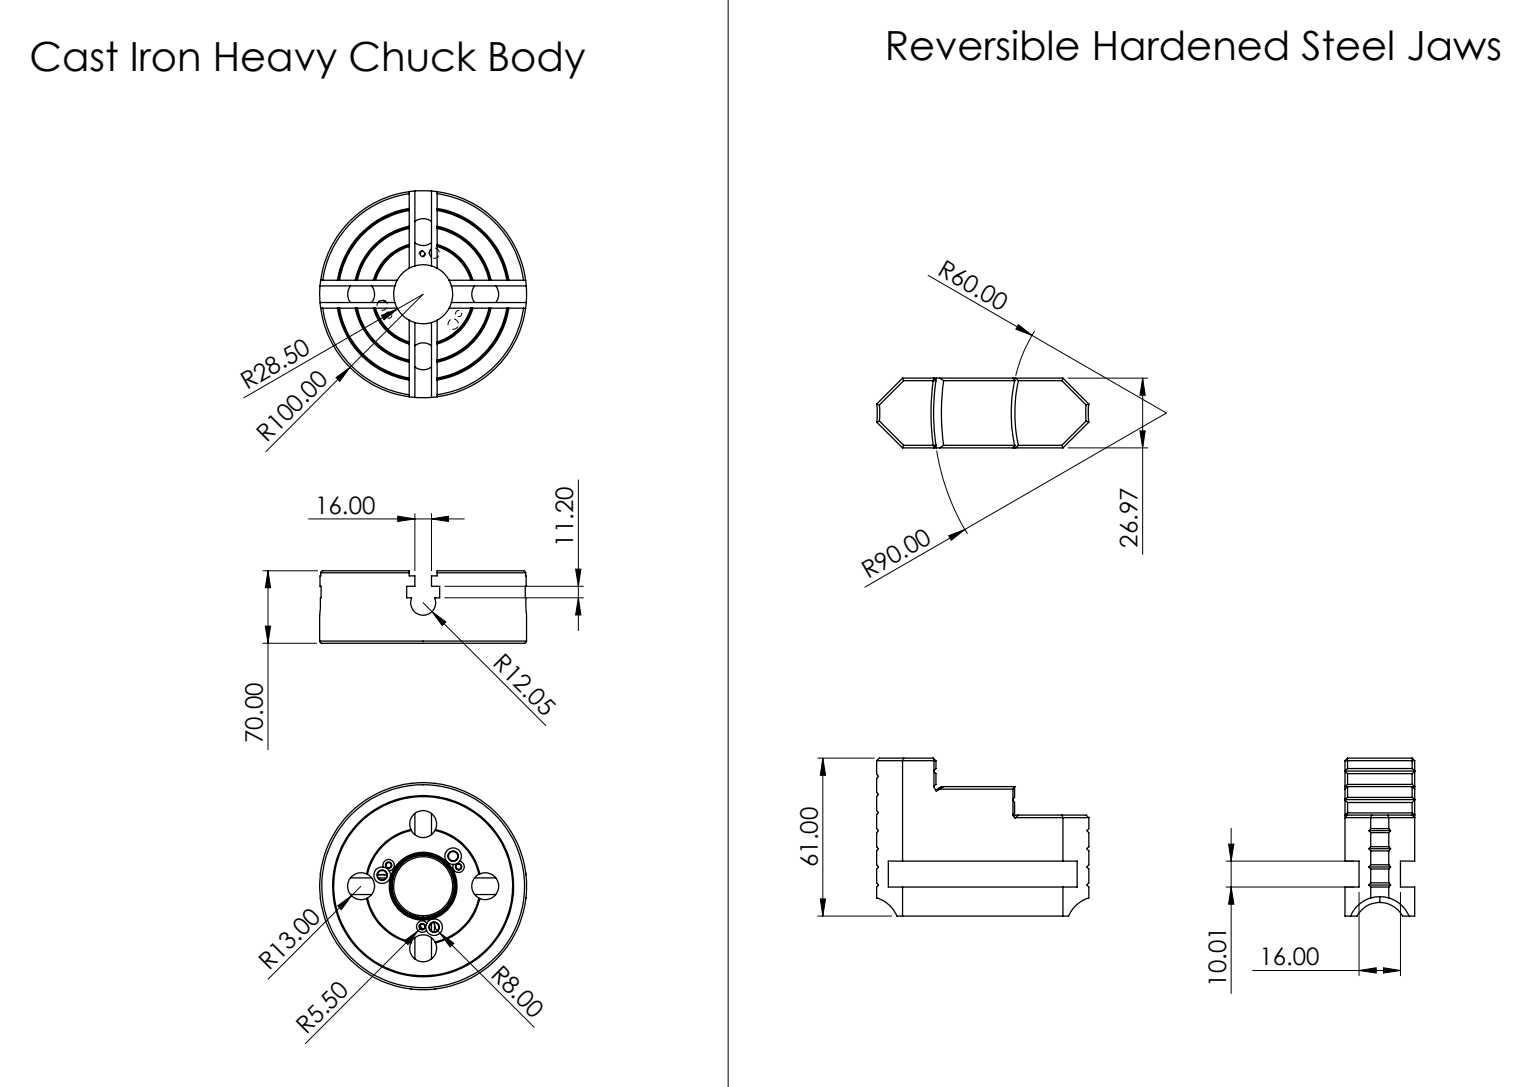
ISO-10303-21;
HEADER;
FILE_DESCRIPTION (('STEP AP214'),
    '1' );
FILE_NAME ('Reversible Hardened Steel Jaws.step',
    '2026-10-09T08:48:44',
    ( '' ),
    ( '' ),
    'SwSTEP 2.0',
    'SolidWorks 2026',
    '' );
FILE_SCHEMA (( 'AUTOMOTIVE_DESIGN' ));
ENDSEC;

DATA;
#3=CARTESIAN_POINT ( 'NONE',  ( -1.404199475065615932, -0.3690944881889765550, -0.3153832671262227771 ) ) ;
#4=CARTESIAN_POINT ( 'NONE',  ( 1.318897637795276356, 0.1660481256975883668, -0.3530559997133364547 ) ) ;
#5=CARTESIAN_POINT ( 'NONE',  ( 1.194225721784777594, 0.05413385826771666132, 0.4176697321401328100 ) ) ;
#6=CARTESIAN_POINT ( 'NONE',  ( 0.3018372703412079971, -0.004921259842519870586, -0.3153832671262229437 ) ) ;
#7=CARTESIAN_POINT ( 'NONE',  ( 1.003937007874016185, 0.1660481256975883668, -0.3530559997133364547 ) ) ;
#9=CARTESIAN_POINT ( 'NONE',  ( 0.1377952755905518800, 0.07958543189024071263, -0.2665933059059888421 ) ) ;
#10=CARTESIAN_POINT ( 'NONE',  ( 0.3149606299212603933, -0.1870078740157479769, 0.4822834645669291653 ) ) ;
#12=CARTESIAN_POINT ( 'NONE',  ( -1.043307086614172707, 0.1660481256975883668, -0.3530559997133364547 ) ) ;
#13=CARTESIAN_POINT ( 'NONE',  ( 0.4330708661417329575, -0.5511811023622047445, 6.969142054262312111E-17 ) ) ;
#14=PLANE ( 'NONE',  #11131 ) ;
#15=CARTESIAN_POINT ( 'NONE',  ( -0.1902887139107604098, -0.6692913385826771977, 0.1292274648535927661 ) ) ;
#16=CARTESIAN_POINT ( 'NONE',  ( -0.1574803149606292529, -0.1870078740157480601, -0.3641732283464567677 ) ) ;
#18=CARTESIAN_POINT ( 'NONE',  ( -0.2493438320209966919, 0.05413385826771626580, -0.4176697321401330321 ) ) ;
#19=CARTESIAN_POINT ( 'NONE',  ( 0.4002624671916016896, -0.2845877964562161244, -0.3641732283464567121 ) ) ;
#21=CARTESIAN_POINT ( 'NONE',  ( -0.03280839895013062252, 0.2952755905511810774, -0.1292274648535930714 ) ) ;
#24=CARTESIAN_POINT ( 'NONE',  ( 1.135170603674541256, -0.5511811023622048555, -0.09757992244046775898 ) ) ;
#26=CARTESIAN_POINT ( 'NONE',  ( -0.8530183727034112984, -0.3690944881889765550, -0.3153832671262227771 ) ) ;
#27=CARTESIAN_POINT ( 'NONE',  ( -0.8792650918635160906, -0.004921259842519870586, -0.3153832671262229437 ) ) ;
#28=CARTESIAN_POINT ( 'NONE',  ( -0.8530183727034112984, 0.05413385826771666132, 0.4176697321401328100 ) ) ;
#29=CARTESIAN_POINT ( 'NONE',  ( -0.3018372703412066094, 0.05413385826771666132, 0.4176697321401328100 ) ) ;
#30=CARTESIAN_POINT ( 'NONE',  ( 0.5905511811023629321, 0.1771653543307087630, 0.000000000000000000 ) ) ;
#32=CARTESIAN_POINT ( 'NONE',  ( 1.351706036745407458, -0.3690944881889765550, -0.3153832671262227771 ) ) ;
#33=CARTESIAN_POINT ( 'NONE',  ( 0.6758530183727039509, -0.6692913385826771977, 0.1292274648535927661 ) ) ;
#35=CARTESIAN_POINT ( 'NONE',  ( -0.09186351706036689768, 0.05413385826771626580, -0.4176697321401330321 ) ) ;
#37=CARTESIAN_POINT ( 'NONE',  ( 1.476377952755906220, 0.07958543189024071263, -0.2665933059059888421 ) ) ;
#38=CARTESIAN_POINT ( 'NONE',  ( 0.7874015748031503170, -0.1870078740157480879, -0.4822834645669291653 ) ) ;
#39=CARTESIAN_POINT ( 'NONE',  ( 8.195543980992789655E-16, -0.1870078740157480879, -0.4822834645669291653 ) ) ;
#41=CARTESIAN_POINT ( 'NONE',  ( 0.1706036745406830368, -0.3690944881889765550, -0.3153832671262227771 ) ) ;
#42=CARTESIAN_POINT ( 'NONE',  ( 1.141732283464567788, -0.6692913385826771977, 8.415575281601705876E-17 ) ) ;
#43=CARTESIAN_POINT ( 'NONE',  ( -0.2952755905511804668, 0.07958543189024085140, 0.2665933059059887866 ) ) ;
#44=CARTESIAN_POINT ( 'NONE',  ( -0.7152230971128602510, -0.3162353388693405765, 0.4822834645669290543 ) ) ;
#46=CARTESIAN_POINT ( 'NONE',  ( 0.3346456692913390985, 0.1660481256975885056, 0.3530559997133364547 ) ) ;
#47=CARTESIAN_POINT ( 'NONE',  ( -0.6758530183727028406, 0.2952755905511811885, 0.1292274648535926551 ) ) ;
#48=CARTESIAN_POINT ( 'NONE',  ( -0.7086614173228339419, -0.1870078740157480601, -0.3641732283464567677 ) ) ;
#49=CARTESIAN_POINT ( 'NONE',  ( 0.1837270341207354329, 0.2306618581243848609, 0.2411417322834645549 ) ) ;
#50=CARTESIAN_POINT ( 'NONE',  ( -1.135170603674539924, -0.6692913385826771977, 0.1292274648535927661 ) ) ;
#51=CARTESIAN_POINT ( 'NONE',  ( -0.3412073490813641308, 0.2306618581243847221, -0.2411417322834647770 ) ) ;
#53=CYLINDRICAL_SURFACE ( 'NONE', #64776, 0.3937007874015748254 ) ;
#54=CARTESIAN_POINT ( 'NONE',  ( 1.161417322834646271, 0.1660481256975883668, -0.3530559997133364547 ) ) ;
#55=CARTESIAN_POINT ( 'NONE',  ( 1.135170603674541256, -0.6692913385826773087, -0.1292274648535924053 ) ) ;
#57=CARTESIAN_POINT ( 'NONE',  ( -1.489501312335957062, -0.05778040916215522460, 0.4822834645669289988 ) ) ;
#58=CARTESIAN_POINT ( 'NONE',  ( -0.7217847769028863381, 0.05413385826771626580, -0.4176697321401330321 ) ) ;
#62=CARTESIAN_POINT ( 'NONE',  ( -0.08530183727034056085, -0.2845877964562159024, 0.3641732283464567677 ) ) ;
#65=CARTESIAN_POINT ( 'NONE',  ( 0.1837270341207354329, 0.2306618581243848609, 0.2411417322834645549 ) ) ;
#67=CYLINDRICAL_SURFACE ( 'NONE', #60105, 0.3937007874015748254 ) ;
#68=CARTESIAN_POINT ( 'NONE',  ( -0.4265091863517051496, -0.5511811023622046335, 0.09757992244046803654 ) ) ;
#69=CARTESIAN_POINT ( 'NONE',  ( 0.3346456692913390985, 0.1660481256975885056, 0.3530559997133364547 ) ) ;
#70=CARTESIAN_POINT ( 'NONE',  ( 1.220472440944882608, 0.2952755905511811885, 0.000000000000000000 ) ) ;
#71=CARTESIAN_POINT ( 'NONE',  ( 0.7283464566929140904, -0.4536011799217368745, -0.2665933059059886201 ) ) ;
#72=AXIS2_PLACEMENT_3D ( 'NONE', #38595, #24309, #82401 ) ;
#73=CARTESIAN_POINT ( 'NONE',  ( -0.04593175853018302557, 0.2952755905511811885, 0.1292274648535926551 ) ) ;
#75=CARTESIAN_POINT ( 'NONE',  ( -0.7414698162729651543, -0.6692913385826771977, 0.1292274648535927661 ) ) ;
#76=CARTESIAN_POINT ( 'NONE',  ( -1.351706036745406347, -0.004921259842519870586, -0.3153832671262229437 ) ) ;
#77=CARTESIAN_POINT ( 'NONE',  ( -0.5839895013123351797, 0.2952755905511810774, -0.1292274648535930714 ) ) ;
#79=CARTESIAN_POINT ( 'NONE',  ( 1.515748031496063408, 0.07958543189024085140, 0.2665933059059887866 ) ) ;
#82=CARTESIAN_POINT ( 'NONE',  ( 0.2362204724409456558, -0.1870078740157479769, 0.4822834645669291653 ) ) ;
#84=CARTESIAN_POINT ( 'NONE',  ( -0.6561679790026240244, -0.6046776061558807314, 0.2411417322834647770 ) ) ;
#85=CARTESIAN_POINT ( 'NONE',  ( 1.332020997375328974, -0.05778040916215560624, -0.4822834645669293319 ) ) ;
#86=CARTESIAN_POINT ( 'NONE',  ( 1.213910761154856299, -0.6692913385826773087, -0.1292274648535924053 ) ) ;
#87=CARTESIAN_POINT ( 'NONE',  ( 0.4724409448818904789, -0.1870078740157479769, 0.4822834645669291653 ) ) ;
#88=CARTESIAN_POINT ( 'NONE',  ( 0.1574803149606306130, -0.1870078740157480879, -0.4822834645669291653 ) ) ;
#90=CARTESIAN_POINT ( 'NONE',  ( -0.9120734908136475250, 0.2952755905511811885, 0.1292274648535926551 ) ) ;
#91=CARTESIAN_POINT ( 'NONE',  ( -0.1968503937007867743, 0.2952755905511811885, 0.000000000000000000 ) ) ;
#92=CARTESIAN_POINT ( 'NONE',  ( -0.006561679790025524116, -0.08942795157528024563, -0.3641732283464568787 ) ) ;
#94=CARTESIAN_POINT ( 'NONE',  ( 0.07217847769028949700, -0.05778040916215560624, -0.4822834645669293319 ) ) ;
#96=CARTESIAN_POINT ( 'NONE',  ( 1.253280839895013710, -0.3162353388693405765, 0.4822834645669290543 ) ) ;
#99=ORIENTED_EDGE ( 'NONE', *, *, #69485, .F. ) ;
#100=CARTESIAN_POINT ( 'NONE',  ( 0.3215223097112867578, -0.3162353388693409650, -0.4822834645669289433 ) ) ;
#101=CARTESIAN_POINT ( 'NONE',  ( -0.3543307086614165824, -0.5511811023622047445, 6.969142054262312111E-17 ) ) ;
#102=CARTESIAN_POINT ( 'NONE',  ( 1.377952755905512472, 0.1771653543307087630, 0.000000000000000000 ) ) ;
#103=CARTESIAN_POINT ( 'NONE',  ( -0.06764250034433647030, -3.915482057279200494E-15, 0.3954985857520088577 ) ) ;
#106=CARTESIAN_POINT ( 'NONE',  ( 1.410761154855643795, -0.08942795157528024563, -0.3641732283464568787 ) ) ;
#107=CARTESIAN_POINT ( 'NONE',  ( -1.423884514435694859, -0.05778040916215560624, -0.4822834645669293319 ) ) ;
#109=CARTESIAN_POINT ( 'NONE',  ( -0.1377952755905504645, 0.1660481256975885056, 0.3530559997133364547 ) ) ;
#110=CARTESIAN_POINT ( 'NONE',  ( -1.056430446194224881, -0.6692913385826771977, 0.1292274648535927661 ) ) ;
#111=CARTESIAN_POINT ( 'NONE',  ( -0.9645669291338575535, -0.5400638737290844871, 0.3530559997133364547 ) ) ;
#112=CARTESIAN_POINT ( 'NONE',  ( 0.1902887139107617975, 0.2952755905511811885, 0.1292274648535926551 ) ) ;
#114=CARTESIAN_POINT ( 'NONE',  ( -1.653543307086613234, -0.1870078740157479769, 0.3641732283464567677 ) ) ;
#115=CARTESIAN_POINT ( 'NONE',  ( 1.108923884514436242, -0.05778040916215522460, 0.4822834645669289988 ) ) ;
#116=CARTESIAN_POINT ( 'NONE',  ( 0.7545931758530189937, 0.1771653543307087075, -0.09757992244046823083 ) ) ;
#118=CARTESIAN_POINT ( 'NONE',  ( 0.9055118110236227702, 0.1771653543307087630, 0.000000000000000000 ) ) ;
#119=CARTESIAN_POINT ( 'NONE',  ( -1.200787401574802349, -0.5400638737290844871, 0.3530559997133364547 ) ) ;
#121=CARTESIAN_POINT ( 'NONE',  ( 1.358267716535433323, 0.1660481256975885056, 0.3530559997133364547 ) ) ;
#123=CARTESIAN_POINT ( 'NONE',  ( 0.6036745406824154392, 0.2306618581243847221, -0.2411417322834647770 ) ) ;
#125=CARTESIAN_POINT ( 'NONE',  ( -1.653543307086613234, -0.1870078740157480601, -0.3641732283464567677 ) ) ;
#126=CARTESIAN_POINT ( 'NONE',  ( 0.01968503937007957949, -0.5400638737290845981, -0.3530559997133363437 ) ) ;
#127=CARTESIAN_POINT ( 'NONE',  ( 0.6102362204724416372, -0.4536011799217367080, 0.2665933059059888421 ) ) ;
#128=CARTESIAN_POINT ( 'NONE',  ( 0.9776902887139113929, -0.6692913385826773087, -0.1292274648535924053 ) ) ;
#129=CARTESIAN_POINT ( 'NONE',  ( 1.640419947506562393, -0.3690944881889763329, 0.3153832671262228327 ) ) ;
#130=CARTESIAN_POINT ( 'NONE',  ( -0.6824146981627291497, -0.5023911411419708095, -0.1820866141732282451 ) ) ;
#131=CARTESIAN_POINT ( 'NONE',  ( -0.6430446194225716283, -0.4281496062992124485, 0.4176697321401328655 ) ) ;
#132=CARTESIAN_POINT ( 'NONE',  ( 1.574803149606299746, -0.1870078740157480879, -0.4822834645669291653 ) ) ;
#133=CARTESIAN_POINT ( 'NONE',  ( -1.246719160104986512, 0.05413385826771666132, 0.4176697321401328100 ) ) ;
#134=CONICAL_SURFACE ( 'NONE', #57903, 2.401574803149606918, 0.7125723459225955514 ) ;
#135=CARTESIAN_POINT ( 'NONE',  ( 0.8923884514435703741, 0.2306618581243848609, 0.2411417322834645549 ) ) ;
#136=CARTESIAN_POINT ( 'NONE',  ( -1.345144356955379816, -0.2845877964562159024, 0.3641732283464567677 ) ) ;
#138=CARTESIAN_POINT ( 'NONE',  ( 0.8070866141732288002, 0.1660481256975885056, 0.3530559997133364547 ) ) ;
#140=CARTESIAN_POINT ( 'NONE',  ( -1.561679790026246017, 0.05413385826771666132, 0.4176697321401328100 ) ) ;
#141=CARTESIAN_POINT ( 'NONE',  ( -1.555118110236219930, -0.4536011799217368745, -0.2665933059059886201 ) ) ;
#142=CARTESIAN_POINT ( 'NONE',  ( -0.8792650918635160906, -0.004921259842519870586, -0.3153832671262229437 ) ) ;
#143=B_SPLINE_CURVE_WITH_KNOTS ( 'NONE', 3,
 ( #64397, #13065, #45854, #433 ),
 .UNSPECIFIED., .F., .F.,
 ( 4, 4 ),
 ( 3.878959614448864246E-18, 0.001357026659661165861 ),
 .UNSPECIFIED. ) ;
#144=CARTESIAN_POINT ( 'NONE',  ( 1.496062992125985147, -0.1870078740157479769, 0.3641732283464567677 ) ) ;
#145=CARTESIAN_POINT ( 'NONE',  ( -0.3280839895013117347, 0.05413385826771626580, -0.4176697321401330321 ) ) ;
#146=CARTESIAN_POINT ( 'NONE',  ( -0.2230971128608915943, -0.004921259842519576551, 0.3153832671262227771 ) ) ;
#147=CARTESIAN_POINT ( 'NONE',  ( -1.660104986876639543, -0.08942795157528024563, -0.3641732283464568787 ) ) ;
#148=CARTESIAN_POINT ( 'NONE',  ( 0.9711286089238851948, 0.1283753931104748280, 0.1820866141732283561 ) ) ;
#149=CARTESIAN_POINT ( 'NONE',  ( 0.6299212598425204535, -0.1870078740157480879, -0.4822834645669291653 ) ) ;
#150=CARTESIAN_POINT ( 'NONE',  ( 1.489501312335958172, -0.05778040916215560624, -0.4822834645669293319 ) ) ;
#151=CARTESIAN_POINT ( 'NONE',  ( 0.4986876640419954376, -0.6046776061558809534, -0.2411417322834644161 ) ) ;
#154=CARTESIAN_POINT ( 'NONE',  ( 0.6889763779527563470, 0.07958543189024071263, -0.2665933059059888421 ) ) ;
#155=CARTESIAN_POINT ( 'NONE',  ( -1.443569553805773564, 0.2306618581243847221, -0.2411417322834647770 ) ) ;
#157=CARTESIAN_POINT ( 'NONE',  ( -1.351706036745406347, -0.4281496062992124485, 0.4176697321401328655 ) ) ;
#158=CARTESIAN_POINT ( 'NONE',  ( -0.4724409448818890911, -0.1870078740157479769, 0.4822834645669291653 ) ) ;
#161=CARTESIAN_POINT ( 'NONE',  ( -0.04593175853018302557, -0.6692913385826773087, -0.1292274648535924053 ) ) ;
#162=CARTESIAN_POINT ( 'NONE',  ( 1.187664041994751285, -0.2845877964562161244, -0.3641732283464567121 ) ) ;
#163=CARTESIAN_POINT ( 'NONE',  ( -0.3608923884514428360, 0.2952755905511811885, 0.1292274648535926551 ) ) ;
#164=CARTESIAN_POINT ( 'NONE',  ( 0.2952755905511816326, -0.5400638737290844871, 0.3530559997133364547 ) ) ;
#170=CARTESIAN_POINT ( 'NONE',  ( -0.8464566929133852113, -0.4536011799217368745, -0.2665933059059886201 ) ) ;
#171=CARTESIAN_POINT ( 'NONE',  ( -1.272965879265091305, -0.4281496062992124485, 0.4176697321401328655 ) ) ;
#173=CARTESIAN_POINT ( 'NONE',  ( 0.3280839895013130669, -0.4281496062992127816, -0.4176697321401328100 ) ) ;
#175=CARTESIAN_POINT ( 'NONE',  ( 1.233595800524935227, -0.6046776061558807314, 0.2411417322834647770 ) ) ;
#176=CARTESIAN_POINT ( 'NONE',  ( 0.8202099737532813073, 0.2952755905511811885, 0.1292274648535926551 ) ) ;
#180=CARTESIAN_POINT ( 'NONE',  ( 1.541994750656168645, 0.2952755905511810774, -0.1292274648535930714 ) ) ;
#181=CARTESIAN_POINT ( 'NONE',  ( 0.4330708661417329575, -0.6692913385826771977, 8.415575281601705876E-17 ) ) ;
#182=CARTESIAN_POINT ( 'NONE',  ( 0.07217847769028949700, -0.05778040916215560624, -0.4822834645669293319 ) ) ;
#183=CARTESIAN_POINT ( 'NONE',  ( 0.7480314960629927956, -0.5511811023622047445, 6.969142054262312111E-17 ) ) ;
#184=CARTESIAN_POINT ( 'NONE',  ( 1.371391076115485941, 0.2952755905511811885, 0.1292274648535926551 ) ) ;
#186=CARTESIAN_POINT ( 'NONE',  ( 0.5643044619422579178, -0.4281496062992127816, -0.4176697321401328100 ) ) ;
#187=CARTESIAN_POINT ( 'NONE',  ( 0.9514435695538062676, -0.3162353388693409650, -0.4822834645669289433 ) ) ;
#188=CARTESIAN_POINT ( 'NONE',  ( 0.2690288713910767848, 0.2952755905511811885, 0.1292274648535926551 ) ) ;
#189=CARTESIAN_POINT ( 'NONE',  ( 1.233595800524935227, 0.1283753931104746893, -0.1820866141732285504 ) ) ;
#190=CARTESIAN_POINT ( 'NONE',  ( -0.9448818897637790704, -0.1870078740157479769, 0.4822834645669291653 ) ) ;
#191=CARTESIAN_POINT ( 'NONE',  ( -1.102362204724408601, -0.1870078740157479769, 0.4822834645669291653 ) ) ;
#193=CARTESIAN_POINT ( 'NONE',  ( 1.089238845144357537, -0.4281496062992124485, 0.4176697321401328655 ) ) ;
#197=ORIENTED_EDGE ( 'NONE', *, *, #73267, .T. ) ;
#199=VERTEX_POINT ( 'NONE', #53305 ) ;
#200=CARTESIAN_POINT ( 'NONE',  ( 1.509186351706037543, 0.05413385826771666132, 0.4176697321401328100 ) ) ;
#201=CARTESIAN_POINT ( 'NONE',  ( 0.9317585301837276734, -0.3690944881889763329, 0.3153832671262228327 ) ) ;
#203=CARTESIAN_POINT ( 'NONE',  ( 1.213910761154856299, 0.1771653543307087630, 0.09757992244046791164 ) ) ;
#205=DIRECTION ( 'NONE',  ( 1.000000000000000000, 0.000000000000000000, -1.692413147294446216E-16 ) ) ;
#206=CARTESIAN_POINT ( 'NONE',  ( -0.6175017169405814244, 0.000000000000000000, 0.3464511005275205946 ) ) ;
#208=CARTESIAN_POINT ( 'NONE',  ( -0.9776902887139098386, 0.1771653543307087075, -0.09757992244046823083 ) ) ;
#209=CARTESIAN_POINT ( 'NONE',  ( -1.640419947506561060, -0.3690944881889765550, -0.3153832671262227771 ) ) ;
#210=CARTESIAN_POINT ( 'NONE',  ( -1.423884514435694859, -0.05778040916215560624, -0.4822834645669293319 ) ) ;
#211=CARTESIAN_POINT ( 'NONE',  ( 5.463695987328526437E-16, -0.1870078740157479769, 0.4822834645669291653 ) ) ;
#212=CARTESIAN_POINT ( 'NONE',  ( 1.312335958005249825, 0.2306618581243847221, -0.2411417322834647770 ) ) ;
#214=CARTESIAN_POINT ( 'NONE',  ( -1.122047244094487306, 0.1012011053420775880, -0.2882089793578256898 ) ) ;
#215=( CONVERSION_BASED_UNIT ( 'INCH', #44794 ) LENGTH_UNIT ( ) NAMED_UNIT ( #76065 ) );
#217=DIRECTION ( 'NONE',  ( 1.000000000000000000, -0.000000000000000000, -0.000000000000000000 ) ) ;
#218=LINE ( 'NONE', #70923, #26406 ) ;
#219=CARTESIAN_POINT ( 'NONE',  ( -0.8727034120734901146, -0.2845877964562159024, 0.3641732283464567677 ) ) ;
#220=CARTESIAN_POINT ( 'NONE',  ( -1.161417322834644716, 0.1660481256975885056, 0.3530559997133364547 ) ) ;
#221=CARTESIAN_POINT ( 'NONE',  ( 0.7283464566929143125, 0.1660481256975885056, 0.3530559997133364547 ) ) ;
#222=ORIENTED_EDGE ( 'NONE', *, *, #16494, .T. ) ;
#226=CARTESIAN_POINT ( 'NONE',  ( 1.161417322834646493, -0.5400638737290844871, 0.3530559997133364547 ) ) ;
#227=CARTESIAN_POINT ( 'NONE',  ( -1.240157480314959759, 0.1660481256975885056, 0.3530559997133364547 ) ) ;
#229=CARTESIAN_POINT ( 'NONE',  ( -0.5380577427821514602, -0.3690944881889765550, -0.3153832671262227771 ) ) ;
#230=CARTESIAN_POINT ( 'NONE',  ( -1.253280839895012377, -0.2845877964562161244, -0.3641732283464567121 ) ) ;
#232=CARTESIAN_POINT ( 'NONE',  ( -0.4855643044619415427, -0.004921259842519870586, -0.3153832671262229437 ) ) ;
#233=CARTESIAN_POINT ( 'NONE',  ( -0.07217847769028813698, -0.2845877964562161244, -0.3641732283464567121 ) ) ;
#234=CARTESIAN_POINT ( 'NONE',  ( 0.3215223097112867578, -0.05778040916215522460, 0.4822834645669289988 ) ) ;
#235=CARTESIAN_POINT ( 'NONE',  ( -1.076115485564303809, -0.5023911411419708095, -0.1820866141732282451 ) ) ;
#237=CARTESIAN_POINT ( 'NONE',  ( 1.167979002624672580, 0.05413385826771626580, -0.4176697321401330321 ) ) ;
#239=CARTESIAN_POINT ( 'NONE',  ( -1.345144356955379816, -0.3162353388693405765, 0.4822834645669290543 ) ) ;
#241=CARTESIAN_POINT ( 'NONE',  ( -0.2952755905511804668, 0.1660481256975885056, 0.3530559997133364547 ) ) ;
#242=CARTESIAN_POINT ( 'NONE',  ( -0.8923884514435688198, -0.6046776061558807314, 0.2411417322834647770 ) ) ;
#243=CARTESIAN_POINT ( 'NONE',  ( 0.9251968503937015864, 0.07958543189024071263, -0.2665933059059888421 ) ) ;
#244=CARTESIAN_POINT ( 'NONE',  ( -0.4986876640419942164, -0.5023911411419708095, 0.1820866141732285504 ) ) ;
#245=CARTESIAN_POINT ( 'NONE',  ( -0.5052493438320203589, -0.6692913385826771977, 0.1292274648535927661 ) ) ;
#246=CARTESIAN_POINT ( 'NONE',  ( -1.364829396325458521, -0.6046776061558807314, 0.2411417322834647770 ) ) ;
#248=CARTESIAN_POINT ( 'NONE',  ( 1.089238845144357759, -0.004921259842519870586, -0.3153832671262229437 ) ) ;
#249=CARTESIAN_POINT ( 'NONE',  ( -0.4330708661417315697, -0.6692913385826771977, 8.415575281601705876E-17 ) ) ;
#250=CARTESIAN_POINT ( 'NONE',  ( -1.561679790026246017, 0.05413385826771666132, 0.4176697321401328100 ) ) ;
#252=ORIENTED_EDGE ( 'NONE', *, *, #19019, .F. ) ;
#254=CARTESIAN_POINT ( 'NONE',  ( -0.9776902887139098386, 0.1771653543307087075, -0.09757992244046823083 ) ) ;
#255=CARTESIAN_POINT ( 'NONE',  ( 0.7349081364829402885, -0.6046776061558809534, -0.2411417322834644161 ) ) ;
#256=CARTESIAN_POINT ( 'NONE',  ( -1.135170603674539924, -0.5511811023622046335, 0.09757992244046803654 ) ) ;
#258=CARTESIAN_POINT ( 'NONE',  ( -1.017060367454067249, -0.3162353388693409650, -0.4822834645669289433 ) ) ;
#259=CARTESIAN_POINT ( 'NONE',  ( 0.7020997375328090762, -0.3162353388693405765, 0.4822834645669290543 ) ) ;
#260=CARTESIAN_POINT ( 'NONE',  ( 0.6955380577427828781, -0.4281496062992124485, 0.4176697321401328655 ) ) ;
#261=CARTESIAN_POINT ( 'NONE',  ( 1.463254593175853824, 0.2952755905511810774, -0.1292274648535930714 ) ) ;
#262=CARTESIAN_POINT ( 'NONE',  ( -1.377952755905511140, 0.1771653543307087630, 0.000000000000000000 ) ) ;
#266=LINE ( 'NONE', #58323, #72192 ) ;
#267=CARTESIAN_POINT ( 'NONE',  ( 1.043307086614173818, 0.07958543189024085140, 0.2665933059059887866 ) ) ;
#268=CARTESIAN_POINT ( 'NONE',  ( 0.3871391076115492380, -0.08942795157528024563, -0.3641732283464568787 ) ) ;
#269=CARTESIAN_POINT ( 'NONE',  ( 0.1377952755905518800, -0.5400638737290844871, 0.3530559997133364547 ) ) ;
#270=CARTESIAN_POINT ( 'NONE',  ( 1.161417322834646271, 0.1660481256975883668, -0.3530559997133364547 ) ) ;
#272=CARTESIAN_POINT ( 'NONE',  ( 0.2887139107611556010, 0.1283753931104746893, -0.1820866141732285504 ) ) ;
#273=CARTESIAN_POINT ( 'NONE',  ( -0.6036745406824141069, -0.6046776061558809534, -0.2411417322834644161 ) ) ;
#274=CARTESIAN_POINT ( 'NONE',  ( -1.246719160104985846, -0.4281496062992127816, -0.4176697321401328100 ) ) ;
#275=CARTESIAN_POINT ( 'NONE',  ( 0.6627296587926517768, -0.6692913385826773087, -0.1292274648535924053 ) ) ;
#279=ORIENTED_EDGE ( 'NONE', *, *, #37675, .F. ) ;
#280=CARTESIAN_POINT ( 'NONE',  ( -1.391076115485563758, 0.2306618581243848609, 0.2411417322834645549 ) ) ;
#281=CARTESIAN_POINT ( 'NONE',  ( -0.7742782152230962556, -0.4281496062992127816, -0.4176697321401328100 ) ) ;
#282=CARTESIAN_POINT ( 'NONE',  ( -0.7020997375328074108, -0.08942795157527998196, 0.3641732283464567121 ) ) ;
#283=CARTESIAN_POINT ( 'NONE',  ( -0.5971128608923877978, -0.6692913385826773087, -0.1292274648535924053 ) ) ;
#286=CARTESIAN_POINT ( 'NONE',  ( -1.607611548556429737, 0.1771653543307087075, -0.09757992244046823083 ) ) ;
#287=CARTESIAN_POINT ( 'NONE',  ( -1.069553805774277722, 0.2952755905511811885, 0.1292274648535926551 ) ) ;
#288=CARTESIAN_POINT ( 'NONE',  ( 0.2952755905511816326, -0.5400638737290844871, 0.3530559997133364547 ) ) ;
#289=CARTESIAN_POINT ( 'NONE',  ( -0.7349081364829387342, -0.6046776061558807314, 0.2411417322834647770 ) ) ;
#291=CARTESIAN_POINT ( 'NONE',  ( -0.8595800524934373854, -0.08942795157527998196, 0.3641732283464567121 ) ) ;
#295=CARTESIAN_POINT ( 'NONE',  ( -1.535433070866141225, 0.1771653543307087630, 0.000000000000000000 ) ) ;
#296=CARTESIAN_POINT ( 'NONE',  ( -1.240157480314959759, 0.1660481256975885056, 0.3530559997133364547 ) ) ;
#297=CARTESIAN_POINT ( 'NONE',  ( -0.7414698162729651543, -0.6692913385826771977, 0.1292274648535927661 ) ) ;
#299=CARTESIAN_POINT ( 'NONE',  ( -0.9645669291338575535, -0.5400638737290844871, 0.3530559997133364547 ) ) ;
#300=CARTESIAN_POINT ( 'NONE',  ( -1.410761154855642463, -0.05778040916215522460, 0.4822834645669289988 ) ) ;
#304=CARTESIAN_POINT ( 'NONE',  ( 0.5971128608923891301, 0.1771653543307087075, -0.09757992244046823083 ) ) ;
#305=DIRECTION ( 'NONE',  ( -3.096699300667737957E-16, 1.000000000000000000, -0.000000000000000000 ) ) ;
#307=CARTESIAN_POINT ( 'NONE',  ( -0.2034120734908131112, -0.5511811023622048555, -0.09757992244046775898 ) ) ;
#308=CARTESIAN_POINT ( 'NONE',  ( -0.6036745406824141069, -0.6046776061558809534, -0.2411417322834644161 ) ) ;
#309=ADVANCED_FACE ( 'NONE', ( #49336 ), #12419, .F. ) ;
#310=CARTESIAN_POINT ( 'NONE',  ( 1.555118110236221041, -0.5400638737290844871, 0.3530559997133364547 ) ) ;
#311=CARTESIAN_POINT ( 'NONE',  ( -0.6233595800524928121, -0.3162353388693409650, -0.4822834645669289433 ) ) ;
#315=CARTESIAN_POINT ( 'NONE',  ( -1.095800524934382292, -0.3162353388693409650, -0.4822834645669289433 ) ) ;
#317=CARTESIAN_POINT ( 'NONE',  ( 1.404199475065617264, -0.4281496062992124485, 0.4176697321401328655 ) ) ;
#318=CARTESIAN_POINT ( 'NONE',  ( -1.043307086614172707, 0.07958543189024071263, -0.2665933059059888421 ) ) ;
#319=CARTESIAN_POINT ( 'NONE',  ( -1.443569553805773564, -0.6046776061558807314, 0.2411417322834647770 ) ) ;
#324=CARTESIAN_POINT ( 'NONE',  ( 0.01312335958005323398, -0.4281496062992127816, -0.4176697321401328100 ) ) ;
#325=CARTESIAN_POINT ( 'NONE',  ( -1.135170603674539924, 0.1771653543307087075, -0.09757992244046823083 ) ) ;
#326=CARTESIAN_POINT ( 'NONE',  ( -0.6299212598425188991, -0.1870078740157479769, 0.4822834645669291653 ) ) ;
#328=CARTESIAN_POINT ( 'NONE',  ( -1.384514435695537005, 0.2952755905511811885, 0.1292274648535926551 ) ) ;
#329=CARTESIAN_POINT ( 'NONE',  ( -1.095800524934382292, -0.05778040916215522460, 0.4822834645669289988 ) ) ;
#330=CARTESIAN_POINT ( 'NONE',  ( 0.2362204724409456558, -0.1870078740157480879, -0.4822834645669291653 ) ) ;
#332=CARTESIAN_POINT ( 'NONE',  ( 0.7349081364829402885, -0.5023911411419708095, -0.1820866141732282451 ) ) ;
#333=CARTESIAN_POINT ( 'NONE',  ( -0.7742782152230965886, -0.004921259842519576551, 0.3153832671262227771 ) ) ;
#335=CARTESIAN_POINT ( 'NONE',  ( 0.8267716535433078384, -0.5511811023622047445, 6.969142054262312111E-17 ) ) ;
#336=CARTESIAN_POINT ( 'NONE',  ( 1.496062992125984703, -0.1870078740157480601, -0.3641732283464567677 ) ) ;
#337=CARTESIAN_POINT ( 'NONE',  ( 1.299212598425197429, 0.2952755905511811885, 0.000000000000000000 ) ) ;
#338=CARTESIAN_POINT ( 'NONE',  ( -0.05905511811023545637, 0.07958543189024085140, 0.2665933059059887866 ) ) ;
#340=CARTESIAN_POINT ( 'NONE',  ( -1.023622047244093558, -0.1870078740157479769, 0.4822834645669291653 ) ) ;
#341=CARTESIAN_POINT ( 'NONE',  ( 1.049868766404200127, -0.6046776061558809534, -0.2411417322834644161 ) ) ;
#343=CARTESIAN_POINT ( 'NONE',  ( -0.3215223097112853146, -0.08942795157528024563, -0.3641732283464568787 ) ) ;
#345=CARTESIAN_POINT ( 'NONE',  ( 0.3937007874015754361, -0.1870078740157479769, 0.4822834645669291653 ) ) ;
#347=CARTESIAN_POINT ( 'NONE',  ( 0.8398950131233602345, 0.1283753931104746893, -0.1820866141732285504 ) ) ;
#348=CARTESIAN_POINT ( 'NONE',  ( 0.02624671916010564918, 0.1283753931104748280, 0.1820866141732283561 ) ) ;
#349=CARTESIAN_POINT ( 'NONE',  ( 0.1181102362204730916, 0.2952755905511811885, 0.000000000000000000 ) ) ;
#350=CARTESIAN_POINT ( 'NONE',  ( -1.207349081364828880, 0.2306618581243847221, -0.2411417322834647770 ) ) ;
#351=CARTESIAN_POINT ( 'NONE',  ( -0.4986876640419939388, 0.1283753931104746893, -0.1820866141732285504 ) ) ;
#352=DIRECTION ( 'NONE',  ( 0.000000000000000000, 1.000000000000000000, 0.000000000000000000 ) ) ;
#353=CARTESIAN_POINT ( 'NONE',  ( -0.9580052493438311334, 0.05413385826771626580, -0.4176697321401330321 ) ) ;
#356=CARTESIAN_POINT ( 'NONE',  ( 0.3608923884514443348, 0.1771653543307087075, -0.09757992244046823083 ) ) ;
#357=CARTESIAN_POINT ( 'NONE',  ( -0.6692913385826764205, 0.2952755905511811885, 0.000000000000000000 ) ) ;
#358=CARTESIAN_POINT ( 'NONE',  ( -1.227034120734907141, -0.6692913385826773087, -0.1292274648535924053 ) ) ;
#359=CARTESIAN_POINT ( 'NONE',  ( -1.023622047244093558, -0.1870078740157479769, 0.3641732283464567677 ) ) ;
#360=CARTESIAN_POINT ( 'NONE',  ( 1.548556430446194954, 0.2306618581243847221, -0.2411417322834647770 ) ) ;
#361=( BOUNDED_SURFACE ( )  B_SPLINE_SURFACE ( 1, 2, ( 
 ( #63527, #18507, #32782, #810, #5858, #57610, #388, #44971, #24798, #82892, #31534, #44150, #60014, #57190, #26473, #37849, #12602, #7111, #44556, #25212, #19741, #21303, #64772, #58024, #6692, #14998, #13435, #70667, #78982, #53273, #58450, #50878, #46956, #26045, #64355, #32362, #76578, #6273, #18906, #63937, #31949, #50466, #72648, #38677, #83301, #25623, #40655, #51704, #51286, #76989, #77406, #19319, #66339, #69842, #8678, #34348, #76170, #12192, #71092, #13023, #39091, #16663, #53684, #36007, #28856, #73906, #54518, #67177, #42303, #79392, #49035, #68001, #22549, #15842, #17080, #21711, #47375, #73065, #16247, #54100, #10346, #68413, #9098, #9506, #10753, #22132, #35179, #29273, #60840, #74732, #22955, #34771, #41076, #47790, #15415, #3607, #66765, #41490, #60430, #2781, #28441, #61677, #4018, #29682, #42717, #73494, #54937, #55344, #79815, #3192, #81051, #23365, #80643, #48211, #2369, #48622, #41894, #80233, #67588, #9918, #36413, #61253, #28025, #35590, #74317, #24189, #49858, #11989, #70043, #37643, #82687, #38054, #12397, #63730, #6070, #51083, #75558, #5658, #31744, #4837, #62918, #57406, #83097, #63320, #82283, #62086, #31325, #18307, #55757, #30093, #68820, #76780, #56989, #44761, #81463, #75146, #17898, #43534, #25006, #25418, #50678, #76377, #19112, #43122, #11582, #18711, #24601, #4427, #36824, #17491, #23781, #12815, #11165, #70457, #62499, #69233, #44352, #81877, #30512, #49452, #56174, #37241, #5251, #43949, #30915, #56582, #50270, #75967, #69645, #65422, #70888, #7756, #1029, #7325, #32994, #45185, #603, #51494, #13238, #38887, #40148, #33422, #64990, #26259, #64566, #27095, #26682, #51920, #45609, #52337, #71302, #20790, #32159, #78465, #72139, #52757, #46446, #46025, #6903, #77625, #14074, #6489, #59083, #19958, #39303, #13650, #58664, #39727, #64156, #14495, #1438, #78044, #32574, #38472, #25835, #182, #77197, #20373, #58236, #57815, #19528, #71719, #55293, #42669, #10291, #35538, #10706, #61200, #28804, #11113, #54047, #81002, #16610, #15785, #47737, #48159, #3141, #23316, #54468, #48985, #55704, #73435, #3557, #29222, #81412, #75094, #80181, #22496, #62037, #54889, #35958, #74684, #23729, #17442, #35122, #17030, #49400, #68368, #68769, #36362, #36770, #62446, #43072, #4782, #60788, #48569, #61627, #41437, #67120, #9451, #4374, #73854, #30042, #79761, #80594, #74267, #16195, #3969, #22078, #41841, #67531, #9869, #22902, #42253, #67948, #29632, #69994, #11939, #70409, #37594, #5202, #70840, #30458, #57351, #76329, #75509, #24138, #24553, #62865, #31692, #30866, #12765, #56531, #82234, #83047, #64517, #37186, #38422, #49808, #12349, #19483, #25370, #63683, #77151, #6021, #13189, #38838, #63267, #5608, #24951, #44303, #51033, #56122, #64104, #131, #38005, #76732, #81828, #17848, #43482, #50219, #31276, #45136, #11529, #75915, #18254, #43896, #69593, #56941, #82638, #44712, #19064, #6439, #32111, #50624, #18659, #57769, #25786, #51447, #69178, #13601, #32948, #52291, #53123, #46397, #52707, #58614, #66197, #71672, #59039, #7708, #33786, #14024, #1802, #45559, #981, #59865, #8534, #27884, #39255, #7277, #14856, #33375, #72090, #27465, #34202, #53544, #71255, #78834, #2218, #21160, #21567, #46816, #47229, #15270, #79252, #72919, #64937, #1393, #14449, #26209, #51871, #77577, #40517, #26637, #59450, #72507, #65373, #27047, #77996, #40100, #40931, #6854, #19909, #20324, #556, #45977, #8121, #32524, #65788, #39681, #58186, #78418, #20747, #23629, #66611, #10195, #29126, #28294, #60287, #60696, #15690, #67857, #67029, #23218, #9361, #41348, #35864, #17347, #73342, #74589, #2637, #22813, #55604, #61529, #16518, #29940, #42162, #49300, #75001, #73764, #41744, #61109, #80497, #3875, #8947, #48888, #36267, #48470, #29534, #34623, #53955, #79668, #35032, #67438, #81316, #47647, #3046, #28711, #54375, #80085, #22405, #48062, #80904, #74171, #55197, #16933, #16099, #9772, #42573, #54794, #68275, #10610, #35443, #3461, #61936, #4279, #21985, #5511, #69080, #18964, #24450, #11845, #43790, #69897, #50118, #37907, #81731, #11431, #12661, #44207 ),
 ( #17751, #37086, #62772, #75405, #49710, #43380, #57247, #24856, #12251, #31592, #5106, #30773, #25269, #31174, #5918, #63584, #56434, #82136, #75815, #82951, #82538, #56840, #18158, #44612, #69496, #37498, #63173, #50935, #50524, #76633, #24040, #76230, #38322, #70308, #63996, #36669, #18564, #6337, #32010, #57670, #32, #25685, #51345, #77049, #42975, #68671, #11010, #62344, #4683, #30354, #56023, #8022, #34099, #65693, #59762, #27783, #21058, #72410, #451, #13922, #58938, #38739, #64416, #6751, #53020, #45456, #71993, #46298, #77893, #39578, #26106, #1296, #78735, #53446, #32423, #58085, #13086, #51768, #20645, #33685, #26946, #877, #59347, #26536, #77470, #2117, #19381, #14346, #65268, #19807, #71154, #13495, #39151, #40006, #64836, #1704, #7174, #32845, #27361, #45033, #58514, #46718, #52189, #52607, #8431, #14759, #78314, #66095, #40414, #70732, #20224, #45873, #71571, #7604, #33278, #16416, #4180, #35757, #34937, #15169, #34520, #72819, #3773, #55096, #29437, #68169, #41246, #22713, #80804, #21882, #79986, #48789, #23121, #80400, #16005, #79154, #48371, #35347, #40825, #47129, #2538, #10512, #54689, #61839, #66510, #8844, #66933, #9266, #29023, #74486, #74070, #42063, #16833, #60186, #28614, #67758, #41652, #21471, #53854, #28196, #79567, #29843, #47546, #42469, #73236, #60599, #61423, #15587, #2949, #10092, #36165, #54271, #22299, #61009, #47960, #73664, #67343, #9676, #3358, #64624, #55921, #37810, #31078, #11751, #37407, #30257, #36990, #36571, #81634, #23945, #7383, #6961, #69399, #62669, #75307, #51977, #56746, #5009, #24353, #5417, #50022, #45663, #74901, #20012, #13706, #77682, #71359, #18471, #49612, #30679, #69806, #23530, #32632, #82039, #43694, #75721, #56340, #12154, #49200, #39361, #58295, #18061, #68982, #65046, #17249, #42878, #68571, #63079, #17651, #660, #10913, #62249, #26316, #55507, #43283, #82444, #24761, #50429, #81215, #76129, #4586, #11330, #44114, #1085, #34308, #26737, #7811, #14553, #14131, #59139, #33477, #67132, #66720, #46917, #40205, #52813, #28399, #8637, #65888, #1908, #66298, #27569, #22088, #52391, #79772, #73447, #54057, #47748, #79353, #1497, #8223, #47333, #78100, #9056, #59553, #21262, #53228, #33887, #73023, #20431, #15797, #15373, #78944, #46500, #41447, #46084, #71777, #39784, #72610, #27149, #41034, #65479, #78523, #34729, #33051, #20847, #14958, #59969, #40615, #58722, #53645, #72200, #2329, #27985, #21672, #60389, #2739, #48580, #28815, #48169, #3151, #17453, #68780, #43083, #81839, #16621, #61211, #75520, #43494, #24150, #4385, #42680, #56134, #68378, #49820, #17859, #42263, #67960, #3979, #23326, #30054, #9461, #49413, #62458, #48996, #10717, #35135, #60797, #54479, #67544, #10302, #80191, #73864, #9879, #35548, #3566, #41852, #16205, #29233, #23740, #74695, #36374, #81425, #54897, #80603, #75106, #55304, #55715, #62048, #22912, #74277, #35968, #11124, #17040, #81013, #61638, #36781, #29643, #4793, #30470, #22508, #50635, #64116, #12360, #57363, #38018, #76340, #25798, #37197, #32534, #142, #6033, #82649, #566, #62878, #5213, #30877, #83059, #37606, #77161, #56544, #75926, #19493, #51882, #5621, #18670, #12776, #44315, #58198, #6451, #18266, #24564, #31287, #82245, #70421, #50230, #24964, #43907, #69605, #11951, #45147, #70850, #13201, #26219, #77587, #38848, #64528, #31705, #70005, #6865, #19921, #38433, #25381, #69190, #32121, #51044, #63280, #56952, #63694, #11541, #44723, #76745, #19075, #57779, #51458, #7717, #78843, #53553, #21169, #66206, #21576, #26646, #78428, #46825, #65797, #45570, #20334, #991, #64947, #79676, #78006, #47238, #58624, #33385, #27893, #65382, #52300, #40527, #40940, #2228, #72517, #27474, #34631, #34211, #8131, #15279, #72928, #79261, #45986, #66619, #14865, #1812, #53132, #71682, #27058, #14034, #39690, #59048, #71264, #8957, #59461, #52717, #1402, #60295, #8545, #20756, #14458, #59874, #40110, #2645, #7287, #28302, #53964, #13611, #39265, #32957, #46406, #72100, #33796, #73350, #55612, #23225, #15698, #61116, #41355, #60704, #67036, #29948, #81323, #23637, #11020 ) ),
 .UNSPECIFIED., .F., .F., .F. ) 
 B_SPLINE_SURFACE_WITH_KNOTS ( ( 2, 2 ),
 ( 3, 2, 2, 2, 2, 2, 2, 2, 2, 2, 2, 2, 2, 2, 2, 2, 2, 2, 2, 2, 2, 2, 2, 2, 2, 2, 2, 2, 2, 2, 2, 2, 2, 2, 2, 2, 2, 2, 2, 2, 2, 2, 2, 2, 2, 2, 2, 2, 2, 2, 2, 2, 2, 2, 2, 2, 2, 2, 2, 2, 2, 2, 2, 2, 2, 2, 2, 2, 2, 2, 2, 2, 2, 2, 2, 2, 2, 2, 2, 2, 2, 2, 2, 2, 2, 2, 2, 2, 2, 2, 2, 2, 2, 2, 2, 2, 2, 2, 2, 2, 2, 2, 2, 2, 2, 2, 2, 2, 2, 2, 2, 2, 2, 2, 2, 2, 2, 2, 2, 2, 2, 2, 2, 2, 2, 2, 2, 2, 2, 2, 2, 2, 2, 2, 2, 2, 2, 2, 2, 2, 2, 2, 2, 2, 2, 2, 2, 2, 2, 2, 2, 2, 2, 2, 2, 2, 2, 2, 2, 2, 2, 2, 2, 2, 2, 2, 2, 2, 2, 2, 2, 2, 2, 2, 2, 2, 2, 2, 2, 2, 2, 2, 2, 2, 2, 2, 2, 2, 2, 2, 2, 2, 2, 2, 2, 2, 2, 2, 2, 2, 2, 2, 2, 2, 2, 2, 2, 2, 2, 2, 2, 2, 2, 2, 2, 2, 2, 2, 2, 2, 2, 2, 2, 2, 2, 2, 2, 2, 2, 2, 2, 2, 2, 2, 2, 2, 2, 2, 2, 2, 2, 2, 2, 2, 2, 2, 2, 2, 2, 2, 2, 2, 2, 2, 2, 3 ),
 ( 0.000000000000000000, 1.000000000000000000 ),
 ( 0.000000000000000000, 0.003787878787878787984, 0.007575757575757575968, 0.01136363636363636395, 0.01515151515151515194, 0.01893939393939393992, 0.02272727272727272790, 0.02651515151515151589, 0.03030303030303030387, 0.03409090909090908839, 0.03787878787878787984, 0.04166666666666666435, 0.04545454545454545581, 0.04924242424242424032, 0.05303030303030303177, 0.05681818181818181629, 0.06060606060606060774, 0.06439393939393939226, 0.06818181818181817677, 0.07196969696969697516, 0.07575757575757575968, 0.07954545454545454419, 0.08333333333333332871, 0.08712121212121212710, 0.09090909090909091161, 0.09469696969696969613, 0.09848484848484848064, 0.1022727272727272790, 0.1060606060606060635, 0.1098484848484848481, 0.1136363636363636326, 0.1174242424242424310, 0.1212121212121212155, 0.1250000000000000000, 0.1287878787878787845, 0.1325757575757575690, 0.1363636363636363535, 0.1401515151515151381, 0.1439393939393939503, 0.1477272727272727348, 0.1515151515151515194, 0.1553030303030303039, 0.1590909090909090884, 0.1628787878787878729, 0.1666666666666666574, 0.1704545454545454419, 0.1742424242424242542, 0.1780303030303030387, 0.1818181818181818232, 0.1856060606060606077, 0.1893939393939393923, 0.1931818181818181768, 0.1969696969696969613, 0.2007575757575757458, 0.2045454545454545581, 0.2083333333333333426, 0.2121212121212121271, 0.2159090909090909116, 0.2196969696969696961, 0.2234848484848484806, 0.2272727272727272652, 0.2310606060606060497, 0.2348484848484848619, 0.2386363636363636465, 0.2424242424242424310, 0.2462121212121212155, 0.2500000000000000000, 0.2537878787878787845, 0.2575757575757575690, 0.2613636363636363535, 0.2651515151515151381, 0.2689393939393939226, 0.2727272727272727071, 0.2765151515151514916, 0.2803030303030302761, 0.2840909090909091161, 0.2878787878787879007, 0.2916666666666666852, 0.2954545454545454697, 0.2992424242424242542, 0.3030303030303030387, 0.3068181818181818232, 0.3106060606060606077, 0.3143939393939393923, 0.3181818181818181768, 0.3219696969696969613, 0.3257575757575757458, 0.3295454545454545303, 0.3333333333333333148, 0.3371212121212120993, 0.3409090909090908839, 0.3446969696969697239, 0.3484848484848485084, 0.3522727272727272929, 0.3560606060606060774, 0.3598484848484848619, 0.3636363636363636465, 0.3674242424242424310, 0.3712121212121212155, 0.3750000000000000000, 0.3787878787878787845, 0.3825757575757575690, 0.3863636363636363535, 0.3901515151515151381, 0.3939393939393939226, 0.3977272727272727071, 0.4015151515151514916, 0.4053030303030302761, 0.4090909090909091161, 0.4128787878787879007, 0.4166666666666666852, 0.4204545454545454697, 0.4242424242424242542, 0.4280303030303030387, 0.4318181818181818232, 0.4356060606060606077, 0.4393939393939393923, 0.4431818181818181768, 0.4469696969696969613, 0.4507575757575757458, 0.4545454545454545303, 0.4583333333333333148, 0.4621212121212120993, 0.4659090909090908839, 0.4696969696969697239, 0.4734848484848485084, 0.4772727272727272929, 0.4810606060606060774, 0.4848484848484848619, 0.4886363636363636465, 0.4924242424242424310, 0.4962121212121212155, 0.5000000000000000000, 0.5037878787878787845, 0.5075757575757575690, 0.5113636363636363535, 0.5151515151515151381, 0.5189393939393939226, 0.5227272727272727071, 0.5265151515151514916, 0.5303030303030302761, 0.5340909090909090606, 0.5378787878787878451, 0.5416666666666666297, 0.5454545454545454142, 0.5492424242424241987, 0.5530303030303029832, 0.5568181818181817677, 0.5606060606060605522, 0.5643939393939394478, 0.5681818181818182323, 0.5719696969696970168, 0.5757575757575758013, 0.5795454545454545858, 0.5833333333333333703, 0.5871212121212121549, 0.5909090909090909394, 0.5946969696969697239, 0.5984848484848485084, 0.6022727272727272929, 0.6060606060606060774, 0.6098484848484848619, 0.6136363636363636465, 0.6174242424242424310, 0.6212121212121212155, 0.6250000000000000000, 0.6287878787878787845, 0.6325757575757575690, 0.6363636363636363535, 0.6401515151515151381, 0.6439393939393939226, 0.6477272727272727071, 0.6515151515151514916, 0.6553030303030302761, 0.6590909090909090606, 0.6628787878787878451, 0.6666666666666666297, 0.6704545454545454142, 0.6742424242424241987, 0.6780303030303029832, 0.6818181818181817677, 0.6856060606060605522, 0.6893939393939394478, 0.6931818181818182323, 0.6969696969696970168, 0.7007575757575758013, 0.7045454545454545858, 0.7083333333333333703, 0.7121212121212121549, 0.7159090909090909394, 0.7196969696969697239, 0.7234848484848485084, 0.7272727272727272929, 0.7310606060606060774, 0.7348484848484848619, 0.7386363636363636465, 0.7424242424242424310, 0.7462121212121212155, 0.7500000000000000000, 0.7537878787878787845, 0.7575757575757575690, 0.7613636363636363535, 0.7651515151515151381, 0.7689393939393939226, 0.7727272727272727071, 0.7765151515151514916, 0.7803030303030302761, 0.7840909090909090606, 0.7878787878787878451, 0.7916666666666666297, 0.7954545454545454142, 0.7992424242424241987, 0.8030303030303029832, 0.8068181818181817677, 0.8106060606060605522, 0.8143939393939394478, 0.8181818181818182323, 0.8219696969696970168, 0.8257575757575758013, 0.8295454545454545858, 0.8333333333333333703, 0.8371212121212121549, 0.8409090909090909394, 0.8446969696969697239, 0.8484848484848485084, 0.8522727272727272929, 0.8560606060606060774, 0.8598484848484848619, 0.8636363636363636465, 0.8674242424242424310, 0.8712121212121212155, 0.8750000000000000000, 0.8787878787878787845, 0.8825757575757575690, 0.8863636363636363535, 0.8901515151515151381, 0.8939393939393939226, 0.8977272727272727071, 0.9015151515151514916, 0.9053030303030302761, 0.9090909090909090606, 0.9128787878787878451, 0.9166666666666666297, 0.9204545454545454142, 0.9242424242424241987, 0.9280303030303029832, 0.9318181818181817677, 0.9356060606060605522, 0.9393939393939394478, 0.9431818181818182323, 0.9469696969696970168, 0.9507575757575758013, 0.9545454545454545858, 0.9583333333333333703, 0.9621212121212121549, 0.9659090909090909394 ),
 .UNSPECIFIED. ) 
 GEOMETRIC_REPRESENTATION_ITEM ( )  RATIONAL_B_SPLINE_SURFACE ( (
 ( 1.000000000000000000, 0.9659258262890683122, 1.000000000000000000, 0.9659258262890683122, 1.000000000000000000, 0.9659258262890683122, 1.000000000000000000, 0.9659258262890683122, 1.000000000000000000, 0.9659258262890683122, 1.000000000000000000, 0.9659258262890683122, 1.000000000000000000, 0.9659258262890683122, 1.000000000000000000, 0.9659258262890683122, 1.000000000000000000, 0.9659258262890683122, 1.000000000000000000, 0.9659258262890683122, 1.000000000000000000, 0.9659258262890683122, 1.000000000000000000, 0.9659258262890683122, 1.000000000000000000, 0.9659258262890683122, 1.000000000000000000, 0.9659258262890683122, 1.000000000000000000, 0.9659258262890683122, 1.000000000000000000, 0.9659258262890683122, 1.000000000000000000, 0.9659258262890683122, 1.000000000000000000, 0.9659258262890683122, 1.000000000000000000, 0.9659258262890683122, 1.000000000000000000, 0.9659258262890683122, 1.000000000000000000, 0.9659258262890683122, 1.000000000000000000, 0.9659258262890683122, 1.000000000000000000, 0.9659258262890683122, 1.000000000000000000, 0.9659258262890683122, 1.000000000000000000, 0.9659258262890683122, 1.000000000000000000, 0.9659258262890683122, 1.000000000000000000, 0.9659258262890683122, 1.000000000000000000, 0.9659258262890683122, 1.000000000000000000, 0.9659258262890683122, 1.000000000000000000, 0.9659258262890683122, 1.000000000000000000, 0.9659258262890683122, 1.000000000000000000, 0.9659258262890683122, 1.000000000000000000, 0.9659258262890683122, 1.000000000000000000, 0.9659258262890683122, 1.000000000000000000, 0.9659258262890683122, 1.000000000000000000, 0.9659258262890683122, 1.000000000000000000, 0.9659258262890683122, 1.000000000000000000, 0.9659258262890683122, 1.000000000000000000, 0.9659258262890683122, 1.000000000000000000, 0.9659258262890683122, 1.000000000000000000, 0.9659258262890683122, 1.000000000000000000, 0.9659258262890683122, 1.000000000000000000, 0.9659258262890683122, 1.000000000000000000, 0.9659258262890683122, 1.000000000000000000, 0.9659258262890683122, 1.000000000000000000, 0.9659258262890683122, 1.000000000000000000, 0.9659258262890683122, 1.000000000000000000, 0.9659258262890683122, 1.000000000000000000, 0.9659258262890683122, 1.000000000000000000, 0.9659258262890683122, 1.000000000000000000, 0.9659258262890683122, 1.000000000000000000, 0.9659258262890683122, 1.000000000000000000, 0.9659258262890683122, 1.000000000000000000, 0.9659258262890683122, 1.000000000000000000, 0.9659258262890683122, 1.000000000000000000, 0.9659258262890683122, 1.000000000000000000, 0.9659258262890683122, 1.000000000000000000, 0.9659258262890683122, 1.000000000000000000, 0.9659258262890683122, 1.000000000000000000, 0.9659258262890683122, 1.000000000000000000, 0.9659258262890683122, 1.000000000000000000, 0.9659258262890683122, 1.000000000000000000, 0.9659258262890683122, 1.000000000000000000, 0.9659258262890683122, 1.000000000000000000, 0.9659258262890683122, 1.000000000000000000, 0.9659258262890683122, 1.000000000000000000, 0.9659258262890683122, 1.000000000000000000, 0.9659258262890683122, 1.000000000000000000, 0.9659258262890683122, 1.000000000000000000, 0.9659258262890683122, 1.000000000000000000, 0.9659258262890683122, 1.000000000000000000, 0.9659258262890683122, 1.000000000000000000, 0.9659258262890683122, 1.000000000000000000, 0.9659258262890683122, 1.000000000000000000, 0.9659258262890683122, 1.000000000000000000, 0.9659258262890683122, 1.000000000000000000, 0.9659258262890683122, 1.000000000000000000, 0.9659258262890683122, 1.000000000000000000, 0.9659258262890683122, 1.000000000000000000, 0.9659258262890683122, 1.000000000000000000, 0.9659258262890683122, 1.000000000000000000, 0.9659258262890683122, 1.000000000000000000, 0.9659258262890683122, 1.000000000000000000, 0.9659258262890683122, 1.000000000000000000, 0.9659258262890683122, 1.000000000000000000, 0.9659258262890683122, 1.000000000000000000, 0.9659258262890683122, 1.000000000000000000, 0.9659258262890683122, 1.000000000000000000, 0.9659258262890683122, 1.000000000000000000, 0.9659258262890683122, 1.000000000000000000, 0.9659258262890683122, 1.000000000000000000, 0.9659258262890683122, 1.000000000000000000, 0.9659258262890683122, 1.000000000000000000, 0.9659258262890683122, 1.000000000000000000, 0.9659258262890683122, 1.000000000000000000, 0.9659258262890683122, 1.000000000000000000, 0.9659258262890683122, 1.000000000000000000, 0.9659258262890683122, 1.000000000000000000, 0.9659258262890683122, 1.000000000000000000, 0.9659258262890683122, 1.000000000000000000, 0.9659258262890683122, 1.000000000000000000, 0.9659258262890683122, 1.000000000000000000, 0.9659258262890683122, 1.000000000000000000, 0.9659258262890683122, 1.000000000000000000, 0.9659258262890683122, 1.000000000000000000, 0.9659258262890683122, 1.000000000000000000, 0.9659258262890683122, 1.000000000000000000, 0.9659258262890683122, 1.000000000000000000, 0.9659258262890683122, 1.000000000000000000, 0.9659258262890683122, 1.000000000000000000, 0.9659258262890683122, 1.000000000000000000, 0.9659258262890683122, 1.000000000000000000, 0.9659258262890683122, 1.000000000000000000, 0.9659258262890683122, 1.000000000000000000, 0.9659258262890683122, 1.000000000000000000, 0.9659258262890683122, 1.000000000000000000, 0.9659258262890683122, 1.000000000000000000, 0.9659258262890683122, 1.000000000000000000, 0.9659258262890683122, 1.000000000000000000, 0.9659258262890683122, 1.000000000000000000, 0.9659258262890683122, 1.000000000000000000, 0.9659258262890683122, 1.000000000000000000, 0.9659258262890683122, 1.000000000000000000, 0.9659258262890683122, 1.000000000000000000, 0.9659258262890683122, 1.000000000000000000, 0.9659258262890683122, 1.000000000000000000, 0.9659258262890683122, 1.000000000000000000, 0.9659258262890683122, 1.000000000000000000, 0.9659258262890683122, 1.000000000000000000, 0.9659258262890683122, 1.000000000000000000, 0.9659258262890683122, 1.000000000000000000, 0.9659258262890683122, 1.000000000000000000, 0.9659258262890683122, 1.000000000000000000, 0.9659258262890683122, 1.000000000000000000, 0.9659258262890683122, 1.000000000000000000, 0.9659258262890683122, 1.000000000000000000, 0.9659258262890683122, 1.000000000000000000, 0.9659258262890683122, 1.000000000000000000, 0.9659258262890683122, 1.000000000000000000, 0.9659258262890683122, 1.000000000000000000, 0.9659258262890683122, 1.000000000000000000, 0.9659258262890683122, 1.000000000000000000, 0.9659258262890683122, 1.000000000000000000, 0.9659258262890683122, 1.000000000000000000, 0.9659258262890683122, 1.000000000000000000, 0.9659258262890683122, 1.000000000000000000, 0.9659258262890683122, 1.000000000000000000, 0.9659258262890683122, 1.000000000000000000, 0.9659258262890683122, 1.000000000000000000, 0.9659258262890683122, 1.000000000000000000, 0.9659258262890683122, 1.000000000000000000, 0.9659258262890683122, 1.000000000000000000, 0.9659258262890683122, 1.000000000000000000, 0.9659258262890683122, 1.000000000000000000, 0.9659258262890683122, 1.000000000000000000, 0.9659258262890683122, 1.000000000000000000, 0.9659258262890683122, 1.000000000000000000, 0.9659258262890683122, 1.000000000000000000, 0.9659258262890683122, 1.000000000000000000, 0.9659258262890683122, 1.000000000000000000, 0.9659258262890683122, 1.000000000000000000, 0.9659258262890683122, 1.000000000000000000, 0.9659258262890683122, 1.000000000000000000, 0.9659258262890683122, 1.000000000000000000, 0.9659258262890683122, 1.000000000000000000, 0.9659258262890683122, 1.000000000000000000, 0.9659258262890683122, 1.000000000000000000, 0.9659258262890683122, 1.000000000000000000, 0.9659258262890683122, 1.000000000000000000, 0.9659258262890683122, 1.000000000000000000, 0.9659258262890683122, 1.000000000000000000, 0.9659258262890683122, 1.000000000000000000, 0.9659258262890683122, 1.000000000000000000, 0.9659258262890683122, 1.000000000000000000, 0.9659258262890683122, 1.000000000000000000, 0.9659258262890683122, 1.000000000000000000, 0.9659258262890683122, 1.000000000000000000, 0.9659258262890683122, 1.000000000000000000, 0.9659258262890683122, 1.000000000000000000, 0.9659258262890683122, 1.000000000000000000, 0.9659258262890683122, 1.000000000000000000, 0.9659258262890683122, 1.000000000000000000, 0.9659258262890683122, 1.000000000000000000, 0.9659258262890683122, 1.000000000000000000, 0.9659258262890683122, 1.000000000000000000, 0.9659258262890683122, 1.000000000000000000, 0.9659258262890683122, 1.000000000000000000, 0.9659258262890683122, 1.000000000000000000, 0.9659258262890683122, 1.000000000000000000, 0.9659258262890683122, 1.000000000000000000, 0.9659258262890683122, 1.000000000000000000, 0.9659258262890683122, 1.000000000000000000, 0.9659258262890683122, 1.000000000000000000, 0.9659258262890683122, 1.000000000000000000, 0.9659258262890683122, 1.000000000000000000, 0.9659258262890683122, 1.000000000000000000, 0.9659258262890683122, 1.000000000000000000, 0.9659258262890683122, 1.000000000000000000, 0.9659258262890683122, 1.000000000000000000, 0.9659258262890683122, 1.000000000000000000, 0.9659258262890683122, 1.000000000000000000, 0.9659258262890683122, 1.000000000000000000, 0.9659258262890683122, 1.000000000000000000, 0.9659258262890683122, 1.000000000000000000, 0.9659258262890683122, 1.000000000000000000, 0.9659258262890683122, 1.000000000000000000, 0.9659258262890683122, 1.000000000000000000, 0.9659258262890683122, 1.000000000000000000, 0.9659258262890683122, 1.000000000000000000, 0.9659258262890683122, 1.000000000000000000, 0.9659258262890683122, 1.000000000000000000, 0.9659258262890683122, 1.000000000000000000, 0.9659258262890683122, 1.000000000000000000, 0.9659258262890683122, 1.000000000000000000, 0.9659258262890683122, 1.000000000000000000, 0.9659258262890683122, 1.000000000000000000, 0.9659258262890683122, 1.000000000000000000, 0.9659258262890683122, 1.000000000000000000, 0.9659258262890683122, 1.000000000000000000, 0.9659258262890683122, 1.000000000000000000, 0.9659258262890683122, 1.000000000000000000, 0.9659258262890683122, 1.000000000000000000, 0.9659258262890683122, 1.000000000000000000, 0.9659258262890683122, 1.000000000000000000, 0.9659258262890683122, 1.000000000000000000, 0.9659258262890683122, 1.000000000000000000, 0.9659258262890683122, 1.000000000000000000, 0.9659258262890683122, 1.000000000000000000, 0.9659258262890683122, 1.000000000000000000, 0.9659258262890683122, 1.000000000000000000, 0.9659258262890683122, 1.000000000000000000, 0.9659258262890683122, 1.000000000000000000, 0.9659258262890683122, 1.000000000000000000, 0.9659258262890683122, 1.000000000000000000, 0.9659258262890683122, 1.000000000000000000, 0.9659258262890683122, 1.000000000000000000, 0.9659258262890683122, 1.000000000000000000, 0.9659258262890683122, 1.000000000000000000, 0.9659258262890683122, 1.000000000000000000, 0.9659258262890683122, 1.000000000000000000, 0.9659258262890683122, 1.000000000000000000, 0.9659258262890683122, 1.000000000000000000, 0.9659258262890683122, 1.000000000000000000, 0.9659258262890683122, 1.000000000000000000, 0.9659258262890683122, 1.000000000000000000, 0.9659258262890683122, 1.000000000000000000, 0.9659258262890683122, 1.000000000000000000, 0.9659258262890683122, 1.000000000000000000, 0.9659258262890683122, 1.000000000000000000, 0.9659258262890683122, 1.000000000000000000, 0.9659258262890683122, 1.000000000000000000, 0.9659258262890683122, 1.000000000000000000, 0.9659258262890683122, 1.000000000000000000, 0.9659258262890683122, 1.000000000000000000, 0.9659258262890683122, 1.000000000000000000),
 ( 1.000000000000000000, 0.9659258262890683122, 1.000000000000000000, 0.9659258262890683122, 1.000000000000000000, 0.9659258262890683122, 1.000000000000000000, 0.9659258262890683122, 1.000000000000000000, 0.9659258262890683122, 1.000000000000000000, 0.9659258262890683122, 1.000000000000000000, 0.9659258262890683122, 1.000000000000000000, 0.9659258262890683122, 1.000000000000000000, 0.9659258262890683122, 1.000000000000000000, 0.9659258262890683122, 1.000000000000000000, 0.9659258262890683122, 1.000000000000000000, 0.9659258262890683122, 1.000000000000000000, 0.9659258262890683122, 1.000000000000000000, 0.9659258262890683122, 1.000000000000000000, 0.9659258262890683122, 1.000000000000000000, 0.9659258262890683122, 1.000000000000000000, 0.9659258262890683122, 1.000000000000000000, 0.9659258262890683122, 1.000000000000000000, 0.9659258262890683122, 1.000000000000000000, 0.9659258262890683122, 1.000000000000000000, 0.9659258262890683122, 1.000000000000000000, 0.9659258262890683122, 1.000000000000000000, 0.9659258262890683122, 1.000000000000000000, 0.9659258262890683122, 1.000000000000000000, 0.9659258262890683122, 1.000000000000000000, 0.9659258262890683122, 1.000000000000000000, 0.9659258262890683122, 1.000000000000000000, 0.9659258262890683122, 1.000000000000000000, 0.9659258262890683122, 1.000000000000000000, 0.9659258262890683122, 1.000000000000000000, 0.9659258262890683122, 1.000000000000000000, 0.9659258262890683122, 1.000000000000000000, 0.9659258262890683122, 1.000000000000000000, 0.9659258262890683122, 1.000000000000000000, 0.9659258262890683122, 1.000000000000000000, 0.9659258262890683122, 1.000000000000000000, 0.9659258262890683122, 1.000000000000000000, 0.9659258262890683122, 1.000000000000000000, 0.9659258262890683122, 1.000000000000000000, 0.9659258262890683122, 1.000000000000000000, 0.9659258262890683122, 1.000000000000000000, 0.9659258262890683122, 1.000000000000000000, 0.9659258262890683122, 1.000000000000000000, 0.9659258262890683122, 1.000000000000000000, 0.9659258262890683122, 1.000000000000000000, 0.9659258262890683122, 1.000000000000000000, 0.9659258262890683122, 1.000000000000000000, 0.9659258262890683122, 1.000000000000000000, 0.9659258262890683122, 1.000000000000000000, 0.9659258262890683122, 1.000000000000000000, 0.9659258262890683122, 1.000000000000000000, 0.9659258262890683122, 1.000000000000000000, 0.9659258262890683122, 1.000000000000000000, 0.9659258262890683122, 1.000000000000000000, 0.9659258262890683122, 1.000000000000000000, 0.9659258262890683122, 1.000000000000000000, 0.9659258262890683122, 1.000000000000000000, 0.9659258262890683122, 1.000000000000000000, 0.9659258262890683122, 1.000000000000000000, 0.9659258262890683122, 1.000000000000000000, 0.9659258262890683122, 1.000000000000000000, 0.9659258262890683122, 1.000000000000000000, 0.9659258262890683122, 1.000000000000000000, 0.9659258262890683122, 1.000000000000000000, 0.9659258262890683122, 1.000000000000000000, 0.9659258262890683122, 1.000000000000000000, 0.9659258262890683122, 1.000000000000000000, 0.9659258262890683122, 1.000000000000000000, 0.9659258262890683122, 1.000000000000000000, 0.9659258262890683122, 1.000000000000000000, 0.9659258262890683122, 1.000000000000000000, 0.9659258262890683122, 1.000000000000000000, 0.9659258262890683122, 1.000000000000000000, 0.9659258262890683122, 1.000000000000000000, 0.9659258262890683122, 1.000000000000000000, 0.9659258262890683122, 1.000000000000000000, 0.9659258262890683122, 1.000000000000000000, 0.9659258262890683122, 1.000000000000000000, 0.9659258262890683122, 1.000000000000000000, 0.9659258262890683122, 1.000000000000000000, 0.9659258262890683122, 1.000000000000000000, 0.9659258262890683122, 1.000000000000000000, 0.9659258262890683122, 1.000000000000000000, 0.9659258262890683122, 1.000000000000000000, 0.9659258262890683122, 1.000000000000000000, 0.9659258262890683122, 1.000000000000000000, 0.9659258262890683122, 1.000000000000000000, 0.9659258262890683122, 1.000000000000000000, 0.9659258262890683122, 1.000000000000000000, 0.9659258262890683122, 1.000000000000000000, 0.9659258262890683122, 1.000000000000000000, 0.9659258262890683122, 1.000000000000000000, 0.9659258262890683122, 1.000000000000000000, 0.9659258262890683122, 1.000000000000000000, 0.9659258262890683122, 1.000000000000000000, 0.9659258262890683122, 1.000000000000000000, 0.9659258262890683122, 1.000000000000000000, 0.9659258262890683122, 1.000000000000000000, 0.9659258262890683122, 1.000000000000000000, 0.9659258262890683122, 1.000000000000000000, 0.9659258262890683122, 1.000000000000000000, 0.9659258262890683122, 1.000000000000000000, 0.9659258262890683122, 1.000000000000000000, 0.9659258262890683122, 1.000000000000000000, 0.9659258262890683122, 1.000000000000000000, 0.9659258262890683122, 1.000000000000000000, 0.9659258262890683122, 1.000000000000000000, 0.9659258262890683122, 1.000000000000000000, 0.9659258262890683122, 1.000000000000000000, 0.9659258262890683122, 1.000000000000000000, 0.9659258262890683122, 1.000000000000000000, 0.9659258262890683122, 1.000000000000000000, 0.9659258262890683122, 1.000000000000000000, 0.9659258262890683122, 1.000000000000000000, 0.9659258262890683122, 1.000000000000000000, 0.9659258262890683122, 1.000000000000000000, 0.9659258262890683122, 1.000000000000000000, 0.9659258262890683122, 1.000000000000000000, 0.9659258262890683122, 1.000000000000000000, 0.9659258262890683122, 1.000000000000000000, 0.9659258262890683122, 1.000000000000000000, 0.9659258262890683122, 1.000000000000000000, 0.9659258262890683122, 1.000000000000000000, 0.9659258262890683122, 1.000000000000000000, 0.9659258262890683122, 1.000000000000000000, 0.9659258262890683122, 1.000000000000000000, 0.9659258262890683122, 1.000000000000000000, 0.9659258262890683122, 1.000000000000000000, 0.9659258262890683122, 1.000000000000000000, 0.9659258262890683122, 1.000000000000000000, 0.9659258262890683122, 1.000000000000000000, 0.9659258262890683122, 1.000000000000000000, 0.9659258262890683122, 1.000000000000000000, 0.9659258262890683122, 1.000000000000000000, 0.9659258262890683122, 1.000000000000000000, 0.9659258262890683122, 1.000000000000000000, 0.9659258262890683122, 1.000000000000000000, 0.9659258262890683122, 1.000000000000000000, 0.9659258262890683122, 1.000000000000000000, 0.9659258262890683122, 1.000000000000000000, 0.9659258262890683122, 1.000000000000000000, 0.9659258262890683122, 1.000000000000000000, 0.9659258262890683122, 1.000000000000000000, 0.9659258262890683122, 1.000000000000000000, 0.9659258262890683122, 1.000000000000000000, 0.9659258262890683122, 1.000000000000000000, 0.9659258262890683122, 1.000000000000000000, 0.9659258262890683122, 1.000000000000000000, 0.9659258262890683122, 1.000000000000000000, 0.9659258262890683122, 1.000000000000000000, 0.9659258262890683122, 1.000000000000000000, 0.9659258262890683122, 1.000000000000000000, 0.9659258262890683122, 1.000000000000000000, 0.9659258262890683122, 1.000000000000000000, 0.9659258262890683122, 1.000000000000000000, 0.9659258262890683122, 1.000000000000000000, 0.9659258262890683122, 1.000000000000000000, 0.9659258262890683122, 1.000000000000000000, 0.9659258262890683122, 1.000000000000000000, 0.9659258262890683122, 1.000000000000000000, 0.9659258262890683122, 1.000000000000000000, 0.9659258262890683122, 1.000000000000000000, 0.9659258262890683122, 1.000000000000000000, 0.9659258262890683122, 1.000000000000000000, 0.9659258262890683122, 1.000000000000000000, 0.9659258262890683122, 1.000000000000000000, 0.9659258262890683122, 1.000000000000000000, 0.9659258262890683122, 1.000000000000000000, 0.9659258262890683122, 1.000000000000000000, 0.9659258262890683122, 1.000000000000000000, 0.9659258262890683122, 1.000000000000000000, 0.9659258262890683122, 1.000000000000000000, 0.9659258262890683122, 1.000000000000000000, 0.9659258262890683122, 1.000000000000000000, 0.9659258262890683122, 1.000000000000000000, 0.9659258262890683122, 1.000000000000000000, 0.9659258262890683122, 1.000000000000000000, 0.9659258262890683122, 1.000000000000000000, 0.9659258262890683122, 1.000000000000000000, 0.9659258262890683122, 1.000000000000000000, 0.9659258262890683122, 1.000000000000000000, 0.9659258262890683122, 1.000000000000000000, 0.9659258262890683122, 1.000000000000000000, 0.9659258262890683122, 1.000000000000000000, 0.9659258262890683122, 1.000000000000000000, 0.9659258262890683122, 1.000000000000000000, 0.9659258262890683122, 1.000000000000000000, 0.9659258262890683122, 1.000000000000000000, 0.9659258262890683122, 1.000000000000000000, 0.9659258262890683122, 1.000000000000000000, 0.9659258262890683122, 1.000000000000000000, 0.9659258262890683122, 1.000000000000000000, 0.9659258262890683122, 1.000000000000000000, 0.9659258262890683122, 1.000000000000000000, 0.9659258262890683122, 1.000000000000000000, 0.9659258262890683122, 1.000000000000000000, 0.9659258262890683122, 1.000000000000000000, 0.9659258262890683122, 1.000000000000000000, 0.9659258262890683122, 1.000000000000000000, 0.9659258262890683122, 1.000000000000000000, 0.9659258262890683122, 1.000000000000000000, 0.9659258262890683122, 1.000000000000000000, 0.9659258262890683122, 1.000000000000000000, 0.9659258262890683122, 1.000000000000000000, 0.9659258262890683122, 1.000000000000000000, 0.9659258262890683122, 1.000000000000000000, 0.9659258262890683122, 1.000000000000000000, 0.9659258262890683122, 1.000000000000000000, 0.9659258262890683122, 1.000000000000000000, 0.9659258262890683122, 1.000000000000000000, 0.9659258262890683122, 1.000000000000000000, 0.9659258262890683122, 1.000000000000000000, 0.9659258262890683122, 1.000000000000000000, 0.9659258262890683122, 1.000000000000000000, 0.9659258262890683122, 1.000000000000000000, 0.9659258262890683122, 1.000000000000000000, 0.9659258262890683122, 1.000000000000000000, 0.9659258262890683122, 1.000000000000000000, 0.9659258262890683122, 1.000000000000000000, 0.9659258262890683122, 1.000000000000000000, 0.9659258262890683122, 1.000000000000000000, 0.9659258262890683122, 1.000000000000000000, 0.9659258262890683122, 1.000000000000000000, 0.9659258262890683122, 1.000000000000000000, 0.9659258262890683122, 1.000000000000000000, 0.9659258262890683122, 1.000000000000000000, 0.9659258262890683122, 1.000000000000000000, 0.9659258262890683122, 1.000000000000000000, 0.9659258262890683122, 1.000000000000000000, 0.9659258262890683122, 1.000000000000000000, 0.9659258262890683122, 1.000000000000000000, 0.9659258262890683122, 1.000000000000000000, 0.9659258262890683122, 1.000000000000000000, 0.9659258262890683122, 1.000000000000000000, 0.9659258262890683122, 1.000000000000000000, 0.9659258262890683122, 1.000000000000000000, 0.9659258262890683122, 1.000000000000000000, 0.9659258262890683122, 1.000000000000000000, 0.9659258262890683122, 1.000000000000000000, 0.9659258262890683122, 1.000000000000000000, 0.9659258262890683122, 1.000000000000000000, 0.9659258262890683122, 1.000000000000000000, 0.9659258262890683122, 1.000000000000000000, 0.9659258262890683122, 1.000000000000000000, 0.9659258262890683122, 1.000000000000000000, 0.9659258262890683122, 1.000000000000000000, 0.9659258262890683122, 1.000000000000000000, 0.9659258262890683122, 1.000000000000000000, 0.9659258262890683122, 1.000000000000000000, 0.9659258262890683122, 1.000000000000000000, 0.9659258262890683122, 1.000000000000000000, 0.9659258262890683122, 1.000000000000000000, 0.9659258262890683122, 1.000000000000000000, 0.9659258262890683122, 1.000000000000000000, 0.9659258262890683122, 1.000000000000000000) ) ) 
 REPRESENTATION_ITEM ( '' )  SURFACE ( )  );
#362=CARTESIAN_POINT ( 'NONE',  ( -0.9580052493438311334, -0.004921259842519870586, -0.3153832671262229437 ) ) ;
#363=CARTESIAN_POINT ( 'NONE',  ( -1.377952755905511140, 0.1771653543307087630, 0.000000000000000000 ) ) ;
#364=CARTESIAN_POINT ( 'NONE',  ( 1.450131233595801428, 0.2952755905511811885, 0.1292274648535926551 ) ) ;
#370=CARTESIAN_POINT ( 'NONE',  ( 1.410761154855643795, -0.2845877964562159024, 0.3641732283464567677 ) ) ;
#371=CARTESIAN_POINT ( 'NONE',  ( -1.351706036745406347, 0.05413385826771626580, -0.4176697321401330321 ) ) ;
#372=CARTESIAN_POINT ( 'NONE',  ( -1.594488188976377119, 0.1660481256975883668, -0.3530559997133364547 ) ) ;
#375=CARTESIAN_POINT ( 'NONE',  ( 0.5971128608923891301, 0.2952755905511810774, -0.1292274648535930714 ) ) ;
#376=CARTESIAN_POINT ( 'NONE',  ( 0.1181102362204730916, 0.2952755905511811885, 0.000000000000000000 ) ) ;
#378=CARTESIAN_POINT ( 'NONE',  ( -0.6430446194225712953, 0.05413385826771626580, -0.4176697321401330321 ) ) ;
#379=CARTESIAN_POINT ( 'NONE',  ( 0.6758530183727039509, 0.1771653543307087075, -0.09757992244046823083 ) ) ;
#384=CARTESIAN_POINT ( 'NONE',  ( -0.07874015748031421014, -0.1870078740157480879, -0.4822834645669291653 ) ) ;
#385=CARTESIAN_POINT ( 'NONE',  ( -1.332020997375327642, -0.05778040916215522460, 0.4822834645669289988 ) ) ;
#386=CARTESIAN_POINT ( 'NONE',  ( 0.5708661417322842269, 0.1660481256975885056, 0.3530559997133364547 ) ) ;
#387=CARTESIAN_POINT ( 'NONE',  ( 1.030183727034121421, -0.05778040916215522460, 0.4822834645669289988 ) ) ;
#388=CARTESIAN_POINT ( 'NONE',  ( 1.574803149606299746, -0.1870078740157479769, 0.4822834645669291653 ) ) ;
#389=CARTESIAN_POINT ( 'NONE',  ( -0.3543307086614165824, 0.2952755905511811885, 0.000000000000000000 ) ) ;
#390=CARTESIAN_POINT ( 'NONE',  ( -0.1640419947506555343, -0.3162353388693405765, 0.4822834645669290543 ) ) ;
#391=CARTESIAN_POINT ( 'NONE',  ( 1.482939632545932307, 0.05413385826771626580, -0.4176697321401330321 ) ) ;
#392=CARTESIAN_POINT ( 'NONE',  ( 1.443569553805774897, 0.2306618581243848609, 0.2411417322834645549 ) ) ;
#393=CARTESIAN_POINT ( 'NONE',  ( 1.345144356955381593, -0.05778040916215522460, 0.4822834645669289988 ) ) ;
#394=CARTESIAN_POINT ( 'NONE',  ( -0.3083989501312330295, -0.05778040916215522460, 0.4822834645669289988 ) ) ;
#396=CARTESIAN_POINT ( 'NONE',  ( 0.2755905511811031494, 0.1771653543307087630, 0.000000000000000000 ) ) ;
#399=B_SPLINE_CURVE_WITH_KNOTS ( 'NONE', 3,
 ( #14331, #45441, #8006, #13068 ),
 .UNSPECIFIED., .F., .F.,
 ( 4, 4 ),
 ( 0.05904796282231847965, 0.06105363127456257810 ),
 .UNSPECIFIED. ) ;
#401=CARTESIAN_POINT ( 'NONE',  ( -0.4593175853018366950, -0.004921259842519576551, 0.3153832671262227771 ) ) ;
#402=CARTESIAN_POINT ( 'NONE',  ( 1.614173228346456712, 2.401574803149606474, 0.5309055118110233007 ) ) ;
#403=CARTESIAN_POINT ( 'NONE',  ( 0.1706036745406830368, 0.05413385826771666132, 0.4176697321401328100 ) ) ;
#404=CARTESIAN_POINT ( 'NONE',  ( -0.1771653543307080136, -0.5400638737290844871, 0.3530559997133364547 ) ) ;
#405=EDGE_CURVE ( 'NONE', #79849, #33739, #16525, .T. ) ;
#406=CARTESIAN_POINT ( 'NONE',  ( -0.9120734908136475250, 0.2952755905511811885, 0.1292274648535926551 ) ) ;
#408=CARTESIAN_POINT ( 'NONE',  ( -1.338582677165353729, -0.1870078740157479769, 0.4822834645669291653 ) ) ;
#410=CARTESIAN_POINT ( 'NONE',  ( 1.056430446194226436, -0.5511811023622048555, -0.09757992244046775898 ) ) ;
#412=CARTESIAN_POINT ( 'NONE',  ( 0.4068241469816281097, 0.05413385826771666132, 0.4176697321401328100 ) ) ;
#413=CARTESIAN_POINT ( 'NONE',  ( 0.8858267716535438430, 0.1660481256975885056, 0.3530559997133364547 ) ) ;
#415=CARTESIAN_POINT ( 'NONE',  ( -1.568241469816272105, -0.05778040916215522460, 0.4822834645669289988 ) ) ;
#418=CARTESIAN_POINT ( 'NONE',  ( -0.01312335958005186876, -0.4281496062992124485, 0.4176697321401328655 ) ) ;
#421=CARTESIAN_POINT ( 'NONE',  ( -1.371391076115484609, -0.5511811023622046335, 0.09757992244046803654 ) ) ;
#422=CARTESIAN_POINT ( 'NONE',  ( 1.246719160104987623, -0.4281496062992124485, 0.4176697321401328655 ) ) ;
#423=CARTESIAN_POINT ( 'NONE',  ( 1.174540682414699111, -0.3162353388693405765, 0.4822834645669290543 ) ) ;
#424=CARTESIAN_POINT ( 'NONE',  ( 0.1049868766404206816, 0.1283753931104748280, 0.1820866141732283561 ) ) ;
#425=CARTESIAN_POINT ( 'NONE',  ( 0.5708661417322841158, -0.5400638737290845981, -0.3530559997133363437 ) ) ;
#427=CARTESIAN_POINT ( 'NONE',  ( 0.5314960629921267055, -0.4536011799217367080, 0.2665933059059888421 ) ) ;
#428=CARTESIAN_POINT ( 'NONE',  ( -0.1246719160104980823, 0.2952755905511811885, 0.1292274648535926551 ) ) ;
#431=CARTESIAN_POINT ( 'NONE',  ( -1.122047244094487306, -0.5400638737290844871, 0.3530559997133364547 ) ) ;
#432=CARTESIAN_POINT ( 'NONE',  ( 0.5971128608923890191, -0.5511811023622046335, 0.09757992244046803654 ) ) ;
#433=CARTESIAN_POINT ( 'NONE',  ( 0.4606732211678742361, 1.778019097314512686, 0.5309055118110234117 ) ) ;
#434=CARTESIAN_POINT ( 'NONE',  ( -0.6299212598425188991, -0.1870078740157479769, 0.4822834645669291653 ) ) ;
#435=CARTESIAN_POINT ( 'NONE',  ( -0.1640419947506553400, -0.08942795157528024563, -0.3641732283464568787 ) ) ;
#437=CARTESIAN_POINT ( 'NONE',  ( -0.2952755905511804668, 0.1660481256975885056, 0.3530559997133364547 ) ) ;
#438=CARTESIAN_POINT ( 'NONE',  ( -0.4002624671916004129, -0.3162353388693405765, 0.4822834645669290543 ) ) ;
#439=CARTESIAN_POINT ( 'NONE',  ( 0.4593175853018379162, -0.3690944881889763329, 0.3153832671262228327 ) ) ;
#441=CARTESIAN_POINT ( 'NONE',  ( -0.1312335958005241554, -0.6046776061558809534, -0.2411417322834644161 ) ) ;
#443=CARTESIAN_POINT ( 'NONE',  ( 0.8661417322834653598, -0.1870078740157479769, 0.3641732283464567677 ) ) ;
#444=CARTESIAN_POINT ( 'NONE',  ( 1.266404199475066328, -0.05778040916215522460, 0.4822834645669289988 ) ) ;
#445=CARTESIAN_POINT ( 'NONE',  ( -0.9842519685039365918, -0.5511811023622047445, 6.969142054262312111E-17 ) ) ;
#446=CARTESIAN_POINT ( 'NONE',  ( -0.7283464566929126471, 0.07958543189024071263, -0.2665933059059888421 ) ) ;
#447=CARTESIAN_POINT ( 'NONE',  ( -0.8727034120734901146, -0.3162353388693405765, 0.4822834645669290543 ) ) ;
#448=CARTESIAN_POINT ( 'NONE',  ( -0.2362204724409442680, -0.1870078740157480879, -0.4822834645669291653 ) ) ;
#449=CARTESIAN_POINT ( 'NONE',  ( 0.3871391076115493490, -0.2845877964562159024, 0.3641732283464567677 ) ) ;
#451=CARTESIAN_POINT ( 'NONE',  ( 1.233595800524935227, -0.5023911411419708095, 0.1820866141732285504 ) ) ;
#452=CARTESIAN_POINT ( 'NONE',  ( 0.5971128608923891301, 0.2952755905511810774, -0.1292274648535930714 ) ) ;
#454=CARTESIAN_POINT ( 'NONE',  ( -0.2362204724409442680, -0.1870078740157480879, -0.4822834645669291653 ) ) ;
#456=CARTESIAN_POINT ( 'NONE',  ( 1.364829396325459854, -0.5023911411419708095, -0.1820866141732282451 ) ) ;
#457=CARTESIAN_POINT ( 'NONE',  ( 0.4986876640419954376, -0.6046776061558809534, -0.2411417322834644161 ) ) ;
#458=CARTESIAN_POINT ( 'NONE',  ( 0.1181102362204730916, 0.2952755905511811885, 0.000000000000000000 ) ) ;
#460=CARTESIAN_POINT ( 'NONE',  ( 0.4986876640419954376, -0.5023911411419708095, -0.1820866141732282451 ) ) ;
#461=CARTESIAN_POINT ( 'NONE',  ( 0.8858267716535438430, 0.1660481256975885056, 0.3530559997133364547 ) ) ;
#462=CARTESIAN_POINT ( 'NONE',  ( -0.2427821522309703550, -0.08942795157528024563, -0.3641732283464568787 ) ) ;
#463=CARTESIAN_POINT ( 'NONE',  ( -0.7217847769028863381, -0.4281496062992124485, 0.4176697321401328655 ) ) ;
#465=CARTESIAN_POINT ( 'NONE',  ( -0.2887139107611542133, 0.2306618581243848609, 0.2411417322834645549 ) ) ;
#466=CARTESIAN_POINT ( 'NONE',  ( -1.200787401574802349, -0.5400638737290844871, 0.3530559997133364547 ) ) ;
#468=CARTESIAN_POINT ( 'NONE',  ( -0.5052493438320203589, -0.5511811023622046335, 0.09757992244046803654 ) ) ;
#469=CARTESIAN_POINT ( 'NONE',  ( 0.5643044619422579178, -0.4281496062992127816, -0.4176697321401328100 ) ) ;
#470=CARTESIAN_POINT ( 'NONE',  ( -1.364829396325458521, 0.2306618581243847221, -0.2411417322834647770 ) ) ;
#471=CARTESIAN_POINT ( 'NONE',  ( -0.5183727034120726440, 0.2952755905511811885, 0.1292274648535926551 ) ) ;
#473=FACE_OUTER_BOUND ( 'NONE', #49663, .T. ) ;
#474=CARTESIAN_POINT ( 'NONE',  ( 1.561679790026247350, -0.4281496062992124485, 0.4176697321401328655 ) ) ;
#475=CARTESIAN_POINT ( 'NONE',  ( 1.259842519685040019, -0.1870078740157480879, -0.4822834645669291653 ) ) ;
#477=CARTESIAN_POINT ( 'NONE',  ( -1.587926509186350810, 0.05413385826771626580, -0.4176697321401330321 ) ) ;
#478=CARTESIAN_POINT ( 'NONE',  ( -1.351706036745406347, 0.05413385826771626580, -0.4176697321401330321 ) ) ;
#481=ORIENTED_EDGE ( 'NONE', *, *, #70225, .T. ) ;
#482=CARTESIAN_POINT ( 'NONE',  ( 0.1181102362204730916, 0.1771653543307087630, 0.000000000000000000 ) ) ;
#486=CARTESIAN_POINT ( 'NONE',  ( 0.3674540682414705883, 0.2306618581243847221, -0.2411417322834647770 ) ) ;
#487=CARTESIAN_POINT ( 'NONE',  ( 0.5577427821522314977, -0.3162353388693409650, -0.4822834645669289433 ) ) ;
#489=CARTESIAN_POINT ( 'NONE',  ( -1.595398199321657717, 0.4829664696085547715, 0.1559797534342468595 ) ) ;
#490=CARTESIAN_POINT ( 'NONE',  ( -0.3215223097112853146, -0.08942795157528024563, -0.3641732283464568787 ) ) ;
#492=CARTESIAN_POINT ( 'NONE',  ( 0.8333333333333340365, -0.6692913385826771977, 0.1292274648535927661 ) ) ;
#493=CARTESIAN_POINT ( 'NONE',  ( 0.8858267716535438430, -0.4536011799217368745, -0.2665933059059886201 ) ) ;
#494=CARTESIAN_POINT ( 'NONE',  ( -0.4002624671916004129, -0.3162353388693405765, 0.4822834645669290543 ) ) ;
#496=CARTESIAN_POINT ( 'NONE',  ( -0.9186351706036736120, -0.6046776061558809534, -0.2411417322834644161 ) ) ;
#497=CARTESIAN_POINT ( 'NONE',  ( -1.135170603674539924, -0.5511811023622046335, 0.09757992244046803654 ) ) ;
#498=ADVANCED_FACE ( 'NONE', ( #29570 ), #56283, .F. ) ;
#499=CARTESIAN_POINT ( 'NONE',  ( -0.9055118110236215490, 0.2952755905511811885, 0.000000000000000000 ) ) ;
#501=CARTESIAN_POINT ( 'NONE',  ( 1.476377952755906442, -0.5400638737290844871, 0.3530559997133364547 ) ) ;
#505=CARTESIAN_POINT ( 'NONE',  ( 0.03937007874015833325, -0.6692913385826771977, 8.415575281601705876E-17 ) ) ;
#506=ORIENTED_EDGE ( 'NONE', *, *, #19297, .F. ) ;
#507=CARTESIAN_POINT ( 'NONE',  ( -0.8136482939632537770, -0.6046776061558807314, 0.2411417322834647770 ) ) ;
#508=CARTESIAN_POINT ( 'NONE',  ( 1.404199475065617264, -0.4281496062992124485, 0.4176697321401328655 ) ) ;
#509=CARTESIAN_POINT ( 'NONE',  ( 1.069553805774278610, -0.6692913385826771977, 0.1292274648535927661 ) ) ;
#510=CARTESIAN_POINT ( 'NONE',  ( 0.05905511811023681640, 0.1660481256975883668, -0.3530559997133364547 ) ) ;
#512=CARTESIAN_POINT ( 'NONE',  ( 0.05249343832021075018, -0.6046776061558807314, 0.2411417322834647770 ) ) ;
#514=CARTESIAN_POINT ( 'NONE',  ( -1.259842519685038686, -0.1870078740157479769, 0.4822834645669291653 ) ) ;
#515=CARTESIAN_POINT ( 'NONE',  ( -0.1115485564304453947, -0.6692913385826771977, 0.1292274648535927661 ) ) ;
#516=CARTESIAN_POINT ( 'NONE',  ( -0.2559055118110227234, -0.4536011799217367080, 0.2665933059059888421 ) ) ;
#517=CARTESIAN_POINT ( 'NONE',  ( 1.660104986876641320, -0.05778040916215522460, 0.4822834645669289988 ) ) ;
#518=CARTESIAN_POINT ( 'NONE',  ( 1.450131233595801428, -0.6692913385826773087, -0.1292274648535924053 ) ) ;
#519=CARTESIAN_POINT ( 'NONE',  ( -0.6036745406824141069, 0.2306618581243848609, 0.2411417322834645549 ) ) ;
#520=CARTESIAN_POINT ( 'NONE',  ( 0.2755905511811031494, 0.2066929133858268208, 0.000000000000000000 ) ) ;
#521=CARTESIAN_POINT ( 'NONE',  ( 1.259842519685040019, -0.1870078740157479769, 0.4822834645669291653 ) ) ;
#522=CARTESIAN_POINT ( 'NONE',  ( 0.5387615594602674918, 2.409604939980833412E-17, -0.3464511005275205946 ) ) ;
#525=CARTESIAN_POINT ( 'NONE',  ( 0.1115485564304470323, 0.2952755905511811885, 0.1292274648535926551 ) ) ;
#526=CARTESIAN_POINT ( 'NONE',  ( -0.3937007874015740483, -0.1870078740157480601, -0.3641732283464567677 ) ) ;
#527=CARTESIAN_POINT ( 'NONE',  ( 1.417322834645670104, -0.1870078740157480601, -0.3641732283464567677 ) ) ;
#530=CARTESIAN_POINT ( 'NONE',  ( 1.614173228346457378, -0.5511811023622047445, 6.969142054262312111E-17 ) ) ;
#531=CARTESIAN_POINT ( 'NONE',  ( -1.443569553805773564, 0.2306618581243847221, -0.2411417322834647770 ) ) ;
#533=CARTESIAN_POINT ( 'NONE',  ( -0.1181102362204717315, 0.2952755905511811885, 0.000000000000000000 ) ) ;
#534=CARTESIAN_POINT ( 'NONE',  ( -1.555118110236219930, -0.5400638737290845981, -0.3530559997133363437 ) ) ;
#536=CARTESIAN_POINT ( 'NONE',  ( -1.371391076115484831, 0.2952755905511810774, -0.1292274648535930714 ) ) ;
#537=CARTESIAN_POINT ( 'NONE',  ( 0.1837270341207354329, 0.2306618581243848609, 0.2411417322834645549 ) ) ;
#539=CARTESIAN_POINT ( 'NONE',  ( -1.646981627296586703, -0.08942795157527998196, 0.3641732283464567121 ) ) ;
#540=CARTESIAN_POINT ( 'NONE',  ( 0.3543307086614179147, 0.2952755905511811885, 0.000000000000000000 ) ) ;
#541=CARTESIAN_POINT ( 'NONE',  ( 0.8923884514435703741, 0.1283753931104748280, 0.1820866141732283561 ) ) ;
#542=CARTESIAN_POINT ( 'NONE',  ( -0.06561679790026180015, 0.05413385826771666132, 0.4176697321401328100 ) ) ;
#543=CARTESIAN_POINT ( 'NONE',  ( 0.6889763779527566800, -0.4536011799217367080, 0.2665933059059888421 ) ) ;
#544=CARTESIAN_POINT ( 'NONE',  ( -1.463254593175852492, 0.2952755905511811885, 0.1292274648535926551 ) ) ;
#546=CARTESIAN_POINT ( 'NONE',  ( 1.194225721784777594, 0.05413385826771666132, 0.4176697321401328100 ) ) ;
#548=CARTESIAN_POINT ( 'NONE',  ( 0.9055118110236227702, 0.2952755905511811885, 0.000000000000000000 ) ) ;
#549=CARTESIAN_POINT ( 'NONE',  ( 1.614173228346457378, 0.7794589730112001513, -0.1372047244094476148 ) ) ;
#551=CARTESIAN_POINT ( 'NONE',  ( 0.4002624671916016896, -0.2845877964562161244, -0.3641732283464567121 ) ) ;
#552=AXIS2_PLACEMENT_3D ( 'NONE', #45585, #8559, #7302 ) ;
#553=CARTESIAN_POINT ( 'NONE',  ( 0.5643044619422579178, 0.05413385826771666132, 0.4176697321401328100 ) ) ;
#554=CARTESIAN_POINT ( 'NONE',  ( 0.7349081364829403995, 0.1539470093639523085, 0.1968503937007873850 ) ) ;
#555=CARTESIAN_POINT ( 'NONE',  ( -0.9842519685039365918, -0.5511811023622047445, 6.969142054262312111E-17 ) ) ;
#556=CARTESIAN_POINT ( 'NONE',  ( -1.174540682414697335, -0.3162353388693409650, -0.4822834645669289433 ) ) ;
#557=CARTESIAN_POINT ( 'NONE',  ( 1.548556430446194954, 0.2306618581243847221, -0.2411417322834647770 ) ) ;
#558=CARTESIAN_POINT ( 'NONE',  ( -1.220472440944881054, 0.2952755905511811885, 0.000000000000000000 ) ) ;
#559=CARTESIAN_POINT ( 'NONE',  ( 0.7545931758530189937, 0.2952755905511810774, -0.1292274648535930714 ) ) ;
#560=CARTESIAN_POINT ( 'NONE',  ( -1.305774278215222184, 0.1771653543307087630, 0.09757992244046791164 ) ) ;
#561=LINE ( 'NONE', #45565, #71983 ) ;
#562=CARTESIAN_POINT ( 'NONE',  ( 0.9317585301837276734, -0.4281496062992124485, 0.4176697321401328655 ) ) ;
#564=CARTESIAN_POINT ( 'NONE',  ( -0.08874907683609993547, 8.471767977567108961E-16, -0.4445507791589058955 ) ) ;
#565=CARTESIAN_POINT ( 'NONE',  ( 1.207349081364829990, 0.2306618581243848609, 0.2411417322834645549 ) ) ;
#566=CARTESIAN_POINT ( 'NONE',  ( -0.8989501312335946848, 0.1771653543307087075, -0.09757992244046823083 ) ) ;
#567=CARTESIAN_POINT ( 'NONE',  ( 1.509186351706037543, -0.004921259842519576551, 0.3153832671262227771 ) ) ;
#568=CARTESIAN_POINT ( 'NONE',  ( -1.430446194225720724, -0.004921259842519870586, -0.3153832671262229437 ) ) ;
#569=CARTESIAN_POINT ( 'NONE',  ( -0.5118110236220466680, 0.1771653543307087630, 0.000000000000000000 ) ) ;
#570=CARTESIAN_POINT ( 'NONE',  ( -1.601049868766403650, -0.5023911411419708095, 0.1820866141732285504 ) ) ;
#571=CARTESIAN_POINT ( 'NONE',  ( 0.7611548556430451917, -0.5023911411419708095, 0.1820866141732285504 ) ) ;
#572=CARTESIAN_POINT ( 'NONE',  ( 0.6955380577427828781, -0.4281496062992124485, 0.4176697321401328655 ) ) ;
#573=CARTESIAN_POINT ( 'NONE',  ( 1.456692913385827515, 0.2952755905511811885, 0.000000000000000000 ) ) ;
#574=CARTESIAN_POINT ( 'NONE',  ( 0.03280839895013198948, -0.6692913385826773087, -0.1292274648535924053 ) ) ;
#575=CARTESIAN_POINT ( 'NONE',  ( 0.5971128608923890191, -0.5511811023622046335, 0.09757992244046803654 ) ) ;
#576=CARTESIAN_POINT ( 'NONE',  ( 1.601049868766404982, 0.2306618581243848609, 0.2411417322834645549 ) ) ;
#577=CARTESIAN_POINT ( 'NONE',  ( -1.364829396325458521, -0.6046776061558807314, 0.2411417322834647770 ) ) ;
#578=CARTESIAN_POINT ( 'NONE',  ( -0.5971128608923877978, 0.2952755905511811885, 0.1292274648535926551 ) ) ;
#581=CARTESIAN_POINT ( 'NONE',  ( 0.1115485564304467270, -0.6692913385826773087, -0.1292274648535924053 ) ) ;
#582=CARTESIAN_POINT ( 'NONE',  ( -0.2755905511811015396, -0.6692913385826771977, 8.415575281601705876E-17 ) ) ;
#583=CARTESIAN_POINT ( 'NONE',  ( 0.1771653543307093182, 0.1660481256975885056, 0.3530559997133364547 ) ) ;
#588=VECTOR ( 'NONE', #6530, 39.37007874015748143 ) ;
#590=CARTESIAN_POINT ( 'NONE',  ( -0.8267716535433065062, -0.5511811023622047445, 6.969142054262312111E-17 ) ) ;
#592=CARTESIAN_POINT ( 'NONE',  ( -1.305774278215222184, -0.6692913385826773087, -0.1292274648535924053 ) ) ;
#594=CARTESIAN_POINT ( 'NONE',  ( 0.5708661417322842269, 0.1660481256975885056, 0.3530559997133364547 ) ) ;
#595=CARTESIAN_POINT ( 'NONE',  ( 0.03937007874015806264, 0.1771653543307087630, 0.000000000000000000 ) ) ;
#596=CARTESIAN_POINT ( 'NONE',  ( 1.174540682414699111, -0.05778040916215560624, -0.4822834645669293319 ) ) ;
#597=CARTESIAN_POINT ( 'NONE',  ( 0.5511811023622054106, -0.1870078740157480879, -0.4822834645669291653 ) ) ;
#601=CARTESIAN_POINT ( 'NONE',  ( 1.141732283464567788, -0.6692913385826771977, 8.415575281601705876E-17 ) ) ;
#602=CARTESIAN_POINT ( 'NONE',  ( 0.5183727034120741983, 0.2952755905511810774, -0.1292274648535930714 ) ) ;
#603=CARTESIAN_POINT ( 'NONE',  ( 0.3280839895013130669, 0.05413385826771666132, 0.4176697321401328100 ) ) ;
#604=CARTESIAN_POINT ( 'NONE',  ( 0.9711286089238851948, 0.1283753931104748280, 0.1820866141732283561 ) ) ;
#605=CARTESIAN_POINT ( 'NONE',  ( 1.115485564304462551, -0.4281496062992127816, -0.4176697321401328100 ) ) ;
#607=CARTESIAN_POINT ( 'NONE',  ( 0.2296587926509192634, -0.05778040916215560624, -0.4822834645669293319 ) ) ;
#608=CARTESIAN_POINT ( 'NONE',  ( 1.062992125984252745, 0.2952755905511811885, 0.000000000000000000 ) ) ;
#609=CARTESIAN_POINT ( 'NONE',  ( 0.5446194225721792126, -0.3162353388693405765, 0.4822834645669290543 ) ) ;
#610=CARTESIAN_POINT ( 'NONE',  ( 1.030183727034121421, -0.08942795157527998196, 0.3641732283464567121 ) ) ;
#611=CARTESIAN_POINT ( 'NONE',  ( -1.017060367454067249, -0.3162353388693409650, -0.4822834645669289433 ) ) ;
#612=CARTESIAN_POINT ( 'NONE',  ( -1.476377952755905110, -0.5400638737290845981, -0.3530559997133363437 ) ) ;
#613=CARTESIAN_POINT ( 'NONE',  ( 1.082677165354331228, -0.5400638737290844871, 0.3530559997133364547 ) ) ;
#620=CARTESIAN_POINT ( 'NONE',  ( 1.404199475065617708, 0.05413385826771626580, -0.4176697321401330321 ) ) ;
#621=CARTESIAN_POINT ( 'NONE',  ( 0.8333333333333340365, 0.1771653543307087075, -0.09757992244046823083 ) ) ;
#624=DIRECTION ( 'NONE',  ( -1.000000000000000000, -3.050063254464715781E-16, 0.000000000000000000 ) ) ;
#626=CARTESIAN_POINT ( 'NONE',  ( -1.056430446194224881, -0.5511811023622046335, 0.09757992244046803654 ) ) ;
#627=CARTESIAN_POINT ( 'NONE',  ( -1.686351706036744558, 0.1771653543307087075, -0.09757992244046823083 ) ) ;
#628=CARTESIAN_POINT ( 'NONE',  ( -1.607611548556429737, 0.2952755905511810774, -0.1292274648535930714 ) ) ;
#629=CARTESIAN_POINT ( 'NONE',  ( -0.1377952755905504645, 0.1660481256975885056, 0.3530559997133364547 ) ) ;
#630=CARTESIAN_POINT ( 'NONE',  ( 1.496062992125984703, -0.1870078740157480879, -0.4822834645669291653 ) ) ;
#631=ORIENTED_EDGE ( 'NONE', *, *, #1460, .F. ) ;
#637=CARTESIAN_POINT ( 'NONE',  ( -1.049868766404198794, -0.5023911411419708095, 0.1820866141732285504 ) ) ;
#638=CARTESIAN_POINT ( 'NONE',  ( -1.443569553805773564, 0.2306618581243847221, -0.2411417322834647770 ) ) ;
#639=CARTESIAN_POINT ( 'NONE',  ( 0.4724409448818904789, -0.1870078740157480879, -0.4822834645669291653 ) ) ;
#642=FACE_OUTER_BOUND ( 'NONE', #22838, .T. ) ;
#643=CARTESIAN_POINT ( 'NONE',  ( 1.305774278215223960, -0.6692913385826771977, 0.1292274648535927661 ) ) ;
#644=CARTESIAN_POINT ( 'NONE',  ( -1.620734908136482577, -0.6692913385826773087, -0.1292274648535924053 ) ) ;
#646=CARTESIAN_POINT ( 'NONE',  ( -0.4330708661417315697, 0.1771653543307087630, 0.000000000000000000 ) ) ;
#647=CARTESIAN_POINT ( 'NONE',  ( -1.463254593175852492, 0.1771653543307087630, 0.09757992244046791164 ) ) ;
#650=CARTESIAN_POINT ( 'NONE',  ( -0.3674540682414689785, 0.1283753931104748280, 0.1820866141732283561 ) ) ;
#651=CARTESIAN_POINT ( 'NONE',  ( 0.1574803149606306130, -0.1870078740157479769, 0.3641732283464567677 ) ) ;
#652=CARTESIAN_POINT ( 'NONE',  ( 0.2493438320209980519, -0.4281496062992127816, -0.4176697321401328100 ) ) ;
#653=CARTESIAN_POINT ( 'NONE',  ( -1.194225721784776262, -0.3690944881889763329, 0.3153832671262228327 ) ) ;
#655=CARTESIAN_POINT ( 'NONE',  ( 0.6824146981627303710, 0.2306618581243847221, -0.2411417322834647770 ) ) ;
#657=CARTESIAN_POINT ( 'NONE',  ( -1.286089238845143479, 0.2306618581243847221, -0.2411417322834647770 ) ) ;
#659=CARTESIAN_POINT ( 'NONE',  ( -0.3280839895013117347, -0.4281496062992124485, 0.4176697321401328655 ) ) ;
#660=CARTESIAN_POINT ( 'NONE',  ( 0.1115485564304467270, -0.5511811023622048555, -0.09757992244046775898 ) ) ;
#661=CARTESIAN_POINT ( 'NONE',  ( -0.9711286089238838626, 0.2306618581243847221, -0.2411417322834647770 ) ) ;
#662=CARTESIAN_POINT ( 'NONE',  ( 0.8136482939632553313, -0.5023911411419708095, -0.1820866141732282451 ) ) ;
#664=CARTESIAN_POINT ( 'NONE',  ( -0.3412073490813641308, -0.5023911411419708095, 0.1820866141732285504 ) ) ;
#665=CARTESIAN_POINT ( 'NONE',  ( -0.4790026246719154557, -0.3162353388693405765, 0.4822834645669290543 ) ) ;
#666=CARTESIAN_POINT ( 'NONE',  ( -1.384514435695537005, -0.6692913385826773087, -0.1292274648535924053 ) ) ;
#667=CARTESIAN_POINT ( 'NONE',  ( -0.4043999638110875594, 5.961526036605507449E-15, -0.4118484887281962381 ) ) ;
#668=CARTESIAN_POINT ( 'NONE',  ( 1.305774278215223960, -0.5511811023622046335, 0.09757992244046803654 ) ) ;
#669=CARTESIAN_POINT ( 'NONE',  ( -1.594488188976377119, 0.1660481256975883668, -0.3530559997133364547 ) ) ;
#670=CARTESIAN_POINT ( 'NONE',  ( -1.417322834645668772, -0.1870078740157479769, 0.4822834645669291653 ) ) ;
#674=CARTESIAN_POINT ( 'NONE',  ( -0.7874015748031489847, -0.1870078740157480601, -0.3641732283464567677 ) ) ;
#675=CARTESIAN_POINT ( 'NONE',  ( 0.6036745406824153282, -0.6046776061558807314, 0.2411417322834647770 ) ) ;
#676=CARTESIAN_POINT ( 'NONE',  ( -0.9317585301837263412, -0.004921259842519576551, 0.3153832671262227771 ) ) ;
#678=CARTESIAN_POINT ( 'NONE',  ( -0.8530183727034112984, -0.4281496062992127816, -0.4176697321401328100 ) ) ;
#679=CARTESIAN_POINT ( 'NONE',  ( 0.9842519685039378130, -0.6692913385826771977, 8.415575281601705876E-17 ) ) ;
#680=CARTESIAN_POINT ( 'NONE',  ( 0.3937007874015754361, -0.1870078740157479769, 0.4822834645669291653 ) ) ;
#681=CARTESIAN_POINT ( 'NONE',  ( -1.351706036745406347, -0.004921259842519870586, -0.3153832671262229437 ) ) ;
#686=CARTESIAN_POINT ( 'NONE',  ( 0.8398950131233602345, -0.5023911411419708095, 0.1820866141732285504 ) ) ;
#687=CARTESIAN_POINT ( 'NONE',  ( 0.4133858267716541968, -0.4536011799217368745, -0.2665933059059886201 ) ) ;
#688=CARTESIAN_POINT ( 'NONE',  ( -0.04593175853018302557, -0.6692913385826773087, -0.1292274648535924053 ) ) ;
#689=CARTESIAN_POINT ( 'NONE',  ( 1.482939632545932307, 0.05413385826771626580, -0.4176697321401330321 ) ) ;
#691=CARTESIAN_POINT ( 'NONE',  ( 0.5446194225721792126, -0.2845877964562159024, 0.3641732283464567677 ) ) ;
#692=CARTESIAN_POINT ( 'NONE',  ( -0.9055118110236215490, -0.6692913385826771977, 8.415575281601705876E-17 ) ) ;
#693=CARTESIAN_POINT ( 'NONE',  ( -1.043307086614172041, -0.5400638737290844871, 0.3530559997133364547 ) ) ;
#694=CARTESIAN_POINT ( 'NONE',  ( 0.9908136482939640111, -0.6692913385826771977, 0.1292274648535927661 ) ) ;
#696=CARTESIAN_POINT ( 'NONE',  ( -0.7742782152230965886, 0.05413385826771666132, 0.4176697321401328100 ) ) ;
#699=CARTESIAN_POINT ( 'NONE',  ( -1.095800524934382292, -0.05778040916215522460, 0.4822834645669289988 ) ) ;
#700=CARTESIAN_POINT ( 'NONE',  ( -0.6692913385826764205, 0.2952755905511811885, 0.000000000000000000 ) ) ;
#701=CARTESIAN_POINT ( 'NONE',  ( -0.8792650918635160906, -0.3690944881889763329, 0.3153832671262228327 ) ) ;
#702=CARTESIAN_POINT ( 'NONE',  ( -0.9448818897637790704, -0.1870078740157480879, -0.4822834645669291653 ) ) ;
#705=CARTESIAN_POINT ( 'NONE',  ( 1.568241469816273659, -0.05778040916215560624, -0.4822834645669293319 ) ) ;
#706=CARTESIAN_POINT ( 'NONE',  ( -1.128608923884513837, -0.6046776061558807314, 0.2411417322834647770 ) ) ;
#707=CARTESIAN_POINT ( 'NONE',  ( 0.3412073490813655186, 0.2306618581243848609, 0.2411417322834645549 ) ) ;
#708=CARTESIAN_POINT ( 'NONE',  ( -0.8398950131233585692, 0.2306618581243848609, 0.2411417322834645549 ) ) ;
#709=CARTESIAN_POINT ( 'NONE',  ( 0.7939632545931766261, -0.05778040916215522460, 0.4822834645669289988 ) ) ;
#711=CARTESIAN_POINT ( 'NONE',  ( -0.8530183727034112984, -0.004921259842519576551, 0.3153832671262227771 ) ) ;
#715=CARTESIAN_POINT ( 'NONE',  ( -1.640419947506561060, -0.3690944881889765550, -0.3153832671262227771 ) ) ;
#717=CARTESIAN_POINT ( 'NONE',  ( -1.036745406824146176, 0.05413385826771626580, -0.4176697321401330321 ) ) ;
#718=CARTESIAN_POINT ( 'NONE',  ( -1.122047244094487306, 0.1660481256975883668, -0.3530559997133364547 ) ) ;
#720=CARTESIAN_POINT ( 'NONE',  ( -1.286089238845143479, -0.6046776061558807314, 0.2411417322834647770 ) ) ;
#721=CARTESIAN_POINT ( 'NONE',  ( -1.279527559055116948, -0.5400638737290844871, 0.3530559997133364547 ) ) ;
#722=CARTESIAN_POINT ( 'NONE',  ( -1.594488188976377119, 0.1660481256975883668, -0.3530559997133364547 ) ) ;
#724=CARTESIAN_POINT ( 'NONE',  ( -0.7426113562972000981, 2.362204724409448620, -0.5309055118110235227 ) ) ;
#726=CARTESIAN_POINT ( 'NONE',  ( 0.2952755905511819101, 0.07958543189024071263, -0.2665933059059888421 ) ) ;
#729=CARTESIAN_POINT ( 'NONE',  ( -0.1574803149606292529, -0.1870078740157479769, 0.3641732283464567677 ) ) ;
#730=CARTESIAN_POINT ( 'NONE',  ( -0.9776902887139098386, 0.2952755905511810774, -0.1292274648535930714 ) ) ;
#731=CARTESIAN_POINT ( 'NONE',  ( 1.220472440944882386, -0.6692913385826771977, 8.415575281601705876E-17 ) ) ;
#732=CARTESIAN_POINT ( 'NONE',  ( -0.3215223097112853146, -0.05778040916215560624, -0.4822834645669293319 ) ) ;
#734=EDGE_LOOP ( 'NONE', ( #77385, #67273, #78260, #71101 ) ) ;
#737=CARTESIAN_POINT ( 'NONE',  ( -0.7874015748031489847, -0.1870078740157480879, -0.4822834645669291653 ) ) ;
#738=CARTESIAN_POINT ( 'NONE',  ( 1.246719160104987623, -0.4281496062992124485, 0.4176697321401328655 ) ) ;
#744=CARTESIAN_POINT ( 'NONE',  ( -0.4461942257217840213, -0.6046776061558809534, -0.2411417322834644161 ) ) ;
#745=CARTESIAN_POINT ( 'NONE',  ( -1.338582677165353729, -0.1870078740157479769, 0.3641732283464567677 ) ) ;
#746=CARTESIAN_POINT ( 'NONE',  ( -0.7677165354330699465, 0.1660481256975885056, 0.3530559997133364547 ) ) ;
#748=CARTESIAN_POINT ( 'NONE',  ( -1.148293963254592542, -0.6692913385826773087, -0.1292274648535924053 ) ) ;
#750=CARTESIAN_POINT ( 'NONE',  ( -1.049868766404198794, 0.2306618581243847221, -0.2411417322834647770 ) ) ;
#751=CARTESIAN_POINT ( 'NONE',  ( -0.1968503937007867743, -0.6692913385826771977, 8.415575281601705876E-17 ) ) ;
#753=CARTESIAN_POINT ( 'NONE',  ( 0.9317585301837276734, -0.3690944881889763329, 0.3153832671262228327 ) ) ;
#755=CARTESIAN_POINT ( 'NONE',  ( 0.6430446194225729606, -0.3690944881889765550, -0.3153832671262227771 ) ) ;
#756=CARTESIAN_POINT ( 'NONE',  ( 1.397637795275591177, -0.4536011799217367080, 0.2665933059059888421 ) ) ;
#757=CARTESIAN_POINT ( 'NONE',  ( 1.469816272965879911, 0.2306618581243847221, -0.2411417322834647770 ) ) ;
#758=CARTESIAN_POINT ( 'NONE',  ( 0.2296587926509192634, -0.2845877964562159024, 0.3641732283464567677 ) ) ;
#760=CARTESIAN_POINT ( 'NONE',  ( -0.9908136482939626788, 0.2952755905511811885, 0.1292274648535926551 ) ) ;
#761=CARTESIAN_POINT ( 'NONE',  ( 1.391076115485564868, -0.6046776061558807314, 0.2411417322834647770 ) ) ;
#763=CARTESIAN_POINT ( 'NONE',  ( -0.5577427821522301654, -0.2845877964562159024, 0.3641732283464567677 ) ) ;
#764=CARTESIAN_POINT ( 'NONE',  ( 1.614173228346456712, 2.401574803149606474, -0.1372047244094476703 ) ) ;
#765=CARTESIAN_POINT ( 'NONE',  ( 0.4461942257217856311, 0.2306618581243847221, -0.2411417322834647770 ) ) ;
#767=CARTESIAN_POINT ( 'NONE',  ( 1.082677165354331228, -0.4536011799217367080, 0.2665933059059888421 ) ) ;
#768=CARTESIAN_POINT ( 'NONE',  ( -0.02624671916010428221, -0.5023911411419708095, 0.1820866141732285504 ) ) ;
#769=CARTESIAN_POINT ( 'NONE',  ( -0.4461942257217840213, -0.6046776061558809534, -0.2411417322834644161 ) ) ;
#770=CARTESIAN_POINT ( 'NONE',  ( -1.272965879265091305, -0.4281496062992124485, 0.4176697321401328655 ) ) ;
#771=CARTESIAN_POINT ( 'NONE',  ( -0.7939632545931750718, -0.08942795157528024563, -0.3641732283464568787 ) ) ;
#773=CARTESIAN_POINT ( 'NONE',  ( 0.7414698162729663755, 0.2952755905511811885, 0.1292274648535926551 ) ) ;
#774=CARTESIAN_POINT ( 'NONE',  ( -0.7939632545931750718, -0.05778040916215560624, -0.4822834645669293319 ) ) ;
#777=CARTESIAN_POINT ( 'NONE',  ( 0.3346456692913390985, 0.07958543189024085140, 0.2665933059059887866 ) ) ;
#778=CARTESIAN_POINT ( 'NONE',  ( -0.8661417322834640276, -0.1870078740157479769, 0.4822834645669291653 ) ) ;
#780=CARTESIAN_POINT ( 'NONE',  ( -1.272965879265091305, 0.05413385826771626580, -0.4176697321401330321 ) ) ;
#781=CARTESIAN_POINT ( 'NONE',  ( -1.108923884514435132, -0.08942795157528024563, -0.3641732283464568787 ) ) ;
#782=CARTESIAN_POINT ( 'NONE',  ( 1.646981627296588035, -0.3162353388693405765, 0.4822834645669290543 ) ) ;
#784=CARTESIAN_POINT ( 'NONE',  ( -1.089238845144356427, -0.3690944881889765550, -0.3153832671262227771 ) ) ;
#785=CARTESIAN_POINT ( 'NONE',  ( -1.541994750656167090, 0.1771653543307087630, 0.09757992244046791164 ) ) ;
#786=CARTESIAN_POINT ( 'NONE',  ( 1.095800524934383846, -0.3162353388693405765, 0.4822834645669290543 ) ) ;
#787=CARTESIAN_POINT ( 'NONE',  ( 0.01193304242178773455, 1.795490347638496118E-16, 0.3627985898453511826 ) ) ;
#789=ORIENTED_EDGE ( 'NONE', *, *, #46286, .F. ) ;
#792=CARTESIAN_POINT ( 'NONE',  ( -1.620734908136482577, -0.6692913385826773087, -0.1292274648535924053 ) ) ;
#793=CARTESIAN_POINT ( 'NONE',  ( -1.181102362204723644, -0.1870078740157480879, -0.4822834645669291653 ) ) ;
#794=CARTESIAN_POINT ( 'NONE',  ( 1.181102362204724976, -0.1870078740157480879, -0.4822834645669291653 ) ) ;
#796=CARTESIAN_POINT ( 'NONE',  ( 1.692913385826772421, 0.1771653543307087630, 0.000000000000000000 ) ) ;
#797=CARTESIAN_POINT ( 'NONE',  ( 0.4461942257217856311, 0.2306618581243847221, -0.2411417322834647770 ) ) ;
#798=CARTESIAN_POINT ( 'NONE',  ( -0.04593175853018302557, 0.2952755905511811885, 0.1292274648535926551 ) ) ;
#801=CARTESIAN_POINT ( 'NONE',  ( 0.7874015748031503170, -0.1870078740157479769, 0.3641732283464567677 ) ) ;
#806=CARTESIAN_POINT ( 'NONE',  ( 0.07217847769028949700, -0.05778040916215560624, -0.4822834645669293319 ) ) ;
#807=CARTESIAN_POINT ( 'NONE',  ( 1.148293963254593653, 0.2952755905511810774, -0.1292274648535930714 ) ) ;
#808=CARTESIAN_POINT ( 'NONE',  ( 0.6889763779527566800, -0.5400638737290844871, 0.3530559997133364547 ) ) ;
#809=CARTESIAN_POINT ( 'NONE',  ( 1.082677165354331228, 0.1660481256975883668, -0.3530559997133364547 ) ) ;
#810=CARTESIAN_POINT ( 'NONE',  ( 1.594488188976378673, 0.1660481256975885056, 0.3530559997133364547 ) ) ;
#811=CARTESIAN_POINT ( 'NONE',  ( -0.6758530183727028406, 0.2952755905511811885, 0.1292274648535926551 ) ) ;
#812=CARTESIAN_POINT ( 'NONE',  ( 0.08530183727034192087, -0.3162353388693409650, -0.4822834645669289433 ) ) ;
#813=CARTESIAN_POINT ( 'NONE',  ( 1.574803149606299746, -0.1870078740157479769, 0.4822834645669291653 ) ) ;
#814=CARTESIAN_POINT ( 'NONE',  ( 1.227034120734908917, -0.6692913385826771977, 0.1292274648535927661 ) ) ;
#815=EDGE_CURVE ( 'NONE', #64851, #29791, #21395, .T. ) ;
#816=CARTESIAN_POINT ( 'NONE',  ( 1.122047244094488860, -0.5400638737290845981, -0.3530559997133363437 ) ) ;
#817=CARTESIAN_POINT ( 'NONE',  ( -0.1968503937007867743, -0.6692913385826771977, 8.415575281601705876E-17 ) ) ;
#819=CARTESIAN_POINT ( 'NONE',  ( 0.6364829396325465405, -0.2845877964562161244, -0.3641732283464567121 ) ) ;
#820=VERTEX_POINT ( 'NONE', #82802 ) ;
#823=ORIENTED_EDGE ( 'NONE', *, *, #81853, .F. ) ;
#824=CARTESIAN_POINT ( 'NONE',  ( -0.4396325459317579898, 0.1771653543307087630, 0.09757992244046791164 ) ) ;
#826=VECTOR ( 'NONE', #11111, 39.37007874015748143 ) ;
#827=CARTESIAN_POINT ( 'NONE',  ( 0.02624671916010564918, -0.6046776061558809534, -0.2411417322834644161 ) ) ;
#829=CARTESIAN_POINT ( 'NONE',  ( -0.01968503937007793844, -0.5400638737290844871, 0.3530559997133364547 ) ) ;
#830=CARTESIAN_POINT ( 'NONE',  ( -0.1181102362204717315, 0.2952755905511811885, 0.000000000000000000 ) ) ;
#831=CARTESIAN_POINT ( 'NONE',  ( -0.8989501312335946848, 0.2952755905511810774, -0.1292274648535930714 ) ) ;
#832=ADVANCED_FACE ( 'NONE', ( #63850 ), #17200, .F. ) ;
#833=CARTESIAN_POINT ( 'NONE',  ( 1.194225721784777594, -0.004921259842519576551, 0.3153832671262227771 ) ) ;
#834=CARTESIAN_POINT ( 'NONE',  ( -1.463254593175852492, 0.2952755905511811885, 0.1292274648535926551 ) ) ;
#836=CARTESIAN_POINT ( 'NONE',  ( 0.8858267716535438430, -0.4536011799217368745, -0.2665933059059886201 ) ) ;
#837=CARTESIAN_POINT ( 'NONE',  ( 0.4921259842519691285, -0.5400638737290845981, -0.3530559997133363437 ) ) ;
#838=CARTESIAN_POINT ( 'NONE',  ( 0.9317585301837276734, 0.05413385826771626580, -0.4176697321401330321 ) ) ;
#840=CARTESIAN_POINT ( 'NONE',  ( -1.587926509186350810, -0.4281496062992124485, 0.4176697321401328655 ) ) ;
#843=CARTESIAN_POINT ( 'NONE',  ( 0.03280839895013198948, 0.2952755905511811885, 0.1292274648535926551 ) ) ;
#847=CARTESIAN_POINT ( 'NONE',  ( -1.122047244094487306, 0.07958543189024071263, -0.2665933059059888421 ) ) ;
#848=CARTESIAN_POINT ( 'NONE',  ( 1.128608923884514947, 0.2306618581243848609, 0.2411417322834645549 ) ) ;
#849=CARTESIAN_POINT ( 'NONE',  ( 1.240157480314961314, 0.1660481256975883668, -0.3530559997133364547 ) ) ;
#850=CARTESIAN_POINT ( 'NONE',  ( -0.4265091863517051496, -0.5511811023622046335, 0.09757992244046803654 ) ) ;
#851=CARTESIAN_POINT ( 'NONE',  ( 0.5905511811023629321, -0.6692913385826771977, 8.415575281601705876E-17 ) ) ;
#853=CARTESIAN_POINT ( 'NONE',  ( 0.2559055118110243332, 0.07958543189024085140, 0.2665933059059887866 ) ) ;
#854=CARTESIAN_POINT ( 'NONE',  ( -0.1509186351706028884, -0.05778040916215522460, 0.4822834645669289988 ) ) ;
#856=CARTESIAN_POINT ( 'NONE',  ( -1.017060367454067249, -0.3162353388693409650, -0.4822834645669289433 ) ) ;
#857=CARTESIAN_POINT ( 'NONE',  ( 0.5183727034120741983, 0.1771653543307087075, -0.09757992244046823083 ) ) ;
#859=CARTESIAN_POINT ( 'NONE',  ( -0.8136482939632537770, -0.6046776061558807314, 0.2411417322834647770 ) ) ;
#860=CARTESIAN_POINT ( 'NONE',  ( -0.3608923884514428360, 0.1771653543307087630, 0.09757992244046791164 ) ) ;
#861=CARTESIAN_POINT ( 'NONE',  ( -1.363814626685861287, 0.1354692512615926214, 0.3875633260700430682 ) ) ;
#862=CARTESIAN_POINT ( 'NONE',  ( -0.5774278215223089816, 0.2306618581243847221, -0.2411417322834647770 ) ) ;
#863=CARTESIAN_POINT ( 'NONE',  ( -0.3149606299212590610, -0.1870078740157480879, -0.4822834645669291653 ) ) ;
#864=CARTESIAN_POINT ( 'NONE',  ( 0.3674540682414705883, 0.1283753931104746893, -0.1820866141732285504 ) ) ;
#866=CARTESIAN_POINT ( 'NONE',  ( 0.08530183727034192087, -0.05778040916215522460, 0.4822834645669289988 ) ) ;
#868=CARTESIAN_POINT ( 'NONE',  ( -1.594488188976377563, -0.4536011799217367080, 0.2665933059059888421 ) ) ;
#869=CARTESIAN_POINT ( 'NONE',  ( 0.6299212598425204535, -0.1870078740157480601, -0.3641732283464567677 ) ) ;
#870=CARTESIAN_POINT ( 'NONE',  ( 1.568241469816273437, -0.3162353388693405765, 0.4822834645669290543 ) ) ;
#871=CARTESIAN_POINT ( 'NONE',  ( -0.6233595800524928121, -0.08942795157527998196, 0.3641732283464567121 ) ) ;
#872=CARTESIAN_POINT ( 'NONE',  ( -1.108923884514435132, -0.2845877964562159024, 0.3641732283464567677 ) ) ;
#873=CARTESIAN_POINT ( 'NONE',  ( -0.5511811023622038563, -0.1870078740157479769, 0.4822834645669291653 ) ) ;
#874=CARTESIAN_POINT ( 'NONE',  ( -0.2624671916010490880, 0.2306618581243847221, -0.2411417322834647770 ) ) ;
#875=CARTESIAN_POINT ( 'NONE',  ( 0.5314960629921267055, -0.4536011799217367080, 0.2665933059059888421 ) ) ;
#877=CARTESIAN_POINT ( 'NONE',  ( 1.082677165354331228, -0.4536011799217367080, 0.2665933059059888421 ) ) ;
#878=CARTESIAN_POINT ( 'NONE',  ( 0.1246719160104994284, 0.2952755905511810774, -0.1292274648535930714 ) ) ;
#880=CARTESIAN_POINT ( 'NONE',  ( -0.3805774278215216522, -0.4281496062992127816, -0.4176697321401328100 ) ) ;
#883=CARTESIAN_POINT ( 'NONE',  ( 1.358267716535433323, -0.4536011799217368745, -0.2665933059059886201 ) ) ;
#885=CARTESIAN_POINT ( 'NONE',  ( 0.6299212598425204535, -0.1870078740157480879, -0.4822834645669291653 ) ) ;
#887=CARTESIAN_POINT ( 'NONE',  ( 0.1640419947506569498, -0.3162353388693409650, -0.4822834645669289433 ) ) ;
#888=CARTESIAN_POINT ( 'NONE',  ( 0.1377952755905518800, 0.07958543189024071263, -0.2665933059059888421 ) ) ;
#889=CARTESIAN_POINT ( 'NONE',  ( 0.7086614173228353852, -0.1870078740157479769, 0.4822834645669291653 ) ) ;
#891=CARTESIAN_POINT ( 'NONE',  ( -0.4790026246719154557, -0.2845877964562159024, 0.3641732283464567677 ) ) ;
#892=CARTESIAN_POINT ( 'NONE',  ( -0.6955380577427815458, 0.05413385826771666132, 0.4176697321401328100 ) ) ;
#894=CARTESIAN_POINT ( 'NONE',  ( -0.2099737532808391705, -0.6046776061558809534, -0.2411417322834644161 ) ) ;
#896=CARTESIAN_POINT ( 'NONE',  ( -1.003937007874014853, 0.1660481256975885056, 0.3530559997133364547 ) ) ;
#897=CARTESIAN_POINT ( 'NONE',  ( -0.5118110236220466680, -0.5511811023622047445, 6.969142054262312111E-17 ) ) ;
#898=CARTESIAN_POINT ( 'NONE',  ( 0.09186351706036799403, -0.4281496062992127816, -0.4176697321401328100 ) ) ;
#899=CARTESIAN_POINT ( 'NONE',  ( -1.102362204724408601, -0.1870078740157479769, 0.4822834645669291653 ) ) ;
#900=CARTESIAN_POINT ( 'NONE',  ( -0.8267716535433065062, 0.2952755905511811885, 0.000000000000000000 ) ) ;
#902=CARTESIAN_POINT ( 'NONE',  ( 1.089238845144357759, 0.05413385826771626580, -0.4176697321401330321 ) ) ;
#903=CARTESIAN_POINT ( 'NONE',  ( 1.056430446194226436, -0.6692913385826773087, -0.1292274648535924053 ) ) ;
#904=CARTESIAN_POINT ( 'NONE',  ( 1.325459317585302665, -0.4281496062992124485, 0.4176697321401328655 ) ) ;
#906=CARTESIAN_POINT ( 'NONE',  ( -1.555118110236219930, -0.5400638737290845981, -0.3530559997133363437 ) ) ;
#907=VECTOR ( 'NONE', #66466, 39.37007874015748143 ) ;
#908=CARTESIAN_POINT ( 'NONE',  ( -1.240157480314959759, 0.1660481256975885056, 0.3530559997133364547 ) ) ;
#912=CARTESIAN_POINT ( 'NONE',  ( 0.08530183727034192087, -0.08942795157527998196, 0.3641732283464567121 ) ) ;
#915=CARTESIAN_POINT ( 'NONE',  ( 0.2427821522309716595, -0.3162353388693409650, -0.4822834645669289433 ) ) ;
#916=CARTESIAN_POINT ( 'NONE',  ( 0.2755905511811031494, -0.6692913385826771977, 8.415575281601705876E-17 ) ) ;
#918=CARTESIAN_POINT ( 'NONE',  ( -0.5400834452262261998, -4.992347309556208597E-15, 0.3954985857520076920 ) ) ;
#919=CARTESIAN_POINT ( 'NONE',  ( -0.9645669291338575535, 0.07958543189024071263, -0.2665933059059888421 ) ) ;
#921=CARTESIAN_POINT ( 'NONE',  ( 0.6561679790026253567, -0.6046776061558809534, -0.2411417322834644161 ) ) ;
#922=CARTESIAN_POINT ( 'NONE',  ( 0.9645669291338588858, 0.07958543189024085140, 0.2665933059059887866 ) ) ;
#923=CARTESIAN_POINT ( 'NONE',  ( -0.4068241469816264999, -0.4281496062992124485, 0.4176697321401328655 ) ) ;
#925=CARTESIAN_POINT ( 'NONE',  ( -0.9120734908136475250, -0.6692913385826773087, -0.1292274648535924053 ) ) ;
#927=CARTESIAN_POINT ( 'NONE',  ( 1.299212598425197429, -0.6692913385826771977, 8.415575281601705876E-17 ) ) ;
#928=CARTESIAN_POINT ( 'NONE',  ( 1.594488188976378673, -0.4536011799217368745, -0.2665933059059886201 ) ) ;
#931=CARTESIAN_POINT ( 'NONE',  ( 0.03280839895013198948, -0.6692913385826773087, -0.1292274648535924053 ) ) ;
#933=CARTESIAN_POINT ( 'NONE',  ( -0.6955380577427815458, -0.4281496062992127816, -0.4176697321401328100 ) ) ;
#934=CARTESIAN_POINT ( 'NONE',  ( 1.496062992125984703, -0.1870078740157480879, -0.4822834645669291653 ) ) ;
#935=CARTESIAN_POINT ( 'NONE',  ( 1.423884514435696191, -0.05778040916215522460, 0.4822834645669289988 ) ) ;
#936=CARTESIAN_POINT ( 'NONE',  ( 0.2755905511811031494, -0.6692913385826771977, 8.415575281601705876E-17 ) ) ;
#937=CARTESIAN_POINT ( 'NONE',  ( -0.5774278215223089816, -0.6046776061558807314, 0.2411417322834647770 ) ) ;
#939=CARTESIAN_POINT ( 'NONE',  ( -1.062992125984250968, 0.2952755905511811885, 0.000000000000000000 ) ) ;
#940=CARTESIAN_POINT ( 'NONE',  ( -0.1377952755905504645, -0.5400638737290845981, -0.3530559997133363437 ) ) ;
#941=CARTESIAN_POINT ( 'NONE',  ( -0.2821522309711278487, -0.5511811023622048555, -0.09757992244046775898 ) ) ;
#942=CARTESIAN_POINT ( 'NONE',  ( 1.568241469816273659, -0.05778040916215560624, -0.4822834645669293319 ) ) ;
#943=CARTESIAN_POINT ( 'NONE',  ( 1.292650918635171564, -0.6692913385826773087, -0.1292274648535924053 ) ) ;
#944=CARTESIAN_POINT ( 'NONE',  ( -0.4986876640419942164, -0.6046776061558807314, 0.2411417322834647770 ) ) ;
#947=CARTESIAN_POINT ( 'NONE',  ( 1.056430446194226436, -0.6692913385826773087, -0.1292274648535924053 ) ) ;
#949=VERTEX_POINT ( 'NONE', #43649 ) ;
#951=CARTESIAN_POINT ( 'NONE',  ( 0.4855643044619430415, -0.4281496062992127816, -0.4176697321401328100 ) ) ;
#952=CARTESIAN_POINT ( 'NONE',  ( -0.3346456692913377662, -0.4536011799217367080, 0.2665933059059888421 ) ) ;
#954=CARTESIAN_POINT ( 'NONE',  ( 1.338582677165355062, -0.1870078740157479769, 0.3641732283464567677 ) ) ;
#955=CARTESIAN_POINT ( 'NONE',  ( -1.614173228346457378, 0.7794589730111965986, 0.1372047244094476981 ) ) ;
#957=CARTESIAN_POINT ( 'NONE',  ( 1.522309711286089939, 0.1283753931104748280, 0.1820866141732283561 ) ) ;
#958=CARTESIAN_POINT ( 'NONE',  ( 1.108923884514436242, -0.05778040916215522460, 0.4822834645669289988 ) ) ;
#961=CARTESIAN_POINT ( 'NONE',  ( 0.1443569553805781891, -0.4281496062992124485, 0.4176697321401328655 ) ) ;
#963=CARTESIAN_POINT ( 'NONE',  ( -1.502624671916009680, -0.05778040916215560624, -0.4822834645669293319 ) ) ;
#964=CARTESIAN_POINT ( 'NONE',  ( -0.1640419947506555343, -0.3162353388693405765, 0.4822834645669290543 ) ) ;
#966=CARTESIAN_POINT ( 'NONE',  ( -1.450131233595799651, 0.1771653543307087075, -0.09757992244046823083 ) ) ;
#967=CARTESIAN_POINT ( 'NONE',  ( 0.6955380577427828781, 0.05413385826771626580, -0.4176697321401330321 ) ) ;
#968=CARTESIAN_POINT ( 'NONE',  ( 0.8989501312335964611, 0.1771653543307087630, 0.09757992244046791164 ) ) ;
#970=CARTESIAN_POINT ( 'NONE',  ( 0.8727034120734913358, -0.08942795157527998196, 0.3641732283464567121 ) ) ;
#971=CARTESIAN_POINT ( 'NONE',  ( -1.391076115485563314, -0.6046776061558809534, -0.2411417322834644161 ) ) ;
#973=CARTESIAN_POINT ( 'NONE',  ( 1.187664041994751285, -0.05778040916215522460, 0.4822834645669289988 ) ) ;
#975=CARTESIAN_POINT ( 'NONE',  ( 0.7349081364829403995, 0.2306618581243848609, 0.2411417322834645549 ) ) ;
#976=CARTESIAN_POINT ( 'NONE',  ( 0.8858267716535438430, 0.1660481256975885056, 0.3530559997133364547 ) ) ;
#977=CARTESIAN_POINT ( 'NONE',  ( -0.3809280630633181675, 0.004960608223778821026, 0.3437734562760189072 ) ) ;
#978=CARTESIAN_POINT ( 'NONE',  ( 0.4330708661417329575, -0.5511811023622047445, 6.969142054262312111E-17 ) ) ;
#979=CARTESIAN_POINT ( 'NONE',  ( 0.4330708661417329575, 0.2952755905511811885, 0.000000000000000000 ) ) ;
#980=CARTESIAN_POINT ( 'NONE',  ( -0.7939632545931754048, -0.2845877964562159024, 0.3641732283464567677 ) ) ;
#981=CARTESIAN_POINT ( 'NONE',  ( -0.9120734908136475250, 0.2952755905511811885, 0.1292274648535926551 ) ) ;
#982=CARTESIAN_POINT ( 'NONE',  ( -1.706036745406823485, 0.2306618581243848609, 0.2411417322834645549 ) ) ;
#983=CARTESIAN_POINT ( 'NONE',  ( 0.8661417322834653598, -0.1870078740157479769, 0.4822834645669291653 ) ) ;
#985=CARTESIAN_POINT ( 'NONE',  ( -1.653543307086613234, -0.1870078740157479769, 0.3641732283464567677 ) ) ;
#987=CARTESIAN_POINT ( 'NONE',  ( 1.108923884514436242, -0.05778040916215522460, 0.4822834645669289988 ) ) ;
#990=CARTESIAN_POINT ( 'NONE',  ( 1.502624671916010790, -0.05778040916215522460, 0.4822834645669289988 ) ) ;
#991=CARTESIAN_POINT ( 'NONE',  ( -1.318897637795274802, -0.4536011799217368745, -0.2665933059059886201 ) ) ;
#992=CARTESIAN_POINT ( 'NONE',  ( 1.122047244094488860, -0.4536011799217368745, -0.2665933059059886201 ) ) ;
#993=CARTESIAN_POINT ( 'NONE',  ( -1.476377952755905110, 0.07958543189024085140, 0.2665933059059887866 ) ) ;
#994=CARTESIAN_POINT ( 'NONE',  ( -0.5905511811023613777, -0.5511811023622047445, 6.969142054262312111E-17 ) ) ;
#996=CARTESIAN_POINT ( 'NONE',  ( -1.686351706036744558, 0.1771653543307087075, -0.09757992244046823083 ) ) ;
#997=CARTESIAN_POINT ( 'NONE',  ( 0.8595800524934390507, -0.08942795157528024563, -0.3641732283464568787 ) ) ;
#998=CARTESIAN_POINT ( 'NONE',  ( 0.5118110236220480003, -0.6692913385826771977, 8.415575281601705876E-17 ) ) ;
#999=CARTESIAN_POINT ( 'NONE',  ( 0.9973753280839902091, 0.2306618581243847221, -0.2411417322834647770 ) ) ;
#1000=CARTESIAN_POINT ( 'NONE',  ( -0.07217847769028787330, -0.05778040916215522460, 0.4822834645669289988 ) ) ;
#1001=CARTESIAN_POINT ( 'NONE',  ( 0.5052493438320215802, 0.1771653543307087630, 0.09757992244046791164 ) ) ;
#1002=CARTESIAN_POINT ( 'NONE',  ( 1.076115485564305141, -0.6046776061558807314, 0.2411417322834647770 ) ) ;
#1004=CARTESIAN_POINT ( 'NONE',  ( -0.7152230971128602510, -0.05778040916215560624, -0.4822834645669293319 ) ) ;
#1008=CARTESIAN_POINT ( 'NONE',  ( 0.2427821522309716595, -0.3162353388693409650, -0.4822834645669289433 ) ) ;
#1009=CARTESIAN_POINT ( 'NONE',  ( -0.5380577427821514602, 0.05413385826771666132, 0.4176697321401328100 ) ) ;
#1010=CARTESIAN_POINT ( 'NONE',  ( 0.09842519685039434474, -0.5400638737290845981, -0.3530559997133363437 ) ) ;
#1016=CARTESIAN_POINT ( 'NONE',  ( -0.7939632545931754048, -0.2845877964562159024, 0.3641732283464567677 ) ) ;
#1018=CARTESIAN_POINT ( 'NONE',  ( -1.351706036745406347, 0.05413385826771626580, -0.4176697321401330321 ) ) ;
#1020=CARTESIAN_POINT ( 'NONE',  ( 0.3018372703412079971, 0.05413385826771626580, -0.4176697321401330321 ) ) ;
#1021=CARTESIAN_POINT ( 'NONE',  ( -0.4724409448818890911, -0.1870078740157479769, 0.3641732283464567677 ) ) ;
#1022=CARTESIAN_POINT ( 'NONE',  ( 1.181102362204724976, -0.1870078740157480879, -0.4822834645669291653 ) ) ;
#1023=CARTESIAN_POINT ( 'NONE',  ( 0.2165354330708668673, 0.1660481256975883668, -0.3530559997133364547 ) ) ;
#1027=CARTESIAN_POINT ( 'NONE',  ( 1.056430446194226658, 0.2952755905511811885, 0.1292274648535926551 ) ) ;
#1028=CARTESIAN_POINT ( 'NONE',  ( 0.2952755905511816326, -0.5400638737290844871, 0.3530559997133364547 ) ) ;
#1029=CARTESIAN_POINT ( 'NONE',  ( 0.3543307086614179147, 0.2952755905511811885, 0.000000000000000000 ) ) ;
#1030=CARTESIAN_POINT ( 'NONE',  ( 1.351706036745407680, 0.05413385826771666132, 0.4176697321401328100 ) ) ;
#1032=CARTESIAN_POINT ( 'NONE',  ( -0.03937007874015669567, -0.6692913385826771977, 8.415575281601705876E-17 ) ) ;
#1033=CARTESIAN_POINT ( 'NONE',  ( 1.102362204724410155, -0.1870078740157480879, -0.4822834645669291653 ) ) ;
#1034=CARTESIAN_POINT ( 'NONE',  ( 0.2099737532808405305, -0.6046776061558807314, 0.2411417322834647770 ) ) ;
#1035=CARTESIAN_POINT ( 'NONE',  ( 0.9776902887139113929, -0.5511811023622048555, -0.09757992244046775898 ) ) ;
#1036=CARTESIAN_POINT ( 'NONE',  ( -1.102362204724408601, -0.1870078740157479769, 0.4822834645669291653 ) ) ;
#1037=CARTESIAN_POINT ( 'NONE',  ( -1.443569553805773564, -0.6046776061558807314, 0.2411417322834647770 ) ) ;
#1038=CARTESIAN_POINT ( 'NONE',  ( 0.7020997375328090762, -0.05778040916215560624, -0.4822834645669293319 ) ) ;
#1039=CARTESIAN_POINT ( 'NONE',  ( -0.7402641841139964152, 2.388450810264987734, -0.4916013665244729491 ) ) ;
#1044=CARTESIAN_POINT ( 'NONE',  ( 1.384514435695538559, 0.2952755905511810774, -0.1292274648535930714 ) ) ;
#1045=CARTESIAN_POINT ( 'NONE',  ( 1.128608923884514947, 0.1283753931104748280, 0.1820866141732283561 ) ) ;
#1050=CARTESIAN_POINT ( 'NONE',  ( -1.312335958005248715, 0.1283753931104748280, 0.1820866141732283561 ) ) ;
#1051=CARTESIAN_POINT ( 'NONE',  ( 1.561679790026247350, -0.4281496062992124485, 0.4176697321401328655 ) ) ;
#1053=CARTESIAN_POINT ( 'NONE',  ( -0.3674540682414692561, -0.6046776061558809534, -0.2411417322834644161 ) ) ;
#1054=CARTESIAN_POINT ( 'NONE',  ( 1.056430446194226436, -0.6692913385826773087, -0.1292274648535924053 ) ) ;
#1056=CARTESIAN_POINT ( 'NONE',  ( -1.522309711286088607, 0.2306618581243847221, -0.2411417322834647770 ) ) ;
#1057=CARTESIAN_POINT ( 'NONE',  ( -0.7190005367825885729, -1.283732188437465593E-15, -0.4281993546915544013 ) ) ;
#1061=CARTESIAN_POINT ( 'NONE',  ( -0.8202099737532799750, 0.1771653543307087075, -0.09757992244046823083 ) ) ;
#1062=CARTESIAN_POINT ( 'NONE',  ( -1.581364829396324945, -0.05778040916215560624, -0.4822834645669293319 ) ) ;
#1063=CARTESIAN_POINT ( 'NONE',  ( 0.4133858267716541968, 0.1660481256975885056, 0.3530559997133364547 ) ) ;
#1065=VERTEX_POINT ( 'NONE', #20078 ) ;
#1066=CARTESIAN_POINT ( 'NONE',  ( -0.7461015469960392554, 2.206450217141186609, 0.5309055118110236338 ) ) ;
#1067=CARTESIAN_POINT ( 'NONE',  ( -2.787279214012418738, 2.401574803149606474, 0.000000000000000000 ) ) ;
#1068=CARTESIAN_POINT ( 'NONE',  ( 1.312335958005250269, -0.6046776061558807314, 0.2411417322834647770 ) ) ;
#1069=CARTESIAN_POINT ( 'NONE',  ( -1.699475065616797398, 0.2952755905511811885, 0.1292274648535926551 ) ) ;
#1071=CARTESIAN_POINT ( 'NONE',  ( -0.9645669291338575535, -0.4536011799217367080, 0.2665933059059888421 ) ) ;
#1072=CARTESIAN_POINT ( 'NONE',  ( -1.489501312335957062, -0.08942795157527998196, 0.3641732283464567121 ) ) ;
#1074=CARTESIAN_POINT ( 'NONE',  ( 0.6036745406824153282, -0.6046776061558807314, 0.2411417322834647770 ) ) ;
#1075=CARTESIAN_POINT ( 'NONE',  ( -0.8727034120734901146, -0.2845877964562159024, 0.3641732283464567677 ) ) ;
#1076=CARTESIAN_POINT ( 'NONE',  ( 0.1115485564304467270, -0.5511811023622048555, -0.09757992244046775898 ) ) ;
#1077=CARTESIAN_POINT ( 'NONE',  ( 0.2624671916010504757, -0.6046776061558809534, -0.2411417322834644161 ) ) ;
#1078=CARTESIAN_POINT ( 'NONE',  ( -1.272965879265091305, -0.004921259842519870586, -0.3153832671262229437 ) ) ;
#1080=CARTESIAN_POINT ( 'NONE',  ( 0.7217847769028878924, -0.4281496062992127816, -0.4176697321401328100 ) ) ;
#1082=CARTESIAN_POINT ( 'NONE',  ( -1.456692913385826182, 0.2952755905511811885, 0.000000000000000000 ) ) ;
#1084=CARTESIAN_POINT ( 'NONE',  ( -0.6167979002624665030, 0.05413385826771666132, 0.4176697321401328100 ) ) ;
#1085=CARTESIAN_POINT ( 'NONE',  ( 0.01968503937007930540, 0.07958543189024085140, 0.2665933059059887866 ) ) ;
#1086=CARTESIAN_POINT ( 'NONE',  ( -1.108923884514435132, -0.05778040916215560624, -0.4822834645669293319 ) ) ;
#1087=CARTESIAN_POINT ( 'NONE',  ( 0.9055118110236227702, 0.1771653543307087630, 0.000000000000000000 ) ) ;
#1088=CARTESIAN_POINT ( 'NONE',  ( -0.1771653543307080136, -0.4536011799217367080, 0.2665933059059888421 ) ) ;
#1089=CARTESIAN_POINT ( 'NONE',  ( -0.6889763779527552368, -0.5400638737290845981, -0.3530559997133363437 ) ) ;
#1090=CARTESIAN_POINT ( 'NONE',  ( -1.017060367454067249, -0.3162353388693409650, -0.4822834645669289433 ) ) ;
#1091=CARTESIAN_POINT ( 'NONE',  ( 1.666666666666667185, 0.05413385826771666132, 0.4176697321401328100 ) ) ;
#1093=CARTESIAN_POINT ( 'NONE',  ( 1.325459317585302665, -0.3690944881889763329, 0.3153832671262228327 ) ) ;
#1094=CARTESIAN_POINT ( 'NONE',  ( 0.2427821522309719648, -0.05778040916215522460, 0.4822834645669289988 ) ) ;
#1096=CARTESIAN_POINT ( 'NONE',  ( -1.673228346456691717, 0.1660481256975883668, -0.3530559997133364547 ) ) ;
#1097=ORIENTED_EDGE ( 'NONE', *, *, #67975, .T. ) ;
#1099=CARTESIAN_POINT ( 'NONE',  ( -0.9908136482939626788, 0.1771653543307087630, 0.09757992244046791164 ) ) ;
#1100=CARTESIAN_POINT ( 'NONE',  ( 0.9055118110236227702, -0.6692913385826771977, 8.415575281601705876E-17 ) ) ;
#1101=CARTESIAN_POINT ( 'NONE',  ( -1.154855643044618851, -0.5023911411419708095, -0.1820866141732282451 ) ) ;
#1103=CARTESIAN_POINT ( 'NONE',  ( -0.9973753280839886548, -0.6046776061558809534, -0.2411417322834644161 ) ) ;
#1104=CARTESIAN_POINT ( 'NONE',  ( 1.036745406824147731, 0.05413385826771666132, 0.4176697321401328100 ) ) ;
#1105=CARTESIAN_POINT ( 'NONE',  ( 0.6167979002624679463, 0.05413385826771626580, -0.4176697321401330321 ) ) ;
#1106=CARTESIAN_POINT ( 'NONE',  ( 1.240157480314961314, -0.5400638737290844871, 0.3530559997133364547 ) ) ;
#1107=CARTESIAN_POINT ( 'NONE',  ( -1.496062992125983815, -0.1870078740157480601, -0.3641732283464567677 ) ) ;
#1112=CARTESIAN_POINT ( 'NONE',  ( 0.7939632545931766261, -0.2845877964562161244, -0.3641732283464567121 ) ) ;
#1113=CARTESIAN_POINT ( 'NONE',  ( 0.3805774278215230400, -0.004921259842519870586, -0.3153832671262229437 ) ) ;
#1114=CARTESIAN_POINT ( 'NONE',  ( 0.05905511811023681640, 0.1660481256975883668, -0.3530559997133364547 ) ) ;
#1115=CARTESIAN_POINT ( 'NONE',  ( 1.108923884514436242, -0.05778040916215522460, 0.4822834645669289988 ) ) ;
#1117=CARTESIAN_POINT ( 'NONE',  ( 0.2165354330708668673, -0.4536011799217367080, 0.2665933059059888421 ) ) ;
#1118=CARTESIAN_POINT ( 'NONE',  ( -0.7742782152230962556, -0.4281496062992127816, -0.4176697321401328100 ) ) ;
#1119=CARTESIAN_POINT ( 'NONE',  ( 1.443569553805774897, 0.2306618581243848609, 0.2411417322834645549 ) ) ;
#1120=CARTESIAN_POINT ( 'NONE',  ( 1.010498687664042716, -0.4281496062992124485, 0.4176697321401328655 ) ) ;
#1123=CARTESIAN_POINT ( 'NONE',  ( 1.167979002624672580, 0.05413385826771626580, -0.4176697321401330321 ) ) ;
#1126=CARTESIAN_POINT ( 'NONE',  ( -1.456692913385826182, -0.6692913385826771977, 8.415575281601705876E-17 ) ) ;
#1127=CARTESIAN_POINT ( 'NONE',  ( -0.8267716535433065062, 0.1771653543307087630, 0.000000000000000000 ) ) ;
#1128=CARTESIAN_POINT ( 'NONE',  ( -0.6561679790026240244, 0.2306618581243847221, -0.2411417322834647770 ) ) ;
#1131=CARTESIAN_POINT ( 'NONE',  ( 1.509186351706037543, 0.05413385826771666132, 0.4176697321401328100 ) ) ;
#1132=CARTESIAN_POINT ( 'NONE',  ( -1.167979002624671470, -0.4281496062992127816, -0.4176697321401328100 ) ) ;
#1133=CARTESIAN_POINT ( 'NONE',  ( 0.3280839895013130669, 0.05413385826771666132, 0.4176697321401328100 ) ) ;
#1134=CARTESIAN_POINT ( 'NONE',  ( -1.227034120734907141, -0.6692913385826773087, -0.1292274648535924053 ) ) ;
#1136=CARTESIAN_POINT ( 'NONE',  ( 0.7742782152230978099, -0.4281496062992124485, 0.4176697321401328655 ) ) ;
#1138=CARTESIAN_POINT ( 'NONE',  ( -0.8464566929133852113, 0.07958543189024085140, 0.2665933059059887866 ) ) ;
#1142=CARTESIAN_POINT ( 'NONE',  ( -0.7426113562971995430, 2.793565526369265584, 0.5309055118110235227 ) ) ;
#1143=CARTESIAN_POINT ( 'NONE',  ( -1.207349081364828880, 0.2306618581243847221, -0.2411417322834647770 ) ) ;
#1144=CARTESIAN_POINT ( 'NONE',  ( -1.456692913385826182, 0.2952755905511811885, 0.000000000000000000 ) ) ;
#1146=CARTESIAN_POINT ( 'NONE',  ( -1.706036745406823485, 0.2306618581243848609, 0.2411417322834645549 ) ) ;
#1147=CARTESIAN_POINT ( 'NONE',  ( -1.141732283464566011, -0.6692913385826771977, 8.415575281601705876E-17 ) ) ;
#1148=CARTESIAN_POINT ( 'NONE',  ( -1.312335958005248715, 0.2306618581243848609, 0.2411417322834645549 ) ) ;
#1149=CARTESIAN_POINT ( 'NONE',  ( -0.3836918680457887532, -2.191421614605370878E-15, 0.4445507791589071167 ) ) ;
#1150=CARTESIAN_POINT ( 'NONE',  ( -0.8136482939632537770, 0.2306618581243847221, -0.2411417322834647770 ) ) ;
#1151=CARTESIAN_POINT ( 'NONE',  ( 0.1312335958005257930, 0.1283753931104746893, -0.1820866141732285504 ) ) ;
#1154=CARTESIAN_POINT ( 'NONE',  ( -0.4855643044619415427, -0.3690944881889763329, 0.3153832671262228327 ) ) ;
#1155=CARTESIAN_POINT ( 'NONE',  ( -0.6364829396325453192, -0.05778040916215560624, -0.4822834645669293319 ) ) ;
#1156=CARTESIAN_POINT ( 'NONE',  ( 0.8727034120734912248, -0.3162353388693409650, -0.4822834645669289433 ) ) ;
#1157=CARTESIAN_POINT ( 'NONE',  ( -0.3871391076115476282, -0.05778040916215522460, 0.4822834645669289988 ) ) ;
#1158=ORIENTED_EDGE ( 'NONE', *, *, #12089, .T. ) ;
#1161=CARTESIAN_POINT ( 'NONE',  ( -1.030183727034119867, -0.3162353388693405765, 0.4822834645669290543 ) ) ;
#1162=CARTESIAN_POINT ( 'NONE',  ( 1.082677165354331228, -0.5400638737290844871, 0.3530559997133364547 ) ) ;
#1163=CARTESIAN_POINT ( 'NONE',  ( -1.732283464566928277, -0.1870078740157479769, 0.3641732283464567677 ) ) ;
#1169=CARTESIAN_POINT ( 'NONE',  ( -0.2624671916010490880, -0.6046776061558807314, 0.2411417322834647770 ) ) ;
#1170=CARTESIAN_POINT ( 'NONE',  ( -1.469816272965878357, 0.1283753931104748280, 0.1820866141732283561 ) ) ;
#1171=CARTESIAN_POINT ( 'NONE',  ( -0.8136482939632537770, -0.6046776061558807314, 0.2411417322834647770 ) ) ;
#1173=CARTESIAN_POINT ( 'NONE',  ( -1.259842519685038686, -0.1870078740157479769, 0.4822834645669291653 ) ) ;
#1175=CARTESIAN_POINT ( 'NONE',  ( -0.8464566929133852113, -0.5400638737290845981, -0.3530559997133363437 ) ) ;
#1176=CARTESIAN_POINT ( 'NONE',  ( -0.3543307086614165824, -0.6692913385826771977, 8.415575281601705876E-17 ) ) ;
#1178=CARTESIAN_POINT ( 'NONE',  ( 0.7939632545931766261, -0.08942795157527998196, 0.3641732283464567121 ) ) ;
#1180=CARTESIAN_POINT ( 'NONE',  ( 0.1246719160104994284, 0.1771653543307087075, -0.09757992244046823083 ) ) ;
#1181=CARTESIAN_POINT ( 'NONE',  ( 1.535433070866142335, -0.5511811023622047445, 6.969142054262312111E-17 ) ) ;
#1182=CARTESIAN_POINT ( 'NONE',  ( 1.548556430446194954, -0.6046776061558807314, 0.2411417322834647770 ) ) ;
#1183=CARTESIAN_POINT ( 'NONE',  ( 0.1574803149606306130, -0.1870078740157480601, -0.3641732283464567677 ) ) ;
#1185=CARTESIAN_POINT ( 'NONE',  ( -1.345144356955379816, -0.3162353388693405765, 0.4822834645669290543 ) ) ;
#1186=CARTESIAN_POINT ( 'NONE',  ( 1.213910761154856299, -0.6692913385826773087, -0.1292274648535924053 ) ) ;
#1189=CARTESIAN_POINT ( 'NONE',  ( -0.7020997375328074108, -0.08942795157527998196, 0.3641732283464567121 ) ) ;
#1190=CARTESIAN_POINT ( 'NONE',  ( -0.4593175853018366950, 0.05413385826771666132, 0.4176697321401328100 ) ) ;
#1191=CARTESIAN_POINT ( 'NONE',  ( 0.2887139107611556010, 0.2306618581243847221, -0.2411417322834647770 ) ) ;
#1193=CARTESIAN_POINT ( 'NONE',  ( 1.122047244094488860, 0.07958543189024085140, 0.2665933059059887866 ) ) ;
#1194=CARTESIAN_POINT ( 'NONE',  ( 0.3477690288713918276, 0.1771653543307087630, 0.09757992244046791164 ) ) ;
#1195=CARTESIAN_POINT ( 'NONE',  ( -0.1837270341207340729, 0.2306618581243847221, -0.2411417322834647770 ) ) ;
#1197=CARTESIAN_POINT ( 'NONE',  ( -0.8661417322834640276, -0.1870078740157479769, 0.3641732283464567677 ) ) ;
#1198=CARTESIAN_POINT ( 'NONE',  ( 0.4606732211678799538, 2.793565526369266028, -0.5309055118110236338 ) ) ;
#1199=CARTESIAN_POINT ( 'NONE',  ( 0.6496062992125991586, -0.5400638737290845981, -0.3530559997133363437 ) ) ;
#1200=CARTESIAN_POINT ( 'NONE',  ( -1.062992125984250968, -0.6692913385826771977, 8.415575281601705876E-17 ) ) ;
#1203=CARTESIAN_POINT ( 'NONE',  ( 0.1115485564304467270, -0.5511811023622048555, -0.09757992244046775898 ) ) ;
#1204=CARTESIAN_POINT ( 'NONE',  ( -0.8267716535433065062, 0.2952755905511811885, 0.000000000000000000 ) ) ;
#1205=CARTESIAN_POINT ( 'NONE',  ( -1.207349081364828436, -0.6046776061558807314, 0.2411417322834647770 ) ) ;
#1206=CARTESIAN_POINT ( 'NONE',  ( -1.148293963254592542, 0.1771653543307087630, 0.09757992244046791164 ) ) ;
#1208=CARTESIAN_POINT ( 'NONE',  ( -0.8398950131233585692, 0.1283753931104748280, 0.1820866141732283561 ) ) ;
#1209=CARTESIAN_POINT ( 'NONE',  ( -1.595398199321655497, 1.860919225514068076, 0.1559797534342490799 ) ) ;
#1210=CARTESIAN_POINT ( 'NONE',  ( 1.128608923884514947, 0.2306618581243848609, 0.2411417322834645549 ) ) ;
#1215=EDGE_CURVE ( 'NONE', #15840, #72947, #65515, .T. ) ;
#1216=CARTESIAN_POINT ( 'NONE',  ( -1.699475065616797398, 0.2952755905511811885, 0.1292274648535926551 ) ) ;
#1217=CARTESIAN_POINT ( 'NONE',  ( -1.417322834645668772, -0.1870078740157479769, 0.4822834645669291653 ) ) ;
#1218=CARTESIAN_POINT ( 'NONE',  ( 1.397637795275591177, -0.5400638737290844871, 0.3530559997133364547 ) ) ;
#1222=CARTESIAN_POINT ( 'NONE',  ( 0.3543307086614181922, -0.6692913385826771977, 8.415575281601705876E-17 ) ) ;
#1223=CARTESIAN_POINT ( 'NONE',  ( -0.4199475065616791736, -0.6046776061558807314, 0.2411417322834647770 ) ) ;
#1226=CARTESIAN_POINT ( 'NONE',  ( 0.7217847769028878924, -0.3690944881889765550, -0.3153832671262227771 ) ) ;
#1230=VERTEX_POINT ( 'NONE', #26801 ) ;
#1231=CARTESIAN_POINT ( 'NONE',  ( -0.1049868766404193215, 0.2306618581243847221, -0.2411417322834647770 ) ) ;
#1232=CARTESIAN_POINT ( 'NONE',  ( 1.456692913385827515, 0.2952755905511811885, 0.000000000000000000 ) ) ;
#1233=CARTESIAN_POINT ( 'NONE',  ( 0.4199475065616805614, 0.2306618581243848609, 0.2411417322834645549 ) ) ;
#1234=CARTESIAN_POINT ( 'NONE',  ( 1.404199475065617708, 0.05413385826771626580, -0.4176697321401330321 ) ) ;
#1235=CARTESIAN_POINT ( 'NONE',  ( -0.6364829396325453192, -0.05778040916215560624, -0.4822834645669293319 ) ) ;
#1236=CARTESIAN_POINT ( 'NONE',  ( 5.463695987328526437E-16, -0.1870078740157479769, 0.4822834645669291653 ) ) ;
#1237=CARTESIAN_POINT ( 'NONE',  ( 1.456692913385827515, 0.2952755905511811885, 0.000000000000000000 ) ) ;
#1238=CARTESIAN_POINT ( 'NONE',  ( 1.233595800524935227, -0.6046776061558807314, 0.2411417322834647770 ) ) ;
#1239=CARTESIAN_POINT ( 'NONE',  ( 1.351706036745407680, 0.05413385826771666132, 0.4176697321401328100 ) ) ;
#1242=CARTESIAN_POINT ( 'NONE',  ( 0.2296587926509192634, -0.2845877964562159024, 0.3641732283464567677 ) ) ;
#1246=CARTESIAN_POINT ( 'NONE',  ( -0.5314960629921254842, -0.4536011799217368745, -0.2665933059059886201 ) ) ;
#1247=CARTESIAN_POINT ( 'NONE',  ( 0.09186351706036827158, 0.05413385826771666132, 0.4176697321401328100 ) ) ;
#1249=CARTESIAN_POINT ( 'NONE',  ( 0.2559055118110243332, -0.5400638737290845981, -0.3530559997133363437 ) ) ;
#1250=CARTESIAN_POINT ( 'NONE',  ( 0.1771653543307093182, 0.1660481256975885056, 0.3530559997133364547 ) ) ;
#1251=EDGE_CURVE ( 'NONE', #57928, #4124, #72516, .T. ) ;
#1252=CARTESIAN_POINT ( 'NONE',  ( -0.7020997375328074108, -0.05778040916215522460, 0.4822834645669289988 ) ) ;
#1253=CARTESIAN_POINT ( 'NONE',  ( -0.8005249343832013809, -0.4281496062992124485, 0.4176697321401328655 ) ) ;
#1254=CARTESIAN_POINT ( 'NONE',  ( 1.200787401574803681, 0.07958543189024085140, 0.2665933059059887866 ) ) ;
#1255=CARTESIAN_POINT ( 'NONE',  ( 1.604771003085129433, 0.4514378173630680946, 0.1466069496707752551 ) ) ;
#1257=CARTESIAN_POINT ( 'NONE',  ( 1.030183727034121421, -0.2845877964562161244, -0.3641732283464567121 ) ) ;
#1258=CARTESIAN_POINT ( 'NONE',  ( 0.5905511811023629321, 0.2952755905511811885, 0.000000000000000000 ) ) ;
#1259=CARTESIAN_POINT ( 'NONE',  ( 0.9251968503937015864, 0.1660481256975883668, -0.3530559997133364547 ) ) ;
#1261=CARTESIAN_POINT ( 'NONE',  ( -1.594488188976377563, -0.5400638737290844871, 0.3530559997133364547 ) ) ;
#1264=CARTESIAN_POINT ( 'NONE',  ( -0.4790026246719154557, -0.3162353388693405765, 0.4822834645669290543 ) ) ;
#1267=CARTESIAN_POINT ( 'NONE',  ( -1.246719160104985846, -0.3690944881889765550, -0.3153832671262227771 ) ) ;
#1268=CARTESIAN_POINT ( 'NONE',  ( 1.213910761154856299, -0.6692913385826773087, -0.1292274648535924053 ) ) ;
#1269=CARTESIAN_POINT ( 'NONE',  ( 1.115485564304462551, -0.4281496062992127816, -0.4176697321401328100 ) ) ;
#1270=CARTESIAN_POINT ( 'NONE',  ( -0.3018372703412066094, -0.3690944881889765550, -0.3153832671262227771 ) ) ;
#1271=CARTESIAN_POINT ( 'NONE',  ( 0.2821522309711292364, -0.6692913385826771977, 0.1292274648535927661 ) ) ;
#1273=CARTESIAN_POINT ( 'NONE',  ( 0.3674540682414705883, -0.5023911411419708095, 0.1820866141732285504 ) ) ;
#1274=CARTESIAN_POINT ( 'NONE',  ( -0.09842519685039295696, 0.1660481256975883668, -0.3530559997133364547 ) ) ;
#1276=CARTESIAN_POINT ( 'NONE',  ( -1.259842519685038686, -0.1870078740157479769, 0.4822834645669291653 ) ) ;
#1277=CARTESIAN_POINT ( 'NONE',  ( 0.6430446194225728496, -0.004921259842519576551, 0.3153832671262227771 ) ) ;
#1278=CARTESIAN_POINT ( 'NONE',  ( 0.3805774278215230400, 0.009842519685039144428, -0.3409548833797004797 ) ) ;
#1279=CARTESIAN_POINT ( 'NONE',  ( -0.8923884514435688198, 0.2306618581243847221, -0.2411417322834647770 ) ) ;
#1280=CARTESIAN_POINT ( 'NONE',  ( -0.1443569553805765515, -0.3690944881889765550, -0.3153832671262227771 ) ) ;
#1281=FACE_OUTER_BOUND ( 'NONE', #60724, .T. ) ;
#1282=CARTESIAN_POINT ( 'NONE',  ( -0.8267716535433065062, -0.6692913385826771977, 8.415575281601705876E-17 ) ) ;
#1283=CARTESIAN_POINT ( 'NONE',  ( -0.7020997375328074108, -0.05778040916215522460, 0.4822834645669289988 ) ) ;
#1284=CARTESIAN_POINT ( 'NONE',  ( 0.1049868766404206816, 0.2306618581243848609, 0.2411417322834645549 ) ) ;
#1288=CARTESIAN_POINT ( 'NONE',  ( 0.8923884514435703741, 0.1283753931104748280, 0.1820866141732283561 ) ) ;
#1289=CARTESIAN_POINT ( 'NONE',  ( 1.450131233595801428, 0.2952755905511811885, 0.1292274648535926551 ) ) ;
#1290=CARTESIAN_POINT ( 'NONE',  ( -0.9055118110236215490, 0.1771653543307087630, 0.000000000000000000 ) ) ;
#1291=CARTESIAN_POINT ( 'NONE',  ( -1.003937007874015297, -0.4536011799217368745, -0.2665933059059886201 ) ) ;
#1292=CARTESIAN_POINT ( 'NONE',  ( -0.7086614173228339419, -0.1870078740157479769, 0.4822834645669291653 ) ) ;
#1293=CARTESIAN_POINT ( 'NONE',  ( -0.2493438320209966919, 0.05413385826771626580, -0.4176697321401330321 ) ) ;
#1294=CARTESIAN_POINT ( 'NONE',  ( 0.7086614173228353852, -0.1870078740157479769, 0.3641732283464567677 ) ) ;
#1296=CARTESIAN_POINT ( 'NONE',  ( 1.148293963254593653, 0.1771653543307087075, -0.09757992244046823083 ) ) ;
#1298=CARTESIAN_POINT ( 'NONE',  ( 0.3083989501312343062, -0.05778040916215560624, -0.4822834645669293319 ) ) ;
#1300=CARTESIAN_POINT ( 'NONE',  ( -0.5511811023622041894, -0.1870078740157480879, -0.4822834645669291653 ) ) ;
#1302=CARTESIAN_POINT ( 'NONE',  ( 1.266404199475066328, -0.08942795157527998196, 0.3641732283464567121 ) ) ;
#1303=CARTESIAN_POINT ( 'NONE',  ( 0.3083989501312343062, -0.05778040916215560624, -0.4822834645669293319 ) ) ;
#1304=CARTESIAN_POINT ( 'NONE',  ( 0.01312335958005323398, -0.4281496062992127816, -0.4176697321401328100 ) ) ;
#1305=CARTESIAN_POINT ( 'NONE',  ( 0.1706036745406830368, -0.3690944881889765550, -0.3153832671262227771 ) ) ;
#1307=CARTESIAN_POINT ( 'NONE',  ( -0.03280839895013062252, 0.1771653543307087075, -0.09757992244046823083 ) ) ;
#1308=CARTESIAN_POINT ( 'NONE',  ( 0.8595800524934390507, -0.3162353388693405765, 0.4822834645669290543 ) ) ;
#1309=CARTESIAN_POINT ( 'NONE',  ( -0.7611548556430438595, 0.1283753931104748280, 0.1820866141732283561 ) ) ;
#1310=CARTESIAN_POINT ( 'NONE',  ( -0.6692913385826764205, 0.2952755905511811885, 0.000000000000000000 ) ) ;
#1311=CARTESIAN_POINT ( 'NONE',  ( -0.8537221893815262197, -2.294479370626195693E-15, 0.3464511005275217603 ) ) ;
#1312=EDGE_LOOP ( 'NONE', ( #54492, #20805, #16795, #50693 ) ) ;
#1313=CARTESIAN_POINT ( 'NONE',  ( -1.279527559055116948, 0.1660481256975883668, -0.3530559997133364547 ) ) ;
#1314=CARTESIAN_POINT ( 'NONE',  ( -1.299212598425196097, -0.5511811023622047445, 6.969142054262312111E-17 ) ) ;
#1315=CARTESIAN_POINT ( 'NONE',  ( -0.03937007874015669567, -0.6692913385826771977, 8.415575281601705876E-17 ) ) ;
#1316=CARTESIAN_POINT ( 'NONE',  ( -1.489501312335957062, -0.3162353388693409650, -0.4822834645669289433 ) ) ;
#1317=CARTESIAN_POINT ( 'NONE',  ( -0.9317585301837263412, -0.4281496062992127816, -0.4176697321401328100 ) ) ;
#1319=CARTESIAN_POINT ( 'NONE',  ( 1.069553805774278832, 0.2952755905511810219, -0.1292274648535930437 ) ) ;
#1320=CARTESIAN_POINT ( 'NONE',  ( 1.069553805774278610, -0.6692913385826771977, 0.1292274648535927661 ) ) ;
#1321=CARTESIAN_POINT ( 'NONE',  ( 1.410761154855643795, -0.05778040916215560624, -0.4822834645669293319 ) ) ;
#1324=CARTESIAN_POINT ( 'NONE',  ( -1.187664041994750175, -0.05778040916215560624, -0.4822834645669293319 ) ) ;
#1328=CARTESIAN_POINT ( 'NONE',  ( -0.2624671916010490880, -0.5023911411419708095, 0.1820866141732285504 ) ) ;
#1331=CARTESIAN_POINT ( 'NONE',  ( 0.1246719160104994284, -0.6692913385826771977, 0.1292274648535927661 ) ) ;
#1332=CARTESIAN_POINT ( 'NONE',  ( 0.1181102362204730916, -0.6692913385826771977, 8.415575281601705876E-17 ) ) ;
#1333=CARTESIAN_POINT ( 'NONE',  ( -0.6561679790026240244, 0.2306618581243847221, -0.2411417322834647770 ) ) ;
#1335=CARTESIAN_POINT ( 'NONE',  ( -0.9514435695538050464, -0.08942795157528024563, -0.3641732283464568787 ) ) ;
#1336=CARTESIAN_POINT ( 'NONE',  ( 0.8070866141732289112, -0.5400638737290845981, -0.3530559997133363437 ) ) ;
#1337=CARTESIAN_POINT ( 'NONE',  ( 0.7152230971128614723, -0.2845877964562161244, -0.3641732283464567121 ) ) ;
#1338=CARTESIAN_POINT ( 'NONE',  ( -0.3346456692913377662, 0.1660481256975883668, -0.3530559997133364547 ) ) ;
#1340=CARTESIAN_POINT ( 'NONE',  ( -0.6561679790026240244, 0.2306618581243847221, -0.2411417322834647770 ) ) ;
#1341=CARTESIAN_POINT ( 'NONE',  ( -1.627296587926508442, -0.5023911411419708095, -0.1820866141732282451 ) ) ;
#1342=EDGE_CURVE ( 'NONE', #17299, #25966, #65115, .T. ) ;
#1343=CARTESIAN_POINT ( 'NONE',  ( 1.141732283464567788, -0.6692913385826771977, 8.415575281601705876E-17 ) ) ;
#1344=CARTESIAN_POINT ( 'NONE',  ( 1.509186351706037543, -0.004921259842519576551, 0.3153832671262227771 ) ) ;
#1347=CARTESIAN_POINT ( 'NONE',  ( -0.1771653543307080136, 0.1660481256975883668, -0.3530559997133364547 ) ) ;
#1349=CARTESIAN_POINT ( 'NONE',  ( -0.8923884514435688198, 0.2306618581243847221, -0.2411417322834647770 ) ) ;
#1350=CARTESIAN_POINT ( 'NONE',  ( 1.299212598425197429, 0.2952755905511811885, 0.000000000000000000 ) ) ;
#1351=CARTESIAN_POINT ( 'NONE',  ( 1.469816272965879911, 0.2306618581243847221, -0.2411417322834647770 ) ) ;
#1352=CARTESIAN_POINT ( 'NONE',  ( 0.08530183727034192087, -0.3162353388693409650, -0.4822834645669289433 ) ) ;
#1353=CARTESIAN_POINT ( 'NONE',  ( -0.2034120734908128059, 0.2952755905511811885, 0.1292274648535926551 ) ) ;
#1355=CARTESIAN_POINT ( 'NONE',  ( -1.049868766404198794, 0.2306618581243847221, -0.2411417322834647770 ) ) ;
#1356=CARTESIAN_POINT ( 'NONE',  ( -0.4199475065616791736, -0.6046776061558807314, 0.2411417322834647770 ) ) ;
#1357=CARTESIAN_POINT ( 'NONE',  ( -0.1246719160104980823, -0.5511811023622048555, -0.09757992244046775898 ) ) ;
#1358=CARTESIAN_POINT ( 'NONE',  ( 1.535433070866142558, 0.2952755905511811885, 0.000000000000000000 ) ) ;
#1359=CARTESIAN_POINT ( 'NONE',  ( -0.6627296587926503335, -0.6692913385826771977, 0.1292274648535927661 ) ) ;
#1360=CARTESIAN_POINT ( 'NONE',  ( -1.213910761154854967, 0.2952755905511810219, -0.1292274648535930437 ) ) ;
#1361=CARTESIAN_POINT ( 'NONE',  ( 0.8005249343832027131, 0.05413385826771666132, 0.4176697321401328100 ) ) ;
#1363=ORIENTED_EDGE ( 'NONE', *, *, #54694, .F. ) ;
#1364=CARTESIAN_POINT ( 'NONE',  ( -0.03937007874015669567, 0.2952755905511811885, 0.000000000000000000 ) ) ;
#1365=CARTESIAN_POINT ( 'NONE',  ( -0.2296587926509179312, -0.2845877964562161244, -0.3641732283464567121 ) ) ;
#1366=CARTESIAN_POINT ( 'NONE',  ( 1.220472440944882608, 0.1771653543307087630, 0.000000000000000000 ) ) ;
#1369=CARTESIAN_POINT ( 'NONE',  ( 1.646981627296588035, -0.2845877964562159024, 0.3641732283464567677 ) ) ;
#1371=CARTESIAN_POINT ( 'NONE',  ( 1.167979002624672580, 0.05413385826771626580, -0.4176697321401330321 ) ) ;
#1373=CARTESIAN_POINT ( 'NONE',  ( 0.2230971128608929543, 0.05413385826771626580, -0.4176697321401330321 ) ) ;
#1374=CARTESIAN_POINT ( 'NONE',  ( -1.489501312335957062, -0.3162353388693409650, -0.4822834645669289433 ) ) ;
#1375=CARTESIAN_POINT ( 'NONE',  ( -0.2690288713910754526, 0.2952755905511810774, -0.1292274648535930714 ) ) ;
#1378=CARTESIAN_POINT ( 'NONE',  ( -1.633858267716534529, 0.07958543189024085140, 0.2665933059059887866 ) ) ;
#1379=CARTESIAN_POINT ( 'NONE',  ( 0.5249343832021003964, 0.2306618581243847221, -0.2411417322834647770 ) ) ;
#1380=CARTESIAN_POINT ( 'NONE',  ( 0.8858267716535438430, 0.07958543189024085140, 0.2665933059059887866 ) ) ;
#1381=CARTESIAN_POINT ( 'NONE',  ( 0.2099737532808405305, -0.5023911411419708095, 0.1820866141732285504 ) ) ;
#1382=CARTESIAN_POINT ( 'NONE',  ( -1.318897637795274802, 0.1660481256975885056, 0.3530559997133364547 ) ) ;
#1384=CARTESIAN_POINT ( 'NONE',  ( 1.286089238845145033, -0.6046776061558809534, -0.2411417322834644161 ) ) ;
#1386=CARTESIAN_POINT ( 'NONE',  ( 0.8070866141732289112, -0.5400638737290845981, -0.3530559997133363437 ) ) ;
#1387=CARTESIAN_POINT ( 'NONE',  ( 0.8792650918635177559, 0.05413385826771666132, 0.4176697321401328100 ) ) ;
#1389=CARTESIAN_POINT ( 'NONE',  ( 0.4265091863517067039, -0.5511811023622048555, -0.09757992244046775898 ) ) ;
#1390=CARTESIAN_POINT ( 'NONE',  ( 0.5577427821522316087, -0.05778040916215522460, 0.4822834645669289988 ) ) ;
#1391=CARTESIAN_POINT ( 'NONE',  ( 1.627296587926509996, -0.5023911411419708095, 0.1820866141732285504 ) ) ;
#1392=CARTESIAN_POINT ( 'NONE',  ( -0.8595800524934373854, -0.2845877964562161244, -0.3641732283464567121 ) ) ;
#1393=CARTESIAN_POINT ( 'NONE',  ( -1.062992125984250968, 0.2952755905511811885, 0.000000000000000000 ) ) ;
#1394=CARTESIAN_POINT ( 'NONE',  ( -1.528871391076114250, 0.2952755905511810774, -0.1292274648535930714 ) ) ;
#1395=CARTESIAN_POINT ( 'NONE',  ( 0.8464566929133866546, -0.5400638737290844871, 0.3530559997133364547 ) ) ;
#1396=CARTESIAN_POINT ( 'NONE',  ( -1.561679790026246017, -0.3690944881889765550, -0.3153832671262227771 ) ) ;
#1398=CARTESIAN_POINT ( 'NONE',  ( 0.6561679790026253567, 0.2306618581243848609, 0.2411417322834645549 ) ) ;
#1400=DIRECTION ( 'NONE',  ( 1.000000000000000000, -0.000000000000000000, -0.000000000000000000 ) ) ;
#1401=CARTESIAN_POINT ( 'NONE',  ( 1.476377952755906442, -0.5400638737290844871, 0.3530559997133364547 ) ) ;
#1402=CARTESIAN_POINT ( 'NONE',  ( -1.548556430446193399, 0.1283753931104748280, 0.1820866141732283561 ) ) ;
#1403=CARTESIAN_POINT ( 'NONE',  ( 1.351706036745407680, -0.004921259842519576551, 0.3153832671262227771 ) ) ;
#1404=CARTESIAN_POINT ( 'NONE',  ( -1.154855643044618851, 0.1283753931104748280, 0.1820866141732283561 ) ) ;
#1405=CARTESIAN_POINT ( 'NONE',  ( -0.5380577427821514602, -0.004921259842519576551, 0.3153832671262227771 ) ) ;
#1407=CARTESIAN_POINT ( 'NONE',  ( 0.9580052493438326877, -0.004921259842519576551, 0.3153832671262227771 ) ) ;
#1408=CARTESIAN_POINT ( 'NONE',  ( 0.4396325459317593221, 0.2952755905511810774, -0.1292274648535930714 ) ) ;
#1409=CARTESIAN_POINT ( 'NONE',  ( 1.181102362204724976, -0.1870078740157480879, -0.4822834645669291653 ) ) ;
#1411=CARTESIAN_POINT ( 'NONE',  ( 0.2034120734908144990, -0.6692913385826771977, 0.1292274648535927661 ) ) ;
#1412=CARTESIAN_POINT ( 'NONE',  ( 0.4133858267716541968, -0.4536011799217368745, -0.2665933059059886201 ) ) ;
#1413=CARTESIAN_POINT ( 'NONE',  ( 1.115485564304462551, 0.05413385826771666132, 0.4176697321401328100 ) ) ;
#1415=CARTESIAN_POINT ( 'NONE',  ( -0.5183727034120726440, -0.6692913385826773087, -0.1292274648535924053 ) ) ;
#1418=CARTESIAN_POINT ( 'NONE',  ( -0.01312335958005186876, -0.4281496062992124485, 0.4176697321401328655 ) ) ;
#1419=CARTESIAN_POINT ( 'NONE',  ( -0.6299212598425188991, -0.1870078740157480879, -0.4822834645669291653 ) ) ;
#1420=CARTESIAN_POINT ( 'NONE',  ( -0.2296587926509179312, -0.3162353388693409650, -0.4822834645669289433 ) ) ;
#1425=CARTESIAN_POINT ( 'NONE',  ( -0.9580052493438311334, -0.3690944881889763329, 0.3153832671262228327 ) ) ;
#1427=CARTESIAN_POINT ( 'NONE',  ( -1.049868766404198794, 0.2306618581243847221, -0.2411417322834647770 ) ) ;
#1429=CARTESIAN_POINT ( 'NONE',  ( 0.4133858267716541968, 0.1660481256975885056, 0.3530559997133364547 ) ) ;
#1430=CARTESIAN_POINT ( 'NONE',  ( -0.4199475065616791736, 0.1283753931104746893, -0.1820866141732285504 ) ) ;
#1431=CARTESIAN_POINT ( 'NONE',  ( 1.437007874015748810, 0.1660481256975885056, 0.3530559997133364547 ) ) ;
#1432=CARTESIAN_POINT ( 'NONE',  ( 0.1968503937007881344, 0.2952755905511811885, 0.000000000000000000 ) ) ;
#1436=CARTESIAN_POINT ( 'NONE',  ( 1.213910761154856299, 0.2952755905511811885, 0.1292274648535926551 ) ) ;
#1437=CARTESIAN_POINT ( 'NONE',  ( 0.6430446194225728496, 0.05413385826771666132, 0.4176697321401328100 ) ) ;
#1438=CARTESIAN_POINT ( 'NONE',  ( 0.1049868766404206816, -0.6046776061558809534, -0.2411417322834644161 ) ) ;
#1439=CARTESIAN_POINT ( 'NONE',  ( 1.607611548556431069, 0.2952755905511811885, 0.1292274648535926551 ) ) ;
#1440=CARTESIAN_POINT ( 'NONE',  ( 0.9251968503937015864, 0.1660481256975883668, -0.3530559997133364547 ) ) ;
#1442=CARTESIAN_POINT ( 'NONE',  ( 0.09186351706036799403, -0.4281496062992127816, -0.4176697321401328100 ) ) ;
#1443=CARTESIAN_POINT ( 'NONE',  ( 1.108923884514436686, -0.3162353388693409650, -0.4822834645669289433 ) ) ;
#1444=CARTESIAN_POINT ( 'NONE',  ( 0.3280839895013130669, -0.4281496062992127816, -0.4176697321401328100 ) ) ;
#1445=CARTESIAN_POINT ( 'NONE',  ( 1.240157480314961314, 0.07958543189024071263, -0.2665933059059888421 ) ) ;
#1446=CARTESIAN_POINT ( 'NONE',  ( -1.489501312335957062, -0.3162353388693409650, -0.4822834645669289433 ) ) ;
#1447=CARTESIAN_POINT ( 'NONE',  ( -1.246719160104986512, 0.05413385826771666132, 0.4176697321401328100 ) ) ;
#1448=CARTESIAN_POINT ( 'NONE',  ( 0.5774278215223103139, -0.6046776061558809534, -0.2411417322834644161 ) ) ;
#1454=CARTESIAN_POINT ( 'NONE',  ( 1.627296587926509996, -0.6046776061558807314, 0.2411417322834647770 ) ) ;
#1455=CARTESIAN_POINT ( 'NONE',  ( 1.003937007874016185, 0.07958543189024071263, -0.2665933059059888421 ) ) ;
#1458=DIRECTION ( 'NONE',  ( -3.096699300667737957E-16, 1.000000000000000000, -0.000000000000000000 ) ) ;
#1460=EDGE_CURVE ( 'NONE', #74234, #57436, #76219, .T. ) ;
#1461=CARTESIAN_POINT ( 'NONE',  ( 1.364829396325459854, -0.6046776061558809534, -0.2411417322834644161 ) ) ;
#1463=CARTESIAN_POINT ( 'NONE',  ( -0.4855643044619415427, -0.4281496062992124485, 0.4176697321401328655 ) ) ;
#1464=CARTESIAN_POINT ( 'NONE',  ( 1.076115485564305141, -0.6046776061558807314, 0.2411417322834647770 ) ) ;
#1466=VECTOR ( 'NONE', #20081, 39.37007874015748143 ) ;
#1467=CARTESIAN_POINT ( 'NONE',  ( -1.502624671916009680, -0.05778040916215560624, -0.4822834645669293319 ) ) ;
#1470=B_SPLINE_CURVE_WITH_KNOTS ( 'NONE', 3,
 ( #22018, #9392, #8152, #74203 ),
 .UNSPECIFIED., .F., .F.,
 ( 4, 4 ),
 ( 0.03364299943132197795, 0.03394594375427735511 ),
 .UNSPECIFIED. ) ;
#1471=CARTESIAN_POINT ( 'NONE',  ( 1.679790026246720025, 0.1283753931104748280, 0.1820866141732283561 ) ) ;
#1472=DIRECTION ( 'NONE',  ( -3.096699300667737957E-16, 1.000000000000000000, -0.000000000000000000 ) ) ;
#1473=CARTESIAN_POINT ( 'NONE',  ( -0.8530183727034112984, -0.004921259842519576551, 0.3153832671262227771 ) ) ;
#1474=CARTESIAN_POINT ( 'NONE',  ( 0.8858267716535437319, 0.1012011053420777407, 0.2882089793578256898 ) ) ;
#1475=CARTESIAN_POINT ( 'NONE',  ( 0.7874015748031503170, -0.1870078740157480879, -0.4822834645669291653 ) ) ;
#1476=ORIENTED_EDGE ( 'NONE', *, *, #70755, .T. ) ;
#1478=DIRECTION ( 'NONE',  ( -0.000000000000000000, 1.000000000000000000, -0.000000000000000000 ) ) ;
#1479=CARTESIAN_POINT ( 'NONE',  ( 0.8727034120734913358, -0.05778040916215522460, 0.4822834645669289988 ) ) ;
#1480=CARTESIAN_POINT ( 'NONE',  ( 1.502624671916010790, -0.2845877964562161244, -0.3641732283464567121 ) ) ;
#1482=CARTESIAN_POINT ( 'NONE',  ( -0.5971128608923877978, 0.1771653543307087630, 0.09757992244046791164 ) ) ;
#1483=CARTESIAN_POINT ( 'NONE',  ( 1.646981627296588035, -0.3162353388693405765, 0.4822834645669290543 ) ) ;
#1485=CARTESIAN_POINT ( 'NONE',  ( 0.5118110236220478892, 0.2952755905511811885, 0.000000000000000000 ) ) ;
#1486=CARTESIAN_POINT ( 'NONE',  ( -1.095800524934382292, -0.2845877964562161244, -0.3641732283464567121 ) ) ;
#1487=CARTESIAN_POINT ( 'NONE',  ( 0.1312335958005255154, -0.5023911411419708095, 0.1820866141732285504 ) ) ;
#1488=AXIS2_PLACEMENT_3D ( 'NONE', #72842, #78337, #8046 ) ;
#1489=CARTESIAN_POINT ( 'NONE',  ( -0.4002624671916004129, -0.05778040916215560624, -0.4822834645669293319 ) ) ;
#1490=CARTESIAN_POINT ( 'NONE',  ( -1.207349081364828436, -0.5023911411419708095, 0.1820866141732285504 ) ) ;
#1492=CARTESIAN_POINT ( 'NONE',  ( 0.9120734908136489683, -0.6692913385826771977, 0.1292274648535927661 ) ) ;
#1493=( BOUNDED_CURVE ( )  B_SPLINE_CURVE ( 2, ( #10605, #74166, #55192, #80899, #29935, #73759, #2632, #61524, #42568, #35027, #41739, #68269, #28288 ),
 .UNSPECIFIED., .F., .F. ) 
 B_SPLINE_CURVE_WITH_KNOTS ( ( 3, 2, 2, 2, 2, 2, 3 ),
 ( 0.4460583673620736045, 0.4469696969696969613, 0.4507575757575757458, 0.4545454545454545303, 0.4583333333333333148, 0.4621212121212120993, 0.4630325417288355672 ),
 .UNSPECIFIED. ) 
 CURVE ( )  GEOMETRIC_REPRESENTATION_ITEM ( )  RATIONAL_B_SPLINE_CURVE ( ( 0.9875488213027530104, 0.9918020599134685922, 1.000000000000000000, 0.9659258262890683122, 1.000000000000000000, 0.9659258262890683122, 1.000000000000000000, 0.9659258262890683122, 1.000000000000000000, 0.9659258262890683122, 1.000000000000000000, 0.9918020599134675930, 0.9875488213027519002 ) ) 
 REPRESENTATION_ITEM ( '' )  );
#1496=CARTESIAN_POINT ( 'NONE',  ( -0.7808398950131225646, -0.05778040916215522460, 0.4822834645669289988 ) ) ;
#1497=CARTESIAN_POINT ( 'NONE',  ( -0.1509186351706028884, -0.08942795157527998196, 0.3641732283464567121 ) ) ;
#1498=CARTESIAN_POINT ( 'NONE',  ( -1.246719160104985846, -0.4281496062992127816, -0.4176697321401328100 ) ) ;
#1499=CARTESIAN_POINT ( 'NONE',  ( 0.8595800524934390507, -0.2845877964562159024, 0.3641732283464567677 ) ) ;
#1500=CARTESIAN_POINT ( 'NONE',  ( -0.7480314960629914633, 0.1771653543307087630, 0.000000000000000000 ) ) ;
#1501=CARTESIAN_POINT ( 'NONE',  ( -1.056430446194224881, 0.2952755905511810774, -0.1292274648535930714 ) ) ;
#1502=CARTESIAN_POINT ( 'NONE',  ( -0.9776902887139098386, -0.6692913385826771977, 0.1292274648535927661 ) ) ;
#1503=CARTESIAN_POINT ( 'NONE',  ( -1.620734908136482577, 0.2952755905511811885, 0.1292274648535926551 ) ) ;
#1505=CARTESIAN_POINT ( 'NONE',  ( 0.8989501312335964611, 0.1771653543307087630, 0.09757992244046791164 ) ) ;
#1506=CARTESIAN_POINT ( 'NONE',  ( 0.3477690288713918276, -0.6692913385826773087, -0.1292274648535924053 ) ) ;
#1507=CARTESIAN_POINT ( 'NONE',  ( -1.482939632545930975, 0.05413385826771666132, 0.4176697321401328100 ) ) ;
#1508=CARTESIAN_POINT ( 'NONE',  ( -1.666666666666665853, 0.05413385826771626580, -0.4176697321401330321 ) ) ;
#1511=CARTESIAN_POINT ( 'NONE',  ( -1.437007874015747477, 0.07958543189024071263, -0.2665933059059888421 ) ) ;
#1512=CARTESIAN_POINT ( 'NONE',  ( -0.4330708661417315697, -0.6692913385826771977, 8.415575281601705876E-17 ) ) ;
#1513=CARTESIAN_POINT ( 'NONE',  ( 0.7742782152230978099, -0.4281496062992124485, 0.4176697321401328655 ) ) ;
#1514=CARTESIAN_POINT ( 'NONE',  ( -1.443569553805773564, -0.5023911411419708095, 0.1820866141732285504 ) ) ;
#1516=CARTESIAN_POINT ( 'NONE',  ( -1.299212598425196097, -0.6692913385826771977, 8.415575281601705876E-17 ) ) ;
#1517=CARTESIAN_POINT ( 'NONE',  ( 1.010498687664042716, -0.4281496062992124485, 0.4176697321401328655 ) ) ;
#1518=CARTESIAN_POINT ( 'NONE',  ( 0.6299212598425204535, -0.1870078740157480879, -0.4822834645669291653 ) ) ;
#1519=CARTESIAN_POINT ( 'NONE',  ( 1.076115485564305141, -0.6046776061558807314, 0.2411417322834647770 ) ) ;
#1524=CARTESIAN_POINT ( 'NONE',  ( 0.4265091863517067039, -0.5511811023622048555, -0.09757992244046775898 ) ) ;
#1525=CARTESIAN_POINT ( 'NONE',  ( 0.1968503937007881344, 0.2952755905511811885, 0.000000000000000000 ) ) ;
#1526=CARTESIAN_POINT ( 'NONE',  ( 1.299212598425197429, 0.2952755905511811885, 0.000000000000000000 ) ) ;
#1528=CARTESIAN_POINT ( 'NONE',  ( 0.1771653543307093182, -0.4536011799217368745, -0.2665933059059886201 ) ) ;
#1529=CARTESIAN_POINT ( 'NONE',  ( -0.7874015748031489847, -0.1870078740157480879, -0.4822834645669291653 ) ) ;
#1530=CARTESIAN_POINT ( 'NONE',  ( 1.568241469816273437, -0.3162353388693405765, 0.4822834645669290543 ) ) ;
#1531=CARTESIAN_POINT ( 'NONE',  ( 0.3477690288713918276, -0.6692913385826773087, -0.1292274648535924053 ) ) ;
#1533=CARTESIAN_POINT ( 'NONE',  ( -0.7137454485294953965, 2.244094488188976388, -0.4917280318828581298 ) ) ;
#1536=CARTESIAN_POINT ( 'NONE',  ( 1.555118110236221041, -0.4536011799217367080, 0.2665933059059888421 ) ) ;
#1537=CARTESIAN_POINT ( 'NONE',  ( -1.154855643044618851, 0.1283753931104748280, 0.1820866141732283561 ) ) ;
#1538=CARTESIAN_POINT ( 'NONE',  ( -1.167979002624671470, 0.05413385826771666132, 0.4176697321401328100 ) ) ;
#1541=CARTESIAN_POINT ( 'NONE',  ( -1.541994750656167090, -0.5511811023622048555, -0.09757992244046775898 ) ) ;
#1543=CARTESIAN_POINT ( 'NONE',  ( -1.233595800524933894, 0.2306618581243848609, 0.2411417322834645549 ) ) ;
#1544=CARTESIAN_POINT ( 'NONE',  ( 0.2624671916010504757, -0.6046776061558809534, -0.2411417322834644161 ) ) ;
#1545=CARTESIAN_POINT ( 'NONE',  ( -1.469816272965878357, 0.2306618581243848609, 0.2411417322834645549 ) ) ;
#1548=CARTESIAN_POINT ( 'NONE',  ( 0.8070866141732288002, 0.1660481256975885056, 0.3530559997133364547 ) ) ;
#1550=CARTESIAN_POINT ( 'NONE',  ( -1.371391076115484609, -0.5511811023622046335, 0.09757992244046803654 ) ) ;
#1554=CARTESIAN_POINT ( 'NONE',  ( -1.587926509186350810, -0.3690944881889763329, 0.3153832671262228327 ) ) ;
#1555=CARTESIAN_POINT ( 'NONE',  ( -1.089238845144356427, 0.05413385826771666132, 0.4176697321401328100 ) ) ;
#1556=CARTESIAN_POINT ( 'NONE',  ( -1.384514435695537005, -0.6692913385826773087, -0.1292274648535924053 ) ) ;
#1558=CARTESIAN_POINT ( 'NONE',  ( -1.476377952755905110, -0.5400638737290845981, -0.3530559997133363437 ) ) ;
#1560=CARTESIAN_POINT ( 'NONE',  ( -1.423884514435694859, -0.05778040916215560624, -0.4822834645669293319 ) ) ;
#1561=CARTESIAN_POINT ( 'NONE',  ( -0.5411721830064186722, -2.191421614605370878E-15, 0.4445507791589071167 ) ) ;
#1563=EDGE_CURVE ( 'NONE', #58566, #38771, #73019, .T. ) ;
#1564=CARTESIAN_POINT ( 'NONE',  ( 0.2427821522309719648, -0.08942795157527998196, 0.3641732283464567121 ) ) ;
#1567=CARTESIAN_POINT ( 'NONE',  ( -0.5314960629921254842, -0.4536011799217368745, -0.2665933059059886201 ) ) ;
#1568=CARTESIAN_POINT ( 'NONE',  ( -0.6496062992125976043, 0.1660481256975883668, -0.3530559997133364547 ) ) ;
#1569=CARTESIAN_POINT ( 'NONE',  ( 1.082677165354331228, -0.5400638737290844871, 0.3530559997133364547 ) ) ;
#1570=CARTESIAN_POINT ( 'NONE',  ( -0.8989501312335946848, -0.6692913385826771977, 0.1292274648535927661 ) ) ;
#1573=CARTESIAN_POINT ( 'NONE',  ( -1.023622047244093558, -0.1870078740157479769, 0.4822834645669291653 ) ) ;
#1574=CARTESIAN_POINT ( 'NONE',  ( 0.6889763779527563470, 0.1660481256975883668, -0.3530559997133364547 ) ) ;
#1575=CARTESIAN_POINT ( 'NONE',  ( -1.581364829396324945, -0.2845877964562159024, 0.3641732283464567677 ) ) ;
#1576=CARTESIAN_POINT ( 'NONE',  ( -1.607611548556429737, -0.6692913385826771977, 0.1292274648535927661 ) ) ;
#1581=CARTESIAN_POINT ( 'NONE',  ( -0.3871391076115476282, -0.05778040916215522460, 0.4822834645669289988 ) ) ;
#1582=CARTESIAN_POINT ( 'NONE',  ( -1.384514435695537005, -0.5511811023622048555, -0.09757992244046775898 ) ) ;
#1584=CARTESIAN_POINT ( 'NONE',  ( -1.489501312335957062, -0.3162353388693409650, -0.4822834645669289433 ) ) ;
#1586=CARTESIAN_POINT ( 'NONE',  ( -1.594488188976377563, -0.5400638737290844871, 0.3530559997133364547 ) ) ;
#1587=CARTESIAN_POINT ( 'NONE',  ( -0.5118110236220466680, -0.6692913385826771977, 8.415575281601705876E-17 ) ) ;
#1589=CARTESIAN_POINT ( 'NONE',  ( 0.5380577427821529035, -0.004921259842519870586, -0.3153832671262229437 ) ) ;
#1591=CARTESIAN_POINT ( 'NONE',  ( 0.1640419947506569498, -0.2845877964562161244, -0.3641732283464567121 ) ) ;
#1592=CARTESIAN_POINT ( 'NONE',  ( 1.161417322834646271, 0.07958543189024071263, -0.2665933059059888421 ) ) ;
#1593=CARTESIAN_POINT ( 'NONE',  ( 0.8661417322834652488, -0.1870078740157480879, -0.4822834645669291653 ) ) ;
#1594=CARTESIAN_POINT ( 'NONE',  ( 0.1443569553805781891, -0.004921259842519870586, -0.3153832671262229437 ) ) ;
#1596=CARTESIAN_POINT ( 'NONE',  ( -1.279527559055116948, 0.1660481256975883668, -0.3530559997133364547 ) ) ;
#1597=CARTESIAN_POINT ( 'NONE',  ( -0.2230971128608915943, -0.3690944881889765550, -0.3153832671262227771 ) ) ;
#1599=CARTESIAN_POINT ( 'NONE',  ( -0.3477690288713902178, 0.1771653543307087075, -0.09757992244046823083 ) ) ;
#1600=CARTESIAN_POINT ( 'NONE',  ( 0.01968503937007957949, -0.5400638737290845981, -0.3530559997133363437 ) ) ;
#1602=CARTESIAN_POINT ( 'NONE',  ( 1.049868766404200127, -0.5023911411419708095, -0.1820866141732282451 ) ) ;
#1603=CARTESIAN_POINT ( 'NONE',  ( -0.3083989501312330295, -0.08942795157527998196, 0.3641732283464567121 ) ) ;
#1604=CARTESIAN_POINT ( 'NONE',  ( -0.1115485564304453947, -0.6692913385826771977, 0.1292274648535927661 ) ) ;
#1606=CARTESIAN_POINT ( 'NONE',  ( -1.305774278215222184, 0.1771653543307087630, 0.09757992244046791164 ) ) ;
#1608=CARTESIAN_POINT ( 'NONE',  ( 0.6955380577427828781, -0.4281496062992124485, 0.4176697321401328655 ) ) ;
#1609=CARTESIAN_POINT ( 'NONE',  ( -0.7808398950131222316, -0.3162353388693409650, -0.4822834645669289433 ) ) ;
#1612=CARTESIAN_POINT ( 'NONE',  ( 0.3215223097112867578, -0.08942795157527998196, 0.3641732283464567121 ) ) ;
#1613=CARTESIAN_POINT ( 'NONE',  ( -0.9908136482939626788, 0.2952755905511811885, 0.1292274648535926551 ) ) ;
#1614=CARTESIAN_POINT ( 'NONE',  ( -1.161417322834644716, 0.1660481256975885056, 0.3530559997133364547 ) ) ;
#1615=CARTESIAN_POINT ( 'NONE',  ( -1.135170603674539924, 0.1771653543307087075, -0.09757992244046823083 ) ) ;
#1616=CARTESIAN_POINT ( 'NONE',  ( 1.594488188976378673, -0.5400638737290845981, -0.3530559997133363437 ) ) ;
#1617=CARTESIAN_POINT ( 'NONE',  ( -0.8005249343832011588, -0.004921259842519870586, -0.3153832671262229437 ) ) ;
#1619=CARTESIAN_POINT ( 'NONE',  ( 0.6758530183727039509, 0.2952755905511810774, -0.1292274648535930714 ) ) ;
#1623=CARTESIAN_POINT ( 'NONE',  ( -1.594488188976377563, -0.5400638737290844871, 0.3530559997133364547 ) ) ;
#1624=CARTESIAN_POINT ( 'NONE',  ( -1.286089238845143479, -0.6046776061558807314, 0.2411417322834647770 ) ) ;
#1625=CARTESIAN_POINT ( 'NONE',  ( 1.043307086614173818, -0.5400638737290845981, -0.3530559997133363437 ) ) ;
#1628=CARTESIAN_POINT ( 'NONE',  ( 0.4068241469816281097, 0.05413385826771666132, 0.4176697321401328100 ) ) ;
#1629=CARTESIAN_POINT ( 'NONE',  ( -0.5446194225721777693, -0.05778040916215522460, 0.4822834645669289988 ) ) ;
#1632=CARTESIAN_POINT ( 'NONE',  ( 0.6036745406824153282, -0.5023911411419708095, 0.1820866141732285504 ) ) ;
#1637=CARTESIAN_POINT ( 'NONE',  ( -0.05249343832020938322, -0.6046776061558809534, -0.2411417322834644161 ) ) ;
#1639=CARTESIAN_POINT ( 'NONE',  ( 1.286089238845145033, 0.2306618581243848609, 0.2411417322834645549 ) ) ;
#1640=CARTESIAN_POINT ( 'NONE',  ( 0.3608923884514443348, -0.6692913385826771977, 0.1292274648535927661 ) ) ;
#1641=CARTESIAN_POINT ( 'NONE',  ( -0.2427821522309703550, -0.2845877964562159024, 0.3641732283464567677 ) ) ;
#1642=CARTESIAN_POINT ( 'NONE',  ( 1.128608923884515169, -0.6046776061558809534, -0.2411417322834644161 ) ) ;
#1643=CARTESIAN_POINT ( 'NONE',  ( -0.4986876640419939388, 0.2306618581243847221, -0.2411417322834647770 ) ) ;
#1644=CARTESIAN_POINT ( 'NONE',  ( -0.1443569553805768291, 0.05413385826771666132, 0.4176697321401328100 ) ) ;
#1645=CARTESIAN_POINT ( 'NONE',  ( -1.646981627296586703, -0.05778040916215522460, 0.4822834645669289988 ) ) ;
#1646=CONICAL_SURFACE ( 'NONE', #8374, 1.220472440944881942, 0.7853981633974621568 ) ;
#1647=CARTESIAN_POINT ( 'NONE',  ( 0.7152230971128614723, -0.3162353388693409650, -0.4822834645669289433 ) ) ;
#1648=CARTESIAN_POINT ( 'NONE',  ( 1.286089238845145033, -0.6046776061558809534, -0.2411417322834644161 ) ) ;
#1650=CARTESIAN_POINT ( 'NONE',  ( 0.4986876640419954376, -0.5023911411419708095, -0.1820866141732282451 ) ) ;
#1651=VERTEX_POINT ( 'NONE', #1773 ) ;
#1654=CARTESIAN_POINT ( 'NONE',  ( -0.6233595800524928121, -0.08942795157527998196, 0.3641732283464567121 ) ) ;
#1655=CARTESIAN_POINT ( 'NONE',  ( -0.2493438320209966919, -0.4281496062992124485, 0.4176697321401328655 ) ) ;
#1657=CARTESIAN_POINT ( 'NONE',  ( -0.2887139107611542133, 0.2306618581243848609, 0.2411417322834645549 ) ) ;
#1658=CARTESIAN_POINT ( 'NONE',  ( -0.07874015748031421014, -0.1870078740157480879, -0.4822834645669291653 ) ) ;
#1659=CARTESIAN_POINT ( 'NONE',  ( -0.9711286089238838626, 0.2306618581243847221, -0.2411417322834647770 ) ) ;
#1660=CARTESIAN_POINT ( 'NONE',  ( -1.108923884514435132, -0.3162353388693405765, 0.4822834645669290543 ) ) ;
#1661=CARTESIAN_POINT ( 'NONE',  ( 1.286089238845145033, -0.5023911411419708095, -0.1820866141732282451 ) ) ;
#1663=CARTESIAN_POINT ( 'NONE',  ( -0.1450607720586916394, 0.000000000000000000, 0.3464511005275205946 ) ) ;
#1664=CARTESIAN_POINT ( 'NONE',  ( 0.8464566929133865436, 0.07958543189024071263, -0.2665933059059888421 ) ) ;
#1665=CARTESIAN_POINT ( 'NONE',  ( 0.2952755905511819101, 0.1660481256975883668, -0.3530559997133364547 ) ) ;
#1666=CARTESIAN_POINT ( 'NONE',  ( 0.2559055118110243332, 0.1660481256975885056, 0.3530559997133364547 ) ) ;
#1668=CARTESIAN_POINT ( 'NONE',  ( 0.6492324815748310440, 2.230753248847788139, 0.2292861212309488528 ) ) ;
#1671=CARTESIAN_POINT ( 'NONE',  ( -0.7283464566929126471, 0.1660481256975883668, -0.3530559997133364547 ) ) ;
#1674=CARTESIAN_POINT ( 'NONE',  ( -1.266404199475064773, -0.08942795157528024563, -0.3641732283464568787 ) ) ;
#1675=CARTESIAN_POINT ( 'NONE',  ( 0.9580052493438326877, 0.05413385826771666132, 0.4176697321401328100 ) ) ;
#1676=CARTESIAN_POINT ( 'NONE',  ( 0.9383202099737538715, -0.05778040916215560624, -0.4822834645669293319 ) ) ;
#1677=CARTESIAN_POINT ( 'NONE',  ( -0.1443569553805765515, -0.3690944881889765550, -0.3153832671262227771 ) ) ;
#1678=CARTESIAN_POINT ( 'NONE',  ( 0.3871391076115492380, -0.05778040916215560624, -0.4822834645669293319 ) ) ;
#1680=CARTESIAN_POINT ( 'NONE',  ( -0.03280839895013062252, 0.1771653543307087075, -0.09757992244046823083 ) ) ;
#1681=CARTESIAN_POINT ( 'NONE',  ( 0.1115485564304467270, -0.6692913385826773087, -0.1292274648535924053 ) ) ;
#1683=CARTESIAN_POINT ( 'NONE',  ( -1.646981627296586703, -0.3162353388693409650, -0.4822834645669289433 ) ) ;
#1684=CARTESIAN_POINT ( 'NONE',  ( 0.4002624671916016896, -0.2845877964562161244, -0.3641732283464567121 ) ) ;
#1685=CARTESIAN_POINT ( 'NONE',  ( 1.535433070866142558, 0.1771653543307087630, 0.000000000000000000 ) ) ;
#1686=CARTESIAN_POINT ( 'NONE',  ( -0.9055118110236215490, 0.2952755905511811885, 0.000000000000000000 ) ) ;
#1687=EDGE_CURVE ( 'NONE', #58735, #20676, #8090, .T. ) ;
#1688=CARTESIAN_POINT ( 'NONE',  ( -0.1706036745406816491, -0.004921259842519870586, -0.3153832671262229437 ) ) ;
#1690=CARTESIAN_POINT ( 'NONE',  ( -0.6692913385826764205, -0.6692913385826771977, 8.415575281601705876E-17 ) ) ;
#1691=CARTESIAN_POINT ( 'NONE',  ( -0.5314960629921250401, 0.1660481256975885056, 0.3530559997133364547 ) ) ;
#1692=CARTESIAN_POINT ( 'NONE',  ( -0.04593175853018302557, 0.2952755905511811885, 0.1292274648535926551 ) ) ;
#1695=CARTESIAN_POINT ( 'NONE',  ( -1.541994750656167090, 0.1771653543307087630, 0.09757992244046791164 ) ) ;
#1696=CARTESIAN_POINT ( 'NONE',  ( 0.9120734908136490793, 0.1771653543307087075, -0.09757992244046823083 ) ) ;
#1697=CARTESIAN_POINT ( 'NONE',  ( 1.338582677165355062, -0.1870078740157480879, -0.4822834645669291653 ) ) ;
#1698=CARTESIAN_POINT ( 'NONE',  ( -0.6167979002624665030, -0.004921259842519576551, 0.3153832671262227771 ) ) ;
#1699=CARTESIAN_POINT ( 'NONE',  ( -1.240157480314959759, 0.07958543189024085140, 0.2665933059059887866 ) ) ;
#1701=CARTESIAN_POINT ( 'NONE',  ( -0.6824146981627291497, -0.6046776061558809534, -0.2411417322834644161 ) ) ;
#1702=CARTESIAN_POINT ( 'NONE',  ( 0.4396325459317593221, 0.1771653543307087075, -0.09757992244046823083 ) ) ;
#1704=CARTESIAN_POINT ( 'NONE',  ( 0.9908136482939640111, 0.1771653543307087075, -0.09757992244046823083 ) ) ;
#1706=CARTESIAN_POINT ( 'NONE',  ( 0.5314960629921267055, -0.5400638737290844871, 0.3530559997133364547 ) ) ;
#1709=CARTESIAN_POINT ( 'NONE',  ( -0.4790026246719154557, -0.3162353388693405765, 0.4822834645669290543 ) ) ;
#1711=CARTESIAN_POINT ( 'NONE',  ( 1.345144356955381593, -0.2845877964562161244, -0.3641732283464567121 ) ) ;
#1712=CARTESIAN_POINT ( 'NONE',  ( 0.6496062992125991586, -0.5400638737290845981, -0.3530559997133363437 ) ) ;
#1713=CARTESIAN_POINT ( 'NONE',  ( 0.1837270341207357105, -0.6046776061558809534, -0.2411417322834644161 ) ) ;
#1714=CARTESIAN_POINT ( 'NONE',  ( -0.05249343832020911260, 0.1283753931104748280, 0.1820866141732283561 ) ) ;
#1715=CARTESIAN_POINT ( 'NONE',  ( 1.113858370737683456, -1.206088964116209378E-16, 0.3791475997938230647 ) ) ;
#1716=CARTESIAN_POINT ( 'NONE',  ( -0.1968503937007867743, 0.1771653543307087630, 0.000000000000000000 ) ) ;
#1717=CARTESIAN_POINT ( 'NONE',  ( 0.8136482939632553313, -0.6046776061558809534, -0.2411417322834644161 ) ) ;
#1718=CARTESIAN_POINT ( 'NONE',  ( -0.7939632545931754048, -0.2845877964562159024, 0.3641732283464567677 ) ) ;
#1719=CARTESIAN_POINT ( 'NONE',  ( -1.095800524934382292, -0.3162353388693409650, -0.4822834645669289433 ) ) ;
#1720=FACE_OUTER_BOUND ( 'NONE', #59119, .T. ) ;
#1721=ORIENTED_EDGE ( 'NONE', *, *, #46438, .T. ) ;
#1722=CARTESIAN_POINT ( 'NONE',  ( -1.345144356955379816, -0.3162353388693405765, 0.4822834645669290543 ) ) ;
#1723=CARTESIAN_POINT ( 'NONE',  ( -1.076115485564303809, 0.1283753931104748280, 0.1820866141732283561 ) ) ;
#1724=CARTESIAN_POINT ( 'NONE',  ( -0.1377952755905504645, 0.1660481256975885056, 0.3530559997133364547 ) ) ;
#1725=CARTESIAN_POINT ( 'NONE',  ( -1.732283464566928277, -0.1870078740157479769, 0.4822834645669291653 ) ) ;
#1726=CARTESIAN_POINT ( 'NONE',  ( -0.7545931758530176614, -0.6692913385826773087, -0.1292274648535924053 ) ) ;
#1728=FACE_OUTER_BOUND ( 'NONE', #20258, .T. ) ;
#1729=CARTESIAN_POINT ( 'NONE',  ( 1.679790026246720025, 0.2306618581243848609, 0.2411417322834645549 ) ) ;
#1730=CARTESIAN_POINT ( 'NONE',  ( 0.9317585301837276734, -0.4281496062992124485, 0.4176697321401328655 ) ) ;
#1731=CARTESIAN_POINT ( 'NONE',  ( 0.9842519685039378130, -0.6692913385826771977, 8.415575281601705876E-17 ) ) ;
#1734=CARTESIAN_POINT ( 'NONE',  ( -1.364829396325458521, 0.2306618581243847221, -0.2411417322834647770 ) ) ;
#1737=CARTESIAN_POINT ( 'NONE',  ( -0.5380577427821514602, -0.004921259842519576551, 0.3153832671262227771 ) ) ;
#1739=ORIENTED_EDGE ( 'NONE', *, *, #20141, .T. ) ;
#1740=CARTESIAN_POINT ( 'NONE',  ( 0.4133858267716541968, -0.5400638737290845981, -0.3530559997133363437 ) ) ;
#1741=CARTESIAN_POINT ( 'NONE',  ( -0.03937007874015669567, -0.6692913385826771977, 8.415575281601705876E-17 ) ) ;
#1742=CARTESIAN_POINT ( 'NONE',  ( -0.7414698162729651543, -0.6692913385826771977, 0.1292274648535927661 ) ) ;
#1743=CARTESIAN_POINT ( 'NONE',  ( 1.437007874015748810, -0.5400638737290845981, -0.3530559997133363437 ) ) ;
#1744=CARTESIAN_POINT ( 'NONE',  ( -1.023622047244093558, -0.1870078740157479769, 0.3641732283464567677 ) ) ;
#1746=CARTESIAN_POINT ( 'NONE',  ( 0.8136482939632553313, -0.6046776061558809534, -0.2411417322834644161 ) ) ;
#1747=CARTESIAN_POINT ( 'NONE',  ( 0.5314960629921264834, 0.07958543189024071263, -0.2665933059059888421 ) ) ;
#1748=CARTESIAN_POINT ( 'NONE',  ( -0.3280839895013117347, 0.05413385826771626580, -0.4176697321401330321 ) ) ;
#1750=CARTESIAN_POINT ( 'NONE',  ( -0.6364829396325453192, -0.05778040916215560624, -0.4822834645669293319 ) ) ;
#1751=CARTESIAN_POINT ( 'NONE',  ( -1.640419947506561060, -0.3690944881889765550, -0.3153832671262227771 ) ) ;
#1752=CARTESIAN_POINT ( 'NONE',  ( 1.555118110236221041, 0.1660481256975883668, -0.3530559997133364547 ) ) ;
#1754=VERTEX_POINT ( 'NONE', #46787 ) ;
#1756=CARTESIAN_POINT ( 'NONE',  ( 0.02624671916010564918, -0.6046776061558809534, -0.2411417322834644161 ) ) ;
#1757=VERTEX_POINT ( 'NONE', #65338 ) ;
#1758=CARTESIAN_POINT ( 'NONE',  ( -1.377952755905511140, 0.2952755905511811885, 0.000000000000000000 ) ) ;
#1759=CARTESIAN_POINT ( 'NONE',  ( 1.030183727034121421, -0.3162353388693409650, -0.4822834645669289433 ) ) ;
#1760=CARTESIAN_POINT ( 'NONE',  ( 1.463254593175853824, 0.2952755905511810774, -0.1292274648535930714 ) ) ;
#1761=CARTESIAN_POINT ( 'NONE',  ( 0.3937007874015754361, -0.1870078740157480879, -0.4822834645669291653 ) ) ;
#1762=CARTESIAN_POINT ( 'NONE',  ( -0.4724409448818890911, -0.1870078740157480879, -0.4822834645669291653 ) ) ;
#1764=CARTESIAN_POINT ( 'NONE',  ( -1.233595800524933894, 0.2306618581243848609, 0.2411417322834645549 ) ) ;
#1765=CARTESIAN_POINT ( 'NONE',  ( -0.4855643044619415427, 0.05413385826771626580, -0.4176697321401330321 ) ) ;
#1766=CARTESIAN_POINT ( 'NONE',  ( -0.5183727034120726440, 0.1771653543307087630, 0.09757992244046791164 ) ) ;
#1768=CARTESIAN_POINT ( 'NONE',  ( -0.6889763779527552368, -0.5400638737290845981, -0.3530559997133363437 ) ) ;
#1771=CARTESIAN_POINT ( 'NONE',  ( 0.5774278215223103139, -0.6046776061558809534, -0.2411417322834644161 ) ) ;
#1773=CARTESIAN_POINT ( 'NONE',  ( -0.8761506516392493227, -2.567464376874931580E-15, -0.4445507791589072832 ) ) ;
#1774=CARTESIAN_POINT ( 'NONE',  ( 0.05905511811023709395, -0.5400638737290844871, 0.3530559997133364547 ) ) ;
#1775=CARTESIAN_POINT ( 'NONE',  ( 0.8398950131233602345, -0.5023911411419708095, 0.1820866141732285504 ) ) ;
#1778=CARTESIAN_POINT ( 'NONE',  ( 1.194225721784777594, -0.004921259842519576551, 0.3153832671262227771 ) ) ;
#1779=CARTESIAN_POINT ( 'NONE',  ( 1.384514435695538337, -0.6692913385826771977, 0.1292274648535927661 ) ) ;
#1781=CARTESIAN_POINT ( 'NONE',  ( 0.1246719160104994284, -0.6692913385826771977, 0.1292274648535927661 ) ) ;
#1783=CARTESIAN_POINT ( 'NONE',  ( -1.377952755905511140, 0.2952755905511811885, 0.000000000000000000 ) ) ;
#1784=CARTESIAN_POINT ( 'NONE',  ( -0.03280839895013062252, -0.6692913385826771977, 0.1292274648535927661 ) ) ;
#1786=CARTESIAN_POINT ( 'NONE',  ( 1.213910761154856299, 0.2952755905511811885, 0.1292274648535926551 ) ) ;
#1787=CARTESIAN_POINT ( 'NONE',  ( 0.4068241469816279987, -0.4281496062992127816, -0.4176697321401328100 ) ) ;
#1788=CARTESIAN_POINT ( 'NONE',  ( 0.9514435695538062676, -0.2845877964562161244, -0.3641732283464567121 ) ) ;
#1789=FACE_OUTER_BOUND ( 'NONE', #58870, .T. ) ;
#1790=CARTESIAN_POINT ( 'NONE',  ( 0.3215223097112867578, -0.2845877964562161244, -0.3641732283464567121 ) ) ;
#1791=CARTESIAN_POINT ( 'NONE',  ( -1.437007874015747477, 0.1660481256975883668, -0.3530559997133364547 ) ) ;
#1793=CARTESIAN_POINT ( 'NONE',  ( 1.154855643044620184, -0.6046776061558807314, 0.2411417322834647770 ) ) ;
#1795=CARTESIAN_POINT ( 'NONE',  ( 0.4986876640419954376, -0.6046776061558809534, -0.2411417322834644161 ) ) ;
#1796=CARTESIAN_POINT ( 'NONE',  ( 0.9186351706036752773, 0.2306618581243847221, -0.2411417322834647770 ) ) ;
#1798=CARTESIAN_POINT ( 'NONE',  ( 0.3280839895013130669, -0.004921259842519576551, 0.3153832671262227771 ) ) ;
#1799=CARTESIAN_POINT ( 'NONE',  ( 0.3871391076115493490, -0.3162353388693405765, 0.4822834645669290543 ) ) ;
#1800=CARTESIAN_POINT ( 'NONE',  ( 0.7749820319012125092, 2.784432375088962958E-17, -0.3464511005275205946 ) ) ;
#1801=CARTESIAN_POINT ( 'NONE',  ( -1.003937007874015297, -0.4536011799217368745, -0.2665933059059886201 ) ) ;
#1802=CARTESIAN_POINT ( 'NONE',  ( -0.8989501312335946848, 0.2952755905511810774, -0.1292274648535930714 ) ) ;
#1804=CARTESIAN_POINT ( 'NONE',  ( -1.391076115485563758, 0.2306618581243848609, 0.2411417322834645549 ) ) ;
#1805=CARTESIAN_POINT ( 'NONE',  ( 0.4527559055118117182, 0.1660481256975883668, -0.3530559997133364547 ) ) ;
#1806=CARTESIAN_POINT ( 'NONE',  ( 1.587926509186352586, -0.4281496062992127816, -0.4176697321401328100 ) ) ;
#1808=CARTESIAN_POINT ( 'NONE',  ( 0.6036745406824153282, -0.6046776061558807314, 0.2411417322834647770 ) ) ;
#1810=FACE_OUTER_BOUND ( 'NONE', #51817, .T. ) ;
#1811=CARTESIAN_POINT ( 'NONE',  ( 1.555118110236221041, 0.1660481256975883668, -0.3530559997133364547 ) ) ;
#1812=CARTESIAN_POINT ( 'NONE',  ( -1.476377952755905110, -0.4536011799217368745, -0.2665933059059886201 ) ) ;
#1813=CARTESIAN_POINT ( 'NONE',  ( 1.010498687664042716, -0.3690944881889763329, 0.3153832671262228327 ) ) ;
#1814=CARTESIAN_POINT ( 'NONE',  ( -1.305774278215222184, 0.1771653543307087630, 0.09757992244046791164 ) ) ;
#1815=CARTESIAN_POINT ( 'NONE',  ( -0.6955380577427815458, -0.004921259842519576551, 0.3153832671262227771 ) ) ;
#1817=CARTESIAN_POINT ( 'NONE',  ( 0.5249343832021003964, 0.1283753931104746893, -0.1820866141732285504 ) ) ;
#1819=CARTESIAN_POINT ( 'NONE',  ( 0.4068241469816281097, 0.05413385826771666132, 0.4176697321401328100 ) ) ;
#1820=CARTESIAN_POINT ( 'NONE',  ( 1.220472440944882386, -0.6692913385826771977, 8.415575281601705876E-17 ) ) ;
#1821=ADVANCED_FACE ( 'NONE', ( #64482 ), #46366, .F. ) ;
#1822=CARTESIAN_POINT ( 'NONE',  ( 0.1377952755905518800, 0.1660481256975883668, -0.3530559997133364547 ) ) ;
#1823=CARTESIAN_POINT ( 'NONE',  ( 0.03937007874015806264, 0.1771653543307087630, 0.000000000000000000 ) ) ;
#1824=CARTESIAN_POINT ( 'NONE',  ( 1.272965879265092637, 0.05413385826771666132, 0.4176697321401328100 ) ) ;
#1825=CARTESIAN_POINT ( 'NONE',  ( -0.1702530392988850783, 0.004960608223778509643, -0.3437734562760191848 ) ) ;
#1826=CARTESIAN_POINT ( 'NONE',  ( -0.9251968503937002541, 0.1660481256975885056, 0.3530559997133364547 ) ) ;
#1828=CARTESIAN_POINT ( 'NONE',  ( 2.795275590551181466, 1.968503937007874960, 0.000000000000000000 ) ) ;
#1829=CARTESIAN_POINT ( 'NONE',  ( -0.006561679790025524116, -0.3162353388693405765, 0.4822834645669290543 ) ) ;
#1830=CARTESIAN_POINT ( 'NONE',  ( -0.9908136482939626788, 0.2952755905511811885, 0.1292274648535926551 ) ) ;
#1831=CARTESIAN_POINT ( 'NONE',  ( 0.03937007874015806264, 0.2952755905511811885, 0.000000000000000000 ) ) ;
#1838=CARTESIAN_POINT ( 'NONE',  ( -1.377952755905511140, 0.1771653543307087630, 0.000000000000000000 ) ) ;
#1840=CARTESIAN_POINT ( 'NONE',  ( -1.646981627296586703, -0.3162353388693409650, -0.4822834645669289433 ) ) ;
#1842=CARTESIAN_POINT ( 'NONE',  ( 0.4396325459317593221, 0.2952755905511810774, -0.1292274648535930714 ) ) ;
#1843=CARTESIAN_POINT ( 'NONE',  ( -0.5643044619422565855, -0.004921259842519870586, -0.3153832671262229437 ) ) ;
#1844=CARTESIAN_POINT ( 'NONE',  ( 0.8464566929133865436, 0.1660481256975883668, -0.3530559997133364547 ) ) ;
#1845=CARTESIAN_POINT ( 'NONE',  ( 0.2230971128608929543, 0.05413385826771626580, -0.4176697321401330321 ) ) ;
#1849=CARTESIAN_POINT ( 'NONE',  ( 1.371391076115485941, 0.2952755905511811885, 0.1292274648535926551 ) ) ;
#1850=CARTESIAN_POINT ( 'NONE',  ( -0.1246719160104980823, 0.2952755905511811885, 0.1292274648535926551 ) ) ;
#1851=CARTESIAN_POINT ( 'NONE',  ( -1.555118110236219930, -0.5400638737290845981, -0.3530559997133363437 ) ) ;
#1852=CARTESIAN_POINT ( 'NONE',  ( 0.8595800524934390507, -0.3162353388693405765, 0.4822834645669290543 ) ) ;
#1854=CARTESIAN_POINT ( 'NONE',  ( 0.2690288713910767848, -0.6692913385826773087, -0.1292274648535924053 ) ) ;
#1855=CARTESIAN_POINT ( 'NONE',  ( 0.8464566929133866546, -0.5400638737290844871, 0.3530559997133364547 ) ) ;
#1856=CARTESIAN_POINT ( 'NONE',  ( -0.2230971128608915943, 0.05413385826771666132, 0.4176697321401328100 ) ) ;
#1857=CARTESIAN_POINT ( 'NONE',  ( 0.6627296587926517768, -0.5511811023622048555, -0.09757992244046775898 ) ) ;
#1858=CARTESIAN_POINT ( 'NONE',  ( -1.167979002624671470, -0.4281496062992127816, -0.4176697321401328100 ) ) ;
#1859=CARTESIAN_POINT ( 'NONE',  ( -1.279527559055116948, -0.5400638737290844871, 0.3530559997133364547 ) ) ;
#1860=CARTESIAN_POINT ( 'NONE',  ( 0.7545931758530188826, -0.6692913385826771977, 0.1292274648535927661 ) ) ;
#1867=CARTESIAN_POINT ( 'NONE',  ( 1.246719160104987623, 0.05413385826771626580, -0.4176697321401330321 ) ) ;
#1868=CARTESIAN_POINT ( 'NONE',  ( 1.023622047244095112, -0.1870078740157480601, -0.3641732283464567677 ) ) ;
#1873=EDGE_CURVE ( 'NONE', #60349, #22261, #70553, .T. ) ;
#1875=CARTESIAN_POINT ( 'NONE',  ( 1.502624671916010790, -0.3162353388693409650, -0.4822834645669289433 ) ) ;
#1877=CARTESIAN_POINT ( 'NONE',  ( -0.5183727034120726440, -0.6692913385826773087, -0.1292274648535924053 ) ) ;
#1878=CARTESIAN_POINT ( 'NONE',  ( 0.9645669291338588858, 0.1660481256975885056, 0.3530559997133364547 ) ) ;
#1880=CARTESIAN_POINT ( 'NONE',  ( -1.535433070866141225, 0.2952755905511811885, 0.000000000000000000 ) ) ;
#1881=CARTESIAN_POINT ( 'NONE',  ( 0.5027385518326215053, 1.496062992125283708, 0.5309055118110234117 ) ) ;
#1883=CARTESIAN_POINT ( 'NONE',  ( 1.502624671916010790, -0.08942795157527998196, 0.3641732283464567121 ) ) ;
#1884=CARTESIAN_POINT ( 'NONE',  ( -1.603475055217291612, 1.881749232079046097, -0.04573490813648262154 ) ) ;
#1885=CARTESIAN_POINT ( 'NONE',  ( -0.7677165354330699465, -0.4536011799217368745, -0.2665933059059886201 ) ) ;
#1886=CARTESIAN_POINT ( 'NONE',  ( -1.594488188976377119, 0.1660481256975883668, -0.3530559997133364547 ) ) ;
#1887=CARTESIAN_POINT ( 'NONE',  ( 0.4396325459317593221, 0.2952755905511810774, -0.1292274648535930714 ) ) ;
#1889=CARTESIAN_POINT ( 'NONE',  ( 1.502624671916010790, -0.05778040916215522460, 0.4822834645669289988 ) ) ;
#1891=CARTESIAN_POINT ( 'NONE',  ( -0.7677165354330699465, 0.07958543189024085140, 0.2665933059059887866 ) ) ;
#1892=CARTESIAN_POINT ( 'NONE',  ( 0.9186351706036752773, 0.2306618581243847221, -0.2411417322834647770 ) ) ;
#1893=CARTESIAN_POINT ( 'NONE',  ( -1.660104986876639543, -0.05778040916215560624, -0.4822834645669293319 ) ) ;
#1895=CARTESIAN_POINT ( 'NONE',  ( -0.7677165354330699465, 0.07958543189024085140, 0.2665933059059887866 ) ) ;
#1896=CARTESIAN_POINT ( 'NONE',  ( 1.640419947506562393, -0.4281496062992124485, 0.4176697321401328655 ) ) ;
#1898=CARTESIAN_POINT ( 'NONE',  ( 0.5380577427821529035, 0.05413385826771626580, -0.4176697321401330321 ) ) ;
#1899=CARTESIAN_POINT ( 'NONE',  ( -0.9186351706036736120, -0.5023911411419708095, -0.1820866141732282451 ) ) ;
#1900=CARTESIAN_POINT ( 'NONE',  ( -0.4921259842519677963, -0.4536011799217367080, 0.2665933059059888421 ) ) ;
#1901=CARTESIAN_POINT ( 'NONE',  ( -0.2427821522309703550, -0.05778040916215560624, -0.4822834645669293319 ) ) ;
#1902=CARTESIAN_POINT ( 'NONE',  ( -1.220472440944881054, -0.5511811023622047445, 6.969142054262312111E-17 ) ) ;
#1904=CARTESIAN_POINT ( 'NONE',  ( 0.6299212598425204535, -0.1870078740157479769, 0.4822834645669291653 ) ) ;
#1905=CARTESIAN_POINT ( 'NONE',  ( 0.8772393894194432384, 4.512065407040659715E-16, 0.3954985857520057491 ) ) ;
#1907=CARTESIAN_POINT ( 'NONE',  ( -0.8595800524934373854, -0.3162353388693409650, -0.4822834645669289433 ) ) ;
#1908=CARTESIAN_POINT ( 'NONE',  ( -0.08530183727034056085, -0.08942795157528024563, -0.3641732283464568787 ) ) ;
#1909=CARTESIAN_POINT ( 'NONE',  ( -1.364829396325458521, -0.6046776061558807314, 0.2411417322834647770 ) ) ;
#1910=CARTESIAN_POINT ( 'NONE',  ( 1.030183727034121421, -0.08942795157527998196, 0.3641732283464567121 ) ) ;
#1911=CARTESIAN_POINT ( 'NONE',  ( -0.6036745406824141069, 0.1283753931104748280, 0.1820866141732283561 ) ) ;
#1912=CARTESIAN_POINT ( 'NONE',  ( -1.115485564304461219, -0.4281496062992124485, 0.4176697321401328655 ) ) ;
#1913=CARTESIAN_POINT ( 'NONE',  ( -1.502624671916009680, -0.05778040916215560624, -0.4822834645669293319 ) ) ;
#1914=CARTESIAN_POINT ( 'NONE',  ( -1.587926509186350810, 0.05413385826771626580, -0.4176697321401330321 ) ) ;
#1916=CARTESIAN_POINT ( 'NONE',  ( 0.8923884514435703741, 0.1283753931104748280, 0.1820866141732283561 ) ) ;
#1917=VECTOR ( 'NONE', #49053, 39.37007874015748854 ) ;
#1918=CARTESIAN_POINT ( 'NONE',  ( 0.5643044619422579178, 0.05413385826771666132, 0.4176697321401328100 ) ) ;
#1919=CARTESIAN_POINT ( 'NONE',  ( -1.568241469816272105, -0.3162353388693409650, -0.4822834645669289433 ) ) ;
#1920=CARTESIAN_POINT ( 'NONE',  ( 1.299212598425197429, 0.1771653543307087630, 0.000000000000000000 ) ) ;
#1923=CARTESIAN_POINT ( 'NONE',  ( -1.318897637795274802, 0.07958543189024085140, 0.2665933059059887866 ) ) ;
#1924=CARTESIAN_POINT ( 'NONE',  ( -0.5905511811023613777, -0.6692913385826771977, 8.415575281601705876E-17 ) ) ;
#1925=CARTESIAN_POINT ( 'NONE',  ( 0.3805774278215230400, 0.05413385826771626580, -0.4176697321401330321 ) ) ;
#1926=CARTESIAN_POINT ( 'NONE',  ( -1.555118110236219930, 0.07958543189024085140, 0.2665933059059887866 ) ) ;
#1928=CARTESIAN_POINT ( 'NONE',  ( -1.364829396325458521, 0.2306618581243847221, -0.2411417322834647770 ) ) ;
#1929=CARTESIAN_POINT ( 'NONE',  ( 0.4986876640419954376, -0.6046776061558809534, -0.2411417322834644161 ) ) ;
#1930=CARTESIAN_POINT ( 'NONE',  ( -0.05905511811023545637, 0.1660481256975885056, 0.3530559997133364547 ) ) ;
#1931=CARTESIAN_POINT ( 'NONE',  ( 1.292650918635171564, 0.2952755905511811885, 0.1292274648535926551 ) ) ;
#1938=CARTESIAN_POINT ( 'NONE',  ( 0.4068241469816279987, -0.3690944881889765550, -0.3153832671262227771 ) ) ;
#1939=CARTESIAN_POINT ( 'NONE',  ( -0.3215223097112853146, -0.3162353388693405765, 0.4822834645669290543 ) ) ;
#1940=CARTESIAN_POINT ( 'NONE',  ( 1.305774278215223960, 0.2952755905511810774, -0.1292274648535930714 ) ) ;
#1942=CARTESIAN_POINT ( 'NONE',  ( 0.07217847769028949700, -0.2845877964562159024, 0.3641732283464567677 ) ) ;
#1943=CARTESIAN_POINT ( 'NONE',  ( -0.9711286089238838626, 0.2306618581243847221, -0.2411417322834647770 ) ) ;
#1944=CARTESIAN_POINT ( 'NONE',  ( 1.509186351706037543, -0.4281496062992127816, -0.4176697321401328100 ) ) ;
#1947=ORIENTED_EDGE ( 'NONE', *, *, #65602, .T. ) ;
#1948=ORIENTED_EDGE ( 'NONE', *, *, #50451, .F. ) ;
#1949=CARTESIAN_POINT ( 'NONE',  ( -1.601049868766403650, -0.6046776061558807314, 0.2411417322834647770 ) ) ;
#1950=CARTESIAN_POINT ( 'NONE',  ( -1.128608923884513837, 0.1283753931104746893, -0.1820866141732285504 ) ) ;
#1951=CARTESIAN_POINT ( 'NONE',  ( -1.332020997375327642, -0.05778040916215522460, 0.4822834645669289988 ) ) ;
#1953=CARTESIAN_POINT ( 'NONE',  ( -1.614173228346457378, 1.267785121476993293, 0.1372047244094476981 ) ) ;
#1954=CARTESIAN_POINT ( 'NONE',  ( 1.102362204724410155, -0.1870078740157480879, -0.4822834645669291653 ) ) ;
#1955=CARTESIAN_POINT ( 'NONE',  ( -1.082677165354329896, 0.1660481256975885056, 0.3530559997133364547 ) ) ;
#1956=CARTESIAN_POINT ( 'NONE',  ( -0.1246719160104980823, 0.2952755905511811885, 0.1292274648535926551 ) ) ;
#1957=CARTESIAN_POINT ( 'NONE',  ( -1.213910761154854745, -0.6692913385826771977, 0.1292274648535927661 ) ) ;
#1959=CARTESIAN_POINT ( 'NONE',  ( 0.4527559055118117182, -0.5400638737290844871, 0.3530559997133364547 ) ) ;
#1961=CARTESIAN_POINT ( 'NONE',  ( -1.207349081364828436, -0.5023911411419708095, 0.1820866141732285504 ) ) ;
#1964=ORIENTED_EDGE ( 'NONE', *, *, #33686, .F. ) ;
#1965=CARTESIAN_POINT ( 'NONE',  ( 1.614173228346456712, 1.267785121476991517, 0.1372047244094478646 ) ) ;
#1966=CARTESIAN_POINT ( 'NONE',  ( -1.076115485564303809, 0.2306618581243848609, 0.2411417322834645549 ) ) ;
#1967=CARTESIAN_POINT ( 'NONE',  ( -1.305774278215222184, 0.2952755905511811885, 0.1292274648535926551 ) ) ;
#1969=CARTESIAN_POINT ( 'NONE',  ( -1.377952755905511140, 0.2952755905511811885, 0.000000000000000000 ) ) ;
#1970=CARTESIAN_POINT ( 'NONE',  ( -1.601049868766403650, -0.6046776061558807314, 0.2411417322834647770 ) ) ;
#1971=CARTESIAN_POINT ( 'NONE',  ( -1.397637795275589623, -0.5400638737290845981, -0.3530559997133363437 ) ) ;
#1973=CARTESIAN_POINT ( 'NONE',  ( 0.2099737532808405305, -0.5023911411419708095, 0.1820866141732285504 ) ) ;
#1975=CARTESIAN_POINT ( 'NONE',  ( -0.8267716535433065062, -0.5511811023622047445, 6.969142054262312111E-17 ) ) ;
#1976=VECTOR ( 'NONE', #64196, 39.37007874015748143 ) ;
#1977=CARTESIAN_POINT ( 'NONE',  ( -1.148293963254592542, 0.2952755905511811885, 0.1292274648535926551 ) ) ;
#1978=CARTESIAN_POINT ( 'NONE',  ( 0.9120734908136489683, -0.6692913385826771977, 0.1292274648535927661 ) ) ;
#1979=CARTESIAN_POINT ( 'NONE',  ( -0.7677165354330699465, -0.5400638737290845981, -0.3530559997133363437 ) ) ;
#1981=ORIENTED_EDGE ( 'NONE', *, *, #28395, .F. ) ;
#1982=CARTESIAN_POINT ( 'NONE',  ( -0.7808398950131222316, -0.3162353388693409650, -0.4822834645669289433 ) ) ;
#1983=CARTESIAN_POINT ( 'NONE',  ( 0.7414698162729663755, -0.6692913385826773087, -0.1292274648535924053 ) ) ;
#1984=CARTESIAN_POINT ( 'NONE',  ( -1.627296587926508442, -0.5023911411419708095, -0.1820866141732282451 ) ) ;
#1985=CARTESIAN_POINT ( 'NONE',  ( -1.601049868766403650, -0.6046776061558807314, 0.2411417322834647770 ) ) ;
#1990=CARTESIAN_POINT ( 'NONE',  ( -0.2755905511811015396, -0.6692913385826771977, 8.415575281601705876E-17 ) ) ;
#1991=CARTESIAN_POINT ( 'NONE',  ( -1.318897637795274802, 0.07958543189024085140, 0.2665933059059887866 ) ) ;
#1993=CARTESIAN_POINT ( 'NONE',  ( -1.227034120734907585, 0.2952755905511811885, 0.1292274648535926551 ) ) ;
#1995=CARTESIAN_POINT ( 'NONE',  ( -1.548556430446193399, 0.2306618581243848609, 0.2411417322834645549 ) ) ;
#1996=CARTESIAN_POINT ( 'NONE',  ( -0.5774278215223089816, 0.2306618581243847221, -0.2411417322834647770 ) ) ;
#1999=CARTESIAN_POINT ( 'NONE',  ( 0.5643044619422579178, -0.3690944881889765550, -0.3153832671262227771 ) ) ;
#2001=CARTESIAN_POINT ( 'NONE',  ( 0.1902887139107617975, -0.5511811023622048555, -0.09757992244046775898 ) ) ;
#2002=CARTESIAN_POINT ( 'NONE',  ( 0.8070866141732288002, 0.07958543189024085140, 0.2665933059059887866 ) ) ;
#2003=CARTESIAN_POINT ( 'NONE',  ( 1.030183727034121421, -0.3162353388693409650, -0.4822834645669289433 ) ) ;
#2004=CARTESIAN_POINT ( 'NONE',  ( -0.04593175853018302557, 0.1771653543307087630, 0.09757992244046791164 ) ) ;
#2006=CARTESIAN_POINT ( 'NONE',  ( -1.292650918635170010, 0.2952755905511810774, -0.1292274648535930714 ) ) ;
#2007=CARTESIAN_POINT ( 'NONE',  ( -0.1049868766404193215, 0.1283753931104746893, -0.1820866141732285504 ) ) ;
#2008=CARTESIAN_POINT ( 'NONE',  ( -1.233595800524933894, -0.5023911411419708095, -0.1820866141732282451 ) ) ;
#2010=CARTESIAN_POINT ( 'NONE',  ( -0.5708661417322825615, -0.4536011799217367080, 0.2665933059059888421 ) ) ;
#2012=CARTESIAN_POINT ( 'NONE',  ( 0.09842519685039434474, 0.1660481256975885056, 0.3530559997133364547 ) ) ;
#2014=CARTESIAN_POINT ( 'NONE',  ( 0.7414698162729663755, -0.5511811023622048555, -0.09757992244046775898 ) ) ;
#2015=CARTESIAN_POINT ( 'NONE',  ( -0.2099737532808391705, -0.5023911411419708095, -0.1820866141732282451 ) ) ;
#2016=CARTESIAN_POINT ( 'NONE',  ( -0.3805774278215216522, 0.05413385826771666132, 0.4176697321401328100 ) ) ;
#2018=CARTESIAN_POINT ( 'NONE',  ( -0.9776902887139098386, 0.1771653543307087075, -0.09757992244046823083 ) ) ;
#2020=CARTESIAN_POINT ( 'NONE',  ( 0.4658792650918641698, -0.05778040916215560624, -0.4822834645669293319 ) ) ;
#2022=EDGE_CURVE ( 'NONE', #72947, #33617, #60258, .T. ) ;
#2024=CARTESIAN_POINT ( 'NONE',  ( -0.2296587926509179312, -0.2845877964562161244, -0.3641732283464567121 ) ) ;
#2025=CARTESIAN_POINT ( 'NONE',  ( -1.404199475065615932, -0.4281496062992127816, -0.4176697321401328100 ) ) ;
#2026=CARTESIAN_POINT ( 'NONE',  ( -1.653543307086613234, -0.1870078740157479769, 0.3641732283464567677 ) ) ;
#2028=CARTESIAN_POINT ( 'NONE',  ( -0.6955380577427815458, -0.3690944881889765550, -0.3153832671262227771 ) ) ;
#2029=CARTESIAN_POINT ( 'NONE',  ( -1.089942661822471459, 0.000000000000000000, 0.3464511005275205946 ) ) ;
#2030=CARTESIAN_POINT ( 'NONE',  ( 0.8333333333333340365, 0.2952755905511810774, -0.1292274648535930714 ) ) ;
#2035=CARTESIAN_POINT ( 'NONE',  ( -1.666666666666665853, 0.05413385826771626580, -0.4176697321401330321 ) ) ;
#2036=CARTESIAN_POINT ( 'NONE',  ( -1.391076115485563758, 0.2306618581243848609, 0.2411417322834645549 ) ) ;
#2037=CARTESIAN_POINT ( 'NONE',  ( 1.167979002624672580, 0.05413385826771626580, -0.4176697321401330321 ) ) ;
#2039=CARTESIAN_POINT ( 'NONE',  ( 1.476377952755906442, -0.4536011799217367080, 0.2665933059059888421 ) ) ;
#2040=CARTESIAN_POINT ( 'NONE',  ( 0.5380577427821529035, -0.4281496062992124485, 0.4176697321401328655 ) ) ;
#2041=CARTESIAN_POINT ( 'NONE',  ( -0.4790026246719152336, -0.05778040916215560624, -0.4822834645669293319 ) ) ;
#2044=CARTESIAN_POINT ( 'NONE',  ( 0.9580052493438326877, -0.004921259842519576551, 0.3153832671262227771 ) ) ;
#2049=CARTESIAN_POINT ( 'NONE',  ( -0.5052493438320203589, -0.6692913385826771977, 0.1292274648535927661 ) ) ;
#2050=CARTESIAN_POINT ( 'NONE',  ( 1.404199475065617264, -0.4281496062992124485, 0.4176697321401328655 ) ) ;
#2051=CARTESIAN_POINT ( 'NONE',  ( 0.09842519685039434474, 0.1660481256975885056, 0.3530559997133364547 ) ) ;
#2052=CARTESIAN_POINT ( 'NONE',  ( -0.3346456692913377662, 0.07958543189024071263, -0.2665933059059888421 ) ) ;
#2053=CARTESIAN_POINT ( 'NONE',  ( 1.102362204724410155, -0.1870078740157480879, -0.4822834645669291653 ) ) ;
#2054=CARTESIAN_POINT ( 'NONE',  ( -0.9908136482939626788, 0.2952755905511811885, 0.1292274648535926551 ) ) ;
#2055=CARTESIAN_POINT ( 'NONE',  ( -0.06561679790026180015, -0.4281496062992127816, -0.4176697321401328100 ) ) ;
#2056=CARTESIAN_POINT ( 'NONE',  ( -0.8989501312335946848, 0.2952755905511810774, -0.1292274648535930714 ) ) ;
#2057=CARTESIAN_POINT ( 'NONE',  ( 1.167979002624672580, 0.05413385826771626580, -0.4176697321401330321 ) ) ;
#2058=CARTESIAN_POINT ( 'NONE',  ( 1.043307086614173818, -0.5400638737290845981, -0.3530559997133363437 ) ) ;
#2059=CARTESIAN_POINT ( 'NONE',  ( 1.220472440944882608, 0.2952755905511811885, 0.000000000000000000 ) ) ;
#2061=CARTESIAN_POINT ( 'NONE',  ( -0.05905511811023545637, 0.07958543189024085140, 0.2665933059059887866 ) ) ;
#2064=EDGE_LOOP ( 'NONE', ( #49645, #3322, #8878, #74804 ) ) ;
#2065=CARTESIAN_POINT ( 'NONE',  ( -0.8398950131233589023, -0.5023911411419708095, -0.1820866141732282451 ) ) ;
#2066=CARTESIAN_POINT ( 'NONE',  ( -0.1049868766404193215, -0.6046776061558807314, 0.2411417322834647770 ) ) ;
#2068=CARTESIAN_POINT ( 'NONE',  ( -0.1246719160104980823, 0.2952755905511811885, 0.1292274648535926551 ) ) ;
#2069=CARTESIAN_POINT ( 'NONE',  ( -0.4461942257217840213, 0.2306618581243848609, 0.2411417322834645549 ) ) ;
#2070=CARTESIAN_POINT ( 'NONE',  ( -0.7808398950131222316, -0.3162353388693409650, -0.4822834645669289433 ) ) ;
#2071=CARTESIAN_POINT ( 'NONE',  ( -0.9645669291338575535, -0.5400638737290844871, 0.3530559997133364547 ) ) ;
#2072=B_SPLINE_CURVE_WITH_KNOTS ( 'NONE', 3,
 ( #19943, #7309, #16917, #30756, #31157, #24433, #82521 ),
 .UNSPECIFIED., .F., .F.,
 ( 4, 3, 4 ),
 ( 3.469446951953614189E-18, 0.001246230184515596025, 0.002492489877932668914 ),
 .UNSPECIFIED. ) ;
#2073=CARTESIAN_POINT ( 'NONE',  ( 1.417322834645670104, -0.1870078740157480601, -0.3641732283464567677 ) ) ;
#2074=CARTESIAN_POINT ( 'NONE',  ( -1.450131233595799651, 0.2952755905511810774, -0.1292274648535930714 ) ) ;
#2076=CARTESIAN_POINT ( 'NONE',  ( 0.5577427821522314977, -0.2845877964562161244, -0.3641732283464567121 ) ) ;
#2077=CARTESIAN_POINT ( 'NONE',  ( 0.1246719160104994284, 0.2952755905511810774, -0.1292274648535930714 ) ) ;
#2078=CARTESIAN_POINT ( 'NONE',  ( 0.5118110236220480003, -0.6692913385826771977, 8.415575281601705876E-17 ) ) ;
#2079=ORIENTED_EDGE ( 'NONE', *, *, #29846, .T. ) ;
#2081=CARTESIAN_POINT ( 'NONE',  ( -0.5643044619422565855, 0.05413385826771626580, -0.4176697321401330321 ) ) ;
#2084=CARTESIAN_POINT ( 'NONE',  ( -0.5971128608923877978, 0.2952755905511811885, 0.1292274648535926551 ) ) ;
#2087=CARTESIAN_POINT ( 'NONE',  ( -1.594488188976377119, 0.07958543189024071263, -0.2665933059059888421 ) ) ;
#2088=CARTESIAN_POINT ( 'NONE',  ( 0.7939632545931766261, -0.05778040916215522460, 0.4822834645669289988 ) ) ;
#2089=CARTESIAN_POINT ( 'NONE',  ( 1.036745406824147731, 0.05413385826771666132, 0.4176697321401328100 ) ) ;
#2090=CARTESIAN_POINT ( 'NONE',  ( -0.3608923884514428360, 0.1771653543307087630, 0.09757992244046791164 ) ) ;
#2091=CARTESIAN_POINT ( 'NONE',  ( 0.3805774278215230400, 0.05413385826771626580, -0.4176697321401330321 ) ) ;
#2093=CARTESIAN_POINT ( 'NONE',  ( -0.05905511811023545637, 0.07958543189024085140, 0.2665933059059887866 ) ) ;
#2094=CARTESIAN_POINT ( 'NONE',  ( -0.06561679790026180015, -0.4281496062992127816, -0.4176697321401328100 ) ) ;
#2096=CARTESIAN_POINT ( 'NONE',  ( -1.489501312335957062, -0.3162353388693409650, -0.4822834645669289433 ) ) ;
#2097=CARTESIAN_POINT ( 'NONE',  ( -0.04593175853018302557, -0.5511811023622048555, -0.09757992244046775898 ) ) ;
#2098=CARTESIAN_POINT ( 'NONE',  ( 1.594488188976378673, -0.4536011799217368745, -0.2665933059059886201 ) ) ;
#2099=CARTESIAN_POINT ( 'NONE',  ( -0.8989501312335946848, 0.2952755905511810774, -0.1292274648535930714 ) ) ;
#2100=CARTESIAN_POINT ( 'NONE',  ( -0.7874015748031489847, -0.1870078740157480601, -0.3641732283464567677 ) ) ;
#2102=CARTESIAN_POINT ( 'NONE',  ( -0.8858267716535425107, 0.1660481256975883668, -0.3530559997133364547 ) ) ;
#2103=CARTESIAN_POINT ( 'NONE',  ( -0.6299212598425188991, -0.1870078740157480879, -0.4822834645669291653 ) ) ;
#2104=CARTESIAN_POINT ( 'NONE',  ( 8.195543980992789655E-16, -0.1870078740157480879, -0.4822834645669291653 ) ) ;
#2109=CARTESIAN_POINT ( 'NONE',  ( 0.8858267716535438430, 0.07958543189024085140, 0.2665933059059887866 ) ) ;
#2110=CARTESIAN_POINT ( 'NONE',  ( 1.581364829396326277, -0.05778040916215522460, 0.4822834645669289988 ) ) ;
#2111=CARTESIAN_POINT ( 'NONE',  ( -1.259842519685038686, -0.1870078740157479769, 0.3641732283464567677 ) ) ;
#2112=CARTESIAN_POINT ( 'NONE',  ( 1.286089238845145033, -0.6046776061558809534, -0.2411417322834644161 ) ) ;
#2113=CARTESIAN_POINT ( 'NONE',  ( -0.9711286089238838626, -0.5023911411419708095, 0.1820866141732285504 ) ) ;
#2114=CARTESIAN_POINT ( 'NONE',  ( -0.5839895013123351797, 0.2952755905511810774, -0.1292274648535930714 ) ) ;
#2115=CARTESIAN_POINT ( 'NONE',  ( 0.2952755905511819101, 0.07958543189024071263, -0.2665933059059888421 ) ) ;
#2117=CARTESIAN_POINT ( 'NONE',  ( 1.056430446194226436, -0.5511811023622048555, -0.09757992244046775898 ) ) ;
#2118=CARTESIAN_POINT ( 'NONE',  ( 0.4330708661417329575, 0.2952755905511811885, 0.000000000000000000 ) ) ;
#2121=CARTESIAN_POINT ( 'NONE',  ( -0.6167979002624665030, 0.05413385826771666132, 0.4176697321401328100 ) ) ;
#2123=CARTESIAN_POINT ( 'NONE',  ( 1.213910761154856299, -0.5511811023622048555, -0.09757992244046775898 ) ) ;
#2124=CARTESIAN_POINT ( 'NONE',  ( 0.5183727034120741983, -0.6692913385826771977, 0.1292274648535927661 ) ) ;
#2125=CARTESIAN_POINT ( 'NONE',  ( -0.2821522309711278487, -0.6692913385826773087, -0.1292274648535924053 ) ) ;
#2126=CARTESIAN_POINT ( 'NONE',  ( -0.1771653543307080136, 0.07958543189024071263, -0.2665933059059888421 ) ) ;
#2128=CARTESIAN_POINT ( 'NONE',  ( 0.1181102362204730916, 0.1771653543307087630, 0.000000000000000000 ) ) ;
#2129=CARTESIAN_POINT ( 'NONE',  ( 0.6102362204724416372, 0.1660481256975883668, -0.3530559997133364547 ) ) ;
#2130=CARTESIAN_POINT ( 'NONE',  ( -0.8989501312335946848, 0.1771653543307087075, -0.09757992244046823083 ) ) ;
#2132=CARTESIAN_POINT ( 'NONE',  ( -1.161417322834644716, 0.1660481256975885056, 0.3530559997133364547 ) ) ;
#2134=ORIENTED_EDGE ( 'NONE', *, *, #48920, .T. ) ;
#2135=CARTESIAN_POINT ( 'NONE',  ( -1.266404199475064773, -0.2845877964562159024, 0.3641732283464567677 ) ) ;
#2136=CARTESIAN_POINT ( 'NONE',  ( -0.2165354330708654795, -0.5400638737290845981, -0.3530559997133363437 ) ) ;
#2138=CARTESIAN_POINT ( 'NONE',  ( -0.9645669291338575535, 0.1660481256975883668, -0.3530559997133364547 ) ) ;
#2140=CARTESIAN_POINT ( 'NONE',  ( 1.581364829396326277, -0.3162353388693409650, -0.4822834645669289433 ) ) ;
#2141=CARTESIAN_POINT ( 'NONE',  ( 0.9645669291338588858, 0.1660481256975885056, 0.3530559997133364547 ) ) ;
#2142=CARTESIAN_POINT ( 'NONE',  ( 1.043307086614173818, 0.1660481256975885056, 0.3530559997133364547 ) ) ;
#2144=CARTESIAN_POINT ( 'NONE',  ( -1.595398199321656607, 1.309738123151862998, 0.1559797534342480529 ) ) ;
#2146=CARTESIAN_POINT ( 'NONE',  ( -1.469816272965878357, -0.6046776061558809534, -0.2411417322834644161 ) ) ;
#2149=CARTESIAN_POINT ( 'NONE',  ( -0.6167979002624665030, -0.3690944881889765550, -0.3153832671262227771 ) ) ;
#2151=ORIENTED_EDGE ( 'NONE', *, *, #58402, .T. ) ;
#2152=CARTESIAN_POINT ( 'NONE',  ( 0.7217847769028878924, -0.4281496062992127816, -0.4176697321401328100 ) ) ;
#2153=CARTESIAN_POINT ( 'NONE',  ( 0.1377952755905518800, -0.5400638737290844871, 0.3530559997133364547 ) ) ;
#2154=CARTESIAN_POINT ( 'NONE',  ( -0.6627296587926501115, 0.2952755905511810774, -0.1292274648535930714 ) ) ;
#2155=CARTESIAN_POINT ( 'NONE',  ( 1.548556430446194954, 0.2306618581243847221, -0.2411417322834647770 ) ) ;
#2156=CARTESIAN_POINT ( 'NONE',  ( -0.7874015748031489847, -0.1870078740157480601, -0.3641732283464567677 ) ) ;
#2158=CARTESIAN_POINT ( 'NONE',  ( 0.8727034120734913358, -0.05778040916215522460, 0.4822834645669289988 ) ) ;
#2159=EDGE_CURVE ( 'NONE', #42372, #16885, #15658, .T. ) ;
#2160=CARTESIAN_POINT ( 'NONE',  ( 0.4986876640419954376, 0.1283753931104748280, 0.1820866141732283561 ) ) ;
#2161=CARTESIAN_POINT ( 'NONE',  ( -0.5511811023622038563, -0.1870078740157479769, 0.4822834645669291653 ) ) ;
#2163=CARTESIAN_POINT ( 'NONE',  ( -1.135170603674539924, 0.2952755905511810774, -0.1292274648535930714 ) ) ;
#2164=DIRECTION ( 'NONE',  ( 0.000000000000000000, -1.000000000000000000, 0.000000000000000000 ) ) ;
#2165=CARTESIAN_POINT ( 'NONE',  ( 1.279527559055118724, -0.5400638737290845981, -0.3530559997133363437 ) ) ;
#2166=CARTESIAN_POINT ( 'NONE',  ( 1.207349081364829990, 0.1283753931104748280, 0.1820866141732283561 ) ) ;
#2169=CARTESIAN_POINT ( 'NONE',  ( -0.1443569553805765515, -0.4281496062992127816, -0.4176697321401328100 ) ) ;
#2170=ORIENTED_EDGE ( 'NONE', *, *, #4245, .F. ) ;
#2171=CARTESIAN_POINT ( 'NONE',  ( 0.8661417322834652488, -0.1870078740157480601, -0.3641732283464567677 ) ) ;
#2172=CARTESIAN_POINT ( 'NONE',  ( -1.102362204724408601, -0.1870078740157479769, 0.4822834645669291653 ) ) ;
#2173=CARTESIAN_POINT ( 'NONE',  ( 1.017060367454068581, -0.05778040916215560624, -0.4822834645669293319 ) ) ;
#2174=CARTESIAN_POINT ( 'NONE',  ( 0.6889763779527563470, 0.1660481256975883668, -0.3530559997133364547 ) ) ;
#2175=CARTESIAN_POINT ( 'NONE',  ( 0.1115485564304467270, -0.6692913385826773087, -0.1292274648535924053 ) ) ;
#2176=CARTESIAN_POINT ( 'NONE',  ( -0.3937007874015740483, -0.1870078740157479769, 0.4822834645669291653 ) ) ;
#2178=CARTESIAN_POINT ( 'NONE',  ( -1.719160104986876103, 0.05413385826771666132, 0.4176697321401328100 ) ) ;
#2179=CARTESIAN_POINT ( 'NONE',  ( -0.5643044619422565855, -0.4281496062992124485, 0.4176697321401328655 ) ) ;
#2180=CARTESIAN_POINT ( 'NONE',  ( -0.6102362204724400829, -0.4536011799217368745, -0.2665933059059886201 ) ) ;
#2183=CARTESIAN_POINT ( 'NONE',  ( -0.5183727034120726440, -0.6692913385826773087, -0.1292274648535924053 ) ) ;
#2185=CARTESIAN_POINT ( 'NONE',  ( 0.6036745406824153282, -0.6046776061558807314, 0.2411417322834647770 ) ) ;
#2188=ADVANCED_FACE ( 'NONE', ( #47199 ), #68532, .T. ) ;
#2189=CARTESIAN_POINT ( 'NONE',  ( 0.06561679790026316017, -0.4281496062992124485, 0.4176697321401328655 ) ) ;
#2190=CARTESIAN_POINT ( 'NONE',  ( 1.062992125984252745, 0.1771653543307087630, 0.000000000000000000 ) ) ;
#2191=CARTESIAN_POINT ( 'NONE',  ( -0.9324623468618411515, 0.000000000000000000, 0.3464511005275205946 ) ) ;
#2193=CARTESIAN_POINT ( 'NONE',  ( 1.305774278215223960, -0.5511811023622046335, 0.09757992244046803654 ) ) ;
#2194=CARTESIAN_POINT ( 'NONE',  ( 1.082677165354331228, -0.5400638737290844871, 0.3530559997133364547 ) ) ;
#2196=CARTESIAN_POINT ( 'NONE',  ( -0.3740157480314953431, -0.5400638737290845981, -0.3530559997133363437 ) ) ;
#2197=CARTESIAN_POINT ( 'NONE',  ( -1.535433070866141225, -0.6692913385826771977, 8.415575281601705876E-17 ) ) ;
#2198=CARTESIAN_POINT ( 'NONE',  ( -1.673228346456691717, 0.1660481256975883668, -0.3530559997133364547 ) ) ;
#2199=CARTESIAN_POINT ( 'NONE',  ( -0.1246719160104980823, 0.2952755905511811885, 0.1292274648535926551 ) ) ;
#2201=CARTESIAN_POINT ( 'NONE',  ( 1.279527559055118724, -0.5400638737290845981, -0.3530559997133363437 ) ) ;
#2202=CARTESIAN_POINT ( 'NONE',  ( 0.5511811023622054106, -0.1870078740157480879, -0.4822834645669291653 ) ) ;
#2203=CARTESIAN_POINT ( 'NONE',  ( 0.7217847769028878924, -0.004921259842519576551, 0.3153832671262227771 ) ) ;
#2205=CARTESIAN_POINT ( 'NONE',  ( 0.4265091863517067594, 0.1771653543307087630, 0.09757992244046791164 ) ) ;
#2206=CARTESIAN_POINT ( 'NONE',  ( -1.036745406824146176, 0.009842519685039144428, -0.3409548833797004797 ) ) ;
#2208=CARTESIAN_POINT ( 'NONE',  ( 0.6167979002624679463, 0.05413385826771626580, -0.4176697321401330321 ) ) ;
#2214=CARTESIAN_POINT ( 'NONE',  ( 0.1509186351706042484, -0.2845877964562159024, 0.3641732283464567677 ) ) ;
#2215=CARTESIAN_POINT ( 'NONE',  ( 0.6233595800524942554, -0.05778040916215560624, -0.4822834645669293319 ) ) ;
#2216=CARTESIAN_POINT ( 'NONE',  ( 1.364829396325460076, 0.1283753931104748280, 0.1820866141732283561 ) ) ;
#2217=CARTESIAN_POINT ( 'NONE',  ( -0.8005249343832013809, -0.3690944881889763329, 0.3153832671262228327 ) ) ;
#2218=CARTESIAN_POINT ( 'NONE',  ( -1.003937007874015297, -0.5400638737290845981, -0.3530559997133363437 ) ) ;
#2219=CARTESIAN_POINT ( 'NONE',  ( -1.522309711286088607, 0.2306618581243847221, -0.2411417322834647770 ) ) ;
#2220=CARTESIAN_POINT ( 'NONE',  ( 0.7020997375328090762, -0.3162353388693405765, 0.4822834645669290543 ) ) ;
#2221=CARTESIAN_POINT ( 'NONE',  ( 1.660104986876641320, -0.05778040916215522460, 0.4822834645669289988 ) ) ;
#2224=CARTESIAN_POINT ( 'NONE',  ( 0.7545931758530188826, -0.6692913385826771977, 0.1292274648535927661 ) ) ;
#2227=CARTESIAN_POINT ( 'NONE',  ( 1.259842519685040019, -0.1870078740157480879, -0.4822834645669291653 ) ) ;
#2228=CARTESIAN_POINT ( 'NONE',  ( -1.397637795275589623, 0.07958543189024085140, 0.2665933059059887866 ) ) ;
#2229=CARTESIAN_POINT ( 'NONE',  ( 1.161417322834646493, -0.4536011799217367080, 0.2665933059059888421 ) ) ;
#2230=CARTESIAN_POINT ( 'NONE',  ( -1.227034120734907141, -0.5511811023622048555, -0.09757992244046775898 ) ) ;
#2231=CARTESIAN_POINT ( 'NONE',  ( -0.8530183727034112984, -0.004921259842519576551, 0.3153832671262227771 ) ) ;
#2233=CARTESIAN_POINT ( 'NONE',  ( 0.5511811023622054106, -0.1870078740157480601, -0.3641732283464567677 ) ) ;
#2234=CARTESIAN_POINT ( 'NONE',  ( -0.006561679790025524116, -0.05778040916215560624, -0.4822834645669293319 ) ) ;
#2235=CARTESIAN_POINT ( 'NONE',  ( 0.9317585301837276734, -0.4281496062992124485, 0.4176697321401328655 ) ) ;
#2236=CARTESIAN_POINT ( 'NONE',  ( 0.1771653543307093182, -0.5400638737290845981, -0.3530559997133363437 ) ) ;
#2237=CARTESIAN_POINT ( 'NONE',  ( 0.1771653543307093182, 0.07958543189024085140, 0.2665933059059887866 ) ) ;
#2238=CARTESIAN_POINT ( 'NONE',  ( 1.128608923884514947, 0.2306618581243848609, 0.2411417322834645549 ) ) ;
#2239=CARTESIAN_POINT ( 'NONE',  ( -1.548556430446193399, -0.6046776061558809534, -0.2411417322834644161 ) ) ;
#2240=CARTESIAN_POINT ( 'NONE',  ( -0.9186351706036736120, 0.2306618581243848609, 0.2411417322834645549 ) ) ;
#2243=CARTESIAN_POINT ( 'NONE',  ( -0.7677165354330699465, -0.5400638737290845981, -0.3530559997133363437 ) ) ;
#2244=CARTESIAN_POINT ( 'NONE',  ( -0.1902887139107604098, -0.6692913385826771977, 0.1292274648535927661 ) ) ;
#2247=ORIENTED_EDGE ( 'NONE', *, *, #83113, .T. ) ;
#2249=LINE ( 'NONE', #3492, #18588 ) ;
#2250=CARTESIAN_POINT ( 'NONE',  ( -1.286089238845143479, -0.5023911411419708095, 0.1820866141732285504 ) ) ;
#2252=EDGE_CURVE ( 'NONE', #41772, #24205, #68941, .T. ) ;
#2253=CARTESIAN_POINT ( 'NONE',  ( -1.627296587926508442, -0.6046776061558809534, -0.2411417322834644161 ) ) ;
#2255=CARTESIAN_POINT ( 'NONE',  ( -0.1246719160104980823, -0.6692913385826773087, -0.1292274648535924053 ) ) ;
#2256=CARTESIAN_POINT ( 'NONE',  ( -0.3149606299212590610, -0.1870078740157479769, 0.3641732283464567677 ) ) ;
#2257=CARTESIAN_POINT ( 'NONE',  ( 0.7086614173228352742, -0.1870078740157480879, -0.4822834645669291653 ) ) ;
#2258=CARTESIAN_POINT ( 'NONE',  ( 0.4658792650918640033, -0.3162353388693405765, 0.4822834645669290543 ) ) ;
#2259=CARTESIAN_POINT ( 'NONE',  ( -0.2262115530851587786, -2.191421614605370878E-15, 0.4445507791589071167 ) ) ;
#2260=VECTOR ( 'NONE', #74675, 39.37007874015748143 ) ;
#2263=CARTESIAN_POINT ( 'NONE',  ( 1.233595800524935227, 0.2306618581243847221, -0.2411417322834647770 ) ) ;
#2264=CIRCLE ( 'NONE', #38528, 2.362204724409449064 ) ;
#2266=CARTESIAN_POINT ( 'NONE',  ( -0.03280839895013062252, -0.6692913385826771977, 0.1292274648535927661 ) ) ;
#2267=CARTESIAN_POINT ( 'NONE',  ( -0.9776902887139098386, 0.2952755905511810774, -0.1292274648535930714 ) ) ;
#2268=CARTESIAN_POINT ( 'NONE',  ( -1.633858267716534529, 0.1660481256975885056, 0.3530559997133364547 ) ) ;
#2269=CARTESIAN_POINT ( 'NONE',  ( 1.030183727034121421, -0.05778040916215522460, 0.4822834645669289988 ) ) ;
#2271=CARTESIAN_POINT ( 'NONE',  ( 0.2230971128608929543, 0.05413385826771626580, -0.4176697321401330321 ) ) ;
#2272=CARTESIAN_POINT ( 'NONE',  ( 0.5052493438320218022, -0.6692913385826773087, -0.1292274648535924053 ) ) ;
#2273=CARTESIAN_POINT ( 'NONE',  ( -0.2296587926509179312, -0.05778040916215522460, 0.4822834645669289988 ) ) ;
#2274=CARTESIAN_POINT ( 'NONE',  ( 0.8530183727034128527, -0.3690944881889763329, 0.3153832671262228327 ) ) ;
#2275=CARTESIAN_POINT ( 'NONE',  ( -1.246719160104986512, 0.05413385826771666132, 0.4176697321401328100 ) ) ;
#2276=CARTESIAN_POINT ( 'NONE',  ( -1.522309711286088607, 0.2306618581243847221, -0.2411417322834647770 ) ) ;
#2277=CARTESIAN_POINT ( 'NONE',  ( 0.6299212598425204535, -0.1870078740157479769, 0.4822834645669291653 ) ) ;
#2281=EDGE_CURVE ( 'NONE', #39084, #5951, #14402, .T. ) ;
#2283=ORIENTED_EDGE ( 'NONE', *, *, #42014, .T. ) ;
#2284=CARTESIAN_POINT ( 'NONE',  ( 1.036745406824147731, 0.05413385826771666132, 0.4176697321401328100 ) ) ;
#2285=CARTESIAN_POINT ( 'NONE',  ( 0.6889763779527563470, 0.07958543189024071263, -0.2665933059059888421 ) ) ;
#2286=CARTESIAN_POINT ( 'NONE',  ( 0.5905511811023629321, 0.2952755905511811885, 0.000000000000000000 ) ) ;
#2287=ADVANCED_FACE ( 'NONE', ( #4547 ), #41788, .F. ) ;
#2288=CARTESIAN_POINT ( 'NONE',  ( 0.8761506516392508770, -4.927456884911482678E-16, 0.4445507791589062840 ) ) ;
#2292=CARTESIAN_POINT ( 'NONE',  ( -1.496062992125983815, -0.1870078740157479769, 0.4822834645669291653 ) ) ;
#2293=CARTESIAN_POINT ( 'NONE',  ( -0.4790026246719154557, -0.3162353388693405765, 0.4822834645669290543 ) ) ;
#2294=CARTESIAN_POINT ( 'NONE',  ( 1.174540682414699111, -0.05778040916215560624, -0.4822834645669293319 ) ) ;
#2296=CARTESIAN_POINT ( 'NONE',  ( -1.423884514435694859, -0.3162353388693405765, 0.4822834645669290543 ) ) ;
#2301=CARTESIAN_POINT ( 'NONE',  ( -1.338582677165353729, -0.1870078740157479769, 0.3641732283464567677 ) ) ;
#2302=CARTESIAN_POINT ( 'NONE',  ( -1.568241469816272105, -0.3162353388693409650, -0.4822834645669289433 ) ) ;
#2303=CARTESIAN_POINT ( 'NONE',  ( 0.2034120734908144990, -0.6692913385826771977, 0.1292274648535927661 ) ) ;
#2305=CARTESIAN_POINT ( 'NONE',  ( 1.587926509186352586, -0.4281496062992127816, -0.4176697321401328100 ) ) ;
#2307=CARTESIAN_POINT ( 'NONE',  ( -0.7349081364829390672, 0.1283753931104746893, -0.1820866141732285504 ) ) ;
#2308=CARTESIAN_POINT ( 'NONE',  ( 0.9120734908136490793, 0.2952755905511810774, -0.1292274648535930714 ) ) ;
#2309=CARTESIAN_POINT ( 'NONE',  ( 1.076115485564305141, -0.5023911411419708095, 0.1820866141732285504 ) ) ;
#2311=CARTESIAN_POINT ( 'NONE',  ( -0.6627296587926503335, -0.5511811023622046335, 0.09757992244046803654 ) ) ;
#2312=CARTESIAN_POINT ( 'NONE',  ( -1.391076115485563314, -0.5023911411419708095, -0.1820866141732282451 ) ) ;
#2314=CARTESIAN_POINT ( 'NONE',  ( 0.3937007874015754361, -0.1870078740157480879, -0.4822834645669291653 ) ) ;
#2315=EDGE_CURVE ( 'NONE', #16662, #77295, #81626, .T. ) ;
#2316=CARTESIAN_POINT ( 'NONE',  ( -0.8005249343832011588, -0.004921259842519870586, -0.3153832671262229437 ) ) ;
#2317=CARTESIAN_POINT ( 'NONE',  ( -0.1115485564304456306, 0.1771653543307087075, -0.09757992244046823083 ) ) ;
#2318=CARTESIAN_POINT ( 'NONE',  ( -0.1049868766404193215, 0.2306618581243847221, -0.2411417322834647770 ) ) ;
#2319=CARTESIAN_POINT ( 'NONE',  ( -1.541994750656167090, -0.5511811023622048555, -0.09757992244046775898 ) ) ;
#2321=CARTESIAN_POINT ( 'NONE',  ( 0.6364829396325465405, -0.05778040916215522460, 0.4822834645669289988 ) ) ;
#2328=CARTESIAN_POINT ( 'NONE',  ( -0.7611548556430438595, 0.2306618581243848609, 0.2411417322834645549 ) ) ;
#2329=CARTESIAN_POINT ( 'NONE',  ( -0.3674540682414692561, -0.5023911411419708095, -0.1820866141732282451 ) ) ;
#2330=CARTESIAN_POINT ( 'NONE',  ( -1.207349081364828436, -0.6046776061558807314, 0.2411417322834647770 ) ) ;
#2331=CARTESIAN_POINT ( 'NONE',  ( 0.4068241469816281097, -0.004921259842519576551, 0.3153832671262227771 ) ) ;
#2332=CARTESIAN_POINT ( 'NONE',  ( -0.5511811023622041894, -0.1870078740157480601, -0.3641732283464567677 ) ) ;
#2333=CARTESIAN_POINT ( 'NONE',  ( -0.9251968503937002541, 0.1660481256975885056, 0.3530559997133364547 ) ) ;
#2334=CARTESIAN_POINT ( 'NONE',  ( -1.699475065616797398, 0.2952755905511811885, 0.1292274648535926551 ) ) ;
#2335=CARTESIAN_POINT ( 'NONE',  ( 1.587926509186352586, -0.4281496062992127816, -0.4176697321401328100 ) ) ;
#2336=CARTESIAN_POINT ( 'NONE',  ( 1.089942661822472569, 9.906153642143428645E-17, -0.3464511005275205946 ) ) ;
#2337=CARTESIAN_POINT ( 'NONE',  ( 0.8333333333333340365, -0.5511811023622046335, 0.09757992244046803654 ) ) ;
#2338=CARTESIAN_POINT ( 'NONE',  ( 0.4265091863517067594, 0.2952755905511811885, 0.1292274648535926551 ) ) ;
#2339=CARTESIAN_POINT ( 'NONE',  ( -1.404199475065615932, -0.4281496062992127816, -0.4176697321401328100 ) ) ;
#2340=CARTESIAN_POINT ( 'NONE',  ( 1.463254593175853824, 0.1771653543307087075, -0.09757992244046823083 ) ) ;
#2341=ORIENTED_EDGE ( 'NONE', *, *, #38343, .T. ) ;
#2344=CARTESIAN_POINT ( 'NONE',  ( -1.246719160104985846, -0.3690944881889765550, -0.3153832671262227771 ) ) ;
#2345=CARTESIAN_POINT ( 'NONE',  ( -0.2690288713910754526, -0.6692913385826771977, 0.1292274648535927661 ) ) ;
#2346=CARTESIAN_POINT ( 'NONE',  ( 0.4068241469816279987, -0.4281496062992127816, -0.4176697321401328100 ) ) ;
#2347=CARTESIAN_POINT ( 'NONE',  ( -1.614173228346456268, -0.5511811023622047445, 6.969142054262312111E-17 ) ) ;
#2349=CARTESIAN_POINT ( 'NONE',  ( -1.496062992125983815, -0.1870078740157480879, -0.4822834645669291653 ) ) ;
#2350=CARTESIAN_POINT ( 'NONE',  ( 0.5971128608923891301, 0.2952755905511810774, -0.1292274648535930714 ) ) ;
#2351=CARTESIAN_POINT ( 'NONE',  ( 0.1377952755905518800, 0.1660481256975883668, -0.3530559997133364547 ) ) ;
#2352=CARTESIAN_POINT ( 'NONE',  ( 1.082677165354331228, -0.5400638737290844871, 0.3530559997133364547 ) ) ;
#2357=CARTESIAN_POINT ( 'NONE',  ( -0.01312335958005186876, -0.3690944881889763329, 0.3153832671262228327 ) ) ;
#2358=CARTESIAN_POINT ( 'NONE',  ( -0.4002624671916004129, -0.05778040916215560624, -0.4822834645669293319 ) ) ;
#2359=CARTESIAN_POINT ( 'NONE',  ( 1.023622047244095112, -0.1870078740157480879, -0.4822834645669291653 ) ) ;
#2361=CARTESIAN_POINT ( 'NONE',  ( -0.1181102362204717315, -0.5511811023622047445, 6.969142054262312111E-17 ) ) ;
#2362=ADVANCED_FACE ( 'NONE', ( #26631 ), #20741, .T. ) ;
#2363=CARTESIAN_POINT ( 'NONE',  ( -1.332020997375327642, -0.05778040916215522460, 0.4822834645669289988 ) ) ;
#2364=CARTESIAN_POINT ( 'NONE',  ( -1.509186351706035767, -0.4281496062992124485, 0.4176697321401328655 ) ) ;
#2369=CARTESIAN_POINT ( 'NONE',  ( 0.8661417322834652488, -0.1870078740157480879, -0.4822834645669291653 ) ) ;
#2370=CARTESIAN_POINT ( 'NONE',  ( -1.725721784776902190, -0.05778040916215522460, 0.4822834645669289988 ) ) ;
#2371=CARTESIAN_POINT ( 'NONE',  ( -1.384514435695537005, -0.5511811023622048555, -0.09757992244046775898 ) ) ;
#2372=CARTESIAN_POINT ( 'NONE',  ( -1.010498687664041384, 0.05413385826771666132, 0.4176697321401328100 ) ) ;
#2375=CARTESIAN_POINT ( 'NONE',  ( 1.036745406824147731, 0.05413385826771666132, 0.4176697321401328100 ) ) ;
#2377=CARTESIAN_POINT ( 'NONE',  ( -0.2624671916010490880, 0.2306618581243847221, -0.2411417322834647770 ) ) ;
#2378=CARTESIAN_POINT ( 'NONE',  ( -0.2821522309711278487, 0.2952755905511811885, 0.1292274648535926551 ) ) ;
#2379=CARTESIAN_POINT ( 'NONE',  ( -1.272965879265091305, 0.05413385826771626580, -0.4176697321401330321 ) ) ;
#2381=CARTESIAN_POINT ( 'NONE',  ( 0.6627296587926515548, 0.2952755905511811885, 0.1292274648535926551 ) ) ;
#2383=CARTESIAN_POINT ( 'NONE',  ( -1.377952755905511140, -0.5511811023622047445, 6.969142054262312111E-17 ) ) ;
#2387=CARTESIAN_POINT ( 'NONE',  ( 1.586052503253845281, 1.299212598425198095, 0.1653254495020587411 ) ) ;
#2389=CARTESIAN_POINT ( 'NONE',  ( -1.496062992125983815, -0.1870078740157480879, -0.4822834645669291653 ) ) ;
#2390=CARTESIAN_POINT ( 'NONE',  ( -1.318897637795274802, 0.1660481256975885056, 0.3530559997133364547 ) ) ;
#2392=CARTESIAN_POINT ( 'NONE',  ( -1.607611548556429737, -0.6692913385826771977, 0.1292274648535927661 ) ) ;
#2393=CARTESIAN_POINT ( 'NONE',  ( -1.719160104986876103, 0.05413385826771666132, 0.4176697321401328100 ) ) ;
#2397=CARTESIAN_POINT ( 'NONE',  ( 0.08530183727034192087, -0.08942795157527998196, 0.3641732283464567121 ) ) ;
#2398=CARTESIAN_POINT ( 'NONE',  ( -0.6299212598425188991, -0.1870078740157479769, 0.3641732283464567677 ) ) ;
#2399=CARTESIAN_POINT ( 'NONE',  ( -1.377952755905511140, -0.6692913385826771977, 8.415575281601705876E-17 ) ) ;
#2400=CARTESIAN_POINT ( 'NONE',  ( 0.7874015748031503170, -0.1870078740157479769, 0.4822834645669291653 ) ) ;
#2401=CARTESIAN_POINT ( 'NONE',  ( -0.9711286089238838626, 0.2306618581243847221, -0.2411417322834647770 ) ) ;
#2404=CARTESIAN_POINT ( 'NONE',  ( -1.325459317585300889, 0.05413385826771666132, 0.4176697321401328100 ) ) ;
#2405=CARTESIAN_POINT ( 'NONE',  ( -1.686351706036744558, 0.1771653543307087075, -0.09757992244046823083 ) ) ;
#2406=DIRECTION ( 'NONE',  ( 0.000000000000000000, 0.000000000000000000, 1.000000000000000000 ) ) ;
#2411=CARTESIAN_POINT ( 'NONE',  ( -0.5249343832020990641, 0.2306618581243848609, 0.2411417322834645549 ) ) ;
#2412=CARTESIAN_POINT ( 'NONE',  ( -1.437007874015747477, 0.07958543189024071263, -0.2665933059059888421 ) ) ;
#2414=CARTESIAN_POINT ( 'NONE',  ( -1.528871391076114250, 0.2952755905511810774, -0.1292274648535930714 ) ) ;
#2417=CARTESIAN_POINT ( 'NONE',  ( -1.614173228346456268, -0.6692913385826771977, 8.415575281601705876E-17 ) ) ;
#2418=CARTESIAN_POINT ( 'NONE',  ( -0.5183727034120726440, -0.6692913385826773087, -0.1292274648535924053 ) ) ;
#2420=CARTESIAN_POINT ( 'NONE',  ( 0.4461942257217855201, -0.5023911411419708095, 0.1820866141732285504 ) ) ;
#2422=EDGE_CURVE ( 'NONE', #38486, #17299, #71250, .T. ) ;
#2423=CARTESIAN_POINT ( 'NONE',  ( 0.3674540682414705883, -0.5023911411419708095, 0.1820866141732285504 ) ) ;
#2424=CARTESIAN_POINT ( 'NONE',  ( 0.7874015748031503170, -0.1870078740157479769, 0.3641732283464567677 ) ) ;
#2425=CARTESIAN_POINT ( 'NONE',  ( 1.135170603674541256, 0.2952755905511811885, 0.1292274648535926551 ) ) ;
#2426=CARTESIAN_POINT ( 'NONE',  ( -0.3477690288713902178, 0.1771653543307087075, -0.09757992244046823083 ) ) ;
#2428=CARTESIAN_POINT ( 'NONE',  ( -1.128608923884513837, 0.2306618581243847221, -0.2411417322834647770 ) ) ;
#2429=CARTESIAN_POINT ( 'NONE',  ( -0.1115485564304456306, 0.1771653543307087075, -0.09757992244046823083 ) ) ;
#2430=CARTESIAN_POINT ( 'NONE',  ( -1.384514435695537005, -0.5511811023622048555, -0.09757992244046775898 ) ) ;
#2432=CARTESIAN_POINT ( 'NONE',  ( -0.8070866141732276899, 0.07958543189024071263, -0.2665933059059888421 ) ) ;
#2434=CARTESIAN_POINT ( 'NONE',  ( -0.2165354330708654795, 0.1660481256975885056, 0.3530559997133364547 ) ) ;
#2435=CARTESIAN_POINT ( 'NONE',  ( 1.555118110236221041, 0.07958543189024071263, -0.2665933059059888421 ) ) ;
#2436=CARTESIAN_POINT ( 'NONE',  ( 0.3608923884514443348, 0.1771653543307087075, -0.09757992244046823083 ) ) ;
#2437=CARTESIAN_POINT ( 'NONE',  ( -0.4199475065616791736, 0.1283753931104746893, -0.1820866141732285504 ) ) ;
#2438=CARTESIAN_POINT ( 'NONE',  ( -0.4396325459317577122, -0.6692913385826773087, -0.1292274648535924053 ) ) ;
#2439=CARTESIAN_POINT ( 'NONE',  ( -1.719160104986876103, 0.05413385826771666132, 0.4176697321401328100 ) ) ;
#2440=CARTESIAN_POINT ( 'NONE',  ( -1.240157480314959759, -0.4536011799217368745, -0.2665933059059886201 ) ) ;
#2441=CARTESIAN_POINT ( 'NONE',  ( -0.9573014326657163231, -2.609869883881465018E-15, -0.3464511005275220379 ) ) ;
#2442=CARTESIAN_POINT ( 'NONE',  ( 0.6102362204724416372, 0.1660481256975883668, -0.3530559997133364547 ) ) ;
#2445=CARTESIAN_POINT ( 'NONE',  ( -1.604771003085130099, 1.320215725944019480, -0.1466069496707743947 ) ) ;
#2446=CARTESIAN_POINT ( 'NONE',  ( -0.03937007874015669567, -0.5511811023622047445, 6.969142054262312111E-17 ) ) ;
#2448=CARTESIAN_POINT ( 'NONE',  ( -0.3608923884514428360, -0.6692913385826773087, -0.1292274648535924053 ) ) ;
#2449=CARTESIAN_POINT ( 'NONE',  ( -1.535433070866141225, -0.6692913385826771977, 8.415575281601705876E-17 ) ) ;
#2450=CARTESIAN_POINT ( 'NONE',  ( 1.555118110236221041, 0.1660481256975883668, -0.3530559997133364547 ) ) ;
#2451=CARTESIAN_POINT ( 'NONE',  ( 1.259842519685040019, -0.1870078740157480879, -0.4822834645669291653 ) ) ;
#2452=CARTESIAN_POINT ( 'NONE',  ( -0.6299212598425188991, -0.1870078740157479769, 0.3641732283464567677 ) ) ;
#2453=CARTESIAN_POINT ( 'NONE',  ( -1.092353285368623750, -2.191421614605370878E-15, 0.4445507791589071167 ) ) ;
#2457=CARTESIAN_POINT ( 'NONE',  ( 0.9711286089238851948, 0.1283753931104748280, 0.1820866141732283561 ) ) ;
#2459=CARTESIAN_POINT ( 'NONE',  ( 0.9645669291338588858, 0.1660481256975885056, 0.3530559997133364547 ) ) ;
#2461=CARTESIAN_POINT ( 'NONE',  ( 1.200787401574803681, 0.07958543189024085140, 0.2665933059059887866 ) ) ;
#2462=CARTESIAN_POINT ( 'NONE',  ( 0.01312335958005323398, -0.4281496062992127816, -0.4176697321401328100 ) ) ;
#2463=CARTESIAN_POINT ( 'NONE',  ( -0.5905511811023613777, -0.6692913385826771977, 8.415575281601705876E-17 ) ) ;
#2464=CARTESIAN_POINT ( 'NONE',  ( 1.574803149606299746, -0.1870078740157480879, -0.4822834645669291653 ) ) ;
#2466=CARTESIAN_POINT ( 'NONE',  ( 0.5183727034120741983, 0.1771653543307087075, -0.09757992244046823083 ) ) ;
#2467=ORIENTED_EDGE ( 'NONE', *, *, #42363, .F. ) ;
#2470=CARTESIAN_POINT ( 'NONE',  ( -0.4330708661417315697, 0.2952755905511811885, 0.000000000000000000 ) ) ;
#2471=CARTESIAN_POINT ( 'NONE',  ( 1.305774278215223960, 0.2952755905511810774, -0.1292274648535930714 ) ) ;
#2472=CARTESIAN_POINT ( 'NONE',  ( 0.1443569553805781891, 0.05413385826771626580, -0.4176697321401330321 ) ) ;
#2473=CARTESIAN_POINT ( 'NONE',  ( -0.4986876640419939388, 0.1283753931104746893, -0.1820866141732285504 ) ) ;
#2474=CARTESIAN_POINT ( 'NONE',  ( 0.6561679790026253567, -0.6046776061558809534, -0.2411417322834644161 ) ) ;
#2475=CARTESIAN_POINT ( 'NONE',  ( -0.9186351706036736120, -0.6046776061558809534, -0.2411417322834644161 ) ) ;
#2476=CARTESIAN_POINT ( 'NONE',  ( -0.4133858267716528645, 0.1660481256975883668, -0.3530559997133364547 ) ) ;
#2477=CARTESIAN_POINT ( 'NONE',  ( -0.7874015748031489847, -0.1870078740157479769, 0.4822834645669291653 ) ) ;
#2478=CARTESIAN_POINT ( 'NONE',  ( 1.108923884514436242, -0.05778040916215522460, 0.4822834645669289988 ) ) ;
#2479=CARTESIAN_POINT ( 'NONE',  ( 0.7611548556430451917, -0.6046776061558807314, 0.2411417322834647770 ) ) ;
#2480=CARTESIAN_POINT ( 'NONE',  ( 0.8989501312335964611, 0.2952755905511811885, 0.1292274648535926551 ) ) ;
#2482=CARTESIAN_POINT ( 'NONE',  ( 0.1968503937007881344, -0.5511811023622047445, 6.969142054262312111E-17 ) ) ;
#2485=ORIENTED_EDGE ( 'NONE', *, *, #41074, .T. ) ;
#2486=CARTESIAN_POINT ( 'NONE',  ( -1.010498687664041384, -0.3690944881889765550, -0.3153832671262227771 ) ) ;
#2487=CARTESIAN_POINT ( 'NONE',  ( -0.1443569553805765515, -0.4281496062992127816, -0.4176697321401328100 ) ) ;
#2489=CARTESIAN_POINT ( 'NONE',  ( -0.1574803149606292529, -0.1870078740157479769, 0.4822834645669291653 ) ) ;
#2490=CARTESIAN_POINT ( 'NONE',  ( -0.3149606299212590610, -0.1870078740157479769, 0.4822834645669291653 ) ) ;
#2491=CARTESIAN_POINT ( 'NONE',  ( -1.489501312335957062, -0.05778040916215522460, 0.4822834645669289988 ) ) ;
#2492=CARTESIAN_POINT ( 'NONE',  ( -1.469816272965878357, -0.6046776061558809534, -0.2411417322834644161 ) ) ;
#2493=CARTESIAN_POINT ( 'NONE',  ( 1.410761154855643795, -0.08942795157528024563, -0.3641732283464568787 ) ) ;
#2496=CARTESIAN_POINT ( 'NONE',  ( 0.6758530183727039509, 0.1771653543307087075, -0.09757992244046823083 ) ) ;
#2498=CARTESIAN_POINT ( 'NONE',  ( 0.1902887139107617975, -0.6692913385826773087, -0.1292274648535924053 ) ) ;
#2499=CARTESIAN_POINT ( 'NONE',  ( 0.3018372703412079971, 0.05413385826771626580, -0.4176697321401330321 ) ) ;
#2502=CARTESIAN_POINT ( 'NONE',  ( -0.5774278215223089816, 0.2306618581243847221, -0.2411417322834647770 ) ) ;
#2505=CARTESIAN_POINT ( 'NONE',  ( -0.7545931758530177724, 0.2952755905511811885, 0.1292274648535926551 ) ) ;
#2508=CARTESIAN_POINT ( 'NONE',  ( -1.541994750656167090, -0.5511811023622048555, -0.09757992244046775898 ) ) ;
#2509=CARTESIAN_POINT ( 'NONE',  ( 0.7808398950131240079, -0.3162353388693405765, 0.4822834645669290543 ) ) ;
#2510=CARTESIAN_POINT ( 'NONE',  ( 0.7677165354330716118, 0.1660481256975883668, -0.3530559997133364547 ) ) ;
#2511=CARTESIAN_POINT ( 'NONE',  ( -0.04593175853018302557, 0.1771653543307087630, 0.09757992244046791164 ) ) ;
#2512=CARTESIAN_POINT ( 'NONE',  ( -0.05249343832020938322, -0.6046776061558809534, -0.2411417322834644161 ) ) ;
#2514=CARTESIAN_POINT ( 'NONE',  ( -0.2099737532808391705, 0.1283753931104748280, 0.1820866141732283561 ) ) ;
#2515=CARTESIAN_POINT ( 'NONE',  ( -0.4921259842519677963, -0.5400638737290844871, 0.3530559997133364547 ) ) ;
#2518=CARTESIAN_POINT ( 'NONE',  ( -1.692913385826770645, 0.2952755905511811885, 0.000000000000000000 ) ) ;
#2519=CARTESIAN_POINT ( 'NONE',  ( 0.08530183727034192087, -0.2845877964562161244, -0.3641732283464567121 ) ) ;
#2520=CARTESIAN_POINT ( 'NONE',  ( 1.692913385826772421, 0.1771653543307087630, 0.000000000000000000 ) ) ;
#2521=CARTESIAN_POINT ( 'NONE',  ( -1.062992125984250968, 0.2952755905511811885, 0.000000000000000000 ) ) ;
#2522=CARTESIAN_POINT ( 'NONE',  ( -0.5971128608923877978, -0.5511811023622048555, -0.09757992244046775898 ) ) ;
#2524=CARTESIAN_POINT ( 'NONE',  ( -0.6233595800524928121, -0.05778040916215522460, 0.4822834645669289988 ) ) ;
#2525=CARTESIAN_POINT ( 'NONE',  ( -0.6233595800524928121, -0.3162353388693409650, -0.4822834645669289433 ) ) ;
#2526=CARTESIAN_POINT ( 'NONE',  ( -0.09186351706036663400, -0.4281496062992124485, 0.4176697321401328655 ) ) ;
#2530=CARTESIAN_POINT ( 'NONE',  ( 0.4724409448818904789, -0.1870078740157480601, -0.3641732283464567677 ) ) ;
#2531=CARTESIAN_POINT ( 'NONE',  ( 1.082677165354331228, -0.5400638737290844871, 0.3530559997133364547 ) ) ;
#2532=CARTESIAN_POINT ( 'NONE',  ( -1.167979002624671470, -0.3690944881889765550, -0.3153832671262227771 ) ) ;
#2533=CARTESIAN_POINT ( 'NONE',  ( 1.266404199475066328, -0.3162353388693409650, -0.4822834645669289433 ) ) ;
#2534=CARTESIAN_POINT ( 'NONE',  ( -1.286089238845143479, -0.5023911411419708095, 0.1820866141732285504 ) ) ;
#2535=CARTESIAN_POINT ( 'NONE',  ( -0.4330708661417315697, 0.2952755905511811885, 0.000000000000000000 ) ) ;
#2536=CARTESIAN_POINT ( 'NONE',  ( 0.1574803149606306130, -0.1870078740157480601, -0.3641732283464567677 ) ) ;
#2537=CARTESIAN_POINT ( 'NONE',  ( 1.606179739637289439, 0.2952685183143916592, 0.01196341948705389145 ) ) ;
#2538=CARTESIAN_POINT ( 'NONE',  ( 0.6955380577427828781, -0.004921259842519870586, -0.3153832671262229437 ) ) ;
#2539=CARTESIAN_POINT ( 'NONE',  ( 0.2230971128608932319, -0.4281496062992124485, 0.4176697321401328655 ) ) ;
#2541=CARTESIAN_POINT ( 'NONE',  ( -0.8267716535433065062, -0.6692913385826771977, 8.415575281601705876E-17 ) ) ;
#2543=CARTESIAN_POINT ( 'NONE',  ( 1.141732283464567566, 0.1771653543307087630, 0.000000000000000000 ) ) ;
#2544=CARTESIAN_POINT ( 'NONE',  ( 0.2230971128608932319, -0.4281496062992124485, 0.4176697321401328655 ) ) ;
#2545=CARTESIAN_POINT ( 'NONE',  ( -0.3477690288713902178, 0.2952755905511810774, -0.1292274648535930714 ) ) ;
#2546=CARTESIAN_POINT ( 'NONE',  ( -0.4658792650918627265, -0.2845877964562161244, -0.3641732283464567121 ) ) ;
#2548=CARTESIAN_POINT ( 'NONE',  ( -0.01968503937007793844, 0.07958543189024071263, -0.2665933059059888421 ) ) ;
#2549=CARTESIAN_POINT ( 'NONE',  ( 0.3412073490813655186, -0.6046776061558809534, -0.2411417322834644161 ) ) ;
#2550=CARTESIAN_POINT ( 'NONE',  ( -0.7086614173228339419, -0.1870078740157480601, -0.3641732283464567677 ) ) ;
#2552=CARTESIAN_POINT ( 'NONE',  ( -1.253280839895012377, -0.3162353388693409650, -0.4822834645669289433 ) ) ;
#2553=CARTESIAN_POINT ( 'NONE',  ( -0.8550440751474861489, -4.966502543501560364E-15, 0.3954985857520076920 ) ) ;
#2554=ORIENTED_EDGE ( 'NONE', *, *, #42674, .T. ) ;
#2555=CARTESIAN_POINT ( 'NONE',  ( -1.049868766404198794, 0.1283753931104746893, -0.1820866141732285504 ) ) ;
#2556=CARTESIAN_POINT ( 'NONE',  ( 0.1181102362204730916, -0.6692913385826771977, 8.415575281601705876E-17 ) ) ;
#2557=CARTESIAN_POINT ( 'NONE',  ( -1.627296587926508442, -0.6046776061558809534, -0.2411417322834644161 ) ) ;
#2558=CARTESIAN_POINT ( 'NONE',  ( -0.6692913385826764205, 0.2952755905511811885, 0.000000000000000000 ) ) ;
#2560=CARTESIAN_POINT ( 'NONE',  ( 1.358267716535433323, 0.1660481256975885056, 0.3530559997133364547 ) ) ;
#2561=CARTESIAN_POINT ( 'NONE',  ( 0.7020997375328090762, -0.3162353388693405765, 0.4822834645669290543 ) ) ;
#2562=CARTESIAN_POINT ( 'NONE',  ( -0.2559055118110230564, 0.1012011053420775880, -0.2882089793578257453 ) ) ;
#2565=CARTESIAN_POINT ( 'NONE',  ( -1.607611548556429737, -0.6692913385826771977, 0.1292274648535927661 ) ) ;
#2568=CARTESIAN_POINT ( 'NONE',  ( -0.4658792650918627265, -0.2845877964562161244, -0.3641732283464567121 ) ) ;
#2571=CARTESIAN_POINT ( 'NONE',  ( 1.023622047244095112, -0.1870078740157480879, -0.4822834645669291653 ) ) ;
#2572=CARTESIAN_POINT ( 'NONE',  ( 0.07874015748031558404, -0.1870078740157480879, -0.4822834645669291653 ) ) ;
#2573=CARTESIAN_POINT ( 'NONE',  ( -0.6299212598425188991, -0.1870078740157480879, -0.4822834645669291653 ) ) ;
#2574=CARTESIAN_POINT ( 'NONE',  ( 1.614173228346457378, -0.6692913385826771977, 8.415575281601705876E-17 ) ) ;
#2575=CARTESIAN_POINT ( 'NONE',  ( -0.7808398950131222316, -0.2845877964562161244, -0.3641732283464567121 ) ) ;
#2577=CARTESIAN_POINT ( 'NONE',  ( 0.3280839895013130669, -0.4281496062992127816, -0.4176697321401328100 ) ) ;
#2578=CARTESIAN_POINT ( 'NONE',  ( 0.4068241469816279987, -0.3690944881889765550, -0.3153832671262227771 ) ) ;
#2579=CARTESIAN_POINT ( 'NONE',  ( -0.6299212598425188991, -0.1870078740157480879, -0.4822834645669291653 ) ) ;
#2581=CARTESIAN_POINT ( 'NONE',  ( -1.154855643044618851, 0.2306618581243848609, 0.2411417322834645549 ) ) ;
#2582=DIRECTION ( 'NONE',  ( -3.096699300667737957E-16, 1.000000000000000000, -0.000000000000000000 ) ) ;
#2583=CARTESIAN_POINT ( 'NONE',  ( 1.010498687664042716, -0.4281496062992124485, 0.4176697321401328655 ) ) ;
#2584=CARTESIAN_POINT ( 'NONE',  ( 1.148293963254593875, -0.5511811023622046335, 0.09757992244046803654 ) ) ;
#2587=CARTESIAN_POINT ( 'NONE',  ( -0.5183727034120726440, 0.2952755905511811885, 0.1292274648535926551 ) ) ;
#2588=VERTEX_POINT ( 'NONE', #46392 ) ;
#2589=CARTESIAN_POINT ( 'NONE',  ( 0.4790026246719167324, -0.08942795157527998196, 0.3641732283464567121 ) ) ;
#2590=CARTESIAN_POINT ( 'NONE',  ( -1.246719160104986512, 0.05413385826771666132, 0.4176697321401328100 ) ) ;
#2591=CARTESIAN_POINT ( 'NONE',  ( 0.8792650918635177559, -0.4281496062992127816, -0.4176697321401328100 ) ) ;
#2592=CARTESIAN_POINT ( 'NONE',  ( 0.6561679790026253567, 0.2306618581243848609, 0.2411417322834645549 ) ) ;
#2593=( BOUNDED_SURFACE ( )  B_SPLINE_SURFACE ( 1, 2, ( 
 ( #66691, #9026, #79743, #22059, #70181, #12534, #30022, #67931, #80577, #22887, #49380, #68751, #80162, #48140, #55686, #48552, #29613, #68348, #75076, #11093, #61184, #17423, #42651, #73837, #10272, #56104, #61609, #3952, #43054, #36750, #28788, #42237, #55274, #67104, #9435, #35105, #74249, #23709, #81393, #10688, #16592, #35940, #54450, #80984, #62426, #81808, #60771, #3122, #22479, #67514, #16177, #4763, #30439, #23297, #41824, #47721, #35522, #73419, #9851, #48967, #3538, #29205, #54871, #74667, #17011, #36343, #62018, #4354, #15768, #41420, #5184, #18643, #63665, #43464, #69161, #11512, #50605, #115, #32092, #44695, #82619, #44287, #30848, #6005, #57753, #58171, #37168, #62848, #56513, #43877, #50200, #51431, #45117, #69575, #25354, #24935, #11923, #69977, #37578, #12332, #25770, #70825, #82216, #83031, #24534, #51016, #75897, #64086, #18237, #63251, #76715, #24120, #5591, #31257, #56925, #77134, #13172, #19048, #57335, #38822, #70392, #64500, #32508, #76312, #37989, #31674, #12747, #38406, #49789, #6423, #19467, #6838, #75491, #17830, #14008, #21146, #58598, #59023, #72904, #64923, #967, #26621, #52275, #32933, #7261, #77979, #14841, #65773, #46801, #72075, #77561, #46382, #66182, #14434, #72492, #27447, #20309, #59432, #40501, #34186, #39665, #7693, #2202, #65355, #33360, #52691, #1379, #53108, #27030, #78817, #39238, #45959, #66597, #26193, #8519, #20731, #78399, #40086, #27870, #21553, #71656, #8105, #59850, #33771, #1787, #53530, #79238, #47214, #15256, #40915, #8931, #34608, #540, #51854, #19895, #45542, #71240, #13584, #15673, #3031, #42961, #2623, #42555, #80482, #9757, #35429, #61920, #81300, #9347, #60682, #68259, #61094, #42146, #80889, #4262, #23614, #73749, #29925, #55180, #28697, #22795, #68655, #74155, #16502, #55588, #49283, #41334, #54779, #67841, #79653, #21970, #47632, #3445, #36251, #10595, #23202, #29109, #48455, #67014, #10180, #74986, #10992, #73326, #35018, #54359, #80071, #22388, #17331, #60273, #48048, #61514, #35845, #16085, #3859, #41730, #29519, #28279, #53941, #67424, #48873, #74573, #16918, #37068, #76618, #62753, #69063, #5903, #70715, #30757, #5089, #56419, #6315, #25669, #31575, #69882, #15, #12236, #77033, #45015, #43774, #11830, #31158, #50507, #57230, #36653, #18949, #31992, #76211, #4665, #18547, #50101, #82932, #11413, #37483, #51329, #17734, #82119, #24434, #75797, #18140, #43362, #69477, #50918, #44192, #25254, #24839, #30338, #82522, #44596, #37892, #70291, #63568, #63156, #12643, #38305, #63979, #5496, #56825, #57653, #19365, #62328, #56004, #81715, #24025, #49693, #75388, #6734, #26089, #71134, #32405, #58067, #19787, #46279, #33668, #72393, #77452, #45855, #71975, #33258, #13066, #13477, #51749, #434, #47111, #71553, #38720, #14743, #45439, #78716, #32827, #39135, #8004, #53429, #64398, #8414, #20628, #66078, #64815, #14329, #13902, #40396, #21041, #7156, #46700, #39987, #52588, #78296, #58495, #39560, #58920, #859, #26516, #52171, #34081, #26928, #20204, #77874, #59745, #65677, #65249, #7586, #59330, #1279, #2099, #1686, #27345, #53003, #27764, #79137, #21454, #21863, #80786, #3755, #40807, #23102, #15988, #60992, #41635, #54254, #29419, #8826, #66491, #74051, #67325, #2933, #4162, #34503, #60167, #2521, #3341, #41229, #48770, #29005, #35329, #79970, #28179, #23515, #54671, #66916, #53836, #29827, #60582, #55490, #79550, #80382, #34920, #15569, #73219, #28597, #47528, #9248, #22283, #74469, #16816, #42452, #61822, #55078, #47943, #73646, #9659, #22695, #68152, #10496, #16399, #48354, #72801, #42045, #67741, #10074, #35738, #61406, #36150, #81200, #15150, #69793, #37392, #42863, #11737, #31478, #63064, #12139, #76116, #17636, #24749, #37795, #82836, #4995, #56326, #50826, #30663, #82025, #18047, #50008, #18457, #24338, #44100, #4572, #75293, #31895, #74887, #57139, #69383, #75706, #43680, #76528, #70193, #81618, #49599, #25158, #5401, #31064, #63473, #18856, #12548, #62654, #44503, #5808, #43268, #56732, #57556, #82430, #50416, #38206, #63880, #30243, #6219, #83247, #68556, #10897, #36557, #49184 ),
 ( #17233, #62234, #68966, #55906, #23932, #36974, #11315, #45343, #20110, #27247, #72297, #32308, #1181, #57969, #26832, #25991, #65574, #51649, #336, #78198, #59646, #19685, #77353, #71039, #78620, #14643, #20529, #58824, #40299, #52490, #65980, #33984, #32729, #756, #45758, #39462, #46181, #25570, #7908, #20943, #65149, #76934, #7485, #39036, #71878, #13383, #26417, #8317, #6636, #64719, #7060, #58396, #52070, #52906, #64302, #33569, #77777, #71455, #14227, #51235, #19262, #46601, #33155, #44915, #70612, #39887, #13804, #12967, #59231, #1592, #38624, #60894, #41541, #67230, #60069, #28494, #22186, #53330, #15471, #36056, #35644, #15892, #9152, #21765, #80694, #3245, #34825, #54154, #35230, #79869, #74370, #48260, #47843, #73956, #79039, #9560, #60482, #34401, #9974, #16303, #21358, #61304, #73549, #28909, #54572, #66819, #41945, #47011, #72705, #80286, #22599, #41128, #16714, #15052, #40708, #66393, #67641, #53738, #3662, #29325, #54986, #2833, #8731, #2002, #23007, #79446, #2424, #42354, #73120, #68052, #28080, #48674, #47428, #10399, #27664, #17539, #81101, #17135, #55394, #69694, #37694, #12037, #50728, #76015, #81512, #75195, #23834, #62554, #31375, #5703, #62967, #81927, #61728, #5305, #17947, #23418, #29732, #68463, #76427, #37292, #44399, #49084, #74784, #36461, #42767, #10801, #62135, #11632, #82332, #63369, #4475, #11216, #30964, #24238, #4065, #30145, #55806, #49502, #12445, #36876, #43171, #68867, #4889, #30563, #56229, #18357, #43584, #24650, #49911, #75608, #69285, #44001, #56631, #50318, #57040, #82734, #25053, #18755, #70091, #77249, #45238, #39774, #19578, #70938, #6953, #38935, #65037, #13283, #33042, #76827, #64204, #20839, #63780, #20423, #58285, #64615, #32623, #65469, #59130, #70506, #38521, #46076, #651, #20004, #58711, #7803, #1487, #51545, #33468, #1076, #6538, #26308, #46491, #51966, #77674, #27141, #52805, #19160, #45655, #71350, #57454, #83147, #25467, #13697, #14122, #71769, #26729, #39353, #7373, #44810, #52383, #78515, #72186, #51133, #12864, #32208, #57866, #233, #38104, #6119, #25884, #78092, #31791, #2317, #9045, #34300, #34720, #16197, #62340, #21252, #73437, #46907, #15787, #14948, #54470, #40607, #72602, #67123, #49706, #8629, #66290, #59961, #67533, #4679, #9453, #47739, #30350, #41439, #56019, #24036, #21663, #73014, #60380, #28389, #35124, #14544, #80183, #9871, #54049, #65879, #79763, #27977, #60790, #53635, #15365, #81727, #78930, #79343, #47323, #59545, #33879, #41026, #73856, #22498, #3143, #66712, #2728, #22080, #28806, #48161, #40196, #1900, #27561, #53220, #41843, #35540, #8214, #13081, #11840, #76628, #76225, #63168, #69892, #37493, #12246, #77044, #38734, #82131, #50930, #24445, #18959, #75810, #32005, #18153, #50113, #44607, #26101, #69491, #43785, #5506, #45028, #64411, #70303, #25264, #6746, #12656, #32418, #446, #82533, #50519, #37902, #5913, #38317, #75401, #57665, #70727, #31587, #43376, #57242, #31169, #63991, #56835, #18558, #58080, #56429, #24851, #44202, #63579, #82946, #6332, #27, #25680, #51340, #19376, #17747, #69076, #11426, #37080, #62767, #5101, #30768, #20219, #27357, #40410, #2113, #7599, #58933, #53442, #33273, #1291, #20640, #52602, #78730, #26940, #46714, #7169, #77888, #34516, #77465, #34095, #71988, #78308, #46292, #79150, #72815, #872, #52184, #59758, #14341, #33680, #72406, #21467, #15164, #65263, #47125, #14755, #45868, #40001, #60181, #65689, #8017, #40821, #66506, #32840, #59342, #1699, #71149, #71566, #53016, #13916, #21054, #8840, #2534, #66091, #8426, #51763, #27778, #19802, #45451, #13490, #58509, #39146, #64830, #26531, #39573, #41241, #2945, #47542, #73232, #34933, #61418, #48783, #4174, #9261, #61005, #3768, #48366, #28192, #28609, #66929, #15583, #62243, #3354, #53850, #29838, #60596, #10507, #47956, #54267, #23116, #68566, #79563, #23525, #35752, #81210, #79982, #29432, #29019, #55501, #36160, #22295, #61834, #55090, #67753, #10087, #73659, #54685, #74065, #21877, #41648, #16001, #49195, #42057, #35342, #67339, #74896, #80799, #80396, #22708, #74481, #16411 ) ),
 .UNSPECIFIED., .F., .F., .F. ) 
 B_SPLINE_SURFACE_WITH_KNOTS ( ( 2, 2 ),
 ( 3, 2, 2, 2, 2, 2, 2, 2, 2, 2, 2, 2, 2, 2, 2, 2, 2, 2, 2, 2, 2, 2, 2, 2, 2, 2, 2, 2, 2, 2, 2, 2, 2, 2, 2, 2, 2, 2, 2, 2, 2, 2, 2, 2, 2, 2, 2, 2, 2, 2, 2, 2, 2, 2, 2, 2, 2, 2, 2, 2, 2, 2, 2, 2, 2, 2, 2, 2, 2, 2, 2, 2, 2, 2, 2, 2, 2, 2, 2, 2, 2, 2, 2, 2, 2, 2, 2, 2, 2, 2, 2, 2, 2, 2, 2, 2, 2, 2, 2, 2, 2, 2, 2, 2, 2, 2, 2, 2, 2, 2, 2, 2, 2, 2, 2, 2, 2, 2, 2, 2, 2, 2, 2, 2, 2, 2, 2, 2, 2, 2, 2, 2, 2, 2, 2, 2, 2, 2, 2, 2, 2, 2, 2, 2, 2, 2, 2, 2, 2, 2, 2, 2, 2, 2, 2, 2, 2, 2, 2, 2, 2, 2, 2, 2, 2, 2, 2, 2, 2, 2, 2, 2, 2, 2, 2, 2, 2, 2, 2, 2, 2, 2, 2, 2, 2, 2, 2, 2, 2, 2, 2, 2, 2, 2, 2, 2, 2, 2, 2, 2, 2, 2, 2, 2, 2, 2, 2, 2, 2, 2, 2, 2, 2, 2, 2, 2, 2, 2, 2, 2, 2, 2, 2, 2, 2, 2, 2, 2, 2, 2, 2, 2, 2, 2, 2, 2, 2, 2, 2, 2, 2, 2, 2, 2, 2, 2, 2, 2, 2, 2, 2, 2, 2, 2, 2, 3 ),
 ( 0.000000000000000000, 1.000000000000000000 ),
 ( 0.000000000000000000, 0.003787878787878787984, 0.007575757575757575968, 0.01136363636363636395, 0.01515151515151515194, 0.01893939393939393992, 0.02272727272727272790, 0.02651515151515151589, 0.03030303030303030387, 0.03409090909090908839, 0.03787878787878787984, 0.04166666666666666435, 0.04545454545454545581, 0.04924242424242424032, 0.05303030303030303177, 0.05681818181818181629, 0.06060606060606060774, 0.06439393939393939226, 0.06818181818181817677, 0.07196969696969697516, 0.07575757575757575968, 0.07954545454545454419, 0.08333333333333332871, 0.08712121212121212710, 0.09090909090909091161, 0.09469696969696969613, 0.09848484848484848064, 0.1022727272727272790, 0.1060606060606060635, 0.1098484848484848481, 0.1136363636363636326, 0.1174242424242424310, 0.1212121212121212155, 0.1250000000000000000, 0.1287878787878787845, 0.1325757575757575690, 0.1363636363636363535, 0.1401515151515151381, 0.1439393939393939503, 0.1477272727272727348, 0.1515151515151515194, 0.1553030303030303039, 0.1590909090909090884, 0.1628787878787878729, 0.1666666666666666574, 0.1704545454545454419, 0.1742424242424242542, 0.1780303030303030387, 0.1818181818181818232, 0.1856060606060606077, 0.1893939393939393923, 0.1931818181818181768, 0.1969696969696969613, 0.2007575757575757458, 0.2045454545454545581, 0.2083333333333333426, 0.2121212121212121271, 0.2159090909090909116, 0.2196969696969696961, 0.2234848484848484806, 0.2272727272727272652, 0.2310606060606060497, 0.2348484848484848619, 0.2386363636363636465, 0.2424242424242424310, 0.2462121212121212155, 0.2500000000000000000, 0.2537878787878787845, 0.2575757575757575690, 0.2613636363636363535, 0.2651515151515151381, 0.2689393939393939226, 0.2727272727272727071, 0.2765151515151514916, 0.2803030303030302761, 0.2840909090909091161, 0.2878787878787879007, 0.2916666666666666852, 0.2954545454545454697, 0.2992424242424242542, 0.3030303030303030387, 0.3068181818181818232, 0.3106060606060606077, 0.3143939393939393923, 0.3181818181818181768, 0.3219696969696969613, 0.3257575757575757458, 0.3295454545454545303, 0.3333333333333333148, 0.3371212121212120993, 0.3409090909090908839, 0.3446969696969697239, 0.3484848484848485084, 0.3522727272727272929, 0.3560606060606060774, 0.3598484848484848619, 0.3636363636363636465, 0.3674242424242424310, 0.3712121212121212155, 0.3750000000000000000, 0.3787878787878787845, 0.3825757575757575690, 0.3863636363636363535, 0.3901515151515151381, 0.3939393939393939226, 0.3977272727272727071, 0.4015151515151514916, 0.4053030303030302761, 0.4090909090909091161, 0.4128787878787879007, 0.4166666666666666852, 0.4204545454545454697, 0.4242424242424242542, 0.4280303030303030387, 0.4318181818181818232, 0.4356060606060606077, 0.4393939393939393923, 0.4431818181818181768, 0.4469696969696969613, 0.4507575757575757458, 0.4545454545454545303, 0.4583333333333333148, 0.4621212121212120993, 0.4659090909090908839, 0.4696969696969697239, 0.4734848484848485084, 0.4772727272727272929, 0.4810606060606060774, 0.4848484848484848619, 0.4886363636363636465, 0.4924242424242424310, 0.4962121212121212155, 0.5000000000000000000, 0.5037878787878787845, 0.5075757575757575690, 0.5113636363636363535, 0.5151515151515151381, 0.5189393939393939226, 0.5227272727272727071, 0.5265151515151514916, 0.5303030303030302761, 0.5340909090909090606, 0.5378787878787878451, 0.5416666666666666297, 0.5454545454545454142, 0.5492424242424241987, 0.5530303030303029832, 0.5568181818181817677, 0.5606060606060605522, 0.5643939393939394478, 0.5681818181818182323, 0.5719696969696970168, 0.5757575757575758013, 0.5795454545454545858, 0.5833333333333333703, 0.5871212121212121549, 0.5909090909090909394, 0.5946969696969697239, 0.5984848484848485084, 0.6022727272727272929, 0.6060606060606060774, 0.6098484848484848619, 0.6136363636363636465, 0.6174242424242424310, 0.6212121212121212155, 0.6250000000000000000, 0.6287878787878787845, 0.6325757575757575690, 0.6363636363636363535, 0.6401515151515151381, 0.6439393939393939226, 0.6477272727272727071, 0.6515151515151514916, 0.6553030303030302761, 0.6590909090909090606, 0.6628787878787878451, 0.6666666666666666297, 0.6704545454545454142, 0.6742424242424241987, 0.6780303030303029832, 0.6818181818181817677, 0.6856060606060605522, 0.6893939393939394478, 0.6931818181818182323, 0.6969696969696970168, 0.7007575757575758013, 0.7045454545454545858, 0.7083333333333333703, 0.7121212121212121549, 0.7159090909090909394, 0.7196969696969697239, 0.7234848484848485084, 0.7272727272727272929, 0.7310606060606060774, 0.7348484848484848619, 0.7386363636363636465, 0.7424242424242424310, 0.7462121212121212155, 0.7500000000000000000, 0.7537878787878787845, 0.7575757575757575690, 0.7613636363636363535, 0.7651515151515151381, 0.7689393939393939226, 0.7727272727272727071, 0.7765151515151514916, 0.7803030303030302761, 0.7840909090909090606, 0.7878787878787878451, 0.7916666666666666297, 0.7954545454545454142, 0.7992424242424241987, 0.8030303030303029832, 0.8068181818181817677, 0.8106060606060605522, 0.8143939393939394478, 0.8181818181818182323, 0.8219696969696970168, 0.8257575757575758013, 0.8295454545454545858, 0.8333333333333333703, 0.8371212121212121549, 0.8409090909090909394, 0.8446969696969697239, 0.8484848484848485084, 0.8522727272727272929, 0.8560606060606060774, 0.8598484848484848619, 0.8636363636363636465, 0.8674242424242424310, 0.8712121212121212155, 0.8750000000000000000, 0.8787878787878787845, 0.8825757575757575690, 0.8863636363636363535, 0.8901515151515151381, 0.8939393939393939226, 0.8977272727272727071, 0.9015151515151514916, 0.9053030303030302761, 0.9090909090909090606, 0.9128787878787878451, 0.9166666666666666297, 0.9204545454545454142, 0.9242424242424241987, 0.9280303030303029832, 0.9318181818181817677, 0.9356060606060605522, 0.9393939393939394478, 0.9431818181818182323, 0.9469696969696970168, 0.9507575757575758013, 0.9545454545454545858, 0.9583333333333333703, 0.9621212121212121549, 0.9659090909090909394 ),
 .UNSPECIFIED. ) 
 GEOMETRIC_REPRESENTATION_ITEM ( )  RATIONAL_B_SPLINE_SURFACE ( (
 ( 1.000000000000000000, 0.9659258262890683122, 1.000000000000000000, 0.9659258262890683122, 1.000000000000000000, 0.9659258262890683122, 1.000000000000000000, 0.9659258262890683122, 1.000000000000000000, 0.9659258262890683122, 1.000000000000000000, 0.9659258262890683122, 1.000000000000000000, 0.9659258262890683122, 1.000000000000000000, 0.9659258262890683122, 1.000000000000000000, 0.9659258262890683122, 1.000000000000000000, 0.9659258262890683122, 1.000000000000000000, 0.9659258262890683122, 1.000000000000000000, 0.9659258262890683122, 1.000000000000000000, 0.9659258262890683122, 1.000000000000000000, 0.9659258262890683122, 1.000000000000000000, 0.9659258262890683122, 1.000000000000000000, 0.9659258262890683122, 1.000000000000000000, 0.9659258262890683122, 1.000000000000000000, 0.9659258262890683122, 1.000000000000000000, 0.9659258262890683122, 1.000000000000000000, 0.9659258262890683122, 1.000000000000000000, 0.9659258262890683122, 1.000000000000000000, 0.9659258262890683122, 1.000000000000000000, 0.9659258262890683122, 1.000000000000000000, 0.9659258262890683122, 1.000000000000000000, 0.9659258262890683122, 1.000000000000000000, 0.9659258262890683122, 1.000000000000000000, 0.9659258262890683122, 1.000000000000000000, 0.9659258262890683122, 1.000000000000000000, 0.9659258262890683122, 1.000000000000000000, 0.9659258262890683122, 1.000000000000000000, 0.9659258262890683122, 1.000000000000000000, 0.9659258262890683122, 1.000000000000000000, 0.9659258262890683122, 1.000000000000000000, 0.9659258262890683122, 1.000000000000000000, 0.9659258262890683122, 1.000000000000000000, 0.9659258262890683122, 1.000000000000000000, 0.9659258262890683122, 1.000000000000000000, 0.9659258262890683122, 1.000000000000000000, 0.9659258262890683122, 1.000000000000000000, 0.9659258262890683122, 1.000000000000000000, 0.9659258262890683122, 1.000000000000000000, 0.9659258262890683122, 1.000000000000000000, 0.9659258262890683122, 1.000000000000000000, 0.9659258262890683122, 1.000000000000000000, 0.9659258262890683122, 1.000000000000000000, 0.9659258262890683122, 1.000000000000000000, 0.9659258262890683122, 1.000000000000000000, 0.9659258262890683122, 1.000000000000000000, 0.9659258262890683122, 1.000000000000000000, 0.9659258262890683122, 1.000000000000000000, 0.9659258262890683122, 1.000000000000000000, 0.9659258262890683122, 1.000000000000000000, 0.9659258262890683122, 1.000000000000000000, 0.9659258262890683122, 1.000000000000000000, 0.9659258262890683122, 1.000000000000000000, 0.9659258262890683122, 1.000000000000000000, 0.9659258262890683122, 1.000000000000000000, 0.9659258262890683122, 1.000000000000000000, 0.9659258262890683122, 1.000000000000000000, 0.9659258262890683122, 1.000000000000000000, 0.9659258262890683122, 1.000000000000000000, 0.9659258262890683122, 1.000000000000000000, 0.9659258262890683122, 1.000000000000000000, 0.9659258262890683122, 1.000000000000000000, 0.9659258262890683122, 1.000000000000000000, 0.9659258262890683122, 1.000000000000000000, 0.9659258262890683122, 1.000000000000000000, 0.9659258262890683122, 1.000000000000000000, 0.9659258262890683122, 1.000000000000000000, 0.9659258262890683122, 1.000000000000000000, 0.9659258262890683122, 1.000000000000000000, 0.9659258262890683122, 1.000000000000000000, 0.9659258262890683122, 1.000000000000000000, 0.9659258262890683122, 1.000000000000000000, 0.9659258262890683122, 1.000000000000000000, 0.9659258262890683122, 1.000000000000000000, 0.9659258262890683122, 1.000000000000000000, 0.9659258262890683122, 1.000000000000000000, 0.9659258262890683122, 1.000000000000000000, 0.9659258262890683122, 1.000000000000000000, 0.9659258262890683122, 1.000000000000000000, 0.9659258262890683122, 1.000000000000000000, 0.9659258262890683122, 1.000000000000000000, 0.9659258262890683122, 1.000000000000000000, 0.9659258262890683122, 1.000000000000000000, 0.9659258262890683122, 1.000000000000000000, 0.9659258262890683122, 1.000000000000000000, 0.9659258262890683122, 1.000000000000000000, 0.9659258262890683122, 1.000000000000000000, 0.9659258262890683122, 1.000000000000000000, 0.9659258262890683122, 1.000000000000000000, 0.9659258262890683122, 1.000000000000000000, 0.9659258262890683122, 1.000000000000000000, 0.9659258262890683122, 1.000000000000000000, 0.9659258262890683122, 1.000000000000000000, 0.9659258262890683122, 1.000000000000000000, 0.9659258262890683122, 1.000000000000000000, 0.9659258262890683122, 1.000000000000000000, 0.9659258262890683122, 1.000000000000000000, 0.9659258262890683122, 1.000000000000000000, 0.9659258262890683122, 1.000000000000000000, 0.9659258262890683122, 1.000000000000000000, 0.9659258262890683122, 1.000000000000000000, 0.9659258262890683122, 1.000000000000000000, 0.9659258262890683122, 1.000000000000000000, 0.9659258262890683122, 1.000000000000000000, 0.9659258262890683122, 1.000000000000000000, 0.9659258262890683122, 1.000000000000000000, 0.9659258262890683122, 1.000000000000000000, 0.9659258262890683122, 1.000000000000000000, 0.9659258262890683122, 1.000000000000000000, 0.9659258262890683122, 1.000000000000000000, 0.9659258262890683122, 1.000000000000000000, 0.9659258262890683122, 1.000000000000000000, 0.9659258262890683122, 1.000000000000000000, 0.9659258262890683122, 1.000000000000000000, 0.9659258262890683122, 1.000000000000000000, 0.9659258262890683122, 1.000000000000000000, 0.9659258262890683122, 1.000000000000000000, 0.9659258262890683122, 1.000000000000000000, 0.9659258262890683122, 1.000000000000000000, 0.9659258262890683122, 1.000000000000000000, 0.9659258262890683122, 1.000000000000000000, 0.9659258262890683122, 1.000000000000000000, 0.9659258262890683122, 1.000000000000000000, 0.9659258262890683122, 1.000000000000000000, 0.9659258262890683122, 1.000000000000000000, 0.9659258262890683122, 1.000000000000000000, 0.9659258262890683122, 1.000000000000000000, 0.9659258262890683122, 1.000000000000000000, 0.9659258262890683122, 1.000000000000000000, 0.9659258262890683122, 1.000000000000000000, 0.9659258262890683122, 1.000000000000000000, 0.9659258262890683122, 1.000000000000000000, 0.9659258262890683122, 1.000000000000000000, 0.9659258262890683122, 1.000000000000000000, 0.9659258262890683122, 1.000000000000000000, 0.9659258262890683122, 1.000000000000000000, 0.9659258262890683122, 1.000000000000000000, 0.9659258262890683122, 1.000000000000000000, 0.9659258262890683122, 1.000000000000000000, 0.9659258262890683122, 1.000000000000000000, 0.9659258262890683122, 1.000000000000000000, 0.9659258262890683122, 1.000000000000000000, 0.9659258262890683122, 1.000000000000000000, 0.9659258262890683122, 1.000000000000000000, 0.9659258262890683122, 1.000000000000000000, 0.9659258262890683122, 1.000000000000000000, 0.9659258262890683122, 1.000000000000000000, 0.9659258262890683122, 1.000000000000000000, 0.9659258262890683122, 1.000000000000000000, 0.9659258262890683122, 1.000000000000000000, 0.9659258262890683122, 1.000000000000000000, 0.9659258262890683122, 1.000000000000000000, 0.9659258262890683122, 1.000000000000000000, 0.9659258262890683122, 1.000000000000000000, 0.9659258262890683122, 1.000000000000000000, 0.9659258262890683122, 1.000000000000000000, 0.9659258262890683122, 1.000000000000000000, 0.9659258262890683122, 1.000000000000000000, 0.9659258262890683122, 1.000000000000000000, 0.9659258262890683122, 1.000000000000000000, 0.9659258262890683122, 1.000000000000000000, 0.9659258262890683122, 1.000000000000000000, 0.9659258262890683122, 1.000000000000000000, 0.9659258262890683122, 1.000000000000000000, 0.9659258262890683122, 1.000000000000000000, 0.9659258262890683122, 1.000000000000000000, 0.9659258262890683122, 1.000000000000000000, 0.9659258262890683122, 1.000000000000000000, 0.9659258262890683122, 1.000000000000000000, 0.9659258262890683122, 1.000000000000000000, 0.9659258262890683122, 1.000000000000000000, 0.9659258262890683122, 1.000000000000000000, 0.9659258262890683122, 1.000000000000000000, 0.9659258262890683122, 1.000000000000000000, 0.9659258262890683122, 1.000000000000000000, 0.9659258262890683122, 1.000000000000000000, 0.9659258262890683122, 1.000000000000000000, 0.9659258262890683122, 1.000000000000000000, 0.9659258262890683122, 1.000000000000000000, 0.9659258262890683122, 1.000000000000000000, 0.9659258262890683122, 1.000000000000000000, 0.9659258262890683122, 1.000000000000000000, 0.9659258262890683122, 1.000000000000000000, 0.9659258262890683122, 1.000000000000000000, 0.9659258262890683122, 1.000000000000000000, 0.9659258262890683122, 1.000000000000000000, 0.9659258262890683122, 1.000000000000000000, 0.9659258262890683122, 1.000000000000000000, 0.9659258262890683122, 1.000000000000000000, 0.9659258262890683122, 1.000000000000000000, 0.9659258262890683122, 1.000000000000000000, 0.9659258262890683122, 1.000000000000000000, 0.9659258262890683122, 1.000000000000000000, 0.9659258262890683122, 1.000000000000000000, 0.9659258262890683122, 1.000000000000000000, 0.9659258262890683122, 1.000000000000000000, 0.9659258262890683122, 1.000000000000000000, 0.9659258262890683122, 1.000000000000000000, 0.9659258262890683122, 1.000000000000000000, 0.9659258262890683122, 1.000000000000000000, 0.9659258262890683122, 1.000000000000000000, 0.9659258262890683122, 1.000000000000000000, 0.9659258262890683122, 1.000000000000000000, 0.9659258262890683122, 1.000000000000000000, 0.9659258262890683122, 1.000000000000000000, 0.9659258262890683122, 1.000000000000000000, 0.9659258262890683122, 1.000000000000000000, 0.9659258262890683122, 1.000000000000000000, 0.9659258262890683122, 1.000000000000000000, 0.9659258262890683122, 1.000000000000000000, 0.9659258262890683122, 1.000000000000000000, 0.9659258262890683122, 1.000000000000000000, 0.9659258262890683122, 1.000000000000000000, 0.9659258262890683122, 1.000000000000000000, 0.9659258262890683122, 1.000000000000000000, 0.9659258262890683122, 1.000000000000000000, 0.9659258262890683122, 1.000000000000000000, 0.9659258262890683122, 1.000000000000000000, 0.9659258262890683122, 1.000000000000000000, 0.9659258262890683122, 1.000000000000000000, 0.9659258262890683122, 1.000000000000000000, 0.9659258262890683122, 1.000000000000000000, 0.9659258262890683122, 1.000000000000000000, 0.9659258262890683122, 1.000000000000000000, 0.9659258262890683122, 1.000000000000000000, 0.9659258262890683122, 1.000000000000000000, 0.9659258262890683122, 1.000000000000000000, 0.9659258262890683122, 1.000000000000000000, 0.9659258262890683122, 1.000000000000000000, 0.9659258262890683122, 1.000000000000000000, 0.9659258262890683122, 1.000000000000000000, 0.9659258262890683122, 1.000000000000000000, 0.9659258262890683122, 1.000000000000000000, 0.9659258262890683122, 1.000000000000000000, 0.9659258262890683122, 1.000000000000000000, 0.9659258262890683122, 1.000000000000000000, 0.9659258262890683122, 1.000000000000000000, 0.9659258262890683122, 1.000000000000000000, 0.9659258262890683122, 1.000000000000000000, 0.9659258262890683122, 1.000000000000000000, 0.9659258262890683122, 1.000000000000000000, 0.9659258262890683122, 1.000000000000000000, 0.9659258262890683122, 1.000000000000000000, 0.9659258262890683122, 1.000000000000000000, 0.9659258262890683122, 1.000000000000000000, 0.9659258262890683122, 1.000000000000000000, 0.9659258262890683122, 1.000000000000000000, 0.9659258262890683122, 1.000000000000000000, 0.9659258262890683122, 1.000000000000000000, 0.9659258262890683122, 1.000000000000000000, 0.9659258262890683122, 1.000000000000000000, 0.9659258262890683122, 1.000000000000000000, 0.9659258262890683122, 1.000000000000000000),
 ( 1.000000000000000000, 0.9659258262890683122, 1.000000000000000000, 0.9659258262890683122, 1.000000000000000000, 0.9659258262890683122, 1.000000000000000000, 0.9659258262890683122, 1.000000000000000000, 0.9659258262890683122, 1.000000000000000000, 0.9659258262890683122, 1.000000000000000000, 0.9659258262890683122, 1.000000000000000000, 0.9659258262890683122, 1.000000000000000000, 0.9659258262890683122, 1.000000000000000000, 0.9659258262890683122, 1.000000000000000000, 0.9659258262890683122, 1.000000000000000000, 0.9659258262890683122, 1.000000000000000000, 0.9659258262890683122, 1.000000000000000000, 0.9659258262890683122, 1.000000000000000000, 0.9659258262890683122, 1.000000000000000000, 0.9659258262890683122, 1.000000000000000000, 0.9659258262890683122, 1.000000000000000000, 0.9659258262890683122, 1.000000000000000000, 0.9659258262890683122, 1.000000000000000000, 0.9659258262890683122, 1.000000000000000000, 0.9659258262890683122, 1.000000000000000000, 0.9659258262890683122, 1.000000000000000000, 0.9659258262890683122, 1.000000000000000000, 0.9659258262890683122, 1.000000000000000000, 0.9659258262890683122, 1.000000000000000000, 0.9659258262890683122, 1.000000000000000000, 0.9659258262890683122, 1.000000000000000000, 0.9659258262890683122, 1.000000000000000000, 0.9659258262890683122, 1.000000000000000000, 0.9659258262890683122, 1.000000000000000000, 0.9659258262890683122, 1.000000000000000000, 0.9659258262890683122, 1.000000000000000000, 0.9659258262890683122, 1.000000000000000000, 0.9659258262890683122, 1.000000000000000000, 0.9659258262890683122, 1.000000000000000000, 0.9659258262890683122, 1.000000000000000000, 0.9659258262890683122, 1.000000000000000000, 0.9659258262890683122, 1.000000000000000000, 0.9659258262890683122, 1.000000000000000000, 0.9659258262890683122, 1.000000000000000000, 0.9659258262890683122, 1.000000000000000000, 0.9659258262890683122, 1.000000000000000000, 0.9659258262890683122, 1.000000000000000000, 0.9659258262890683122, 1.000000000000000000, 0.9659258262890683122, 1.000000000000000000, 0.9659258262890683122, 1.000000000000000000, 0.9659258262890683122, 1.000000000000000000, 0.9659258262890683122, 1.000000000000000000, 0.9659258262890683122, 1.000000000000000000, 0.9659258262890683122, 1.000000000000000000, 0.9659258262890683122, 1.000000000000000000, 0.9659258262890683122, 1.000000000000000000, 0.9659258262890683122, 1.000000000000000000, 0.9659258262890683122, 1.000000000000000000, 0.9659258262890683122, 1.000000000000000000, 0.9659258262890683122, 1.000000000000000000, 0.9659258262890683122, 1.000000000000000000, 0.9659258262890683122, 1.000000000000000000, 0.9659258262890683122, 1.000000000000000000, 0.9659258262890683122, 1.000000000000000000, 0.9659258262890683122, 1.000000000000000000, 0.9659258262890683122, 1.000000000000000000, 0.9659258262890683122, 1.000000000000000000, 0.9659258262890683122, 1.000000000000000000, 0.9659258262890683122, 1.000000000000000000, 0.9659258262890683122, 1.000000000000000000, 0.9659258262890683122, 1.000000000000000000, 0.9659258262890683122, 1.000000000000000000, 0.9659258262890683122, 1.000000000000000000, 0.9659258262890683122, 1.000000000000000000, 0.9659258262890683122, 1.000000000000000000, 0.9659258262890683122, 1.000000000000000000, 0.9659258262890683122, 1.000000000000000000, 0.9659258262890683122, 1.000000000000000000, 0.9659258262890683122, 1.000000000000000000, 0.9659258262890683122, 1.000000000000000000, 0.9659258262890683122, 1.000000000000000000, 0.9659258262890683122, 1.000000000000000000, 0.9659258262890683122, 1.000000000000000000, 0.9659258262890683122, 1.000000000000000000, 0.9659258262890683122, 1.000000000000000000, 0.9659258262890683122, 1.000000000000000000, 0.9659258262890683122, 1.000000000000000000, 0.9659258262890683122, 1.000000000000000000, 0.9659258262890683122, 1.000000000000000000, 0.9659258262890683122, 1.000000000000000000, 0.9659258262890683122, 1.000000000000000000, 0.9659258262890683122, 1.000000000000000000, 0.9659258262890683122, 1.000000000000000000, 0.9659258262890683122, 1.000000000000000000, 0.9659258262890683122, 1.000000000000000000, 0.9659258262890683122, 1.000000000000000000, 0.9659258262890683122, 1.000000000000000000, 0.9659258262890683122, 1.000000000000000000, 0.9659258262890683122, 1.000000000000000000, 0.9659258262890683122, 1.000000000000000000, 0.9659258262890683122, 1.000000000000000000, 0.9659258262890683122, 1.000000000000000000, 0.9659258262890683122, 1.000000000000000000, 0.9659258262890683122, 1.000000000000000000, 0.9659258262890683122, 1.000000000000000000, 0.9659258262890683122, 1.000000000000000000, 0.9659258262890683122, 1.000000000000000000, 0.9659258262890683122, 1.000000000000000000, 0.9659258262890683122, 1.000000000000000000, 0.9659258262890683122, 1.000000000000000000, 0.9659258262890683122, 1.000000000000000000, 0.9659258262890683122, 1.000000000000000000, 0.9659258262890683122, 1.000000000000000000, 0.9659258262890683122, 1.000000000000000000, 0.9659258262890683122, 1.000000000000000000, 0.9659258262890683122, 1.000000000000000000, 0.9659258262890683122, 1.000000000000000000, 0.9659258262890683122, 1.000000000000000000, 0.9659258262890683122, 1.000000000000000000, 0.9659258262890683122, 1.000000000000000000, 0.9659258262890683122, 1.000000000000000000, 0.9659258262890683122, 1.000000000000000000, 0.9659258262890683122, 1.000000000000000000, 0.9659258262890683122, 1.000000000000000000, 0.9659258262890683122, 1.000000000000000000, 0.9659258262890683122, 1.000000000000000000, 0.9659258262890683122, 1.000000000000000000, 0.9659258262890683122, 1.000000000000000000, 0.9659258262890683122, 1.000000000000000000, 0.9659258262890683122, 1.000000000000000000, 0.9659258262890683122, 1.000000000000000000, 0.9659258262890683122, 1.000000000000000000, 0.9659258262890683122, 1.000000000000000000, 0.9659258262890683122, 1.000000000000000000, 0.9659258262890683122, 1.000000000000000000, 0.9659258262890683122, 1.000000000000000000, 0.9659258262890683122, 1.000000000000000000, 0.9659258262890683122, 1.000000000000000000, 0.9659258262890683122, 1.000000000000000000, 0.9659258262890683122, 1.000000000000000000, 0.9659258262890683122, 1.000000000000000000, 0.9659258262890683122, 1.000000000000000000, 0.9659258262890683122, 1.000000000000000000, 0.9659258262890683122, 1.000000000000000000, 0.9659258262890683122, 1.000000000000000000, 0.9659258262890683122, 1.000000000000000000, 0.9659258262890683122, 1.000000000000000000, 0.9659258262890683122, 1.000000000000000000, 0.9659258262890683122, 1.000000000000000000, 0.9659258262890683122, 1.000000000000000000, 0.9659258262890683122, 1.000000000000000000, 0.9659258262890683122, 1.000000000000000000, 0.9659258262890683122, 1.000000000000000000, 0.9659258262890683122, 1.000000000000000000, 0.9659258262890683122, 1.000000000000000000, 0.9659258262890683122, 1.000000000000000000, 0.9659258262890683122, 1.000000000000000000, 0.9659258262890683122, 1.000000000000000000, 0.9659258262890683122, 1.000000000000000000, 0.9659258262890683122, 1.000000000000000000, 0.9659258262890683122, 1.000000000000000000, 0.9659258262890683122, 1.000000000000000000, 0.9659258262890683122, 1.000000000000000000, 0.9659258262890683122, 1.000000000000000000, 0.9659258262890683122, 1.000000000000000000, 0.9659258262890683122, 1.000000000000000000, 0.9659258262890683122, 1.000000000000000000, 0.9659258262890683122, 1.000000000000000000, 0.9659258262890683122, 1.000000000000000000, 0.9659258262890683122, 1.000000000000000000, 0.9659258262890683122, 1.000000000000000000, 0.9659258262890683122, 1.000000000000000000, 0.9659258262890683122, 1.000000000000000000, 0.9659258262890683122, 1.000000000000000000, 0.9659258262890683122, 1.000000000000000000, 0.9659258262890683122, 1.000000000000000000, 0.9659258262890683122, 1.000000000000000000, 0.9659258262890683122, 1.000000000000000000, 0.9659258262890683122, 1.000000000000000000, 0.9659258262890683122, 1.000000000000000000, 0.9659258262890683122, 1.000000000000000000, 0.9659258262890683122, 1.000000000000000000, 0.9659258262890683122, 1.000000000000000000, 0.9659258262890683122, 1.000000000000000000, 0.9659258262890683122, 1.000000000000000000, 0.9659258262890683122, 1.000000000000000000, 0.9659258262890683122, 1.000000000000000000, 0.9659258262890683122, 1.000000000000000000, 0.9659258262890683122, 1.000000000000000000, 0.9659258262890683122, 1.000000000000000000, 0.9659258262890683122, 1.000000000000000000, 0.9659258262890683122, 1.000000000000000000, 0.9659258262890683122, 1.000000000000000000, 0.9659258262890683122, 1.000000000000000000, 0.9659258262890683122, 1.000000000000000000, 0.9659258262890683122, 1.000000000000000000, 0.9659258262890683122, 1.000000000000000000, 0.9659258262890683122, 1.000000000000000000, 0.9659258262890683122, 1.000000000000000000, 0.9659258262890683122, 1.000000000000000000, 0.9659258262890683122, 1.000000000000000000, 0.9659258262890683122, 1.000000000000000000, 0.9659258262890683122, 1.000000000000000000, 0.9659258262890683122, 1.000000000000000000, 0.9659258262890683122, 1.000000000000000000, 0.9659258262890683122, 1.000000000000000000, 0.9659258262890683122, 1.000000000000000000, 0.9659258262890683122, 1.000000000000000000, 0.9659258262890683122, 1.000000000000000000, 0.9659258262890683122, 1.000000000000000000, 0.9659258262890683122, 1.000000000000000000, 0.9659258262890683122, 1.000000000000000000, 0.9659258262890683122, 1.000000000000000000, 0.9659258262890683122, 1.000000000000000000, 0.9659258262890683122, 1.000000000000000000, 0.9659258262890683122, 1.000000000000000000, 0.9659258262890683122, 1.000000000000000000, 0.9659258262890683122, 1.000000000000000000, 0.9659258262890683122, 1.000000000000000000, 0.9659258262890683122, 1.000000000000000000, 0.9659258262890683122, 1.000000000000000000, 0.9659258262890683122, 1.000000000000000000, 0.9659258262890683122, 1.000000000000000000, 0.9659258262890683122, 1.000000000000000000, 0.9659258262890683122, 1.000000000000000000, 0.9659258262890683122, 1.000000000000000000, 0.9659258262890683122, 1.000000000000000000, 0.9659258262890683122, 1.000000000000000000, 0.9659258262890683122, 1.000000000000000000, 0.9659258262890683122, 1.000000000000000000, 0.9659258262890683122, 1.000000000000000000, 0.9659258262890683122, 1.000000000000000000, 0.9659258262890683122, 1.000000000000000000, 0.9659258262890683122, 1.000000000000000000, 0.9659258262890683122, 1.000000000000000000, 0.9659258262890683122, 1.000000000000000000, 0.9659258262890683122, 1.000000000000000000, 0.9659258262890683122, 1.000000000000000000, 0.9659258262890683122, 1.000000000000000000, 0.9659258262890683122, 1.000000000000000000, 0.9659258262890683122, 1.000000000000000000, 0.9659258262890683122, 1.000000000000000000, 0.9659258262890683122, 1.000000000000000000, 0.9659258262890683122, 1.000000000000000000, 0.9659258262890683122, 1.000000000000000000, 0.9659258262890683122, 1.000000000000000000, 0.9659258262890683122, 1.000000000000000000, 0.9659258262890683122, 1.000000000000000000, 0.9659258262890683122, 1.000000000000000000, 0.9659258262890683122, 1.000000000000000000, 0.9659258262890683122, 1.000000000000000000, 0.9659258262890683122, 1.000000000000000000, 0.9659258262890683122, 1.000000000000000000, 0.9659258262890683122, 1.000000000000000000, 0.9659258262890683122, 1.000000000000000000, 0.9659258262890683122, 1.000000000000000000, 0.9659258262890683122, 1.000000000000000000, 0.9659258262890683122, 1.000000000000000000, 0.9659258262890683122, 1.000000000000000000) ) ) 
 REPRESENTATION_ITEM ( '' )  SURFACE ( )  );
#2594=CARTESIAN_POINT ( 'NONE',  ( -0.1312335958005241554, 0.2306618581243848609, 0.2411417322834645549 ) ) ;
#2595=CARTESIAN_POINT ( 'NONE',  ( -0.3805774278215216522, 0.05413385826771666132, 0.4176697321401328100 ) ) ;
#2597=CARTESIAN_POINT ( 'NONE',  ( -1.725721784776902190, -0.05778040916215522460, 0.4822834645669289988 ) ) ;
#2598=CARTESIAN_POINT ( 'NONE',  ( -0.4593175853018364174, -0.4281496062992127816, -0.4176697321401328100 ) ) ;
#2599=CARTESIAN_POINT ( 'NONE',  ( -0.3412073490813641308, 0.1283753931104746893, -0.1820866141732285504 ) ) ;
#2600=CARTESIAN_POINT ( 'NONE',  ( 1.286089238845145033, -0.6046776061558809534, -0.2411417322834644161 ) ) ;
#2602=CARTESIAN_POINT ( 'NONE',  ( -0.8202099737532801971, -0.6692913385826771977, 0.1292274648535927661 ) ) ;
#2604=CARTESIAN_POINT ( 'NONE',  ( 0.8923884514435701520, -0.6046776061558809534, -0.2411417322834644161 ) ) ;
#2607=EDGE_CURVE ( 'NONE', #26484, #9025, #73534, .T. ) ;
#2608=CARTESIAN_POINT ( 'NONE',  ( 0.01968503937007957949, -0.5400638737290845981, -0.3530559997133363437 ) ) ;
#2609=CARTESIAN_POINT ( 'NONE',  ( -1.187664041994749731, -0.2845877964562159024, 0.3641732283464567677 ) ) ;
#2610=CARTESIAN_POINT ( 'NONE',  ( 1.213910761154856299, 0.1771653543307087630, 0.09757992244046791164 ) ) ;
#2611=LINE ( 'NONE', #53519, #82778 ) ;
#2613=CARTESIAN_POINT ( 'NONE',  ( 1.227034120734908917, 0.1771653543307087075, -0.09757992244046823083 ) ) ;
#2615=CARTESIAN_POINT ( 'NONE',  ( 1.371391076115485719, -0.6692913385826773087, -0.1292274648535924053 ) ) ;
#2617=CARTESIAN_POINT ( 'NONE',  ( -0.3083989501312330295, -0.05778040916215522460, 0.4822834645669289988 ) ) ;
#2619=CARTESIAN_POINT ( 'NONE',  ( 1.351706036745407458, -0.3690944881889765550, -0.3153832671262227771 ) ) ;
#2620=CARTESIAN_POINT ( 'NONE',  ( -0.1902887139107604098, -0.6692913385826771977, 0.1292274648535927661 ) ) ;
#2622=CARTESIAN_POINT ( 'NONE',  ( 1.141732283464567788, -0.6692913385826771977, 8.415575281601705876E-17 ) ) ;
#2623=CARTESIAN_POINT ( 'NONE',  ( 0.2952755905511816326, -0.5400638737290844871, 0.3530559997133364547 ) ) ;
#2624=CARTESIAN_POINT ( 'NONE',  ( 0.6758530183727039509, -0.5511811023622046335, 0.09757992244046803654 ) ) ;
#2626=CARTESIAN_POINT ( 'NONE',  ( 0.4790026246719168435, -0.2845877964562161244, -0.3641732283464567121 ) ) ;
#2629=CARTESIAN_POINT ( 'NONE',  ( 0.9383202099737538715, -0.05778040916215560624, -0.4822834645669293319 ) ) ;
#2632=CARTESIAN_POINT ( 'NONE',  ( 0.1181102362204730916, 0.2952755905511811885, 0.000000000000000000 ) ) ;
#2633=CARTESIAN_POINT ( 'NONE',  ( -0.1443569553805768291, -0.004921259842519576551, 0.3153832671262227771 ) ) ;
#2634=CARTESIAN_POINT ( 'NONE',  ( 0.1706036745406830368, -0.4281496062992127816, -0.4176697321401328100 ) ) ;
#2635=CARTESIAN_POINT ( 'NONE',  ( 1.227034120734908917, 0.1771653543307087075, -0.09757992244046823083 ) ) ;
#2636=CARTESIAN_POINT ( 'NONE',  ( -1.509186351706035767, -0.004921259842519870586, -0.3153832671262229437 ) ) ;
#2637=CARTESIAN_POINT ( 'NONE',  ( -1.345144356955379816, -0.05778040916215560624, -0.4822834645669293319 ) ) ;
#2638=CARTESIAN_POINT ( 'NONE',  ( 0.6430446194225729606, -0.4281496062992127816, -0.4176697321401328100 ) ) ;
#2639=CARTESIAN_POINT ( 'NONE',  ( 1.417322834645670104, -0.1870078740157480879, -0.4822834645669291653 ) ) ;
#2641=CARTESIAN_POINT ( 'NONE',  ( 0.4002624671916016896, -0.3162353388693409650, -0.4822834645669289433 ) ) ;
#2643=CARTESIAN_POINT ( 'NONE',  ( 1.528871391076116026, 0.2952755905511811885, 0.1292274648535926551 ) ) ;
#2644=CARTESIAN_POINT ( 'NONE',  ( 1.141732283464567788, -0.6692913385826771977, 8.415575281601705876E-17 ) ) ;
#2645=CARTESIAN_POINT ( 'NONE',  ( -1.594488188976377563, -0.4536011799217367080, 0.2665933059059888421 ) ) ;
#2646=CARTESIAN_POINT ( 'NONE',  ( 1.220472440944882608, 0.1771653543307087630, 0.000000000000000000 ) ) ;
#2647=CARTESIAN_POINT ( 'NONE',  ( -1.594488188976377119, 0.07958543189024071263, -0.2665933059059888421 ) ) ;
#2648=CARTESIAN_POINT ( 'NONE',  ( -0.8202099737532799750, 0.1771653543307087075, -0.09757992244046823083 ) ) ;
#2649=CARTESIAN_POINT ( 'NONE',  ( 1.574803149606299746, -0.1870078740157479769, 0.4822834645669291653 ) ) ;
#2650=CARTESIAN_POINT ( 'NONE',  ( 0.4199475065616803948, -0.5023911411419708095, -0.1820866141732282451 ) ) ;
#2651=CARTESIAN_POINT ( 'NONE',  ( 0.1574803149606306130, -0.1870078740157480879, -0.4822834645669291653 ) ) ;
#2652=CARTESIAN_POINT ( 'NONE',  ( 0.8595800524934390507, -0.05778040916215560624, -0.4822834645669293319 ) ) ;
#2653=CARTESIAN_POINT ( 'NONE',  ( -0.3674540682414689785, 0.2306618581243848609, 0.2411417322834645549 ) ) ;
#2654=CARTESIAN_POINT ( 'NONE',  ( 0.3149606299212603933, -0.1870078740157479769, 0.3641732283464567677 ) ) ;
#2655=CARTESIAN_POINT ( 'NONE',  ( 1.023622047244095112, -0.1870078740157480879, -0.4822834645669291653 ) ) ;
#2656=DIRECTION ( 'NONE',  ( 1.000000000000000000, 3.096699300667737957E-16, 0.000000000000000000 ) ) ;
#2657=CARTESIAN_POINT ( 'NONE',  ( -0.8333333333333323711, -0.6692913385826773087, -0.1292274648535924053 ) ) ;
#2658=CARTESIAN_POINT ( 'NONE',  ( -1.568241469816272105, -0.08942795157527998196, 0.3641732283464567121 ) ) ;
#2661=CARTESIAN_POINT ( 'NONE',  ( -0.8070866141732276899, 0.1660481256975883668, -0.3530559997133364547 ) ) ;
#2662=CARTESIAN_POINT ( 'NONE',  ( -0.2099737532808391705, -0.6046776061558809534, -0.2411417322834644161 ) ) ;
#2666=CARTESIAN_POINT ( 'NONE',  ( 0.8530183727034128527, -0.3690944881889763329, 0.3153832671262228327 ) ) ;
#2668=CARTESIAN_POINT ( 'NONE',  ( 1.167979002624672580, 0.05413385826771626580, -0.4176697321401330321 ) ) ;
#2669=CARTESIAN_POINT ( 'NONE',  ( -0.2486400153428821869, 2.660739321503277841E-15, -0.3464511005275191513 ) ) ;
#2670=CARTESIAN_POINT ( 'NONE',  ( -1.515748031496062076, 0.07958543189024071263, -0.2665933059059888421 ) ) ;
#2671=CARTESIAN_POINT ( 'NONE',  ( 1.528871391076116026, 0.2952755905511811885, 0.1292274648535926551 ) ) ;
#2672=CARTESIAN_POINT ( 'NONE',  ( -1.377952755905511140, 0.2952755905511811885, 0.000000000000000000 ) ) ;
#2674=CARTESIAN_POINT ( 'NONE',  ( 0.03280839895013198948, -0.6692913385826773087, -0.1292274648535924053 ) ) ;
#2675=CARTESIAN_POINT ( 'NONE',  ( -0.3871391076115479057, -0.2845877964562161244, -0.3641732283464567121 ) ) ;
#2676=CARTESIAN_POINT ( 'NONE',  ( 1.062992125984252745, -0.6692913385826771977, 8.415575281601705876E-17 ) ) ;
#2677=CARTESIAN_POINT ( 'NONE',  ( -0.1049868766404193215, 0.2306618581243847221, -0.2411417322834647770 ) ) ;
#2681=CARTESIAN_POINT ( 'NONE',  ( 1.003937007874016407, -0.5400638737290844871, 0.3530559997133364547 ) ) ;
#2682=CARTESIAN_POINT ( 'NONE',  ( 0.2690288713910767848, -0.6692913385826773087, -0.1292274648535924053 ) ) ;
#2683=CARTESIAN_POINT ( 'NONE',  ( -1.240157480314959759, -0.5400638737290845981, -0.3530559997133363437 ) ) ;
#2684=CARTESIAN_POINT ( 'NONE',  ( 1.456692913385827515, 0.2952755905511811885, 0.000000000000000000 ) ) ;
#2685=CARTESIAN_POINT ( 'NONE',  ( 0.7086614173228353852, -0.1870078740157479769, 0.4822834645669291653 ) ) ;
#2687=CARTESIAN_POINT ( 'NONE',  ( -0.4002624671916004129, -0.05778040916215560624, -0.4822834645669293319 ) ) ;
#2688=CARTESIAN_POINT ( 'NONE',  ( 0.6889763779527566800, -0.5400638737290844871, 0.3530559997133364547 ) ) ;
#2689=CARTESIAN_POINT ( 'NONE',  ( -0.09842519685039295696, -0.5400638737290844871, 0.3530559997133364547 ) ) ;
#2690=CARTESIAN_POINT ( 'NONE',  ( 0.8595800524934390507, -0.2845877964562159024, 0.3641732283464567677 ) ) ;
#2691=CARTESIAN_POINT ( 'NONE',  ( -1.141732283464566011, -0.6692913385826771977, 8.415575281601705876E-17 ) ) ;
#2692=CARTESIAN_POINT ( 'NONE',  ( -1.706036745406823485, 0.2306618581243848609, 0.2411417322834645549 ) ) ;
#2693=CARTESIAN_POINT ( 'NONE',  ( 0.5839895013123367340, -0.6692913385826773087, -0.1292274648535924053 ) ) ;
#2697=ORIENTED_EDGE ( 'NONE', *, *, #5292, .T. ) ;
#2698=CARTESIAN_POINT ( 'NONE',  ( 1.259842519685040019, -0.1870078740157480879, -0.4822834645669291653 ) ) ;
#2699=CARTESIAN_POINT ( 'NONE',  ( 0.4002624671916016896, -0.2845877964562161244, -0.3641732283464567121 ) ) ;
#2700=CARTESIAN_POINT ( 'NONE',  ( 0.5774278215223104249, 0.2306618581243848609, 0.2411417322834645549 ) ) ;
#2705=CARTESIAN_POINT ( 'NONE',  ( -0.9645669291338575535, 0.1660481256975883668, -0.3530559997133364547 ) ) ;
#2706=CARTESIAN_POINT ( 'NONE',  ( -0.6955380577427815458, -0.4281496062992127816, -0.4176697321401328100 ) ) ;
#2707=CARTESIAN_POINT ( 'NONE',  ( 1.299212598425197429, 0.2952755905511811885, 0.000000000000000000 ) ) ;
#2709=CARTESIAN_POINT ( 'NONE',  ( -1.509186351706035767, 0.05413385826771626580, -0.4176697321401330321 ) ) ;
#2710=CARTESIAN_POINT ( 'NONE',  ( -1.170403185795210632, -4.983732387537991731E-15, 0.4118484887281982920 ) ) ;
#2711=CARTESIAN_POINT ( 'NONE',  ( 1.587926509186352586, -0.3690944881889765550, -0.3153832671262227771 ) ) ;
#2713=CARTESIAN_POINT ( 'NONE',  ( -1.259842519685038686, -0.1870078740157480601, -0.3641732283464567677 ) ) ;
#2714=( BOUNDED_CURVE ( )  B_SPLINE_CURVE ( 2, ( #22978, #74756, #69258, #10368, #55778, #80666, #29705, #49475, #23389, #68435, #62521, #17513, #56198 ),
 .UNSPECIFIED., .F., .F. ) 
 B_SPLINE_CURVE_WITH_KNOTS ( ( 3, 2, 2, 2, 2, 2, 3 ),
 ( 0.4581241751160508580, 0.4583333333333333703, 0.4621212121212121549, 0.4659090909090909394, 0.4696969696969697239, 0.4734848484848485084, 0.4736940067021309653 ),
 .UNSPECIFIED. ) 
 CURVE ( )  GEOMETRIC_REPRESENTATION_ITEM ( )  RATIONAL_B_SPLINE_CURVE ( ( 0.9964447847208419695, 0.9981185001348091834, 1.000000000000000000, 0.9659258262890683122, 1.000000000000000000, 0.9659258262890683122, 1.000000000000000000, 0.9659258262890683122, 1.000000000000000000, 0.9659258262890683122, 1.000000000000000000, 0.9981185001348097385, 0.9964447847208430797 ) ) 
 REPRESENTATION_ITEM ( '' )  );
#2716=CARTESIAN_POINT ( 'NONE',  ( 0.2821522309711292364, 0.2952755905511810774, -0.1292274648535930714 ) ) ;
#2717=CARTESIAN_POINT ( 'NONE',  ( 1.482939632545932307, -0.4281496062992124485, 0.4176697321401328655 ) ) ;
#2719=CARTESIAN_POINT ( 'NONE',  ( -0.9317585301837263412, -0.004921259842519576551, 0.3153832671262227771 ) ) ;
#2720=CARTESIAN_POINT ( 'NONE',  ( 0.7677165354330716118, 0.1660481256975883668, -0.3530559997133364547 ) ) ;
#2721=CARTESIAN_POINT ( 'NONE',  ( 1.463254593175853824, 0.1771653543307087075, -0.09757992244046823083 ) ) ;
#2723=CARTESIAN_POINT ( 'NONE',  ( -0.8530183727034112984, -0.3690944881889765550, -0.3153832671262227771 ) ) ;
#2724=CARTESIAN_POINT ( 'NONE',  ( 1.187664041994751285, -0.05778040916215522460, 0.4822834645669289988 ) ) ;
#2726=CARTESIAN_POINT ( 'NONE',  ( 0.3412073490813655186, 0.2306618581243848609, 0.2411417322834645549 ) ) ;
#2727=CARTESIAN_POINT ( 'NONE',  ( -0.7808398950131222316, -0.2845877964562161244, -0.3641732283464567121 ) ) ;
#2728=CARTESIAN_POINT ( 'NONE',  ( -0.4593175853018366950, -0.004921259842519576551, 0.3153832671262227771 ) ) ;
#2730=CARTESIAN_POINT ( 'NONE',  ( -0.2296587926509179312, -0.3162353388693409650, -0.4822834645669289433 ) ) ;
#2731=CARTESIAN_POINT ( 'NONE',  ( 1.686351706036745890, 0.2952755905511811885, 0.1292274648535926551 ) ) ;
#2733=CARTESIAN_POINT ( 'NONE',  ( 0.5249343832021003964, 0.2306618581243847221, -0.2411417322834647770 ) ) ;
#2736=DIRECTION ( 'NONE',  ( -3.096699300667737957E-16, 1.000000000000000000, -0.000000000000000000 ) ) ;
#2738=CARTESIAN_POINT ( 'NONE',  ( -0.9908136482939626788, -0.6692913385826773087, -0.1292274648535924053 ) ) ;
#2739=CARTESIAN_POINT ( 'NONE',  ( -0.3937007874015740483, -0.1870078740157480601, -0.3641732283464567677 ) ) ;
#2740=CARTESIAN_POINT ( 'NONE',  ( -1.233595800524933894, -0.6046776061558809534, -0.2411417322834644161 ) ) ;
#2741=CARTESIAN_POINT ( 'NONE',  ( 0.2296587926509192634, -0.3162353388693405765, 0.4822834645669290543 ) ) ;
#2742=CARTESIAN_POINT ( 'NONE',  ( 0.3149606299212606708, -0.1870078740157480601, -0.3641732283464567677 ) ) ;
#2743=CARTESIAN_POINT ( 'NONE',  ( -0.6167979002624665030, -0.004921259842519576551, 0.3153832671262227771 ) ) ;
#2744=CARTESIAN_POINT ( 'NONE',  ( -1.141732283464566011, -0.6692913385826771977, 8.415575281601705876E-17 ) ) ;
#2745=CARTESIAN_POINT ( 'NONE',  ( 1.614173228346457378, 0.1771653543307087630, 0.000000000000000000 ) ) ;
#2746=CARTESIAN_POINT ( 'NONE',  ( 1.200787401574803681, 0.1660481256975885056, 0.3530559997133364547 ) ) ;
#2748=CARTESIAN_POINT ( 'NONE',  ( 0.7808398950131241190, -0.08942795157528024563, -0.3641732283464568787 ) ) ;
#2749=CARTESIAN_POINT ( 'NONE',  ( 0.5511811023622055217, -0.1870078740157479769, 0.4822834645669291653 ) ) ;
#2751=CARTESIAN_POINT ( 'NONE',  ( 1.496062992125984703, -0.1870078740157480601, -0.3641732283464567677 ) ) ;
#2752=ORIENTED_EDGE ( 'NONE', *, *, #26244, .T. ) ;
#2754=EDGE_CURVE ( 'NONE', #50981, #74234, #27338, .T. ) ;
#2755=CARTESIAN_POINT ( 'NONE',  ( -1.128608923884513837, 0.1283753931104746893, -0.1820866141732285504 ) ) ;
#2756=CARTESIAN_POINT ( 'NONE',  ( -0.4921259842519677963, 0.1660481256975883668, -0.3530559997133364547 ) ) ;
#2757=CARTESIAN_POINT ( 'NONE',  ( 0.2296587926509192634, -0.05778040916215560624, -0.4822834645669293319 ) ) ;
#2758=CARTESIAN_POINT ( 'NONE',  ( -1.679790026246718693, 0.1283753931104746893, -0.1820866141732285504 ) ) ;
#2760=CARTESIAN_POINT ( 'NONE',  ( -1.318897637795274802, -0.5400638737290845981, -0.3530559997133363437 ) ) ;
#2761=CARTESIAN_POINT ( 'NONE',  ( 0.5774278215223104249, 0.2306618581243848609, 0.2411417322834645549 ) ) ;
#2762=CARTESIAN_POINT ( 'NONE',  ( -0.1115485564304453947, -0.6692913385826771977, 0.1292274648535927661 ) ) ;
#2763=CARTESIAN_POINT ( 'NONE',  ( 1.266404199475066328, -0.05778040916215522460, 0.4822834645669289988 ) ) ;
#2764=CARTESIAN_POINT ( 'NONE',  ( 1.627296587926509996, -0.6046776061558807314, 0.2411417322834647770 ) ) ;
#2770=CARTESIAN_POINT ( 'NONE',  ( -0.1246719160104980823, 0.1771653543307087630, 0.09757992244046791164 ) ) ;
#2771=CARTESIAN_POINT ( 'NONE',  ( -0.1377952755905504645, 0.1660481256975885056, 0.3530559997133364547 ) ) ;
#2772=CARTESIAN_POINT ( 'NONE',  ( 0.7283464566929140904, -0.5400638737290845981, -0.3530559997133363437 ) ) ;
#2774=CARTESIAN_POINT ( 'NONE',  ( -0.2362204724409440182, -0.1870078740157479769, 0.3641732283464567677 ) ) ;
#2775=CARTESIAN_POINT ( 'NONE',  ( -1.089238845144356427, -0.4281496062992127816, -0.4176697321401328100 ) ) ;
#2776=CARTESIAN_POINT ( 'NONE',  ( -1.601049868766403650, 0.2306618581243847221, -0.2411417322834647770 ) ) ;
#2781=CARTESIAN_POINT ( 'NONE',  ( 0.9645669291338588858, 0.1660481256975885056, 0.3530559997133364547 ) ) ;
#2782=CARTESIAN_POINT ( 'NONE',  ( -1.587926509186350810, -0.4281496062992124485, 0.4176697321401328655 ) ) ;
#2783=CARTESIAN_POINT ( 'NONE',  ( -1.391076115485563314, -0.5023911411419708095, -0.1820866141732282451 ) ) ;
#2784=CARTESIAN_POINT ( 'NONE',  ( -1.089238845144356427, -0.4281496062992127816, -0.4176697321401328100 ) ) ;
#2786=CARTESIAN_POINT ( 'NONE',  ( -1.614173228346456712, 1.267785121476993737, -0.1372047244094478091 ) ) ;
#2787=CARTESIAN_POINT ( 'NONE',  ( 1.364829396325460076, 0.2306618581243848609, 0.2411417322834645549 ) ) ;
#2789=CARTESIAN_POINT ( 'NONE',  ( -0.1115485564304456306, 0.2952755905511810774, -0.1292274648535930714 ) ) ;
#2790=CARTESIAN_POINT ( 'NONE',  ( -0.1771653543307080136, -0.5400638737290844871, 0.3530559997133364547 ) ) ;
#2792=CARTESIAN_POINT ( 'NONE',  ( -1.200787401574802349, -0.5400638737290844871, 0.3530559997133364547 ) ) ;
#2794=CARTESIAN_POINT ( 'NONE',  ( 0.1443569553805781891, -0.4281496062992124485, 0.4176697321401328655 ) ) ;
#2796=CARTESIAN_POINT ( 'NONE',  ( -1.056430446194224881, -0.5511811023622046335, 0.09757992244046803654 ) ) ;
#2799=ORIENTED_EDGE ( 'NONE', *, *, #25562, .T. ) ;
#2801=CARTESIAN_POINT ( 'NONE',  ( -1.456692913385826182, -0.6692913385826771977, 8.415575281601705876E-17 ) ) ;
#2803=CARTESIAN_POINT ( 'NONE',  ( -1.456692913385826182, -0.6692913385826771977, 8.415575281601705876E-17 ) ) ;
#2806=DIRECTION ( 'NONE',  ( 0.000000000000000000, 0.000000000000000000, 1.000000000000000000 ) ) ;
#2808=CARTESIAN_POINT ( 'NONE',  ( -0.3280839895013117347, -0.004921259842519870586, -0.3153832671262229437 ) ) ;
#2809=CARTESIAN_POINT ( 'NONE',  ( -0.8070866141732276899, -0.4536011799217367080, 0.2665933059059888421 ) ) ;
#2810=CARTESIAN_POINT ( 'NONE',  ( -1.207349081364828436, -0.6046776061558807314, 0.2411417322834647770 ) ) ;
#2811=CARTESIAN_POINT ( 'NONE',  ( 0.9973753280839902091, 0.2306618581243847221, -0.2411417322834647770 ) ) ;
#2812=CARTESIAN_POINT ( 'NONE',  ( -1.017060367454067249, -0.05778040916215522460, 0.4822834645669289988 ) ) ;
#2814=ORIENTED_EDGE ( 'NONE', *, *, #55092, .T. ) ;
#2815=CARTESIAN_POINT ( 'NONE',  ( -1.430446194225720724, 0.05413385826771626580, -0.4176697321401330321 ) ) ;
#2822=CARTESIAN_POINT ( 'NONE',  ( -0.7742782152230962556, -0.4281496062992127816, -0.4176697321401328100 ) ) ;
#2823=CARTESIAN_POINT ( 'NONE',  ( 1.509186351706037543, 0.05413385826771666132, 0.4176697321401328100 ) ) ;
#2825=LINE ( 'NONE', #66811, #26107 ) ;
#2827=CARTESIAN_POINT ( 'NONE',  ( -1.391076115485563758, 0.2306618581243848609, 0.2411417322834645549 ) ) ;
#2828=CARTESIAN_POINT ( 'NONE',  ( -0.6036745406824141069, 0.2306618581243848609, 0.2411417322834645549 ) ) ;
#2830=CARTESIAN_POINT ( 'NONE',  ( 0.3543307086614179147, 0.1771653543307087630, 0.000000000000000000 ) ) ;
#2832=CARTESIAN_POINT ( 'NONE',  ( 0.3477690288713918276, -0.5511811023622048555, -0.09757992244046775898 ) ) ;
#2833=CARTESIAN_POINT ( 'NONE',  ( 0.8202099737532813073, 0.1771653543307087630, 0.09757992244046791164 ) ) ;
#2834=CARTESIAN_POINT ( 'NONE',  ( 0.9448818897637802916, -0.1870078740157479769, 0.4822834645669291653 ) ) ;
#2835=CARTESIAN_POINT ( 'NONE',  ( -0.4921259842519677963, 0.07958543189024071263, -0.2665933059059888421 ) ) ;
#2837=CARTESIAN_POINT ( 'NONE',  ( -1.076115485564303809, -0.6046776061558809534, -0.2411417322834644161 ) ) ;
#2838=B_SPLINE_CURVE_WITH_KNOTS ( 'NONE', 3,
 ( #62091, #69649, #75151, #62504 ),
 .UNSPECIFIED., .F., .F.,
 ( 4, 4 ),
 ( 3.593986969187450165E-07, 0.001287825409103201223 ),
 .UNSPECIFIED. ) ;
#2839=CARTESIAN_POINT ( 'NONE',  ( -1.279527559055116948, 0.07958543189024071263, -0.2665933059059888421 ) ) ;
#2841=CARTESIAN_POINT ( 'NONE',  ( -1.003937007874014853, 0.07958543189024085140, 0.2665933059059887866 ) ) ;
#2842=CARTESIAN_POINT ( 'NONE',  ( -0.2755905511811015396, -0.6692913385826771977, 8.415575281601705876E-17 ) ) ;
#2843=CARTESIAN_POINT ( 'NONE',  ( 1.620734908136483465, -0.5511811023622046335, 0.09757992244046803654 ) ) ;
#2844=CARTESIAN_POINT ( 'NONE',  ( 0.5643044619422579178, -0.3690944881889765550, -0.3153832671262227771 ) ) ;
#2845=CARTESIAN_POINT ( 'NONE',  ( -0.1181102362204717315, 0.1771653543307087630, 0.000000000000000000 ) ) ;
#2846=CARTESIAN_POINT ( 'NONE',  ( -0.8923884514435688198, -0.6046776061558807314, 0.2411417322834647770 ) ) ;
#2847=FACE_OUTER_BOUND ( 'NONE', #21596, .T. ) ;
#2848=FACE_OUTER_BOUND ( 'NONE', #8362, .T. ) ;
#2849=CARTESIAN_POINT ( 'NONE',  ( -0.03280839895013062252, 0.2952755905511810774, -0.1292274648535930714 ) ) ;
#2850=AXIS2_PLACEMENT_3D ( 'NONE', #63849, #17605, #18426 ) ;
#2853=CARTESIAN_POINT ( 'NONE',  ( 1.391076115485564868, -0.6046776061558807314, 0.2411417322834647770 ) ) ;
#2854=CARTESIAN_POINT ( 'NONE',  ( -0.1246719160104980823, 0.1771653543307087630, 0.09757992244046791164 ) ) ;
#2855=CARTESIAN_POINT ( 'NONE',  ( -0.1181102362204717315, 0.2952755905511811885, 0.000000000000000000 ) ) ;
#2856=CARTESIAN_POINT ( 'NONE',  ( -1.620734908136482577, 0.2952755905511811885, 0.1292274648535926551 ) ) ;
#2857=CARTESIAN_POINT ( 'NONE',  ( -1.607611548556429737, 0.1771653543307087075, -0.09757992244046823083 ) ) ;
#2858=CARTESIAN_POINT ( 'NONE',  ( 1.141732283464567788, -0.6692913385826771977, 8.415575281601705876E-17 ) ) ;
#2859=CARTESIAN_POINT ( 'NONE',  ( -0.7020997375328076329, -0.2845877964562161244, -0.3641732283464567121 ) ) ;
#2860=CARTESIAN_POINT ( 'NONE',  ( 0.4531182788721078158, 1.535433070866141447, 0.5309055118110234117 ) ) ;
#2865=CARTESIAN_POINT ( 'NONE',  ( 1.345144356955381593, -0.2845877964562161244, -0.3641732283464567121 ) ) ;
#2866=CARTESIAN_POINT ( 'NONE',  ( -1.601049868766403650, -0.6046776061558807314, 0.2411417322834647770 ) ) ;
#2867=CARTESIAN_POINT ( 'NONE',  ( 0.9776902887139113929, 0.2952755905511811885, 0.1292274648535926551 ) ) ;
#2869=CARTESIAN_POINT ( 'NONE',  ( 1.417322834645670104, -0.1870078740157480601, -0.3641732283464567677 ) ) ;
#2870=CARTESIAN_POINT ( 'NONE',  ( 0.06561679790026316017, -0.4281496062992124485, 0.4176697321401328655 ) ) ;
#2871=CARTESIAN_POINT ( 'NONE',  ( -0.3412073490813641308, 0.2306618581243847221, -0.2411417322834647770 ) ) ;
#2872=CARTESIAN_POINT ( 'NONE',  ( 1.476377952755906442, -0.5400638737290844871, 0.3530559997133364547 ) ) ;
#2875=CARTESIAN_POINT ( 'NONE',  ( 0.5577427821522314977, -0.2845877964562161244, -0.3641732283464567121 ) ) ;
#2877=ORIENTED_EDGE ( 'NONE', *, *, #3202, .F. ) ;
#2879=ORIENTED_EDGE ( 'NONE', *, *, #24425, .T. ) ;
#2880=CARTESIAN_POINT ( 'NONE',  ( -0.2427821522309703550, -0.05778040916215560624, -0.4822834645669293319 ) ) ;
#2881=CARTESIAN_POINT ( 'NONE',  ( 0.7020997375328090762, -0.05778040916215560624, -0.4822834645669293319 ) ) ;
#2882=CARTESIAN_POINT ( 'NONE',  ( 0.1574803149606306130, -0.1870078740157480879, -0.4822834645669291653 ) ) ;
#2883=CARTESIAN_POINT ( 'NONE',  ( -0.5052493438320203589, 0.1771653543307087075, -0.09757992244046823083 ) ) ;
#2884=CARTESIAN_POINT ( 'NONE',  ( 0.9711286089238851948, -0.6046776061558809534, -0.2411417322834644161 ) ) ;
#2886=CARTESIAN_POINT ( 'NONE',  ( -0.7086614173228339419, -0.1870078740157479769, 0.4822834645669291653 ) ) ;
#2887=CARTESIAN_POINT ( 'NONE',  ( -0.5774278215223089816, 0.2306618581243847221, -0.2411417322834647770 ) ) ;
#2888=CARTESIAN_POINT ( 'NONE',  ( -0.9645669291338575535, -0.5400638737290844871, 0.3530559997133364547 ) ) ;
#2889=CARTESIAN_POINT ( 'NONE',  ( 1.358267716535433323, -0.5400638737290845981, -0.3530559997133363437 ) ) ;
#2890=CARTESIAN_POINT ( 'NONE',  ( 0.8858267716535438430, -0.5400638737290845981, -0.3530559997133363437 ) ) ;
#2891=CARTESIAN_POINT ( 'NONE',  ( 0.8267716535433078384, -0.6692913385826771977, 8.415575281601705876E-17 ) ) ;
#2893=CARTESIAN_POINT ( 'NONE',  ( 0.07217847769028949700, -0.2845877964562159024, 0.3641732283464567677 ) ) ;
#2897=CARTESIAN_POINT ( 'NONE',  ( -0.9973753280839886548, -0.5023911411419708095, -0.1820866141732282451 ) ) ;
#2898=CARTESIAN_POINT ( 'NONE',  ( -0.4527559055118102749, -0.5400638737290845981, -0.3530559997133363437 ) ) ;
#2900=CARTESIAN_POINT ( 'NONE',  ( -0.3346456692913377662, -0.5400638737290844871, 0.3530559997133364547 ) ) ;
#2901=CARTESIAN_POINT ( 'NONE',  ( -0.4002624671916004129, -0.05778040916215560624, -0.4822834645669293319 ) ) ;
#2902=CARTESIAN_POINT ( 'NONE',  ( -1.476377952755905110, 0.1660481256975885056, 0.3530559997133364547 ) ) ;
#2903=CARTESIAN_POINT ( 'NONE',  ( -1.384514435695537005, 0.2952755905511811885, 0.1292274648535926551 ) ) ;
#2904=CARTESIAN_POINT ( 'NONE',  ( 1.056430446194226658, 0.1771653543307087630, 0.09757992244046791164 ) ) ;
#2907=CARTESIAN_POINT ( 'NONE',  ( 0.4724409448818904789, -0.1870078740157479769, 0.3641732283464567677 ) ) ;
#2908=CARTESIAN_POINT ( 'NONE',  ( -0.1049868766404193215, -0.6046776061558807314, 0.2411417322834647770 ) ) ;
#2909=CARTESIAN_POINT ( 'NONE',  ( 0.3674540682414705883, -0.6046776061558807314, 0.2411417322834647770 ) ) ;
#2913=CARTESIAN_POINT ( 'NONE',  ( -0.5774278215223089816, 0.1539470093639521697, -0.1968503937007875793 ) ) ;
#2914=VERTEX_POINT ( 'NONE', #9356 ) ;
#2917=CARTESIAN_POINT ( 'NONE',  ( -0.5971128608923877978, 0.1771653543307087630, 0.09757992244046791164 ) ) ;
#2918=CARTESIAN_POINT ( 'NONE',  ( -0.5118110236220466680, -0.6692913385826771977, 8.415575281601705876E-17 ) ) ;
#2921=CARTESIAN_POINT ( 'NONE',  ( 1.601049868766404982, -0.6046776061558809534, -0.2411417322834644161 ) ) ;
#2922=CARTESIAN_POINT ( 'NONE',  ( 0.6955380577427828781, 0.05413385826771626580, -0.4176697321401330321 ) ) ;
#2923=CARTESIAN_POINT ( 'NONE',  ( 1.003937007874016407, -0.5400638737290844871, 0.3530559997133364547 ) ) ;
#2924=CARTESIAN_POINT ( 'NONE',  ( -0.5577427821522301654, -0.2845877964562159024, 0.3641732283464567677 ) ) ;
#2925=CARTESIAN_POINT ( 'NONE',  ( 0.2099737532808405305, 0.2306618581243847221, -0.2411417322834647770 ) ) ;
#2927=CARTESIAN_POINT ( 'NONE',  ( -0.07874015748031421014, -0.1870078740157479769, 0.3641732283464567677 ) ) ;
#2928=CARTESIAN_POINT ( 'NONE',  ( -0.6299212598425188991, -0.1870078740157479769, 0.4822834645669291653 ) ) ;
#2930=CARTESIAN_POINT ( 'NONE',  ( 1.528871391076116026, -0.5511811023622048555, -0.09757992244046775898 ) ) ;
#2931=CARTESIAN_POINT ( 'NONE',  ( 0.2427821522309716595, -0.2845877964562161244, -0.3641732283464567121 ) ) ;
#2933=CARTESIAN_POINT ( 'NONE',  ( -1.036745406824146176, 0.05413385826771626580, -0.4176697321401330321 ) ) ;
#2934=CARTESIAN_POINT ( 'NONE',  ( -0.5905511811023613777, -0.5511811023622047445, 6.969142054262312111E-17 ) ) ;
#2936=CARTESIAN_POINT ( 'NONE',  ( -1.036745406824146176, 0.05413385826771626580, -0.4176697321401330321 ) ) ;
#2937=CARTESIAN_POINT ( 'NONE',  ( 0.09186351706036827158, 0.05413385826771666132, 0.4176697321401328100 ) ) ;
#2941=CARTESIAN_POINT ( 'NONE',  ( 0.2559055118110243332, 0.07958543189024085140, 0.2665933059059887866 ) ) ;
#2942=CARTESIAN_POINT ( 'NONE',  ( 0.8989501312335963501, -0.6692913385826773087, -0.1292274648535924053 ) ) ;
#2943=CARTESIAN_POINT ( 'NONE',  ( -1.246719160104986512, -0.004921259842519576551, 0.3153832671262227771 ) ) ;
#2944=CARTESIAN_POINT ( 'NONE',  ( 1.056430446194226658, 0.2952755905511811885, 0.1292274648535926551 ) ) ;
#2945=CARTESIAN_POINT ( 'NONE',  ( -1.377952755905511140, 0.1771653543307087630, 0.000000000000000000 ) ) ;
#2946=CARTESIAN_POINT ( 'NONE',  ( -0.6102362204724400829, 0.1660481256975885056, 0.3530559997133364547 ) ) ;
#2947=CARTESIAN_POINT ( 'NONE',  ( 0.1443569553805781891, -0.004921259842519870586, -0.3153832671262229437 ) ) ;
#2949=CARTESIAN_POINT ( 'NONE',  ( 0.5118110236220478892, 0.1771653543307087630, 0.000000000000000000 ) ) ;
#2950=CARTESIAN_POINT ( 'NONE',  ( 0.09842519685039434474, 0.1660481256975885056, 0.3530559997133364547 ) ) ;
#2952=CARTESIAN_POINT ( 'NONE',  ( -1.207349081364828880, 0.2306618581243847221, -0.2411417322834647770 ) ) ;
#2954=CARTESIAN_POINT ( 'NONE',  ( 1.095800524934383846, -0.2845877964562159024, 0.3641732283464567677 ) ) ;
#2955=CARTESIAN_POINT ( 'NONE',  ( -0.04593175853018302557, 0.2952755905511811885, 0.1292274648535926551 ) ) ;
#2956=CARTESIAN_POINT ( 'NONE',  ( -0.4265091863517051496, -0.6692913385826771977, 0.1292274648535927661 ) ) ;
#2957=CARTESIAN_POINT ( 'NONE',  ( -0.2690288713910754526, -0.5511811023622046335, 0.09757992244046803654 ) ) ;
#2958=CARTESIAN_POINT ( 'NONE',  ( 1.200787401574803903, 0.1660481256975885056, 0.3530559997133364547 ) ) ;
#2959=CARTESIAN_POINT ( 'NONE',  ( -0.4527559055118102749, -0.4536011799217368745, -0.2665933059059886201 ) ) ;
#2960=CARTESIAN_POINT ( 'NONE',  ( 0.2624671916010504757, 0.2306618581243848609, 0.2411417322834645549 ) ) ;
#2961=CARTESIAN_POINT ( 'NONE',  ( -0.9186351706036736120, 0.1283753931104748280, 0.1820866141732283561 ) ) ;
#2963=CARTESIAN_POINT ( 'NONE',  ( -1.200787401574802349, -0.5400638737290844871, 0.3530559997133364547 ) ) ;
#2965=ORIENTED_EDGE ( 'NONE', *, *, #41074, .F. ) ;
#2966=CARTESIAN_POINT ( 'NONE',  ( -1.069553805774277722, 0.1771653543307087630, 0.09757992244046791164 ) ) ;
#2968=CARTESIAN_POINT ( 'NONE',  ( -0.2755905511811018171, 0.2952755905511811885, 0.000000000000000000 ) ) ;
#2970=CARTESIAN_POINT ( 'NONE',  ( -1.345144356955379816, -0.3162353388693405765, 0.4822834645669290543 ) ) ;
#2971=DIRECTION ( 'NONE',  ( -1.000000000000000000, -2.312964634635741971E-16, 0.000000000000000000 ) ) ;
#2972=CARTESIAN_POINT ( 'NONE',  ( 1.528871391076116026, 0.2952755905511811885, 0.1292274648535926551 ) ) ;
#2973=CARTESIAN_POINT ( 'NONE',  ( 0.6561679790026253567, -0.6046776061558809534, -0.2411417322834644161 ) ) ;
#2976=CARTESIAN_POINT ( 'NONE',  ( -1.719160104986876103, 0.05413385826771666132, 0.4176697321401328100 ) ) ;
#2977=ADVANCED_FACE ( 'NONE', ( #73336 ), #66183, .F. ) ;
#2980=CARTESIAN_POINT ( 'NONE',  ( -0.6233595800524928121, -0.2845877964562161244, -0.3641732283464567121 ) ) ;
#2983=CARTESIAN_POINT ( 'NONE',  ( 0.6430446194225728496, 0.05413385826771666132, 0.4176697321401328100 ) ) ;
#2984=CARTESIAN_POINT ( 'NONE',  ( -0.3937007874015740483, -0.1870078740157480879, -0.4822834645669291653 ) ) ;
#2985=CARTESIAN_POINT ( 'NONE',  ( -0.7217847769028863381, -0.4281496062992124485, 0.4176697321401328655 ) ) ;
#2986=CARTESIAN_POINT ( 'NONE',  ( 1.299212598425197429, -0.6692913385826771977, 8.415575281601705876E-17 ) ) ;
#2987=CARTESIAN_POINT ( 'NONE',  ( -1.502624671916009680, -0.2845877964562159024, 0.3641732283464567677 ) ) ;
#2989=CARTESIAN_POINT ( 'NONE',  ( 0.5380577427821529035, -0.4281496062992124485, 0.4176697321401328655 ) ) ;
#2990=CARTESIAN_POINT ( 'NONE',  ( -0.7939632545931750718, -0.05778040916215560624, -0.4822834645669293319 ) ) ;
#2992=CARTESIAN_POINT ( 'NONE',  ( -1.161417322834644716, 0.1660481256975885056, 0.3530559997133364547 ) ) ;
#2993=PLANE ( 'NONE',  #27790 ) ;
#2994=CARTESIAN_POINT ( 'NONE',  ( 1.036745406824147731, 0.05413385826771666132, 0.4176697321401328100 ) ) ;
#2995=CARTESIAN_POINT ( 'NONE',  ( 1.082677165354331228, 0.07958543189024071263, -0.2665933059059888421 ) ) ;
#2996=EDGE_LOOP ( 'NONE', ( #15859, #23992, #77417, #3808 ) ) ;
#2998=CARTESIAN_POINT ( 'NONE',  ( -0.6299212598425188991, -0.1870078740157480879, -0.4822834645669291653 ) ) ;
#2999=EDGE_LOOP ( 'NONE', ( #27644, #63108, #51265, #67302 ) ) ;
#3000=CARTESIAN_POINT ( 'NONE',  ( 0.2165354330708668673, 0.07958543189024071263, -0.2665933059059888421 ) ) ;
#3001=CARTESIAN_POINT ( 'NONE',  ( -1.010498687664041384, -0.4281496062992127816, -0.4176697321401328100 ) ) ;
#3002=CARTESIAN_POINT ( 'NONE',  ( 0.9055118110236227702, -0.6692913385826771977, 8.415575281601705876E-17 ) ) ;
#3003=CARTESIAN_POINT ( 'NONE',  ( 0.8661417322834652488, -0.1870078740157480879, -0.4822834645669291653 ) ) ;
#3004=CARTESIAN_POINT ( 'NONE',  ( -0.3149606299212590610, -0.1870078740157479769, 0.4822834645669291653 ) ) ;
#3005=CARTESIAN_POINT ( 'NONE',  ( -0.8333333333333323711, 0.2952755905511811885, 0.1292274648535926551 ) ) ;
#3007=CARTESIAN_POINT ( 'NONE',  ( -1.456692913385826182, -0.6692913385826771977, 8.415575281601705876E-17 ) ) ;
#3008=CARTESIAN_POINT ( 'NONE',  ( -0.6561679790026240244, 0.2306618581243847221, -0.2411417322834647770 ) ) ;
#3009=CARTESIAN_POINT ( 'NONE',  ( -0.5380577427821514602, -0.004921259842519576551, 0.3153832671262227771 ) ) ;
#3010=CARTESIAN_POINT ( 'NONE',  ( 1.482939632545932307, -0.4281496062992124485, 0.4176697321401328655 ) ) ;
#3011=CARTESIAN_POINT ( 'NONE',  ( 1.482939632545932307, -0.4281496062992124485, 0.4176697321401328655 ) ) ;
#3012=CARTESIAN_POINT ( 'NONE',  ( -0.7939632545931754048, -0.3162353388693405765, 0.4822834645669290543 ) ) ;
#3014=CARTESIAN_POINT ( 'NONE',  ( 0.8202099737532813073, 0.2952755905511811885, 0.1292274648535926551 ) ) ;
#3016=DIRECTION ( 'NONE',  ( -0.000000000000000000, 1.000000000000000000, -0.000000000000000000 ) ) ;
#3017=CARTESIAN_POINT ( 'NONE',  ( -0.2624671916010490880, -0.6046776061558807314, 0.2411417322834647770 ) ) ;
#3018=CARTESIAN_POINT ( 'NONE',  ( -1.023622047244093558, -0.1870078740157479769, 0.3641732283464567677 ) ) ;
#3019=CARTESIAN_POINT ( 'NONE',  ( 0.9448818897637802916, -0.1870078740157480601, -0.3641732283464567677 ) ) ;
#3021=CARTESIAN_POINT ( 'NONE',  ( 1.325459317585302665, -0.3690944881889763329, 0.3153832671262228327 ) ) ;
#3022=CARTESIAN_POINT ( 'NONE',  ( 0.6824146981627303710, 0.2306618581243847221, -0.2411417322834647770 ) ) ;
#3024=PRODUCT ( 'Reversible Hardened Steel Jaws', 'Reversible Hardened Steel Jaws', '', ( #41826 ) ) ;
#3025=CARTESIAN_POINT ( 'NONE',  ( -0.3215223097112853146, -0.3162353388693405765, 0.4822834645669290543 ) ) ;
#3027=CARTESIAN_POINT ( 'NONE',  ( 1.312335958005249825, 0.1283753931104746893, -0.1820866141732285504 ) ) ;
#3028=CARTESIAN_POINT ( 'NONE',  ( -0.3937007874015740483, -0.1870078740157480879, -0.4822834645669291653 ) ) ;
#3030=CARTESIAN_POINT ( 'NONE',  ( 1.292650918635171564, -0.6692913385826773087, -0.1292274648535924053 ) ) ;
#3031=CARTESIAN_POINT ( 'NONE',  ( 0.3083989501312343062, -0.3162353388693405765, 0.4822834645669290543 ) ) ;
#3032=AXIS2_PLACEMENT_3D ( 'NONE', #58636, #79273, #2656 ) ;
#3033=CARTESIAN_POINT ( 'NONE',  ( 0.5971128608923891301, 0.1771653543307087075, -0.09757992244046823083 ) ) ;
#3035=CARTESIAN_POINT ( 'NONE',  ( 0.5314960629921267055, -0.4536011799217367080, 0.2665933059059888421 ) ) ;
#3036=CARTESIAN_POINT ( 'NONE',  ( -1.509186351706035767, -0.4281496062992124485, 0.4176697321401328655 ) ) ;
#3038=CARTESIAN_POINT ( 'NONE',  ( 0.9120734908136490793, 0.2952755905511810774, -0.1292274648535930714 ) ) ;
#3042=CARTESIAN_POINT ( 'NONE',  ( -0.05249343832020938322, -0.5023911411419708095, -0.1820866141732282451 ) ) ;
#3043=CARTESIAN_POINT ( 'NONE',  ( 0.2362204724409456558, -0.1870078740157479769, 0.4822834645669291653 ) ) ;
#3044=CARTESIAN_POINT ( 'NONE',  ( 1.312335958005250269, -0.5023911411419708095, 0.1820866141732285504 ) ) ;
#3045=CARTESIAN_POINT ( 'NONE',  ( -1.181102362204723644, -0.1870078740157480601, -0.3641732283464567677 ) ) ;
#3046=CARTESIAN_POINT ( 'NONE',  ( -1.515748031496062076, 0.1660481256975883668, -0.3530559997133364547 ) ) ;
#3047=CARTESIAN_POINT ( 'NONE',  ( 0.3871391076115493490, -0.3162353388693405765, 0.4822834645669290543 ) ) ;
#3048=CARTESIAN_POINT ( 'NONE',  ( 1.102362204724410155, -0.1870078740157480879, -0.4822834645669291653 ) ) ;
#3049=CARTESIAN_POINT ( 'NONE',  ( 1.603475055217291612, 0.7793870273546370520, 0.04573490813648269093 ) ) ;
#3050=CARTESIAN_POINT ( 'NONE',  ( 0.6692913385826777528, 0.2952755905511811885, 0.000000000000000000 ) ) ;
#3051=CARTESIAN_POINT ( 'NONE',  ( 1.384514435695538559, 0.2952755905511810774, -0.1292274648535930714 ) ) ;
#3052=CARTESIAN_POINT ( 'NONE',  ( 1.122047244094488860, -0.5400638737290845981, -0.3530559997133363437 ) ) ;
#3054=CARTESIAN_POINT ( 'NONE',  ( 0.6364829396325465405, -0.2845877964562161244, -0.3641732283464567121 ) ) ;
#3055=CARTESIAN_POINT ( 'NONE',  ( -1.555118110236219930, -0.4536011799217368745, -0.2665933059059886201 ) ) ;
#3056=CARTESIAN_POINT ( 'NONE',  ( -0.7217847769028863381, -0.3690944881889763329, 0.3153832671262228327 ) ) ;
#3057=CARTESIAN_POINT ( 'NONE',  ( 0.6627296587926515548, 0.1771653543307087630, 0.09757992244046791164 ) ) ;
#3058=CARTESIAN_POINT ( 'NONE',  ( 0.03280839895013198948, -0.6692913385826773087, -0.1292274648535924053 ) ) ;
#3059=CARTESIAN_POINT ( 'NONE',  ( 0.6233595800524939223, -0.3162353388693405765, 0.4822834645669290543 ) ) ;
#3060=CARTESIAN_POINT ( 'NONE',  ( -0.4921259842519677963, 0.1660481256975883668, -0.3530559997133364547 ) ) ;
#3061=CARTESIAN_POINT ( 'NONE',  ( 0.3018372703412079971, -0.3690944881889763329, 0.3153832671262228327 ) ) ;
#3062=CARTESIAN_POINT ( 'NONE',  ( 0.8661417322834652488, -0.1870078740157480879, -0.4822834645669291653 ) ) ;
#3063=EDGE_CURVE ( 'NONE', #8792, #38980, #1493, .T. ) ;
#3064=DIRECTION ( 'NONE',  ( 0.000000000000000000, -1.000000000000000000, -0.000000000000000000 ) ) ;
#3065=CARTESIAN_POINT ( 'NONE',  ( -0.7874015748031489847, -0.1870078740157479769, 0.4822834645669291653 ) ) ;
#3068=CARTESIAN_POINT ( 'NONE',  ( 1.012125901091929681, 2.412178165100495768E-16, -0.3791483426435169890 ) ) ;
#3069=CARTESIAN_POINT ( 'NONE',  ( -0.6955380577427815458, 0.05413385826771666132, 0.4176697321401328100 ) ) ;
#3070=CARTESIAN_POINT ( 'NONE',  ( -0.6233595800524928121, -0.05778040916215522460, 0.4822834645669289988 ) ) ;
#3071=( BOUNDED_SURFACE ( )  B_SPLINE_SURFACE ( 1, 2, ( 
 ( #13545, #26994, #19856, #45505, #25732, #33326, #14807, #46345, #64884, #58562, #33735, #78782, #71202, #39201, #65739, #928, #26585, #52657, #77942, #20271, #45921, #78363, #27410, #20694, #46766, #72040, #40466, #79, #1344, #59395, #13971, #58988, #41695, #74118, #72869, #79202, #42109, #34569, #61058, #35393, #66978, #47594, #48010, #80853, #67806, #42519, #53493, #27832, #80031, #21934, #3409, #16881, #74535, #48834, #10143, #28661, #40877, #16464, #23165, #29071, #34150, #80447, #61474, #21518, #8481, #54742, #47177, #35808, #3822, #29483, #59811, #22350, #15217, #41293, #2166, #9311, #55142, #66559, #9722, #73709, #8892, #60236, #15636, #2584, #28243, #73288, #22757, #34981, #54322, #53903, #79617, #60645, #48419, #2995, #16049, #67388, #29888, #82898, #37448, #55551, #76176, #44156, #18513, #57196, #82084, #81260, #17697, #68222, #69025, #37857, #12199, #69443, #56385, #50884, #36214, #61883, #4224, #23575, #74949, #25218, #43738, #76584, #49246, #17295, #10957, #11795, #18913, #63122, #18105, #5460, #69848, #42922, #43325, #31122, #5053, #10556, #68617, #36615, #62293, #4630, #30301, #63533, #55967, #81680, #50472, #23991, #49659, #56789, #5864, #24805, #82489, #50068, #75349, #31540, #30723, #11376, #37033, #62715, #24398, #75763, #20168, #819, #26481, #19328, #20590, #77414, #58033, #81349, #78680, #78259, #58459, #51713, #64363, #39951, #45818, #19750, #13863, #14287, #26891, #63944, #6281, #7967, #1650, #65637, #33630, #7547, #44980, #45404, #52550, #76997, #7119, #51294, #59293, #70676, #12609, #6700, #38267, #27307, #58883, #64781, #46242, #52966, #31957, #32790, #57618, #52132, #13032, #71938, #44563, #38685, #25631, #70254, #32369, #39522, #71517, #71100, #396, #77839, #26054, #13443, #39099, #65210, #33220, #1242, #34462, #73607, #29381, #60542, #2482, #60951, #28141, #53797, #21825, #16359, #72357, #47899, #40768, #8378, #66453, #79509, #55041, #8789, #3717, #47072, #53392, #15949, #21001, #2893, #15114, #66040, #34043, #10034, #41595, #54213, #67698, #59706, #74012, #46663, #14705, #47488, #15530, #34881, #67285, #40360, #3301, #42004, #28557, #2061, #72763, #9208, #27725, #79099, #73180, #35698, #21418, #60131, #41188, #66878, #79929, #22244, #9618, #35289, #28966, #54630, #80343, #22656, #48315, #61365, #43227, #43638, #24296, #4123, #23474, #42823, #69341, #36932, #68924, #49141, #56689, #62193, #49557, #81572, #49966, #4530, #75664, #36111, #74846, #74427, #81982, #63428, #11692, #30200, #55862, #82388, #18414, #29788, #81158, #5360, #23891, #55449, #18004, #68516, #75251, #61783, #37349, #76072, #63022, #12095, #31021, #37753, #5764, #24706, #50374, #44057, #31433, #30620, #69749, #17190, #10857, #36517, #80748, #62610, #11273, #17595, #23062, #4950, #56285, #48730, #16774, #42412, #68109, #10457, #83205, #50785, #58350, #39842, #71414, #6595, #32267, #58778, #78155, #6177, #57514, #65102, #57927, #31852, #52028, #19220, #64261, #38165, #77734, #52445, #45717, #71835, #20065, #14184, #65531, #26370, #13761, #39418, #7864, #7015, #7439, #63839, #44460, #33110, #25527, #1138, #711, #291, #12923, #13339, #46140, #26788, #57096, #18813, #76486, #45300, #70569, #20486, #82791, #38993, #38582, #25113, #25947, #51605, #77310, #70151, #12504, #51192, #76890, #44870, #19640, #70996, #64676, #32683, #16263, #59606, #65940, #2796, #67602, #15430, #27623, #78577, #20903, #22564, #28455, #66779, #80248, #72254, #3208, #33528, #27204, #8692, #28040, #47389, #54115, #41908, #73508, #28870, #73080, #59191, #1961, #21726, #14603, #8276, #34362, #48225, #40257, #33942, #53286, #78997, #21317, #46970, #72664, #47805, #41090, #34785, #22147, #15013, #40669, #15856, #79407, #79830, #60444, #66354, #60028, #1550, #2383, #52867, #53698, #9113, #41505, #46556, #67190, #9521, #35193, #60854, #73921, #54532, #43137, #56596, #48637, #62932, #9933, #3621, #68427, #4443, #23794, #30526, #18321, #49873, #5265, #49466, #35605, #36020, #81477, #74331, #68016, #10767, #82296, #16678, #10360, #61692, #4032, #42317, #29697, #55360, #24202, #75160, #11180 ),
 ( #37256, #17913, #81065, #75573, #68834, #17505, #36841, #23381, #69250, #42731, #49049, #74747, #43962, #43549, #62513, #17096, #36427, #30929, #4851, #62100, #56189, #24615, #11596, #29288, #54951, #50282, #75980, #61267, #80658, #81891, #30108, #55770, #22970, #32486, #13562, #58149, #71635, #518, #12002, #26171, #69658, #39643, #77959, #64901, #45937, #13987, #63334, #7238, #6816, #32912, #51832, #65334, #37656, #39216, #26601, #77537, #58578, #52253, #19872, #20288, #45521, #943, #71217, #13654, #39307, #6494, #57411, #32164, #6075, #58242, #38477, #78049, #52762, #76785, #77204, #78470, #57820, #51499, #64994, #19533, #59088, #7330, #19117, #25423, #32998, #12402, #58668, #39732, #31749, #1443, #1033, #83104, #20378, #46030, #71724, #27100, #608, #51088, #45190, #70047, #70893, #65428, #14080, #71307, #26264, #20795, #38059, #63736, #44766, #70463, #12820, #64161, #45613, #187, #25840, #13243, #38892, #26687, #64571, #52342, #19962, #7761, #33427, #6908, #32580, #51925, #77630, #46451, #21209, #1855, #65837, #80552, #78888, #22458, #59502, #8584, #28764, #66246, #53173, #41398, #41799, #3100, #79721, #28348, #35496, #35082, #9005, #16152, #73815, #54427, #46864, #80137, #22038, #2688, #54009, #72558, #48117, #79302, #59917, #27517, #72144, #67490, #60340, #53593, #34256, #9826, #47698, #21620, #15744, #61161, #3512, #8170, #33835, #29181, #54848, #14500, #40153, #9412, #14905, #47280, #40565, #2272, #34677, #27935, #72970, #15321, #40986, #66666, #73393, #67080, #60748, #43031, #82193, #75872, #16570, #11067, #18215, #67911, #37555, #75466, #10247, #30826, #24510, #56491, #11901, #36725, #35918, #55660, #22864, #23683, #43850, #50177, #24097, #62401, #5569, #74225, #42215, #61584, #3929, #29588, #63229, #81786, #31234, #55251, #80958, #48942, #49766, #56901, #17805, #56081, #43439, #69553, #23273, #81370, #69136, #68726, #48525, #74644, #16986, #42629, #68326, #10664, #36319, #61994, #4331, #5162, #29997, #49357, #11488, #75054, #62827, #37142, #4740, #17401, #30413, #45092, #52250, #26598, #7235, #83006, #64898, #58146, #38799, #64475, #57308, #58575, #32067, #12721, #37965, #33339, #32908, #13148, #6397, #19023, #77955, #515, #57728, #51829, #20284, #940, #18620, #44263, #45933, #39640, #71632, #13984, #45518, #25327, #91, #65331, #31650, #70796, #5979, #7668, #50991, #50582, #44671, #76289, #82595, #13557, #19441, #24914, #69954, #12308, #6812, #63641, #32483, #76689, #70366, #38381, #64057, #25744, #51407, #77109, #26168, #77534, #19869, #71214, #39213, #65751, #14410, #79630, #1356, #47607, #34994, #40479, #27846, #59824, #2598, #66157, #53917, #40064, #1765, #52669, #60250, #41710, #73301, #8496, #34163, #60659, #80046, #8084, #59408, #66992, #2179, #33747, #21948, #21120, #53507, #27422, #15650, #54336, #41306, #73724, #9324, #16063, #67402, #28256, #3008, #28675, #9737, #8906, #22365, #53083, #46359, #48024, #78796, #59001, #27007, #79215, #14820, #15231, #78376, #20707, #72053, #46780, #72471, #47190, #21531, #72882, #40890, #66572, #34582, #75363, #16895, #10157, #75777, #35408, #62307, #4644, #55156, #22771, #80867, #10571, #43751, #23179, #18118, #61489, #67820, #30315, #69457, #17309, #29497, #80462, #48434, #24411, #55983, #68631, #82097, #74133, #5067, #61072, #29086, #36228, #29902, #49261, #81694, #3423, #17711, #30736, #74963, #54756, #3837, #23590, #16478, #35823, #61897, #50081, #42125, #48849, #74550, #42534, #68236, #4238, #55566, #49673, #42937, #36630, #24005, #81274, #10971, #43339, #69040, #11390, #37047, #62729, #56399, #58360, #59201, #52455, #58790, #37871, #59616, #27214, #33120, #72265, #65950, #5474, #1148, #31136, #26799, #64686, #20913, #79008, #18526, #20076, #21328, #32693, #77744, #39852, #45727, #1971, #33538, #44169, #50485, #1560, #37462, #52877, #8286, #56803, #27634, #65543, #82502, #46566, #14613, #40267, #53296, #78165, #24818, #71424, #11807, #13771, #33952, #46980, #14195, #20496, #63135, #76189, #69862, #12213, #7025, #722, #26380, #71845, #52040, #39428, #65112, #7450, #7874, #46150, #78587 ) ),
 .UNSPECIFIED., .F., .F., .F. ) 
 B_SPLINE_SURFACE_WITH_KNOTS ( ( 2, 2 ),
 ( 3, 2, 2, 2, 2, 2, 2, 2, 2, 2, 2, 2, 2, 2, 2, 2, 2, 2, 2, 2, 2, 2, 2, 2, 2, 2, 2, 2, 2, 2, 2, 2, 2, 2, 2, 2, 2, 2, 2, 2, 2, 2, 2, 2, 2, 2, 2, 2, 2, 2, 2, 2, 2, 2, 2, 2, 2, 2, 2, 2, 2, 2, 2, 2, 2, 2, 2, 2, 2, 2, 2, 2, 2, 2, 2, 2, 2, 2, 2, 2, 2, 2, 2, 2, 2, 2, 2, 2, 2, 2, 2, 2, 2, 2, 2, 2, 2, 2, 2, 2, 2, 2, 2, 2, 2, 2, 2, 2, 2, 2, 2, 2, 2, 2, 2, 2, 2, 2, 2, 2, 2, 2, 2, 2, 2, 2, 2, 2, 2, 2, 2, 2, 2, 2, 2, 2, 2, 2, 2, 2, 2, 2, 2, 2, 2, 2, 2, 2, 2, 2, 2, 2, 2, 2, 2, 2, 2, 2, 2, 2, 2, 2, 2, 2, 2, 2, 2, 2, 2, 2, 2, 2, 2, 2, 2, 2, 2, 2, 2, 2, 2, 2, 2, 2, 2, 2, 2, 2, 2, 2, 2, 2, 2, 2, 2, 2, 2, 2, 2, 2, 2, 2, 2, 2, 2, 2, 2, 2, 2, 2, 2, 2, 2, 2, 2, 2, 2, 2, 2, 2, 2, 2, 2, 2, 2, 2, 2, 2, 2, 2, 2, 2, 2, 2, 2, 2, 2, 2, 2, 2, 2, 2, 2, 2, 2, 2, 2, 2, 2, 2, 2, 2, 2, 2, 2, 3 ),
 ( 0.000000000000000000, 1.000000000000000000 ),
 ( 0.000000000000000000, 0.003787878787878787984, 0.007575757575757575968, 0.01136363636363636395, 0.01515151515151515194, 0.01893939393939393992, 0.02272727272727272790, 0.02651515151515151589, 0.03030303030303030387, 0.03409090909090908839, 0.03787878787878787984, 0.04166666666666666435, 0.04545454545454545581, 0.04924242424242424032, 0.05303030303030303177, 0.05681818181818181629, 0.06060606060606060774, 0.06439393939393939226, 0.06818181818181817677, 0.07196969696969697516, 0.07575757575757575968, 0.07954545454545454419, 0.08333333333333332871, 0.08712121212121212710, 0.09090909090909091161, 0.09469696969696969613, 0.09848484848484848064, 0.1022727272727272790, 0.1060606060606060635, 0.1098484848484848481, 0.1136363636363636326, 0.1174242424242424310, 0.1212121212121212155, 0.1250000000000000000, 0.1287878787878787845, 0.1325757575757575690, 0.1363636363636363535, 0.1401515151515151381, 0.1439393939393939503, 0.1477272727272727348, 0.1515151515151515194, 0.1553030303030303039, 0.1590909090909090884, 0.1628787878787878729, 0.1666666666666666574, 0.1704545454545454419, 0.1742424242424242542, 0.1780303030303030387, 0.1818181818181818232, 0.1856060606060606077, 0.1893939393939393923, 0.1931818181818181768, 0.1969696969696969613, 0.2007575757575757458, 0.2045454545454545581, 0.2083333333333333426, 0.2121212121212121271, 0.2159090909090909116, 0.2196969696969696961, 0.2234848484848484806, 0.2272727272727272652, 0.2310606060606060497, 0.2348484848484848619, 0.2386363636363636465, 0.2424242424242424310, 0.2462121212121212155, 0.2500000000000000000, 0.2537878787878787845, 0.2575757575757575690, 0.2613636363636363535, 0.2651515151515151381, 0.2689393939393939226, 0.2727272727272727071, 0.2765151515151514916, 0.2803030303030302761, 0.2840909090909091161, 0.2878787878787879007, 0.2916666666666666852, 0.2954545454545454697, 0.2992424242424242542, 0.3030303030303030387, 0.3068181818181818232, 0.3106060606060606077, 0.3143939393939393923, 0.3181818181818181768, 0.3219696969696969613, 0.3257575757575757458, 0.3295454545454545303, 0.3333333333333333148, 0.3371212121212120993, 0.3409090909090908839, 0.3446969696969697239, 0.3484848484848485084, 0.3522727272727272929, 0.3560606060606060774, 0.3598484848484848619, 0.3636363636363636465, 0.3674242424242424310, 0.3712121212121212155, 0.3750000000000000000, 0.3787878787878787845, 0.3825757575757575690, 0.3863636363636363535, 0.3901515151515151381, 0.3939393939393939226, 0.3977272727272727071, 0.4015151515151514916, 0.4053030303030302761, 0.4090909090909091161, 0.4128787878787879007, 0.4166666666666666852, 0.4204545454545454697, 0.4242424242424242542, 0.4280303030303030387, 0.4318181818181818232, 0.4356060606060606077, 0.4393939393939393923, 0.4431818181818181768, 0.4469696969696969613, 0.4507575757575757458, 0.4545454545454545303, 0.4583333333333333148, 0.4621212121212120993, 0.4659090909090908839, 0.4696969696969697239, 0.4734848484848485084, 0.4772727272727272929, 0.4810606060606060774, 0.4848484848484848619, 0.4886363636363636465, 0.4924242424242424310, 0.4962121212121212155, 0.5000000000000000000, 0.5037878787878787845, 0.5075757575757575690, 0.5113636363636363535, 0.5151515151515151381, 0.5189393939393939226, 0.5227272727272727071, 0.5265151515151514916, 0.5303030303030302761, 0.5340909090909090606, 0.5378787878787878451, 0.5416666666666666297, 0.5454545454545454142, 0.5492424242424241987, 0.5530303030303029832, 0.5568181818181817677, 0.5606060606060605522, 0.5643939393939394478, 0.5681818181818182323, 0.5719696969696970168, 0.5757575757575758013, 0.5795454545454545858, 0.5833333333333333703, 0.5871212121212121549, 0.5909090909090909394, 0.5946969696969697239, 0.5984848484848485084, 0.6022727272727272929, 0.6060606060606060774, 0.6098484848484848619, 0.6136363636363636465, 0.6174242424242424310, 0.6212121212121212155, 0.6250000000000000000, 0.6287878787878787845, 0.6325757575757575690, 0.6363636363636363535, 0.6401515151515151381, 0.6439393939393939226, 0.6477272727272727071, 0.6515151515151514916, 0.6553030303030302761, 0.6590909090909090606, 0.6628787878787878451, 0.6666666666666666297, 0.6704545454545454142, 0.6742424242424241987, 0.6780303030303029832, 0.6818181818181817677, 0.6856060606060605522, 0.6893939393939394478, 0.6931818181818182323, 0.6969696969696970168, 0.7007575757575758013, 0.7045454545454545858, 0.7083333333333333703, 0.7121212121212121549, 0.7159090909090909394, 0.7196969696969697239, 0.7234848484848485084, 0.7272727272727272929, 0.7310606060606060774, 0.7348484848484848619, 0.7386363636363636465, 0.7424242424242424310, 0.7462121212121212155, 0.7500000000000000000, 0.7537878787878787845, 0.7575757575757575690, 0.7613636363636363535, 0.7651515151515151381, 0.7689393939393939226, 0.7727272727272727071, 0.7765151515151514916, 0.7803030303030302761, 0.7840909090909090606, 0.7878787878787878451, 0.7916666666666666297, 0.7954545454545454142, 0.7992424242424241987, 0.8030303030303029832, 0.8068181818181817677, 0.8106060606060605522, 0.8143939393939394478, 0.8181818181818182323, 0.8219696969696970168, 0.8257575757575758013, 0.8295454545454545858, 0.8333333333333333703, 0.8371212121212121549, 0.8409090909090909394, 0.8446969696969697239, 0.8484848484848485084, 0.8522727272727272929, 0.8560606060606060774, 0.8598484848484848619, 0.8636363636363636465, 0.8674242424242424310, 0.8712121212121212155, 0.8750000000000000000, 0.8787878787878787845, 0.8825757575757575690, 0.8863636363636363535, 0.8901515151515151381, 0.8939393939393939226, 0.8977272727272727071, 0.9015151515151514916, 0.9053030303030302761, 0.9090909090909090606, 0.9128787878787878451, 0.9166666666666666297, 0.9204545454545454142, 0.9242424242424241987, 0.9280303030303029832, 0.9318181818181817677, 0.9356060606060605522, 0.9393939393939394478, 0.9431818181818182323, 0.9469696969696970168, 0.9507575757575758013, 0.9545454545454545858, 0.9583333333333333703, 0.9621212121212121549, 0.9659090909090909394 ),
 .UNSPECIFIED. ) 
 GEOMETRIC_REPRESENTATION_ITEM ( )  RATIONAL_B_SPLINE_SURFACE ( (
 ( 1.000000000000000000, 0.9659258262890683122, 1.000000000000000000, 0.9659258262890683122, 1.000000000000000000, 0.9659258262890683122, 1.000000000000000000, 0.9659258262890683122, 1.000000000000000000, 0.9659258262890683122, 1.000000000000000000, 0.9659258262890683122, 1.000000000000000000, 0.9659258262890683122, 1.000000000000000000, 0.9659258262890683122, 1.000000000000000000, 0.9659258262890683122, 1.000000000000000000, 0.9659258262890683122, 1.000000000000000000, 0.9659258262890683122, 1.000000000000000000, 0.9659258262890683122, 1.000000000000000000, 0.9659258262890683122, 1.000000000000000000, 0.9659258262890683122, 1.000000000000000000, 0.9659258262890683122, 1.000000000000000000, 0.9659258262890683122, 1.000000000000000000, 0.9659258262890683122, 1.000000000000000000, 0.9659258262890683122, 1.000000000000000000, 0.9659258262890683122, 1.000000000000000000, 0.9659258262890683122, 1.000000000000000000, 0.9659258262890683122, 1.000000000000000000, 0.9659258262890683122, 1.000000000000000000, 0.9659258262890683122, 1.000000000000000000, 0.9659258262890683122, 1.000000000000000000, 0.9659258262890683122, 1.000000000000000000, 0.9659258262890683122, 1.000000000000000000, 0.9659258262890683122, 1.000000000000000000, 0.9659258262890683122, 1.000000000000000000, 0.9659258262890683122, 1.000000000000000000, 0.9659258262890683122, 1.000000000000000000, 0.9659258262890683122, 1.000000000000000000, 0.9659258262890683122, 1.000000000000000000, 0.9659258262890683122, 1.000000000000000000, 0.9659258262890683122, 1.000000000000000000, 0.9659258262890683122, 1.000000000000000000, 0.9659258262890683122, 1.000000000000000000, 0.9659258262890683122, 1.000000000000000000, 0.9659258262890683122, 1.000000000000000000, 0.9659258262890683122, 1.000000000000000000, 0.9659258262890683122, 1.000000000000000000, 0.9659258262890683122, 1.000000000000000000, 0.9659258262890683122, 1.000000000000000000, 0.9659258262890683122, 1.000000000000000000, 0.9659258262890683122, 1.000000000000000000, 0.9659258262890683122, 1.000000000000000000, 0.9659258262890683122, 1.000000000000000000, 0.9659258262890683122, 1.000000000000000000, 0.9659258262890683122, 1.000000000000000000, 0.9659258262890683122, 1.000000000000000000, 0.9659258262890683122, 1.000000000000000000, 0.9659258262890683122, 1.000000000000000000, 0.9659258262890683122, 1.000000000000000000, 0.9659258262890683122, 1.000000000000000000, 0.9659258262890683122, 1.000000000000000000, 0.9659258262890683122, 1.000000000000000000, 0.9659258262890683122, 1.000000000000000000, 0.9659258262890683122, 1.000000000000000000, 0.9659258262890683122, 1.000000000000000000, 0.9659258262890683122, 1.000000000000000000, 0.9659258262890683122, 1.000000000000000000, 0.9659258262890683122, 1.000000000000000000, 0.9659258262890683122, 1.000000000000000000, 0.9659258262890683122, 1.000000000000000000, 0.9659258262890683122, 1.000000000000000000, 0.9659258262890683122, 1.000000000000000000, 0.9659258262890683122, 1.000000000000000000, 0.9659258262890683122, 1.000000000000000000, 0.9659258262890683122, 1.000000000000000000, 0.9659258262890683122, 1.000000000000000000, 0.9659258262890683122, 1.000000000000000000, 0.9659258262890683122, 1.000000000000000000, 0.9659258262890683122, 1.000000000000000000, 0.9659258262890683122, 1.000000000000000000, 0.9659258262890683122, 1.000000000000000000, 0.9659258262890683122, 1.000000000000000000, 0.9659258262890683122, 1.000000000000000000, 0.9659258262890683122, 1.000000000000000000, 0.9659258262890683122, 1.000000000000000000, 0.9659258262890683122, 1.000000000000000000, 0.9659258262890683122, 1.000000000000000000, 0.9659258262890683122, 1.000000000000000000, 0.9659258262890683122, 1.000000000000000000, 0.9659258262890683122, 1.000000000000000000, 0.9659258262890683122, 1.000000000000000000, 0.9659258262890683122, 1.000000000000000000, 0.9659258262890683122, 1.000000000000000000, 0.9659258262890683122, 1.000000000000000000, 0.9659258262890683122, 1.000000000000000000, 0.9659258262890683122, 1.000000000000000000, 0.9659258262890683122, 1.000000000000000000, 0.9659258262890683122, 1.000000000000000000, 0.9659258262890683122, 1.000000000000000000, 0.9659258262890683122, 1.000000000000000000, 0.9659258262890683122, 1.000000000000000000, 0.9659258262890683122, 1.000000000000000000, 0.9659258262890683122, 1.000000000000000000, 0.9659258262890683122, 1.000000000000000000, 0.9659258262890683122, 1.000000000000000000, 0.9659258262890683122, 1.000000000000000000, 0.9659258262890683122, 1.000000000000000000, 0.9659258262890683122, 1.000000000000000000, 0.9659258262890683122, 1.000000000000000000, 0.9659258262890683122, 1.000000000000000000, 0.9659258262890683122, 1.000000000000000000, 0.9659258262890683122, 1.000000000000000000, 0.9659258262890683122, 1.000000000000000000, 0.9659258262890683122, 1.000000000000000000, 0.9659258262890683122, 1.000000000000000000, 0.9659258262890683122, 1.000000000000000000, 0.9659258262890683122, 1.000000000000000000, 0.9659258262890683122, 1.000000000000000000, 0.9659258262890683122, 1.000000000000000000, 0.9659258262890683122, 1.000000000000000000, 0.9659258262890683122, 1.000000000000000000, 0.9659258262890683122, 1.000000000000000000, 0.9659258262890683122, 1.000000000000000000, 0.9659258262890683122, 1.000000000000000000, 0.9659258262890683122, 1.000000000000000000, 0.9659258262890683122, 1.000000000000000000, 0.9659258262890683122, 1.000000000000000000, 0.9659258262890683122, 1.000000000000000000, 0.9659258262890683122, 1.000000000000000000, 0.9659258262890683122, 1.000000000000000000, 0.9659258262890683122, 1.000000000000000000, 0.9659258262890683122, 1.000000000000000000, 0.9659258262890683122, 1.000000000000000000, 0.9659258262890683122, 1.000000000000000000, 0.9659258262890683122, 1.000000000000000000, 0.9659258262890683122, 1.000000000000000000, 0.9659258262890683122, 1.000000000000000000, 0.9659258262890683122, 1.000000000000000000, 0.9659258262890683122, 1.000000000000000000, 0.9659258262890683122, 1.000000000000000000, 0.9659258262890683122, 1.000000000000000000, 0.9659258262890683122, 1.000000000000000000, 0.9659258262890683122, 1.000000000000000000, 0.9659258262890683122, 1.000000000000000000, 0.9659258262890683122, 1.000000000000000000, 0.9659258262890683122, 1.000000000000000000, 0.9659258262890683122, 1.000000000000000000, 0.9659258262890683122, 1.000000000000000000, 0.9659258262890683122, 1.000000000000000000, 0.9659258262890683122, 1.000000000000000000, 0.9659258262890683122, 1.000000000000000000, 0.9659258262890683122, 1.000000000000000000, 0.9659258262890683122, 1.000000000000000000, 0.9659258262890683122, 1.000000000000000000, 0.9659258262890683122, 1.000000000000000000, 0.9659258262890683122, 1.000000000000000000, 0.9659258262890683122, 1.000000000000000000, 0.9659258262890683122, 1.000000000000000000, 0.9659258262890683122, 1.000000000000000000, 0.9659258262890683122, 1.000000000000000000, 0.9659258262890683122, 1.000000000000000000, 0.9659258262890683122, 1.000000000000000000, 0.9659258262890683122, 1.000000000000000000, 0.9659258262890683122, 1.000000000000000000, 0.9659258262890683122, 1.000000000000000000, 0.9659258262890683122, 1.000000000000000000, 0.9659258262890683122, 1.000000000000000000, 0.9659258262890683122, 1.000000000000000000, 0.9659258262890683122, 1.000000000000000000, 0.9659258262890683122, 1.000000000000000000, 0.9659258262890683122, 1.000000000000000000, 0.9659258262890683122, 1.000000000000000000, 0.9659258262890683122, 1.000000000000000000, 0.9659258262890683122, 1.000000000000000000, 0.9659258262890683122, 1.000000000000000000, 0.9659258262890683122, 1.000000000000000000, 0.9659258262890683122, 1.000000000000000000, 0.9659258262890683122, 1.000000000000000000, 0.9659258262890683122, 1.000000000000000000, 0.9659258262890683122, 1.000000000000000000, 0.9659258262890683122, 1.000000000000000000, 0.9659258262890683122, 1.000000000000000000, 0.9659258262890683122, 1.000000000000000000, 0.9659258262890683122, 1.000000000000000000, 0.9659258262890683122, 1.000000000000000000, 0.9659258262890683122, 1.000000000000000000, 0.9659258262890683122, 1.000000000000000000, 0.9659258262890683122, 1.000000000000000000, 0.9659258262890683122, 1.000000000000000000, 0.9659258262890683122, 1.000000000000000000, 0.9659258262890683122, 1.000000000000000000, 0.9659258262890683122, 1.000000000000000000, 0.9659258262890683122, 1.000000000000000000, 0.9659258262890683122, 1.000000000000000000, 0.9659258262890683122, 1.000000000000000000, 0.9659258262890683122, 1.000000000000000000, 0.9659258262890683122, 1.000000000000000000, 0.9659258262890683122, 1.000000000000000000, 0.9659258262890683122, 1.000000000000000000, 0.9659258262890683122, 1.000000000000000000, 0.9659258262890683122, 1.000000000000000000, 0.9659258262890683122, 1.000000000000000000, 0.9659258262890683122, 1.000000000000000000, 0.9659258262890683122, 1.000000000000000000, 0.9659258262890683122, 1.000000000000000000, 0.9659258262890683122, 1.000000000000000000, 0.9659258262890683122, 1.000000000000000000, 0.9659258262890683122, 1.000000000000000000, 0.9659258262890683122, 1.000000000000000000, 0.9659258262890683122, 1.000000000000000000, 0.9659258262890683122, 1.000000000000000000, 0.9659258262890683122, 1.000000000000000000, 0.9659258262890683122, 1.000000000000000000, 0.9659258262890683122, 1.000000000000000000, 0.9659258262890683122, 1.000000000000000000, 0.9659258262890683122, 1.000000000000000000, 0.9659258262890683122, 1.000000000000000000, 0.9659258262890683122, 1.000000000000000000, 0.9659258262890683122, 1.000000000000000000, 0.9659258262890683122, 1.000000000000000000, 0.9659258262890683122, 1.000000000000000000, 0.9659258262890683122, 1.000000000000000000, 0.9659258262890683122, 1.000000000000000000, 0.9659258262890683122, 1.000000000000000000, 0.9659258262890683122, 1.000000000000000000, 0.9659258262890683122, 1.000000000000000000, 0.9659258262890683122, 1.000000000000000000, 0.9659258262890683122, 1.000000000000000000, 0.9659258262890683122, 1.000000000000000000, 0.9659258262890683122, 1.000000000000000000, 0.9659258262890683122, 1.000000000000000000, 0.9659258262890683122, 1.000000000000000000, 0.9659258262890683122, 1.000000000000000000, 0.9659258262890683122, 1.000000000000000000, 0.9659258262890683122, 1.000000000000000000, 0.9659258262890683122, 1.000000000000000000, 0.9659258262890683122, 1.000000000000000000, 0.9659258262890683122, 1.000000000000000000, 0.9659258262890683122, 1.000000000000000000, 0.9659258262890683122, 1.000000000000000000, 0.9659258262890683122, 1.000000000000000000, 0.9659258262890683122, 1.000000000000000000, 0.9659258262890683122, 1.000000000000000000, 0.9659258262890683122, 1.000000000000000000, 0.9659258262890683122, 1.000000000000000000, 0.9659258262890683122, 1.000000000000000000, 0.9659258262890683122, 1.000000000000000000, 0.9659258262890683122, 1.000000000000000000, 0.9659258262890683122, 1.000000000000000000, 0.9659258262890683122, 1.000000000000000000, 0.9659258262890683122, 1.000000000000000000, 0.9659258262890683122, 1.000000000000000000, 0.9659258262890683122, 1.000000000000000000, 0.9659258262890683122, 1.000000000000000000, 0.9659258262890683122, 1.000000000000000000, 0.9659258262890683122, 1.000000000000000000, 0.9659258262890683122, 1.000000000000000000, 0.9659258262890683122, 1.000000000000000000, 0.9659258262890683122, 1.000000000000000000, 0.9659258262890683122, 1.000000000000000000, 0.9659258262890683122, 1.000000000000000000, 0.9659258262890683122, 1.000000000000000000),
 ( 1.000000000000000000, 0.9659258262890683122, 1.000000000000000000, 0.9659258262890683122, 1.000000000000000000, 0.9659258262890683122, 1.000000000000000000, 0.9659258262890683122, 1.000000000000000000, 0.9659258262890683122, 1.000000000000000000, 0.9659258262890683122, 1.000000000000000000, 0.9659258262890683122, 1.000000000000000000, 0.9659258262890683122, 1.000000000000000000, 0.9659258262890683122, 1.000000000000000000, 0.9659258262890683122, 1.000000000000000000, 0.9659258262890683122, 1.000000000000000000, 0.9659258262890683122, 1.000000000000000000, 0.9659258262890683122, 1.000000000000000000, 0.9659258262890683122, 1.000000000000000000, 0.9659258262890683122, 1.000000000000000000, 0.9659258262890683122, 1.000000000000000000, 0.9659258262890683122, 1.000000000000000000, 0.9659258262890683122, 1.000000000000000000, 0.9659258262890683122, 1.000000000000000000, 0.9659258262890683122, 1.000000000000000000, 0.9659258262890683122, 1.000000000000000000, 0.9659258262890683122, 1.000000000000000000, 0.9659258262890683122, 1.000000000000000000, 0.9659258262890683122, 1.000000000000000000, 0.9659258262890683122, 1.000000000000000000, 0.9659258262890683122, 1.000000000000000000, 0.9659258262890683122, 1.000000000000000000, 0.9659258262890683122, 1.000000000000000000, 0.9659258262890683122, 1.000000000000000000, 0.9659258262890683122, 1.000000000000000000, 0.9659258262890683122, 1.000000000000000000, 0.9659258262890683122, 1.000000000000000000, 0.9659258262890683122, 1.000000000000000000, 0.9659258262890683122, 1.000000000000000000, 0.9659258262890683122, 1.000000000000000000, 0.9659258262890683122, 1.000000000000000000, 0.9659258262890683122, 1.000000000000000000, 0.9659258262890683122, 1.000000000000000000, 0.9659258262890683122, 1.000000000000000000, 0.9659258262890683122, 1.000000000000000000, 0.9659258262890683122, 1.000000000000000000, 0.9659258262890683122, 1.000000000000000000, 0.9659258262890683122, 1.000000000000000000, 0.9659258262890683122, 1.000000000000000000, 0.9659258262890683122, 1.000000000000000000, 0.9659258262890683122, 1.000000000000000000, 0.9659258262890683122, 1.000000000000000000, 0.9659258262890683122, 1.000000000000000000, 0.9659258262890683122, 1.000000000000000000, 0.9659258262890683122, 1.000000000000000000, 0.9659258262890683122, 1.000000000000000000, 0.9659258262890683122, 1.000000000000000000, 0.9659258262890683122, 1.000000000000000000, 0.9659258262890683122, 1.000000000000000000, 0.9659258262890683122, 1.000000000000000000, 0.9659258262890683122, 1.000000000000000000, 0.9659258262890683122, 1.000000000000000000, 0.9659258262890683122, 1.000000000000000000, 0.9659258262890683122, 1.000000000000000000, 0.9659258262890683122, 1.000000000000000000, 0.9659258262890683122, 1.000000000000000000, 0.9659258262890683122, 1.000000000000000000, 0.9659258262890683122, 1.000000000000000000, 0.9659258262890683122, 1.000000000000000000, 0.9659258262890683122, 1.000000000000000000, 0.9659258262890683122, 1.000000000000000000, 0.9659258262890683122, 1.000000000000000000, 0.9659258262890683122, 1.000000000000000000, 0.9659258262890683122, 1.000000000000000000, 0.9659258262890683122, 1.000000000000000000, 0.9659258262890683122, 1.000000000000000000, 0.9659258262890683122, 1.000000000000000000, 0.9659258262890683122, 1.000000000000000000, 0.9659258262890683122, 1.000000000000000000, 0.9659258262890683122, 1.000000000000000000, 0.9659258262890683122, 1.000000000000000000, 0.9659258262890683122, 1.000000000000000000, 0.9659258262890683122, 1.000000000000000000, 0.9659258262890683122, 1.000000000000000000, 0.9659258262890683122, 1.000000000000000000, 0.9659258262890683122, 1.000000000000000000, 0.9659258262890683122, 1.000000000000000000, 0.9659258262890683122, 1.000000000000000000, 0.9659258262890683122, 1.000000000000000000, 0.9659258262890683122, 1.000000000000000000, 0.9659258262890683122, 1.000000000000000000, 0.9659258262890683122, 1.000000000000000000, 0.9659258262890683122, 1.000000000000000000, 0.9659258262890683122, 1.000000000000000000, 0.9659258262890683122, 1.000000000000000000, 0.9659258262890683122, 1.000000000000000000, 0.9659258262890683122, 1.000000000000000000, 0.9659258262890683122, 1.000000000000000000, 0.9659258262890683122, 1.000000000000000000, 0.9659258262890683122, 1.000000000000000000, 0.9659258262890683122, 1.000000000000000000, 0.9659258262890683122, 1.000000000000000000, 0.9659258262890683122, 1.000000000000000000, 0.9659258262890683122, 1.000000000000000000, 0.9659258262890683122, 1.000000000000000000, 0.9659258262890683122, 1.000000000000000000, 0.9659258262890683122, 1.000000000000000000, 0.9659258262890683122, 1.000000000000000000, 0.9659258262890683122, 1.000000000000000000, 0.9659258262890683122, 1.000000000000000000, 0.9659258262890683122, 1.000000000000000000, 0.9659258262890683122, 1.000000000000000000, 0.9659258262890683122, 1.000000000000000000, 0.9659258262890683122, 1.000000000000000000, 0.9659258262890683122, 1.000000000000000000, 0.9659258262890683122, 1.000000000000000000, 0.9659258262890683122, 1.000000000000000000, 0.9659258262890683122, 1.000000000000000000, 0.9659258262890683122, 1.000000000000000000, 0.9659258262890683122, 1.000000000000000000, 0.9659258262890683122, 1.000000000000000000, 0.9659258262890683122, 1.000000000000000000, 0.9659258262890683122, 1.000000000000000000, 0.9659258262890683122, 1.000000000000000000, 0.9659258262890683122, 1.000000000000000000, 0.9659258262890683122, 1.000000000000000000, 0.9659258262890683122, 1.000000000000000000, 0.9659258262890683122, 1.000000000000000000, 0.9659258262890683122, 1.000000000000000000, 0.9659258262890683122, 1.000000000000000000, 0.9659258262890683122, 1.000000000000000000, 0.9659258262890683122, 1.000000000000000000, 0.9659258262890683122, 1.000000000000000000, 0.9659258262890683122, 1.000000000000000000, 0.9659258262890683122, 1.000000000000000000, 0.9659258262890683122, 1.000000000000000000, 0.9659258262890683122, 1.000000000000000000, 0.9659258262890683122, 1.000000000000000000, 0.9659258262890683122, 1.000000000000000000, 0.9659258262890683122, 1.000000000000000000, 0.9659258262890683122, 1.000000000000000000, 0.9659258262890683122, 1.000000000000000000, 0.9659258262890683122, 1.000000000000000000, 0.9659258262890683122, 1.000000000000000000, 0.9659258262890683122, 1.000000000000000000, 0.9659258262890683122, 1.000000000000000000, 0.9659258262890683122, 1.000000000000000000, 0.9659258262890683122, 1.000000000000000000, 0.9659258262890683122, 1.000000000000000000, 0.9659258262890683122, 1.000000000000000000, 0.9659258262890683122, 1.000000000000000000, 0.9659258262890683122, 1.000000000000000000, 0.9659258262890683122, 1.000000000000000000, 0.9659258262890683122, 1.000000000000000000, 0.9659258262890683122, 1.000000000000000000, 0.9659258262890683122, 1.000000000000000000, 0.9659258262890683122, 1.000000000000000000, 0.9659258262890683122, 1.000000000000000000, 0.9659258262890683122, 1.000000000000000000, 0.9659258262890683122, 1.000000000000000000, 0.9659258262890683122, 1.000000000000000000, 0.9659258262890683122, 1.000000000000000000, 0.9659258262890683122, 1.000000000000000000, 0.9659258262890683122, 1.000000000000000000, 0.9659258262890683122, 1.000000000000000000, 0.9659258262890683122, 1.000000000000000000, 0.9659258262890683122, 1.000000000000000000, 0.9659258262890683122, 1.000000000000000000, 0.9659258262890683122, 1.000000000000000000, 0.9659258262890683122, 1.000000000000000000, 0.9659258262890683122, 1.000000000000000000, 0.9659258262890683122, 1.000000000000000000, 0.9659258262890683122, 1.000000000000000000, 0.9659258262890683122, 1.000000000000000000, 0.9659258262890683122, 1.000000000000000000, 0.9659258262890683122, 1.000000000000000000, 0.9659258262890683122, 1.000000000000000000, 0.9659258262890683122, 1.000000000000000000, 0.9659258262890683122, 1.000000000000000000, 0.9659258262890683122, 1.000000000000000000, 0.9659258262890683122, 1.000000000000000000, 0.9659258262890683122, 1.000000000000000000, 0.9659258262890683122, 1.000000000000000000, 0.9659258262890683122, 1.000000000000000000, 0.9659258262890683122, 1.000000000000000000, 0.9659258262890683122, 1.000000000000000000, 0.9659258262890683122, 1.000000000000000000, 0.9659258262890683122, 1.000000000000000000, 0.9659258262890683122, 1.000000000000000000, 0.9659258262890683122, 1.000000000000000000, 0.9659258262890683122, 1.000000000000000000, 0.9659258262890683122, 1.000000000000000000, 0.9659258262890683122, 1.000000000000000000, 0.9659258262890683122, 1.000000000000000000, 0.9659258262890683122, 1.000000000000000000, 0.9659258262890683122, 1.000000000000000000, 0.9659258262890683122, 1.000000000000000000, 0.9659258262890683122, 1.000000000000000000, 0.9659258262890683122, 1.000000000000000000, 0.9659258262890683122, 1.000000000000000000, 0.9659258262890683122, 1.000000000000000000, 0.9659258262890683122, 1.000000000000000000, 0.9659258262890683122, 1.000000000000000000, 0.9659258262890683122, 1.000000000000000000, 0.9659258262890683122, 1.000000000000000000, 0.9659258262890683122, 1.000000000000000000, 0.9659258262890683122, 1.000000000000000000, 0.9659258262890683122, 1.000000000000000000, 0.9659258262890683122, 1.000000000000000000, 0.9659258262890683122, 1.000000000000000000, 0.9659258262890683122, 1.000000000000000000, 0.9659258262890683122, 1.000000000000000000, 0.9659258262890683122, 1.000000000000000000, 0.9659258262890683122, 1.000000000000000000, 0.9659258262890683122, 1.000000000000000000, 0.9659258262890683122, 1.000000000000000000, 0.9659258262890683122, 1.000000000000000000, 0.9659258262890683122, 1.000000000000000000, 0.9659258262890683122, 1.000000000000000000, 0.9659258262890683122, 1.000000000000000000, 0.9659258262890683122, 1.000000000000000000, 0.9659258262890683122, 1.000000000000000000, 0.9659258262890683122, 1.000000000000000000, 0.9659258262890683122, 1.000000000000000000, 0.9659258262890683122, 1.000000000000000000, 0.9659258262890683122, 1.000000000000000000, 0.9659258262890683122, 1.000000000000000000, 0.9659258262890683122, 1.000000000000000000, 0.9659258262890683122, 1.000000000000000000, 0.9659258262890683122, 1.000000000000000000, 0.9659258262890683122, 1.000000000000000000, 0.9659258262890683122, 1.000000000000000000, 0.9659258262890683122, 1.000000000000000000, 0.9659258262890683122, 1.000000000000000000, 0.9659258262890683122, 1.000000000000000000, 0.9659258262890683122, 1.000000000000000000, 0.9659258262890683122, 1.000000000000000000, 0.9659258262890683122, 1.000000000000000000, 0.9659258262890683122, 1.000000000000000000, 0.9659258262890683122, 1.000000000000000000, 0.9659258262890683122, 1.000000000000000000, 0.9659258262890683122, 1.000000000000000000, 0.9659258262890683122, 1.000000000000000000, 0.9659258262890683122, 1.000000000000000000, 0.9659258262890683122, 1.000000000000000000, 0.9659258262890683122, 1.000000000000000000, 0.9659258262890683122, 1.000000000000000000, 0.9659258262890683122, 1.000000000000000000, 0.9659258262890683122, 1.000000000000000000, 0.9659258262890683122, 1.000000000000000000, 0.9659258262890683122, 1.000000000000000000, 0.9659258262890683122, 1.000000000000000000, 0.9659258262890683122, 1.000000000000000000, 0.9659258262890683122, 1.000000000000000000, 0.9659258262890683122, 1.000000000000000000, 0.9659258262890683122, 1.000000000000000000, 0.9659258262890683122, 1.000000000000000000, 0.9659258262890683122, 1.000000000000000000, 0.9659258262890683122, 1.000000000000000000, 0.9659258262890683122, 1.000000000000000000) ) ) 
 REPRESENTATION_ITEM ( '' )  SURFACE ( )  );
#3074=ORIENTED_EDGE ( 'NONE', *, *, #76299, .F. ) ;
#3075=CARTESIAN_POINT ( 'NONE',  ( 0.6364829396325465405, -0.2845877964562161244, -0.3641732283464567121 ) ) ;
#3076=AXIS2_PLACEMENT_3D ( 'NONE', #17291, #17694, #10954 ) ;
#3078=ADVANCED_FACE ( 'NONE', ( #35438 ), #1646, .F. ) ;
#3079=CARTESIAN_POINT ( 'NONE',  ( 1.266404199475066328, -0.05778040916215522460, 0.4822834645669289988 ) ) ;
#3080=LINE ( 'NONE', #79283, #82937 ) ;
#3081=CARTESIAN_POINT ( 'NONE',  ( -1.227034120734907585, 0.1771653543307087630, 0.09757992244046791164 ) ) ;
#3082=CARTESIAN_POINT ( 'NONE',  ( 1.535433070866142558, 0.2952755905511811885, 0.000000000000000000 ) ) ;
#3083=CARTESIAN_POINT ( 'NONE',  ( -1.410761154855642463, -0.05778040916215522460, 0.4822834645669289988 ) ) ;
#3084=CARTESIAN_POINT ( 'NONE',  ( 0.2952755905511819101, 0.1660481256975883668, -0.3530559997133364547 ) ) ;
#3086=CARTESIAN_POINT ( 'NONE',  ( -0.1837270341207340729, 0.2306618581243847221, -0.2411417322834647770 ) ) ;
#3087=CARTESIAN_POINT ( 'NONE',  ( -0.8530183727034112984, -0.3690944881889765550, -0.3153832671262227771 ) ) ;
#3088=CARTESIAN_POINT ( 'NONE',  ( 0.8398950131233602345, 0.2306618581243847221, -0.2411417322834647770 ) ) ;
#3089=CARTESIAN_POINT ( 'NONE',  ( 5.463695987328526437E-16, -0.1870078740157479769, 0.4822834645669291653 ) ) ;
#3090=CARTESIAN_POINT ( 'NONE',  ( 0.5395952360118035918, 0.02791078216816508459, -0.4328096321851889194 ) ) ;
#3093=CARTESIAN_POINT ( 'NONE',  ( 0.9842519685039378130, -0.6692913385826771977, 8.415575281601705876E-17 ) ) ;
#3094=CARTESIAN_POINT ( 'NONE',  ( 0.09186351706036799403, -0.4281496062992127816, -0.4176697321401328100 ) ) ;
#3095=CARTESIAN_POINT ( 'NONE',  ( -0.9120734908136475250, -0.6692913385826773087, -0.1292274648535924053 ) ) ;
#3096=CARTESIAN_POINT ( 'NONE',  ( 0.9514435695538062676, -0.05778040916215522460, 0.4822834645669289988 ) ) ;
#3097=CARTESIAN_POINT ( 'NONE',  ( 1.036745406824147731, 0.05413385826771666132, 0.4176697321401328100 ) ) ;
#3099=CARTESIAN_POINT ( 'NONE',  ( -0.4921259842519677963, -0.5400638737290844871, 0.3530559997133364547 ) ) ;
#3100=CARTESIAN_POINT ( 'NONE',  ( 0.7677165354330716118, 0.1660481256975883668, -0.3530559997133364547 ) ) ;
#3101=CARTESIAN_POINT ( 'NONE',  ( -0.1377952755905504645, -0.5400638737290845981, -0.3530559997133363437 ) ) ;
#3102=CARTESIAN_POINT ( 'NONE',  ( 0.8792650918635177559, -0.004921259842519576551, 0.3153832671262227771 ) ) ;
#3103=CARTESIAN_POINT ( 'NONE',  ( -1.463254593175852492, -0.6692913385826773087, -0.1292274648535924053 ) ) ;
#3104=CARTESIAN_POINT ( 'NONE',  ( -1.633858267716534529, -0.5400638737290845981, -0.3530559997133363437 ) ) ;
#3105=CARTESIAN_POINT ( 'NONE',  ( 0.4658792650918640033, -0.3162353388693405765, 0.4822834645669290543 ) ) ;
#3106=( LENGTH_UNIT ( ) NAMED_UNIT ( * ) SI_UNIT ( $, .METRE. ) );
#3108=ORIENTED_EDGE ( 'NONE', *, *, #19583, .F. ) ;
#3109=ORIENTED_EDGE ( 'NONE', *, *, #31497, .T. ) ;
#3110=CARTESIAN_POINT ( 'NONE',  ( 0.9251968503937015864, 0.1660481256975883668, -0.3530559997133364547 ) ) ;
#3111=CARTESIAN_POINT ( 'NONE',  ( 0.5511811023622054106, -0.1870078740157480601, -0.3641732283464567677 ) ) ;
#3114=CARTESIAN_POINT ( 'NONE',  ( -0.7478466213799872531, 2.204724409448818978, -0.5309055118110235227 ) ) ;
#3117=CARTESIAN_POINT ( 'NONE',  ( -0.6430446194225712953, 0.05413385826771626580, -0.4176697321401330321 ) ) ;
#3119=CARTESIAN_POINT ( 'NONE',  ( -0.5446194225721777693, -0.3162353388693409650, -0.4822834645669289433 ) ) ;
#3120=CARTESIAN_POINT ( 'NONE',  ( 0.5183727034120741983, 0.2952755905511810774, -0.1292274648535930714 ) ) ;
#3122=CARTESIAN_POINT ( 'NONE',  ( 1.305774278215223960, 0.2952755905511810774, -0.1292274648535930714 ) ) ;
#3123=CARTESIAN_POINT ( 'NONE',  ( 1.213910761154856077, 0.2066929133858248224, 0.1054918080437525219 ) ) ;
#3125=CARTESIAN_POINT ( 'NONE',  ( 1.607611548556431069, -0.5511811023622048555, -0.09757992244046775898 ) ) ;
#3127=CARTESIAN_POINT ( 'NONE',  ( -1.482939632545930975, -0.004921259842519576551, 0.3153832671262227771 ) ) ;
#3129=CARTESIAN_POINT ( 'NONE',  ( 0.03280839895013198948, -0.6692913385826773087, -0.1292274648535924053 ) ) ;
#3130=CARTESIAN_POINT ( 'NONE',  ( 1.607611548556431069, -0.6692913385826773087, -0.1292274648535924053 ) ) ;
#3132=B_SPLINE_CURVE_WITH_KNOTS ( 'NONE', 3,
 ( #60581, #66490, #71974, #53835 ),
 .UNSPECIFIED., .F., .F.,
 ( 4, 4 ),
 ( 1.734723475976807094E-18, 0.001434885020664811769 ),
 .UNSPECIFIED. ) ;
#3133=CARTESIAN_POINT ( 'NONE',  ( -1.240157480314959759, 0.07958543189024085140, 0.2665933059059887866 ) ) ;
#3134=CARTESIAN_POINT ( 'NONE',  ( 0.8398950131233602345, -0.6046776061558807314, 0.2411417322834647770 ) ) ;
#3135=CARTESIAN_POINT ( 'NONE',  ( 1.233595800524935227, -0.5023911411419708095, 0.1820866141732285504 ) ) ;
#3138=CARTESIAN_POINT ( 'NONE',  ( -1.056430446194224881, 0.1771653543307087075, -0.09757992244046823083 ) ) ;
#3139=CARTESIAN_POINT ( 'NONE',  ( 1.358267716535433323, 0.1660481256975885056, 0.3530559997133364547 ) ) ;
#3141=CARTESIAN_POINT ( 'NONE',  ( -0.06561679790026180015, -0.4281496062992127816, -0.4176697321401328100 ) ) ;
#3142=CARTESIAN_POINT ( 'NONE',  ( -1.496062992125983815, -0.1870078740157479769, 0.3641732283464567677 ) ) ;
#3143=CARTESIAN_POINT ( 'NONE',  ( -0.4461942257217840213, 0.1283753931104748280, 0.1820866141732283561 ) ) ;
#3144=CARTESIAN_POINT ( 'NONE',  ( -0.2230971128608915943, -0.4281496062992127816, -0.4176697321401328100 ) ) ;
#3145=CARTESIAN_POINT ( 'NONE',  ( -1.377952755905511140, -0.5511811023622047445, 6.969142054262312111E-17 ) ) ;
#3147=CARTESIAN_POINT ( 'NONE',  ( 0.3740157480314966754, 0.1660481256975883668, -0.3530559997133364547 ) ) ;
#3150=CARTESIAN_POINT ( 'NONE',  ( -1.095800524934382292, -0.05778040916215522460, 0.4822834645669289988 ) ) ;
#3151=CARTESIAN_POINT ( 'NONE',  ( -0.4199475065616791736, 0.1283753931104746893, -0.1820866141732285504 ) ) ;
#3152=CARTESIAN_POINT ( 'NONE',  ( -1.292650918635170010, 0.2952755905511810774, -0.1292274648535930714 ) ) ;
#3153=CARTESIAN_POINT ( 'NONE',  ( 0.2099737532808405305, -0.6046776061558807314, 0.2411417322834647770 ) ) ;
#3154=CARTESIAN_POINT ( 'NONE',  ( 0.4265091863517067594, 0.1771653543307087630, 0.09757992244046791164 ) ) ;
#3155=CARTESIAN_POINT ( 'NONE',  ( -0.7874015748031489847, -0.1870078740157479769, 0.3641732283464567677 ) ) ;
#3156=CARTESIAN_POINT ( 'NONE',  ( -1.108923884514435132, -0.3162353388693405765, 0.4822834645669290543 ) ) ;
#3157=CARTESIAN_POINT ( 'NONE',  ( -1.443569553805773564, -0.6046776061558807314, 0.2411417322834647770 ) ) ;
#3158=CARTESIAN_POINT ( 'NONE',  ( 1.410761154855643795, -0.05778040916215560624, -0.4822834645669293319 ) ) ;
#3159=DIRECTION ( 'NONE',  ( -3.096699300667737957E-16, 1.000000000000000000, -0.000000000000000000 ) ) ;
#3160=CARTESIAN_POINT ( 'NONE',  ( 0.6627296587926517768, -0.5511811023622048555, -0.09757992244046775898 ) ) ;
#3161=CARTESIAN_POINT ( 'NONE',  ( 0.9514435695538062676, -0.3162353388693409650, -0.4822834645669289433 ) ) ;
#3163=CARTESIAN_POINT ( 'NONE',  ( 1.489501312335958172, -0.08942795157528024563, -0.3641732283464568787 ) ) ;
#3165=CARTESIAN_POINT ( 'NONE',  ( -0.7414698162729651543, -0.6692913385826771977, 0.1292274648535927661 ) ) ;
#3166=CARTESIAN_POINT ( 'NONE',  ( -0.9120734908136475250, -0.6692913385826773087, -0.1292274648535924053 ) ) ;
#3167=CARTESIAN_POINT ( 'NONE',  ( 0.4199475065616803948, -0.6046776061558809534, -0.2411417322834644161 ) ) ;
#3168=CARTESIAN_POINT ( 'NONE',  ( -1.574803149606298636, -0.1870078740157479769, 0.3641732283464567677 ) ) ;
#3170=CARTESIAN_POINT ( 'NONE',  ( -1.325459317585300889, -0.4281496062992127816, -0.4176697321401328100 ) ) ;
#3171=CARTESIAN_POINT ( 'NONE',  ( 0.2559055118110243332, 0.1660481256975885056, 0.3530559997133364547 ) ) ;
#3172=CARTESIAN_POINT ( 'NONE',  ( 0.9711286089238851948, 0.2306618581243848609, 0.2411417322834645549 ) ) ;
#3173=CARTESIAN_POINT ( 'NONE',  ( -1.586052503253847501, 1.299212598425198095, -0.1653254495020571035 ) ) ;
#3180=CARTESIAN_POINT ( 'NONE',  ( -0.1377952755905504645, 0.07958543189024085140, 0.2665933059059887866 ) ) ;
#3181=CARTESIAN_POINT ( 'NONE',  ( -0.4986876640419942164, -0.6046776061558807314, 0.2411417322834647770 ) ) ;
#3182=CARTESIAN_POINT ( 'NONE',  ( 0.7742782152230978099, -0.4281496062992124485, 0.4176697321401328655 ) ) ;
#3184=CARTESIAN_POINT ( 'NONE',  ( 0.1115485564304470323, 0.1771653543307087630, 0.09757992244046791164 ) ) ;
#3185=CARTESIAN_POINT ( 'NONE',  ( -1.003937007874014853, 0.1660481256975885056, 0.3530559997133364547 ) ) ;
#3186=CARTESIAN_POINT ( 'NONE',  ( 1.325459317585302665, 0.05413385826771626580, -0.4176697321401330321 ) ) ;
#3189=CARTESIAN_POINT ( 'NONE',  ( 1.141732283464567566, 0.2952755905511811885, 0.000000000000000000 ) ) ;
#3192=CARTESIAN_POINT ( 'NONE',  ( 0.8989501312335963501, -0.6692913385826773087, -0.1292274648535924053 ) ) ;
#3193=CARTESIAN_POINT ( 'NONE',  ( -1.555118110236219930, 0.1660481256975885056, 0.3530559997133364547 ) ) ;
#3194=CARTESIAN_POINT ( 'NONE',  ( -1.148293963254592542, 0.1771653543307087630, 0.09757992244046791164 ) ) ;
#3195=CARTESIAN_POINT ( 'NONE',  ( -1.095800524934382292, -0.3162353388693409650, -0.4822834645669289433 ) ) ;
#3197=CARTESIAN_POINT ( 'NONE',  ( -0.9711286089238838626, 0.1539470093639521697, -0.1968503937007875793 ) ) ;
#3198=CARTESIAN_POINT ( 'NONE',  ( 1.351706036745407680, 0.05413385826771666132, 0.4176697321401328100 ) ) ;
#3200=CARTESIAN_POINT ( 'NONE',  ( -0.2887139107611542133, 0.2306618581243848609, 0.2411417322834645549 ) ) ;
#3201=CARTESIAN_POINT ( 'NONE',  ( -0.6627296587926503335, -0.6692913385826771977, 0.1292274648535927661 ) ) ;
#3202=EDGE_CURVE ( 'NONE', #46767, #50394, #10096, .T. ) ;
#3203=CARTESIAN_POINT ( 'NONE',  ( 1.561679790026247350, -0.4281496062992124485, 0.4176697321401328655 ) ) ;
#3205=CARTESIAN_POINT ( 'NONE',  ( 0.3412073490813655186, 0.2306618581243848609, 0.2411417322834645549 ) ) ;
#3206=( BOUNDED_CURVE ( )  B_SPLINE_CURVE ( 2, ( #2191, #26610, #46370, #33758, #14423, #72481, #52262, #71645, #40074, #65761, #59420, #78806, #21135 ),
 .UNSPECIFIED., .F., .F. ) 
 B_SPLINE_CURVE_WITH_KNOTS ( ( 3, 2, 2, 2, 2, 2, 3 ),
 ( 0.2308514478433235373, 0.2310606060606060774, 0.2348484848484848619, 0.2386363636363636465, 0.2424242424242424310, 0.2462121212121212155, 0.2464212794294037556 ),
 .UNSPECIFIED. ) 
 CURVE ( )  GEOMETRIC_REPRESENTATION_ITEM ( )  RATIONAL_B_SPLINE_CURVE ( ( 0.9964447847208416364, 0.9981185001348089614, 1.000000000000000000, 0.9659258262890683122, 1.000000000000000000, 0.9659258262890683122, 1.000000000000000000, 0.9659258262890683122, 1.000000000000000000, 0.9659258262890683122, 1.000000000000000000, 0.9981185001348089614, 0.9964447847208417475 ) ) 
 REPRESENTATION_ITEM ( '' )  );
#3208=CARTESIAN_POINT ( 'NONE',  ( -1.128608923884513837, 0.1283753931104746893, -0.1820866141732285504 ) ) ;
#3211=VERTEX_POINT ( 'NONE', #4676 ) ;
#3213=CARTESIAN_POINT ( 'NONE',  ( -1.594488188976377563, -0.5400638737290844871, 0.3530559997133364547 ) ) ;
#3215=CARTESIAN_POINT ( 'NONE',  ( 1.568241469816273659, -0.08942795157528024563, -0.3641732283464568787 ) ) ;
#3216=CARTESIAN_POINT ( 'NONE',  ( -1.712598425196849572, 0.1660481256975885056, 0.3530559997133364547 ) ) ;
#3217=DIRECTION ( 'NONE',  ( -3.096699300667737957E-16, 1.000000000000000000, -0.000000000000000000 ) ) ;
#3218=CARTESIAN_POINT ( 'NONE',  ( 0.9341826970036752886, -6.978086149529499157E-16, -0.4118477457932994135 ) ) ;
#3220=CARTESIAN_POINT ( 'NONE',  ( -0.2427821522309703550, -0.2845877964562159024, 0.3641732283464567677 ) ) ;
#3221=CARTESIAN_POINT ( 'NONE',  ( -0.8202099737532801971, -0.5511811023622046335, 0.09757992244046803654 ) ) ;
#3222=CARTESIAN_POINT ( 'NONE',  ( -1.318897637795274802, 0.1660481256975885056, 0.3530559997133364547 ) ) ;
#3223=CARTESIAN_POINT ( 'NONE',  ( 0.5249343832021003964, 0.2306618581243847221, -0.2411417322834647770 ) ) ;
#3224=CARTESIAN_POINT ( 'NONE',  ( -1.069553805774277722, -0.6692913385826773087, -0.1292274648535924053 ) ) ;
#3227=CARTESIAN_POINT ( 'NONE',  ( -1.194225721784776262, -0.4281496062992124485, 0.4176697321401328655 ) ) ;
#3230=CARTESIAN_POINT ( 'NONE',  ( -1.595398199321656829, 1.034147571970760238, -0.1559797534342476366 ) ) ;
#3234=CARTESIAN_POINT ( 'NONE',  ( -0.6758530183727028406, 0.2952755905511811885, 0.1292274648535926551 ) ) ;
#3235=CARTESIAN_POINT ( 'NONE',  ( 1.430446194225722500, -0.4281496062992127816, -0.4176697321401328100 ) ) ;
#3236=CARTESIAN_POINT ( 'NONE',  ( -1.712598425196849572, 0.1660481256975885056, 0.3530559997133364547 ) ) ;
#3238=CARTESIAN_POINT ( 'NONE',  ( -1.384514435695537005, 0.2952755905511811885, 0.1292274648535926551 ) ) ;
#3239=CARTESIAN_POINT ( 'NONE',  ( -0.8923884514435688198, 0.2306618581243847221, -0.2411417322834647770 ) ) ;
#3241=CARTESIAN_POINT ( 'NONE',  ( 0.2887139107611556010, -0.5023911411419708095, 0.1820866141732285504 ) ) ;
#3244=CARTESIAN_POINT ( 'NONE',  ( -0.1115485564304453947, -0.5511811023622046335, 0.09757992244046803654 ) ) ;
#3245=CARTESIAN_POINT ( 'NONE',  ( 1.056430446194226436, -0.5511811023622048555, -0.09757992244046775898 ) ) ;
#3246=CARTESIAN_POINT ( 'NONE',  ( 0.9055118110236227702, -0.6692913385826771977, 8.415575281601705876E-17 ) ) ;
#3248=CARTESIAN_POINT ( 'NONE',  ( -0.2690288713910754526, -0.5511811023622046335, 0.09757992244046803654 ) ) ;
#3250=CARTESIAN_POINT ( 'NONE',  ( 1.391076115485564868, -0.6046776061558807314, 0.2411417322834647770 ) ) ;
#3251=EDGE_CURVE ( 'NONE', #68517, #7209, #62522, .T. ) ;
#3252=CARTESIAN_POINT ( 'NONE',  ( -1.397637795275589623, -0.4536011799217368745, -0.2665933059059886201 ) ) ;
#3254=CARTESIAN_POINT ( 'NONE',  ( 0.07217847769028949700, -0.3162353388693405765, 0.4822834645669290543 ) ) ;
#3255=CARTESIAN_POINT ( 'NONE',  ( 1.679790026246720025, 0.1283753931104748280, 0.1820866141732283561 ) ) ;
#3256=VECTOR ( 'NONE', #49580, 39.37007874015748143 ) ;
#3257=CARTESIAN_POINT ( 'NONE',  ( 0.6889763779527563470, 0.07958543189024071263, -0.2665933059059888421 ) ) ;
#3258=CARTESIAN_POINT ( 'NONE',  ( -0.1968503937007867743, -0.5511811023622047445, 6.969142054262312111E-17 ) ) ;
#3259=CARTESIAN_POINT ( 'NONE',  ( -0.6364829396325453192, -0.05778040916215560624, -0.4822834645669293319 ) ) ;
#3262=CARTESIAN_POINT ( 'NONE',  ( -0.006561679790025524116, -0.05778040916215560624, -0.4822834645669293319 ) ) ;
#3265=CARTESIAN_POINT ( 'NONE',  ( -0.09842519685039295696, 0.07958543189024071263, -0.2665933059059888421 ) ) ;
#3266=CARTESIAN_POINT ( 'NONE',  ( -0.03280839895013062252, -0.6692913385826771977, 0.1292274648535927661 ) ) ;
#3267=CARTESIAN_POINT ( 'NONE',  ( -1.489501312335957062, -0.05778040916215522460, 0.4822834645669289988 ) ) ;
#3268=CARTESIAN_POINT ( 'NONE',  ( -1.528871391076114250, -0.5511811023622046335, 0.09757992244046803654 ) ) ;
#3269=CARTESIAN_POINT ( 'NONE',  ( 1.404199475065617708, 0.05413385826771626580, -0.4176697321401330321 ) ) ;
#3270=CARTESIAN_POINT ( 'NONE',  ( -1.332020997375327642, -0.05778040916215522460, 0.4822834645669289988 ) ) ;
#3271=CARTESIAN_POINT ( 'NONE',  ( -0.5839895013123351797, 0.1771653543307087075, -0.09757992244046823083 ) ) ;
#3275=CARTESIAN_POINT ( 'NONE',  ( 1.443569553805774897, -0.5023911411419708095, -0.1820866141732282451 ) ) ;
#3276=CARTESIAN_POINT ( 'NONE',  ( 1.194225721784777594, -0.3690944881889765550, -0.3153832671262227771 ) ) ;
#3277=CARTESIAN_POINT ( 'NONE',  ( 0.4061203303035133549, 3.421639014772782816E-16, 0.3464511005275203726 ) ) ;
#3278=CARTESIAN_POINT ( 'NONE',  ( 0.8989501312335963501, -0.6692913385826773087, -0.1292274648535924053 ) ) ;
#3280=CARTESIAN_POINT ( 'NONE',  ( 1.076115485564305141, 0.1283753931104746893, -0.1820866141732285504 ) ) ;
#3281=CARTESIAN_POINT ( 'NONE',  ( 0.2427821522309719648, -0.05778040916215522460, 0.4822834645669289988 ) ) ;
#3282=CARTESIAN_POINT ( 'NONE',  ( -0.9317585301837263412, -0.4281496062992127816, -0.4176697321401328100 ) ) ;
#3283=CARTESIAN_POINT ( 'NONE',  ( 2.795275590551181466, 2.401574803149606474, 0.000000000000000000 ) ) ;
#3286=CARTESIAN_POINT ( 'NONE',  ( 0.4068241469816279987, -0.3690944881889765550, -0.3153832671262227771 ) ) ;
#3287=EDGE_LOOP ( 'NONE', ( #48332, #50283, #2170, #53603 ) ) ;
#3289=ORIENTED_EDGE ( 'NONE', *, *, #62867, .T. ) ;
#3290=CARTESIAN_POINT ( 'NONE',  ( -0.6299212598425188991, -0.1870078740157479769, 0.4822834645669291653 ) ) ;
#3291=CARTESIAN_POINT ( 'NONE',  ( -0.03280839895013062252, 0.2952755905511810774, -0.1292274648535930714 ) ) ;
#3292=CARTESIAN_POINT ( 'NONE',  ( -0.3477690288713902178, 0.1771653543307087075, -0.09757992244046823083 ) ) ;
#3294=CARTESIAN_POINT ( 'NONE',  ( 0.6036745406824154392, 0.2306618581243847221, -0.2411417322834647770 ) ) ;
#3295=CARTESIAN_POINT ( 'NONE',  ( -0.7480314960629914633, -0.6692913385826771977, 8.415575281601705876E-17 ) ) ;
#3296=CARTESIAN_POINT ( 'NONE',  ( -0.3477690288713905509, -0.6692913385826771977, 0.1292274648535927661 ) ) ;
#3297=CARTESIAN_POINT ( 'NONE',  ( 1.286089238845145033, 0.2306618581243848609, 0.2411417322834645549 ) ) ;
#3298=CARTESIAN_POINT ( 'NONE',  ( 0.8989501312335963501, -0.6692913385826773087, -0.1292274648535924053 ) ) ;
#3299=CARTESIAN_POINT ( 'NONE',  ( 0.8858267716535438430, 0.1660481256975885056, 0.3530559997133364547 ) ) ;
#3301=CARTESIAN_POINT ( 'NONE',  ( -0.03937007874015669567, 0.1771653543307087630, 0.000000000000000000 ) ) ;
#3305=CARTESIAN_POINT ( 'NONE',  ( -0.6692913385826764205, -0.5511811023622047445, 6.969142054262312111E-17 ) ) ;
#3306=CARTESIAN_POINT ( 'NONE',  ( -0.4265091863517051496, -0.6692913385826771977, 0.1292274648535927661 ) ) ;
#3308=CARTESIAN_POINT ( 'NONE',  ( -0.1312335958005241554, 0.2306618581243848609, 0.2411417322834645549 ) ) ;
#3309=CARTESIAN_POINT ( 'NONE',  ( -0.6233595800524928121, -0.05778040916215522460, 0.4822834645669289988 ) ) ;
#3310=CARTESIAN_POINT ( 'NONE',  ( -1.181102362204723644, -0.1870078740157479769, 0.4822834645669291653 ) ) ;
#3311=CARTESIAN_POINT ( 'NONE',  ( -1.318897637795274802, -0.5400638737290845981, -0.3530559997133363437 ) ) ;
#3312=VECTOR ( 'NONE', #47726, 39.37007874015748143 ) ;
#3313=CARTESIAN_POINT ( 'NONE',  ( 1.102362204724410155, -0.1870078740157480601, -0.3641732283464567677 ) ) ;
#3316=CARTESIAN_POINT ( 'NONE',  ( 0.6692913385826777528, 0.1771653543307087630, 0.000000000000000000 ) ) ;
#3317=CARTESIAN_POINT ( 'NONE',  ( 0.09186351706036827158, 0.05413385826771666132, 0.4176697321401328100 ) ) ;
#3318=CARTESIAN_POINT ( 'NONE',  ( 0.3083989501312343062, -0.05778040916215560624, -0.4822834645669293319 ) ) ;
#3321=CARTESIAN_POINT ( 'NONE',  ( -0.5839895013123352907, 0.2952755905511810219, -0.1292274648535930437 ) ) ;
#3322=ORIENTED_EDGE ( 'NONE', *, *, #33628, .F. ) ;
#3325=CARTESIAN_POINT ( 'NONE',  ( -0.5774278215223089816, 0.1283753931104746893, -0.1820866141732285504 ) ) ;
#3326=CARTESIAN_POINT ( 'NONE',  ( -0.8005249343832013809, -0.4281496062992124485, 0.4176697321401328655 ) ) ;
#3329=CARTESIAN_POINT ( 'NONE',  ( 1.568241469816273659, -0.05778040916215560624, -0.4822834645669293319 ) ) ;
#3330=CARTESIAN_POINT ( 'NONE',  ( 0.8923884514435701520, -0.6046776061558809534, -0.2411417322834644161 ) ) ;
#3331=CARTESIAN_POINT ( 'NONE',  ( 0.7020997375328090762, -0.3162353388693405765, 0.4822834645669290543 ) ) ;
#3332=CARTESIAN_POINT ( 'NONE',  ( -0.6430446194225712953, -0.004921259842519870586, -0.3153832671262229437 ) ) ;
#3333=CARTESIAN_POINT ( 'NONE',  ( 0.07874015748031558404, -0.1870078740157480879, -0.4822834645669291653 ) ) ;
#3335=CARTESIAN_POINT ( 'NONE',  ( -0.5249343832020990641, 0.1283753931104748280, 0.1820866141732283561 ) ) ;
#3336=CARTESIAN_POINT ( 'NONE',  ( -0.2821522309711278487, 0.2952755905511811885, 0.1292274648535926551 ) ) ;
#3338=CARTESIAN_POINT ( 'NONE',  ( -1.456692913385826182, -0.6692913385826771977, 8.415575281601705876E-17 ) ) ;
#3339=CARTESIAN_POINT ( 'NONE',  ( -0.09842519685039295696, 0.07958543189024071263, -0.2665933059059888421 ) ) ;
#3340=CARTESIAN_POINT ( 'NONE',  ( 1.489501312335958172, -0.2845877964562159024, 0.3641732283464567677 ) ) ;
#3341=CARTESIAN_POINT ( 'NONE',  ( -1.069553805774277722, 0.2952755905511811885, 0.1292274648535926551 ) ) ;
#3342=CARTESIAN_POINT ( 'NONE',  ( -0.5183727034120726440, 0.1771653543307087630, 0.09757992244046791164 ) ) ;
#3344=CARTESIAN_POINT ( 'NONE',  ( -0.9580052493438311334, -0.4281496062992124485, 0.4176697321401328655 ) ) ;
#3345=CARTESIAN_POINT ( 'NONE',  ( -0.4724409448818890911, -0.1870078740157480879, -0.4822834645669291653 ) ) ;
#3346=CARTESIAN_POINT ( 'NONE',  ( 0.3346456692913393205, -0.5400638737290845981, -0.3530559997133363437 ) ) ;
#3349=CARTESIAN_POINT ( 'NONE',  ( 0.2034120734908144990, -0.5511811023622046335, 0.09757992244046803654 ) ) ;
#3350=CARTESIAN_POINT ( 'NONE',  ( 0.9711286089238851948, 0.2306618581243848609, 0.2411417322834645549 ) ) ;
#3351=CARTESIAN_POINT ( 'NONE',  ( -1.397637795275589623, 0.07958543189024085140, 0.2665933059059887866 ) ) ;
#3353=CARTESIAN_POINT ( 'NONE',  ( 1.030183727034121421, -0.05778040916215522460, 0.4822834645669289988 ) ) ;
#3354=CARTESIAN_POINT ( 'NONE',  ( -1.482939632545930975, -0.3690944881889765550, -0.3153832671262227771 ) ) ;
#3355=CARTESIAN_POINT ( 'NONE',  ( -0.5577427821522301654, -0.05778040916215560624, -0.4822834645669293319 ) ) ;
#3356=CARTESIAN_POINT ( 'NONE',  ( 0.2755905511811031494, 0.1771653543307087630, 0.000000000000000000 ) ) ;
#3357=CARTESIAN_POINT ( 'NONE',  ( -0.8764808517432188806, 2.130908986194174812E-15, -0.4281993546915511817 ) ) ;
#3358=CARTESIAN_POINT ( 'NONE',  ( 0.4461942257217855201, -0.5023911411419708095, 0.1820866141732285504 ) ) ;
#3359=CARTESIAN_POINT ( 'NONE',  ( -0.01968503937007793844, -0.5400638737290844871, 0.3530559997133364547 ) ) ;
#3360=EDGE_CURVE ( 'NONE', #56464, #69946, #43407, .T. ) ;
#3361=CARTESIAN_POINT ( 'NONE',  ( -0.2099737532808391705, 0.2306618581243848609, 0.2411417322834645549 ) ) ;
#3363=CARTESIAN_POINT ( 'NONE',  ( -1.253280839895012377, -0.05778040916215522460, 0.4822834645669289988 ) ) ;
#3365=CARTESIAN_POINT ( 'NONE',  ( 0.9186351706036751663, -0.5023911411419708095, 0.1820866141732285504 ) ) ;
#3366=CARTESIAN_POINT ( 'NONE',  ( 0.06561679790026316017, -0.4281496062992124485, 0.4176697321401328655 ) ) ;
#3367=CARTESIAN_POINT ( 'NONE',  ( -0.2690288713910754526, -0.6692913385826771977, 0.1292274648535927661 ) ) ;
#3368=CARTESIAN_POINT ( 'NONE',  ( -0.3674540682414689785, 0.1283753931104748280, 0.1820866141732283561 ) ) ;
#3370=CARTESIAN_POINT ( 'NONE',  ( -0.2624671916010490880, -0.5023911411419708095, 0.1820866141732285504 ) ) ;
#3371=CARTESIAN_POINT ( 'NONE',  ( 0.3740157480314966754, -0.5400638737290844871, 0.3530559997133364547 ) ) ;
#3372=CARTESIAN_POINT ( 'NONE',  ( -1.332020997375327642, -0.2845877964562161244, -0.3641732283464567121 ) ) ;
#3375=CARTESIAN_POINT ( 'NONE',  ( -1.043307086614172041, -0.5400638737290844871, 0.3530559997133364547 ) ) ;
#3378=CARTESIAN_POINT ( 'NONE',  ( -1.443569553805773564, -0.5023911411419708095, 0.1820866141732285504 ) ) ;
#3379=CARTESIAN_POINT ( 'NONE',  ( -0.2624671916010490880, 0.2306618581243847221, -0.2411417322834647770 ) ) ;
#3382=CARTESIAN_POINT ( 'NONE',  ( -1.364829396325458521, -0.6046776061558807314, 0.2411417322834647770 ) ) ;
#3385=CARTESIAN_POINT ( 'NONE',  ( 1.371391076115485941, 0.2952755905511811885, 0.1292274648535926551 ) ) ;
#3386=CARTESIAN_POINT ( 'NONE',  ( 0.8005249343832028242, -0.4281496062992127816, -0.4176697321401328100 ) ) ;
#3389=CARTESIAN_POINT ( 'NONE',  ( 1.568241469816273437, -0.2845877964562159024, 0.3641732283464567677 ) ) ;
#3392=EDGE_CURVE ( 'NONE', #82899, #20923, #18685, .T. ) ;
#3393=CARTESIAN_POINT ( 'NONE',  ( -0.6758530183727028406, 0.1771653543307087630, 0.09757992244046791164 ) ) ;
#3395=ORIENTED_EDGE ( 'NONE', *, *, #75224, .F. ) ;
#3396=CARTESIAN_POINT ( 'NONE',  ( 1.030183727034121421, -0.3162353388693409650, -0.4822834645669289433 ) ) ;
#3397=CARTESIAN_POINT ( 'NONE',  ( -0.2755905511811018171, 0.2952755905511811885, 0.000000000000000000 ) ) ;
#3398=CARTESIAN_POINT ( 'NONE',  ( -1.220472440944881054, -0.6692913385826771977, 8.415575281601705876E-17 ) ) ;
#3399=CARTESIAN_POINT ( 'NONE',  ( 1.417322834645670104, -0.1870078740157480879, -0.4822834645669291653 ) ) ;
#3400=CARTESIAN_POINT ( 'NONE',  ( -1.161417322834644716, 0.07958543189024085140, 0.2665933059059887866 ) ) ;
#3401=CARTESIAN_POINT ( 'NONE',  ( 0.4996603843015406943, 1.493546695279807990, -0.5309055118110237448 ) ) ;
#3402=CARTESIAN_POINT ( 'NONE',  ( 0.3608923884514443348, -0.6692913385826771977, 0.1292274648535927661 ) ) ;
#3403=CARTESIAN_POINT ( 'NONE',  ( -0.6824146981627288167, 0.2306618581243848609, 0.2411417322834645549 ) ) ;
#3405=CARTESIAN_POINT ( 'NONE',  ( -1.417322834645668772, -0.1870078740157480879, -0.4822834645669291653 ) ) ;
#3407=EDGE_CURVE ( 'NONE', #58566, #35196, #5274, .T. ) ;
#3408=CARTESIAN_POINT ( 'NONE',  ( 0.9055118110236227702, 0.2952755905511811885, 0.000000000000000000 ) ) ;
#3409=CARTESIAN_POINT ( 'NONE',  ( 1.364829396325460076, 0.1283753931104748280, 0.1820866141732283561 ) ) ;
#3410=ORIENTED_EDGE ( 'NONE', *, *, #52110, .F. ) ;
#3412=CARTESIAN_POINT ( 'NONE',  ( -0.3608923884514428360, 0.2952755905511811885, 0.1292274648535926551 ) ) ;
#3413=EDGE_LOOP ( 'NONE', ( #79310, #76893, #82001, #45320 ) ) ;
#3414=CARTESIAN_POINT ( 'NONE',  ( 0.4527559055118117182, -0.4536011799217367080, 0.2665933059059888421 ) ) ;
#3415=CARTESIAN_POINT ( 'NONE',  ( -1.581364829396324945, -0.3162353388693405765, 0.4822834645669290543 ) ) ;
#3416=CARTESIAN_POINT ( 'NONE',  ( 0.9317585301837276734, -0.4281496062992124485, 0.4176697321401328655 ) ) ;
#3417=CARTESIAN_POINT ( 'NONE',  ( 0.8464566929133865436, 0.1660481256975883668, -0.3530559997133364547 ) ) ;
#3418=CARTESIAN_POINT ( 'NONE',  ( -0.1574803149606292529, -0.1870078740157479769, 0.4822834645669291653 ) ) ;
#3420=CARTESIAN_POINT ( 'NONE',  ( -0.6692913385826764205, 0.2952755905511811885, 0.000000000000000000 ) ) ;
#3422=CARTESIAN_POINT ( 'NONE',  ( -1.686351706036744558, 0.2952755905511810774, -0.1292274648535930714 ) ) ;
#3423=CARTESIAN_POINT ( 'NONE',  ( -1.043307086614172041, -0.5400638737290844871, 0.3530559997133364547 ) ) ;
#3424=CARTESIAN_POINT ( 'NONE',  ( 1.154855643044620184, -0.6046776061558807314, 0.2411417322834647770 ) ) ;
#3425=CARTESIAN_POINT ( 'NONE',  ( 1.469816272965879911, -0.6046776061558807314, 0.2411417322834647770 ) ) ;
#3426=CARTESIAN_POINT ( 'NONE',  ( -1.043307086614172707, 0.1660481256975883668, -0.3530559997133364547 ) ) ;
#3428=CARTESIAN_POINT ( 'NONE',  ( 0.1771653543307093182, 0.1660481256975885056, 0.3530559997133364547 ) ) ;
#3430=CARTESIAN_POINT ( 'NONE',  ( -0.7414698162729651543, -0.6692913385826771977, 0.1292274648535927661 ) ) ;
#3431=VECTOR ( 'NONE', #51039, 39.37007874015748143 ) ;
#3432=CARTESIAN_POINT ( 'NONE',  ( 1.587926509186352586, -0.4281496062992127816, -0.4176697321401328100 ) ) ;
#3433=CARTESIAN_POINT ( 'NONE',  ( 0.5511811023622055217, -0.1870078740157479769, 0.3641732283464567677 ) ) ;
#3434=CARTESIAN_POINT ( 'NONE',  ( 1.423884514435696191, -0.05778040916215522460, 0.4822834645669289988 ) ) ;
#3436=CARTESIAN_POINT ( 'NONE',  ( 1.371391076115485941, 0.1771653543307087630, 0.09757992244046791164 ) ) ;
#3437=CARTESIAN_POINT ( 'NONE',  ( 0.8070866141732288002, 0.1660481256975885056, 0.3530559997133364547 ) ) ;
#3439=CARTESIAN_POINT ( 'NONE',  ( -0.5380577427821514602, -0.4281496062992127816, -0.4176697321401328100 ) ) ;
#3440=CARTESIAN_POINT ( 'NONE',  ( 1.586052503253845281, 1.299212598425198095, 0.1653254495020587411 ) ) ;
#3441=CARTESIAN_POINT ( 'NONE',  ( 1.259842519685040019, -0.1870078740157479769, 0.3641732283464567677 ) ) ;
#3442=CARTESIAN_POINT ( 'NONE',  ( -0.6561679790026240244, -0.6046776061558807314, 0.2411417322834647770 ) ) ;
#3444=CARTESIAN_POINT ( 'NONE',  ( 1.423884514435696413, -0.3162353388693409650, -0.4822834645669289433 ) ) ;
#3445=CARTESIAN_POINT ( 'NONE',  ( 0.09186351706036799403, -0.4281496062992127816, -0.4176697321401328100 ) ) ;
#3446=CARTESIAN_POINT ( 'NONE',  ( 0.5118110236220480003, -0.5511811023622047445, 6.969142054262312111E-17 ) ) ;
#3448=CARTESIAN_POINT ( 'NONE',  ( -0.1049868766404193215, -0.5023911411419708095, 0.1820866141732285504 ) ) ;
#3449=CARTESIAN_POINT ( 'NONE',  ( -1.522309711286088607, -0.6046776061558807314, 0.2411417322834647770 ) ) ;
#3451=CARTESIAN_POINT ( 'NONE',  ( 0.8267716535433078384, -0.6692913385826771977, 8.415575281601705876E-17 ) ) ;
#3453=CARTESIAN_POINT ( 'NONE',  ( 1.653543307086614789, -0.1870078740157479769, 0.3641732283464567677 ) ) ;
#3456=CARTESIAN_POINT ( 'NONE',  ( -0.1377952755905504645, 0.07958543189024085140, 0.2665933059059887866 ) ) ;
#3457=EDGE_CURVE ( 'NONE', #61268, #4549, #29861, .T. ) ;
#3458=CARTESIAN_POINT ( 'NONE',  ( 0.2755905511811031494, 0.2952755905511811885, 0.000000000000000000 ) ) ;
#3459=CARTESIAN_POINT ( 'NONE',  ( 1.332020997375329197, -0.2845877964562159024, 0.3641732283464567677 ) ) ;
#3460=CARTESIAN_POINT ( 'NONE',  ( -1.312335958005248715, -0.5023911411419708095, -0.1820866141732282451 ) ) ;
#3461=CARTESIAN_POINT ( 'NONE',  ( -1.627296587926508442, -0.6046776061558809534, -0.2411417322834644161 ) ) ;
#3462=CARTESIAN_POINT ( 'NONE',  ( 0.4199475065616805614, 0.2306618581243848609, 0.2411417322834645549 ) ) ;
#3463=CARTESIAN_POINT ( 'NONE',  ( 1.332020997375329197, -0.3162353388693405765, 0.4822834645669290543 ) ) ;
#3465=CARTESIAN_POINT ( 'NONE',  ( 0.06561679790026316017, 0.05413385826771626580, -0.4176697321401330321 ) ) ;
#3466=CARTESIAN_POINT ( 'NONE',  ( 1.299212598425197429, -0.6692913385826771977, 8.415575281601705876E-17 ) ) ;
#3467=CARTESIAN_POINT ( 'NONE',  ( 1.115485564304462551, -0.4281496062992127816, -0.4176697321401328100 ) ) ;
#3469=CARTESIAN_POINT ( 'NONE',  ( 0.7020997375328090762, -0.2845877964562159024, 0.3641732283464567677 ) ) ;
#3470=CARTESIAN_POINT ( 'NONE',  ( 1.561679790026247350, 0.05413385826771626580, -0.4176697321401330321 ) ) ;
#3471=CARTESIAN_POINT ( 'NONE',  ( 0.3477690288713918276, 0.1771653543307087630, 0.09757992244046791164 ) ) ;
#3472=CARTESIAN_POINT ( 'NONE',  ( 0.3018372703412079971, 0.05413385826771626580, -0.4176697321401330321 ) ) ;
#3473=CARTESIAN_POINT ( 'NONE',  ( 0.5577427821522314977, -0.3162353388693409650, -0.4822834645669289433 ) ) ;
#3474=CARTESIAN_POINT ( 'NONE',  ( -0.3477690288713902178, 0.2952755905511810774, -0.1292274648535930714 ) ) ;
#3475=CARTESIAN_POINT ( 'NONE',  ( 0.1968503937007881344, 0.1771653543307087630, 0.000000000000000000 ) ) ;
#3476=CARTESIAN_POINT ( 'NONE',  ( 0.9973753280839902091, 0.2306618581243847221, -0.2411417322834647770 ) ) ;
#3478=CARTESIAN_POINT ( 'NONE',  ( -1.135170603674539924, -0.6692913385826771977, 0.1292274648535927661 ) ) ;
#3482=CARTESIAN_POINT ( 'NONE',  ( -1.082677165354329896, -0.5400638737290845981, -0.3530559997133363437 ) ) ;
#3483=VECTOR ( 'NONE', #32080, 39.37007874015748143 ) ;
#3484=CARTESIAN_POINT ( 'NONE',  ( -0.4593175853018366950, 0.05413385826771666132, 0.4176697321401328100 ) ) ;
#3487=VERTEX_POINT ( 'NONE', #30766 ) ;
#3488=CARTESIAN_POINT ( 'NONE',  ( 0.9317585301837276734, -0.004921259842519870586, -0.3153832671262229437 ) ) ;
#3490=CARTESIAN_POINT ( 'NONE',  ( 1.161417322834646271, 0.1660481256975883668, -0.3530559997133364547 ) ) ;
#3492=CARTESIAN_POINT ( 'NONE',  ( 0.4606732211678790101, 2.401574803149606030, 0.5309055118110234117 ) ) ;
#3493=CARTESIAN_POINT ( 'NONE',  ( -1.555118110236219930, 0.07958543189024085140, 0.2665933059059887866 ) ) ;
#3494=CARTESIAN_POINT ( 'NONE',  ( 1.430446194225722500, -0.4281496062992127816, -0.4176697321401328100 ) ) ;
#3495=CARTESIAN_POINT ( 'NONE',  ( 1.305774278215223960, 0.1771653543307087075, -0.09757992244046823083 ) ) ;
#3496=CARTESIAN_POINT ( 'NONE',  ( 0.5380577427821529035, -0.4281496062992124485, 0.4176697321401328655 ) ) ;
#3498=CARTESIAN_POINT ( 'NONE',  ( -0.08530183727034056085, -0.3162353388693405765, 0.4822834645669290543 ) ) ;
#3499=CARTESIAN_POINT ( 'NONE',  ( -0.8333333333333323711, -0.5511811023622048555, -0.09757992244046775898 ) ) ;
#3500=CARTESIAN_POINT ( 'NONE',  ( 0.8727034120734912248, -0.3162353388693409650, -0.4822834645669289433 ) ) ;
#3501=CARTESIAN_POINT ( 'NONE',  ( -0.2165354330708654795, -0.5400638737290845981, -0.3530559997133363437 ) ) ;
#3502=CARTESIAN_POINT ( 'NONE',  ( 0.5183727034120741983, 0.2952755905511810219, -0.1292274648535930437 ) ) ;
#3505=CARTESIAN_POINT ( 'NONE',  ( 0.8792650918635177559, 0.05413385826771666132, 0.4176697321401328100 ) ) ;
#3506=CARTESIAN_POINT ( 'NONE',  ( 0.09842519685039434474, -0.5400638737290845981, -0.3530559997133363437 ) ) ;
#3507=CARTESIAN_POINT ( 'NONE',  ( -1.115485564304461219, 0.05413385826771626580, -0.4176697321401330321 ) ) ;
#3508=CARTESIAN_POINT ( 'NONE',  ( 0.9842519685039375910, 0.2952755905511811885, 0.000000000000000000 ) ) ;
#3509=CARTESIAN_POINT ( 'NONE',  ( 0.5774278215223104249, 0.2306618581243848609, 0.2411417322834645549 ) ) ;
#3511=CARTESIAN_POINT ( 'NONE',  ( -0.2427821522309703550, -0.05778040916215560624, -0.4822834645669293319 ) ) ;
#3512=CARTESIAN_POINT ( 'NONE',  ( 0.5774278215223104249, 0.2306618581243848609, 0.2411417322834645549 ) ) ;
#3513=CARTESIAN_POINT ( 'NONE',  ( -0.1312335958005241554, -0.6046776061558809534, -0.2411417322834644161 ) ) ;
#3514=CARTESIAN_POINT ( 'NONE',  ( 0.6102362204724416372, 0.07958543189024071263, -0.2665933059059888421 ) ) ;
#3515=CARTESIAN_POINT ( 'NONE',  ( -2.787279214012418738, 0.000000000000000000, 0.000000000000000000 ) ) ;
#3516=CARTESIAN_POINT ( 'NONE',  ( -1.653543307086613234, -0.1870078740157480879, -0.4822834645669291653 ) ) ;
#3517=CARTESIAN_POINT ( 'NONE',  ( 0.1443569553805781891, -0.4281496062992124485, 0.4176697321401328655 ) ) ;
#3520=ORIENTED_EDGE ( 'NONE', *, *, #72820, .F. ) ;
#3521=ORIENTED_EDGE ( 'NONE', *, *, #17984, .T. ) ;
#3523=CARTESIAN_POINT ( 'NONE',  ( 0.6627296587926517768, -0.6692913385826773087, -0.1292274648535924053 ) ) ;
#3524=CARTESIAN_POINT ( 'NONE',  ( 0.4593175853018379162, -0.3690944881889763329, 0.3153832671262228327 ) ) ;
#3528=DIRECTION ( 'NONE',  ( 3.096699300667737957E-16, -1.000000000000000000, 0.000000000000000000 ) ) ;
#3534=CARTESIAN_POINT ( 'NONE',  ( 0.8727034120734912248, -0.3162353388693409650, -0.4822834645669289433 ) ) ;
#3535=CARTESIAN_POINT ( 'NONE',  ( -0.6364829396325453192, -0.05778040916215560624, -0.4822834645669293319 ) ) ;
#3536=CARTESIAN_POINT ( 'NONE',  ( -0.8005249343832013809, -0.4281496062992124485, 0.4176697321401328655 ) ) ;
#3537=CARTESIAN_POINT ( 'NONE',  ( 0.5971128608923890191, -0.6692913385826771977, 0.1292274648535927661 ) ) ;
#3538=CARTESIAN_POINT ( 'NONE',  ( 1.220472440944882386, -0.6692913385826771977, 8.415575281601705876E-17 ) ) ;
#3539=CARTESIAN_POINT ( 'NONE',  ( 1.633858267716535639, -0.4536011799217367080, 0.2665933059059888421 ) ) ;
#3541=CARTESIAN_POINT ( 'NONE',  ( 1.069553805774278832, 0.1771653543307087075, -0.09757992244046823083 ) ) ;
#3543=CARTESIAN_POINT ( 'NONE',  ( -1.430446194225720724, -0.004921259842519870586, -0.3153832671262229437 ) ) ;
#3545=CARTESIAN_POINT ( 'NONE',  ( 0.08530183727034192087, -0.05778040916215522460, 0.4822834645669289988 ) ) ;
#3547=CARTESIAN_POINT ( 'NONE',  ( 1.614173228346457378, -0.6692913385826771977, 8.415575281601705876E-17 ) ) ;
#3548=CARTESIAN_POINT ( 'NONE',  ( -1.603475055217291612, 1.543447618314657932, 0.04573490813648255215 ) ) ;
#3549=CARTESIAN_POINT ( 'NONE',  ( -1.213910761154854745, 0.1771653543307087075, -0.09757992244046823083 ) ) ;
#3550=CARTESIAN_POINT ( 'NONE',  ( 0.5380577427821529035, -0.4281496062992124485, 0.4176697321401328655 ) ) ;
#3551=CARTESIAN_POINT ( 'NONE',  ( 1.384514435695538337, -0.5511811023622046335, 0.09757992244046803654 ) ) ;
#3554=CARTESIAN_POINT ( 'NONE',  ( -1.286089238845143479, -0.5023911411419708095, 0.1820866141732285504 ) ) ;
#3555=CARTESIAN_POINT ( 'NONE',  ( 1.213910761154856299, 0.2952755905511811885, 0.1292274648535926551 ) ) ;
#3557=CARTESIAN_POINT ( 'NONE',  ( -0.1049868766404193215, 0.2306618581243847221, -0.2411417322834647770 ) ) ;
#3558=CARTESIAN_POINT ( 'NONE',  ( -1.410761154855641575, -0.2845877964562161244, -0.3641732283464567121 ) ) ;
#3559=CARTESIAN_POINT ( 'NONE',  ( -0.5314960629921254842, -0.5400638737290845981, -0.3530559997133363437 ) ) ;
#3560=CARTESIAN_POINT ( 'NONE',  ( -1.640419947506561060, -0.004921259842519576551, 0.3153832671262227771 ) ) ;
#3562=CARTESIAN_POINT ( 'NONE',  ( 0.4199475065616803948, -0.6046776061558809534, -0.2411417322834644161 ) ) ;
#3563=CARTESIAN_POINT ( 'NONE',  ( 1.443569553805774897, 0.2306618581243848609, 0.2411417322834645549 ) ) ;
#3565=CARTESIAN_POINT ( 'NONE',  ( -1.240157480314959759, 0.1660481256975885056, 0.3530559997133364547 ) ) ;
#3566=CARTESIAN_POINT ( 'NONE',  ( -0.6496062992125976043, -0.4536011799217367080, 0.2665933059059888421 ) ) ;
#3567=CARTESIAN_POINT ( 'NONE',  ( -1.627296587926508442, 0.2306618581243848609, 0.2411417322834645549 ) ) ;
#3568=CARTESIAN_POINT ( 'NONE',  ( 0.1049868766404206816, 0.2306618581243848609, 0.2411417322834645549 ) ) ;
#3569=CARTESIAN_POINT ( 'NONE',  ( 0.2296587926509192634, -0.2845877964562159024, 0.3641732283464567677 ) ) ;
#3570=CARTESIAN_POINT ( 'NONE',  ( -1.194225721784776262, -0.004921259842519870586, -0.3153832671262229437 ) ) ;
#3571=CARTESIAN_POINT ( 'NONE',  ( -1.594488188976377563, -0.5400638737290844871, 0.3530559997133364547 ) ) ;
#3572=CARTESIAN_POINT ( 'NONE',  ( -1.568241469816272105, -0.05778040916215522460, 0.4822834645669289988 ) ) ;
#3573=CARTESIAN_POINT ( 'NONE',  ( 1.463254593175853824, -0.6692913385826771977, 0.1292274648535927661 ) ) ;
#3575=CARTESIAN_POINT ( 'NONE',  ( 0.4265091863517067594, 0.1771653543307087630, 0.09757992244046791164 ) ) ;
#3576=CARTESIAN_POINT ( 'NONE',  ( 1.030183727034121421, -0.05778040916215522460, 0.4822834645669289988 ) ) ;
#3577=CARTESIAN_POINT ( 'NONE',  ( -1.595398199321657051, 0.7375059713363285585, 0.1559797534342473035 ) ) ;
#3578=CARTESIAN_POINT ( 'NONE',  ( 1.325459317585302665, -0.004921259842519870586, -0.3153832671262229437 ) ) ;
#3580=CARTESIAN_POINT ( 'NONE',  ( -1.036745406824146176, -0.4281496062992124485, 0.4176697321401328655 ) ) ;
#3581=CARTESIAN_POINT ( 'NONE',  ( -0.8858267716535425107, -0.5400638737290844871, 0.3530559997133364547 ) ) ;
#3582=CARTESIAN_POINT ( 'NONE',  ( 0.3083989501312343062, -0.3162353388693405765, 0.4822834645669290543 ) ) ;
#3584=CARTESIAN_POINT ( 'NONE',  ( 0.5411721830064198935, 8.471767977567108961E-16, -0.4445507791589058955 ) ) ;
#3586=CARTESIAN_POINT ( 'NONE',  ( 1.023622047244095112, -0.1870078740157480879, -0.4822834645669291653 ) ) ;
#3587=CARTESIAN_POINT ( 'NONE',  ( 1.476377952755906220, 0.07958543189024071263, -0.2665933059059888421 ) ) ;
#3588=VECTOR ( 'NONE', #70655, 39.37007874015748143 ) ;
#3589=CARTESIAN_POINT ( 'NONE',  ( 0.3412073490813655186, -0.6046776061558809534, -0.2411417322834644161 ) ) ;
#3590=CARTESIAN_POINT ( 'NONE',  ( 0.6430446194225728496, 0.05413385826771666132, 0.4176697321401328100 ) ) ;
#3596=CARTESIAN_POINT ( 'NONE',  ( -0.2230971128608915943, -0.3690944881889765550, -0.3153832671262227771 ) ) ;
#3597=CARTESIAN_POINT ( 'NONE',  ( -0.1574803149606292529, -0.1870078740157479769, 0.4822834645669291653 ) ) ;
#3598=CARTESIAN_POINT ( 'NONE',  ( 0.7349081364829402885, -0.6046776061558809534, -0.2411417322834644161 ) ) ;
#3600=CARTESIAN_POINT ( 'NONE',  ( -0.1968503937007867743, 0.1771653543307087630, 0.000000000000000000 ) ) ;
#3601=CARTESIAN_POINT ( 'NONE',  ( -1.010498687664041384, 0.05413385826771666132, 0.4176697321401328100 ) ) ;
#3602=CARTESIAN_POINT ( 'NONE',  ( 1.056430446194226436, -0.6692913385826773087, -0.1292274648535924053 ) ) ;
#3605=CARTESIAN_POINT ( 'NONE',  ( 0.5387615594602676028, 2.409604939980833412E-17, -0.3464511005275205946 ) ) ;
#3606=VERTEX_POINT ( 'NONE', #31166 ) ;
#3607=CARTESIAN_POINT ( 'NONE',  ( 0.9908136482939640111, 0.2952755905511810774, -0.1292274648535930714 ) ) ;
#3608=CARTESIAN_POINT ( 'NONE',  ( 1.299212598425197429, 0.1771653543307087630, 0.000000000000000000 ) ) ;
#3609=CARTESIAN_POINT ( 'NONE',  ( -1.443569553805773564, 0.1283753931104746893, -0.1820866141732285504 ) ) ;
#3610=CARTESIAN_POINT ( 'NONE',  ( -1.482939632545930975, 0.05413385826771666132, 0.4176697321401328100 ) ) ;
#3612=CARTESIAN_POINT ( 'NONE',  ( 1.193035393573956160, 6.860680731889873434E-16, 0.3627989612356145033 ) ) ;
#3613=CARTESIAN_POINT ( 'NONE',  ( 1.122047244094488860, -0.5400638737290845981, -0.3530559997133363437 ) ) ;
#3614=CARTESIAN_POINT ( 'NONE',  ( -1.640419947506561060, -0.4281496062992127816, -0.4176697321401328100 ) ) ;
#3615=CARTESIAN_POINT ( 'NONE',  ( -0.006561679790025524116, -0.3162353388693405765, 0.4822834645669290543 ) ) ;
#3616=CARTESIAN_POINT ( 'NONE',  ( -0.6496062992125976043, -0.5400638737290844871, 0.3530559997133364547 ) ) ;
#3617=CARTESIAN_POINT ( 'NONE',  ( 1.509186351706037543, -0.4281496062992127816, -0.4176697321401328100 ) ) ;
#3619=CARTESIAN_POINT ( 'NONE',  ( 0.3346456692913390985, 0.1660481256975885056, 0.3530559997133364547 ) ) ;
#3621=CARTESIAN_POINT ( 'NONE',  ( -1.489501312335957062, -0.08942795157527998196, 0.3641732283464567121 ) ) ;
#3626=CARTESIAN_POINT ( 'NONE',  ( -1.719160104986876103, 0.05413385826771666132, 0.4176697321401328100 ) ) ;
#3628=CARTESIAN_POINT ( 'NONE',  ( 1.436417322834643961, 0.4405861044731111953, 0.3149606299212599492 ) ) ;
#3630=CARTESIAN_POINT ( 'NONE',  ( -1.010498687664041384, 0.05413385826771666132, 0.4176697321401328100 ) ) ;
#3633=CARTESIAN_POINT ( 'NONE',  ( -0.1837270341207340729, 0.1283753931104746893, -0.1820866141732285504 ) ) ;
#3634=CARTESIAN_POINT ( 'NONE',  ( -1.069553805774277722, 0.1771653543307087630, 0.09757992244046791164 ) ) ;
#3635=CARTESIAN_POINT ( 'NONE',  ( -1.404199475065615932, -0.4281496062992127816, -0.4176697321401328100 ) ) ;
#3636=CARTESIAN_POINT ( 'NONE',  ( 0.4593175853018379162, -0.4281496062992124485, 0.4176697321401328655 ) ) ;
#3637=CARTESIAN_POINT ( 'NONE',  ( -1.266404199475064773, -0.05778040916215560624, -0.4822834645669293319 ) ) ;
#3639=ORIENTED_EDGE ( 'NONE', *, *, #62545, .F. ) ;
#3640=CARTESIAN_POINT ( 'NONE',  ( -1.207349081364828436, -0.6046776061558807314, 0.2411417322834647770 ) ) ;
#3641=LINE ( 'NONE', #41930, #8427 ) ;
#3646=ADVANCED_FACE ( 'NONE', ( #63166 ), #27286, .F. ) ;
#3649=LINE ( 'NONE', #62124, #47966 ) ;
#3650=CARTESIAN_POINT ( 'NONE',  ( -0.9186351706036736120, -0.6046776061558809534, -0.2411417322834644161 ) ) ;
#3651=CARTESIAN_POINT ( 'NONE',  ( 1.377952755905512472, 0.2952755905511811885, 0.000000000000000000 ) ) ;
#3656=CARTESIAN_POINT ( 'NONE',  ( 1.515748031496063408, 0.1660481256975885056, 0.3530559997133364547 ) ) ;
#3657=CARTESIAN_POINT ( 'NONE',  ( -0.8398950131233589023, -0.6046776061558809534, -0.2411417322834644161 ) ) ;
#3659=CARTESIAN_POINT ( 'NONE',  ( 0.2165354330708668673, 0.07958543189024071263, -0.2665933059059888421 ) ) ;
#3661=CARTESIAN_POINT ( 'NONE',  ( 0.03280839895013198948, -0.5511811023622048555, -0.09757992244046775898 ) ) ;
#3662=CARTESIAN_POINT ( 'NONE',  ( 0.8398950131233602345, 0.1283753931104746893, -0.1820866141732285504 ) ) ;
#3663=CARTESIAN_POINT ( 'NONE',  ( 0.7480314960629927956, -0.6692913385826771977, 8.415575281601705876E-17 ) ) ;
#3664=CARTESIAN_POINT ( 'NONE',  ( -0.3805774278215216522, -0.004921259842519576551, 0.3153832671262227771 ) ) ;
#3666=CARTESIAN_POINT ( 'NONE',  ( -1.555118110236219930, -0.5400638737290845981, -0.3530559997133363437 ) ) ;
#3667=CARTESIAN_POINT ( 'NONE',  ( -1.174540682414697335, -0.08942795157527998196, 0.3641732283464567121 ) ) ;
#3669=CARTESIAN_POINT ( 'NONE',  ( 0.1115485564304467270, -0.6692913385826773087, -0.1292274648535924053 ) ) ;
#3670=CARTESIAN_POINT ( 'NONE',  ( -0.5643044619422565855, -0.4281496062992124485, 0.4176697321401328655 ) ) ;
#3672=CARTESIAN_POINT ( 'NONE',  ( 0.4527559055118117182, -0.4536011799217367080, 0.2665933059059888421 ) ) ;
#3673=CARTESIAN_POINT ( 'NONE',  ( -0.2952755905511804668, 0.1660481256975885056, 0.3530559997133364547 ) ) ;
#3674=CARTESIAN_POINT ( 'NONE',  ( -0.7677165354330699465, -0.5400638737290845981, -0.3530559997133363437 ) ) ;
#3675=CARTESIAN_POINT ( 'NONE',  ( -1.604771003085129433, 2.146987379487327985, 0.1466069496707750608 ) ) ;
#3677=CARTESIAN_POINT ( 'NONE',  ( 0.06561679790026316017, -0.4281496062992124485, 0.4176697321401328655 ) ) ;
#3679=DIRECTION ( 'NONE',  ( -0.000000000000000000, 1.000000000000000000, -0.000000000000000000 ) ) ;
#3680=CARTESIAN_POINT ( 'NONE',  ( -0.05905511811023545637, -0.4536011799217368745, -0.2665933059059886201 ) ) ;
#3681=CARTESIAN_POINT ( 'NONE',  ( -0.3937007874015740483, -0.1870078740157480879, -0.4822834645669291653 ) ) ;
#3682=CARTESIAN_POINT ( 'NONE',  ( -1.594488188976377119, 0.07958543189024071263, -0.2665933059059888421 ) ) ;
#3683=CARTESIAN_POINT ( 'NONE',  ( 1.154855643044620184, -0.6046776061558807314, 0.2411417322834647770 ) ) ;
#3684=CARTESIAN_POINT ( 'NONE',  ( -1.469816272965878357, 0.2306618581243848609, 0.2411417322834645549 ) ) ;
#3685=CARTESIAN_POINT ( 'NONE',  ( -0.8267716535433065062, -0.5511811023622047445, 6.969142054262312111E-17 ) ) ;
#3689=CARTESIAN_POINT ( 'NONE',  ( 1.673228346456693494, 0.07958543189024085140, 0.2665933059059887866 ) ) ;
#3690=CARTESIAN_POINT ( 'NONE',  ( 1.181102362204724976, -0.1870078740157480601, -0.3641732283464567677 ) ) ;
#3691=CARTESIAN_POINT ( 'NONE',  ( 0.9776902887139113929, 0.2952755905511811885, 0.1292274648535926551 ) ) ;
#3692=CARTESIAN_POINT ( 'NONE',  ( -1.541994750656167090, 0.2952755905511811885, 0.1292274648535926551 ) ) ;
#3693=CARTESIAN_POINT ( 'NONE',  ( 0.7545931758530188826, -0.6692913385826771977, 0.1292274648535927661 ) ) ;
#3695=CARTESIAN_POINT ( 'NONE',  ( 1.181102362204725198, -0.1870078740157479769, 0.3641732283464567677 ) ) ;
#3696=CARTESIAN_POINT ( 'NONE',  ( -0.01968503937007793844, 0.1660481256975883668, -0.3530559997133364547 ) ) ;
#3697=CARTESIAN_POINT ( 'NONE',  ( -0.7611548556430438595, -0.6046776061558809534, -0.2411417322834644161 ) ) ;
#3699=VECTOR ( 'NONE', #46610, 39.37007874015748143 ) ;
#3703=CARTESIAN_POINT ( 'NONE',  ( 0.3215223097112867578, -0.08942795157527998196, 0.3641732283464567121 ) ) ;
#3704=ORIENTED_EDGE ( 'NONE', *, *, #54370, .F. ) ;
#3706=VERTEX_POINT ( 'NONE', #49014 ) ;
#3707=CARTESIAN_POINT ( 'NONE',  ( -0.5577427821522301654, -0.05778040916215560624, -0.4822834645669293319 ) ) ;
#3708=CARTESIAN_POINT ( 'NONE',  ( -0.1706036745406816491, 0.05413385826771626580, -0.4176697321401330321 ) ) ;
#3709=CARTESIAN_POINT ( 'NONE',  ( -0.1640419947506553400, -0.05778040916215560624, -0.4822834645669293319 ) ) ;
#3710=CARTESIAN_POINT ( 'NONE',  ( 0.8005249343832028242, -0.4281496062992127816, -0.4176697321401328100 ) ) ;
#3711=CARTESIAN_POINT ( 'NONE',  ( -0.8595800524934373854, -0.05778040916215522460, 0.4822834645669289988 ) ) ;
#3712=CARTESIAN_POINT ( 'NONE',  ( -0.4855643044619415427, -0.4281496062992124485, 0.4176697321401328655 ) ) ;
#3713=CARTESIAN_POINT ( 'NONE',  ( 1.279527559055118724, 0.1660481256975885056, 0.3530559997133364547 ) ) ;
#3714=CARTESIAN_POINT ( 'NONE',  ( 0.3346456692913390985, 0.1660481256975885056, 0.3530559997133364547 ) ) ;
#3715=CARTESIAN_POINT ( 'NONE',  ( 0.6561679790026253567, -0.6046776061558809534, -0.2411417322834644161 ) ) ;
#3717=CARTESIAN_POINT ( 'NONE',  ( 0.1049868766404206816, 0.1283753931104748280, 0.1820866141732283561 ) ) ;
#3718=ORIENTED_EDGE ( 'NONE', *, *, #15170, .T. ) ;
#3721=CARTESIAN_POINT ( 'NONE',  ( -0.8070866141732276899, -0.4536011799217367080, 0.2665933059059888421 ) ) ;
#3722=CARTESIAN_POINT ( 'NONE',  ( -0.4002624671916004129, -0.3162353388693405765, 0.4822834645669290543 ) ) ;
#3723=CARTESIAN_POINT ( 'NONE',  ( 0.7767023820430452030, 2.575861430505332611E-15, -0.4118477457932988584 ) ) ;
#3724=CARTESIAN_POINT ( 'NONE',  ( -0.5511811023622041894, -0.1870078740157480879, -0.4822834645669291653 ) ) ;
#3725=CARTESIAN_POINT ( 'NONE',  ( -0.2427821522309703550, -0.05778040916215560624, -0.4822834645669293319 ) ) ;
#3726=CARTESIAN_POINT ( 'NONE',  ( -1.246719160104985846, -0.4281496062992127816, -0.4176697321401328100 ) ) ;
#3727=CARTESIAN_POINT ( 'NONE',  ( -1.541994750656167090, 0.2952755905511811885, 0.1292274648535926551 ) ) ;
#3728=CARTESIAN_POINT ( 'NONE',  ( 1.076115485564305141, 0.1283753931104746893, -0.1820866141732285504 ) ) ;
#3731=CARTESIAN_POINT ( 'NONE',  ( 0.6233595800524939223, -0.2845877964562159024, 0.3641732283464567677 ) ) ;
#3732=CARTESIAN_POINT ( 'NONE',  ( 0.1115485564304470323, 0.2952755905511811885, 0.1292274648535926551 ) ) ;
#3733=CARTESIAN_POINT ( 'NONE',  ( -0.2230971128608915943, 0.05413385826771666132, 0.4176697321401328100 ) ) ;
#3734=ORIENTED_EDGE ( 'NONE', *, *, #76855, .F. ) ;
#3740=CARTESIAN_POINT ( 'NONE',  ( -0.6496062992125976043, -0.4536011799217367080, 0.2665933059059888421 ) ) ;
#3741=CARTESIAN_POINT ( 'NONE',  ( -0.7742782152230965886, 0.05413385826771666132, 0.4176697321401328100 ) ) ;
#3744=CARTESIAN_POINT ( 'NONE',  ( 1.620734908136483465, -0.6692913385826771977, 0.1292274648535927661 ) ) ;
#3745=CARTESIAN_POINT ( 'NONE',  ( 0.4921259842519691285, 0.1660481256975885056, 0.3530559997133364547 ) ) ;
#3746=CARTESIAN_POINT ( 'NONE',  ( 0.5511811023622055217, -0.1870078740157479769, 0.4822834645669291653 ) ) ;
#3747=CARTESIAN_POINT ( 'NONE',  ( -0.7480314960629914633, -0.5511811023622047445, 6.969142054262312111E-17 ) ) ;
#3748=CARTESIAN_POINT ( 'NONE',  ( 0.2690288713910767848, -0.6692913385826773087, -0.1292274648535924053 ) ) ;
#3750=CARTESIAN_POINT ( 'NONE',  ( -0.6167979002624665030, 0.05413385826771666132, 0.4176697321401328100 ) ) ;
#3752=CARTESIAN_POINT ( 'NONE',  ( 1.272965879265092637, -0.004921259842519576551, 0.3153832671262227771 ) ) ;
#3753=CARTESIAN_POINT ( 'NONE',  ( 0.1902887139107617975, 0.1771653543307087630, 0.09757992244046791164 ) ) ;
#3754=CARTESIAN_POINT ( 'NONE',  ( 1.233595800524935227, 0.1283753931104746893, -0.1820866141732285504 ) ) ;
#3755=CARTESIAN_POINT ( 'NONE',  ( -0.9580052493438311334, -0.4281496062992124485, 0.4176697321401328655 ) ) ;
#3756=CARTESIAN_POINT ( 'NONE',  ( -0.5249343832020990641, 0.1283753931104748280, 0.1820866141732283561 ) ) ;
#3758=CARTESIAN_POINT ( 'NONE',  ( -1.174540682414697335, -0.3162353388693409650, -0.4822834645669289433 ) ) ;
#3759=CARTESIAN_POINT ( 'NONE',  ( -0.6167979002624665030, -0.4281496062992127816, -0.4176697321401328100 ) ) ;
#3760=CARTESIAN_POINT ( 'NONE',  ( 0.1837270341207357105, -0.6046776061558809534, -0.2411417322834644161 ) ) ;
#3764=CARTESIAN_POINT ( 'NONE',  ( 0.3674540682414705883, -0.5023911411419708095, 0.1820866141732285504 ) ) ;
#3765=CARTESIAN_POINT ( 'NONE',  ( 1.036745406824147508, -0.4281496062992127816, -0.4176697321401328100 ) ) ;
#3767=CARTESIAN_POINT ( 'NONE',  ( 0.8530183727034128527, -0.4281496062992124485, 0.4176697321401328655 ) ) ;
#3768=CARTESIAN_POINT ( 'NONE',  ( -1.437007874015747477, -0.4536011799217367080, 0.2665933059059888421 ) ) ;
#3769=CARTESIAN_POINT ( 'NONE',  ( -1.614173228346456268, -0.6692913385826771977, 8.415575281601705876E-17 ) ) ;
#3770=CARTESIAN_POINT ( 'NONE',  ( -1.017060367454067249, -0.3162353388693409650, -0.4822834645669289433 ) ) ;
#3771=CARTESIAN_POINT ( 'NONE',  ( -0.01312335958005186876, -0.004921259842519870586, -0.3153832671262229437 ) ) ;
#3773=CARTESIAN_POINT ( 'NONE',  ( 0.8136482939632553313, 0.1283753931104748280, 0.1820866141732283561 ) ) ;
#3775=CARTESIAN_POINT ( 'NONE',  ( 8.195543980992789655E-16, -0.1870078740157480879, -0.4822834645669291653 ) ) ;
#3778=CARTESIAN_POINT ( 'NONE',  ( -1.292650918635170010, -0.6692913385826771977, 0.1292274648535927661 ) ) ;
#3780=CARTESIAN_POINT ( 'NONE',  ( 0.8661417322834652488, -0.1870078740157480601, -0.3641732283464567677 ) ) ;
#3781=CARTESIAN_POINT ( 'NONE',  ( 0.1312335958005257930, 0.2306618581243847221, -0.2411417322834647770 ) ) ;
#3782=CARTESIAN_POINT ( 'NONE',  ( -0.2624671916010490880, -0.6046776061558807314, 0.2411417322834647770 ) ) ;
#3783=CARTESIAN_POINT ( 'NONE',  ( -0.2034120734908128059, 0.1771653543307087630, 0.09757992244046791164 ) ) ;
#3784=LINE ( 'NONE', #16843, #18536 ) ;
#3785=CARTESIAN_POINT ( 'NONE',  ( -0.3346456692913377662, 0.07958543189024071263, -0.2665933059059888421 ) ) ;
#3786=CARTESIAN_POINT ( 'NONE',  ( 0.3477690288713918276, -0.6692913385826773087, -0.1292274648535924053 ) ) ;
#3787=CARTESIAN_POINT ( 'NONE',  ( -1.272965879265091305, -0.3690944881889763329, 0.3153832671262228327 ) ) ;
#3789=CARTESIAN_POINT ( 'NONE',  ( -1.568241469816272105, -0.3162353388693409650, -0.4822834645669289433 ) ) ;
#3792=CARTESIAN_POINT ( 'NONE',  ( -1.535433070866141225, 0.1771653543307087630, 0.000000000000000000 ) ) ;
#3793=CARTESIAN_POINT ( 'NONE',  ( -0.3871391076115479057, -0.3162353388693409650, -0.4822834645669289433 ) ) ;
#3794=CARTESIAN_POINT ( 'NONE',  ( -1.128608923884513837, 0.2306618581243847221, -0.2411417322834647770 ) ) ;
#3797=EDGE_CURVE ( 'NONE', #65491, #44566, #56560, .T. ) ;
#3798=CARTESIAN_POINT ( 'NONE',  ( 1.535433070866142558, 0.2952755905511811885, 0.000000000000000000 ) ) ;
#3799=CARTESIAN_POINT ( 'NONE',  ( 0.6233595800524942554, -0.05778040916215560624, -0.4822834645669293319 ) ) ;
#3803=CARTESIAN_POINT ( 'NONE',  ( 1.614173228346457378, 0.1771653543307087630, 0.000000000000000000 ) ) ;
#3806=CARTESIAN_POINT ( 'NONE',  ( -0.8923884514435688198, -0.5023911411419708095, 0.1820866141732285504 ) ) ;
#3808=ORIENTED_EDGE ( 'NONE', *, *, #17740, .F. ) ;
#3809=CARTESIAN_POINT ( 'NONE',  ( 0.7939632545931766261, -0.05778040916215522460, 0.4822834645669289988 ) ) ;
#3810=CARTESIAN_POINT ( 'NONE',  ( -0.3608923884514428360, -0.6692913385826773087, -0.1292274648535924053 ) ) ;
#3811=CARTESIAN_POINT ( 'NONE',  ( -1.305774278215222184, 0.2952755905511811885, 0.1292274648535926551 ) ) ;
#3812=CARTESIAN_POINT ( 'NONE',  ( 1.207349081364829990, 0.2306618581243848609, 0.2411417322834645549 ) ) ;
#3813=CARTESIAN_POINT ( 'NONE',  ( -1.213910761154854745, -0.5511811023622046335, 0.09757992244046803654 ) ) ;
#3815=CARTESIAN_POINT ( 'NONE',  ( 0.1968503937007881344, -0.6692913385826771977, 8.415575281601705876E-17 ) ) ;
#3816=CARTESIAN_POINT ( 'NONE',  ( -0.7152230971128602510, -0.3162353388693405765, 0.4822834645669290543 ) ) ;
#3818=CARTESIAN_POINT ( 'NONE',  ( -1.056430446194224881, -0.6692913385826771977, 0.1292274648535927661 ) ) ;
#3820=CARTESIAN_POINT ( 'NONE',  ( 0.9383202099737538715, -0.05778040916215560624, -0.4822834645669293319 ) ) ;
#3822=CARTESIAN_POINT ( 'NONE',  ( 1.246719160104987623, -0.004921259842519870586, -0.3153832671262229437 ) ) ;
#3823=ORIENTED_EDGE ( 'NONE', *, *, #26568, .T. ) ;
#3825=CARTESIAN_POINT ( 'NONE',  ( -0.3871391076115476282, -0.05778040916215522460, 0.4822834645669289988 ) ) ;
#3826=ORIENTED_EDGE ( 'NONE', *, *, #68575, .T. ) ;
#3828=CARTESIAN_POINT ( 'NONE',  ( 0.3083989501312343062, -0.2845877964562159024, 0.3641732283464567677 ) ) ;
#3829=CARTESIAN_POINT ( 'NONE',  ( -1.673228346456691717, 0.1660481256975883668, -0.3530559997133364547 ) ) ;
#3830=CARTESIAN_POINT ( 'NONE',  ( 0.6627296587926515548, 0.2952755905511811885, 0.1292274648535926551 ) ) ;
#3831=CARTESIAN_POINT ( 'NONE',  ( 0.7611548556430451917, -0.6046776061558807314, 0.2411417322834647770 ) ) ;
#3832=CARTESIAN_POINT ( 'NONE',  ( -0.1443569553805768291, 0.05413385826771666132, 0.4176697321401328100 ) ) ;
#3834=CARTESIAN_POINT ( 'NONE',  ( -0.9448818897637790704, -0.1870078740157480879, -0.4822834645669291653 ) ) ;
#3836=CARTESIAN_POINT ( 'NONE',  ( -1.535433070866141225, 0.2952755905511811885, 0.000000000000000000 ) ) ;
#3837=CARTESIAN_POINT ( 'NONE',  ( -1.076115485564303809, -0.6046776061558809534, -0.2411417322834644161 ) ) ;
#3838=CARTESIAN_POINT ( 'NONE',  ( 1.115485564304462551, -0.4281496062992127816, -0.4176697321401328100 ) ) ;
#3839=CARTESIAN_POINT ( 'NONE',  ( 1.587926509186352586, -0.4281496062992127816, -0.4176697321401328100 ) ) ;
#3841=CARTESIAN_POINT ( 'NONE',  ( -1.069553805774277722, 0.2952755905511811885, 0.1292274648535926551 ) ) ;
#3843=CARTESIAN_POINT ( 'NONE',  ( 0.1968503937007881344, 0.2952755905511811885, 0.000000000000000000 ) ) ;
#3845=CARTESIAN_POINT ( 'NONE',  ( -0.4265091863517051496, -0.6692913385826771977, 0.1292274648535927661 ) ) ;
#3846=CARTESIAN_POINT ( 'NONE',  ( -1.633858267716534529, 0.07958543189024085140, 0.2665933059059887866 ) ) ;
#3847=CARTESIAN_POINT ( 'NONE',  ( 0.7874015748031503170, -0.1870078740157480601, -0.3641732283464567677 ) ) ;
#3848=CARTESIAN_POINT ( 'NONE',  ( 1.154855643044620184, 0.2306618581243847221, -0.2411417322834647770 ) ) ;
#3850=CARTESIAN_POINT ( 'NONE',  ( 0.5905511811023629321, 0.1771653543307087630, 0.000000000000000000 ) ) ;
#3851=CARTESIAN_POINT ( 'NONE',  ( 0.7349081364829402885, -0.6046776061558809534, -0.2411417322834644161 ) ) ;
#3853=CARTESIAN_POINT ( 'NONE',  ( -0.5839895013123351797, 0.2952755905511810774, -0.1292274648535930714 ) ) ;
#3855=CARTESIAN_POINT ( 'NONE',  ( 1.345144356955381593, -0.2845877964562161244, -0.3641732283464567121 ) ) ;
#3856=CARTESIAN_POINT ( 'NONE',  ( -0.7545931758530177724, 0.2952755905511811885, 0.1292274648535926551 ) ) ;
#3857=CARTESIAN_POINT ( 'NONE',  ( 0.1443569553805781891, -0.4281496062992124485, 0.4176697321401328655 ) ) ;
#3858=CARTESIAN_POINT ( 'NONE',  ( -1.141732283464566011, 0.2952755905511811885, 0.000000000000000000 ) ) ;
#3859=CARTESIAN_POINT ( 'NONE',  ( -0.04593175853018302557, -0.6692913385826773087, -0.1292274648535924053 ) ) ;
#3860=CARTESIAN_POINT ( 'NONE',  ( 0.3412073490813655186, -0.5023911411419708095, -0.1820866141732282451 ) ) ;
#3862=CARTESIAN_POINT ( 'NONE',  ( 0.1312335958005257930, 0.1283753931104746893, -0.1820866141732285504 ) ) ;
#3863=CARTESIAN_POINT ( 'NONE',  ( 0.6758530183727039509, 0.1771653543307087075, -0.09757992244046823083 ) ) ;
#3864=CARTESIAN_POINT ( 'NONE',  ( -1.627296587926508442, 0.2306618581243848609, 0.2411417322834645549 ) ) ;
#3865=EDGE_CURVE ( 'NONE', #29791, #38771, #7201, .T. ) ;
#3867=CARTESIAN_POINT ( 'NONE',  ( 0.7217847769028878924, 0.05413385826771666132, 0.4176697321401328100 ) ) ;
#3869=CARTESIAN_POINT ( 'NONE',  ( 1.522309711286089939, 0.1283753931104748280, 0.1820866141732283561 ) ) ;
#3871=CARTESIAN_POINT ( 'NONE',  ( 0.1706036745406830368, -0.004921259842519576551, 0.3153832671262227771 ) ) ;
#3872=CARTESIAN_POINT ( 'NONE',  ( 0.2296587926509192634, -0.3162353388693405765, 0.4822834645669290543 ) ) ;
#3873=CARTESIAN_POINT ( 'NONE',  ( 1.456692913385827515, -0.5511811023622047445, 6.969142054262312111E-17 ) ) ;
#3874=CARTESIAN_POINT ( 'NONE',  ( -1.253280839895012377, -0.08942795157527998196, 0.3641732283464567121 ) ) ;
#3875=CARTESIAN_POINT ( 'NONE',  ( -1.430446194225721390, -0.4281496062992124485, 0.4176697321401328655 ) ) ;
#3876=CARTESIAN_POINT ( 'NONE',  ( 0.2624671916010504757, 0.2306618581243848609, 0.2411417322834645549 ) ) ;
#3877=CARTESIAN_POINT ( 'NONE',  ( 1.351706036745407680, 0.05413385826771666132, 0.4176697321401328100 ) ) ;
#3879=CARTESIAN_POINT ( 'NONE',  ( 0.04593175853018440641, 0.2952755905511810774, -0.1292274648535930714 ) ) ;
#3880=CARTESIAN_POINT ( 'NONE',  ( 1.318897637795276356, -0.5400638737290844871, 0.3530559997133364547 ) ) ;
#3881=CARTESIAN_POINT ( 'NONE',  ( 0.9383202099737538715, -0.05778040916215560624, -0.4822834645669293319 ) ) ;
#3883=CARTESIAN_POINT ( 'NONE',  ( 0.8530183727034128527, -0.3690944881889763329, 0.3153832671262228327 ) ) ;
#3884=CARTESIAN_POINT ( 'NONE',  ( 1.528871391076116026, 0.2952755905511811885, 0.1292274648535926551 ) ) ;
#3885=CARTESIAN_POINT ( 'NONE',  ( -0.01312335958005186876, -0.3690944881889763329, 0.3153832671262228327 ) ) ;
#3886=CARTESIAN_POINT ( 'NONE',  ( 0.2887139107611556010, 0.2306618581243847221, -0.2411417322834647770 ) ) ;
#3887=CARTESIAN_POINT ( 'NONE',  ( 0.7874015748031503170, -0.1870078740157479769, 0.4822834645669291653 ) ) ;
#3888=CARTESIAN_POINT ( 'NONE',  ( -0.5249343832020990641, 0.2306618581243848609, 0.2411417322834645549 ) ) ;
#3890=CARTESIAN_POINT ( 'NONE',  ( -0.07217847769028813698, -0.2845877964562161244, -0.3641732283464567121 ) ) ;
#3891=CARTESIAN_POINT ( 'NONE',  ( 0.6430446194225728496, 0.05413385826771666132, 0.4176697321401328100 ) ) ;
#3892=CARTESIAN_POINT ( 'NONE',  ( 1.089238845144357759, -0.004921259842519870586, -0.3153832671262229437 ) ) ;
#3898=CARTESIAN_POINT ( 'NONE',  ( -1.371391076115484609, -0.6692913385826771977, 0.1292274648535927661 ) ) ;
#3899=CARTESIAN_POINT ( 'NONE',  ( -0.4855643044619415427, -0.4281496062992124485, 0.4176697321401328655 ) ) ;
#3902=ORIENTED_EDGE ( 'NONE', *, *, #31743, .F. ) ;
#3903=CARTESIAN_POINT ( 'NONE',  ( 0.2624671916010504757, 0.1283753931104748280, 0.1820866141732283561 ) ) ;
#3905=CARTESIAN_POINT ( 'NONE',  ( 1.062992125984252745, -0.6692913385826771977, 8.415575281601705876E-17 ) ) ;
#3909=CARTESIAN_POINT ( 'NONE',  ( 1.574803149606299746, -0.1870078740157480879, -0.4822834645669291653 ) ) ;
#3910=CARTESIAN_POINT ( 'NONE',  ( 1.391076115485564868, -0.5023911411419708095, 0.1820866141732285504 ) ) ;
#3911=CARTESIAN_POINT ( 'NONE',  ( 0.2362204724409456558, -0.1870078740157479769, 0.4822834645669291653 ) ) ;
#3913=CARTESIAN_POINT ( 'NONE',  ( 0.05249343832021075018, -0.6046776061558807314, 0.2411417322834647770 ) ) ;
#3914=CARTESIAN_POINT ( 'NONE',  ( -0.9186351706036736120, 0.1283753931104748280, 0.1820866141732283561 ) ) ;
#3915=CARTESIAN_POINT ( 'NONE',  ( 0.3543307086614179147, 0.2952755905511811885, 0.000000000000000000 ) ) ;
#3916=CARTESIAN_POINT ( 'NONE',  ( -0.02624671916010428221, -0.6046776061558807314, 0.2411417322834647770 ) ) ;
#3917=CARTESIAN_POINT ( 'NONE',  ( 1.220472440944881942, 0.8346805926620878280, -0.5309055118110238558 ) ) ;
#3920=CARTESIAN_POINT ( 'NONE',  ( 0.7939632545931766261, -0.3162353388693409650, -0.4822834645669289433 ) ) ;
#3921=CARTESIAN_POINT ( 'NONE',  ( -0.1706036745406816491, -0.4281496062992124485, 0.4176697321401328655 ) ) ;
#3922=CARTESIAN_POINT ( 'NONE',  ( -1.174540682414697335, -0.05778040916215522460, 0.4822834645669289988 ) ) ;
#3925=CARTESIAN_POINT ( 'NONE',  ( 1.102362204724410155, -0.1870078740157479769, 0.4822834645669291653 ) ) ;
#3926=CARTESIAN_POINT ( 'NONE',  ( 0.6496062992125991586, -0.5400638737290845981, -0.3530559997133363437 ) ) ;
#3928=CARTESIAN_POINT ( 'NONE',  ( -0.5643044619422565855, 0.05413385826771626580, -0.4176697321401330321 ) ) ;
#3929=CARTESIAN_POINT ( 'NONE',  ( 0.2624671916010504757, 0.2306618581243848609, 0.2411417322834645549 ) ) ;
#3930=CARTESIAN_POINT ( 'NONE',  ( -0.2493438320209966919, -0.4281496062992124485, 0.4176697321401328655 ) ) ;
#3931=EDGE_CURVE ( 'NONE', #8463, #50964, #10215, .T. ) ;
#3932=CARTESIAN_POINT ( 'NONE',  ( 0.1771653543307093182, -0.4536011799217368745, -0.2665933059059886201 ) ) ;
#3933=CARTESIAN_POINT ( 'NONE',  ( 1.679790026246720025, 0.1283753931104748280, 0.1820866141732283561 ) ) ;
#3935=CARTESIAN_POINT ( 'NONE',  ( 0.2296587926509192634, -0.05778040916215560624, -0.4822834645669293319 ) ) ;
#3936=FILL_AREA_STYLE_COLOUR ( '', #47970 ) ;
#3937=CARTESIAN_POINT ( 'NONE',  ( -1.561679790026246017, -0.4281496062992127816, -0.4176697321401328100 ) ) ;
#3941=CARTESIAN_POINT ( 'NONE',  ( 0.5052493438320218022, -0.6692913385826773087, -0.1292274648535924053 ) ) ;
#3942=CARTESIAN_POINT ( 'NONE',  ( 0.4330708661417329575, -0.5511811023622047445, 6.969142054262312111E-17 ) ) ;
#3944=DIRECTION ( 'NONE',  ( -1.000000000000000000, -3.083952846180990774E-16, 0.000000000000000000 ) ) ;
#3948=CARTESIAN_POINT ( 'NONE',  ( 0.8661417322834652488, -0.1870078740157480879, -0.4822834645669291653 ) ) ;
#3949=CARTESIAN_POINT ( 'NONE',  ( -0.6824146981627288167, 0.2306618581243848609, 0.2411417322834645549 ) ) ;
#3950=CARTESIAN_POINT ( 'NONE',  ( -0.7086614173228339419, -0.1870078740157480879, -0.4822834645669291653 ) ) ;
#3951=CARTESIAN_POINT ( 'NONE',  ( 0.4921259842519691285, 0.1660481256975885056, 0.3530559997133364547 ) ) ;
#3952=CARTESIAN_POINT ( 'NONE',  ( 1.437007874015748810, 0.1660481256975885056, 0.3530559997133364547 ) ) ;
#3953=CARTESIAN_POINT ( 'NONE',  ( 1.193875086542981023, 0.004960608223779470680, 0.3437734562760185741 ) ) ;
#3954=CARTESIAN_POINT ( 'NONE',  ( 1.259842519685040019, -0.1870078740157480601, -0.3641732283464567677 ) ) ;
#3956=CARTESIAN_POINT ( 'NONE',  ( -1.332020997375327642, -0.08942795157527998196, 0.3641732283464567121 ) ) ;
#3958=CARTESIAN_POINT ( 'NONE',  ( 0.3280839895013130669, -0.4281496062992127816, -0.4176697321401328100 ) ) ;
#3959=CARTESIAN_POINT ( 'NONE',  ( 1.148293963254593875, -0.6692913385826771977, 0.1292274648535927661 ) ) ;
#3960=CARTESIAN_POINT ( 'NONE',  ( 0.4606732211678803424, 1.778019097314518016, -0.5309055118110237448 ) ) ;
#3961=CARTESIAN_POINT ( 'NONE',  ( -1.036745406824146176, -0.004921259842519870586, -0.3153832671262229437 ) ) ;
#3962=CARTESIAN_POINT ( 'NONE',  ( 0.4396325459317593221, 0.2952755905511810774, -0.1292274648535930714 ) ) ;
#3963=CARTESIAN_POINT ( 'NONE',  ( 1.122047244094488860, 0.07958543189024085140, 0.2665933059059887866 ) ) ;
#3965=CARTESIAN_POINT ( 'NONE',  ( -1.312335958005248715, -0.5023911411419708095, -0.1820866141732282451 ) ) ;
#3966=CARTESIAN_POINT ( 'NONE',  ( 1.279527559055118724, -0.5400638737290845981, -0.3530559997133363437 ) ) ;
#3968=CARTESIAN_POINT ( 'NONE',  ( -0.2755905511811018171, 0.1771653543307087630, 0.000000000000000000 ) ) ;
#3969=CARTESIAN_POINT ( 'NONE',  ( -0.3346456692913377662, -0.5400638737290844871, 0.3530559997133364547 ) ) ;
#3970=CARTESIAN_POINT ( 'NONE',  ( -1.555118110236219930, -0.4536011799217368745, -0.2665933059059886201 ) ) ;
#3971=CARTESIAN_POINT ( 'NONE',  ( -0.6561679790026240244, -0.6046776061558807314, 0.2411417322834647770 ) ) ;
#3972=CARTESIAN_POINT ( 'NONE',  ( -1.443569553805773564, 0.1283753931104746893, -0.1820866141732285504 ) ) ;
#3974=LINE ( 'NONE', #61633, #3699 ) ;
#3975=CARTESIAN_POINT ( 'NONE',  ( 1.535433070866142335, -0.6692913385826771977, 8.415575281601705876E-17 ) ) ;
#3977=CARTESIAN_POINT ( 'NONE',  ( -1.056430446194224881, 0.2952755905511810774, -0.1292274648535930714 ) ) ;
#3978=CARTESIAN_POINT ( 'NONE',  ( -1.148293963254592542, 0.1771653543307087630, 0.09757992244046791164 ) ) ;
#3979=CARTESIAN_POINT ( 'NONE',  ( -0.5380577427821514602, -0.3690944881889765550, -0.3153832671262227771 ) ) ;
#3980=CARTESIAN_POINT ( 'NONE',  ( -1.633858267716534529, 0.1660481256975885056, 0.3530559997133364547 ) ) ;
#3981=CARTESIAN_POINT ( 'NONE',  ( 0.1837270341207357105, -0.6046776061558809534, -0.2411417322834644161 ) ) ;
#3982=CARTESIAN_POINT ( 'NONE',  ( 0.2690288713910767848, 0.1771653543307087630, 0.09757992244046791164 ) ) ;
#3983=CARTESIAN_POINT ( 'NONE',  ( -1.220472440944881054, 0.1771653543307087630, 0.000000000000000000 ) ) ;
#3984=CARTESIAN_POINT ( 'NONE',  ( -1.541994750656167090, 0.2952755905511811885, 0.1292274648535926551 ) ) ;
#3985=CARTESIAN_POINT ( 'NONE',  ( 1.213910761154856299, -0.5511811023622048555, -0.09757992244046775898 ) ) ;
#3986=CARTESIAN_POINT ( 'NONE',  ( 1.286089238845145033, -0.6046776061558809534, -0.2411417322834644161 ) ) ;
#3988=CARTESIAN_POINT ( 'NONE',  ( 0.2755905511811031494, 0.1771653543307087630, 0.000000000000000000 ) ) ;
#3989=CARTESIAN_POINT ( 'NONE',  ( 1.056430446194226658, 0.2952755905511811885, 0.1292274648535926551 ) ) ;
#3990=CARTESIAN_POINT ( 'NONE',  ( 0.06873123812453012238, 8.471767977567108961E-16, -0.4445507791589058955 ) ) ;
#3991=CARTESIAN_POINT ( 'NONE',  ( 1.135170603674541256, 0.1771653543307087630, 0.09757992244046791164 ) ) ;
#3993=CARTESIAN_POINT ( 'NONE',  ( -1.187664041994749731, -0.3162353388693405765, 0.4822834645669290543 ) ) ;
#3994=CARTESIAN_POINT ( 'NONE',  ( -0.8202099737532799750, 0.2952755905511810774, -0.1292274648535930714 ) ) ;
#3995=CARTESIAN_POINT ( 'NONE',  ( -0.05905511811023545637, -0.5400638737290845981, -0.3530559997133363437 ) ) ;
#3998=CARTESIAN_POINT ( 'NONE',  ( 1.036745406824147508, -0.4281496062992127816, -0.4176697321401328100 ) ) ;
#3999=CARTESIAN_POINT ( 'NONE',  ( 1.587926509186352142, -0.004921259842519576551, 0.3153832671262227771 ) ) ;
#4000=CARTESIAN_POINT ( 'NONE',  ( -0.09842519685039295696, -0.5400638737290844871, 0.3530559997133364547 ) ) ;
#4001=CARTESIAN_POINT ( 'NONE',  ( 0.9055118110236227702, -0.6692913385826771977, 8.415575281601705876E-17 ) ) ;
#4007=CARTESIAN_POINT ( 'NONE',  ( -0.2887139107611542133, 0.1283753931104748280, 0.1820866141732283561 ) ) ;
#4008=CARTESIAN_POINT ( 'NONE',  ( -0.6233595800524928121, -0.05778040916215522460, 0.4822834645669289988 ) ) ;
#4009=CARTESIAN_POINT ( 'NONE',  ( 0.8202099737532813073, 0.2952755905511811885, 0.1292274648535926551 ) ) ;
#4011=CARTESIAN_POINT ( 'NONE',  ( -0.6036745406824141069, -0.5023911411419708095, -0.1820866141732282451 ) ) ;
#4012=CARTESIAN_POINT ( 'NONE',  ( -1.371391076115484609, -0.6692913385826771977, 0.1292274648535927661 ) ) ;
#4013=CARTESIAN_POINT ( 'NONE',  ( 1.351706036745407458, -0.4281496062992127816, -0.4176697321401328100 ) ) ;
#4016=DIRECTION ( 'NONE',  ( -0.000000000000000000, 1.000000000000000000, -0.000000000000000000 ) ) ;
#4018=CARTESIAN_POINT ( 'NONE',  ( 0.9448818897637802916, -0.1870078740157479769, 0.4822834645669291653 ) ) ;
#4019=CARTESIAN_POINT ( 'NONE',  ( 1.437007874015748810, 0.07958543189024085140, 0.2665933059059887866 ) ) ;
#4020=CARTESIAN_POINT ( 'NONE',  ( 1.692913385826772421, 0.2952755905511811885, 0.000000000000000000 ) ) ;
#4021=CARTESIAN_POINT ( 'NONE',  ( -1.410761154855641575, -0.3162353388693409650, -0.4822834645669289433 ) ) ;
#4024=CARTESIAN_POINT ( 'NONE',  ( 0.8530183727034128527, -0.4281496062992124485, 0.4176697321401328655 ) ) ;
#4025=CARTESIAN_POINT ( 'NONE',  ( -1.489501312335957062, -0.3162353388693409650, -0.4822834645669289433 ) ) ;
#4026=CARTESIAN_POINT ( 'NONE',  ( -0.6167979002624665030, 0.05413385826771666132, 0.4176697321401328100 ) ) ;
#4027=CARTESIAN_POINT ( 'NONE',  ( -0.4461942257217840213, 0.2306618581243848609, 0.2411417322834645549 ) ) ;
#4028=CARTESIAN_POINT ( 'NONE',  ( -1.489501312335957062, -0.05778040916215522460, 0.4822834645669289988 ) ) ;
#4030=CARTESIAN_POINT ( 'NONE',  ( 0.06561679790026316017, 0.05413385826771626580, -0.4176697321401330321 ) ) ;
#4032=CARTESIAN_POINT ( 'NONE',  ( -1.614173228346455824, 0.1771653543307087630, 0.000000000000000000 ) ) ;
#4033=ORIENTED_EDGE ( 'NONE', *, *, #62252, .T. ) ;
#4036=CARTESIAN_POINT ( 'NONE',  ( -0.06561679790026180015, 0.009842519685039467087, 0.3409548833797002021 ) ) ;
#4037=CARTESIAN_POINT ( 'NONE',  ( -1.555118110236219930, 0.1660481256975885056, 0.3530559997133364547 ) ) ;
#4039=CARTESIAN_POINT ( 'NONE',  ( 1.633858267716535639, -0.4536011799217367080, 0.2665933059059888421 ) ) ;
#4044=CARTESIAN_POINT ( 'NONE',  ( -0.1509186351706028884, -0.2845877964562161244, -0.3641732283464567121 ) ) ;
#4045=CARTESIAN_POINT ( 'NONE',  ( -1.049868766404198794, 0.1283753931104746893, -0.1820866141732285504 ) ) ;
#4046=CARTESIAN_POINT ( 'NONE',  ( -1.601049868766403650, 0.2306618581243847221, -0.2411417322834647770 ) ) ;
#4047=CARTESIAN_POINT ( 'NONE',  ( 0.6889763779527563470, 0.1660481256975883668, -0.3530559997133364547 ) ) ;
#4048=CARTESIAN_POINT ( 'NONE',  ( -1.371391076115484609, -0.6692913385826771977, 0.1292274648535927661 ) ) ;
#4051=CARTESIAN_POINT ( 'NONE',  ( -1.233595800524933894, -0.6046776061558809534, -0.2411417322834644161 ) ) ;
#4053=CARTESIAN_POINT ( 'NONE',  ( 1.595398199321655275, 1.034147571970761126, -0.1559797534342494130 ) ) ;
#4055=CARTESIAN_POINT ( 'NONE',  ( -0.8070866141732276899, 0.1660481256975883668, -0.3530559997133364547 ) ) ;
#4056=CARTESIAN_POINT ( 'NONE',  ( 1.423884514435696413, -0.3162353388693409650, -0.4822834645669289433 ) ) ;
#4057=CARTESIAN_POINT ( 'NONE',  ( -1.535433070866141225, 0.2952755905511811885, 0.000000000000000000 ) ) ;
#4059=CARTESIAN_POINT ( 'NONE',  ( 1.594488188976378673, -0.5400638737290845981, -0.3530559997133363437 ) ) ;
#4060=CARTESIAN_POINT ( 'NONE',  ( -0.6758530183727028406, -0.6692913385826773087, -0.1292274648535924053 ) ) ;
#4062=CARTESIAN_POINT ( 'NONE',  ( 0.02624671916010564918, 0.1283753931104748280, 0.1820866141732283561 ) ) ;
#4064=CARTESIAN_POINT ( 'NONE',  ( 0.1115485564304470323, 0.1771653543307087630, 0.09757992244046791164 ) ) ;
#4065=CARTESIAN_POINT ( 'NONE',  ( 0.4724409448818904789, -0.1870078740157479769, 0.3641732283464567677 ) ) ;
#4066=CARTESIAN_POINT ( 'NONE',  ( 0.5249343832021003964, 0.2306618581243847221, -0.2411417322834647770 ) ) ;
#4067=CARTESIAN_POINT ( 'NONE',  ( -0.2493438320209966919, -0.3690944881889763329, 0.3153832671262228327 ) ) ;
#4069=CARTESIAN_POINT ( 'NONE',  ( -1.594488188976377119, 0.1660481256975883668, -0.3530559997133364547 ) ) ;
#4070=CARTESIAN_POINT ( 'NONE',  ( -1.010498687664041384, 0.05413385826771666132, 0.4176697321401328100 ) ) ;
#4072=CARTESIAN_POINT ( 'NONE',  ( 0.1312335958005255154, -0.6046776061558807314, 0.2411417322834647770 ) ) ;
#4073=CARTESIAN_POINT ( 'NONE',  ( -0.4396325459317577122, -0.6692913385826773087, -0.1292274648535924053 ) ) ;
#4074=CARTESIAN_POINT ( 'NONE',  ( 1.535433070866142558, 0.1771653543307087630, 0.000000000000000000 ) ) ;
#4075=CARTESIAN_POINT ( 'NONE',  ( -0.03280839895013062252, -0.5511811023622046335, 0.09757992244046803654 ) ) ;
#4076=CARTESIAN_POINT ( 'NONE',  ( -0.04593175853018302557, -0.6692913385826773087, -0.1292274648535924053 ) ) ;
#4077=CARTESIAN_POINT ( 'NONE',  ( -0.6758530183727028406, 0.2952755905511811885, 0.1292274648535926551 ) ) ;
#4080=CARTESIAN_POINT ( 'NONE',  ( 0.1968503937007881344, -0.6692913385826771977, 8.415575281601705876E-17 ) ) ;
#4081=EDGE_LOOP ( 'NONE', ( #47562, #17698, #57169 ) ) ;
#4084=CARTESIAN_POINT ( 'NONE',  ( -0.6364829396325453192, -0.2845877964562159024, 0.3641732283464567677 ) ) ;
#4085=CARTESIAN_POINT ( 'NONE',  ( -0.7152230971128602510, -0.05778040916215560624, -0.4822834645669293319 ) ) ;
#4086=CARTESIAN_POINT ( 'NONE',  ( 1.332020997375329197, -0.3162353388693405765, 0.4822834645669290543 ) ) ;
#4087=CARTESIAN_POINT ( 'NONE',  ( 1.187664041994751285, -0.05778040916215522460, 0.4822834645669289988 ) ) ;
#4088=CARTESIAN_POINT ( 'NONE',  ( -1.607611548556429737, 0.2952755905511810774, -0.1292274648535930714 ) ) ;
#4089=CARTESIAN_POINT ( 'NONE',  ( -1.181102362204723644, -0.1870078740157480601, -0.3641732283464567677 ) ) ;
#4093=CARTESIAN_POINT ( 'NONE',  ( 1.587926509186352586, -0.3690944881889765550, -0.3153832671262227771 ) ) ;
#4094=CARTESIAN_POINT ( 'NONE',  ( 1.148293963254593653, 0.1771653543307087075, -0.09757992244046823083 ) ) ;
#4096=CARTESIAN_POINT ( 'NONE',  ( 0.4002624671916016896, -0.3162353388693409650, -0.4822834645669289433 ) ) ;
#4097=CARTESIAN_POINT ( 'NONE',  ( -1.679790026246718693, 0.2306618581243847221, -0.2411417322834647770 ) ) ;
#4098=CARTESIAN_POINT ( 'NONE',  ( 0.9251968503937015864, -0.5400638737290844871, 0.3530559997133364547 ) ) ;
#4100=CARTESIAN_POINT ( 'NONE',  ( 1.253280839895013710, -0.08942795157528024563, -0.3641732283464568787 ) ) ;
#4101=( BOUNDED_SURFACE ( )  B_SPLINE_SURFACE ( 1, 2, ( 
 ( #66159, #27848, #53509, #6814, #58577, #517, #78378, #79217, #46782, #14822, #13559, #58148, #8086, #39215, #64900, #26600, #26170, #52252, #32911, #942, #71634, #13986, #39642, #20709, #1358, #46362, #72055, #79632, #10572, #74134, #21950, #15652, #3010, #16896, #28677, #74551, #67821, #41308, #42126, #66994, #23591, #54338, #60661, #80048, #23180, #29087, #22367, #66574, #36229, #68237, #16065, #48850, #80868, #10158, #48026, #9738, #53919, #54757, #42535, #72884, #34584, #8908, #2600, #9326, #34996, #61898, #4239, #73726, #16479, #41711, #35824, #47609, #55157, #73304, #29903, #55567, #67403, #48435, #81275, #35409, #15233, #40893, #3424, #61073, #80463, #60252, #22772, #61490, #3838, #28258, #29498, #6295, #63958, #17712, #82503, #31970, #57631, #56400, #68632, #43340, #18119, #12623, #31572, #5880, #18927, #63136, #18527, #30737, #43752, #70269, #24006, #24412, #38282, #30316, #11808, #44576, #62308, #42938, #31553, #37872, #37463, #24819, #49262, #55984, #69458, #74964, #5068, #82098, #5475, #17310, #10972, #50897, #50082, #57210, #31137, #69863, #4645, #56804, #50486, #76190, #82911, #36631, #44170, #25232, #81695, #49674, #75364, #12214, #69041, #63546, #76597, #11391, #75778, #37048, #62730, #71113, #64376, #77429, #7133, #40374, #27322, #52565, #46679, #20182, #25645, #8393, #33236, #6713, #1258, #32806, #72372, #13045, #52982, #78274, #77011, #51308, #19343, #14306, #7982, #65226, #34059, #58898, #33646, #837, #78695, #59722, #71953, #45832, #39966, #44993, #14721, #19764, #21018, #66056, #59308, #70692, #412, #7564, #13456, #26495, #65653, #71531, #38698, #32382, #26906, #52147, #39112, #58046, #26068, #51727, #45417, #13879, #64794, #1665, #39538, #20606, #58473, #77853, #46258, #67300, #79525, #47088, #23077, #9223, #16373, #28157, #47917, #47504, #53812, #2498, #15546, #21840, #80763, #60146, #36125, #10472, #21433, #48745, #73622, #2077, #9634, #3732, #72778, #55055, #3317, #48330, #22259, #27742, #28981, #41611, #42427, #74444, #34896, #53407, #60966, #68127, #79115, #15128, #73196, #40784, #60558, #28572, #35304, #22671, #61383, #66469, #66893, #16790, #8804, #34480, #54648, #80358, #42020, #74027, #2908, #29396, #41205, #54229, #67714, #10050, #79946, #15964, #35713, #75680, #24312, #18021, #12520, #49982, #30216, #43655, #18830, #4138, #44476, #76502, #55878, #11711, #70167, #61798, #68940, #81174, #81590, #30636, #25131, #29803, #18432, #31450, #69357, #31037, #43242, #56301, #82807, #36532, #36949, #50801, #42838, #37366, #57113, #74863, #55464, #44074, #50391, #63038, #5376, #23491, #68531, #81998, #49157, #17611, #11290, #56705, #17205, #10872, #63444, #62626, #69766, #82404, #24723, #62208, #76088, #12111, #37769, #5780, #4546, #23907, #49572, #75268, #4969, #59207, #78595, #6193, #308, #25543, #52046, #65550, #78172, #1155, #44887, #1568, #39434, #70586, #64276, #51621, #7881, #77326, #39859, #33127, #6611, #7457, #32282, #72271, #19655, #25963, #45317, #71853, #77751, #71012, #31871, #27222, #33545, #64693, #14202, #46157, #58797, #13356, #58368, #19236, #20084, #52883, #38181, #83222, #57531, #51209, #57942, #39009, #20919, #46573, #7032, #65121, #32701, #26806, #12940, #20503, #38598, #26388, #63856, #45734, #76906, #730, #71430, #52464, #13777, #34800, #14619, #41519, #54130, #54965, #9947, #47406, #48651, #73522, #80672, #8292, #27640, #40684, #59622, #73095, #41106, #47821, #35207, #73935, #79014, #79421, #29303, #1977, #40273, #79845, #15871, #54547, #22162, #21741, #9536, #67617, #2810, #67204, #22985, #53714, #46986, #65956, #60043, #53302, #66370, #15447, #33960, #16278, #60869, #35620, #9129, #21334, #72680, #3222, #15028, #28887, #66794, #61283, #8707, #41923, #80262, #34378, #2399, #28056, #22578, #48239, #3635, #60459, #28469, #107, #49481, #19458, #531, #38398, #69971, #64077, #42332, #13164, #68441, #45109, #70815, #25761, #68030, #49064, #31668, #62114, #75174, #6415, #12325, #10375, #36032, #76707, #18637, #4457, #6830, #61706, #4046, #29711, #63658, #42746, #51423, #5998, #37983, #55785, #55374 ),
 ( #38814, #58163, #57329, #83023, #25346, #17111, #64492, #32499, #10781, #19040, #44281, #44687, #81080, #57745, #23396, #77125, #26184, #74762, #51008, #74347, #70383, #16692, #36441, #12738, #32084, #30122, #81492, #23808, #20301, #33762, #8923, #77553, #34600, #66587, #45950, #1779, #60265, #2615, #59015, #71232, #71648, #20722, #15247, #51846, #8511, #21545, #65765, #21138, #33352, #46373, #72896, #26613, #27022, #40906, #32924, #14426, #47206, #64915, #45534, #34177, #40493, #40077, #27438, #19886, #58590, #72067, #13576, #7684, #1371, #8097, #39230, #7252, #53522, #52683, #59841, #59423, #72484, #958, #53099, #78809, #46793, #2194, #52266, #14833, #27862, #77971, #13999, #39656, #65347, #78391, #66172, #79230, #42138, #55580, #68251, #74564, #35009, #49275, #29511, #60674, #54350, #41722, #81290, #67415, #29916, #23193, #80062, #80881, #22380, #62320, #9749, #16077, #35421, #61912, #67833, #61086, #21962, #74978, #23606, #54771, #4254, #36243, #48864, #3437, #48447, #9339, #10172, #17323, #28271, #73317, #47622, #41325, #48039, #67006, #3851, #29100, #42952, #15664, #68646, #55172, #79645, #53933, #3022, #16910, #10586, #35837, #36644, #61505, #10984, #80475, #28689, #73741, #42548, #22787, #74147, #16492, #25663, #82112, #31987, #57647, #12638, #55996, #62745, #44185, #75791, #5490, #18943, #82516, #24018, #81708, #5897, #31151, #18133, #19360, #49686, #75379, #17727, #76204, #56413, #38298, #18542, #50501, #69471, #43354, #38715, #69877, #24426, #69055, #51324, #11824, #44591, #30750, #12230, #50095, #43766, #5081, #37477, #63149, #10, #56818, #4657, #13061, #11404, #77027, #37887, #30330, #63562, #6310, #37061, #45009, #31569, #50912, #24832, #57226, #82927, #25248, #70709, #76613, #70285, #63974, #39982, #47106, #58062, #77447, #7149, #26084, #39554, #7581, #14324, #1681, #40390, #45434, #45849, #79132, #51744, #6729, #46274, #65672, #21035, #71969, #71548, #59325, #34076, #52582, #7999, #72795, #20198, #13472, #15145, #26511, #19781, #32822, #13896, #21449, #66073, #33662, #2094, #58915, #64393, #32399, #27339, #1274, #71129, #20622, #14738, #428, #39129, #64810, #58489, #854, #52165, #8409, #27759, #77869, #52998, #65243, #78711, #33253, #46695, #26922, #59740, #53423, #78291, #72388, #48764, #35323, #36145, #23510, #54666, #3336, #80377, #74882, #29000, #9242, #22690, #81193, #66486, #49178, #55484, #34914, #74046, #40801, #8821, #47938, #60163, #60577, #9654, #4157, #34498, #80781, #10491, #48349, #10069, #22278, #60986, #61817, #15564, #15983, #29822, #21858, #16393, #2515, #53831, #28174, #23097, #29414, #42040, #67734, #79545, #47522, #35733, #73214, #79965, #73641, #61401, #41224, #66911, #42447, #41630, #74463, #3750, #55073, #2928, #16810, #68147, #28592, #54248, #67319, #18452, #57133, #51228, #70187, #38199, #57549, #68551, #62648, #4566, #31059, #44496, #82830, #63468, #23927, #63874, #44094, #49594, #43263, #30657, #12541, #56321, #18850, #12133, #68960, #69788, #11310, #17227, #82020, #4990, #24333, #50820, #56727, #50003, #10892, #6213, #31889, #43675, #76521, #25152, #37790, #75700, #36969, #83240, #25561, #42858, #36552, #75288, #82424, #18041, #69378, #31471, #11731, #62228, #30237, #5801, #37387, #63058, #55901, #81612, #17631, #5396, #24743, #50411, #76111, #7476, #39452, #58387, #32300, #27656, #58816, #71030, #38616, #14635, #748, #7900, #19676, #65140, #39027, #45335, #77345, #7051, #13374, #72289, #51640, #76926, #1993, #12959, #40291, #33147, #19254, #1173, #78611, #64294, #46593, #78190, #39879, #13795, #44906, #20521, #26824, #33976, #65972, #26409, #70604, #52482, #59637, #6628, #57960, #64711, #328, #52063, #20101, #46173, #14219, #52898, #25982, #77769, #8309, #32720, #45752, #71869, #65566, #33561, #59223, #71447, #1584, #27239, #20934, #54562, #61719, #9144, #2414, #4057, #15462, #8722, #21757, #34815, #68044, #54978, #80278, #74362, #47835, #53321, #36047, #60886, #34393, #28900, #60474, #16705, #40700, #80685, #22591, #21350, #79031, #47003, #41937, #35635, #9552, #72697, #3236, #61296, #28486, #22999 ) ),
 .UNSPECIFIED., .F., .F., .F. ) 
 B_SPLINE_SURFACE_WITH_KNOTS ( ( 2, 2 ),
 ( 3, 2, 2, 2, 2, 2, 2, 2, 2, 2, 2, 2, 2, 2, 2, 2, 2, 2, 2, 2, 2, 2, 2, 2, 2, 2, 2, 2, 2, 2, 2, 2, 2, 2, 2, 2, 2, 2, 2, 2, 2, 2, 2, 2, 2, 2, 2, 2, 2, 2, 2, 2, 2, 2, 2, 2, 2, 2, 2, 2, 2, 2, 2, 2, 2, 2, 2, 2, 2, 2, 2, 2, 2, 2, 2, 2, 2, 2, 2, 2, 2, 2, 2, 2, 2, 2, 2, 2, 2, 2, 2, 2, 2, 2, 2, 2, 2, 2, 2, 2, 2, 2, 2, 2, 2, 2, 2, 2, 2, 2, 2, 2, 2, 2, 2, 2, 2, 2, 2, 2, 2, 2, 2, 2, 2, 2, 2, 2, 2, 2, 2, 2, 2, 2, 2, 2, 2, 2, 2, 2, 2, 2, 2, 2, 2, 2, 2, 2, 2, 2, 2, 2, 2, 2, 2, 2, 2, 2, 2, 2, 2, 2, 2, 2, 2, 2, 2, 2, 2, 2, 2, 2, 2, 2, 2, 2, 2, 2, 2, 2, 2, 2, 2, 2, 2, 2, 2, 2, 2, 2, 2, 2, 2, 2, 2, 2, 2, 2, 2, 2, 2, 2, 2, 2, 2, 2, 2, 2, 2, 2, 2, 2, 2, 2, 2, 2, 2, 2, 2, 2, 2, 2, 2, 2, 2, 2, 2, 2, 2, 2, 2, 2, 2, 2, 2, 2, 2, 2, 2, 2, 2, 2, 2, 2, 2, 2, 2, 2, 2, 2, 2, 2, 2, 2, 2, 3 ),
 ( 0.000000000000000000, 1.000000000000000000 ),
 ( 0.000000000000000000, 0.003787878787878787984, 0.007575757575757575968, 0.01136363636363636395, 0.01515151515151515194, 0.01893939393939393992, 0.02272727272727272790, 0.02651515151515151589, 0.03030303030303030387, 0.03409090909090908839, 0.03787878787878787984, 0.04166666666666666435, 0.04545454545454545581, 0.04924242424242424032, 0.05303030303030303177, 0.05681818181818181629, 0.06060606060606060774, 0.06439393939393939226, 0.06818181818181817677, 0.07196969696969697516, 0.07575757575757575968, 0.07954545454545454419, 0.08333333333333332871, 0.08712121212121212710, 0.09090909090909091161, 0.09469696969696969613, 0.09848484848484848064, 0.1022727272727272790, 0.1060606060606060635, 0.1098484848484848481, 0.1136363636363636326, 0.1174242424242424310, 0.1212121212121212155, 0.1250000000000000000, 0.1287878787878787845, 0.1325757575757575690, 0.1363636363636363535, 0.1401515151515151381, 0.1439393939393939503, 0.1477272727272727348, 0.1515151515151515194, 0.1553030303030303039, 0.1590909090909090884, 0.1628787878787878729, 0.1666666666666666574, 0.1704545454545454419, 0.1742424242424242542, 0.1780303030303030387, 0.1818181818181818232, 0.1856060606060606077, 0.1893939393939393923, 0.1931818181818181768, 0.1969696969696969613, 0.2007575757575757458, 0.2045454545454545581, 0.2083333333333333426, 0.2121212121212121271, 0.2159090909090909116, 0.2196969696969696961, 0.2234848484848484806, 0.2272727272727272652, 0.2310606060606060497, 0.2348484848484848619, 0.2386363636363636465, 0.2424242424242424310, 0.2462121212121212155, 0.2500000000000000000, 0.2537878787878787845, 0.2575757575757575690, 0.2613636363636363535, 0.2651515151515151381, 0.2689393939393939226, 0.2727272727272727071, 0.2765151515151514916, 0.2803030303030302761, 0.2840909090909091161, 0.2878787878787879007, 0.2916666666666666852, 0.2954545454545454697, 0.2992424242424242542, 0.3030303030303030387, 0.3068181818181818232, 0.3106060606060606077, 0.3143939393939393923, 0.3181818181818181768, 0.3219696969696969613, 0.3257575757575757458, 0.3295454545454545303, 0.3333333333333333148, 0.3371212121212120993, 0.3409090909090908839, 0.3446969696969697239, 0.3484848484848485084, 0.3522727272727272929, 0.3560606060606060774, 0.3598484848484848619, 0.3636363636363636465, 0.3674242424242424310, 0.3712121212121212155, 0.3750000000000000000, 0.3787878787878787845, 0.3825757575757575690, 0.3863636363636363535, 0.3901515151515151381, 0.3939393939393939226, 0.3977272727272727071, 0.4015151515151514916, 0.4053030303030302761, 0.4090909090909091161, 0.4128787878787879007, 0.4166666666666666852, 0.4204545454545454697, 0.4242424242424242542, 0.4280303030303030387, 0.4318181818181818232, 0.4356060606060606077, 0.4393939393939393923, 0.4431818181818181768, 0.4469696969696969613, 0.4507575757575757458, 0.4545454545454545303, 0.4583333333333333148, 0.4621212121212120993, 0.4659090909090908839, 0.4696969696969697239, 0.4734848484848485084, 0.4772727272727272929, 0.4810606060606060774, 0.4848484848484848619, 0.4886363636363636465, 0.4924242424242424310, 0.4962121212121212155, 0.5000000000000000000, 0.5037878787878787845, 0.5075757575757575690, 0.5113636363636363535, 0.5151515151515151381, 0.5189393939393939226, 0.5227272727272727071, 0.5265151515151514916, 0.5303030303030302761, 0.5340909090909090606, 0.5378787878787878451, 0.5416666666666666297, 0.5454545454545454142, 0.5492424242424241987, 0.5530303030303029832, 0.5568181818181817677, 0.5606060606060605522, 0.5643939393939394478, 0.5681818181818182323, 0.5719696969696970168, 0.5757575757575758013, 0.5795454545454545858, 0.5833333333333333703, 0.5871212121212121549, 0.5909090909090909394, 0.5946969696969697239, 0.5984848484848485084, 0.6022727272727272929, 0.6060606060606060774, 0.6098484848484848619, 0.6136363636363636465, 0.6174242424242424310, 0.6212121212121212155, 0.6250000000000000000, 0.6287878787878787845, 0.6325757575757575690, 0.6363636363636363535, 0.6401515151515151381, 0.6439393939393939226, 0.6477272727272727071, 0.6515151515151514916, 0.6553030303030302761, 0.6590909090909090606, 0.6628787878787878451, 0.6666666666666666297, 0.6704545454545454142, 0.6742424242424241987, 0.6780303030303029832, 0.6818181818181817677, 0.6856060606060605522, 0.6893939393939394478, 0.6931818181818182323, 0.6969696969696970168, 0.7007575757575758013, 0.7045454545454545858, 0.7083333333333333703, 0.7121212121212121549, 0.7159090909090909394, 0.7196969696969697239, 0.7234848484848485084, 0.7272727272727272929, 0.7310606060606060774, 0.7348484848484848619, 0.7386363636363636465, 0.7424242424242424310, 0.7462121212121212155, 0.7500000000000000000, 0.7537878787878787845, 0.7575757575757575690, 0.7613636363636363535, 0.7651515151515151381, 0.7689393939393939226, 0.7727272727272727071, 0.7765151515151514916, 0.7803030303030302761, 0.7840909090909090606, 0.7878787878787878451, 0.7916666666666666297, 0.7954545454545454142, 0.7992424242424241987, 0.8030303030303029832, 0.8068181818181817677, 0.8106060606060605522, 0.8143939393939394478, 0.8181818181818182323, 0.8219696969696970168, 0.8257575757575758013, 0.8295454545454545858, 0.8333333333333333703, 0.8371212121212121549, 0.8409090909090909394, 0.8446969696969697239, 0.8484848484848485084, 0.8522727272727272929, 0.8560606060606060774, 0.8598484848484848619, 0.8636363636363636465, 0.8674242424242424310, 0.8712121212121212155, 0.8750000000000000000, 0.8787878787878787845, 0.8825757575757575690, 0.8863636363636363535, 0.8901515151515151381, 0.8939393939393939226, 0.8977272727272727071, 0.9015151515151514916, 0.9053030303030302761, 0.9090909090909090606, 0.9128787878787878451, 0.9166666666666666297, 0.9204545454545454142, 0.9242424242424241987, 0.9280303030303029832, 0.9318181818181817677, 0.9356060606060605522, 0.9393939393939394478, 0.9431818181818182323, 0.9469696969696970168, 0.9507575757575758013, 0.9545454545454545858, 0.9583333333333333703, 0.9621212121212121549, 0.9659090909090909394 ),
 .UNSPECIFIED. ) 
 GEOMETRIC_REPRESENTATION_ITEM ( )  RATIONAL_B_SPLINE_SURFACE ( (
 ( 1.000000000000000000, 0.9659258262890683122, 1.000000000000000000, 0.9659258262890683122, 1.000000000000000000, 0.9659258262890683122, 1.000000000000000000, 0.9659258262890683122, 1.000000000000000000, 0.9659258262890683122, 1.000000000000000000, 0.9659258262890683122, 1.000000000000000000, 0.9659258262890683122, 1.000000000000000000, 0.9659258262890683122, 1.000000000000000000, 0.9659258262890683122, 1.000000000000000000, 0.9659258262890683122, 1.000000000000000000, 0.9659258262890683122, 1.000000000000000000, 0.9659258262890683122, 1.000000000000000000, 0.9659258262890683122, 1.000000000000000000, 0.9659258262890683122, 1.000000000000000000, 0.9659258262890683122, 1.000000000000000000, 0.9659258262890683122, 1.000000000000000000, 0.9659258262890683122, 1.000000000000000000, 0.9659258262890683122, 1.000000000000000000, 0.9659258262890683122, 1.000000000000000000, 0.9659258262890683122, 1.000000000000000000, 0.9659258262890683122, 1.000000000000000000, 0.9659258262890683122, 1.000000000000000000, 0.9659258262890683122, 1.000000000000000000, 0.9659258262890683122, 1.000000000000000000, 0.9659258262890683122, 1.000000000000000000, 0.9659258262890683122, 1.000000000000000000, 0.9659258262890683122, 1.000000000000000000, 0.9659258262890683122, 1.000000000000000000, 0.9659258262890683122, 1.000000000000000000, 0.9659258262890683122, 1.000000000000000000, 0.9659258262890683122, 1.000000000000000000, 0.9659258262890683122, 1.000000000000000000, 0.9659258262890683122, 1.000000000000000000, 0.9659258262890683122, 1.000000000000000000, 0.9659258262890683122, 1.000000000000000000, 0.9659258262890683122, 1.000000000000000000, 0.9659258262890683122, 1.000000000000000000, 0.9659258262890683122, 1.000000000000000000, 0.9659258262890683122, 1.000000000000000000, 0.9659258262890683122, 1.000000000000000000, 0.9659258262890683122, 1.000000000000000000, 0.9659258262890683122, 1.000000000000000000, 0.9659258262890683122, 1.000000000000000000, 0.9659258262890683122, 1.000000000000000000, 0.9659258262890683122, 1.000000000000000000, 0.9659258262890683122, 1.000000000000000000, 0.9659258262890683122, 1.000000000000000000, 0.9659258262890683122, 1.000000000000000000, 0.9659258262890683122, 1.000000000000000000, 0.9659258262890683122, 1.000000000000000000, 0.9659258262890683122, 1.000000000000000000, 0.9659258262890683122, 1.000000000000000000, 0.9659258262890683122, 1.000000000000000000, 0.9659258262890683122, 1.000000000000000000, 0.9659258262890683122, 1.000000000000000000, 0.9659258262890683122, 1.000000000000000000, 0.9659258262890683122, 1.000000000000000000, 0.9659258262890683122, 1.000000000000000000, 0.9659258262890683122, 1.000000000000000000, 0.9659258262890683122, 1.000000000000000000, 0.9659258262890683122, 1.000000000000000000, 0.9659258262890683122, 1.000000000000000000, 0.9659258262890683122, 1.000000000000000000, 0.9659258262890683122, 1.000000000000000000, 0.9659258262890683122, 1.000000000000000000, 0.9659258262890683122, 1.000000000000000000, 0.9659258262890683122, 1.000000000000000000, 0.9659258262890683122, 1.000000000000000000, 0.9659258262890683122, 1.000000000000000000, 0.9659258262890683122, 1.000000000000000000, 0.9659258262890683122, 1.000000000000000000, 0.9659258262890683122, 1.000000000000000000, 0.9659258262890683122, 1.000000000000000000, 0.9659258262890683122, 1.000000000000000000, 0.9659258262890683122, 1.000000000000000000, 0.9659258262890683122, 1.000000000000000000, 0.9659258262890683122, 1.000000000000000000, 0.9659258262890683122, 1.000000000000000000, 0.9659258262890683122, 1.000000000000000000, 0.9659258262890683122, 1.000000000000000000, 0.9659258262890683122, 1.000000000000000000, 0.9659258262890683122, 1.000000000000000000, 0.9659258262890683122, 1.000000000000000000, 0.9659258262890683122, 1.000000000000000000, 0.9659258262890683122, 1.000000000000000000, 0.9659258262890683122, 1.000000000000000000, 0.9659258262890683122, 1.000000000000000000, 0.9659258262890683122, 1.000000000000000000, 0.9659258262890683122, 1.000000000000000000, 0.9659258262890683122, 1.000000000000000000, 0.9659258262890683122, 1.000000000000000000, 0.9659258262890683122, 1.000000000000000000, 0.9659258262890683122, 1.000000000000000000, 0.9659258262890683122, 1.000000000000000000, 0.9659258262890683122, 1.000000000000000000, 0.9659258262890683122, 1.000000000000000000, 0.9659258262890683122, 1.000000000000000000, 0.9659258262890683122, 1.000000000000000000, 0.9659258262890683122, 1.000000000000000000, 0.9659258262890683122, 1.000000000000000000, 0.9659258262890683122, 1.000000000000000000, 0.9659258262890683122, 1.000000000000000000, 0.9659258262890683122, 1.000000000000000000, 0.9659258262890683122, 1.000000000000000000, 0.9659258262890683122, 1.000000000000000000, 0.9659258262890683122, 1.000000000000000000, 0.9659258262890683122, 1.000000000000000000, 0.9659258262890683122, 1.000000000000000000, 0.9659258262890683122, 1.000000000000000000, 0.9659258262890683122, 1.000000000000000000, 0.9659258262890683122, 1.000000000000000000, 0.9659258262890683122, 1.000000000000000000, 0.9659258262890683122, 1.000000000000000000, 0.9659258262890683122, 1.000000000000000000, 0.9659258262890683122, 1.000000000000000000, 0.9659258262890683122, 1.000000000000000000, 0.9659258262890683122, 1.000000000000000000, 0.9659258262890683122, 1.000000000000000000, 0.9659258262890683122, 1.000000000000000000, 0.9659258262890683122, 1.000000000000000000, 0.9659258262890683122, 1.000000000000000000, 0.9659258262890683122, 1.000000000000000000, 0.9659258262890683122, 1.000000000000000000, 0.9659258262890683122, 1.000000000000000000, 0.9659258262890683122, 1.000000000000000000, 0.9659258262890683122, 1.000000000000000000, 0.9659258262890683122, 1.000000000000000000, 0.9659258262890683122, 1.000000000000000000, 0.9659258262890683122, 1.000000000000000000, 0.9659258262890683122, 1.000000000000000000, 0.9659258262890683122, 1.000000000000000000, 0.9659258262890683122, 1.000000000000000000, 0.9659258262890683122, 1.000000000000000000, 0.9659258262890683122, 1.000000000000000000, 0.9659258262890683122, 1.000000000000000000, 0.9659258262890683122, 1.000000000000000000, 0.9659258262890683122, 1.000000000000000000, 0.9659258262890683122, 1.000000000000000000, 0.9659258262890683122, 1.000000000000000000, 0.9659258262890683122, 1.000000000000000000, 0.9659258262890683122, 1.000000000000000000, 0.9659258262890683122, 1.000000000000000000, 0.9659258262890683122, 1.000000000000000000, 0.9659258262890683122, 1.000000000000000000, 0.9659258262890683122, 1.000000000000000000, 0.9659258262890683122, 1.000000000000000000, 0.9659258262890683122, 1.000000000000000000, 0.9659258262890683122, 1.000000000000000000, 0.9659258262890683122, 1.000000000000000000, 0.9659258262890683122, 1.000000000000000000, 0.9659258262890683122, 1.000000000000000000, 0.9659258262890683122, 1.000000000000000000, 0.9659258262890683122, 1.000000000000000000, 0.9659258262890683122, 1.000000000000000000, 0.9659258262890683122, 1.000000000000000000, 0.9659258262890683122, 1.000000000000000000, 0.9659258262890683122, 1.000000000000000000, 0.9659258262890683122, 1.000000000000000000, 0.9659258262890683122, 1.000000000000000000, 0.9659258262890683122, 1.000000000000000000, 0.9659258262890683122, 1.000000000000000000, 0.9659258262890683122, 1.000000000000000000, 0.9659258262890683122, 1.000000000000000000, 0.9659258262890683122, 1.000000000000000000, 0.9659258262890683122, 1.000000000000000000, 0.9659258262890683122, 1.000000000000000000, 0.9659258262890683122, 1.000000000000000000, 0.9659258262890683122, 1.000000000000000000, 0.9659258262890683122, 1.000000000000000000, 0.9659258262890683122, 1.000000000000000000, 0.9659258262890683122, 1.000000000000000000, 0.9659258262890683122, 1.000000000000000000, 0.9659258262890683122, 1.000000000000000000, 0.9659258262890683122, 1.000000000000000000, 0.9659258262890683122, 1.000000000000000000, 0.9659258262890683122, 1.000000000000000000, 0.9659258262890683122, 1.000000000000000000, 0.9659258262890683122, 1.000000000000000000, 0.9659258262890683122, 1.000000000000000000, 0.9659258262890683122, 1.000000000000000000, 0.9659258262890683122, 1.000000000000000000, 0.9659258262890683122, 1.000000000000000000, 0.9659258262890683122, 1.000000000000000000, 0.9659258262890683122, 1.000000000000000000, 0.9659258262890683122, 1.000000000000000000, 0.9659258262890683122, 1.000000000000000000, 0.9659258262890683122, 1.000000000000000000, 0.9659258262890683122, 1.000000000000000000, 0.9659258262890683122, 1.000000000000000000, 0.9659258262890683122, 1.000000000000000000, 0.9659258262890683122, 1.000000000000000000, 0.9659258262890683122, 1.000000000000000000, 0.9659258262890683122, 1.000000000000000000, 0.9659258262890683122, 1.000000000000000000, 0.9659258262890683122, 1.000000000000000000, 0.9659258262890683122, 1.000000000000000000, 0.9659258262890683122, 1.000000000000000000, 0.9659258262890683122, 1.000000000000000000, 0.9659258262890683122, 1.000000000000000000, 0.9659258262890683122, 1.000000000000000000, 0.9659258262890683122, 1.000000000000000000, 0.9659258262890683122, 1.000000000000000000, 0.9659258262890683122, 1.000000000000000000, 0.9659258262890683122, 1.000000000000000000, 0.9659258262890683122, 1.000000000000000000, 0.9659258262890683122, 1.000000000000000000, 0.9659258262890683122, 1.000000000000000000, 0.9659258262890683122, 1.000000000000000000, 0.9659258262890683122, 1.000000000000000000, 0.9659258262890683122, 1.000000000000000000, 0.9659258262890683122, 1.000000000000000000, 0.9659258262890683122, 1.000000000000000000, 0.9659258262890683122, 1.000000000000000000, 0.9659258262890683122, 1.000000000000000000, 0.9659258262890683122, 1.000000000000000000, 0.9659258262890683122, 1.000000000000000000, 0.9659258262890683122, 1.000000000000000000, 0.9659258262890683122, 1.000000000000000000, 0.9659258262890683122, 1.000000000000000000, 0.9659258262890683122, 1.000000000000000000, 0.9659258262890683122, 1.000000000000000000, 0.9659258262890683122, 1.000000000000000000, 0.9659258262890683122, 1.000000000000000000, 0.9659258262890683122, 1.000000000000000000, 0.9659258262890683122, 1.000000000000000000, 0.9659258262890683122, 1.000000000000000000, 0.9659258262890683122, 1.000000000000000000, 0.9659258262890683122, 1.000000000000000000, 0.9659258262890683122, 1.000000000000000000, 0.9659258262890683122, 1.000000000000000000, 0.9659258262890683122, 1.000000000000000000, 0.9659258262890683122, 1.000000000000000000, 0.9659258262890683122, 1.000000000000000000, 0.9659258262890683122, 1.000000000000000000, 0.9659258262890683122, 1.000000000000000000, 0.9659258262890683122, 1.000000000000000000, 0.9659258262890683122, 1.000000000000000000, 0.9659258262890683122, 1.000000000000000000, 0.9659258262890683122, 1.000000000000000000, 0.9659258262890683122, 1.000000000000000000, 0.9659258262890683122, 1.000000000000000000, 0.9659258262890683122, 1.000000000000000000, 0.9659258262890683122, 1.000000000000000000, 0.9659258262890683122, 1.000000000000000000, 0.9659258262890683122, 1.000000000000000000, 0.9659258262890683122, 1.000000000000000000, 0.9659258262890683122, 1.000000000000000000, 0.9659258262890683122, 1.000000000000000000, 0.9659258262890683122, 1.000000000000000000, 0.9659258262890683122, 1.000000000000000000, 0.9659258262890683122, 1.000000000000000000, 0.9659258262890683122, 1.000000000000000000, 0.9659258262890683122, 1.000000000000000000, 0.9659258262890683122, 1.000000000000000000, 0.9659258262890683122, 1.000000000000000000),
 ( 1.000000000000000000, 0.9659258262890683122, 1.000000000000000000, 0.9659258262890683122, 1.000000000000000000, 0.9659258262890683122, 1.000000000000000000, 0.9659258262890683122, 1.000000000000000000, 0.9659258262890683122, 1.000000000000000000, 0.9659258262890683122, 1.000000000000000000, 0.9659258262890683122, 1.000000000000000000, 0.9659258262890683122, 1.000000000000000000, 0.9659258262890683122, 1.000000000000000000, 0.9659258262890683122, 1.000000000000000000, 0.9659258262890683122, 1.000000000000000000, 0.9659258262890683122, 1.000000000000000000, 0.9659258262890683122, 1.000000000000000000, 0.9659258262890683122, 1.000000000000000000, 0.9659258262890683122, 1.000000000000000000, 0.9659258262890683122, 1.000000000000000000, 0.9659258262890683122, 1.000000000000000000, 0.9659258262890683122, 1.000000000000000000, 0.9659258262890683122, 1.000000000000000000, 0.9659258262890683122, 1.000000000000000000, 0.9659258262890683122, 1.000000000000000000, 0.9659258262890683122, 1.000000000000000000, 0.9659258262890683122, 1.000000000000000000, 0.9659258262890683122, 1.000000000000000000, 0.9659258262890683122, 1.000000000000000000, 0.9659258262890683122, 1.000000000000000000, 0.9659258262890683122, 1.000000000000000000, 0.9659258262890683122, 1.000000000000000000, 0.9659258262890683122, 1.000000000000000000, 0.9659258262890683122, 1.000000000000000000, 0.9659258262890683122, 1.000000000000000000, 0.9659258262890683122, 1.000000000000000000, 0.9659258262890683122, 1.000000000000000000, 0.9659258262890683122, 1.000000000000000000, 0.9659258262890683122, 1.000000000000000000, 0.9659258262890683122, 1.000000000000000000, 0.9659258262890683122, 1.000000000000000000, 0.9659258262890683122, 1.000000000000000000, 0.9659258262890683122, 1.000000000000000000, 0.9659258262890683122, 1.000000000000000000, 0.9659258262890683122, 1.000000000000000000, 0.9659258262890683122, 1.000000000000000000, 0.9659258262890683122, 1.000000000000000000, 0.9659258262890683122, 1.000000000000000000, 0.9659258262890683122, 1.000000000000000000, 0.9659258262890683122, 1.000000000000000000, 0.9659258262890683122, 1.000000000000000000, 0.9659258262890683122, 1.000000000000000000, 0.9659258262890683122, 1.000000000000000000, 0.9659258262890683122, 1.000000000000000000, 0.9659258262890683122, 1.000000000000000000, 0.9659258262890683122, 1.000000000000000000, 0.9659258262890683122, 1.000000000000000000, 0.9659258262890683122, 1.000000000000000000, 0.9659258262890683122, 1.000000000000000000, 0.9659258262890683122, 1.000000000000000000, 0.9659258262890683122, 1.000000000000000000, 0.9659258262890683122, 1.000000000000000000, 0.9659258262890683122, 1.000000000000000000, 0.9659258262890683122, 1.000000000000000000, 0.9659258262890683122, 1.000000000000000000, 0.9659258262890683122, 1.000000000000000000, 0.9659258262890683122, 1.000000000000000000, 0.9659258262890683122, 1.000000000000000000, 0.9659258262890683122, 1.000000000000000000, 0.9659258262890683122, 1.000000000000000000, 0.9659258262890683122, 1.000000000000000000, 0.9659258262890683122, 1.000000000000000000, 0.9659258262890683122, 1.000000000000000000, 0.9659258262890683122, 1.000000000000000000, 0.9659258262890683122, 1.000000000000000000, 0.9659258262890683122, 1.000000000000000000, 0.9659258262890683122, 1.000000000000000000, 0.9659258262890683122, 1.000000000000000000, 0.9659258262890683122, 1.000000000000000000, 0.9659258262890683122, 1.000000000000000000, 0.9659258262890683122, 1.000000000000000000, 0.9659258262890683122, 1.000000000000000000, 0.9659258262890683122, 1.000000000000000000, 0.9659258262890683122, 1.000000000000000000, 0.9659258262890683122, 1.000000000000000000, 0.9659258262890683122, 1.000000000000000000, 0.9659258262890683122, 1.000000000000000000, 0.9659258262890683122, 1.000000000000000000, 0.9659258262890683122, 1.000000000000000000, 0.9659258262890683122, 1.000000000000000000, 0.9659258262890683122, 1.000000000000000000, 0.9659258262890683122, 1.000000000000000000, 0.9659258262890683122, 1.000000000000000000, 0.9659258262890683122, 1.000000000000000000, 0.9659258262890683122, 1.000000000000000000, 0.9659258262890683122, 1.000000000000000000, 0.9659258262890683122, 1.000000000000000000, 0.9659258262890683122, 1.000000000000000000, 0.9659258262890683122, 1.000000000000000000, 0.9659258262890683122, 1.000000000000000000, 0.9659258262890683122, 1.000000000000000000, 0.9659258262890683122, 1.000000000000000000, 0.9659258262890683122, 1.000000000000000000, 0.9659258262890683122, 1.000000000000000000, 0.9659258262890683122, 1.000000000000000000, 0.9659258262890683122, 1.000000000000000000, 0.9659258262890683122, 1.000000000000000000, 0.9659258262890683122, 1.000000000000000000, 0.9659258262890683122, 1.000000000000000000, 0.9659258262890683122, 1.000000000000000000, 0.9659258262890683122, 1.000000000000000000, 0.9659258262890683122, 1.000000000000000000, 0.9659258262890683122, 1.000000000000000000, 0.9659258262890683122, 1.000000000000000000, 0.9659258262890683122, 1.000000000000000000, 0.9659258262890683122, 1.000000000000000000, 0.9659258262890683122, 1.000000000000000000, 0.9659258262890683122, 1.000000000000000000, 0.9659258262890683122, 1.000000000000000000, 0.9659258262890683122, 1.000000000000000000, 0.9659258262890683122, 1.000000000000000000, 0.9659258262890683122, 1.000000000000000000, 0.9659258262890683122, 1.000000000000000000, 0.9659258262890683122, 1.000000000000000000, 0.9659258262890683122, 1.000000000000000000, 0.9659258262890683122, 1.000000000000000000, 0.9659258262890683122, 1.000000000000000000, 0.9659258262890683122, 1.000000000000000000, 0.9659258262890683122, 1.000000000000000000, 0.9659258262890683122, 1.000000000000000000, 0.9659258262890683122, 1.000000000000000000, 0.9659258262890683122, 1.000000000000000000, 0.9659258262890683122, 1.000000000000000000, 0.9659258262890683122, 1.000000000000000000, 0.9659258262890683122, 1.000000000000000000, 0.9659258262890683122, 1.000000000000000000, 0.9659258262890683122, 1.000000000000000000, 0.9659258262890683122, 1.000000000000000000, 0.9659258262890683122, 1.000000000000000000, 0.9659258262890683122, 1.000000000000000000, 0.9659258262890683122, 1.000000000000000000, 0.9659258262890683122, 1.000000000000000000, 0.9659258262890683122, 1.000000000000000000, 0.9659258262890683122, 1.000000000000000000, 0.9659258262890683122, 1.000000000000000000, 0.9659258262890683122, 1.000000000000000000, 0.9659258262890683122, 1.000000000000000000, 0.9659258262890683122, 1.000000000000000000, 0.9659258262890683122, 1.000000000000000000, 0.9659258262890683122, 1.000000000000000000, 0.9659258262890683122, 1.000000000000000000, 0.9659258262890683122, 1.000000000000000000, 0.9659258262890683122, 1.000000000000000000, 0.9659258262890683122, 1.000000000000000000, 0.9659258262890683122, 1.000000000000000000, 0.9659258262890683122, 1.000000000000000000, 0.9659258262890683122, 1.000000000000000000, 0.9659258262890683122, 1.000000000000000000, 0.9659258262890683122, 1.000000000000000000, 0.9659258262890683122, 1.000000000000000000, 0.9659258262890683122, 1.000000000000000000, 0.9659258262890683122, 1.000000000000000000, 0.9659258262890683122, 1.000000000000000000, 0.9659258262890683122, 1.000000000000000000, 0.9659258262890683122, 1.000000000000000000, 0.9659258262890683122, 1.000000000000000000, 0.9659258262890683122, 1.000000000000000000, 0.9659258262890683122, 1.000000000000000000, 0.9659258262890683122, 1.000000000000000000, 0.9659258262890683122, 1.000000000000000000, 0.9659258262890683122, 1.000000000000000000, 0.9659258262890683122, 1.000000000000000000, 0.9659258262890683122, 1.000000000000000000, 0.9659258262890683122, 1.000000000000000000, 0.9659258262890683122, 1.000000000000000000, 0.9659258262890683122, 1.000000000000000000, 0.9659258262890683122, 1.000000000000000000, 0.9659258262890683122, 1.000000000000000000, 0.9659258262890683122, 1.000000000000000000, 0.9659258262890683122, 1.000000000000000000, 0.9659258262890683122, 1.000000000000000000, 0.9659258262890683122, 1.000000000000000000, 0.9659258262890683122, 1.000000000000000000, 0.9659258262890683122, 1.000000000000000000, 0.9659258262890683122, 1.000000000000000000, 0.9659258262890683122, 1.000000000000000000, 0.9659258262890683122, 1.000000000000000000, 0.9659258262890683122, 1.000000000000000000, 0.9659258262890683122, 1.000000000000000000, 0.9659258262890683122, 1.000000000000000000, 0.9659258262890683122, 1.000000000000000000, 0.9659258262890683122, 1.000000000000000000, 0.9659258262890683122, 1.000000000000000000, 0.9659258262890683122, 1.000000000000000000, 0.9659258262890683122, 1.000000000000000000, 0.9659258262890683122, 1.000000000000000000, 0.9659258262890683122, 1.000000000000000000, 0.9659258262890683122, 1.000000000000000000, 0.9659258262890683122, 1.000000000000000000, 0.9659258262890683122, 1.000000000000000000, 0.9659258262890683122, 1.000000000000000000, 0.9659258262890683122, 1.000000000000000000, 0.9659258262890683122, 1.000000000000000000, 0.9659258262890683122, 1.000000000000000000, 0.9659258262890683122, 1.000000000000000000, 0.9659258262890683122, 1.000000000000000000, 0.9659258262890683122, 1.000000000000000000, 0.9659258262890683122, 1.000000000000000000, 0.9659258262890683122, 1.000000000000000000, 0.9659258262890683122, 1.000000000000000000, 0.9659258262890683122, 1.000000000000000000, 0.9659258262890683122, 1.000000000000000000, 0.9659258262890683122, 1.000000000000000000, 0.9659258262890683122, 1.000000000000000000, 0.9659258262890683122, 1.000000000000000000, 0.9659258262890683122, 1.000000000000000000, 0.9659258262890683122, 1.000000000000000000, 0.9659258262890683122, 1.000000000000000000, 0.9659258262890683122, 1.000000000000000000, 0.9659258262890683122, 1.000000000000000000, 0.9659258262890683122, 1.000000000000000000, 0.9659258262890683122, 1.000000000000000000, 0.9659258262890683122, 1.000000000000000000, 0.9659258262890683122, 1.000000000000000000, 0.9659258262890683122, 1.000000000000000000, 0.9659258262890683122, 1.000000000000000000, 0.9659258262890683122, 1.000000000000000000, 0.9659258262890683122, 1.000000000000000000, 0.9659258262890683122, 1.000000000000000000, 0.9659258262890683122, 1.000000000000000000, 0.9659258262890683122, 1.000000000000000000, 0.9659258262890683122, 1.000000000000000000, 0.9659258262890683122, 1.000000000000000000, 0.9659258262890683122, 1.000000000000000000, 0.9659258262890683122, 1.000000000000000000, 0.9659258262890683122, 1.000000000000000000, 0.9659258262890683122, 1.000000000000000000, 0.9659258262890683122, 1.000000000000000000, 0.9659258262890683122, 1.000000000000000000, 0.9659258262890683122, 1.000000000000000000, 0.9659258262890683122, 1.000000000000000000, 0.9659258262890683122, 1.000000000000000000, 0.9659258262890683122, 1.000000000000000000, 0.9659258262890683122, 1.000000000000000000, 0.9659258262890683122, 1.000000000000000000, 0.9659258262890683122, 1.000000000000000000, 0.9659258262890683122, 1.000000000000000000, 0.9659258262890683122, 1.000000000000000000, 0.9659258262890683122, 1.000000000000000000, 0.9659258262890683122, 1.000000000000000000, 0.9659258262890683122, 1.000000000000000000, 0.9659258262890683122, 1.000000000000000000, 0.9659258262890683122, 1.000000000000000000, 0.9659258262890683122, 1.000000000000000000, 0.9659258262890683122, 1.000000000000000000, 0.9659258262890683122, 1.000000000000000000, 0.9659258262890683122, 1.000000000000000000, 0.9659258262890683122, 1.000000000000000000, 0.9659258262890683122, 1.000000000000000000) ) ) 
 REPRESENTATION_ITEM ( '' )  SURFACE ( )  );
#4103=CARTESIAN_POINT ( 'NONE',  ( 0.09186351706036827158, 0.05413385826771666132, 0.4176697321401328100 ) ) ;
#4104=CARTESIAN_POINT ( 'NONE',  ( -0.8923884514435688198, -0.6046776061558807314, 0.2411417322834647770 ) ) ;
#4105=CARTESIAN_POINT ( 'NONE',  ( 1.246719160104987623, 0.05413385826771626580, -0.4176697321401330321 ) ) ;
#4108=CARTESIAN_POINT ( 'NONE',  ( 0.3018372703412079971, -0.3690944881889763329, 0.3153832671262228327 ) ) ;
#4109=ORIENTED_EDGE ( 'NONE', *, *, #79680, .F. ) ;
#4113=CARTESIAN_POINT ( 'NONE',  ( -0.6561679790026240244, -0.6046776061558807314, 0.2411417322834647770 ) ) ;
#4114=CARTESIAN_POINT ( 'NONE',  ( -0.2493438320209966919, -0.4281496062992124485, 0.4176697321401328655 ) ) ;
#4115=CARTESIAN_POINT ( 'NONE',  ( -0.2362204724409440182, -0.1870078740157479769, 0.4822834645669291653 ) ) ;
#4116=CARTESIAN_POINT ( 'NONE',  ( 0.7742782152230979209, 0.05413385826771626580, -0.4176697321401330321 ) ) ;
#4117=CARTESIAN_POINT ( 'NONE',  ( -1.397637795275589623, -0.5400638737290845981, -0.3530559997133363437 ) ) ;
#4118=CARTESIAN_POINT ( 'NONE',  ( -0.5643044619422565855, 0.05413385826771626580, -0.4176697321401330321 ) ) ;
#4119=CARTESIAN_POINT ( 'NONE',  ( 0.5839895013123367340, -0.6692913385826773087, -0.1292274648535924053 ) ) ;
#4120=CARTESIAN_POINT ( 'NONE',  ( 0.2821522309711292364, -0.6692913385826771977, 0.1292274648535927661 ) ) ;
#4121=CARTESIAN_POINT ( 'NONE',  ( 0.8398950131233602345, -0.6046776061558807314, 0.2411417322834647770 ) ) ;
#4123=CARTESIAN_POINT ( 'NONE',  ( -0.2165354330708654795, 0.07958543189024085140, 0.2665933059059887866 ) ) ;
#4124=VERTEX_POINT ( 'NONE', #61129 ) ;
#4126=ORIENTED_EDGE ( 'NONE', *, *, #32799, .F. ) ;
#4127=CARTESIAN_POINT ( 'NONE',  ( -1.089238845144356427, -0.004921259842519576551, 0.3153832671262227771 ) ) ;
#4128=CARTESIAN_POINT ( 'NONE',  ( -0.5249343832020990641, 0.2306618581243848609, 0.2411417322834645549 ) ) ;
#4130=CARTESIAN_POINT ( 'NONE',  ( -0.8727034120734901146, -0.05778040916215560624, -0.4822834645669293319 ) ) ;
#4131=CARTESIAN_POINT ( 'NONE',  ( -0.9251968503937002541, 0.1660481256975885056, 0.3530559997133364547 ) ) ;
#4132=CARTESIAN_POINT ( 'NONE',  ( -1.220472440944881054, -0.6692913385826771977, 8.415575281601705876E-17 ) ) ;
#4133=CARTESIAN_POINT ( 'NONE',  ( -1.272965879265091305, -0.4281496062992124485, 0.4176697321401328655 ) ) ;
#4134=CARTESIAN_POINT ( 'NONE',  ( 0.8989501312335964611, 0.1771653543307087630, 0.09757992244046791164 ) ) ;
#4137=CARTESIAN_POINT ( 'NONE',  ( 0.01968503937007930540, 0.07958543189024085140, 0.2665933059059887866 ) ) ;
#4138=CARTESIAN_POINT ( 'NONE',  ( -0.2165354330708654795, 0.1660481256975885056, 0.3530559997133364547 ) ) ;
#4139=CARTESIAN_POINT ( 'NONE',  ( 0.03280839895013198948, -0.6692913385826773087, -0.1292274648535924053 ) ) ;
#4146=CARTESIAN_POINT ( 'NONE',  ( -0.8398950131233589023, -0.5023911411419708095, -0.1820866141732282451 ) ) ;
#4147=CARTESIAN_POINT ( 'NONE',  ( -0.8989501312335946848, 0.2952755905511810774, -0.1292274648535930714 ) ) ;
#4151=CARTESIAN_POINT ( 'NONE',  ( 1.391076115485564868, 0.2306618581243847221, -0.2411417322834647770 ) ) ;
#4152=CARTESIAN_POINT ( 'NONE',  ( 0.4461942257217855201, -0.6046776061558807314, 0.2411417322834647770 ) ) ;
#4153=CARTESIAN_POINT ( 'NONE',  ( 0.6496062992125991586, -0.5400638737290845981, -0.3530559997133363437 ) ) ;
#4154=CARTESIAN_POINT ( 'NONE',  ( -0.8398950131233585692, 0.1283753931104748280, 0.1820866141732283561 ) ) ;
#4155=CARTESIAN_POINT ( 'NONE',  ( 0.1443569553805781891, -0.4281496062992124485, 0.4176697321401328655 ) ) ;
#4157=CARTESIAN_POINT ( 'NONE',  ( -0.4002624671916004129, -0.05778040916215560624, -0.4822834645669293319 ) ) ;
#4159=CARTESIAN_POINT ( 'NONE',  ( 1.397637795275591177, -0.4536011799217367080, 0.2665933059059888421 ) ) ;
#4160=CARTESIAN_POINT ( 'NONE',  ( -0.4593175853018366950, -0.004921259842519576551, 0.3153832671262227771 ) ) ;
#4161=CARTESIAN_POINT ( 'NONE',  ( 0.9776902887139113929, -0.5511811023622048555, -0.09757992244046775898 ) ) ;
#4162=CARTESIAN_POINT ( 'NONE',  ( -1.043307086614172707, 0.1660481256975883668, -0.3530559997133364547 ) ) ;
#4164=CARTESIAN_POINT ( 'NONE',  ( -1.102362204724408601, -0.1870078740157480601, -0.3641732283464567677 ) ) ;
#4165=CARTESIAN_POINT ( 'NONE',  ( 0.1467811222005255545, 2.110655687203366066E-15, -0.4118477457932985253 ) ) ;
#4166=CARTESIAN_POINT ( 'NONE',  ( -1.187664041994750175, -0.05778040916215560624, -0.4822834645669293319 ) ) ;
#4167=CARTESIAN_POINT ( 'NONE',  ( -0.3608923884514428360, 0.2952755905511811885, 0.1292274648535926551 ) ) ;
#4168=CARTESIAN_POINT ( 'NONE',  ( 0.3740157480314966754, -0.5400638737290844871, 0.3530559997133364547 ) ) ;
#4170=CARTESIAN_POINT ( 'NONE',  ( 0.2887139107611556010, 0.2306618581243847221, -0.2411417322834647770 ) ) ;
#4171=CARTESIAN_POINT ( 'NONE',  ( 0.3412073490813655186, -0.5023911411419708095, -0.1820866141732282451 ) ) ;
#4172=CARTESIAN_POINT ( 'NONE',  ( -1.450131233595799651, -0.5511811023622046335, 0.09757992244046803654 ) ) ;
#4173=CARTESIAN_POINT ( 'NONE',  ( 0.8727034120734913358, -0.05778040916215522460, 0.4822834645669289988 ) ) ;
#4174=CARTESIAN_POINT ( 'NONE',  ( -1.417322834645668772, -0.1870078740157479769, 0.3641732283464567677 ) ) ;
#4175=CARTESIAN_POINT ( 'NONE',  ( 1.207349081364829990, -0.5023911411419708095, -0.1820866141732282451 ) ) ;
#4177=CARTESIAN_POINT ( 'NONE',  ( -0.8989501312335946848, 0.2952755905511810774, -0.1292274648535930714 ) ) ;
#4178=CARTESIAN_POINT ( 'NONE',  ( -0.3346456692913377662, 0.07958543189024071263, -0.2665933059059888421 ) ) ;
#4179=CARTESIAN_POINT ( 'NONE',  ( 1.034321223653608346, 4.339766966676338660E-16, 0.4118484887281966822 ) ) ;
#4180=CARTESIAN_POINT ( 'NONE',  ( 0.8530183727034126306, -0.004921259842519870586, -0.3153832671262229437 ) ) ;
#4182=CARTESIAN_POINT ( 'NONE',  ( 0.1115485564304470323, 0.2952755905511811885, 0.1292274648535926551 ) ) ;
#4185=CARTESIAN_POINT ( 'NONE',  ( 0.5118110236220478892, 0.1771653543307087630, 0.000000000000000000 ) ) ;
#4186=CARTESIAN_POINT ( 'NONE',  ( 0.1509186351706045259, -0.05778040916215560624, -0.4822834645669293319 ) ) ;
#4187=CARTESIAN_POINT ( 'NONE',  ( -0.5446194225721777693, -0.05778040916215522460, 0.4822834645669289988 ) ) ;
#4188=CARTESIAN_POINT ( 'NONE',  ( -0.3477690288713902178, 0.1771653543307087075, -0.09757992244046823083 ) ) ;
#4190=CARTESIAN_POINT ( 'NONE',  ( -0.4396325459317577122, -0.5511811023622048555, -0.09757992244046775898 ) ) ;
#4191=CARTESIAN_POINT ( 'NONE',  ( -0.1443569553805765515, -0.4281496062992127816, -0.4176697321401328100 ) ) ;
#4192=CARTESIAN_POINT ( 'NONE',  ( -1.076115485564303809, 0.1283753931104748280, 0.1820866141732283561 ) ) ;
#4194=CARTESIAN_POINT ( 'NONE',  ( 1.535433070866142335, -0.6692913385826771977, 8.415575281601705876E-17 ) ) ;
#4197=CARTESIAN_POINT ( 'NONE',  ( -1.345144356955379816, -0.08942795157528024563, -0.3641732283464568787 ) ) ;
#4198=CARTESIAN_POINT ( 'NONE',  ( -0.6627296587926503335, -0.6692913385826771977, 0.1292274648535927661 ) ) ;
#4199=CARTESIAN_POINT ( 'NONE',  ( -1.259842519685038686, -0.1870078740157480879, -0.4822834645669291653 ) ) ;
#4202=CARTESIAN_POINT ( 'NONE',  ( 1.318897637795276356, -0.5400638737290844871, 0.3530559997133364547 ) ) ;
#4203=CARTESIAN_POINT ( 'NONE',  ( 0.4593175853018380828, 0.05413385826771626580, -0.4176697321401330321 ) ) ;
#4206=CARTESIAN_POINT ( 'NONE',  ( 1.469816272965879911, 0.1283753931104746893, -0.1820866141732285504 ) ) ;
#4208=VERTEX_POINT ( 'NONE', #74610 ) ;
#4209=CARTESIAN_POINT ( 'NONE',  ( -0.9383202099737524282, -0.2845877964562161244, -0.3641732283464567121 ) ) ;
#4212=CARTESIAN_POINT ( 'NONE',  ( 0.5118110236220478892, 0.2952755905511811885, 0.000000000000000000 ) ) ;
#4213=CARTESIAN_POINT ( 'NONE',  ( -0.3805774278215216522, -0.4281496062992127816, -0.4176697321401328100 ) ) ;
#4214=CARTESIAN_POINT ( 'NONE',  ( -0.9776902887139098386, 0.2952755905511810774, -0.1292274648535930714 ) ) ;
#4215=CARTESIAN_POINT ( 'NONE',  ( 0.8858267716535438430, 0.1660481256975885056, 0.3530559997133364547 ) ) ;
#4216=CARTESIAN_POINT ( 'NONE',  ( -1.318897637795274802, 0.07958543189024085140, 0.2665933059059887866 ) ) ;
#4218=CARTESIAN_POINT ( 'NONE',  ( -0.1902887139107604098, 0.2952755905511810774, -0.1292274648535930714 ) ) ;
#4219=CARTESIAN_POINT ( 'NONE',  ( -0.9776902887139098386, 0.2952755905511810774, -0.1292274648535930714 ) ) ;
#4221=CARTESIAN_POINT ( 'NONE',  ( -1.469816272965878357, 0.2306618581243848609, 0.2411417322834645549 ) ) ;
#4222=CARTESIAN_POINT ( 'NONE',  ( -0.7426113562971992099, 2.401574803149605586, 0.5309055118110236338 ) ) ;
#4224=CARTESIAN_POINT ( 'NONE',  ( 0.9317585301837276734, -0.004921259842519870586, -0.3153832671262229437 ) ) ;
#4227=CARTESIAN_POINT ( 'NONE',  ( -0.2362204724409440182, -0.1870078740157479769, 0.4822834645669291653 ) ) ;
#4229=CARTESIAN_POINT ( 'NONE',  ( 0.4396325459317590445, -0.5511811023622046335, 0.09757992244046803654 ) ) ;
#4230=CARTESIAN_POINT ( 'NONE',  ( -1.417322834645668772, -0.1870078740157479769, 0.4822834645669291653 ) ) ;
#4231=CARTESIAN_POINT ( 'NONE',  ( 0.5052493438320215802, 0.2952755905511811885, 0.1292274648535926551 ) ) ;
#4232=CARTESIAN_POINT ( 'NONE',  ( 0.5380577427821529035, 0.05413385826771626580, -0.4176697321401330321 ) ) ;
#4233=CARTESIAN_POINT ( 'NONE',  ( 0.04593175853018440641, 0.2952755905511810774, -0.1292274648535930714 ) ) ;
#4235=CARTESIAN_POINT ( 'NONE',  ( -0.9383202099737524282, -0.3162353388693409650, -0.4822834645669289433 ) ) ;
#4237=CARTESIAN_POINT ( 'NONE',  ( 1.253280839895013710, -0.2845877964562159024, 0.3641732283464567677 ) ) ;
#4238=CARTESIAN_POINT ( 'NONE',  ( -1.148293963254592542, 0.2952755905511811885, 0.1292274648535926551 ) ) ;
#4239=CARTESIAN_POINT ( 'NONE',  ( 1.259842519685040019, -0.1870078740157480879, -0.4822834645669291653 ) ) ;
#4240=CARTESIAN_POINT ( 'NONE',  ( 1.364829396325460076, 0.2306618581243848609, 0.2411417322834645549 ) ) ;
#4241=ADVANCED_FACE ( 'NONE', ( #16954 ), #53093, .F. ) ;
#4243=CARTESIAN_POINT ( 'NONE',  ( -0.8858267716535425107, 0.1660481256975883668, -0.3530559997133364547 ) ) ;
#4245=EDGE_CURVE ( 'NONE', #44871, #73939, #73410, .T. ) ;
#4246=CARTESIAN_POINT ( 'NONE',  ( 0.1443569553805781891, -0.4281496062992124485, 0.4176697321401328655 ) ) ;
#4248=CARTESIAN_POINT ( 'NONE',  ( -0.6824146981627288167, 0.2306618581243848609, 0.2411417322834645549 ) ) ;
#4249=CARTESIAN_POINT ( 'NONE',  ( 1.607611548556431069, -0.6692913385826773087, -0.1292274648535924053 ) ) ;
#4250=CARTESIAN_POINT ( 'NONE',  ( 0.5249343832021005074, -0.5023911411419708095, 0.1820866141732285504 ) ) ;
#4251=CARTESIAN_POINT ( 'NONE',  ( 1.181102362204724976, -0.1870078740157480879, -0.4822834645669291653 ) ) ;
#4253=CARTESIAN_POINT ( 'NONE',  ( 0.7808398950131241190, -0.08942795157528024563, -0.3641732283464568787 ) ) ;
#4254=CARTESIAN_POINT ( 'NONE',  ( 0.8267716535433077274, 0.2952755905511811885, 0.000000000000000000 ) ) ;
#4256=CARTESIAN_POINT ( 'NONE',  ( -0.7414698162729651543, 0.2952755905511810774, -0.1292274648535930714 ) ) ;
#4258=CARTESIAN_POINT ( 'NONE',  ( 1.437007874015748810, 0.07958543189024085140, 0.2665933059059887866 ) ) ;
#4259=CARTESIAN_POINT ( 'NONE',  ( -0.4133858267716528645, 0.1660481256975883668, -0.3530559997133364547 ) ) ;
#4260=CARTESIAN_POINT ( 'NONE',  ( 0.02624671916010564918, 0.2306618581243848609, 0.2411417322834645549 ) ) ;
#4261=DIRECTION ( 'NONE',  ( 0.000000000000000000, 0.000000000000000000, 1.000000000000000000 ) ) ;
#4262=CARTESIAN_POINT ( 'NONE',  ( 0.2099737532808405305, 0.2306618581243847221, -0.2411417322834647770 ) ) ;
#4263=CARTESIAN_POINT ( 'NONE',  ( -0.02624671916010428221, 0.1283753931104746893, -0.1820866141732285504 ) ) ;
#4266=CARTESIAN_POINT ( 'NONE',  ( 0.1049868766404206816, 0.1283753931104748280, 0.1820866141732283561 ) ) ;
#4267=CARTESIAN_POINT ( 'NONE',  ( 0.8923884514435701520, -0.5023911411419708095, -0.1820866141732282451 ) ) ;
#4268=CARTESIAN_POINT ( 'NONE',  ( 1.614173228346457378, 1.330640075373405118, 0.1372047244094478369 ) ) ;
#4270=CARTESIAN_POINT ( 'NONE',  ( 0.2690288713910767848, 0.2952755905511811885, 0.1292274648535926551 ) ) ;
#4273=CARTESIAN_POINT ( 'NONE',  ( 1.397637795275591177, 0.07958543189024071263, -0.2665933059059888421 ) ) ;
#4274=CARTESIAN_POINT ( 'NONE',  ( -2.795275590551183242, 1.574803149606300412, -1.327125379919507468E-16 ) ) ;
#4275=CARTESIAN_POINT ( 'NONE',  ( -0.3740157480314953431, -0.4536011799217368745, -0.2665933059059886201 ) ) ;
#4276=CARTESIAN_POINT ( 'NONE',  ( -0.05249343832020911260, 0.2306618581243848609, 0.2411417322834645549 ) ) ;
#4277=CARTESIAN_POINT ( 'NONE',  ( 1.187664041994751285, -0.08942795157527998196, 0.3641732283464567121 ) ) ;
#4278=CARTESIAN_POINT ( 'NONE',  ( -1.640419947506561060, -0.3690944881889765550, -0.3153832671262227771 ) ) ;
#4279=CARTESIAN_POINT ( 'NONE',  ( -1.640419947506561060, -0.4281496062992127816, -0.4176697321401328100 ) ) ;
#4280=CARTESIAN_POINT ( 'NONE',  ( 0.05249343832021075018, -0.6046776061558807314, 0.2411417322834647770 ) ) ;
#4281=CARTESIAN_POINT ( 'NONE',  ( 1.292650918635171564, -0.6692913385826773087, -0.1292274648535924053 ) ) ;
#4283=CARTESIAN_POINT ( 'NONE',  ( 0.01968503937007930540, 0.1660481256975885056, 0.3530559997133364547 ) ) ;
#4284=CARTESIAN_POINT ( 'NONE',  ( 1.410761154855643795, -0.05778040916215560624, -0.4822834645669293319 ) ) ;
#4285=CARTESIAN_POINT ( 'NONE',  ( 0.8005249343832028242, -0.4281496062992127816, -0.4176697321401328100 ) ) ;
#4287=CARTESIAN_POINT ( 'NONE',  ( 0.5971128608923891301, 0.1771653543307087075, -0.09757992244046823083 ) ) ;
#4288=CARTESIAN_POINT ( 'NONE',  ( 1.430446194225722500, -0.4281496062992127816, -0.4176697321401328100 ) ) ;
#4289=CARTESIAN_POINT ( 'NONE',  ( 0.2230971128608929543, -0.004921259842519870586, -0.3153832671262229437 ) ) ;
#4290=CARTESIAN_POINT ( 'NONE',  ( -0.2887139107611542133, -0.6046776061558809534, -0.2411417322834644161 ) ) ;
#4291=CARTESIAN_POINT ( 'NONE',  ( 0.5446194225721792126, -0.05778040916215560624, -0.4822834645669293319 ) ) ;
#4292=CARTESIAN_POINT ( 'NONE',  ( -0.5774278215223089816, -0.6046776061558807314, 0.2411417322834647770 ) ) ;
#4294=CARTESIAN_POINT ( 'NONE',  ( -0.1509186351706028884, -0.08942795157527998196, 0.3641732283464567121 ) ) ;
#4295=CARTESIAN_POINT ( 'NONE',  ( 0.6758530183727039509, 0.2952755905511810774, -0.1292274648535930714 ) ) ;
#4296=CARTESIAN_POINT ( 'NONE',  ( 1.167979002624672580, -0.3690944881889763329, 0.3153832671262228327 ) ) ;
#4297=CARTESIAN_POINT ( 'NONE',  ( 0.1246719160104994284, 0.2952755905511810774, -0.1292274648535930714 ) ) ;
#4302=CARTESIAN_POINT ( 'NONE',  ( -1.410761154855641575, -0.3162353388693409650, -0.4822834645669289433 ) ) ;
#4303=CARTESIAN_POINT ( 'NONE',  ( -0.5380577427821514602, -0.4281496062992127816, -0.4176697321401328100 ) ) ;
#4306=ORIENTED_EDGE ( 'NONE', *, *, #63106, .F. ) ;
#4307=CARTESIAN_POINT ( 'NONE',  ( 0.3149606299212606708, -0.1870078740157480601, -0.3641732283464567677 ) ) ;
#4309=CARTESIAN_POINT ( 'NONE',  ( 0.9383202099737536495, -0.3162353388693405765, 0.4822834645669290543 ) ) ;
#4312=CARTESIAN_POINT ( 'NONE',  ( -1.640419947506561060, -0.3690944881889765550, -0.3153832671262227771 ) ) ;
#4313=CARTESIAN_POINT ( 'NONE',  ( 1.548556430446194954, 0.2306618581243847221, -0.2411417322834647770 ) ) ;
#4314=CARTESIAN_POINT ( 'NONE',  ( 1.220472440944882386, -0.5511811023622047445, 6.969142054262312111E-17 ) ) ;
#4315=CARTESIAN_POINT ( 'NONE',  ( 0.4986876640419954376, -0.6046776061558809534, -0.2411417322834644161 ) ) ;
#4317=CARTESIAN_POINT ( 'NONE',  ( -0.2559055118110227234, -0.5400638737290844871, 0.3530559997133364547 ) ) ;
#4318=CARTESIAN_POINT ( 'NONE',  ( -0.9580052493438311334, -0.3690944881889763329, 0.3153832671262228327 ) ) ;
#4319=CARTESIAN_POINT ( 'NONE',  ( 0.4068241469816279987, -0.4281496062992127816, -0.4176697321401328100 ) ) ;
#4320=CARTESIAN_POINT ( 'NONE',  ( -0.05905511811023545637, -0.5400638737290845981, -0.3530559997133363437 ) ) ;
#4324=CARTESIAN_POINT ( 'NONE',  ( 0.6364829396325465405, -0.3162353388693409650, -0.4822834645669289433 ) ) ;
#4325=CARTESIAN_POINT ( 'NONE',  ( -0.3937007874015740483, -0.1870078740157480879, -0.4822834645669291653 ) ) ;
#4326=CARTESIAN_POINT ( 'NONE',  ( -1.614173228346455824, 0.2952755905511811885, 0.000000000000000000 ) ) ;
#4327=CARTESIAN_POINT ( 'NONE',  ( 0.9383202099737536495, -0.3162353388693405765, 0.4822834645669290543 ) ) ;
#4328=CARTESIAN_POINT ( 'NONE',  ( 0.5118110236220480003, -0.6692913385826771977, 8.415575281601705876E-17 ) ) ;
#4330=CARTESIAN_POINT ( 'NONE',  ( -0.5314960629921254842, -0.5400638737290845981, -0.3530559997133363437 ) ) ;
#4331=CARTESIAN_POINT ( 'NONE',  ( 0.09186351706036827158, 0.05413385826771666132, 0.4176697321401328100 ) ) ;
#4332=CARTESIAN_POINT ( 'NONE',  ( -0.4199475065616791736, -0.6046776061558807314, 0.2411417322834647770 ) ) ;
#4333=CARTESIAN_POINT ( 'NONE',  ( 0.3937007874015754361, -0.1870078740157479769, 0.3641732283464567677 ) ) ;
#4334=CARTESIAN_POINT ( 'NONE',  ( -1.587926509186350810, -0.4281496062992124485, 0.4176697321401328655 ) ) ;
#4336=CARTESIAN_POINT ( 'NONE',  ( 0.4921259842519691285, 0.1660481256975885056, 0.3530559997133364547 ) ) ;
#4338=CARTESIAN_POINT ( 'NONE',  ( 1.482939632545932307, 0.05413385826771626580, -0.4176697321401330321 ) ) ;
#4341=ORIENTED_EDGE ( 'NONE', *, *, #41805, .F. ) ;
#4342=CARTESIAN_POINT ( 'NONE',  ( 0.5708661417322842269, 0.1660481256975885056, 0.3530559997133364547 ) ) ;
#4343=CARTESIAN_POINT ( 'NONE',  ( 0.3280839895013130669, -0.004921259842519576551, 0.3153832671262227771 ) ) ;
#4347=DIRECTION ( 'NONE',  ( -3.096699300667737957E-16, 1.000000000000000000, -0.000000000000000000 ) ) ;
#4350=CARTESIAN_POINT ( 'NONE',  ( 0.6561679790026253567, 0.2306618581243848609, 0.2411417322834645549 ) ) ;
#4351=CARTESIAN_POINT ( 'NONE',  ( -0.8858267716535425107, -0.5400638737290844871, 0.3530559997133364547 ) ) ;
#4352=CARTESIAN_POINT ( 'NONE',  ( -0.8727034120734901146, -0.05778040916215560624, -0.4822834645669293319 ) ) ;
#4353=CARTESIAN_POINT ( 'NONE',  ( 0.6036745406824153282, -0.6046776061558807314, 0.2411417322834647770 ) ) ;
#4354=CARTESIAN_POINT ( 'NONE',  ( 1.174540682414699111, -0.05778040916215560624, -0.4822834645669293319 ) ) ;
#4355=CARTESIAN_POINT ( 'NONE',  ( 1.246719160104987623, -0.004921259842519870586, -0.3153832671262229437 ) ) ;
#4357=CARTESIAN_POINT ( 'NONE',  ( 1.128608923884515169, -0.5023911411419708095, -0.1820866141732282451 ) ) ;
#4358=CARTESIAN_POINT ( 'NONE',  ( -0.8858267716535425107, -0.5400638737290844871, 0.3530559997133364547 ) ) ;
#4360=CARTESIAN_POINT ( 'NONE',  ( 1.627296587926509996, -0.6046776061558807314, 0.2411417322834647770 ) ) ;
#4361=DIRECTION ( 'NONE',  ( 0.000000000000000000, 0.000000000000000000, 1.000000000000000000 ) ) ;
#4362=CARTESIAN_POINT ( 'NONE',  ( -0.3608923884514428360, 0.2952755905511811885, 0.1292274648535926551 ) ) ;
#4363=CARTESIAN_POINT ( 'NONE',  ( 1.089238845144357759, 0.05413385826771626580, -0.4176697321401330321 ) ) ;
#4364=CARTESIAN_POINT ( 'NONE',  ( -0.7345763322112005556, 1.945772888393059175, 0.5309055118110236338 ) ) ;
#4365=CARTESIAN_POINT ( 'NONE',  ( -1.135170603674539924, -0.5511811023622046335, 0.09757992244046803654 ) ) ;
#4366=CARTESIAN_POINT ( 'NONE',  ( 0.3871391076115493490, -0.3162353388693405765, 0.4822834645669290543 ) ) ;
#4367=CARTESIAN_POINT ( 'NONE',  ( 0.7152230971128614723, -0.2845877964562161244, -0.3641732283464567121 ) ) ;
#4369=CARTESIAN_POINT ( 'NONE',  ( -1.253280839895012377, -0.08942795157527998196, 0.3641732283464567121 ) ) ;
#4370=CARTESIAN_POINT ( 'NONE',  ( 1.364829396325460076, 0.2306618581243848609, 0.2411417322834645549 ) ) ;
#4373=CARTESIAN_POINT ( 'NONE',  ( -0.2427821522309703550, -0.08942795157528024563, -0.3641732283464568787 ) ) ;
#4374=CARTESIAN_POINT ( 'NONE',  ( -0.2887139107611542133, 0.2306618581243848609, 0.2411417322834645549 ) ) ;
#4375=CARTESIAN_POINT ( 'NONE',  ( -1.338582677165353729, -0.1870078740157479769, 0.3641732283464567677 ) ) ;
#4376=CARTESIAN_POINT ( 'NONE',  ( -0.5118110236220466680, -0.6692913385826771977, 8.415575281601705876E-17 ) ) ;
#4377=CARTESIAN_POINT ( 'NONE',  ( 1.384514435695538559, 0.2952755905511810774, -0.1292274648535930714 ) ) ;
#4379=CARTESIAN_POINT ( 'NONE',  ( -0.8661417322834640276, -0.1870078740157479769, 0.3641732283464567677 ) ) ;
#4381=CARTESIAN_POINT ( 'NONE',  ( 1.423884514435696191, -0.05778040916215522460, 0.4822834645669289988 ) ) ;
#4383=CARTESIAN_POINT ( 'NONE',  ( -1.043307086614172707, 0.1660481256975883668, -0.3530559997133364547 ) ) ;
#4384=CARTESIAN_POINT ( 'NONE',  ( -0.9251968503937002541, -0.4536011799217368745, -0.2665933059059886201 ) ) ;
#4385=CARTESIAN_POINT ( 'NONE',  ( -0.4855643044619415427, -0.3690944881889763329, 0.3153832671262228327 ) ) ;
#4387=CARTESIAN_POINT ( 'NONE',  ( -0.5118110236220466680, 0.2066929133858268208, 0.000000000000000000 ) ) ;
#4388=CARTESIAN_POINT ( 'NONE',  ( 0.1509186351706045259, -0.05778040916215560624, -0.4822834645669293319 ) ) ;
#4389=CARTESIAN_POINT ( 'NONE',  ( 0.1115485564304470323, 0.1771653543307087630, 0.09757992244046791164 ) ) ;
#4390=CARTESIAN_POINT ( 'NONE',  ( -1.305774278215222184, -0.5511811023622048555, -0.09757992244046775898 ) ) ;
#4391=CARTESIAN_POINT ( 'NONE',  ( -1.364829396325458521, 0.2306618581243847221, -0.2411417322834647770 ) ) ;
#4392=CARTESIAN_POINT ( 'NONE',  ( 1.404199475065617264, -0.3690944881889763329, 0.3153832671262228327 ) ) ;
#4393=CARTESIAN_POINT ( 'NONE',  ( 1.161417322834646493, -0.5400638737290844871, 0.3530559997133364547 ) ) ;
#4395=CARTESIAN_POINT ( 'NONE',  ( 0.2952755905511819101, 0.07958543189024071263, -0.2665933059059888421 ) ) ;
#4396=CARTESIAN_POINT ( 'NONE',  ( 0.8005249343832028242, -0.4281496062992127816, -0.4176697321401328100 ) ) ;
#4398=CARTESIAN_POINT ( 'NONE',  ( 0.9973753280839902091, 0.1283753931104746893, -0.1820866141732285504 ) ) ;
#4400=CARTESIAN_POINT ( 'NONE',  ( -1.122047244094487306, 0.1660481256975883668, -0.3530559997133364547 ) ) ;
#4401=CARTESIAN_POINT ( 'NONE',  ( -1.082677165354329896, -0.5400638737290845981, -0.3530559997133363437 ) ) ;
#4402=CARTESIAN_POINT ( 'NONE',  ( -0.2230971128608915943, -0.4281496062992127816, -0.4176697321401328100 ) ) ;
#4405=CARTESIAN_POINT ( 'NONE',  ( 0.7086614173228352742, -0.1870078740157480879, -0.4822834645669291653 ) ) ;
#4406=CARTESIAN_POINT ( 'NONE',  ( 1.437007874015748810, 0.07958543189024085140, 0.2665933059059887866 ) ) ;
#4407=CARTESIAN_POINT ( 'NONE',  ( 0.1377952755905518800, 0.1660481256975883668, -0.3530559997133364547 ) ) ;
#4408=CARTESIAN_POINT ( 'NONE',  ( 0.7939632545931766261, -0.05778040916215522460, 0.4822834645669289988 ) ) ;
#4414=CARTESIAN_POINT ( 'NONE',  ( -0.3215223097112853146, -0.2845877964562159024, 0.3641732283464567677 ) ) ;
#4415=CARTESIAN_POINT ( 'NONE',  ( -0.5577427821522301654, -0.05778040916215560624, -0.4822834645669293319 ) ) ;
#4416=CARTESIAN_POINT ( 'NONE',  ( 0.4855643044619428750, 0.05413385826771666132, 0.4176697321401328100 ) ) ;
#4419=( BOUNDED_CURVE ( )  B_SPLINE_CURVE ( 1, ( #14614, #1561 ),
 .UNSPECIFIED., .F., .F. ) 
 B_SPLINE_CURVE_WITH_KNOTS ( ( 2, 2 ),
 ( 3.469446951953614189E-18, 0.001999999999999998307 ),
 .UNSPECIFIED. ) 
 CURVE ( )  GEOMETRIC_REPRESENTATION_ITEM ( )  RATIONAL_B_SPLINE_CURVE ( ( 0.9875488213027523443, 0.9875488213027523443 ) ) 
 REPRESENTATION_ITEM ( '' )  );
#4420=CARTESIAN_POINT ( 'NONE',  ( -1.423884514435694859, -0.05778040916215560624, -0.4822834645669293319 ) ) ;
#4421=CARTESIAN_POINT ( 'NONE',  ( 1.095800524934383846, -0.3162353388693405765, 0.4822834645669290543 ) ) ;
#4423=B_SPLINE_CURVE_WITH_KNOTS ( 'NONE', 3,
 ( #50920, #70293, #12645, #38307 ),
 .UNSPECIFIED., .F., .F.,
 ( 4, 4 ),
 ( 0.02954100249761015817, 0.02979193122353610695 ),
 .UNSPECIFIED. ) ;
#4426=CARTESIAN_POINT ( 'NONE',  ( 1.030183727034121421, -0.3162353388693409650, -0.4822834645669289433 ) ) ;
#4427=CARTESIAN_POINT ( 'NONE',  ( 0.5183727034120741983, 0.2952755905511810774, -0.1292274648535930714 ) ) ;
#4429=CARTESIAN_POINT ( 'NONE',  ( 1.391076115485564868, -0.5023911411419708095, 0.1820866141732285504 ) ) ;
#4430=CARTESIAN_POINT ( 'NONE',  ( -1.620734908136482577, 0.1771653543307087630, 0.09757992244046791164 ) ) ;
#4431=CARTESIAN_POINT ( 'NONE',  ( -1.548556430446193399, -0.6046776061558809534, -0.2411417322834644161 ) ) ;
#4433=CARTESIAN_POINT ( 'NONE',  ( 0.7808398950131241190, -0.05778040916215560624, -0.4822834645669293319 ) ) ;
#4435=CARTESIAN_POINT ( 'NONE',  ( 1.515748031496063408, 0.07958543189024085140, 0.2665933059059887866 ) ) ;
#4436=CARTESIAN_POINT ( 'NONE',  ( -0.7020997375328076329, -0.3162353388693409650, -0.4822834645669289433 ) ) ;
#4437=CARTESIAN_POINT ( 'NONE',  ( -0.5971128608923877978, 0.2952755905511811885, 0.1292274648535926551 ) ) ;
#4438=CARTESIAN_POINT ( 'NONE',  ( 1.404199475065617264, -0.4281496062992124485, 0.4176697321401328655 ) ) ;
#4440=CARTESIAN_POINT ( 'NONE',  ( 0.3018372703412079971, -0.4281496062992124485, 0.4176697321401328655 ) ) ;
#4442=EDGE_CURVE ( 'NONE', #72462, #7970, #61715, .T. ) ;
#4443=CARTESIAN_POINT ( 'NONE',  ( -1.502624671916009680, -0.2845877964562159024, 0.3641732283464567677 ) ) ;
#4446=VERTEX_POINT ( 'NONE', #80924 ) ;
#4447=CARTESIAN_POINT ( 'NONE',  ( -1.614173228346457378, 1.606230626554505658, -0.1372047244094477536 ) ) ;
#4448=CARTESIAN_POINT ( 'NONE',  ( 1.207349081364829990, -0.5023911411419708095, -0.1820866141732282451 ) ) ;
#4450=CARTESIAN_POINT ( 'NONE',  ( 1.555118110236221041, 0.07958543189024071263, -0.2665933059059888421 ) ) ;
#4455=CARTESIAN_POINT ( 'NONE',  ( -0.3477690288713902178, 0.1771653543307087075, -0.09757992244046823083 ) ) ;
#4456=CARTESIAN_POINT ( 'NONE',  ( -1.122047244094487306, -0.4536011799217367080, 0.2665933059059888421 ) ) ;
#4457=CARTESIAN_POINT ( 'NONE',  ( -1.581364829396324945, -0.05778040916215560624, -0.4822834645669293319 ) ) ;
#4458=CARTESIAN_POINT ( 'NONE',  ( 0.5577427821522314977, -0.3162353388693409650, -0.4822834645669289433 ) ) ;
#4459=CARTESIAN_POINT ( 'NONE',  ( -1.194225721784776262, -0.4281496062992124485, 0.4176697321401328655 ) ) ;
#4462=CARTESIAN_POINT ( 'NONE',  ( 1.548556430446194954, -0.6046776061558807314, 0.2411417322834647770 ) ) ;
#4463=DIRECTION ( 'NONE',  ( 0.7071067811865489050, -0.000000000000000000, -0.7071067811865460184 ) ) ;
#4466=CARTESIAN_POINT ( 'NONE',  ( 0.4849061582275019378, 1.967896864084105024, 0.4921425059946345493 ) ) ;
#4467=CARTESIAN_POINT ( 'NONE',  ( -0.5511811023622038563, -0.1870078740157479769, 0.4822834645669291653 ) ) ;
#4468=CARTESIAN_POINT ( 'NONE',  ( 1.292650918635171564, -0.6692913385826773087, -0.1292274648535924053 ) ) ;
#4470=CARTESIAN_POINT ( 'NONE',  ( -0.8792650918635160906, 0.05413385826771626580, -0.4176697321401330321 ) ) ;
#4472=CARTESIAN_POINT ( 'NONE',  ( -0.1246719160104980823, 0.1771653543307087630, 0.09757992244046791164 ) ) ;
#4474=CARTESIAN_POINT ( 'NONE',  ( -0.2296587926509179312, -0.08942795157527998196, 0.3641732283464567121 ) ) ;
#4475=CARTESIAN_POINT ( 'NONE',  ( 0.4986876640419954376, 0.1283753931104748280, 0.1820866141732283561 ) ) ;
#4476=CARTESIAN_POINT ( 'NONE',  ( 0.6824146981627303710, 0.2306618581243847221, -0.2411417322834647770 ) ) ;
#4477=CARTESIAN_POINT ( 'NONE',  ( -0.8858267716535425107, -0.4536011799217367080, 0.2665933059059888421 ) ) ;
#4479=CARTESIAN_POINT ( 'NONE',  ( 1.423884514435696191, -0.05778040916215522460, 0.4822834645669289988 ) ) ;
#4480=CARTESIAN_POINT ( 'NONE',  ( -0.9645669291338575535, 0.1660481256975883668, -0.3530559997133364547 ) ) ;
#4482=CARTESIAN_POINT ( 'NONE',  ( -0.1246719160104980823, 0.2952755905511811885, 0.1292274648535926551 ) ) ;
#4485=CARTESIAN_POINT ( 'NONE',  ( -0.3543307086614165824, 0.2952755905511811885, 0.000000000000000000 ) ) ;
#4486=CARTESIAN_POINT ( 'NONE',  ( 1.056430446194226658, 0.1771653543307087630, 0.09757992244046791164 ) ) ;
#4487=CARTESIAN_POINT ( 'NONE',  ( 0.1312335958005255154, -0.5023911411419708095, 0.1820866141732285504 ) ) ;
#4488=CARTESIAN_POINT ( 'NONE',  ( -0.4002624671916004129, -0.05778040916215560624, -0.4822834645669293319 ) ) ;
#4489=CARTESIAN_POINT ( 'NONE',  ( -0.7742782152230962556, -0.4281496062992127816, -0.4176697321401328100 ) ) ;
#4491=CARTESIAN_POINT ( 'NONE',  ( 1.653543307086614789, -0.1870078740157479769, 0.3641732283464567677 ) ) ;
#4493=CARTESIAN_POINT ( 'NONE',  ( 0.1902887139107617975, -0.6692913385826773087, -0.1292274648535924053 ) ) ;
#4496=CARTESIAN_POINT ( 'NONE',  ( 1.286089238845145033, 0.2306618581243848609, 0.2411417322834645549 ) ) ;
#4497=CARTESIAN_POINT ( 'NONE',  ( -0.6955380577427815458, -0.3690944881889765550, -0.3153832671262227771 ) ) ;
#4498=CARTESIAN_POINT ( 'NONE',  ( -0.7545931758530177724, 0.2952755905511811885, 0.1292274648535926551 ) ) ;
#4499=CARTESIAN_POINT ( 'NONE',  ( 1.325459317585302665, -0.4281496062992124485, 0.4176697321401328655 ) ) ;
#4500=CARTESIAN_POINT ( 'NONE',  ( 1.076115485564305141, 0.2306618581243847221, -0.2411417322834647770 ) ) ;
#4502=CARTESIAN_POINT ( 'NONE',  ( -1.194225721784776262, -0.004921259842519870586, -0.3153832671262229437 ) ) ;
#4506=CARTESIAN_POINT ( 'NONE',  ( 0.7677165354330716118, -0.4536011799217367080, 0.2665933059059888421 ) ) ;
#4507=CARTESIAN_POINT ( 'NONE',  ( 0.6692913385826777528, 0.2952755905511811885, 0.000000000000000000 ) ) ;
#4508=CARTESIAN_POINT ( 'NONE',  ( 1.561679790026247350, -0.4281496062992124485, 0.4176697321401328655 ) ) ;
#4510=CARTESIAN_POINT ( 'NONE',  ( 0.6889763779527566800, -0.4536011799217367080, 0.2665933059059888421 ) ) ;
#4511=CARTESIAN_POINT ( 'NONE',  ( -0.2690288713910754526, -0.6692913385826771977, 0.1292274648535927661 ) ) ;
#4512=CARTESIAN_POINT ( 'NONE',  ( -0.6889763779527552368, 0.1660481256975885056, 0.3530559997133364547 ) ) ;
#4513=CARTESIAN_POINT ( 'NONE',  ( 1.332020997375329197, -0.3162353388693405765, 0.4822834645669290543 ) ) ;
#4516=CARTESIAN_POINT ( 'NONE',  ( -0.1049868766404193215, 0.1283753931104746893, -0.1820866141732285504 ) ) ;
#4520=CARTESIAN_POINT ( 'NONE',  ( -0.6627296587926503335, -0.6692913385826771977, 0.1292274648535927661 ) ) ;
#4521=CARTESIAN_POINT ( 'NONE',  ( -0.1574803149606292529, -0.1870078740157480879, -0.4822834645669291653 ) ) ;
#4522=CARTESIAN_POINT ( 'NONE',  ( -0.5249343832020990641, 0.2306618581243848609, 0.2411417322834645549 ) ) ;
#4523=CARTESIAN_POINT ( 'NONE',  ( 0.5774278215223104249, 0.2306618581243848609, 0.2411417322834645549 ) ) ;
#4524=CARTESIAN_POINT ( 'NONE',  ( -0.6233595800524928121, -0.3162353388693409650, -0.4822834645669289433 ) ) ;
#4525=CARTESIAN_POINT ( 'NONE',  ( -1.430446194225720724, 0.05413385826771626580, -0.4176697321401330321 ) ) ;
#4526=CARTESIAN_POINT ( 'NONE',  ( -0.7414698162729651543, 0.2952755905511810774, -0.1292274648535930714 ) ) ;
#4527=CARTESIAN_POINT ( 'NONE',  ( 0.7545931758530188826, -0.6692913385826771977, 0.1292274648535927661 ) ) ;
#4528=CARTESIAN_POINT ( 'NONE',  ( 0.4002624671916016896, -0.3162353388693409650, -0.4822834645669289433 ) ) ;
#4530=CARTESIAN_POINT ( 'NONE',  ( -0.2952755905511803003, -0.4536011799217368745, -0.2665933059059886201 ) ) ;
#4534=CARTESIAN_POINT ( 'NONE',  ( -1.299212598425196097, -0.5511811023622047445, 6.969142054262312111E-17 ) ) ;
#4535=CARTESIAN_POINT ( 'NONE',  ( -0.4330708661417315697, -0.6692913385826771977, 8.415575281601705876E-17 ) ) ;
#4536=CARTESIAN_POINT ( 'NONE',  ( 2.795275590551181466, 2.362204724409448620, 0.000000000000000000 ) ) ;
#4537=CARTESIAN_POINT ( 'NONE',  ( -0.7086614173228339419, -0.1870078740157480879, -0.4822834645669291653 ) ) ;
#4538=CARTESIAN_POINT ( 'NONE',  ( -0.6364829396325453192, -0.3162353388693405765, 0.4822834645669290543 ) ) ;
#4539=PLANE ( 'NONE',  #70052 ) ;
#4540=CARTESIAN_POINT ( 'NONE',  ( -1.660104986876639543, -0.05778040916215560624, -0.4822834645669293319 ) ) ;
#4541=CARTESIAN_POINT ( 'NONE',  ( 0.9776902887139113929, -0.5511811023622048555, -0.09757992244046775898 ) ) ;
#4544=CARTESIAN_POINT ( 'NONE',  ( -0.07874015748031421014, -0.1870078740157480601, -0.3641732283464567677 ) ) ;
#4545=VECTOR ( 'NONE', #15434, 39.37007874015748143 ) ;
#4546=CARTESIAN_POINT ( 'NONE',  ( -0.5511811023622038563, -0.1870078740157479769, 0.4822834645669291653 ) ) ;
#4547=FACE_OUTER_BOUND ( 'NONE', #79584, .T. ) ;
#4548=CARTESIAN_POINT ( 'NONE',  ( -0.2755905511811015396, -0.6692913385826771977, 8.415575281601705876E-17 ) ) ;
#4549=VERTEX_POINT ( 'NONE', #61959 ) ;
#4552=ORIENTED_EDGE ( 'NONE', *, *, #29199, .T. ) ;
#4554=CARTESIAN_POINT ( 'NONE',  ( 1.586052503253845281, 0.4724409448818907564, -0.1653254495020589354 ) ) ;
#4555=CARTESIAN_POINT ( 'NONE',  ( -0.8464566929133852113, -0.4536011799217368745, -0.2665933059059886201 ) ) ;
#4556=CARTESIAN_POINT ( 'NONE',  ( -0.7808398950131225646, -0.05778040916215522460, 0.4822834645669289988 ) ) ;
#4560=CARTESIAN_POINT ( 'NONE',  ( 1.227034120734908917, 0.2952755905511810774, -0.1292274648535930714 ) ) ;
#4561=CARTESIAN_POINT ( 'NONE',  ( 0.3346456692913390985, 0.1660481256975885056, 0.3530559997133364547 ) ) ;
#4562=CARTESIAN_POINT ( 'NONE',  ( 0.6167979002624679463, 0.05413385826771626580, -0.4176697321401330321 ) ) ;
#4563=CARTESIAN_POINT ( 'NONE',  ( -0.6561679790026240244, 0.1283753931104746893, -0.1820866141732285504 ) ) ;
#4564=CARTESIAN_POINT ( 'NONE',  ( -0.1640419947506555343, -0.3162353388693405765, 0.4822834645669290543 ) ) ;
#4566=CARTESIAN_POINT ( 'NONE',  ( -0.7217847769028863381, 0.05413385826771626580, -0.4176697321401330321 ) ) ;
#4569=CARTESIAN_POINT ( 'NONE',  ( 1.181102362204724976, -0.1870078740157480601, -0.3641732283464567677 ) ) ;
#4570=CARTESIAN_POINT ( 'NONE',  ( -0.4396325459317579898, 0.1771653543307087630, 0.09757992244046791164 ) ) ;
#4571=CARTESIAN_POINT ( 'NONE',  ( 1.325459317585302665, -0.3690944881889763329, 0.3153832671262228327 ) ) ;
#4572=CARTESIAN_POINT ( 'NONE',  ( -1.509186351706035767, 0.05413385826771626580, -0.4176697321401330321 ) ) ;
#4573=CARTESIAN_POINT ( 'NONE',  ( -1.128608923884513837, 0.1283753931104746893, -0.1820866141732285504 ) ) ;
#4574=CARTESIAN_POINT ( 'NONE',  ( 0.1471411879992355343, 1.702998256715020864E-15, -0.4281989832122452544 ) ) ;
#4575=CARTESIAN_POINT ( 'NONE',  ( 0.3412073490813655186, -0.5023911411419708095, -0.1820866141732282451 ) ) ;
#4576=CARTESIAN_POINT ( 'NONE',  ( -0.3083989501312330295, -0.3162353388693409650, -0.4822834645669289433 ) ) ;
#4578=CARTESIAN_POINT ( 'NONE',  ( 0.06561679790026316017, -0.3690944881889763329, 0.3153832671262228327 ) ) ;
#4579=CARTESIAN_POINT ( 'NONE',  ( -1.706036745406823485, 0.1283753931104748280, 0.1820866141732283561 ) ) ;
#4580=CARTESIAN_POINT ( 'NONE',  ( 0.9448818897637802916, -0.1870078740157480879, -0.4822834645669291653 ) ) ;
#4581=FACE_OUTER_BOUND ( 'NONE', #14274, .T. ) ;
#4582=CARTESIAN_POINT ( 'NONE',  ( 1.391076115485564868, -0.5023911411419708095, 0.1820866141732285504 ) ) ;
#4583=CARTESIAN_POINT ( 'NONE',  ( -0.7480314960629914633, 0.2952755905511811885, 0.000000000000000000 ) ) ;
#4584=CARTESIAN_POINT ( 'NONE',  ( -0.4855643044619415427, -0.004921259842519870586, -0.3153832671262229437 ) ) ;
#4586=CARTESIAN_POINT ( 'NONE',  ( 0.03937007874015806264, 0.1771653543307087630, 0.000000000000000000 ) ) ;
#4587=CARTESIAN_POINT ( 'NONE',  ( -0.2952755905511803003, -0.5400638737290845981, -0.3530559997133363437 ) ) ;
#4590=CARTESIAN_POINT ( 'NONE',  ( 0.7808398950131240079, -0.2845877964562159024, 0.3641732283464567677 ) ) ;
#4591=CARTESIAN_POINT ( 'NONE',  ( -0.2165354330708654795, 0.1660481256975885056, 0.3530559997133364547 ) ) ;
#4592=CARTESIAN_POINT ( 'NONE',  ( -0.5314960629921250401, 0.1660481256975885056, 0.3530559997133364547 ) ) ;
#4593=CARTESIAN_POINT ( 'NONE',  ( -0.6496062992125976043, 0.07958543189024071263, -0.2665933059059888421 ) ) ;
#4595=CARTESIAN_POINT ( 'NONE',  ( -0.2559055118110227234, -0.4536011799217367080, 0.2665933059059888421 ) ) ;
#4596=CARTESIAN_POINT ( 'NONE',  ( 0.006561679790026889343, -0.3162353388693409650, -0.4822834645669289433 ) ) ;
#4597=CARTESIAN_POINT ( 'NONE',  ( -1.115485564304461219, -0.3690944881889763329, 0.3153832671262228327 ) ) ;
#4598=CARTESIAN_POINT ( 'NONE',  ( -1.496062992125983815, -0.1870078740157479769, 0.4822834645669291653 ) ) ;
#4599=CARTESIAN_POINT ( 'NONE',  ( 0.4624320255261049062, 8.471767977567108961E-16, -0.4445507791589058955 ) ) ;
#4602=CARTESIAN_POINT ( 'NONE',  ( -1.640419947506561060, -0.3690944881889765550, -0.3153832671262227771 ) ) ;
#4603=CARTESIAN_POINT ( 'NONE',  ( -0.4855643044619415427, -0.4281496062992124485, 0.4176697321401328655 ) ) ;
#4604=CARTESIAN_POINT ( 'NONE',  ( -1.062992125984250968, -0.6692913385826771977, 8.415575281601705876E-17 ) ) ;
#4607=CARTESIAN_POINT ( 'NONE',  ( 1.049868766404200349, 0.2306618581243848609, 0.2411417322834645549 ) ) ;
#4608=CARTESIAN_POINT ( 'NONE',  ( 0.5905511811023629321, 0.2952755905511811885, 0.000000000000000000 ) ) ;
#4611=CARTESIAN_POINT ( 'NONE',  ( 1.233595800524935227, -0.5023911411419708095, 0.1820866141732285504 ) ) ;
#4614=CARTESIAN_POINT ( 'NONE',  ( -0.9251968503937002541, -0.4536011799217368745, -0.2665933059059886201 ) ) ;
#4615=CIRCLE ( 'NONE', #54371, 1.181102362204724310 ) ;
#4617=VERTEX_POINT ( 'NONE', #10214 ) ;
#4618=CARTESIAN_POINT ( 'NONE',  ( 0.3608923884514443348, 0.2952755905511810774, -0.1292274648535930714 ) ) ;
#4619=CARTESIAN_POINT ( 'NONE',  ( -0.3412073490813641308, -0.6046776061558807314, 0.2411417322834647770 ) ) ;
#4620=CARTESIAN_POINT ( 'NONE',  ( -0.8989501312335946848, -0.6692913385826771977, 0.1292274648535927661 ) ) ;
#4621=CARTESIAN_POINT ( 'NONE',  ( 0.9908136482939640111, -0.6692913385826771977, 0.1292274648535927661 ) ) ;
#4622=CARTESIAN_POINT ( 'NONE',  ( -1.108923884514435132, -0.08942795157528024563, -0.3641732283464568787 ) ) ;
#4624=CARTESIAN_POINT ( 'NONE',  ( -0.006561679790025524116, -0.05778040916215560624, -0.4822834645669293319 ) ) ;
#4625=CARTESIAN_POINT ( 'NONE',  ( -1.312335958005248715, 0.2306618581243848609, 0.2411417322834645549 ) ) ;
#4627=CARTESIAN_POINT ( 'NONE',  ( -1.633858267716534529, 0.1660481256975885056, 0.3530559997133364547 ) ) ;
#4630=CARTESIAN_POINT ( 'NONE',  ( 0.7808398950131241190, -0.08942795157528024563, -0.3641732283464568787 ) ) ;
#4633=CARTESIAN_POINT ( 'NONE',  ( -0.8530183727034112984, 0.05413385826771666132, 0.4176697321401328100 ) ) ;
#4635=CARTESIAN_POINT ( 'NONE',  ( -0.2034120734908131112, -0.5511811023622048555, -0.09757992244046775898 ) ) ;
#4636=CARTESIAN_POINT ( 'NONE',  ( -1.660104986876639543, -0.05778040916215560624, -0.4822834645669293319 ) ) ;
#4637=CARTESIAN_POINT ( 'NONE',  ( 0.3871391076115492380, -0.05778040916215560624, -0.4822834645669293319 ) ) ;
#4638=CARTESIAN_POINT ( 'NONE',  ( 0.5905511811023629321, -0.6692913385826771977, 8.415575281601705876E-17 ) ) ;
#4639=CARTESIAN_POINT ( 'NONE',  ( -0.5249343832020990641, -0.6046776061558809534, -0.2411417322834644161 ) ) ;
#4641=CARTESIAN_POINT ( 'NONE',  ( -0.8070866141732276899, 0.1660481256975883668, -0.3530559997133364547 ) ) ;
#4643=CARTESIAN_POINT ( 'NONE',  ( 1.397637795275591177, -0.4536011799217367080, 0.2665933059059888421 ) ) ;
#4644=CARTESIAN_POINT ( 'NONE',  ( -0.8595800524934373854, -0.05778040916215522460, 0.4822834645669289988 ) ) ;
#4645=CARTESIAN_POINT ( 'NONE',  ( 0.8005249343832028242, -0.4281496062992127816, -0.4176697321401328100 ) ) ;
#4646=CARTESIAN_POINT ( 'NONE',  ( 1.384514435695538559, 0.2952755905511810774, -0.1292274648535930714 ) ) ;
#4648=CARTESIAN_POINT ( 'NONE',  ( -1.489501312335957062, -0.3162353388693409650, -0.4822834645669289433 ) ) ;
#4650=CARTESIAN_POINT ( 'NONE',  ( 0.3083989501312343062, -0.3162353388693405765, 0.4822834645669290543 ) ) ;
#4652=CARTESIAN_POINT ( 'NONE',  ( -1.509186351706035767, -0.3690944881889763329, 0.3153832671262228327 ) ) ;
#4653=CARTESIAN_POINT ( 'NONE',  ( 0.4461942257217856311, 0.1283753931104746893, -0.1820866141732285504 ) ) ;
#4654=CARTESIAN_POINT ( 'NONE',  ( 0.8398950131233602345, 0.2306618581243847221, -0.2411417322834647770 ) ) ;
#4656=CARTESIAN_POINT ( 'NONE',  ( 0.8661417322834653598, -0.1870078740157479769, 0.3641732283464567677 ) ) ;
#4657=CARTESIAN_POINT ( 'NONE',  ( 0.3018372703412079971, -0.4281496062992124485, 0.4176697321401328655 ) ) ;
#4659=CARTESIAN_POINT ( 'NONE',  ( -0.8727034120734901146, -0.05778040916215560624, -0.4822834645669293319 ) ) ;
#4660=DIRECTION ( 'NONE',  ( 1.000000000000000000, -0.000000000000000000, -0.000000000000000000 ) ) ;
#4662=CARTESIAN_POINT ( 'NONE',  ( 0.8858267716535438430, -0.4536011799217368745, -0.2665933059059886201 ) ) ;
#4663=CARTESIAN_POINT ( 'NONE',  ( -0.1377952755905504645, 0.1660481256975885056, 0.3530559997133364547 ) ) ;
#4665=CARTESIAN_POINT ( 'NONE',  ( -0.2755905511811018171, 0.2952755905511811885, 0.000000000000000000 ) ) ;
#4666=CARTESIAN_POINT ( 'NONE',  ( 0.08530183727034192087, -0.08942795157527998196, 0.3641732283464567121 ) ) ;
#4668=CARTESIAN_POINT ( 'NONE',  ( 0.1181102362204730916, 0.1771653543307087630, 0.000000000000000000 ) ) ;
#4669=CARTESIAN_POINT ( 'NONE',  ( 0.7808398950131240079, -0.2845877964562159024, 0.3641732283464567677 ) ) ;
#4672=CARTESIAN_POINT ( 'NONE',  ( 0.3740157480314966754, -0.5400638737290844871, 0.3530559997133364547 ) ) ;
#4675=CARTESIAN_POINT ( 'NONE',  ( 1.056430446194226658, 0.1771653543307087630, 0.09757992244046791164 ) ) ;
#4676=CARTESIAN_POINT ( 'NONE',  ( 0.4330708661417321248, 1.968503937007873850, 0.000000000000000000 ) ) ;
#4677=CARTESIAN_POINT ( 'NONE',  ( -0.4461942257217840213, 0.1283753931104748280, 0.1820866141732283561 ) ) ;
#4678=VECTOR ( 'NONE', #82708, 39.37007874015748143 ) ;
#4679=CARTESIAN_POINT ( 'NONE',  ( -0.2427821522309703550, -0.08942795157528024563, -0.3641732283464568787 ) ) ;
#4680=CARTESIAN_POINT ( 'NONE',  ( -0.4068241469816264999, -0.4281496062992124485, 0.4176697321401328655 ) ) ;
#4681=CARTESIAN_POINT ( 'NONE',  ( 0.8661417322834653598, -0.1870078740157479769, 0.3641732283464567677 ) ) ;
#4682=CARTESIAN_POINT ( 'NONE',  ( -1.679790026246718693, 0.1283753931104746893, -0.1820866141732285504 ) ) ;
#4683=CARTESIAN_POINT ( 'NONE',  ( 1.299212598425197429, 0.1771653543307087630, 0.000000000000000000 ) ) ;
#4684=CARTESIAN_POINT ( 'NONE',  ( 0.07874015748031558404, -0.1870078740157479769, 0.4822834645669291653 ) ) ;
#4685=CARTESIAN_POINT ( 'NONE',  ( 1.128608923884515169, -0.6046776061558809534, -0.2411417322834644161 ) ) ;
#4687=CARTESIAN_POINT ( 'NONE',  ( 5.463695987328526437E-16, -0.1870078740157479769, 0.4822834645669291653 ) ) ;
#4688=CARTESIAN_POINT ( 'NONE',  ( 1.482939632545932307, -0.4281496062992124485, 0.4176697321401328655 ) ) ;
#4689=CARTESIAN_POINT ( 'NONE',  ( 0.7414698162729663755, 0.2952755905511811885, 0.1292274648535926551 ) ) ;
#4691=CARTESIAN_POINT ( 'NONE',  ( 0.9908136482939640111, -0.5511811023622046335, 0.09757992244046803654 ) ) ;
#4692=CARTESIAN_POINT ( 'NONE',  ( 1.102362204724410155, -0.1870078740157480879, -0.4822834645669291653 ) ) ;
#4693=CARTESIAN_POINT ( 'NONE',  ( -0.006561679790025524116, -0.2845877964562159024, 0.3641732283464567677 ) ) ;
#4694=CARTESIAN_POINT ( 'NONE',  ( -0.3412073490813641308, 0.2306618581243847221, -0.2411417322834647770 ) ) ;
#4695=CARTESIAN_POINT ( 'NONE',  ( 0.2559055118110243332, -0.5400638737290845981, -0.3530559997133363437 ) ) ;
#4696=CARTESIAN_POINT ( 'NONE',  ( -0.7086614173228339419, -0.1870078740157479769, 0.4822834645669291653 ) ) ;
#4698=CARTESIAN_POINT ( 'NONE',  ( -0.09186351706036689768, -0.004921259842519870586, -0.3153832671262229437 ) ) ;
#4699=CARTESIAN_POINT ( 'NONE',  ( 0.8858267716535438430, -0.5400638737290845981, -0.3530559997133363437 ) ) ;
#4700=CARTESIAN_POINT ( 'NONE',  ( 0.9514435695538062676, -0.2845877964562161244, -0.3641732283464567121 ) ) ;
#4701=CARTESIAN_POINT ( 'NONE',  ( 0.1968503937007881344, -0.6692913385826771977, 8.415575281601705876E-17 ) ) ;
#4703=CARTESIAN_POINT ( 'NONE',  ( -1.062992125984250968, 0.2952755905511811885, 0.000000000000000000 ) ) ;
#4707=CARTESIAN_POINT ( 'NONE',  ( -1.187664041994749731, -0.3162353388693405765, 0.4822834645669290543 ) ) ;
#4708=CARTESIAN_POINT ( 'NONE',  ( -0.2952755905511804668, 0.1660481256975885056, 0.3530559997133364547 ) ) ;
#4712=CARTESIAN_POINT ( 'NONE',  ( 0.1640419947506569498, -0.2845877964562161244, -0.3641732283464567121 ) ) ;
#4714=CARTESIAN_POINT ( 'NONE',  ( 0.7283464566929140904, -0.5400638737290845981, -0.3530559997133363437 ) ) ;
#4716=CARTESIAN_POINT ( 'NONE',  ( 0.9548908091195654757, -4.927456884911482678E-16, 0.4445507791589062840 ) ) ;
#4717=CARTESIAN_POINT ( 'NONE',  ( -1.660104986876639543, -0.08942795157528024563, -0.3641732283464568787 ) ) ;
#4718=CARTESIAN_POINT ( 'NONE',  ( 1.036745406824147731, 0.05413385826771666132, 0.4176697321401328100 ) ) ;
#4719=CARTESIAN_POINT ( 'NONE',  ( 1.259842519685040019, -0.1870078740157479769, 0.3641732283464567677 ) ) ;
#4720=CARTESIAN_POINT ( 'NONE',  ( 0.1443569553805781891, 0.05413385826771626580, -0.4176697321401330321 ) ) ;
#4722=CARTESIAN_POINT ( 'NONE',  ( -0.2296587926509179312, -0.05778040916215522460, 0.4822834645669289988 ) ) ;
#4723=CARTESIAN_POINT ( 'NONE',  ( -0.9448818897637790704, -0.1870078740157479769, 0.3641732283464567677 ) ) ;
#4725=CARTESIAN_POINT ( 'NONE',  ( 0.5839895013123367340, -0.6692913385826773087, -0.1292274648535924053 ) ) ;
#4726=CARTESIAN_POINT ( 'NONE',  ( -0.6692913385826764205, -0.6692913385826771977, 8.415575281601705876E-17 ) ) ;
#4727=CARTESIAN_POINT ( 'NONE',  ( -1.586052503253848167, 1.023622047244095556, 0.1653254495020564929 ) ) ;
#4729=ORIENTED_EDGE ( 'NONE', *, *, #31019, .T. ) ;
#4731=CARTESIAN_POINT ( 'NONE',  ( 0.4658792650918641698, -0.05778040916215560624, -0.4822834645669293319 ) ) ;
#4732=VECTOR ( 'NONE', #8701, 39.37007874015748143 ) ;
#4733=CARTESIAN_POINT ( 'NONE',  ( -0.4461942257217840213, 0.2306618581243848609, 0.2411417322834645549 ) ) ;
#4734=CARTESIAN_POINT ( 'NONE',  ( -1.581364829396324945, -0.05778040916215560624, -0.4822834645669293319 ) ) ;
#4736=CARTESIAN_POINT ( 'NONE',  ( 0.9120734908136489683, -0.6692913385826771977, 0.1292274648535927661 ) ) ;
#4737=CARTESIAN_POINT ( 'NONE',  ( 0.3018372703412079971, 0.05413385826771626580, -0.4176697321401330321 ) ) ;
#4739=CARTESIAN_POINT ( 'NONE',  ( -0.8792650918635160906, 0.05413385826771626580, -0.4176697321401330321 ) ) ;
#4740=CARTESIAN_POINT ( 'NONE',  ( 0.03937007874015833325, -0.6692913385826771977, 8.415575281601705876E-17 ) ) ;
#4741=CARTESIAN_POINT ( 'NONE',  ( -0.5249343832020990641, 0.2306618581243848609, 0.2411417322834645549 ) ) ;
#4742=CARTESIAN_POINT ( 'NONE',  ( 0.1246719160104994284, 0.1771653543307087075, -0.09757992244046823083 ) ) ;
#4743=CARTESIAN_POINT ( 'NONE',  ( -1.601049868766403650, -0.6046776061558807314, 0.2411417322834647770 ) ) ;
#4745=CARTESIAN_POINT ( 'NONE',  ( 0.3543307086614179147, 0.2952755905511811885, 0.000000000000000000 ) ) ;
#4747=CARTESIAN_POINT ( 'NONE',  ( -1.594488188976377119, 0.1660481256975883668, -0.3530559997133364547 ) ) ;
#4749=VERTEX_POINT ( 'NONE', #38345 ) ;
#4750=EDGE_LOOP ( 'NONE', ( #33633, #26354, #54234, #43979 ) ) ;
#4751=CARTESIAN_POINT ( 'NONE',  ( 0.8333333333333340365, -0.6692913385826771977, 0.1292274648535927661 ) ) ;
#4752=CARTESIAN_POINT ( 'NONE',  ( 0.3083989501312343062, -0.2845877964562159024, 0.3641732283464567677 ) ) ;
#4759=CARTESIAN_POINT ( 'NONE',  ( 0.5577427821522314977, -0.3162353388693409650, -0.4822834645669289433 ) ) ;
#4760=CARTESIAN_POINT ( 'NONE',  ( -1.358267716535432434, -0.5400638737290844871, 0.3530559997133364547 ) ) ;
#4761=CARTESIAN_POINT ( 'NONE',  ( -1.279527559055116948, -0.5400638737290844871, 0.3530559997133364547 ) ) ;
#4762=CARTESIAN_POINT ( 'NONE',  ( 0.8792650918635177559, -0.4281496062992127816, -0.4176697321401328100 ) ) ;
#4763=CARTESIAN_POINT ( 'NONE',  ( 1.279527559055118724, 0.1660481256975885056, 0.3530559997133364547 ) ) ;
#4764=CARTESIAN_POINT ( 'NONE',  ( 1.489501312335958172, -0.2845877964562159024, 0.3641732283464567677 ) ) ;
#4766=CARTESIAN_POINT ( 'NONE',  ( 1.076115485564305141, 0.1283753931104746893, -0.1820866141732285504 ) ) ;
#4767=CARTESIAN_POINT ( 'NONE',  ( -0.7152230971128602510, -0.3162353388693405765, 0.4822834645669290543 ) ) ;
#4769=CARTESIAN_POINT ( 'NONE',  ( 1.404199475065617708, 0.05413385826771626580, -0.4176697321401330321 ) ) ;
#4771=CARTESIAN_POINT ( 'NONE',  ( -0.4330708661417315697, -0.6692913385826771977, 8.415575281601705876E-17 ) ) ;
#4772=CARTESIAN_POINT ( 'NONE',  ( 1.299212598425197429, -0.6692913385826771977, 8.415575281601705876E-17 ) ) ;
#4774=CARTESIAN_POINT ( 'NONE',  ( -1.023622047244094002, -0.1870078740157480601, -0.3641732283464567677 ) ) ;
#4775=CARTESIAN_POINT ( 'NONE',  ( 0.5183727034120741983, -0.6692913385826771977, 0.1292274648535927661 ) ) ;
#4776=CARTESIAN_POINT ( 'NONE',  ( 0.8858267716535438430, -0.4536011799217368745, -0.2665933059059886201 ) ) ;
#4778=CARTESIAN_POINT ( 'NONE',  ( -1.240157480314959759, 0.07958543189024085140, 0.2665933059059887866 ) ) ;
#4779=CARTESIAN_POINT ( 'NONE',  ( 1.049868766404200349, 0.2306618581243848609, 0.2411417322834645549 ) ) ;
#4781=CARTESIAN_POINT ( 'NONE',  ( -0.5118110236220466680, -0.5511811023622047445, 6.969142054262312111E-17 ) ) ;
#4782=CARTESIAN_POINT ( 'NONE',  ( -0.2427821522309703550, -0.05778040916215560624, -0.4822834645669293319 ) ) ;
#4783=CARTESIAN_POINT ( 'NONE',  ( -1.292650918635170010, 0.1771653543307087075, -0.09757992244046823083 ) ) ;
#4784=CARTESIAN_POINT ( 'NONE',  ( -0.8792650918635160906, 0.05413385826771626580, -0.4176697321401330321 ) ) ;
#4785=CARTESIAN_POINT ( 'NONE',  ( 1.476377952755906442, -0.5400638737290844871, 0.3530559997133364547 ) ) ;
#4787=CARTESIAN_POINT ( 'NONE',  ( -0.9908136482939626788, 0.1771653543307087630, 0.09757992244046791164 ) ) ;
#4789=CARTESIAN_POINT ( 'NONE',  ( 1.292650918635171564, 0.2952755905511811885, 0.1292274648535926551 ) ) ;
#4791=CARTESIAN_POINT ( 'NONE',  ( -1.377952755905511140, 0.2952755905511811885, 0.000000000000000000 ) ) ;
#4792=CARTESIAN_POINT ( 'NONE',  ( -1.443569553805773564, 0.1283753931104746893, -0.1820866141732285504 ) ) ;
#4793=CARTESIAN_POINT ( 'NONE',  ( -0.8005249343832013809, -0.3690944881889763329, 0.3153832671262228327 ) ) ;
#4794=CARTESIAN_POINT ( 'NONE',  ( -1.601049868766403650, 0.2306618581243847221, -0.2411417322834647770 ) ) ;
#4795=CARTESIAN_POINT ( 'NONE',  ( -0.1837270341207340729, 0.2306618581243847221, -0.2411417322834647770 ) ) ;
#4796=CARTESIAN_POINT ( 'NONE',  ( 0.1640419947506569498, -0.2845877964562161244, -0.3641732283464567121 ) ) ;
#4797=CARTESIAN_POINT ( 'NONE',  ( -1.089238845144356427, -0.004921259842519576551, 0.3153832671262227771 ) ) ;
#4798=CARTESIAN_POINT ( 'NONE',  ( -1.627296587926508442, -0.6046776061558809534, -0.2411417322834644161 ) ) ;
#4799=CARTESIAN_POINT ( 'NONE',  ( 1.371391076115485719, -0.5511811023622048555, -0.09757992244046775898 ) ) ;
#4800=CARTESIAN_POINT ( 'NONE',  ( 1.148293963254593875, -0.6692913385826771977, 0.1292274648535927661 ) ) ;
#4802=CARTESIAN_POINT ( 'NONE',  ( 0.3871391076115493490, -0.2845877964562159024, 0.3641732283464567677 ) ) ;
#4803=CARTESIAN_POINT ( 'NONE',  ( 0.5118110236220480003, -0.6692913385826771977, 8.415575281601705876E-17 ) ) ;
#4805=CARTESIAN_POINT ( 'NONE',  ( 0.9448818897637802916, -0.1870078740157479769, 0.3641732283464567677 ) ) ;
#4807=CARTESIAN_POINT ( 'NONE',  ( -1.279527559055116948, 0.1660481256975883668, -0.3530559997133364547 ) ) ;
#4808=EDGE_CURVE ( 'NONE', #31839, #73164, #12686, .T. ) ;
#4809=CARTESIAN_POINT ( 'NONE',  ( -0.7939632545931750718, -0.05778040916215560624, -0.4822834645669293319 ) ) ;
#4810=CARTESIAN_POINT ( 'NONE',  ( -0.2755905511811018171, 0.2952755905511811885, 0.000000000000000000 ) ) ;
#4813=CARTESIAN_POINT ( 'NONE',  ( 0.3215223097112867578, -0.05778040916215522460, 0.4822834645669289988 ) ) ;
#4814=CARTESIAN_POINT ( 'NONE',  ( 1.607611548556431069, 0.1771653543307087630, 0.09757992244046791164 ) ) ;
#4815=CARTESIAN_POINT ( 'NONE',  ( 0.2230971128608932319, -0.4281496062992124485, 0.4176697321401328655 ) ) ;
#4816=CARTESIAN_POINT ( 'NONE',  ( 0.9645669291338588858, 0.1660481256975885056, 0.3530559997133364547 ) ) ;
#4822=CARTESIAN_POINT ( 'NONE',  ( -0.5380577427821514602, -0.3690944881889765550, -0.3153832671262227771 ) ) ;
#4823=CARTESIAN_POINT ( 'NONE',  ( -0.8464566929133852113, -0.5400638737290845981, -0.3530559997133363437 ) ) ;
#4824=CARTESIAN_POINT ( 'NONE',  ( 0.2952755905511816326, -0.5400638737290844871, 0.3530559997133364547 ) ) ;
#4826=CARTESIAN_POINT ( 'NONE',  ( 0.9317585301837276734, 0.05413385826771626580, -0.4176697321401330321 ) ) ;
#4828=CARTESIAN_POINT ( 'NONE',  ( 1.496062992125984703, -0.1870078740157480879, -0.4822834645669291653 ) ) ;
#4829=CARTESIAN_POINT ( 'NONE',  ( 1.167979002624672580, 0.05413385826771626580, -0.4176697321401330321 ) ) ;
#4832=DIRECTION ( 'NONE',  ( 1.000000000000000000, -0.000000000000000000, -0.000000000000000000 ) ) ;
#4833=VECTOR ( 'NONE', #62107, 39.37007874015748143 ) ;
#4836=CARTESIAN_POINT ( 'NONE',  ( 0.8595800524934390507, -0.05778040916215560624, -0.4822834645669293319 ) ) ;
#4837=CARTESIAN_POINT ( 'NONE',  ( 0.7020997375328090762, -0.05778040916215560624, -0.4822834645669293319 ) ) ;
#4838=CARTESIAN_POINT ( 'NONE',  ( 1.194225721784777594, -0.3690944881889765550, -0.3153832671262227771 ) ) ;
#4839=CARTESIAN_POINT ( 'NONE',  ( 1.653543307086614789, -0.1870078740157479769, 0.4822834645669291653 ) ) ;
#4840=CARTESIAN_POINT ( 'NONE',  ( 1.581364829396326277, -0.05778040916215522460, 0.4822834645669289988 ) ) ;
#4842=DIRECTION ( 'NONE',  ( -0.000000000000000000, 1.000000000000000000, -0.000000000000000000 ) ) ;
#4843=CARTESIAN_POINT ( 'NONE',  ( 0.6824146981627303710, -0.6046776061558807314, 0.2411417322834647770 ) ) ;
#4844=CARTESIAN_POINT ( 'NONE',  ( 1.450131233595801428, -0.5511811023622048555, -0.09757992244046775898 ) ) ;
#4845=CARTESIAN_POINT ( 'NONE',  ( -0.3215223097112853146, -0.3162353388693405765, 0.4822834645669290543 ) ) ;
#4846=CARTESIAN_POINT ( 'NONE',  ( -0.4527559055118102749, 0.1660481256975885056, 0.3530559997133364547 ) ) ;
#4847=CARTESIAN_POINT ( 'NONE',  ( -1.627296587926508442, 0.2306618581243848609, 0.2411417322834645549 ) ) ;
#4851=CARTESIAN_POINT ( 'NONE',  ( 1.574803149606299746, -0.1870078740157480879, -0.4822834645669291653 ) ) ;
#4852=ORIENTED_EDGE ( 'NONE', *, *, #13917, .T. ) ;
#4857=CARTESIAN_POINT ( 'NONE',  ( 1.548556430446194954, -0.5023911411419708095, 0.1820866141732285504 ) ) ;
#4862=CARTESIAN_POINT ( 'NONE',  ( 0.4556364816766638737, 1.768811104025900249, 0.5309055118110234117 ) ) ;
#4864=CARTESIAN_POINT ( 'NONE',  ( -0.5446194225721777693, -0.08942795157527998196, 0.3641732283464567121 ) ) ;
#4865=CARTESIAN_POINT ( 'NONE',  ( -1.318897637795274802, -0.4536011799217368745, -0.2665933059059886201 ) ) ;
#4867=CARTESIAN_POINT ( 'NONE',  ( 0.6036745406824153282, -0.6046776061558807314, 0.2411417322834647770 ) ) ;
#4868=CARTESIAN_POINT ( 'NONE',  ( -1.161417322834644716, 0.1660481256975885056, 0.3530559997133364547 ) ) ;
#4870=ORIENTED_EDGE ( 'NONE', *, *, #2252, .F. ) ;
#4871=CARTESIAN_POINT ( 'NONE',  ( 1.351706036745407458, -0.4281496062992127816, -0.4176697321401328100 ) ) ;
#4875=FACE_OUTER_BOUND ( 'NONE', #5056, .T. ) ;
#4876=CARTESIAN_POINT ( 'NONE',  ( -0.5708661417322825615, -0.4536011799217367080, 0.2665933059059888421 ) ) ;
#4878=CARTESIAN_POINT ( 'NONE',  ( -0.9645669291338575535, 0.1660481256975883668, -0.3530559997133364547 ) ) ;
#4879=CARTESIAN_POINT ( 'NONE',  ( 1.148293963254593875, -0.6692913385826771977, 0.1292274648535927661 ) ) ;
#4881=CARTESIAN_POINT ( 'NONE',  ( 0.7545931758530189937, 0.2952755905511810219, -0.1292274648535930437 ) ) ;
#4882=CARTESIAN_POINT ( 'NONE',  ( 0.6758530183727039509, 0.2066929133858267098, -0.1054918080437494132 ) ) ;
#4883=CARTESIAN_POINT ( 'NONE',  ( 1.666666666666667185, 0.05413385826771666132, 0.4176697321401328100 ) ) ;
#4884=CARTESIAN_POINT ( 'NONE',  ( -1.030183727034119867, -0.05778040916215560624, -0.4822834645669293319 ) ) ;
#4886=CARTESIAN_POINT ( 'NONE',  ( 0.1312335958005255154, -0.5023911411419708095, 0.1820866141732285504 ) ) ;
#4888=CARTESIAN_POINT ( 'NONE',  ( -0.2034120734908128059, 0.1771653543307087630, 0.09757992244046791164 ) ) ;
#4889=CARTESIAN_POINT ( 'NONE',  ( 0.4199475065616803948, -0.5023911411419708095, -0.1820866141732282451 ) ) ;
#4890=CARTESIAN_POINT ( 'NONE',  ( 0.6496062992125991586, 0.1660481256975885056, 0.3530559997133364547 ) ) ;
#4891=CARTESIAN_POINT ( 'NONE',  ( -0.9120734908136475250, -0.5511811023622048555, -0.09757992244046775898 ) ) ;
#4893=CARTESIAN_POINT ( 'NONE',  ( 1.410761154855643795, -0.3162353388693405765, 0.4822834645669290543 ) ) ;
#4896=CARTESIAN_POINT ( 'NONE',  ( -0.9711286089238838626, 0.2306618581243847221, -0.2411417322834647770 ) ) ;
#4900=CARTESIAN_POINT ( 'NONE',  ( 0.1640419947506569498, -0.05778040916215522460, 0.4822834645669289988 ) ) ;
#4901=CARTESIAN_POINT ( 'NONE',  ( -0.6824146981627288167, 0.2306618581243848609, 0.2411417322834645549 ) ) ;
#4902=CARTESIAN_POINT ( 'NONE',  ( 1.259842519685040019, -0.1870078740157480601, -0.3641732283464567677 ) ) ;
#4903=CARTESIAN_POINT ( 'NONE',  ( 0.09842519685039434474, -0.4536011799217368745, -0.2665933059059886201 ) ) ;
#4904=CARTESIAN_POINT ( 'NONE',  ( -0.1049868766404193215, 0.2306618581243847221, -0.2411417322834647770 ) ) ;
#4905=CARTESIAN_POINT ( 'NONE',  ( -1.056430446194224881, -0.6692913385826771977, 0.1292274648535927661 ) ) ;
#4906=CARTESIAN_POINT ( 'NONE',  ( 1.614173228346456712, 2.401574803149606474, 0.1372047244094478646 ) ) ;
#4908=CARTESIAN_POINT ( 'NONE',  ( -0.1246719160104980823, -0.6692913385826773087, -0.1292274648535924053 ) ) ;
#4911=( BOUNDED_CURVE ( )  B_SPLINE_CURVE ( 3, ( #22328, #47991, #39286, #67369 ),
 .UNSPECIFIED., .F., .F. ) 
 B_SPLINE_CURVE_WITH_KNOTS ( ( 4, 4 ),
 ( 1.859270518042427600, 2.743397753083149926 ),
 .UNSPECIFIED. ) 
 CURVE ( )  GEOMETRIC_REPRESENTATION_ITEM ( )  RATIONAL_B_SPLINE_CURVE ( ( 1.000000000000000000, 0.9359138408343250504, 0.9359138408343250504, 1.000000000000000000 ) ) 
 REPRESENTATION_ITEM ( '' )  );
#4912=EDGE_CURVE ( 'NONE', #71641, #53395, #37929, .T. ) ;
#4913=CARTESIAN_POINT ( 'NONE',  ( 1.312335958005249825, 0.2306618581243847221, -0.2411417322834647770 ) ) ;
#4914=CARTESIAN_POINT ( 'NONE',  ( -0.5052493438320203589, -0.5511811023622046335, 0.09757992244046803654 ) ) ;
#4915=AXIS2_PLACEMENT_3D ( 'NONE', #67213, #9546, #29312 ) ;
#4916=CARTESIAN_POINT ( 'NONE',  ( -0.6167979002624665030, 0.05413385826771666132, 0.4176697321401328100 ) ) ;
#4917=CARTESIAN_POINT ( 'NONE',  ( 1.161417322834646493, -0.5400638737290844871, 0.3530559997133364547 ) ) ;
#4918=CARTESIAN_POINT ( 'NONE',  ( 1.082677165354331228, 0.1660481256975883668, -0.3530559997133364547 ) ) ;
#4919=CARTESIAN_POINT ( 'NONE',  ( -1.574803149606298192, -0.1870078740157480879, -0.4822834645669291653 ) ) ;
#4920=CARTESIAN_POINT ( 'NONE',  ( -1.207349081364828880, 0.1283753931104746893, -0.1820866141732285504 ) ) ;
#4926=CARTESIAN_POINT ( 'NONE',  ( 0.6364829396325465405, -0.08942795157527998196, 0.3641732283464567121 ) ) ;
#4927=CARTESIAN_POINT ( 'NONE',  ( 0.3346456692913390985, 0.1660481256975885056, 0.3530559997133364547 ) ) ;
#4930=CARTESIAN_POINT ( 'NONE',  ( 0.8530183727034128527, -0.3690944881889763329, 0.3153832671262228327 ) ) ;
#4931=CARTESIAN_POINT ( 'NONE',  ( -0.4199475065616791736, -0.6046776061558807314, 0.2411417322834647770 ) ) ;
#4932=CARTESIAN_POINT ( 'NONE',  ( -0.7086614173228339419, -0.1870078740157479769, 0.4822834645669291653 ) ) ;
#4933=CARTESIAN_POINT ( 'NONE',  ( 1.187664041994751285, -0.05778040916215522460, 0.4822834645669289988 ) ) ;
#4937=CARTESIAN_POINT ( 'NONE',  ( -0.2559055118110230564, 0.07958543189024071263, -0.2665933059059888421 ) ) ;
#4941=CARTESIAN_POINT ( 'NONE',  ( -0.6889763779527552368, -0.5400638737290845981, -0.3530559997133363437 ) ) ;
#4942=CARTESIAN_POINT ( 'NONE',  ( -0.2887139107611542133, -0.6046776061558809534, -0.2411417322834644161 ) ) ;
#4943=CARTESIAN_POINT ( 'NONE',  ( -0.2690288713910754526, -0.6692913385826771977, 0.1292274648535927661 ) ) ;
#4944=CARTESIAN_POINT ( 'NONE',  ( 0.5708661417322842269, 0.1660481256975885056, 0.3530559997133364547 ) ) ;
#4945=CARTESIAN_POINT ( 'NONE',  ( -0.5052493438320203589, 0.2952755905511810774, -0.1292274648535930714 ) ) ;
#4946=CARTESIAN_POINT ( 'NONE',  ( -1.469816272965878357, 0.2306618581243848609, 0.2411417322834645549 ) ) ;
#4947=CARTESIAN_POINT ( 'NONE',  ( -0.8202099737532801971, -0.6692913385826771977, 0.1292274648535927661 ) ) ;
#4948=CARTESIAN_POINT ( 'NONE',  ( 0.8136482939632553313, 0.2306618581243848609, 0.2411417322834645549 ) ) ;
#4950=CARTESIAN_POINT ( 'NONE',  ( -0.5708661417322825615, -0.4536011799217367080, 0.2665933059059888421 ) ) ;
#4955=CARTESIAN_POINT ( 'NONE',  ( -1.423884514435694859, -0.2845877964562159024, 0.3641732283464567677 ) ) ;
#4957=CARTESIAN_POINT ( 'NONE',  ( -1.049868766404198794, -0.6046776061558807314, 0.2411417322834647770 ) ) ;
#4958=CARTESIAN_POINT ( 'NONE',  ( -0.9580052493438311334, 0.05413385826771626580, -0.4176697321401330321 ) ) ;
#4960=CARTESIAN_POINT ( 'NONE',  ( -0.9055118110236215490, 0.2952755905511811885, 0.000000000000000000 ) ) ;
#4961=CARTESIAN_POINT ( 'NONE',  ( -0.7020997375328076329, -0.3162353388693409650, -0.4822834645669289433 ) ) ;
#4963=EDGE_CURVE ( 'NONE', #3706, #81247, #78485, .T. ) ;
#4965=CARTESIAN_POINT ( 'NONE',  ( 0.6430446194225729606, -0.3690944881889765550, -0.3153832671262227771 ) ) ;
#4968=CARTESIAN_POINT ( 'NONE',  ( 0.1771653543307093182, 0.07958543189024085140, 0.2665933059059887866 ) ) ;
#4969=CARTESIAN_POINT ( 'NONE',  ( -0.5774278215223089816, -0.6046776061558807314, 0.2411417322834647770 ) ) ;
#4972=CARTESIAN_POINT ( 'NONE',  ( -0.09842519685039295696, -0.5400638737290844871, 0.3530559997133364547 ) ) ;
#4975=CARTESIAN_POINT ( 'NONE',  ( -0.8398950131233585692, 0.1539470093639523085, 0.1968503937007873850 ) ) ;
#4976=VERTEX_POINT ( 'NONE', #50140 ) ;
#4978=CARTESIAN_POINT ( 'NONE',  ( 1.555118110236221041, -0.5400638737290844871, 0.3530559997133364547 ) ) ;
#4979=CARTESIAN_POINT ( 'NONE',  ( -1.338582677165353729, -0.1870078740157480601, -0.3641732283464567677 ) ) ;
#4980=CARTESIAN_POINT ( 'NONE',  ( -0.8727034120734901146, -0.05778040916215560624, -0.4822834645669293319 ) ) ;
#4984=CARTESIAN_POINT ( 'NONE',  ( 1.450131233595801428, -0.6692913385826773087, -0.1292274648535924053 ) ) ;
#4985=CARTESIAN_POINT ( 'NONE',  ( 0.2493438320209980519, -0.4281496062992127816, -0.4176697321401328100 ) ) ;
#4986=CARTESIAN_POINT ( 'NONE',  ( 0.3740157480314966754, -0.5400638737290844871, 0.3530559997133364547 ) ) ;
#4987=CARTESIAN_POINT ( 'NONE',  ( -1.246719160104985846, -0.3690944881889765550, -0.3153832671262227771 ) ) ;
#4988=CARTESIAN_POINT ( 'NONE',  ( -0.4790026246719154557, -0.3162353388693405765, 0.4822834645669290543 ) ) ;
#4990=CARTESIAN_POINT ( 'NONE',  ( -0.8530183727034112984, -0.4281496062992127816, -0.4176697321401328100 ) ) ;
#4992=CARTESIAN_POINT ( 'NONE',  ( 1.410761154855643795, -0.2845877964562159024, 0.3641732283464567677 ) ) ;
#4993=CARTESIAN_POINT ( 'NONE',  ( -0.2099737532808391705, -0.5023911411419708095, -0.1820866141732282451 ) ) ;
#4994=CARTESIAN_POINT ( 'NONE',  ( 1.095800524934383846, -0.08942795157528024563, -0.3641732283464568787 ) ) ;
#4995=CARTESIAN_POINT ( 'NONE',  ( -1.443569553805773564, -0.6046776061558807314, 0.2411417322834647770 ) ) ;
#4996=CARTESIAN_POINT ( 'NONE',  ( -1.240157480314959759, -0.4536011799217368745, -0.2665933059059886201 ) ) ;
#4997=CARTESIAN_POINT ( 'NONE',  ( 0.9348729704079946634, -8.644661201599092366E-16, -0.4445507791589066171 ) ) ;
#4998=CARTESIAN_POINT ( 'NONE',  ( 0.4133858267716541968, 0.07958543189024085140, 0.2665933059059887866 ) ) ;
#4999=CARTESIAN_POINT ( 'NONE',  ( -0.4986876640419939388, 0.2306618581243847221, -0.2411417322834647770 ) ) ;
#5001=CARTESIAN_POINT ( 'NONE',  ( -0.05249343832020911260, 0.1283753931104748280, 0.1820866141732283561 ) ) ;
#5002=CARTESIAN_POINT ( 'NONE',  ( -1.732283464566928277, -0.1870078740157479769, 0.3641732283464567677 ) ) ;
#5003=CARTESIAN_POINT ( 'NONE',  ( 0.6036745406824154392, 0.2306618581243847221, -0.2411417322834647770 ) ) ;
#5005=CARTESIAN_POINT ( 'NONE',  ( 1.423884514435696191, -0.08942795157527998196, 0.3641732283464567121 ) ) ;
#5006=CARTESIAN_POINT ( 'NONE',  ( -1.115485564304461219, -0.4281496062992124485, 0.4176697321401328655 ) ) ;
#5007=CARTESIAN_POINT ( 'NONE',  ( -0.08530183727034056085, -0.2845877964562159024, 0.3641732283464567677 ) ) ;
#5009=CARTESIAN_POINT ( 'NONE',  ( 0.3215223097112867578, -0.08942795157527998196, 0.3641732283464567121 ) ) ;
#5010=CARTESIAN_POINT ( 'NONE',  ( -1.332020997375327642, -0.3162353388693409650, -0.4822834645669289433 ) ) ;
#5011=CARTESIAN_POINT ( 'NONE',  ( -0.4068241469816264999, -0.4281496062992124485, 0.4176697321401328655 ) ) ;
#5015=CARTESIAN_POINT ( 'NONE',  ( 0.4527559055118117182, -0.4536011799217367080, 0.2665933059059888421 ) ) ;
#5016=CARTESIAN_POINT ( 'NONE',  ( -0.3215223097112853146, -0.05778040916215560624, -0.4822834645669293319 ) ) ;
#5018=CARTESIAN_POINT ( 'NONE',  ( -0.7152230971128602510, -0.3162353388693405765, 0.4822834645669290543 ) ) ;
#5019=CARTESIAN_POINT ( 'NONE',  ( -0.7545931758530176614, -0.5511811023622048555, -0.09757992244046775898 ) ) ;
#5021=CARTESIAN_POINT ( 'NONE',  ( -0.07874015748031421014, -0.1870078740157479769, 0.4822834645669291653 ) ) ;
#5022=CARTESIAN_POINT ( 'NONE',  ( -1.102362204724408601, -0.1870078740157479769, 0.3641732283464567677 ) ) ;
#5023=CARTESIAN_POINT ( 'NONE',  ( -1.587926509186350810, 0.05413385826771626580, -0.4176697321401330321 ) ) ;
#5026=CARTESIAN_POINT ( 'NONE',  ( -1.548556430446193399, 0.1283753931104748280, 0.1820866141732283561 ) ) ;
#5027=CARTESIAN_POINT ( 'NONE',  ( -1.233595800524933894, 0.2306618581243848609, 0.2411417322834645549 ) ) ;
#5028=CARTESIAN_POINT ( 'NONE',  ( -0.7152230971128602510, -0.05778040916215560624, -0.4822834645669293319 ) ) ;
#5029=CARTESIAN_POINT ( 'NONE',  ( -1.417322834645668772, -0.1870078740157480879, -0.4822834645669291653 ) ) ;
#5032=CARTESIAN_POINT ( 'NONE',  ( 1.076115485564305141, 0.2306618581243847221, -0.2411417322834647770 ) ) ;
#5033=CARTESIAN_POINT ( 'NONE',  ( 0.5511811023622055217, -0.1870078740157479769, 0.4822834645669291653 ) ) ;
#5036=CARTESIAN_POINT ( 'NONE',  ( 1.128608923884514947, 0.1283753931104748280, 0.1820866141732283561 ) ) ;
#5039=CARTESIAN_POINT ( 'NONE',  ( -0.7414698162729651543, -0.5511811023622046335, 0.09757992244046803654 ) ) ;
#5042=CARTESIAN_POINT ( 'NONE',  ( 0.4658792650918640033, -0.3162353388693405765, 0.4822834645669290543 ) ) ;
#5043=CARTESIAN_POINT ( 'NONE',  ( -0.7414698162729651543, 0.2952755905511810774, -0.1292274648535930714 ) ) ;
#5044=CARTESIAN_POINT ( 'NONE',  ( -1.043307086614172041, -0.5400638737290844871, 0.3530559997133364547 ) ) ;
#5045=CARTESIAN_POINT ( 'NONE',  ( 0.9514435695538062676, -0.3162353388693409650, -0.4822834645669289433 ) ) ;
#5046=CARTESIAN_POINT ( 'NONE',  ( 1.666666666666667185, 0.05413385826771666132, 0.4176697321401328100 ) ) ;
#5048=CARTESIAN_POINT ( 'NONE',  ( -0.2099737532808391705, 0.2306618581243848609, 0.2411417322834645549 ) ) ;
#5049=CARTESIAN_POINT ( 'NONE',  ( -1.377952755905511140, -0.6692913385826771977, 8.415575281601705876E-17 ) ) ;
#5051=CARTESIAN_POINT ( 'NONE',  ( 1.601049868766404982, -0.6046776061558809534, -0.2411417322834644161 ) ) ;
#5053=CARTESIAN_POINT ( 'NONE',  ( 0.8136482939632553313, -0.5023911411419708095, -0.1820866141732282451 ) ) ;
#5056=EDGE_LOOP ( 'NONE', ( #31226, #15117, #67513, #8693 ) ) ;
#5057=CARTESIAN_POINT ( 'NONE',  ( 0.1181102362204730916, -0.5511811023622047445, 6.969142054262312111E-17 ) ) ;
#5058=CARTESIAN_POINT ( 'NONE',  ( -1.489501312335957062, -0.3162353388693409650, -0.4822834645669289433 ) ) ;
#5059=CARTESIAN_POINT ( 'NONE',  ( 0.5577427821522314977, -0.3162353388693409650, -0.4822834645669289433 ) ) ;
#5060=CARTESIAN_POINT ( 'NONE',  ( 0.5314960629921264834, 0.1660481256975883668, -0.3530559997133364547 ) ) ;
#5062=CARTESIAN_POINT ( 'NONE',  ( -0.5708661417322828946, 0.1660481256975883668, -0.3530559997133364547 ) ) ;
#5064=CARTESIAN_POINT ( 'NONE',  ( -1.240157480314959759, -0.5400638737290845981, -0.3530559997133363437 ) ) ;
#5066=CARTESIAN_POINT ( 'NONE',  ( 1.476377952755906220, 0.07958543189024071263, -0.2665933059059888421 ) ) ;
#5067=CARTESIAN_POINT ( 'NONE',  ( -0.9973753280839886548, 0.2306618581243848609, 0.2411417322834645549 ) ) ;
#5068=CARTESIAN_POINT ( 'NONE',  ( 0.8661417322834653598, -0.1870078740157479769, 0.4822834645669291653 ) ) ;
#5069=CARTESIAN_POINT ( 'NONE',  ( 1.345144356955381593, -0.05778040916215522460, 0.4822834645669289988 ) ) ;
#5071=CARTESIAN_POINT ( 'NONE',  ( -1.535433070866141225, 0.2952755905511811885, 0.000000000000000000 ) ) ;
#5073=CARTESIAN_POINT ( 'NONE',  ( 0.4461942257217855201, -0.6046776061558807314, 0.2411417322834647770 ) ) ;
#5076=CARTESIAN_POINT ( 'NONE',  ( -1.515748031496062076, -0.4536011799217367080, 0.2665933059059888421 ) ) ;
#5077=CARTESIAN_POINT ( 'NONE',  ( 0.4133858267716541968, 0.07958543189024085140, 0.2665933059059887866 ) ) ;
#5078=CARTESIAN_POINT ( 'NONE',  ( 0.7742782152230978099, -0.4281496062992124485, 0.4176697321401328655 ) ) ;
#5080=CARTESIAN_POINT ( 'NONE',  ( 0.6692913385826778638, -0.5511811023622047445, 6.969142054262312111E-17 ) ) ;
#5081=CARTESIAN_POINT ( 'NONE',  ( 0.3346456692913390985, 0.1660481256975885056, 0.3530559997133364547 ) ) ;
#5083=CARTESIAN_POINT ( 'NONE',  ( -0.8005249343832013809, -0.4281496062992124485, 0.4176697321401328655 ) ) ;
#5086=CARTESIAN_POINT ( 'NONE',  ( 0.8989501312335963501, -0.5511811023622048555, -0.09757992244046775898 ) ) ;
#5087=CARTESIAN_POINT ( 'NONE',  ( -0.1509186351706028884, -0.05778040916215522460, 0.4822834645669289988 ) ) ;
#5088=CARTESIAN_POINT ( 'NONE',  ( -1.115485564304461219, 0.05413385826771626580, -0.4176697321401330321 ) ) ;
#5089=CARTESIAN_POINT ( 'NONE',  ( -0.1509186351706028884, -0.05778040916215522460, 0.4822834645669289988 ) ) ;
#5090=CARTESIAN_POINT ( 'NONE',  ( 0.05905511811023709395, -0.4536011799217367080, 0.2665933059059888421 ) ) ;
#5092=CARTESIAN_POINT ( 'NONE',  ( -0.4593175853018366950, 0.05413385826771666132, 0.4176697321401328100 ) ) ;
#5093=CARTESIAN_POINT ( 'NONE',  ( 0.6102362204724416372, -0.4536011799217367080, 0.2665933059059888421 ) ) ;
#5094=CARTESIAN_POINT ( 'NONE',  ( 1.604771003085129433, 1.320215725944020813, 0.1466069496707751441 ) ) ;
#5096=CARTESIAN_POINT ( 'NONE',  ( 0.3346456692913393205, -0.5400638737290845981, -0.3530559997133363437 ) ) ;
#5097=( BOUNDED_CURVE ( )  B_SPLINE_CURVE ( 2, ( #2336, #73030, #14139, #47340, #40212, #8230, #65053, #78951, #14965, #53652, #21269, #9064, #65486 ),
 .UNSPECIFIED., .F., .F. ) 
 B_SPLINE_CURVE_WITH_KNOTS ( ( 3, 2, 2, 2, 2, 2, 3 ),
 ( 0.1740332660251417696, 0.1742424242424242542, 0.1780303030303030387, 0.1818181818181818232, 0.1856060606060606077, 0.1893939393939393923, 0.1896030976112218769 ),
 .UNSPECIFIED. ) 
 CURVE ( )  GEOMETRIC_REPRESENTATION_ITEM ( )  RATIONAL_B_SPLINE_CURVE ( ( 0.9964447847208424136, 0.9981185001348094055, 1.000000000000000000, 0.9659258262890683122, 1.000000000000000000, 0.9659258262890683122, 1.000000000000000000, 0.9659258262890683122, 1.000000000000000000, 0.9659258262890683122, 1.000000000000000000, 0.9981185001348095165, 0.9964447847208426357 ) ) 
 REPRESENTATION_ITEM ( '' )  );
#5098=CARTESIAN_POINT ( 'NONE',  ( 1.338582677165355062, -0.1870078740157479769, 0.3641732283464567677 ) ) ;
#5099=DIRECTION ( 'NONE',  ( -1.000000000000000000, -3.469446951953613696E-16, 0.000000000000000000 ) ) ;
#5100=CARTESIAN_POINT ( 'NONE',  ( -0.3280839895013117347, -0.3690944881889763329, 0.3153832671262228327 ) ) ;
#5101=CARTESIAN_POINT ( 'NONE',  ( -0.9383202099737524282, -0.08942795157527998196, 0.3641732283464567121 ) ) ;
#5102=CARTESIAN_POINT ( 'NONE',  ( -0.3412073490813641308, 0.2306618581243847221, -0.2411417322834647770 ) ) ;
#5103=CARTESIAN_POINT ( 'NONE',  ( 0.2034120734908142214, 0.2952755905511810774, -0.1292274648535930714 ) ) ;
#5104=CARTESIAN_POINT ( 'NONE',  ( 1.108923884514436686, -0.2845877964562161244, -0.3641732283464567121 ) ) ;
#5106=CARTESIAN_POINT ( 'NONE',  ( 1.548556430446194954, -0.5023911411419708095, 0.1820866141732285504 ) ) ;
#5107=CARTESIAN_POINT ( 'NONE',  ( 0.7283464566929143125, 0.1660481256975885056, 0.3530559997133364547 ) ) ;
#5109=CARTESIAN_POINT ( 'NONE',  ( 0.1246719160104994284, -0.6692913385826771977, 0.1292274648535927661 ) ) ;
#5111=CARTESIAN_POINT ( 'NONE',  ( 0.9842519685039378130, -0.6692913385826771977, 8.415575281601705876E-17 ) ) ;
#5112=CARTESIAN_POINT ( 'NONE',  ( 0.6036745406824154392, 0.2306618581243847221, -0.2411417322834647770 ) ) ;
#5114=CARTESIAN_POINT ( 'NONE',  ( 0.3346456692913393205, -0.4536011799217368745, -0.2665933059059886201 ) ) ;
#5115=CARTESIAN_POINT ( 'NONE',  ( 1.305774278215223960, -0.6692913385826771977, 0.1292274648535927661 ) ) ;
#5116=CARTESIAN_POINT ( 'NONE',  ( 0.2952755905511816326, -0.4536011799217367080, 0.2665933059059888421 ) ) ;
#5117=CARTESIAN_POINT ( 'NONE',  ( -0.4527559055118102749, -0.5400638737290845981, -0.3530559997133363437 ) ) ;
#5118=CARTESIAN_POINT ( 'NONE',  ( 0.4330708661417329575, -0.6692913385826771977, 8.415575281601705876E-17 ) ) ;
#5119=CARTESIAN_POINT ( 'NONE',  ( -0.6102362204724400829, -0.5400638737290845981, -0.3530559997133363437 ) ) ;
#5120=CARTESIAN_POINT ( 'NONE',  ( -0.2624671916010490880, 0.1283753931104746893, -0.1820866141732285504 ) ) ;
#5121=CARTESIAN_POINT ( 'NONE',  ( 0.4461942257217855201, -0.6046776061558807314, 0.2411417322834647770 ) ) ;
#5122=CARTESIAN_POINT ( 'NONE',  ( 0.9383202099737538715, -0.08942795157528024563, -0.3641732283464568787 ) ) ;
#5123=CARTESIAN_POINT ( 'NONE',  ( -0.2624671916010490880, -0.6046776061558807314, 0.2411417322834647770 ) ) ;
#5127=CARTESIAN_POINT ( 'NONE',  ( 1.541994750656168645, 0.2952755905511810774, -0.1292274648535930714 ) ) ;
#5130=CARTESIAN_POINT ( 'NONE',  ( -1.167979002624671470, 0.05413385826771666132, 0.4176697321401328100 ) ) ;
#5131=CARTESIAN_POINT ( 'NONE',  ( -0.9120734908136475250, 0.2952755905511811885, 0.1292274648535926551 ) ) ;
#5135=CARTESIAN_POINT ( 'NONE',  ( 0.3280839895013130669, -0.3690944881889765550, -0.3153832671262227771 ) ) ;
#5137=CARTESIAN_POINT ( 'NONE',  ( 0.7020997375328090762, -0.05778040916215560624, -0.4822834645669293319 ) ) ;
#5139=CARTESIAN_POINT ( 'NONE',  ( 0.9776902887139113929, 0.2952755905511811885, 0.1292274648535926551 ) ) ;
#5140=CARTESIAN_POINT ( 'NONE',  ( -1.673228346456691717, 0.07958543189024071263, -0.2665933059059888421 ) ) ;
#5141=CARTESIAN_POINT ( 'NONE',  ( 1.253280839895013710, -0.05778040916215560624, -0.4822834645669293319 ) ) ;
#5142=CARTESIAN_POINT ( 'NONE',  ( 1.292650918635171564, 0.1771653543307087630, 0.09757992244046791164 ) ) ;
#5143=CARTESIAN_POINT ( 'NONE',  ( 0.05249343832021075018, -0.6046776061558807314, 0.2411417322834647770 ) ) ;
#5145=CARTESIAN_POINT ( 'NONE',  ( -0.5052493438320203589, 0.2952755905511810774, -0.1292274648535930714 ) ) ;
#5146=CARTESIAN_POINT ( 'NONE',  ( -1.233595800524933894, 0.1283753931104748280, 0.1820866141732283561 ) ) ;
#5147=ADVANCED_FACE ( 'NONE', ( #18584 ), #53, .F. ) ;
#5148=CARTESIAN_POINT ( 'NONE',  ( -0.4265091863517051496, 0.2952755905511810774, -0.1292274648535930714 ) ) ;
#5149=CARTESIAN_POINT ( 'NONE',  ( 1.601049868766404982, -0.6046776061558809534, -0.2411417322834644161 ) ) ;
#5150=DIRECTION ( 'NONE',  ( 1.000000000000000000, 0.000000000000000000, -1.692413147294446216E-16 ) ) ;
#5153=CARTESIAN_POINT ( 'NONE',  ( 0.3674540682414705883, -0.6046776061558807314, 0.2411417322834647770 ) ) ;
#5155=CARTESIAN_POINT ( 'NONE',  ( -0.2690288713910754526, 0.2952755905511810774, -0.1292274648535930714 ) ) ;
#5156=CARTESIAN_POINT ( 'NONE',  ( -1.561679790026246017, -0.4281496062992127816, -0.4176697321401328100 ) ) ;
#5157=CARTESIAN_POINT ( 'NONE',  ( 0.6167979002624678353, -0.4281496062992124485, 0.4176697321401328655 ) ) ;
#5159=CARTESIAN_POINT ( 'NONE',  ( 0.09842519685039434474, 0.1660481256975885056, 0.3530559997133364547 ) ) ;
#5161=CARTESIAN_POINT ( 'NONE',  ( -0.8070866141732276899, -0.5400638737290844871, 0.3530559997133364547 ) ) ;
#5162=CARTESIAN_POINT ( 'NONE',  ( 0.08530183727034192087, -0.05778040916215522460, 0.4822834645669289988 ) ) ;
#5163=CARTESIAN_POINT ( 'NONE',  ( -0.2559055118110227234, -0.5400638737290844871, 0.3530559997133364547 ) ) ;
#5164=CARTESIAN_POINT ( 'NONE',  ( 0.3805774278215230400, -0.3690944881889763329, 0.3153832671262228327 ) ) ;
#5166=CARTESIAN_POINT ( 'NONE',  ( -0.2887139107611542133, 0.2306618581243848609, 0.2411417322834645549 ) ) ;
#5168=CARTESIAN_POINT ( 'NONE',  ( -1.568241469816272105, -0.3162353388693409650, -0.4822834645669289433 ) ) ;
#5170=VERTEX_POINT ( 'NONE', #18179 ) ;
#5172=CARTESIAN_POINT ( 'NONE',  ( 0.9055118110236227702, 0.2952755905511811885, 0.000000000000000000 ) ) ;
#5173=CARTESIAN_POINT ( 'NONE',  ( 0.3018372703412079971, -0.3690944881889763329, 0.3153832671262228327 ) ) ;
#5175=CARTESIAN_POINT ( 'NONE',  ( 2.795275590551181910, 1.568468489416428469, 0.000000000000000000 ) ) ;
#5180=CARTESIAN_POINT ( 'NONE',  ( 0.5314960629921264834, 0.1660481256975883668, -0.3530559997133364547 ) ) ;
#5181=CARTESIAN_POINT ( 'NONE',  ( -1.299212598425196097, 0.2952755905511811885, 0.000000000000000000 ) ) ;
#5182=CARTESIAN_POINT ( 'NONE',  ( -1.030183727034119867, -0.05778040916215560624, -0.4822834645669293319 ) ) ;
#5183=CARTESIAN_POINT ( 'NONE',  ( 0.4461942257217855201, -0.6046776061558807314, 0.2411417322834647770 ) ) ;
#5184=CARTESIAN_POINT ( 'NONE',  ( 1.154855643044620184, 0.2306618581243847221, -0.2411417322834647770 ) ) ;
#5185=CARTESIAN_POINT ( 'NONE',  ( 1.227034120734908917, 0.1771653543307087075, -0.09757992244046823083 ) ) ;
#5186=CARTESIAN_POINT ( 'NONE',  ( 1.292650918635171564, -0.5511811023622048555, -0.09757992244046775898 ) ) ;
#5187=CARTESIAN_POINT ( 'NONE',  ( -0.6561679790026240244, 0.2306618581243847221, -0.2411417322834647770 ) ) ;
#5189=CARTESIAN_POINT ( 'NONE',  ( 1.548556430446194954, 0.2306618581243847221, -0.2411417322834647770 ) ) ;
#5191=CARTESIAN_POINT ( 'NONE',  ( -0.2493438320209966919, -0.4281496062992124485, 0.4176697321401328655 ) ) ;
#5192=CARTESIAN_POINT ( 'NONE',  ( 0.9973753280839902091, -0.6046776061558807314, 0.2411417322834647770 ) ) ;
#5194=CARTESIAN_POINT ( 'NONE',  ( -1.561679790026246017, -0.004921259842519576551, 0.3153832671262227771 ) ) ;
#5195=CARTESIAN_POINT ( 'NONE',  ( 0.2493438320209980519, 0.05413385826771666132, 0.4176697321401328100 ) ) ;
#5196=CARTESIAN_POINT ( 'NONE',  ( 0.7939632545931766261, -0.08942795157527998196, 0.3641732283464567121 ) ) ;
#5198=CARTESIAN_POINT ( 'NONE',  ( -1.587926509186350810, -0.3690944881889763329, 0.3153832671262228327 ) ) ;
#5199=CARTESIAN_POINT ( 'NONE',  ( 0.8005249343832028242, -0.4281496062992127816, -0.4176697321401328100 ) ) ;
#5201=CARTESIAN_POINT ( 'NONE',  ( -0.4921259842519677963, -0.4536011799217367080, 0.2665933059059888421 ) ) ;
#5202=CARTESIAN_POINT ( 'NONE',  ( -0.4199475065616791736, 0.2306618581243847221, -0.2411417322834647770 ) ) ;
#5203=CARTESIAN_POINT ( 'NONE',  ( 1.555118110236221041, 0.1660481256975883668, -0.3530559997133364547 ) ) ;
#5204=CARTESIAN_POINT ( 'NONE',  ( -1.128608923884513837, -0.6046776061558807314, 0.2411417322834647770 ) ) ;
#5205=CARTESIAN_POINT ( 'NONE',  ( 1.325459317585302665, -0.4281496062992124485, 0.4176697321401328655 ) ) ;
#5207=CARTESIAN_POINT ( 'NONE',  ( -0.9842519685039360366, 0.1771653543307087630, 0.000000000000000000 ) ) ;
#5209=CARTESIAN_POINT ( 'NONE',  ( 1.338582677165355062, -0.1870078740157480879, -0.4822834645669291653 ) ) ;
#5212=CARTESIAN_POINT ( 'NONE',  ( -1.417322834645668772, -0.1870078740157480601, -0.3641732283464567677 ) ) ;
#5213=CARTESIAN_POINT ( 'NONE',  ( -0.9120734908136475250, 0.1771653543307087630, 0.09757992244046791164 ) ) ;
#5214=CARTESIAN_POINT ( 'NONE',  ( 1.601049868766404982, -0.5023911411419708095, -0.1820866141732282451 ) ) ;
#5215=CARTESIAN_POINT ( 'NONE',  ( -0.3871391076115476282, -0.05778040916215522460, 0.4822834645669289988 ) ) ;
#5216=CARTESIAN_POINT ( 'NONE',  ( 0.1706036745406830368, -0.3690944881889765550, -0.3153832671262227771 ) ) ;
#5217=CARTESIAN_POINT ( 'NONE',  ( -1.181102362204723644, -0.1870078740157480601, -0.3641732283464567677 ) ) ;
#5218=CARTESIAN_POINT ( 'NONE',  ( 1.450131233595801428, 0.1771653543307087630, 0.09757992244046791164 ) ) ;
#5219=CARTESIAN_POINT ( 'NONE',  ( 1.082677165354331228, 0.1660481256975883668, -0.3530559997133364547 ) ) ;
#5220=CARTESIAN_POINT ( 'NONE',  ( 1.522309711286089939, -0.6046776061558809534, -0.2411417322834644161 ) ) ;
#5221=CARTESIAN_POINT ( 'NONE',  ( 0.4921259842519691285, -0.4536011799217368745, -0.2665933059059886201 ) ) ;
#5222=EDGE_CURVE ( 'NONE', #4446, #39863, #37318, .T. ) ;
#5223=CARTESIAN_POINT ( 'NONE',  ( 0.6561679790026253567, -0.6046776061558809534, -0.2411417322834644161 ) ) ;
#5224=CARTESIAN_POINT ( 'NONE',  ( 0.8005249343832027131, -0.004921259842519576551, 0.3153832671262227771 ) ) ;
#5226=CARTESIAN_POINT ( 'NONE',  ( -1.213910761154854745, -0.6692913385826771977, 0.1292274648535927661 ) ) ;
#5227=CARTESIAN_POINT ( 'NONE',  ( -1.450131233595799651, 0.2952755905511810774, -0.1292274648535930714 ) ) ;
#5228=CARTESIAN_POINT ( 'NONE',  ( -0.07874015748031421014, -0.1870078740157480879, -0.4822834645669291653 ) ) ;
#5231=CARTESIAN_POINT ( 'NONE',  ( 0.4855643044619428750, 0.05413385826771666132, 0.4176697321401328100 ) ) ;
#5232=CARTESIAN_POINT ( 'NONE',  ( 1.207349081364829990, -0.5023911411419708095, -0.1820866141732282451 ) ) ;
#5233=CARTESIAN_POINT ( 'NONE',  ( 0.07874015748031558404, -0.1870078740157479769, 0.4822834645669291653 ) ) ;
#5234=CARTESIAN_POINT ( 'NONE',  ( 0.2821522309711292364, -0.6692913385826771977, 0.1292274648535927661 ) ) ;
#5240=CARTESIAN_POINT ( 'NONE',  ( -0.4724409448818890911, -0.1870078740157479769, 0.3641732283464567677 ) ) ;
#5241=CARTESIAN_POINT ( 'NONE',  ( -0.5511811023622041894, -0.1870078740157480879, -0.4822834645669291653 ) ) ;
#5242=CARTESIAN_POINT ( 'NONE',  ( 0.5511811023622054106, -0.1870078740157480879, -0.4822834645669291653 ) ) ;
#5244=CARTESIAN_POINT ( 'NONE',  ( 0.9251968503937015864, 0.1660481256975883668, -0.3530559997133364547 ) ) ;
#5245=CARTESIAN_POINT ( 'NONE',  ( -1.482939632545930975, 0.05413385826771666132, 0.4176697321401328100 ) ) ;
#5246=CARTESIAN_POINT ( 'NONE',  ( 0.8989501312335963501, -0.6692913385826773087, -0.1292274648535924053 ) ) ;
#5249=CARTESIAN_POINT ( 'NONE',  ( -0.7478466213799872531, 2.204724409448818978, 0.5309055118110236338 ) ) ;
#5250=CARTESIAN_POINT ( 'NONE',  ( 1.017060367454068581, -0.05778040916215560624, -0.4822834645669293319 ) ) ;
#5251=CARTESIAN_POINT ( 'NONE',  ( 0.4199475065616803948, -0.6046776061558809534, -0.2411417322834644161 ) ) ;
#5252=CARTESIAN_POINT ( 'NONE',  ( 1.030183727034121421, -0.2845877964562161244, -0.3641732283464567121 ) ) ;
#5253=CARTESIAN_POINT ( 'NONE',  ( 1.601049868766404982, -0.6046776061558809534, -0.2411417322834644161 ) ) ;
#5254=CARTESIAN_POINT ( 'NONE',  ( 1.292650918635171564, 0.2952755905511811885, 0.1292274648535926551 ) ) ;
#5257=CARTESIAN_POINT ( 'NONE',  ( 0.9908136482939640111, -0.6692913385826771977, 0.1292274648535927661 ) ) ;
#5258=CARTESIAN_POINT ( 'NONE',  ( 1.561679790026247350, -0.004921259842519870586, -0.3153832671262229437 ) ) ;
#5259=CARTESIAN_POINT ( 'NONE',  ( -0.3740157480314953431, -0.5400638737290845981, -0.3530559997133363437 ) ) ;
#5260=CARTESIAN_POINT ( 'NONE',  ( -1.023622047244094002, -0.1870078740157480879, -0.4822834645669291653 ) ) ;
#5261=CARTESIAN_POINT ( 'NONE',  ( 1.003937007874016185, 0.1660481256975883668, -0.3530559997133364547 ) ) ;
#5265=CARTESIAN_POINT ( 'NONE',  ( -1.535433070866141225, -0.5511811023622047445, 6.969142054262312111E-17 ) ) ;
#5268=ORIENTED_EDGE ( 'NONE', *, *, #46085, .F. ) ;
#5269=CARTESIAN_POINT ( 'NONE',  ( -0.7330049731600569718, 2.221336660396575624, -0.5178675056770626339 ) ) ;
#5270=CARTESIAN_POINT ( 'NONE',  ( 1.528871391076116026, -0.5511811023622048555, -0.09757992244046775898 ) ) ;
#5272=CARTESIAN_POINT ( 'NONE',  ( 1.522309711286089939, 0.1283753931104748280, 0.1820866141732283561 ) ) ;
#5274=B_SPLINE_CURVE_WITH_KNOTS ( 'NONE', 3,
 ( #19374, #45024, #11838, #70725, #82944, #17745, #36664 ),
 .UNSPECIFIED., .F., .F.,
 ( 4, 3, 4 ),
 ( 5.204170427930421283E-18, 0.001246230184515548971, 0.002492489877932633786 ),
 .UNSPECIFIED. ) ;
#5279=CARTESIAN_POINT ( 'NONE',  ( -0.6561679790026240244, 0.1283753931104746893, -0.1820866141732285504 ) ) ;
#5280=CARTESIAN_POINT ( 'NONE',  ( -1.325459317585300889, -0.3690944881889765550, -0.3153832671262227771 ) ) ;
#5281=CARTESIAN_POINT ( 'NONE',  ( -1.108923884514435132, -0.05778040916215560624, -0.4822834645669293319 ) ) ;
#5282=CARTESIAN_POINT ( 'NONE',  ( -0.006561679790025524116, -0.3162353388693405765, 0.4822834645669290543 ) ) ;
#5283=CARTESIAN_POINT ( 'NONE',  ( -1.167979002624671470, 0.05413385826771666132, 0.4176697321401328100 ) ) ;
#5285=EDGE_CURVE ( 'NONE', #1651, #39863, #70298, .T. ) ;
#5286=CARTESIAN_POINT ( 'NONE',  ( 1.358267716535433323, -0.5400638737290845981, -0.3530559997133363437 ) ) ;
#5290=DIRECTION ( 'NONE',  ( 0.000000000000000000, -1.000000000000000000, 0.000000000000000000 ) ) ;
#5291=CARTESIAN_POINT ( 'NONE',  ( -0.4330708661417315697, -0.5511811023622047445, 6.969142054262312111E-17 ) ) ;
#5292=EDGE_CURVE ( 'NONE', #18339, #58371, #78937, .T. ) ;
#5293=CARTESIAN_POINT ( 'NONE',  ( -1.233595800524933894, -0.6046776061558809534, -0.2411417322834644161 ) ) ;
#5294=CARTESIAN_POINT ( 'NONE',  ( 1.062992125984252745, 0.2952755905511811885, 0.000000000000000000 ) ) ;
#5300=CARTESIAN_POINT ( 'NONE',  ( -1.082677165354329896, 0.1660481256975885056, 0.3530559997133364547 ) ) ;
#5302=CARTESIAN_POINT ( 'NONE',  ( -0.1509186351706028884, -0.08942795157527998196, 0.3641732283464567121 ) ) ;
#5304=CARTESIAN_POINT ( 'NONE',  ( -0.5774278215223089816, -0.5023911411419708095, 0.1820866141732285504 ) ) ;
#5305=CARTESIAN_POINT ( 'NONE',  ( 0.6102362204724416372, -0.4536011799217367080, 0.2665933059059888421 ) ) ;
#5306=CARTESIAN_POINT ( 'NONE',  ( 0.7086614173228352742, -0.1870078740157480879, -0.4822834645669291653 ) ) ;
#5307=CARTESIAN_POINT ( 'NONE',  ( -0.5446194225721777693, -0.08942795157527998196, 0.3641732283464567121 ) ) ;
#5309=CARTESIAN_POINT ( 'NONE',  ( 1.036745406824147508, -0.4281496062992127816, -0.4176697321401328100 ) ) ;
#5311=CARTESIAN_POINT ( 'NONE',  ( -1.115485564304461219, 0.05413385826771626580, -0.4176697321401330321 ) ) ;
#5313=CARTESIAN_POINT ( 'NONE',  ( -0.07874015748031421014, -0.1870078740157480879, -0.4822834645669291653 ) ) ;
#5314=CARTESIAN_POINT ( 'NONE',  ( -0.4593175853018364174, -0.4281496062992127816, -0.4176697321401328100 ) ) ;
#5315=CARTESIAN_POINT ( 'NONE',  ( 1.220472440944882608, 0.1771653543307087630, 0.000000000000000000 ) ) ;
#5316=CARTESIAN_POINT ( 'NONE',  ( 0.04593175853018440641, 0.1771653543307087075, -0.09757992244046823083 ) ) ;
#5317=CARTESIAN_POINT ( 'NONE',  ( -0.03280839895013062252, -0.6692913385826771977, 0.1292274648535927661 ) ) ;
#5318=CARTESIAN_POINT ( 'NONE',  ( -1.181102362204723644, -0.1870078740157479769, 0.4822834645669291653 ) ) ;
#5319=CARTESIAN_POINT ( 'NONE',  ( -0.7535225988626923499, 2.401574803149606474, 0.4915354330708645025 ) ) ;
#5320=CARTESIAN_POINT ( 'NONE',  ( 1.541994750656168645, 0.1771653543307087075, -0.09757992244046823083 ) ) ;
#5321=CARTESIAN_POINT ( 'NONE',  ( -0.1181102362204717315, -0.6692913385826771977, 8.415575281601705876E-17 ) ) ;
#5322=CARTESIAN_POINT ( 'NONE',  ( -1.305774278215222184, -0.6692913385826773087, -0.1292274648535924053 ) ) ;
#5323=ORIENTED_EDGE ( 'NONE', *, *, #31050, .F. ) ;
#5325=CARTESIAN_POINT ( 'NONE',  ( 1.023622047244095112, -0.1870078740157480879, -0.4822834645669291653 ) ) ;
#5326=CARTESIAN_POINT ( 'NONE',  ( -0.7217847769028863381, -0.004921259842519870586, -0.3153832671262229437 ) ) ;
#5327=CARTESIAN_POINT ( 'NONE',  ( -0.6627296587926503335, -0.6692913385826771977, 0.1292274648535927661 ) ) ;
#5328=CARTESIAN_POINT ( 'NONE',  ( 1.181102362204725198, -0.1870078740157479769, 0.4822834645669291653 ) ) ;
#5329=CARTESIAN_POINT ( 'NONE',  ( 1.095800524934383846, -0.05778040916215560624, -0.4822834645669293319 ) ) ;
#5331=CARTESIAN_POINT ( 'NONE',  ( -0.9317585301837263412, -0.004921259842519576551, 0.3153832671262227771 ) ) ;
#5336=CARTESIAN_POINT ( 'NONE',  ( 1.095800524934383846, -0.08942795157528024563, -0.3641732283464568787 ) ) ;
#5337=CARTESIAN_POINT ( 'NONE',  ( 0.5577427821522314977, -0.2845877964562161244, -0.3641732283464567121 ) ) ;
#5338=CARTESIAN_POINT ( 'NONE',  ( 0.6167979002624678353, -0.4281496062992124485, 0.4176697321401328655 ) ) ;
#5339=CARTESIAN_POINT ( 'NONE',  ( 1.594488188976378673, 0.1660481256975885056, 0.3530559997133364547 ) ) ;
#5341=CARTESIAN_POINT ( 'NONE',  ( 0.8858267716535438430, 0.07958543189024085140, 0.2665933059059887866 ) ) ;
#5342=CARTESIAN_POINT ( 'NONE',  ( -0.1115485564304453947, -0.6692913385826771977, 0.1292274648535927661 ) ) ;
#5343=CARTESIAN_POINT ( 'NONE',  ( -1.062992125984250968, -0.6692913385826771977, 8.415575281601705876E-17 ) ) ;
#5344=CARTESIAN_POINT ( 'NONE',  ( 1.463254593175853824, -0.6692913385826771977, 0.1292274648535927661 ) ) ;
#5347=CARTESIAN_POINT ( 'NONE',  ( 0.04593175853018440641, 0.1771653543307087075, -0.09757992244046823083 ) ) ;
#5348=ORIENTED_EDGE ( 'NONE', *, *, #39869, .F. ) ;
#5350=CARTESIAN_POINT ( 'NONE',  ( -0.9251968503937002541, 0.1660481256975885056, 0.3530559997133364547 ) ) ;
#5351=CARTESIAN_POINT ( 'NONE',  ( -0.4593175853018364174, -0.4281496062992127816, -0.4176697321401328100 ) ) ;
#5352=CARTESIAN_POINT ( 'NONE',  ( -0.2624671916010490880, -0.6046776061558807314, 0.2411417322834647770 ) ) ;
#5353=CARTESIAN_POINT ( 'NONE',  ( 0.5380577427821529035, -0.4281496062992124485, 0.4176697321401328655 ) ) ;
#5354=CARTESIAN_POINT ( 'NONE',  ( -0.2755905511811015396, -0.6692913385826771977, 8.415575281601705876E-17 ) ) ;
#5355=CARTESIAN_POINT ( 'NONE',  ( -1.338582677165353729, -0.1870078740157479769, 0.4822834645669291653 ) ) ;
#5356=CARTESIAN_POINT ( 'NONE',  ( -0.9908136482939626788, -0.6692913385826773087, -0.1292274648535924053 ) ) ;
#5357=CARTESIAN_POINT ( 'NONE',  ( 0.9317585301837276734, -0.4281496062992124485, 0.4176697321401328655 ) ) ;
#5358=EDGE_CURVE ( 'NONE', #35363, #59927, #28223, .T. ) ;
#5360=CARTESIAN_POINT ( 'NONE',  ( -0.3871391076115476282, -0.08942795157527998196, 0.3641732283464567121 ) ) ;
#5364=CARTESIAN_POINT ( 'NONE',  ( -1.187664041994750175, -0.08942795157528024563, -0.3641732283464568787 ) ) ;
#5365=CARTESIAN_POINT ( 'NONE',  ( -1.154855643044618851, 0.2306618581243848609, 0.2411417322834645549 ) ) ;
#5366=CARTESIAN_POINT ( 'NONE',  ( -1.030183727034119867, -0.3162353388693405765, 0.4822834645669290543 ) ) ;
#5368=CARTESIAN_POINT ( 'NONE',  ( -0.6233595800524928121, -0.05778040916215522460, 0.4822834645669289988 ) ) ;
#5369=CARTESIAN_POINT ( 'NONE',  ( -0.8267716535433065062, -0.6692913385826771977, 8.415575281601705876E-17 ) ) ;
#5372=CARTESIAN_POINT ( 'NONE',  ( 0.5314960629921267055, -0.4536011799217367080, 0.2665933059059888421 ) ) ;
#5375=CARTESIAN_POINT ( 'NONE',  ( -0.1443569553805768291, -0.004921259842519576551, 0.3153832671262227771 ) ) ;
#5376=CARTESIAN_POINT ( 'NONE',  ( -0.4199475065616791736, -0.6046776061558807314, 0.2411417322834647770 ) ) ;
#5377=CARTESIAN_POINT ( 'NONE',  ( 1.410761154855643795, -0.3162353388693405765, 0.4822834645669290543 ) ) ;
#5378=CARTESIAN_POINT ( 'NONE',  ( -0.07874015748031421014, -0.1870078740157479769, 0.4822834645669291653 ) ) ;
#5379=ORIENTED_EDGE ( 'NONE', *, *, #44186, .F. ) ;
#5381=CARTESIAN_POINT ( 'NONE',  ( -0.8136482939632537770, 0.1539470093639521697, -0.1968503937007875793 ) ) ;
#5384=CARTESIAN_POINT ( 'NONE',  ( -1.646051170424378096, 0.000000000000000000, -0.3464511005275205946 ) ) ;
#5385=CARTESIAN_POINT ( 'NONE',  ( -0.9317585301837263412, -0.004921259842519576551, 0.3153832671262227771 ) ) ;
#5386=CARTESIAN_POINT ( 'NONE',  ( -1.213910761154854745, 0.2952755905511810774, -0.1292274648535930714 ) ) ;
#5390=CARTESIAN_POINT ( 'NONE',  ( 1.187664041994751285, -0.05778040916215522460, 0.4822834645669289988 ) ) ;
#5391=CARTESIAN_POINT ( 'NONE',  ( 0.2952755905511816326, -0.5400638737290844871, 0.3530559997133364547 ) ) ;
#5392=CARTESIAN_POINT ( 'NONE',  ( 0.1706036745406830368, -0.4281496062992127816, -0.4176697321401328100 ) ) ;
#5393=CARTESIAN_POINT ( 'NONE',  ( -1.023622047244093558, -0.1870078740157479769, 0.3641732283464567677 ) ) ;
#5394=CARTESIAN_POINT ( 'NONE',  ( -0.4199475065616791736, 0.2306618581243847221, -0.2411417322834647770 ) ) ;
#5396=CARTESIAN_POINT ( 'NONE',  ( -1.062992125984250968, 0.2952755905511811885, 0.000000000000000000 ) ) ;
#5398=CARTESIAN_POINT ( 'NONE',  ( 1.227034120734908917, -0.5511811023622046335, 0.09757992244046803654 ) ) ;
#5399=CARTESIAN_POINT ( 'NONE',  ( -0.3674540682414692561, -0.5023911411419708095, -0.1820866141732282451 ) ) ;
#5400=CARTESIAN_POINT ( 'NONE',  ( 1.082677165354331228, 0.07958543189024071263, -0.2665933059059888421 ) ) ;
#5401=CARTESIAN_POINT ( 'NONE',  ( -1.594488188976377563, -0.5400638737290844871, 0.3530559997133364547 ) ) ;
#5402=CARTESIAN_POINT ( 'NONE',  ( -1.036745406824146176, -0.3690944881889763329, 0.3153832671262228327 ) ) ;
#5403=CARTESIAN_POINT ( 'NONE',  ( 0.4849061582275022153, 1.726086921369708538, 0.4921425059946342717 ) ) ;
#5404=CARTESIAN_POINT ( 'NONE',  ( 0.5446194225721792126, -0.2845877964562159024, 0.3641732283464567677 ) ) ;
#5405=CARTESIAN_POINT ( 'NONE',  ( -0.6955380577427815458, 0.05413385826771666132, 0.4176697321401328100 ) ) ;
#5406=( BOUNDED_SURFACE ( )  B_SPLINE_SURFACE ( 1, 2, ( 
 ( #56545, #77162, #58199, #12361, #64529, #64117, #6034, #5622, #11952, #6866, #24965, #19076, #37607, #31706, #5214, #57366, #83061, #25382, #13202, #76746, #71265, #82246, #50231, #63282, #32122, #31288, #57780, #56953, #567, #82650, #144, #25799, #32535, #51460, #51883, #19922, #45572, #13612, #50637, #76341, #70006, #65383, #14459, #7718, #40528, #72929, #52718, #40111, #39692, #64948, #46407, #47239, #1403, #71683, #59875, #60296, #21577, #14866, #46826, #53965, #53554, #27475, #34632, #8958, #15280, #33386, #40941, #66207, #21171, #72518, #59049, #66620, #2646, #8546, #20335, #15699, #28303, #78844, #72101, #53133, #59462, #2229, #47655, #34212, #27059, #78429, #79677, #992, #21994, #73351, #7288, #65798, #26647, #27894, #20757, #32958, #45987, #79262, #58625, #52301, #78007, #8132, #14035, #33797, #1813, #22413, #61538, #4691, #41752, #74180, #67447, #16941, #49308, #29135, #16527, #16108, #41356, #22821, #23638, #61117, #48070, #36275, #36677, #81324, #74598, #23226, #30365, #29949, #3883, #11021, #68679, #75009, #9781, #17356, #42582, #80913, #48896, #35452, #42984, #62353, #68283, #80093, #75416, #56032, #55205, #48479, #29543, #35872, #61947, #24049, #10618, #3469, #54802, #81740, #60705, #49720, #67037, #9369, #73772, #80506, #35040, #3054, #28720, #54383, #42171, #67866, #10203, #4287, #55613, #37506, #82547, #18973, #11853, #58095, #77058, #70744, #11439, #5928, #37095, #31600, #69504, #25694, #460, #24460, #24866, #26116, #13096, #82145, #51777, #43800, #37916, #50126, #51355, #6760, #38331, #43391, #6348, #38749, #50534, #19391, #57260, #18572, #18167, #30781, #45043, #63181, #82959, #5114, #76238, #17760, #44215, #69905, #12259, #57679, #25277, #69091, #62780, #56442, #64426, #44622, #75826, #5519, #32432, #50945, #63593, #76642, #70317, #64007, #31185, #12672, #56849, #32019, #41, #13504, #40837, #34532, #72830, #888, #39588, #59773, #2128, #66522, #39160, #65277, #52619, #15180, #26546, #45466, #13931, #58949, #78745, #71580, #60197, #53456, #47139, #71164, #65703, #64845, #8033, #45882, #27796, #2548, #52199, #1307, #28206, #8854, #58523, #77482, #20234, #14359, #77903, #79164, #19817, #14769, #7183, #66106, #32854, #26956, #21481, #33696, #78325, #7616, #33288, #20656, #46309, #59357, #72003, #40016, #1716, #27371, #53032, #21070, #34112, #46728, #72420, #40425, #8442, #4595, #3370, #73249, #42073, #79998, #49209, #34947, #67768, #74497, #36176, #10104, #61019, #3785, #16844, #29853, #60610, #74081, #17259, #54282, #29034, #22312, #29448, #61849, #41662, #54705, #28624, #53865, #35357, #4190, #73674, #2959, #48799, #74913, #10522, #55107, #35768, #42887, #42478, #16427, #23540, #81224, #55516, #47975, #68582, #80816, #61438, #23131, #16016, #10923, #68183, #36580, #67353, #62259, #79577, #21893, #47556, #15598, #41258, #9686, #66944, #9276, #80411, #22723, #48382, #13722, #12464, #18775, #65061, #30266, #70113, #32644, #6557, #70528, #70957, #20447, #7399, #65493, #76448, #50748, #19598, #44830, #674, #39799, #6138, #76848, #51153, #64638, #64223, #32229, #26750, #82752, #58309, #19181, #44418, #12883, #6975, #77269, #57887, #38126, #31813, #20025, #25906, #55930, #13302, #25487, #63800, #57473, #46100, #45676, #77695, #254, #83167, #1099, #25074, #38543, #45261, #51566, #26328, #38954, #51990, #71372, #71793, #39376, #33067, #58737, #52405, #78114, #14146, #46932, #15815, #46514, #78958, #60404, #2755, #47349, #73038, #41049, #52827, #66313, #33903, #53660, #9073, #20864, #28414, #8652, #66734, #21686, #72216, #65901, #59567, #34744, #2344, #34323, #8237, #54074, #53243, #14972, #72624, #15387, #21277, #79789, #14567, #1923, #59985, #40219, #28000, #79367, #40631, #22105, #47765, #73463, #41464, #35153, #67149, #59154, #9478, #27586, #7825, #33492, #27165, #1511, #78539, #966, #77133, #40085, #59022, #52690, #76714, #71239, #19047, #13583, #51430, #7692, #65772, #6422, #6837, #8104, #78398, #64085, #33770, #25769, #19894, #32091, #33359, #72074, #20308, #25353, #71655, #20730, #32507, #1378, #39237, #539, #114 ),
 ( #44694, #83030, #58170, #70391, #64922, #19466, #46381, #57752, #7260, #45958, #65354, #32932, #26192, #58597, #14007, #27029, #45116, #45541, #14433, #70824, #51853, #13171, #26620, #51015, #38821, #77560, #64499, #12746, #52274, #38405, #77978, #39664, #54358, #54778, #16084, #9346, #41333, #48454, #48047, #21969, #29108, #3444, #67423, #59849, #41729, #35017, #15672, #67013, #34185, #9756, #80481, #60681, #14840, #10179, #35428, #73325, #66596, #47631, #53940, #80070, #42145, #3030, #21552, #2201, #61093, #78816, #22794, #16501, #74154, #66181, #47213, #67840, #59431, #1786, #21145, #72903, #34607, #8930, #27446, #53107, #46800, #72491, #79652, #40500, #2622, #15255, #73748, #28696, #8518, #22387, #27869, #53529, #79237, #40914, #60272, #28278, #68812, #64147, #49445, #76773, #30505, #75139, #17890, #62910, #82679, #75551, #38461, #57399, #51074, #17484, #69636, #43115, #11982, #49851, #6063, #6481, #4826, #5244, #32151, #19105, #62492, #81457, #24182, #18298, #56167, #31734, #70449, #18703, #23774, #70036, #44753, #30908, #83090, #37636, #82276, #81870, #11158, #25411, #43527, #63313, #36817, #56575, #69226, #24594, #50262, #75960, #38047, #5651, #11573, #37232, #43942, #31317, #56982, #24996, #50671, #76370, #12807, #44345, #12390, #63723, #40139, #46016, #64980, #7747, #78456, #33822, #38879, #78034, #21196, #58227, #7316, #594, #33412, #65824, #45599, #32985, #32565, #57807, #39294, #8157, #77616, #64558, #52748, #53160, #14485, #59074, #39718, #46850, #46436, #20364, #27503, #1842, #59488, #26250, #78871, #1429, #14064, #65409, #51909, #72545, #14892, #27085, #13229, #8571, #40552, #58653, #66233, #71710, #173, #25827, #51486, #77189, #1020, #19521, #20781, #19949, #45174, #6895, #72127, #70880, #71293, #13641, #26673, #52328, #54833, #10234, #15307, #54412, #80943, #34662, #67065, #60325, #9810, #42200, #22023, #9397, #8989, #34241, #15728, #16556, #53995, #40970, #29164, #29574, #74210, #67476, #16137, #23258, #22850, #80123, #3913, #61570, #67896, #2674, #35901, #35482, #73801, #41783, #28333, #55237, #48928, #61146, #72956, #68312, #74628, #48102, #41384, #22442, #28750, #80538, #16972, #3498, #79707, #47683, #42612, #53579, #59903, #2255, #27920, #66652, #73378, #79288, #21606, #35068, #47266, #60734, #3086, #48510, #43017, #61980, #30396, #75451, #11886, #4722, #50976, #69937, #63626, #4317, #82178, #29982, #24494, #62385, #18605, #76674, #17386, #17789, #19006, #5963, #75040, #44655, #36710, #30810, #68711, #44248, #82991, #31218, #36304, #82579, #31633, #43424, #12293, #50161, #11470, #11052, #23668, #37949, #56062, #75857, #81356, #69121, #10649, #37127, #62811, #81771, #24898, #5145, #55645, #18199, #24081, #49340, #49751, #25312, #50567, #56886, #56475, #43834, #57293, #69536, #37538, #63214, #5554, #76271, #51388, #52235, #38782, #1750, #33323, #46342, #1340, #77938, #8069, #45077, #45501, #59392, #77093, #77517, #78360, #52654, #13968, #39625, #58985, #75, #7219, #6796, #20268, #26991, #19425, #20691, #32890, #72036, #65314, #70780, #13131, #32467, #14392, #26582, #58559, #64459, #40050, #51812, #39197, #71198, #7653, #19852, #65736, #25728, #58129, #925, #496, #45918, #71616, #13541, #64880, #33731, #27407, #53068, #21104, #78779, #64041, #70351, #26151, #12706, #38365, #6380, #32052, #57712, #35390, #10139, #35803, #3818, #60231, #54739, #53900, #16460, #22347, #80028, #29068, #27829, #34147, #80444, #46762, #2163, #48007, #21930, #2581, #2992, #61470, #22754, #80849, #8478, #66140, #34978, #28240, #16046, #55138, #21515, #8889, #66556, #73706, #79613, #47591, #42105, #14804, #41692, #34566, #59808, #73285, #67385, #9308, #15633, #53489, #9719, #41290, #79199, #67802, #72455, #40462, #60642, #47174, #61055, #72865, #28658, #15214, #29479, #3405, #48414, #74114, #54317, #40874, #66975, #81677, #12195, #4221, #30298, #31119, #5457, #50065, #75760, #69439, #36211, #43322, #42919, #56382, #37445, #29885, #56786, #69022, #11792, #18102, #55548, #49243, #68614, #63119, #62712, #11373, #74946, #82486, #4627, #75346, #23988, #43735 ) ),
 .UNSPECIFIED., .F., .F., .F. ) 
 B_SPLINE_SURFACE_WITH_KNOTS ( ( 2, 2 ),
 ( 3, 2, 2, 2, 2, 2, 2, 2, 2, 2, 2, 2, 2, 2, 2, 2, 2, 2, 2, 2, 2, 2, 2, 2, 2, 2, 2, 2, 2, 2, 2, 2, 2, 2, 2, 2, 2, 2, 2, 2, 2, 2, 2, 2, 2, 2, 2, 2, 2, 2, 2, 2, 2, 2, 2, 2, 2, 2, 2, 2, 2, 2, 2, 2, 2, 2, 2, 2, 2, 2, 2, 2, 2, 2, 2, 2, 2, 2, 2, 2, 2, 2, 2, 2, 2, 2, 2, 2, 2, 2, 2, 2, 2, 2, 2, 2, 2, 2, 2, 2, 2, 2, 2, 2, 2, 2, 2, 2, 2, 2, 2, 2, 2, 2, 2, 2, 2, 2, 2, 2, 2, 2, 2, 2, 2, 2, 2, 2, 2, 2, 2, 2, 2, 2, 2, 2, 2, 2, 2, 2, 2, 2, 2, 2, 2, 2, 2, 2, 2, 2, 2, 2, 2, 2, 2, 2, 2, 2, 2, 2, 2, 2, 2, 2, 2, 2, 2, 2, 2, 2, 2, 2, 2, 2, 2, 2, 2, 2, 2, 2, 2, 2, 2, 2, 2, 2, 2, 2, 2, 2, 2, 2, 2, 2, 2, 2, 2, 2, 2, 2, 2, 2, 2, 2, 2, 2, 2, 2, 2, 2, 2, 2, 2, 2, 2, 2, 2, 2, 2, 2, 2, 2, 2, 2, 2, 2, 2, 2, 2, 2, 2, 2, 2, 2, 2, 2, 2, 2, 2, 2, 2, 2, 2, 2, 2, 2, 2, 2, 2, 2, 2, 2, 2, 2, 2, 3 ),
 ( 0.000000000000000000, 1.000000000000000000 ),
 ( 0.000000000000000000, 0.003787878787878787984, 0.007575757575757575968, 0.01136363636363636395, 0.01515151515151515194, 0.01893939393939393992, 0.02272727272727272790, 0.02651515151515151589, 0.03030303030303030387, 0.03409090909090908839, 0.03787878787878787984, 0.04166666666666666435, 0.04545454545454545581, 0.04924242424242424032, 0.05303030303030303177, 0.05681818181818181629, 0.06060606060606060774, 0.06439393939393939226, 0.06818181818181817677, 0.07196969696969697516, 0.07575757575757575968, 0.07954545454545454419, 0.08333333333333332871, 0.08712121212121212710, 0.09090909090909091161, 0.09469696969696969613, 0.09848484848484848064, 0.1022727272727272790, 0.1060606060606060635, 0.1098484848484848481, 0.1136363636363636326, 0.1174242424242424310, 0.1212121212121212155, 0.1250000000000000000, 0.1287878787878787845, 0.1325757575757575690, 0.1363636363636363535, 0.1401515151515151381, 0.1439393939393939503, 0.1477272727272727348, 0.1515151515151515194, 0.1553030303030303039, 0.1590909090909090884, 0.1628787878787878729, 0.1666666666666666574, 0.1704545454545454419, 0.1742424242424242542, 0.1780303030303030387, 0.1818181818181818232, 0.1856060606060606077, 0.1893939393939393923, 0.1931818181818181768, 0.1969696969696969613, 0.2007575757575757458, 0.2045454545454545581, 0.2083333333333333426, 0.2121212121212121271, 0.2159090909090909116, 0.2196969696969696961, 0.2234848484848484806, 0.2272727272727272652, 0.2310606060606060497, 0.2348484848484848619, 0.2386363636363636465, 0.2424242424242424310, 0.2462121212121212155, 0.2500000000000000000, 0.2537878787878787845, 0.2575757575757575690, 0.2613636363636363535, 0.2651515151515151381, 0.2689393939393939226, 0.2727272727272727071, 0.2765151515151514916, 0.2803030303030302761, 0.2840909090909091161, 0.2878787878787879007, 0.2916666666666666852, 0.2954545454545454697, 0.2992424242424242542, 0.3030303030303030387, 0.3068181818181818232, 0.3106060606060606077, 0.3143939393939393923, 0.3181818181818181768, 0.3219696969696969613, 0.3257575757575757458, 0.3295454545454545303, 0.3333333333333333148, 0.3371212121212120993, 0.3409090909090908839, 0.3446969696969697239, 0.3484848484848485084, 0.3522727272727272929, 0.3560606060606060774, 0.3598484848484848619, 0.3636363636363636465, 0.3674242424242424310, 0.3712121212121212155, 0.3750000000000000000, 0.3787878787878787845, 0.3825757575757575690, 0.3863636363636363535, 0.3901515151515151381, 0.3939393939393939226, 0.3977272727272727071, 0.4015151515151514916, 0.4053030303030302761, 0.4090909090909091161, 0.4128787878787879007, 0.4166666666666666852, 0.4204545454545454697, 0.4242424242424242542, 0.4280303030303030387, 0.4318181818181818232, 0.4356060606060606077, 0.4393939393939393923, 0.4431818181818181768, 0.4469696969696969613, 0.4507575757575757458, 0.4545454545454545303, 0.4583333333333333148, 0.4621212121212120993, 0.4659090909090908839, 0.4696969696969697239, 0.4734848484848485084, 0.4772727272727272929, 0.4810606060606060774, 0.4848484848484848619, 0.4886363636363636465, 0.4924242424242424310, 0.4962121212121212155, 0.5000000000000000000, 0.5037878787878787845, 0.5075757575757575690, 0.5113636363636363535, 0.5151515151515151381, 0.5189393939393939226, 0.5227272727272727071, 0.5265151515151514916, 0.5303030303030302761, 0.5340909090909090606, 0.5378787878787878451, 0.5416666666666666297, 0.5454545454545454142, 0.5492424242424241987, 0.5530303030303029832, 0.5568181818181817677, 0.5606060606060605522, 0.5643939393939394478, 0.5681818181818182323, 0.5719696969696970168, 0.5757575757575758013, 0.5795454545454545858, 0.5833333333333333703, 0.5871212121212121549, 0.5909090909090909394, 0.5946969696969697239, 0.5984848484848485084, 0.6022727272727272929, 0.6060606060606060774, 0.6098484848484848619, 0.6136363636363636465, 0.6174242424242424310, 0.6212121212121212155, 0.6250000000000000000, 0.6287878787878787845, 0.6325757575757575690, 0.6363636363636363535, 0.6401515151515151381, 0.6439393939393939226, 0.6477272727272727071, 0.6515151515151514916, 0.6553030303030302761, 0.6590909090909090606, 0.6628787878787878451, 0.6666666666666666297, 0.6704545454545454142, 0.6742424242424241987, 0.6780303030303029832, 0.6818181818181817677, 0.6856060606060605522, 0.6893939393939394478, 0.6931818181818182323, 0.6969696969696970168, 0.7007575757575758013, 0.7045454545454545858, 0.7083333333333333703, 0.7121212121212121549, 0.7159090909090909394, 0.7196969696969697239, 0.7234848484848485084, 0.7272727272727272929, 0.7310606060606060774, 0.7348484848484848619, 0.7386363636363636465, 0.7424242424242424310, 0.7462121212121212155, 0.7500000000000000000, 0.7537878787878787845, 0.7575757575757575690, 0.7613636363636363535, 0.7651515151515151381, 0.7689393939393939226, 0.7727272727272727071, 0.7765151515151514916, 0.7803030303030302761, 0.7840909090909090606, 0.7878787878787878451, 0.7916666666666666297, 0.7954545454545454142, 0.7992424242424241987, 0.8030303030303029832, 0.8068181818181817677, 0.8106060606060605522, 0.8143939393939394478, 0.8181818181818182323, 0.8219696969696970168, 0.8257575757575758013, 0.8295454545454545858, 0.8333333333333333703, 0.8371212121212121549, 0.8409090909090909394, 0.8446969696969697239, 0.8484848484848485084, 0.8522727272727272929, 0.8560606060606060774, 0.8598484848484848619, 0.8636363636363636465, 0.8674242424242424310, 0.8712121212121212155, 0.8750000000000000000, 0.8787878787878787845, 0.8825757575757575690, 0.8863636363636363535, 0.8901515151515151381, 0.8939393939393939226, 0.8977272727272727071, 0.9015151515151514916, 0.9053030303030302761, 0.9090909090909090606, 0.9128787878787878451, 0.9166666666666666297, 0.9204545454545454142, 0.9242424242424241987, 0.9280303030303029832, 0.9318181818181817677, 0.9356060606060605522, 0.9393939393939394478, 0.9431818181818182323, 0.9469696969696970168, 0.9507575757575758013, 0.9545454545454545858, 0.9583333333333333703, 0.9621212121212121549, 0.9659090909090909394 ),
 .UNSPECIFIED. ) 
 GEOMETRIC_REPRESENTATION_ITEM ( )  RATIONAL_B_SPLINE_SURFACE ( (
 ( 1.000000000000000000, 0.9659258262890683122, 1.000000000000000000, 0.9659258262890683122, 1.000000000000000000, 0.9659258262890683122, 1.000000000000000000, 0.9659258262890683122, 1.000000000000000000, 0.9659258262890683122, 1.000000000000000000, 0.9659258262890683122, 1.000000000000000000, 0.9659258262890683122, 1.000000000000000000, 0.9659258262890683122, 1.000000000000000000, 0.9659258262890683122, 1.000000000000000000, 0.9659258262890683122, 1.000000000000000000, 0.9659258262890683122, 1.000000000000000000, 0.9659258262890683122, 1.000000000000000000, 0.9659258262890683122, 1.000000000000000000, 0.9659258262890683122, 1.000000000000000000, 0.9659258262890683122, 1.000000000000000000, 0.9659258262890683122, 1.000000000000000000, 0.9659258262890683122, 1.000000000000000000, 0.9659258262890683122, 1.000000000000000000, 0.9659258262890683122, 1.000000000000000000, 0.9659258262890683122, 1.000000000000000000, 0.9659258262890683122, 1.000000000000000000, 0.9659258262890683122, 1.000000000000000000, 0.9659258262890683122, 1.000000000000000000, 0.9659258262890683122, 1.000000000000000000, 0.9659258262890683122, 1.000000000000000000, 0.9659258262890683122, 1.000000000000000000, 0.9659258262890683122, 1.000000000000000000, 0.9659258262890683122, 1.000000000000000000, 0.9659258262890683122, 1.000000000000000000, 0.9659258262890683122, 1.000000000000000000, 0.9659258262890683122, 1.000000000000000000, 0.9659258262890683122, 1.000000000000000000, 0.9659258262890683122, 1.000000000000000000, 0.9659258262890683122, 1.000000000000000000, 0.9659258262890683122, 1.000000000000000000, 0.9659258262890683122, 1.000000000000000000, 0.9659258262890683122, 1.000000000000000000, 0.9659258262890683122, 1.000000000000000000, 0.9659258262890683122, 1.000000000000000000, 0.9659258262890683122, 1.000000000000000000, 0.9659258262890683122, 1.000000000000000000, 0.9659258262890683122, 1.000000000000000000, 0.9659258262890683122, 1.000000000000000000, 0.9659258262890683122, 1.000000000000000000, 0.9659258262890683122, 1.000000000000000000, 0.9659258262890683122, 1.000000000000000000, 0.9659258262890683122, 1.000000000000000000, 0.9659258262890683122, 1.000000000000000000, 0.9659258262890683122, 1.000000000000000000, 0.9659258262890683122, 1.000000000000000000, 0.9659258262890683122, 1.000000000000000000, 0.9659258262890683122, 1.000000000000000000, 0.9659258262890683122, 1.000000000000000000, 0.9659258262890683122, 1.000000000000000000, 0.9659258262890683122, 1.000000000000000000, 0.9659258262890683122, 1.000000000000000000, 0.9659258262890683122, 1.000000000000000000, 0.9659258262890683122, 1.000000000000000000, 0.9659258262890683122, 1.000000000000000000, 0.9659258262890683122, 1.000000000000000000, 0.9659258262890683122, 1.000000000000000000, 0.9659258262890683122, 1.000000000000000000, 0.9659258262890683122, 1.000000000000000000, 0.9659258262890683122, 1.000000000000000000, 0.9659258262890683122, 1.000000000000000000, 0.9659258262890683122, 1.000000000000000000, 0.9659258262890683122, 1.000000000000000000, 0.9659258262890683122, 1.000000000000000000, 0.9659258262890683122, 1.000000000000000000, 0.9659258262890683122, 1.000000000000000000, 0.9659258262890683122, 1.000000000000000000, 0.9659258262890683122, 1.000000000000000000, 0.9659258262890683122, 1.000000000000000000, 0.9659258262890683122, 1.000000000000000000, 0.9659258262890683122, 1.000000000000000000, 0.9659258262890683122, 1.000000000000000000, 0.9659258262890683122, 1.000000000000000000, 0.9659258262890683122, 1.000000000000000000, 0.9659258262890683122, 1.000000000000000000, 0.9659258262890683122, 1.000000000000000000, 0.9659258262890683122, 1.000000000000000000, 0.9659258262890683122, 1.000000000000000000, 0.9659258262890683122, 1.000000000000000000, 0.9659258262890683122, 1.000000000000000000, 0.9659258262890683122, 1.000000000000000000, 0.9659258262890683122, 1.000000000000000000, 0.9659258262890683122, 1.000000000000000000, 0.9659258262890683122, 1.000000000000000000, 0.9659258262890683122, 1.000000000000000000, 0.9659258262890683122, 1.000000000000000000, 0.9659258262890683122, 1.000000000000000000, 0.9659258262890683122, 1.000000000000000000, 0.9659258262890683122, 1.000000000000000000, 0.9659258262890683122, 1.000000000000000000, 0.9659258262890683122, 1.000000000000000000, 0.9659258262890683122, 1.000000000000000000, 0.9659258262890683122, 1.000000000000000000, 0.9659258262890683122, 1.000000000000000000, 0.9659258262890683122, 1.000000000000000000, 0.9659258262890683122, 1.000000000000000000, 0.9659258262890683122, 1.000000000000000000, 0.9659258262890683122, 1.000000000000000000, 0.9659258262890683122, 1.000000000000000000, 0.9659258262890683122, 1.000000000000000000, 0.9659258262890683122, 1.000000000000000000, 0.9659258262890683122, 1.000000000000000000, 0.9659258262890683122, 1.000000000000000000, 0.9659258262890683122, 1.000000000000000000, 0.9659258262890683122, 1.000000000000000000, 0.9659258262890683122, 1.000000000000000000, 0.9659258262890683122, 1.000000000000000000, 0.9659258262890683122, 1.000000000000000000, 0.9659258262890683122, 1.000000000000000000, 0.9659258262890683122, 1.000000000000000000, 0.9659258262890683122, 1.000000000000000000, 0.9659258262890683122, 1.000000000000000000, 0.9659258262890683122, 1.000000000000000000, 0.9659258262890683122, 1.000000000000000000, 0.9659258262890683122, 1.000000000000000000, 0.9659258262890683122, 1.000000000000000000, 0.9659258262890683122, 1.000000000000000000, 0.9659258262890683122, 1.000000000000000000, 0.9659258262890683122, 1.000000000000000000, 0.9659258262890683122, 1.000000000000000000, 0.9659258262890683122, 1.000000000000000000, 0.9659258262890683122, 1.000000000000000000, 0.9659258262890683122, 1.000000000000000000, 0.9659258262890683122, 1.000000000000000000, 0.9659258262890683122, 1.000000000000000000, 0.9659258262890683122, 1.000000000000000000, 0.9659258262890683122, 1.000000000000000000, 0.9659258262890683122, 1.000000000000000000, 0.9659258262890683122, 1.000000000000000000, 0.9659258262890683122, 1.000000000000000000, 0.9659258262890683122, 1.000000000000000000, 0.9659258262890683122, 1.000000000000000000, 0.9659258262890683122, 1.000000000000000000, 0.9659258262890683122, 1.000000000000000000, 0.9659258262890683122, 1.000000000000000000, 0.9659258262890683122, 1.000000000000000000, 0.9659258262890683122, 1.000000000000000000, 0.9659258262890683122, 1.000000000000000000, 0.9659258262890683122, 1.000000000000000000, 0.9659258262890683122, 1.000000000000000000, 0.9659258262890683122, 1.000000000000000000, 0.9659258262890683122, 1.000000000000000000, 0.9659258262890683122, 1.000000000000000000, 0.9659258262890683122, 1.000000000000000000, 0.9659258262890683122, 1.000000000000000000, 0.9659258262890683122, 1.000000000000000000, 0.9659258262890683122, 1.000000000000000000, 0.9659258262890683122, 1.000000000000000000, 0.9659258262890683122, 1.000000000000000000, 0.9659258262890683122, 1.000000000000000000, 0.9659258262890683122, 1.000000000000000000, 0.9659258262890683122, 1.000000000000000000, 0.9659258262890683122, 1.000000000000000000, 0.9659258262890683122, 1.000000000000000000, 0.9659258262890683122, 1.000000000000000000, 0.9659258262890683122, 1.000000000000000000, 0.9659258262890683122, 1.000000000000000000, 0.9659258262890683122, 1.000000000000000000, 0.9659258262890683122, 1.000000000000000000, 0.9659258262890683122, 1.000000000000000000, 0.9659258262890683122, 1.000000000000000000, 0.9659258262890683122, 1.000000000000000000, 0.9659258262890683122, 1.000000000000000000, 0.9659258262890683122, 1.000000000000000000, 0.9659258262890683122, 1.000000000000000000, 0.9659258262890683122, 1.000000000000000000, 0.9659258262890683122, 1.000000000000000000, 0.9659258262890683122, 1.000000000000000000, 0.9659258262890683122, 1.000000000000000000, 0.9659258262890683122, 1.000000000000000000, 0.9659258262890683122, 1.000000000000000000, 0.9659258262890683122, 1.000000000000000000, 0.9659258262890683122, 1.000000000000000000, 0.9659258262890683122, 1.000000000000000000, 0.9659258262890683122, 1.000000000000000000, 0.9659258262890683122, 1.000000000000000000, 0.9659258262890683122, 1.000000000000000000, 0.9659258262890683122, 1.000000000000000000, 0.9659258262890683122, 1.000000000000000000, 0.9659258262890683122, 1.000000000000000000, 0.9659258262890683122, 1.000000000000000000, 0.9659258262890683122, 1.000000000000000000, 0.9659258262890683122, 1.000000000000000000, 0.9659258262890683122, 1.000000000000000000, 0.9659258262890683122, 1.000000000000000000, 0.9659258262890683122, 1.000000000000000000, 0.9659258262890683122, 1.000000000000000000, 0.9659258262890683122, 1.000000000000000000, 0.9659258262890683122, 1.000000000000000000, 0.9659258262890683122, 1.000000000000000000, 0.9659258262890683122, 1.000000000000000000, 0.9659258262890683122, 1.000000000000000000, 0.9659258262890683122, 1.000000000000000000, 0.9659258262890683122, 1.000000000000000000, 0.9659258262890683122, 1.000000000000000000, 0.9659258262890683122, 1.000000000000000000, 0.9659258262890683122, 1.000000000000000000, 0.9659258262890683122, 1.000000000000000000, 0.9659258262890683122, 1.000000000000000000, 0.9659258262890683122, 1.000000000000000000, 0.9659258262890683122, 1.000000000000000000, 0.9659258262890683122, 1.000000000000000000, 0.9659258262890683122, 1.000000000000000000, 0.9659258262890683122, 1.000000000000000000, 0.9659258262890683122, 1.000000000000000000, 0.9659258262890683122, 1.000000000000000000, 0.9659258262890683122, 1.000000000000000000, 0.9659258262890683122, 1.000000000000000000, 0.9659258262890683122, 1.000000000000000000, 0.9659258262890683122, 1.000000000000000000, 0.9659258262890683122, 1.000000000000000000, 0.9659258262890683122, 1.000000000000000000, 0.9659258262890683122, 1.000000000000000000, 0.9659258262890683122, 1.000000000000000000, 0.9659258262890683122, 1.000000000000000000, 0.9659258262890683122, 1.000000000000000000, 0.9659258262890683122, 1.000000000000000000, 0.9659258262890683122, 1.000000000000000000, 0.9659258262890683122, 1.000000000000000000, 0.9659258262890683122, 1.000000000000000000, 0.9659258262890683122, 1.000000000000000000, 0.9659258262890683122, 1.000000000000000000, 0.9659258262890683122, 1.000000000000000000, 0.9659258262890683122, 1.000000000000000000, 0.9659258262890683122, 1.000000000000000000, 0.9659258262890683122, 1.000000000000000000, 0.9659258262890683122, 1.000000000000000000, 0.9659258262890683122, 1.000000000000000000, 0.9659258262890683122, 1.000000000000000000, 0.9659258262890683122, 1.000000000000000000, 0.9659258262890683122, 1.000000000000000000, 0.9659258262890683122, 1.000000000000000000, 0.9659258262890683122, 1.000000000000000000, 0.9659258262890683122, 1.000000000000000000, 0.9659258262890683122, 1.000000000000000000, 0.9659258262890683122, 1.000000000000000000, 0.9659258262890683122, 1.000000000000000000, 0.9659258262890683122, 1.000000000000000000, 0.9659258262890683122, 1.000000000000000000, 0.9659258262890683122, 1.000000000000000000, 0.9659258262890683122, 1.000000000000000000, 0.9659258262890683122, 1.000000000000000000, 0.9659258262890683122, 1.000000000000000000, 0.9659258262890683122, 1.000000000000000000, 0.9659258262890683122, 1.000000000000000000, 0.9659258262890683122, 1.000000000000000000, 0.9659258262890683122, 1.000000000000000000, 0.9659258262890683122, 1.000000000000000000, 0.9659258262890683122, 1.000000000000000000, 0.9659258262890683122, 1.000000000000000000, 0.9659258262890683122, 1.000000000000000000),
 ( 1.000000000000000000, 0.9659258262890683122, 1.000000000000000000, 0.9659258262890683122, 1.000000000000000000, 0.9659258262890683122, 1.000000000000000000, 0.9659258262890683122, 1.000000000000000000, 0.9659258262890683122, 1.000000000000000000, 0.9659258262890683122, 1.000000000000000000, 0.9659258262890683122, 1.000000000000000000, 0.9659258262890683122, 1.000000000000000000, 0.9659258262890683122, 1.000000000000000000, 0.9659258262890683122, 1.000000000000000000, 0.9659258262890683122, 1.000000000000000000, 0.9659258262890683122, 1.000000000000000000, 0.9659258262890683122, 1.000000000000000000, 0.9659258262890683122, 1.000000000000000000, 0.9659258262890683122, 1.000000000000000000, 0.9659258262890683122, 1.000000000000000000, 0.9659258262890683122, 1.000000000000000000, 0.9659258262890683122, 1.000000000000000000, 0.9659258262890683122, 1.000000000000000000, 0.9659258262890683122, 1.000000000000000000, 0.9659258262890683122, 1.000000000000000000, 0.9659258262890683122, 1.000000000000000000, 0.9659258262890683122, 1.000000000000000000, 0.9659258262890683122, 1.000000000000000000, 0.9659258262890683122, 1.000000000000000000, 0.9659258262890683122, 1.000000000000000000, 0.9659258262890683122, 1.000000000000000000, 0.9659258262890683122, 1.000000000000000000, 0.9659258262890683122, 1.000000000000000000, 0.9659258262890683122, 1.000000000000000000, 0.9659258262890683122, 1.000000000000000000, 0.9659258262890683122, 1.000000000000000000, 0.9659258262890683122, 1.000000000000000000, 0.9659258262890683122, 1.000000000000000000, 0.9659258262890683122, 1.000000000000000000, 0.9659258262890683122, 1.000000000000000000, 0.9659258262890683122, 1.000000000000000000, 0.9659258262890683122, 1.000000000000000000, 0.9659258262890683122, 1.000000000000000000, 0.9659258262890683122, 1.000000000000000000, 0.9659258262890683122, 1.000000000000000000, 0.9659258262890683122, 1.000000000000000000, 0.9659258262890683122, 1.000000000000000000, 0.9659258262890683122, 1.000000000000000000, 0.9659258262890683122, 1.000000000000000000, 0.9659258262890683122, 1.000000000000000000, 0.9659258262890683122, 1.000000000000000000, 0.9659258262890683122, 1.000000000000000000, 0.9659258262890683122, 1.000000000000000000, 0.9659258262890683122, 1.000000000000000000, 0.9659258262890683122, 1.000000000000000000, 0.9659258262890683122, 1.000000000000000000, 0.9659258262890683122, 1.000000000000000000, 0.9659258262890683122, 1.000000000000000000, 0.9659258262890683122, 1.000000000000000000, 0.9659258262890683122, 1.000000000000000000, 0.9659258262890683122, 1.000000000000000000, 0.9659258262890683122, 1.000000000000000000, 0.9659258262890683122, 1.000000000000000000, 0.9659258262890683122, 1.000000000000000000, 0.9659258262890683122, 1.000000000000000000, 0.9659258262890683122, 1.000000000000000000, 0.9659258262890683122, 1.000000000000000000, 0.9659258262890683122, 1.000000000000000000, 0.9659258262890683122, 1.000000000000000000, 0.9659258262890683122, 1.000000000000000000, 0.9659258262890683122, 1.000000000000000000, 0.9659258262890683122, 1.000000000000000000, 0.9659258262890683122, 1.000000000000000000, 0.9659258262890683122, 1.000000000000000000, 0.9659258262890683122, 1.000000000000000000, 0.9659258262890683122, 1.000000000000000000, 0.9659258262890683122, 1.000000000000000000, 0.9659258262890683122, 1.000000000000000000, 0.9659258262890683122, 1.000000000000000000, 0.9659258262890683122, 1.000000000000000000, 0.9659258262890683122, 1.000000000000000000, 0.9659258262890683122, 1.000000000000000000, 0.9659258262890683122, 1.000000000000000000, 0.9659258262890683122, 1.000000000000000000, 0.9659258262890683122, 1.000000000000000000, 0.9659258262890683122, 1.000000000000000000, 0.9659258262890683122, 1.000000000000000000, 0.9659258262890683122, 1.000000000000000000, 0.9659258262890683122, 1.000000000000000000, 0.9659258262890683122, 1.000000000000000000, 0.9659258262890683122, 1.000000000000000000, 0.9659258262890683122, 1.000000000000000000, 0.9659258262890683122, 1.000000000000000000, 0.9659258262890683122, 1.000000000000000000, 0.9659258262890683122, 1.000000000000000000, 0.9659258262890683122, 1.000000000000000000, 0.9659258262890683122, 1.000000000000000000, 0.9659258262890683122, 1.000000000000000000, 0.9659258262890683122, 1.000000000000000000, 0.9659258262890683122, 1.000000000000000000, 0.9659258262890683122, 1.000000000000000000, 0.9659258262890683122, 1.000000000000000000, 0.9659258262890683122, 1.000000000000000000, 0.9659258262890683122, 1.000000000000000000, 0.9659258262890683122, 1.000000000000000000, 0.9659258262890683122, 1.000000000000000000, 0.9659258262890683122, 1.000000000000000000, 0.9659258262890683122, 1.000000000000000000, 0.9659258262890683122, 1.000000000000000000, 0.9659258262890683122, 1.000000000000000000, 0.9659258262890683122, 1.000000000000000000, 0.9659258262890683122, 1.000000000000000000, 0.9659258262890683122, 1.000000000000000000, 0.9659258262890683122, 1.000000000000000000, 0.9659258262890683122, 1.000000000000000000, 0.9659258262890683122, 1.000000000000000000, 0.9659258262890683122, 1.000000000000000000, 0.9659258262890683122, 1.000000000000000000, 0.9659258262890683122, 1.000000000000000000, 0.9659258262890683122, 1.000000000000000000, 0.9659258262890683122, 1.000000000000000000, 0.9659258262890683122, 1.000000000000000000, 0.9659258262890683122, 1.000000000000000000, 0.9659258262890683122, 1.000000000000000000, 0.9659258262890683122, 1.000000000000000000, 0.9659258262890683122, 1.000000000000000000, 0.9659258262890683122, 1.000000000000000000, 0.9659258262890683122, 1.000000000000000000, 0.9659258262890683122, 1.000000000000000000, 0.9659258262890683122, 1.000000000000000000, 0.9659258262890683122, 1.000000000000000000, 0.9659258262890683122, 1.000000000000000000, 0.9659258262890683122, 1.000000000000000000, 0.9659258262890683122, 1.000000000000000000, 0.9659258262890683122, 1.000000000000000000, 0.9659258262890683122, 1.000000000000000000, 0.9659258262890683122, 1.000000000000000000, 0.9659258262890683122, 1.000000000000000000, 0.9659258262890683122, 1.000000000000000000, 0.9659258262890683122, 1.000000000000000000, 0.9659258262890683122, 1.000000000000000000, 0.9659258262890683122, 1.000000000000000000, 0.9659258262890683122, 1.000000000000000000, 0.9659258262890683122, 1.000000000000000000, 0.9659258262890683122, 1.000000000000000000, 0.9659258262890683122, 1.000000000000000000, 0.9659258262890683122, 1.000000000000000000, 0.9659258262890683122, 1.000000000000000000, 0.9659258262890683122, 1.000000000000000000, 0.9659258262890683122, 1.000000000000000000, 0.9659258262890683122, 1.000000000000000000, 0.9659258262890683122, 1.000000000000000000, 0.9659258262890683122, 1.000000000000000000, 0.9659258262890683122, 1.000000000000000000, 0.9659258262890683122, 1.000000000000000000, 0.9659258262890683122, 1.000000000000000000, 0.9659258262890683122, 1.000000000000000000, 0.9659258262890683122, 1.000000000000000000, 0.9659258262890683122, 1.000000000000000000, 0.9659258262890683122, 1.000000000000000000, 0.9659258262890683122, 1.000000000000000000, 0.9659258262890683122, 1.000000000000000000, 0.9659258262890683122, 1.000000000000000000, 0.9659258262890683122, 1.000000000000000000, 0.9659258262890683122, 1.000000000000000000, 0.9659258262890683122, 1.000000000000000000, 0.9659258262890683122, 1.000000000000000000, 0.9659258262890683122, 1.000000000000000000, 0.9659258262890683122, 1.000000000000000000, 0.9659258262890683122, 1.000000000000000000, 0.9659258262890683122, 1.000000000000000000, 0.9659258262890683122, 1.000000000000000000, 0.9659258262890683122, 1.000000000000000000, 0.9659258262890683122, 1.000000000000000000, 0.9659258262890683122, 1.000000000000000000, 0.9659258262890683122, 1.000000000000000000, 0.9659258262890683122, 1.000000000000000000, 0.9659258262890683122, 1.000000000000000000, 0.9659258262890683122, 1.000000000000000000, 0.9659258262890683122, 1.000000000000000000, 0.9659258262890683122, 1.000000000000000000, 0.9659258262890683122, 1.000000000000000000, 0.9659258262890683122, 1.000000000000000000, 0.9659258262890683122, 1.000000000000000000, 0.9659258262890683122, 1.000000000000000000, 0.9659258262890683122, 1.000000000000000000, 0.9659258262890683122, 1.000000000000000000, 0.9659258262890683122, 1.000000000000000000, 0.9659258262890683122, 1.000000000000000000, 0.9659258262890683122, 1.000000000000000000, 0.9659258262890683122, 1.000000000000000000, 0.9659258262890683122, 1.000000000000000000, 0.9659258262890683122, 1.000000000000000000, 0.9659258262890683122, 1.000000000000000000, 0.9659258262890683122, 1.000000000000000000, 0.9659258262890683122, 1.000000000000000000, 0.9659258262890683122, 1.000000000000000000, 0.9659258262890683122, 1.000000000000000000, 0.9659258262890683122, 1.000000000000000000, 0.9659258262890683122, 1.000000000000000000, 0.9659258262890683122, 1.000000000000000000, 0.9659258262890683122, 1.000000000000000000, 0.9659258262890683122, 1.000000000000000000, 0.9659258262890683122, 1.000000000000000000, 0.9659258262890683122, 1.000000000000000000, 0.9659258262890683122, 1.000000000000000000, 0.9659258262890683122, 1.000000000000000000, 0.9659258262890683122, 1.000000000000000000, 0.9659258262890683122, 1.000000000000000000, 0.9659258262890683122, 1.000000000000000000, 0.9659258262890683122, 1.000000000000000000, 0.9659258262890683122, 1.000000000000000000, 0.9659258262890683122, 1.000000000000000000, 0.9659258262890683122, 1.000000000000000000, 0.9659258262890683122, 1.000000000000000000, 0.9659258262890683122, 1.000000000000000000, 0.9659258262890683122, 1.000000000000000000, 0.9659258262890683122, 1.000000000000000000, 0.9659258262890683122, 1.000000000000000000, 0.9659258262890683122, 1.000000000000000000, 0.9659258262890683122, 1.000000000000000000, 0.9659258262890683122, 1.000000000000000000, 0.9659258262890683122, 1.000000000000000000, 0.9659258262890683122, 1.000000000000000000, 0.9659258262890683122, 1.000000000000000000, 0.9659258262890683122, 1.000000000000000000, 0.9659258262890683122, 1.000000000000000000, 0.9659258262890683122, 1.000000000000000000, 0.9659258262890683122, 1.000000000000000000, 0.9659258262890683122, 1.000000000000000000, 0.9659258262890683122, 1.000000000000000000, 0.9659258262890683122, 1.000000000000000000, 0.9659258262890683122, 1.000000000000000000, 0.9659258262890683122, 1.000000000000000000, 0.9659258262890683122, 1.000000000000000000, 0.9659258262890683122, 1.000000000000000000, 0.9659258262890683122, 1.000000000000000000, 0.9659258262890683122, 1.000000000000000000, 0.9659258262890683122, 1.000000000000000000, 0.9659258262890683122, 1.000000000000000000, 0.9659258262890683122, 1.000000000000000000, 0.9659258262890683122, 1.000000000000000000, 0.9659258262890683122, 1.000000000000000000, 0.9659258262890683122, 1.000000000000000000, 0.9659258262890683122, 1.000000000000000000, 0.9659258262890683122, 1.000000000000000000, 0.9659258262890683122, 1.000000000000000000, 0.9659258262890683122, 1.000000000000000000, 0.9659258262890683122, 1.000000000000000000, 0.9659258262890683122, 1.000000000000000000, 0.9659258262890683122, 1.000000000000000000, 0.9659258262890683122, 1.000000000000000000, 0.9659258262890683122, 1.000000000000000000, 0.9659258262890683122, 1.000000000000000000, 0.9659258262890683122, 1.000000000000000000, 0.9659258262890683122, 1.000000000000000000, 0.9659258262890683122, 1.000000000000000000, 0.9659258262890683122, 1.000000000000000000, 0.9659258262890683122, 1.000000000000000000) ) ) 
 REPRESENTATION_ITEM ( '' )  SURFACE ( )  );
#5408=CARTESIAN_POINT ( 'NONE',  ( -0.1312335958005241554, -0.5023911411419708095, -0.1820866141732282451 ) ) ;
#5409=CARTESIAN_POINT ( 'NONE',  ( -1.574803149606298636, -0.1870078740157479769, 0.3641732283464567677 ) ) ;
#5410=CARTESIAN_POINT ( 'NONE',  ( 0.6299212598425204535, -0.1870078740157480879, -0.4822834645669291653 ) ) ;
#5412=CARTESIAN_POINT ( 'NONE',  ( 1.417322834645670104, -0.1870078740157479769, 0.3641732283464567677 ) ) ;
#5414=CARTESIAN_POINT ( 'NONE',  ( -0.9580052493438311334, -0.4281496062992124485, 0.4176697321401328655 ) ) ;
#5415=CARTESIAN_POINT ( 'NONE',  ( -0.3937007874015740483, -0.1870078740157479769, 0.3641732283464567677 ) ) ;
#5416=FACE_OUTER_BOUND ( 'NONE', #31024, .T. ) ;
#5417=CARTESIAN_POINT ( 'NONE',  ( 0.3083989501312343062, -0.2845877964562159024, 0.3641732283464567677 ) ) ;
#5418=CARTESIAN_POINT ( 'NONE',  ( -1.220472440944881054, 0.2952755905511811885, 0.000000000000000000 ) ) ;
#5419=CARTESIAN_POINT ( 'NONE',  ( -0.4330708661417315697, -0.6692913385826771977, 8.415575281601705876E-17 ) ) ;
#5422=CARTESIAN_POINT ( 'NONE',  ( 0.6364829396325465405, -0.08942795157527998196, 0.3641732283464567121 ) ) ;
#5423=CARTESIAN_POINT ( 'NONE',  ( -0.4724409448818890911, -0.1870078740157480879, -0.4822834645669291653 ) ) ;
#5424=CARTESIAN_POINT ( 'NONE',  ( -0.8267716535433065062, 0.2952755905511811885, 0.000000000000000000 ) ) ;
#5425=CARTESIAN_POINT ( 'NONE',  ( -1.003937007874014853, 0.07958543189024085140, 0.2665933059059887866 ) ) ;
#5427=CARTESIAN_POINT ( 'NONE',  ( -0.2165354330708654795, 0.1660481256975885056, 0.3530559997133364547 ) ) ;
#5429=CARTESIAN_POINT ( 'NONE',  ( -1.660104986876639543, -0.08942795157528024563, -0.3641732283464568787 ) ) ;
#5430=CARTESIAN_POINT ( 'NONE',  ( -1.463254593175852492, 0.2952755905511811885, 0.1292274648535926551 ) ) ;
#5435=CARTESIAN_POINT ( 'NONE',  ( -1.305774278215222184, -0.6692913385826773087, -0.1292274648535924053 ) ) ;
#5436=CARTESIAN_POINT ( 'NONE',  ( -0.7086614173228339419, -0.1870078740157480879, -0.4822834645669291653 ) ) ;
#5437=CARTESIAN_POINT ( 'NONE',  ( 1.502624671916010790, -0.3162353388693409650, -0.4822834645669289433 ) ) ;
#5440=CARTESIAN_POINT ( 'NONE',  ( 0.8989501312335964611, 0.2952755905511811885, 0.1292274648535926551 ) ) ;
#5441=CARTESIAN_POINT ( 'NONE',  ( 0.3871391076115493490, -0.3162353388693405765, 0.4822834645669290543 ) ) ;
#5443=DIRECTION ( 'NONE',  ( -1.000000000000000000, 0.000000000000000000, 1.692413147294445970E-16 ) ) ;
#5444=CARTESIAN_POINT ( 'NONE',  ( 1.181102362204724976, -0.1870078740157480601, -0.3641732283464567677 ) ) ;
#5449=CARTESIAN_POINT ( 'NONE',  ( 0.3543307086614179147, 0.2952755905511811885, 0.000000000000000000 ) ) ;
#5450=CARTESIAN_POINT ( 'NONE',  ( -0.8398950131233589023, -0.6046776061558809534, -0.2411417322834644161 ) ) ;
#5451=CARTESIAN_POINT ( 'NONE',  ( -1.338582677165353729, -0.1870078740157479769, 0.4822834645669291653 ) ) ;
#5452=CARTESIAN_POINT ( 'NONE',  ( 0.8727034120734913358, -0.05778040916215522460, 0.4822834645669289988 ) ) ;
#5453=CARTESIAN_POINT ( 'NONE',  ( 1.548556430446194954, 0.2306618581243847221, -0.2411417322834647770 ) ) ;
#5455=CARTESIAN_POINT ( 'NONE',  ( -0.2493438320209966919, -0.4281496062992124485, 0.4176697321401328655 ) ) ;
#5456=CARTESIAN_POINT ( 'NONE',  ( -1.430446194225720724, 0.05413385826771626580, -0.4176697321401330321 ) ) ;
#5457=CARTESIAN_POINT ( 'NONE',  ( -1.489501312335957062, -0.05778040916215522460, 0.4822834645669289988 ) ) ;
#5458=CARTESIAN_POINT ( 'NONE',  ( 1.640419947506562393, -0.4281496062992124485, 0.4176697321401328655 ) ) ;
#5460=CARTESIAN_POINT ( 'NONE',  ( 0.8464566929133866546, -0.4536011799217367080, 0.2665933059059888421 ) ) ;
#5464=CARTESIAN_POINT ( 'NONE',  ( 0.1049868766404206816, -0.5023911411419708095, -0.1820866141732282451 ) ) ;
#5466=CARTESIAN_POINT ( 'NONE',  ( 0.7152230971128614723, -0.3162353388693409650, -0.4822834645669289433 ) ) ;
#5467=CARTESIAN_POINT ( 'NONE',  ( 0.2624671916010504757, -0.6046776061558809534, -0.2411417322834644161 ) ) ;
#5468=CARTESIAN_POINT ( 'NONE',  ( -0.7414698162729651543, 0.2952755905511810774, -0.1292274648535930714 ) ) ;
#5469=ADVANCED_FACE ( 'NONE', ( #473 ), #47200, .F. ) ;
#5471=CARTESIAN_POINT ( 'NONE',  ( -1.391076115485563314, -0.6046776061558809534, -0.2411417322834644161 ) ) ;
#5473=CARTESIAN_POINT ( 'NONE',  ( 1.194225721784777594, -0.3690944881889765550, -0.3153832671262227771 ) ) ;
#5474=CARTESIAN_POINT ( 'NONE',  ( -1.305774278215222184, 0.2952755905511811885, 0.1292274648535926551 ) ) ;
#5475=CARTESIAN_POINT ( 'NONE',  ( 0.8530183727034128527, -0.4281496062992124485, 0.4176697321401328655 ) ) ;
#5476=CARTESIAN_POINT ( 'NONE',  ( 1.043307086614173818, 0.1660481256975885056, 0.3530559997133364547 ) ) ;
#5479=CARTESIAN_POINT ( 'NONE',  ( -1.167979002624671470, -0.4281496062992127816, -0.4176697321401328100 ) ) ;
#5481=B_SPLINE_CURVE_WITH_KNOTS ( 'NONE', 3,
 ( #21600, #40965, #61140, #60320, #22435, #67059, #2669 ),
 .UNSPECIFIED., .F., .F.,
 ( 4, 3, 4 ),
 ( 0.000000000000000000, 0.001246232571205312112, 0.002492492258783314020 ),
 .UNSPECIFIED. ) ;
#5482=CARTESIAN_POINT ( 'NONE',  ( -0.2034120734908131112, -0.6692913385826773087, -0.1292274648535924053 ) ) ;
#5485=CARTESIAN_POINT ( 'NONE',  ( 1.430446194225722500, -0.4281496062992127816, -0.4176697321401328100 ) ) ;
#5486=CARTESIAN_POINT ( 'NONE',  ( 0.08530183727034192087, -0.08942795157527998196, 0.3641732283464567121 ) ) ;
#5487=CARTESIAN_POINT ( 'NONE',  ( 1.036745406824147508, -0.4281496062992127816, -0.4176697321401328100 ) ) ;
#5489=CARTESIAN_POINT ( 'NONE',  ( 0.6627296587926517768, -0.5511811023622048555, -0.09757992244046775898 ) ) ;
#5490=CARTESIAN_POINT ( 'NONE',  ( 0.5314960629921264834, 0.1660481256975883668, -0.3530559997133364547 ) ) ;
#5492=CARTESIAN_POINT ( 'NONE',  ( -0.9186351706036736120, 0.2306618581243848609, 0.2411417322834645549 ) ) ;
#5494=CARTESIAN_POINT ( 'NONE',  ( 1.049868766404200127, -0.5023911411419708095, -0.1820866141732282451 ) ) ;
#5496=CARTESIAN_POINT ( 'NONE',  ( -0.4593175853018366950, 0.05413385826771666132, 0.4176697321401328100 ) ) ;
#5497=CARTESIAN_POINT ( 'NONE',  ( 0.2099737532808405305, -0.5023911411419708095, 0.1820866141732285504 ) ) ;
#5499=CARTESIAN_POINT ( 'NONE',  ( -0.5249343832020990641, -0.6046776061558809534, -0.2411417322834644161 ) ) ;
#5500=CARTESIAN_POINT ( 'NONE',  ( 0.8136482939632553313, 0.1283753931104748280, 0.1820866141732283561 ) ) ;
#5502=CARTESIAN_POINT ( 'NONE',  ( 0.5118110236220480003, -0.6692913385826771977, 8.415575281601705876E-17 ) ) ;
#5503=CARTESIAN_POINT ( 'NONE',  ( 1.200787401574803681, 0.07958543189024085140, 0.2665933059059887866 ) ) ;
#5504=CARTESIAN_POINT ( 'NONE',  ( 0.2262115530851599166, 8.471767977567108961E-16, -0.4445507791589058955 ) ) ;
#5505=CARTESIAN_POINT ( 'NONE',  ( -0.5643044619422565855, -0.004921259842519870586, -0.3153832671262229437 ) ) ;
#5506=CARTESIAN_POINT ( 'NONE',  ( -0.6758530183727028406, -0.5511811023622048555, -0.09757992244046775898 ) ) ;
#5507=CARTESIAN_POINT ( 'NONE',  ( -0.1574803149606292529, -0.1870078740157480879, -0.4822834645669291653 ) ) ;
#5508=CARTESIAN_POINT ( 'NONE',  ( 0.5118110236220478892, 0.2952755905511811885, 0.000000000000000000 ) ) ;
#5509=CARTESIAN_POINT ( 'NONE',  ( 0.8464566929133866546, -0.4536011799217367080, 0.2665933059059888421 ) ) ;
#5510=CARTESIAN_POINT ( 'NONE',  ( -1.712598425196849572, 0.07958543189024085140, 0.2665933059059887866 ) ) ;
#5511=CARTESIAN_POINT ( 'NONE',  ( -1.653543307086613234, -0.1870078740157480879, -0.4822834645669291653 ) ) ;
#5512=CARTESIAN_POINT ( 'NONE',  ( 0.8136482939632553313, -0.6046776061558809534, -0.2411417322834644161 ) ) ;
#5513=CARTESIAN_POINT ( 'NONE',  ( -1.604771003085129433, 1.829390573268580455, -0.1466069496707752273 ) ) ;
#5514=CARTESIAN_POINT ( 'NONE',  ( -0.4330708661417315697, 0.2952755905511811885, 0.000000000000000000 ) ) ;
#5516=CARTESIAN_POINT ( 'NONE',  ( 0.7611548556430454138, 0.2306618581243847221, -0.2411417322834647770 ) ) ;
#5517=CARTESIAN_POINT ( 'NONE',  ( 0.5183727034120741983, -0.6692913385826771977, 0.1292274648535927661 ) ) ;
#5519=CARTESIAN_POINT ( 'NONE',  ( 0.2427821522309719648, -0.08942795157527998196, 0.3641732283464567121 ) ) ;
#5520=CARTESIAN_POINT ( 'NONE',  ( 1.227034120734908917, 0.2952755905511810774, -0.1292274648535930714 ) ) ;
#5522=CARTESIAN_POINT ( 'NONE',  ( -0.1181102362204717315, 0.1771653543307087630, 0.000000000000000000 ) ) ;
#5523=CARTESIAN_POINT ( 'NONE',  ( -0.1640419947506553400, -0.05778040916215560624, -0.4822834645669293319 ) ) ;
#5524=CARTESIAN_POINT ( 'NONE',  ( -1.614173228346456712, 2.401574803149606474, 0.1372047244094477536 ) ) ;
#5525=CARTESIAN_POINT ( 'NONE',  ( 0.4133858267716541968, -0.5400638737290845981, -0.3530559997133363437 ) ) ;
#5526=CARTESIAN_POINT ( 'NONE',  ( -0.7611548556430438595, -0.6046776061558809534, -0.2411417322834644161 ) ) ;
#5527=CARTESIAN_POINT ( 'NONE',  ( -0.5183727034120726440, -0.5511811023622048555, -0.09757992244046775898 ) ) ;
#5528=VECTOR ( 'NONE', #43648, 39.37007874015748143 ) ;
#5529=CARTESIAN_POINT ( 'NONE',  ( 0.2624671916010504757, -0.6046776061558809534, -0.2411417322834644161 ) ) ;
#5530=CARTESIAN_POINT ( 'NONE',  ( -1.377952755905511140, 0.2952755905511811885, 0.000000000000000000 ) ) ;
#5531=CARTESIAN_POINT ( 'NONE',  ( -0.4658792650918627265, -0.3162353388693409650, -0.4822834645669289433 ) ) ;
#5533=CARTESIAN_POINT ( 'NONE',  ( -0.9329488473419921268, -1.146068349578384814E-15, 0.3627985898453523483 ) ) ;
#5534=CARTESIAN_POINT ( 'NONE',  ( 1.312335958005249825, 0.2306618581243847221, -0.2411417322834647770 ) ) ;
#5535=CARTESIAN_POINT ( 'NONE',  ( 1.620734908136483465, -0.6692913385826771977, 0.1292274648535927661 ) ) ;
#5537=PLANE ( 'NONE',  #27442 ) ;
#5538=CARTESIAN_POINT ( 'NONE',  ( -1.023622047244094002, -0.1870078740157480879, -0.4822834645669291653 ) ) ;
#5541=VERTEX_POINT ( 'NONE', #41498 ) ;
#5542=CARTESIAN_POINT ( 'NONE',  ( 0.2821522309711292364, 0.1771653543307087075, -0.09757992244046823083 ) ) ;
#5544=CARTESIAN_POINT ( 'NONE',  ( 0.6233595800524939223, -0.3162353388693405765, 0.4822834645669290543 ) ) ;
#5547=CARTESIAN_POINT ( 'NONE',  ( -0.5708661417322825615, -0.4536011799217367080, 0.2665933059059888421 ) ) ;
#5548=CARTESIAN_POINT ( 'NONE',  ( -1.706036745406823485, 0.1283753931104748280, 0.1820866141732283561 ) ) ;
#5550=CARTESIAN_POINT ( 'NONE',  ( 1.233595800524935227, 0.2306618581243847221, -0.2411417322834647770 ) ) ;
#5551=CARTESIAN_POINT ( 'NONE',  ( 0.8202099737532813073, 0.1771653543307087630, 0.09757992244046791164 ) ) ;
#5552=CARTESIAN_POINT ( 'NONE',  ( -0.1771653543307080136, 0.1660481256975883668, -0.3530559997133364547 ) ) ;
#5554=CARTESIAN_POINT ( 'NONE',  ( -0.6036745406824141069, -0.6046776061558809534, -0.2411417322834644161 ) ) ;
#5555=CARTESIAN_POINT ( 'NONE',  ( -1.266404199475064773, -0.2845877964562159024, 0.3641732283464567677 ) ) ;
#5556=CARTESIAN_POINT ( 'NONE',  ( -0.4527559055118102749, 0.1660481256975885056, 0.3530559997133364547 ) ) ;
#5557=LINE ( 'NONE', #70354, #7207 ) ;
#5561=CARTESIAN_POINT ( 'NONE',  ( 0.5118110236220480003, -0.6692913385826771977, 8.415575281601705876E-17 ) ) ;
#5562=ORIENTED_EDGE ( 'NONE', *, *, #58189, .T. ) ;
#5563=CARTESIAN_POINT ( 'NONE',  ( -0.3543307086614165824, -0.6692913385826771977, 8.415575281601705876E-17 ) ) ;
#5564=CARTESIAN_POINT ( 'NONE',  ( -1.305774278215222184, 0.2952755905511811885, 0.1292274648535926551 ) ) ;
#5565=CARTESIAN_POINT ( 'NONE',  ( 0.5774278215223103139, -0.6046776061558809534, -0.2411417322834644161 ) ) ;
#5566=CARTESIAN_POINT ( 'NONE',  ( 0.03280839895013198948, -0.6692913385826773087, -0.1292274648535924053 ) ) ;
#5568=CARTESIAN_POINT ( 'NONE',  ( -0.9055118110236215490, 0.2952755905511811885, 0.000000000000000000 ) ) ;
#5569=CARTESIAN_POINT ( 'NONE',  ( 0.2887139107611556010, 0.2306618581243847221, -0.2411417322834647770 ) ) ;
#5570=CARTESIAN_POINT ( 'NONE',  ( -0.4002624671916004129, -0.3162353388693405765, 0.4822834645669290543 ) ) ;
#5571=CARTESIAN_POINT ( 'NONE',  ( 0.4330708661417329575, 0.1771653543307087630, 0.000000000000000000 ) ) ;
#5573=CARTESIAN_POINT ( 'NONE',  ( -0.2034120734908131112, -0.6692913385826773087, -0.1292274648535924053 ) ) ;
#5575=CARTESIAN_POINT ( 'NONE',  ( 1.476377952755906220, 0.1660481256975883668, -0.3530559997133364547 ) ) ;
#5578=ORIENTED_EDGE ( 'NONE', *, *, #44328, .F. ) ;
#5579=CARTESIAN_POINT ( 'NONE',  ( 0.4002624671916016896, -0.05778040916215522460, 0.4822834645669289988 ) ) ;
#5580=CARTESIAN_POINT ( 'NONE',  ( -0.01968503937007793844, -0.4536011799217367080, 0.2665933059059888421 ) ) ;
#5581=CARTESIAN_POINT ( 'NONE',  ( 1.259842519685040019, -0.1870078740157480601, -0.3641732283464567677 ) ) ;
#5582=CARTESIAN_POINT ( 'NONE',  ( -0.06804098107080119862, -3.915482057279200494E-15, 0.4118484887281999574 ) ) ;
#5586=CARTESIAN_POINT ( 'NONE',  ( 0.3871391076115492380, -0.05778040916215560624, -0.4822834645669293319 ) ) ;
#5587=CARTESIAN_POINT ( 'NONE',  ( -1.430446194225720724, 0.05413385826771626580, -0.4176697321401330321 ) ) ;
#5588=CARTESIAN_POINT ( 'NONE',  ( -1.089238845144356427, 0.05413385826771666132, 0.4176697321401328100 ) ) ;
#5589=CARTESIAN_POINT ( 'NONE',  ( 0.1377952755905518800, -0.5400638737290844871, 0.3530559997133364547 ) ) ;
#5591=CARTESIAN_POINT ( 'NONE',  ( 0.8792650918635177559, -0.4281496062992127816, -0.4176697321401328100 ) ) ;
#5592=CARTESIAN_POINT ( 'NONE',  ( 1.456692913385827515, -0.5511811023622047445, 6.969142054262312111E-17 ) ) ;
#5594=CARTESIAN_POINT ( 'NONE',  ( 0.6824146981627303710, -0.5023911411419708095, 0.1820866141732285504 ) ) ;
#5595=CARTESIAN_POINT ( 'NONE',  ( -1.049868766404198794, -0.6046776061558807314, 0.2411417322834647770 ) ) ;
#5597=CARTESIAN_POINT ( 'NONE',  ( 1.482939632545932307, -0.4281496062992124485, 0.4176697321401328655 ) ) ;
#5599=CARTESIAN_POINT ( 'NONE',  ( 1.351706036745407680, 0.05413385826771666132, 0.4176697321401328100 ) ) ;
#5601=CARTESIAN_POINT ( 'NONE',  ( -1.673228346456691717, 0.07958543189024071263, -0.2665933059059888421 ) ) ;
#5602=CARTESIAN_POINT ( 'NONE',  ( 0.006561679790026889343, -0.3162353388693409650, -0.4822834645669289433 ) ) ;
#5603=CARTESIAN_POINT ( 'NONE',  ( 0.6692913385826777528, 0.1771653543307087630, 0.000000000000000000 ) ) ;
#5604=CARTESIAN_POINT ( 'NONE',  ( -1.522309711286088607, 0.1283753931104746893, -0.1820866141732285504 ) ) ;
#5605=CARTESIAN_POINT ( 'NONE',  ( 1.108923884514436686, -0.3162353388693409650, -0.4822834645669289433 ) ) ;
#5606=CARTESIAN_POINT ( 'NONE',  ( -0.5314960629921250401, 0.1660481256975885056, 0.3530559997133364547 ) ) ;
#5607=CARTESIAN_POINT ( 'NONE',  ( -0.5249343832020990641, -0.5023911411419708095, -0.1820866141732282451 ) ) ;
#5608=CARTESIAN_POINT ( 'NONE',  ( -0.6036745406824141069, 0.2306618581243848609, 0.2411417322834645549 ) ) ;
#5609=CARTESIAN_POINT ( 'NONE',  ( 1.417322834645670104, -0.1870078740157480879, -0.4822834645669291653 ) ) ;
#5610=CARTESIAN_POINT ( 'NONE',  ( -1.043307086614172707, 0.1660481256975883668, -0.3530559997133364547 ) ) ;
#5611=CARTESIAN_POINT ( 'NONE',  ( 1.496062992125985147, -0.1870078740157479769, 0.4822834645669291653 ) ) ;
#5613=CARTESIAN_POINT ( 'NONE',  ( -1.292650918635170010, 0.1771653543307087075, -0.09757992244046823083 ) ) ;
#5616=CARTESIAN_POINT ( 'NONE',  ( 0.8858267716535438430, -0.5400638737290845981, -0.3530559997133363437 ) ) ;
#5619=CARTESIAN_POINT ( 'NONE',  ( -1.548556430446193399, 0.2306618581243848609, 0.2411417322834645549 ) ) ;
#5620=CARTESIAN_POINT ( 'NONE',  ( -1.653543307086613234, -0.1870078740157479769, 0.3641732283464567677 ) ) ;
#5621=CARTESIAN_POINT ( 'NONE',  ( -0.9711286089238838626, -0.5023911411419708095, 0.1820866141732285504 ) ) ;
#5622=CARTESIAN_POINT ( 'NONE',  ( 1.646981627296588035, -0.2845877964562159024, 0.3641732283464567677 ) ) ;
#5623=CARTESIAN_POINT ( 'NONE',  ( -0.5577427821522301654, -0.3162353388693405765, 0.4822834645669290543 ) ) ;
#5624=CARTESIAN_POINT ( 'NONE',  ( -0.04593175853018302557, 0.1771653543307087630, 0.09757992244046791164 ) ) ;
#5625=CARTESIAN_POINT ( 'NONE',  ( -1.456692913385826182, -0.5511811023622047445, 6.969142054262312111E-17 ) ) ;
#5626=CARTESIAN_POINT ( 'NONE',  ( 1.522309711286089939, -0.5023911411419708095, -0.1820866141732282451 ) ) ;
#5627=CARTESIAN_POINT ( 'NONE',  ( 0.8989501312335964611, 0.2952755905511811885, 0.1292274648535926551 ) ) ;
#5628=CARTESIAN_POINT ( 'NONE',  ( 1.397637795275591177, -0.5400638737290844871, 0.3530559997133364547 ) ) ;
#5629=CARTESIAN_POINT ( 'NONE',  ( 0.05905511811023709395, -0.4536011799217367080, 0.2665933059059888421 ) ) ;
#5630=CARTESIAN_POINT ( 'NONE',  ( 0.6430446194225729606, -0.4281496062992127816, -0.4176697321401328100 ) ) ;
#5631=CARTESIAN_POINT ( 'NONE',  ( 1.148293963254593653, 0.1771653543307087075, -0.09757992244046823083 ) ) ;
#5633=CARTESIAN_POINT ( 'NONE',  ( -1.522309711286088607, -0.6046776061558807314, 0.2411417322834647770 ) ) ;
#5634=CARTESIAN_POINT ( 'NONE',  ( -1.456692913385826182, 0.2952755905511811885, 0.000000000000000000 ) ) ;
#5635=CARTESIAN_POINT ( 'NONE',  ( -0.3083989501312330295, -0.05778040916215522460, 0.4822834645669289988 ) ) ;
#5638=CARTESIAN_POINT ( 'NONE',  ( 0.3608923884514443348, 0.2952755905511810774, -0.1292274648535930714 ) ) ;
#5639=CARTESIAN_POINT ( 'NONE',  ( 1.292650918635171564, 0.1771653543307087630, 0.09757992244046791164 ) ) ;
#5640=CARTESIAN_POINT ( 'NONE',  ( 0.1837270341207357105, -0.6046776061558809534, -0.2411417322834644161 ) ) ;
#5641=CARTESIAN_POINT ( 'NONE',  ( 0.1640419947506569498, -0.05778040916215522460, 0.4822834645669289988 ) ) ;
#5647=CARTESIAN_POINT ( 'NONE',  ( -0.6299212598425188991, -0.1870078740157479769, 0.3641732283464567677 ) ) ;
#5648=CARTESIAN_POINT ( 'NONE',  ( -0.7414698162729651543, 0.2952755905511810774, -0.1292274648535930714 ) ) ;
#5649=VECTOR ( 'NONE', #69209, 39.37007874015748143 ) ;
#5651=CARTESIAN_POINT ( 'NONE',  ( 0.7283464566929143125, 0.1660481256975885056, 0.3530559997133364547 ) ) ;
#5652=CARTESIAN_POINT ( 'NONE',  ( -1.410761154855641575, -0.3162353388693409650, -0.4822834645669289433 ) ) ;
#5653=CARTESIAN_POINT ( 'NONE',  ( 0.6758530183727039509, 0.2952755905511810774, -0.1292274648535930714 ) ) ;
#5656=CARTESIAN_POINT ( 'NONE',  ( 1.594488188976378673, -0.5400638737290845981, -0.3530559997133363437 ) ) ;
#5657=CARTESIAN_POINT ( 'NONE',  ( 0.7086614173228352742, -0.1870078740157480879, -0.4822834645669291653 ) ) ;
#5658=CARTESIAN_POINT ( 'NONE',  ( 0.7152230971128614723, -0.3162353388693409650, -0.4822834645669289433 ) ) ;
#5659=CARTESIAN_POINT ( 'NONE',  ( 0.9776902887139113929, 0.1771653543307087630, 0.09757992244046791164 ) ) ;
#5660=CARTESIAN_POINT ( 'NONE',  ( 1.377952755905512472, 0.2952755905511811885, 0.000000000000000000 ) ) ;
#5663=CARTESIAN_POINT ( 'NONE',  ( 0.7545931758530189937, 0.2952755905511810774, -0.1292274648535930714 ) ) ;
#5664=DIRECTION ( 'NONE',  ( 0.000000000000000000, 0.000000000000000000, -1.000000000000000000 ) ) ;
#5665=CARTESIAN_POINT ( 'NONE',  ( -0.5249343832020990641, -0.6046776061558809534, -0.2411417322834644161 ) ) ;
#5666=CARTESIAN_POINT ( 'NONE',  ( -1.049868766404198794, 0.2306618581243847221, -0.2411417322834647770 ) ) ;
#5667=CARTESIAN_POINT ( 'NONE',  ( 0.9776902887139113929, 0.2952755905511811885, 0.1292274648535926551 ) ) ;
#5674=CARTESIAN_POINT ( 'NONE',  ( 1.345144356955381593, -0.2845877964562161244, -0.3641732283464567121 ) ) ;
#5676=CARTESIAN_POINT ( 'NONE',  ( 1.358267716535433323, 0.07958543189024085140, 0.2665933059059887866 ) ) ;
#5677=CARTESIAN_POINT ( 'NONE',  ( -0.7759054087898756835, -3.623651218081290895E-15, 0.3791475997938233977 ) ) ;
#5681=CARTESIAN_POINT ( 'NONE',  ( -0.8202099737532799750, 0.1771653543307087075, -0.09757992244046823083 ) ) ;
#5682=CARTESIAN_POINT ( 'NONE',  ( -1.660104986876639543, -0.08942795157528024563, -0.3641732283464568787 ) ) ;
#5683=CARTESIAN_POINT ( 'NONE',  ( -1.240157480314959759, -0.5400638737290845981, -0.3530559997133363437 ) ) ;
#5684=CARTESIAN_POINT ( 'NONE',  ( 0.03280839895013198948, 0.2952755905511811885, 0.1292274648535926551 ) ) ;
#5685=CARTESIAN_POINT ( 'NONE',  ( -1.653543307086613234, -0.1870078740157479769, 0.4822834645669291653 ) ) ;
#5686=ORIENTED_EDGE ( 'NONE', *, *, #74381, .F. ) ;
#5687=CARTESIAN_POINT ( 'NONE',  ( 1.568241469816273437, -0.3162353388693405765, 0.4822834645669290543 ) ) ;
#5691=CARTESIAN_POINT ( 'NONE',  ( -0.3805774278215216522, -0.004921259842519576551, 0.3153832671262227771 ) ) ;
#5692=CARTESIAN_POINT ( 'NONE',  ( -1.259842519685038686, -0.1870078740157480879, -0.4822834645669291653 ) ) ;
#5693=CARTESIAN_POINT ( 'NONE',  ( 1.135170603674541256, -0.6692913385826773087, -0.1292274648535924053 ) ) ;
#5694=VERTEX_POINT ( 'NONE', #6077 ) ;
#5695=CARTESIAN_POINT ( 'NONE',  ( 0.7742782152230979209, 0.05413385826771626580, -0.4176697321401330321 ) ) ;
#5696=CARTESIAN_POINT ( 'NONE',  ( -1.614173228346457378, 0.7794589730111965986, 0.1372047244094476981 ) ) ;
#5697=CARTESIAN_POINT ( 'NONE',  ( 1.095800524934383846, -0.05778040916215560624, -0.4822834645669293319 ) ) ;
#5698=CARTESIAN_POINT ( 'NONE',  ( -1.272965879265091305, -0.4281496062992124485, 0.4176697321401328655 ) ) ;
#5700=CARTESIAN_POINT ( 'NONE',  ( -0.3018372703412066094, -0.004921259842519576551, 0.3153832671262227771 ) ) ;
#5702=CARTESIAN_POINT ( 'NONE',  ( -0.5118110236220466680, 0.1771653543307087630, 0.000000000000000000 ) ) ;
#5703=CARTESIAN_POINT ( 'NONE',  ( 0.6364829396325465405, -0.08942795157527998196, 0.3641732283464567121 ) ) ;
#5704=CARTESIAN_POINT ( 'NONE',  ( 0.2296587926509192634, -0.05778040916215560624, -0.4822834645669293319 ) ) ;
#5706=CARTESIAN_POINT ( 'NONE',  ( -0.6036745406824141069, -0.5023911411419708095, -0.1820866141732282451 ) ) ;
#5708=CARTESIAN_POINT ( 'NONE',  ( 1.181102362204724976, -0.1870078740157480879, -0.4822834645669291653 ) ) ;
#5709=ADVANCED_FACE ( 'NONE', ( #11589 ), #39292, .F. ) ;
#5710=CARTESIAN_POINT ( 'NONE',  ( -0.8398950131233585692, 0.2306618581243848609, 0.2411417322834645549 ) ) ;
#5712=CARTESIAN_POINT ( 'NONE',  ( -0.1902887139107604098, -0.6692913385826771977, 0.1292274648535927661 ) ) ;
#5713=CARTESIAN_POINT ( 'NONE',  ( -0.7283464566929126471, -0.5400638737290844871, 0.3530559997133364547 ) ) ;
#5714=CARTESIAN_POINT ( 'NONE',  ( 1.364829396325460076, 0.1283753931104748280, 0.1820866141732283561 ) ) ;
#5715=CARTESIAN_POINT ( 'NONE',  ( 0.1049868766404206816, -0.5023911411419708095, -0.1820866141732282451 ) ) ;
#5716=CARTESIAN_POINT ( 'NONE',  ( -0.6036745406824141069, 0.2306618581243848609, 0.2411417322834645549 ) ) ;
#5717=CARTESIAN_POINT ( 'NONE',  ( -1.194225721784776262, -0.4281496062992124485, 0.4176697321401328655 ) ) ;
#5719=CARTESIAN_POINT ( 'NONE',  ( 1.154855643044620184, -0.5023911411419708095, 0.1820866141732285504 ) ) ;
#5720=CARTESIAN_POINT ( 'NONE',  ( -0.1443569553805765515, -0.4281496062992127816, -0.4176697321401328100 ) ) ;
#5721=CARTESIAN_POINT ( 'NONE',  ( -1.122047244094487306, -0.5400638737290844871, 0.3530559997133364547 ) ) ;
#5724=CARTESIAN_POINT ( 'NONE',  ( 1.128608923884514947, 0.2306618581243848609, 0.2411417322834645549 ) ) ;
#5725=CARTESIAN_POINT ( 'NONE',  ( -0.6889763779527552368, -0.4536011799217368745, -0.2665933059059886201 ) ) ;
#5727=CARTESIAN_POINT ( 'NONE',  ( -1.003937007874015297, -0.5400638737290845981, -0.3530559997133363437 ) ) ;
#5728=CARTESIAN_POINT ( 'NONE',  ( 1.259842519685040019, -0.1870078740157480879, -0.4822834645669291653 ) ) ;
#5729=CARTESIAN_POINT ( 'NONE',  ( 1.115485564304462551, -0.4281496062992127816, -0.4176697321401328100 ) ) ;
#5730=CARTESIAN_POINT ( 'NONE',  ( 1.515748031496063186, -0.5400638737290845981, -0.3530559997133363437 ) ) ;
#5731=CARTESIAN_POINT ( 'NONE',  ( -0.9711286089238838626, -0.5023911411419708095, 0.1820866141732285504 ) ) ;
#5736=CARTESIAN_POINT ( 'NONE',  ( 1.351706036745407680, -0.004921259842519576551, 0.3153832671262227771 ) ) ;
#5737=ADVANCED_FACE ( 'NONE', ( #75153 ), #31239, .F. ) ;
#5738=CARTESIAN_POINT ( 'NONE',  ( 0.8464566929133865436, 0.07958543189024071263, -0.2665933059059888421 ) ) ;
#5739=CARTESIAN_POINT ( 'NONE',  ( 0.4921259842519691285, 0.1660481256975885056, 0.3530559997133364547 ) ) ;
#5740=CARTESIAN_POINT ( 'NONE',  ( 1.555118110236221041, -0.5400638737290844871, 0.3530559997133364547 ) ) ;
#5742=CARTESIAN_POINT ( 'NONE',  ( 0.9580052493438327987, -0.3690944881889765550, -0.3153832671262227771 ) ) ;
#5743=CARTESIAN_POINT ( 'NONE',  ( -0.3412073490813641308, 0.2306618581243847221, -0.2411417322834647770 ) ) ;
#5744=CARTESIAN_POINT ( 'NONE',  ( -1.253280839895012377, -0.3162353388693409650, -0.4822834645669289433 ) ) ;
#5745=CARTESIAN_POINT ( 'NONE',  ( 1.404199475065617708, 0.05413385826771626580, -0.4176697321401330321 ) ) ;
#5748=CARTESIAN_POINT ( 'NONE',  ( 0.07874015748031558404, -0.1870078740157480601, -0.3641732283464567677 ) ) ;
#5749=( BOUNDED_CURVE ( )  B_SPLINE_CURVE ( 2, ( #64966, #19936, #72114, #14881, #33810, #52732, #59062, #66221, #65812, #65397, #40541, #21184, #53146 ),
 .UNSPECIFIED., .F., .F. ) 
 B_SPLINE_CURVE_WITH_KNOTS ( ( 3, 2, 2, 2, 2, 2, 3 ),
 ( 0.5035787205705963832, 0.5037878787878788955, 0.5075757575757575690, 0.5113636363636364646, 0.5151515151515151381, 0.5189393939393940336, 0.5191485521566765460 ),
 .UNSPECIFIED. ) 
 CURVE ( )  GEOMETRIC_REPRESENTATION_ITEM ( )  RATIONAL_B_SPLINE_CURVE ( ( 0.9964447847208420805, 0.9981185001348091834, 1.000000000000000000, 0.9659258262890683122, 1.000000000000000000, 0.9659258262890683122, 1.000000000000000000, 0.9659258262890683122, 1.000000000000000000, 0.9659258262890683122, 1.000000000000000000, 0.9981185001348090724, 0.9964447847208418585 ) ) 
 REPRESENTATION_ITEM ( '' )  );
#5753=CARTESIAN_POINT ( 'NONE',  ( -0.8398950131233589023, -0.6046776061558809534, -0.2411417322834644161 ) ) ;
#5754=CARTESIAN_POINT ( 'NONE',  ( -0.4724409448818890911, -0.1870078740157480879, -0.4822834645669291653 ) ) ;
#5755=CARTESIAN_POINT ( 'NONE',  ( -0.7414698162729651543, -0.5511811023622046335, 0.09757992244046803654 ) ) ;
#5756=CARTESIAN_POINT ( 'NONE',  ( -0.8136482939632537770, 0.2306618581243847221, -0.2411417322834647770 ) ) ;
#5757=CARTESIAN_POINT ( 'NONE',  ( 0.2690288713910767848, 0.2952755905511811885, 0.1292274648535926551 ) ) ;
#5758=CARTESIAN_POINT ( 'NONE',  ( -0.5511811023622038563, -0.1870078740157479769, 0.4822834645669291653 ) ) ;
#5759=CARTESIAN_POINT ( 'NONE',  ( -1.450131233595799651, 0.2952755905511810774, -0.1292274648535930714 ) ) ;
#5760=CARTESIAN_POINT ( 'NONE',  ( -0.8070866141732276899, -0.5400638737290844871, 0.3530559997133364547 ) ) ;
#5761=CARTESIAN_POINT ( 'NONE',  ( 0.7939632545931766261, -0.05778040916215522460, 0.4822834645669289988 ) ) ;
#5762=ADVANCED_FACE ( 'NONE', ( #62093 ), #63407, .F. ) ;
#5764=CARTESIAN_POINT ( 'NONE',  ( -0.4724409448818890911, -0.1870078740157480601, -0.3641732283464567677 ) ) ;
#5768=CARTESIAN_POINT ( 'NONE',  ( -1.253280839895012377, -0.08942795157527998196, 0.3641732283464567121 ) ) ;
#5769=CARTESIAN_POINT ( 'NONE',  ( -0.9973753280839886548, 0.2306618581243848609, 0.2411417322834645549 ) ) ;
#5770=CARTESIAN_POINT ( 'NONE',  ( -0.9251968503937002541, -0.5400638737290845981, -0.3530559997133363437 ) ) ;
#5772=CARTESIAN_POINT ( 'NONE',  ( -1.200787401574802349, 0.1660481256975883668, -0.3530559997133364547 ) ) ;
#5773=CARTESIAN_POINT ( 'NONE',  ( -0.8202099737532801971, -0.6692913385826771977, 0.1292274648535927661 ) ) ;
#5774=CARTESIAN_POINT ( 'NONE',  ( -1.574803149606298192, -0.1870078740157480879, -0.4822834645669291653 ) ) ;
#5776=CARTESIAN_POINT ( 'NONE',  ( 0.3412073490813655186, -0.5023911411419708095, -0.1820866141732282451 ) ) ;
#5779=CARTESIAN_POINT ( 'NONE',  ( 0.1968503937007881344, 0.1771653543307087630, 0.000000000000000000 ) ) ;
#5780=CARTESIAN_POINT ( 'NONE',  ( -0.5446194225721777693, -0.05778040916215522460, 0.4822834645669289988 ) ) ;
#5781=CARTESIAN_POINT ( 'NONE',  ( 1.200787401574803681, -0.5400638737290845981, -0.3530559997133363437 ) ) ;
#5782=CARTESIAN_POINT ( 'NONE',  ( -0.5314960629921250401, 0.1660481256975885056, 0.3530559997133364547 ) ) ;
#5783=ORIENTED_EDGE ( 'NONE', *, *, #78238, .F. ) ;
#5788=CARTESIAN_POINT ( 'NONE',  ( -0.7217847769028863381, -0.4281496062992124485, 0.4176697321401328655 ) ) ;
#5789=CARTESIAN_POINT ( 'NONE',  ( 1.253280839895013710, -0.3162353388693405765, 0.4822834645669290543 ) ) ;
#5790=CARTESIAN_POINT ( 'NONE',  ( -1.076115485564303809, 0.1283753931104748280, 0.1820866141732283561 ) ) ;
#5791=CARTESIAN_POINT ( 'NONE',  ( -1.423884514435694859, -0.3162353388693405765, 0.4822834645669290543 ) ) ;
#5793=DIRECTION ( 'NONE',  ( 0.000000000000000000, 1.000000000000000000, 0.000000000000000000 ) ) ;
#5795=CARTESIAN_POINT ( 'NONE',  ( 1.482939632545932307, -0.4281496062992124485, 0.4176697321401328655 ) ) ;
#5797=CARTESIAN_POINT ( 'NONE',  ( 0.05249343832021075018, -0.6046776061558807314, 0.2411417322834647770 ) ) ;
#5798=CARTESIAN_POINT ( 'NONE',  ( -0.9055118110236215490, -0.5511811023622047445, 6.969142054262312111E-17 ) ) ;
#5799=CARTESIAN_POINT ( 'NONE',  ( -0.2427821522309703550, -0.05778040916215560624, -0.4822834645669293319 ) ) ;
#5801=CARTESIAN_POINT ( 'NONE',  ( -1.023622047244094002, -0.1870078740157480879, -0.4822834645669291653 ) ) ;
#5802=CARTESIAN_POINT ( 'NONE',  ( -0.7480314960629914633, 0.2952755905511811885, 0.000000000000000000 ) ) ;
#5804=CARTESIAN_POINT ( 'NONE',  ( 0.6824146981627303710, 0.1283753931104746893, -0.1820866141732285504 ) ) ;
#5805=CARTESIAN_POINT ( 'NONE',  ( -0.1902887139107604098, -0.5511811023622046335, 0.09757992244046803654 ) ) ;
#5807=CARTESIAN_POINT ( 'NONE',  ( 0.7545931758530189937, 0.1771653543307087075, -0.09757992244046823083 ) ) ;
#5808=CARTESIAN_POINT ( 'NONE',  ( -1.640419947506561060, -0.4281496062992127816, -0.4176697321401328100 ) ) ;
#5809=CARTESIAN_POINT ( 'NONE',  ( 1.345144356955381593, -0.3162353388693409650, -0.4822834645669289433 ) ) ;
#5810=CARTESIAN_POINT ( 'NONE',  ( 0.6364829396325465405, -0.2845877964562161244, -0.3641732283464567121 ) ) ;
#5811=CARTESIAN_POINT ( 'NONE',  ( -0.8005249343832011588, 0.05413385826771626580, -0.4176697321401330321 ) ) ;
#5812=CARTESIAN_POINT ( 'NONE',  ( 1.246719160104987623, -0.4281496062992124485, 0.4176697321401328655 ) ) ;
#5813=CARTESIAN_POINT ( 'NONE',  ( 1.090429162302623212, 1.606403293320555813E-17, -0.3627985898453514602 ) ) ;
#5814=CARTESIAN_POINT ( 'NONE',  ( -0.1246719160104980823, -0.5511811023622048555, -0.09757992244046775898 ) ) ;
#5815=CARTESIAN_POINT ( 'NONE',  ( 0.1771653543307093182, -0.5400638737290845981, -0.3530559997133363437 ) ) ;
#5818=CARTESIAN_POINT ( 'NONE',  ( 1.318897637795276356, 0.07958543189024071263, -0.2665933059059888421 ) ) ;
#5819=CARTESIAN_POINT ( 'NONE',  ( -1.279527559055116948, -0.5400638737290844871, 0.3530559997133364547 ) ) ;
#5820=CARTESIAN_POINT ( 'NONE',  ( -0.4527559055118102749, -0.4536011799217368745, -0.2665933059059886201 ) ) ;
#5822=CARTESIAN_POINT ( 'NONE',  ( -1.141732283464566011, -0.6692913385826771977, 8.415575281601705876E-17 ) ) ;
#5823=CARTESIAN_POINT ( 'NONE',  ( -0.4855643044619415427, 0.05413385826771626580, -0.4176697321401330321 ) ) ;
#5826=CARTESIAN_POINT ( 'NONE',  ( 0.6561679790026253567, 0.1283753931104748280, 0.1820866141732283561 ) ) ;
#5827=CARTESIAN_POINT ( 'NONE',  ( -0.3543307086614165824, 0.2952755905511811885, 0.000000000000000000 ) ) ;
#5828=CARTESIAN_POINT ( 'NONE',  ( -0.4986876640419939388, 0.2306618581243847221, -0.2411417322834647770 ) ) ;
#5829=CARTESIAN_POINT ( 'NONE',  ( -0.6692913385826764205, 0.1771653543307087630, 0.000000000000000000 ) ) ;
#5831=CARTESIAN_POINT ( 'NONE',  ( 0.01312335958005323398, -0.4281496062992127816, -0.4176697321401328100 ) ) ;
#5832=DIRECTION ( 'NONE',  ( 3.386413887818972582E-16, -0.7071067811865514585, 0.7071067811865435759 ) ) ;
#5833=CARTESIAN_POINT ( 'NONE',  ( 1.404199475065617264, -0.4281496062992124485, 0.4176697321401328655 ) ) ;
#5838=CARTESIAN_POINT ( 'NONE',  ( -1.463254593175852492, -0.6692913385826773087, -0.1292274648535924053 ) ) ;
#5839=CARTESIAN_POINT ( 'NONE',  ( -0.6955380577427815458, -0.4281496062992127816, -0.4176697321401328100 ) ) ;
#5840=CARTESIAN_POINT ( 'NONE',  ( -1.614173228346455824, 0.2952755905511811885, 0.000000000000000000 ) ) ;
#5843=CARTESIAN_POINT ( 'NONE',  ( 0.8464566929133866546, -0.5400638737290844871, 0.3530559997133364547 ) ) ;
#5844=CARTESIAN_POINT ( 'NONE',  ( 0.03280839895013198948, -0.6692913385826773087, -0.1292274648535924053 ) ) ;
#5846=CARTESIAN_POINT ( 'NONE',  ( -0.6496062992125976043, 0.1660481256975883391, -0.3530559997133364547 ) ) ;
#5847=CARTESIAN_POINT ( 'NONE',  ( 1.292650918635171564, 0.1771653543307087630, 0.09757992244046791164 ) ) ;
#5849=ORIENTED_EDGE ( 'NONE', *, *, #24051, .T. ) ;
#5851=ORIENTED_EDGE ( 'NONE', *, *, #79270, .T. ) ;
#5852=CARTESIAN_POINT ( 'NONE',  ( 0.5249343832021003964, 0.2306618581243847221, -0.2411417322834647770 ) ) ;
#5853=CARTESIAN_POINT ( 'NONE',  ( -0.8070866141732276899, -0.5400638737290844871, 0.3530559997133364547 ) ) ;
#5854=CARTESIAN_POINT ( 'NONE',  ( -1.384514435695537005, -0.6692913385826773087, -0.1292274648535924053 ) ) ;
#5855=CARTESIAN_POINT ( 'NONE',  ( 0.4921259842519691285, -0.5400638737290845981, -0.3530559997133363437 ) ) ;
#5857=CARTESIAN_POINT ( 'NONE',  ( -1.522309711286088607, -0.5023911411419708095, 0.1820866141732285504 ) ) ;
#5858=CARTESIAN_POINT ( 'NONE',  ( 1.587926509186352142, 0.05413385826771666132, 0.4176697321401328100 ) ) ;
#5859=CARTESIAN_POINT ( 'NONE',  ( 8.195543980992789655E-16, -0.1870078740157480879, -0.4822834645669291653 ) ) ;
#5860=CARTESIAN_POINT ( 'NONE',  ( -1.443569553805773564, 0.2306618581243847221, -0.2411417322834647770 ) ) ;
#5861=CARTESIAN_POINT ( 'NONE',  ( 1.574803149606299746, -0.1870078740157479769, 0.4822834645669291653 ) ) ;
#5864=CARTESIAN_POINT ( 'NONE',  ( 0.7217847769028878924, -0.004921259842519576551, 0.3153832671262227771 ) ) ;
#5867=ORIENTED_EDGE ( 'NONE', *, *, #17807, .T. ) ;
#5868=CARTESIAN_POINT ( 'NONE',  ( -0.2296587926509179312, -0.2845877964562161244, -0.3641732283464567121 ) ) ;
#5870=CARTESIAN_POINT ( 'NONE',  ( 0.1902887139107617975, 0.2952755905511811885, 0.1292274648535926551 ) ) ;
#5871=CARTESIAN_POINT ( 'NONE',  ( 0.5643044619422579178, -0.4281496062992127816, -0.4176697321401328100 ) ) ;
#5873=CARTESIAN_POINT ( 'NONE',  ( -0.6299212598425188991, -0.1870078740157479769, 0.4822834645669291653 ) ) ;
#5876=CARTESIAN_POINT ( 'NONE',  ( -1.227034120734907141, -0.6692913385826773087, -0.1292274648535924053 ) ) ;
#5877=PRODUCT_DEFINITION ( 'UNKNOWN', '', #73237, #9976 ) ;
#5879=CARTESIAN_POINT ( 'NONE',  ( 1.207349081364829990, -0.5023911411419708095, -0.1820866141732282451 ) ) ;
#5880=CARTESIAN_POINT ( 'NONE',  ( 1.017060367454068803, -0.3162353388693405765, 0.4822834645669290543 ) ) ;
#5881=CARTESIAN_POINT ( 'NONE',  ( 0.9645669291338591078, -0.5400638737290845981, -0.3530559997133363437 ) ) ;
#5883=CARTESIAN_POINT ( 'NONE',  ( -1.181102362204723644, -0.1870078740157480879, -0.4822834645669291653 ) ) ;
#5886=CARTESIAN_POINT ( 'NONE',  ( -0.3149606299212590610, -0.1870078740157479769, 0.4822834645669291653 ) ) ;
#5890=CARTESIAN_POINT ( 'NONE',  ( 1.089238845144357537, -0.4281496062992124485, 0.4176697321401328655 ) ) ;
#5891=CARTESIAN_POINT ( 'NONE',  ( 1.338582677165355062, -0.1870078740157479769, 0.4822834645669291653 ) ) ;
#5892=CARTESIAN_POINT ( 'NONE',  ( 0.3412073490813655186, -0.5023911411419708095, -0.1820866141732282451 ) ) ;
#5893=CARTESIAN_POINT ( 'NONE',  ( 0.9120734908136489683, -0.6692913385826771977, 0.1292274648535927661 ) ) ;
#5895=CARTESIAN_POINT ( 'NONE',  ( 0.4527559055118117182, 0.07958543189024071263, -0.2665933059059888421 ) ) ;
#5897=CARTESIAN_POINT ( 'NONE',  ( 0.4986876640419954376, 0.2306618581243848609, 0.2411417322834645549 ) ) ;
#5899=CARTESIAN_POINT ( 'NONE',  ( -0.7611548556430438595, 0.2306618581243848609, 0.2411417322834645549 ) ) ;
#5900=CARTESIAN_POINT ( 'NONE',  ( 0.9186351706036751663, -0.5023911411419708095, 0.1820866141732285504 ) ) ;
#5901=EDGE_CURVE ( 'NONE', #68517, #51509, #31698, .T. ) ;
#5903=CARTESIAN_POINT ( 'NONE',  ( -0.1312335958005241554, 0.2306618581243848609, 0.2411417322834645549 ) ) ;
#5904=CARTESIAN_POINT ( 'NONE',  ( 0.2165354330708668673, -0.4536011799217367080, 0.2665933059059888421 ) ) ;
#5906=CARTESIAN_POINT ( 'NONE',  ( -0.3149606299212590610, -0.1870078740157479769, 0.4822834645669291653 ) ) ;
#5907=CARTESIAN_POINT ( 'NONE',  ( 0.5118110236220478892, 0.1771653543307087630, 0.000000000000000000 ) ) ;
#5909=CARTESIAN_POINT ( 'NONE',  ( -0.1771653543307080136, 0.1660481256975883668, -0.3530559997133364547 ) ) ;
#5910=CARTESIAN_POINT ( 'NONE',  ( 1.030183727034121421, -0.08942795157527998196, 0.3641732283464567121 ) ) ;
#5911=CARTESIAN_POINT ( 'NONE',  ( 0.2099737532808405305, 0.2306618581243847221, -0.2411417322834647770 ) ) ;
#5912=CARTESIAN_POINT ( 'NONE',  ( -0.2230971128608915943, -0.3690944881889765550, -0.3153832671262227771 ) ) ;
#5913=CARTESIAN_POINT ( 'NONE',  ( -0.7545931758530177724, 0.1771653543307087630, 0.09757992244046791164 ) ) ;
#5914=CARTESIAN_POINT ( 'NONE',  ( -0.1902887139107604098, 0.2952755905511810774, -0.1292274648535930714 ) ) ;
#5915=CARTESIAN_POINT ( 'NONE',  ( 0.08530183727034192087, -0.3162353388693409650, -0.4822834645669289433 ) ) ;
#5916=CARTESIAN_POINT ( 'NONE',  ( 1.017060367454068803, -0.2845877964562159024, 0.3641732283464567677 ) ) ;
#5918=CARTESIAN_POINT ( 'NONE',  ( 1.522309711286089939, -0.5023911411419708095, -0.1820866141732282451 ) ) ;
#5919=AXIS2_PLACEMENT_3D ( 'NONE', #1142, #19644, #27208 ) ;
#5920=EDGE_CURVE ( 'NONE', #57945, #32176, #21821, .T. ) ;
#5921=CARTESIAN_POINT ( 'NONE',  ( 0.8333333333333340365, -0.6692913385826771977, 0.1292274648535927661 ) ) ;
#5923=CARTESIAN_POINT ( 'NONE',  ( -0.3937007874015740483, -0.1870078740157480879, -0.4822834645669291653 ) ) ;
#5925=CARTESIAN_POINT ( 'NONE',  ( 0.7677165354330716118, 0.1660481256975883668, -0.3530559997133364547 ) ) ;
#5926=CARTESIAN_POINT ( 'NONE',  ( 0.7217847769028878924, 0.05413385826771666132, 0.4176697321401328100 ) ) ;
#5928=CARTESIAN_POINT ( 'NONE',  ( 0.5314960629921267055, -0.4536011799217367080, 0.2665933059059888421 ) ) ;
#5929=CARTESIAN_POINT ( 'NONE',  ( 1.174540682414699111, -0.3162353388693405765, 0.4822834645669290543 ) ) ;
#5930=EDGE_CURVE ( 'NONE', #47146, #19860, #59885, .T. ) ;
#5931=CARTESIAN_POINT ( 'NONE',  ( -0.1706036745406816491, -0.3690944881889763329, 0.3153832671262228327 ) ) ;
#5933=CARTESIAN_POINT ( 'NONE',  ( -0.3215223097112853146, -0.05778040916215560624, -0.4822834645669293319 ) ) ;
#5935=CARTESIAN_POINT ( 'NONE',  ( 0.3215223097112867578, -0.05778040916215522460, 0.4822834645669289988 ) ) ;
#5936=CARTESIAN_POINT ( 'NONE',  ( -0.9448818897637790704, -0.1870078740157480879, -0.4822834645669291653 ) ) ;
#5937=CARTESIAN_POINT ( 'NONE',  ( -0.8595800524934373854, -0.2845877964562161244, -0.3641732283464567121 ) ) ;
#5938=CARTESIAN_POINT ( 'NONE',  ( 0.5708661417322841158, -0.5400638737290845981, -0.3530559997133363437 ) ) ;
#5939=CARTESIAN_POINT ( 'NONE',  ( -1.404199475065615932, 0.05413385826771666132, 0.4176697321401328100 ) ) ;
#5940=CARTESIAN_POINT ( 'NONE',  ( -0.5577427821522301654, -0.3162353388693405765, 0.4822834645669290543 ) ) ;
#5941=ADVANCED_FACE ( 'NONE', ( #19933 ), #46836, .F. ) ;
#5944=CARTESIAN_POINT ( 'NONE',  ( 1.233595800524935227, -0.6046776061558807314, 0.2411417322834647770 ) ) ;
#5945=CARTESIAN_POINT ( 'NONE',  ( 1.318897637795276356, -0.5400638737290844871, 0.3530559997133364547 ) ) ;
#5947=CARTESIAN_POINT ( 'NONE',  ( -1.614173228346455824, 0.2952755905511811885, 0.000000000000000000 ) ) ;
#5948=CARTESIAN_POINT ( 'NONE',  ( -1.010498687664041384, -0.4281496062992127816, -0.4176697321401328100 ) ) ;
#5951=VERTEX_POINT ( 'NONE', #45582 ) ;
#5952=CARTESIAN_POINT ( 'NONE',  ( -0.07874015748031421014, -0.1870078740157479769, 0.3641732283464567677 ) ) ;
#5954=CARTESIAN_POINT ( 'NONE',  ( 0.6627296587926515548, 0.2952755905511811885, 0.1292274648535926551 ) ) ;
#5955=DIRECTION ( 'NONE',  ( 0.7071067811865454633, 0.000000000000000000, 0.7071067811865495711 ) ) ;
#5956=CARTESIAN_POINT ( 'NONE',  ( -1.604771003085130765, 0.4934440724007105872, 0.1466069496707737840 ) ) ;
#5957=CARTESIAN_POINT ( 'NONE',  ( -0.6561679790026240244, 0.1283753931104746893, -0.1820866141732285504 ) ) ;
#5959=CARTESIAN_POINT ( 'NONE',  ( 0.9908136482939640111, -0.6692913385826771977, 0.1292274648535927661 ) ) ;
#5960=CARTESIAN_POINT ( 'NONE',  ( 1.128608923884514947, 0.1283753931104748280, 0.1820866141732283561 ) ) ;
#5961=CARTESIAN_POINT ( 'NONE',  ( 0.05905511811023709395, -0.5400638737290844871, 0.3530559997133364547 ) ) ;
#5963=CARTESIAN_POINT ( 'NONE',  ( -0.3215223097112853146, -0.05778040916215560624, -0.4822834645669293319 ) ) ;
#5964=CARTESIAN_POINT ( 'NONE',  ( -1.522309711286088607, 0.1283753931104746893, -0.1820866141732285504 ) ) ;
#5965=CARTESIAN_POINT ( 'NONE',  ( -0.4133858267716528645, 0.1660481256975883668, -0.3530559997133364547 ) ) ;
#5966=CARTESIAN_POINT ( 'NONE',  ( 1.581364829396326277, -0.3162353388693409650, -0.4822834645669289433 ) ) ;
#5967=B_SPLINE_CURVE_WITH_KNOTS ( 'NONE', 3,
 ( #44372, #70064, #32181, #70908 ),
 .UNSPECIFIED., .F., .F.,
 ( 4, 4 ),
 ( 0.03467931754515478360, 0.03492726069669743055 ),
 .UNSPECIFIED. ) ;
#5971=CARTESIAN_POINT ( 'NONE',  ( 0.3608923884514443348, -0.6692913385826771977, 0.1292274648535927661 ) ) ;
#5973=CARTESIAN_POINT ( 'NONE',  ( -0.6167979002624665030, 0.05413385826771666132, 0.4176697321401328100 ) ) ;
#5974=CARTESIAN_POINT ( 'NONE',  ( -1.318897637795274802, 0.1660481256975885056, 0.3530559997133364547 ) ) ;
#5975=CARTESIAN_POINT ( 'NONE',  ( 0.6299212598425204535, -0.1870078740157479769, 0.4822834645669291653 ) ) ;
#5976=CARTESIAN_POINT ( 'NONE',  ( -0.1049868766404193215, -0.6046776061558807314, 0.2411417322834647770 ) ) ;
#5978=CARTESIAN_POINT ( 'NONE',  ( -0.7152230971128602510, -0.05778040916215560624, -0.4822834645669293319 ) ) ;
#5979=CARTESIAN_POINT ( 'NONE',  ( -0.2230971128608915943, 0.05413385826771666132, 0.4176697321401328100 ) ) ;
#5980=CARTESIAN_POINT ( 'NONE',  ( -1.043307086614172041, -0.5400638737290844871, 0.3530559997133364547 ) ) ;
#5982=CARTESIAN_POINT ( 'NONE',  ( -0.2624671916010490880, -0.5023911411419708095, 0.1820866141732285504 ) ) ;
#5984=CARTESIAN_POINT ( 'NONE',  ( 0.1115485564304467270, -0.6692913385826773087, -0.1292274648535924053 ) ) ;
#5986=CARTESIAN_POINT ( 'NONE',  ( 1.240157480314961314, -0.5400638737290844871, 0.3530559997133364547 ) ) ;
#5988=ORIENTED_EDGE ( 'NONE', *, *, #1342, .T. ) ;
#5990=CARTESIAN_POINT ( 'NONE',  ( 0.1246719160104994284, 0.2952755905511810774, -0.1292274648535930714 ) ) ;
#5991=CARTESIAN_POINT ( 'NONE',  ( -0.01312335958005186876, -0.3690944881889763329, 0.3153832671262228327 ) ) ;
#5992=CARTESIAN_POINT ( 'NONE',  ( 1.620734908136483465, -0.5511811023622046335, 0.09757992244046803654 ) ) ;
#5993=FACE_OUTER_BOUND ( 'NONE', #26791, .T. ) ;
#5996=CARTESIAN_POINT ( 'NONE',  ( 1.489501312335958172, -0.2845877964562159024, 0.3641732283464567677 ) ) ;
#5998=CARTESIAN_POINT ( 'NONE',  ( -1.633858267716534529, 0.1660481256975885056, 0.3530559997133364547 ) ) ;
#6001=CARTESIAN_POINT ( 'NONE',  ( 0.5774278215223103139, -0.6046776061558809534, -0.2411417322834644161 ) ) ;
#6002=CARTESIAN_POINT ( 'NONE',  ( -1.102362204724408601, -0.1870078740157480879, -0.4822834645669291653 ) ) ;
#6003=CARTESIAN_POINT ( 'NONE',  ( -1.286089238845143479, -0.6046776061558807314, 0.2411417322834647770 ) ) ;
#6004=CARTESIAN_POINT ( 'NONE',  ( 0.2296587926509192634, -0.05778040916215560624, -0.4822834645669293319 ) ) ;
#6005=CARTESIAN_POINT ( 'NONE',  ( 1.069553805774278610, -0.6692913385826771977, 0.1292274648535927661 ) ) ;
#6006=CARTESIAN_POINT ( 'NONE',  ( 1.443569553805774897, -0.5023911411419708095, -0.1820866141732282451 ) ) ;
#6008=CARTESIAN_POINT ( 'NONE',  ( 0.9514435695538062676, -0.2845877964562161244, -0.3641732283464567121 ) ) ;
#6009=CARTESIAN_POINT ( 'NONE',  ( -0.9186351706036736120, -0.6046776061558809534, -0.2411417322834644161 ) ) ;
#6011=CARTESIAN_POINT ( 'NONE',  ( -1.627296587926508442, 0.1283753931104748280, 0.1820866141732283561 ) ) ;
#6013=CARTESIAN_POINT ( 'NONE',  ( 0.7808398950131241190, -0.05778040916215560624, -0.4822834645669293319 ) ) ;
#6015=CARTESIAN_POINT ( 'NONE',  ( -1.666666666666665853, -0.004921259842519870586, -0.3153832671262229437 ) ) ;
#6016=CARTESIAN_POINT ( 'NONE',  ( 0.03280839895013198948, -0.6692913385826773087, -0.1292274648535924053 ) ) ;
#6017=CARTESIAN_POINT ( 'NONE',  ( 0.9448818897637802916, -0.1870078740157479769, 0.3641732283464567677 ) ) ;
#6018=CARTESIAN_POINT ( 'NONE',  ( 0.8202099737532814183, -0.6692913385826773087, -0.1292274648535924053 ) ) ;
#6020=CARTESIAN_POINT ( 'NONE',  ( -0.3608923884514428360, -0.5511811023622048555, -0.09757992244046775898 ) ) ;
#6021=CARTESIAN_POINT ( 'NONE',  ( -0.5774278215223089816, 0.2306618581243847221, -0.2411417322834647770 ) ) ;
#6022=CARTESIAN_POINT ( 'NONE',  ( 1.594488188976378673, -0.5400638737290845981, -0.3530559997133363437 ) ) ;
#6023=CARTESIAN_POINT ( 'NONE',  ( -1.312335958005248715, -0.6046776061558809534, -0.2411417322834644161 ) ) ;
#6024=CARTESIAN_POINT ( 'NONE',  ( 1.089238845144357759, 0.05413385826771626580, -0.4176697321401330321 ) ) ;
#6027=CARTESIAN_POINT ( 'NONE',  ( -1.135170603674539924, 0.1771653543307087075, -0.09757992244046823083 ) ) ;
#6029=CARTESIAN_POINT ( 'NONE',  ( 0.9186351706036751663, -0.6046776061558807314, 0.2411417322834647770 ) ) ;
#6031=CARTESIAN_POINT ( 'NONE',  ( -1.528871391076114250, 0.2952755905511810774, -0.1292274648535930714 ) ) ;
#6032=CARTESIAN_POINT ( 'NONE',  ( 1.653543307086614789, -0.1870078740157479769, 0.4822834645669291653 ) ) ;
#6033=CARTESIAN_POINT ( 'NONE',  ( -0.8858267716535425107, 0.07958543189024071263, -0.2665933059059888421 ) ) ;
#6034=CARTESIAN_POINT ( 'NONE',  ( 1.653543307086614789, -0.1870078740157479769, 0.3641732283464567677 ) ) ;
#6035=CARTESIAN_POINT ( 'NONE',  ( -0.5971128608923877978, -0.6692913385826773087, -0.1292274648535924053 ) ) ;
#6036=CARTESIAN_POINT ( 'NONE',  ( -0.5446194225721777693, -0.08942795157527998196, 0.3641732283464567121 ) ) ;
#6037=CARTESIAN_POINT ( 'NONE',  ( -1.666666666666665853, -0.004921259842519870586, -0.3153832671262229437 ) ) ;
#6038=CARTESIAN_POINT ( 'NONE',  ( 1.128608923884514947, 0.1283753931104748280, 0.1820866141732283561 ) ) ;
#6039=CARTESIAN_POINT ( 'NONE',  ( 0.7742782152230979209, 0.05413385826771626580, -0.4176697321401330321 ) ) ;
#6040=CARTESIAN_POINT ( 'NONE',  ( 1.594488188976378673, 0.1660481256975885056, 0.3530559997133364547 ) ) ;
#6041=CARTESIAN_POINT ( 'NONE',  ( -0.06561679790026180015, -0.004921259842519576551, 0.3153832671262227771 ) ) ;
#6043=CARTESIAN_POINT ( 'NONE',  ( 0.3871391076115493490, -0.3162353388693405765, 0.4822834645669290543 ) ) ;
#6044=CARTESIAN_POINT ( 'NONE',  ( 0.3805774278215230400, -0.004921259842519870586, -0.3153832671262229437 ) ) ;
#6045=CARTESIAN_POINT ( 'NONE',  ( 1.587926509186352142, 0.05413385826771666132, 0.4176697321401328100 ) ) ;
#6046=CARTESIAN_POINT ( 'NONE',  ( -1.358267716535432434, -0.5400638737290844871, 0.3530559997133364547 ) ) ;
#6047=CARTESIAN_POINT ( 'NONE',  ( -0.4527559055118102749, 0.1660481256975885056, 0.3530559997133364547 ) ) ;
#6050=CARTESIAN_POINT ( 'NONE',  ( 0.6299212598425204535, -0.1870078740157479769, 0.4822834645669291653 ) ) ;
#6051=CARTESIAN_POINT ( 'NONE',  ( 1.095800524934383846, -0.2845877964562159024, 0.3641732283464567677 ) ) ;
#6052=CARTESIAN_POINT ( 'NONE',  ( -0.4921259842519677963, 0.1660481256975883668, -0.3530559997133364547 ) ) ;
#6053=CARTESIAN_POINT ( 'NONE',  ( 0.2034120734908142214, 0.2952755905511810774, -0.1292274648535930714 ) ) ;
#6055=AXIS2_PLACEMENT_3D ( 'NONE', #41101, #74340, #73517 ) ;
#6060=CARTESIAN_POINT ( 'NONE',  ( -0.5643044619422565855, -0.004921259842519870586, -0.3153832671262229437 ) ) ;
#6061=CARTESIAN_POINT ( 'NONE',  ( -1.076115485564303809, 0.2306618581243848609, 0.2411417322834645549 ) ) ;
#6063=CARTESIAN_POINT ( 'NONE',  ( 0.9448818897637802916, -0.1870078740157480879, -0.4822834645669291653 ) ) ;
#6064=CARTESIAN_POINT ( 'NONE',  ( 1.167979002624672580, 0.05413385826771626580, -0.4176697321401330321 ) ) ;
#6065=CARTESIAN_POINT ( 'NONE',  ( 0.6102362204724416372, -0.5400638737290844871, 0.3530559997133364547 ) ) ;
#6069=CARTESIAN_POINT ( 'NONE',  ( 0.6627296587926515548, 0.2952755905511811885, 0.1292274648535926551 ) ) ;
#6070=CARTESIAN_POINT ( 'NONE',  ( 0.7349081364829402885, -0.6046776061558809534, -0.2411417322834644161 ) ) ;
#6071=CARTESIAN_POINT ( 'NONE',  ( 0.8792650918635177559, -0.3690944881889765550, -0.3153832671262227771 ) ) ;
#6072=CARTESIAN_POINT ( 'NONE',  ( 1.384514435695538559, 0.2952755905511810774, -0.1292274648535930714 ) ) ;
#6074=CARTESIAN_POINT ( 'NONE',  ( 0.3937007874015754361, -0.1870078740157480879, -0.4822834645669291653 ) ) ;
#6075=CARTESIAN_POINT ( 'NONE',  ( 1.246719160104987623, 0.05413385826771626580, -0.4176697321401330321 ) ) ;
#6076=CARTESIAN_POINT ( 'NONE',  ( 0.5643044619422579178, 0.05413385826771666132, 0.4176697321401328100 ) ) ;
#6077=CARTESIAN_POINT ( 'NONE',  ( -0.7426113562972006532, 2.209901789876323797, -0.5309055118110235227 ) ) ;
#6078=CARTESIAN_POINT ( 'NONE',  ( -0.8792650918635160906, 0.05413385826771626580, -0.4176697321401330321 ) ) ;
#6079=CARTESIAN_POINT ( 'NONE',  ( -0.9448818897637790704, -0.1870078740157479769, 0.4822834645669291653 ) ) ;
#6080=CARTESIAN_POINT ( 'NONE',  ( 1.318897637795276356, 0.1660481256975883668, -0.3530559997133364547 ) ) ;
#6088=CARTESIAN_POINT ( 'NONE',  ( 1.377952755905512472, -0.5511811023622047445, 6.969142054262312111E-17 ) ) ;
#6090=CARTESIAN_POINT ( 'NONE',  ( 1.220472440944882608, 0.1771653543307087630, 0.000000000000000000 ) ) ;
#6096=CARTESIAN_POINT ( 'NONE',  ( -0.6167979002624665030, -0.3690944881889765550, -0.3153832671262227771 ) ) ;
#6097=CARTESIAN_POINT ( 'NONE',  ( -1.463254593175852492, -0.5511811023622048555, -0.09757992244046775898 ) ) ;
#6098=CARTESIAN_POINT ( 'NONE',  ( -1.325459317585300889, 0.05413385826771666132, 0.4176697321401328100 ) ) ;
#6099=CARTESIAN_POINT ( 'NONE',  ( 0.07874015748031558404, -0.1870078740157480879, -0.4822834645669291653 ) ) ;
#6100=CARTESIAN_POINT ( 'NONE',  ( -1.581364829396324945, -0.05778040916215560624, -0.4822834645669293319 ) ) ;
#6101=VERTEX_POINT ( 'NONE', #48079 ) ;
#6105=CARTESIAN_POINT ( 'NONE',  ( -1.595398199321656385, 1.564277624879635509, 0.1559797534342483860 ) ) ;
#6106=CARTESIAN_POINT ( 'NONE',  ( -0.4658792650918627265, -0.2845877964562161244, -0.3641732283464567121 ) ) ;
#6107=CARTESIAN_POINT ( 'NONE',  ( -1.128608923884513837, 0.2306618581243847221, -0.2411417322834647770 ) ) ;
#6108=CARTESIAN_POINT ( 'NONE',  ( 1.056430446194226658, 0.2952755905511811885, 0.1292274648535926551 ) ) ;
#6109=AXIS2_PLACEMENT_3D ( 'NONE', #66614, #8951, #63175 ) ;
#6111=CARTESIAN_POINT ( 'NONE',  ( -1.614173228346457378, 0.5038684218300933937, -0.1372047244094477536 ) ) ;
#6113=CARTESIAN_POINT ( 'NONE',  ( 1.076115485564305141, 0.2306618581243847221, -0.2411417322834647770 ) ) ;
#6114=CARTESIAN_POINT ( 'NONE',  ( -1.135170603674539924, -0.6692913385826771977, 0.1292274648535927661 ) ) ;
#6116=CARTESIAN_POINT ( 'NONE',  ( -0.5052493438320203589, -0.5511811023622046335, 0.09757992244046803654 ) ) ;
#6118=CARTESIAN_POINT ( 'NONE',  ( -0.7020997375328074108, -0.08942795157527998196, 0.3641732283464567121 ) ) ;
#6119=CARTESIAN_POINT ( 'NONE',  ( -0.08530183727034056085, -0.08942795157528024563, -0.3641732283464568787 ) ) ;
#6120=CARTESIAN_POINT ( 'NONE',  ( 5.463695987328526437E-16, -0.1870078740157479769, 0.4822834645669291653 ) ) ;
#6121=CARTESIAN_POINT ( 'NONE',  ( -0.8267716535433065062, 0.1771653543307087630, 0.000000000000000000 ) ) ;
#6123=CARTESIAN_POINT ( 'NONE',  ( 1.266404199475066328, -0.05778040916215522460, 0.4822834645669289988 ) ) ;
#6124=CARTESIAN_POINT ( 'NONE',  ( -1.423884514435694859, -0.05778040916215560624, -0.4822834645669293319 ) ) ;
#6126=CARTESIAN_POINT ( 'NONE',  ( -0.3543307086614165824, -0.6692913385826771977, 8.415575281601705876E-17 ) ) ;
#6127=CARTESIAN_POINT ( 'NONE',  ( -1.135170603674539924, 0.2952755905511810774, -0.1292274648535930714 ) ) ;
#6128=CARTESIAN_POINT ( 'NONE',  ( 1.384514435695538559, 0.1771653543307087075, -0.09757992244046823083 ) ) ;
#6129=CARTESIAN_POINT ( 'NONE',  ( -0.4068241469816267775, -0.004921259842519870586, -0.3153832671262229437 ) ) ;
#6130=CARTESIAN_POINT ( 'NONE',  ( -0.7152230971128602510, -0.05778040916215560624, -0.4822834645669293319 ) ) ;
#6131=CARTESIAN_POINT ( 'NONE',  ( -1.141732283464566011, 0.2952755905511811885, 0.000000000000000000 ) ) ;
#6133=CARTESIAN_POINT ( 'NONE',  ( 1.095800524934383846, -0.08942795157528024563, -0.3641732283464568787 ) ) ;
#6134=CARTESIAN_POINT ( 'NONE',  ( -0.1837270341207340729, 0.2306618581243847221, -0.2411417322834647770 ) ) ;
#6135=CARTESIAN_POINT ( 'NONE',  ( -1.712598425196849572, 0.1660481256975885056, 0.3530559997133364547 ) ) ;
#6138=CARTESIAN_POINT ( 'NONE',  ( -0.8005249343832011588, -0.004921259842519870586, -0.3153832671262229437 ) ) ;
#6139=CARTESIAN_POINT ( 'NONE',  ( 1.069553805774278610, -0.6692913385826771977, 0.1292274648535927661 ) ) ;
#6140=CARTESIAN_POINT ( 'NONE',  ( -1.003937007874015297, -0.4536011799217368745, -0.2665933059059886201 ) ) ;
#6142=CARTESIAN_POINT ( 'NONE',  ( -0.8070866141732276899, -0.5400638737290844871, 0.3530559997133364547 ) ) ;
#6143=VECTOR ( 'NONE', #26306, 39.37007874015748143 ) ;
#6144=CARTESIAN_POINT ( 'NONE',  ( 0.8595800524934390507, -0.3162353388693405765, 0.4822834645669290543 ) ) ;
#6145=CARTESIAN_POINT ( 'NONE',  ( 0.8661417322834653598, -0.1870078740157479769, 0.4822834645669291653 ) ) ;
#6147=CARTESIAN_POINT ( 'NONE',  ( -1.620734908136482577, -0.5511811023622048555, -0.09757992244046775898 ) ) ;
#6152=CARTESIAN_POINT ( 'NONE',  ( 1.325459317585302665, -0.3690944881889763329, 0.3153832671262228327 ) ) ;
#6153=CARTESIAN_POINT ( 'NONE',  ( 0.7545931758530188826, -0.5511811023622046335, 0.09757992244046803654 ) ) ;
#6154=CARTESIAN_POINT ( 'NONE',  ( 0.2034120734908142214, 0.2952755905511810774, -0.1292274648535930714 ) ) ;
#6157=CARTESIAN_POINT ( 'NONE',  ( 0.8333333333333340365, -0.5511811023622046335, 0.09757992244046803654 ) ) ;
#6158=CARTESIAN_POINT ( 'NONE',  ( -0.4986876640419939388, 0.2306618581243847221, -0.2411417322834647770 ) ) ;
#6159=CARTESIAN_POINT ( 'NONE',  ( -1.299212598425196097, 0.2952755905511811885, 0.000000000000000000 ) ) ;
#6160=CARTESIAN_POINT ( 'NONE',  ( 0.7480314960629927956, 0.2952755905511811885, 0.000000000000000000 ) ) ;
#6163=VERTEX_POINT ( 'NONE', #48908 ) ;
#6165=CARTESIAN_POINT ( 'NONE',  ( -1.318897637795274802, -0.5400638737290845981, -0.3530559997133363437 ) ) ;
#6166=CARTESIAN_POINT ( 'NONE',  ( -0.4199475065616791736, -0.6046776061558807314, 0.2411417322834647770 ) ) ;
#6167=CARTESIAN_POINT ( 'NONE',  ( -0.7349081364829387342, -0.5023911411419708095, 0.1820866141732285504 ) ) ;
#6168=CARTESIAN_POINT ( 'NONE',  ( -0.5839895013123351797, -0.6692913385826771977, 0.1292274648535927661 ) ) ;
#6170=CARTESIAN_POINT ( 'NONE',  ( -0.3280839895013117347, 0.05413385826771626580, -0.4176697321401330321 ) ) ;
#6171=CARTESIAN_POINT ( 'NONE',  ( 1.581364829396326277, -0.05778040916215522460, 0.4822834645669289988 ) ) ;
#6172=CARTESIAN_POINT ( 'NONE',  ( -0.7020997375328076329, -0.3162353388693409650, -0.4822834645669289433 ) ) ;
#6173=CARTESIAN_POINT ( 'NONE',  ( 0.2362204724409456558, -0.1870078740157480879, -0.4822834645669291653 ) ) ;
#6174=CARTESIAN_POINT ( 'NONE',  ( -0.8792650918635160906, -0.4281496062992124485, 0.4176697321401328655 ) ) ;
#6177=CARTESIAN_POINT ( 'NONE',  ( -0.6758530183727028406, 0.1771653543307087630, 0.09757992244046791164 ) ) ;
#6181=CARTESIAN_POINT ( 'NONE',  ( -1.686351706036744558, 0.1771653543307087075, -0.09757992244046823083 ) ) ;
#6182=CARTESIAN_POINT ( 'NONE',  ( -1.207349081364828436, -0.6046776061558807314, 0.2411417322834647770 ) ) ;
#6183=CARTESIAN_POINT ( 'NONE',  ( -1.036745406824146176, -0.4281496062992124485, 0.4176697321401328655 ) ) ;
#6185=CARTESIAN_POINT ( 'NONE',  ( -1.207349081364828880, 0.2306618581243847221, -0.2411417322834647770 ) ) ;
#6186=CARTESIAN_POINT ( 'NONE',  ( -1.089238845144356427, 0.05413385826771666132, 0.4176697321401328100 ) ) ;
#6187=DIRECTION ( 'NONE',  ( -1.000000000000000000, -0.000000000000000000, 1.692413147294446216E-16 ) ) ;
#6188=CARTESIAN_POINT ( 'NONE',  ( -1.646051170424378096, -0.1870078740157480046, 1.254653134982923898E-17 ) ) ;
#6189=CARTESIAN_POINT ( 'NONE',  ( 0.4855643044619430415, -0.3690944881889765550, -0.3153832671262227771 ) ) ;
#6192=CARTESIAN_POINT ( 'NONE',  ( -0.3805774278215216522, -0.3690944881889765550, -0.3153832671262227771 ) ) ;
#6193=CARTESIAN_POINT ( 'NONE',  ( -0.5971128608923877978, -0.6692913385826773087, -0.1292274648535924053 ) ) ;
#6194=CARTESIAN_POINT ( 'NONE',  ( 1.469816272965879911, 0.2306618581243847221, -0.2411417322834647770 ) ) ;
#6195=CARTESIAN_POINT ( 'NONE',  ( -0.3477690288713902178, 0.2952755905511810774, -0.1292274648535930714 ) ) ;
#6199=CARTESIAN_POINT ( 'NONE',  ( -0.5839895013123351797, -0.6692913385826771977, 0.1292274648535927661 ) ) ;
#6200=CARTESIAN_POINT ( 'NONE',  ( 1.371391076115485719, -0.6692913385826773087, -0.1292274648535924053 ) ) ;
#6201=CARTESIAN_POINT ( 'NONE',  ( -0.9645669291338575535, -0.4536011799217367080, 0.2665933059059888421 ) ) ;
#6202=CARTESIAN_POINT ( 'NONE',  ( -1.299212598425196097, -0.6692913385826771977, 8.415575281601705876E-17 ) ) ;
#6208=CARTESIAN_POINT ( 'NONE',  ( 0.03280839895013198948, -0.6692913385826773087, -0.1292274648535924053 ) ) ;
#6209=CARTESIAN_POINT ( 'NONE',  ( -0.9186351706036736120, -0.5023911411419708095, -0.1820866141732282451 ) ) ;
#6211=CARTESIAN_POINT ( 'NONE',  ( -0.6824146981627291497, -0.6046776061558809534, -0.2411417322834644161 ) ) ;
#6213=CARTESIAN_POINT ( 'NONE',  ( -0.8923884514435688198, 0.2306618581243847221, -0.2411417322834647770 ) ) ;
#6214=CARTESIAN_POINT ( 'NONE',  ( -1.122047244094487306, -0.5400638737290844871, 0.3530559997133364547 ) ) ;
#6216=CARTESIAN_POINT ( 'NONE',  ( 0.8923884514435701520, -0.5023911411419708095, -0.1820866141732282451 ) ) ;
#6217=CARTESIAN_POINT ( 'NONE',  ( -0.8333333333333323711, -0.5511811023622048555, -0.09757992244046775898 ) ) ;
#6218=CARTESIAN_POINT ( 'NONE',  ( 0.6167979002624679463, -0.004921259842519870586, -0.3153832671262229437 ) ) ;
#6219=CARTESIAN_POINT ( 'NONE',  ( -1.699475065616797398, 0.2952755905511811885, 0.1292274648535926551 ) ) ;
#6220=CARTESIAN_POINT ( 'NONE',  ( 1.443569553805774897, 0.2306618581243848609, 0.2411417322834645549 ) ) ;
#6221=CARTESIAN_POINT ( 'NONE',  ( 0.4724409448818904789, -0.1870078740157480601, -0.3641732283464567677 ) ) ;
#6223=CARTESIAN_POINT ( 'NONE',  ( -0.7480314960629914633, -0.6692913385826771977, 8.415575281601705876E-17 ) ) ;
#6224=CARTESIAN_POINT ( 'NONE',  ( 1.135170603674541256, 0.2952755905511811885, 0.1292274648535926551 ) ) ;
#6227=CARTESIAN_POINT ( 'NONE',  ( -0.2559055118110227234, -0.4536011799217367080, 0.2665933059059888421 ) ) ;
#6229=CARTESIAN_POINT ( 'NONE',  ( 0.5183727034120741983, -0.6692913385826771977, 0.1292274648535927661 ) ) ;
#6230=CARTESIAN_POINT ( 'NONE',  ( 1.141732283464567566, 0.1771653543307087630, 0.000000000000000000 ) ) ;
#6231=CARTESIAN_POINT ( 'NONE',  ( 0.1115485564304467270, -0.5511811023622048555, -0.09757992244046775898 ) ) ;
#6232=CARTESIAN_POINT ( 'NONE',  ( -0.07217847769028787330, -0.05778040916215522460, 0.4822834645669289988 ) ) ;
#6233=CARTESIAN_POINT ( 'NONE',  ( -1.377952755905511140, 0.2952755905511811885, 0.000000000000000000 ) ) ;
#6234=CARTESIAN_POINT ( 'NONE',  ( -0.8530183727034112984, -0.004921259842519576551, 0.3153832671262227771 ) ) ;
#6235=DIRECTION ( 'NONE',  ( 0.000000000000000000, 0.000000000000000000, 1.000000000000000000 ) ) ;
#6236=CARTESIAN_POINT ( 'NONE',  ( -0.3937007874015740483, -0.1870078740157479769, 0.4822834645669291653 ) ) ;
#6239=CARTESIAN_POINT ( 'NONE',  ( 0.07217847769028949700, -0.08942795157528024563, -0.3641732283464568787 ) ) ;
#6240=CARTESIAN_POINT ( 'NONE',  ( -0.4855643044619415427, 0.05413385826771626580, -0.4176697321401330321 ) ) ;
#6241=CARTESIAN_POINT ( 'NONE',  ( -1.266404199475064773, -0.05778040916215560624, -0.4822834645669293319 ) ) ;
#6242=CARTESIAN_POINT ( 'NONE',  ( -0.6758530183727028406, 0.1771653543307087630, 0.09757992244046791164 ) ) ;
#6244=CARTESIAN_POINT ( 'NONE',  ( -0.6430446194225712953, 0.05413385826771626580, -0.4176697321401330321 ) ) ;
#6245=CARTESIAN_POINT ( 'NONE',  ( -0.7217847769028863381, -0.3690944881889763329, 0.3153832671262228327 ) ) ;
#6246=CARTESIAN_POINT ( 'NONE',  ( -1.594488188976377563, -0.4536011799217367080, 0.2665933059059888421 ) ) ;
#6247=CARTESIAN_POINT ( 'NONE',  ( 1.299212598425197429, 0.2952755905511811885, 0.000000000000000000 ) ) ;
#6252=CARTESIAN_POINT ( 'NONE',  ( -1.240157480314959759, 0.1660481256975885056, 0.3530559997133364547 ) ) ;
#6253=CARTESIAN_POINT ( 'NONE',  ( -0.6758530183727028406, -0.6692913385826773087, -0.1292274648535924053 ) ) ;
#6254=CARTESIAN_POINT ( 'NONE',  ( 1.607611548556431069, 0.2952755905511811885, 0.1292274648535926551 ) ) ;
#6257=CARTESIAN_POINT ( 'NONE',  ( 1.102362204724410155, -0.1870078740157480879, -0.4822834645669291653 ) ) ;
#6258=CARTESIAN_POINT ( 'NONE',  ( -0.09186351706036663400, -0.4281496062992124485, 0.4176697321401328655 ) ) ;
#6261=VECTOR ( 'NONE', #17148, 39.37007874015748143 ) ;
#6263=CARTESIAN_POINT ( 'NONE',  ( 1.358267716535433323, -0.4536011799217368745, -0.2665933059059886201 ) ) ;
#6267=ORIENTED_EDGE ( 'NONE', *, *, #36825, .T. ) ;
#6268=CARTESIAN_POINT ( 'NONE',  ( 5.463695987328526437E-16, -0.1870078740157479769, 0.4822834645669291653 ) ) ;
#6269=CARTESIAN_POINT ( 'NONE',  ( -0.9120734908136475250, 0.2952755905511811885, 0.1292274648535926551 ) ) ;
#6270=CARTESIAN_POINT ( 'NONE',  ( -1.469816272965878357, 0.2306618581243848609, 0.2411417322834645549 ) ) ;
#6271=CARTESIAN_POINT ( 'NONE',  ( 0.5643044619422579178, 0.05413385826771666132, 0.4176697321401328100 ) ) ;
#6272=CARTESIAN_POINT ( 'NONE',  ( 1.437007874015748810, -0.5400638737290845981, -0.3530559997133363437 ) ) ;
#6273=CARTESIAN_POINT ( 'NONE',  ( 1.371391076115485719, -0.6692913385826773087, -0.1292274648535924053 ) ) ;
#6274=CARTESIAN_POINT ( 'NONE',  ( -0.4921259842519677963, 0.1660481256975883668, -0.3530559997133364547 ) ) ;
#6275=CARTESIAN_POINT ( 'NONE',  ( 0.3215223097112867578, -0.05778040916215522460, 0.4822834645669289988 ) ) ;
#6276=CARTESIAN_POINT ( 'NONE',  ( -1.154855643044618851, 0.2306618581243848609, 0.2411417322834645549 ) ) ;
#6277=CARTESIAN_POINT ( 'NONE',  ( 1.351706036745407458, -0.4281496062992127816, -0.4176697321401328100 ) ) ;
#6278=CARTESIAN_POINT ( 'NONE',  ( 1.568241469816273659, -0.05778040916215560624, -0.4822834645669293319 ) ) ;
#6279=CARTESIAN_POINT ( 'NONE',  ( 0.02624671916010564918, 0.2306618581243848609, 0.2411417322834645549 ) ) ;
#6281=CARTESIAN_POINT ( 'NONE',  ( 0.5118110236220480003, -0.5511811023622047445, 6.969142054262312111E-17 ) ) ;
#6285=CARTESIAN_POINT ( 'NONE',  ( -0.09186351706036689768, -0.004921259842519870586, -0.3153832671262229437 ) ) ;
#6286=B_SPLINE_CURVE_WITH_KNOTS ( 'NONE', 3,
 ( #29701, #5269, #56600, #56193 ),
 .UNSPECIFIED., .F., .F.,
 ( 4, 4 ),
 ( 9.341771812940338307E-18, 0.001510660848375616110 ),
 .UNSPECIFIED. ) ;
#6288=CARTESIAN_POINT ( 'NONE',  ( -0.05249343832020938322, -0.6046776061558809534, -0.2411417322834644161 ) ) ;
#6289=CARTESIAN_POINT ( 'NONE',  ( -0.1049868766404193215, 0.2306618581243847221, -0.2411417322834647770 ) ) ;
#6290=CARTESIAN_POINT ( 'NONE',  ( -0.3937007874015740483, -0.1870078740157480879, -0.4822834645669291653 ) ) ;
#6292=CARTESIAN_POINT ( 'NONE',  ( -1.332020997375327642, -0.05778040916215522460, 0.4822834645669289988 ) ) ;
#6294=CARTESIAN_POINT ( 'NONE',  ( 0.7152230971128614723, -0.2845877964562161244, -0.3641732283464567121 ) ) ;
#6295=CARTESIAN_POINT ( 'NONE',  ( 1.095800524934383846, -0.05778040916215560624, -0.4822834645669293319 ) ) ;
#6296=CARTESIAN_POINT ( 'NONE',  ( 0.8923884514435703741, 0.2306618581243848609, 0.2411417322834645549 ) ) ;
#6298=CARTESIAN_POINT ( 'NONE',  ( -1.391076115485563758, 0.2306618581243848609, 0.2411417322834645549 ) ) ;
#6301=CARTESIAN_POINT ( 'NONE',  ( -0.1115485564304456306, 0.2952755905511810774, -0.1292274648535930714 ) ) ;
#6304=CARTESIAN_POINT ( 'NONE',  ( 1.482939632545932307, 0.05413385826771626580, -0.4176697321401330321 ) ) ;
#6305=CARTESIAN_POINT ( 'NONE',  ( 1.213910761154856299, 0.2952755905511811885, 0.1292274648535926551 ) ) ;
#6306=CARTESIAN_POINT ( 'NONE',  ( 0.1443569553805781891, -0.004921259842519870586, -0.3153832671262229437 ) ) ;
#6307=CARTESIAN_POINT ( 'NONE',  ( 0.9317585301837276734, -0.4281496062992124485, 0.4176697321401328655 ) ) ;
#6309=CARTESIAN_POINT ( 'NONE',  ( 0.5249343832021005074, -0.5023911411419708095, 0.1820866141732285504 ) ) ;
#6310=CARTESIAN_POINT ( 'NONE',  ( 0.2559055118110243332, -0.5400638737290845981, -0.3530559997133363437 ) ) ;
#6312=CARTESIAN_POINT ( 'NONE',  ( -1.102362204724408601, -0.1870078740157479769, 0.4822834645669291653 ) ) ;
#6313=CARTESIAN_POINT ( 'NONE',  ( 0.9645669291338588858, 0.07958543189024085140, 0.2665933059059887866 ) ) ;
#6315=CARTESIAN_POINT ( 'NONE',  ( -0.1640419947506555343, -0.3162353388693405765, 0.4822834645669290543 ) ) ;
#6317=CARTESIAN_POINT ( 'NONE',  ( -0.2887139107611542133, -0.5023911411419708095, -0.1820866141732282451 ) ) ;
#6319=CARTESIAN_POINT ( 'NONE',  ( -0.4265091863517051496, 0.2952755905511810774, -0.1292274648535930714 ) ) ;
#6320=CARTESIAN_POINT ( 'NONE',  ( 0.3805774278215230400, -0.004921259842519870586, -0.3153832671262229437 ) ) ;
#6321=AXIS2_PLACEMENT_3D ( 'NONE', #26144, #18999, #70773 ) ;
#6323=CARTESIAN_POINT ( 'NONE',  ( 0.05905511811023709395, -0.5400638737290844871, 0.3530559997133364547 ) ) ;
#6329=CARTESIAN_POINT ( 'NONE',  ( 1.345144356955381593, -0.08942795157527998196, 0.3641732283464567121 ) ) ;
#6330=CARTESIAN_POINT ( 'NONE',  ( 1.607611548556431069, 0.2952755905511811885, 0.1292274648535926551 ) ) ;
#6331=CARTESIAN_POINT ( 'NONE',  ( -0.9711286089238838626, -0.5023911411419708095, 0.1820866141732285504 ) ) ;
#6332=CARTESIAN_POINT ( 'NONE',  ( -0.8727034120734901146, -0.08942795157528024563, -0.3641732283464568787 ) ) ;
#6333=CARTESIAN_POINT ( 'NONE',  ( -0.2427821522309703550, -0.3162353388693405765, 0.4822834645669290543 ) ) ;
#6334=CARTESIAN_POINT ( 'NONE',  ( -0.04593175853018302557, -0.6692913385826773087, -0.1292274648535924053 ) ) ;
#6335=CARTESIAN_POINT ( 'NONE',  ( 0.4593175853018380828, -0.004921259842519870586, -0.3153832671262229437 ) ) ;
#6337=CARTESIAN_POINT ( 'NONE',  ( 1.371391076115485719, -0.5511811023622048555, -0.09757992244046775898 ) ) ;
#6338=CARTESIAN_POINT ( 'NONE',  ( 0.6233595800524942554, -0.05778040916215560624, -0.4822834645669293319 ) ) ;
#6339=ADVANCED_FACE ( 'NONE', ( #67456 ), #35881, .F. ) ;
#6341=CARTESIAN_POINT ( 'NONE',  ( -0.2559055118110230564, 0.1660481256975883668, -0.3530559997133364547 ) ) ;
#6343=CARTESIAN_POINT ( 'NONE',  ( -1.574803149606298636, -0.1870078740157479769, 0.4822834645669291653 ) ) ;
#6344=CARTESIAN_POINT ( 'NONE',  ( 0.8792650918635177559, 0.05413385826771666132, 0.4176697321401328100 ) ) ;
#6345=CARTESIAN_POINT ( 'NONE',  ( 0.3805774278215230400, -0.4281496062992124485, 0.4176697321401328655 ) ) ;
#6348=CARTESIAN_POINT ( 'NONE',  ( 0.4068241469816281097, -0.004921259842519576551, 0.3153832671262227771 ) ) ;
#6349=CARTESIAN_POINT ( 'NONE',  ( 1.194225721784777594, 0.05413385826771666132, 0.4176697321401328100 ) ) ;
#6350=CARTESIAN_POINT ( 'NONE',  ( -0.4002624671916004129, -0.08942795157528024563, -0.3641732283464568787 ) ) ;
#6351=CARTESIAN_POINT ( 'NONE',  ( -0.8727034120734901146, -0.3162353388693405765, 0.4822834645669290543 ) ) ;
#6353=CARTESIAN_POINT ( 'NONE',  ( 0.07217847769028949700, -0.05778040916215560624, -0.4822834645669293319 ) ) ;
#6354=CARTESIAN_POINT ( 'NONE',  ( -0.9908136482939626788, 0.2952755905511811885, 0.1292274648535926551 ) ) ;
#6355=CARTESIAN_POINT ( 'NONE',  ( -0.7414698162729651543, 0.1771653543307087075, -0.09757992244046823083 ) ) ;
#6356=CARTESIAN_POINT ( 'NONE',  ( 0.1902887139107617975, 0.2952755905511811885, 0.1292274648535926551 ) ) ;
#6357=CARTESIAN_POINT ( 'NONE',  ( -1.345144356955379816, -0.05778040916215560624, -0.4822834645669293319 ) ) ;
#6358=CARTESIAN_POINT ( 'NONE',  ( -0.3215223097112853146, -0.05778040916215560624, -0.4822834645669293319 ) ) ;
#6361=CARTESIAN_POINT ( 'NONE',  ( 1.541994750656168645, -0.6692913385826771977, 0.1292274648535927661 ) ) ;
#6362=CARTESIAN_POINT ( 'NONE',  ( 1.154855643044620184, -0.6046776061558807314, 0.2411417322834647770 ) ) ;
#6364=CARTESIAN_POINT ( 'NONE',  ( 0.4687286201624442095, 1.750728371878954803, -0.5180200956804339452 ) ) ;
#6365=CARTESIAN_POINT ( 'NONE',  ( -0.7545931758530177724, 0.2952755905511811885, 0.1292274648535926551 ) ) ;
#6369=CARTESIAN_POINT ( 'NONE',  ( 8.195543980992789655E-16, -0.1870078740157480601, -0.3641732283464567677 ) ) ;
#6371=CARTESIAN_POINT ( 'NONE',  ( 0.8661417322834652488, -0.1870078740157480879, -0.4822834645669291653 ) ) ;
#6372=FACE_OUTER_BOUND ( 'NONE', #54551, .T. ) ;
#6374=CARTESIAN_POINT ( 'NONE',  ( -0.5971128608923877978, -0.5511811023622048555, -0.09757992244046775898 ) ) ;
#6375=CARTESIAN_POINT ( 'NONE',  ( 0.3805774278215230400, 0.05413385826771626580, -0.4176697321401330321 ) ) ;
#6376=CARTESIAN_POINT ( 'NONE',  ( 1.351706036745407680, 0.05413385826771666132, 0.4176697321401328100 ) ) ;
#6377=CARTESIAN_POINT ( 'NONE',  ( 0.7480314960629927956, -0.5511811023622047445, 6.969142054262312111E-17 ) ) ;
#6378=CARTESIAN_POINT ( 'NONE',  ( -0.1377952755905504645, -0.5400638737290845981, -0.3530559997133363437 ) ) ;
#6380=CARTESIAN_POINT ( 'NONE',  ( -1.017060367454067249, -0.05778040916215522460, 0.4822834645669289988 ) ) ;
#6381=CARTESIAN_POINT ( 'NONE',  ( -1.338582677165353729, -0.1870078740157480601, -0.3641732283464567677 ) ) ;
#6382=CARTESIAN_POINT ( 'NONE',  ( -0.5511811023622041894, -0.1870078740157480879, -0.4822834645669291653 ) ) ;
#6383=( BOUNDED_SURFACE ( )  B_SPLINE_SURFACE ( 1, 2, ( 
 ( #796, #27284, #45797, #13420, #52530, #51689, #58009, #20148, #34023, #46639, #77817, #65189, #32348, #13006, #78237, #52944, #64758, #77392, #39926, #40339, #78658, #20570, #46221, #13843, #19723, #71917, #65615, #33607, #72334, #66019, #8355, #59683, #44955, #2039, #71078, #70651, #27704, #19303, #38662, #64339, #29360, #9597, #2869, #72742, #28532, #10012, #22221, #61762, #80728, #79486, #10434, #21800, #42390, #15506, #34441, #47050, #60930, #34858, #74407, #29768, #55019, #35265, #54189, #15089, #79904, #35677, #47877, #4100, #23042, #47464, #36091, #73156, #68089, #41164, #73581, #2461, #66854, #61342, #3695, #79078, #40747, #9186, #15927, #60108, #48709, #16339, #28119, #60520, #41574, #21394, #66431, #53774, #8766, #67264, #3280, #16751, #28944, #54610, #80319, #22634, #48295, #73992, #41982, #67676, #43620, #49118, #38146, #63406, #18793, #81550, #30598, #76052, #5742, #69321, #24687, #50354, #57077, #49535, #82771, #74824, #44038, #69730, #62171, #5341, #43206, #42802, #12075, #62588, #4930, #63818, #11672, #6157, #50766, #49946, #18396, #10836, #25094, #75644, #76467, #75229, #17168, #31000, #56668, #55841, #37733, #31413, #30179, #37329, #11254, #44438, #81960, #17573, #63002, #4510, #36495, #56264, #70131, #12482, #24275, #17983, #68496, #23868, #82368, #55429, #68901, #36912, #81137, #23453, #71813, #65080, #13740, #45280, #6576, #26347, #70975, #691, #14164, #52008, #39396, #77713, #57492, #27182, #25927, #38973, #32662, #64656, #57907, #51585, #52846, #46534, #6994, #38561, #14583, #12902, #45694, #72234, #39820, #83184, #78557, #19618, #65509, #64241, #7418, #33088, #7841, #19200, #20882, #77287, #25506, #26768, #46119, #13320, #44849, #32247, #272, #40236, #58329, #65919, #51172, #20043, #76868, #71391, #31831, #70547, #58755, #1117, #52423, #78133, #20466, #33508, #59170, #1528, #22948, #79385, #60832, #21704, #15835, #21296, #42296, #48615, #9498, #3184, #28848, #34763, #34341, #74309, #53677, #1942, #16656, #79808, #35171, #29265, #22124, #73058, #80224, #47783, #8256, #33920, #46949, #73898, #54093, #54510, #22540, #14991, #60006, #47368, #48203, #72641, #41483, #16238, #61246, #8670, #73485, #59585, #15408, #67579, #2361, #27604, #54929, #53264, #67168, #35583, #40648, #41068, #66757, #9911, #80636, #41886, #3600, #78975, #66332, #28017, #9091, #60423, #2774, #28434, #64035, #19420, #11880, #32461, #58123, #26145, #82573, #55338, #76667, #50155, #51382, #490, #38776, #19846, #67993, #51806, #81046, #77087, #31627, #32046, #12700, #75851, #37532, #31212, #57705, #18193, #19000, #68, #64453, #69530, #50970, #10338, #24892, #45071, #63208, #77511, #6788, #29675, #44649, #13125, #43826, #18599, #44242, #70774, #36000, #25305, #70346, #25722, #38359, #5547, #69931, #61670, #82985, #6374, #4011, #24488, #56880, #50561, #76264, #12287, #37943, #63620, #5957, #57288, #27823, #8883, #15208, #79607, #39619, #52649, #46337, #78353, #71609, #65308, #66550, #60225, #20685, #52229, #28234, #26576, #59386, #2575, #2156, #13534, #34559, #33317, #79193, #77932, #53061, #78773, #21509, #32884, #40868, #7647, #71192, #40455, #59802, #58979, #58553, #45912, #20262, #53893, #13962, #45495, #64874, #72030, #7214, #1335, #39190, #919, #26984, #14386, #27401, #40044, #21097, #65730, #8063, #33724, #1744, #46756, #14798, #72449, #66134, #8472, #34141, #53483, #47167, #72859, #16872, #48409, #48002, #4622, #67380, #15627, #30293, #10134, #23156, #42914, #35798, #3400, #10548, #61465, #48825, #22342, #68211, #42509, #80023, #3813, #61050, #61875, #74109, #16041, #29475, #28653, #60636, #22749, #36606, #23567, #80439, #42100, #34973, #41284, #67797, #4216, #41687, #54312, #36206, #17286, #29880, #55133, #80843, #35385, #73701, #16455, #29063, #74526, #55543, #81252, #49238, #74941, #47585, #68609, #10949, #66970, #62285, #55959, #9714, #54734, #21924, #73279, #9303, #2987, #63526, #44555, #5857, #82077, #82482, #51285, #12191, #25211, #76577, #31948, #24390, #44970, #70666, #38676, #11788, #69018, #31533, #62708, #63936, #13022, #76988, #32361, #75756 ),
 ( #49650, #19318, #69435, #57609, #5046, #57189, #82891, #83300, #11369, #64354, #18098, #23983, #18905, #12601, #37441, #37026, #50061, #30715, #6691, #56378, #81672, #17689, #5453, #43319, #63115, #75342, #43731, #31114, #56782, #50877, #24797, #70245, #50465, #76169, #18506, #44149, #69841, #38259, #37848, #6272, #25622, #71931, #13856, #14697, #1234, #52123, #65629, #64771, #13434, #58876, #72755, #59698, #33212, #78252, #71091, #51703, #20583, #40353, #77831, #7110, #52959, #53384, #66032, #7960, #39943, #71509, #32781, #52543, #39515, #26883, #8370, #46235, #33622, #15104, #26044, #78673, #66445, #77405, #59285, #65203, #79091, #8781, #34036, #14280, #7539, #19740, #1642, #72349, #27300, #40760, #2053, #58449, #58023, #809, #21409, #20161, #20994, #26472, #45811, #27717, #47063, #387, #45394, #46656, #39090, #15522, #42404, #55034, #41180, #47891, #2884, #81151, #17182, #73172, #74838, #22236, #53788, #68102, #73599, #23467, #67690, #29781, #55443, #15941, #54203, #80334, #22649, #28133, #42815, #10448, #49133, #60534, #9611, #80741, #36104, #48308, #3710, #29373, #61775, #28547, #4116, #79500, #23055, #48723, #66870, #10026, #41588, #21815, #74420, #67278, #35280, #68509, #74005, #34454, #60123, #28958, #16766, #9200, #2474, #54623, #47479, #79920, #34873, #35691, #61356, #60943, #3294, #16352, #41996, #81974, #4523, #4944, #70144, #30193, #30613, #82785, #5353, #12496, #31012, #17998, #49548, #43632, #18807, #62603, #24699, #56277, #56681, #55855, #10849, #44452, #50368, #76066, #18408, #69335, #68917, #36510, #24288, #81564, #62186, #44051, #12088, #23883, #69743, #37343, #25106, #37745, #75243, #17587, #49960, #43219, #63420, #11267, #50779, #75657, #11685, #82382, #36926, #5757, #63015, #31427, #57089, #76480, #67962, #2741, #41854, #22090, #3153, #35970, #61640, #47750, #3981, #30056, #35137, #35550, #61213, #4388, #23742, #42265, #10304, #48998, #29645, #28816, #3568, #55717, #16623, #55307, #81015, #36376, #54481, #49415, #75109, #43085, #16207, #73449, #23328, #67134, #68380, #17455, #81427, #36784, #80192, #9881, #29235, #54899, #22510, #48171, #68782, #11126, #80605, #9463, #28401, #60799, #74697, #54059, #42682, #79774, #15799, #73867, #62050, #67546, #17042, #10719, #41450, #22915, #48582, #74279, #4795, #57367, #76747, #75928, #49822, #62880, #11543, #19495, #37199, #51461, #30879, #25800, #45149, #17861, #70852, #50232, #81841, #70422, #18269, #77163, #12362, #57781, #145, #43909, #82247, #24966, #50638, #56136, #13203, #12778, #62460, #5215, #37608, #83062, #38435, #76342, #31707, #25383, #64118, #56546, #6453, #24152, #51046, #19077, #69194, #38020, #69607, #75522, #44725, #11953, #63283, #30472, #18672, #43496, #24565, #56954, #32123, #5623, #31289, #82651, #44317, #70007, #63696, #6035, #80574, #75073, #61606, #55270, #80981, #3535, #3117, #43051, #22475, #54027, #68747, #48548, #3949, #81390, #74246, #41819, #48964, #16588, #11090, #17420, #73415, #42648, #22884, #23293, #29610, #67100, #28784, #48136, #74664, #41416, #10269, #17008, #30018, #60767, #42234, #60358, #16173, #79738, #54446, #35937, #68345, #22055, #10685, #4351, #9431, #9846, #35518, #62014, #23706, #67928, #36340, #55683, #49377, #80158, #61181, #2705, #28365, #47717, #15764, #35100, #73833, #67510, #29202, #54868, #50196, #24117, #44284, #17827, #19043, #110, #6418, #70819, #30845, #43874, #51426, #24531, #6002, #69974, #44690, #11509, #56921, #77128, #37986, #31671, #57332, #63248, #62845, #19462, #82212, #30436, #45112, #24932, #63661, #57748, #50602, #18234, #25349, #76309, #36746, #62423, #49786, #70386, #82616, #83026, #51011, #43460, #5181, #75894, #76710, #69158, #12328, #12742, #32087, #37165, #18640, #4760, #69572, #56101, #56510, #38401, #64081, #81805, #25765, #75487, #11920, #37575, #5587, #31254, #34180, #52686, #78394, #59427, #20725, #13579, #14002, #66176, #27025, #40081, #8100, #46796, #39233, #59845, #2197, #53525, #26616, #534, #46377, #77556, #78812, #27865, #8514, #47209, #7255, #20304, #39660, #45954, #64918, #32928, #79233, #21548, #71651 ) ),
 .UNSPECIFIED., .F., .F., .F. ) 
 B_SPLINE_SURFACE_WITH_KNOTS ( ( 2, 2 ),
 ( 3, 2, 2, 2, 2, 2, 2, 2, 2, 2, 2, 2, 2, 2, 2, 2, 2, 2, 2, 2, 2, 2, 2, 2, 2, 2, 2, 2, 2, 2, 2, 2, 2, 2, 2, 2, 2, 2, 2, 2, 2, 2, 2, 2, 2, 2, 2, 2, 2, 2, 2, 2, 2, 2, 2, 2, 2, 2, 2, 2, 2, 2, 2, 2, 2, 2, 2, 2, 2, 2, 2, 2, 2, 2, 2, 2, 2, 2, 2, 2, 2, 2, 2, 2, 2, 2, 2, 2, 2, 2, 2, 2, 2, 2, 2, 2, 2, 2, 2, 2, 2, 2, 2, 2, 2, 2, 2, 2, 2, 2, 2, 2, 2, 2, 2, 2, 2, 2, 2, 2, 2, 2, 2, 2, 2, 2, 2, 2, 2, 2, 2, 2, 2, 2, 2, 2, 2, 2, 2, 2, 2, 2, 2, 2, 2, 2, 2, 2, 2, 2, 2, 2, 2, 2, 2, 2, 2, 2, 2, 2, 2, 2, 2, 2, 2, 2, 2, 2, 2, 2, 2, 2, 2, 2, 2, 2, 2, 2, 2, 2, 2, 2, 2, 2, 2, 2, 2, 2, 2, 2, 2, 2, 2, 2, 2, 2, 2, 2, 2, 2, 2, 2, 2, 2, 2, 2, 2, 2, 2, 2, 2, 2, 2, 2, 2, 2, 2, 2, 2, 2, 2, 2, 2, 2, 2, 2, 2, 2, 2, 2, 2, 2, 2, 2, 2, 2, 2, 2, 2, 2, 2, 2, 2, 2, 2, 2, 2, 2, 2, 2, 2, 2, 2, 2, 2, 3 ),
 ( 0.000000000000000000, 1.000000000000000000 ),
 ( 0.000000000000000000, 0.003787878787878787984, 0.007575757575757575968, 0.01136363636363636395, 0.01515151515151515194, 0.01893939393939393992, 0.02272727272727272790, 0.02651515151515151589, 0.03030303030303030387, 0.03409090909090908839, 0.03787878787878787984, 0.04166666666666666435, 0.04545454545454545581, 0.04924242424242424032, 0.05303030303030303177, 0.05681818181818181629, 0.06060606060606060774, 0.06439393939393939226, 0.06818181818181817677, 0.07196969696969697516, 0.07575757575757575968, 0.07954545454545454419, 0.08333333333333332871, 0.08712121212121212710, 0.09090909090909091161, 0.09469696969696969613, 0.09848484848484848064, 0.1022727272727272790, 0.1060606060606060635, 0.1098484848484848481, 0.1136363636363636326, 0.1174242424242424310, 0.1212121212121212155, 0.1250000000000000000, 0.1287878787878787845, 0.1325757575757575690, 0.1363636363636363535, 0.1401515151515151381, 0.1439393939393939503, 0.1477272727272727348, 0.1515151515151515194, 0.1553030303030303039, 0.1590909090909090884, 0.1628787878787878729, 0.1666666666666666574, 0.1704545454545454419, 0.1742424242424242542, 0.1780303030303030387, 0.1818181818181818232, 0.1856060606060606077, 0.1893939393939393923, 0.1931818181818181768, 0.1969696969696969613, 0.2007575757575757458, 0.2045454545454545581, 0.2083333333333333426, 0.2121212121212121271, 0.2159090909090909116, 0.2196969696969696961, 0.2234848484848484806, 0.2272727272727272652, 0.2310606060606060497, 0.2348484848484848619, 0.2386363636363636465, 0.2424242424242424310, 0.2462121212121212155, 0.2500000000000000000, 0.2537878787878787845, 0.2575757575757575690, 0.2613636363636363535, 0.2651515151515151381, 0.2689393939393939226, 0.2727272727272727071, 0.2765151515151514916, 0.2803030303030302761, 0.2840909090909091161, 0.2878787878787879007, 0.2916666666666666852, 0.2954545454545454697, 0.2992424242424242542, 0.3030303030303030387, 0.3068181818181818232, 0.3106060606060606077, 0.3143939393939393923, 0.3181818181818181768, 0.3219696969696969613, 0.3257575757575757458, 0.3295454545454545303, 0.3333333333333333148, 0.3371212121212120993, 0.3409090909090908839, 0.3446969696969697239, 0.3484848484848485084, 0.3522727272727272929, 0.3560606060606060774, 0.3598484848484848619, 0.3636363636363636465, 0.3674242424242424310, 0.3712121212121212155, 0.3750000000000000000, 0.3787878787878787845, 0.3825757575757575690, 0.3863636363636363535, 0.3901515151515151381, 0.3939393939393939226, 0.3977272727272727071, 0.4015151515151514916, 0.4053030303030302761, 0.4090909090909091161, 0.4128787878787879007, 0.4166666666666666852, 0.4204545454545454697, 0.4242424242424242542, 0.4280303030303030387, 0.4318181818181818232, 0.4356060606060606077, 0.4393939393939393923, 0.4431818181818181768, 0.4469696969696969613, 0.4507575757575757458, 0.4545454545454545303, 0.4583333333333333148, 0.4621212121212120993, 0.4659090909090908839, 0.4696969696969697239, 0.4734848484848485084, 0.4772727272727272929, 0.4810606060606060774, 0.4848484848484848619, 0.4886363636363636465, 0.4924242424242424310, 0.4962121212121212155, 0.5000000000000000000, 0.5037878787878787845, 0.5075757575757575690, 0.5113636363636363535, 0.5151515151515151381, 0.5189393939393939226, 0.5227272727272727071, 0.5265151515151514916, 0.5303030303030302761, 0.5340909090909090606, 0.5378787878787878451, 0.5416666666666666297, 0.5454545454545454142, 0.5492424242424241987, 0.5530303030303029832, 0.5568181818181817677, 0.5606060606060605522, 0.5643939393939394478, 0.5681818181818182323, 0.5719696969696970168, 0.5757575757575758013, 0.5795454545454545858, 0.5833333333333333703, 0.5871212121212121549, 0.5909090909090909394, 0.5946969696969697239, 0.5984848484848485084, 0.6022727272727272929, 0.6060606060606060774, 0.6098484848484848619, 0.6136363636363636465, 0.6174242424242424310, 0.6212121212121212155, 0.6250000000000000000, 0.6287878787878787845, 0.6325757575757575690, 0.6363636363636363535, 0.6401515151515151381, 0.6439393939393939226, 0.6477272727272727071, 0.6515151515151514916, 0.6553030303030302761, 0.6590909090909090606, 0.6628787878787878451, 0.6666666666666666297, 0.6704545454545454142, 0.6742424242424241987, 0.6780303030303029832, 0.6818181818181817677, 0.6856060606060605522, 0.6893939393939394478, 0.6931818181818182323, 0.6969696969696970168, 0.7007575757575758013, 0.7045454545454545858, 0.7083333333333333703, 0.7121212121212121549, 0.7159090909090909394, 0.7196969696969697239, 0.7234848484848485084, 0.7272727272727272929, 0.7310606060606060774, 0.7348484848484848619, 0.7386363636363636465, 0.7424242424242424310, 0.7462121212121212155, 0.7500000000000000000, 0.7537878787878787845, 0.7575757575757575690, 0.7613636363636363535, 0.7651515151515151381, 0.7689393939393939226, 0.7727272727272727071, 0.7765151515151514916, 0.7803030303030302761, 0.7840909090909090606, 0.7878787878787878451, 0.7916666666666666297, 0.7954545454545454142, 0.7992424242424241987, 0.8030303030303029832, 0.8068181818181817677, 0.8106060606060605522, 0.8143939393939394478, 0.8181818181818182323, 0.8219696969696970168, 0.8257575757575758013, 0.8295454545454545858, 0.8333333333333333703, 0.8371212121212121549, 0.8409090909090909394, 0.8446969696969697239, 0.8484848484848485084, 0.8522727272727272929, 0.8560606060606060774, 0.8598484848484848619, 0.8636363636363636465, 0.8674242424242424310, 0.8712121212121212155, 0.8750000000000000000, 0.8787878787878787845, 0.8825757575757575690, 0.8863636363636363535, 0.8901515151515151381, 0.8939393939393939226, 0.8977272727272727071, 0.9015151515151514916, 0.9053030303030302761, 0.9090909090909090606, 0.9128787878787878451, 0.9166666666666666297, 0.9204545454545454142, 0.9242424242424241987, 0.9280303030303029832, 0.9318181818181817677, 0.9356060606060605522, 0.9393939393939394478, 0.9431818181818182323, 0.9469696969696970168, 0.9507575757575758013, 0.9545454545454545858, 0.9583333333333333703, 0.9621212121212121549, 0.9659090909090909394 ),
 .UNSPECIFIED. ) 
 GEOMETRIC_REPRESENTATION_ITEM ( )  RATIONAL_B_SPLINE_SURFACE ( (
 ( 1.000000000000000000, 0.9659258262890683122, 1.000000000000000000, 0.9659258262890683122, 1.000000000000000000, 0.9659258262890683122, 1.000000000000000000, 0.9659258262890683122, 1.000000000000000000, 0.9659258262890683122, 1.000000000000000000, 0.9659258262890683122, 1.000000000000000000, 0.9659258262890683122, 1.000000000000000000, 0.9659258262890683122, 1.000000000000000000, 0.9659258262890683122, 1.000000000000000000, 0.9659258262890683122, 1.000000000000000000, 0.9659258262890683122, 1.000000000000000000, 0.9659258262890683122, 1.000000000000000000, 0.9659258262890683122, 1.000000000000000000, 0.9659258262890683122, 1.000000000000000000, 0.9659258262890683122, 1.000000000000000000, 0.9659258262890683122, 1.000000000000000000, 0.9659258262890683122, 1.000000000000000000, 0.9659258262890683122, 1.000000000000000000, 0.9659258262890683122, 1.000000000000000000, 0.9659258262890683122, 1.000000000000000000, 0.9659258262890683122, 1.000000000000000000, 0.9659258262890683122, 1.000000000000000000, 0.9659258262890683122, 1.000000000000000000, 0.9659258262890683122, 1.000000000000000000, 0.9659258262890683122, 1.000000000000000000, 0.9659258262890683122, 1.000000000000000000, 0.9659258262890683122, 1.000000000000000000, 0.9659258262890683122, 1.000000000000000000, 0.9659258262890683122, 1.000000000000000000, 0.9659258262890683122, 1.000000000000000000, 0.9659258262890683122, 1.000000000000000000, 0.9659258262890683122, 1.000000000000000000, 0.9659258262890683122, 1.000000000000000000, 0.9659258262890683122, 1.000000000000000000, 0.9659258262890683122, 1.000000000000000000, 0.9659258262890683122, 1.000000000000000000, 0.9659258262890683122, 1.000000000000000000, 0.9659258262890683122, 1.000000000000000000, 0.9659258262890683122, 1.000000000000000000, 0.9659258262890683122, 1.000000000000000000, 0.9659258262890683122, 1.000000000000000000, 0.9659258262890683122, 1.000000000000000000, 0.9659258262890683122, 1.000000000000000000, 0.9659258262890683122, 1.000000000000000000, 0.9659258262890683122, 1.000000000000000000, 0.9659258262890683122, 1.000000000000000000, 0.9659258262890683122, 1.000000000000000000, 0.9659258262890683122, 1.000000000000000000, 0.9659258262890683122, 1.000000000000000000, 0.9659258262890683122, 1.000000000000000000, 0.9659258262890683122, 1.000000000000000000, 0.9659258262890683122, 1.000000000000000000, 0.9659258262890683122, 1.000000000000000000, 0.9659258262890683122, 1.000000000000000000, 0.9659258262890683122, 1.000000000000000000, 0.9659258262890683122, 1.000000000000000000, 0.9659258262890683122, 1.000000000000000000, 0.9659258262890683122, 1.000000000000000000, 0.9659258262890683122, 1.000000000000000000, 0.9659258262890683122, 1.000000000000000000, 0.9659258262890683122, 1.000000000000000000, 0.9659258262890683122, 1.000000000000000000, 0.9659258262890683122, 1.000000000000000000, 0.9659258262890683122, 1.000000000000000000, 0.9659258262890683122, 1.000000000000000000, 0.9659258262890683122, 1.000000000000000000, 0.9659258262890683122, 1.000000000000000000, 0.9659258262890683122, 1.000000000000000000, 0.9659258262890683122, 1.000000000000000000, 0.9659258262890683122, 1.000000000000000000, 0.9659258262890683122, 1.000000000000000000, 0.9659258262890683122, 1.000000000000000000, 0.9659258262890683122, 1.000000000000000000, 0.9659258262890683122, 1.000000000000000000, 0.9659258262890683122, 1.000000000000000000, 0.9659258262890683122, 1.000000000000000000, 0.9659258262890683122, 1.000000000000000000, 0.9659258262890683122, 1.000000000000000000, 0.9659258262890683122, 1.000000000000000000, 0.9659258262890683122, 1.000000000000000000, 0.9659258262890683122, 1.000000000000000000, 0.9659258262890683122, 1.000000000000000000, 0.9659258262890683122, 1.000000000000000000, 0.9659258262890683122, 1.000000000000000000, 0.9659258262890683122, 1.000000000000000000, 0.9659258262890683122, 1.000000000000000000, 0.9659258262890683122, 1.000000000000000000, 0.9659258262890683122, 1.000000000000000000, 0.9659258262890683122, 1.000000000000000000, 0.9659258262890683122, 1.000000000000000000, 0.9659258262890683122, 1.000000000000000000, 0.9659258262890683122, 1.000000000000000000, 0.9659258262890683122, 1.000000000000000000, 0.9659258262890683122, 1.000000000000000000, 0.9659258262890683122, 1.000000000000000000, 0.9659258262890683122, 1.000000000000000000, 0.9659258262890683122, 1.000000000000000000, 0.9659258262890683122, 1.000000000000000000, 0.9659258262890683122, 1.000000000000000000, 0.9659258262890683122, 1.000000000000000000, 0.9659258262890683122, 1.000000000000000000, 0.9659258262890683122, 1.000000000000000000, 0.9659258262890683122, 1.000000000000000000, 0.9659258262890683122, 1.000000000000000000, 0.9659258262890683122, 1.000000000000000000, 0.9659258262890683122, 1.000000000000000000, 0.9659258262890683122, 1.000000000000000000, 0.9659258262890683122, 1.000000000000000000, 0.9659258262890683122, 1.000000000000000000, 0.9659258262890683122, 1.000000000000000000, 0.9659258262890683122, 1.000000000000000000, 0.9659258262890683122, 1.000000000000000000, 0.9659258262890683122, 1.000000000000000000, 0.9659258262890683122, 1.000000000000000000, 0.9659258262890683122, 1.000000000000000000, 0.9659258262890683122, 1.000000000000000000, 0.9659258262890683122, 1.000000000000000000, 0.9659258262890683122, 1.000000000000000000, 0.9659258262890683122, 1.000000000000000000, 0.9659258262890683122, 1.000000000000000000, 0.9659258262890683122, 1.000000000000000000, 0.9659258262890683122, 1.000000000000000000, 0.9659258262890683122, 1.000000000000000000, 0.9659258262890683122, 1.000000000000000000, 0.9659258262890683122, 1.000000000000000000, 0.9659258262890683122, 1.000000000000000000, 0.9659258262890683122, 1.000000000000000000, 0.9659258262890683122, 1.000000000000000000, 0.9659258262890683122, 1.000000000000000000, 0.9659258262890683122, 1.000000000000000000, 0.9659258262890683122, 1.000000000000000000, 0.9659258262890683122, 1.000000000000000000, 0.9659258262890683122, 1.000000000000000000, 0.9659258262890683122, 1.000000000000000000, 0.9659258262890683122, 1.000000000000000000, 0.9659258262890683122, 1.000000000000000000, 0.9659258262890683122, 1.000000000000000000, 0.9659258262890683122, 1.000000000000000000, 0.9659258262890683122, 1.000000000000000000, 0.9659258262890683122, 1.000000000000000000, 0.9659258262890683122, 1.000000000000000000, 0.9659258262890683122, 1.000000000000000000, 0.9659258262890683122, 1.000000000000000000, 0.9659258262890683122, 1.000000000000000000, 0.9659258262890683122, 1.000000000000000000, 0.9659258262890683122, 1.000000000000000000, 0.9659258262890683122, 1.000000000000000000, 0.9659258262890683122, 1.000000000000000000, 0.9659258262890683122, 1.000000000000000000, 0.9659258262890683122, 1.000000000000000000, 0.9659258262890683122, 1.000000000000000000, 0.9659258262890683122, 1.000000000000000000, 0.9659258262890683122, 1.000000000000000000, 0.9659258262890683122, 1.000000000000000000, 0.9659258262890683122, 1.000000000000000000, 0.9659258262890683122, 1.000000000000000000, 0.9659258262890683122, 1.000000000000000000, 0.9659258262890683122, 1.000000000000000000, 0.9659258262890683122, 1.000000000000000000, 0.9659258262890683122, 1.000000000000000000, 0.9659258262890683122, 1.000000000000000000, 0.9659258262890683122, 1.000000000000000000, 0.9659258262890683122, 1.000000000000000000, 0.9659258262890683122, 1.000000000000000000, 0.9659258262890683122, 1.000000000000000000, 0.9659258262890683122, 1.000000000000000000, 0.9659258262890683122, 1.000000000000000000, 0.9659258262890683122, 1.000000000000000000, 0.9659258262890683122, 1.000000000000000000, 0.9659258262890683122, 1.000000000000000000, 0.9659258262890683122, 1.000000000000000000, 0.9659258262890683122, 1.000000000000000000, 0.9659258262890683122, 1.000000000000000000, 0.9659258262890683122, 1.000000000000000000, 0.9659258262890683122, 1.000000000000000000, 0.9659258262890683122, 1.000000000000000000, 0.9659258262890683122, 1.000000000000000000, 0.9659258262890683122, 1.000000000000000000, 0.9659258262890683122, 1.000000000000000000, 0.9659258262890683122, 1.000000000000000000, 0.9659258262890683122, 1.000000000000000000, 0.9659258262890683122, 1.000000000000000000, 0.9659258262890683122, 1.000000000000000000, 0.9659258262890683122, 1.000000000000000000, 0.9659258262890683122, 1.000000000000000000, 0.9659258262890683122, 1.000000000000000000, 0.9659258262890683122, 1.000000000000000000, 0.9659258262890683122, 1.000000000000000000, 0.9659258262890683122, 1.000000000000000000, 0.9659258262890683122, 1.000000000000000000, 0.9659258262890683122, 1.000000000000000000, 0.9659258262890683122, 1.000000000000000000, 0.9659258262890683122, 1.000000000000000000, 0.9659258262890683122, 1.000000000000000000, 0.9659258262890683122, 1.000000000000000000, 0.9659258262890683122, 1.000000000000000000, 0.9659258262890683122, 1.000000000000000000, 0.9659258262890683122, 1.000000000000000000, 0.9659258262890683122, 1.000000000000000000, 0.9659258262890683122, 1.000000000000000000, 0.9659258262890683122, 1.000000000000000000, 0.9659258262890683122, 1.000000000000000000, 0.9659258262890683122, 1.000000000000000000, 0.9659258262890683122, 1.000000000000000000, 0.9659258262890683122, 1.000000000000000000, 0.9659258262890683122, 1.000000000000000000, 0.9659258262890683122, 1.000000000000000000, 0.9659258262890683122, 1.000000000000000000, 0.9659258262890683122, 1.000000000000000000, 0.9659258262890683122, 1.000000000000000000, 0.9659258262890683122, 1.000000000000000000, 0.9659258262890683122, 1.000000000000000000, 0.9659258262890683122, 1.000000000000000000, 0.9659258262890683122, 1.000000000000000000, 0.9659258262890683122, 1.000000000000000000, 0.9659258262890683122, 1.000000000000000000, 0.9659258262890683122, 1.000000000000000000, 0.9659258262890683122, 1.000000000000000000, 0.9659258262890683122, 1.000000000000000000, 0.9659258262890683122, 1.000000000000000000, 0.9659258262890683122, 1.000000000000000000, 0.9659258262890683122, 1.000000000000000000, 0.9659258262890683122, 1.000000000000000000, 0.9659258262890683122, 1.000000000000000000, 0.9659258262890683122, 1.000000000000000000, 0.9659258262890683122, 1.000000000000000000, 0.9659258262890683122, 1.000000000000000000, 0.9659258262890683122, 1.000000000000000000, 0.9659258262890683122, 1.000000000000000000, 0.9659258262890683122, 1.000000000000000000, 0.9659258262890683122, 1.000000000000000000, 0.9659258262890683122, 1.000000000000000000, 0.9659258262890683122, 1.000000000000000000, 0.9659258262890683122, 1.000000000000000000, 0.9659258262890683122, 1.000000000000000000, 0.9659258262890683122, 1.000000000000000000, 0.9659258262890683122, 1.000000000000000000, 0.9659258262890683122, 1.000000000000000000, 0.9659258262890683122, 1.000000000000000000, 0.9659258262890683122, 1.000000000000000000, 0.9659258262890683122, 1.000000000000000000, 0.9659258262890683122, 1.000000000000000000, 0.9659258262890683122, 1.000000000000000000, 0.9659258262890683122, 1.000000000000000000, 0.9659258262890683122, 1.000000000000000000, 0.9659258262890683122, 1.000000000000000000, 0.9659258262890683122, 1.000000000000000000, 0.9659258262890683122, 1.000000000000000000, 0.9659258262890683122, 1.000000000000000000, 0.9659258262890683122, 1.000000000000000000, 0.9659258262890683122, 1.000000000000000000, 0.9659258262890683122, 1.000000000000000000, 0.9659258262890683122, 1.000000000000000000, 0.9659258262890683122, 1.000000000000000000, 0.9659258262890683122, 1.000000000000000000),
 ( 1.000000000000000000, 0.9659258262890683122, 1.000000000000000000, 0.9659258262890683122, 1.000000000000000000, 0.9659258262890683122, 1.000000000000000000, 0.9659258262890683122, 1.000000000000000000, 0.9659258262890683122, 1.000000000000000000, 0.9659258262890683122, 1.000000000000000000, 0.9659258262890683122, 1.000000000000000000, 0.9659258262890683122, 1.000000000000000000, 0.9659258262890683122, 1.000000000000000000, 0.9659258262890683122, 1.000000000000000000, 0.9659258262890683122, 1.000000000000000000, 0.9659258262890683122, 1.000000000000000000, 0.9659258262890683122, 1.000000000000000000, 0.9659258262890683122, 1.000000000000000000, 0.9659258262890683122, 1.000000000000000000, 0.9659258262890683122, 1.000000000000000000, 0.9659258262890683122, 1.000000000000000000, 0.9659258262890683122, 1.000000000000000000, 0.9659258262890683122, 1.000000000000000000, 0.9659258262890683122, 1.000000000000000000, 0.9659258262890683122, 1.000000000000000000, 0.9659258262890683122, 1.000000000000000000, 0.9659258262890683122, 1.000000000000000000, 0.9659258262890683122, 1.000000000000000000, 0.9659258262890683122, 1.000000000000000000, 0.9659258262890683122, 1.000000000000000000, 0.9659258262890683122, 1.000000000000000000, 0.9659258262890683122, 1.000000000000000000, 0.9659258262890683122, 1.000000000000000000, 0.9659258262890683122, 1.000000000000000000, 0.9659258262890683122, 1.000000000000000000, 0.9659258262890683122, 1.000000000000000000, 0.9659258262890683122, 1.000000000000000000, 0.9659258262890683122, 1.000000000000000000, 0.9659258262890683122, 1.000000000000000000, 0.9659258262890683122, 1.000000000000000000, 0.9659258262890683122, 1.000000000000000000, 0.9659258262890683122, 1.000000000000000000, 0.9659258262890683122, 1.000000000000000000, 0.9659258262890683122, 1.000000000000000000, 0.9659258262890683122, 1.000000000000000000, 0.9659258262890683122, 1.000000000000000000, 0.9659258262890683122, 1.000000000000000000, 0.9659258262890683122, 1.000000000000000000, 0.9659258262890683122, 1.000000000000000000, 0.9659258262890683122, 1.000000000000000000, 0.9659258262890683122, 1.000000000000000000, 0.9659258262890683122, 1.000000000000000000, 0.9659258262890683122, 1.000000000000000000, 0.9659258262890683122, 1.000000000000000000, 0.9659258262890683122, 1.000000000000000000, 0.9659258262890683122, 1.000000000000000000, 0.9659258262890683122, 1.000000000000000000, 0.9659258262890683122, 1.000000000000000000, 0.9659258262890683122, 1.000000000000000000, 0.9659258262890683122, 1.000000000000000000, 0.9659258262890683122, 1.000000000000000000, 0.9659258262890683122, 1.000000000000000000, 0.9659258262890683122, 1.000000000000000000, 0.9659258262890683122, 1.000000000000000000, 0.9659258262890683122, 1.000000000000000000, 0.9659258262890683122, 1.000000000000000000, 0.9659258262890683122, 1.000000000000000000, 0.9659258262890683122, 1.000000000000000000, 0.9659258262890683122, 1.000000000000000000, 0.9659258262890683122, 1.000000000000000000, 0.9659258262890683122, 1.000000000000000000, 0.9659258262890683122, 1.000000000000000000, 0.9659258262890683122, 1.000000000000000000, 0.9659258262890683122, 1.000000000000000000, 0.9659258262890683122, 1.000000000000000000, 0.9659258262890683122, 1.000000000000000000, 0.9659258262890683122, 1.000000000000000000, 0.9659258262890683122, 1.000000000000000000, 0.9659258262890683122, 1.000000000000000000, 0.9659258262890683122, 1.000000000000000000, 0.9659258262890683122, 1.000000000000000000, 0.9659258262890683122, 1.000000000000000000, 0.9659258262890683122, 1.000000000000000000, 0.9659258262890683122, 1.000000000000000000, 0.9659258262890683122, 1.000000000000000000, 0.9659258262890683122, 1.000000000000000000, 0.9659258262890683122, 1.000000000000000000, 0.9659258262890683122, 1.000000000000000000, 0.9659258262890683122, 1.000000000000000000, 0.9659258262890683122, 1.000000000000000000, 0.9659258262890683122, 1.000000000000000000, 0.9659258262890683122, 1.000000000000000000, 0.9659258262890683122, 1.000000000000000000, 0.9659258262890683122, 1.000000000000000000, 0.9659258262890683122, 1.000000000000000000, 0.9659258262890683122, 1.000000000000000000, 0.9659258262890683122, 1.000000000000000000, 0.9659258262890683122, 1.000000000000000000, 0.9659258262890683122, 1.000000000000000000, 0.9659258262890683122, 1.000000000000000000, 0.9659258262890683122, 1.000000000000000000, 0.9659258262890683122, 1.000000000000000000, 0.9659258262890683122, 1.000000000000000000, 0.9659258262890683122, 1.000000000000000000, 0.9659258262890683122, 1.000000000000000000, 0.9659258262890683122, 1.000000000000000000, 0.9659258262890683122, 1.000000000000000000, 0.9659258262890683122, 1.000000000000000000, 0.9659258262890683122, 1.000000000000000000, 0.9659258262890683122, 1.000000000000000000, 0.9659258262890683122, 1.000000000000000000, 0.9659258262890683122, 1.000000000000000000, 0.9659258262890683122, 1.000000000000000000, 0.9659258262890683122, 1.000000000000000000, 0.9659258262890683122, 1.000000000000000000, 0.9659258262890683122, 1.000000000000000000, 0.9659258262890683122, 1.000000000000000000, 0.9659258262890683122, 1.000000000000000000, 0.9659258262890683122, 1.000000000000000000, 0.9659258262890683122, 1.000000000000000000, 0.9659258262890683122, 1.000000000000000000, 0.9659258262890683122, 1.000000000000000000, 0.9659258262890683122, 1.000000000000000000, 0.9659258262890683122, 1.000000000000000000, 0.9659258262890683122, 1.000000000000000000, 0.9659258262890683122, 1.000000000000000000, 0.9659258262890683122, 1.000000000000000000, 0.9659258262890683122, 1.000000000000000000, 0.9659258262890683122, 1.000000000000000000, 0.9659258262890683122, 1.000000000000000000, 0.9659258262890683122, 1.000000000000000000, 0.9659258262890683122, 1.000000000000000000, 0.9659258262890683122, 1.000000000000000000, 0.9659258262890683122, 1.000000000000000000, 0.9659258262890683122, 1.000000000000000000, 0.9659258262890683122, 1.000000000000000000, 0.9659258262890683122, 1.000000000000000000, 0.9659258262890683122, 1.000000000000000000, 0.9659258262890683122, 1.000000000000000000, 0.9659258262890683122, 1.000000000000000000, 0.9659258262890683122, 1.000000000000000000, 0.9659258262890683122, 1.000000000000000000, 0.9659258262890683122, 1.000000000000000000, 0.9659258262890683122, 1.000000000000000000, 0.9659258262890683122, 1.000000000000000000, 0.9659258262890683122, 1.000000000000000000, 0.9659258262890683122, 1.000000000000000000, 0.9659258262890683122, 1.000000000000000000, 0.9659258262890683122, 1.000000000000000000, 0.9659258262890683122, 1.000000000000000000, 0.9659258262890683122, 1.000000000000000000, 0.9659258262890683122, 1.000000000000000000, 0.9659258262890683122, 1.000000000000000000, 0.9659258262890683122, 1.000000000000000000, 0.9659258262890683122, 1.000000000000000000, 0.9659258262890683122, 1.000000000000000000, 0.9659258262890683122, 1.000000000000000000, 0.9659258262890683122, 1.000000000000000000, 0.9659258262890683122, 1.000000000000000000, 0.9659258262890683122, 1.000000000000000000, 0.9659258262890683122, 1.000000000000000000, 0.9659258262890683122, 1.000000000000000000, 0.9659258262890683122, 1.000000000000000000, 0.9659258262890683122, 1.000000000000000000, 0.9659258262890683122, 1.000000000000000000, 0.9659258262890683122, 1.000000000000000000, 0.9659258262890683122, 1.000000000000000000, 0.9659258262890683122, 1.000000000000000000, 0.9659258262890683122, 1.000000000000000000, 0.9659258262890683122, 1.000000000000000000, 0.9659258262890683122, 1.000000000000000000, 0.9659258262890683122, 1.000000000000000000, 0.9659258262890683122, 1.000000000000000000, 0.9659258262890683122, 1.000000000000000000, 0.9659258262890683122, 1.000000000000000000, 0.9659258262890683122, 1.000000000000000000, 0.9659258262890683122, 1.000000000000000000, 0.9659258262890683122, 1.000000000000000000, 0.9659258262890683122, 1.000000000000000000, 0.9659258262890683122, 1.000000000000000000, 0.9659258262890683122, 1.000000000000000000, 0.9659258262890683122, 1.000000000000000000, 0.9659258262890683122, 1.000000000000000000, 0.9659258262890683122, 1.000000000000000000, 0.9659258262890683122, 1.000000000000000000, 0.9659258262890683122, 1.000000000000000000, 0.9659258262890683122, 1.000000000000000000, 0.9659258262890683122, 1.000000000000000000, 0.9659258262890683122, 1.000000000000000000, 0.9659258262890683122, 1.000000000000000000, 0.9659258262890683122, 1.000000000000000000, 0.9659258262890683122, 1.000000000000000000, 0.9659258262890683122, 1.000000000000000000, 0.9659258262890683122, 1.000000000000000000, 0.9659258262890683122, 1.000000000000000000, 0.9659258262890683122, 1.000000000000000000, 0.9659258262890683122, 1.000000000000000000, 0.9659258262890683122, 1.000000000000000000, 0.9659258262890683122, 1.000000000000000000, 0.9659258262890683122, 1.000000000000000000, 0.9659258262890683122, 1.000000000000000000, 0.9659258262890683122, 1.000000000000000000, 0.9659258262890683122, 1.000000000000000000, 0.9659258262890683122, 1.000000000000000000, 0.9659258262890683122, 1.000000000000000000, 0.9659258262890683122, 1.000000000000000000, 0.9659258262890683122, 1.000000000000000000, 0.9659258262890683122, 1.000000000000000000, 0.9659258262890683122, 1.000000000000000000, 0.9659258262890683122, 1.000000000000000000, 0.9659258262890683122, 1.000000000000000000, 0.9659258262890683122, 1.000000000000000000, 0.9659258262890683122, 1.000000000000000000, 0.9659258262890683122, 1.000000000000000000, 0.9659258262890683122, 1.000000000000000000, 0.9659258262890683122, 1.000000000000000000, 0.9659258262890683122, 1.000000000000000000, 0.9659258262890683122, 1.000000000000000000, 0.9659258262890683122, 1.000000000000000000, 0.9659258262890683122, 1.000000000000000000, 0.9659258262890683122, 1.000000000000000000, 0.9659258262890683122, 1.000000000000000000, 0.9659258262890683122, 1.000000000000000000, 0.9659258262890683122, 1.000000000000000000, 0.9659258262890683122, 1.000000000000000000, 0.9659258262890683122, 1.000000000000000000, 0.9659258262890683122, 1.000000000000000000, 0.9659258262890683122, 1.000000000000000000, 0.9659258262890683122, 1.000000000000000000, 0.9659258262890683122, 1.000000000000000000, 0.9659258262890683122, 1.000000000000000000, 0.9659258262890683122, 1.000000000000000000, 0.9659258262890683122, 1.000000000000000000, 0.9659258262890683122, 1.000000000000000000, 0.9659258262890683122, 1.000000000000000000, 0.9659258262890683122, 1.000000000000000000, 0.9659258262890683122, 1.000000000000000000, 0.9659258262890683122, 1.000000000000000000, 0.9659258262890683122, 1.000000000000000000, 0.9659258262890683122, 1.000000000000000000, 0.9659258262890683122, 1.000000000000000000, 0.9659258262890683122, 1.000000000000000000, 0.9659258262890683122, 1.000000000000000000, 0.9659258262890683122, 1.000000000000000000, 0.9659258262890683122, 1.000000000000000000, 0.9659258262890683122, 1.000000000000000000, 0.9659258262890683122, 1.000000000000000000, 0.9659258262890683122, 1.000000000000000000, 0.9659258262890683122, 1.000000000000000000, 0.9659258262890683122, 1.000000000000000000, 0.9659258262890683122, 1.000000000000000000, 0.9659258262890683122, 1.000000000000000000, 0.9659258262890683122, 1.000000000000000000, 0.9659258262890683122, 1.000000000000000000, 0.9659258262890683122, 1.000000000000000000, 0.9659258262890683122, 1.000000000000000000, 0.9659258262890683122, 1.000000000000000000, 0.9659258262890683122, 1.000000000000000000, 0.9659258262890683122, 1.000000000000000000) ) ) 
 REPRESENTATION_ITEM ( '' )  SURFACE ( )  );
#6388=CARTESIAN_POINT ( 'NONE',  ( 0.4068241469816281097, 0.05413385826771666132, 0.4176697321401328100 ) ) ;
#6390=CARTESIAN_POINT ( 'NONE',  ( -0.8727034120734901146, -0.05778040916215560624, -0.4822834645669293319 ) ) ;
#6392=CARTESIAN_POINT ( 'NONE',  ( 1.364829396325459854, -0.6046776061558809534, -0.2411417322834644161 ) ) ;
#6393=CARTESIAN_POINT ( 'NONE',  ( 0.5183727034120741983, 0.2952755905511810774, -0.1292274648535930714 ) ) ;
#6394=CARTESIAN_POINT ( 'NONE',  ( 0.2165354330708668673, -0.5400638737290844871, 0.3530559997133364547 ) ) ;
#6396=CARTESIAN_POINT ( 'NONE',  ( -0.7939632545931754048, -0.3162353388693405765, 0.4822834645669290543 ) ) ;
#6397=CARTESIAN_POINT ( 'NONE',  ( -0.09186351706036663400, -0.4281496062992124485, 0.4176697321401328655 ) ) ;
#6398=CARTESIAN_POINT ( 'NONE',  ( 0.07217847769028949700, -0.2845877964562159024, 0.3641732283464567677 ) ) ;
#6400=CARTESIAN_POINT ( 'NONE',  ( 0.01968503937007930540, 0.1660481256975885056, 0.3530559997133364547 ) ) ;
#6403=CARTESIAN_POINT ( 'NONE',  ( 0.9908136482939640111, 0.2952755905511810774, -0.1292274648535930714 ) ) ;
#6406=ORIENTED_EDGE ( 'NONE', *, *, #10993, .F. ) ;
#6407=CARTESIAN_POINT ( 'NONE',  ( 0.2034120734908144990, -0.6692913385826771977, 0.1292274648535927661 ) ) ;
#6408=CARTESIAN_POINT ( 'NONE',  ( -0.2624671916010490880, 0.1283753931104746893, -0.1820866141732285504 ) ) ;
#6409=CARTESIAN_POINT ( 'NONE',  ( 1.646981627296588035, -0.2845877964562159024, 0.3641732283464567677 ) ) ;
#6413=CARTESIAN_POINT ( 'NONE',  ( 1.430446194225722500, -0.3690944881889765550, -0.3153832671262227771 ) ) ;
#6415=CARTESIAN_POINT ( 'NONE',  ( -1.541994750656167090, -0.6692913385826773087, -0.1292274648535924053 ) ) ;
#6417=CARTESIAN_POINT ( 'NONE',  ( -0.1246719160104980823, 0.2952755905511811885, 0.1292274648535926551 ) ) ;
#6418=CARTESIAN_POINT ( 'NONE',  ( -1.062992125984250968, -0.6692913385826771977, 8.415575281601705876E-17 ) ) ;
#6419=CARTESIAN_POINT ( 'NONE',  ( -1.017060367454067249, -0.3162353388693409650, -0.4822834645669289433 ) ) ;
#6420=CARTESIAN_POINT ( 'NONE',  ( 0.4330708661417329575, -0.6692913385826771977, 8.415575281601705876E-17 ) ) ;
#6422=CARTESIAN_POINT ( 'NONE',  ( -1.528871391076114250, -0.5511811023622046335, 0.09757992244046803654 ) ) ;
#6423=CARTESIAN_POINT ( 'NONE',  ( 0.7677165354330716118, -0.5400638737290844871, 0.3530559997133364547 ) ) ;
#6424=CARTESIAN_POINT ( 'NONE',  ( 0.7742782152230979209, -0.004921259842519870586, -0.3153832671262229437 ) ) ;
#6425=CARTESIAN_POINT ( 'NONE',  ( 0.8005249343832027131, 0.009842519685039463617, 0.3409548833797002576 ) ) ;
#6426=CARTESIAN_POINT ( 'NONE',  ( 1.023622047244095334, -0.1870078740157479769, 0.3641732283464567677 ) ) ;
#6427=CARTESIAN_POINT ( 'NONE',  ( -1.469816272965878357, 0.2306618581243848609, 0.2411417322834645549 ) ) ;
#6429=CARTESIAN_POINT ( 'NONE',  ( 1.135170603674541256, -0.6692913385826773087, -0.1292274648535924053 ) ) ;
#6431=CARTESIAN_POINT ( 'NONE',  ( 0.5446194225721792126, -0.3162353388693405765, 0.4822834645669290543 ) ) ;
#6433=CARTESIAN_POINT ( 'NONE',  ( -1.456692913385826182, -0.5511811023622047445, 6.969142054262312111E-17 ) ) ;
#6434=CARTESIAN_POINT ( 'NONE',  ( 0.08530183727034192087, -0.05778040916215522460, 0.4822834645669289988 ) ) ;
#6435=CARTESIAN_POINT ( 'NONE',  ( 0.3215223097112867578, -0.08942795157527998196, 0.3641732283464567121 ) ) ;
#6436=CARTESIAN_POINT ( 'NONE',  ( 0.9908136482939640111, -0.6692913385826771977, 0.1292274648535927661 ) ) ;
#6438=CARTESIAN_POINT ( 'NONE',  ( -0.4986876640419942164, -0.5023911411419708095, 0.1820866141732285504 ) ) ;
#6439=CARTESIAN_POINT ( 'NONE',  ( -0.7611548556430438595, 0.2306618581243848609, 0.2411417322834645549 ) ) ;
#6440=CARTESIAN_POINT ( 'NONE',  ( 1.673228346456693494, 0.1660481256975885056, 0.3530559997133364547 ) ) ;
#6441=CARTESIAN_POINT ( 'NONE',  ( -1.089238845144356427, 0.05413385826771666132, 0.4176697321401328100 ) ) ;
#6442=CARTESIAN_POINT ( 'NONE',  ( 0.9383202099737538715, -0.05778040916215560624, -0.4822834645669293319 ) ) ;
#6444=CARTESIAN_POINT ( 'NONE',  ( -1.272965879265091305, -0.004921259842519870586, -0.3153832671262229437 ) ) ;
#6446=CARTESIAN_POINT ( 'NONE',  ( 1.069553805774278610, -0.6692913385826771977, 0.1292274648535927661 ) ) ;
#6447=VECTOR ( 'NONE', #46627, 39.37007874015748854 ) ;
#6449=CARTESIAN_POINT ( 'NONE',  ( -1.535433070866141225, 0.2952755905511811885, 0.000000000000000000 ) ) ;
#6450=CARTESIAN_POINT ( 'NONE',  ( -1.509186351706035767, -0.3690944881889763329, 0.3153832671262228327 ) ) ;
#6451=CARTESIAN_POINT ( 'NONE',  ( -1.003937007874015297, -0.4536011799217368745, -0.2665933059059886201 ) ) ;
#6452=CARTESIAN_POINT ( 'NONE',  ( 1.171093442848939681, -8.644661201599092366E-16, -0.4445507791589066171 ) ) ;
#6453=CARTESIAN_POINT ( 'NONE',  ( -0.4461942257217840213, -0.6046776061558809534, -0.2411417322834644161 ) ) ;
#6454=CARTESIAN_POINT ( 'NONE',  ( -0.2821522309711278487, -0.5511811023622048555, -0.09757992244046775898 ) ) ;
#6455=CARTESIAN_POINT ( 'NONE',  ( -1.541994750656167090, 0.1771653543307087630, 0.09757992244046791164 ) ) ;
#6456=CARTESIAN_POINT ( 'NONE',  ( 0.8202099737532813073, 0.1771653543307087630, 0.09757992244046791164 ) ) ;
#6457=CARTESIAN_POINT ( 'NONE',  ( 0.4199475065616805614, 0.2306618581243848609, 0.2411417322834645549 ) ) ;
#6458=CARTESIAN_POINT ( 'NONE',  ( 1.568241469816273437, -0.3162353388693405765, 0.4822834645669290543 ) ) ;
#6459=CARTESIAN_POINT ( 'NONE',  ( 0.2230971128608932319, -0.3690944881889763329, 0.3153832671262228327 ) ) ;
#6460=CARTESIAN_POINT ( 'NONE',  ( 0.6758530183727039509, -0.6692913385826771977, 0.1292274648535927661 ) ) ;
#6461=CARTESIAN_POINT ( 'NONE',  ( 0.6561679790026253567, 0.1283753931104748280, 0.1820866141732283561 ) ) ;
#6462=CARTESIAN_POINT ( 'NONE',  ( 1.535433070866142335, -0.6692913385826771977, 8.415575281601705876E-17 ) ) ;
#6463=CARTESIAN_POINT ( 'NONE',  ( -1.174540682414697335, -0.05778040916215522460, 0.4822834645669289988 ) ) ;
#6464=CARTESIAN_POINT ( 'NONE',  ( -0.4461942257217840213, 0.2306618581243848609, 0.2411417322834645549 ) ) ;
#6467=CARTESIAN_POINT ( 'NONE',  ( 0.6167979002624678353, -0.4281496062992124485, 0.4176697321401328655 ) ) ;
#6468=CARTESIAN_POINT ( 'NONE',  ( 1.102362204724410155, -0.1870078740157479769, 0.3641732283464567677 ) ) ;
#6469=CARTESIAN_POINT ( 'NONE',  ( -0.3018372703412066094, -0.4281496062992127816, -0.4176697321401328100 ) ) ;
#6470=CARTESIAN_POINT ( 'NONE',  ( 0.3937007874015754361, -0.1870078740157480879, -0.4822834645669291653 ) ) ;
#6471=EDGE_CURVE ( 'NONE', #74748, #6972, #29553, .T. ) ;
#6478=CARTESIAN_POINT ( 'NONE',  ( -0.8727034120734901146, -0.08942795157528024563, -0.3641732283464568787 ) ) ;
#6479=CARTESIAN_POINT ( 'NONE',  ( -0.9711286089238838626, -0.6046776061558807314, 0.2411417322834647770 ) ) ;
#6481=CARTESIAN_POINT ( 'NONE',  ( 0.9383202099737538715, -0.05778040916215560624, -0.4822834645669293319 ) ) ;
#6482=CARTESIAN_POINT ( 'NONE',  ( 1.325459317585302665, 0.05413385826771626580, -0.4176697321401330321 ) ) ;
#6483=CARTESIAN_POINT ( 'NONE',  ( 0.9711286089238851948, 0.2306618581243848609, 0.2411417322834645549 ) ) ;
#6484=CARTESIAN_POINT ( 'NONE',  ( -0.6175017169405814244, 0.000000000000000000, 0.3464511005275205946 ) ) ;
#6487=CARTESIAN_POINT ( 'NONE',  ( 1.620734908136483465, -0.6692913385826771977, 0.1292274648535927661 ) ) ;
#6488=CARTESIAN_POINT ( 'NONE',  ( 0.6889763779527563470, 0.1660481256975883668, -0.3530559997133364547 ) ) ;
#6489=CARTESIAN_POINT ( 'NONE',  ( 0.1640419947506569498, -0.05778040916215522460, 0.4822834645669289988 ) ) ;
#6490=CARTESIAN_POINT ( 'NONE',  ( 0.9055118110236227702, -0.5511811023622047445, 6.969142054262312111E-17 ) ) ;
#6491=CARTESIAN_POINT ( 'NONE',  ( 1.325459317585302665, -0.4281496062992124485, 0.4176697321401328655 ) ) ;
#6493=CARTESIAN_POINT ( 'NONE',  ( 0.5249343832021003964, 0.2306618581243847221, -0.2411417322834647770 ) ) ;
#6494=CARTESIAN_POINT ( 'NONE',  ( 1.266404199475066328, -0.3162353388693409650, -0.4822834645669289433 ) ) ;
#6495=CARTESIAN_POINT ( 'NONE',  ( 0.3871391076115493490, -0.3162353388693405765, 0.4822834645669290543 ) ) ;
#6496=CARTESIAN_POINT ( 'NONE',  ( 1.200787401574803681, 0.07958543189024085140, 0.2665933059059887866 ) ) ;
#6497=CARTESIAN_POINT ( 'NONE',  ( -0.9973753280839886548, -0.6046776061558809534, -0.2411417322834644161 ) ) ;
#6498=CARTESIAN_POINT ( 'NONE',  ( -0.8202099737532801971, -0.6692913385826771977, 0.1292274648535927661 ) ) ;
#6499=CARTESIAN_POINT ( 'NONE',  ( 1.102362204724410155, -0.1870078740157479769, 0.4822834645669291653 ) ) ;
#6505=ORIENTED_EDGE ( 'NONE', *, *, #45400, .T. ) ;
#6507=CARTESIAN_POINT ( 'NONE',  ( 1.463254593175853824, -0.6692913385826771977, 0.1292274648535927661 ) ) ;
#6508=CARTESIAN_POINT ( 'NONE',  ( 1.135170603674541256, 0.1771653543307087630, 0.09757992244046791164 ) ) ;
#6510=CARTESIAN_POINT ( 'NONE',  ( 1.240157480314961314, 0.07958543189024071263, -0.2665933059059888421 ) ) ;
#6511=LINE ( 'NONE', #69667, #55911 ) ;
#6512=CARTESIAN_POINT ( 'NONE',  ( -0.1049868766404193215, 0.2306618581243847221, -0.2411417322834647770 ) ) ;
#6515=CARTESIAN_POINT ( 'NONE',  ( -0.8070866141732276899, 0.07958543189024071263, -0.2665933059059888421 ) ) ;
#6516=CARTESIAN_POINT ( 'NONE',  ( -1.496062992125983815, -0.1870078740157480601, -0.3641732283464567677 ) ) ;
#6517=CARTESIAN_POINT ( 'NONE',  ( -1.391076115485563314, -0.6046776061558809534, -0.2411417322834644161 ) ) ;
#6518=CARTESIAN_POINT ( 'NONE',  ( -0.05249343832020938322, -0.6046776061558809534, -0.2411417322834644161 ) ) ;
#6519=CARTESIAN_POINT ( 'NONE',  ( 1.469816272965879911, 0.2306618581243847221, -0.2411417322834647770 ) ) ;
#6521=CARTESIAN_POINT ( 'NONE',  ( -1.168329637866467818, 0.004960608223778821026, 0.3437734562760189072 ) ) ;
#6522=( NAMED_UNIT ( * ) SI_UNIT ( $, .STERADIAN. ) SOLID_ANGLE_UNIT ( ) );
#6524=CARTESIAN_POINT ( 'NONE',  ( -1.646051170424378096, 0.000000000000000000, 0.3464511005275205946 ) ) ;
#6526=CARTESIAN_POINT ( 'NONE',  ( -0.8595800524934373854, -0.08942795157527998196, 0.3641732283464567121 ) ) ;
#6527=CARTESIAN_POINT ( 'NONE',  ( -1.135170603674539924, 0.2952755905511810774, -0.1292274648535930714 ) ) ;
#6528=CARTESIAN_POINT ( 'NONE',  ( 0.9120734908136490793, 0.2952755905511810774, -0.1292274648535930714 ) ) ;
#6529=ORIENTED_EDGE ( 'NONE', *, *, #39869, .T. ) ;
#6530=DIRECTION ( 'NONE',  ( 0.000000000000000000, 1.000000000000000000, 0.000000000000000000 ) ) ;
#6532=CARTESIAN_POINT ( 'NONE',  ( 1.384514435695538559, 0.2952755905511810774, -0.1292274648535930714 ) ) ;
#6533=CARTESIAN_POINT ( 'NONE',  ( -1.062992125984250968, 0.2952755905511811885, 0.000000000000000000 ) ) ;
#6535=CARTESIAN_POINT ( 'NONE',  ( -0.2690288713910754526, 0.1771653543307087075, -0.09757992244046823083 ) ) ;
#6537=CARTESIAN_POINT ( 'NONE',  ( -0.6364829396325453192, -0.08942795157528024563, -0.3641732283464568787 ) ) ;
#6538=CARTESIAN_POINT ( 'NONE',  ( 0.1049868766404206816, -0.5023911411419708095, -0.1820866141732282451 ) ) ;
#6539=CARTESIAN_POINT ( 'NONE',  ( 0.2755905511811031494, -0.6692913385826771977, 8.415575281601705876E-17 ) ) ;
#6540=CARTESIAN_POINT ( 'NONE',  ( -0.9842519685039360366, 0.1771653543307087630, 0.000000000000000000 ) ) ;
#6542=CARTESIAN_POINT ( 'NONE',  ( 1.312335958005249825, 0.2306618581243847221, -0.2411417322834647770 ) ) ;
#6543=CARTESIAN_POINT ( 'NONE',  ( -1.259842519685038686, -0.1870078740157480879, -0.4822834645669291653 ) ) ;
#6545=CARTESIAN_POINT ( 'NONE',  ( -0.1706036745406816491, -0.4281496062992124485, 0.4176697321401328655 ) ) ;
#6546=CARTESIAN_POINT ( 'NONE',  ( -0.7480314960629914633, -0.6692913385826771977, 8.415575281601705876E-17 ) ) ;
#6547=CARTESIAN_POINT ( 'NONE',  ( 0.6233595800524942554, -0.08942795157528024563, -0.3641732283464568787 ) ) ;
#6548=CARTESIAN_POINT ( 'NONE',  ( -0.2690288713910754526, 0.1771653543307087075, -0.09757992244046823083 ) ) ;
#6549=CARTESIAN_POINT ( 'NONE',  ( -0.5380577427821514602, -0.4281496062992127816, -0.4176697321401328100 ) ) ;
#6550=CARTESIAN_POINT ( 'NONE',  ( -1.102362204724408601, -0.1870078740157480879, -0.4822834645669291653 ) ) ;
#6551=CARTESIAN_POINT ( 'NONE',  ( -0.4051969335537399797, 5.961526036605507449E-15, -0.3791483426435156012 ) ) ;
#6552=CARTESIAN_POINT ( 'NONE',  ( 1.102362204724410155, -0.1870078740157480601, -0.3641732283464567677 ) ) ;
#6553=CARTESIAN_POINT ( 'NONE',  ( -0.4133858267716528645, -0.5400638737290844871, 0.3530559997133364547 ) ) ;
#6554=CARTESIAN_POINT ( 'NONE',  ( -1.555118110236219930, 0.1660481256975885056, 0.3530559997133364547 ) ) ;
#6557=CARTESIAN_POINT ( 'NONE',  ( -0.7217847769028863381, -0.3690944881889763329, 0.3153832671262228327 ) ) ;
#6558=CARTESIAN_POINT ( 'NONE',  ( 0.9120734908136489683, -0.6692913385826771977, 0.1292274648535927661 ) ) ;
#6559=CARTESIAN_POINT ( 'NONE',  ( -1.200787401574802349, 0.07958543189024071263, -0.2665933059059888421 ) ) ;
#6561=CARTESIAN_POINT ( 'NONE',  ( -0.8595800524934373854, -0.3162353388693409650, -0.4822834645669289433 ) ) ;
#6562=CARTESIAN_POINT ( 'NONE',  ( 0.9973753280839902091, -0.6046776061558807314, 0.2411417322834647770 ) ) ;
#6563=CARTESIAN_POINT ( 'NONE',  ( 0.5380577427821529035, -0.4281496062992124485, 0.4176697321401328655 ) ) ;
#6565=CARTESIAN_POINT ( 'NONE',  ( -1.555118110236219930, 0.07958543189024085140, 0.2665933059059887866 ) ) ;
#6571=CARTESIAN_POINT ( 'NONE',  ( 1.115485564304462551, -0.3690944881889765550, -0.3153832671262227771 ) ) ;
#6572=CARTESIAN_POINT ( 'NONE',  ( 0.4921259842519691285, 0.07958543189024085140, 0.2665933059059887866 ) ) ;
#6573=CARTESIAN_POINT ( 'NONE',  ( 0.07874015748031558404, -0.1870078740157480879, -0.4822834645669291653 ) ) ;
#6574=CARTESIAN_POINT ( 'NONE',  ( 1.502624671916010790, -0.3162353388693409650, -0.4822834645669289433 ) ) ;
#6576=CARTESIAN_POINT ( 'NONE',  ( 0.5643044619422579178, -0.004921259842519576551, 0.3153832671262227771 ) ) ;
#6577=CARTESIAN_POINT ( 'NONE',  ( -0.8464566929133852113, 0.1660481256975885056, 0.3530559997133364547 ) ) ;
#6578=CARTESIAN_POINT ( 'NONE',  ( -1.148293963254592542, 0.2952755905511811885, 0.1292274648535926551 ) ) ;
#6579=CARTESIAN_POINT ( 'NONE',  ( 0.8661417322834653598, -0.1870078740157479769, 0.4822834645669291653 ) ) ;
#6582=VERTEX_POINT ( 'NONE', #42181 ) ;
#6584=CARTESIAN_POINT ( 'NONE',  ( -1.220472440944881054, 0.2952755905511811885, 0.000000000000000000 ) ) ;
#6585=CARTESIAN_POINT ( 'NONE',  ( -0.4068241469816264999, -0.4281496062992124485, 0.4176697321401328655 ) ) ;
#6586=CARTESIAN_POINT ( 'NONE',  ( -0.8333333333333323711, 0.1771653543307087630, 0.09757992244046791164 ) ) ;
#6587=CARTESIAN_POINT ( 'NONE',  ( -0.6430446194225712953, 0.05413385826771626580, -0.4176697321401330321 ) ) ;
#6590=CARTESIAN_POINT ( 'NONE',  ( 1.640419947506562393, -0.4281496062992124485, 0.4176697321401328655 ) ) ;
#6591=CARTESIAN_POINT ( 'NONE',  ( -1.397637795275589623, 0.1660481256975885056, 0.3530559997133364547 ) ) ;
#6592=CARTESIAN_POINT ( 'NONE',  ( 0.5380577427821529035, 0.05413385826771626580, -0.4176697321401330321 ) ) ;
#6593=CARTESIAN_POINT ( 'NONE',  ( -0.9973753280839886548, 0.2306618581243848609, 0.2411417322834645549 ) ) ;
#6595=CARTESIAN_POINT ( 'NONE',  ( -0.6496062992125976043, 0.07958543189024071263, -0.2665933059059888421 ) ) ;
#6598=ORIENTED_EDGE ( 'NONE', *, *, #78238, .T. ) ;
#6599=CARTESIAN_POINT ( 'NONE',  ( -1.666666666666665853, -0.004921259842519870586, -0.3153832671262229437 ) ) ;
#6600=CARTESIAN_POINT ( 'NONE',  ( -1.227034120734907141, -0.6692913385826773087, -0.1292274648535924053 ) ) ;
#6601=CARTESIAN_POINT ( 'NONE',  ( -0.7611548556430438595, -0.6046776061558809534, -0.2411417322834644161 ) ) ;
#6603=CARTESIAN_POINT ( 'NONE',  ( -1.161417322834644716, -0.5400638737290845981, -0.3530559997133363437 ) ) ;
#6604=CARTESIAN_POINT ( 'NONE',  ( -1.167979002624671470, -0.4281496062992127816, -0.4176697321401328100 ) ) ;
#6607=CARTESIAN_POINT ( 'NONE',  ( 0.4265091863517067594, 0.1771653543307087630, 0.09757992244046791164 ) ) ;
#6608=CARTESIAN_POINT ( 'NONE',  ( 1.586052503253845503, 0.4724409448818907564, 0.1653254495020587411 ) ) ;
#6610=CARTESIAN_POINT ( 'NONE',  ( -0.4527559055118102749, 0.07958543189024085140, 0.2665933059059887866 ) ) ;
#6611=CARTESIAN_POINT ( 'NONE',  ( -0.7086614173228339419, -0.1870078740157479769, 0.4822834645669291653 ) ) ;
#6612=CARTESIAN_POINT ( 'NONE',  ( 1.161417322834646271, 0.1660481256975883668, -0.3530559997133364547 ) ) ;
#6613=CARTESIAN_POINT ( 'NONE',  ( -0.4330708661417315697, -0.6692913385826771977, 8.415575281601705876E-17 ) ) ;
#6617=CARTESIAN_POINT ( 'NONE',  ( -0.9120734908136475250, -0.6692913385826773087, -0.1292274648535924053 ) ) ;
#6618=CARTESIAN_POINT ( 'NONE',  ( 1.141732283464567566, 0.2952755905511811885, 0.000000000000000000 ) ) ;
#6619=CARTESIAN_POINT ( 'NONE',  ( -1.122047244094487306, -0.4536011799217367080, 0.2665933059059888421 ) ) ;
#6620=CARTESIAN_POINT ( 'NONE',  ( -1.220472440944881054, 0.2952755905511811885, 0.000000000000000000 ) ) ;
#6624=CARTESIAN_POINT ( 'NONE',  ( 0.08530183727034192087, -0.05778040916215522460, 0.4822834645669289988 ) ) ;
#6625=CARTESIAN_POINT ( 'NONE',  ( -1.043307086614172041, -0.4536011799217367080, 0.2665933059059888421 ) ) ;
#6626=CARTESIAN_POINT ( 'NONE',  ( -0.7874015748031489847, -0.1870078740157479769, 0.4822834645669291653 ) ) ;
#6628=CARTESIAN_POINT ( 'NONE',  ( -1.364829396325458521, 0.2306618581243847221, -0.2411417322834647770 ) ) ;
#6629=CARTESIAN_POINT ( 'NONE',  ( -0.9120734908136475250, 0.2952755905511811885, 0.1292274648535926551 ) ) ;
#6630=CARTESIAN_POINT ( 'NONE',  ( 0.09186351706036799403, -0.4281496062992127816, -0.4176697321401328100 ) ) ;
#6632=CARTESIAN_POINT ( 'NONE',  ( 0.7874015748031503170, -0.1870078740157479769, 0.3641732283464567677 ) ) ;
#6633=CARTESIAN_POINT ( 'NONE',  ( -0.7020997375328076329, -0.2845877964562161244, -0.3641732283464567121 ) ) ;
#6634=DIRECTION ( 'NONE',  ( -0.7071067811865462405, -0.000000000000000000, -0.7071067811865486830 ) ) ;
#6635=CARTESIAN_POINT ( 'NONE',  ( 0.7742782152230979209, -0.004921259842519870586, -0.3153832671262229437 ) ) ;
#6636=CARTESIAN_POINT ( 'NONE',  ( 1.299212598425197429, 0.1771653543307087630, 0.000000000000000000 ) ) ;
#6637=CARTESIAN_POINT ( 'NONE',  ( 1.213910761154856299, -0.6692913385826773087, -0.1292274648535924053 ) ) ;
#6638=CARTESIAN_POINT ( 'NONE',  ( -0.05249343832020911260, 0.1283753931104748280, 0.1820866141732283561 ) ) ;
#6640=CARTESIAN_POINT ( 'NONE',  ( -0.7349081364829387342, -0.6046776061558807314, 0.2411417322834647770 ) ) ;
#6641=CARTESIAN_POINT ( 'NONE',  ( 1.076115485564305141, -0.6046776061558807314, 0.2411417322834647770 ) ) ;
#6643=CARTESIAN_POINT ( 'NONE',  ( -0.3412073490813641308, 0.1283753931104746893, -0.1820866141732285504 ) ) ;
#6644=CARTESIAN_POINT ( 'NONE',  ( 0.01312335958005323398, 0.05413385826771666132, 0.4176697321401328100 ) ) ;
#6645=CARTESIAN_POINT ( 'NONE',  ( 0.1377952755905518800, 0.1660481256975883668, -0.3530559997133364547 ) ) ;
#6647=CARTESIAN_POINT ( 'NONE',  ( 0.9383202099737536495, -0.2845877964562159024, 0.3641732283464567677 ) ) ;
#6648=CARTESIAN_POINT ( 'NONE',  ( 0.1837270341207354329, 0.1283753931104748280, 0.1820866141732283561 ) ) ;
#6649=CARTESIAN_POINT ( 'NONE',  ( -0.04593175853018302557, 0.2952755905511811885, 0.1292274648535926551 ) ) ;
#6650=CARTESIAN_POINT ( 'NONE',  ( -1.312335958005248715, -0.6046776061558809534, -0.2411417322834644161 ) ) ;
#6651=CARTESIAN_POINT ( 'NONE',  ( -0.7611548556430438595, -0.5023911411419708095, -0.1820866141732282451 ) ) ;
#6653=CARTESIAN_POINT ( 'NONE',  ( -0.6889763779527552368, 0.1660481256975885056, 0.3530559997133364547 ) ) ;
#6655=EDGE_CURVE ( 'NONE', #66254, #65491, #69322, .T. ) ;
#6657=B_SPLINE_CURVE_WITH_KNOTS ( 'NONE', 3,
 ( #23197, #48868, #16913, #37064 ),
 .UNSPECIFIED., .F., .F.,
 ( 4, 4 ),
 ( 1.999999999927407068E-07, 0.006970199999999936863 ),
 .UNSPECIFIED. ) ;
#6658=CARTESIAN_POINT ( 'NONE',  ( 0.2559055118110243332, -0.4536011799217368745, -0.2665933059059886201 ) ) ;
#6659=CARTESIAN_POINT ( 'NONE',  ( -0.9645669291338575535, 0.1660481256975883668, -0.3530559997133364547 ) ) ;
#6660=CARTESIAN_POINT ( 'NONE',  ( -1.332020997375327642, -0.05778040916215522460, 0.4822834645669289988 ) ) ;
#6661=CARTESIAN_POINT ( 'NONE',  ( -1.174540682414697335, -0.08942795157527998196, 0.3641732283464567121 ) ) ;
#6662=CARTESIAN_POINT ( 'NONE',  ( 1.568241469816273659, -0.05778040916215560624, -0.4822834645669293319 ) ) ;
#6663=CARTESIAN_POINT ( 'NONE',  ( -0.4855643044619415427, 0.05413385826771626580, -0.4176697321401330321 ) ) ;
#6664=CARTESIAN_POINT ( 'NONE',  ( -0.8727034120734901146, -0.2845877964562159024, 0.3641732283464567677 ) ) ;
#6665=CARTESIAN_POINT ( 'NONE',  ( -1.725721784776902190, -0.08942795157527998196, 0.3641732283464567121 ) ) ;
#6666=CARTESIAN_POINT ( 'NONE',  ( 1.476377952755906220, 0.1660481256975883668, -0.3530559997133364547 ) ) ;
#6670=ORIENTED_EDGE ( 'NONE', *, *, #81439, .T. ) ;
#6672=CARTESIAN_POINT ( 'NONE',  ( -1.299212598425196097, -0.6692913385826771977, 8.415575281601705876E-17 ) ) ;
#6673=CARTESIAN_POINT ( 'NONE',  ( -0.9251968503937002541, 0.1660481256975885056, 0.3530559997133364547 ) ) ;
#6674=CARTESIAN_POINT ( 'NONE',  ( -1.574803149606298192, -0.1870078740157480879, -0.4822834645669291653 ) ) ;
#6677=CARTESIAN_POINT ( 'NONE',  ( 0.7152230971128616943, -0.05778040916215522460, 0.4822834645669289988 ) ) ;
#6678=CARTESIAN_POINT ( 'NONE',  ( -0.1377952755905504645, -0.5400638737290845981, -0.3530559997133363437 ) ) ;
#6680=CARTESIAN_POINT ( 'NONE',  ( -0.6986524979670485358, -2.191421614605370878E-15, 0.4445507791589071167 ) ) ;
#6681=CARTESIAN_POINT ( 'NONE',  ( 0.8661417322834652488, -0.1870078740157480601, -0.3641732283464567677 ) ) ;
#6686=ORIENTED_EDGE ( 'NONE', *, *, #14239, .T. ) ;
#6687=CARTESIAN_POINT ( 'NONE',  ( -0.2165354330708654795, -0.5400638737290845981, -0.3530559997133363437 ) ) ;
#6688=CARTESIAN_POINT ( 'NONE',  ( -0.8005249343832013809, -0.4281496062992124485, 0.4176697321401328655 ) ) ;
#6689=CARTESIAN_POINT ( 'NONE',  ( -1.423884514435694859, -0.05778040916215560624, -0.4822834645669293319 ) ) ;
#6690=CARTESIAN_POINT ( 'NONE',  ( 0.5511811023622055217, -0.1870078740157479769, 0.4822834645669291653 ) ) ;
#6691=CARTESIAN_POINT ( 'NONE',  ( 1.574803149606299746, -0.1870078740157480879, -0.4822834645669291653 ) ) ;
#6692=CARTESIAN_POINT ( 'NONE',  ( 1.456692913385827515, 0.2952755905511811885, 0.000000000000000000 ) ) ;
#6693=CARTESIAN_POINT ( 'NONE',  ( -0.4790026246719152336, -0.05778040916215560624, -0.4822834645669293319 ) ) ;
#6694=CARTESIAN_POINT ( 'NONE',  ( 0.4330708661417329575, -0.6692913385826771977, 8.415575281601705876E-17 ) ) ;
#6695=CARTESIAN_POINT ( 'NONE',  ( -1.509186351706035767, -0.4281496062992124485, 0.4176697321401328655 ) ) ;
#6696=CARTESIAN_POINT ( 'NONE',  ( 1.377952755905512472, -0.6692913385826771977, 8.415575281601705876E-17 ) ) ;
#6697=CARTESIAN_POINT ( 'NONE',  ( 1.469816272965879911, -0.6046776061558807314, 0.2411417322834647770 ) ) ;
#6698=CARTESIAN_POINT ( 'NONE',  ( -0.2624671916010490880, 0.2306618581243847221, -0.2411417322834647770 ) ) ;
#6700=CARTESIAN_POINT ( 'NONE',  ( 0.4133858267716541968, 0.07958543189024085140, 0.2665933059059887866 ) ) ;
#6703=ORIENTED_EDGE ( 'NONE', *, *, #63585, .F. ) ;
#6704=CARTESIAN_POINT ( 'NONE',  ( -0.4790026246719154557, -0.2845877964562159024, 0.3641732283464567677 ) ) ;
#6706=CARTESIAN_POINT ( 'NONE',  ( 0.2624671916010504757, -0.6046776061558809534, -0.2411417322834644161 ) ) ;
#6707=CARTESIAN_POINT ( 'NONE',  ( 0.01968503937007930540, 0.1660481256975885056, 0.3530559997133364547 ) ) ;
#6708=CARTESIAN_POINT ( 'NONE',  ( -0.9908136482939626788, -0.6692913385826773087, -0.1292274648535924053 ) ) ;
#6710=CARTESIAN_POINT ( 'NONE',  ( -1.292650918635170010, 0.2952755905511810774, -0.1292274648535930714 ) ) ;
#6712=CARTESIAN_POINT ( 'NONE',  ( 0.8267716535433077274, 0.1771653543307087630, 0.000000000000000000 ) ) ;
#6713=CARTESIAN_POINT ( 'NONE',  ( 0.5971128608923891301, 0.2952755905511810774, -0.1292274648535930714 ) ) ;
#6714=CARTESIAN_POINT ( 'NONE',  ( 0.6496062992125991586, -0.5400638737290845981, -0.3530559997133363437 ) ) ;
#6716=CARTESIAN_POINT ( 'NONE',  ( -1.620734908136482577, -0.6692913385826773087, -0.1292274648535924053 ) ) ;
#6719=CARTESIAN_POINT ( 'NONE',  ( -0.2427821522309703550, -0.05778040916215560624, -0.4822834645669293319 ) ) ;
#6722=CARTESIAN_POINT ( 'NONE',  ( -1.089238845144356427, -0.3690944881889765550, -0.3153832671262227771 ) ) ;
#6723=CARTESIAN_POINT ( 'NONE',  ( 1.371391076115485719, -0.6692913385826773087, -0.1292274648535924053 ) ) ;
#6724=CARTESIAN_POINT ( 'NONE',  ( 1.345144356955381593, -0.05778040916215522460, 0.4822834645669289988 ) ) ;
#6725=CARTESIAN_POINT ( 'NONE',  ( 0.1902887139107617975, -0.5511811023622048555, -0.09757992244046775898 ) ) ;
#6726=CARTESIAN_POINT ( 'NONE',  ( 0.3412073490813655186, 0.2306618581243848609, 0.2411417322834645549 ) ) ;
#6728=CARTESIAN_POINT ( 'NONE',  ( 0.2887139107611556010, 0.1283753931104746893, -0.1820866141732285504 ) ) ;
#6729=CARTESIAN_POINT ( 'NONE',  ( 0.07217847769028949700, -0.05778040916215560624, -0.4822834645669293319 ) ) ;
#6731=CARTESIAN_POINT ( 'NONE',  ( -1.076115485564303809, 0.2306618581243848609, 0.2411417322834645549 ) ) ;
#6732=CARTESIAN_POINT ( 'NONE',  ( 0.7086614173228352742, -0.1870078740157480601, -0.3641732283464567677 ) ) ;
#6734=CARTESIAN_POINT ( 'NONE',  ( -0.5249343832020990641, -0.6046776061558809534, -0.2411417322834644161 ) ) ;
#6735=CARTESIAN_POINT ( 'NONE',  ( -0.4068241469816264999, -0.3690944881889763329, 0.3153832671262228327 ) ) ;
#6737=CARTESIAN_POINT ( 'NONE',  ( -0.4461942257217840213, 0.2306618581243848609, 0.2411417322834645549 ) ) ;
#6738=CARTESIAN_POINT ( 'NONE',  ( -0.05249343832020911260, 0.2306618581243848609, 0.2411417322834645549 ) ) ;
#6739=CARTESIAN_POINT ( 'NONE',  ( 0.3280839895013130669, -0.004921259842519576551, 0.3153832671262227771 ) ) ;
#6741=CARTESIAN_POINT ( 'NONE',  ( 0.01312335958005323398, -0.4281496062992127816, -0.4176697321401328100 ) ) ;
#6743=CARTESIAN_POINT ( 'NONE',  ( 0.7611548556430454138, 0.1283753931104746893, -0.1820866141732285504 ) ) ;
#6744=CARTESIAN_POINT ( 'NONE',  ( 1.443569553805774897, 0.2306618581243848609, 0.2411417322834645549 ) ) ;
#6745=CARTESIAN_POINT ( 'NONE',  ( -0.9186351706036736120, 0.1283753931104748280, 0.1820866141732283561 ) ) ;
#6746=CARTESIAN_POINT ( 'NONE',  ( -0.7086614173228339419, -0.1870078740157480601, -0.3641732283464567677 ) ) ;
#6747=CARTESIAN_POINT ( 'NONE',  ( -0.5446194225721777693, -0.05778040916215522460, 0.4822834645669289988 ) ) ;
#6748=CARTESIAN_POINT ( 'NONE',  ( -0.09186351706036689768, 0.05413385826771626580, -0.4176697321401330321 ) ) ;
#6749=CARTESIAN_POINT ( 'NONE',  ( 0.5249343832021005074, -0.5023911411419708095, 0.1820866141732285504 ) ) ;
#6751=CARTESIAN_POINT ( 'NONE',  ( 1.200787401574803681, -0.4536011799217368745, -0.2665933059059886201 ) ) ;
#6752=CARTESIAN_POINT ( 'NONE',  ( 0.8661417322834653598, -0.1870078740157479769, 0.4822834645669291653 ) ) ;
#6754=CARTESIAN_POINT ( 'NONE',  ( -0.1902887139107604098, -0.6692913385826771977, 0.1292274648535927661 ) ) ;
#6756=CARTESIAN_POINT ( 'NONE',  ( 1.384514435695538337, -0.5511811023622046335, 0.09757992244046803654 ) ) ;
#6757=CARTESIAN_POINT ( 'NONE',  ( 0.7217847769028878924, 0.05413385826771666132, 0.4176697321401328100 ) ) ;
#6758=CARTESIAN_POINT ( 'NONE',  ( 0.2624671916010504757, 0.2306618581243848609, 0.2411417322834645549 ) ) ;
#6760=CARTESIAN_POINT ( 'NONE',  ( 0.4265091863517067594, 0.1771653543307087630, 0.09757992244046791164 ) ) ;
#6761=CARTESIAN_POINT ( 'NONE',  ( 0.9580052493438327987, -0.4281496062992127816, -0.4176697321401328100 ) ) ;
#6762=CARTESIAN_POINT ( 'NONE',  ( -0.1640419947506555343, -0.2845877964562159024, 0.3641732283464567677 ) ) ;
#6763=CARTESIAN_POINT ( 'NONE',  ( -0.5118110236220466680, 0.2952755905511811885, 0.000000000000000000 ) ) ;
#6765=CARTESIAN_POINT ( 'NONE',  ( -0.03937007874015669567, -0.6692913385826771977, 8.415575281601705876E-17 ) ) ;
#6767=CARTESIAN_POINT ( 'NONE',  ( -1.108923884514435132, -0.05778040916215560624, -0.4822834645669293319 ) ) ;
#6768=CARTESIAN_POINT ( 'NONE',  ( -0.6233595800524928121, -0.08942795157527998196, 0.3641732283464567121 ) ) ;
#6769=CARTESIAN_POINT ( 'NONE',  ( 0.5380577427821529035, 0.05413385826771626580, -0.4176697321401330321 ) ) ;
#6770=CARTESIAN_POINT ( 'NONE',  ( -1.266404199475064773, -0.3162353388693405765, 0.4822834645669290543 ) ) ;
#6771=CARTESIAN_POINT ( 'NONE',  ( -0.2099737532808391705, 0.2306618581243848609, 0.2411417322834645549 ) ) ;
#6773=CARTESIAN_POINT ( 'NONE',  ( 1.090776338374008336, 0.02791078216816447743, -0.4328096321851892525 ) ) ;
#6774=CARTESIAN_POINT ( 'NONE',  ( 1.259842519685040019, -0.1870078740157479769, 0.4822834645669291653 ) ) ;
#6775=CARTESIAN_POINT ( 'NONE',  ( 1.299212598425197429, -0.6692913385826771977, 8.415575281601705876E-17 ) ) ;
#6777=CARTESIAN_POINT ( 'NONE',  ( -1.627296587926508442, 0.2306618581243848609, 0.2411417322834645549 ) ) ;
#6778=CARTESIAN_POINT ( 'NONE',  ( -0.8530183727034112984, -0.4281496062992127816, -0.4176697321401328100 ) ) ;
#6781=EDGE_LOOP ( 'NONE', ( #54619, #28159, #27295, #66337 ) ) ;
#6782=CARTESIAN_POINT ( 'NONE',  ( -0.2493438320209966919, -0.3690944881889763329, 0.3153832671262228327 ) ) ;
#6784=ORIENTED_EDGE ( 'NONE', *, *, #83113, .F. ) ;
#6785=CARTESIAN_POINT ( 'NONE',  ( 0.3740157480314966754, 0.1660481256975883668, -0.3530559997133364547 ) ) ;
#6786=CARTESIAN_POINT ( 'NONE',  ( 0.5643044619422579178, -0.4281496062992127816, -0.4176697321401328100 ) ) ;
#6788=CARTESIAN_POINT ( 'NONE',  ( -0.4855643044619415427, -0.004921259842519870586, -0.3153832671262229437 ) ) ;
#6790=CARTESIAN_POINT ( 'NONE',  ( 0.9055118110236227702, 0.2952755905511811885, 0.000000000000000000 ) ) ;
#6792=CARTESIAN_POINT ( 'NONE',  ( 1.069553805774278610, -0.5511811023622046335, 0.09757992244046803654 ) ) ;
#6794=CARTESIAN_POINT ( 'NONE',  ( -0.6102362204724400829, -0.5400638737290845981, -0.3530559997133363437 ) ) ;
#6796=CARTESIAN_POINT ( 'NONE',  ( -0.7545931758530176614, -0.6692913385826773087, -0.1292274648535924053 ) ) ;
#6797=CARTESIAN_POINT ( 'NONE',  ( -1.358267716535432434, 0.07958543189024071263, -0.2665933059059888421 ) ) ;
#6798=CARTESIAN_POINT ( 'NONE',  ( -0.8070866141732276899, -0.5400638737290844871, 0.3530559997133364547 ) ) ;
#6799=CARTESIAN_POINT ( 'NONE',  ( 1.548556430446194954, 0.2306618581243847221, -0.2411417322834647770 ) ) ;
#6801=EDGE_LOOP ( 'NONE', ( #22046, #21938, #57621, #75683 ) ) ;
#6803=CARTESIAN_POINT ( 'NONE',  ( 0.1312335958005257930, 0.2306618581243847221, -0.2411417322834647770 ) ) ;
#6805=CARTESIAN_POINT ( 'NONE',  ( -0.8792650918635160906, 0.05413385826771626580, -0.4176697321401330321 ) ) ;
#6806=CARTESIAN_POINT ( 'NONE',  ( 1.417322834645670104, -0.1870078740157479769, 0.4822834645669291653 ) ) ;
#6807=CARTESIAN_POINT ( 'NONE',  ( 1.148293963254593653, 0.2952755905511810774, -0.1292274648535930714 ) ) ;
#6808=CARTESIAN_POINT ( 'NONE',  ( 0.09186351706036799403, -0.4281496062992127816, -0.4176697321401328100 ) ) ;
#6809=CARTESIAN_POINT ( 'NONE',  ( 0.09186351706036827158, 0.05413385826771666132, 0.4176697321401328100 ) ) ;
#6811=CARTESIAN_POINT ( 'NONE',  ( -1.154855643044618851, -0.6046776061558809534, -0.2411417322834644161 ) ) ;
#6812=CARTESIAN_POINT ( 'NONE',  ( -0.3018372703412066094, -0.4281496062992127816, -0.4176697321401328100 ) ) ;
#6813=CARTESIAN_POINT ( 'NONE',  ( -0.2230971128608915943, -0.004921259842519576551, 0.3153832671262227771 ) ) ;
#6814=CARTESIAN_POINT ( 'NONE',  ( 1.673228346456693494, 0.1660481256975885056, 0.3530559997133364547 ) ) ;
#6816=CARTESIAN_POINT ( 'NONE',  ( 1.377952755905512472, 0.2952755905511811885, 0.000000000000000000 ) ) ;
#6817=CARTESIAN_POINT ( 'NONE',  ( -0.006561679790025524116, -0.3162353388693405765, 0.4822834645669290543 ) ) ;
#6819=CARTESIAN_POINT ( 'NONE',  ( 1.017060367454068581, -0.05778040916215560624, -0.4822834645669293319 ) ) ;
#6820=CARTESIAN_POINT ( 'NONE',  ( 0.5118110236220478892, 0.2066929133858268208, 0.000000000000000000 ) ) ;
#6821=ORIENTED_EDGE ( 'NONE', *, *, #24369, .F. ) ;
#6824=CARTESIAN_POINT ( 'NONE',  ( 0.4921259842519691285, -0.5400638737290845981, -0.3530559997133363437 ) ) ;
#6825=CARTESIAN_POINT ( 'NONE',  ( -0.2362204724409442680, -0.1870078740157480601, -0.3641732283464567677 ) ) ;
#6826=CARTESIAN_POINT ( 'NONE',  ( 1.450131233595801428, -0.5511811023622048555, -0.09757992244046775898 ) ) ;
#6829=DIRECTION ( 'NONE',  ( 1.000000000000000000, -0.000000000000000000, -0.000000000000000000 ) ) ;
#6830=CARTESIAN_POINT ( 'NONE',  ( -1.587926509186350810, 0.05413385826771626580, -0.4176697321401330321 ) ) ;
#6832=CARTESIAN_POINT ( 'NONE',  ( 0.07217847769028949700, -0.05778040916215560624, -0.4822834645669293319 ) ) ;
#6833=LINE ( 'NONE', #13167, #53920 ) ;
#6834=CARTESIAN_POINT ( 'NONE',  ( -1.482939632545930975, -0.4281496062992127816, -0.4176697321401328100 ) ) ;
#6835=CARTESIAN_POINT ( 'NONE',  ( 0.3740157480314966754, 0.1660481256975883668, -0.3530559997133364547 ) ) ;
#6837=CARTESIAN_POINT ( 'NONE',  ( -1.535433070866141225, -0.5511811023622047445, 6.969142054262312111E-17 ) ) ;
#6838=CARTESIAN_POINT ( 'NONE',  ( 0.7545931758530188826, -0.6692913385826771977, 0.1292274648535927661 ) ) ;
#6839=CARTESIAN_POINT ( 'NONE',  ( 1.095800524934383846, -0.08942795157528024563, -0.3641732283464568787 ) ) ;
#6840=CARTESIAN_POINT ( 'NONE',  ( 0.8333333333333340365, 0.2066929133858267098, -0.1054918080437494132 ) ) ;
#6841=CARTESIAN_POINT ( 'NONE',  ( 0.7545931758530189937, 0.1771653543307087075, -0.09757992244046823083 ) ) ;
#6843=CARTESIAN_POINT ( 'NONE',  ( -1.450131233595799651, 0.2952755905511810774, -0.1292274648535930714 ) ) ;
#6845=CARTESIAN_POINT ( 'NONE',  ( 1.246719160104987623, 0.05413385826771626580, -0.4176697321401330321 ) ) ;
#6847=CARTESIAN_POINT ( 'NONE',  ( 0.9186351706036752773, 0.2306618581243847221, -0.2411417322834647770 ) ) ;
#6849=CARTESIAN_POINT ( 'NONE',  ( -1.614173228346457378, 1.055049524192299693, 0.1372047244094476981 ) ) ;
#6850=CARTESIAN_POINT ( 'NONE',  ( 0.4068241469816279987, -0.3690944881889765550, -0.3153832671262227771 ) ) ;
#6851=CARTESIAN_POINT ( 'NONE',  ( 0.6758530183727039509, -0.6692913385826771977, 0.1292274648535927661 ) ) ;
#6853=CARTESIAN_POINT ( 'NONE',  ( -1.056430446194224881, 0.1771653543307087075, -0.09757992244046823083 ) ) ;
#6854=CARTESIAN_POINT ( 'NONE',  ( -1.154855643044618851, -0.6046776061558809534, -0.2411417322834644161 ) ) ;
#6855=CARTESIAN_POINT ( 'NONE',  ( 1.653543307086614789, -0.1870078740157479769, 0.4822834645669291653 ) ) ;
#6856=CARTESIAN_POINT ( 'NONE',  ( -1.253280839895012377, -0.05778040916215522460, 0.4822834645669289988 ) ) ;
#6857=VECTOR ( 'NONE', #7092, 39.37007874015748143 ) ;
#6858=CARTESIAN_POINT ( 'NONE',  ( 1.122047244094488860, -0.5400638737290845981, -0.3530559997133363437 ) ) ;
#6859=CARTESIAN_POINT ( 'NONE',  ( -1.220472440944881054, -0.5511811023622047445, 6.969142054262312111E-17 ) ) ;
#6861=CARTESIAN_POINT ( 'NONE',  ( 0.9383202099737536495, -0.3162353388693405765, 0.4822834645669290543 ) ) ;
#6864=CARTESIAN_POINT ( 'NONE',  ( 1.227034120734908917, 0.2952755905511810774, -0.1292274648535930714 ) ) ;
#6865=CARTESIAN_POINT ( 'NONE',  ( -1.135170603674539924, -0.5511811023622046335, 0.09757992244046803654 ) ) ;
#6866=CARTESIAN_POINT ( 'NONE',  ( 1.633858267716535639, -0.4536011799217367080, 0.2665933059059888421 ) ) ;
#6867=CARTESIAN_POINT ( 'NONE',  ( -1.181102362204723644, -0.1870078740157479769, 0.3641732283464567677 ) ) ;
#6868=CARTESIAN_POINT ( 'NONE',  ( -0.4921259842519677963, 0.07958543189024071263, -0.2665933059059888421 ) ) ;
#6869=CARTESIAN_POINT ( 'NONE',  ( -1.410761154855642463, -0.08942795157527998196, 0.3641732283464567121 ) ) ;
#6870=CARTESIAN_POINT ( 'NONE',  ( 0.8792650918635177559, -0.3690944881889765550, -0.3153832671262227771 ) ) ;
#6871=CARTESIAN_POINT ( 'NONE',  ( 0.3477690288713918276, -0.6692913385826773087, -0.1292274648535924053 ) ) ;
#6872=CARTESIAN_POINT ( 'NONE',  ( -1.646051170424378096, -0.1870078740157480046, 1.254653134982923898E-17 ) ) ;
#6873=CARTESIAN_POINT ( 'NONE',  ( 0.2165354330708668673, -0.5400638737290844871, 0.3530559997133364547 ) ) ;
#6875=CARTESIAN_POINT ( 'NONE',  ( 0.6102362204724416372, -0.4536011799217367080, 0.2665933059059888421 ) ) ;
#6876=CARTESIAN_POINT ( 'NONE',  ( -1.614173228346455824, 0.2952755905511811885, 0.000000000000000000 ) ) ;
#6877=CARTESIAN_POINT ( 'NONE',  ( -1.397637795275589623, -0.5400638737290845981, -0.3530559997133363437 ) ) ;
#6878=CARTESIAN_POINT ( 'NONE',  ( -0.6627296587926503335, -0.6692913385826771977, 0.1292274648535927661 ) ) ;
#6881=CARTESIAN_POINT ( 'NONE',  ( 0.04593175853018440641, 0.2952755905511810774, -0.1292274648535930714 ) ) ;
#6882=CARTESIAN_POINT ( 'NONE',  ( 1.272965879265092637, -0.004921259842519576551, 0.3153832671262227771 ) ) ;
#6883=CARTESIAN_POINT ( 'NONE',  ( -0.3674540682414689785, 0.2306618581243848609, 0.2411417322834645549 ) ) ;
#6884=CARTESIAN_POINT ( 'NONE',  ( 0.4986876640419954376, 0.2306618581243848609, 0.2411417322834645549 ) ) ;
#6891=CARTESIAN_POINT ( 'NONE',  ( -1.115485564304461219, -0.3690944881889763329, 0.3153832671262228327 ) ) ;
#6893=CARTESIAN_POINT ( 'NONE',  ( -1.312335958005248715, -0.6046776061558809534, -0.2411417322834644161 ) ) ;
#6895=CARTESIAN_POINT ( 'NONE',  ( 0.2690288713910767848, 0.2952755905511811885, 0.1292274648535926551 ) ) ;
#6896=CARTESIAN_POINT ( 'NONE',  ( 1.141732283464567566, 0.2952755905511811885, 0.000000000000000000 ) ) ;
#6897=CARTESIAN_POINT ( 'NONE',  ( 0.6955380577427828781, 0.05413385826771626580, -0.4176697321401330321 ) ) ;
#6901=CARTESIAN_POINT ( 'NONE',  ( 1.312335958005250269, -0.6046776061558807314, 0.2411417322834647770 ) ) ;
#6902=CARTESIAN_POINT ( 'NONE',  ( 0.3805774278215230400, 0.05413385826771626580, -0.4176697321401330321 ) ) ;
#6903=CARTESIAN_POINT ( 'NONE',  ( 0.1837270341207354329, 0.2306618581243848609, 0.2411417322834645549 ) ) ;
#6904=CARTESIAN_POINT ( 'NONE',  ( 0.6167979002624678353, -0.3690944881889763329, 0.3153832671262228327 ) ) ;
#6905=CARTESIAN_POINT ( 'NONE',  ( 1.102362204724410155, -0.1870078740157480879, -0.4822834645669291653 ) ) ;
#6907=CARTESIAN_POINT ( 'NONE',  ( 0.1771653543307093182, 0.1660481256975885056, 0.3530559997133364547 ) ) ;
#6908=CARTESIAN_POINT ( 'NONE',  ( 0.8858267716535438430, 0.1660481256975885056, 0.3530559997133364547 ) ) ;
#6909=CARTESIAN_POINT ( 'NONE',  ( 0.5052493438320218022, -0.6692913385826773087, -0.1292274648535924053 ) ) ;
#6910=CARTESIAN_POINT ( 'NONE',  ( 1.292650918635171564, -0.5511811023622048555, -0.09757992244046775898 ) ) ;
#6911=CARTESIAN_POINT ( 'NONE',  ( -0.9251968503937002541, 0.1660481256975885056, 0.3530559997133364547 ) ) ;
#6912=CARTESIAN_POINT ( 'NONE',  ( -1.148293963254592542, -0.6692913385826773087, -0.1292274648535924053 ) ) ;
#6914=CARTESIAN_POINT ( 'NONE',  ( 1.312335958005249825, 0.2306618581243847221, -0.2411417322834647770 ) ) ;
#6921=CARTESIAN_POINT ( 'NONE',  ( 1.528871391076116026, 0.2952755905511811885, 0.1292274648535926551 ) ) ;
#6922=CARTESIAN_POINT ( 'NONE',  ( 1.161417322834646271, 0.07958543189024071263, -0.2665933059059888421 ) ) ;
#6924=CARTESIAN_POINT ( 'NONE',  ( 0.6199123404867349363, 8.471767977567108961E-16, -0.4445507791589058955 ) ) ;
#6928=CARTESIAN_POINT ( 'NONE',  ( -1.128608923884513837, 0.1283753931104746893, -0.1820866141732285504 ) ) ;
#6929=CARTESIAN_POINT ( 'NONE',  ( -1.437007874015747477, -0.4536011799217367080, 0.2665933059059888421 ) ) ;
#6930=CARTESIAN_POINT ( 'NONE',  ( -1.102362204724408601, -0.1870078740157480879, -0.4822834645669291653 ) ) ;
#6931=CARTESIAN_POINT ( 'NONE',  ( 0.2821522309711292364, -0.6692913385826771977, 0.1292274648535927661 ) ) ;
#6932=CARTESIAN_POINT ( 'NONE',  ( 1.410761154855643795, -0.3162353388693405765, 0.4822834645669290543 ) ) ;
#6937=DIRECTION ( 'NONE',  ( 0.000000000000000000, -1.000000000000000000, -0.000000000000000000 ) ) ;
#6938=CARTESIAN_POINT ( 'NONE',  ( -0.8858267716535425107, -0.4536011799217367080, 0.2665933059059888421 ) ) ;
#6939=CARTESIAN_POINT ( 'NONE',  ( 0.9317585301837276734, 0.009842519685039147898, -0.3409548833797004797 ) ) ;
#6940=CARTESIAN_POINT ( 'NONE',  ( 0.5643044619422579178, 0.05413385826771666132, 0.4176697321401328100 ) ) ;
#6943=DIRECTION ( 'NONE',  ( 1.000000000000000000, -0.000000000000000000, -0.000000000000000000 ) ) ;
#6945=CARTESIAN_POINT ( 'NONE',  ( 1.194225721784777594, 0.05413385826771666132, 0.4176697321401328100 ) ) ;
#6946=CARTESIAN_POINT ( 'NONE',  ( -1.450131233595799651, -0.6692913385826771977, 0.1292274648535927661 ) ) ;
#6948=CARTESIAN_POINT ( 'NONE',  ( -0.4133858267716528645, 0.07958543189024071263, -0.2665933059059888421 ) ) ;
#6949=CARTESIAN_POINT ( 'NONE',  ( -1.594488188976377119, 0.07958543189024071263, -0.2665933059059888421 ) ) ;
#6952=CARTESIAN_POINT ( 'NONE',  ( -0.5643044619422565855, -0.3690944881889763329, 0.3153832671262228327 ) ) ;
#6953=CARTESIAN_POINT ( 'NONE',  ( 0.2755905511811031494, -0.5511811023622047445, 6.969142054262312111E-17 ) ) ;
#6954=CARTESIAN_POINT ( 'NONE',  ( -0.05905511811023545637, -0.5400638737290845981, -0.3530559997133363437 ) ) ;
#6955=CARTESIAN_POINT ( 'NONE',  ( -1.141732283464566011, 0.1771653543307087630, 0.000000000000000000 ) ) ;
#6957=CARTESIAN_POINT ( 'NONE',  ( 1.227034120734908917, -0.6692913385826771977, 0.1292274648535927661 ) ) ;
#6958=CARTESIAN_POINT ( 'NONE',  ( -1.417322834645668772, -0.1870078740157480879, -0.4822834645669291653 ) ) ;
#6960=CARTESIAN_POINT ( 'NONE',  ( -0.2690288713910754526, 0.2952755905511810774, -0.1292274648535930714 ) ) ;
#6961=CARTESIAN_POINT ( 'NONE',  ( 0.3608923884514443348, 0.1771653543307087075, -0.09757992244046823083 ) ) ;
#6962=CARTESIAN_POINT ( 'NONE',  ( -1.115485564304461219, 0.05413385826771626580, -0.4176697321401330321 ) ) ;
#6963=CARTESIAN_POINT ( 'NONE',  ( 0.9908136482939640111, -0.5511811023622046335, 0.09757992244046803654 ) ) ;
#6964=CARTESIAN_POINT ( 'NONE',  ( -0.4002624671916004129, -0.08942795157528024563, -0.3641732283464568787 ) ) ;
#6965=CARTESIAN_POINT ( 'NONE',  ( -0.8267716535433065062, -0.6692913385826771977, 8.415575281601705876E-17 ) ) ;
#6966=CARTESIAN_POINT ( 'NONE',  ( -1.646981627296586703, -0.05778040916215522460, 0.4822834645669289988 ) ) ;
#6967=CARTESIAN_POINT ( 'NONE',  ( -0.4040399068613288458, -1.283732188437465593E-15, -0.4281993546915532911 ) ) ;
#6968=CARTESIAN_POINT ( 'NONE',  ( 1.450131233595801428, -0.5511811023622048555, -0.09757992244046775898 ) ) ;
#6969=CARTESIAN_POINT ( 'NONE',  ( -1.515748031496062076, -0.5400638737290844871, 0.3530559997133364547 ) ) ;
#6970=CARTESIAN_POINT ( 'NONE',  ( -1.607611548556429737, -0.6692913385826771977, 0.1292274648535927661 ) ) ;
#6972=VERTEX_POINT ( 'NONE', #53467 ) ;
#6975=CARTESIAN_POINT ( 'NONE',  ( -0.8792650918635160906, -0.3690944881889763329, 0.3153832671262228327 ) ) ;
#6976=CARTESIAN_POINT ( 'NONE',  ( 0.8136482939632553313, 0.2306618581243848609, 0.2411417322834645549 ) ) ;
#6977=CARTESIAN_POINT ( 'NONE',  ( -0.9973753280839886548, -0.5023911411419708095, -0.1820866141732282451 ) ) ;
#6979=CARTESIAN_POINT ( 'NONE',  ( -0.9251968503937002541, 0.1660481256975885056, 0.3530559997133364547 ) ) ;
#6980=CARTESIAN_POINT ( 'NONE',  ( 0.6627296587926517768, -0.6692913385826773087, -0.1292274648535924053 ) ) ;
#6981=CARTESIAN_POINT ( 'NONE',  ( 0.4068241469816281097, 0.05413385826771666132, 0.4176697321401328100 ) ) ;
#6982=FACE_OUTER_BOUND ( 'NONE', #33928, .T. ) ;
#6983=CARTESIAN_POINT ( 'NONE',  ( -1.653543307086613234, -0.1870078740157480601, -0.3641732283464567677 ) ) ;
#6989=CARTESIAN_POINT ( 'NONE',  ( 0.8989501312335964611, 0.1771653543307087630, 0.09757992244046791164 ) ) ;
#6990=CARTESIAN_POINT ( 'NONE',  ( 0.3346456692913390985, 0.07958543189024085140, 0.2665933059059887866 ) ) ;
#6991=CARTESIAN_POINT ( 'NONE',  ( -0.02624671916010428221, -0.6046776061558807314, 0.2411417322834647770 ) ) ;
#6992=CARTESIAN_POINT ( 'NONE',  ( 1.253280839895013710, -0.3162353388693405765, 0.4822834645669290543 ) ) ;
#6994=CARTESIAN_POINT ( 'NONE',  ( 0.4461942257217856311, 0.1283753931104746893, -0.1820866141732285504 ) ) ;
#6996=CARTESIAN_POINT ( 'NONE',  ( -0.5643044619422565855, -0.4281496062992124485, 0.4176697321401328655 ) ) ;
#6997=CARTESIAN_POINT ( 'NONE',  ( -1.404199475065615932, -0.4281496062992127816, -0.4176697321401328100 ) ) ;
#6998=CARTESIAN_POINT ( 'NONE',  ( 0.8464566929133866546, -0.5400638737290844871, 0.3530559997133364547 ) ) ;
#7000=CARTESIAN_POINT ( 'NONE',  ( -0.7677165354330700575, 0.1660481256975885056, 0.3530559997133364547 ) ) ;
#7003=CARTESIAN_POINT ( 'NONE',  ( -1.305774278215222184, -0.6692913385826773087, -0.1292274648535924053 ) ) ;
#7004=CARTESIAN_POINT ( 'NONE',  ( -0.8202099737532799750, 0.2952755905511810774, -0.1292274648535930714 ) ) ;
#7005=CARTESIAN_POINT ( 'NONE',  ( -0.6889763779527552368, 0.07958543189024085140, 0.2665933059059887866 ) ) ;
#7006=CARTESIAN_POINT ( 'NONE',  ( -0.9383202099737524282, -0.3162353388693409650, -0.4822834645669289433 ) ) ;
#7009=CARTESIAN_POINT ( 'NONE',  ( 1.535433070866142558, 0.2952755905511811885, 0.000000000000000000 ) ) ;
#7010=CARTESIAN_POINT ( 'NONE',  ( -1.266404199475064773, -0.3162353388693405765, 0.4822834645669290543 ) ) ;
#7011=CARTESIAN_POINT ( 'NONE',  ( 0.2034120734908142214, 0.2952755905511810774, -0.1292274648535930714 ) ) ;
#7012=CARTESIAN_POINT ( 'NONE',  ( -0.7152230971128602510, -0.3162353388693405765, 0.4822834645669290543 ) ) ;
#7013=CARTESIAN_POINT ( 'NONE',  ( 0.6692913385826777528, 0.2952755905511811885, 0.000000000000000000 ) ) ;
#7015=CARTESIAN_POINT ( 'NONE',  ( -0.8070866141732276899, 0.07958543189024071263, -0.2665933059059888421 ) ) ;
#7019=DIRECTION ( 'NONE',  ( -0.7071067811865472397, 0.000000000000000000, -0.7071067811865476838 ) ) ;
#7020=CARTESIAN_POINT ( 'NONE',  ( -0.9580052493438311334, -0.4281496062992124485, 0.4176697321401328655 ) ) ;
#7021=CARTESIAN_POINT ( 'NONE',  ( -1.148293963254592542, 0.2952755905511811885, 0.1292274648535926551 ) ) ;
#7023=CARTESIAN_POINT ( 'NONE',  ( -1.135170603674539924, -0.6692913385826771977, 0.1292274648535927661 ) ) ;
#7024=CARTESIAN_POINT ( 'NONE',  ( -1.108923884514435132, -0.3162353388693405765, 0.4822834645669290543 ) ) ;
#7025=CARTESIAN_POINT ( 'NONE',  ( -1.587926509186350810, 0.05413385826771626580, -0.4176697321401330321 ) ) ;
#7026=CARTESIAN_POINT ( 'NONE',  ( 0.9324623468618423727, 2.784432375088962958E-17, -0.3464511005275205946 ) ) ;
#7028=CARTESIAN_POINT ( 'NONE',  ( -0.1049868766404193215, -0.5023911411419708095, 0.1820866141732285504 ) ) ;
#7031=CARTESIAN_POINT ( 'NONE',  ( -0.3149606299212590610, -0.1870078740157479769, 0.3641732283464567677 ) ) ;
#7032=CARTESIAN_POINT ( 'NONE',  ( -0.9055118110236215490, -0.6692913385826771977, 8.415575281601705876E-17 ) ) ;
#7033=CARTESIAN_POINT ( 'NONE',  ( 1.312335958005249825, 0.2306618581243847221, -0.2411417322834647770 ) ) ;
#7034=CARTESIAN_POINT ( 'NONE',  ( -0.6496062992125976043, 0.1660481256975883668, -0.3530559997133364547 ) ) ;
#7035=ORIENTED_EDGE ( 'NONE', *, *, #5292, .F. ) ;
#7038=CARTESIAN_POINT ( 'NONE',  ( -1.181102362204723644, -0.1870078740157479769, 0.4822834645669291653 ) ) ;
#7039=VECTOR ( 'NONE', #77599, 39.37007874015748143 ) ;
#7040=CARTESIAN_POINT ( 'NONE',  ( 1.463254593175853824, 0.2952755905511810774, -0.1292274648535930714 ) ) ;
#7041=CARTESIAN_POINT ( 'NONE',  ( -1.561679790026246017, -0.004921259842519576551, 0.3153832671262227771 ) ) ;
#7042=CARTESIAN_POINT ( 'NONE',  ( -1.279527559055116948, -0.5400638737290844871, 0.3530559997133364547 ) ) ;
#7047=CARTESIAN_POINT ( 'NONE',  ( -0.07874015748031421014, -0.1870078740157479769, 0.4822834645669291653 ) ) ;
#7048=CARTESIAN_POINT ( 'NONE',  ( -1.587926509186350810, -0.004921259842519870586, -0.3153832671262229437 ) ) ;
#7049=CARTESIAN_POINT ( 'NONE',  ( -0.6430446194225716283, -0.4281496062992124485, 0.4176697321401328655 ) ) ;
#7051=CARTESIAN_POINT ( 'NONE',  ( -1.194225721784776262, 0.05413385826771626580, -0.4176697321401330321 ) ) ;
#7052=DIRECTION ( 'NONE',  ( -1.000000000000000000, 0.000000000000000000, 0.000000000000000000 ) ) ;
#7053=ADVANCED_FACE ( 'NONE', ( #39173 ), #32342, .F. ) ;
#7054=CARTESIAN_POINT ( 'NONE',  ( -0.8661417322834640276, -0.1870078740157480879, -0.4822834645669291653 ) ) ;
#7055=CARTESIAN_POINT ( 'NONE',  ( -0.2690288713910754526, 0.2952755905511810774, -0.1292274648535930714 ) ) ;
#7057=CARTESIAN_POINT ( 'NONE',  ( 0.9514435695538062676, -0.08942795157527998196, 0.3641732283464567121 ) ) ;
#7059=CARTESIAN_POINT ( 'NONE',  ( 0.6496062992125991586, -0.4536011799217368745, -0.2665933059059886201 ) ) ;
#7060=CARTESIAN_POINT ( 'NONE',  ( 1.286089238845145033, 0.1283753931104748280, 0.1820866141732283561 ) ) ;
#7061=CARTESIAN_POINT ( 'NONE',  ( 1.266404199475066328, -0.05778040916215522460, 0.4822834645669289988 ) ) ;
#7062=CARTESIAN_POINT ( 'NONE',  ( 0.2690288713910767848, 0.1771653543307087630, 0.09757992244046791164 ) ) ;
#7064=CARTESIAN_POINT ( 'NONE',  ( -0.8202099737532799750, 0.2952755905511810774, -0.1292274648535930714 ) ) ;
#7065=CARTESIAN_POINT ( 'NONE',  ( 1.220472440944882386, -0.6692913385826771977, 8.415575281601705876E-17 ) ) ;
#7067=CARTESIAN_POINT ( 'NONE',  ( -0.6102362204724400829, -0.4536011799217368745, -0.2665933059059886201 ) ) ;
#7068=CARTESIAN_POINT ( 'NONE',  ( -0.4265091863517051496, 0.2952755905511810219, -0.1292274648535930437 ) ) ;
#7069=CARTESIAN_POINT ( 'NONE',  ( 0.2493438320209980519, 0.05413385826771666132, 0.4176697321401328100 ) ) ;
#7070=CARTESIAN_POINT ( 'NONE',  ( -1.646051170424378096, -0.1870078740157480046, 1.254653134982923898E-17 ) ) ;
#7071=CARTESIAN_POINT ( 'NONE',  ( 0.8333333333333340365, 0.1771653543307087075, -0.09757992244046823083 ) ) ;
#7072=CARTESIAN_POINT ( 'NONE',  ( 0.09842519685039434474, -0.4536011799217368745, -0.2665933059059886201 ) ) ;
#7073=CARTESIAN_POINT ( 'NONE',  ( -0.2427821522309703550, -0.3162353388693405765, 0.4822834645669290543 ) ) ;
#7074=CARTESIAN_POINT ( 'NONE',  ( -1.541994750656167090, 0.2952755905511811885, 0.1292274648535926551 ) ) ;
#7075=CARTESIAN_POINT ( 'NONE',  ( -0.6036745406824141069, -0.5023911411419708095, -0.1820866141732282451 ) ) ;
#7076=CARTESIAN_POINT ( 'NONE',  ( -1.614173228346457378, 1.055049524192299693, -0.1372047244094477536 ) ) ;
#7077=CARTESIAN_POINT ( 'NONE',  ( -1.003937007874014853, 0.1660481256975885056, 0.3530559997133364547 ) ) ;
#7080=CARTESIAN_POINT ( 'NONE',  ( -0.01312335958005186876, -0.3690944881889763329, 0.3153832671262228327 ) ) ;
#7081=CARTESIAN_POINT ( 'NONE',  ( -0.5839895013123351797, -0.6692913385826771977, 0.1292274648535927661 ) ) ;
#7082=CARTESIAN_POINT ( 'NONE',  ( -0.9251968503937002541, -0.5400638737290845981, -0.3530559997133363437 ) ) ;
#7083=CARTESIAN_POINT ( 'NONE',  ( -1.181102362204723644, -0.1870078740157479769, 0.3641732283464567677 ) ) ;
#7084=CARTESIAN_POINT ( 'NONE',  ( -1.646051170424378096, 0.000000000000000000, -0.3464511005275205946 ) ) ;
#7085=CARTESIAN_POINT ( 'NONE',  ( -0.9514435695538050464, -0.08942795157528024563, -0.3641732283464568787 ) ) ;
#7086=CARTESIAN_POINT ( 'NONE',  ( -1.417322834645668772, -0.1870078740157479769, 0.3641732283464567677 ) ) ;
#7087=CARTESIAN_POINT ( 'NONE',  ( 1.364829396325459854, -0.6046776061558809534, -0.2411417322834644161 ) ) ;
#7092=DIRECTION ( 'NONE',  ( 1.000000000000000000, -0.000000000000000000, -0.000000000000000000 ) ) ;
#7093=CARTESIAN_POINT ( 'NONE',  ( -1.679790026246718693, 0.2306618581243847221, -0.2411417322834647770 ) ) ;
#7094=CARTESIAN_POINT ( 'NONE',  ( -1.102362204724408601, -0.1870078740157479769, 0.4822834645669291653 ) ) ;
#7095=CARTESIAN_POINT ( 'NONE',  ( 1.325459317585302665, 0.05413385826771626580, -0.4176697321401330321 ) ) ;
#7098=CARTESIAN_POINT ( 'NONE',  ( 0.5643044619422579178, 0.05413385826771666132, 0.4176697321401328100 ) ) ;
#7099=CARTESIAN_POINT ( 'NONE',  ( 0.01968503937007957949, -0.5400638737290845981, -0.3530559997133363437 ) ) ;
#7102=CARTESIAN_POINT ( 'NONE',  ( 0.8464566929133865436, 0.07958543189024071263, -0.2665933059059888421 ) ) ;
#7107=CARTESIAN_POINT ( 'NONE',  ( 0.1509186351706042484, -0.3162353388693405765, 0.4822834645669290543 ) ) ;
#7108=CARTESIAN_POINT ( 'NONE',  ( 1.601049868766404982, 0.2306618581243848609, 0.2411417322834645549 ) ) ;
#7109=CARTESIAN_POINT ( 'NONE',  ( 0.6692913385826778638, -0.6692913385826771977, 8.415575281601705876E-17 ) ) ;
#7110=CARTESIAN_POINT ( 'NONE',  ( 1.305774278215223960, -0.6692913385826771977, 0.1292274648535927661 ) ) ;
#7111=CARTESIAN_POINT ( 'NONE',  ( 1.502624671916010790, -0.3162353388693409650, -0.4822834645669289433 ) ) ;
#7112=CARTESIAN_POINT ( 'NONE',  ( -0.5839895013123351797, -0.6692913385826771977, 0.1292274648535927661 ) ) ;
#7113=CARTESIAN_POINT ( 'NONE',  ( 0.2034120734908142214, 0.2952755905511810774, -0.1292274648535930714 ) ) ;
#7114=CARTESIAN_POINT ( 'NONE',  ( -1.482939632545930975, 0.05413385826771666132, 0.4176697321401328100 ) ) ;
#7115=CARTESIAN_POINT ( 'NONE',  ( 1.384514435695538337, -0.6692913385826771977, 0.1292274648535927661 ) ) ;
#7116=CARTESIAN_POINT ( 'NONE',  ( 1.010498687664042716, -0.4281496062992124485, 0.4176697321401328655 ) ) ;
#7117=CARTESIAN_POINT ( 'NONE',  ( -0.03937007874015669567, -0.6692913385826771977, 8.415575281601705876E-17 ) ) ;
#7119=CARTESIAN_POINT ( 'NONE',  ( 0.4461942257217856311, 0.1283753931104746893, -0.1820866141732285504 ) ) ;
#7120=VERTEX_POINT ( 'NONE', #45895 ) ;
#7123=CARTESIAN_POINT ( 'NONE',  ( -0.3018372703412066094, -0.004921259842519576551, 0.3153832671262227771 ) ) ;
#7125=CARTESIAN_POINT ( 'NONE',  ( 0.03937007874015806264, 0.2952755905511811885, 0.000000000000000000 ) ) ;
#7126=CARTESIAN_POINT ( 'NONE',  ( -0.03280839895013062252, -0.6692913385826771977, 0.1292274648535927661 ) ) ;
#7127=CARTESIAN_POINT ( 'NONE',  ( -1.095800524934382292, -0.05778040916215522460, 0.4822834645669289988 ) ) ;
#7128=CARTESIAN_POINT ( 'NONE',  ( 1.496062992125985147, -0.1870078740157479769, 0.3641732283464567677 ) ) ;
#7129=CARTESIAN_POINT ( 'NONE',  ( -1.640419947506561060, 0.05413385826771666132, 0.4176697321401328100 ) ) ;
#7131=CARTESIAN_POINT ( 'NONE',  ( 0.8070866141732288002, 0.07958543189024085140, 0.2665933059059887866 ) ) ;
#7133=CARTESIAN_POINT ( 'NONE',  ( 0.6561679790026253567, -0.6046776061558809534, -0.2411417322834644161 ) ) ;
#7134=CARTESIAN_POINT ( 'NONE',  ( 0.8070866141732289112, -0.5400638737290845981, -0.3530559997133363437 ) ) ;
#7136=CARTESIAN_POINT ( 'NONE',  ( -1.640419947506561060, -0.4281496062992127816, -0.4176697321401328100 ) ) ;
#7139=CARTESIAN_POINT ( 'NONE',  ( 5.463695987328526437E-16, -0.1870078740157479769, 0.4822834645669291653 ) ) ;
#7142=CARTESIAN_POINT ( 'NONE',  ( -1.017060367454067249, -0.08942795157527998196, 0.3641732283464567121 ) ) ;
#7143=CARTESIAN_POINT ( 'NONE',  ( 1.305774278215223960, 0.2952755905511810774, -0.1292274648535930714 ) ) ;
#7144=CARTESIAN_POINT ( 'NONE',  ( 1.148293963254593875, -0.6692913385826771977, 0.1292274648535927661 ) ) ;
#7145=CARTESIAN_POINT ( 'NONE',  ( 0.1771653543307093182, -0.4536011799217368745, -0.2665933059059886201 ) ) ;
#7146=CARTESIAN_POINT ( 'NONE',  ( 0.3346456692913390985, 0.1660481256975885056, 0.3530559997133364547 ) ) ;
#7148=CARTESIAN_POINT ( 'NONE',  ( 0.4396325459317593221, 0.1771653543307087075, -0.09757992244046823083 ) ) ;
#7149=CARTESIAN_POINT ( 'NONE',  ( 0.1443569553805781891, -0.4281496062992124485, 0.4176697321401328655 ) ) ;
#7151=CIRCLE ( 'NONE', #29971, 3.582677165354331450 ) ;
#7153=CARTESIAN_POINT ( 'NONE',  ( -1.233595800524933894, 0.2306618581243848609, 0.2411417322834645549 ) ) ;
#7154=CARTESIAN_POINT ( 'NONE',  ( 0.3805774278215230400, -0.004921259842519870586, -0.3153832671262229437 ) ) ;
#7155=CARTESIAN_POINT ( 'NONE',  ( -1.167979002624671470, 0.05413385826771666132, 0.4176697321401328100 ) ) ;
#7156=CARTESIAN_POINT ( 'NONE',  ( -0.7611548556430438595, 0.2306618581243848609, 0.2411417322834645549 ) ) ;
#7157=CARTESIAN_POINT ( 'NONE',  ( -0.1312335958005241554, -0.5023911411419708095, -0.1820866141732282451 ) ) ;
#7159=CARTESIAN_POINT ( 'NONE',  ( -0.9448818897637790704, -0.1870078740157479769, 0.4822834645669291653 ) ) ;
#7160=CARTESIAN_POINT ( 'NONE',  ( -0.05905511811023545637, 0.1660481256975885056, 0.3530559997133364547 ) ) ;
#7161=CARTESIAN_POINT ( 'NONE',  ( 0.4921259842519691285, 0.07958543189024085140, 0.2665933059059887866 ) ) ;
#7163=CARTESIAN_POINT ( 'NONE',  ( 0.03280839895013198948, -0.6692913385826773087, -0.1292274648535924053 ) ) ;
#7166=CARTESIAN_POINT ( 'NONE',  ( 0.7677165354330716118, 0.07958543189024071263, -0.2665933059059888421 ) ) ;
#7167=CARTESIAN_POINT ( 'NONE',  ( 1.417322834645670104, -0.1870078740157479769, 0.4822834645669291653 ) ) ;
#7168=CARTESIAN_POINT ( 'NONE',  ( -0.8005249343832013809, -0.3690944881889763329, 0.3153832671262228327 ) ) ;
#7169=CARTESIAN_POINT ( 'NONE',  ( -1.043307086614172707, 0.07958543189024071263, -0.2665933059059888421 ) ) ;
#7170=CARTESIAN_POINT ( 'NONE',  ( -0.6496062992125976043, 0.1660481256975883668, -0.3530559997133364547 ) ) ;
#7171=CARTESIAN_POINT ( 'NONE',  ( -0.1640419947506555343, -0.3162353388693405765, 0.4822834645669290543 ) ) ;
#7172=CARTESIAN_POINT ( 'NONE',  ( 0.3937007874015754361, -0.1870078740157479769, 0.3641732283464567677 ) ) ;
#7174=CARTESIAN_POINT ( 'NONE',  ( 0.9842519685039375910, 0.1771653543307087630, 0.000000000000000000 ) ) ;
#7175=CARTESIAN_POINT ( 'NONE',  ( 0.3215223097112867578, -0.3162353388693409650, -0.4822834645669289433 ) ) ;
#7177=CARTESIAN_POINT ( 'NONE',  ( -0.3608923884514428360, -0.6692913385826773087, -0.1292274648535924053 ) ) ;
#7179=CARTESIAN_POINT ( 'NONE',  ( 1.450131233595801428, 0.1771653543307087630, 0.09757992244046791164 ) ) ;
#7180=CARTESIAN_POINT ( 'NONE',  ( 0.4790026246719168435, -0.3162353388693409650, -0.4822834645669289433 ) ) ;
#7181=CARTESIAN_POINT ( 'NONE',  ( 0.3346456692913393205, -0.5400638737290845981, -0.3530559997133363437 ) ) ;
#7182=CARTESIAN_POINT ( 'NONE',  ( 1.113061397484515158, -1.206088964116209378E-16, 0.4118477457932991359 ) ) ;
#7183=CARTESIAN_POINT ( 'NONE',  ( -0.1049868766404193215, -0.5023911411419708095, 0.1820866141732285504 ) ) ;
#7184=CARTESIAN_POINT ( 'NONE',  ( 0.8267716535433078384, -0.6692913385826771977, 8.415575281601705876E-17 ) ) ;
#7185=CARTESIAN_POINT ( 'NONE',  ( -0.1312335958005241554, 0.1283753931104748280, 0.1820866141732283561 ) ) ;
#7186=CARTESIAN_POINT ( 'NONE',  ( -0.8070866141732276899, 0.1660481256975883668, -0.3530559997133364547 ) ) ;
#7187=CARTESIAN_POINT ( 'NONE',  ( -0.3149606299212590610, -0.1870078740157479769, 0.4822834645669291653 ) ) ;
#7189=CARTESIAN_POINT ( 'NONE',  ( -1.161417322834644716, 0.1660481256975885056, 0.3530559997133364547 ) ) ;
#7190=AXIS2_PLACEMENT_3D ( 'NONE', #65591, #352, #7503 ) ;
#7191=CARTESIAN_POINT ( 'NONE',  ( -0.6955380577427815458, -0.3690944881889765550, -0.3153832671262227771 ) ) ;
#7192=CARTESIAN_POINT ( 'NONE',  ( 0.09842519685039434474, -0.5400638737290845981, -0.3530559997133363437 ) ) ;
#7193=CARTESIAN_POINT ( 'NONE',  ( -1.437007874015747477, -0.5400638737290844871, 0.3530559997133364547 ) ) ;
#7194=CARTESIAN_POINT ( 'NONE',  ( -0.7808398950131222316, -0.3162353388693409650, -0.4822834645669289433 ) ) ;
#7196=CARTESIAN_POINT ( 'NONE',  ( 1.653543307086614789, -0.1870078740157479769, 0.4822834645669291653 ) ) ;
#7197=CARTESIAN_POINT ( 'NONE',  ( 1.279527559055118724, 0.1660481256975885056, 0.3530559997133364547 ) ) ;
#7198=CARTESIAN_POINT ( 'NONE',  ( 1.391076115485564868, 0.2306618581243847221, -0.2411417322834647770 ) ) ;
#7201=B_SPLINE_CURVE_WITH_KNOTS ( 'NONE', 3,
 ( #3584, #82261, #42280, #29250, #43100, #74711, #24579 ),
 .UNSPECIFIED., .F., .F.,
 ( 4, 3, 4 ),
 ( 3.642919299551295515E-17, 0.001246232571205268744, 0.002492492258783277591 ),
 .UNSPECIFIED. ) ;
#7202=CARTESIAN_POINT ( 'NONE',  ( -1.515748031496062076, 0.1660481256975883668, -0.3530559997133364547 ) ) ;
#7206=CARTESIAN_POINT ( 'NONE',  ( -0.1837270341207340729, 0.1283753931104746893, -0.1820866141732285504 ) ) ;
#7207=VECTOR ( 'NONE', #69539, 39.37007874015748143 ) ;
#7209=VERTEX_POINT ( 'NONE', #78757 ) ;
#7210=CARTESIAN_POINT ( 'NONE',  ( 0.2690288713910767848, -0.6692913385826773087, -0.1292274648535924053 ) ) ;
#7211=CARTESIAN_POINT ( 'NONE',  ( 0.3346456692913390985, 0.1660481256975885056, 0.3530559997133364547 ) ) ;
#7213=CARTESIAN_POINT ( 'NONE',  ( 2.795275590551181466, 0.4724409448818907564, -3.234977217930338483E-16 ) ) ;
#7214=CARTESIAN_POINT ( 'NONE',  ( -0.9448818897637790704, -0.1870078740157480601, -0.3641732283464567677 ) ) ;
#7215=CARTESIAN_POINT ( 'NONE',  ( 0.9448818897637802916, -0.1870078740157480879, -0.4822834645669291653 ) ) ;
#7216=CARTESIAN_POINT ( 'NONE',  ( 0.9448818897637802916, -0.1870078740157479769, 0.3641732283464567677 ) ) ;
#7217=CARTESIAN_POINT ( 'NONE',  ( -0.3149606299212590610, -0.1870078740157480879, -0.4822834645669291653 ) ) ;
#7219=CARTESIAN_POINT ( 'NONE',  ( -0.7480314960629914633, -0.6692913385826771977, 8.415575281601705876E-17 ) ) ;
#7220=CARTESIAN_POINT ( 'NONE',  ( -1.653543307086613234, -0.1870078740157480601, -0.3641732283464567677 ) ) ;
#7221=CARTESIAN_POINT ( 'NONE',  ( -0.8661417322834640276, -0.1870078740157480879, -0.4822834645669291653 ) ) ;
#7222=CARTESIAN_POINT ( 'NONE',  ( 1.463254593175853824, -0.6692913385826771977, 0.1292274648535927661 ) ) ;
#7226=CARTESIAN_POINT ( 'NONE',  ( 0.006561679790026889343, -0.3162353388693409650, -0.4822834645669289433 ) ) ;
#7228=CARTESIAN_POINT ( 'NONE',  ( -0.8530183727034112984, -0.4281496062992127816, -0.4176697321401328100 ) ) ;
#7229=CARTESIAN_POINT ( 'NONE',  ( 1.351706036745407458, -0.4281496062992127816, -0.4176697321401328100 ) ) ;
#7230=CARTESIAN_POINT ( 'NONE',  ( 1.108923884514436242, -0.05778040916215522460, 0.4822834645669289988 ) ) ;
#7231=CARTESIAN_POINT ( 'NONE',  ( 0.3740157480314966754, 0.1660481256975883668, -0.3530559997133364547 ) ) ;
#7232=CARTESIAN_POINT ( 'NONE',  ( -0.3543307086614165824, 0.2952755905511811885, 0.000000000000000000 ) ) ;
#7234=CARTESIAN_POINT ( 'NONE',  ( -1.391076115485563758, 0.2306618581243848609, 0.2411417322834645549 ) ) ;
#7235=CARTESIAN_POINT ( 'NONE',  ( 8.195543980992789655E-16, -0.1870078740157480879, -0.4822834645669291653 ) ) ;
#7236=CARTESIAN_POINT ( 'NONE',  ( -0.07217847769028787330, -0.08942795157527998196, 0.3641732283464567121 ) ) ;
#7238=CARTESIAN_POINT ( 'NONE',  ( 1.384514435695538559, 0.2952755905511810774, -0.1292274648535930714 ) ) ;
#7239=CARTESIAN_POINT ( 'NONE',  ( -0.7020997375328076329, -0.3162353388693409650, -0.4822834645669289433 ) ) ;
#7240=CARTESIAN_POINT ( 'NONE',  ( 0.2486400153428833526, 3.421639014772782816E-16, 0.3464511005275203726 ) ) ;
#7241=CARTESIAN_POINT ( 'NONE',  ( 1.213910761154856299, -0.6692913385826773087, -0.1292274648535924053 ) ) ;
#7242=CARTESIAN_POINT ( 'NONE',  ( -1.646051170424378096, 0.000000000000000000, 0.3464511005275205946 ) ) ;
#7244=EDGE_CURVE ( 'NONE', #51509, #69851, #21492, .T. ) ;
#7245=EDGE_LOOP ( 'NONE', ( #17930, #40654, #64677, #18814 ) ) ;
#7246=CARTESIAN_POINT ( 'NONE',  ( 0.4199475065616805614, 0.2306618581243848609, 0.2411417322834645549 ) ) ;
#7247=CARTESIAN_POINT ( 'NONE',  ( -0.4068241469816267775, -0.004921259842519870586, -0.3153832671262229437 ) ) ;
#7248=CARTESIAN_POINT ( 'NONE',  ( 1.607611548556431069, -0.5511811023622048555, -0.09757992244046775898 ) ) ;
#7249=CARTESIAN_POINT ( 'NONE',  ( 1.614173228346457378, 0.5038684218300978346, -0.1372047244094476148 ) ) ;
#7251=CARTESIAN_POINT ( 'NONE',  ( 1.660104986876641320, -0.08942795157527998196, 0.3641732283464567121 ) ) ;
#7252=CARTESIAN_POINT ( 'NONE',  ( 1.148293963254593653, 0.2952755905511810774, -0.1292274648535930714 ) ) ;
#7254=CARTESIAN_POINT ( 'NONE',  ( 0.1902887139107617975, 0.2952755905511811885, 0.1292274648535926551 ) ) ;
#7255=CARTESIAN_POINT ( 'NONE',  ( -1.601049868766403650, 0.2306618581243847221, -0.2411417322834647770 ) ) ;
#7257=CARTESIAN_POINT ( 'NONE',  ( -1.699475065616797398, 0.2952755905511811885, 0.1292274648535926551 ) ) ;
#7258=CARTESIAN_POINT ( 'NONE',  ( 0.03937007874015806264, 0.2952755905511811885, 0.000000000000000000 ) ) ;
#7260=CARTESIAN_POINT ( 'NONE',  ( 1.640419947506562393, -0.4281496062992124485, 0.4176697321401328655 ) ) ;
#7261=CARTESIAN_POINT ( 'NONE',  ( 0.6692913385826777528, 0.2952755905511811885, 0.000000000000000000 ) ) ;
#7262=CARTESIAN_POINT ( 'NONE',  ( 0.9186351706036752773, 0.1283753931104746893, -0.1820866141732285504 ) ) ;
#7264=CARTESIAN_POINT ( 'NONE',  ( 1.030183727034121421, -0.08942795157527998196, 0.3641732283464567121 ) ) ;
#7265=CARTESIAN_POINT ( 'NONE',  ( -1.148293963254592542, 0.2952755905511811885, 0.1292274648535926551 ) ) ;
#7267=CARTESIAN_POINT ( 'NONE',  ( 1.200787401574803681, 0.1660481256975885056, 0.3530559997133364547 ) ) ;
#7269=CARTESIAN_POINT ( 'NONE',  ( 0.6758530183727039509, -0.6692913385826771977, 0.1292274648535927661 ) ) ;
#7272=CARTESIAN_POINT ( 'NONE',  ( 0.2755905511811031494, -0.5511811023622047445, 6.969142054262312111E-17 ) ) ;
#7274=CARTESIAN_POINT ( 'NONE',  ( 0.5380577427821529035, -0.4281496062992124485, 0.4176697321401328655 ) ) ;
#7276=CARTESIAN_POINT ( 'NONE',  ( -0.9580052493438311334, -0.3690944881889763329, 0.3153832671262228327 ) ) ;
#7277=CARTESIAN_POINT ( 'NONE',  ( -0.9448818897637790704, -0.1870078740157479769, 0.4822834645669291653 ) ) ;
#7278=CARTESIAN_POINT ( 'NONE',  ( 1.187664041994751285, -0.05778040916215522460, 0.4822834645669289988 ) ) ;
#7279=CARTESIAN_POINT ( 'NONE',  ( -1.574803149606298636, -0.1870078740157479769, 0.4822834645669291653 ) ) ;
#7280=CARTESIAN_POINT ( 'NONE',  ( 1.102362204724410155, -0.1870078740157480879, -0.4822834645669291653 ) ) ;
#7281=CARTESIAN_POINT ( 'NONE',  ( 1.450131233595801428, -0.6692913385826773087, -0.1292274648535924053 ) ) ;
#7283=CARTESIAN_POINT ( 'NONE',  ( 0.9514435695538062676, -0.05778040916215522460, 0.4822834645669289988 ) ) ;
#7285=CARTESIAN_POINT ( 'NONE',  ( 1.522309711286089939, 0.2306618581243848609, 0.2411417322834645549 ) ) ;
#7286=CARTESIAN_POINT ( 'NONE',  ( 1.574803149606299746, -0.1870078740157480879, -0.4822834645669291653 ) ) ;
#7287=CARTESIAN_POINT ( 'NONE',  ( -1.601049868766403650, -0.5023911411419708095, 0.1820866141732285504 ) ) ;
#7288=CARTESIAN_POINT ( 'NONE',  ( 1.102362204724410155, -0.1870078740157480601, -0.3641732283464567677 ) ) ;
#7289=CARTESIAN_POINT ( 'NONE',  ( -1.364829396325458521, -0.5023911411419708095, 0.1820866141732285504 ) ) ;
#7290=CARTESIAN_POINT ( 'NONE',  ( -0.5708661417322825615, -0.4536011799217367080, 0.2665933059059888421 ) ) ;
#7291=CARTESIAN_POINT ( 'NONE',  ( -1.377952755905511140, 0.1771653543307087630, 0.000000000000000000 ) ) ;
#7292=CARTESIAN_POINT ( 'NONE',  ( 0.7545931758530188826, -0.5511811023622046335, 0.09757992244046803654 ) ) ;
#7293=CARTESIAN_POINT ( 'NONE',  ( 0.7414698162729663755, 0.2952755905511811885, 0.1292274648535926551 ) ) ;
#7294=CARTESIAN_POINT ( 'NONE',  ( 1.030183727034121421, -0.3162353388693409650, -0.4822834645669289433 ) ) ;
#7295=CARTESIAN_POINT ( 'NONE',  ( 0.2296587926509192634, -0.3162353388693405765, 0.4822834645669290543 ) ) ;
#7296=CARTESIAN_POINT ( 'NONE',  ( 0.4199475065616803948, -0.5023911411419708095, -0.1820866141732282451 ) ) ;
#7297=CARTESIAN_POINT ( 'NONE',  ( 1.502624671916010790, -0.3162353388693409650, -0.4822834645669289433 ) ) ;
#7300=CARTESIAN_POINT ( 'NONE',  ( -0.5905511811023615998, 0.2952755905511811885, 0.000000000000000000 ) ) ;
#7302=DIRECTION ( 'NONE',  ( 0.000000000000000000, 0.000000000000000000, 1.000000000000000000 ) ) ;
#7303=CARTESIAN_POINT ( 'NONE',  ( 0.1509186351706042484, -0.3162353388693405765, 0.4822834645669290543 ) ) ;
#7304=CARTESIAN_POINT ( 'NONE',  ( -0.5118110236220466680, 0.2952755905511811885, 0.000000000000000000 ) ) ;
#7305=CARTESIAN_POINT ( 'NONE',  ( -0.1377952755905504645, 0.1660481256975885056, 0.3530559997133364547 ) ) ;
#7309=CARTESIAN_POINT ( 'NONE',  ( 0.1694133573824175565, 1.763362281772084768E-16, 0.3627985898453517377 ) ) ;
#7312=CARTESIAN_POINT ( 'NONE',  ( -0.9448818897637790704, -0.1870078740157479769, 0.3641732283464567677 ) ) ;
#7314=CARTESIAN_POINT ( 'NONE',  ( -1.286089238845143479, -0.6046776061558807314, 0.2411417322834647770 ) ) ;
#7316=CARTESIAN_POINT ( 'NONE',  ( 0.5774278215223104249, 0.2306618581243848609, 0.2411417322834645549 ) ) ;
#7317=CARTESIAN_POINT ( 'NONE',  ( 0.01312335958005323398, -0.004921259842519576551, 0.3153832671262227771 ) ) ;
#7318=CARTESIAN_POINT ( 'NONE',  ( 1.410761154855643795, -0.3162353388693405765, 0.4822834645669290543 ) ) ;
#7319=CARTESIAN_POINT ( 'NONE',  ( 0.2362204724409456558, -0.1870078740157480879, -0.4822834645669291653 ) ) ;
#7323=CARTESIAN_POINT ( 'NONE',  ( 1.345144356955381593, -0.05778040916215522460, 0.4822834645669289988 ) ) ;
#7324=CARTESIAN_POINT ( 'NONE',  ( 0.3083989501312343062, -0.3162353388693405765, 0.4822834645669290543 ) ) ;
#7325=CARTESIAN_POINT ( 'NONE',  ( 0.3477690288713918276, 0.2952755905511811885, 0.1292274648535926551 ) ) ;
#7327=CARTESIAN_POINT ( 'NONE',  ( 1.397637795275591177, 0.1660481256975883668, -0.3530559997133364547 ) ) ;
#7329=CARTESIAN_POINT ( 'NONE',  ( 0.2427821522309716595, -0.3162353388693409650, -0.4822834645669289433 ) ) ;
#7330=CARTESIAN_POINT ( 'NONE',  ( 1.161417322834646493, -0.5400638737290844871, 0.3530559997133364547 ) ) ;
#7331=CARTESIAN_POINT ( 'NONE',  ( 0.5839895013123367340, 0.2952755905511811885, 0.1292274648535926551 ) ) ;
#7332=CARTESIAN_POINT ( 'NONE',  ( 1.128608923884515169, -0.5023911411419708095, -0.1820866141732282451 ) ) ;
#7333=CARTESIAN_POINT ( 'NONE',  ( -1.043307086614172707, 0.1660481256975883668, -0.3530559997133364547 ) ) ;
#7334=CARTESIAN_POINT ( 'NONE',  ( -1.489501312335957062, -0.3162353388693409650, -0.4822834645669289433 ) ) ;
#7335=CARTESIAN_POINT ( 'NONE',  ( 0.7414698162729663755, -0.6692913385826773087, -0.1292274648535924053 ) ) ;
#7338=VERTEX_POINT ( 'NONE', #77915 ) ;
#7341=CARTESIAN_POINT ( 'NONE',  ( 1.417322834645670104, -0.1870078740157480879, -0.4822834645669291653 ) ) ;
#7342=CARTESIAN_POINT ( 'NONE',  ( 0.8989501312335963501, -0.5511811023622048555, -0.09757992244046775898 ) ) ;
#7343=CARTESIAN_POINT ( 'NONE',  ( 0.6179882174207333989, 6.425613173282222329E-18, -0.3627985898453512936 ) ) ;
#7344=CARTESIAN_POINT ( 'NONE',  ( -0.1474713956048439301, -2.191421614605370878E-15, 0.4445507791589071167 ) ) ;
#7347=CARTESIAN_POINT ( 'NONE',  ( -1.240157480314959759, -0.4536011799217368745, -0.2665933059059886201 ) ) ;
#7348=CARTESIAN_POINT ( 'NONE',  ( 1.574803149606299746, -0.1870078740157479769, 0.4822834645669291653 ) ) ;
#7349=CARTESIAN_POINT ( 'NONE',  ( -1.548556430446193399, -0.6046776061558809534, -0.2411417322834644161 ) ) ;
#7350=CARTESIAN_POINT ( 'NONE',  ( -0.3477690288713905509, -0.6692913385826771977, 0.1292274648535927661 ) ) ;
#7351=CARTESIAN_POINT ( 'NONE',  ( 1.154855643044620184, 0.2306618581243847221, -0.2411417322834647770 ) ) ;
#7353=CARTESIAN_POINT ( 'NONE',  ( -1.476377952755905110, -0.5400638737290845981, -0.3530559997133363437 ) ) ;
#7358=CARTESIAN_POINT ( 'NONE',  ( -0.7742782152230962556, -0.3690944881889765550, -0.3153832671262227771 ) ) ;
#7359=CARTESIAN_POINT ( 'NONE',  ( 0.4849061582275016602, 2.793565526369266028, 0.4921425059946345493 ) ) ;
#7360=CARTESIAN_POINT ( 'NONE',  ( 0.4265091863517067594, 0.2952755905511811885, 0.1292274648535926551 ) ) ;
#7364=CARTESIAN_POINT ( 'NONE',  ( 1.417322834645670104, -0.1870078740157480879, -0.4822834645669291653 ) ) ;
#7365=CARTESIAN_POINT ( 'NONE',  ( -1.496062992125983815, -0.1870078740157480879, -0.4822834645669291653 ) ) ;
#7367=CARTESIAN_POINT ( 'NONE',  ( -0.2296587926509179312, -0.2845877964562161244, -0.3641732283464567121 ) ) ;
#7368=CARTESIAN_POINT ( 'NONE',  ( -1.614173228346455824, 0.1771653543307087630, 0.000000000000000000 ) ) ;
#7371=CARTESIAN_POINT ( 'NONE',  ( 0.2821522309711292364, -0.6692913385826771977, 0.1292274648535927661 ) ) ;
#7372=CARTESIAN_POINT ( 'NONE',  ( -0.9383202099737524282, -0.2845877964562161244, -0.3641732283464567121 ) ) ;
#7373=CARTESIAN_POINT ( 'NONE',  ( -0.01312335958005186876, -0.3690944881889763329, 0.3153832671262228327 ) ) ;
#7374=ADVANCED_FACE ( 'NONE', ( #1728 ), #48504, .F. ) ;
#7375=CARTESIAN_POINT ( 'NONE',  ( -0.01968503937007793844, -0.5400638737290844871, 0.3530559997133364547 ) ) ;
#7376=CARTESIAN_POINT ( 'NONE',  ( -1.246719160104985846, -0.3690944881889765550, -0.3153832671262227771 ) ) ;
#7378=CARTESIAN_POINT ( 'NONE',  ( 0.7020997375328090762, -0.05778040916215560624, -0.4822834645669293319 ) ) ;
#7380=CARTESIAN_POINT ( 'NONE',  ( -1.640419947506561060, 0.05413385826771666132, 0.4176697321401328100 ) ) ;
#7382=CARTESIAN_POINT ( 'NONE',  ( -0.6824146981627291497, -0.6046776061558809534, -0.2411417322834644161 ) ) ;
#7383=CARTESIAN_POINT ( 'NONE',  ( 0.3674540682414705883, 0.1283753931104746893, -0.1820866141732285504 ) ) ;
#7384=CARTESIAN_POINT ( 'NONE',  ( -1.089238845144356427, -0.4281496062992127816, -0.4176697321401328100 ) ) ;
#7385=CARTESIAN_POINT ( 'NONE',  ( 1.010498687664042716, -0.3690944881889763329, 0.3153832671262228327 ) ) ;
#7386=AXIS2_PLACEMENT_3D ( 'NONE', #38077, #44373, #12011 ) ;
#7387=CARTESIAN_POINT ( 'NONE',  ( -0.2296587926509179312, -0.2845877964562161244, -0.3641732283464567121 ) ) ;
#7388=CARTESIAN_POINT ( 'NONE',  ( -0.5971128608923877978, 0.2952755905511811885, 0.1292274648535926551 ) ) ;
#7389=CARTESIAN_POINT ( 'NONE',  ( -1.272965879265091305, -0.4281496062992124485, 0.4176697321401328655 ) ) ;
#7390=CARTESIAN_POINT ( 'NONE',  ( -1.423884514435694859, -0.05778040916215560624, -0.4822834645669293319 ) ) ;
#7391=CARTESIAN_POINT ( 'NONE',  ( -0.6912002287759484442, 1.909921116465415958, 0.5309055118110236338 ) ) ;
#7392=CARTESIAN_POINT ( 'NONE',  ( 1.312335958005250269, -0.5023911411419708095, 0.1820866141732285504 ) ) ;
#7393=CARTESIAN_POINT ( 'NONE',  ( 0.2887139107611556010, 0.2306618581243847221, -0.2411417322834647770 ) ) ;
#7394=CARTESIAN_POINT ( 'NONE',  ( -1.640419947506561060, 0.05413385826771666132, 0.4176697321401328100 ) ) ;
#7395=CARTESIAN_POINT ( 'NONE',  ( -1.633858267716534529, -0.5400638737290845981, -0.3530559997133363437 ) ) ;
#7399=CARTESIAN_POINT ( 'NONE',  ( -0.7480314960629914633, -0.5511811023622047445, 6.969142054262312111E-17 ) ) ;
#7400=CARTESIAN_POINT ( 'NONE',  ( 0.8398950131233602345, 0.2306618581243847221, -0.2411417322834647770 ) ) ;
#7401=CARTESIAN_POINT ( 'NONE',  ( -1.017060367454067249, -0.2845877964562161244, -0.3641732283464567121 ) ) ;
#7403=CARTESIAN_POINT ( 'NONE',  ( -0.8136482939632537770, -0.6046776061558807314, 0.2411417322834647770 ) ) ;
#7404=CARTESIAN_POINT ( 'NONE',  ( 0.9645669291338591078, -0.5400638737290845981, -0.3530559997133363437 ) ) ;
#7405=CARTESIAN_POINT ( 'NONE',  ( 0.3215223097112867578, -0.3162353388693409650, -0.4822834645669289433 ) ) ;
#7407=CARTESIAN_POINT ( 'NONE',  ( 1.089238845144357537, -0.4281496062992124485, 0.4176697321401328655 ) ) ;
#7408=CARTESIAN_POINT ( 'NONE',  ( -1.410761154855642463, -0.08942795157527998196, 0.3641732283464567121 ) ) ;
#7413=CARTESIAN_POINT ( 'NONE',  ( 0.7217847769028878924, -0.004921259842519576551, 0.3153832671262227771 ) ) ;
#7414=CARTESIAN_POINT ( 'NONE',  ( 0.4199475065616803948, -0.5023911411419708095, -0.1820866141732282451 ) ) ;
#7415=CARTESIAN_POINT ( 'NONE',  ( -0.07874015748031421014, -0.1870078740157480879, -0.4822834645669291653 ) ) ;
#7416=CARTESIAN_POINT ( 'NONE',  ( 1.135170603674541256, 0.2952755905511811885, 0.1292274648535926551 ) ) ;
#7418=CARTESIAN_POINT ( 'NONE',  ( 0.3674540682414705883, -0.5023911411419708095, 0.1820866141732285504 ) ) ;
#7419=CARTESIAN_POINT ( 'NONE',  ( -0.9317585301837263412, -0.4281496062992127816, -0.4176697321401328100 ) ) ;
#7420=CARTESIAN_POINT ( 'NONE',  ( 1.574803149606299746, -0.1870078740157479769, 0.4822834645669291653 ) ) ;
#7421=CARTESIAN_POINT ( 'NONE',  ( 0.9711286089238851948, -0.6046776061558809534, -0.2411417322834644161 ) ) ;
#7423=CARTESIAN_POINT ( 'NONE',  ( 1.169516495854323379, 0.02791078216816427274, -0.4328096321851894190 ) ) ;
#7424=ORIENTED_EDGE ( 'NONE', *, *, #24704, .T. ) ;
#7426=CARTESIAN_POINT ( 'NONE',  ( -1.154855643044618851, -0.6046776061558809534, -0.2411417322834644161 ) ) ;
#7427=CARTESIAN_POINT ( 'NONE',  ( -1.187664041994749731, -0.3162353388693405765, 0.4822834645669290543 ) ) ;
#7428=CARTESIAN_POINT ( 'NONE',  ( -0.6233595800524928121, -0.2845877964562161244, -0.3641732283464567121 ) ) ;
#7429=CARTESIAN_POINT ( 'NONE',  ( -0.6167979002624665030, -0.4281496062992127816, -0.4176697321401328100 ) ) ;
#7432=CARTESIAN_POINT ( 'NONE',  ( 1.653543307086614789, -0.1870078740157479769, 0.4822834645669291653 ) ) ;
#7433=CARTESIAN_POINT ( 'NONE',  ( -1.443569553805773564, -0.6046776061558807314, 0.2411417322834647770 ) ) ;
#7434=CARTESIAN_POINT ( 'NONE',  ( 0.3740157480314966754, 0.1660481256975883668, -0.3530559997133364547 ) ) ;
#7435=CARTESIAN_POINT ( 'NONE',  ( -1.062992125984250968, -0.6692913385826771977, 8.415575281601705876E-17 ) ) ;
#7437=CARTESIAN_POINT ( 'NONE',  ( 0.4855643044619428750, 0.05413385826771666132, 0.4176697321401328100 ) ) ;
#7439=CARTESIAN_POINT ( 'NONE',  ( -0.8136482939632537770, 0.1283753931104746893, -0.1820866141732285504 ) ) ;
#7442=ORIENTED_EDGE ( 'NONE', *, *, #73660, .T. ) ;
#7445=CARTESIAN_POINT ( 'NONE',  ( -1.122047244094487306, -0.5400638737290844871, 0.3530559997133364547 ) ) ;
#7446=CARTESIAN_POINT ( 'NONE',  ( -1.417322834645668772, -0.1870078740157480879, -0.4822834645669291653 ) ) ;
#7448=CARTESIAN_POINT ( 'NONE',  ( -1.082677165354329896, 0.1660481256975885056, 0.3530559997133364547 ) ) ;
#7449=CARTESIAN_POINT ( 'NONE',  ( -1.305774278215222184, -0.6692913385826773087, -0.1292274648535924053 ) ) ;
#7450=CARTESIAN_POINT ( 'NONE',  ( -1.633858267716534529, 0.1660481256975885056, 0.3530559997133364547 ) ) ;
#7451=CARTESIAN_POINT ( 'NONE',  ( 0.9329488473419933481, 3.212806586641111164E-18, -0.3627985898453516267 ) ) ;
#7452=CARTESIAN_POINT ( 'NONE',  ( -0.8070866141732276899, 0.1660481256975883391, -0.3530559997133364547 ) ) ;
#7453=CARTESIAN_POINT ( 'NONE',  ( 0.1771653543307093182, -0.4536011799217368745, -0.2665933059059886201 ) ) ;
#7456=CARTESIAN_POINT ( 'NONE',  ( -0.4593175853018366950, -0.004921259842519576551, 0.3153832671262227771 ) ) ;
#7457=CARTESIAN_POINT ( 'NONE',  ( -0.7152230971128602510, -0.3162353388693405765, 0.4822834645669290543 ) ) ;
#7458=CARTESIAN_POINT ( 'NONE',  ( 1.122047244094488860, 0.1660481256975885056, 0.3530559997133364547 ) ) ;
#7459=CARTESIAN_POINT ( 'NONE',  ( -0.5183727034120726440, 0.2952755905511811885, 0.1292274648535926551 ) ) ;
#7461=EDGE_LOOP ( 'NONE', ( #52350, #72426, #9133 ) ) ;
#7463=CARTESIAN_POINT ( 'NONE',  ( -0.8398950131233585692, 0.2306618581243848609, 0.2411417322834645549 ) ) ;
#7464=CARTESIAN_POINT ( 'NONE',  ( 0.9514435695538062676, -0.05778040916215522460, 0.4822834645669289988 ) ) ;
#7465=CARTESIAN_POINT ( 'NONE',  ( -1.601049868766403650, -0.5023911411419708095, 0.1820866141732285504 ) ) ;
#7466=CARTESIAN_POINT ( 'NONE',  ( -1.633858267716534529, -0.5400638737290845981, -0.3530559997133363437 ) ) ;
#7472=CARTESIAN_POINT ( 'NONE',  ( -0.2034120734908128059, 0.2952755905511811885, 0.1292274648535926551 ) ) ;
#7473=CARTESIAN_POINT ( 'NONE',  ( -1.646981627296586703, -0.08942795157527998196, 0.3641732283464567121 ) ) ;
#7474=CARTESIAN_POINT ( 'NONE',  ( -0.7283464566929126471, 0.1660481256975883668, -0.3530559997133364547 ) ) ;
#7476=CARTESIAN_POINT ( 'NONE',  ( -1.089238845144356427, 0.05413385826771666132, 0.4176697321401328100 ) ) ;
#7479=CARTESIAN_POINT ( 'NONE',  ( -1.135170603674539924, -0.6692913385826771977, 0.1292274648535927661 ) ) ;
#7480=CARTESIAN_POINT ( 'NONE',  ( -0.5249343832020990641, -0.6046776061558809534, -0.2411417322834644161 ) ) ;
#7482=CARTESIAN_POINT ( 'NONE',  ( 0.9055118110236227702, -0.5511811023622047445, 6.969142054262312111E-17 ) ) ;
#7484=CARTESIAN_POINT ( 'NONE',  ( 0.5577427821522316087, -0.08942795157527998196, 0.3641732283464567121 ) ) ;
#7485=CARTESIAN_POINT ( 'NONE',  ( 1.338582677165355062, -0.1870078740157480601, -0.3641732283464567677 ) ) ;
#7486=CARTESIAN_POINT ( 'NONE',  ( 1.174540682414699111, -0.05778040916215560624, -0.4822834645669293319 ) ) ;
#7488=CARTESIAN_POINT ( 'NONE',  ( 0.03280839895013198948, -0.5511811023622048555, -0.09757992244046775898 ) ) ;
#7490=CARTESIAN_POINT ( 'NONE',  ( -1.397637795275589623, -0.5400638737290845981, -0.3530559997133363437 ) ) ;
#7491=CARTESIAN_POINT ( 'NONE',  ( 1.404199475065617264, -0.4281496062992124485, 0.4176697321401328655 ) ) ;
#7494=CARTESIAN_POINT ( 'NONE',  ( -0.4658792650918627265, -0.2845877964562161244, -0.3641732283464567121 ) ) ;
#7496=CARTESIAN_POINT ( 'NONE',  ( 0.2362204724409456558, -0.1870078740157479769, 0.4822834645669291653 ) ) ;
#7497=CARTESIAN_POINT ( 'NONE',  ( -0.6423408027444563739, -2.609869883881465018E-15, -0.3464511005275220379 ) ) ;
#7498=CARTESIAN_POINT ( 'NONE',  ( 0.8005249343832027131, -0.004921259842519576551, 0.3153832671262227771 ) ) ;
#7499=CARTESIAN_POINT ( 'NONE',  ( 0.1181102362204730916, -0.5511811023622047445, 6.969142054262312111E-17 ) ) ;
#7500=CARTESIAN_POINT ( 'NONE',  ( -0.4658792650918627265, -0.3162353388693409650, -0.4822834645669289433 ) ) ;
#7501=CARTESIAN_POINT ( 'NONE',  ( -1.213910761154854745, 0.2952755905511810774, -0.1292274648535930714 ) ) ;
#7502=CARTESIAN_POINT ( 'NONE',  ( -0.6299212598425188991, -0.1870078740157480601, -0.3641732283464567677 ) ) ;
#7503=DIRECTION ( 'NONE',  ( 0.000000000000000000, -0.000000000000000000, 1.000000000000000000 ) ) ;
#7504=CARTESIAN_POINT ( 'NONE',  ( 0.4593175853018380828, 0.05413385826771626580, -0.4176697321401330321 ) ) ;
#7505=CARTESIAN_POINT ( 'NONE',  ( -0.8530183727034112984, 0.05413385826771666132, 0.4176697321401328100 ) ) ;
#7508=CARTESIAN_POINT ( 'NONE',  ( 0.1181102362204730916, -0.5511811023622047445, 6.969142054262312111E-17 ) ) ;
#7509=CARTESIAN_POINT ( 'NONE',  ( -0.7808398950131222316, -0.3162353388693409650, -0.4822834645669289433 ) ) ;
#7511=CARTESIAN_POINT ( 'NONE',  ( -0.9842519685039360366, 0.2952755905511811885, 0.000000000000000000 ) ) ;
#7512=CARTESIAN_POINT ( 'NONE',  ( -1.246719160104985846, -0.3690944881889765550, -0.3153832671262227771 ) ) ;
#7513=CARTESIAN_POINT ( 'NONE',  ( 1.587926509186352586, -0.4281496062992127816, -0.4176697321401328100 ) ) ;
#7514=CARTESIAN_POINT ( 'NONE',  ( -0.9055118110236215490, -0.5511811023622047445, 6.969142054262312111E-17 ) ) ;
#7516=CARTESIAN_POINT ( 'NONE',  ( 1.496062992125984703, -0.1870078740157480879, -0.4822834645669291653 ) ) ;
#7521=CARTESIAN_POINT ( 'NONE',  ( -1.653543307086613234, -0.1870078740157480879, -0.4822834645669291653 ) ) ;
#7522=CARTESIAN_POINT ( 'NONE',  ( -1.266404199475064773, -0.3162353388693405765, 0.4822834645669290543 ) ) ;
#7523=CARTESIAN_POINT ( 'NONE',  ( 1.108923884514436242, -0.05778040916215522460, 0.4822834645669289988 ) ) ;
#7526=CARTESIAN_POINT ( 'NONE',  ( 0.4724409448818904789, -0.1870078740157480879, -0.4822834645669291653 ) ) ;
#7527=CARTESIAN_POINT ( 'NONE',  ( -0.1181102362204717315, -0.6692913385826771977, 8.415575281601705876E-17 ) ) ;
#7530=CARTESIAN_POINT ( 'NONE',  ( 0.7152230971128614723, -0.2845877964562161244, -0.3641732283464567121 ) ) ;
#7536=CARTESIAN_POINT ( 'NONE',  ( 0.08530183727034192087, -0.3162353388693409650, -0.4822834645669289433 ) ) ;
#7537=CARTESIAN_POINT ( 'NONE',  ( 1.391076115485564868, -0.6046776061558807314, 0.2411417322834647770 ) ) ;
#7538=CARTESIAN_POINT ( 'NONE',  ( 0.8005249343832028242, -0.4281496062992127816, -0.4176697321401328100 ) ) ;
#7539=CARTESIAN_POINT ( 'NONE',  ( 1.141732283464567788, -0.6692913385826771977, 8.415575281601705876E-17 ) ) ;
#7540=EDGE_CURVE ( 'NONE', #3606, #39084, #61449, .T. ) ;
#7541=CARTESIAN_POINT ( 'NONE',  ( -0.3674540682414689785, 0.2306618581243848609, 0.2411417322834645549 ) ) ;
#7542=CARTESIAN_POINT ( 'NONE',  ( -0.09842519685039295696, 0.1660481256975883668, -0.3530559997133364547 ) ) ;
#7543=CARTESIAN_POINT ( 'NONE',  ( 1.601049868766404982, 0.2306618581243848609, 0.2411417322834645549 ) ) ;
#7544=CARTESIAN_POINT ( 'NONE',  ( 1.305774278215223960, 0.2952755905511810774, -0.1292274648535930714 ) ) ;
#7545=CARTESIAN_POINT ( 'NONE',  ( 1.233595800524935227, 0.2306618581243847221, -0.2411417322834647770 ) ) ;
#7547=CARTESIAN_POINT ( 'NONE',  ( 0.4790026246719168435, -0.2845877964562161244, -0.3641732283464567121 ) ) ;
#7548=ORIENTED_EDGE ( 'NONE', *, *, #29541, .T. ) ;
#7551=EDGE_LOOP ( 'NONE', ( #79618, #48716, #45301, #46126 ) ) ;
#7552=CARTESIAN_POINT ( 'NONE',  ( -0.3149606299212590610, -0.1870078740157479769, 0.3641732283464567677 ) ) ;
#7554=CARTESIAN_POINT ( 'NONE',  ( -0.1771653543307080136, 0.1660481256975883668, -0.3530559997133364547 ) ) ;
#7556=CARTESIAN_POINT ( 'NONE',  ( 0.2952755905511816326, -0.5400638737290844871, 0.3530559997133364547 ) ) ;
#7557=CARTESIAN_POINT ( 'NONE',  ( 0.06561679790026316017, 0.05413385826771626580, -0.4176697321401330321 ) ) ;
#7558=CARTESIAN_POINT ( 'NONE',  ( -0.6692913385826764205, 0.2952755905511811885, 0.000000000000000000 ) ) ;
#7559=CARTESIAN_POINT ( 'NONE',  ( -1.141732283464566011, -0.6692913385826771977, 8.415575281601705876E-17 ) ) ;
#7560=CARTESIAN_POINT ( 'NONE',  ( 1.345144356955381593, -0.08942795157527998196, 0.3641732283464567121 ) ) ;
#7561=CARTESIAN_POINT ( 'NONE',  ( 1.586052503253845503, 0.4724409448818907564, 0.1653254495020587411 ) ) ;
#7563=CARTESIAN_POINT ( 'NONE',  ( 0.9448818897637802916, -0.1870078740157479769, 0.3641732283464567677 ) ) ;
#7564=CARTESIAN_POINT ( 'NONE',  ( 0.4002624671916016896, -0.05778040916215522460, 0.4822834645669289988 ) ) ;
#7565=CARTESIAN_POINT ( 'NONE',  ( 0.6692913385826778638, -0.6692913385826771977, 8.415575281601705876E-17 ) ) ;
#7567=DIRECTION ( 'NONE',  ( -0.000000000000000000, -1.000000000000000000, -0.000000000000000000 ) ) ;
#7570=CARTESIAN_POINT ( 'NONE',  ( -0.4724409448818890911, -0.1870078740157479769, 0.4822834645669291653 ) ) ;
#7573=CARTESIAN_POINT ( 'NONE',  ( -1.030183727034119867, -0.2845877964562159024, 0.3641732283464567677 ) ) ;
#7574=CARTESIAN_POINT ( 'NONE',  ( 1.272965879265092637, 0.05413385826771666132, 0.4176697321401328100 ) ) ;
#7575=VECTOR ( 'NONE', #5793, 39.37007874015748143 ) ;
#7576=CARTESIAN_POINT ( 'NONE',  ( 0.8661417322834653598, -0.1870078740157479769, 0.4822834645669291653 ) ) ;
#7577=CARTESIAN_POINT ( 'NONE',  ( -0.2362204724409440182, -0.1870078740157479769, 0.3641732283464567677 ) ) ;
#7578=CARTESIAN_POINT ( 'NONE',  ( 0.4002624671916016896, -0.3162353388693409650, -0.4822834645669289433 ) ) ;
#7580=CARTESIAN_POINT ( 'NONE',  ( 0.2493438320209980519, -0.004921259842519576551, 0.3153832671262227771 ) ) ;
#7581=CARTESIAN_POINT ( 'NONE',  ( 0.1246719160104994284, -0.6692913385826771977, 0.1292274648535927661 ) ) ;
#7583=CARTESIAN_POINT ( 'NONE',  ( -1.115485564304461219, -0.4281496062992124485, 0.4176697321401328655 ) ) ;
#7584=CARTESIAN_POINT ( 'NONE',  ( 0.3477690288713918276, 0.1771653543307087630, 0.09757992244046791164 ) ) ;
#7585=CARTESIAN_POINT ( 'NONE',  ( -1.169516495854322269, 0.02791078216816064370, 0.4328096321851915285 ) ) ;
#7586=CARTESIAN_POINT ( 'NONE',  ( -0.8792650918635160906, 0.05413385826771626580, -0.4176697321401330321 ) ) ;
#7587=CARTESIAN_POINT ( 'NONE',  ( -0.4658792650918627265, -0.2845877964562161244, -0.3641732283464567121 ) ) ;
#7588=CARTESIAN_POINT ( 'NONE',  ( -1.473278426072734293, 0.2335363939278408130, 0.2780995266831702284 ) ) ;
#7589=CARTESIAN_POINT ( 'NONE',  ( -0.8136482939632537770, -0.6046776061558807314, 0.2411417322834647770 ) ) ;
#7590=CARTESIAN_POINT ( 'NONE',  ( -0.7545931758530176614, -0.6692913385826773087, -0.1292274648535924053 ) ) ;
#7591=CARTESIAN_POINT ( 'NONE',  ( 0.4855643044619428750, -0.004921259842519576551, 0.3153832671262227771 ) ) ;
#7593=CARTESIAN_POINT ( 'NONE',  ( -0.05249343832020911260, 0.2306618581243848609, 0.2411417322834645549 ) ) ;
#7595=CARTESIAN_POINT ( 'NONE',  ( -1.607611548556429737, -0.5511811023622046335, 0.09757992244046803654 ) ) ;
#7596=CARTESIAN_POINT ( 'NONE',  ( 0.8136482939632553313, -0.5023911411419708095, -0.1820866141732282451 ) ) ;
#7597=CARTESIAN_POINT ( 'NONE',  ( 1.587926509186352142, 0.05413385826771666132, 0.4176697321401328100 ) ) ;
#7598=CARTESIAN_POINT ( 'NONE',  ( -0.8727034120734901146, -0.08942795157528024563, -0.3641732283464568787 ) ) ;
#7599=CARTESIAN_POINT ( 'NONE',  ( -0.9776902887139098386, -0.5511811023622046335, 0.09757992244046803654 ) ) ;
#7600=CARTESIAN_POINT ( 'NONE',  ( -0.6430446194225712953, 0.05413385826771626580, -0.4176697321401330321 ) ) ;
#7601=CARTESIAN_POINT ( 'NONE',  ( -0.03280839895013062252, -0.6692913385826771977, 0.1292274648535927661 ) ) ;
#7602=CARTESIAN_POINT ( 'NONE',  ( 0.4986876640419954376, -0.5023911411419708095, -0.1820866141732282451 ) ) ;
#7604=CARTESIAN_POINT ( 'NONE',  ( 0.8727034120734912248, -0.2845877964562161244, -0.3641732283464567121 ) ) ;
#7605=CARTESIAN_POINT ( 'NONE',  ( 0.3346456692913393205, -0.5400638737290845981, -0.3530559997133363437 ) ) ;
#7606=FACE_OUTER_BOUND ( 'NONE', #4750, .T. ) ;
#7607=CARTESIAN_POINT ( 'NONE',  ( -0.7611548556430438595, 0.2306618581243848609, 0.2411417322834645549 ) ) ;
#7610=CARTESIAN_POINT ( 'NONE',  ( 1.437007874015748810, 0.07958543189024085140, 0.2665933059059887866 ) ) ;
#7612=CARTESIAN_POINT ( 'NONE',  ( 0.5577427821522316087, -0.05778040916215522460, 0.4822834645669289988 ) ) ;
#7614=CARTESIAN_POINT ( 'NONE',  ( 0.1049868766404206816, 0.2306618581243848609, 0.2411417322834645549 ) ) ;
#7616=CARTESIAN_POINT ( 'NONE',  ( -0.1509186351706028884, -0.2845877964562161244, -0.3641732283464567121 ) ) ;
#7617=CARTESIAN_POINT ( 'NONE',  ( 0.7283464566929143125, 0.1660481256975885056, 0.3530559997133364547 ) ) ;
#7618=CARTESIAN_POINT ( 'NONE',  ( -0.7152230971128602510, -0.08942795157528024563, -0.3641732283464568787 ) ) ;
#7619=CARTESIAN_POINT ( 'NONE',  ( -0.6889763779527552368, 0.1660481256975885056, 0.3530559997133364547 ) ) ;
#7621=CARTESIAN_POINT ( 'NONE',  ( -0.1115485564304456306, 0.2952755905511810774, -0.1292274648535930714 ) ) ;
#7623=CARTESIAN_POINT ( 'NONE',  ( -1.266404199475064773, -0.05778040916215560624, -0.4822834645669293319 ) ) ;
#7624=CARTESIAN_POINT ( 'NONE',  ( -1.220472440944881054, 0.1771653543307087630, 0.000000000000000000 ) ) ;
#7625=CARTESIAN_POINT ( 'NONE',  ( -0.1312335958005241554, 0.2306618581243848609, 0.2411417322834645549 ) ) ;
#7627=CARTESIAN_POINT ( 'NONE',  ( -0.8464566929133852113, 0.1660481256975885056, 0.3530559997133364547 ) ) ;
#7630=CARTESIAN_POINT ( 'NONE',  ( -0.9120734908136473029, 0.2952755905511811885, 0.1292274648535926551 ) ) ;
#7631=CARTESIAN_POINT ( 'NONE',  ( 1.122047244094488860, 0.1660481256975885056, 0.3530559997133364547 ) ) ;
#7632=CARTESIAN_POINT ( 'NONE',  ( 1.417322834645670104, -0.1870078740157480879, -0.4822834645669291653 ) ) ;
#7634=FACE_OUTER_BOUND ( 'NONE', #38153, .T. ) ;
#7635=CARTESIAN_POINT ( 'NONE',  ( -1.141732283464566011, -0.6692913385826771977, 8.415575281601705876E-17 ) ) ;
#7640=CARTESIAN_POINT ( 'NONE',  ( -0.07217847769028787330, -0.08942795157527998196, 0.3641732283464567121 ) ) ;
#7643=CARTESIAN_POINT ( 'NONE',  ( 0.07217847769028949700, -0.05778040916215560624, -0.4822834645669293319 ) ) ;
#7644=CARTESIAN_POINT ( 'NONE',  ( 0.1049868766404206816, -0.6046776061558809534, -0.2411417322834644161 ) ) ;
#7645=CARTESIAN_POINT ( 'NONE',  ( -0.5118110236220466680, 0.2952755905511811885, 0.000000000000000000 ) ) ;
#7647=CARTESIAN_POINT ( 'NONE',  ( -0.8595800524934373854, -0.08942795157527998196, 0.3641732283464567121 ) ) ;
#7649=CARTESIAN_POINT ( 'NONE',  ( 0.7874015748031503170, -0.1870078740157480879, -0.4822834645669291653 ) ) ;
#7650=CARTESIAN_POINT ( 'NONE',  ( 0.6496062992125991586, 0.07958543189024085140, 0.2665933059059887866 ) ) ;
#7651=CARTESIAN_POINT ( 'NONE',  ( -0.2887139107611542133, -0.6046776061558809534, -0.2411417322834644161 ) ) ;
#7653=CARTESIAN_POINT ( 'NONE',  ( -0.8792650918635160906, -0.4281496062992124485, 0.4176697321401328655 ) ) ;
#7654=CARTESIAN_POINT ( 'NONE',  ( -1.541994750656167090, 0.1771653543307087630, 0.09757992244046791164 ) ) ;
#7655=CARTESIAN_POINT ( 'NONE',  ( 1.351706036745407680, 0.05413385826771666132, 0.4176697321401328100 ) ) ;
#7659=CARTESIAN_POINT ( 'NONE',  ( 0.08530183727034192087, -0.05778040916215522460, 0.4822834645669289988 ) ) ;
#7661=CARTESIAN_POINT ( 'NONE',  ( -0.7742782152230965886, 0.05413385826771666132, 0.4176697321401328100 ) ) ;
#7662=CARTESIAN_POINT ( 'NONE',  ( 1.568241469816273437, -0.3162353388693405765, 0.4822834645669290543 ) ) ;
#7663=CARTESIAN_POINT ( 'NONE',  ( 1.345144356955381593, -0.3162353388693409650, -0.4822834645669289433 ) ) ;
#7664=CARTESIAN_POINT ( 'NONE',  ( 0.2690288713910767848, -0.6692913385826773087, -0.1292274648535924053 ) ) ;
#7665=CARTESIAN_POINT ( 'NONE',  ( -0.2099737532808391705, 0.2306618581243848609, 0.2411417322834645549 ) ) ;
#7667=CARTESIAN_POINT ( 'NONE',  ( -1.102362204724408601, -0.1870078740157479769, 0.4822834645669291653 ) ) ;
#7668=CARTESIAN_POINT ( 'NONE',  ( -0.2296587926509179312, -0.05778040916215522460, 0.4822834645669289988 ) ) ;
#7669=CARTESIAN_POINT ( 'NONE',  ( -0.05249343832020911260, 0.1283753931104748280, 0.1820866141732283561 ) ) ;
#7670=DIRECTION ( 'NONE',  ( -0.000000000000000000, -1.000000000000000000, 0.000000000000000000 ) ) ;
#7671=CARTESIAN_POINT ( 'NONE',  ( -0.3543307086614165824, -0.6692913385826771977, 8.415575281601705876E-17 ) ) ;
#7672=CARTESIAN_POINT ( 'NONE',  ( 1.148293963254593653, 0.2952755905511810774, -0.1292274648535930714 ) ) ;
#7673=DIRECTION ( 'NONE',  ( -1.000000000000000000, -3.083952846180990774E-16, 0.000000000000000000 ) ) ;
#7674=ORIENTED_EDGE ( 'NONE', *, *, #34817, .T. ) ;
#7676=CARTESIAN_POINT ( 'NONE',  ( -0.07217847769028787330, -0.05778040916215522460, 0.4822834645669289988 ) ) ;
#7677=CARTESIAN_POINT ( 'NONE',  ( -0.09186351706036689768, -0.004921259842519870586, -0.3153832671262229437 ) ) ;
#7679=CIRCLE ( 'NONE', #68116, 3.543307086614173596 ) ;
#7680=CARTESIAN_POINT ( 'NONE',  ( 0.9973753280839902091, -0.5023911411419708095, 0.1820866141732285504 ) ) ;
#7681=CARTESIAN_POINT ( 'NONE',  ( -1.436417322834643739, 0.8346805926620878280, -0.3149606299212598381 ) ) ;
#7684=CARTESIAN_POINT ( 'NONE',  ( 1.174540682414699111, -0.05778040916215560624, -0.4822834645669293319 ) ) ;
#7687=CARTESIAN_POINT ( 'NONE',  ( -0.05905511811023545637, -0.5400638737290845981, -0.3530559997133363437 ) ) ;
#7689=CARTESIAN_POINT ( 'NONE',  ( -1.423884514435694859, -0.3162353388693405765, 0.4822834645669290543 ) ) ;
#7690=CARTESIAN_POINT ( 'NONE',  ( -0.1509186351706028884, -0.05778040916215522460, 0.4822834645669289988 ) ) ;
#7692=CARTESIAN_POINT ( 'NONE',  ( -1.515748031496062076, -0.4536011799217367080, 0.2665933059059888421 ) ) ;
#7693=CARTESIAN_POINT ( 'NONE',  ( 0.5577427821522314977, -0.3162353388693409650, -0.4822834645669289433 ) ) ;
#7694=CARTESIAN_POINT ( 'NONE',  ( 1.108923884514436686, -0.2845877964562161244, -0.3641732283464567121 ) ) ;
#7695=DIRECTION ( 'NONE',  ( -0.000000000000000000, 1.000000000000000000, -0.000000000000000000 ) ) ;
#7696=CARTESIAN_POINT ( 'NONE',  ( 0.2165354330708668673, -0.4536011799217367080, 0.2665933059059888421 ) ) ;
#7697=CARTESIAN_POINT ( 'NONE',  ( -1.371391076115484609, -0.6692913385826771977, 0.1292274648535927661 ) ) ;
#7699=CARTESIAN_POINT ( 'NONE',  ( 0.9842519685039378130, -0.6692913385826771977, 8.415575281601705876E-17 ) ) ;
#7701=CARTESIAN_POINT ( 'NONE',  ( 0.6692913385826778638, -0.6692913385826771977, 8.415575281601705876E-17 ) ) ;
#7704=CARTESIAN_POINT ( 'NONE',  ( 0.2559055118110243332, -0.4536011799217368745, -0.2665933059059886201 ) ) ;
#7705=CARTESIAN_POINT ( 'NONE',  ( 0.6299212598425204535, -0.1870078740157480879, -0.4822834645669291653 ) ) ;
#7707=CARTESIAN_POINT ( 'NONE',  ( -0.7742782152230965886, -0.004921259842519576551, 0.3153832671262227771 ) ) ;
#7708=CARTESIAN_POINT ( 'NONE',  ( -0.8792650918635160906, 0.05413385826771626580, -0.4176697321401330321 ) ) ;
#7709=CARTESIAN_POINT ( 'NONE',  ( -1.509186351706035767, 0.05413385826771626580, -0.4176697321401330321 ) ) ;
#7710=CARTESIAN_POINT ( 'NONE',  ( 0.8989501312335964611, 0.2952755905511811885, 0.1292274648535926551 ) ) ;
#7711=CARTESIAN_POINT ( 'NONE',  ( 1.568241469816273659, -0.05778040916215560624, -0.4822834645669293319 ) ) ;
#7713=CARTESIAN_POINT ( 'NONE',  ( 0.7611548556430451917, -0.6046776061558807314, 0.2411417322834647770 ) ) ;
#7715=CARTESIAN_POINT ( 'NONE',  ( 1.653543307086614789, -0.1870078740157479769, 0.4822834645669291653 ) ) ;
#7716=CARTESIAN_POINT ( 'NONE',  ( 1.332020997375329197, -0.3162353388693405765, 0.4822834645669290543 ) ) ;
#7717=CARTESIAN_POINT ( 'NONE',  ( -1.240157480314959759, 0.07958543189024085140, 0.2665933059059887866 ) ) ;
#7718=CARTESIAN_POINT ( 'NONE',  ( 1.410761154855643795, -0.08942795157528024563, -0.3641732283464568787 ) ) ;
#7719=CARTESIAN_POINT ( 'NONE',  ( -1.128608923884513837, 0.1283753931104746893, -0.1820866141732285504 ) ) ;
#7720=CARTESIAN_POINT ( 'NONE',  ( -0.3871391076115476282, -0.08942795157527998196, 0.3641732283464567121 ) ) ;
#7722=CARTESIAN_POINT ( 'NONE',  ( 0.9251968503937015864, -0.4536011799217367080, 0.2665933059059888421 ) ) ;
#7723=CARTESIAN_POINT ( 'NONE',  ( 0.7349081364829403995, 0.2306618581243848609, 0.2411417322834645549 ) ) ;
#7724=CARTESIAN_POINT ( 'NONE',  ( 1.128608923884514947, 0.2306618581243848609, 0.2411417322834645549 ) ) ;
#7725=CARTESIAN_POINT ( 'NONE',  ( 0.01312335958005323398, -0.4281496062992127816, -0.4176697321401328100 ) ) ;
#7726=CARTESIAN_POINT ( 'NONE',  ( 0.6627296587926515548, 0.1771653543307087630, 0.09757992244046791164 ) ) ;
#7727=CARTESIAN_POINT ( 'NONE',  ( 1.056430446194226436, -0.6692913385826773087, -0.1292274648535924053 ) ) ;
#7728=ADVANCED_FACE ( 'NONE', ( #15610 ), #81236, .F. ) ;
#7729=CARTESIAN_POINT ( 'NONE',  ( -1.587926509186350810, 0.05413385826771626580, -0.4176697321401330321 ) ) ;
#7730=CARTESIAN_POINT ( 'NONE',  ( -0.6955380577427815458, -0.4281496062992127816, -0.4176697321401328100 ) ) ;
#7734=CARTESIAN_POINT ( 'NONE',  ( 0.01968503937007930540, 0.1660481256975885056, 0.3530559997133364547 ) ) ;
#7736=CARTESIAN_POINT ( 'NONE',  ( -0.2165354330708654795, 0.1660481256975885056, 0.3530559997133364547 ) ) ;
#7737=CARTESIAN_POINT ( 'NONE',  ( -0.08530183727034056085, -0.05778040916215560624, -0.4822834645669293319 ) ) ;
#7743=CARTESIAN_POINT ( 'NONE',  ( -0.9317585301837263412, -0.004921259842519576551, 0.3153832671262227771 ) ) ;
#7745=CARTESIAN_POINT ( 'NONE',  ( -0.9908136482939626788, -0.6692913385826773087, -0.1292274648535924053 ) ) ;
#7747=CARTESIAN_POINT ( 'NONE',  ( 0.6233595800524942554, -0.05778040916215560624, -0.4822834645669293319 ) ) ;
#7748=CARTESIAN_POINT ( 'NONE',  ( -0.6627296587926503335, -0.5511811023622046335, 0.09757992244046803654 ) ) ;
#7749=CARTESIAN_POINT ( 'NONE',  ( 1.200787401574803681, -0.5400638737290845981, -0.3530559997133363437 ) ) ;
#7750=CARTESIAN_POINT ( 'NONE',  ( 0.3412073490813655186, 0.2306618581243848609, 0.2411417322834645549 ) ) ;
#7754=CARTESIAN_POINT ( 'NONE',  ( 1.200787401574803681, 0.1660481256975885056, 0.3530559997133364547 ) ) ;
#7755=CARTESIAN_POINT ( 'NONE',  ( 0.6167979002624678353, -0.4281496062992124485, 0.4176697321401328655 ) ) ;
#7756=CARTESIAN_POINT ( 'NONE',  ( 0.3608923884514443348, 0.2952755905511810774, -0.1292274648535930714 ) ) ;
#7757=CARTESIAN_POINT ( 'NONE',  ( -1.594488188976377119, 0.1660481256975883668, -0.3530559997133364547 ) ) ;
#7758=CARTESIAN_POINT ( 'NONE',  ( 0.8005249343832028242, -0.4281496062992127816, -0.4176697321401328100 ) ) ;
#7760=CARTESIAN_POINT ( 'NONE',  ( 0.2624671916010504757, -0.6046776061558809534, -0.2411417322834644161 ) ) ;
#7761=CARTESIAN_POINT ( 'NONE',  ( 0.8989501312335964611, 0.2952755905511811885, 0.1292274648535926551 ) ) ;
#7762=CARTESIAN_POINT ( 'NONE',  ( 0.4461942257217856311, 0.2306618581243847221, -0.2411417322834647770 ) ) ;
#7763=CARTESIAN_POINT ( 'NONE',  ( 0.9448818897637802916, -0.1870078740157480601, -0.3641732283464567677 ) ) ;
#7764=CARTESIAN_POINT ( 'NONE',  ( -0.7349081364829390672, 0.2306618581243847221, -0.2411417322834647770 ) ) ;
#7765=CARTESIAN_POINT ( 'NONE',  ( -1.404199475065615932, 0.05413385826771666132, 0.4176697321401328100 ) ) ;
#7766=CARTESIAN_POINT ( 'NONE',  ( 0.8792650918635177559, -0.4281496062992127816, -0.4176697321401328100 ) ) ;
#7769=ORIENTED_EDGE ( 'NONE', *, *, #56823, .F. ) ;
#7773=CARTESIAN_POINT ( 'NONE',  ( 0.7808398950131240079, -0.2845877964562159024, 0.3641732283464567677 ) ) ;
#7774=CARTESIAN_POINT ( 'NONE',  ( 0.5627669687126071185, 0.02791078216816386681, 0.4328096321851896966 ) ) ;
#7777=CARTESIAN_POINT ( 'NONE',  ( 1.463254593175853824, 0.2952755905511810774, -0.1292274648535930714 ) ) ;
#7778=CARTESIAN_POINT ( 'NONE',  ( 1.036041590146032698, 3.421639014772782816E-16, 0.3464511005275203726 ) ) ;
#7779=CARTESIAN_POINT ( 'NONE',  ( -0.3149606299212590610, -0.1870078740157479769, 0.4822834645669291653 ) ) ;
#7780=CARTESIAN_POINT ( 'NONE',  ( 1.049868766404200127, -0.6046776061558809534, -0.2411417322834644161 ) ) ;
#7782=CARTESIAN_POINT ( 'NONE',  ( -1.679790026246718693, 0.2306618581243847221, -0.2411417322834647770 ) ) ;
#7787=CARTESIAN_POINT ( 'NONE',  ( -0.9842519685039360366, 0.1771653543307087630, 0.000000000000000000 ) ) ;
#7788=CARTESIAN_POINT ( 'NONE',  ( 0.9055118110236227702, 0.2066929133858268208, 0.000000000000000000 ) ) ;
#7789=CARTESIAN_POINT ( 'NONE',  ( 0.6299212598425204535, -0.1870078740157480879, -0.4822834645669291653 ) ) ;
#7792=CARTESIAN_POINT ( 'NONE',  ( 0.2262115530851599166, 8.471767977567108961E-16, -0.4445507791589058955 ) ) ;
#7794=CARTESIAN_POINT ( 'NONE',  ( 0.8858267716535438430, 0.1660481256975885056, 0.3530559997133364547 ) ) ;
#7795=CARTESIAN_POINT ( 'NONE',  ( -1.719160104986876103, 0.05413385826771666132, 0.4176697321401328100 ) ) ;
#7797=CARTESIAN_POINT ( 'NONE',  ( -0.7480314960629914633, 0.1771653543307087630, 0.000000000000000000 ) ) ;
#7799=CARTESIAN_POINT ( 'NONE',  ( 1.673228346456693494, 0.1660481256975885056, 0.3530559997133364547 ) ) ;
#7801=CARTESIAN_POINT ( 'NONE',  ( 0.2690288713910767848, -0.6692913385826773087, -0.1292274648535924053 ) ) ;
#7802=CARTESIAN_POINT ( 'NONE',  ( -1.062992125984250968, -0.5511811023622047445, 6.969142054262312111E-17 ) ) ;
#7803=CARTESIAN_POINT ( 'NONE',  ( 0.1377952755905518800, -0.4536011799217367080, 0.2665933059059888421 ) ) ;
#7804=CARTESIAN_POINT ( 'NONE',  ( -0.4199475065616791736, 0.2306618581243847221, -0.2411417322834647770 ) ) ;
#7805=CARTESIAN_POINT ( 'NONE',  ( -1.312335958005248715, 0.1283753931104748280, 0.1820866141732283561 ) ) ;
#7807=CARTESIAN_POINT ( 'NONE',  ( 0.6561679790026253567, 0.2306618581243848609, 0.2411417322834645549 ) ) ;
#7808=CARTESIAN_POINT ( 'NONE',  ( -1.607611548556429737, 0.2952755905511810774, -0.1292274648535930714 ) ) ;
#7810=CARTESIAN_POINT ( 'NONE',  ( -0.7349081364829390672, 0.2306618581243847221, -0.2411417322834647770 ) ) ;
#7811=CARTESIAN_POINT ( 'NONE',  ( 5.463695987328526437E-16, -0.1870078740157479769, 0.3641732283464567677 ) ) ;
#7812=CARTESIAN_POINT ( 'NONE',  ( -1.161417322834644716, 0.1660481256975885056, 0.3530559997133364547 ) ) ;
#7813=CARTESIAN_POINT ( 'NONE',  ( 0.9120734908136490793, 0.1771653543307087075, -0.09757992244046823083 ) ) ;
#7814=CARTESIAN_POINT ( 'NONE',  ( -0.6364829396325453192, -0.2845877964562159024, 0.3641732283464567677 ) ) ;
#7815=CARTESIAN_POINT ( 'NONE',  ( -0.8923884514435688198, 0.2306618581243847221, -0.2411417322834647770 ) ) ;
#7816=CARTESIAN_POINT ( 'NONE',  ( -1.023622047244094002, -0.1870078740157480879, -0.4822834645669291653 ) ) ;
#7817=CARTESIAN_POINT ( 'NONE',  ( 1.653543307086614789, -0.1870078740157479769, 0.4822834645669291653 ) ) ;
#7819=CARTESIAN_POINT ( 'NONE',  ( 1.030183727034121421, -0.08942795157527998196, 0.3641732283464567121 ) ) ;
#7820=CARTESIAN_POINT ( 'NONE',  ( 0.3543307086614181922, -0.6692913385826771977, 8.415575281601705876E-17 ) ) ;
#7821=CARTESIAN_POINT ( 'NONE',  ( -1.417322834645668772, -0.1870078740157480879, -0.4822834645669291653 ) ) ;
#7822=CARTESIAN_POINT ( 'NONE',  ( -1.614173228346456268, -0.6692913385826771977, 8.415575281601705876E-17 ) ) ;
#7823=ORIENTED_EDGE ( 'NONE', *, *, #67121, .F. ) ;
#7825=CARTESIAN_POINT ( 'NONE',  ( -1.417322834645668772, -0.1870078740157480601, -0.3641732283464567677 ) ) ;
#7826=CARTESIAN_POINT ( 'NONE',  ( 0.5577427821522314977, -0.3162353388693409650, -0.4822834645669289433 ) ) ;
#7827=CARTESIAN_POINT ( 'NONE',  ( -1.030183727034119867, -0.08942795157528024563, -0.3641732283464568787 ) ) ;
#7829=CARTESIAN_POINT ( 'NONE',  ( -1.555118110236219930, 0.1660481256975885056, 0.3530559997133364547 ) ) ;
#7830=CARTESIAN_POINT ( 'NONE',  ( 0.9514435695538062676, -0.3162353388693409650, -0.4822834645669289433 ) ) ;
#7831=CARTESIAN_POINT ( 'NONE',  ( 0.6627296587926517768, -0.6692913385826773087, -0.1292274648535924053 ) ) ;
#7832=CARTESIAN_POINT ( 'NONE',  ( 1.371391076115485719, -0.6692913385826773087, -0.1292274648535924053 ) ) ;
#7837=CARTESIAN_POINT ( 'NONE',  ( 0.3018372703412079971, -0.3690944881889763329, 0.3153832671262228327 ) ) ;
#7838=CARTESIAN_POINT ( 'NONE',  ( -0.1115485564304456306, 0.2952755905511810774, -0.1292274648535930714 ) ) ;
#7839=CARTESIAN_POINT ( 'NONE',  ( 1.338582677165355062, -0.1870078740157480879, -0.4822834645669291653 ) ) ;
#7841=CARTESIAN_POINT ( 'NONE',  ( 0.3543307086614181922, -0.5511811023622047445, 6.969142054262312111E-17 ) ) ;
#7842=CARTESIAN_POINT ( 'NONE',  ( -0.6496062992125976043, 0.1660481256975883668, -0.3530559997133364547 ) ) ;
#7843=CARTESIAN_POINT ( 'NONE',  ( 1.614173228346457378, 0.2952755905511811885, 0.000000000000000000 ) ) ;
#7844=CARTESIAN_POINT ( 'NONE',  ( 0.3740157480314966754, -0.5400638737290844871, 0.3530559997133364547 ) ) ;
#7846=VECTOR ( 'NONE', #8983, 39.37007874015748143 ) ;
#7850=CARTESIAN_POINT ( 'NONE',  ( -1.404199475065615932, 0.05413385826771666132, 0.4176697321401328100 ) ) ;
#7851=CARTESIAN_POINT ( 'NONE',  ( -1.358267716535432434, -0.4536011799217367080, 0.2665933059059888421 ) ) ;
#7852=CARTESIAN_POINT ( 'NONE',  ( -1.299212598425196097, 0.2952755905511811885, 0.000000000000000000 ) ) ;
#7854=CARTESIAN_POINT ( 'NONE',  ( -2.795275590551181466, 2.125984251968505045, 0.000000000000000000 ) ) ;
#7855=CARTESIAN_POINT ( 'NONE',  ( -1.568241469816272105, -0.2845877964562161244, -0.3641732283464567121 ) ) ;
#7856=CARTESIAN_POINT ( 'NONE',  ( -1.102362204724408601, -0.1870078740157479769, 0.4822834645669291653 ) ) ;
#7857=CARTESIAN_POINT ( 'NONE',  ( 0.3149606299212603933, -0.1870078740157479769, 0.4822834645669291653 ) ) ;
#7859=CARTESIAN_POINT ( 'NONE',  ( -1.266404199475064773, -0.05778040916215560624, -0.4822834645669293319 ) ) ;
#7862=CARTESIAN_POINT ( 'NONE',  ( 0.6102362204724416372, -0.5400638737290844871, 0.3530559997133364547 ) ) ;
#7864=CARTESIAN_POINT ( 'NONE',  ( -0.8005249343832011588, -0.004921259842519870586, -0.3153832671262229437 ) ) ;
#7867=ORIENTED_EDGE ( 'NONE', *, *, #56862, .T. ) ;
#7868=CARTESIAN_POINT ( 'NONE',  ( -0.6406204526026236801, -3.721645946415733147E-15, -0.4118477457933000796 ) ) ;
#7869=CARTESIAN_POINT ( 'NONE',  ( -1.062992125984250968, 0.2952755905511811885, 0.000000000000000000 ) ) ;
#7870=CARTESIAN_POINT ( 'NONE',  ( -1.108923884514435132, -0.05778040916215560624, -0.4822834645669293319 ) ) ;
#7872=CARTESIAN_POINT ( 'NONE',  ( -1.673228346456691717, 0.1660481256975883668, -0.3530559997133364547 ) ) ;
#7873=CARTESIAN_POINT ( 'NONE',  ( -1.673228346456691717, 0.1660481256975883668, -0.3530559997133364547 ) ) ;
#7874=CARTESIAN_POINT ( 'NONE',  ( -1.640419947506561060, 0.05413385826771666132, 0.4176697321401328100 ) ) ;
#7877=CARTESIAN_POINT ( 'NONE',  ( 0.1509186351706045259, -0.08942795157528024563, -0.3641732283464568787 ) ) ;
#7880=CARTESIAN_POINT ( 'NONE',  ( -0.5183727034120726440, -0.5511811023622048555, -0.09757992244046775898 ) ) ;
#7881=CARTESIAN_POINT ( 'NONE',  ( -0.6824146981627288167, 0.2306618581243848609, 0.2411417322834645549 ) ) ;
#7882=CARTESIAN_POINT ( 'NONE',  ( 0.8923884514435701520, -0.6046776061558809534, -0.2411417322834644161 ) ) ;
#7883=CARTESIAN_POINT ( 'NONE',  ( -1.115485564304461219, 0.05413385826771626580, -0.4176697321401330321 ) ) ;
#7886=CARTESIAN_POINT ( 'NONE',  ( -1.122047244094487306, 0.1660481256975883668, -0.3530559997133364547 ) ) ;
#7887=CARTESIAN_POINT ( 'NONE',  ( 0.8005249343832027131, 0.05413385826771666132, 0.4176697321401328100 ) ) ;
#7889=CARTESIAN_POINT ( 'NONE',  ( -1.528871391076114250, 0.1771653543307087075, -0.09757992244046823083 ) ) ;
#7896=CARTESIAN_POINT ( 'NONE',  ( -0.3412073490813641308, 0.2306618581243847221, -0.2411417322834647770 ) ) ;
#7897=CARTESIAN_POINT ( 'NONE',  ( -1.430446194225720724, -0.004921259842519870586, -0.3153832671262229437 ) ) ;
#7898=CARTESIAN_POINT ( 'NONE',  ( -0.8595800524934373854, -0.3162353388693409650, -0.4822834645669289433 ) ) ;
#7900=CARTESIAN_POINT ( 'NONE',  ( -1.154855643044618851, -0.6046776061558809534, -0.2411417322834644161 ) ) ;
#7902=CARTESIAN_POINT ( 'NONE',  ( -1.128608923884513837, -0.6046776061558807314, 0.2411417322834647770 ) ) ;
#7903=CARTESIAN_POINT ( 'NONE',  ( -0.4265091863517051496, 0.2952755905511810774, -0.1292274648535930714 ) ) ;
#7905=CARTESIAN_POINT ( 'NONE',  ( 0.2559055118110243332, -0.4536011799217368745, -0.2665933059059886201 ) ) ;
#7907=CARTESIAN_POINT ( 'NONE',  ( 0.4855643044619430415, -0.3690944881889765550, -0.3153832671262227771 ) ) ;
#7908=CARTESIAN_POINT ( 'NONE',  ( 1.364829396325459854, -0.5023911411419708095, -0.1820866141732282451 ) ) ;
#7909=CARTESIAN_POINT ( 'NONE',  ( 0.9514435695538062676, -0.05778040916215522460, 0.4822834645669289988 ) ) ;
#7910=CARTESIAN_POINT ( 'NONE',  ( 0.1902887139107617975, -0.5511811023622048555, -0.09757992244046775898 ) ) ;
#7912=CARTESIAN_POINT ( 'NONE',  ( -1.430446194225720724, 0.05413385826771626580, -0.4176697321401330321 ) ) ;
#7913=CARTESIAN_POINT ( 'NONE',  ( -0.2099737532808391705, -0.5023911411419708095, -0.1820866141732282451 ) ) ;
#7915=CARTESIAN_POINT ( 'NONE',  ( -0.5183727034120726440, 0.1771653543307087630, 0.09757992244046791164 ) ) ;
#7917=CARTESIAN_POINT ( 'NONE',  ( -0.1771653543307080136, 0.1660481256975883668, -0.3530559997133364547 ) ) ;
#7919=CARTESIAN_POINT ( 'NONE',  ( 1.161417322834646271, 0.07958543189024071263, -0.2665933059059888421 ) ) ;
#7920=CARTESIAN_POINT ( 'NONE',  ( -0.05249343832020938322, -0.5023911411419708095, -0.1820866141732282451 ) ) ;
#7921=CARTESIAN_POINT ( 'NONE',  ( -0.1706036745406816491, 0.05413385826771626580, -0.4176697321401330321 ) ) ;
#7923=CARTESIAN_POINT ( 'NONE',  ( -0.6889763779527552368, 0.07958543189024085140, 0.2665933059059887866 ) ) ;
#7925=CARTESIAN_POINT ( 'NONE',  ( 0.6889763779527566800, -0.5400638737290844871, 0.3530559997133364547 ) ) ;
#7926=CARTESIAN_POINT ( 'NONE',  ( -0.7677165354330699465, -0.5400638737290845981, -0.3530559997133363437 ) ) ;
#7929=CARTESIAN_POINT ( 'NONE',  ( 0.1837270341207354329, 0.1283753931104748280, 0.1820866141732283561 ) ) ;
#7930=CARTESIAN_POINT ( 'NONE',  ( -0.9514435695538050464, -0.05778040916215560624, -0.4822834645669293319 ) ) ;
#7931=CARTESIAN_POINT ( 'NONE',  ( -0.9908136482939626788, 0.2952755905511811885, 0.1292274648535926551 ) ) ;
#7932=CARTESIAN_POINT ( 'NONE',  ( -1.384514435695537005, -0.5511811023622048555, -0.09757992244046775898 ) ) ;
#7933=CARTESIAN_POINT ( 'NONE',  ( 1.686351706036745890, 0.2952755905511811885, 0.1292274648535926551 ) ) ;
#7934=CARTESIAN_POINT ( 'NONE',  ( -1.069553805774277722, -0.5511811023622048555, -0.09757992244046775898 ) ) ;
#7935=CARTESIAN_POINT ( 'NONE',  ( -0.7414698162729651543, 0.2066929133858267098, -0.1054918080437494132 ) ) ;
#7936=CARTESIAN_POINT ( 'NONE',  ( 0.7480314960629927956, -0.6692913385826771977, 8.415575281601705876E-17 ) ) ;
#7939=ORIENTED_EDGE ( 'NONE', *, *, #28626, .T. ) ;
#7941=CARTESIAN_POINT ( 'NONE',  ( 1.502624671916010790, -0.2845877964562161244, -0.3641732283464567121 ) ) ;
#7942=CARTESIAN_POINT ( 'NONE',  ( -1.135170603674539924, -0.6692913385826771977, 0.1292274648535927661 ) ) ;
#7944=CARTESIAN_POINT ( 'NONE',  ( 1.351706036745407458, -0.4281496062992127816, -0.4176697321401328100 ) ) ;
#7947=CARTESIAN_POINT ( 'NONE',  ( 0.5183727034120741983, -0.6692913385826771977, 0.1292274648535927661 ) ) ;
#7948=CARTESIAN_POINT ( 'NONE',  ( -0.2165354330708654795, 0.1660481256975885056, 0.3530559997133364547 ) ) ;
#7950=CARTESIAN_POINT ( 'NONE',  ( 0.06632061457837788720, 2.409604939980833412E-17, -0.3464511005275205946 ) ) ;
#7951=CARTESIAN_POINT ( 'NONE',  ( 0.6233595800524939223, -0.2845877964562159024, 0.3641732283464567677 ) ) ;
#7953=ORIENTED_EDGE ( 'NONE', *, *, #1563, .T. ) ;
#7956=CARTESIAN_POINT ( 'NONE',  ( 0.1706036745406830368, 0.05413385826771666132, 0.4176697321401328100 ) ) ;
#7957=CARTESIAN_POINT ( 'NONE',  ( 1.272965879265092637, 0.05413385826771666132, 0.4176697321401328100 ) ) ;
#7958=CARTESIAN_POINT ( 'NONE',  ( 0.2230971128608932319, -0.4281496062992124485, 0.4176697321401328655 ) ) ;
#7959=CARTESIAN_POINT ( 'NONE',  ( -0.5511811023622038563, -0.1870078740157479769, 0.3641732283464567677 ) ) ;
#7960=CARTESIAN_POINT ( 'NONE',  ( 1.279527559055118724, -0.5400638737290845981, -0.3530559997133363437 ) ) ;
#7961=CARTESIAN_POINT ( 'NONE',  ( -0.3280839895013117347, 0.05413385826771626580, -0.4176697321401330321 ) ) ;
#7962=CARTESIAN_POINT ( 'NONE',  ( 0.05905511811023681640, 0.1660481256975883668, -0.3530559997133364547 ) ) ;
#7963=CARTESIAN_POINT ( 'NONE',  ( -1.581364829396324945, -0.05778040916215560624, -0.4822834645669293319 ) ) ;
#7964=CARTESIAN_POINT ( 'NONE',  ( 1.154855643044620184, 0.2306618581243847221, -0.2411417322834647770 ) ) ;
#7965=CARTESIAN_POINT ( 'NONE',  ( 1.318897637795276356, -0.5400638737290844871, 0.3530559997133364547 ) ) ;
#7967=CARTESIAN_POINT ( 'NONE',  ( 0.5052493438320218022, -0.5511811023622048555, -0.09757992244046775898 ) ) ;
#7970=VERTEX_POINT ( 'NONE', #54295 ) ;
#7971=CARTESIAN_POINT ( 'NONE',  ( -0.4133858267716528645, 0.07958543189024071263, -0.2665933059059888421 ) ) ;
#7972=CARTESIAN_POINT ( 'NONE',  ( -0.03937007874015669567, 0.2952755905511811885, 0.000000000000000000 ) ) ;
#7974=CARTESIAN_POINT ( 'NONE',  ( -0.09842519685039295696, 0.1660481256975883668, -0.3530559997133364547 ) ) ;
#7975=CARTESIAN_POINT ( 'NONE',  ( 0.2034120734908142214, 0.2952755905511810774, -0.1292274648535930714 ) ) ;
#7976=CARTESIAN_POINT ( 'NONE',  ( -0.9055118110236215490, -0.6692913385826771977, 8.415575281601705876E-17 ) ) ;
#7977=CARTESIAN_POINT ( 'NONE',  ( -0.9317585301837263412, 0.05413385826771666132, 0.4176697321401328100 ) ) ;
#7978=CARTESIAN_POINT ( 'NONE',  ( 1.167979002624672580, -0.3690944881889763329, 0.3153832671262228327 ) ) ;
#7979=CARTESIAN_POINT ( 'NONE',  ( -1.528871391076114250, -0.6692913385826771977, 0.1292274648535927661 ) ) ;
#7981=CARTESIAN_POINT ( 'NONE',  ( 0.8923884514435701520, -0.5023911411419708095, -0.1820866141732282451 ) ) ;
#7982=CARTESIAN_POINT ( 'NONE',  ( 0.5249343832021005074, -0.6046776061558807314, 0.2411417322834647770 ) ) ;
#7983=CARTESIAN_POINT ( 'NONE',  ( 0.3477690288713918276, -0.6692913385826773087, -0.1292274648535924053 ) ) ;
#7985=CARTESIAN_POINT ( 'NONE',  ( 0.3256598226813657848, 2.726622551019859153E-15, 0.4118477457932983032 ) ) ;
#7988=CARTESIAN_POINT ( 'NONE',  ( -0.4855643044619415427, -0.4281496062992124485, 0.4176697321401328655 ) ) ;
#7991=CARTESIAN_POINT ( 'NONE',  ( -1.115485564304461219, -0.004921259842519870586, -0.3153832671262229437 ) ) ;
#7992=CARTESIAN_POINT ( 'NONE',  ( 0.9908136482939640111, 0.2952755905511810774, -0.1292274648535930714 ) ) ;
#7993=CARTESIAN_POINT ( 'NONE',  ( 0.9908136482939640111, -0.6692913385826771977, 0.1292274648535927661 ) ) ;
#7994=CARTESIAN_POINT ( 'NONE',  ( -0.2230971128608915943, -0.004921259842519576551, 0.3153832671262227771 ) ) ;
#7995=CARTESIAN_POINT ( 'NONE',  ( 0.2887139107611556010, -0.6046776061558807314, 0.2411417322834647770 ) ) ;
#7997=CARTESIAN_POINT ( 'NONE',  ( 0.1115485564304470323, 0.1771653543307087630, 0.09757992244046791164 ) ) ;
#7999=CARTESIAN_POINT ( 'NONE',  ( 0.01312335958005323398, 0.05413385826771666132, 0.4176697321401328100 ) ) ;
#8001=CARTESIAN_POINT ( 'NONE',  ( -1.325459317585300889, -0.4281496062992127816, -0.4176697321401328100 ) ) ;
#8002=CARTESIAN_POINT ( 'NONE',  ( 0.4133858267716541968, -0.4536011799217368745, -0.2665933059059886201 ) ) ;
#8003=CARTESIAN_POINT ( 'NONE',  ( 1.627296587926509996, -0.5023911411419708095, 0.1820866141732285504 ) ) ;
#8004=CARTESIAN_POINT ( 'NONE',  ( -0.6889763779527552368, -0.5400638737290845981, -0.3530559997133363437 ) ) ;
#8005=CARTESIAN_POINT ( 'NONE',  ( -0.3937007874015740483, -0.1870078740157479769, 0.3641732283464567677 ) ) ;
#8006=CARTESIAN_POINT ( 'NONE',  ( -0.7213048242569877200, 1.923042556024872285, -0.5309055118110235227 ) ) ;
#8007=CARTESIAN_POINT ( 'NONE',  ( -0.7545931758530177724, 0.2952755905511811885, 0.1292274648535926551 ) ) ;
#8008=CARTESIAN_POINT ( 'NONE',  ( -0.6758530183727028406, 0.2952755905511811885, 0.1292274648535926551 ) ) ;
#8009=CARTESIAN_POINT ( 'NONE',  ( 0.05905511811023709395, -0.5400638737290844871, 0.3530559997133364547 ) ) ;
#8012=CARTESIAN_POINT ( 'NONE',  ( -1.633858267716534529, -0.4536011799217368745, -0.2665933059059886201 ) ) ;
#8013=CARTESIAN_POINT ( 'NONE',  ( 0.5643044619422579178, -0.004921259842519576551, 0.3153832671262227771 ) ) ;
#8014=CARTESIAN_POINT ( 'NONE',  ( 1.377952755905512472, -0.6692913385826771977, 8.415575281601705876E-17 ) ) ;
#8015=CARTESIAN_POINT ( 'NONE',  ( -0.7349081364829390672, 0.1283753931104746893, -0.1820866141732285504 ) ) ;
#8017=CARTESIAN_POINT ( 'NONE',  ( -1.207349081364828880, 0.1283753931104746893, -0.1820866141732285504 ) ) ;
#8018=CARTESIAN_POINT ( 'NONE',  ( -0.6955380577427815458, 0.05413385826771666132, 0.4176697321401328100 ) ) ;
#8019=CARTESIAN_POINT ( 'NONE',  ( -0.5052493438320203589, -0.6692913385826771977, 0.1292274648535927661 ) ) ;
#8020=CARTESIAN_POINT ( 'NONE',  ( 0.4790026246719168435, -0.2845877964562161244, -0.3641732283464567121 ) ) ;
#8022=CARTESIAN_POINT ( 'NONE',  ( 1.279527559055118724, 0.07958543189024085140, 0.2665933059059887866 ) ) ;
#8024=CARTESIAN_POINT ( 'NONE',  ( 0.5183727034120741983, -0.6692913385826771977, 0.1292274648535927661 ) ) ;
#8026=CARTESIAN_POINT ( 'NONE',  ( -0.5839895013123351797, 0.2952755905511810774, -0.1292274648535930714 ) ) ;
#8028=CARTESIAN_POINT ( 'NONE',  ( 1.456692913385827515, 0.1771653543307087630, 0.000000000000000000 ) ) ;
#8029=CARTESIAN_POINT ( 'NONE',  ( 0.5839895013123367340, 0.2952755905511811885, 0.1292274648535926551 ) ) ;
#8030=CARTESIAN_POINT ( 'NONE',  ( 0.3280839895013130669, -0.4281496062992127816, -0.4176697321401328100 ) ) ;
#8031=CARTESIAN_POINT ( 'NONE',  ( -0.02624671916010428221, 0.1283753931104746893, -0.1820866141732285504 ) ) ;
#8033=CARTESIAN_POINT ( 'NONE',  ( 8.195543980992789655E-16, -0.1870078740157480601, -0.3641732283464567677 ) ) ;
#8034=CARTESIAN_POINT ( 'NONE',  ( 0.9908136482939640111, -0.6692913385826771977, 0.1292274648535927661 ) ) ;
#8035=CARTESIAN_POINT ( 'NONE',  ( -0.5839895013123351797, 0.1771653543307087075, -0.09757992244046823083 ) ) ;
#8036=CARTESIAN_POINT ( 'NONE',  ( -0.5577427821522301654, -0.3162353388693405765, 0.4822834645669290543 ) ) ;
#8038=B_SPLINE_CURVE_WITH_KNOTS ( 'NONE', 3,
 ( #40201, #73020, #60385, #1905, #21259, #59550, #73861 ),
 .UNSPECIFIED., .F., .F.,
 ( 4, 3, 4 ),
 ( 7.703719777548943412E-34, 0.001246232571205256601, 0.002492492258783257208 ),
 .UNSPECIFIED. ) ;
#8039=ORIENTED_EDGE ( 'NONE', *, *, #31019, .F. ) ;
#8040=CARTESIAN_POINT ( 'NONE',  ( -1.312335958005248715, 0.2306618581243848609, 0.2411417322834645549 ) ) ;
#8041=CARTESIAN_POINT ( 'NONE',  ( -1.128608923884513837, -0.5023911411419708095, 0.1820866141732285504 ) ) ;
#8042=CARTESIAN_POINT ( 'NONE',  ( 0.1640419947506569498, -0.05778040916215522460, 0.4822834645669289988 ) ) ;
#8044=CARTESIAN_POINT ( 'NONE',  ( -1.660104986876639543, -0.05778040916215560624, -0.4822834645669293319 ) ) ;
#8045=CARTESIAN_POINT ( 'NONE',  ( -0.6627296587926501115, 0.2952755905511810774, -0.1292274648535930714 ) ) ;
#8046=DIRECTION ( 'NONE',  ( 0.000000000000000000, 0.000000000000000000, 1.000000000000000000 ) ) ;
#8048=CARTESIAN_POINT ( 'NONE',  ( 0.8070866141732288002, 0.1660481256975885056, 0.3530559997133364547 ) ) ;
#8049=CARTESIAN_POINT ( 'NONE',  ( 0.7808398950131241190, -0.05778040916215560624, -0.4822834645669293319 ) ) ;
#8051=CARTESIAN_POINT ( 'NONE',  ( 1.522309711286089939, -0.6046776061558809534, -0.2411417322834644161 ) ) ;
#8052=CARTESIAN_POINT ( 'NONE',  ( -1.213910761154854745, 0.2952755905511810774, -0.1292274648535930714 ) ) ;
#8056=CARTESIAN_POINT ( 'NONE',  ( -0.3674540682414689785, 0.1283753931104748280, 0.1820866141732283561 ) ) ;
#8059=CARTESIAN_POINT ( 'NONE',  ( 0.2821522309711292364, -0.6692913385826771977, 0.1292274648535927661 ) ) ;
#8060=CARTESIAN_POINT ( 'NONE',  ( 0.1115485564304467270, -0.6692913385826773087, -0.1292274648535924053 ) ) ;
#8061=CARTESIAN_POINT ( 'NONE',  ( -0.6102362204724400829, -0.5400638737290845981, -0.3530559997133363437 ) ) ;
#8062=CARTESIAN_POINT ( 'NONE',  ( 1.496062992125985147, -0.1870078740157479769, 0.4822834645669291653 ) ) ;
#8063=CARTESIAN_POINT ( 'NONE',  ( -1.010498687664041384, -0.004921259842519576551, 0.3153832671262227771 ) ) ;
#8065=CARTESIAN_POINT ( 'NONE',  ( 0.9383202099737538715, -0.05778040916215560624, -0.4822834645669293319 ) ) ;
#8066=CARTESIAN_POINT ( 'NONE',  ( 0.5446194225721792126, -0.08942795157528024563, -0.3641732283464568787 ) ) ;
#8067=CARTESIAN_POINT ( 'NONE',  ( -0.2952755905511803003, -0.5400638737290845981, -0.3530559997133363437 ) ) ;
#8069=CARTESIAN_POINT ( 'NONE',  ( -0.6692913385826764205, 0.2952755905511811885, 0.000000000000000000 ) ) ;
#8070=CARTESIAN_POINT ( 'NONE',  ( -1.581364829396324945, -0.2845877964562159024, 0.3641732283464567677 ) ) ;
#8071=CARTESIAN_POINT ( 'NONE',  ( 1.338582677165355062, -0.1870078740157479769, 0.4822834645669291653 ) ) ;
#8075=CARTESIAN_POINT ( 'NONE',  ( 0.1837270341207357105, -0.6046776061558809534, -0.2411417322834644161 ) ) ;
#8077=CARTESIAN_POINT ( 'NONE',  ( -1.174540682414697335, -0.3162353388693409650, -0.4822834645669289433 ) ) ;
#8078=CARTESIAN_POINT ( 'NONE',  ( 1.377952755905512472, -0.6692913385826771977, 8.415575281601705876E-17 ) ) ;
#8079=CARTESIAN_POINT ( 'NONE',  ( 1.194225721784777594, -0.4281496062992127816, -0.4176697321401328100 ) ) ;
#8080=CARTESIAN_POINT ( 'NONE',  ( 0.2821522309711292364, -0.6692913385826771977, 0.1292274648535927661 ) ) ;
#8081=CARTESIAN_POINT ( 'NONE',  ( -0.2952755905511803003, -0.5400638737290845981, -0.3530559997133363437 ) ) ;
#8083=CARTESIAN_POINT ( 'NONE',  ( -1.240157480314959759, 0.1660481256975885056, 0.3530559997133364547 ) ) ;
#8084=CARTESIAN_POINT ( 'NONE',  ( -0.5446194225721777693, -0.05778040916215522460, 0.4822834645669289988 ) ) ;
#8085=CARTESIAN_POINT ( 'NONE',  ( -0.6167979002624665030, -0.3690944881889765550, -0.3153832671262227771 ) ) ;
#8086=CARTESIAN_POINT ( 'NONE',  ( 1.614173228346457378, -0.6692913385826771977, 8.415575281601705876E-17 ) ) ;
#8087=CARTESIAN_POINT ( 'NONE',  ( -0.6496062992125976043, -0.5400638737290844871, 0.3530559997133364547 ) ) ;
#8089=CARTESIAN_POINT ( 'NONE',  ( 0.5839895013123367340, -0.6692913385826773087, -0.1292274648535924053 ) ) ;
#8090=LINE ( 'NONE', #7242, #77886 ) ;
#8091=CARTESIAN_POINT ( 'NONE',  ( 0.05249343832021075018, -0.6046776061558807314, 0.2411417322834647770 ) ) ;
#8092=CARTESIAN_POINT ( 'NONE',  ( -0.1246719160104980823, 0.1771653543307087630, 0.09757992244046791164 ) ) ;
#8093=CARTESIAN_POINT ( 'NONE',  ( 1.161417322834646493, -0.4536011799217367080, 0.2665933059059888421 ) ) ;
#8094=CARTESIAN_POINT ( 'NONE',  ( 0.6967283859536044233, -4.069555009745408348E-17, -0.3627989612356146698 ) ) ;
#8096=CARTESIAN_POINT ( 'NONE',  ( 1.246719160104987623, -0.004921259842519870586, -0.3153832671262229437 ) ) ;
#8097=CARTESIAN_POINT ( 'NONE',  ( 1.161417322834646271, 0.1660481256975883668, -0.3530559997133364547 ) ) ;
#8099=CARTESIAN_POINT ( 'NONE',  ( 0.006561679790026889343, -0.05778040916215522460, 0.4822834645669289988 ) ) ;
#8100=CARTESIAN_POINT ( 'NONE',  ( -1.509186351706035767, -0.4281496062992124485, 0.4176697321401328655 ) ) ;
#8101=CARTESIAN_POINT ( 'NONE',  ( 1.607611548556431069, 0.1771653543307087630, 0.09757992244046791164 ) ) ;
#8102=CARTESIAN_POINT ( 'NONE',  ( -0.2362204724409442680, -0.1870078740157480879, -0.4822834645669291653 ) ) ;
#8104=CARTESIAN_POINT ( 'NONE',  ( -1.541994750656167090, -0.5511811023622048555, -0.09757992244046775898 ) ) ;
#8105=CARTESIAN_POINT ( 'NONE',  ( 0.4265091863517067039, -0.6692913385826773087, -0.1292274648535924053 ) ) ;
#8106=CARTESIAN_POINT ( 'NONE',  ( 0.8136482939632553313, -0.5023911411419708095, -0.1820866141732282451 ) ) ;
#8108=CARTESIAN_POINT ( 'NONE',  ( 0.5511811023622055217, -0.1870078740157479769, 0.3641732283464567677 ) ) ;
#8109=CARTESIAN_POINT ( 'NONE',  ( -1.397637795275589623, -0.5400638737290845981, -0.3530559997133363437 ) ) ;
#8111=CARTESIAN_POINT ( 'NONE',  ( 1.253280839895013710, -0.05778040916215560624, -0.4822834645669293319 ) ) ;
#8113=CARTESIAN_POINT ( 'NONE',  ( 0.2887139107611556010, 0.2306618581243847221, -0.2411417322834647770 ) ) ;
#8116=CARTESIAN_POINT ( 'NONE',  ( 0.6430446194225728496, -0.004921259842519576551, 0.3153832671262227771 ) ) ;
#8118=CARTESIAN_POINT ( 'NONE',  ( 0.6955380577427828781, -0.4281496062992124485, 0.4176697321401328655 ) ) ;
#8119=CARTESIAN_POINT ( 'NONE',  ( 0.7210809602247731931, 4.888820689338890882E-16, 0.3464511005275202615 ) ) ;
#8120=CARTESIAN_POINT ( 'NONE',  ( -0.9251968503937002541, 0.07958543189024085140, 0.2665933059059887866 ) ) ;
#8121=CARTESIAN_POINT ( 'NONE',  ( -1.187664041994750175, -0.05778040916215560624, -0.4822834645669293319 ) ) ;
#8122=CARTESIAN_POINT ( 'NONE',  ( -1.732283464566928277, -0.1870078740157479769, 0.4822834645669291653 ) ) ;
#8123=CARTESIAN_POINT ( 'NONE',  ( 0.3740157480314966754, -0.5400638737290844871, 0.3530559997133364547 ) ) ;
#8124=CARTESIAN_POINT ( 'NONE',  ( -1.614173228346455824, 0.1771653543307087630, 0.000000000000000000 ) ) ;
#8127=CARTESIAN_POINT ( 'NONE',  ( 0.6167979002624678353, -0.4281496062992124485, 0.4176697321401328655 ) ) ;
#8129=LINE ( 'NONE', #59459, #15912 ) ;
#8130=CARTESIAN_POINT ( 'NONE',  ( 1.397637795275591177, 0.1660481256975883668, -0.3530559997133364547 ) ) ;
#8131=CARTESIAN_POINT ( 'NONE',  ( -1.430446194225721390, -0.3690944881889763329, 0.3153832671262228327 ) ) ;
#8132=CARTESIAN_POINT ( 'NONE',  ( 1.030183727034121421, -0.08942795157527998196, 0.3641732283464567121 ) ) ;
#8133=CARTESIAN_POINT ( 'NONE',  ( -1.450131233595799651, 0.1771653543307087075, -0.09757992244046823083 ) ) ;
#8134=CARTESIAN_POINT ( 'NONE',  ( -0.7808398950131222316, -0.2845877964562161244, -0.3641732283464567121 ) ) ;
#8135=CARTESIAN_POINT ( 'NONE',  ( 1.581364829396326277, -0.05778040916215522460, 0.4822834645669289988 ) ) ;
#8136=CARTESIAN_POINT ( 'NONE',  ( 0.5905511811023629321, -0.5511811023622047445, 6.969142054262312111E-17 ) ) ;
#8137=CARTESIAN_POINT ( 'NONE',  ( 0.5183727034120741983, -0.6692913385826771977, 0.1292274648535927661 ) ) ;
#8138=CARTESIAN_POINT ( 'NONE',  ( 1.312335958005249825, 0.2306618581243847221, -0.2411417322834647770 ) ) ;
#8139=CARTESIAN_POINT ( 'NONE',  ( 0.2559055118110243332, 0.1660481256975885056, 0.3530559997133364547 ) ) ;
#8140=CARTESIAN_POINT ( 'NONE',  ( 0.3477690288713918276, 0.1771653543307087630, 0.09757992244046791164 ) ) ;
#8141=CARTESIAN_POINT ( 'NONE',  ( 1.377952755905512472, -0.6692913385826771977, 8.415575281601705876E-17 ) ) ;
#8143=CARTESIAN_POINT ( 'NONE',  ( -1.069553805774277722, 0.2952755905511811885, 0.1292274648535926551 ) ) ;
#8146=CARTESIAN_POINT ( 'NONE',  ( -0.01968503937007793844, -0.5400638737290844871, 0.3530559997133364547 ) ) ;
#8147=CARTESIAN_POINT ( 'NONE',  ( -0.8333333333333323711, 0.2952755905511811885, 0.1292274648535926551 ) ) ;
#8148=CARTESIAN_POINT ( 'NONE',  ( 0.05249343832021075018, 0.2306618581243847221, -0.2411417322834647770 ) ) ;
#8152=CARTESIAN_POINT ( 'NONE',  ( 0.4965823432763554757, 1.491030243898183949, 0.5309055118110234117 ) ) ;
#8153=CARTESIAN_POINT ( 'NONE',  ( -0.7677165354330699465, 0.07958543189024085140, 0.2665933059059887866 ) ) ;
#8155=CARTESIAN_POINT ( 'NONE',  ( -1.541994750656167090, 0.2952755905511811885, 0.1292274648535926551 ) ) ;
#8157=CARTESIAN_POINT ( 'NONE',  ( 0.5183727034120741983, -0.6692913385826771977, 0.1292274648535927661 ) ) ;
#8158=CARTESIAN_POINT ( 'NONE',  ( -0.5708661417322828946, 0.07958543189024071263, -0.2665933059059888421 ) ) ;
#8159=CARTESIAN_POINT ( 'NONE',  ( 0.8595800524934390507, -0.05778040916215560624, -0.4822834645669293319 ) ) ;
#8160=CARTESIAN_POINT ( 'NONE',  ( 0.3280839895013130669, 0.05413385826771666132, 0.4176697321401328100 ) ) ;
#8164=CARTESIAN_POINT ( 'NONE',  ( 1.115485564304462551, -0.4281496062992127816, -0.4176697321401328100 ) ) ;
#8165=CARTESIAN_POINT ( 'NONE',  ( -0.1049868766404193215, 0.2306618581243847221, -0.2411417322834647770 ) ) ;
#8166=CARTESIAN_POINT ( 'NONE',  ( -1.614173228346455824, 0.2952755905511811885, 0.000000000000000000 ) ) ;
#8167=CARTESIAN_POINT ( 'NONE',  ( 0.7349081364829403995, 0.2306618581243848609, 0.2411417322834645549 ) ) ;
#8169=CARTESIAN_POINT ( 'NONE',  ( 0.1574803149606306130, -0.1870078740157479769, 0.4822834645669291653 ) ) ;
#8170=CARTESIAN_POINT ( 'NONE',  ( 0.5708661417322842269, 0.1660481256975885056, 0.3530559997133364547 ) ) ;
#8171=CARTESIAN_POINT ( 'NONE',  ( -0.1509186351706028884, -0.3162353388693409650, -0.4822834645669289433 ) ) ;
#8172=CARTESIAN_POINT ( 'NONE',  ( 1.194225721784777594, -0.004921259842519576551, 0.3153832671262227771 ) ) ;
#8173=CARTESIAN_POINT ( 'NONE',  ( -1.227034120734907585, 0.2952755905511811885, 0.1292274648535926551 ) ) ;
#8174=CARTESIAN_POINT ( 'NONE',  ( -1.423884514435694859, -0.3162353388693405765, 0.4822834645669290543 ) ) ;
#8175=CARTESIAN_POINT ( 'NONE',  ( 0.7677165354330716118, -0.5400638737290844871, 0.3530559997133364547 ) ) ;
#8180=VERTEX_POINT ( 'NONE', #63100 ) ;
#8181=CARTESIAN_POINT ( 'NONE',  ( 1.299212598425197429, -0.6692913385826771977, 8.415575281601705876E-17 ) ) ;
#8182=CARTESIAN_POINT ( 'NONE',  ( 1.069553805774278610, -0.5511811023622046335, 0.09757992244046803654 ) ) ;
#8183=CARTESIAN_POINT ( 'NONE',  ( 0.5611900217179910388, 1.223219560026271499E-15, 0.4445507791589056734 ) ) ;
#8187=CARTESIAN_POINT ( 'NONE',  ( 1.299212598425197429, 0.2952755905511811885, 0.000000000000000000 ) ) ;
#8188=CARTESIAN_POINT ( 'NONE',  ( -1.646981627296586703, -0.05778040916215522460, 0.4822834645669289988 ) ) ;
#8189=CARTESIAN_POINT ( 'NONE',  ( -0.4986876640419942164, -0.6046776061558807314, 0.2411417322834647770 ) ) ;
#8190=CARTESIAN_POINT ( 'NONE',  ( 1.043307086614173818, -0.5400638737290845981, -0.3530559997133363437 ) ) ;
#8193=CARTESIAN_POINT ( 'NONE',  ( -1.496062992125983815, -0.1870078740157480879, -0.4822834645669291653 ) ) ;
#8196=CARTESIAN_POINT ( 'NONE',  ( 1.653543307086614789, -0.1870078740157479769, 0.3641732283464567677 ) ) ;
#8198=CARTESIAN_POINT ( 'NONE',  ( -0.7152230971128602510, -0.2845877964562159024, 0.3641732283464567677 ) ) ;
#8200=CARTESIAN_POINT ( 'NONE',  ( -1.541994750656167090, -0.6692913385826773087, -0.1292274648535924053 ) ) ;
#8201=CARTESIAN_POINT ( 'NONE',  ( 0.5905511811023629321, 0.2952755905511811885, 0.000000000000000000 ) ) ;
#8203=CARTESIAN_POINT ( 'NONE',  ( 1.581364829396326277, -0.3162353388693409650, -0.4822834645669289433 ) ) ;
#8204=CARTESIAN_POINT ( 'NONE',  ( -0.4061203303035118561, -2.613618158232546091E-15, -0.3464511005275220379 ) ) ;
#8205=CARTESIAN_POINT ( 'NONE',  ( -0.8727034120734901146, -0.08942795157528024563, -0.3641732283464568787 ) ) ;
#8206=CARTESIAN_POINT ( 'NONE',  ( 0.8333333333333340365, -0.6692913385826771977, 0.1292274648535927661 ) ) ;
#8207=CARTESIAN_POINT ( 'NONE',  ( -1.535433070866141225, 0.2952755905511811885, 0.000000000000000000 ) ) ;
#8209=CARTESIAN_POINT ( 'NONE',  ( -0.7217847769028863381, -0.004921259842519870586, -0.3153832671262229437 ) ) ;
#8210=CARTESIAN_POINT ( 'NONE',  ( 1.594488188976378673, -0.5400638737290845981, -0.3530559997133363437 ) ) ;
#8212=CARTESIAN_POINT ( 'NONE',  ( 0.5314960629921264834, 0.1660481256975883668, -0.3530559997133364547 ) ) ;
#8213=CARTESIAN_POINT ( 'NONE',  ( -0.9514435695538050464, -0.08942795157528024563, -0.3641732283464568787 ) ) ;
#8214=CARTESIAN_POINT ( 'NONE',  ( -0.5249343832020990641, -0.5023911411419708095, -0.1820866141732282451 ) ) ;
#8216=CARTESIAN_POINT ( 'NONE',  ( -0.1377952755905504645, 0.1660481256975885056, 0.3530559997133364547 ) ) ;
#8217=CARTESIAN_POINT ( 'NONE',  ( -1.187664041994749731, -0.2845877964562159024, 0.3641732283464567677 ) ) ;
#8219=CARTESIAN_POINT ( 'NONE',  ( 0.7349081364829402885, -0.6046776061558809534, -0.2411417322834644161 ) ) ;
#8222=CARTESIAN_POINT ( 'NONE',  ( -0.8530183727034112984, -0.4281496062992127816, -0.4176697321401328100 ) ) ;
#8223=CARTESIAN_POINT ( 'NONE',  ( -0.1574803149606292529, -0.1870078740157479769, 0.3641732283464567677 ) ) ;
#8224=CARTESIAN_POINT ( 'NONE',  ( -1.266404199475064773, -0.05778040916215560624, -0.4822834645669293319 ) ) ;
#8225=CARTESIAN_POINT ( 'NONE',  ( 0.6692913385826778638, -0.5511811023622047445, 6.969142054262312111E-17 ) ) ;
#8226=CARTESIAN_POINT ( 'NONE',  ( -0.8202099737532801971, -0.5511811023622046335, 0.09757992244046803654 ) ) ;
#8227=CARTESIAN_POINT ( 'NONE',  ( -1.043307086614172707, 0.1660481256975883668, -0.3530559997133364547 ) ) ;
#8228=CARTESIAN_POINT ( 'NONE',  ( -1.673228346456691717, 0.1660481256975883668, -0.3530559997133364547 ) ) ;
#8229=CARTESIAN_POINT ( 'NONE',  ( -1.535433070866141225, -0.6692913385826771977, 8.415575281601705876E-17 ) ) ;
#8230=CARTESIAN_POINT ( 'NONE',  ( 1.069553805774278832, 0.2066929133858267098, -0.1054918080437494132 ) ) ;
#8231=CARTESIAN_POINT ( 'NONE',  ( 0.7611548556430454138, 0.1283753931104746893, -0.1820866141732285504 ) ) ;
#8232=CARTESIAN_POINT ( 'NONE',  ( 0.3412073490813655186, -0.6046776061558809534, -0.2411417322834644161 ) ) ;
#8233=CARTESIAN_POINT ( 'NONE',  ( -1.653543307086613234, -0.1870078740157479769, 0.4822834645669291653 ) ) ;
#8234=CARTESIAN_POINT ( 'NONE',  ( 1.253280839895013710, -0.2845877964562159024, 0.3641732283464567677 ) ) ;
#8235=ORIENTED_EDGE ( 'NONE', *, *, #75011, .T. ) ;
#8237=CARTESIAN_POINT ( 'NONE',  ( -1.259842519685038686, -0.1870078740157480601, -0.3641732283464567677 ) ) ;
#8238=CARTESIAN_POINT ( 'NONE',  ( -0.5314960629921250401, 0.1660481256975885056, 0.3530559997133364547 ) ) ;
#8239=CARTESIAN_POINT ( 'NONE',  ( 0.1377952755905518800, -0.5400638737290844871, 0.3530559997133364547 ) ) ;
#8240=CARTESIAN_POINT ( 'NONE',  ( -1.620734908136482577, -0.5511811023622048555, -0.09757992244046775898 ) ) ;
#8242=CARTESIAN_POINT ( 'NONE',  ( -1.272965879265091305, -0.4281496062992124485, 0.4176697321401328655 ) ) ;
#8243=CARTESIAN_POINT ( 'NONE',  ( 0.4658792650918641698, -0.05778040916215560624, -0.4822834645669293319 ) ) ;
#8245=CARTESIAN_POINT ( 'NONE',  ( 0.3149606299212606708, -0.1870078740157480879, -0.4822834645669291653 ) ) ;
#8246=CARTESIAN_POINT ( 'NONE',  ( 1.023622047244095112, -0.1870078740157480879, -0.4822834645669291653 ) ) ;
#8251=CARTESIAN_POINT ( 'NONE',  ( 0.1115485564304467270, -0.5511811023622048555, -0.09757992244046775898 ) ) ;
#8253=CARTESIAN_POINT ( 'NONE',  ( -0.1246719160104980823, 0.2952755905511811885, 0.1292274648535926551 ) ) ;
#8254=CARTESIAN_POINT ( 'NONE',  ( 1.318897637795276356, 0.1660481256975883668, -0.3530559997133364547 ) ) ;
#8256=CARTESIAN_POINT ( 'NONE',  ( 0.01312335958005323398, -0.3690944881889765550, -0.3153832671262227771 ) ) ;
#8257=CARTESIAN_POINT ( 'NONE',  ( -1.345144356955379816, -0.3162353388693405765, 0.4822834645669290543 ) ) ;
#8258=CARTESIAN_POINT ( 'NONE',  ( 1.555118110236221041, -0.5400638737290844871, 0.3530559997133364547 ) ) ;
#8259=CARTESIAN_POINT ( 'NONE',  ( 0.5971128608923891301, 0.2952755905511810774, -0.1292274648535930714 ) ) ;
#8264=CARTESIAN_POINT ( 'NONE',  ( -1.594488188976377563, -0.5400638737290844871, 0.3530559997133364547 ) ) ;
#8265=CARTESIAN_POINT ( 'NONE',  ( -1.266404199475064773, -0.08942795157528024563, -0.3641732283464568787 ) ) ;
#8266=CARTESIAN_POINT ( 'NONE',  ( -1.318897637795274802, 0.1660481256975885056, 0.3530559997133364547 ) ) ;
#8269=CARTESIAN_POINT ( 'NONE',  ( -1.561679790026246017, -0.3690944881889765550, -0.3153832671262227771 ) ) ;
#8270=CARTESIAN_POINT ( 'NONE',  ( -1.161417322834644716, -0.5400638737290845981, -0.3530559997133363437 ) ) ;
#8271=CARTESIAN_POINT ( 'NONE',  ( 0.03937007874015806264, 0.2952755905511811885, 0.000000000000000000 ) ) ;
#8272=CARTESIAN_POINT ( 'NONE',  ( -1.194225721784776262, -0.4281496062992124485, 0.4176697321401328655 ) ) ;
#8274=CARTESIAN_POINT ( 'NONE',  ( 0.5249343832021003964, 0.2306618581243847221, -0.2411417322834647770 ) ) ;
#8276=CARTESIAN_POINT ( 'NONE',  ( -1.227034120734907141, -0.5511811023622048555, -0.09757992244046775898 ) ) ;
#8277=ORIENTED_EDGE ( 'NONE', *, *, #17800, .T. ) ;
#8279=ORIENTED_EDGE ( 'NONE', *, *, #49168, .F. ) ;
#8280=CARTESIAN_POINT ( 'NONE',  ( 1.220472440944882386, 0.000000000000000000, 0.000000000000000000 ) ) ;
#8281=CARTESIAN_POINT ( 'NONE',  ( -1.030183727034119867, -0.05778040916215560624, -0.4822834645669293319 ) ) ;
#8282=CARTESIAN_POINT ( 'NONE',  ( -1.194225721784776262, -0.4281496062992124485, 0.4176697321401328655 ) ) ;
#8284=CARTESIAN_POINT ( 'NONE',  ( -1.391076115485563758, 0.2306618581243848609, 0.2411417322834645549 ) ) ;
#8285=CARTESIAN_POINT ( 'NONE',  ( -1.528871391076114250, 0.2952755905511810774, -0.1292274648535930714 ) ) ;
#8286=CARTESIAN_POINT ( 'NONE',  ( -1.443569553805773564, 0.2306618581243847221, -0.2411417322834647770 ) ) ;
#8287=CARTESIAN_POINT ( 'NONE',  ( 1.614173228346456712, 2.401574803149606474, 0.1372047244094478646 ) ) ;
#8289=CARTESIAN_POINT ( 'NONE',  ( 0.2296587926509192634, -0.2845877964562159024, 0.3641732283464567677 ) ) ;
#8291=CARTESIAN_POINT ( 'NONE',  ( -0.5905511811023615998, 0.1771653543307087630, 0.000000000000000000 ) ) ;
#8292=CARTESIAN_POINT ( 'NONE',  ( -1.069553805774277722, -0.6692913385826773087, -0.1292274648535924053 ) ) ;
#8293=CARTESIAN_POINT ( 'NONE',  ( 1.076115485564305141, -0.6046776061558807314, 0.2411417322834647770 ) ) ;
#8294=CARTESIAN_POINT ( 'NONE',  ( -0.9383202099737524282, -0.3162353388693409650, -0.4822834645669289433 ) ) ;
#8296=ORIENTED_EDGE ( 'NONE', *, *, #45555, .F. ) ;
#8297=CARTESIAN_POINT ( 'NONE',  ( -0.9514435695538050464, -0.05778040916215560624, -0.4822834645669293319 ) ) ;
#8298=CARTESIAN_POINT ( 'NONE',  ( 0.9383202099737536495, -0.3162353388693405765, 0.4822834645669290543 ) ) ;
#8299=CARTESIAN_POINT ( 'NONE',  ( -1.699475065616797398, 0.1771653543307087630, 0.09757992244046791164 ) ) ;
#8300=CARTESIAN_POINT ( 'NONE',  ( -1.732283464566928277, -0.1870078740157479769, 0.4822834645669291653 ) ) ;
#8306=CARTESIAN_POINT ( 'NONE',  ( -0.2296587926509179312, -0.05778040916215522460, 0.4822834645669289988 ) ) ;
#8307=CARTESIAN_POINT ( 'NONE',  ( -1.653543307086613234, -0.1870078740157479769, 0.3641732283464567677 ) ) ;
#8309=CARTESIAN_POINT ( 'NONE',  ( -1.437007874015747477, -0.5400638737290844871, 0.3530559997133364547 ) ) ;
#8311=CARTESIAN_POINT ( 'NONE',  ( -1.253280839895012377, -0.05778040916215522460, 0.4822834645669289988 ) ) ;
#8312=CARTESIAN_POINT ( 'NONE',  ( -0.2165354330708654795, -0.5400638737290845981, -0.3530559997133363437 ) ) ;
#8314=CARTESIAN_POINT ( 'NONE',  ( 0.6299212598425204535, -0.1870078740157479769, 0.3641732283464567677 ) ) ;
#8316=CARTESIAN_POINT ( 'NONE',  ( 0.3740157480314966754, -0.4536011799217367080, 0.2665933059059888421 ) ) ;
#8317=CARTESIAN_POINT ( 'NONE',  ( 1.305774278215223960, 0.1771653543307087075, -0.09757992244046823083 ) ) ;
#8319=CARTESIAN_POINT ( 'NONE',  ( 0.7545931758530188826, -0.6692913385826771977, 0.1292274648535927661 ) ) ;
#8320=CARTESIAN_POINT ( 'NONE',  ( -0.03937007874015669567, 0.1771653543307087630, 0.000000000000000000 ) ) ;
#8322=CARTESIAN_POINT ( 'NONE',  ( -1.272965879265091305, 0.05413385826771626580, -0.4176697321401330321 ) ) ;
#8323=CARTESIAN_POINT ( 'NONE',  ( 0.1049868766404206816, -0.5023911411419708095, -0.1820866141732282451 ) ) ;
#8324=CARTESIAN_POINT ( 'NONE',  ( -1.364829396325458521, -0.5023911411419708095, 0.1820866141732285504 ) ) ;
#8326=CARTESIAN_POINT ( 'NONE',  ( -0.3740157480314953431, 0.07958543189024085140, 0.2665933059059887866 ) ) ;
#8328=CARTESIAN_POINT ( 'NONE',  ( -0.2296587926509179312, -0.05778040916215522460, 0.4822834645669289988 ) ) ;
#8330=CARTESIAN_POINT ( 'NONE',  ( 0.6233595800524939223, -0.2845877964562159024, 0.3641732283464567677 ) ) ;
#8331=CARTESIAN_POINT ( 'NONE',  ( -0.08530183727034056085, -0.08942795157528024563, -0.3641732283464568787 ) ) ;
#8332=CARTESIAN_POINT ( 'NONE',  ( -0.4199475065616791736, -0.6046776061558807314, 0.2411417322834647770 ) ) ;
#8334=CARTESIAN_POINT ( 'NONE',  ( -1.023622047244093558, -0.1870078740157479769, 0.3641732283464567677 ) ) ;
#8335=CYLINDRICAL_SURFACE ( 'NONE', #27379, 0.3937007874015748254 ) ;
#8336=EDGE_CURVE ( 'NONE', #54436, #17596, #44540, .T. ) ;
#8337=CARTESIAN_POINT ( 'NONE',  ( 0.5118110236220480003, -0.6692913385826771977, 8.415575281601705876E-17 ) ) ;
#8338=CARTESIAN_POINT ( 'NONE',  ( -0.9645669291338575535, 0.1660481256975883668, -0.3530559997133364547 ) ) ;
#8341=CARTESIAN_POINT ( 'NONE',  ( -0.07217847769028813698, -0.2845877964562161244, -0.3641732283464567121 ) ) ;
#8342=CARTESIAN_POINT ( 'NONE',  ( -1.338582677165353729, -0.1870078740157479769, 0.4822834645669291653 ) ) ;
#8343=CARTESIAN_POINT ( 'NONE',  ( 1.541994750656168645, 0.2952755905511810774, -0.1292274648535930714 ) ) ;
#8345=CARTESIAN_POINT ( 'NONE',  ( -0.5052493438320203589, -0.5511811023622046335, 0.09757992244046803654 ) ) ;
#8346=CARTESIAN_POINT ( 'NONE',  ( 0.4606732211681152100, 1.541615089183626441, 0.5309055118110234117 ) ) ;
#8347=CARTESIAN_POINT ( 'NONE',  ( 0.7742782152230978099, -0.4281496062992124485, 0.4176697321401328655 ) ) ;
#8351=CARTESIAN_POINT ( 'NONE',  ( 1.607611548556431069, 0.1771653543307087630, 0.09757992244046791164 ) ) ;
#8352=CARTESIAN_POINT ( 'NONE',  ( -1.174540682414697335, -0.3162353388693409650, -0.4822834645669289433 ) ) ;
#8353=CARTESIAN_POINT ( 'NONE',  ( 1.122047244094488860, 0.1660481256975885056, 0.3530559997133364547 ) ) ;
#8355=CARTESIAN_POINT ( 'NONE',  ( 1.496062992125985147, -0.1870078740157479769, 0.3641732283464567677 ) ) ;
#8357=CARTESIAN_POINT ( 'NONE',  ( 0.6824146981627303710, -0.6046776061558807314, 0.2411417322834647770 ) ) ;
#8358=CARTESIAN_POINT ( 'NONE',  ( -0.4724409448818890911, -0.1870078740157480879, -0.4822834645669291653 ) ) ;
#8359=CARTESIAN_POINT ( 'NONE',  ( 1.482939632545932307, -0.4281496062992124485, 0.4176697321401328655 ) ) ;
#8361=CARTESIAN_POINT ( 'NONE',  ( 0.8792650918635177559, -0.3690944881889765550, -0.3153832671262227771 ) ) ;
#8362=EDGE_LOOP ( 'NONE', ( #48731, #59177, #43741, #30607 ) ) ;
#8365=CARTESIAN_POINT ( 'NONE',  ( -0.2624671916010490880, 0.2306618581243847221, -0.2411417322834647770 ) ) ;
#8367=CARTESIAN_POINT ( 'NONE',  ( 1.496062992125984703, -0.1870078740157480879, -0.4822834645669291653 ) ) ;
#8368=CARTESIAN_POINT ( 'NONE',  ( 0.3215223097112867578, -0.3162353388693409650, -0.4822834645669289433 ) ) ;
#8369=CARTESIAN_POINT ( 'NONE',  ( -0.5249343832020990641, 0.1283753931104748280, 0.1820866141732283561 ) ) ;
#8370=CARTESIAN_POINT ( 'NONE',  ( 1.233595800524935227, 0.2306618581243847221, -0.2411417322834647770 ) ) ;
#8371=CARTESIAN_POINT ( 'NONE',  ( -1.017060367454067249, -0.05778040916215522460, 0.4822834645669289988 ) ) ;
#8372=CARTESIAN_POINT ( 'NONE',  ( 0.03280839895013198948, 0.2952755905511811885, 0.1292274648535926551 ) ) ;
#8373=CARTESIAN_POINT ( 'NONE',  ( 1.528871391076116026, -0.6692913385826773087, -0.1292274648535924053 ) ) ;
#8374=AXIS2_PLACEMENT_3D ( 'NONE', #61103, #54789, #80492 ) ;
#8375=CARTESIAN_POINT ( 'NONE',  ( 0.9448818897637802916, -0.1870078740157479769, 0.4822834645669291653 ) ) ;
#8376=CARTESIAN_POINT ( 'NONE',  ( 1.364829396325460076, 0.2306618581243848609, 0.2411417322834645549 ) ) ;
#8378=CARTESIAN_POINT ( 'NONE',  ( 0.1377952755905518800, 0.07958543189024071263, -0.2665933059059888421 ) ) ;
#8382=CARTESIAN_POINT ( 'NONE',  ( -0.3346456692913377662, -0.4536011799217367080, 0.2665933059059888421 ) ) ;
#8383=CARTESIAN_POINT ( 'NONE',  ( 8.195543980992789655E-16, -0.1870078740157480879, -0.4822834645669291653 ) ) ;
#8385=CARTESIAN_POINT ( 'NONE',  ( -0.3412073490813641308, -0.6046776061558807314, 0.2411417322834647770 ) ) ;
#8386=CARTESIAN_POINT ( 'NONE',  ( -0.3805774278215216522, -0.4281496062992127816, -0.4176697321401328100 ) ) ;
#8387=CARTESIAN_POINT ( 'NONE',  ( -0.7349081364829387342, -0.6046776061558807314, 0.2411417322834647770 ) ) ;
#8388=CARTESIAN_POINT ( 'NONE',  ( -1.043307086614172707, 0.1660481256975883668, -0.3530559997133364547 ) ) ;
#8389=CARTESIAN_POINT ( 'NONE',  ( 1.548556430446194954, 0.1283753931104746893, -0.1820866141732285504 ) ) ;
#8392=CARTESIAN_POINT ( 'NONE',  ( 0.2690288713910767848, -0.5511811023622048555, -0.09757992244046775898 ) ) ;
#8393=CARTESIAN_POINT ( 'NONE',  ( 0.6102362204724416372, 0.1660481256975883668, -0.3530559997133364547 ) ) ;
#8394=CARTESIAN_POINT ( 'NONE',  ( 0.4461942257217856311, 0.2306618581243847221, -0.2411417322834647770 ) ) ;
#8399=CARTESIAN_POINT ( 'NONE',  ( -0.4330708661417315697, 0.2952755905511811885, 0.000000000000000000 ) ) ;
#8402=CARTESIAN_POINT ( 'NONE',  ( -1.377952755905511140, -0.5511811023622047445, 6.969142054262312111E-17 ) ) ;
#8403=CARTESIAN_POINT ( 'NONE',  ( 0.8398950131233602345, 0.2306618581243847221, -0.2411417322834647770 ) ) ;
#8404=CARTESIAN_POINT ( 'NONE',  ( 0.8070866141732289112, -0.5400638737290845981, -0.3530559997133363437 ) ) ;
#8405=CARTESIAN_POINT ( 'NONE',  ( -0.3215223097112853146, -0.08942795157528024563, -0.3641732283464568787 ) ) ;
#8406=CARTESIAN_POINT ( 'NONE',  ( 0.4265091863517067039, -0.6692913385826773087, -0.1292274648535924053 ) ) ;
#8408=CARTESIAN_POINT ( 'NONE',  ( 0.02624671916010564918, -0.5023911411419708095, -0.1820866141732282451 ) ) ;
#8409=CARTESIAN_POINT ( 'NONE',  ( -0.1640419947506555343, -0.3162353388693405765, 0.4822834645669290543 ) ) ;
#8411=CARTESIAN_POINT ( 'NONE',  ( 1.607611548556431069, 0.1771653543307087630, 0.09757992244046791164 ) ) ;
#8412=CARTESIAN_POINT ( 'NONE',  ( 0.6036745406824153282, -0.5023911411419708095, 0.1820866141732285504 ) ) ;
#8413=CARTESIAN_POINT ( 'NONE',  ( 1.456692913385827515, -0.5511811023622047445, 6.969142054262312111E-17 ) ) ;
#8414=CARTESIAN_POINT ( 'NONE',  ( -0.7086614173228339419, -0.1870078740157480879, -0.4822834645669291653 ) ) ;
#8415=CARTESIAN_POINT ( 'NONE',  ( -0.6692913385826764205, 0.1771653543307087630, 0.000000000000000000 ) ) ;
#8417=CARTESIAN_POINT ( 'NONE',  ( -0.5971128608923877978, 0.2952755905511811885, 0.1292274648535926551 ) ) ;
#8418=CARTESIAN_POINT ( 'NONE',  ( -0.7677165354330699465, -0.5400638737290845981, -0.3530559997133363437 ) ) ;
#8419=CARTESIAN_POINT ( 'NONE',  ( 0.1443569553805781891, 0.05413385826771626580, -0.4176697321401330321 ) ) ;
#8423=CARTESIAN_POINT ( 'NONE',  ( 0.6430446194225729606, -0.3690944881889765550, -0.3153832671262227771 ) ) ;
#8424=CARTESIAN_POINT ( 'NONE',  ( 1.482939632545932307, 0.05413385826771626580, -0.4176697321401330321 ) ) ;
#8425=CARTESIAN_POINT ( 'NONE',  ( -1.128608923884513837, -0.5023911411419708095, 0.1820866141732285504 ) ) ;
#8426=CARTESIAN_POINT ( 'NONE',  ( -1.299212598425196097, -0.5511811023622047445, 6.969142054262312111E-17 ) ) ;
#8427=VECTOR ( 'NONE', #41525, 39.37007874015748143 ) ;
#8428=CARTESIAN_POINT ( 'NONE',  ( -0.7217847769028863381, 0.05413385826771626580, -0.4176697321401330321 ) ) ;
#8429=CARTESIAN_POINT ( 'NONE',  ( -0.05249343832020911260, 0.1283753931104748280, 0.1820866141732283561 ) ) ;
#8431=CARTESIAN_POINT ( 'NONE',  ( 0.9317585301837276734, -0.3690944881889763329, 0.3153832671262228327 ) ) ;
#8433=CARTESIAN_POINT ( 'NONE',  ( 0.2296587926509192634, -0.3162353388693405765, 0.4822834645669290543 ) ) ;
#8435=CARTESIAN_POINT ( 'NONE',  ( -0.6889763779527552368, -0.5400638737290845981, -0.3530559997133363437 ) ) ;
#8437=CARTESIAN_POINT ( 'NONE',  ( 1.489501312335958172, -0.08942795157528024563, -0.3641732283464568787 ) ) ;
#8438=CARTESIAN_POINT ( 'NONE',  ( 0.3412073490813655186, -0.6046776061558809534, -0.2411417322834644161 ) ) ;
#8439=CARTESIAN_POINT ( 'NONE',  ( -0.02624671916010428221, 0.2306618581243847221, -0.2411417322834647770 ) ) ;
#8440=CARTESIAN_POINT ( 'NONE',  ( -0.1574803149606292529, -0.1870078740157480601, -0.3641732283464567677 ) ) ;
#8441=CARTESIAN_POINT ( 'NONE',  ( 0.6036745406824154392, 0.1539470093639521697, -0.1968503937007875793 ) ) ;
#8442=CARTESIAN_POINT ( 'NONE',  ( -0.2493438320209966919, -0.3690944881889763329, 0.3153832671262228327 ) ) ;
#8443=CARTESIAN_POINT ( 'NONE',  ( 0.6692913385826778638, -0.6692913385826771977, 8.415575281601705876E-17 ) ) ;
#8444=CARTESIAN_POINT ( 'NONE',  ( -0.8595800524934373854, -0.2845877964562161244, -0.3641732283464567121 ) ) ;
#8446=CARTESIAN_POINT ( 'NONE',  ( -1.141732283464566011, 0.2952755905511811885, 0.000000000000000000 ) ) ;
#8447=CARTESIAN_POINT ( 'NONE',  ( -1.614173228346456712, 2.362204724409448620, -0.1372047244094478091 ) ) ;
#8449=CARTESIAN_POINT ( 'NONE',  ( -1.259842519685038686, -0.1870078740157479769, 0.3641732283464567677 ) ) ;
#8450=CARTESIAN_POINT ( 'NONE',  ( 0.05249343832021075018, 0.2306618581243847221, -0.2411417322834647770 ) ) ;
#8451=CARTESIAN_POINT ( 'NONE',  ( -1.469816272965878357, -0.6046776061558809534, -0.2411417322834644161 ) ) ;
#8452=CARTESIAN_POINT ( 'NONE',  ( -0.9580052493438311334, 0.05413385826771626580, -0.4176697321401330321 ) ) ;
#8454=EDGE_CURVE ( 'NONE', #24205, #6101, #33195, .T. ) ;
#8455=CARTESIAN_POINT ( 'NONE',  ( 1.587926509186352586, -0.4281496062992127816, -0.4176697321401328100 ) ) ;
#8456=CARTESIAN_POINT ( 'NONE',  ( 0.9842519685039375910, 0.2952755905511811885, 0.000000000000000000 ) ) ;
#8457=CARTESIAN_POINT ( 'NONE',  ( 0.8792650918635177559, 0.05413385826771666132, 0.4176697321401328100 ) ) ;
#8458=CARTESIAN_POINT ( 'NONE',  ( -0.3021879055830032357, 0.004960608223778823628, 0.3437734562760190182 ) ) ;
#8459=CARTESIAN_POINT ( 'NONE',  ( 1.496062992125984703, -0.1870078740157480879, -0.4822834645669291653 ) ) ;
#8461=CARTESIAN_POINT ( 'NONE',  ( -1.167979002624671470, -0.4281496062992127816, -0.4176697321401328100 ) ) ;
#8463=VERTEX_POINT ( 'NONE', #26457 ) ;
#8464=CARTESIAN_POINT ( 'NONE',  ( -0.7020997375328074108, -0.08942795157527998196, 0.3641732283464567121 ) ) ;
#8467=CARTESIAN_POINT ( 'NONE',  ( 0.4658792650918640033, -0.3162353388693405765, 0.4822834645669290543 ) ) ;
#8468=CARTESIAN_POINT ( 'NONE',  ( 0.1246719160104994284, -0.6692913385826771977, 0.1292274648535927661 ) ) ;
#8469=CARTESIAN_POINT ( 'NONE',  ( -0.6364829396325453192, -0.05778040916215560624, -0.4822834645669293319 ) ) ;
#8470=CARTESIAN_POINT ( 'NONE',  ( 1.371391076115485941, 0.2952755905511811885, 0.1292274648535926551 ) ) ;
#8471=AXIS2_PLACEMENT_3D ( 'NONE', #49421, #3159, #10725 ) ;
#8472=CARTESIAN_POINT ( 'NONE',  ( -1.056430446194224881, -0.5511811023622046335, 0.09757992244046803654 ) ) ;
#8473=CARTESIAN_POINT ( 'NONE',  ( -0.7443564587111910491, 2.208176010582810989, -0.5309055118110235227 ) ) ;
#8474=CARTESIAN_POINT ( 'NONE',  ( 0.6036745406824154392, 0.2306618581243847221, -0.2411417322834647770 ) ) ;
#8475=CARTESIAN_POINT ( 'NONE',  ( 0.5643044619422579178, -0.3690944881889765550, -0.3153832671262227771 ) ) ;
#8476=CARTESIAN_POINT ( 'NONE',  ( -0.5314960629921250401, 0.1660481256975885056, 0.3530559997133364547 ) ) ;
#8478=CARTESIAN_POINT ( 'NONE',  ( -1.187664041994749731, -0.3162353388693405765, 0.4822834645669290543 ) ) ;
#8480=CARTESIAN_POINT ( 'NONE',  ( 1.259842519685040019, -0.1870078740157480879, -0.4822834645669291653 ) ) ;
#8481=CARTESIAN_POINT ( 'NONE',  ( 1.272965879265092637, -0.3690944881889765550, -0.3153832671262227771 ) ) ;
#8482=ORIENTED_EDGE ( 'NONE', *, *, #49112, .T. ) ;
#8484=CARTESIAN_POINT ( 'NONE',  ( 0.09842519685039434474, 0.1660481256975885056, 0.3530559997133364547 ) ) ;
#8486=CARTESIAN_POINT ( 'NONE',  ( 0.8727034120734912248, -0.2845877964562161244, -0.3641732283464567121 ) ) ;
#8487=CARTESIAN_POINT ( 'NONE',  ( -1.017060367454067249, -0.3162353388693409650, -0.4822834645669289433 ) ) ;
#8488=CARTESIAN_POINT ( 'NONE',  ( 1.122047244094488860, 0.1660481256975885056, 0.3530559997133364547 ) ) ;
#8489=CARTESIAN_POINT ( 'NONE',  ( 0.8267716535433077274, 0.2952755905511811885, 0.000000000000000000 ) ) ;
#8492=CARTESIAN_POINT ( 'NONE',  ( 0.1181102362204730916, -0.6692913385826771977, 8.415575281601705876E-17 ) ) ;
#8493=CARTESIAN_POINT ( 'NONE',  ( -0.5052493438320203589, 0.2952755905511810774, -0.1292274648535930714 ) ) ;
#8495=CARTESIAN_POINT ( 'NONE',  ( -1.364829396325458521, 0.2306618581243847221, -0.2411417322834647770 ) ) ;
#8496=CARTESIAN_POINT ( 'NONE',  ( -0.5183727034120726440, 0.2952755905511811885, 0.1292274648535926551 ) ) ;
#8498=CARTESIAN_POINT ( 'NONE',  ( -0.4986876640419939388, 0.1283753931104746893, -0.1820866141732285504 ) ) ;
#8500=CARTESIAN_POINT ( 'NONE',  ( 1.476377952755906442, -0.5400638737290844871, 0.3530559997133364547 ) ) ;
#8501=CARTESIAN_POINT ( 'NONE',  ( -0.5249343832020990641, -0.6046776061558809534, -0.2411417322834644161 ) ) ;
#8503=CARTESIAN_POINT ( 'NONE',  ( 0.5314960629921264834, 0.1660481256975883668, -0.3530559997133364547 ) ) ;
#8506=CARTESIAN_POINT ( 'NONE',  ( -0.3346456692913377662, 0.1660481256975883668, -0.3530559997133364547 ) ) ;
#8507=CARTESIAN_POINT ( 'NONE',  ( 1.128608923884515169, -0.5023911411419708095, -0.1820866141732282451 ) ) ;
#8510=CARTESIAN_POINT ( 'NONE',  ( 1.174540682414699111, -0.2845877964562159024, 0.3641732283464567677 ) ) ;
#8511=CARTESIAN_POINT ( 'NONE',  ( 1.325459317585302665, 0.05413385826771626580, -0.4176697321401330321 ) ) ;
#8513=CARTESIAN_POINT ( 'NONE',  ( -0.2559055118110230564, 0.1660481256975883668, -0.3530559997133364547 ) ) ;
#8514=CARTESIAN_POINT ( 'NONE',  ( -1.587926509186350810, 0.05413385826771626580, -0.4176697321401330321 ) ) ;
#8515=CARTESIAN_POINT ( 'NONE',  ( -1.581364829396324945, -0.3162353388693405765, 0.4822834645669290543 ) ) ;
#8516=CARTESIAN_POINT ( 'NONE',  ( -0.3149606299212590610, -0.1870078740157479769, 0.4822834645669291653 ) ) ;
#8518=CARTESIAN_POINT ( 'NONE',  ( 1.115485564304462551, -0.4281496062992127816, -0.4176697321401328100 ) ) ;
#8519=CARTESIAN_POINT ( 'NONE',  ( 0.4724409448818904789, -0.1870078740157479769, 0.4822834645669291653 ) ) ;
#8520=CARTESIAN_POINT ( 'NONE',  ( 0.6364829396325465405, -0.2845877964562161244, -0.3641732283464567121 ) ) ;
#8521=CARTESIAN_POINT ( 'NONE',  ( 0.3937007874015754361, -0.1870078740157479769, 0.3641732283464567677 ) ) ;
#8522=CARTESIAN_POINT ( 'NONE',  ( -1.620734908136482577, 0.2952755905511811885, 0.1292274648535926551 ) ) ;
#8525=CARTESIAN_POINT ( 'NONE',  ( 0.7283464566929143125, 0.1660481256975885056, 0.3530559997133364547 ) ) ;
#8528=CARTESIAN_POINT ( 'NONE',  ( -0.7974104941589342799, -2.567464376874931580E-15, -0.4445507791589072832 ) ) ;
#8529=CARTESIAN_POINT ( 'NONE',  ( -0.07217847769028813698, -0.2845877964562161244, -0.3641732283464567121 ) ) ;
#8530=ADVANCED_FACE ( 'NONE', ( #52109 ), #6383, .F. ) ;
#8531=CARTESIAN_POINT ( 'NONE',  ( 0.3937007874015754361, -0.1870078740157479769, 0.4822834645669291653 ) ) ;
#8532=CARTESIAN_POINT ( 'NONE',  ( 1.220472440944882608, 0.1771653543307087630, 0.000000000000000000 ) ) ;
#8533=CARTESIAN_POINT ( 'NONE',  ( -0.7808398950131225646, -0.08942795157527998196, 0.3641732283464567121 ) ) ;
#8534=CARTESIAN_POINT ( 'NONE',  ( -0.9251968503937002541, 0.1660481256975885056, 0.3530559997133364547 ) ) ;
#8535=CONICAL_SURFACE ( 'NONE', #74443, 3.543307086614174484, 0.8726646259971734265 ) ;
#8536=CARTESIAN_POINT ( 'NONE',  ( -1.607611548556429737, -0.6692913385826771977, 0.1292274648535927661 ) ) ;
#8537=CARTESIAN_POINT ( 'NONE',  ( 0.4724409448818904789, -0.1870078740157480879, -0.4822834645669291653 ) ) ;
#8538=CARTESIAN_POINT ( 'NONE',  ( 1.430446194225722500, -0.4281496062992127816, -0.4176697321401328100 ) ) ;
#8539=EDGE_CURVE ( 'NONE', #9025, #20402, #6833, .T. ) ;
#8541=CARTESIAN_POINT ( 'NONE',  ( 0.4986876640419954376, 0.2306618581243848609, 0.2411417322834645549 ) ) ;
#8543=CARTESIAN_POINT ( 'NONE',  ( 1.673228346456693494, 0.1660481256975885056, 0.3530559997133364547 ) ) ;
#8544=CARTESIAN_POINT ( 'NONE',  ( 1.384514435695538559, 0.2952755905511810774, -0.1292274648535930714 ) ) ;
#8545=CARTESIAN_POINT ( 'NONE',  ( -1.561679790026246017, -0.004921259842519576551, 0.3153832671262227771 ) ) ;
#8546=CARTESIAN_POINT ( 'NONE',  ( 1.213910761154856299, 0.1771653543307087630, 0.09757992244046791164 ) ) ;
#8547=CARTESIAN_POINT ( 'NONE',  ( -1.332020997375327642, -0.08942795157527998196, 0.3641732283464567121 ) ) ;
#8548=CARTESIAN_POINT ( 'NONE',  ( -0.8005249343832011588, -0.004921259842519870586, -0.3153832671262229437 ) ) ;
#8549=CARTESIAN_POINT ( 'NONE',  ( 0.4265091863517067039, -0.5511811023622048555, -0.09757992244046775898 ) ) ;
#8551=CARTESIAN_POINT ( 'NONE',  ( -0.07874015748031421014, -0.1870078740157479769, 0.4822834645669291653 ) ) ;
#8552=CARTESIAN_POINT ( 'NONE',  ( 0.9580052493438326877, 0.05413385826771666132, 0.4176697321401328100 ) ) ;
#8553=CARTESIAN_POINT ( 'NONE',  ( 0.1312335958005257930, 0.2306618581243847221, -0.2411417322834647770 ) ) ;
#8554=CARTESIAN_POINT ( 'NONE',  ( 0.05249343832021075018, 0.1283753931104746893, -0.1820866141732285504 ) ) ;
#8555=CARTESIAN_POINT ( 'NONE',  ( 1.364829396325459854, -0.6046776061558809534, -0.2411417322834644161 ) ) ;
#8556=DIRECTION ( 'NONE',  ( -3.096699300667737957E-16, 1.000000000000000000, -0.000000000000000000 ) ) ;
#8557=CARTESIAN_POINT ( 'NONE',  ( -0.9711286089238838626, -0.6046776061558807314, 0.2411417322834647770 ) ) ;
#8559=DIRECTION ( 'NONE',  ( -0.000000000000000000, 1.000000000000000000, -0.000000000000000000 ) ) ;
#8560=CARTESIAN_POINT ( 'NONE',  ( -0.6889763779527552368, 0.1660481256975885056, 0.3530559997133364547 ) ) ;
#8561=CARTESIAN_POINT ( 'NONE',  ( 0.006561679790026889343, -0.05778040916215522460, 0.4822834645669289988 ) ) ;
#8567=CARTESIAN_POINT ( 'NONE',  ( -1.259842519685038686, -0.1870078740157479769, 0.3641732283464567677 ) ) ;
#8569=CARTESIAN_POINT ( 'NONE',  ( 1.594488188976378673, 0.07958543189024085140, 0.2665933059059887866 ) ) ;
#8571=CARTESIAN_POINT ( 'NONE',  ( 0.3608923884514443348, -0.6692913385826771977, 0.1292274648535927661 ) ) ;
#8572=CARTESIAN_POINT ( 'NONE',  ( -0.4461942257217840213, 0.1283753931104748280, 0.1820866141732283561 ) ) ;
#8573=CARTESIAN_POINT ( 'NONE',  ( 0.7152230971128614723, -0.3162353388693409650, -0.4822834645669289433 ) ) ;
#8574=CARTESIAN_POINT ( 'NONE',  ( 0.4461942257217855201, -0.6046776061558807314, 0.2411417322834647770 ) ) ;
#8577=CARTESIAN_POINT ( 'NONE',  ( 1.430446194225722500, -0.4281496062992127816, -0.4176697321401328100 ) ) ;
#8578=CARTESIAN_POINT ( 'NONE',  ( -0.1377952755905504645, 0.1660481256975885056, 0.3530559997133364547 ) ) ;
#8579=EDGE_CURVE ( 'NONE', #78909, #25966, #72070, .T. ) ;
#8580=CARTESIAN_POINT ( 'NONE',  ( 1.423884514435696191, -0.05778040916215522460, 0.4822834645669289988 ) ) ;
#8581=CARTESIAN_POINT ( 'NONE',  ( 0.8727034120734913358, -0.05778040916215522460, 0.4822834645669289988 ) ) ;
#8583=CARTESIAN_POINT ( 'NONE',  ( 0.08530183727034192087, -0.3162353388693409650, -0.4822834645669289433 ) ) ;
#8584=CARTESIAN_POINT ( 'NONE',  ( 0.8070866141732289112, -0.5400638737290845981, -0.3530559997133363437 ) ) ;
#8585=CARTESIAN_POINT ( 'NONE',  ( 0.01312335958005323398, -0.4281496062992127816, -0.4176697321401328100 ) ) ;
#8586=CIRCLE ( 'NONE', #61027, 3.543307086614173596 ) ;
#8587=CARTESIAN_POINT ( 'NONE',  ( 0.6036745406824154392, 0.1283753931104746893, -0.1820866141732285504 ) ) ;
#8588=CARTESIAN_POINT ( 'NONE',  ( -1.200787401574802349, 0.1660481256975883668, -0.3530559997133364547 ) ) ;
#8589=CARTESIAN_POINT ( 'NONE',  ( -1.213910761154854745, 0.2952755905511810774, -0.1292274648535930714 ) ) ;
#8590=CARTESIAN_POINT ( 'NONE',  ( 0.8989501312335963501, -0.6692913385826773087, -0.1292274648535924053 ) ) ;
#8596=CARTESIAN_POINT ( 'NONE',  ( 1.062992125984252745, 0.2952755905511811885, 0.000000000000000000 ) ) ;
#8597=CARTESIAN_POINT ( 'NONE',  ( 0.3346456692913390985, 0.07958543189024085140, 0.2665933059059887866 ) ) ;
#8603=CARTESIAN_POINT ( 'NONE',  ( 1.207349081364829990, -0.6046776061558809534, -0.2411417322834644161 ) ) ;
#8605=CARTESIAN_POINT ( 'NONE',  ( -0.4068241469816267775, 0.05413385826771626580, -0.4176697321401330321 ) ) ;
#8606=CARTESIAN_POINT ( 'NONE',  ( 1.030183727034121421, -0.3162353388693409650, -0.4822834645669289433 ) ) ;
#8608=FACE_OUTER_BOUND ( 'NONE', #10442, .T. ) ;
#8611=CARTESIAN_POINT ( 'NONE',  ( 1.692913385826772421, 0.1771653543307087630, 0.000000000000000000 ) ) ;
#8613=CARTESIAN_POINT ( 'NONE',  ( -1.509186351706035767, -0.3690944881889763329, 0.3153832671262228327 ) ) ;
#8614=( BOUNDED_CURVE ( )  B_SPLINE_CURVE ( 2, ( #72912, #15264, #71249, #20318, #1796, #27458, #13595, #53117, #79246, #976, #1387, #27040, #66605 ),
 .UNSPECIFIED., .F., .F. ) 
 B_SPLINE_CURVE_WITH_KNOTS ( ( 3, 2, 2, 2, 2, 2, 3 ),
 ( 0.2187856400893463116, 0.2196969696969696961, 0.2234848484848484806, 0.2272727272727272652, 0.2310606060606060497, 0.2348484848484848619, 0.2357598144561083298 ),
 .UNSPECIFIED. ) 
 CURVE ( )  GEOMETRIC_REPRESENTATION_ITEM ( )  RATIONAL_B_SPLINE_CURVE ( ( 0.9875488213027527884, 0.9918020599134683701, 1.000000000000000000, 0.9659258262890683122, 1.000000000000000000, 0.9659258262890683122, 1.000000000000000000, 0.9659258262890683122, 1.000000000000000000, 0.9659258262890683122, 1.000000000000000000, 0.9918020599134675930, 0.9875488213027519002 ) ) 
 REPRESENTATION_ITEM ( '' )  );
#8615=CARTESIAN_POINT ( 'NONE',  ( -1.653543307086613234, -0.1870078740157479769, 0.4822834645669291653 ) ) ;
#8616=CARTESIAN_POINT ( 'NONE',  ( 0.6561679790026253567, -0.6046776061558809534, -0.2411417322834644161 ) ) ;
#8620=CARTESIAN_POINT ( 'NONE',  ( -0.8398950131233589023, -0.5023911411419708095, -0.1820866141732282451 ) ) ;
#8621=CARTESIAN_POINT ( 'NONE',  ( 0.8005249343832028242, -0.4281496062992127816, -0.4176697321401328100 ) ) ;
#8622=CARTESIAN_POINT ( 'NONE',  ( -1.463254593175852492, -0.6692913385826773087, -0.1292274648535924053 ) ) ;
#8624=CARTESIAN_POINT ( 'NONE',  ( -0.8792650918635160906, -0.004921259842519870586, -0.3153832671262229437 ) ) ;
#8625=CARTESIAN_POINT ( 'NONE',  ( -1.548556430446193399, -0.5023911411419708095, -0.1820866141732282451 ) ) ;
#8627=CARTESIAN_POINT ( 'NONE',  ( 0.6299212598425204535, -0.1870078740157479769, 0.4822834645669291653 ) ) ;
#8628=CARTESIAN_POINT ( 'NONE',  ( -1.082677165354329896, -0.4536011799217368745, -0.2665933059059886201 ) ) ;
#8629=CARTESIAN_POINT ( 'NONE',  ( -0.2165354330708654795, -0.4536011799217368745, -0.2665933059059886201 ) ) ;
#8630=CARTESIAN_POINT ( 'NONE',  ( -0.2362204724409442680, -0.1870078740157480879, -0.4822834645669291653 ) ) ;
#8631=CARTESIAN_POINT ( 'NONE',  ( 1.594488188976378673, -0.5400638737290845981, -0.3530559997133363437 ) ) ;
#8633=CARTESIAN_POINT ( 'NONE',  ( 0.8202099737532813073, 0.2952755905511811885, 0.1292274648535926551 ) ) ;
#8634=DIRECTION ( 'NONE',  ( -1.000000000000000000, 0.000000000000000000, 0.000000000000000000 ) ) ;
#8636=CARTESIAN_POINT ( 'NONE',  ( -0.6299212598425188991, -0.1870078740157479769, 0.4822834645669291653 ) ) ;
#8637=CARTESIAN_POINT ( 'NONE',  ( -0.07217847769028813698, -0.2845877964562161244, -0.3641732283464567121 ) ) ;
#8638=CARTESIAN_POINT ( 'NONE',  ( -1.272965879265091305, 0.05413385826771626580, -0.4176697321401330321 ) ) ;
#8639=CARTESIAN_POINT ( 'NONE',  ( 0.4593175853018380828, -0.004921259842519870586, -0.3153832671262229437 ) ) ;
#8640=CARTESIAN_POINT ( 'NONE',  ( -0.7086614173228339419, -0.1870078740157480601, -0.3641732283464567677 ) ) ;
#8641=CARTESIAN_POINT ( 'NONE',  ( -1.135170603674539924, -0.6692913385826771977, 0.1292274648535927661 ) ) ;
#8642=CARTESIAN_POINT ( 'NONE',  ( -1.646981627296586703, -0.3162353388693409650, -0.4822834645669289433 ) ) ;
#8643=CARTESIAN_POINT ( 'NONE',  ( 1.233595800524935227, 0.2306618581243847221, -0.2411417322834647770 ) ) ;
#8645=CARTESIAN_POINT ( 'NONE',  ( 0.7349081364829403995, 0.1283753931104748280, 0.1820866141732283561 ) ) ;
#8646=VECTOR ( 'NONE', #43185, 39.37007874015748854 ) ;
#8647=CARTESIAN_POINT ( 'NONE',  ( 0.5052493438320218022, -0.6692913385826773087, -0.1292274648535924053 ) ) ;
#8648=CARTESIAN_POINT ( 'NONE',  ( -1.633858267716534529, 0.1660481256975885056, 0.3530559997133364547 ) ) ;
#8649=CARTESIAN_POINT ( 'NONE',  ( 1.541994750656168645, -0.5511811023622046335, 0.09757992244046803654 ) ) ;
#8650=VERTEX_POINT ( 'NONE', #19889 ) ;
#8652=CARTESIAN_POINT ( 'NONE',  ( -1.200787401574802349, -0.4536011799217367080, 0.2665933059059888421 ) ) ;
#8653=CARTESIAN_POINT ( 'NONE',  ( -0.3543307086614165824, 0.2952755905511811885, 0.000000000000000000 ) ) ;
#8654=CARTESIAN_POINT ( 'NONE',  ( 0.3412073490813655186, 0.2306618581243848609, 0.2411417322834645549 ) ) ;
#8655=CARTESIAN_POINT ( 'NONE',  ( -1.502624671916009680, -0.08942795157528024563, -0.3641732283464568787 ) ) ;
#8657=CARTESIAN_POINT ( 'NONE',  ( -1.489501312335957062, -0.3162353388693409650, -0.4822834645669289433 ) ) ;
#8658=CARTESIAN_POINT ( 'NONE',  ( 0.3346456692913393205, -0.5400638737290845981, -0.3530559997133363437 ) ) ;
#8659=CARTESIAN_POINT ( 'NONE',  ( 0.1049868766404206816, 0.2306618581243848609, 0.2411417322834645549 ) ) ;
#8660=CARTESIAN_POINT ( 'NONE',  ( 1.181102362204724976, -0.1870078740157480879, -0.4822834645669291653 ) ) ;
#8666=CARTESIAN_POINT ( 'NONE',  ( -0.2362204724409442680, -0.1870078740157480601, -0.3641732283464567677 ) ) ;
#8667=CARTESIAN_POINT ( 'NONE',  ( -0.3674540682414692561, -0.6046776061558809534, -0.2411417322834644161 ) ) ;
#8668=CARTESIAN_POINT ( 'NONE',  ( 1.030183727034121421, -0.3162353388693409650, -0.4822834645669289433 ) ) ;
#8670=CARTESIAN_POINT ( 'NONE',  ( -0.08530183727034056085, -0.2845877964562159024, 0.3641732283464567677 ) ) ;
#8671=CARTESIAN_POINT ( 'NONE',  ( -1.207349081364828436, -0.6046776061558807314, 0.2411417322834647770 ) ) ;
#8672=CARTESIAN_POINT ( 'NONE',  ( -1.640419947506561060, 0.05413385826771666132, 0.4176697321401328100 ) ) ;
#8675=ORIENTED_EDGE ( 'NONE', *, *, #29379, .T. ) ;
#8678=CARTESIAN_POINT ( 'NONE',  ( 1.259842519685040019, -0.1870078740157479769, 0.4822834645669291653 ) ) ;
#8679=CARTESIAN_POINT ( 'NONE',  ( -1.699475065616797398, 0.2952755905511811885, 0.1292274648535926551 ) ) ;
#8680=CARTESIAN_POINT ( 'NONE',  ( -1.364829396325458521, -0.5023911411419708095, 0.1820866141732285504 ) ) ;
#8681=CARTESIAN_POINT ( 'NONE',  ( -1.272965879265091305, 0.05413385826771626580, -0.4176697321401330321 ) ) ;
#8683=CARTESIAN_POINT ( 'NONE',  ( 1.220472440944882386, -0.1870078740157480046, 1.254653134982923898E-17 ) ) ;
#8684=CARTESIAN_POINT ( 'NONE',  ( 1.312335958005250269, -0.6046776061558807314, 0.2411417322834647770 ) ) ;
#8686=CARTESIAN_POINT ( 'NONE',  ( -0.2427821522309703550, -0.05778040916215560624, -0.4822834645669293319 ) ) ;
#8687=CARTESIAN_POINT ( 'NONE',  ( -0.1509186351706028884, -0.05778040916215522460, 0.4822834645669289988 ) ) ;
#8688=CARTESIAN_POINT ( 'NONE',  ( -1.076115485564303809, -0.6046776061558809534, -0.2411417322834644161 ) ) ;
#8690=CARTESIAN_POINT ( 'NONE',  ( 0.4199475065616803948, -0.6046776061558809534, -0.2411417322834644161 ) ) ;
#8692=CARTESIAN_POINT ( 'NONE',  ( -1.148293963254592542, 0.1771653543307087630, 0.09757992244046791164 ) ) ;
#8693=ORIENTED_EDGE ( 'NONE', *, *, #22304, .F. ) ;
#8696=CARTESIAN_POINT ( 'NONE',  ( -1.614173228346456712, 2.401574803149606474, -0.1372047244094478091 ) ) ;
#8697=CARTESIAN_POINT ( 'NONE',  ( -1.233595800524933894, 0.2306618581243848609, 0.2411417322834645549 ) ) ;
#8698=CARTESIAN_POINT ( 'NONE',  ( -1.253280839895012377, -0.3162353388693409650, -0.4822834645669289433 ) ) ;
#8700=CARTESIAN_POINT ( 'NONE',  ( -1.528871391076114250, 0.2952755905511810774, -0.1292274648535930714 ) ) ;
#8701=DIRECTION ( 'NONE',  ( 0.5931762764594944448, -9.392846415265724076E-15, -0.8050726085550603539 ) ) ;
#8703=CARTESIAN_POINT ( 'NONE',  ( -0.3280839895013117347, 0.05413385826771626580, -0.4176697321401330321 ) ) ;
#8705=CARTESIAN_POINT ( 'NONE',  ( 0.3018372703412079971, -0.004921259842519870586, -0.3153832671262229437 ) ) ;
#8706=CARTESIAN_POINT ( 'NONE',  ( -0.6889763779527552368, -0.4536011799217368745, -0.2665933059059886201 ) ) ;
#8707=CARTESIAN_POINT ( 'NONE',  ( -1.351706036745406347, -0.4281496062992124485, 0.4176697321401328655 ) ) ;
#8708=CARTESIAN_POINT ( 'NONE',  ( 1.049868766404200127, -0.6046776061558809534, -0.2411417322834644161 ) ) ;
#8709=CARTESIAN_POINT ( 'NONE',  ( -0.7349081364829387342, -0.6046776061558807314, 0.2411417322834647770 ) ) ;
#8711=ORIENTED_EDGE ( 'NONE', *, *, #51054, .T. ) ;
#8712=CARTESIAN_POINT ( 'NONE',  ( -1.535433070866141225, -0.6692913385826771977, 8.415575281601705876E-17 ) ) ;
#8713=CARTESIAN_POINT ( 'NONE',  ( -1.364829396325458521, 0.1283753931104746893, -0.1820866141732285504 ) ) ;
#8714=CARTESIAN_POINT ( 'NONE',  ( -1.646981627296586703, -0.3162353388693409650, -0.4822834645669289433 ) ) ;
#8719=CARTESIAN_POINT ( 'NONE',  ( -0.2559055118110227234, -0.5400638737290844871, 0.3530559997133364547 ) ) ;
#8720=CARTESIAN_POINT ( 'NONE',  ( -1.450131233595799651, 0.1771653543307087075, -0.09757992244046823083 ) ) ;
#8722=CARTESIAN_POINT ( 'NONE',  ( -1.548556430446193399, 0.2306618581243848609, 0.2411417322834645549 ) ) ;
#8724=CARTESIAN_POINT ( 'NONE',  ( -1.299212598425196097, -0.6692913385826771977, 8.415575281601705876E-17 ) ) ;
#8725=CARTESIAN_POINT ( 'NONE',  ( -0.4986876640419942164, -0.6046776061558807314, 0.2411417322834647770 ) ) ;
#8728=CARTESIAN_POINT ( 'NONE',  ( 0.5511811023622054106, -0.1870078740157480601, -0.3641732283464567677 ) ) ;
#8730=CARTESIAN_POINT ( 'NONE',  ( 0.3937007874015754361, -0.1870078740157479769, 0.3641732283464567677 ) ) ;
#8731=CARTESIAN_POINT ( 'NONE',  ( 0.8136482939632553313, 0.1283753931104748280, 0.1820866141732283561 ) ) ;
#8732=CARTESIAN_POINT ( 'NONE',  ( 0.8464566929133865436, 0.1660481256975883668, -0.3530559997133364547 ) ) ;
#8733=CARTESIAN_POINT ( 'NONE',  ( -0.4068241469816264999, -0.3690944881889763329, 0.3153832671262228327 ) ) ;
#8735=CARTESIAN_POINT ( 'NONE',  ( -1.338582677165353729, -0.1870078740157479769, 0.4822834645669291653 ) ) ;
#8736=CARTESIAN_POINT ( 'NONE',  ( -0.2362204724409442680, -0.1870078740157480601, -0.3641732283464567677 ) ) ;
#8737=CARTESIAN_POINT ( 'NONE',  ( -1.154855643044618851, 0.1283753931104748280, 0.1820866141732283561 ) ) ;
#8739=CARTESIAN_POINT ( 'NONE',  ( -0.7349081364829387342, -0.5023911411419708095, 0.1820866141732285504 ) ) ;
#8741=CARTESIAN_POINT ( 'NONE',  ( -0.1902887139107604098, 0.2952755905511810774, -0.1292274648535930714 ) ) ;
#8743=CARTESIAN_POINT ( 'NONE',  ( 0.4855643044619428750, -0.004921259842519576551, 0.3153832671262227771 ) ) ;
#8744=CARTESIAN_POINT ( 'NONE',  ( -0.09186351706036689768, -0.004921259842519870586, -0.3153832671262229437 ) ) ;
#8745=CARTESIAN_POINT ( 'NONE',  ( -0.2952755905511803003, -0.5400638737290845981, -0.3530559997133363437 ) ) ;
#8747=CARTESIAN_POINT ( 'NONE',  ( -0.9120734908136475250, -0.5511811023622048555, -0.09757992244046775898 ) ) ;
#8749=CARTESIAN_POINT ( 'NONE',  ( 0.5708661417322842269, 0.1660481256975885056, 0.3530559997133364547 ) ) ;
#8751=CARTESIAN_POINT ( 'NONE',  ( 1.410761154855643795, -0.3162353388693405765, 0.4822834645669290543 ) ) ;
#8752=CARTESIAN_POINT ( 'NONE',  ( -0.2624671916010490880, 0.1283753931104746893, -0.1820866141732285504 ) ) ;
#8753=CARTESIAN_POINT ( 'NONE',  ( -1.574803149606298192, -0.1870078740157480879, -0.4822834645669291653 ) ) ;
#8754=CARTESIAN_POINT ( 'NONE',  ( 1.509186351706037543, 0.05413385826771666132, 0.4176697321401328100 ) ) ;
#8755=CARTESIAN_POINT ( 'NONE',  ( 1.358267716535433323, 0.1660481256975885056, 0.3530559997133364547 ) ) ;
#8756=CARTESIAN_POINT ( 'NONE',  ( -0.5774278215223089816, 0.1283753931104746893, -0.1820866141732285504 ) ) ;
#8757=CARTESIAN_POINT ( 'NONE',  ( -1.614173228346457378, 1.881821177735609085, 0.1372047244094476981 ) ) ;
#8758=CARTESIAN_POINT ( 'NONE',  ( 0.8923884514435701520, -0.6046776061558809534, -0.2411417322834644161 ) ) ;
#8762=CARTESIAN_POINT ( 'NONE',  ( 1.548556430446194954, -0.5023911411419708095, 0.1820866141732285504 ) ) ;
#8763=CARTESIAN_POINT ( 'NONE',  ( -1.345144356955379816, -0.05778040916215560624, -0.4822834645669293319 ) ) ;
#8764=CARTESIAN_POINT ( 'NONE',  ( 1.272965879265092637, 0.05413385826771666132, 0.4176697321401328100 ) ) ;
#8766=CARTESIAN_POINT ( 'NONE',  ( 1.089238845144357759, -0.004921259842519870586, -0.3153832671262229437 ) ) ;
#8768=CARTESIAN_POINT ( 'NONE',  ( -0.02624671916010428221, 0.2306618581243847221, -0.2411417322834647770 ) ) ;
#8769=CARTESIAN_POINT ( 'NONE',  ( -0.1968503937007867743, 0.2952755905511811885, 0.000000000000000000 ) ) ;
#8770=CARTESIAN_POINT ( 'NONE',  ( 1.614173228346457378, -0.6692913385826771977, 8.415575281601705876E-17 ) ) ;
#8772=CARTESIAN_POINT ( 'NONE',  ( 0.2624671916010504757, -0.5023911411419708095, -0.1820866141732282451 ) ) ;
#8776=ORIENTED_EDGE ( 'NONE', *, *, #34523, .T. ) ;
#8777=CARTESIAN_POINT ( 'NONE',  ( -0.3083989501312330295, -0.05778040916215522460, 0.4822834645669289988 ) ) ;
#8778=CARTESIAN_POINT ( 'NONE',  ( 1.332020997375328974, -0.05778040916215560624, -0.4822834645669293319 ) ) ;
#8779=CARTESIAN_POINT ( 'NONE',  ( 0.08530183727034192087, -0.05778040916215522460, 0.4822834645669289988 ) ) ;
#8780=CARTESIAN_POINT ( 'NONE',  ( -0.2952755905511803003, -0.4536011799217368745, -0.2665933059059886201 ) ) ;
#8781=CARTESIAN_POINT ( 'NONE',  ( 1.161417322834646493, -0.5400638737290844871, 0.3530559997133364547 ) ) ;
#8782=CARTESIAN_POINT ( 'NONE',  ( -0.7414698162729651543, -0.6692913385826771977, 0.1292274648535927661 ) ) ;
#8783=CARTESIAN_POINT ( 'NONE',  ( 0.1246719160104994284, -0.6692913385826771977, 0.1292274648535927661 ) ) ;
#8784=CARTESIAN_POINT ( 'NONE',  ( -0.9251968503937002541, 0.1660481256975885056, 0.3530559997133364547 ) ) ;
#8785=CARTESIAN_POINT ( 'NONE',  ( 1.371391076115485719, -0.6692913385826773087, -0.1292274648535924053 ) ) ;
#8786=CARTESIAN_POINT ( 'NONE',  ( 0.9055118110236227702, -0.6692913385826771977, 8.415575281601705876E-17 ) ) ;
#8787=CARTESIAN_POINT ( 'NONE',  ( 1.279527559055118724, -0.5400638737290845981, -0.3530559997133363437 ) ) ;
#8789=CARTESIAN_POINT ( 'NONE',  ( 0.1115485564304470323, 0.1771653543307087630, 0.09757992244046791164 ) ) ;
#8792=VERTEX_POINT ( 'NONE', #51849 ) ;
#8793=CARTESIAN_POINT ( 'NONE',  ( -0.7545931758530177724, 0.1771653543307087630, 0.09757992244046791164 ) ) ;
#8794=CARTESIAN_POINT ( 'NONE',  ( -0.06561679790026180015, 0.05413385826771666132, 0.4176697321401328100 ) ) ;
#8796=CARTESIAN_POINT ( 'NONE',  ( -0.3871391076115479057, -0.3162353388693409650, -0.4822834645669289433 ) ) ;
#8797=CARTESIAN_POINT ( 'NONE',  ( -0.5314960629921254842, -0.5400638737290845981, -0.3530559997133363437 ) ) ;
#8798=CARTESIAN_POINT ( 'NONE',  ( -0.6824146981627288167, 0.2306618581243848609, 0.2411417322834645549 ) ) ;
#8799=CARTESIAN_POINT ( 'NONE',  ( -1.371391076115484831, 0.2952755905511810774, -0.1292274648535930714 ) ) ;
#8800=CARTESIAN_POINT ( 'NONE',  ( 1.456692913385827515, -0.5511811023622047445, 6.969142054262312111E-17 ) ) ;
#8803=CARTESIAN_POINT ( 'NONE',  ( 0.3083989501312343062, -0.2845877964562159024, 0.3641732283464567677 ) ) ;
#8804=CARTESIAN_POINT ( 'NONE',  ( -0.06561679790026180015, 0.05413385826771666132, 0.4176697321401328100 ) ) ;
#8805=CARTESIAN_POINT ( 'NONE',  ( 0.1902887139107617975, -0.6692913385826773087, -0.1292274648535924053 ) ) ;
#8808=CARTESIAN_POINT ( 'NONE',  ( -0.6175017169405814244, 0.000000000000000000, 0.3464511005275205946 ) ) ;
#8811=CARTESIAN_POINT ( 'NONE',  ( -0.4199475065616791736, 0.2306618581243847221, -0.2411417322834647770 ) ) ;
#8814=CARTESIAN_POINT ( 'NONE',  ( -1.640419947506561060, -0.004921259842519576551, 0.3153832671262227771 ) ) ;
#8815=CARTESIAN_POINT ( 'NONE',  ( 1.017060367454068581, -0.05778040916215560624, -0.4822834645669293319 ) ) ;
#8816=CARTESIAN_POINT ( 'NONE',  ( 0.7808398950131241190, -0.05778040916215560624, -0.4822834645669293319 ) ) ;
#8817=CARTESIAN_POINT ( 'NONE',  ( -0.2165354330708654795, 0.07958543189024085140, 0.2665933059059887866 ) ) ;
#8818=CARTESIAN_POINT ( 'NONE',  ( -0.1181102362204717315, 0.2952755905511811885, 0.000000000000000000 ) ) ;
#8820=CARTESIAN_POINT ( 'NONE',  ( -0.1377952755905504645, -0.4536011799217368745, -0.2665933059059886201 ) ) ;
#8821=CARTESIAN_POINT ( 'NONE',  ( -0.3674540682414692561, -0.6046776061558809534, -0.2411417322834644161 ) ) ;
#8823=CARTESIAN_POINT ( 'NONE',  ( -1.673228346456691717, 0.1660481256975883668, -0.3530559997133364547 ) ) ;
#8824=CARTESIAN_POINT ( 'NONE',  ( 0.2362204724409456558, -0.1870078740157480601, -0.3641732283464567677 ) ) ;
#8825=CARTESIAN_POINT ( 'NONE',  ( 1.673228346456693494, 0.07958543189024085140, 0.2665933059059887866 ) ) ;
#8826=CARTESIAN_POINT ( 'NONE',  ( -1.010498687664041384, -0.4281496062992127816, -0.4176697321401328100 ) ) ;
#8827=CARTESIAN_POINT ( 'NONE',  ( -0.6430446194225712953, -0.004921259842519870586, -0.3153832671262229437 ) ) ;
#8828=CYLINDRICAL_SURFACE ( 'NONE', #64130, 0.3937007874015748254 ) ;
#8829=CARTESIAN_POINT ( 'NONE',  ( -0.6889763779527552368, -0.5400638737290845981, -0.3530559997133363437 ) ) ;
#8830=CARTESIAN_POINT ( 'NONE',  ( -0.4986876640419939388, 0.2306618581243847221, -0.2411417322834647770 ) ) ;
#8831=CARTESIAN_POINT ( 'NONE',  ( 0.09842519685039434474, 0.1660481256975885056, 0.3530559997133364547 ) ) ;
#8834=VECTOR ( 'NONE', #20180, 39.37007874015748143 ) ;
#8835=DIRECTION ( 'NONE',  ( -0.2810846377148240594, -0.6785983445458320107, 0.6785983445458603214 ) ) ;
#8836=CARTESIAN_POINT ( 'NONE',  ( 0.2952755905511819101, 0.07958543189024071263, -0.2665933059059888421 ) ) ;
#8837=CARTESIAN_POINT ( 'NONE',  ( 1.010498687664042716, 0.05413385826771626580, -0.4176697321401330321 ) ) ;
#8838=CARTESIAN_POINT ( 'NONE',  ( -1.272965879265091305, -0.3690944881889763329, 0.3153832671262228327 ) ) ;
#8839=CARTESIAN_POINT ( 'NONE',  ( 1.364829396325460076, 0.2306618581243848609, 0.2411417322834645549 ) ) ;
#8840=CARTESIAN_POINT ( 'NONE',  ( -1.279527559055116948, -0.4536011799217367080, 0.2665933059059888421 ) ) ;
#8841=CARTESIAN_POINT ( 'NONE',  ( -0.3543307086614165824, -0.6692913385826771977, 8.415575281601705876E-17 ) ) ;
#8842=CARTESIAN_POINT ( 'NONE',  ( 0.2493438320209980519, -0.004921259842519576551, 0.3153832671262227771 ) ) ;
#8844=CARTESIAN_POINT ( 'NONE',  ( 0.6627296587926515548, 0.1771653543307087630, 0.09757992244046791164 ) ) ;
#8845=CARTESIAN_POINT ( 'NONE',  ( 0.1443569553805781891, 0.05413385826771626580, -0.4176697321401330321 ) ) ;
#8847=CARTESIAN_POINT ( 'NONE',  ( -0.6627296587926503335, -0.6692913385826771977, 0.1292274648535927661 ) ) ;
#8849=CARTESIAN_POINT ( 'NONE',  ( 1.122047244094488860, 0.07958543189024085140, 0.2665933059059887866 ) ) ;
#8850=CARTESIAN_POINT ( 'NONE',  ( -0.01968503937007793844, 0.1660481256975883668, -0.3530559997133364547 ) ) ;
#8851=CARTESIAN_POINT ( 'NONE',  ( -0.4527559055118102749, -0.5400638737290845981, -0.3530559997133363437 ) ) ;
#8852=CARTESIAN_POINT ( 'NONE',  ( -0.3937007874015740483, -0.1870078740157479769, 0.3641732283464567677 ) ) ;
#8853=CARTESIAN_POINT ( 'NONE',  ( 0.5971128608923891301, 0.2066929133858267098, -0.1054918080437494132 ) ) ;
#8854=CARTESIAN_POINT ( 'NONE',  ( -0.04593175853018302557, 0.1771653543307087630, 0.09757992244046791164 ) ) ;
#8855=CARTESIAN_POINT ( 'NONE',  ( 0.4790026246719168435, -0.3162353388693409650, -0.4822834645669289433 ) ) ;
#8856=CARTESIAN_POINT ( 'NONE',  ( -0.6627296587926503335, -0.5511811023622046335, 0.09757992244046803654 ) ) ;
#8858=CARTESIAN_POINT ( 'NONE',  ( -1.233595800524933894, -0.6046776061558809534, -0.2411417322834644161 ) ) ;
#8860=ORIENTED_EDGE ( 'NONE', *, *, #32904, .F. ) ;
#8861=CARTESIAN_POINT ( 'NONE',  ( -1.043307086614172707, 0.07958543189024071263, -0.2665933059059888421 ) ) ;
#8862=CARTESIAN_POINT ( 'NONE',  ( -0.2427821522309703550, -0.05778040916215560624, -0.4822834645669293319 ) ) ;
#8863=CARTESIAN_POINT ( 'NONE',  ( -1.601049868766403650, -0.6046776061558807314, 0.2411417322834647770 ) ) ;
#8864=CARTESIAN_POINT ( 'NONE',  ( -0.6299212598425188991, -0.1870078740157480879, -0.4822834645669291653 ) ) ;
#8866=CARTESIAN_POINT ( 'NONE',  ( 1.233595800524935227, 0.2306618581243847221, -0.2411417322834647770 ) ) ;
#8867=CARTESIAN_POINT ( 'NONE',  ( 0.9776902887139113929, -0.6692913385826773087, -0.1292274648535924053 ) ) ;
#8872=VECTOR ( 'NONE', #78927, 39.37007874015748143 ) ;
#8873=CARTESIAN_POINT ( 'NONE',  ( 1.450131233595801428, 0.1771653543307087630, 0.09757992244046791164 ) ) ;
#8875=ORIENTED_EDGE ( 'NONE', *, *, #68645, .T. ) ;
#8876=CARTESIAN_POINT ( 'NONE',  ( -0.4593175853018364174, -0.3690944881889765550, -0.3153832671262227771 ) ) ;
#8878=ORIENTED_EDGE ( 'NONE', *, *, #60399, .T. ) ;
#8879=CARTESIAN_POINT ( 'NONE',  ( 0.7808398950131240079, -0.3162353388693405765, 0.4822834645669290543 ) ) ;
#8880=CARTESIAN_POINT ( 'NONE',  ( 0.2427821522309716595, -0.3162353388693409650, -0.4822834645669289433 ) ) ;
#8881=CARTESIAN_POINT ( 'NONE',  ( -0.7742782152230962556, -0.4281496062992127816, -0.4176697321401328100 ) ) ;
#8882=CARTESIAN_POINT ( 'NONE',  ( 1.561679790026247350, 0.05413385826771626580, -0.4176697321401330321 ) ) ;
#8883=CARTESIAN_POINT ( 'NONE',  ( -0.6758530183727028406, 0.1771653543307087630, 0.09757992244046791164 ) ) ;
#8885=CARTESIAN_POINT ( 'NONE',  ( 0.4461942257217856311, 0.2306618581243847221, -0.2411417322834647770 ) ) ;
#8886=CARTESIAN_POINT ( 'NONE',  ( 0.4855643044619428750, -0.004921259842519576551, 0.3153832671262227771 ) ) ;
#8887=CARTESIAN_POINT ( 'NONE',  ( -1.036745406824146176, -0.4281496062992124485, 0.4176697321401328655 ) ) ;
#8889=CARTESIAN_POINT ( 'NONE',  ( -1.233595800524933894, -0.6046776061558809534, -0.2411417322834644161 ) ) ;
#8890=CARTESIAN_POINT ( 'NONE',  ( -1.660104986876639543, -0.08942795157528024563, -0.3641732283464568787 ) ) ;
#8891=CARTESIAN_POINT ( 'NONE',  ( 0.9776902887139113929, -0.6692913385826773087, -0.1292274648535924053 ) ) ;
#8892=CARTESIAN_POINT ( 'NONE',  ( 1.167979002624672580, -0.3690944881889763329, 0.3153832671262228327 ) ) ;
#8895=CARTESIAN_POINT ( 'NONE',  ( -0.4002624671916004129, -0.3162353388693405765, 0.4822834645669290543 ) ) ;
#8896=ORIENTED_EDGE ( 'NONE', *, *, #64509, .T. ) ;
#8897=CARTESIAN_POINT ( 'NONE',  ( 0.5839895013123367340, -0.5511811023622048555, -0.09757992244046775898 ) ) ;
#8899=CARTESIAN_POINT ( 'NONE',  ( -1.364829396325458521, 0.2306618581243847221, -0.2411417322834647770 ) ) ;
#8900=CARTESIAN_POINT ( 'NONE',  ( 1.089238845144357537, -0.4281496062992124485, 0.4176697321401328655 ) ) ;
#8901=CARTESIAN_POINT ( 'NONE',  ( 0.8333333333333340365, 0.2952755905511810774, -0.1292274648535930714 ) ) ;
#8902=CARTESIAN_POINT ( 'NONE',  ( -0.2952755905511804668, 0.1660481256975885056, 0.3530559997133364547 ) ) ;
#8903=CARTESIAN_POINT ( 'NONE',  ( -0.2559055118110227234, -0.5400638737290844871, 0.3530559997133364547 ) ) ;
#8905=CARTESIAN_POINT ( 'NONE',  ( -1.607611548556429737, -0.6692913385826771977, 0.1292274648535927661 ) ) ;
#8906=CARTESIAN_POINT ( 'NONE',  ( -0.6758530183727028406, 0.2952755905511811885, 0.1292274648535926551 ) ) ;
#8907=CARTESIAN_POINT ( 'NONE',  ( -0.6496062992125976043, 0.07958543189024071263, -0.2665933059059888421 ) ) ;
#8908=CARTESIAN_POINT ( 'NONE',  ( 1.292650918635171564, -0.6692913385826773087, -0.1292274648535924053 ) ) ;
#8911=CARTESIAN_POINT ( 'NONE',  ( -1.036745406824146176, 0.05413385826771626580, -0.4176697321401330321 ) ) ;
#8913=CARTESIAN_POINT ( 'NONE',  ( 0.5446194225721792126, -0.05778040916215560624, -0.4822834645669293319 ) ) ;
#8915=CARTESIAN_POINT ( 'NONE',  ( -0.6575345472709128725, 1.929133858267715773, -0.5309055118110235227 ) ) ;
#8917=CARTESIAN_POINT ( 'NONE',  ( -0.2165354330708654795, 0.1660481256975885056, 0.3530559997133364547 ) ) ;
#8918=CARTESIAN_POINT ( 'NONE',  ( -1.332020997375327642, -0.08942795157527998196, 0.3641732283464567121 ) ) ;
#8919=CARTESIAN_POINT ( 'NONE',  ( 1.167979002624672580, -0.3690944881889763329, 0.3153832671262228327 ) ) ;
#8922=CARTESIAN_POINT ( 'NONE',  ( 1.259842519685040019, -0.1870078740157480601, -0.3641732283464567677 ) ) ;
#8923=CARTESIAN_POINT ( 'NONE',  ( 1.417322834645670104, -0.1870078740157479769, 0.4822834645669291653 ) ) ;
#8925=CARTESIAN_POINT ( 'NONE',  ( -0.2493438320209966919, 0.05413385826771626580, -0.4176697321401330321 ) ) ;
#8927=CARTESIAN_POINT ( 'NONE',  ( 1.561679790026247350, -0.3690944881889763329, 0.3153832671262228327 ) ) ;
#8928=CARTESIAN_POINT ( 'NONE',  ( -0.2165354330708654795, -0.5400638737290845981, -0.3530559997133363437 ) ) ;
#8930=CARTESIAN_POINT ( 'NONE',  ( 1.187664041994751285, -0.05778040916215522460, 0.4822834645669289988 ) ) ;
#8931=CARTESIAN_POINT ( 'NONE',  ( 0.3674540682414705883, 0.2306618581243847221, -0.2411417322834647770 ) ) ;
#8932=CARTESIAN_POINT ( 'NONE',  ( 0.4396325459317593221, 0.1771653543307087075, -0.09757992244046823083 ) ) ;
#8934=CARTESIAN_POINT ( 'NONE',  ( 0.2755905511811031494, 0.1771653543307087630, 0.000000000000000000 ) ) ;
#8936=CARTESIAN_POINT ( 'NONE',  ( 0.5839895013123367340, 0.2952755905511811885, 0.1292274648535926551 ) ) ;
#8937=EDGE_CURVE ( 'NONE', #6163, #59008, #25792, .T. ) ;
#8940=VECTOR ( 'NONE', #5443, 39.37007874015748143 ) ;
#8943=CARTESIAN_POINT ( 'NONE',  ( 0.1049868766404206816, -0.5023911411419708095, -0.1820866141732282451 ) ) ;
#8944=CARTESIAN_POINT ( 'NONE',  ( -0.09842519685039295696, -0.5400638737290844871, 0.3530559997133364547 ) ) ;
#8945=CARTESIAN_POINT ( 'NONE',  ( 1.200787401574803681, 0.07958543189024085140, 0.2665933059059887866 ) ) ;
#8946=CARTESIAN_POINT ( 'NONE',  ( -1.272965879265091305, -0.3690944881889763329, 0.3153832671262228327 ) ) ;
#8947=CARTESIAN_POINT ( 'NONE',  ( -1.437007874015747477, -0.5400638737290844871, 0.3530559997133364547 ) ) ;
#8948=CARTESIAN_POINT ( 'NONE',  ( 0.5774278215223104249, 0.2306618581243848609, 0.2411417322834645549 ) ) ;
#8949=B_SPLINE_CURVE_WITH_KNOTS ( 'NONE', 3,
 ( #49882, #49476, #43971, #11189 ),
 .UNSPECIFIED., .F., .F.,
 ( 4, 4 ),
 ( 0.02789255478306693070, 0.02946499057610776906 ),
 .UNSPECIFIED. ) ;
#8950=CARTESIAN_POINT ( 'NONE',  ( -1.627296587926508442, 0.1283753931104748280, 0.1820866141732283561 ) ) ;
#8951=DIRECTION ( 'NONE',  ( -3.096699300667737957E-16, 1.000000000000000000, -0.000000000000000000 ) ) ;
#8952=CARTESIAN_POINT ( 'NONE',  ( 0.4199475065616803948, -0.6046776061558809534, -0.2411417322834644161 ) ) ;
#8955=CARTESIAN_POINT ( 'NONE',  ( 1.548556430446194954, 0.2306618581243847221, -0.2411417322834647770 ) ) ;
#8956=CARTESIAN_POINT ( 'NONE',  ( 1.089238845144357759, 0.05413385826771626580, -0.4176697321401330321 ) ) ;
#8957=CARTESIAN_POINT ( 'NONE',  ( -1.528871391076114250, 0.1771653543307087075, -0.09757992244046823083 ) ) ;
#8958=CARTESIAN_POINT ( 'NONE',  ( 1.279527559055118724, -0.4536011799217368745, -0.2665933059059886201 ) ) ;
#8959=CARTESIAN_POINT ( 'NONE',  ( 1.574803149606299746, -0.1870078740157480879, -0.4822834645669291653 ) ) ;
#8960=CARTESIAN_POINT ( 'NONE',  ( -0.9120734908136475250, -0.5511811023622048555, -0.09757992244046775898 ) ) ;
#8962=CARTESIAN_POINT ( 'NONE',  ( 0.6561679790026253567, 0.1283753931104748280, 0.1820866141732283561 ) ) ;
#8963=CARTESIAN_POINT ( 'NONE',  ( 0.2755905511811031494, 0.2952755905511811885, 0.000000000000000000 ) ) ;
#8964=CARTESIAN_POINT ( 'NONE',  ( 1.213910761154856299, -0.6692913385826773087, -0.1292274648535924053 ) ) ;
#8965=CARTESIAN_POINT ( 'NONE',  ( -0.2821522309711278487, -0.6692913385826773087, -0.1292274648535924053 ) ) ;
#8966=CARTESIAN_POINT ( 'NONE',  ( 0.1837270341207354329, 0.1283753931104748280, 0.1820866141732283561 ) ) ;
#8967=CARTESIAN_POINT ( 'NONE',  ( 1.417322834645670104, -0.1870078740157479769, 0.4822834645669291653 ) ) ;
#8968=CARTESIAN_POINT ( 'NONE',  ( -0.2238009295390064879, -2.294479370626195693E-15, 0.3464511005275217603 ) ) ;
#8969=CARTESIAN_POINT ( 'NONE',  ( -1.076115485564303809, 0.2306618581243848609, 0.2411417322834645549 ) ) ;
#8970=CARTESIAN_POINT ( 'NONE',  ( -1.443569553805773564, -0.5023911411419708095, 0.1820866141732285504 ) ) ;
#8972=CARTESIAN_POINT ( 'NONE',  ( 1.013282927784340259, -2.226000259411765883E-16, -0.4281993546915530136 ) ) ;
#8973=CARTESIAN_POINT ( 'NONE',  ( -0.9055118110236215490, -0.6692913385826771977, 8.415575281601705876E-17 ) ) ;
#8975=CARTESIAN_POINT ( 'NONE',  ( -0.1181102362204717315, 0.2952755905511811885, 0.000000000000000000 ) ) ;
#8976=( BOUNDED_CURVE ( )  B_SPLINE_CURVE ( 2, ( #55230, #82574, #76265, #31213, #24893, #50156, #10644, #11047, #80937, #23253, #23664, #11464, #49745 ),
 .UNSPECIFIED., .F., .F. ) 
 B_SPLINE_CURVE_WITH_KNOTS ( ( 3, 2, 2, 2, 2, 2, 3 ),
 ( 0.5369674582711644328, 0.5378787878787878451, 0.5416666666666666297, 0.5454545454545454142, 0.5492424242424241987, 0.5530303030303029832, 0.5539416326379265065 ),
 .UNSPECIFIED. ) 
 CURVE ( )  GEOMETRIC_REPRESENTATION_ITEM ( )  RATIONAL_B_SPLINE_CURVE ( ( 0.9875488213027523443, 0.9918020599134680371, 1.000000000000000000, 0.9659258262890683122, 1.000000000000000000, 0.9659258262890683122, 1.000000000000000000, 0.9659258262890683122, 1.000000000000000000, 0.9659258262890683122, 1.000000000000000000, 0.9918020599134671489, 0.9875488213027514561 ) ) 
 REPRESENTATION_ITEM ( '' )  );
#8980=CARTESIAN_POINT ( 'NONE',  ( 0.7152230971128616943, -0.08942795157527998196, 0.3641732283464567121 ) ) ;
#8982=CARTESIAN_POINT ( 'NONE',  ( 0.9448818897637802916, -0.1870078740157479769, 0.4822834645669291653 ) ) ;
#8983=DIRECTION ( 'NONE',  ( 1.000000000000000000, -0.000000000000000000, -0.000000000000000000 ) ) ;
#8984=CARTESIAN_POINT ( 'NONE',  ( -1.384514435695537005, 0.1771653543307087630, 0.09757992244046791164 ) ) ;
#8985=CARTESIAN_POINT ( 'NONE',  ( 1.404199475065617708, 0.05413385826771626580, -0.4176697321401330321 ) ) ;
#8986=CARTESIAN_POINT ( 'NONE',  ( -1.430446194225721390, -0.4281496062992124485, 0.4176697321401328655 ) ) ;
#8989=CARTESIAN_POINT ( 'NONE',  ( 0.1443569553805781891, 0.05413385826771626580, -0.4176697321401330321 ) ) ;
#8990=CARTESIAN_POINT ( 'NONE',  ( -0.2821522309711278487, 0.1771653543307087630, 0.09757992244046791164 ) ) ;
#8991=CARTESIAN_POINT ( 'NONE',  ( 0.6561679790026253567, 0.2306618581243848609, 0.2411417322834645549 ) ) ;
#8992=CARTESIAN_POINT ( 'NONE',  ( 0.3937007874015754361, -0.1870078740157480879, -0.4822834645669291653 ) ) ;
#8995=CARTESIAN_POINT ( 'NONE',  ( -1.614173228346456712, 1.543375672658095610, -0.1372047244094478091 ) ) ;
#8997=CARTESIAN_POINT ( 'NONE',  ( 0.9186351706036752773, 0.2306618581243847221, -0.2411417322834647770 ) ) ;
#8999=CARTESIAN_POINT ( 'NONE',  ( 5.463695987328526437E-16, -0.1870078740157479769, 0.4822834645669291653 ) ) ;
#9000=CARTESIAN_POINT ( 'NONE',  ( -1.161417322834644716, 0.1660481256975885056, 0.3530559997133364547 ) ) ;
#9001=CARTESIAN_POINT ( 'NONE',  ( 1.496062992125984703, -0.1870078740157480879, -0.4822834645669291653 ) ) ;
#9002=CARTESIAN_POINT ( 'NONE',  ( 0.6824146981627303710, -0.6046776061558807314, 0.2411417322834647770 ) ) ;
#9004=CARTESIAN_POINT ( 'NONE',  ( -0.2230971128608915943, -0.4281496062992127816, -0.4176697321401328100 ) ) ;
#9005=CARTESIAN_POINT ( 'NONE',  ( 0.7349081364829403995, 0.2306618581243848609, 0.2411417322834645549 ) ) ;
#9006=CARTESIAN_POINT ( 'NONE',  ( 0.04593175853018440641, -0.6692913385826771977, 0.1292274648535927661 ) ) ;
#9007=CARTESIAN_POINT ( 'NONE',  ( 0.5511811023622055217, -0.1870078740157479769, 0.3641732283464567677 ) ) ;
#9008=CARTESIAN_POINT ( 'NONE',  ( -1.358267716535432434, 0.1660481256975883668, -0.3530559997133364547 ) ) ;
#9009=CARTESIAN_POINT ( 'NONE',  ( -1.482939632545930975, -0.4281496062992127816, -0.4176697321401328100 ) ) ;
#9010=CARTESIAN_POINT ( 'NONE',  ( 0.9448818897637802916, -0.1870078740157479769, 0.4822834645669291653 ) ) ;
#9014=ORIENTED_EDGE ( 'NONE', *, *, #27043, .T. ) ;
#9015=CARTESIAN_POINT ( 'NONE',  ( 1.200787401574803681, 0.1660481256975885056, 0.3530559997133364547 ) ) ;
#9016=CARTESIAN_POINT ( 'NONE',  ( 0.6692913385826777528, 0.1771653543307087630, 0.000000000000000000 ) ) ;
#9023=CARTESIAN_POINT ( 'NONE',  ( -0.9383202099737524282, -0.05778040916215522460, 0.4822834645669289988 ) ) ;
#9024=CARTESIAN_POINT ( 'NONE',  ( 1.240157480314961314, -0.5400638737290844871, 0.3530559997133364547 ) ) ;
#9025=VERTEX_POINT ( 'NONE', #28692 ) ;
#9026=CARTESIAN_POINT ( 'NONE',  ( 1.607611548556431069, 0.2952755905511811885, 0.1292274648535926551 ) ) ;
#9027=CARTESIAN_POINT ( 'NONE',  ( 1.587926509186352586, -0.3690944881889765550, -0.3153832671262227771 ) ) ;
#9029=CYLINDRICAL_SURFACE ( 'NONE', #80230, 0.3937007874015748254 ) ;
#9031=CARTESIAN_POINT ( 'NONE',  ( -1.292650918635170010, 0.1771653543307087075, -0.09757992244046823083 ) ) ;
#9033=CARTESIAN_POINT ( 'NONE',  ( 0.3805774278215230400, -0.4281496062992124485, 0.4176697321401328655 ) ) ;
#9034=CARTESIAN_POINT ( 'NONE',  ( 1.515748031496063408, 0.1660481256975885056, 0.3530559997133364547 ) ) ;
#9036=CARTESIAN_POINT ( 'NONE',  ( -0.6627296587926503335, -0.5511811023622046335, 0.09757992244046803654 ) ) ;
#9037=CARTESIAN_POINT ( 'NONE',  ( 0.6364829396325465405, -0.3162353388693409650, -0.4822834645669289433 ) ) ;
#9038=CARTESIAN_POINT ( 'NONE',  ( 1.325459317585302665, -0.004921259842519870586, -0.3153832671262229437 ) ) ;
#9040=CARTESIAN_POINT ( 'NONE',  ( -0.7611548556430438595, 0.1283753931104748280, 0.1820866141732283561 ) ) ;
#9041=CARTESIAN_POINT ( 'NONE',  ( 1.509186351706037543, 0.05413385826771666132, 0.4176697321401328100 ) ) ;
#9043=CARTESIAN_POINT ( 'NONE',  ( 0.3674540682414705883, 0.2306618581243847221, -0.2411417322834647770 ) ) ;
#9044=CARTESIAN_POINT ( 'NONE',  ( -0.8070866141732276899, 0.07958543189024071263, -0.2665933059059888421 ) ) ;
#9045=CARTESIAN_POINT ( 'NONE',  ( -0.1181102362204717315, 0.1771653543307087630, 0.000000000000000000 ) ) ;
#9046=CARTESIAN_POINT ( 'NONE',  ( -0.09842519685039295696, 0.1660481256975883668, -0.3530559997133364547 ) ) ;
#9047=CARTESIAN_POINT ( 'NONE',  ( 1.653543307086614789, -0.1870078740157479769, 0.4822834645669291653 ) ) ;
#9049=CARTESIAN_POINT ( 'NONE',  ( 0.7874015748031503170, -0.1870078740157479769, 0.4822834645669291653 ) ) ;
#9055=CARTESIAN_POINT ( 'NONE',  ( -0.6955380577427815458, -0.4281496062992127816, -0.4176697321401328100 ) ) ;
#9056=CARTESIAN_POINT ( 'NONE',  ( -0.1771653543307080136, -0.4536011799217367080, 0.2665933059059888421 ) ) ;
#9058=CARTESIAN_POINT ( 'NONE',  ( -1.502624671916009680, -0.3162353388693405765, 0.4822834645669290543 ) ) ;
#9059=CARTESIAN_POINT ( 'NONE',  ( 0.3477690288713918276, -0.5511811023622048555, -0.09757992244046775898 ) ) ;
#9060=CARTESIAN_POINT ( 'NONE',  ( -0.5905511811023615998, 0.1771653543307087630, 0.000000000000000000 ) ) ;
#9061=CARTESIAN_POINT ( 'NONE',  ( -1.082677165354329896, 0.1660481256975885056, 0.3530559997133364547 ) ) ;
#9062=CARTESIAN_POINT ( 'NONE',  ( -1.627296587926508442, -0.6046776061558809534, -0.2411417322834644161 ) ) ;
#9063=CARTESIAN_POINT ( 'NONE',  ( 1.384514435695538559, 0.2952755905511810774, -0.1292274648535930714 ) ) ;
#9064=CARTESIAN_POINT ( 'NONE',  ( 1.036394771582350938, 0.004960608223779470680, 0.3437734562760185741 ) ) ;
#9065=CARTESIAN_POINT ( 'NONE',  ( 0.8464566929133866546, -0.4536011799217367080, 0.2665933059059888421 ) ) ;
#9066=CARTESIAN_POINT ( 'NONE',  ( 0.5971128608923891301, 0.2952755905511810774, -0.1292274648535930714 ) ) ;
#9067=EDGE_CURVE ( 'NONE', #31420, #71641, #54353, .T. ) ;
#9069=CARTESIAN_POINT ( 'NONE',  ( 1.292650918635171564, 0.1771653543307087630, 0.09757992244046791164 ) ) ;
#9071=B_SPLINE_CURVE_WITH_KNOTS ( 'NONE', 3,
 ( #61008, #3357, #72818, #15168, #74069, #16415, #68570 ),
 .UNSPECIFIED., .F., .F.,
 ( 4, 3, 4 ),
 ( 7.285838599102589797E-17, 0.001246232571205252914, 0.002492492258783168303 ),
 .UNSPECIFIED. ) ;
#9073=CARTESIAN_POINT ( 'NONE',  ( -1.181102362204723644, -0.1870078740157479769, 0.3641732283464567677 ) ) ;
#9074=CARTESIAN_POINT ( 'NONE',  ( -0.3149606299212590610, -0.1870078740157480879, -0.4822834645669291653 ) ) ;
#9075=CARTESIAN_POINT ( 'NONE',  ( 0.4396325459317590445, -0.6692913385826771977, 0.1292274648535927661 ) ) ;
#9076=CARTESIAN_POINT ( 'NONE',  ( -1.482939632545930975, -0.3690944881889765550, -0.3153832671262227771 ) ) ;
#9078=CARTESIAN_POINT ( 'NONE',  ( -1.240157480314959759, 0.1660481256975885056, 0.3530559997133364547 ) ) ;
#9079=CARTESIAN_POINT ( 'NONE',  ( 0.6299212598425204535, -0.1870078740157480879, -0.4822834645669291653 ) ) ;
#9080=CARTESIAN_POINT ( 'NONE',  ( -0.09186351706036663400, -0.4281496062992124485, 0.4176697321401328655 ) ) ;
#9081=CARTESIAN_POINT ( 'NONE',  ( 1.010498687664042716, 0.05413385826771626580, -0.4176697321401330321 ) ) ;
#9082=CARTESIAN_POINT ( 'NONE',  ( 1.692913385826772421, 0.2952755905511811885, 0.000000000000000000 ) ) ;
#9087=CARTESIAN_POINT ( 'NONE',  ( 0.07217847769028949700, -0.08942795157528024563, -0.3641732283464568787 ) ) ;
#9088=CARTESIAN_POINT ( 'NONE',  ( -0.5183727034120726440, -0.6692913385826773087, -0.1292274648535924053 ) ) ;
#9089=CARTESIAN_POINT ( 'NONE',  ( 1.017060367454068581, -0.05778040916215560624, -0.4822834645669293319 ) ) ;
#9091=CARTESIAN_POINT ( 'NONE',  ( -0.2230971128608915943, -0.004921259842519576551, 0.3153832671262227771 ) ) ;
#9092=CARTESIAN_POINT ( 'NONE',  ( -1.049868766404198794, -0.6046776061558807314, 0.2411417322834647770 ) ) ;
#9093=CARTESIAN_POINT ( 'NONE',  ( -1.469816272965878357, 0.2306618581243848609, 0.2411417322834645549 ) ) ;
#9098=CARTESIAN_POINT ( 'NONE',  ( 1.076115485564305141, -0.6046776061558807314, 0.2411417322834647770 ) ) ;
#9099=CARTESIAN_POINT ( 'NONE',  ( 1.482939632545932307, -0.004921259842519870586, -0.3153832671262229437 ) ) ;
#9100=CARTESIAN_POINT ( 'NONE',  ( -1.305774278215222184, 0.1771653543307087630, 0.09757992244046791164 ) ) ;
#9101=CARTESIAN_POINT ( 'NONE',  ( -1.187664041994749731, -0.3162353388693405765, 0.4822834645669290543 ) ) ;
#9103=CARTESIAN_POINT ( 'NONE',  ( 1.033630966599880630, -4.927456884911482678E-16, 0.4445507791589062840 ) ) ;
#9104=CARTESIAN_POINT ( 'NONE',  ( 1.286089238845145033, -0.6046776061558809534, -0.2411417322834644161 ) ) ;
#9105=CARTESIAN_POINT ( 'NONE',  ( -1.712598425196849572, 0.1660481256975885056, 0.3530559997133364547 ) ) ;
#9106=CARTESIAN_POINT ( 'NONE',  ( -0.2099737532808391705, -0.6046776061558809534, -0.2411417322834644161 ) ) ;
#9107=CARTESIAN_POINT ( 'NONE',  ( 0.01968503937007930540, 0.1660481256975885056, 0.3530559997133364547 ) ) ;
#9108=CARTESIAN_POINT ( 'NONE',  ( -1.351706036745406347, -0.4281496062992124485, 0.4176697321401328655 ) ) ;
#9110=CARTESIAN_POINT ( 'NONE',  ( 0.2099737532808405305, 0.2306618581243847221, -0.2411417322834647770 ) ) ;
#9113=CARTESIAN_POINT ( 'NONE',  ( -1.397637795275589623, -0.4536011799217368745, -0.2665933059059886201 ) ) ;
#9119=CARTESIAN_POINT ( 'NONE',  ( -1.469816272965878357, -0.6046776061558809534, -0.2411417322834644161 ) ) ;
#9120=CARTESIAN_POINT ( 'NONE',  ( -1.574803149606298192, -0.1870078740157480879, -0.4822834645669291653 ) ) ;
#9122=CARTESIAN_POINT ( 'NONE',  ( -1.482939632545930975, -0.4281496062992127816, -0.4176697321401328100 ) ) ;
#9123=CARTESIAN_POINT ( 'NONE',  ( -1.607611548556429737, -0.6692913385826771977, 0.1292274648535927661 ) ) ;
#9124=CARTESIAN_POINT ( 'NONE',  ( -0.9645669291338576645, 0.1660481256975883391, -0.3530559997133364547 ) ) ;
#9127=CARTESIAN_POINT ( 'NONE',  ( -0.3608923884514428360, 0.1771653543307087630, 0.09757992244046791164 ) ) ;
#9128=CARTESIAN_POINT ( 'NONE',  ( -0.6496062992125976043, -0.4536011799217367080, 0.2665933059059888421 ) ) ;
#9129=CARTESIAN_POINT ( 'NONE',  ( -1.299212598425196097, 0.2952755905511811885, 0.000000000000000000 ) ) ;
#9130=CARTESIAN_POINT ( 'NONE',  ( 0.9514435695538062676, -0.05778040916215522460, 0.4822834645669289988 ) ) ;
#9131=CARTESIAN_POINT ( 'NONE',  ( -0.8464566929133852113, 0.1660481256975885056, 0.3530559997133364547 ) ) ;
#9133=ORIENTED_EDGE ( 'NONE', *, *, #19008, .F. ) ;
#9134=CARTESIAN_POINT ( 'NONE',  ( -1.351706036745406347, -0.4281496062992124485, 0.4176697321401328655 ) ) ;
#9135=CARTESIAN_POINT ( 'NONE',  ( -0.7773926554473638006, -2.191421614605370878E-15, 0.4445507791589071167 ) ) ;
#9136=CARTESIAN_POINT ( 'NONE',  ( 0.000000000000000000, 0.000000000000000000, 0.000000000000000000 ) ) ;
#9141=CARTESIAN_POINT ( 'NONE',  ( -0.3149606299212590610, -0.1870078740157480879, -0.4822834645669291653 ) ) ;
#9142=CARTESIAN_POINT ( 'NONE',  ( 1.259842519685040019, -0.1870078740157480879, -0.4822834645669291653 ) ) ;
#9144=CARTESIAN_POINT ( 'NONE',  ( -1.522309711286088607, 0.2306618581243847221, -0.2411417322834647770 ) ) ;
#9145=DIRECTION ( 'NONE',  ( -0.000000000000000000, 1.000000000000000000, -0.000000000000000000 ) ) ;
#9146=CARTESIAN_POINT ( 'NONE',  ( -1.272965879265091305, -0.4281496062992124485, 0.4176697321401328655 ) ) ;
#9147=CARTESIAN_POINT ( 'NONE',  ( -0.9645669291338575535, -0.5400638737290844871, 0.3530559997133364547 ) ) ;
#9149=CARTESIAN_POINT ( 'NONE',  ( 0.4396325459317590445, -0.5511811023622046335, 0.09757992244046803654 ) ) ;
#9151=CARTESIAN_POINT ( 'NONE',  ( 0.3018372703412079971, -0.004921259842519870586, -0.3153832671262229437 ) ) ;
#9152=CARTESIAN_POINT ( 'NONE',  ( 1.076115485564305141, -0.5023911411419708095, 0.1820866141732285504 ) ) ;
#9153=CARTESIAN_POINT ( 'NONE',  ( 0.8792650918635177559, -0.4281496062992127816, -0.4176697321401328100 ) ) ;
#9154=CARTESIAN_POINT ( 'NONE',  ( -0.4724409448818890911, -0.1870078740157480601, -0.3641732283464567677 ) ) ;
#9156=CARTESIAN_POINT ( 'NONE',  ( -1.115485564304461219, 0.05413385826771626580, -0.4176697321401330321 ) ) ;
#9157=CARTESIAN_POINT ( 'NONE',  ( -1.299212598425196097, 0.1771653543307087630, 0.000000000000000000 ) ) ;
#9159=CARTESIAN_POINT ( 'NONE',  ( -0.8989501312335946848, -0.5511811023622046335, 0.09757992244046803654 ) ) ;
#9161=CARTESIAN_POINT ( 'NONE',  ( -0.2624671916010490880, -0.6046776061558807314, 0.2411417322834647770 ) ) ;
#9163=CARTESIAN_POINT ( 'NONE',  ( 0.5380577427821529035, -0.004921259842519870586, -0.3153832671262229437 ) ) ;
#9164=CARTESIAN_POINT ( 'NONE',  ( -0.4461942257217840213, 0.1283753931104748280, 0.1820866141732283561 ) ) ;
#9165=CARTESIAN_POINT ( 'NONE',  ( -0.8858267716535425107, -0.5400638737290844871, 0.3530559997133364547 ) ) ;
#9166=CARTESIAN_POINT ( 'NONE',  ( -1.574803149606298636, -0.1870078740157479769, 0.4822834645669291653 ) ) ;
#9168=CARTESIAN_POINT ( 'NONE',  ( 0.006561679790026889343, -0.3162353388693409650, -0.4822834645669289433 ) ) ;
#9171=CARTESIAN_POINT ( 'NONE',  ( 1.437007874015748810, 0.1660481256975885056, 0.3530559997133364547 ) ) ;
#9172=CARTESIAN_POINT ( 'NONE',  ( -0.4199475065616791736, 0.1283753931104746893, -0.1820866141732285504 ) ) ;
#9173=CARTESIAN_POINT ( 'NONE',  ( -0.2230971128608915943, -0.4281496062992127816, -0.4176697321401328100 ) ) ;
#9174=CARTESIAN_POINT ( 'NONE',  ( -1.456692913385826182, 0.2952755905511811885, 0.000000000000000000 ) ) ;
#9175=CARTESIAN_POINT ( 'NONE',  ( 1.673228346456693494, 0.1660481256975885056, 0.3530559997133364547 ) ) ;
#9176=CARTESIAN_POINT ( 'NONE',  ( 1.345144356955381593, -0.05778040916215522460, 0.4822834645669289988 ) ) ;
#9177=CARTESIAN_POINT ( 'NONE',  ( -0.6233595800524928121, -0.08942795157527998196, 0.3641732283464567121 ) ) ;
#9178=CARTESIAN_POINT ( 'NONE',  ( -1.090429162302622101, -1.142320075227303543E-15, 0.3627985898453523483 ) ) ;
#9182=CARTESIAN_POINT ( 'NONE',  ( 1.358267716535433323, -0.4536011799217368745, -0.2665933059059886201 ) ) ;
#9183=CARTESIAN_POINT ( 'NONE',  ( -1.627296587926508442, -0.6046776061558809534, -0.2411417322834644161 ) ) ;
#9184=CARTESIAN_POINT ( 'NONE',  ( 1.023622047244095112, -0.1870078740157480879, -0.4822834645669291653 ) ) ;
#9186=CARTESIAN_POINT ( 'NONE',  ( 1.161417322834646493, -0.4536011799217367080, 0.2665933059059888421 ) ) ;
#9187=CARTESIAN_POINT ( 'NONE',  ( 0.1246719160104994284, 0.2952755905511810774, -0.1292274648535930714 ) ) ;
#9188=CARTESIAN_POINT ( 'NONE',  ( -0.2493438320209966919, -0.4281496062992124485, 0.4176697321401328655 ) ) ;
#9191=CARTESIAN_POINT ( 'NONE',  ( 0.06840103802056105020, -1.283732188437465593E-15, -0.4281993546915538462 ) ) ;
#9192=CARTESIAN_POINT ( 'NONE',  ( 0.1443569553805781891, -0.3690944881889763329, 0.3153832671262228327 ) ) ;
#9195=ORIENTED_EDGE ( 'NONE', *, *, #9262, .T. ) ;
#9196=CARTESIAN_POINT ( 'NONE',  ( -0.4002624671916004129, -0.05778040916215560624, -0.4822834645669293319 ) ) ;
#9197=CARTESIAN_POINT ( 'NONE',  ( 1.161417322834646271, 0.1660481256975883668, -0.3530559997133364547 ) ) ;
#9198=CARTESIAN_POINT ( 'NONE',  ( 0.2099737532808405305, -0.6046776061558807314, 0.2411417322834647770 ) ) ;
#9199=CARTESIAN_POINT ( 'NONE',  ( -0.1706036745406816491, -0.004921259842519870586, -0.3153832671262229437 ) ) ;
#9200=CARTESIAN_POINT ( 'NONE',  ( 0.6627296587926517768, -0.6692913385826773087, -0.1292274648535924053 ) ) ;
#9201=CARTESIAN_POINT ( 'NONE',  ( -1.089238845144356427, -0.4281496062992127816, -0.4176697321401328100 ) ) ;
#9202=CARTESIAN_POINT ( 'NONE',  ( -0.5446194225721777693, -0.3162353388693409650, -0.4822834645669289433 ) ) ;
#9203=CARTESIAN_POINT ( 'NONE',  ( -0.9580052493438311334, -0.4281496062992124485, 0.4176697321401328655 ) ) ;
#9204=CARTESIAN_POINT ( 'NONE',  ( 1.141732283464567566, 0.2952755905511811885, 0.000000000000000000 ) ) ;
#9205=CARTESIAN_POINT ( 'NONE',  ( 0.8464566929133865436, 0.1660481256975883668, -0.3530559997133364547 ) ) ;
#9206=CARTESIAN_POINT ( 'NONE',  ( 0.7677165354330716118, 0.1660481256975883668, -0.3530559997133364547 ) ) ;
#9208=CARTESIAN_POINT ( 'NONE',  ( -0.07217847769028787330, -0.08942795157527998196, 0.3641732283464567121 ) ) ;
#9209=ORIENTED_EDGE ( 'NONE', *, *, #76941, .F. ) ;
#9212=CARTESIAN_POINT ( 'NONE',  ( -0.8595800524934373854, -0.2845877964562161244, -0.3641732283464567121 ) ) ;
#9213=CARTESIAN_POINT ( 'NONE',  ( -0.6364829396325453192, -0.05778040916215560624, -0.4822834645669293319 ) ) ;
#9215=CARTESIAN_POINT ( 'NONE',  ( -0.2362204724409442680, -0.1870078740157480879, -0.4822834645669291653 ) ) ;
#9216=CARTESIAN_POINT ( 'NONE',  ( -0.2296587926509179312, -0.3162353388693409650, -0.4822834645669289433 ) ) ;
#9217=CARTESIAN_POINT ( 'NONE',  ( -1.364829396325458521, -0.6046776061558807314, 0.2411417322834647770 ) ) ;
#9218=CARTESIAN_POINT ( 'NONE',  ( -1.391076115485563758, 0.2306618581243848609, 0.2411417322834645549 ) ) ;
#9219=CARTESIAN_POINT ( 'NONE',  ( 1.128608923884515169, -0.5023911411419708095, -0.1820866141732282451 ) ) ;
#9222=CARTESIAN_POINT ( 'NONE',  ( 0.3740157480314966754, 0.07958543189024071263, -0.2665933059059888421 ) ) ;
#9223=CARTESIAN_POINT ( 'NONE',  ( 0.2296587926509192634, -0.3162353388693405765, 0.4822834645669290543 ) ) ;
#9224=CARTESIAN_POINT ( 'NONE',  ( 0.1837270341207357105, -0.6046776061558809534, -0.2411417322834644161 ) ) ;
#9227=CARTESIAN_POINT ( 'NONE',  ( -1.604771003085130321, 1.002618919725274393, 0.1466069496707742281 ) ) ;
#9231=CARTESIAN_POINT ( 'NONE',  ( -0.3871391076115479057, -0.3162353388693409650, -0.4822834645669289433 ) ) ;
#9235=CARTESIAN_POINT ( 'NONE',  ( 1.666666666666667185, 0.05413385826771666132, 0.4176697321401328100 ) ) ;
#9236=CARTESIAN_POINT ( 'NONE',  ( 1.036745406824147508, -0.4281496062992127816, -0.4176697321401328100 ) ) ;
#9237=CARTESIAN_POINT ( 'NONE',  ( 0.8333333333333340365, -0.6692913385826771977, 0.1292274648535927661 ) ) ;
#9238=CARTESIAN_POINT ( 'NONE',  ( -0.7742782152230962556, -0.3690944881889765550, -0.3153832671262227771 ) ) ;
#9239=CARTESIAN_POINT ( 'NONE',  ( -0.1443569553805768291, 0.05413385826771666132, 0.4176697321401328100 ) ) ;
#9241=CARTESIAN_POINT ( 'NONE',  ( 0.1049868766404206816, 0.1283753931104748280, 0.1820866141732283561 ) ) ;
#9242=CARTESIAN_POINT ( 'NONE',  ( -0.3083989501312330295, -0.05778040916215522460, 0.4822834645669289988 ) ) ;
#9244=B_SPLINE_CURVE_WITH_KNOTS ( 'NONE', 3,
 ( #71082, #52114, #45802, #57599 ),
 .UNSPECIFIED., .F., .F.,
 ( 4, 4 ),
 ( 9.341771812940338307E-18, 0.001510660848364197726 ),
 .UNSPECIFIED. ) ;
#9245=CARTESIAN_POINT ( 'NONE',  ( 1.574803149606299746, -0.1870078740157479769, 0.3641732283464567677 ) ) ;
#9246=CARTESIAN_POINT ( 'NONE',  ( 0.09186351706036799403, -0.3690944881889765550, -0.3153832671262227771 ) ) ;
#9247=CARTESIAN_POINT ( 'NONE',  ( 1.666666666666667185, -0.004921259842519576551, 0.3153832671262227771 ) ) ;
#9248=CARTESIAN_POINT ( 'NONE',  ( -1.207349081364828880, 0.2306618581243847221, -0.2411417322834647770 ) ) ;
#9249=CARTESIAN_POINT ( 'NONE',  ( -0.9120734908136475250, -0.5511811023622048555, -0.09757992244046775898 ) ) ;
#9251=CARTESIAN_POINT ( 'NONE',  ( -1.056430446194224881, 0.2952755905511810774, -0.1292274648535930714 ) ) ;
#9252=CARTESIAN_POINT ( 'NONE',  ( -0.05249343832020911260, 0.2306618581243848609, 0.2411417322834645549 ) ) ;
#9257=CARTESIAN_POINT ( 'NONE',  ( 0.2427821522309719648, -0.08942795157527998196, 0.3641732283464567121 ) ) ;
#9258=CARTESIAN_POINT ( 'NONE',  ( 0.9908136482939640111, 0.2952755905511810774, -0.1292274648535930714 ) ) ;
#9259=CARTESIAN_POINT ( 'NONE',  ( -1.030183727034119867, -0.08942795157528024563, -0.3641732283464568787 ) ) ;
#9260=CARTESIAN_POINT ( 'NONE',  ( 1.194225721784777594, 0.05413385826771666132, 0.4176697321401328100 ) ) ;
#9261=CARTESIAN_POINT ( 'NONE',  ( -1.423884514435694859, -0.2845877964562159024, 0.3641732283464567677 ) ) ;
#9262=EDGE_CURVE ( 'NONE', #71339, #38980, #26293, .T. ) ;
#9263=CARTESIAN_POINT ( 'NONE',  ( -0.4199475065616791736, 0.2306618581243847221, -0.2411417322834647770 ) ) ;
#9264=CARTESIAN_POINT ( 'NONE',  ( 0.06561679790026316017, -0.3690944881889763329, 0.3153832671262228327 ) ) ;
#9266=CARTESIAN_POINT ( 'NONE',  ( 0.6496062992125991586, 0.07958543189024085140, 0.2665933059059887866 ) ) ;
#9267=CARTESIAN_POINT ( 'NONE',  ( -0.05249343832020911260, 0.2306618581243848609, 0.2411417322834645549 ) ) ;
#9269=CARTESIAN_POINT ( 'NONE',  ( -0.8595800524934373854, -0.3162353388693409650, -0.4822834645669289433 ) ) ;
#9271=CARTESIAN_POINT ( 'NONE',  ( 0.9055118110236227702, -0.5511811023622047445, 6.969142054262312111E-17 ) ) ;
#9272=CARTESIAN_POINT ( 'NONE',  ( 0.1837270341207357105, -0.6046776061558809534, -0.2411417322834644161 ) ) ;
#9273=CARTESIAN_POINT ( 'NONE',  ( -0.2165354330708654795, 0.1660481256975885056, 0.3530559997133364547 ) ) ;
#9274=CARTESIAN_POINT ( 'NONE',  ( -0.5052493438320203589, 0.1771653543307087075, -0.09757992244046823083 ) ) ;
#9276=CARTESIAN_POINT ( 'NONE',  ( -0.6496062992125976043, 0.07958543189024071263, -0.2665933059059888421 ) ) ;
#9277=CARTESIAN_POINT ( 'NONE',  ( 0.3280839895013130669, -0.4281496062992127816, -0.4176697321401328100 ) ) ;
#9278=CARTESIAN_POINT ( 'NONE',  ( -0.9055118110236215490, 0.1771653543307087630, 0.000000000000000000 ) ) ;
#9280=CARTESIAN_POINT ( 'NONE',  ( -1.115485564304461219, 0.05413385826771626580, -0.4176697321401330321 ) ) ;
#9281=LINE ( 'NONE', #8447, #78434 ) ;
#9283=CARTESIAN_POINT ( 'NONE',  ( -1.167979002624671470, -0.3690944881889765550, -0.3153832671262227771 ) ) ;
#9284=CARTESIAN_POINT ( 'NONE',  ( -0.3937007874015740483, -0.1870078740157480879, -0.4822834645669291653 ) ) ;
#9286=CARTESIAN_POINT ( 'NONE',  ( -1.187664041994749731, -0.3162353388693405765, 0.4822834645669290543 ) ) ;
#9287=CARTESIAN_POINT ( 'NONE',  ( 2.795275590551181466, 2.793565526369266916, 0.000000000000000000 ) ) ;
#9288=CARTESIAN_POINT ( 'NONE',  ( 1.476377952755906442, -0.5400638737290844871, 0.3530559997133364547 ) ) ;
#9289=CARTESIAN_POINT ( 'NONE',  ( 0.7086614173228353852, -0.1870078740157479769, 0.4822834645669291653 ) ) ;
#9291=DIRECTION ( 'NONE',  ( -3.096699300667737957E-16, 1.000000000000000000, -0.000000000000000000 ) ) ;
#9292=B_SPLINE_CURVE_WITH_KNOTS ( 'NONE', 3,
 ( #26792, #52449, #71839, #14188, #7868, #33532, #22568 ),
 .UNSPECIFIED., .F., .F.,
 ( 4, 3, 4 ),
 ( 5.551115123125782702E-17, 0.001246230184515611638, 0.002492489877932689731 ),
 .UNSPECIFIED. ) ;
#9293=CARTESIAN_POINT ( 'NONE',  ( 1.456692913385827515, 0.1771653543307087630, 0.000000000000000000 ) ) ;
#9295=VERTEX_POINT ( 'NONE', #3440 ) ;
#9296=CARTESIAN_POINT ( 'NONE',  ( -0.6627296587926501115, 0.1771653543307087075, -0.09757992244046823083 ) ) ;
#9298=EDGE_LOOP ( 'NONE', ( #39317, #3639, #72459, #73369 ) ) ;
#9299=CARTESIAN_POINT ( 'NONE',  ( 0.9251968503937015864, -0.5400638737290844871, 0.3530559997133364547 ) ) ;
#9300=CARTESIAN_POINT ( 'NONE',  ( -0.006561679790025524116, -0.3162353388693405765, 0.4822834645669290543 ) ) ;
#9301=CARTESIAN_POINT ( 'NONE',  ( -0.5905511811023613777, -0.6692913385826771977, 8.415575281601705876E-17 ) ) ;
#9302=CARTESIAN_POINT ( 'NONE',  ( 1.286089238845145033, -0.6046776061558809534, -0.2411417322834644161 ) ) ;
#9303=CARTESIAN_POINT ( 'NONE',  ( -1.496062992125983815, -0.1870078740157479769, 0.3641732283464567677 ) ) ;
#9304=CARTESIAN_POINT ( 'NONE',  ( -0.7478466213799872531, 2.204724409448818978, -0.5309055118110235227 ) ) ;
#9305=CARTESIAN_POINT ( 'NONE',  ( 0.4658792650918641698, -0.05778040916215560624, -0.4822834645669293319 ) ) ;
#9306=CARTESIAN_POINT ( 'NONE',  ( -0.7480314960629914633, -0.6692913385826771977, 8.415575281601705876E-17 ) ) ;
#9308=CARTESIAN_POINT ( 'NONE',  ( -1.312335958005248715, 0.2306618581243848609, 0.2411417322834645549 ) ) ;
#9310=CARTESIAN_POINT ( 'NONE',  ( 1.122047244094488860, -0.5400638737290845981, -0.3530559997133363437 ) ) ;
#9311=CARTESIAN_POINT ( 'NONE',  ( 1.200787401574803681, 0.07958543189024085140, 0.2665933059059887866 ) ) ;
#9314=CARTESIAN_POINT ( 'NONE',  ( -0.4199475065616791736, -0.6046776061558807314, 0.2411417322834647770 ) ) ;
#9316=CARTESIAN_POINT ( 'NONE',  ( 0.2296587926509192634, -0.08942795157528024563, -0.3641732283464568787 ) ) ;
#9317=CARTESIAN_POINT ( 'NONE',  ( -1.259842519685038686, -0.1870078740157479769, 0.4822834645669291653 ) ) ;
#9318=CARTESIAN_POINT ( 'NONE',  ( 1.115485564304462551, 0.05413385826771666132, 0.4176697321401328100 ) ) ;
#9319=CARTESIAN_POINT ( 'NONE',  ( 0.7217847769028878924, -0.4281496062992127816, -0.4176697321401328100 ) ) ;
#9320=CARTESIAN_POINT ( 'NONE',  ( -0.1706036745406816491, -0.4281496062992124485, 0.4176697321401328655 ) ) ;
#9321=CARTESIAN_POINT ( 'NONE',  ( -0.8923884514435688198, -0.6046776061558807314, 0.2411417322834647770 ) ) ;
#9323=CARTESIAN_POINT ( 'NONE',  ( -1.469816272965878357, -0.6046776061558809534, -0.2411417322834644161 ) ) ;
#9324=CARTESIAN_POINT ( 'NONE',  ( -0.6299212598425188991, -0.1870078740157480879, -0.4822834645669291653 ) ) ;
#9325=CARTESIAN_POINT ( 'NONE',  ( -0.5249343832020990641, 0.1283753931104748280, 0.1820866141732283561 ) ) ;
#9326=CARTESIAN_POINT ( 'NONE',  ( 1.279527559055118724, -0.5400638737290845981, -0.3530559997133363437 ) ) ;
#9327=DIRECTION ( 'NONE',  ( 0.000000000000000000, 0.000000000000000000, 1.000000000000000000 ) ) ;
#9328=CARTESIAN_POINT ( 'NONE',  ( -0.9908136482939626788, -0.6692913385826773087, -0.1292274648535924053 ) ) ;
#9330=CARTESIAN_POINT ( 'NONE',  ( 0.6758530183727039509, 0.2952755905511810774, -0.1292274648535930714 ) ) ;
#9332=CARTESIAN_POINT ( 'NONE',  ( -0.6743677390038179675, 1.919528098118540305, -0.5309055118110235227 ) ) ;
#9333=CARTESIAN_POINT ( 'NONE',  ( -0.04593175853018302557, 0.2952755905511811885, 0.1292274648535926551 ) ) ;
#9334=CARTESIAN_POINT ( 'NONE',  ( -1.017060367454067249, -0.08942795157527998196, 0.3641732283464567121 ) ) ;
#9335=CARTESIAN_POINT ( 'NONE',  ( 1.115485564304462551, -0.3690944881889765550, -0.3153832671262227771 ) ) ;
#9337=CARTESIAN_POINT ( 'NONE',  ( 1.122047244094488860, -0.4536011799217368745, -0.2665933059059886201 ) ) ;
#9339=CARTESIAN_POINT ( 'NONE',  ( 0.7939632545931766261, -0.05778040916215522460, 0.4822834645669289988 ) ) ;
#9341=CARTESIAN_POINT ( 'NONE',  ( -0.4002624671916004129, -0.05778040916215560624, -0.4822834645669293319 ) ) ;
#9343=CARTESIAN_POINT ( 'NONE',  ( 1.502624671916010790, -0.2845877964562161244, -0.3641732283464567121 ) ) ;
#9344=CARTESIAN_POINT ( 'NONE',  ( -0.6758530183727028406, -0.6692913385826773087, -0.1292274648535924053 ) ) ;
#9346=CARTESIAN_POINT ( 'NONE',  ( 1.463254593175853824, -0.6692913385826771977, 0.1292274648535927661 ) ) ;
#9347=CARTESIAN_POINT ( 'NONE',  ( 0.2493438320209980519, -0.4281496062992127816, -0.4176697321401328100 ) ) ;
#9348=CARTESIAN_POINT ( 'NONE',  ( 0.4461942257217856311, 0.1283753931104746893, -0.1820866141732285504 ) ) ;
#9349=PLANE ( 'NONE',  #53314 ) ;
#9350=CARTESIAN_POINT ( 'NONE',  ( 0.6036745406824154392, 0.1283753931104746893, -0.1820866141732285504 ) ) ;
#9353=CARTESIAN_POINT ( 'NONE',  ( 0.6824146981627303710, -0.6046776061558807314, 0.2411417322834647770 ) ) ;
#9355=CARTESIAN_POINT ( 'NONE',  ( 0.2255212960314322279, -4.135162568743707313E-16, -0.4118484887281965712 ) ) ;
#9356=CARTESIAN_POINT ( 'NONE',  ( 0.9324623468618423727, 2.784432375088962958E-17, -0.3464511005275205946 ) ) ;
#9357=CARTESIAN_POINT ( 'NONE',  ( -0.006561679790025524116, -0.2845877964562159024, 0.3641732283464567677 ) ) ;
#9358=CARTESIAN_POINT ( 'NONE',  ( 0.01968503937007957949, -0.5400638737290845981, -0.3530559997133363437 ) ) ;
#9359=CARTESIAN_POINT ( 'NONE',  ( 1.476377952755906442, -0.4536011799217367080, 0.2665933059059888421 ) ) ;
#9360=CARTESIAN_POINT ( 'NONE',  ( -1.371391076115484831, 0.1771653543307087075, -0.09757992244046823083 ) ) ;
#9361=CARTESIAN_POINT ( 'NONE',  ( -1.305774278215222184, -0.6692913385826773087, -0.1292274648535924053 ) ) ;
#9362=CARTESIAN_POINT ( 'NONE',  ( 0.5314960629921267055, -0.5400638737290844871, 0.3530559997133364547 ) ) ;
#9363=CARTESIAN_POINT ( 'NONE',  ( 1.076115485564305141, 0.2306618581243847221, -0.2411417322834647770 ) ) ;
#9365=CARTESIAN_POINT ( 'NONE',  ( 0.6627296587926515548, 0.2952755905511811885, 0.1292274648535926551 ) ) ;
#9366=CARTESIAN_POINT ( 'NONE',  ( 1.358267716535433323, 0.1660481256975885056, 0.3530559997133364547 ) ) ;
#9367=CARTESIAN_POINT ( 'NONE',  ( 1.069553805774278832, 0.2952755905511810774, -0.1292274648535930714 ) ) ;
#9369=CARTESIAN_POINT ( 'NONE',  ( 0.6627296587926517768, -0.5511811023622048555, -0.09757992244046775898 ) ) ;
#9370=CARTESIAN_POINT ( 'NONE',  ( -1.607611548556429737, 0.1771653543307087075, -0.09757992244046823083 ) ) ;
#9371=CARTESIAN_POINT ( 'NONE',  ( -0.9645669291338575535, 0.07958543189024071263, -0.2665933059059888421 ) ) ;
#9372=CARTESIAN_POINT ( 'NONE',  ( 0.4002624671916016896, -0.2845877964562161244, -0.3641732283464567121 ) ) ;
#9373=CARTESIAN_POINT ( 'NONE',  ( -0.01312335958005186876, 0.05413385826771626580, -0.4176697321401330321 ) ) ;
#9374=CARTESIAN_POINT ( 'NONE',  ( 0.6758530183727039509, 0.2952755905511810774, -0.1292274648535930714 ) ) ;
#9375=CARTESIAN_POINT ( 'NONE',  ( -0.2296587926509179312, -0.05778040916215522460, 0.4822834645669289988 ) ) ;
#9377=CARTESIAN_POINT ( 'NONE',  ( 0.3215223097112867578, -0.08942795157527998196, 0.3641732283464567121 ) ) ;
#9378=CARTESIAN_POINT ( 'NONE',  ( 1.423884514435696191, -0.05778040916215522460, 0.4822834645669289988 ) ) ;
#9380=CARTESIAN_POINT ( 'NONE',  ( -0.8464566929133852113, -0.5400638737290845981, -0.3530559997133363437 ) ) ;
#9383=CARTESIAN_POINT ( 'NONE',  ( -0.7535225988626923499, 2.401574803149606474, 0.4915354330708645025 ) ) ;
#9384=CARTESIAN_POINT ( 'NONE',  ( -0.8858267716535425107, -0.5400638737290844871, 0.3530559997133364547 ) ) ;
#9385=CARTESIAN_POINT ( 'NONE',  ( -0.6167979002624665030, 0.05413385826771666132, 0.4176697321401328100 ) ) ;
#9388=ORIENTED_EDGE ( 'NONE', *, *, #16612, .T. ) ;
#9389=CARTESIAN_POINT ( 'NONE',  ( 0.6167979002624679463, -0.004921259842519870586, -0.3153832671262229437 ) ) ;
#9391=CARTESIAN_POINT ( 'NONE',  ( 1.259842519685040019, -0.1870078740157479769, 0.4822834645669291653 ) ) ;
#9392=CARTESIAN_POINT ( 'NONE',  ( 0.4996603849959059263, 1.493546695847427719, 0.5309055118110234117 ) ) ;
#9393=CARTESIAN_POINT ( 'NONE',  ( -1.351706036745406347, -0.004921259842519870586, -0.3153832671262229437 ) ) ;
#9394=CARTESIAN_POINT ( 'NONE',  ( 1.594488188976378673, -0.5400638737290845981, -0.3530559997133363437 ) ) ;
#9395=CARTESIAN_POINT ( 'NONE',  ( -1.548556430446193399, 0.2306618581243848609, 0.2411417322834645549 ) ) ;
#9397=CARTESIAN_POINT ( 'NONE',  ( 0.1509186351706045259, -0.05778040916215560624, -0.4822834645669293319 ) ) ;
#9398=CARTESIAN_POINT ( 'NONE',  ( -0.4396325459317579898, 0.1771653543307087630, 0.09757992244046791164 ) ) ;
#9400=CARTESIAN_POINT ( 'NONE',  ( 0.7808398950131240079, -0.3162353388693405765, 0.4822834645669290543 ) ) ;
#9401=CARTESIAN_POINT ( 'NONE',  ( 0.06561679790026316017, 0.05413385826771626580, -0.4176697321401330321 ) ) ;
#9402=CARTESIAN_POINT ( 'NONE',  ( -1.192598508356889520, -5.582469467804009507E-15, -0.3791483426435192650 ) ) ;
#9405=CARTESIAN_POINT ( 'NONE',  ( 0.7217847769028878924, 0.05413385826771666132, 0.4176697321401328100 ) ) ;
#9406=CARTESIAN_POINT ( 'NONE',  ( 0.1312335958005255154, -0.6046776061558807314, 0.2411417322834647770 ) ) ;
#9407=CARTESIAN_POINT ( 'NONE',  ( -0.8530183727034112984, 0.05413385826771666132, 0.4176697321401328100 ) ) ;
#9408=CARTESIAN_POINT ( 'NONE',  ( 1.161417322834646271, 0.1660481256975883668, -0.3530559997133364547 ) ) ;
#9409=CARTESIAN_POINT ( 'NONE',  ( 0.8070866141732289112, -0.5400638737290845981, -0.3530559997133363437 ) ) ;
#9411=CARTESIAN_POINT ( 'NONE',  ( -0.1771653543307080136, -0.5400638737290844871, 0.3530559997133364547 ) ) ;
#9412=CARTESIAN_POINT ( 'NONE',  ( 0.5314960629921267055, -0.5400638737290844871, 0.3530559997133364547 ) ) ;
#9413=CARTESIAN_POINT ( 'NONE',  ( 0.03937007874015833325, -0.6692913385826771977, 8.415575281601705876E-17 ) ) ;
#9414=CARTESIAN_POINT ( 'NONE',  ( 0.6889763779527566800, -0.4536011799217367080, 0.2665933059059888421 ) ) ;
#9415=CARTESIAN_POINT ( 'NONE',  ( -1.240157480314959759, 0.1660481256975885056, 0.3530559997133364547 ) ) ;
#9417=CARTESIAN_POINT ( 'NONE',  ( 0.1312335958005255154, -0.6046776061558807314, 0.2411417322834647770 ) ) ;
#9422=ORIENTED_EDGE ( 'NONE', *, *, #79479, .T. ) ;
#9423=CARTESIAN_POINT ( 'NONE',  ( 1.292650918635171564, -0.6692913385826773087, -0.1292274648535924053 ) ) ;
#9424=CARTESIAN_POINT ( 'NONE',  ( 0.4724409448818904789, -0.1870078740157479769, 0.3641732283464567677 ) ) ;
#9425=CARTESIAN_POINT ( 'NONE',  ( -1.220472440944882386, -3.283890673957456492E-15, 0.4445507791589070057 ) ) ;
#9431=CARTESIAN_POINT ( 'NONE',  ( -0.8923884514435688198, -0.6046776061558807314, 0.2411417322834647770 ) ) ;
#9432=CARTESIAN_POINT ( 'NONE',  ( -0.6496062992125976043, -0.5400638737290844871, 0.3530559997133364547 ) ) ;
#9433=CARTESIAN_POINT ( 'NONE',  ( 0.6627296587926515548, 0.2952755905511811885, 0.1292274648535926551 ) ) ;
#9435=CARTESIAN_POINT ( 'NONE',  ( 1.391076115485564868, -0.6046776061558807314, 0.2411417322834647770 ) ) ;
#9436=CARTESIAN_POINT ( 'NONE',  ( -1.169169330835493126, -3.926852850522101851E-15, 0.3627989612356165572 ) ) ;
#9439=CARTESIAN_POINT ( 'NONE',  ( -1.535433070866141225, -0.5511811023622047445, 6.969142054262312111E-17 ) ) ;
#9441=CARTESIAN_POINT ( 'NONE',  ( 0.3018372703412079971, 0.05413385826771626580, -0.4176697321401330321 ) ) ;
#9442=CARTESIAN_POINT ( 'NONE',  ( 1.673228346456693494, 0.1660481256975885056, 0.3530559997133364547 ) ) ;
#9444=CARTESIAN_POINT ( 'NONE',  ( -1.076115485564303809, 0.1283753931104748280, 0.1820866141732283561 ) ) ;
#9445=CARTESIAN_POINT ( 'NONE',  ( 0.9776902887139113929, -0.6692913385826773087, -0.1292274648535924053 ) ) ;
#9446=CARTESIAN_POINT ( 'NONE',  ( 1.240157480314961314, -0.4536011799217367080, 0.2665933059059888421 ) ) ;
#9448=CARTESIAN_POINT ( 'NONE',  ( -0.9514435695538050464, -0.2845877964562159024, 0.3641732283464567677 ) ) ;
#9449=CARTESIAN_POINT ( 'NONE',  ( 1.437007874015748810, -0.5400638737290845981, -0.3530559997133363437 ) ) ;
#9451=CARTESIAN_POINT ( 'NONE',  ( -0.2821522309711278487, 0.2952755905511811885, 0.1292274648535926551 ) ) ;
#9452=CARTESIAN_POINT ( 'NONE',  ( -1.318897637795274802, 0.07958543189024085140, 0.2665933059059887866 ) ) ;
#9453=CARTESIAN_POINT ( 'NONE',  ( -0.2493438320209966919, -0.004921259842519870586, -0.3153832671262229437 ) ) ;
#9454=CARTESIAN_POINT ( 'NONE',  ( -0.2952755905511804668, 0.1660481256975885056, 0.3530559997133364547 ) ) ;
#9455=CARTESIAN_POINT ( 'NONE',  ( -1.463254593175852492, 0.1771653543307087630, 0.09757992244046791164 ) ) ;
#9457=CARTESIAN_POINT ( 'NONE',  ( 0.4790026246719167324, -0.05778040916215522460, 0.4822834645669289988 ) ) ;
#9458=CARTESIAN_POINT ( 'NONE',  ( 0.4040399068613302891, -1.094630224652485432E-15, 0.4281993546915535687 ) ) ;
#9460=CARTESIAN_POINT ( 'NONE',  ( -1.253280839895012377, -0.05778040916215522460, 0.4822834645669289988 ) ) ;
#9461=CARTESIAN_POINT ( 'NONE',  ( -0.5577427821522301654, -0.08942795157528024563, -0.3641732283464568787 ) ) ;
#9462=CARTESIAN_POINT ( 'NONE',  ( -1.167979002624671470, 0.05413385826771666132, 0.4176697321401328100 ) ) ;
#9463=CARTESIAN_POINT ( 'NONE',  ( -0.07217847769028787330, -0.05778040916215522460, 0.4822834645669289988 ) ) ;
#9464=CARTESIAN_POINT ( 'NONE',  ( 0.5905511811023629321, 0.1771653543307087630, 0.000000000000000000 ) ) ;
#9465=CARTESIAN_POINT ( 'NONE',  ( -0.7217847769028863381, -0.004921259842519870586, -0.3153832671262229437 ) ) ;
#9466=CARTESIAN_POINT ( 'NONE',  ( -0.9448818897637790704, -0.1870078740157479769, 0.4822834645669291653 ) ) ;
#9467=CARTESIAN_POINT ( 'NONE',  ( 1.568241469816273437, -0.2845877964562159024, 0.3641732283464567677 ) ) ;
#9468=CARTESIAN_POINT ( 'NONE',  ( 1.482939632545932307, -0.4281496062992124485, 0.4176697321401328655 ) ) ;
#9470=CARTESIAN_POINT ( 'NONE',  ( 0.6692913385826778638, -0.5511811023622047445, 6.969142054262312111E-17 ) ) ;
#9471=CARTESIAN_POINT ( 'NONE',  ( 0.9317585301837276734, 0.05413385826771626580, -0.4176697321401330321 ) ) ;
#9474=CARTESIAN_POINT ( 'NONE',  ( 1.482939632545932307, -0.004921259842519870586, -0.3153832671262229437 ) ) ;
#9475=VERTEX_POINT ( 'NONE', #60677 ) ;
#9476=CARTESIAN_POINT ( 'NONE',  ( -0.8792650918635160906, -0.4281496062992124485, 0.4176697321401328655 ) ) ;
#9478=CARTESIAN_POINT ( 'NONE',  ( -1.404199475065615932, -0.3690944881889765550, -0.3153832671262227771 ) ) ;
#9479=CARTESIAN_POINT ( 'NONE',  ( -0.7480314960629914633, -0.6692913385826771977, 8.415575281601705876E-17 ) ) ;
#9480=CARTESIAN_POINT ( 'NONE',  ( 0.3937007874015754361, -0.1870078740157480879, -0.4822834645669291653 ) ) ;
#9481=CARTESIAN_POINT ( 'NONE',  ( -1.463254593175852492, -0.5511811023622048555, -0.09757992244046775898 ) ) ;
#9483=CARTESIAN_POINT ( 'NONE',  ( -1.528871391076114250, 0.2952755905511810774, -0.1292274648535930714 ) ) ;
#9484=CARTESIAN_POINT ( 'NONE',  ( 0.4068241469816281097, 0.05413385826771666132, 0.4176697321401328100 ) ) ;
#9485=CARTESIAN_POINT ( 'NONE',  ( 0.03937007874015833325, -0.6692913385826771977, 8.415575281601705876E-17 ) ) ;
#9486=CARTESIAN_POINT ( 'NONE',  ( 0.8989501312335963501, -0.6692913385826773087, -0.1292274648535924053 ) ) ;
#9487=DIRECTION ( 'NONE',  ( 1.000000000000000000, 3.096699300667737957E-16, -1.692413147294446216E-16 ) ) ;
#9491=LINE ( 'NONE', #34757, #17063 ) ;
#9492=APPLICATION_CONTEXT ( 'automotive_design' ) ;
#9494=CARTESIAN_POINT ( 'NONE',  ( -0.09186351706036689768, -0.004921259842519870586, -0.3153832671262229437 ) ) ;
#9495=CARTESIAN_POINT ( 'NONE',  ( -0.2755905511811018171, 0.2952755905511811885, 0.000000000000000000 ) ) ;
#9496=CARTESIAN_POINT ( 'NONE',  ( 1.069553805774278610, -0.6692913385826771977, 0.1292274648535927661 ) ) ;
#9498=CARTESIAN_POINT ( 'NONE',  ( 0.1181102362204730916, 0.1771653543307087630, 0.000000000000000000 ) ) ;
#9499=CARTESIAN_POINT ( 'NONE',  ( -1.240157480314959759, -0.5400638737290845981, -0.3530559997133363437 ) ) ;
#9500=CARTESIAN_POINT ( 'NONE',  ( 1.227034120734908917, -0.6692913385826771977, 0.1292274648535927661 ) ) ;
#9503=CARTESIAN_POINT ( 'NONE',  ( 1.161417322834646271, 0.1660481256975883391, -0.3530559997133364547 ) ) ;
#9505=ORIENTED_EDGE ( 'NONE', *, *, #35324, .F. ) ;
#9506=CARTESIAN_POINT ( 'NONE',  ( 1.069553805774278610, -0.6692913385826771977, 0.1292274648535927661 ) ) ;
#9507=CARTESIAN_POINT ( 'NONE',  ( -1.686351706036744558, 0.2952755905511810774, -0.1292274648535930714 ) ) ;
#9508=CARTESIAN_POINT ( 'NONE',  ( -1.049868766404198794, -0.5023911411419708095, 0.1820866141732285504 ) ) ;
#9509=CARTESIAN_POINT ( 'NONE',  ( -1.220472440944881054, -0.6692913385826771977, 8.415575281601705876E-17 ) ) ;
#9511=CARTESIAN_POINT ( 'NONE',  ( -0.9908136482939625678, 0.2066929133858267931, 0.1054918080437490802 ) ) ;
#9512=CARTESIAN_POINT ( 'NONE',  ( 1.095800524934383846, -0.05778040916215560624, -0.4822834645669293319 ) ) ;
#9514=CARTESIAN_POINT ( 'NONE',  ( -0.1443569553805768291, 0.05413385826771666132, 0.4176697321401328100 ) ) ;
#9515=CARTESIAN_POINT ( 'NONE',  ( -0.5118110236220466680, -0.6692913385826771977, 8.415575281601705876E-17 ) ) ;
#9517=CARTESIAN_POINT ( 'NONE',  ( -1.640419947506561060, 0.05413385826771666132, 0.4176697321401328100 ) ) ;
#9519=CARTESIAN_POINT ( 'NONE',  ( 0.2952755905511816326, -0.5400638737290844871, 0.3530559997133364547 ) ) ;
#9521=CARTESIAN_POINT ( 'NONE',  ( -1.423884514435694859, -0.08942795157528024563, -0.3641732283464568787 ) ) ;
#9522=ORIENTED_EDGE ( 'NONE', *, *, #26035, .F. ) ;
#9525=CARTESIAN_POINT ( 'NONE',  ( 0.5419760673063066525, 1.535433070866141447, 0.4915354330708653907 ) ) ;
#9526=CARTESIAN_POINT ( 'NONE',  ( -1.515748031496062076, 0.1660481256975883668, -0.3530559997133364547 ) ) ;
#9528=CARTESIAN_POINT ( 'NONE',  ( -1.692913385826770645, 0.2952755905511811885, 0.000000000000000000 ) ) ;
#9531=CARTESIAN_POINT ( 'NONE',  ( -0.3805774278215216522, 0.05413385826771666132, 0.4176697321401328100 ) ) ;
#9534=CARTESIAN_POINT ( 'NONE',  ( -0.4593175853018364174, -0.3690944881889765550, -0.3153832671262227771 ) ) ;
#9535=CARTESIAN_POINT ( 'NONE',  ( -0.5839895013123351797, 0.1771653543307087075, -0.09757992244046823083 ) ) ;
#9536=CARTESIAN_POINT ( 'NONE',  ( -1.194225721784776262, -0.4281496062992124485, 0.4176697321401328655 ) ) ;
#9538=CARTESIAN_POINT ( 'NONE',  ( 0.6299212598425204535, -0.1870078740157479769, 0.4822834645669291653 ) ) ;
#9539=CARTESIAN_POINT ( 'NONE',  ( -0.9120734908136475250, -0.6692913385826773087, -0.1292274648535924053 ) ) ;
#9542=ORIENTED_EDGE ( 'NONE', *, *, #81853, .T. ) ;
#9543=CARTESIAN_POINT ( 'NONE',  ( -1.279527559055116948, 0.1660481256975883668, -0.3530559997133364547 ) ) ;
#9546=DIRECTION ( 'NONE',  ( 0.6236670536615054328, 0.6323634944239198141, -0.4595169388576945124 ) ) ;
#9549=CARTESIAN_POINT ( 'NONE',  ( -0.8136482939632537770, 0.2306618581243847221, -0.2411417322834647770 ) ) ;
#9550=CARTESIAN_POINT ( 'NONE',  ( 1.266404199475066328, -0.3162353388693409650, -0.4822834645669289433 ) ) ;
#9552=CARTESIAN_POINT ( 'NONE',  ( -1.699475065616797398, 0.2952755905511811885, 0.1292274648535926551 ) ) ;
#9553=CARTESIAN_POINT ( 'NONE',  ( -0.6692913385826764205, 0.2066929133858268208, 0.000000000000000000 ) ) ;
#9554=CARTESIAN_POINT ( 'NONE',  ( -1.423884514435694859, -0.3162353388693405765, 0.4822834645669290543 ) ) ;
#9555=CARTESIAN_POINT ( 'NONE',  ( -0.9711286089238838626, -0.6046776061558807314, 0.2411417322834647770 ) ) ;
#9557=CARTESIAN_POINT ( 'NONE',  ( 0.3083989501312343062, -0.2845877964562159024, 0.3641732283464567677 ) ) ;
#9559=CARTESIAN_POINT ( 'NONE',  ( 0.1377952755905518800, 0.07958543189024071263, -0.2665933059059888421 ) ) ;
#9560=CARTESIAN_POINT ( 'NONE',  ( 0.9908136482939640111, 0.1771653543307087075, -0.09757992244046823083 ) ) ;
#9561=CARTESIAN_POINT ( 'NONE',  ( 0.9120734908136489683, -0.6692913385826771977, 0.1292274648535927661 ) ) ;
#9562=CARTESIAN_POINT ( 'NONE',  ( -0.1049868766404193215, -0.5023911411419708095, 0.1820866141732285504 ) ) ;
#9564=CARTESIAN_POINT ( 'NONE',  ( -1.614173228346455824, 0.2952755905511811885, 0.000000000000000000 ) ) ;
#9566=CARTESIAN_POINT ( 'NONE',  ( -1.358267716535432434, -0.4536011799217367080, 0.2665933059059888421 ) ) ;
#9568=CARTESIAN_POINT ( 'NONE',  ( -0.2952755905511803003, -0.5400638737290845981, -0.3530559997133363437 ) ) ;
#9569=CARTESIAN_POINT ( 'NONE',  ( 1.640419947506562393, -0.3690944881889763329, 0.3153832671262228327 ) ) ;
#9571=CARTESIAN_POINT ( 'NONE',  ( 0.5708661417322841158, -0.4536011799217368745, -0.2665933059059886201 ) ) ;
#9572=CARTESIAN_POINT ( 'NONE',  ( -0.3280839895013117347, -0.3690944881889763329, 0.3153832671262228327 ) ) ;
#9573=CARTESIAN_POINT ( 'NONE',  ( -0.9251968503937002541, -0.5400638737290845981, -0.3530559997133363437 ) ) ;
#9574=CARTESIAN_POINT ( 'NONE',  ( -1.594488188976377563, -0.5400638737290844871, 0.3530559997133364547 ) ) ;
#9575=DIRECTION ( 'NONE',  ( 0.000000000000000000, 0.000000000000000000, -1.000000000000000000 ) ) ;
#9576=CARTESIAN_POINT ( 'NONE',  ( 0.2034120734908144990, -0.6692913385826771977, 0.1292274648535927661 ) ) ;
#9577=EDGE_LOOP ( 'NONE', ( #12413, #57116, #63450, #41679 ) ) ;
#9579=EDGE_CURVE ( 'NONE', #20803, #6972, #6657, .T. ) ;
#9580=CARTESIAN_POINT ( 'NONE',  ( 1.601049868766404982, 0.2306618581243848609, 0.2411417322834645549 ) ) ;
#9581=CARTESIAN_POINT ( 'NONE',  ( -0.1377952755905504645, 0.07958543189024085140, 0.2665933059059887866 ) ) ;
#9582=CARTESIAN_POINT ( 'NONE',  ( -0.1837270341207343505, -0.6046776061558807314, 0.2411417322834647770 ) ) ;
#9583=CARTESIAN_POINT ( 'NONE',  ( -1.548556430446193399, -0.6046776061558809534, -0.2411417322834644161 ) ) ;
#9584=CARTESIAN_POINT ( 'NONE',  ( -1.482939632545930975, -0.004921259842519576551, 0.3153832671262227771 ) ) ;
#9585=CARTESIAN_POINT ( 'NONE',  ( 1.423884514435696413, -0.3162353388693409650, -0.4822834645669289433 ) ) ;
#9586=CARTESIAN_POINT ( 'NONE',  ( -1.305774278215222184, 0.2952755905511811885, 0.1292274648535926551 ) ) ;
#9587=CARTESIAN_POINT ( 'NONE',  ( -0.7874015748031489847, -0.1870078740157479769, 0.3641732283464567677 ) ) ;
#9592=CARTESIAN_POINT ( 'NONE',  ( 1.482939632545932307, -0.3690944881889763329, 0.3153832671262228327 ) ) ;
#9593=CARTESIAN_POINT ( 'NONE',  ( 1.122047244094488860, 0.07958543189024085140, 0.2665933059059887866 ) ) ;
#9594=CARTESIAN_POINT ( 'NONE',  ( 0.4068241469816281097, 0.009842519685039467087, 0.3409548833797002021 ) ) ;
#9595=CARTESIAN_POINT ( 'NONE',  ( 0.9055118110236227702, -0.6692913385826771977, 8.415575281601705876E-17 ) ) ;
#9597=CARTESIAN_POINT ( 'NONE',  ( 1.423884514435696413, -0.2845877964562161244, -0.3641732283464567121 ) ) ;
#9598=CARTESIAN_POINT ( 'NONE',  ( 0.1771653543307093182, -0.5400638737290845981, -0.3530559997133363437 ) ) ;
#9599=CARTESIAN_POINT ( 'NONE',  ( -0.8267716535433065062, 0.2952755905511811885, 0.000000000000000000 ) ) ;
#9600=CARTESIAN_POINT ( 'NONE',  ( 1.673228346456693494, 0.1660481256975885056, 0.3530559997133364547 ) ) ;
#9603=CARTESIAN_POINT ( 'NONE',  ( 0.4724409448818904789, -0.1870078740157479769, 0.3641732283464567677 ) ) ;
#9607=CARTESIAN_POINT ( 'NONE',  ( -0.4461942257217840213, 0.2306618581243848609, 0.2411417322834645549 ) ) ;
#9608=CARTESIAN_POINT ( 'NONE',  ( 0.7808398950131240079, -0.3162353388693405765, 0.4822834645669290543 ) ) ;
#9609=CARTESIAN_POINT ( 'NONE',  ( -0.3280839895013117347, 0.05413385826771626580, -0.4176697321401330321 ) ) ;
#9610=CARTESIAN_POINT ( 'NONE',  ( -0.1968503937007867743, 0.1771653543307087630, 0.000000000000000000 ) ) ;
#9611=CARTESIAN_POINT ( 'NONE',  ( 0.8267716535433078384, -0.6692913385826771977, 8.415575281601705876E-17 ) ) ;
#9612=CARTESIAN_POINT ( 'NONE',  ( -0.9055118110236215490, -0.6692913385826771977, 8.415575281601705876E-17 ) ) ;
#9613=CARTESIAN_POINT ( 'NONE',  ( -0.2493438320209966919, 0.05413385826771626580, -0.4176697321401330321 ) ) ;
#9614=CARTESIAN_POINT ( 'NONE',  ( 1.299212598425197429, 0.2952755905511811885, 0.000000000000000000 ) ) ;
#9615=CARTESIAN_POINT ( 'NONE',  ( 1.102362204724410155, -0.1870078740157479769, 0.4822834645669291653 ) ) ;
#9616=CARTESIAN_POINT ( 'NONE',  ( 0.7217847769028878924, 0.05413385826771666132, 0.4176697321401328100 ) ) ;
#9618=CARTESIAN_POINT ( 'NONE',  ( -0.1443569553805765515, -0.3690944881889765550, -0.3153832671262227771 ) ) ;
#9619=ORIENTED_EDGE ( 'NONE', *, *, #44498, .T. ) ;
#9622=CARTESIAN_POINT ( 'NONE',  ( -1.056430446194224881, 0.1771653543307087075, -0.09757992244046823083 ) ) ;
#9623=CARTESIAN_POINT ( 'NONE',  ( -0.3149606299212590610, -0.1870078740157480879, -0.4822834645669291653 ) ) ;
#9625=CARTESIAN_POINT ( 'NONE',  ( -0.4790026246719154557, -0.3162353388693405765, 0.4822834645669290543 ) ) ;
#9626=CARTESIAN_POINT ( 'NONE',  ( -0.6036745406824141069, 0.2306618581243848609, 0.2411417322834645549 ) ) ;
#9627=CARTESIAN_POINT ( 'NONE',  ( -1.174540682414697335, -0.05778040916215522460, 0.4822834645669289988 ) ) ;
#9629=CARTESIAN_POINT ( 'NONE',  ( -1.345144356955379816, -0.05778040916215560624, -0.4822834645669293319 ) ) ;
#9630=CARTESIAN_POINT ( 'NONE',  ( 0.9251968503937015864, 0.07958543189024071263, -0.2665933059059888421 ) ) ;
#9631=DIRECTION ( 'NONE',  ( -0.4999999999999965028, 0.8660254037844405950, 0.000000000000000000 ) ) ;
#9633=CARTESIAN_POINT ( 'NONE',  ( 0.6496062992125991586, 0.07958543189024085140, 0.2665933059059887866 ) ) ;
#9634=CARTESIAN_POINT ( 'NONE',  ( 0.1181102362204730916, 0.2952755905511811885, 0.000000000000000000 ) ) ;
#9635=CARTESIAN_POINT ( 'NONE',  ( 0.4593175853018380828, 0.05413385826771626580, -0.4176697321401330321 ) ) ;
#9639=DIRECTION ( 'NONE',  ( 0.000000000000000000, -1.000000000000000000, 0.000000000000000000 ) ) ;
#9640=ORIENTED_EDGE ( 'NONE', *, *, #14239, .F. ) ;
#9643=CARTESIAN_POINT ( 'NONE',  ( -0.6889763779527552368, -0.4536011799217368745, -0.2665933059059886201 ) ) ;
#9644=CARTESIAN_POINT ( 'NONE',  ( -1.082677165354329896, 0.1660481256975885056, 0.3530559997133364547 ) ) ;
#9647=CARTESIAN_POINT ( 'NONE',  ( -1.614173228346455824, 0.1771653543307087630, 0.000000000000000000 ) ) ;
#9648=CARTESIAN_POINT ( 'NONE',  ( 1.010498687664042716, 0.05413385826771626580, -0.4176697321401330321 ) ) ;
#9649=CARTESIAN_POINT ( 'NONE',  ( 0.3149606299212606708, -0.1870078740157480879, -0.4822834645669291653 ) ) ;
#9650=CARTESIAN_POINT ( 'NONE',  ( -0.6036745406824141069, -0.5023911411419708095, -0.1820866141732282451 ) ) ;
#9651=CARTESIAN_POINT ( 'NONE',  ( 0.2624671916010504757, -0.6046776061558809534, -0.2411417322834644161 ) ) ;
#9653=CARTESIAN_POINT ( 'NONE',  ( -0.1706036745406816491, -0.004921259842519870586, -0.3153832671262229437 ) ) ;
#9654=CARTESIAN_POINT ( 'NONE',  ( -0.3937007874015740483, -0.1870078740157480879, -0.4822834645669291653 ) ) ;
#9656=CARTESIAN_POINT ( 'NONE',  ( -1.450131233595799651, -0.6692913385826771977, 0.1292274648535927661 ) ) ;
#9657=CARTESIAN_POINT ( 'NONE',  ( 0.2755905511811031494, -0.5511811023622047445, 6.969142054262312111E-17 ) ) ;
#9659=CARTESIAN_POINT ( 'NONE',  ( -1.266404199475064773, -0.3162353388693405765, 0.4822834645669290543 ) ) ;
#9660=CARTESIAN_POINT ( 'NONE',  ( -0.8267716535433065062, 0.1771653543307087630, 0.000000000000000000 ) ) ;
#9662=CARTESIAN_POINT ( 'NONE',  ( -1.213910761154854745, 0.2952755905511810774, -0.1292274648535930714 ) ) ;
#9663=CARTESIAN_POINT ( 'NONE',  ( -0.5118110236220466680, 0.2952755905511811885, 0.000000000000000000 ) ) ;
#9665=CARTESIAN_POINT ( 'NONE',  ( 0.2427821522309719648, -0.05778040916215522460, 0.4822834645669289988 ) ) ;
#9668=CARTESIAN_POINT ( 'NONE',  ( 0.1706036745406830368, -0.3690944881889765550, -0.3153832671262227771 ) ) ;
#9669=CARTESIAN_POINT ( 'NONE',  ( 1.135170603674541256, 0.2952755905511811885, 0.1292274648535926551 ) ) ;
#9670=CARTESIAN_POINT ( 'NONE',  ( -1.135170603674539924, -0.5511811023622046335, 0.09757992244046803654 ) ) ;
#9671=CARTESIAN_POINT ( 'NONE',  ( 1.115485564304462551, -0.4281496062992127816, -0.4176697321401328100 ) ) ;
#9673=CARTESIAN_POINT ( 'NONE',  ( -0.3346456692913377662, -0.5400638737290844871, 0.3530559997133364547 ) ) ;
#9674=CARTESIAN_POINT ( 'NONE',  ( 0.1968503937007881344, -0.5511811023622047445, 6.969142054262312111E-17 ) ) ;
#9675=CARTESIAN_POINT ( 'NONE',  ( 1.614173228346457378, 0.2753471884572480932, -0.1372047244094471152 ) ) ;
#9676=CARTESIAN_POINT ( 'NONE',  ( 0.4527559055118117182, -0.4536011799217367080, 0.2665933059059888421 ) ) ;
#9677=CARTESIAN_POINT ( 'NONE',  ( -0.1246719160104980823, -0.6692913385826773087, -0.1292274648535924053 ) ) ;
#9679=CARTESIAN_POINT ( 'NONE',  ( -0.9776902887139098386, -0.6692913385826771977, 0.1292274648535927661 ) ) ;
#9681=CARTESIAN_POINT ( 'NONE',  ( 0.9711286089238851948, 0.1283753931104748280, 0.1820866141732283561 ) ) ;
#9682=CARTESIAN_POINT ( 'NONE',  ( 0.1706036745406830368, -0.4281496062992127816, -0.4176697321401328100 ) ) ;
#9683=CARTESIAN_POINT ( 'NONE',  ( -0.2099737532808391705, 0.2306618581243848609, 0.2411417322834645549 ) ) ;
#9684=CARTESIAN_POINT ( 'NONE',  ( -0.2099737532808391705, 0.1283753931104748280, 0.1820866141732283561 ) ) ;
#9686=CARTESIAN_POINT ( 'NONE',  ( -0.6364829396325453192, -0.08942795157528024563, -0.3641732283464568787 ) ) ;
#9687=CARTESIAN_POINT ( 'NONE',  ( 0.1837270341207357105, -0.6046776061558809534, -0.2411417322834644161 ) ) ;
#9688=CARTESIAN_POINT ( 'NONE',  ( -1.312335958005248715, -0.5023911411419708095, -0.1820866141732282451 ) ) ;
#9690=CARTESIAN_POINT ( 'NONE',  ( -0.9908136482939626788, 0.2952755905511811885, 0.1292274648535926551 ) ) ;
#9691=CARTESIAN_POINT ( 'NONE',  ( -1.436417322834644850, 0.8346805926620876059, 0.3149606299212598381 ) ) ;
#9692=ORIENTED_EDGE ( 'NONE', *, *, #55305, .F. ) ;
#9693=CARTESIAN_POINT ( 'NONE',  ( -1.732283464566928277, -0.1870078740157479769, 0.3641732283464567677 ) ) ;
#9695=CARTESIAN_POINT ( 'NONE',  ( -0.4461942257217840213, 0.2306618581243848609, 0.2411417322834645549 ) ) ;
#9697=CARTESIAN_POINT ( 'NONE',  ( -1.286089238845143479, 0.2306618581243847221, -0.2411417322834647770 ) ) ;
#9699=DIRECTION ( 'NONE',  ( 0.000000000000000000, -1.000000000000000000, 0.000000000000000000 ) ) ;
#9700=CARTESIAN_POINT ( 'NONE',  ( 1.430446194225722500, -0.4281496062992127816, -0.4176697321401328100 ) ) ;
#9701=CARTESIAN_POINT ( 'NONE',  ( 1.017060367454068803, -0.3162353388693405765, 0.4822834645669290543 ) ) ;
#9702=CARTESIAN_POINT ( 'NONE',  ( -0.2624671916010490880, 0.1539470093639521697, -0.1968503937007875793 ) ) ;
#9704=CARTESIAN_POINT ( 'NONE',  ( 1.404199475065617264, -0.3690944881889763329, 0.3153832671262228327 ) ) ;
#9707=CARTESIAN_POINT ( 'NONE',  ( -0.5511811023622038563, -0.1870078740157479769, 0.3641732283464567677 ) ) ;
#9710=CARTESIAN_POINT ( 'NONE',  ( 0.7742782152230978099, -0.4281496062992124485, 0.4176697321401328655 ) ) ;
#9711=CARTESIAN_POINT ( 'NONE',  ( -0.2427821522309703550, -0.05778040916215560624, -0.4822834645669293319 ) ) ;
#9712=CARTESIAN_POINT ( 'NONE',  ( -1.148293963254592542, 0.2952755905511811885, 0.1292274648535926551 ) ) ;
#9713=CARTESIAN_POINT ( 'NONE',  ( 1.646981627296588035, -0.3162353388693405765, 0.4822834645669290543 ) ) ;
#9714=CARTESIAN_POINT ( 'NONE',  ( -1.469816272965878357, 0.1283753931104748280, 0.1820866141732283561 ) ) ;
#9716=CARTESIAN_POINT ( 'NONE',  ( 0.2099737532808405305, -0.6046776061558807314, 0.2411417322834647770 ) ) ;
#9717=CARTESIAN_POINT ( 'NONE',  ( -0.7742782152230962556, -0.4281496062992127816, -0.4176697321401328100 ) ) ;
#9719=CARTESIAN_POINT ( 'NONE',  ( -1.332020997375327642, -0.05778040916215522460, 0.4822834645669289988 ) ) ;
#9721=CARTESIAN_POINT ( 'NONE',  ( 1.135170603674541256, -0.6692913385826773087, -0.1292274648535924053 ) ) ;
#9722=CARTESIAN_POINT ( 'NONE',  ( 1.181102362204725198, -0.1870078740157479769, 0.3641732283464567677 ) ) ;
#9723=ORIENTED_EDGE ( 'NONE', *, *, #7244, .F. ) ;
#9725=CARTESIAN_POINT ( 'NONE',  ( -0.4265091863517051496, -0.6692913385826771977, 0.1292274648535927661 ) ) ;
#9727=CARTESIAN_POINT ( 'NONE',  ( 0.4199475065616803948, -0.5023911411419708095, -0.1820866141732282451 ) ) ;
#9728=CARTESIAN_POINT ( 'NONE',  ( -1.279527559055116948, -0.5400638737290844871, 0.3530559997133364547 ) ) ;
#9729=CARTESIAN_POINT ( 'NONE',  ( 0.9120734908136489683, -0.6692913385826771977, 0.1292274648535927661 ) ) ;
#9730=CARTESIAN_POINT ( 'NONE',  ( 0.8989501312335963501, -0.6692913385826773087, -0.1292274648535924053 ) ) ;
#9732=CARTESIAN_POINT ( 'NONE',  ( -0.2493438320209966919, 0.05413385826771626580, -0.4176697321401330321 ) ) ;
#9734=CARTESIAN_POINT ( 'NONE',  ( -0.8136482939632537770, 0.2306618581243847221, -0.2411417322834647770 ) ) ;
#9736=CARTESIAN_POINT ( 'NONE',  ( -1.561679790026246017, 0.05413385826771666132, 0.4176697321401328100 ) ) ;
#9737=CARTESIAN_POINT ( 'NONE',  ( -0.6692913385826764205, 0.2952755905511811885, 0.000000000000000000 ) ) ;
#9738=CARTESIAN_POINT ( 'NONE',  ( 1.332020997375329197, -0.3162353388693405765, 0.4822834645669290543 ) ) ;
#9739=CARTESIAN_POINT ( 'NONE',  ( 1.404199475065617708, 0.05413385826771626580, -0.4176697321401330321 ) ) ;
#9740=CARTESIAN_POINT ( 'NONE',  ( -0.9448818897637790704, -0.1870078740157479769, 0.4822834645669291653 ) ) ;
#9742=CARTESIAN_POINT ( 'NONE',  ( 0.6889763779527563470, 0.1660481256975883668, -0.3530559997133364547 ) ) ;
#9744=CARTESIAN_POINT ( 'NONE',  ( -0.4593175853018364174, -0.4281496062992127816, -0.4176697321401328100 ) ) ;
#9745=CARTESIAN_POINT ( 'NONE',  ( -1.430446194225720724, -0.004921259842519870586, -0.3153832671262229437 ) ) ;
#9746=CARTESIAN_POINT ( 'NONE',  ( 0.6167979002624679463, -0.004921259842519870586, -0.3153832671262229437 ) ) ;
#9748=CARTESIAN_POINT ( 'NONE',  ( 1.049868766404200349, 0.1283753931104748280, 0.1820866141732283561 ) ) ;
#9749=CARTESIAN_POINT ( 'NONE',  ( 0.8923884514435701520, -0.6046776061558809534, -0.2411417322834644161 ) ) ;
#9751=CARTESIAN_POINT ( 'NONE',  ( -0.4396325459317579898, 0.2952755905511811885, 0.1292274648535926551 ) ) ;
#9753=CARTESIAN_POINT ( 'NONE',  ( 1.410761154855643795, -0.2845877964562159024, 0.3641732283464567677 ) ) ;
#9754=CARTESIAN_POINT ( 'NONE',  ( -0.5971128608923877978, 0.2952755905511811885, 0.1292274648535926551 ) ) ;
#9756=CARTESIAN_POINT ( 'NONE',  ( 1.371391076115485941, 0.2952755905511811885, 0.1292274648535926551 ) ) ;
#9757=CARTESIAN_POINT ( 'NONE',  ( 0.2755905511811031494, -0.6692913385826771977, 8.415575281601705876E-17 ) ) ;
#9759=CARTESIAN_POINT ( 'NONE',  ( 0.6955380577427828781, -0.3690944881889763329, 0.3153832671262228327 ) ) ;
#9761=CARTESIAN_POINT ( 'NONE',  ( 0.07874015748031558404, -0.1870078740157479769, 0.3641732283464567677 ) ) ;
#9762=CARTESIAN_POINT ( 'NONE',  ( -1.502624671916009680, -0.3162353388693405765, 0.4822834645669290543 ) ) ;
#9764=CARTESIAN_POINT ( 'NONE',  ( 0.8464566929133866546, -0.5400638737290844871, 0.3530559997133364547 ) ) ;
#9766=CARTESIAN_POINT ( 'NONE',  ( 1.489501312335958172, -0.2845877964562159024, 0.3641732283464567677 ) ) ;
#9768=CARTESIAN_POINT ( 'NONE',  ( -0.07874015748031421014, -0.1870078740157480601, -0.3641732283464567677 ) ) ;
#9769=CARTESIAN_POINT ( 'NONE',  ( 0.09842519685039434474, 0.1660481256975885056, 0.3530559997133364547 ) ) ;
#9770=CARTESIAN_POINT ( 'NONE',  ( 1.272965879265092637, -0.3690944881889765550, -0.3153832671262227771 ) ) ;
#9771=CARTESIAN_POINT ( 'NONE',  ( -1.305774278215222184, -0.5511811023622048555, -0.09757992244046775898 ) ) ;
#9772=CARTESIAN_POINT ( 'NONE',  ( -1.587926509186350810, -0.4281496062992124485, 0.4176697321401328655 ) ) ;
#9773=CARTESIAN_POINT ( 'NONE',  ( 0.4330708661417329575, 0.2952755905511811885, 0.000000000000000000 ) ) ;
#9774=CARTESIAN_POINT ( 'NONE',  ( 1.358267716535433323, 0.1660481256975885056, 0.3530559997133364547 ) ) ;
#9776=CARTESIAN_POINT ( 'NONE',  ( -0.03937007874015669567, -0.6692913385826771977, 8.415575281601705876E-17 ) ) ;
#9777=CARTESIAN_POINT ( 'NONE',  ( 1.181102362204725198, -0.1870078740157479769, 0.4822834645669291653 ) ) ;
#9778=CARTESIAN_POINT ( 'NONE',  ( 0.9645669291338591078, -0.5400638737290845981, -0.3530559997133363437 ) ) ;
#9781=CARTESIAN_POINT ( 'NONE',  ( 0.8267716535433078384, -0.5511811023622047445, 6.969142054262312111E-17 ) ) ;
#9782=CARTESIAN_POINT ( 'NONE',  ( 1.443569553805774897, -0.6046776061558809534, -0.2411417322834644161 ) ) ;
#9783=CARTESIAN_POINT ( 'NONE',  ( -0.8792650918635160906, -0.3690944881889763329, 0.3153832671262228327 ) ) ;
#9784=CARTESIAN_POINT ( 'NONE',  ( 0.3608923884514443348, 0.1771653543307087075, -0.09757992244046823083 ) ) ;
#9785=CARTESIAN_POINT ( 'NONE',  ( -0.02624671916010428221, 0.2306618581243847221, -0.2411417322834647770 ) ) ;
#9786=CARTESIAN_POINT ( 'NONE',  ( 0.7086614173228352742, -0.1870078740157480879, -0.4822834645669291653 ) ) ;
#9787=CARTESIAN_POINT ( 'NONE',  ( -0.2559055118110227234, -0.5400638737290844871, 0.3530559997133364547 ) ) ;
#9788=CARTESIAN_POINT ( 'NONE',  ( 0.03280839895013198948, 0.1771653543307087630, 0.09757992244046791164 ) ) ;
#9789=CARTESIAN_POINT ( 'NONE',  ( 0.8464566929133865436, 0.1660481256975883668, -0.3530559997133364547 ) ) ;
#9790=CARTESIAN_POINT ( 'NONE',  ( 2.787279214012418738, 0.000000000000000000, 0.000000000000000000 ) ) ;
#9791=CARTESIAN_POINT ( 'NONE',  ( -0.8398950131233589023, -0.6046776061558809534, -0.2411417322834644161 ) ) ;
#9795=CARTESIAN_POINT ( 'NONE',  ( -1.338582677165353729, -0.1870078740157479769, 0.4822834645669291653 ) ) ;
#9796=CARTESIAN_POINT ( 'NONE',  ( -0.6692913385826764205, -0.6692913385826771977, 8.415575281601705876E-17 ) ) ;
#9800=CARTESIAN_POINT ( 'NONE',  ( 0.7480314960629927956, 0.1771653543307087630, 0.000000000000000000 ) ) ;
#9801=VECTOR ( 'NONE', #4463, 39.37007874015748854 ) ;
#9803=CARTESIAN_POINT ( 'NONE',  ( 1.003937007874016185, 0.1660481256975883668, -0.3530559997133364547 ) ) ;
#9804=DIRECTION ( 'NONE',  ( -3.096699300667737957E-16, 1.000000000000000000, -0.000000000000000000 ) ) ;
#9805=CARTESIAN_POINT ( 'NONE',  ( -1.423884514435694859, -0.2845877964562159024, 0.3641732283464567677 ) ) ;
#9807=CARTESIAN_POINT ( 'NONE',  ( -1.555118110236219930, 0.1660481256975885056, 0.3530559997133364547 ) ) ;
#9808=CARTESIAN_POINT ( 'NONE',  ( 0.2624671916010504757, 0.2306618581243848609, 0.2411417322834645549 ) ) ;
#9810=CARTESIAN_POINT ( 'NONE',  ( 0.1706036745406830368, -0.4281496062992127816, -0.4176697321401328100 ) ) ;
#9811=CARTESIAN_POINT ( 'NONE',  ( -0.9842519685039365918, -0.5511811023622047445, 6.969142054262312111E-17 ) ) ;
#9812=CARTESIAN_POINT ( 'NONE',  ( 0.9711286089238851948, 0.2306618581243848609, 0.2411417322834645549 ) ) ;
#9814=CARTESIAN_POINT ( 'NONE',  ( -0.1181102362204717315, 0.2952755905511811885, 0.000000000000000000 ) ) ;
#9815=CARTESIAN_POINT ( 'NONE',  ( -1.603475055217291612, 2.094628720676861011, -0.04573490813648263542 ) ) ;
#9816=CARTESIAN_POINT ( 'NONE',  ( -0.01241954290193713825, 2.784432375088962958E-17, -0.3464511005275205946 ) ) ;
#9818=CARTESIAN_POINT ( 'NONE',  ( 0.7874015748031503170, -0.1870078740157480879, -0.4822834645669291653 ) ) ;
#9819=CARTESIAN_POINT ( 'NONE',  ( 0.1246719160104994284, -0.6692913385826771977, 0.1292274648535927661 ) ) ;
#9820=CARTESIAN_POINT ( 'NONE',  ( -0.8727034120734901146, -0.3162353388693405765, 0.4822834645669290543 ) ) ;
#9821=CARTESIAN_POINT ( 'NONE',  ( 1.056430446194226436, -0.6692913385826773087, -0.1292274648535924053 ) ) ;
#9823=CARTESIAN_POINT ( 'NONE',  ( 0.3674540682414705883, -0.6046776061558807314, 0.2411417322834647770 ) ) ;
#9825=CARTESIAN_POINT ( 'NONE',  ( -0.3149606299212590610, -0.1870078740157479769, 0.4822834645669291653 ) ) ;
#9826=CARTESIAN_POINT ( 'NONE',  ( 0.6102362204724416372, 0.1660481256975883668, -0.3530559997133364547 ) ) ;
#9827=CARTESIAN_POINT ( 'NONE',  ( -0.1181102362204717315, -0.6692913385826771977, 8.415575281601705876E-17 ) ) ;
#9828=CARTESIAN_POINT ( 'NONE',  ( 0.6167979002624679463, -0.004921259842519870586, -0.3153832671262229437 ) ) ;
#9829=CARTESIAN_POINT ( 'NONE',  ( -1.443569553805773564, -0.6046776061558807314, 0.2411417322834647770 ) ) ;
#9831=CARTESIAN_POINT ( 'NONE',  ( 0.1706036745406830368, 0.05413385826771666132, 0.4176697321401328100 ) ) ;
#9836=CARTESIAN_POINT ( 'NONE',  ( 1.167979002624672580, -0.4281496062992124485, 0.4176697321401328655 ) ) ;
#9837=CARTESIAN_POINT ( 'NONE',  ( 0.5708661417322841158, -0.4536011799217368745, -0.2665933059059886201 ) ) ;
#9841=FACE_OUTER_BOUND ( 'NONE', #23892, .T. ) ;
#9845=CARTESIAN_POINT ( 'NONE',  ( 0.9645669291338588858, 0.1660481256975885056, 0.3530559997133364547 ) ) ;
#9846=CARTESIAN_POINT ( 'NONE',  ( -0.8989501312335946848, -0.6692913385826771977, 0.1292274648535927661 ) ) ;
#9848=CARTESIAN_POINT ( 'NONE',  ( -0.8989501312335946848, 0.2952755905511810774, -0.1292274648535930714 ) ) ;
#9849=CARTESIAN_POINT ( 'NONE',  ( 0.5380577427821529035, 0.05413385826771626580, -0.4176697321401330321 ) ) ;
#9851=CARTESIAN_POINT ( 'NONE',  ( 1.233595800524935227, -0.6046776061558807314, 0.2411417322834647770 ) ) ;
#9856=CARTESIAN_POINT ( 'NONE',  ( -1.377952755905511140, -0.5511811023622047445, 6.969142054262312111E-17 ) ) ;
#9858=CARTESIAN_POINT ( 'NONE',  ( 0.3608923884514443348, -0.6692913385826771977, 0.1292274648535927661 ) ) ;
#9861=CARTESIAN_POINT ( 'NONE',  ( -1.049868766404198794, 0.1283753931104746893, -0.1820866141732285504 ) ) ;
#9862=CARTESIAN_POINT ( 'NONE',  ( 0.3215223097112867578, -0.3162353388693409650, -0.4822834645669289433 ) ) ;
#9863=CARTESIAN_POINT ( 'NONE',  ( 1.253280839895013710, -0.2845877964562159024, 0.3641732283464567677 ) ) ;
#9866=CARTESIAN_POINT ( 'NONE',  ( -1.122047244094487306, -0.4536011799217367080, 0.2665933059059888421 ) ) ;
#9867=CARTESIAN_POINT ( 'NONE',  ( 1.259842519685040019, -0.1870078740157480879, -0.4822834645669291653 ) ) ;
#9869=CARTESIAN_POINT ( 'NONE',  ( -0.3608923884514428360, -0.6692913385826773087, -0.1292274648535924053 ) ) ;
#9870=CARTESIAN_POINT ( 'NONE',  ( -1.364829396325458521, -0.5023911411419708095, 0.1820866141732285504 ) ) ;
#9871=CARTESIAN_POINT ( 'NONE',  ( -0.3346456692913377662, -0.4536011799217367080, 0.2665933059059888421 ) ) ;
#9872=CARTESIAN_POINT ( 'NONE',  ( -0.7152230971128602510, -0.05778040916215560624, -0.4822834645669293319 ) ) ;
#9873=CARTESIAN_POINT ( 'NONE',  ( -1.450131233595799651, 0.1771653543307087075, -0.09757992244046823083 ) ) ;
#9875=CARTESIAN_POINT ( 'NONE',  ( 0.1771653543307093182, 0.1660481256975885056, 0.3530559997133364547 ) ) ;
#9878=CARTESIAN_POINT ( 'NONE',  ( -1.207349081364828880, 0.2306618581243847221, -0.2411417322834647770 ) ) ;
#9879=CARTESIAN_POINT ( 'NONE',  ( -0.6364829396325453192, -0.2845877964562159024, 0.3641732283464567677 ) ) ;
#9880=CARTESIAN_POINT ( 'NONE',  ( -1.568241469816272105, -0.3162353388693409650, -0.4822834645669289433 ) ) ;
#9881=CARTESIAN_POINT ( 'NONE',  ( -0.01968503937007793844, 0.1660481256975883668, -0.3530559997133364547 ) ) ;
#9882=CARTESIAN_POINT ( 'NONE',  ( 0.2427821522309719648, -0.08942795157527998196, 0.3641732283464567121 ) ) ;
#9883=CARTESIAN_POINT ( 'NONE',  ( -1.017060367454067249, -0.2845877964562161244, -0.3641732283464567121 ) ) ;
#9884=CARTESIAN_POINT ( 'NONE',  ( -1.456692913385826182, -0.6692913385826771977, 8.415575281601705876E-17 ) ) ;
#9885=CARTESIAN_POINT ( 'NONE',  ( -1.469816272965878357, -0.6046776061558809534, -0.2411417322834644161 ) ) ;
#9886=CARTESIAN_POINT ( 'NONE',  ( 1.312335958005250269, -0.6046776061558807314, 0.2411417322834647770 ) ) ;
#9888=CARTESIAN_POINT ( 'NONE',  ( 0.4658792650918641698, -0.08942795157528024563, -0.3641732283464568787 ) ) ;
#9889=CARTESIAN_POINT ( 'NONE',  ( 0.7742782152230979209, 0.05413385826771626580, -0.4176697321401330321 ) ) ;
#9890=DIRECTION ( 'NONE',  ( 3.096699300667737957E-16, -1.000000000000000000, 0.000000000000000000 ) ) ;
#9891=CARTESIAN_POINT ( 'NONE',  ( 1.332020997375328974, -0.08942795157528024563, -0.3641732283464568787 ) ) ;
#9893=CARTESIAN_POINT ( 'NONE',  ( -1.069553805774277722, -0.6692913385826773087, -0.1292274648535924053 ) ) ;
#9894=CARTESIAN_POINT ( 'NONE',  ( -0.9645669291338575535, 0.1660481256975883668, -0.3530559997133364547 ) ) ;
#9895=CARTESIAN_POINT ( 'NONE',  ( 0.3871391076115492380, -0.05778040916215560624, -0.4822834645669293319 ) ) ;
#9896=CARTESIAN_POINT ( 'NONE',  ( -1.423884514435694859, -0.2845877964562159024, 0.3641732283464567677 ) ) ;
#9898=CARTESIAN_POINT ( 'NONE',  ( 1.574803149606299746, -0.1870078740157479769, 0.3641732283464567677 ) ) ;
#9899=CARTESIAN_POINT ( 'NONE',  ( 0.2362204724409456558, -0.1870078740157479769, 0.4822834645669291653 ) ) ;
#9900=CARTESIAN_POINT ( 'NONE',  ( 0.8267716535433077274, 0.2952755905511811885, 0.000000000000000000 ) ) ;
#9905=DIRECTION ( 'NONE',  ( 0.000000000000000000, -0.000000000000000000, 1.000000000000000000 ) ) ;
#9907=CARTESIAN_POINT ( 'NONE',  ( -0.09842519685039295696, 0.07958543189024071263, -0.2665933059059888421 ) ) ;
#9908=CARTESIAN_POINT ( 'NONE',  ( -0.3543307086614165824, -0.6692913385826771977, 8.415575281601705876E-17 ) ) ;
#9909=CARTESIAN_POINT ( 'NONE',  ( 1.082677165354331228, -0.5400638737290844871, 0.3530559997133364547 ) ) ;
#9911=CARTESIAN_POINT ( 'NONE',  ( -0.1771653543307080136, 0.07958543189024071263, -0.2665933059059888421 ) ) ;
#9912=CARTESIAN_POINT ( 'NONE',  ( -0.9448818897637790704, -0.1870078740157480879, -0.4822834645669291653 ) ) ;
#9913=CARTESIAN_POINT ( 'NONE',  ( 1.036745406824147508, -0.4281496062992127816, -0.4176697321401328100 ) ) ;
#9917=VERTEX_POINT ( 'NONE', #30753 ) ;
#9918=CARTESIAN_POINT ( 'NONE',  ( 0.8333333333333340365, 0.2952755905511810774, -0.1292274648535930714 ) ) ;
#9919=VECTOR ( 'NONE', #21831, 39.37007874015748143 ) ;
#9920=CARTESIAN_POINT ( 'NONE',  ( -1.502624671916009680, -0.05778040916215560624, -0.4822834645669293319 ) ) ;
#9921=CARTESIAN_POINT ( 'NONE',  ( 1.548556430446194954, 0.2306618581243847221, -0.2411417322834647770 ) ) ;
#9922=CARTESIAN_POINT ( 'NONE',  ( -1.640419947506561060, 0.05413385826771666132, 0.4176697321401328100 ) ) ;
#9924=CARTESIAN_POINT ( 'NONE',  ( -1.003937007874014853, 0.1012011053420777407, 0.2882089793578256898 ) ) ;
#9925=CARTESIAN_POINT ( 'NONE',  ( 1.266404199475066328, -0.3162353388693409650, -0.4822834645669289433 ) ) ;
#9927=CARTESIAN_POINT ( 'NONE',  ( -0.1837270341207343505, -0.6046776061558807314, 0.2411417322834647770 ) ) ;
#9928=CARTESIAN_POINT ( 'NONE',  ( -0.6692913385826764205, -0.6692913385826771977, 8.415575281601705876E-17 ) ) ;
#9929=CARTESIAN_POINT ( 'NONE',  ( 1.614173228346457378, 0.2952755905511811885, 0.000000000000000000 ) ) ;
#9931=CARTESIAN_POINT ( 'NONE',  ( 0.2230971128608929543, 0.05413385826771626580, -0.4176697321401330321 ) ) ;
#9933=CARTESIAN_POINT ( 'NONE',  ( -1.482939632545930975, -0.004921259842519576551, 0.3153832671262227771 ) ) ;
#9936=VERTEX_POINT ( 'NONE', #82519 ) ;
#9938=CARTESIAN_POINT ( 'NONE',  ( -1.666666666666665853, 0.05413385826771626580, -0.4176697321401330321 ) ) ;
#9940=CARTESIAN_POINT ( 'NONE',  ( 0.5626772485143710645, 7.570362723507360306E-16, 0.3791483426435171555 ) ) ;
#9945=CARTESIAN_POINT ( 'NONE',  ( -0.2362204724409440182, -0.1870078740157479769, 0.3641732283464567677 ) ) ;
#9946=CARTESIAN_POINT ( 'NONE',  ( -0.8923884514435688198, 0.1283753931104746893, -0.1820866141732285504 ) ) ;
#9947=CARTESIAN_POINT ( 'NONE',  ( -1.036745406824146176, -0.4281496062992124485, 0.4176697321401328655 ) ) ;
#9948=CARTESIAN_POINT ( 'NONE',  ( 0.7020997375328090762, -0.05778040916215560624, -0.4822834645669293319 ) ) ;
#9949=CARTESIAN_POINT ( 'NONE',  ( -1.476377952755905110, 0.1660481256975885056, 0.3530559997133364547 ) ) ;
#9952=EDGE_CURVE ( 'NONE', #60445, #26484, #56416, .T. ) ;
#9954=CARTESIAN_POINT ( 'NONE',  ( -1.227034120734907141, -0.6692913385826773087, -0.1292274648535924053 ) ) ;
#9955=LINE ( 'NONE', #35626, #23194 ) ;
#9961=FACE_OUTER_BOUND ( 'NONE', #63745, .T. ) ;
#9962=CARTESIAN_POINT ( 'NONE',  ( -0.8595800524934373854, -0.05778040916215522460, 0.4822834645669289988 ) ) ;
#9963=CARTESIAN_POINT ( 'NONE',  ( 1.587926509186352586, -0.4281496062992127816, -0.4176697321401328100 ) ) ;
#9966=CARTESIAN_POINT ( 'NONE',  ( 1.673228346456693494, 0.1660481256975885056, 0.3530559997133364547 ) ) ;
#9967=CARTESIAN_POINT ( 'NONE',  ( -0.8530183727034112984, -0.4281496062992127816, -0.4176697321401328100 ) ) ;
#9969=B_SPLINE_CURVE_WITH_KNOTS ( 'NONE', 3,
 ( #65544, #33121, #46151, #33539 ),
 .UNSPECIFIED., .F., .F.,
 ( 4, 4 ),
 ( 3.593986969187450165E-07, 0.001287825409103264106 ),
 .UNSPECIFIED. ) ;
#9970=CARTESIAN_POINT ( 'NONE',  ( 0.1181102362204730916, -0.5511811023622047445, 6.969142054262312111E-17 ) ) ;
#9973=CARTESIAN_POINT ( 'NONE',  ( -0.1377952755905504645, -0.4536011799217368745, -0.2665933059059886201 ) ) ;
#9974=CARTESIAN_POINT ( 'NONE',  ( 0.9711286089238851948, 0.1283753931104748280, 0.1820866141732283561 ) ) ;
#9975=CARTESIAN_POINT ( 'NONE',  ( 0.6955380577427828781, 0.05413385826771626580, -0.4176697321401330321 ) ) ;
#9976=PRODUCT_DEFINITION_CONTEXT ( 'detailed design', #45472, 'design' ) ;
#9977=CARTESIAN_POINT ( 'NONE',  ( -0.3740157480314953431, 0.07958543189024085140, 0.2665933059059887866 ) ) ;
#9979=CARTESIAN_POINT ( 'NONE',  ( -1.568241469816272105, -0.3162353388693409650, -0.4822834645669289433 ) ) ;
#9980=EDGE_CURVE ( 'NONE', #7209, #75163, #77940, .T. ) ;
#9981=CARTESIAN_POINT ( 'NONE',  ( -1.377952755905511140, -0.5511811023622047445, 6.969142054262312111E-17 ) ) ;
#9983=CARTESIAN_POINT ( 'NONE',  ( 0.1049868766404206816, -0.6046776061558809534, -0.2411417322834644161 ) ) ;
#9984=EDGE_CURVE ( 'NONE', #55534, #1065, #26410, .T. ) ;
#9985=CARTESIAN_POINT ( 'NONE',  ( -0.5511811023622038563, -0.1870078740157479769, 0.4822834645669291653 ) ) ;
#9986=CARTESIAN_POINT ( 'NONE',  ( 1.686351706036745890, 0.1771653543307087630, 0.09757992244046791164 ) ) ;
#9988=CARTESIAN_POINT ( 'NONE',  ( 0.4986876640419954376, 0.1283753931104748280, 0.1820866141732283561 ) ) ;
#9989=CARTESIAN_POINT ( 'NONE',  ( -0.1771653543307080136, -0.5400638737290844871, 0.3530559997133364547 ) ) ;
#9990=CARTESIAN_POINT ( 'NONE',  ( -0.5905511811023613777, -0.6692913385826771977, 8.415575281601705876E-17 ) ) ;
#9993=CARTESIAN_POINT ( 'NONE',  ( -0.03937007874015669567, 0.2952755905511811885, 0.000000000000000000 ) ) ;
#9994=EDGE_LOOP ( 'NONE', ( #81531, #69446, #25715, #3520 ) ) ;
#9996=CARTESIAN_POINT ( 'NONE',  ( 1.509186351706037543, -0.4281496062992127816, -0.4176697321401328100 ) ) ;
#9997=CARTESIAN_POINT ( 'NONE',  ( -0.2034120734908131112, -0.5511811023622048555, -0.09757992244046775898 ) ) ;
#9998=CARTESIAN_POINT ( 'NONE',  ( -0.6102362204724400829, 0.1660481256975885056, 0.3530559997133364547 ) ) ;
#9999=CARTESIAN_POINT ( 'NONE',  ( -1.522309711286088607, -0.5023911411419708095, 0.1820866141732285504 ) ) ;
#10000=CARTESIAN_POINT ( 'NONE',  ( 1.522309711286089939, 0.2306618581243848609, 0.2411417322834645549 ) ) ;
#10001=CARTESIAN_POINT ( 'NONE',  ( -1.646981627296586703, -0.05778040916215522460, 0.4822834645669289988 ) ) ;
#10002=CARTESIAN_POINT ( 'NONE',  ( -0.8070866141732276899, -0.4536011799217367080, 0.2665933059059888421 ) ) ;
#10006=CARTESIAN_POINT ( 'NONE',  ( 1.456692913385827515, -0.5511811023622047445, 6.969142054262312111E-17 ) ) ;
#10007=CARTESIAN_POINT ( 'NONE',  ( 0.9842519685039375910, 0.1771653543307087630, 0.000000000000000000 ) ) ;
#10008=CARTESIAN_POINT ( 'NONE',  ( 0.9055118110236227702, -0.6692913385826771977, 8.415575281601705876E-17 ) ) ;
#10009=CARTESIAN_POINT ( 'NONE',  ( 0.4133858267716541968, 0.1012011053420777407, 0.2882089793578256898 ) ) ;
#10010=CARTESIAN_POINT ( 'NONE',  ( 0.8530183727034126306, 0.05413385826771626580, -0.4176697321401330321 ) ) ;
#10012=CARTESIAN_POINT ( 'NONE',  ( 1.397637795275591177, 0.07958543189024071263, -0.2665933059059888421 ) ) ;
#10013=CARTESIAN_POINT ( 'NONE',  ( -0.07874015748031421014, -0.1870078740157479769, 0.4822834645669291653 ) ) ;
#10014=CARTESIAN_POINT ( 'NONE',  ( -0.6627296587926501115, 0.2952755905511810774, -0.1292274648535930714 ) ) ;
#10015=CARTESIAN_POINT ( 'NONE',  ( 1.587926509186352586, -0.4281496062992127816, -0.4176697321401328100 ) ) ;
#10018=CARTESIAN_POINT ( 'NONE',  ( 0.5118110236220478892, 0.1771653543307087630, 0.000000000000000000 ) ) ;
#10019=ORIENTED_EDGE ( 'NONE', *, *, #19613, .F. ) ;
#10022=CARTESIAN_POINT ( 'NONE',  ( -0.3608923884514428360, -0.6692913385826773087, -0.1292274648535924053 ) ) ;
#10023=CARTESIAN_POINT ( 'NONE',  ( -0.2362204724409440182, -0.1870078740157479769, 0.4822834645669291653 ) ) ;
#10024=CARTESIAN_POINT ( 'NONE',  ( -0.1312335958005241554, -0.6046776061558809534, -0.2411417322834644161 ) ) ;
#10026=CARTESIAN_POINT ( 'NONE',  ( 0.7414698162729663755, 0.2952755905511811885, 0.1292274648535926551 ) ) ;
#10027=CARTESIAN_POINT ( 'NONE',  ( -1.082677165354329896, -0.5400638737290845981, -0.3530559997133363437 ) ) ;
#10028=CARTESIAN_POINT ( 'NONE',  ( -0.3805774278215216522, -0.4281496062992127816, -0.4176697321401328100 ) ) ;
#10029=CARTESIAN_POINT ( 'NONE',  ( 1.213910761154856299, -0.6692913385826773087, -0.1292274648535924053 ) ) ;
#10030=CARTESIAN_POINT ( 'NONE',  ( 1.108923884514436242, -0.05778040916215522460, 0.4822834645669289988 ) ) ;
#10032=CARTESIAN_POINT ( 'NONE',  ( 0.6692913385826778638, -0.6692913385826771977, 8.415575281601705876E-17 ) ) ;
#10034=CARTESIAN_POINT ( 'NONE',  ( 0.04593175853018440641, -0.5511811023622046335, 0.09757992244046803654 ) ) ;
#10038=CARTESIAN_POINT ( 'NONE',  ( -0.9186351706036736120, 0.1283753931104748280, 0.1820866141732283561 ) ) ;
#10039=CARTESIAN_POINT ( 'NONE',  ( -0.4790026246719152336, -0.05778040916215560624, -0.4822834645669293319 ) ) ;
#10041=CARTESIAN_POINT ( 'NONE',  ( -0.7545931758530177724, 0.2952755905511811885, 0.1292274648535926551 ) ) ;
#10042=CARTESIAN_POINT ( 'NONE',  ( -0.4986876640419942164, -0.6046776061558807314, 0.2411417322834647770 ) ) ;
#10043=CARTESIAN_POINT ( 'NONE',  ( -1.135170603674539924, 0.2952755905511810774, -0.1292274648535930714 ) ) ;
#10044=CARTESIAN_POINT ( 'NONE',  ( -1.502624671916009680, -0.05778040916215560624, -0.4822834645669293319 ) ) ;
#10046=CARTESIAN_POINT ( 'NONE',  ( 0.8464566929133866546, -0.4536011799217367080, 0.2665933059059888421 ) ) ;
#10049=CARTESIAN_POINT ( 'NONE',  ( 0.6430446194225728496, -0.004921259842519576551, 0.3153832671262227771 ) ) ;
#10050=CARTESIAN_POINT ( 'NONE',  ( -0.1377952755905504645, -0.5400638737290845981, -0.3530559997133363437 ) ) ;
#10051=CARTESIAN_POINT ( 'NONE',  ( -0.1902887139107604098, 0.2952755905511810774, -0.1292274648535930714 ) ) ;
#10054=CARTESIAN_POINT ( 'NONE',  ( -1.595398199321656829, 1.013096522517430875, 0.1559797534342477754 ) ) ;
#10057=CARTESIAN_POINT ( 'NONE',  ( 1.515748031496063186, -0.5400638737290845981, -0.3530559997133363437 ) ) ;
#10058=CARTESIAN_POINT ( 'NONE',  ( -0.7874015748031489847, -0.1870078740157479769, 0.3641732283464567677 ) ) ;
#10059=CARTESIAN_POINT ( 'NONE',  ( -0.8858267716535425107, 0.1660481256975883668, -0.3530559997133364547 ) ) ;
#10062=CARTESIAN_POINT ( 'NONE',  ( -1.489501312335957062, -0.08942795157527998196, 0.3641732283464567121 ) ) ;
#10063=CARTESIAN_POINT ( 'NONE',  ( 0.5511811023622054106, -0.1870078740157480879, -0.4822834645669291653 ) ) ;
#10064=CARTESIAN_POINT ( 'NONE',  ( 0.5905511811023629321, 0.2952755905511811885, 0.000000000000000000 ) ) ;
#10065=CARTESIAN_POINT ( 'NONE',  ( -0.6824146981627288167, 0.1283753931104748280, 0.1820866141732283561 ) ) ;
#10066=CARTESIAN_POINT ( 'NONE',  ( 0.1771653543307093182, 0.1660481256975885056, 0.3530559997133364547 ) ) ;
#10068=CARTESIAN_POINT ( 'NONE',  ( -0.5446194225721777693, -0.08942795157527998196, 0.3641732283464567121 ) ) ;
#10069=CARTESIAN_POINT ( 'NONE',  ( -0.4330708661417315697, 0.2952755905511811885, 0.000000000000000000 ) ) ;
#10071=CARTESIAN_POINT ( 'NONE',  ( 1.279527559055118724, 0.07958543189024085140, 0.2665933059059887866 ) ) ;
#10072=CARTESIAN_POINT ( 'NONE',  ( 0.04593175853018440641, 0.1771653543307087075, -0.09757992244046823083 ) ) ;
#10073=CARTESIAN_POINT ( 'NONE',  ( 0.9711286089238851948, -0.5023911411419708095, -0.1820866141732282451 ) ) ;
#10074=CARTESIAN_POINT ( 'NONE',  ( -1.325459317585300889, -0.4281496062992127816, -0.4176697321401328100 ) ) ;
#10075=CARTESIAN_POINT ( 'NONE',  ( -0.8727034120734901146, -0.2845877964562159024, 0.3641732283464567677 ) ) ;
#10077=CARTESIAN_POINT ( 'NONE',  ( -1.017060367454067249, -0.3162353388693409650, -0.4822834645669289433 ) ) ;
#10078=CARTESIAN_POINT ( 'NONE',  ( -0.5839895013123351797, -0.6692913385826771977, 0.1292274648535927661 ) ) ;
#10080=CARTESIAN_POINT ( 'NONE',  ( 0.2165354330708668673, -0.5400638737290844871, 0.3530559997133364547 ) ) ;
#10083=CARTESIAN_POINT ( 'NONE',  ( 0.4986876640419954376, -0.5023911411419708095, -0.1820866141732282451 ) ) ;
#10084=CARTESIAN_POINT ( 'NONE',  ( 0.9776902887139113929, 0.2952755905511811885, 0.1292274648535926551 ) ) ;
#10085=CARTESIAN_POINT ( 'NONE',  ( -1.102362204724408601, -0.1870078740157479769, 0.3641732283464567677 ) ) ;
#10086=CARTESIAN_POINT ( 'NONE',  ( 1.089238845144357759, 0.05413385826771626580, -0.4176697321401330321 ) ) ;
#10087=CARTESIAN_POINT ( 'NONE',  ( -1.627296587926508442, -0.5023911411419708095, -0.1820866141732282451 ) ) ;
#10088=CARTESIAN_POINT ( 'NONE',  ( 1.587926509186352142, -0.004921259842519576551, 0.3153832671262227771 ) ) ;
#10089=CARTESIAN_POINT ( 'NONE',  ( -0.7677165354330699465, 0.1660481256975885056, 0.3530559997133364547 ) ) ;
#10090=CARTESIAN_POINT ( 'NONE',  ( 0.3018372703412079971, -0.004921259842519870586, -0.3153832671262229437 ) ) ;
#10091=CARTESIAN_POINT ( 'NONE',  ( 1.607037972344098176, 0.2931805072228713116, 0.04654416842230573587 ) ) ;
#10092=CARTESIAN_POINT ( 'NONE',  ( 0.5052493438320215802, 0.1771653543307087630, 0.09757992244046791164 ) ) ;
#10094=CARTESIAN_POINT ( 'NONE',  ( -0.1640419947506553400, -0.05778040916215560624, -0.4822834645669293319 ) ) ;
#10096=( BOUNDED_CURVE ( )  B_SPLINE_CURVE ( 1, ( #70301, #43374 ),
 .UNSPECIFIED., .F., .F. ) 
 B_SPLINE_CURVE_WITH_KNOTS ( ( 2, 2 ),
 ( 3.469446951953614189E-18, 0.002000000000000008715 ),
 .UNSPECIFIED. ) 
 CURVE ( )  GEOMETRIC_REPRESENTATION_ITEM ( )  RATIONAL_B_SPLINE_CURVE ( ( 0.9875488213027523443, 0.9875488213027523443 ) ) 
 REPRESENTATION_ITEM ( '' )  );
#10097=CARTESIAN_POINT ( 'NONE',  ( -1.010498687664041384, -0.4281496062992127816, -0.4176697321401328100 ) ) ;
#10099=CARTESIAN_POINT ( 'NONE',  ( 0.9776902887139113929, 0.1771653543307087630, 0.09757992244046791164 ) ) ;
#10100=CARTESIAN_POINT ( 'NONE',  ( 0.2362204724409456558, -0.1870078740157479769, 0.4822834645669291653 ) ) ;
#10101=CARTESIAN_POINT ( 'NONE',  ( -0.08530183727034056085, -0.3162353388693405765, 0.4822834645669290543 ) ) ;
#10102=CARTESIAN_POINT ( 'NONE',  ( -0.2755905511811015396, -0.5511811023622047445, 6.969142054262312111E-17 ) ) ;
#10104=CARTESIAN_POINT ( 'NONE',  ( -0.3215223097112853146, -0.08942795157528024563, -0.3641732283464568787 ) ) ;
#10105=CARTESIAN_POINT ( 'NONE',  ( 0.4658792650918641698, -0.05778040916215560624, -0.4822834645669293319 ) ) ;
#10106=EDGE_CURVE ( 'NONE', #43155, #5951, #54578, .T. ) ;
#10107=CARTESIAN_POINT ( 'NONE',  ( -1.233595800524933894, 0.1283753931104748280, 0.1820866141732283561 ) ) ;
#10110=CARTESIAN_POINT ( 'NONE',  ( -1.509186351706035767, -0.4281496062992124485, 0.4176697321401328655 ) ) ;
#10111=CARTESIAN_POINT ( 'NONE',  ( 0.2099737532808405305, 0.1539470093639521697, -0.1968503937007875793 ) ) ;
#10113=EDGE_CURVE ( 'NONE', #71072, #1230, #45695, .T. ) ;
#10114=CARTESIAN_POINT ( 'NONE',  ( -1.653543307086613234, -0.1870078740157480601, -0.3641732283464567677 ) ) ;
#10115=CARTESIAN_POINT ( 'NONE',  ( -0.3674540682414692561, -0.6046776061558809534, -0.2411417322834644161 ) ) ;
#10116=CARTESIAN_POINT ( 'NONE',  ( -1.036745406824146176, -0.4281496062992124485, 0.4176697321401328655 ) ) ;
#10119=CARTESIAN_POINT ( 'NONE',  ( 1.286089238845145033, -0.6046776061558809534, -0.2411417322834644161 ) ) ;
#10120=CARTESIAN_POINT ( 'NONE',  ( 0.6496062992125991586, -0.5400638737290845981, -0.3530559997133363437 ) ) ;
#10123=CARTESIAN_POINT ( 'NONE',  ( -1.614173228346456268, -0.6692913385826771977, 8.415575281601705876E-17 ) ) ;
#10126=CARTESIAN_POINT ( 'NONE',  ( -0.9908136482939626788, 0.1771653543307087630, 0.09757992244046791164 ) ) ;
#10128=ORIENTED_EDGE ( 'NONE', *, *, #55786, .F. ) ;
#10129=B_SPLINE_CURVE_WITH_KNOTS ( 'NONE', 3,
 ( #29259, #22534, #16232, #74720 ),
 .UNSPECIFIED., .F., .F.,
 ( 4, 4 ),
 ( 0.08225757503446740060, 0.08243036250299845547 ),
 .UNSPECIFIED. ) ;
#10130=CARTESIAN_POINT ( 'NONE',  ( 0.9448818897637802916, -0.1870078740157479769, 0.4822834645669291653 ) ) ;
#10131=CARTESIAN_POINT ( 'NONE',  ( -0.4855643044619415427, -0.4281496062992124485, 0.4176697321401328655 ) ) ;
#10132=CARTESIAN_POINT ( 'NONE',  ( -1.253280839895012377, -0.3162353388693409650, -0.4822834645669289433 ) ) ;
#10133=CARTESIAN_POINT ( 'NONE',  ( 1.174540682414699111, -0.3162353388693405765, 0.4822834645669290543 ) ) ;
#10134=CARTESIAN_POINT ( 'NONE',  ( -1.135170603674539924, 0.1771653543307087075, -0.09757992244046823083 ) ) ;
#10135=FACE_OUTER_BOUND ( 'NONE', #66863, .T. ) ;
#10136=CARTESIAN_POINT ( 'NONE',  ( 0.3805774278215230400, -0.4281496062992124485, 0.4176697321401328655 ) ) ;
#10137=CARTESIAN_POINT ( 'NONE',  ( -0.6955380577427815458, 0.05413385826771666132, 0.4176697321401328100 ) ) ;
#10139=CARTESIAN_POINT ( 'NONE',  ( -1.043307086614172041, -0.5400638737290844871, 0.3530559997133364547 ) ) ;
#10141=CARTESIAN_POINT ( 'NONE',  ( 1.023622047244095334, -0.1870078740157479769, 0.4822834645669291653 ) ) ;
#10143=CARTESIAN_POINT ( 'NONE',  ( 1.338582677165355062, -0.1870078740157479769, 0.3641732283464567677 ) ) ;
#10146=CARTESIAN_POINT ( 'NONE',  ( -0.4855643044619415427, 0.05413385826771626580, -0.4176697321401330321 ) ) ;
#10147=EDGE_LOOP ( 'NONE', ( #41508, #10843, #43820, #62935 ) ) ;
#10148=CARTESIAN_POINT ( 'NONE',  ( 0.6036745406824153282, -0.5023911411419708095, 0.1820866141732285504 ) ) ;
#10149=CARTESIAN_POINT ( 'NONE',  ( -1.601049868766403650, -0.6046776061558807314, 0.2411417322834647770 ) ) ;
#10150=CARTESIAN_POINT ( 'NONE',  ( 1.043307086614173818, -0.5400638737290845981, -0.3530559997133363437 ) ) ;
#10151=CARTESIAN_POINT ( 'NONE',  ( 0.9448818897637802916, -0.1870078740157479769, 0.4822834645669291653 ) ) ;
#10152=CARTESIAN_POINT ( 'NONE',  ( -0.1246719160104980823, 0.2952755905511811885, 0.1292274648535926551 ) ) ;
#10154=CARTESIAN_POINT ( 'NONE',  ( -0.6561679790026240244, 0.2306618581243847221, -0.2411417322834647770 ) ) ;
#10156=CARTESIAN_POINT ( 'NONE',  ( -1.660104986876639543, -0.05778040916215560624, -0.4822834645669293319 ) ) ;
#10157=CARTESIAN_POINT ( 'NONE',  ( -0.8333333333333323711, 0.2952755905511811885, 0.1292274648535926551 ) ) ;
#10158=CARTESIAN_POINT ( 'NONE',  ( 1.345144356955381593, -0.05778040916215522460, 0.4822834645669289988 ) ) ;
#10159=CARTESIAN_POINT ( 'NONE',  ( 1.614173228346457378, -0.6692913385826771977, 8.415575281601705876E-17 ) ) ;
#10161=CARTESIAN_POINT ( 'NONE',  ( -0.7874015748031489847, -0.1870078740157479769, 0.4822834645669291653 ) ) ;
#10163=CARTESIAN_POINT ( 'NONE',  ( 0.4199475065616803948, -0.6046776061558809534, -0.2411417322834644161 ) ) ;
#10165=CARTESIAN_POINT ( 'NONE',  ( -0.4068241469816264999, -0.4281496062992124485, 0.4176697321401328655 ) ) ;
#10167=CARTESIAN_POINT ( 'NONE',  ( -1.587926509186350810, -0.004921259842519870586, -0.3153832671262229437 ) ) ;
#10168=CARTESIAN_POINT ( 'NONE',  ( 0.5314960629921267055, -0.4536011799217367080, 0.2665933059059888421 ) ) ;
#10169=CARTESIAN_POINT ( 'NONE',  ( 1.522309711286089939, -0.6046776061558809534, -0.2411417322834644161 ) ) ;
#10171=CARTESIAN_POINT ( 'NONE',  ( 0.5971128608923891301, 0.1771653543307087075, -0.09757992244046823083 ) ) ;
#10172=CARTESIAN_POINT ( 'NONE',  ( 0.7874015748031503170, -0.1870078740157479769, 0.4822834645669291653 ) ) ;
#10174=CARTESIAN_POINT ( 'NONE',  ( -0.3477690288713905509, -0.6692913385826771977, 0.1292274648535927661 ) ) ;
#10176=CARTESIAN_POINT ( 'NONE',  ( 1.332020997375328974, -0.08942795157528024563, -0.3641732283464568787 ) ) ;
#10177=CARTESIAN_POINT ( 'NONE',  ( -0.5314960629921254842, -0.5400638737290845981, -0.3530559997133363437 ) ) ;
#10179=CARTESIAN_POINT ( 'NONE',  ( 1.345144356955381593, -0.05778040916215522460, 0.4822834645669289988 ) ) ;
#10180=CARTESIAN_POINT ( 'NONE',  ( 0.04593175853018440641, 0.2952755905511810774, -0.1292274648535930714 ) ) ;
#10181=CARTESIAN_POINT ( 'NONE',  ( 0.4921259842519691285, -0.4536011799217368745, -0.2665933059059886201 ) ) ;
#10183=CARTESIAN_POINT ( 'NONE',  ( -0.01312335958005186876, -0.004921259842519870586, -0.3153832671262229437 ) ) ;
#10184=CARTESIAN_POINT ( 'NONE',  ( 0.6955380577427828781, -0.004921259842519870586, -0.3153832671262229437 ) ) ;
#10187=CARTESIAN_POINT ( 'NONE',  ( 0.7414698162729663755, 0.2952755905511811885, 0.1292274648535926551 ) ) ;
#10189=CARTESIAN_POINT ( 'NONE',  ( 1.660104986876641320, -0.08942795157527998196, 0.3641732283464567121 ) ) ;
#10191=CARTESIAN_POINT ( 'NONE',  ( 0.1181102362204730916, -0.5511811023622047445, 6.969142054262312111E-17 ) ) ;
#10192=CARTESIAN_POINT ( 'NONE',  ( 0.2821522309711292364, 0.2952755905511810774, -0.1292274648535930714 ) ) ;
#10193=CARTESIAN_POINT ( 'NONE',  ( 1.496062992125985147, -0.1870078740157479769, 0.3641732283464567677 ) ) ;
#10194=CARTESIAN_POINT ( 'NONE',  ( -1.148293963254592542, -0.5511811023622048555, -0.09757992244046775898 ) ) ;
#10195=CARTESIAN_POINT ( 'NONE',  ( -1.246719160104986512, 0.05413385826771666132, 0.4176697321401328100 ) ) ;
#10196=CARTESIAN_POINT ( 'NONE',  ( 0.3215223097112867578, -0.3162353388693409650, -0.4822834645669289433 ) ) ;
#10197=CARTESIAN_POINT ( 'NONE',  ( 1.010498687664042716, -0.4281496062992124485, 0.4176697321401328655 ) ) ;
#10199=CARTESIAN_POINT ( 'NONE',  ( 0.2952755905511816326, -0.5400638737290844871, 0.3530559997133364547 ) ) ;
#10200=CARTESIAN_POINT ( 'NONE',  ( 1.102362204724410155, -0.1870078740157480879, -0.4822834645669291653 ) ) ;
#10201=CARTESIAN_POINT ( 'NONE',  ( 1.167979002624672580, -0.4281496062992124485, 0.4176697321401328655 ) ) ;
#10202=CARTESIAN_POINT ( 'NONE',  ( -1.614173228346457378, 2.157411728916712068, -0.1372047244094477536 ) ) ;
#10203=CARTESIAN_POINT ( 'NONE',  ( 0.6036745406824154392, 0.1283753931104746893, -0.1820866141732285504 ) ) ;
#10204=CARTESIAN_POINT ( 'NONE',  ( -1.620734908136482577, 0.1771653543307087630, 0.09757992244046791164 ) ) ;
#10206=CARTESIAN_POINT ( 'NONE',  ( 0.1312335958005255154, -0.5023911411419708095, 0.1820866141732285504 ) ) ;
#10207=CARTESIAN_POINT ( 'NONE',  ( 0.1443569553805781891, 0.05413385826771626580, -0.4176697321401330321 ) ) ;
#10208=CARTESIAN_POINT ( 'NONE',  ( 0.6889763779527563470, 0.1660481256975883668, -0.3530559997133364547 ) ) ;
#10209=CARTESIAN_POINT ( 'NONE',  ( -0.2099737532808391705, 0.2306618581243848609, 0.2411417322834645549 ) ) ;
#10210=CARTESIAN_POINT ( 'NONE',  ( -0.2296587926509179312, -0.2845877964562161244, -0.3641732283464567121 ) ) ;
#10211=CARTESIAN_POINT ( 'NONE',  ( 0.9251968503937015864, -0.5400638737290844871, 0.3530559997133364547 ) ) ;
#10212=CARTESIAN_POINT ( 'NONE',  ( 1.069553805774278832, 0.1771653543307087075, -0.09757992244046823083 ) ) ;
#10214=CARTESIAN_POINT ( 'NONE',  ( 1.220472440944882164, 0.2066929133858268208, 4.479895975645240118E-15 ) ) ;
#10215=LINE ( 'NONE', #29555, #27162 ) ;
#10217=CARTESIAN_POINT ( 'NONE',  ( -1.384514435695537005, -0.6692913385826773087, -0.1292274648535924053 ) ) ;
#10219=CARTESIAN_POINT ( 'NONE',  ( -0.3149606299212590610, -0.1870078740157479769, 0.4822834645669291653 ) ) ;
#10223=CARTESIAN_POINT ( 'NONE',  ( 0.4002624671916016896, -0.08942795157527998196, 0.3641732283464567121 ) ) ;
#10225=CARTESIAN_POINT ( 'NONE',  ( 0.9186351706036751663, -0.6046776061558807314, 0.2411417322834647770 ) ) ;
#10228=CARTESIAN_POINT ( 'NONE',  ( -1.305774278215222184, -0.5511811023622048555, -0.09757992244046775898 ) ) ;
#10229=CARTESIAN_POINT ( 'NONE',  ( 1.489501312335958172, -0.3162353388693405765, 0.4822834645669290543 ) ) ;
#10230=CARTESIAN_POINT ( 'NONE',  ( 1.535433070866142335, -0.5511811023622047445, 6.969142054262312111E-17 ) ) ;
#10231=CARTESIAN_POINT ( 'NONE',  ( 0.4921259842519691285, -0.5400638737290845981, -0.3530559997133363437 ) ) ;
#10232=B_SPLINE_CURVE_WITH_KNOTS ( 'NONE', 3,
 ( #955, #28268, #65344, #20719 ),
 .UNSPECIFIED., .F., .F.,
 ( 4, 4 ),
 ( 1.999999999927407068E-07, 0.006970199999999936863 ),
 .UNSPECIFIED. ) ;
#10234=CARTESIAN_POINT ( 'NONE',  ( 0.2165354330708668673, -0.5400638737290844871, 0.3530559997133364547 ) ) ;
#10235=CARTESIAN_POINT ( 'NONE',  ( -0.9908136482939626788, -0.5511811023622048555, -0.09757992244046775898 ) ) ;
#10236=CARTESIAN_POINT ( 'NONE',  ( 0.3083989501312343062, -0.3162353388693405765, 0.4822834645669290543 ) ) ;
#10237=CARTESIAN_POINT ( 'NONE',  ( 0.01968503937007930540, 0.1660481256975885056, 0.3530559997133364547 ) ) ;
#10240=CARTESIAN_POINT ( 'NONE',  ( 0.8923884514435703741, 0.2306618581243848609, 0.2411417322834645549 ) ) ;
#10241=CARTESIAN_POINT ( 'NONE',  ( -0.5577427821522301654, -0.05778040916215560624, -0.4822834645669293319 ) ) ;
#10242=CARTESIAN_POINT ( 'NONE',  ( -1.089238845144356427, -0.4281496062992127816, -0.4176697321401328100 ) ) ;
#10243=CARTESIAN_POINT ( 'NONE',  ( 1.148293963254593653, 0.2952755905511810774, -0.1292274648535930714 ) ) ;
#10244=CARTESIAN_POINT ( 'NONE',  ( 0.5446194225721792126, -0.3162353388693405765, 0.4822834645669290543 ) ) ;
#10246=CARTESIAN_POINT ( 'NONE',  ( -0.3412073490813641308, -0.6046776061558807314, 0.2411417322834647770 ) ) ;
#10247=CARTESIAN_POINT ( 'NONE',  ( 0.3805774278215230400, -0.4281496062992124485, 0.4176697321401328655 ) ) ;
#10248=CARTESIAN_POINT ( 'NONE',  ( -0.5380577427821514602, 0.05413385826771666132, 0.4176697321401328100 ) ) ;
#10249=CARTESIAN_POINT ( 'NONE',  ( 0.8923884514435703741, 0.1283753931104748280, 0.1820866141732283561 ) ) ;
#10250=CARTESIAN_POINT ( 'NONE',  ( 1.646981627296588035, -0.2845877964562159024, 0.3641732283464567677 ) ) ;
#10251=CARTESIAN_POINT ( 'NONE',  ( -1.660104986876639543, -0.05778040916215560624, -0.4822834645669293319 ) ) ;
#10252=CARTESIAN_POINT ( 'NONE',  ( 0.4133858267716541968, -0.5400638737290845981, -0.3530559997133363437 ) ) ;
#10253=SURFACE_SIDE_STYLE ('',( #42221 ) ) ;
#10255=ORIENTED_EDGE ( 'NONE', *, *, #3392, .T. ) ;
#10258=CARTESIAN_POINT ( 'NONE',  ( 0.7480314960629927956, 0.2952755905511811885, 0.000000000000000000 ) ) ;
#10259=CARTESIAN_POINT ( 'NONE',  ( 0.5052493438320215802, 0.1771653543307087630, 0.09757992244046791164 ) ) ;
#10268=CARTESIAN_POINT ( 'NONE',  ( 0.9120734908136489683, -0.6692913385826771977, 0.1292274648535927661 ) ) ;
#10269=CARTESIAN_POINT ( 'NONE',  ( -0.8005249343832011588, 0.05413385826771626580, -0.4176697321401330321 ) ) ;
#10270=CARTESIAN_POINT ( 'NONE',  ( -0.5643044619422565855, 0.05413385826771626580, -0.4176697321401330321 ) ) ;
#10271=CARTESIAN_POINT ( 'NONE',  ( 0.4986876640419954376, 0.2306618581243848609, 0.2411417322834645549 ) ) ;
#10272=CARTESIAN_POINT ( 'NONE',  ( 1.456692913385827515, 0.2952755905511811885, 0.000000000000000000 ) ) ;
#10275=CARTESIAN_POINT ( 'NONE',  ( 1.240157480314961314, 0.07958543189024071263, -0.2665933059059888421 ) ) ;
#10277=CARTESIAN_POINT ( 'NONE',  ( -1.233595800524933894, -0.5023911411419708095, -0.1820866141732282451 ) ) ;
#10279=CARTESIAN_POINT ( 'NONE',  ( 0.1902887139107617975, -0.6692913385826773087, -0.1292274648535924053 ) ) ;
#10281=CARTESIAN_POINT ( 'NONE',  ( 1.213910761154856299, 0.2952755905511811885, 0.1292274648535926551 ) ) ;
#10283=CARTESIAN_POINT ( 'NONE',  ( -1.108923884514435132, -0.2845877964562159024, 0.3641732283464567677 ) ) ;
#10284=CARTESIAN_POINT ( 'NONE',  ( 0.3346456692913393205, -0.5400638737290845981, -0.3530559997133363437 ) ) ;
#10285=CARTESIAN_POINT ( 'NONE',  ( 1.102362204724410155, -0.1870078740157479769, 0.3641732283464567677 ) ) ;
#10287=CARTESIAN_POINT ( 'NONE',  ( -1.102362204724408601, -0.1870078740157479769, 0.3641732283464567677 ) ) ;
#10288=CARTESIAN_POINT ( 'NONE',  ( 1.528871391076116026, 0.2952755905511811885, 0.1292274648535926551 ) ) ;
#10290=CARTESIAN_POINT ( 'NONE',  ( -0.1968503937007867743, -0.5511811023622047445, 6.969142054262312111E-17 ) ) ;
#10291=CARTESIAN_POINT ( 'NONE',  ( 0.01312335958005323398, 0.05413385826771666132, 0.4176697321401328100 ) ) ;
#10292=CARTESIAN_POINT ( 'NONE',  ( -1.325459317585300889, -0.004921259842519576551, 0.3153832671262227771 ) ) ;
#10293=CARTESIAN_POINT ( 'NONE',  ( -0.8464566929133852113, -0.5400638737290845981, -0.3530559997133363437 ) ) ;
#10294=CARTESIAN_POINT ( 'NONE',  ( -1.397637795275589623, -0.4536011799217368745, -0.2665933059059886201 ) ) ;
#10297=CARTESIAN_POINT ( 'NONE',  ( 1.092353285368624860, -4.408777212815537393E-16, -0.4445507791589063395 ) ) ;
#10298=CARTESIAN_POINT ( 'NONE',  ( 1.220472440944882386, -0.6692913385826771977, 8.415575281601705876E-17 ) ) ;
#10300=CARTESIAN_POINT ( 'NONE',  ( -1.338582677165353729, -0.1870078740157480879, -0.4822834645669291653 ) ) ;
#10301=CARTESIAN_POINT ( 'NONE',  ( -1.246719160104985846, -0.3690944881889765550, -0.3153832671262227771 ) ) ;
#10302=CARTESIAN_POINT ( 'NONE',  ( -0.6167979002624665030, -0.004921259842519576551, 0.3153832671262227771 ) ) ;
#10304=CARTESIAN_POINT ( 'NONE',  ( 0.1312335958005257930, 0.2306618581243847221, -0.2411417322834647770 ) ) ;
#10305=CARTESIAN_POINT ( 'NONE',  ( 0.2099737532808405305, -0.5023911411419708095, 0.1820866141732285504 ) ) ;
#10306=CARTESIAN_POINT ( 'NONE',  ( -1.010498687664041384, -0.3690944881889765550, -0.3153832671262227771 ) ) ;
#10307=CARTESIAN_POINT ( 'NONE',  ( -1.482939632545930975, -0.4281496062992127816, -0.4176697321401328100 ) ) ;
#10308=CARTESIAN_POINT ( 'NONE',  ( 1.194225721784777594, -0.3690944881889765550, -0.3153832671262227771 ) ) ;
#10310=CARTESIAN_POINT ( 'NONE',  ( 1.509186351706037543, 0.05413385826771666132, 0.4176697321401328100 ) ) ;
#10312=CARTESIAN_POINT ( 'NONE',  ( 0.6430446194225729606, -0.3690944881889765550, -0.3153832671262227771 ) ) ;
#10313=CARTESIAN_POINT ( 'NONE',  ( 1.095800524934383846, -0.05778040916215560624, -0.4822834645669293319 ) ) ;
#10315=CARTESIAN_POINT ( 'NONE',  ( 0.9908136482939640111, 0.1771653543307087075, -0.09757992244046823083 ) ) ;
#10317=CARTESIAN_POINT ( 'NONE',  ( -1.292650918635170010, 0.2952755905511810774, -0.1292274648535930714 ) ) ;
#10318=CARTESIAN_POINT ( 'NONE',  ( -0.6955380577427815458, 0.05413385826771666132, 0.4176697321401328100 ) ) ;
#10319=CARTESIAN_POINT ( 'NONE',  ( -0.1115485564304456306, 0.2952755905511810774, -0.1292274648535930714 ) ) ;
#10323=CARTESIAN_POINT ( 'NONE',  ( 0.9973753280839902091, 0.2306618581243847221, -0.2411417322834647770 ) ) ;
#10324=CARTESIAN_POINT ( 'NONE',  ( 1.423884514435696191, -0.08942795157527998196, 0.3641732283464567121 ) ) ;
#10327=CARTESIAN_POINT ( 'NONE',  ( -0.02624671916010428221, 0.2306618581243847221, -0.2411417322834647770 ) ) ;
#10328=CARTESIAN_POINT ( 'NONE',  ( 0.8070866141732288002, 0.1660481256975885056, 0.3530559997133364547 ) ) ;
#10334=CARTESIAN_POINT ( 'NONE',  ( -0.2624671916010490880, 0.1283753931104746893, -0.1820866141732285504 ) ) ;
#10335=CARTESIAN_POINT ( 'NONE',  ( -0.6036745406824141069, 0.2306618581243848609, 0.2411417322834645549 ) ) ;
#10336=CARTESIAN_POINT ( 'NONE',  ( 0.6692913385826777528, 0.2952755905511811885, 0.000000000000000000 ) ) ;
#10338=CARTESIAN_POINT ( 'NONE',  ( -0.4527559055118102749, -0.4536011799217368745, -0.2665933059059886201 ) ) ;
#10339=( BOUNDED_CURVE ( )  B_SPLINE_CURVE ( 2, ( #42205, #3090, #74215, #67900, #61150, #3502, #29987, #49344, #67070, #67480, #35906, #73382, #54837 ),
 .UNSPECIFIED., .F., .F. ) 
 B_SPLINE_CURVE_WITH_KNOTS ( ( 3, 2, 2, 2, 2, 2, 3 ),
 ( 0.3096947309984372509, 0.3106060606060606077, 0.3143939393939393923, 0.3181818181818181768, 0.3219696969696969613, 0.3257575757575757458, 0.3266689053651991581 ),
 .UNSPECIFIED. ) 
 CURVE ( )  GEOMETRIC_REPRESENTATION_ITEM ( )  RATIONAL_B_SPLINE_CURVE ( ( 0.9875488213027530104, 0.9918020599134685922, 1.000000000000000000, 0.9659258262890683122, 1.000000000000000000, 0.9659258262890683122, 1.000000000000000000, 0.9659258262890683122, 1.000000000000000000, 0.9659258262890683122, 1.000000000000000000, 0.9918020599134680371, 0.9875488213027523443 ) ) 
 REPRESENTATION_ITEM ( '' )  );
#10340=CARTESIAN_POINT ( 'NONE',  ( 1.607611548556431069, 0.2952755905511811885, 0.1292274648535926551 ) ) ;
#10341=CARTESIAN_POINT ( 'NONE',  ( 1.069553805774278610, -0.6692913385826771977, 0.1292274648535927661 ) ) ;
#10345=ORIENTED_EDGE ( 'NONE', *, *, #23671, .T. ) ;
#10346=CARTESIAN_POINT ( 'NONE',  ( 1.089238845144357537, -0.4281496062992124485, 0.4176697321401328655 ) ) ;
#10347=CARTESIAN_POINT ( 'NONE',  ( 1.128608923884514947, 0.1283753931104748280, 0.1820866141732283561 ) ) ;
#10348=CARTESIAN_POINT ( 'NONE',  ( -1.561679790026246017, -0.3690944881889765550, -0.3153832671262227771 ) ) ;
#10349=CARTESIAN_POINT ( 'NONE',  ( -1.515748031496062076, -0.5400638737290844871, 0.3530559997133364547 ) ) ;
#10352=CARTESIAN_POINT ( 'NONE',  ( 0.6364829396325465405, -0.3162353388693409650, -0.4822834645669289433 ) ) ;
#10353=CARTESIAN_POINT ( 'NONE',  ( -1.476377952755905110, -0.5400638737290845981, -0.3530559997133363437 ) ) ;
#10354=CARTESIAN_POINT ( 'NONE',  ( -0.5118110236220466680, -0.6692913385826771977, 8.415575281601705876E-17 ) ) ;
#10355=CARTESIAN_POINT ( 'NONE',  ( -0.7808398950131225646, -0.05778040916215522460, 0.4822834645669289988 ) ) ;
#10356=CARTESIAN_POINT ( 'NONE',  ( -1.502624671916009680, -0.3162353388693405765, 0.4822834645669290543 ) ) ;
#10358=CARTESIAN_POINT ( 'NONE',  ( 0.2624671916010504757, -0.6046776061558809534, -0.2411417322834644161 ) ) ;
#10360=CARTESIAN_POINT ( 'NONE',  ( -1.601049868766403650, 0.1283753931104746893, -0.1820866141732285504 ) ) ;
#10363=ORIENTED_EDGE ( 'NONE', *, *, #50107, .F. ) ;
#10365=CARTESIAN_POINT ( 'NONE',  ( -1.476377952755905110, -0.5400638737290845981, -0.3530559997133363437 ) ) ;
#10367=CARTESIAN_POINT ( 'NONE',  ( 0.5611900217179910388, 1.223219560026271499E-15, 0.4445507791589056734 ) ) ;
#10368=CARTESIAN_POINT ( 'NONE',  ( -0.1377952755905504645, 0.1012011053420777407, 0.2882089793578257453 ) ) ;
#10369=CARTESIAN_POINT ( 'NONE',  ( 2.795275590551181466, 2.244094488188977277, 0.000000000000000000 ) ) ;
#10372=CARTESIAN_POINT ( 'NONE',  ( -0.4199475065616791736, -0.5023911411419708095, 0.1820866141732285504 ) ) ;
#10374=CARTESIAN_POINT ( 'NONE',  ( -1.161417322834644716, -0.4536011799217368745, -0.2665933059059886201 ) ) ;
#10375=CARTESIAN_POINT ( 'NONE',  ( -1.555118110236219930, -0.5400638737290845981, -0.3530559997133363437 ) ) ;
#10376=CARTESIAN_POINT ( 'NONE',  ( 0.3280839895013130669, 0.05413385826771666132, 0.4176697321401328100 ) ) ;
#10377=CARTESIAN_POINT ( 'NONE',  ( -1.496062992125983815, -0.1870078740157479769, 0.4822834645669291653 ) ) ;
#10379=ORIENTED_EDGE ( 'NONE', *, *, #3797, .T. ) ;
#10380=CARTESIAN_POINT ( 'NONE',  ( -1.253280839895012377, -0.3162353388693409650, -0.4822834645669289433 ) ) ;
#10386=CIRCLE ( 'NONE', #29169, 1.220472440944881942 ) ;
#10388=CARTESIAN_POINT ( 'NONE',  ( -0.7349081364829387342, -0.6046776061558807314, 0.2411417322834647770 ) ) ;
#10389=CARTESIAN_POINT ( 'NONE',  ( 1.345144356955381593, -0.05778040916215522460, 0.4822834645669289988 ) ) ;
#10391=CARTESIAN_POINT ( 'NONE',  ( -2.787279214012418738, 0.000000000000000000, 0.000000000000000000 ) ) ;
#10393=CARTESIAN_POINT ( 'NONE',  ( -1.646981627296586703, -0.3162353388693409650, -0.4822834645669289433 ) ) ;
#10394=CARTESIAN_POINT ( 'NONE',  ( -0.9580052493438311334, -0.4281496062992124485, 0.4176697321401328655 ) ) ;
#10396=CARTESIAN_POINT ( 'NONE',  ( 5.463695987328526437E-16, -0.1870078740157479769, 0.3641732283464567677 ) ) ;
#10398=CARTESIAN_POINT ( 'NONE',  ( 0.05249343832021075018, -0.5023911411419708095, 0.1820866141732285504 ) ) ;
#10399=CARTESIAN_POINT ( 'NONE',  ( 0.7414698162729663755, -0.5511811023622048555, -0.09757992244046775898 ) ) ;
#10400=CARTESIAN_POINT ( 'NONE',  ( 0.4068241469816279987, -0.4281496062992127816, -0.4176697321401328100 ) ) ;
#10401=CARTESIAN_POINT ( 'NONE',  ( -0.3083989501312330295, -0.2845877964562161244, -0.3641732283464567121 ) ) ;
#10403=CARTESIAN_POINT ( 'NONE',  ( 1.541994750656168645, -0.6692913385826771977, 0.1292274648535927661 ) ) ;
#10404=CARTESIAN_POINT ( 'NONE',  ( -0.9973753280839886548, 0.2306618581243848609, 0.2411417322834645549 ) ) ;
#10406=CARTESIAN_POINT ( 'NONE',  ( 0.07217847769028949700, -0.05778040916215560624, -0.4822834645669293319 ) ) ;
#10407=CARTESIAN_POINT ( 'NONE',  ( -0.5249343832020990641, 0.2306618581243848609, 0.2411417322834645549 ) ) ;
#10408=CARTESIAN_POINT ( 'NONE',  ( 1.627296587926509996, -0.5023911411419708095, 0.1820866141732285504 ) ) ;
#10409=CARTESIAN_POINT ( 'NONE',  ( -0.02624671916010428221, -0.5023911411419708095, 0.1820866141732285504 ) ) ;
#10410=CARTESIAN_POINT ( 'NONE',  ( -0.09186351706036689768, 0.05413385826771626580, -0.4176697321401330321 ) ) ;
#10411=CARTESIAN_POINT ( 'NONE',  ( -0.8070866141732276899, 0.1660481256975883668, -0.3530559997133364547 ) ) ;
#10412=CARTESIAN_POINT ( 'NONE',  ( 1.586052503253845281, 0.7480314960629931287, -0.1653254495020588799 ) ) ;
#10414=CARTESIAN_POINT ( 'NONE',  ( 0.2493438320209980519, 0.05413385826771666132, 0.4176697321401328100 ) ) ;
#10415=ORIENTED_EDGE ( 'NONE', *, *, #16161, .T. ) ;
#10417=CARTESIAN_POINT ( 'NONE',  ( 1.423884514435696191, -0.05778040916215522460, 0.4822834645669289988 ) ) ;
#10418=CARTESIAN_POINT ( 'NONE',  ( -0.4724409448818890911, -0.1870078740157479769, 0.3641732283464567677 ) ) ;
#10419=CARTESIAN_POINT ( 'NONE',  ( -0.7217847769028863381, 0.05413385826771626580, -0.4176697321401330321 ) ) ;
#10420=CARTESIAN_POINT ( 'NONE',  ( 1.463254593175853824, -0.6692913385826771977, 0.1292274648535927661 ) ) ;
#10421=CARTESIAN_POINT ( 'NONE',  ( 1.528871391076116026, 0.2952755905511811885, 0.1292274648535926551 ) ) ;
#10422=CARTESIAN_POINT ( 'NONE',  ( -1.581364829396324945, -0.05778040916215560624, -0.4822834645669293319 ) ) ;
#10423=CARTESIAN_POINT ( 'NONE',  ( -0.8923884514435688198, 0.1283753931104746893, -0.1820866141732285504 ) ) ;
#10427=CARTESIAN_POINT ( 'NONE',  ( 1.686351706036745890, 0.1771653543307087630, 0.09757992244046791164 ) ) ;
#10429=CARTESIAN_POINT ( 'NONE',  ( 1.207349081364829990, -0.5023911411419708095, -0.1820866141732282451 ) ) ;
#10430=CARTESIAN_POINT ( 'NONE',  ( 0.8398950131233602345, 0.2306618581243847221, -0.2411417322834647770 ) ) ;
#10431=CARTESIAN_POINT ( 'NONE',  ( -1.653543307086613234, -0.1870078740157480879, -0.4822834645669291653 ) ) ;
#10432=CARTESIAN_POINT ( 'NONE',  ( 0.9383202099737536495, -0.3162353388693405765, 0.4822834645669290543 ) ) ;
#10434=CARTESIAN_POINT ( 'NONE',  ( 1.364829396325460076, 0.1283753931104748280, 0.1820866141732283561 ) ) ;
#10435=CARTESIAN_POINT ( 'NONE',  ( 0.1377952755905518800, 0.1660481256975883668, -0.3530559997133364547 ) ) ;
#10436=CARTESIAN_POINT ( 'NONE',  ( -1.023622047244093558, -0.1870078740157479769, 0.4822834645669291653 ) ) ;
#10437=CARTESIAN_POINT ( 'NONE',  ( 1.338582677165355062, -0.1870078740157479769, 0.4822834645669291653 ) ) ;
#10441=CARTESIAN_POINT ( 'NONE',  ( 0.5249343832021003964, 0.1283753931104746893, -0.1820866141732285504 ) ) ;
#10442=EDGE_LOOP ( 'NONE', ( #23462, #62611, #68519, #46459 ) ) ;
#10445=CARTESIAN_POINT ( 'NONE',  ( -0.8792650918635160906, 0.05413385826771626580, -0.4176697321401330321 ) ) ;
#10446=CARTESIAN_POINT ( 'NONE',  ( -0.1377952755905504645, -0.5400638737290845981, -0.3530559997133363437 ) ) ;
#10447=CARTESIAN_POINT ( 'NONE',  ( -0.1509186351706028884, -0.3162353388693409650, -0.4822834645669289433 ) ) ;
#10448=CARTESIAN_POINT ( 'NONE',  ( 0.8464566929133866546, -0.5400638737290844871, 0.3530559997133364547 ) ) ;
#10449=CARTESIAN_POINT ( 'NONE',  ( -1.187664041994749731, -0.3162353388693405765, 0.4822834645669290543 ) ) ;
#10450=CARTESIAN_POINT ( 'NONE',  ( -0.5577427821522301654, -0.05778040916215560624, -0.4822834645669293319 ) ) ;
#10451=CARTESIAN_POINT ( 'NONE',  ( 0.5971128608923890191, -0.6692913385826771977, 0.1292274648535927661 ) ) ;
#10453=CARTESIAN_POINT ( 'NONE',  ( 0.6889763779527563470, 0.1660481256975883668, -0.3530559997133364547 ) ) ;
#10454=CARTESIAN_POINT ( 'NONE',  ( 0.9120734908136490793, 0.2952755905511810774, -0.1292274648535930714 ) ) ;
#10455=EDGE_CURVE ( 'NONE', #4549, #3211, #20935, .T. ) ;
#10457=CARTESIAN_POINT ( 'NONE',  ( -0.6102362204724400829, -0.4536011799217368745, -0.2665933059059886201 ) ) ;
#10461=CARTESIAN_POINT ( 'NONE',  ( -0.9580052493438311334, -0.3690944881889763329, 0.3153832671262228327 ) ) ;
#10462=CARTESIAN_POINT ( 'NONE',  ( -0.3543307086614165824, 0.2952755905511811885, 0.000000000000000000 ) ) ;
#10464=CARTESIAN_POINT ( 'NONE',  ( -0.7808398950131225646, -0.05778040916215522460, 0.4822834645669289988 ) ) ;
#10465=CARTESIAN_POINT ( 'NONE',  ( -0.8136482939632537770, -0.6046776061558807314, 0.2411417322834647770 ) ) ;
#10466=CARTESIAN_POINT ( 'NONE',  ( -1.384514435695537005, -0.6692913385826773087, -0.1292274648535924053 ) ) ;
#10467=CARTESIAN_POINT ( 'NONE',  ( -1.496062992125983815, -0.1870078740157480879, -0.4822834645669291653 ) ) ;
#10468=CARTESIAN_POINT ( 'NONE',  ( 0.9514435695538062676, -0.2845877964562161244, -0.3641732283464567121 ) ) ;
#10469=CARTESIAN_POINT ( 'NONE',  ( 1.193521905106662784, 3.421639014772782816E-16, 0.3464511005275203726 ) ) ;
#10470=CARTESIAN_POINT ( 'NONE',  ( 0.3273801728231982566, 0.000000000000000000, 0.3464511005275205946 ) ) ;
#10471=CARTESIAN_POINT ( 'NONE',  ( 0.1837270341207354329, 0.1283753931104748280, 0.1820866141732283561 ) ) ;
#10472=CARTESIAN_POINT ( 'NONE',  ( 0.1509186351706045259, -0.05778040916215560624, -0.4822834645669293319 ) ) ;
#10473=CARTESIAN_POINT ( 'NONE',  ( -0.2559055118110227234, -0.5400638737290844871, 0.3530559997133364547 ) ) ;
#10479=CARTESIAN_POINT ( 'NONE',  ( 1.541994750656168645, -0.6692913385826771977, 0.1292274648535927661 ) ) ;
#10480=CARTESIAN_POINT ( 'NONE',  ( -0.7086614173228339419, -0.1870078740157480601, -0.3641732283464567677 ) ) ;
#10481=CARTESIAN_POINT ( 'NONE',  ( -1.108923884514435132, -0.3162353388693405765, 0.4822834645669290543 ) ) ;
#10485=CARTESIAN_POINT ( 'NONE',  ( 1.240157480314961314, 0.1660481256975883668, -0.3530559997133364547 ) ) ;
#10486=CARTESIAN_POINT ( 'NONE',  ( 0.5774278215223103139, -0.6046776061558809534, -0.2411417322834644161 ) ) ;
#10487=CARTESIAN_POINT ( 'NONE',  ( 0.5577427821522316087, -0.05778040916215522460, 0.4822834645669289988 ) ) ;
#10488=CARTESIAN_POINT ( 'NONE',  ( -0.7086614173228339419, -0.1870078740157479769, 0.3641732283464567677 ) ) ;
#10489=CARTESIAN_POINT ( 'NONE',  ( -0.09842519685039295696, 0.1660481256975883668, -0.3530559997133364547 ) ) ;
#10491=CARTESIAN_POINT ( 'NONE',  ( -0.4199475065616791736, 0.2306618581243847221, -0.2411417322834647770 ) ) ;
#10493=CARTESIAN_POINT ( 'NONE',  ( 1.384514435695538337, -0.5511811023622046335, 0.09757992244046803654 ) ) ;
#10494=CARTESIAN_POINT ( 'NONE',  ( -0.4002624671916004129, -0.08942795157528024563, -0.3641732283464568787 ) ) ;
#10495=CARTESIAN_POINT ( 'NONE',  ( 0.9645669291338591078, -0.4536011799217368745, -0.2665933059059886201 ) ) ;
#10496=CARTESIAN_POINT ( 'NONE',  ( -1.286089238845143479, -0.6046776061558807314, 0.2411417322834647770 ) ) ;
#10497=CARTESIAN_POINT ( 'NONE',  ( -1.148293963254592542, 0.1771653543307087630, 0.09757992244046791164 ) ) ;
#10499=CARTESIAN_POINT ( 'NONE',  ( -1.141732283464566011, -0.6692913385826771977, 8.415575281601705876E-17 ) ) ;
#10500=CARTESIAN_POINT ( 'NONE',  ( -0.6364829396325453192, -0.05778040916215560624, -0.4822834645669293319 ) ) ;
#10501=CARTESIAN_POINT ( 'NONE',  ( 0.4330708661417329575, 0.2952755905511811885, 0.000000000000000000 ) ) ;
#10503=CARTESIAN_POINT ( 'NONE',  ( 1.092023077763014882, -8.904001037647063530E-16, -0.4281989832122458095 ) ) ;
#10504=CARTESIAN_POINT ( 'NONE',  ( 0.5380577427821529035, -0.3690944881889763329, 0.3153832671262228327 ) ) ;
#10505=CARTESIAN_POINT ( 'NONE',  ( -1.463254593175852492, -0.5511811023622048555, -0.09757992244046775898 ) ) ;
#10506=CARTESIAN_POINT ( 'NONE',  ( 0.7611548556430454138, 0.2306618581243847221, -0.2411417322834647770 ) ) ;
#10507=CARTESIAN_POINT ( 'NONE',  ( -1.509186351706035767, -0.004921259842519870586, -0.3153832671262229437 ) ) ;
#10508=CARTESIAN_POINT ( 'NONE',  ( 1.253280839895013710, -0.2845877964562159024, 0.3641732283464567677 ) ) ;
#10509=CARTESIAN_POINT ( 'NONE',  ( -0.8136482939632537770, -0.6046776061558807314, 0.2411417322834647770 ) ) ;
#10510=CARTESIAN_POINT ( 'NONE',  ( -0.4593175853018364174, -0.3690944881889765550, -0.3153832671262227771 ) ) ;
#10512=CARTESIAN_POINT ( 'NONE',  ( 0.6889763779527563470, 0.07958543189024071263, -0.2665933059059888421 ) ) ;
#10514=CARTESIAN_POINT ( 'NONE',  ( -0.2493438320209966919, -0.4281496062992124485, 0.4176697321401328655 ) ) ;
#10517=CARTESIAN_POINT ( 'NONE',  ( 0.5249343832021003964, 0.1283753931104746893, -0.1820866141732285504 ) ) ;
#10518=CARTESIAN_POINT ( 'NONE',  ( 0.2296587926509192634, -0.3162353388693405765, 0.4822834645669290543 ) ) ;
#10519=CARTESIAN_POINT ( 'NONE',  ( -0.1443569553805765515, -0.4281496062992127816, -0.4176697321401328100 ) ) ;
#10520=CARTESIAN_POINT ( 'NONE',  ( -0.5577427821522301654, -0.2845877964562159024, 0.3641732283464567677 ) ) ;
#10522=CARTESIAN_POINT ( 'NONE',  ( -0.4724409448818890911, -0.1870078740157480601, -0.3641732283464567677 ) ) ;
#10523=CARTESIAN_POINT ( 'NONE',  ( 0.5380577427821529035, -0.4281496062992124485, 0.4176697321401328655 ) ) ;
#10524=CARTESIAN_POINT ( 'NONE',  ( -0.9580052493438311334, -0.3690944881889763329, 0.3153832671262228327 ) ) ;
#10526=CARTESIAN_POINT ( 'NONE',  ( -1.364829396325458521, -0.6046776061558807314, 0.2411417322834647770 ) ) ;
#10529=CARTESIAN_POINT ( 'NONE',  ( -1.496062992125983815, -0.1870078740157480601, -0.3641732283464567677 ) ) ;
#10530=CARTESIAN_POINT ( 'NONE',  ( -0.5971128608923877978, 0.2952755905511811885, 0.1292274648535926551 ) ) ;
#10531=CARTESIAN_POINT ( 'NONE',  ( -1.135170603674539924, 0.2952755905511810774, -0.1292274648535930714 ) ) ;
#10534=CARTESIAN_POINT ( 'NONE',  ( 1.568241469816273659, -0.05778040916215560624, -0.4822834645669293319 ) ) ;
#10535=CARTESIAN_POINT ( 'NONE',  ( 0.2493438320209980519, 0.05413385826771666132, 0.4176697321401328100 ) ) ;
#10538=CARTESIAN_POINT ( 'NONE',  ( 1.496062992125984703, -0.1870078740157480601, -0.3641732283464567677 ) ) ;
#10541=CARTESIAN_POINT ( 'NONE',  ( -0.9973753280839886548, 0.1283753931104748280, 0.1820866141732283561 ) ) ;
#10544=CARTESIAN_POINT ( 'NONE',  ( 0.3477690288713918276, 0.2952755905511811885, 0.1292274648535926551 ) ) ;
#10545=CARTESIAN_POINT ( 'NONE',  ( -0.4593175853018366950, 0.05413385826771666132, 0.4176697321401328100 ) ) ;
#10546=CARTESIAN_POINT ( 'NONE',  ( -1.194225721784776262, -0.4281496062992124485, 0.4176697321401328655 ) ) ;
#10547=CARTESIAN_POINT ( 'NONE',  ( 0.9448818897637802916, -0.1870078740157480879, -0.4822834645669291653 ) ) ;
#10548=CARTESIAN_POINT ( 'NONE',  ( -1.167979002624671470, -0.004921259842519576551, 0.3153832671262227771 ) ) ;
#10549=CARTESIAN_POINT ( 'NONE',  ( 0.08943933388982898414, 7.699586553780600482E-16, 0.4118484887281971263 ) ) ;
#10550=CARTESIAN_POINT ( 'NONE',  ( 0.1443569553805781891, 0.05413385826771626580, -0.4176697321401330321 ) ) ;
#10551=CARTESIAN_POINT ( 'NONE',  ( -0.9580052493438311334, 0.05413385826771626580, -0.4176697321401330321 ) ) ;
#10556=CARTESIAN_POINT ( 'NONE',  ( 0.8070866141732289112, -0.4536011799217368745, -0.2665933059059886201 ) ) ;
#10557=VERTEX_POINT ( 'NONE', #54147 ) ;
#10559=CARTESIAN_POINT ( 'NONE',  ( -0.2952755905511803003, -0.5400638737290845981, -0.3530559997133363437 ) ) ;
#10560=VERTEX_POINT ( 'NONE', #46594 ) ;
#10561=CARTESIAN_POINT ( 'NONE',  ( 0.5774278215223103139, -0.5023911411419708095, -0.1820866141732282451 ) ) ;
#10562=CARTESIAN_POINT ( 'NONE',  ( -1.712598425196849572, 0.1660481256975885056, 0.3530559997133364547 ) ) ;
#10563=CARTESIAN_POINT ( 'NONE',  ( 0.6167979002624678353, -0.4281496062992124485, 0.4176697321401328655 ) ) ;
#10564=CARTESIAN_POINT ( 'NONE',  ( 0.2887139107611556010, -0.6046776061558807314, 0.2411417322834647770 ) ) ;
#10565=CARTESIAN_POINT ( 'NONE',  ( -0.1509186351706028884, -0.05778040916215522460, 0.4822834645669289988 ) ) ;
#10567=CARTESIAN_POINT ( 'NONE',  ( -0.9645669291338575535, 0.1660481256975883668, -0.3530559997133364547 ) ) ;
#10570=CARTESIAN_POINT ( 'NONE',  ( 1.568241469816273437, -0.2845877964562159024, 0.3641732283464567677 ) ) ;
#10571=CARTESIAN_POINT ( 'NONE',  ( -0.8858267716535425107, -0.5400638737290844871, 0.3530559997133364547 ) ) ;
#10572=CARTESIAN_POINT ( 'NONE',  ( 1.509186351706037543, 0.05413385826771666132, 0.4176697321401328100 ) ) ;
#10573=CARTESIAN_POINT ( 'NONE',  ( 1.135170603674541256, -0.6692913385826773087, -0.1292274648535924053 ) ) ;
#10575=CARTESIAN_POINT ( 'NONE',  ( -0.9251968503937002541, 0.1660481256975885056, 0.3530559997133364547 ) ) ;
#10577=CARTESIAN_POINT ( 'NONE',  ( 0.08530183727034192087, -0.3162353388693409650, -0.4822834645669289433 ) ) ;
#10579=CARTESIAN_POINT ( 'NONE',  ( -0.6692913385826764205, 0.2952755905511811885, 0.000000000000000000 ) ) ;
#10580=CARTESIAN_POINT ( 'NONE',  ( 1.679790026246720025, 0.2306618581243848609, 0.2411417322834645549 ) ) ;
#10581=CARTESIAN_POINT ( 'NONE',  ( 0.5577427821522316087, -0.08942795157527998196, 0.3641732283464567121 ) ) ;
#10582=CARTESIAN_POINT ( 'NONE',  ( 1.286089238845145033, 0.2306618581243848609, 0.2411417322834645549 ) ) ;
#10584=CARTESIAN_POINT ( 'NONE',  ( 0.5577427821522316087, -0.08942795157527998196, 0.3641732283464567121 ) ) ;
#10586=CARTESIAN_POINT ( 'NONE',  ( 0.6692913385826777528, 0.2952755905511811885, 0.000000000000000000 ) ) ;
#10588=CARTESIAN_POINT ( 'NONE',  ( -0.6758530183727028406, -0.6692913385826773087, -0.1292274648535924053 ) ) ;
#10590=CARTESIAN_POINT ( 'NONE',  ( 1.391076115485564868, -0.5023911411419708095, 0.1820866141732285504 ) ) ;
#10591=CARTESIAN_POINT ( 'NONE',  ( -0.7349081364829390672, 0.2306618581243847221, -0.2411417322834647770 ) ) ;
#10592=EDGE_CURVE ( 'NONE', #83014, #54436, #23653, .T. ) ;
#10593=CARTESIAN_POINT ( 'NONE',  ( 0.2165354330708668673, 0.1660481256975883668, -0.3530559997133364547 ) ) ;
#10594=CARTESIAN_POINT ( 'NONE',  ( 0.1115485564304470045, 0.2066929133858267931, 0.1054918080437490802 ) ) ;
#10595=CARTESIAN_POINT ( 'NONE',  ( 0.07874015748031558404, -0.1870078740157480879, -0.4822834645669291653 ) ) ;
#10596=CARTESIAN_POINT ( 'NONE',  ( -0.03280839895013062252, 0.1771653543307087075, -0.09757992244046823083 ) ) ;
#10598=CARTESIAN_POINT ( 'NONE',  ( 0.006561679790026889343, -0.2845877964562161244, -0.3641732283464567121 ) ) ;
#10599=CARTESIAN_POINT ( 'NONE',  ( 0.5905511811023629321, -0.5511811023622047445, 6.969142054262312111E-17 ) ) ;
#10600=LINE ( 'NONE', #37073, #16191 ) ;
#10602=CARTESIAN_POINT ( 'NONE',  ( 0.5249343832021005074, -0.6046776061558807314, 0.2411417322834647770 ) ) ;
#10604=CARTESIAN_POINT ( 'NONE',  ( 0.2251228153049674996, -4.135162568743707313E-16, -0.3954985857520057491 ) ) ;
#10605=CARTESIAN_POINT ( 'NONE',  ( 0.1474713956048451791, 8.471767977567108961E-16, -0.4445507791589058955 ) ) ;
#10606=CARTESIAN_POINT ( 'NONE',  ( -0.6036745406824141069, 0.1283753931104748280, 0.1820866141732283561 ) ) ;
#10607=CARTESIAN_POINT ( 'NONE',  ( 0.3018372703412079971, 0.05413385826771626580, -0.4176697321401330321 ) ) ;
#10608=CARTESIAN_POINT ( 'NONE',  ( 0.8333333333333340365, -0.5511811023622046335, 0.09757992244046803654 ) ) ;
#10609=CARTESIAN_POINT ( 'NONE',  ( -1.456692913385826182, -0.5511811023622047445, 6.969142054262312111E-17 ) ) ;
#10610=CARTESIAN_POINT ( 'NONE',  ( -1.614173228346456268, -0.6692913385826771977, 8.415575281601705876E-17 ) ) ;
#10611=CARTESIAN_POINT ( 'NONE',  ( 0.1312335958005257930, 0.2306618581243847221, -0.2411417322834647770 ) ) ;
#10613=CARTESIAN_POINT ( 'NONE',  ( 1.213910761154856299, 0.2952755905511811885, 0.1292274648535926551 ) ) ;
#10614=CARTESIAN_POINT ( 'NONE',  ( 0.1049868766404206816, -0.6046776061558809534, -0.2411417322834644161 ) ) ;
#10615=CARTESIAN_POINT ( 'NONE',  ( 1.135170603674541256, -0.6692913385826773087, -0.1292274648535924053 ) ) ;
#10616=CARTESIAN_POINT ( 'NONE',  ( 0.7874015748031503170, -0.1870078740157480879, -0.4822834645669291653 ) ) ;
#10618=CARTESIAN_POINT ( 'NONE',  ( 0.7086614173228353852, -0.1870078740157479769, 0.3641732283464567677 ) ) ;
#10619=CARTESIAN_POINT ( 'NONE',  ( -1.601049868766403650, 0.1283753931104746893, -0.1820866141732285504 ) ) ;
#10620=EDGE_CURVE ( 'NONE', #44077, #43739, #27688, .T. ) ;
#10621=CARTESIAN_POINT ( 'NONE',  ( 0.2887139107611556010, -0.5023911411419708095, 0.1820866141732285504 ) ) ;
#10622=CARTESIAN_POINT ( 'NONE',  ( -0.2821522309711278487, -0.6692913385826773087, -0.1292274648535924053 ) ) ;
#10623=CARTESIAN_POINT ( 'NONE',  ( 0.8530183727034126306, 0.05413385826771626580, -0.4176697321401330321 ) ) ;
#10624=CARTESIAN_POINT ( 'NONE',  ( -0.5511811023622038563, -0.1870078740157479769, 0.4822834645669291653 ) ) ;
#10626=CARTESIAN_POINT ( 'NONE',  ( -0.06561679790026180015, -0.3690944881889765550, -0.3153832671262227771 ) ) ;
#10627=CARTESIAN_POINT ( 'NONE',  ( 0.9514435695538062676, -0.05778040916215522460, 0.4822834645669289988 ) ) ;
#10628=CARTESIAN_POINT ( 'NONE',  ( 0.9055118110236227702, 0.1771653543307087630, 0.000000000000000000 ) ) ;
#10632=CARTESIAN_POINT ( 'NONE',  ( 1.607611548556431069, 0.2952755905511811885, 0.1292274648535926551 ) ) ;
#10633=CARTESIAN_POINT ( 'NONE',  ( -1.194225721784776262, 0.009842519685039144428, -0.3409548833797004797 ) ) ;
#10634=CARTESIAN_POINT ( 'NONE',  ( -1.391076115485563314, -0.6046776061558809534, -0.2411417322834644161 ) ) ;
#10635=CARTESIAN_POINT ( 'NONE',  ( -0.4068241469816267775, 0.05413385826771626580, -0.4176697321401330321 ) ) ;
#10638=ORIENTED_EDGE ( 'NONE', *, *, #68819, .F. ) ;
#10639=CARTESIAN_POINT ( 'NONE',  ( 0.4330708661417329575, 0.1771653543307087630, 0.000000000000000000 ) ) ;
#10641=CARTESIAN_POINT ( 'NONE',  ( 1.049868766404200127, -0.6046776061558809534, -0.2411417322834644161 ) ) ;
#10643=CARTESIAN_POINT ( 'NONE',  ( 1.614173228346456712, 0.7166040191147866611, 0.1372047244094478646 ) ) ;
#10644=CARTESIAN_POINT ( 'NONE',  ( -0.2755905511811018171, 0.2952755905511811885, 0.000000000000000000 ) ) ;
#10646=CARTESIAN_POINT ( 'NONE',  ( 1.332020997375328974, -0.08942795157528024563, -0.3641732283464568787 ) ) ;
#10647=CARTESIAN_POINT ( 'NONE',  ( 0.4133858267716541968, 0.1660481256975885056, 0.3530559997133364547 ) ) ;
#10649=CARTESIAN_POINT ( 'NONE',  ( -0.4724409448818890911, -0.1870078740157480879, -0.4822834645669291653 ) ) ;
#10650=CARTESIAN_POINT ( 'NONE',  ( -1.049868766404198794, 0.1283753931104746893, -0.1820866141732285504 ) ) ;
#10651=CARTESIAN_POINT ( 'NONE',  ( 0.4658792650918640033, -0.3162353388693405765, 0.4822834645669290543 ) ) ;
#10652=CARTESIAN_POINT ( 'NONE',  ( -0.2624671916010490880, 0.2306618581243847221, -0.2411417322834647770 ) ) ;
#10656=CARTESIAN_POINT ( 'NONE',  ( 0.7742782152230979209, 0.05413385826771626580, -0.4176697321401330321 ) ) ;
#10657=CARTESIAN_POINT ( 'NONE',  ( -0.1640419947506555343, -0.3162353388693405765, 0.4822834645669290543 ) ) ;
#10658=CARTESIAN_POINT ( 'NONE',  ( -1.568241469816272105, -0.3162353388693409650, -0.4822834645669289433 ) ) ;
#10660=CARTESIAN_POINT ( 'NONE',  ( 0.9776902887139113929, 0.2952755905511811885, 0.1292274648535926551 ) ) ;
#10661=CARTESIAN_POINT ( 'NONE',  ( 0.6692913385826778638, -0.6692913385826771977, 8.415575281601705876E-17 ) ) ;
#10663=CARTESIAN_POINT ( 'NONE',  ( -0.2887139107611542133, 0.2306618581243848609, 0.2411417322834645549 ) ) ;
#10664=CARTESIAN_POINT ( 'NONE',  ( 0.1115485564304470323, 0.2952755905511811885, 0.1292274648535926551 ) ) ;
#10665=CARTESIAN_POINT ( 'NONE',  ( -0.5643044619422565855, -0.4281496062992124485, 0.4176697321401328655 ) ) ;
#10666=CARTESIAN_POINT ( 'NONE',  ( 0.1312335958005257930, 0.1283753931104746893, -0.1820866141732285504 ) ) ;
#10667=CARTESIAN_POINT ( 'NONE',  ( -1.660104986876639543, -0.05778040916215560624, -0.4822834645669293319 ) ) ;
#10669=CARTESIAN_POINT ( 'NONE',  ( 0.5249343832021003964, 0.2306618581243847221, -0.2411417322834647770 ) ) ;
#10671=CARTESIAN_POINT ( 'NONE',  ( 1.528871391076116026, -0.6692913385826773087, -0.1292274648535924053 ) ) ;
#10675=CARTESIAN_POINT ( 'NONE',  ( 0.6561679790026253567, -0.6046776061558809534, -0.2411417322834644161 ) ) ;
#10676=CARTESIAN_POINT ( 'NONE',  ( 0.2755905511811031494, -0.5511811023622047445, 6.969142054262312111E-17 ) ) ;
#10680=PLANE ( 'NONE',  #49079 ) ;
#10684=CARTESIAN_POINT ( 'NONE',  ( 0.4330708661417329575, -0.6692913385826771977, 8.415575281601705876E-17 ) ) ;
#10685=CARTESIAN_POINT ( 'NONE',  ( -0.8792650918635160906, -0.4281496062992124485, 0.4176697321401328655 ) ) ;
#10686=CARTESIAN_POINT ( 'NONE',  ( -0.5380577427821514602, -0.4281496062992127816, -0.4176697321401328100 ) ) ;
#10687=CARTESIAN_POINT ( 'NONE',  ( 0.6299212598425204535, -0.1870078740157479769, 0.4822834645669291653 ) ) ;
#10688=CARTESIAN_POINT ( 'NONE',  ( 1.358267716535433323, -0.5400638737290845981, -0.3530559997133363437 ) ) ;
#10690=SHAPE_DEFINITION_REPRESENTATION ( #28543, #48103 ) ;
#10691=CARTESIAN_POINT ( 'NONE',  ( 1.358267716535433323, 0.07958543189024085140, 0.2665933059059887866 ) ) ;
#10692=CARTESIAN_POINT ( 'NONE',  ( -0.8267716535433065062, 0.2952755905511811885, 0.000000000000000000 ) ) ;
#10693=CARTESIAN_POINT ( 'NONE',  ( 1.443569553805774897, -0.6046776061558809534, -0.2411417322834644161 ) ) ;
#10694=LINE ( 'NONE', #73424, #14075 ) ;
#10695=CARTESIAN_POINT ( 'NONE',  ( -0.2624671916010490880, -0.6046776061558807314, 0.2411417322834647770 ) ) ;
#10696=CARTESIAN_POINT ( 'NONE',  ( 1.272965879265092637, -0.4281496062992127816, -0.4176697321401328100 ) ) ;
#10698=CARTESIAN_POINT ( 'NONE',  ( -1.148293963254592542, -0.5511811023622048555, -0.09757992244046775898 ) ) ;
#10699=CARTESIAN_POINT ( 'NONE',  ( 0.1771653543307093182, -0.5400638737290845981, -0.3530559997133363437 ) ) ;
#10700=CARTESIAN_POINT ( 'NONE',  ( 1.108923884514436242, -0.08942795157527998196, 0.3641732283464567121 ) ) ;
#10702=CARTESIAN_POINT ( 'NONE',  ( -1.089238845144356427, -0.004921259842519576551, 0.3153832671262227771 ) ) ;
#10703=CARTESIAN_POINT ( 'NONE',  ( 1.325459317585302665, -0.4281496062992124485, 0.4176697321401328655 ) ) ;
#10705=CARTESIAN_POINT ( 'NONE',  ( -0.3018372703412066094, -0.004921259842519576551, 0.3153832671262227771 ) ) ;
#10706=CARTESIAN_POINT ( 'NONE',  ( 5.463695987328526437E-16, -0.1870078740157479769, 0.4822834645669291653 ) ) ;
#10707=CARTESIAN_POINT ( 'NONE',  ( -1.345144356955379816, -0.2845877964562159024, 0.3641732283464567677 ) ) ;
#10708=CARTESIAN_POINT ( 'NONE',  ( -0.7217847769028863381, 0.05413385826771626580, -0.4176697321401330321 ) ) ;
#10709=CARTESIAN_POINT ( 'NONE',  ( 1.541994750656168645, 0.2952755905511810774, -0.1292274648535930714 ) ) ;
#10711=CARTESIAN_POINT ( 'NONE',  ( -0.9973753280839886548, 0.1283753931104748280, 0.1820866141732283561 ) ) ;
#10712=DIRECTION ( 'NONE',  ( 0.000000000000000000, 0.000000000000000000, -1.000000000000000000 ) ) ;
#10713=CARTESIAN_POINT ( 'NONE',  ( 1.574803149606299746, -0.1870078740157479769, 0.4822834645669291653 ) ) ;
#10715=CARTESIAN_POINT ( 'NONE',  ( -1.115485564304461219, -0.4281496062992124485, 0.4176697321401328655 ) ) ;
#10716=CARTESIAN_POINT ( 'NONE',  ( -1.003937007874014853, 0.07958543189024085140, 0.2665933059059887866 ) ) ;
#10717=CARTESIAN_POINT ( 'NONE',  ( -0.5839895013123351797, 0.1771653543307087075, -0.09757992244046823083 ) ) ;
#10718=CARTESIAN_POINT ( 'NONE',  ( -1.574803149606298192, -0.1870078740157480879, -0.4822834645669291653 ) ) ;
#10719=CARTESIAN_POINT ( 'NONE',  ( -0.1509186351706028884, -0.3162353388693409650, -0.4822834645669289433 ) ) ;
#10720=CARTESIAN_POINT ( 'NONE',  ( -0.1509186351706028884, -0.2845877964562161244, -0.3641732283464567121 ) ) ;
#10721=CARTESIAN_POINT ( 'NONE',  ( -0.9645669291338575535, -0.4536011799217367080, 0.2665933059059888421 ) ) ;
#10722=CARTESIAN_POINT ( 'NONE',  ( -1.430446194225721390, -0.4281496062992124485, 0.4176697321401328655 ) ) ;
#10723=CARTESIAN_POINT ( 'NONE',  ( 1.476377952755906220, 0.07958543189024071263, -0.2665933059059888421 ) ) ;
#10724=CARTESIAN_POINT ( 'NONE',  ( 0.8267716535433078384, -0.6692913385826771977, 8.415575281601705876E-17 ) ) ;
#10725=DIRECTION ( 'NONE',  ( -1.000000000000000000, -3.412570772413390973E-16, 0.000000000000000000 ) ) ;
#10726=CARTESIAN_POINT ( 'NONE',  ( 0.2624671916010504757, 0.1283753931104748280, 0.1820866141732283561 ) ) ;
#10727=CARTESIAN_POINT ( 'NONE',  ( 0.8464566929133866546, -0.5400638737290844871, 0.3530559997133364547 ) ) ;
#10728=CARTESIAN_POINT ( 'NONE',  ( 1.167979002624672580, -0.004921259842519870586, -0.3153832671262229437 ) ) ;
#10729=ORIENTED_EDGE ( 'NONE', *, *, #55755, .T. ) ;
#10730=CARTESIAN_POINT ( 'NONE',  ( -1.397637795275589623, -0.5400638737290845981, -0.3530559997133363437 ) ) ;
#10731=CARTESIAN_POINT ( 'NONE',  ( -1.069553805774277722, -0.6692913385826773087, -0.1292274648535924053 ) ) ;
#10732=CARTESIAN_POINT ( 'NONE',  ( -0.01968503937007793844, -0.5400638737290844871, 0.3530559997133364547 ) ) ;
#10735=CARTESIAN_POINT ( 'NONE',  ( 0.7217847769028878924, -0.4281496062992127816, -0.4176697321401328100 ) ) ;
#10736=CARTESIAN_POINT ( 'NONE',  ( 1.404199475065617264, -0.3690944881889763329, 0.3153832671262228327 ) ) ;
#10737=CARTESIAN_POINT ( 'NONE',  ( 0.05249343832021075018, -0.6046776061558807314, 0.2411417322834647770 ) ) ;
#10738=CARTESIAN_POINT ( 'NONE',  ( 0.8923884514435701520, -0.6046776061558809534, -0.2411417322834644161 ) ) ;
#10744=CARTESIAN_POINT ( 'NONE',  ( -0.4199475065616791736, 0.1283753931104746893, -0.1820866141732285504 ) ) ;
#10745=CARTESIAN_POINT ( 'NONE',  ( -0.8398950131233589023, -0.6046776061558809534, -0.2411417322834644161 ) ) ;
#10746=CARTESIAN_POINT ( 'NONE',  ( 0.2821522309711292364, -0.6692913385826771977, 0.1292274648535927661 ) ) ;
#10748=CARTESIAN_POINT ( 'NONE',  ( -1.469816272965878357, 0.2306618581243848609, 0.2411417322834645549 ) ) ;
#10749=CARTESIAN_POINT ( 'NONE',  ( 1.305774278215223960, 0.2952755905511810774, -0.1292274648535930714 ) ) ;
#10752=CARTESIAN_POINT ( 'NONE',  ( 1.154855643044620184, 0.2306618581243847221, -0.2411417322834647770 ) ) ;
#10753=CARTESIAN_POINT ( 'NONE',  ( 1.062992125984252745, -0.6692913385826771977, 8.415575281601705876E-17 ) ) ;
#10754=CARTESIAN_POINT ( 'NONE',  ( 1.266404199475066328, -0.08942795157527998196, 0.3641732283464567121 ) ) ;
#10755=CARTESIAN_POINT ( 'NONE',  ( -1.502624671916009680, -0.2845877964562159024, 0.3641732283464567677 ) ) ;
#10756=CARTESIAN_POINT ( 'NONE',  ( -1.391076115485563314, -0.6046776061558809534, -0.2411417322834644161 ) ) ;
#10759=CARTESIAN_POINT ( 'NONE',  ( 0.9842519685039378130, -0.6692913385826771977, 8.415575281601705876E-17 ) ) ;
#10760=CARTESIAN_POINT ( 'NONE',  ( 1.679790026246720025, 0.1283753931104748280, 0.1820866141732283561 ) ) ;
#10761=CARTESIAN_POINT ( 'NONE',  ( -0.6955380577427815458, -0.4281496062992127816, -0.4176697321401328100 ) ) ;
#10762=CARTESIAN_POINT ( 'NONE',  ( -0.4199475065616791736, 0.2306618581243847221, -0.2411417322834647770 ) ) ;
#10763=CARTESIAN_POINT ( 'NONE',  ( 1.450131233595801428, 0.2952755905511811885, 0.1292274648535926551 ) ) ;
#10765=CARTESIAN_POINT ( 'NONE',  ( 0.01312335958005323398, 0.05413385826771666132, 0.4176697321401328100 ) ) ;
#10767=CARTESIAN_POINT ( 'NONE',  ( -1.581364829396324945, -0.08942795157528024563, -0.3641732283464568787 ) ) ;
#10768=ORIENTED_EDGE ( 'NONE', *, *, #43922, .T. ) ;
#10770=ORIENTED_EDGE ( 'NONE', *, *, #45969, .F. ) ;
#10772=CARTESIAN_POINT ( 'NONE',  ( -1.450131233595799651, -0.6692913385826771977, 0.1292274648535927661 ) ) ;
#10774=CARTESIAN_POINT ( 'NONE',  ( 1.561679790026247350, -0.004921259842519870586, -0.3153832671262229437 ) ) ;
#10779=CARTESIAN_POINT ( 'NONE',  ( -0.3215223097112853146, -0.08942795157528024563, -0.3641732283464568787 ) ) ;
#10780=CARTESIAN_POINT ( 'NONE',  ( -1.259842519685038686, -0.1870078740157479769, 0.3641732283464567677 ) ) ;
#10781=CARTESIAN_POINT ( 'NONE',  ( 1.561679790026247350, -0.4281496062992124485, 0.4176697321401328655 ) ) ;
#10782=CARTESIAN_POINT ( 'NONE',  ( 0.3149606299212603933, -0.1870078740157479769, 0.4822834645669291653 ) ) ;
#10783=CARTESIAN_POINT ( 'NONE',  ( -1.364829396325458521, -0.6046776061558807314, 0.2411417322834647770 ) ) ;
#10786=CARTESIAN_POINT ( 'NONE',  ( -1.627296587926508442, 0.2306618581243848609, 0.2411417322834645549 ) ) ;
#10791=CARTESIAN_POINT ( 'NONE',  ( -0.8202099737532799750, 0.2952755905511810774, -0.1292274648535930714 ) ) ;
#10792=CARTESIAN_POINT ( 'NONE',  ( 1.397637795275591177, 0.1660481256975883668, -0.3530559997133364547 ) ) ;
#10793=CARTESIAN_POINT ( 'NONE',  ( 0.7414698162729664865, 0.2952755905511811885, 0.1292274648535926551 ) ) ;
#10794=DIRECTION ( 'NONE',  ( 0.000000000000000000, -1.000000000000000000, -0.000000000000000000 ) ) ;
#10795=CARTESIAN_POINT ( 'NONE',  ( 1.469816272965879911, -0.6046776061558807314, 0.2411417322834647770 ) ) ;
#10796=CARTESIAN_POINT ( 'NONE',  ( -0.7874015748031489847, -0.1870078740157479769, 0.4822834645669291653 ) ) ;
#10798=CARTESIAN_POINT ( 'NONE',  ( 0.03280839895013198948, 0.1771653543307087630, 0.09757992244046791164 ) ) ;
#10800=CARTESIAN_POINT ( 'NONE',  ( -0.01968503937007793844, 0.07958543189024071263, -0.2665933059059888421 ) ) ;
#10801=CARTESIAN_POINT ( 'NONE',  ( 0.5314960629921264834, 0.07958543189024071263, -0.2665933059059888421 ) ) ;
#10802=CARTESIAN_POINT ( 'NONE',  ( 0.3346456692913390985, 0.1660481256975885056, 0.3530559997133364547 ) ) ;
#10803=CARTESIAN_POINT ( 'NONE',  ( -0.5511811023622038563, -0.1870078740157479769, 0.3641732283464567677 ) ) ;
#10805=CARTESIAN_POINT ( 'NONE',  ( 1.450131233595801428, 0.2952755905511811885, 0.1292274648535926551 ) ) ;
#10806=CARTESIAN_POINT ( 'NONE',  ( -1.049868766404198794, -0.6046776061558807314, 0.2411417322834647770 ) ) ;
#10808=CARTESIAN_POINT ( 'NONE',  ( -0.05249343832020938322, -0.6046776061558809534, -0.2411417322834644161 ) ) ;
#10809=CARTESIAN_POINT ( 'NONE',  ( -0.3608923884514428360, 0.2952755905511811885, 0.1292274648535926551 ) ) ;
#10810=CARTESIAN_POINT ( 'NONE',  ( 1.062992125984252745, 0.1771653543307087630, 0.000000000000000000 ) ) ;
#10811=CARTESIAN_POINT ( 'NONE',  ( 0.2952755905511816326, -0.4536011799217367080, 0.2665933059059888421 ) ) ;
#10812=CARTESIAN_POINT ( 'NONE',  ( -0.2362204724409442680, -0.1870078740157480879, -0.4822834645669291653 ) ) ;
#10813=CARTESIAN_POINT ( 'NONE',  ( -0.8398950131233585692, 0.2306618581243848609, 0.2411417322834645549 ) ) ;
#10815=CARTESIAN_POINT ( 'NONE',  ( 1.679790026246720025, 0.1283753931104748280, 0.1820866141732283561 ) ) ;
#10816=CARTESIAN_POINT ( 'NONE',  ( 0.2362204724409456558, -0.1870078740157479769, 0.4822834645669291653 ) ) ;
#10819=( BOUNDED_CURVE ( )  B_SPLINE_CURVE ( 1, ( #59907, #2259 ),
 .UNSPECIFIED., .F., .F. ) 
 B_SPLINE_CURVE_WITH_KNOTS ( ( 2, 2 ),
 ( 0.000000000000000000, 0.002000000000000001776 ),
 .UNSPECIFIED. ) 
 CURVE ( )  GEOMETRIC_REPRESENTATION_ITEM ( )  RATIONAL_B_SPLINE_CURVE ( ( 0.9875488213027523443, 0.9875488213027523443 ) ) 
 REPRESENTATION_ITEM ( '' )  );
#10820=CARTESIAN_POINT ( 'NONE',  ( 1.351706036745407458, -0.4281496062992127816, -0.4176697321401328100 ) ) ;
#10821=CARTESIAN_POINT ( 'NONE',  ( -0.6233595800524928121, -0.08942795157527998196, 0.3641732283464567121 ) ) ;
#10822=CARTESIAN_POINT ( 'NONE',  ( -0.5249343832020990641, -0.6046776061558809534, -0.2411417322834644161 ) ) ;
#10823=CARTESIAN_POINT ( 'NONE',  ( 1.128608923884515169, -0.6046776061558809534, -0.2411417322834644161 ) ) ;
#10824=CARTESIAN_POINT ( 'NONE',  ( 0.8267716535433078384, -0.6692913385826771977, 8.415575281601705876E-17 ) ) ;
#10826=CARTESIAN_POINT ( 'NONE',  ( -1.056430446194224881, 0.1771653543307087075, -0.09757992244046823083 ) ) ;
#10830=CARTESIAN_POINT ( 'NONE',  ( 1.469816272965879911, -0.5023911411419708095, 0.1820866141732285504 ) ) ;
#10831=CARTESIAN_POINT ( 'NONE',  ( 0.7939632545931766261, -0.08942795157527998196, 0.3641732283464567121 ) ) ;
#10833=CARTESIAN_POINT ( 'NONE',  ( 0.6102362204724416372, -0.5400638737290844871, 0.3530559997133364547 ) ) ;
#10834=CARTESIAN_POINT ( 'NONE',  ( 0.4265091863517068149, 0.2066929133858267931, 0.1054918080437490802 ) ) ;
#10836=CARTESIAN_POINT ( 'NONE',  ( 0.8070866141732289112, -0.4536011799217368745, -0.2665933059059886201 ) ) ;
#10837=CARTESIAN_POINT ( 'NONE',  ( -0.1968503937007867743, 0.2952755905511811885, 0.000000000000000000 ) ) ;
#10838=CARTESIAN_POINT ( 'NONE',  ( -0.6496062992125976043, 0.1660481256975883668, -0.3530559997133364547 ) ) ;
#10839=CARTESIAN_POINT ( 'NONE',  ( 1.430446194225722500, -0.4281496062992127816, -0.4176697321401328100 ) ) ;
#10842=CARTESIAN_POINT ( 'NONE',  ( 0.03280839895013198948, 0.1771653543307087630, 0.09757992244046791164 ) ) ;
#10843=ORIENTED_EDGE ( 'NONE', *, *, #9952, .F. ) ;
#10845=VERTEX_POINT ( 'NONE', #62128 ) ;
#10846=CARTESIAN_POINT ( 'NONE',  ( -1.030183727034119867, -0.05778040916215560624, -0.4822834645669293319 ) ) ;
#10847=CARTESIAN_POINT ( 'NONE',  ( -0.07874015748031421014, -0.1870078740157479769, 0.4822834645669291653 ) ) ;
#10848=CARTESIAN_POINT ( 'NONE',  ( -0.2230971128608915943, 0.05413385826771666132, 0.4176697321401328100 ) ) ;
#10849=CARTESIAN_POINT ( 'NONE',  ( 0.4593175853018380828, 0.05413385826771626580, -0.4176697321401330321 ) ) ;
#10850=CARTESIAN_POINT ( 'NONE',  ( -0.6102362204724400829, -0.5400638737290845981, -0.3530559997133363437 ) ) ;
#10851=CARTESIAN_POINT ( 'NONE',  ( -1.141732283464566011, 0.2952755905511811885, 0.000000000000000000 ) ) ;
#10852=CARTESIAN_POINT ( 'NONE',  ( -0.9251968503937002541, 0.1660481256975885056, 0.3530559997133364547 ) ) ;
#10853=CARTESIAN_POINT ( 'NONE',  ( 0.9055118110236227702, -0.6692913385826771977, 8.415575281601705876E-17 ) ) ;
#10854=CARTESIAN_POINT ( 'NONE',  ( 0.6627296587926515548, 0.2952755905511811885, 0.1292274648535926551 ) ) ;
#10857=CARTESIAN_POINT ( 'NONE',  ( -0.5249343832020990641, 0.1283753931104748280, 0.1820866141732283561 ) ) ;
#10861=CARTESIAN_POINT ( 'NONE',  ( -1.095800524934382292, -0.08942795157527998196, 0.3641732283464567121 ) ) ;
#10862=CARTESIAN_POINT ( 'NONE',  ( -0.3608923884514428360, 0.2952755905511811885, 0.1292274648535926551 ) ) ;
#10863=CARTESIAN_POINT ( 'NONE',  ( 0.7749820319012125092, 2.784432375088962958E-17, -0.3464511005275205946 ) ) ;
#10864=CARTESIAN_POINT ( 'NONE',  ( -0.6627296587926503335, -0.6692913385826771977, 0.1292274648535927661 ) ) ;
#10865=CARTESIAN_POINT ( 'NONE',  ( -0.7349081364829390672, 0.2306618581243847221, -0.2411417322834647770 ) ) ;
#10866=CARTESIAN_POINT ( 'NONE',  ( -1.240157480314959759, -0.5400638737290845981, -0.3530559997133363437 ) ) ;
#10868=CARTESIAN_POINT ( 'NONE',  ( 0.8530183727034128527, -0.3690944881889763329, 0.3153832671262228327 ) ) ;
#10871=CARTESIAN_POINT ( 'NONE',  ( 0.006561679790026889343, -0.08942795157527998196, 0.3641732283464567121 ) ) ;
#10872=CARTESIAN_POINT ( 'NONE',  ( -0.4790026246719152336, -0.05778040916215560624, -0.4822834645669293319 ) ) ;
#10873=CARTESIAN_POINT ( 'NONE',  ( -0.2690288713910754526, -0.6692913385826771977, 0.1292274648535927661 ) ) ;
#10880=CARTESIAN_POINT ( 'NONE',  ( -0.7939632545931754048, -0.2845877964562159024, 0.3641732283464567677 ) ) ;
#10881=CARTESIAN_POINT ( 'NONE',  ( -1.095800524934382292, -0.05778040916215522460, 0.4822834645669289988 ) ) ;
#10886=CARTESIAN_POINT ( 'NONE',  ( 1.167979002624672580, -0.4281496062992124485, 0.4176697321401328655 ) ) ;
#10887=CARTESIAN_POINT ( 'NONE',  ( 0.3018372703412079971, -0.4281496062992124485, 0.4176697321401328655 ) ) ;
#10888=CARTESIAN_POINT ( 'NONE',  ( 0.6364829396325465405, -0.3162353388693409650, -0.4822834645669289433 ) ) ;
#10889=CARTESIAN_POINT ( 'NONE',  ( -0.5905511811023613777, -0.5511811023622047445, 6.969142054262312111E-17 ) ) ;
#10890=CARTESIAN_POINT ( 'NONE',  ( -0.3477690288713905509, -0.6692913385826771977, 0.1292274648535927661 ) ) ;
#10892=CARTESIAN_POINT ( 'NONE',  ( -0.8858267716535425107, 0.1660481256975883668, -0.3530559997133364547 ) ) ;
#10894=CARTESIAN_POINT ( 'NONE',  ( 1.430446194225722500, -0.004921259842519576551, 0.3153832671262227771 ) ) ;
#10895=CARTESIAN_POINT ( 'NONE',  ( -0.2362204724409442680, -0.1870078740157480601, -0.3641732283464567677 ) ) ;
#10896=CARTESIAN_POINT ( 'NONE',  ( 1.207349081364829990, 0.1283753931104748280, 0.1820866141732283561 ) ) ;
#10897=CARTESIAN_POINT ( 'NONE',  ( -1.719160104986876103, 0.05413385826771666132, 0.4176697321401328100 ) ) ;
#10900=CARTESIAN_POINT ( 'NONE',  ( -1.043307086614172041, -0.4536011799217367080, 0.2665933059059888421 ) ) ;
#10901=CARTESIAN_POINT ( 'NONE',  ( 1.601049868766404982, 0.2306618581243848609, 0.2411417322834645549 ) ) ;
#10902=CARTESIAN_POINT ( 'NONE',  ( -1.272965879265091305, -0.4281496062992124485, 0.4176697321401328655 ) ) ;
#10903=CARTESIAN_POINT ( 'NONE',  ( -0.4527559055118102749, -0.5400638737290845981, -0.3530559997133363437 ) ) ;
#10904=CARTESIAN_POINT ( 'NONE',  ( 0.2821522309711292364, 0.2952755905511810219, -0.1292274648535930437 ) ) ;
#10905=CARTESIAN_POINT ( 'NONE',  ( -0.1377952755905504645, -0.4536011799217368745, -0.2665933059059886201 ) ) ;
#10906=CARTESIAN_POINT ( 'NONE',  ( -1.692913385826770645, 0.1771653543307087630, 0.000000000000000000 ) ) ;
#10907=CARTESIAN_POINT ( 'NONE',  ( 0.6627296587926517768, -0.6692913385826773087, -0.1292274648535924053 ) ) ;
#10909=CARTESIAN_POINT ( 'NONE',  ( 1.345144356955381593, -0.2845877964562161244, -0.3641732283464567121 ) ) ;
#10910=CARTESIAN_POINT ( 'NONE',  ( -0.8530183727034112984, -0.4281496062992127816, -0.4176697321401328100 ) ) ;
#10911=CARTESIAN_POINT ( 'NONE',  ( -0.07217847769028787330, -0.08942795157527998196, 0.3641732283464567121 ) ) ;
#10913=CARTESIAN_POINT ( 'NONE',  ( 0.1049868766404206816, -0.5023911411419708095, -0.1820866141732282451 ) ) ;
#10914=CARTESIAN_POINT ( 'NONE',  ( -0.02624671916010428221, 0.2306618581243847221, -0.2411417322834647770 ) ) ;
#10915=ADVANCED_FACE ( 'NONE', ( #16706 ), #42347, .F. ) ;
#10918=CARTESIAN_POINT ( 'NONE',  ( 0.6102362204724416372, -0.4536011799217367080, 0.2665933059059888421 ) ) ;
#10919=CARTESIAN_POINT ( 'NONE',  ( -0.5774278215223089816, -0.6046776061558807314, 0.2411417322834647770 ) ) ;
#10920=CARTESIAN_POINT ( 'NONE',  ( -0.7939632545931750718, -0.05778040916215560624, -0.4822834645669293319 ) ) ;
#10921=CARTESIAN_POINT ( 'NONE',  ( -0.7414698162729651543, -0.5511811023622046335, 0.09757992244046803654 ) ) ;
#10922=CARTESIAN_POINT ( 'NONE',  ( 2.795275590551181466, 2.793565526369266916, 0.000000000000000000 ) ) ;
#10923=CARTESIAN_POINT ( 'NONE',  ( -0.5708661417322825615, -0.4536011799217367080, 0.2665933059059888421 ) ) ;
#10924=CARTESIAN_POINT ( 'NONE',  ( -0.03280839895013062252, 0.2952755905511810774, -0.1292274648535930714 ) ) ;
#10925=CARTESIAN_POINT ( 'NONE',  ( -1.371391076115484831, 0.1771653543307087075, -0.09757992244046823083 ) ) ;
#10927=CARTESIAN_POINT ( 'NONE',  ( 1.568241469816273437, -0.3162353388693405765, 0.4822834645669290543 ) ) ;
#10930=CARTESIAN_POINT ( 'NONE',  ( -1.338582677165353729, -0.1870078740157480601, -0.3641732283464567677 ) ) ;
#10931=CARTESIAN_POINT ( 'NONE',  ( -0.3149606299212590610, -0.1870078740157479769, 0.4822834645669291653 ) ) ;
#10932=CARTESIAN_POINT ( 'NONE',  ( -1.332020997375327642, -0.05778040916215522460, 0.4822834645669289988 ) ) ;
#10934=CARTESIAN_POINT ( 'NONE',  ( 1.614173228346456712, 2.401574803149606474, 0.1372047244094478646 ) ) ;
#10935=CARTESIAN_POINT ( 'NONE',  ( 0.8661417322834653598, -0.1870078740157479769, 0.4822834645669291653 ) ) ;
#10936=CARTESIAN_POINT ( 'NONE',  ( 0.4658792650918641698, -0.05778040916215560624, -0.4822834645669293319 ) ) ;
#10939=CARTESIAN_POINT ( 'NONE',  ( 1.030183727034121421, -0.2845877964562161244, -0.3641732283464567121 ) ) ;
#10942=CARTESIAN_POINT ( 'NONE',  ( -0.7742782152230962556, -0.3690944881889765550, -0.3153832671262227771 ) ) ;
#10945=CARTESIAN_POINT ( 'NONE',  ( 0.2493438320209980519, -0.4281496062992127816, -0.4176697321401328100 ) ) ;
#10946=CARTESIAN_POINT ( 'NONE',  ( -0.3083989501312330295, -0.05778040916215522460, 0.4822834645669289988 ) ) ;
#10947=CARTESIAN_POINT ( 'NONE',  ( -1.082677165354329896, -0.5400638737290845981, -0.3530559997133363437 ) ) ;
#10948=CARTESIAN_POINT ( 'NONE',  ( 0.8989501312335964611, 0.2952755905511811885, 0.1292274648535926551 ) ) ;
#10949=CARTESIAN_POINT ( 'NONE',  ( -1.443569553805773564, 0.1283753931104746893, -0.1820866141732285504 ) ) ;
#10951=CARTESIAN_POINT ( 'NONE',  ( 0.1312335958005257930, 0.2306618581243847221, -0.2411417322834647770 ) ) ;
#10952=CARTESIAN_POINT ( 'NONE',  ( -1.227034120734907141, -0.6692913385826773087, -0.1292274648535924053 ) ) ;
#10954=DIRECTION ( 'NONE',  ( 0.000000000000000000, 0.000000000000000000, -1.000000000000000000 ) ) ;
#10957=CARTESIAN_POINT ( 'NONE',  ( 0.8792650918635177559, -0.004921259842519576551, 0.3153832671262227771 ) ) ;
#10960=CARTESIAN_POINT ( 'NONE',  ( -0.7086614173228339419, -0.1870078740157479769, 0.4822834645669291653 ) ) ;
#10961=ORIENTED_EDGE ( 'NONE', *, *, #27771, .F. ) ;
#10962=CARTESIAN_POINT ( 'NONE',  ( 0.006561679790026889343, -0.08942795157527998196, 0.3641732283464567121 ) ) ;
#10963=CARTESIAN_POINT ( 'NONE',  ( -1.620734908136482577, -0.6692913385826773087, -0.1292274648535924053 ) ) ;
#10964=CARTESIAN_POINT ( 'NONE',  ( 0.5118110236220478892, 0.2952755905511811885, 0.000000000000000000 ) ) ;
#10965=CARTESIAN_POINT ( 'NONE',  ( 0.5446194225721792126, -0.05778040916215560624, -0.4822834645669293319 ) ) ;
#10966=CARTESIAN_POINT ( 'NONE',  ( -0.5511811023622041894, -0.1870078740157480879, -0.4822834645669291653 ) ) ;
#10968=CARTESIAN_POINT ( 'NONE',  ( -0.7677165354330699465, -0.5400638737290845981, -0.3530559997133363437 ) ) ;
#10970=CARTESIAN_POINT ( 'NONE',  ( 1.227034120734908917, -0.5511811023622046335, 0.09757992244046803654 ) ) ;
#10971=CARTESIAN_POINT ( 'NONE',  ( -1.194225721784776262, -0.4281496062992124485, 0.4176697321401328655 ) ) ;
#10972=CARTESIAN_POINT ( 'NONE',  ( 0.8398950131233602345, -0.6046776061558807314, 0.2411417322834647770 ) ) ;
#10973=CARTESIAN_POINT ( 'NONE',  ( 1.017060367454068803, -0.3162353388693405765, 0.4822834645669290543 ) ) ;
#10975=CARTESIAN_POINT ( 'NONE',  ( -1.332020997375327642, -0.3162353388693409650, -0.4822834645669289433 ) ) ;
#10977=CARTESIAN_POINT ( 'NONE',  ( 0.2034120734908142214, 0.2952755905511810774, -0.1292274648535930714 ) ) ;
#10979=CARTESIAN_POINT ( 'NONE',  ( -1.377952755905511140, -0.5511811023622047445, 6.969142054262312111E-17 ) ) ;
#10980=CARTESIAN_POINT ( 'NONE',  ( 0.4527559055118117182, 0.07958543189024071263, -0.2665933059059888421 ) ) ;
#10981=CARTESIAN_POINT ( 'NONE',  ( 1.043307086614173818, -0.5400638737290845981, -0.3530559997133363437 ) ) ;
#10983=CARTESIAN_POINT ( 'NONE',  ( 0.7677165354330716118, 0.07958543189024071263, -0.2665933059059888421 ) ) ;
#10984=CARTESIAN_POINT ( 'NONE',  ( 0.6430446194225728496, 0.05413385826771666132, 0.4176697321401328100 ) ) ;
#10986=CARTESIAN_POINT ( 'NONE',  ( -0.8464566929133852113, -0.5400638737290845981, -0.3530559997133363437 ) ) ;
#10987=CARTESIAN_POINT ( 'NONE',  ( -0.2165354330708654795, 0.1660481256975885056, 0.3530559997133364547 ) ) ;
#10988=CARTESIAN_POINT ( 'NONE',  ( 1.056430446194226436, -0.5511811023622048555, -0.09757992244046775898 ) ) ;
#10989=CARTESIAN_POINT ( 'NONE',  ( -0.6496062992125976043, -0.5400638737290844871, 0.3530559997133364547 ) ) ;
#10990=CARTESIAN_POINT ( 'NONE',  ( 0.1640419947506569498, -0.05778040916215522460, 0.4822834645669289988 ) ) ;
#10992=CARTESIAN_POINT ( 'NONE',  ( 0.03280839895013198948, 0.2952755905511811885, 0.1292274648535926551 ) ) ;
#10993=EDGE_CURVE ( 'NONE', #13510, #52467, #57990, .T. ) ;
#10994=CARTESIAN_POINT ( 'NONE',  ( -0.01968503937007793844, 0.07958543189024071263, -0.2665933059059888421 ) ) ;
#10996=CARTESIAN_POINT ( 'NONE',  ( 0.1246719160104994284, 0.1771653543307087075, -0.09757992244046823083 ) ) ;
#10997=CARTESIAN_POINT ( 'NONE',  ( 0.9514435695538062676, -0.08942795157527998196, 0.3641732283464567121 ) ) ;
#10999=B_SPLINE_CURVE_WITH_KNOTS ( 'NONE', 3,
 ( #42780, #36474, #30158, #36891 ),
 .UNSPECIFIED., .F., .F.,
 ( 4, 4 ),
 ( 2.453269466693398698E-18, 0.002136818956423001525 ),
 .UNSPECIFIED. ) ;
#11001=CARTESIAN_POINT ( 'NONE',  ( 0.1706036745406830368, -0.4281496062992127816, -0.4176697321401328100 ) ) ;
#11002=EDGE_CURVE ( 'NONE', #4749, #26176, #76873, .T. ) ;
#11004=CARTESIAN_POINT ( 'NONE',  ( 1.535433070866142558, 0.1771653543307087630, 0.000000000000000000 ) ) ;
#11005=DIRECTION ( 'NONE',  ( 0.000000000000000000, 1.000000000000000000, 0.000000000000000000 ) ) ;
#11006=CARTESIAN_POINT ( 'NONE',  ( -0.3674540682414692561, -0.5023911411419708095, -0.1820866141732282451 ) ) ;
#11007=CARTESIAN_POINT ( 'NONE',  ( -0.5183727034120726440, 0.2952755905511811885, 0.1292274648535926551 ) ) ;
#11008=CARTESIAN_POINT ( 'NONE',  ( 1.115485564304462551, -0.3690944881889765550, -0.3153832671262227771 ) ) ;
#11010=CARTESIAN_POINT ( 'NONE',  ( 1.312335958005249825, 0.1283753931104746893, -0.1820866141732285504 ) ) ;
#11011=CARTESIAN_POINT ( 'NONE',  ( -0.05905511811023545637, 0.1660481256975885056, 0.3530559997133364547 ) ) ;
#11013=CARTESIAN_POINT ( 'NONE',  ( 0.9711286089238851948, -0.6046776061558809534, -0.2411417322834644161 ) ) ;
#11016=CARTESIAN_POINT ( 'NONE',  ( 0.05905511811023681640, 0.1660481256975883668, -0.3530559997133364547 ) ) ;
#11017=CARTESIAN_POINT ( 'NONE',  ( 1.502624671916010790, -0.05778040916215522460, 0.4822834645669289988 ) ) ;
#11018=CARTESIAN_POINT ( 'NONE',  ( 0.4986876640419954376, -0.6046776061558809534, -0.2411417322834644161 ) ) ;
#11020=CARTESIAN_POINT ( 'NONE',  ( -1.732283464566928277, -0.1870078740157479769, 0.3641732283464567677 ) ) ;
#11021=CARTESIAN_POINT ( 'NONE',  ( 0.8464566929133866546, -0.4536011799217367080, 0.2665933059059888421 ) ) ;
#11022=CARTESIAN_POINT ( 'NONE',  ( 1.187664041994751285, -0.05778040916215522460, 0.4822834645669289988 ) ) ;
#11023=CARTESIAN_POINT ( 'NONE',  ( 0.1574803149606306130, -0.1870078740157479769, 0.3641732283464567677 ) ) ;
#11024=CARTESIAN_POINT ( 'NONE',  ( -0.1181102362204717315, -0.6692913385826771977, 8.415575281601705876E-17 ) ) ;
#11025=CARTESIAN_POINT ( 'NONE',  ( 0.5839895013123367340, -0.6692913385826773087, -0.1292274648535924053 ) ) ;
#11027=CARTESIAN_POINT ( 'NONE',  ( -0.6430446194225712953, 0.05413385826771626580, -0.4176697321401330321 ) ) ;
#11028=CARTESIAN_POINT ( 'NONE',  ( -0.3280839895013117347, -0.3690944881889763329, 0.3153832671262228327 ) ) ;
#11029=CARTESIAN_POINT ( 'NONE',  ( 0.6036745406824153282, -0.6046776061558807314, 0.2411417322834647770 ) ) ;
#11030=CARTESIAN_POINT ( 'NONE',  ( 1.108923884514436686, -0.2845877964562161244, -0.3641732283464567121 ) ) ;
#11031=CARTESIAN_POINT ( 'NONE',  ( 0.1443569553805781891, 0.05413385826771626580, -0.4176697321401330321 ) ) ;
#11036=CARTESIAN_POINT ( 'NONE',  ( -1.043307086614172041, -0.5400638737290844871, 0.3530559997133364547 ) ) ;
#11037=CARTESIAN_POINT ( 'NONE',  ( -0.4265091863517051496, 0.2952755905511810774, -0.1292274648535930714 ) ) ;
#11041=CARTESIAN_POINT ( 'NONE',  ( 0.2034120734908144990, -0.5511811023622046335, 0.09757992244046803654 ) ) ;
#11043=CARTESIAN_POINT ( 'NONE',  ( 0.7742782152230978099, -0.4281496062992124485, 0.4176697321401328655 ) ) ;
#11046=ADVANCED_FACE ( 'NONE', ( #642 ), #77664, .F. ) ;
#11047=CARTESIAN_POINT ( 'NONE',  ( -0.2821522309711278487, 0.2952755905511811885, 0.1292274648535926551 ) ) ;
#11048=CARTESIAN_POINT ( 'NONE',  ( 1.089238845144357759, 0.05413385826771626580, -0.4176697321401330321 ) ) ;
#11049=CARTESIAN_POINT ( 'NONE',  ( 1.463254593175853824, 0.1771653543307087075, -0.09757992244046823083 ) ) ;
#11050=CARTESIAN_POINT ( 'NONE',  ( 0.01312335958005323398, -0.4281496062992127816, -0.4176697321401328100 ) ) ;
#11052=CARTESIAN_POINT ( 'NONE',  ( -0.4265091863517051496, -0.6692913385826771977, 0.1292274648535927661 ) ) ;
#11053=CARTESIAN_POINT ( 'NONE',  ( -1.095800524934382292, -0.08942795157527998196, 0.3641732283464567121 ) ) ;
#11054=CARTESIAN_POINT ( 'NONE',  ( 0.5183727034120741983, 0.2952755905511810774, -0.1292274648535930714 ) ) ;
#11055=CARTESIAN_POINT ( 'NONE',  ( -0.5643044619422565855, 0.05413385826771626580, -0.4176697321401330321 ) ) ;
#11060=CARTESIAN_POINT ( 'NONE',  ( 0.2821522309711292364, 0.2952755905511810774, -0.1292274648535930714 ) ) ;
#11061=CARTESIAN_POINT ( 'NONE',  ( -0.4855643044619415427, -0.4281496062992124485, 0.4176697321401328655 ) ) ;
#11062=CARTESIAN_POINT ( 'NONE',  ( -1.437007874015747477, 0.1660481256975883668, -0.3530559997133364547 ) ) ;
#11063=CARTESIAN_POINT ( 'NONE',  ( 1.128608923884514947, 0.2306618581243848609, 0.2411417322834645549 ) ) ;
#11064=CARTESIAN_POINT ( 'NONE',  ( 0.4658792650918641698, -0.05778040916215560624, -0.4822834645669293319 ) ) ;
#11066=CARTESIAN_POINT ( 'NONE',  ( -0.9317585301837263412, 0.05413385826771666132, 0.4176697321401328100 ) ) ;
#11067=CARTESIAN_POINT ( 'NONE',  ( 0.4133858267716541968, 0.1660481256975885056, 0.3530559997133364547 ) ) ;
#11068=CARTESIAN_POINT ( 'NONE',  ( -0.4461942257217840213, -0.6046776061558809534, -0.2411417322834644161 ) ) ;
#11069=CARTESIAN_POINT ( 'NONE',  ( 0.1574803149606306130, -0.1870078740157480601, -0.3641732283464567677 ) ) ;
#11070=DIRECTION ( 'NONE',  ( 0.000000000000000000, 0.000000000000000000, 1.000000000000000000 ) ) ;
#11071=CARTESIAN_POINT ( 'NONE',  ( -1.586052503253847501, 1.299212598425198095, -0.1653254495020571035 ) ) ;
#11072=CARTESIAN_POINT ( 'NONE',  ( 0.1771653543307093182, 0.1660481256975885056, 0.3530559997133364547 ) ) ;
#11075=ADVANCED_FACE ( 'NONE', ( #25046 ), #24643, .F. ) ;
#11076=CARTESIAN_POINT ( 'NONE',  ( -1.640419947506561060, 0.05413385826771666132, 0.4176697321401328100 ) ) ;
#11080=CARTESIAN_POINT ( 'NONE',  ( 0.5971128608923891301, 0.2952755905511810774, -0.1292274648535930714 ) ) ;
#11081=CARTESIAN_POINT ( 'NONE',  ( 0.2296587926509192634, -0.08942795157528024563, -0.3641732283464568787 ) ) ;
#11086=CARTESIAN_POINT ( 'NONE',  ( 0.7186703366786207914, -1.374501131054255944E-15, 0.4445507791589066726 ) ) ;
#11089=CARTESIAN_POINT ( 'NONE',  ( 0.4265091863517067039, -0.6692913385826773087, -0.1292274648535924053 ) ) ;
#11090=CARTESIAN_POINT ( 'NONE',  ( -0.7217847769028863381, -0.4281496062992124485, 0.4176697321401328655 ) ) ;
#11091=CARTESIAN_POINT ( 'NONE',  ( -1.351706036745406347, 0.05413385826771626580, -0.4176697321401330321 ) ) ;
#11092=CARTESIAN_POINT ( 'NONE',  ( 0.5708661417322841158, -0.5400638737290845981, -0.3530559997133363437 ) ) ;
#11093=CARTESIAN_POINT ( 'NONE',  ( 1.489501312335958172, -0.05778040916215560624, -0.4822834645669293319 ) ) ;
#11094=CARTESIAN_POINT ( 'NONE',  ( 1.509186351706037543, -0.004921259842519576551, 0.3153832671262227771 ) ) ;
#11095=CARTESIAN_POINT ( 'NONE',  ( 1.220472440944882608, 0.1771653543307087630, 0.000000000000000000 ) ) ;
#11096=CARTESIAN_POINT ( 'NONE',  ( -0.9120734908136475250, -0.6692913385826773087, -0.1292274648535924053 ) ) ;
#11098=CARTESIAN_POINT ( 'NONE',  ( 1.423884514435696413, -0.3162353388693409650, -0.4822834645669289433 ) ) ;
#11101=CARTESIAN_POINT ( 'NONE',  ( -0.2821522309711278487, -0.6692913385826773087, -0.1292274648535924053 ) ) ;
#11103=CARTESIAN_POINT ( 'NONE',  ( 1.187664041994751285, -0.05778040916215522460, 0.4822834645669289988 ) ) ;
#11105=CARTESIAN_POINT ( 'NONE',  ( -1.030183727034119867, -0.08942795157528024563, -0.3641732283464568787 ) ) ;
#11106=CARTESIAN_POINT ( 'NONE',  ( 0.5905511811023629321, 0.2952755905511811885, 0.000000000000000000 ) ) ;
#11107=CARTESIAN_POINT ( 'NONE',  ( 0.9711286089238851948, 0.1283753931104748280, 0.1820866141732283561 ) ) ;
#11109=CARTESIAN_POINT ( 'NONE',  ( -1.332020997375327642, -0.2845877964562161244, -0.3641732283464567121 ) ) ;
#11110=CARTESIAN_POINT ( 'NONE',  ( 0.7611548556430454138, 0.2306618581243847221, -0.2411417322834647770 ) ) ;
#11111=DIRECTION ( 'NONE',  ( 0.000000000000000000, 1.000000000000000000, 0.000000000000000000 ) ) ;
#11112=CARTESIAN_POINT ( 'NONE',  ( -0.4658792650918627265, -0.08942795157527998196, 0.3641732283464567121 ) ) ;
#11113=CARTESIAN_POINT ( 'NONE',  ( -0.01968503937007793844, -0.5400638737290844871, 0.3530559997133364547 ) ) ;
#11114=CARTESIAN_POINT ( 'NONE',  ( -1.391076115485563314, -0.5023911411419708095, -0.1820866141732282451 ) ) ;
#11115=CARTESIAN_POINT ( 'NONE',  ( -0.8267716535433065062, -0.6692913385826771977, 8.415575281601705876E-17 ) ) ;
#11116=CARTESIAN_POINT ( 'NONE',  ( 1.397637795275591177, 0.1660481256975883668, -0.3530559997133364547 ) ) ;
#11118=CARTESIAN_POINT ( 'NONE',  ( -0.8267716535433065062, 0.1771653543307087630, 0.000000000000000000 ) ) ;
#11120=CARTESIAN_POINT ( 'NONE',  ( 1.502624671916010790, -0.3162353388693409650, -0.4822834645669289433 ) ) ;
#11122=CARTESIAN_POINT ( 'NONE',  ( -1.312335958005248715, -0.6046776061558809534, -0.2411417322834644161 ) ) ;
#11123=CARTESIAN_POINT ( 'NONE',  ( -1.627296587926508442, 0.1283753931104748280, 0.1820866141732283561 ) ) ;
#11124=CARTESIAN_POINT ( 'NONE',  ( -0.7611548556430438595, 0.1283753931104748280, 0.1820866141732283561 ) ) ;
#11125=CARTESIAN_POINT ( 'NONE',  ( -0.4848604877838266214, -2.609869883881465018E-15, -0.3464511005275220379 ) ) ;
#11126=CARTESIAN_POINT ( 'NONE',  ( -0.05905511811023545637, 0.1660481256975885056, 0.3530559997133364547 ) ) ;
#11127=CARTESIAN_POINT ( 'NONE',  ( -0.09186351706036663400, -0.3690944881889763329, 0.3153832671262228327 ) ) ;
#11128=CARTESIAN_POINT ( 'NONE',  ( -1.351706036745406347, -0.004921259842519870586, -0.3153832671262229437 ) ) ;
#11129=CARTESIAN_POINT ( 'NONE',  ( -1.673228346456691717, 0.1660481256975883668, -0.3530559997133364547 ) ) ;
#11130=CARTESIAN_POINT ( 'NONE',  ( 1.240157480314961314, -0.4536011799217367080, 0.2665933059059888421 ) ) ;
#11131=AXIS2_PLACEMENT_3D ( 'NONE', #46278, #63567, #31574 ) ;
#11132=CARTESIAN_POINT ( 'NONE',  ( 1.141732283464567788, -0.6692913385826771977, 8.415575281601705876E-17 ) ) ;
#11134=CARTESIAN_POINT ( 'NONE',  ( 0.4724409448818904789, -0.1870078740157480601, -0.3641732283464567677 ) ) ;
#11135=CARTESIAN_POINT ( 'NONE',  ( 1.049868766404200349, 0.2306618581243848609, 0.2411417322834645549 ) ) ;
#11136=CARTESIAN_POINT ( 'NONE',  ( 0.9776902887139113929, 0.1771653543307087630, 0.09757992244046791164 ) ) ;
#11138=CARTESIAN_POINT ( 'NONE',  ( -1.364829396325458521, -0.6046776061558807314, 0.2411417322834647770 ) ) ;
#11139=CARTESIAN_POINT ( 'NONE',  ( -1.102362204724408601, -0.1870078740157480879, -0.4822834645669291653 ) ) ;
#11140=CARTESIAN_POINT ( 'NONE',  ( -0.2690288713910754526, 0.2952755905511810774, -0.1292274648535930714 ) ) ;
#11143=CARTESIAN_POINT ( 'NONE',  ( 0.2559055118110243332, -0.5400638737290845981, -0.3530559997133363437 ) ) ;
#11144=CARTESIAN_POINT ( 'NONE',  ( 1.469816272965879911, 0.1283753931104746893, -0.1820866141732285504 ) ) ;
#11145=CARTESIAN_POINT ( 'NONE',  ( -0.05249343832020911260, 0.2306618581243848609, 0.2411417322834645549 ) ) ;
#11146=CARTESIAN_POINT ( 'NONE',  ( 0.7217847769028878924, -0.4281496062992127816, -0.4176697321401328100 ) ) ;
#11154=CARTESIAN_POINT ( 'NONE',  ( -0.6430446194225716283, -0.3690944881889763329, 0.3153832671262228327 ) ) ;
#11155=CARTESIAN_POINT ( 'NONE',  ( -0.6758530183727028406, -0.6692913385826773087, -0.1292274648535924053 ) ) ;
#11156=CARTESIAN_POINT ( 'NONE',  ( 0.4133858267716541968, -0.5400638737290845981, -0.3530559997133363437 ) ) ;
#11158=CARTESIAN_POINT ( 'NONE',  ( 0.8005249343832028242, -0.4281496062992127816, -0.4176697321401328100 ) ) ;
#11159=CARTESIAN_POINT ( 'NONE',  ( 1.509186351706037543, -0.4281496062992127816, -0.4176697321401328100 ) ) ;
#11160=CARTESIAN_POINT ( 'NONE',  ( 1.266404199475066328, -0.05778040916215522460, 0.4822834645669289988 ) ) ;
#11164=CARTESIAN_POINT ( 'NONE',  ( 0.9055118110236227702, -0.6692913385826771977, 8.415575281601705876E-17 ) ) ;
#11165=CARTESIAN_POINT ( 'NONE',  ( 0.4855643044619428750, 0.05413385826771666132, 0.4176697321401328100 ) ) ;
#11166=CARTESIAN_POINT ( 'NONE',  ( 1.305774278215223960, 0.1771653543307087075, -0.09757992244046823083 ) ) ;
#11167=CARTESIAN_POINT ( 'NONE',  ( 1.581364829396326277, -0.3162353388693409650, -0.4822834645669289433 ) ) ;
#11168=CARTESIAN_POINT ( 'NONE',  ( 1.528871391076116026, -0.6692913385826773087, -0.1292274648535924053 ) ) ;
#11171=CARTESIAN_POINT ( 'NONE',  ( 0.7283464566929143125, 0.1660481256975885056, 0.3530559997133364547 ) ) ;
#11173=CARTESIAN_POINT ( 'NONE',  ( 1.535433070866142558, 0.1771653543307087630, 0.000000000000000000 ) ) ;
#11174=CARTESIAN_POINT ( 'NONE',  ( -0.6233595800524928121, -0.05778040916215522460, 0.4822834645669289988 ) ) ;
#11175=CARTESIAN_POINT ( 'NONE',  ( -0.6233595800524928121, -0.05778040916215522460, 0.4822834645669289988 ) ) ;
#11176=CARTESIAN_POINT ( 'NONE',  ( 1.568241469816273437, -0.3162353388693405765, 0.4822834645669290543 ) ) ;
#11180=CARTESIAN_POINT ( 'NONE',  ( -1.653543307086613234, -0.1870078740157479769, 0.3641732283464567677 ) ) ;
#11183=ORIENTED_EDGE ( 'NONE', *, *, #80420, .F. ) ;
#11184=CARTESIAN_POINT ( 'NONE',  ( -1.586052503253847057, 1.574803149606300412, -0.1653254495020572423 ) ) ;
#11185=CARTESIAN_POINT ( 'NONE',  ( 1.476377952755906220, 0.07958543189024071263, -0.2665933059059888421 ) ) ;
#11189=CARTESIAN_POINT ( 'NONE',  ( 0.4531182788721078158, 1.535433070866141447, 0.5309055118110234117 ) ) ;
#11194=CARTESIAN_POINT ( 'NONE',  ( -0.8136482939632537770, 0.1283753931104746893, -0.1820866141732285504 ) ) ;
#11195=CARTESIAN_POINT ( 'NONE',  ( -1.181102362204723644, -0.1870078740157480601, -0.3641732283464567677 ) ) ;
#11196=CARTESIAN_POINT ( 'NONE',  ( 0.6496062992125991586, 0.1660481256975885056, 0.3530559997133364547 ) ) ;
#11197=CARTESIAN_POINT ( 'NONE',  ( -1.279527559055116948, 0.1660481256975883668, -0.3530559997133364547 ) ) ;
#11200=CARTESIAN_POINT ( 'NONE',  ( 1.391076115485564868, -0.6046776061558807314, 0.2411417322834647770 ) ) ;
#11206=CARTESIAN_POINT ( 'NONE',  ( -1.049868766404198794, -0.6046776061558807314, 0.2411417322834647770 ) ) ;
#11207=CARTESIAN_POINT ( 'NONE',  ( 1.161417322834646493, -0.5400638737290844871, 0.3530559997133364547 ) ) ;
#11210=CARTESIAN_POINT ( 'NONE',  ( -1.725721784776902190, -0.05778040916215522460, 0.4822834645669289988 ) ) ;
#11211=CARTESIAN_POINT ( 'NONE',  ( -1.200787401574802349, 0.1660481256975883668, -0.3530559997133364547 ) ) ;
#11213=CARTESIAN_POINT ( 'NONE',  ( 0.1968503937007881344, 0.1771653543307087630, 0.000000000000000000 ) ) ;
#11215=CARTESIAN_POINT ( 'NONE',  ( -0.1246719160104980823, -0.5511811023622048555, -0.09757992244046775898 ) ) ;
#11216=CARTESIAN_POINT ( 'NONE',  ( 0.4921259842519691285, 0.07958543189024085140, 0.2665933059059887866 ) ) ;
#11217=CARTESIAN_POINT ( 'NONE',  ( 0.5183727034120741983, 0.2952755905511810774, -0.1292274648535930714 ) ) ;
#11218=CARTESIAN_POINT ( 'NONE',  ( -0.6889763779527552368, 0.07958543189024085140, 0.2665933059059887866 ) ) ;
#11220=CARTESIAN_POINT ( 'NONE',  ( 1.476377952755906220, 0.1660481256975883668, -0.3530559997133364547 ) ) ;
#11221=CARTESIAN_POINT ( 'NONE',  ( -0.8333333333333323711, 0.2952755905511811885, 0.1292274648535926551 ) ) ;
#11223=B_SPLINE_CURVE_WITH_KNOTS ( 'NONE', 3,
 ( #58700, #1066, #78081, #72176 ),
 .UNSPECIFIED., .F., .F.,
 ( 4, 4 ),
 ( 0.07239528109754661545, 0.07258229963060301715 ),
 .UNSPECIFIED. ) ;
#11224=CARTESIAN_POINT ( 'NONE',  ( -0.1509186351706028884, -0.05778040916215522460, 0.4822834645669289988 ) ) ;
#11225=CARTESIAN_POINT ( 'NONE',  ( -0.7086614173228339419, -0.1870078740157479769, 0.4822834645669291653 ) ) ;
#11226=CARTESIAN_POINT ( 'NONE',  ( 1.154855643044620184, -0.5023911411419708095, 0.1820866141732285504 ) ) ;
#11227=CARTESIAN_POINT ( 'NONE',  ( -0.03937007874015669567, -0.5511811023622047445, 6.969142054262312111E-17 ) ) ;
#11228=CARTESIAN_POINT ( 'NONE',  ( -0.1902887139107604098, -0.6692913385826771977, 0.1292274648535927661 ) ) ;
#11229=CARTESIAN_POINT ( 'NONE',  ( -1.325459317585300889, 0.05413385826771666132, 0.4176697321401328100 ) ) ;
#11231=CARTESIAN_POINT ( 'NONE',  ( 1.673228346456693494, 0.07958543189024085140, 0.2665933059059887866 ) ) ;
#11233=CARTESIAN_POINT ( 'NONE',  ( -0.2427821522309703550, -0.3162353388693405765, 0.4822834645669290543 ) ) ;
#11236=CARTESIAN_POINT ( 'NONE',  ( 0.9580052493438326877, 0.05413385826771666132, 0.4176697321401328100 ) ) ;
#11237=CARTESIAN_POINT ( 'NONE',  ( -0.7152230971128602510, -0.08942795157528024563, -0.3641732283464568787 ) ) ;
#11238=CARTESIAN_POINT ( 'NONE',  ( -0.6430446194225716283, -0.4281496062992124485, 0.4176697321401328655 ) ) ;
#11239=CARTESIAN_POINT ( 'NONE',  ( 1.076115485564305141, 0.2306618581243847221, -0.2411417322834647770 ) ) ;
#11240=CARTESIAN_POINT ( 'NONE',  ( 0.7217847769028878924, 0.05413385826771666132, 0.4176697321401328100 ) ) ;
#11242=CARTESIAN_POINT ( 'NONE',  ( -1.128608923884513837, -0.5023911411419708095, 0.1820866141732285504 ) ) ;
#11246=VECTOR ( 'NONE', #43428, 39.37007874015748143 ) ;
#11250=CARTESIAN_POINT ( 'NONE',  ( 0.6889763779527563470, 0.07958543189024071263, -0.2665933059059888421 ) ) ;
#11251=CARTESIAN_POINT ( 'NONE',  ( 0.3477690288713918276, 0.2952755905511811885, 0.1292274648535926551 ) ) ;
#11254=CARTESIAN_POINT ( 'NONE',  ( 0.7217847769028878924, -0.004921259842519576551, 0.3153832671262227771 ) ) ;
#11255=CARTESIAN_POINT ( 'NONE',  ( -0.1574803149606292529, -0.1870078740157480879, -0.4822834645669291653 ) ) ;
#11256=CARTESIAN_POINT ( 'NONE',  ( -0.9580052493438311334, 0.05413385826771626580, -0.4176697321401330321 ) ) ;
#11257=CARTESIAN_POINT ( 'NONE',  ( 1.423884514435696413, -0.3162353388693409650, -0.4822834645669289433 ) ) ;
#11260=CARTESIAN_POINT ( 'NONE',  ( -0.2755905511811018171, 0.1771653543307087630, 0.000000000000000000 ) ) ;
#11263=ORIENTED_EDGE ( 'NONE', *, *, #64557, .T. ) ;
#11264=CARTESIAN_POINT ( 'NONE',  ( -1.056430446194224881, 0.2952755905511810774, -0.1292274648535930714 ) ) ;
#11265=CARTESIAN_POINT ( 'NONE',  ( -0.2165354330708654795, 0.1660481256975885056, 0.3530559997133364547 ) ) ;
#11266=CARTESIAN_POINT ( 'NONE',  ( -0.4002624671916004129, -0.3162353388693405765, 0.4822834645669290543 ) ) ;
#11267=CARTESIAN_POINT ( 'NONE',  ( 0.3083989501312343062, -0.05778040916215560624, -0.4822834645669293319 ) ) ;
#11268=CARTESIAN_POINT ( 'NONE',  ( -0.2624671916010490880, -0.6046776061558807314, 0.2411417322834647770 ) ) ;
#11269=CARTESIAN_POINT ( 'NONE',  ( -1.240157480314959759, -0.5400638737290845981, -0.3530559997133363437 ) ) ;
#11270=CARTESIAN_POINT ( 'NONE',  ( -0.9120734908136475250, 0.2952755905511811885, 0.1292274648535926551 ) ) ;
#11271=CARTESIAN_POINT ( 'NONE',  ( 0.9514435695538062676, -0.05778040916215522460, 0.4822834645669289988 ) ) ;
#11273=CARTESIAN_POINT ( 'NONE',  ( -0.5511811023622038563, -0.1870078740157479769, 0.3641732283464567677 ) ) ;
#11277=CARTESIAN_POINT ( 'NONE',  ( -1.377952755905511140, 0.1771653543307087630, 0.000000000000000000 ) ) ;
#11278=CARTESIAN_POINT ( 'NONE',  ( -0.9317585301837263412, -0.4281496062992127816, -0.4176697321401328100 ) ) ;
#11279=CARTESIAN_POINT ( 'NONE',  ( -0.8464566929133852113, 0.1660481256975885056, 0.3530559997133364547 ) ) ;
#11281=CARTESIAN_POINT ( 'NONE',  ( -0.8923884514435688198, 0.2306618581243847221, -0.2411417322834647770 ) ) ;
#11282=CARTESIAN_POINT ( 'NONE',  ( -0.8333333333333323711, -0.6692913385826773087, -0.1292274648535924053 ) ) ;
#11283=CARTESIAN_POINT ( 'NONE',  ( -1.522309711286088607, -0.6046776061558807314, 0.2411417322834647770 ) ) ;
#11285=CARTESIAN_POINT ( 'NONE',  ( 0.5577427821522316087, -0.08942795157527998196, 0.3641732283464567121 ) ) ;
#11288=CARTESIAN_POINT ( 'NONE',  ( 0.1049868766404206816, -0.5023911411419708095, -0.1820866141732282451 ) ) ;
#11290=CARTESIAN_POINT ( 'NONE',  ( -0.4593175853018364174, -0.4281496062992127816, -0.4176697321401328100 ) ) ;
#11291=CARTESIAN_POINT ( 'NONE',  ( 1.587926509186352142, 0.05413385826771666132, 0.4176697321401328100 ) ) ;
#11292=CARTESIAN_POINT ( 'NONE',  ( -0.06561679790026180015, 0.05413385826771666132, 0.4176697321401328100 ) ) ;
#11295=CARTESIAN_POINT ( 'NONE',  ( -0.5636006452641416642, -2.613618158232546091E-15, -0.3464511005275220379 ) ) ;
#11299=CARTESIAN_POINT ( 'NONE',  ( -0.9120734908136475250, 0.1771653543307087630, 0.09757992244046791164 ) ) ;
#11300=CARTESIAN_POINT ( 'NONE',  ( -0.9645669291338575535, -0.5400638737290844871, 0.3530559997133364547 ) ) ;
#11304=CARTESIAN_POINT ( 'NONE',  ( 1.154855643044620184, -0.6046776061558807314, 0.2411417322834647770 ) ) ;
#11305=CARTESIAN_POINT ( 'NONE',  ( 0.3740157480314966754, 0.1660481256975883668, -0.3530559997133364547 ) ) ;
#11306=CARTESIAN_POINT ( 'NONE',  ( 0.7086614173228353852, -0.1870078740157479769, 0.4822834645669291653 ) ) ;
#11307=CARTESIAN_POINT ( 'NONE',  ( -1.003937007874014853, 0.07958543189024085140, 0.2665933059059887866 ) ) ;
#11308=CARTESIAN_POINT ( 'NONE',  ( -0.3937007874015740483, -0.1870078740157480879, -0.4822834645669291653 ) ) ;
#11310=CARTESIAN_POINT ( 'NONE',  ( -0.8333333333333323711, -0.6692913385826773087, -0.1292274648535924053 ) ) ;
#11312=CARTESIAN_POINT ( 'NONE',  ( 1.128608923884514947, 0.1283753931104748280, 0.1820866141732283561 ) ) ;
#11313=CARTESIAN_POINT ( 'NONE',  ( -0.4986876640419942164, -0.5023911411419708095, 0.1820866141732285504 ) ) ;
#11314=CARTESIAN_POINT ( 'NONE',  ( 1.108923884514436686, -0.2845877964562161244, -0.3641732283464567121 ) ) ;
#11315=CARTESIAN_POINT ( 'NONE',  ( 1.574803149606299746, -0.1870078740157479769, 0.3641732283464567677 ) ) ;
#11316=CARTESIAN_POINT ( 'NONE',  ( -1.108923884514435132, -0.08942795157528024563, -0.3641732283464568787 ) ) ;
#11317=CARTESIAN_POINT ( 'NONE',  ( 0.1455472725388437250, -8.032016466602779066E-18, -0.3627985898453512936 ) ) ;
#11318=CARTESIAN_POINT ( 'NONE',  ( 0.4855643044619430415, -0.3690944881889765550, -0.3153832671262227771 ) ) ;
#11319=CARTESIAN_POINT ( 'NONE',  ( -0.5380577427821514602, 0.05413385826771666132, 0.4176697321401328100 ) ) ;
#11320=( BOUNDED_SURFACE ( )  B_SPLINE_SURFACE ( 1, 2, ( 
 ( #11502, #23286, #24110, #48956, #74657, #17001, #24927, #6409, #31247, #38811, #50595, #5992, #51418, #7248, #32495, #57740, #19881, #19035, #38392, #18632, #44682, #32920, #76303, #51003, #51842, #26180, #70810, #64488, #37567, #12320, #64911, #63653, #77120, #58159, #44276, #77549, #32079, #6826, #13160, #69966, #37978, #31663, #527, #57324, #76702, #71228, #52261, #45530, #102, #83018, #58586, #13572, #39226, #69565, #954, #25756, #25341, #19453, #45104, #70378, #12733, #26609, #77967, #43866, #11913, #63241, #5581, #56913, #82609, #64072, #53518, #34596, #1366, #2610, #66167, #66583, #47202, #27018, #46369, #65760, #8919, #8093, #27433, #47618, #28686, #40902, #8507, #52679, #9335, #28267, #15661, #45946, #53929, #34173, #78387, #59837, #2190, #53095, #78805, #21959, #41322, #79641, #72892, #15242, #65343, #67003, #7680, #73314, #27859, #60261, #40489, #60671, #20297, #35006, #3019, #54347, #33757, #33349, #79225, #20718, #71644, #13995, #39652, #59011, #14422, #72063, #40073, #21541, #59419, #21134, #1775, #46789, #72480, #14829, #30746, #41719, #16073, #35417, #3847, #81704, #54767, #74560, #37057, #42134, #16906, #35833, #55168, #81286, #42544, #68247, #55576, #73738, #49271, #36640, #17723, #61500, #49682, #62316, #74143, #29507, #23189, #61908, #16488, #67412, #9746, #11400, #24014, #67829, #80877, #80058, #29912, #48860, #61082, #10581, #3433, #74974, #29095, #10168, #4250, #43349, #68641, #36238, #55992, #23602, #17319, #80471, #42947, #69051, #22783, #10980, #4653, #30326, #75374, #62741, #48443, #5077, #22376, #48036, #38711, #51740, #82108, #64389, #70281, #31147, #18939, #12634, #5892, #31564, #58058, #77443, #32395, #25658, #6, #18129, #19776, #43762, #26080, #38293, #51320, #76609, #13468, #56409, #45430, #71125, #39125, #69873, #69467, #63970, #37472, #6725, #64806, #7145, #24421, #50497, #77023, #50091, #6306, #57643, #57222, #12226, #31983, #75787, #424, #11820, #63145, #5486, #56813, #63558, #82512, #24828, #50908, #76200, #18538, #44587, #37883, #82923, #19356, #45005, #70705, #13057, #44181, #25244, #72791, #53827, #71965, #2511, #15141, #26918, #65668, #59321, #14734, #52578, #77865, #20194, #47518, #60159, #20618, #33658, #66907, #66069, #1677, #13891, #78707, #45845, #27755, #39550, #78287, #40386, #79541, #21445, #46691, #8817, #7994, #27334, #7577, #52994, #21854, #65239, #39978, #40797, #66482, #59736, #53419, #26507, #1270, #73210, #46270, #8405, #47102, #33249, #34494, #21031, #79128, #2090, #58911, #14320, #72384, #28170, #34072, #15560, #41220, #32818, #58485, #850, #52161, #71544, #54662, #74879, #17223, #55896, #54244, #80373, #67730, #73637, #42855, #29819, #15979, #28996, #41626, #67315, #23094, #68548, #62225, #2924, #80778, #28588, #48761, #60982, #10889, #74042, #9650, #47934, #74460, #68143, #35319, #22686, #3332, #81608, #4563, #79961, #48345, #49590, #10065, #36549, #23924, #16389, #10488, #42036, #22274, #35728, #61398, #30234, #3747, #16807, #29411, #55070, #9238, #60573, #34910, #75285, #42443, #43260, #17628, #36142, #55480, #61814, #4154, #81190, #23507, #49174, #82825, #38613, #11728, #19251, #37384, #38196, #5798, #18847, #6209, #44903, #50000, #31468, #32297, #69375, #18449, #64291, #68957, #44091, #44493, #69785, #43672, #11307, #50408, #51225, #5393, #75697, #63871, #6625, #25558, #70184, #50817, #70601, #12955, #57957, #37787, #31886, #31055, #76106, #57130, #12130, #56318, #325, #82421, #76923, #25979, #12537, #24330, #19671, #51637, #25149, #63464, #76518, #77342, #57546, #83237, #36966, #62643, #63055, #4987, #30654, #82016, #56724, #18038, #24740, #33558, #20518, #32717, #60057, #58813, #1991, #72695, #46589, #745, #79436, #79029, #59221, #52479, #27237, #15042, #1582, #72287, #40698, #65563, #26404, #45332, #14633, #7897, #2412, #71027, #8720, #34391, #28070, #1170, #58384, #52896, #52060, #27654, #53728, #66383, #13371, #39449, #40289, #39024, #78609, #65970, #46170, #26821, #20932, #64708, #21348, #7048, #77766, #20098, #45749, #78187, #47001, #71444, #39874, #13792, #7473, #8307 ),
 ( #65137, #33974, #33142, #71866, #14216, #59635, #53317, #81091, #79858, #55796, #17124, #16292, #42345, #21755, #54561, #41118, #9963, #61295, #35634, #74775, #47833, #55385, #73538, #74361, #41936, #54977, #68043, #23408, #2823, #67632, #68453, #22175, #80276, #42758, #47418, #22590, #80684, #48251, #15883, #73109, #3235, #4056, #41531, #28484, #16704, #10792, #61718, #22998, #3651, #49075, #36452, #62126, #73947, #10389, #67217, #28899, #29316, #48663, #15460, #36046, #29723, #4468, #60884, #30133, #66808, #9550, #9142, #34813, #60472, #35220, #54144, #68858, #12853, #25455, #69274, #82321, #32198, #31364, #50307, #62541, #43988, #11207, #76415, #4879, #43573, #5693, #44800, #70081, #12027, #57443, #56621, #76005, #56219, #24640, #70495, #30553, #5294, #6108, #63768, #25043, #18745, #75185, #49900, #19149, #17937, #57029, #12434, #81917, #31781, #69684, #44388, #50717, #24228, #75598, #11620, #38094, #37282, #30954, #51122, #6528, #83136, #37684, #62957, #38511, #76817, #64193, #23824, #81503, #63359, #18347, #82723, #49493, #17531, #43162, #36866, #78917, #33866, #27129, #1475, #19566, #52793, #70926, #13272, #57854, #78503, #78079, #14935, #221, #21238, #46894, #40594, #71338, #45226, #65457, #38924, #40182, #72588, #27547, #8616, #51955, #20825, #66276, #7789, #59118, #33029, #13685, #14109, #25872, #8201, #51534, #64604, #77237, #6940, #65025, #59530, #32612, #52371, #58274, #19992, #20411, #39338, #58698, #46478, #46062, #65866, #72174, #639, #77661, #26295, #45643, #71755, #1887, #53204, #7360, #39761, #1063, #33456, #26717, #14531, #15776, #9033, #73000, #22485, #9858, #34706, #54037, #60368, #23304, #3958, #21650, #79750, #74673, #9441, #61616, #80991, #2716, #35528, #28376, #79330, #60778, #47310, #29621, #22067, #48148, #15352, #67110, #34286, #2303, #59947, #10279, #47727, #68356, #55281, #28794, #54878, #27963, #35112, #53622, #73844, #16184, #41831, #48974, #73425, #67938, #41426, #3545, #54457, #67521, #80585, #35946, #41014, #80170, #17018, #3129, #61190, #42658, #66699, #29212, #22891, #48559, #74257, #16598, #42243, #77456, #30446, #17430, #6738, #7160, #51753, #43885, #75905, #45443, #71139, #32831, #62855, #32409, #56111, #17837, #82223, #69168, #81401, #26520, #24127, #19791, #39138, #13070, #49388, #45859, #13481, #24543, #43472, #18244, #64819, #50207, #38725, #43061, #5191, #69583, #10695, #64402, #58072, #11101, #36350, #68758, #81817, #58499, #863, #52175, #55693, #49796, #11519, #75083, #62026, #4362, #77878, #36758, #30030, #20209, #30856, #438, #23717, #37175, #62434, #26093, #4771, #75498, #56521, #20632, #66496, #46283, #27768, #46704, #34086, #79141, #8830, #26932, #72397, #53841, #71979, #1691, #60170, #71557, #53007, #59749, #27349, #14333, #13906, #78720, #34507, #65681, #78300, #21458, #79554, #2525, #2103, #53433, #28183, #21867, #47532, #14747, #47116, #8008, #21045, #66082, #40401, #1283, #73223, #59334, #15574, #39564, #72805, #39991, #65253, #7590, #15154, #8418, #40811, #33262, #58924, #52593, #33672, #36466, #37298, #68873, #17952, #11221, #5710, #48680, #12043, #37701, #31380, #62141, #36061, #56235, #29737, #30969, #63374, #18363, #82739, #42772, #75614, #57045, #81932, #49916, #23840, #4480, #4896, #74376, #82337, #16719, #10404, #68058, #4070, #55812, #50323, #23424, #43176, #42360, #10806, #36881, #30150, #49507, #43589, #62559, #30569, #24243, #61733, #69290, #5311, #69700, #81519, #44006, #56636, #68468, #75200, #17544, #11638, #62972, #55400, #81107, #49089, #24655, #76021, #74790, #17140, #13288, #44404, #38940, #76833, #33048, #6543, #83152, #63785, #64621, #657, #25472, #44815, #51139, #14128, #78097, #12450, #70512, #65475, #239, #52388, #71774, #19167, #26313, #12869, #70098, #51551, #38111, #20428, #38527, #6958, #6124, #57872, #25059, #76432, #50733, #1082, #64209, #59136, #46081, #19584, #45660, #18761, #25891, #31797, #32629, #58292, #51972, #39781, #32213, #58718, #77254, #77679, #45244, #20009, #71356, #26734, #57459, #70943, #7808, #13703, #39358, #33474, #65043, #7380, #34726, #34305 ) ),
 .UNSPECIFIED., .F., .F., .F. ) 
 B_SPLINE_SURFACE_WITH_KNOTS ( ( 2, 2 ),
 ( 3, 2, 2, 2, 2, 2, 2, 2, 2, 2, 2, 2, 2, 2, 2, 2, 2, 2, 2, 2, 2, 2, 2, 2, 2, 2, 2, 2, 2, 2, 2, 2, 2, 2, 2, 2, 2, 2, 2, 2, 2, 2, 2, 2, 2, 2, 2, 2, 2, 2, 2, 2, 2, 2, 2, 2, 2, 2, 2, 2, 2, 2, 2, 2, 2, 2, 2, 2, 2, 2, 2, 2, 2, 2, 2, 2, 2, 2, 2, 2, 2, 2, 2, 2, 2, 2, 2, 2, 2, 2, 2, 2, 2, 2, 2, 2, 2, 2, 2, 2, 2, 2, 2, 2, 2, 2, 2, 2, 2, 2, 2, 2, 2, 2, 2, 2, 2, 2, 2, 2, 2, 2, 2, 2, 2, 2, 2, 2, 2, 2, 2, 2, 2, 2, 2, 2, 2, 2, 2, 2, 2, 2, 2, 2, 2, 2, 2, 2, 2, 2, 2, 2, 2, 2, 2, 2, 2, 2, 2, 2, 2, 2, 2, 2, 2, 2, 2, 2, 2, 2, 2, 2, 2, 2, 2, 2, 2, 2, 2, 2, 2, 2, 2, 2, 2, 2, 2, 2, 2, 2, 2, 2, 2, 2, 2, 2, 2, 2, 2, 2, 2, 2, 2, 2, 2, 2, 2, 2, 2, 2, 2, 2, 2, 2, 2, 2, 2, 2, 2, 2, 2, 2, 2, 2, 2, 2, 2, 2, 2, 2, 2, 2, 2, 2, 2, 2, 2, 2, 2, 2, 2, 2, 2, 2, 2, 2, 2, 2, 2, 2, 2, 2, 2, 2, 2, 3 ),
 ( 0.000000000000000000, 1.000000000000000000 ),
 ( 0.000000000000000000, 0.003787878787878787984, 0.007575757575757575968, 0.01136363636363636395, 0.01515151515151515194, 0.01893939393939393992, 0.02272727272727272790, 0.02651515151515151589, 0.03030303030303030387, 0.03409090909090908839, 0.03787878787878787984, 0.04166666666666666435, 0.04545454545454545581, 0.04924242424242424032, 0.05303030303030303177, 0.05681818181818181629, 0.06060606060606060774, 0.06439393939393939226, 0.06818181818181817677, 0.07196969696969697516, 0.07575757575757575968, 0.07954545454545454419, 0.08333333333333332871, 0.08712121212121212710, 0.09090909090909091161, 0.09469696969696969613, 0.09848484848484848064, 0.1022727272727272790, 0.1060606060606060635, 0.1098484848484848481, 0.1136363636363636326, 0.1174242424242424310, 0.1212121212121212155, 0.1250000000000000000, 0.1287878787878787845, 0.1325757575757575690, 0.1363636363636363535, 0.1401515151515151381, 0.1439393939393939503, 0.1477272727272727348, 0.1515151515151515194, 0.1553030303030303039, 0.1590909090909090884, 0.1628787878787878729, 0.1666666666666666574, 0.1704545454545454419, 0.1742424242424242542, 0.1780303030303030387, 0.1818181818181818232, 0.1856060606060606077, 0.1893939393939393923, 0.1931818181818181768, 0.1969696969696969613, 0.2007575757575757458, 0.2045454545454545581, 0.2083333333333333426, 0.2121212121212121271, 0.2159090909090909116, 0.2196969696969696961, 0.2234848484848484806, 0.2272727272727272652, 0.2310606060606060497, 0.2348484848484848619, 0.2386363636363636465, 0.2424242424242424310, 0.2462121212121212155, 0.2500000000000000000, 0.2537878787878787845, 0.2575757575757575690, 0.2613636363636363535, 0.2651515151515151381, 0.2689393939393939226, 0.2727272727272727071, 0.2765151515151514916, 0.2803030303030302761, 0.2840909090909091161, 0.2878787878787879007, 0.2916666666666666852, 0.2954545454545454697, 0.2992424242424242542, 0.3030303030303030387, 0.3068181818181818232, 0.3106060606060606077, 0.3143939393939393923, 0.3181818181818181768, 0.3219696969696969613, 0.3257575757575757458, 0.3295454545454545303, 0.3333333333333333148, 0.3371212121212120993, 0.3409090909090908839, 0.3446969696969697239, 0.3484848484848485084, 0.3522727272727272929, 0.3560606060606060774, 0.3598484848484848619, 0.3636363636363636465, 0.3674242424242424310, 0.3712121212121212155, 0.3750000000000000000, 0.3787878787878787845, 0.3825757575757575690, 0.3863636363636363535, 0.3901515151515151381, 0.3939393939393939226, 0.3977272727272727071, 0.4015151515151514916, 0.4053030303030302761, 0.4090909090909091161, 0.4128787878787879007, 0.4166666666666666852, 0.4204545454545454697, 0.4242424242424242542, 0.4280303030303030387, 0.4318181818181818232, 0.4356060606060606077, 0.4393939393939393923, 0.4431818181818181768, 0.4469696969696969613, 0.4507575757575757458, 0.4545454545454545303, 0.4583333333333333148, 0.4621212121212120993, 0.4659090909090908839, 0.4696969696969697239, 0.4734848484848485084, 0.4772727272727272929, 0.4810606060606060774, 0.4848484848484848619, 0.4886363636363636465, 0.4924242424242424310, 0.4962121212121212155, 0.5000000000000000000, 0.5037878787878787845, 0.5075757575757575690, 0.5113636363636363535, 0.5151515151515151381, 0.5189393939393939226, 0.5227272727272727071, 0.5265151515151514916, 0.5303030303030302761, 0.5340909090909090606, 0.5378787878787878451, 0.5416666666666666297, 0.5454545454545454142, 0.5492424242424241987, 0.5530303030303029832, 0.5568181818181817677, 0.5606060606060605522, 0.5643939393939394478, 0.5681818181818182323, 0.5719696969696970168, 0.5757575757575758013, 0.5795454545454545858, 0.5833333333333333703, 0.5871212121212121549, 0.5909090909090909394, 0.5946969696969697239, 0.5984848484848485084, 0.6022727272727272929, 0.6060606060606060774, 0.6098484848484848619, 0.6136363636363636465, 0.6174242424242424310, 0.6212121212121212155, 0.6250000000000000000, 0.6287878787878787845, 0.6325757575757575690, 0.6363636363636363535, 0.6401515151515151381, 0.6439393939393939226, 0.6477272727272727071, 0.6515151515151514916, 0.6553030303030302761, 0.6590909090909090606, 0.6628787878787878451, 0.6666666666666666297, 0.6704545454545454142, 0.6742424242424241987, 0.6780303030303029832, 0.6818181818181817677, 0.6856060606060605522, 0.6893939393939394478, 0.6931818181818182323, 0.6969696969696970168, 0.7007575757575758013, 0.7045454545454545858, 0.7083333333333333703, 0.7121212121212121549, 0.7159090909090909394, 0.7196969696969697239, 0.7234848484848485084, 0.7272727272727272929, 0.7310606060606060774, 0.7348484848484848619, 0.7386363636363636465, 0.7424242424242424310, 0.7462121212121212155, 0.7500000000000000000, 0.7537878787878787845, 0.7575757575757575690, 0.7613636363636363535, 0.7651515151515151381, 0.7689393939393939226, 0.7727272727272727071, 0.7765151515151514916, 0.7803030303030302761, 0.7840909090909090606, 0.7878787878787878451, 0.7916666666666666297, 0.7954545454545454142, 0.7992424242424241987, 0.8030303030303029832, 0.8068181818181817677, 0.8106060606060605522, 0.8143939393939394478, 0.8181818181818182323, 0.8219696969696970168, 0.8257575757575758013, 0.8295454545454545858, 0.8333333333333333703, 0.8371212121212121549, 0.8409090909090909394, 0.8446969696969697239, 0.8484848484848485084, 0.8522727272727272929, 0.8560606060606060774, 0.8598484848484848619, 0.8636363636363636465, 0.8674242424242424310, 0.8712121212121212155, 0.8750000000000000000, 0.8787878787878787845, 0.8825757575757575690, 0.8863636363636363535, 0.8901515151515151381, 0.8939393939393939226, 0.8977272727272727071, 0.9015151515151514916, 0.9053030303030302761, 0.9090909090909090606, 0.9128787878787878451, 0.9166666666666666297, 0.9204545454545454142, 0.9242424242424241987, 0.9280303030303029832, 0.9318181818181817677, 0.9356060606060605522, 0.9393939393939394478, 0.9431818181818182323, 0.9469696969696970168, 0.9507575757575758013, 0.9545454545454545858, 0.9583333333333333703, 0.9621212121212121549, 0.9659090909090909394 ),
 .UNSPECIFIED. ) 
 GEOMETRIC_REPRESENTATION_ITEM ( )  RATIONAL_B_SPLINE_SURFACE ( (
 ( 1.000000000000000000, 0.9659258262890683122, 1.000000000000000000, 0.9659258262890683122, 1.000000000000000000, 0.9659258262890683122, 1.000000000000000000, 0.9659258262890683122, 1.000000000000000000, 0.9659258262890683122, 1.000000000000000000, 0.9659258262890683122, 1.000000000000000000, 0.9659258262890683122, 1.000000000000000000, 0.9659258262890683122, 1.000000000000000000, 0.9659258262890683122, 1.000000000000000000, 0.9659258262890683122, 1.000000000000000000, 0.9659258262890683122, 1.000000000000000000, 0.9659258262890683122, 1.000000000000000000, 0.9659258262890683122, 1.000000000000000000, 0.9659258262890683122, 1.000000000000000000, 0.9659258262890683122, 1.000000000000000000, 0.9659258262890683122, 1.000000000000000000, 0.9659258262890683122, 1.000000000000000000, 0.9659258262890683122, 1.000000000000000000, 0.9659258262890683122, 1.000000000000000000, 0.9659258262890683122, 1.000000000000000000, 0.9659258262890683122, 1.000000000000000000, 0.9659258262890683122, 1.000000000000000000, 0.9659258262890683122, 1.000000000000000000, 0.9659258262890683122, 1.000000000000000000, 0.9659258262890683122, 1.000000000000000000, 0.9659258262890683122, 1.000000000000000000, 0.9659258262890683122, 1.000000000000000000, 0.9659258262890683122, 1.000000000000000000, 0.9659258262890683122, 1.000000000000000000, 0.9659258262890683122, 1.000000000000000000, 0.9659258262890683122, 1.000000000000000000, 0.9659258262890683122, 1.000000000000000000, 0.9659258262890683122, 1.000000000000000000, 0.9659258262890683122, 1.000000000000000000, 0.9659258262890683122, 1.000000000000000000, 0.9659258262890683122, 1.000000000000000000, 0.9659258262890683122, 1.000000000000000000, 0.9659258262890683122, 1.000000000000000000, 0.9659258262890683122, 1.000000000000000000, 0.9659258262890683122, 1.000000000000000000, 0.9659258262890683122, 1.000000000000000000, 0.9659258262890683122, 1.000000000000000000, 0.9659258262890683122, 1.000000000000000000, 0.9659258262890683122, 1.000000000000000000, 0.9659258262890683122, 1.000000000000000000, 0.9659258262890683122, 1.000000000000000000, 0.9659258262890683122, 1.000000000000000000, 0.9659258262890683122, 1.000000000000000000, 0.9659258262890683122, 1.000000000000000000, 0.9659258262890683122, 1.000000000000000000, 0.9659258262890683122, 1.000000000000000000, 0.9659258262890683122, 1.000000000000000000, 0.9659258262890683122, 1.000000000000000000, 0.9659258262890683122, 1.000000000000000000, 0.9659258262890683122, 1.000000000000000000, 0.9659258262890683122, 1.000000000000000000, 0.9659258262890683122, 1.000000000000000000, 0.9659258262890683122, 1.000000000000000000, 0.9659258262890683122, 1.000000000000000000, 0.9659258262890683122, 1.000000000000000000, 0.9659258262890683122, 1.000000000000000000, 0.9659258262890683122, 1.000000000000000000, 0.9659258262890683122, 1.000000000000000000, 0.9659258262890683122, 1.000000000000000000, 0.9659258262890683122, 1.000000000000000000, 0.9659258262890683122, 1.000000000000000000, 0.9659258262890683122, 1.000000000000000000, 0.9659258262890683122, 1.000000000000000000, 0.9659258262890683122, 1.000000000000000000, 0.9659258262890683122, 1.000000000000000000, 0.9659258262890683122, 1.000000000000000000, 0.9659258262890683122, 1.000000000000000000, 0.9659258262890683122, 1.000000000000000000, 0.9659258262890683122, 1.000000000000000000, 0.9659258262890683122, 1.000000000000000000, 0.9659258262890683122, 1.000000000000000000, 0.9659258262890683122, 1.000000000000000000, 0.9659258262890683122, 1.000000000000000000, 0.9659258262890683122, 1.000000000000000000, 0.9659258262890683122, 1.000000000000000000, 0.9659258262890683122, 1.000000000000000000, 0.9659258262890683122, 1.000000000000000000, 0.9659258262890683122, 1.000000000000000000, 0.9659258262890683122, 1.000000000000000000, 0.9659258262890683122, 1.000000000000000000, 0.9659258262890683122, 1.000000000000000000, 0.9659258262890683122, 1.000000000000000000, 0.9659258262890683122, 1.000000000000000000, 0.9659258262890683122, 1.000000000000000000, 0.9659258262890683122, 1.000000000000000000, 0.9659258262890683122, 1.000000000000000000, 0.9659258262890683122, 1.000000000000000000, 0.9659258262890683122, 1.000000000000000000, 0.9659258262890683122, 1.000000000000000000, 0.9659258262890683122, 1.000000000000000000, 0.9659258262890683122, 1.000000000000000000, 0.9659258262890683122, 1.000000000000000000, 0.9659258262890683122, 1.000000000000000000, 0.9659258262890683122, 1.000000000000000000, 0.9659258262890683122, 1.000000000000000000, 0.9659258262890683122, 1.000000000000000000, 0.9659258262890683122, 1.000000000000000000, 0.9659258262890683122, 1.000000000000000000, 0.9659258262890683122, 1.000000000000000000, 0.9659258262890683122, 1.000000000000000000, 0.9659258262890683122, 1.000000000000000000, 0.9659258262890683122, 1.000000000000000000, 0.9659258262890683122, 1.000000000000000000, 0.9659258262890683122, 1.000000000000000000, 0.9659258262890683122, 1.000000000000000000, 0.9659258262890683122, 1.000000000000000000, 0.9659258262890683122, 1.000000000000000000, 0.9659258262890683122, 1.000000000000000000, 0.9659258262890683122, 1.000000000000000000, 0.9659258262890683122, 1.000000000000000000, 0.9659258262890683122, 1.000000000000000000, 0.9659258262890683122, 1.000000000000000000, 0.9659258262890683122, 1.000000000000000000, 0.9659258262890683122, 1.000000000000000000, 0.9659258262890683122, 1.000000000000000000, 0.9659258262890683122, 1.000000000000000000, 0.9659258262890683122, 1.000000000000000000, 0.9659258262890683122, 1.000000000000000000, 0.9659258262890683122, 1.000000000000000000, 0.9659258262890683122, 1.000000000000000000, 0.9659258262890683122, 1.000000000000000000, 0.9659258262890683122, 1.000000000000000000, 0.9659258262890683122, 1.000000000000000000, 0.9659258262890683122, 1.000000000000000000, 0.9659258262890683122, 1.000000000000000000, 0.9659258262890683122, 1.000000000000000000, 0.9659258262890683122, 1.000000000000000000, 0.9659258262890683122, 1.000000000000000000, 0.9659258262890683122, 1.000000000000000000, 0.9659258262890683122, 1.000000000000000000, 0.9659258262890683122, 1.000000000000000000, 0.9659258262890683122, 1.000000000000000000, 0.9659258262890683122, 1.000000000000000000, 0.9659258262890683122, 1.000000000000000000, 0.9659258262890683122, 1.000000000000000000, 0.9659258262890683122, 1.000000000000000000, 0.9659258262890683122, 1.000000000000000000, 0.9659258262890683122, 1.000000000000000000, 0.9659258262890683122, 1.000000000000000000, 0.9659258262890683122, 1.000000000000000000, 0.9659258262890683122, 1.000000000000000000, 0.9659258262890683122, 1.000000000000000000, 0.9659258262890683122, 1.000000000000000000, 0.9659258262890683122, 1.000000000000000000, 0.9659258262890683122, 1.000000000000000000, 0.9659258262890683122, 1.000000000000000000, 0.9659258262890683122, 1.000000000000000000, 0.9659258262890683122, 1.000000000000000000, 0.9659258262890683122, 1.000000000000000000, 0.9659258262890683122, 1.000000000000000000, 0.9659258262890683122, 1.000000000000000000, 0.9659258262890683122, 1.000000000000000000, 0.9659258262890683122, 1.000000000000000000, 0.9659258262890683122, 1.000000000000000000, 0.9659258262890683122, 1.000000000000000000, 0.9659258262890683122, 1.000000000000000000, 0.9659258262890683122, 1.000000000000000000, 0.9659258262890683122, 1.000000000000000000, 0.9659258262890683122, 1.000000000000000000, 0.9659258262890683122, 1.000000000000000000, 0.9659258262890683122, 1.000000000000000000, 0.9659258262890683122, 1.000000000000000000, 0.9659258262890683122, 1.000000000000000000, 0.9659258262890683122, 1.000000000000000000, 0.9659258262890683122, 1.000000000000000000, 0.9659258262890683122, 1.000000000000000000, 0.9659258262890683122, 1.000000000000000000, 0.9659258262890683122, 1.000000000000000000, 0.9659258262890683122, 1.000000000000000000, 0.9659258262890683122, 1.000000000000000000, 0.9659258262890683122, 1.000000000000000000, 0.9659258262890683122, 1.000000000000000000, 0.9659258262890683122, 1.000000000000000000, 0.9659258262890683122, 1.000000000000000000, 0.9659258262890683122, 1.000000000000000000, 0.9659258262890683122, 1.000000000000000000, 0.9659258262890683122, 1.000000000000000000, 0.9659258262890683122, 1.000000000000000000, 0.9659258262890683122, 1.000000000000000000, 0.9659258262890683122, 1.000000000000000000, 0.9659258262890683122, 1.000000000000000000, 0.9659258262890683122, 1.000000000000000000, 0.9659258262890683122, 1.000000000000000000, 0.9659258262890683122, 1.000000000000000000, 0.9659258262890683122, 1.000000000000000000, 0.9659258262890683122, 1.000000000000000000, 0.9659258262890683122, 1.000000000000000000, 0.9659258262890683122, 1.000000000000000000, 0.9659258262890683122, 1.000000000000000000, 0.9659258262890683122, 1.000000000000000000, 0.9659258262890683122, 1.000000000000000000, 0.9659258262890683122, 1.000000000000000000, 0.9659258262890683122, 1.000000000000000000, 0.9659258262890683122, 1.000000000000000000, 0.9659258262890683122, 1.000000000000000000, 0.9659258262890683122, 1.000000000000000000, 0.9659258262890683122, 1.000000000000000000, 0.9659258262890683122, 1.000000000000000000, 0.9659258262890683122, 1.000000000000000000, 0.9659258262890683122, 1.000000000000000000, 0.9659258262890683122, 1.000000000000000000, 0.9659258262890683122, 1.000000000000000000, 0.9659258262890683122, 1.000000000000000000, 0.9659258262890683122, 1.000000000000000000, 0.9659258262890683122, 1.000000000000000000, 0.9659258262890683122, 1.000000000000000000, 0.9659258262890683122, 1.000000000000000000, 0.9659258262890683122, 1.000000000000000000, 0.9659258262890683122, 1.000000000000000000, 0.9659258262890683122, 1.000000000000000000, 0.9659258262890683122, 1.000000000000000000, 0.9659258262890683122, 1.000000000000000000, 0.9659258262890683122, 1.000000000000000000, 0.9659258262890683122, 1.000000000000000000, 0.9659258262890683122, 1.000000000000000000, 0.9659258262890683122, 1.000000000000000000, 0.9659258262890683122, 1.000000000000000000, 0.9659258262890683122, 1.000000000000000000, 0.9659258262890683122, 1.000000000000000000, 0.9659258262890683122, 1.000000000000000000, 0.9659258262890683122, 1.000000000000000000, 0.9659258262890683122, 1.000000000000000000, 0.9659258262890683122, 1.000000000000000000, 0.9659258262890683122, 1.000000000000000000, 0.9659258262890683122, 1.000000000000000000, 0.9659258262890683122, 1.000000000000000000, 0.9659258262890683122, 1.000000000000000000, 0.9659258262890683122, 1.000000000000000000, 0.9659258262890683122, 1.000000000000000000, 0.9659258262890683122, 1.000000000000000000, 0.9659258262890683122, 1.000000000000000000, 0.9659258262890683122, 1.000000000000000000, 0.9659258262890683122, 1.000000000000000000, 0.9659258262890683122, 1.000000000000000000, 0.9659258262890683122, 1.000000000000000000, 0.9659258262890683122, 1.000000000000000000, 0.9659258262890683122, 1.000000000000000000, 0.9659258262890683122, 1.000000000000000000, 0.9659258262890683122, 1.000000000000000000, 0.9659258262890683122, 1.000000000000000000, 0.9659258262890683122, 1.000000000000000000, 0.9659258262890683122, 1.000000000000000000, 0.9659258262890683122, 1.000000000000000000, 0.9659258262890683122, 1.000000000000000000, 0.9659258262890683122, 1.000000000000000000, 0.9659258262890683122, 1.000000000000000000, 0.9659258262890683122, 1.000000000000000000, 0.9659258262890683122, 1.000000000000000000, 0.9659258262890683122, 1.000000000000000000, 0.9659258262890683122, 1.000000000000000000),
 ( 1.000000000000000000, 0.9659258262890683122, 1.000000000000000000, 0.9659258262890683122, 1.000000000000000000, 0.9659258262890683122, 1.000000000000000000, 0.9659258262890683122, 1.000000000000000000, 0.9659258262890683122, 1.000000000000000000, 0.9659258262890683122, 1.000000000000000000, 0.9659258262890683122, 1.000000000000000000, 0.9659258262890683122, 1.000000000000000000, 0.9659258262890683122, 1.000000000000000000, 0.9659258262890683122, 1.000000000000000000, 0.9659258262890683122, 1.000000000000000000, 0.9659258262890683122, 1.000000000000000000, 0.9659258262890683122, 1.000000000000000000, 0.9659258262890683122, 1.000000000000000000, 0.9659258262890683122, 1.000000000000000000, 0.9659258262890683122, 1.000000000000000000, 0.9659258262890683122, 1.000000000000000000, 0.9659258262890683122, 1.000000000000000000, 0.9659258262890683122, 1.000000000000000000, 0.9659258262890683122, 1.000000000000000000, 0.9659258262890683122, 1.000000000000000000, 0.9659258262890683122, 1.000000000000000000, 0.9659258262890683122, 1.000000000000000000, 0.9659258262890683122, 1.000000000000000000, 0.9659258262890683122, 1.000000000000000000, 0.9659258262890683122, 1.000000000000000000, 0.9659258262890683122, 1.000000000000000000, 0.9659258262890683122, 1.000000000000000000, 0.9659258262890683122, 1.000000000000000000, 0.9659258262890683122, 1.000000000000000000, 0.9659258262890683122, 1.000000000000000000, 0.9659258262890683122, 1.000000000000000000, 0.9659258262890683122, 1.000000000000000000, 0.9659258262890683122, 1.000000000000000000, 0.9659258262890683122, 1.000000000000000000, 0.9659258262890683122, 1.000000000000000000, 0.9659258262890683122, 1.000000000000000000, 0.9659258262890683122, 1.000000000000000000, 0.9659258262890683122, 1.000000000000000000, 0.9659258262890683122, 1.000000000000000000, 0.9659258262890683122, 1.000000000000000000, 0.9659258262890683122, 1.000000000000000000, 0.9659258262890683122, 1.000000000000000000, 0.9659258262890683122, 1.000000000000000000, 0.9659258262890683122, 1.000000000000000000, 0.9659258262890683122, 1.000000000000000000, 0.9659258262890683122, 1.000000000000000000, 0.9659258262890683122, 1.000000000000000000, 0.9659258262890683122, 1.000000000000000000, 0.9659258262890683122, 1.000000000000000000, 0.9659258262890683122, 1.000000000000000000, 0.9659258262890683122, 1.000000000000000000, 0.9659258262890683122, 1.000000000000000000, 0.9659258262890683122, 1.000000000000000000, 0.9659258262890683122, 1.000000000000000000, 0.9659258262890683122, 1.000000000000000000, 0.9659258262890683122, 1.000000000000000000, 0.9659258262890683122, 1.000000000000000000, 0.9659258262890683122, 1.000000000000000000, 0.9659258262890683122, 1.000000000000000000, 0.9659258262890683122, 1.000000000000000000, 0.9659258262890683122, 1.000000000000000000, 0.9659258262890683122, 1.000000000000000000, 0.9659258262890683122, 1.000000000000000000, 0.9659258262890683122, 1.000000000000000000, 0.9659258262890683122, 1.000000000000000000, 0.9659258262890683122, 1.000000000000000000, 0.9659258262890683122, 1.000000000000000000, 0.9659258262890683122, 1.000000000000000000, 0.9659258262890683122, 1.000000000000000000, 0.9659258262890683122, 1.000000000000000000, 0.9659258262890683122, 1.000000000000000000, 0.9659258262890683122, 1.000000000000000000, 0.9659258262890683122, 1.000000000000000000, 0.9659258262890683122, 1.000000000000000000, 0.9659258262890683122, 1.000000000000000000, 0.9659258262890683122, 1.000000000000000000, 0.9659258262890683122, 1.000000000000000000, 0.9659258262890683122, 1.000000000000000000, 0.9659258262890683122, 1.000000000000000000, 0.9659258262890683122, 1.000000000000000000, 0.9659258262890683122, 1.000000000000000000, 0.9659258262890683122, 1.000000000000000000, 0.9659258262890683122, 1.000000000000000000, 0.9659258262890683122, 1.000000000000000000, 0.9659258262890683122, 1.000000000000000000, 0.9659258262890683122, 1.000000000000000000, 0.9659258262890683122, 1.000000000000000000, 0.9659258262890683122, 1.000000000000000000, 0.9659258262890683122, 1.000000000000000000, 0.9659258262890683122, 1.000000000000000000, 0.9659258262890683122, 1.000000000000000000, 0.9659258262890683122, 1.000000000000000000, 0.9659258262890683122, 1.000000000000000000, 0.9659258262890683122, 1.000000000000000000, 0.9659258262890683122, 1.000000000000000000, 0.9659258262890683122, 1.000000000000000000, 0.9659258262890683122, 1.000000000000000000, 0.9659258262890683122, 1.000000000000000000, 0.9659258262890683122, 1.000000000000000000, 0.9659258262890683122, 1.000000000000000000, 0.9659258262890683122, 1.000000000000000000, 0.9659258262890683122, 1.000000000000000000, 0.9659258262890683122, 1.000000000000000000, 0.9659258262890683122, 1.000000000000000000, 0.9659258262890683122, 1.000000000000000000, 0.9659258262890683122, 1.000000000000000000, 0.9659258262890683122, 1.000000000000000000, 0.9659258262890683122, 1.000000000000000000, 0.9659258262890683122, 1.000000000000000000, 0.9659258262890683122, 1.000000000000000000, 0.9659258262890683122, 1.000000000000000000, 0.9659258262890683122, 1.000000000000000000, 0.9659258262890683122, 1.000000000000000000, 0.9659258262890683122, 1.000000000000000000, 0.9659258262890683122, 1.000000000000000000, 0.9659258262890683122, 1.000000000000000000, 0.9659258262890683122, 1.000000000000000000, 0.9659258262890683122, 1.000000000000000000, 0.9659258262890683122, 1.000000000000000000, 0.9659258262890683122, 1.000000000000000000, 0.9659258262890683122, 1.000000000000000000, 0.9659258262890683122, 1.000000000000000000, 0.9659258262890683122, 1.000000000000000000, 0.9659258262890683122, 1.000000000000000000, 0.9659258262890683122, 1.000000000000000000, 0.9659258262890683122, 1.000000000000000000, 0.9659258262890683122, 1.000000000000000000, 0.9659258262890683122, 1.000000000000000000, 0.9659258262890683122, 1.000000000000000000, 0.9659258262890683122, 1.000000000000000000, 0.9659258262890683122, 1.000000000000000000, 0.9659258262890683122, 1.000000000000000000, 0.9659258262890683122, 1.000000000000000000, 0.9659258262890683122, 1.000000000000000000, 0.9659258262890683122, 1.000000000000000000, 0.9659258262890683122, 1.000000000000000000, 0.9659258262890683122, 1.000000000000000000, 0.9659258262890683122, 1.000000000000000000, 0.9659258262890683122, 1.000000000000000000, 0.9659258262890683122, 1.000000000000000000, 0.9659258262890683122, 1.000000000000000000, 0.9659258262890683122, 1.000000000000000000, 0.9659258262890683122, 1.000000000000000000, 0.9659258262890683122, 1.000000000000000000, 0.9659258262890683122, 1.000000000000000000, 0.9659258262890683122, 1.000000000000000000, 0.9659258262890683122, 1.000000000000000000, 0.9659258262890683122, 1.000000000000000000, 0.9659258262890683122, 1.000000000000000000, 0.9659258262890683122, 1.000000000000000000, 0.9659258262890683122, 1.000000000000000000, 0.9659258262890683122, 1.000000000000000000, 0.9659258262890683122, 1.000000000000000000, 0.9659258262890683122, 1.000000000000000000, 0.9659258262890683122, 1.000000000000000000, 0.9659258262890683122, 1.000000000000000000, 0.9659258262890683122, 1.000000000000000000, 0.9659258262890683122, 1.000000000000000000, 0.9659258262890683122, 1.000000000000000000, 0.9659258262890683122, 1.000000000000000000, 0.9659258262890683122, 1.000000000000000000, 0.9659258262890683122, 1.000000000000000000, 0.9659258262890683122, 1.000000000000000000, 0.9659258262890683122, 1.000000000000000000, 0.9659258262890683122, 1.000000000000000000, 0.9659258262890683122, 1.000000000000000000, 0.9659258262890683122, 1.000000000000000000, 0.9659258262890683122, 1.000000000000000000, 0.9659258262890683122, 1.000000000000000000, 0.9659258262890683122, 1.000000000000000000, 0.9659258262890683122, 1.000000000000000000, 0.9659258262890683122, 1.000000000000000000, 0.9659258262890683122, 1.000000000000000000, 0.9659258262890683122, 1.000000000000000000, 0.9659258262890683122, 1.000000000000000000, 0.9659258262890683122, 1.000000000000000000, 0.9659258262890683122, 1.000000000000000000, 0.9659258262890683122, 1.000000000000000000, 0.9659258262890683122, 1.000000000000000000, 0.9659258262890683122, 1.000000000000000000, 0.9659258262890683122, 1.000000000000000000, 0.9659258262890683122, 1.000000000000000000, 0.9659258262890683122, 1.000000000000000000, 0.9659258262890683122, 1.000000000000000000, 0.9659258262890683122, 1.000000000000000000, 0.9659258262890683122, 1.000000000000000000, 0.9659258262890683122, 1.000000000000000000, 0.9659258262890683122, 1.000000000000000000, 0.9659258262890683122, 1.000000000000000000, 0.9659258262890683122, 1.000000000000000000, 0.9659258262890683122, 1.000000000000000000, 0.9659258262890683122, 1.000000000000000000, 0.9659258262890683122, 1.000000000000000000, 0.9659258262890683122, 1.000000000000000000, 0.9659258262890683122, 1.000000000000000000, 0.9659258262890683122, 1.000000000000000000, 0.9659258262890683122, 1.000000000000000000, 0.9659258262890683122, 1.000000000000000000, 0.9659258262890683122, 1.000000000000000000, 0.9659258262890683122, 1.000000000000000000, 0.9659258262890683122, 1.000000000000000000, 0.9659258262890683122, 1.000000000000000000, 0.9659258262890683122, 1.000000000000000000, 0.9659258262890683122, 1.000000000000000000, 0.9659258262890683122, 1.000000000000000000, 0.9659258262890683122, 1.000000000000000000, 0.9659258262890683122, 1.000000000000000000, 0.9659258262890683122, 1.000000000000000000, 0.9659258262890683122, 1.000000000000000000, 0.9659258262890683122, 1.000000000000000000, 0.9659258262890683122, 1.000000000000000000, 0.9659258262890683122, 1.000000000000000000, 0.9659258262890683122, 1.000000000000000000, 0.9659258262890683122, 1.000000000000000000, 0.9659258262890683122, 1.000000000000000000, 0.9659258262890683122, 1.000000000000000000, 0.9659258262890683122, 1.000000000000000000, 0.9659258262890683122, 1.000000000000000000, 0.9659258262890683122, 1.000000000000000000, 0.9659258262890683122, 1.000000000000000000, 0.9659258262890683122, 1.000000000000000000, 0.9659258262890683122, 1.000000000000000000, 0.9659258262890683122, 1.000000000000000000, 0.9659258262890683122, 1.000000000000000000, 0.9659258262890683122, 1.000000000000000000, 0.9659258262890683122, 1.000000000000000000, 0.9659258262890683122, 1.000000000000000000, 0.9659258262890683122, 1.000000000000000000, 0.9659258262890683122, 1.000000000000000000, 0.9659258262890683122, 1.000000000000000000, 0.9659258262890683122, 1.000000000000000000, 0.9659258262890683122, 1.000000000000000000, 0.9659258262890683122, 1.000000000000000000, 0.9659258262890683122, 1.000000000000000000, 0.9659258262890683122, 1.000000000000000000, 0.9659258262890683122, 1.000000000000000000, 0.9659258262890683122, 1.000000000000000000, 0.9659258262890683122, 1.000000000000000000, 0.9659258262890683122, 1.000000000000000000, 0.9659258262890683122, 1.000000000000000000, 0.9659258262890683122, 1.000000000000000000, 0.9659258262890683122, 1.000000000000000000, 0.9659258262890683122, 1.000000000000000000, 0.9659258262890683122, 1.000000000000000000, 0.9659258262890683122, 1.000000000000000000, 0.9659258262890683122, 1.000000000000000000, 0.9659258262890683122, 1.000000000000000000, 0.9659258262890683122, 1.000000000000000000, 0.9659258262890683122, 1.000000000000000000, 0.9659258262890683122, 1.000000000000000000, 0.9659258262890683122, 1.000000000000000000, 0.9659258262890683122, 1.000000000000000000, 0.9659258262890683122, 1.000000000000000000, 0.9659258262890683122, 1.000000000000000000) ) ) 
 REPRESENTATION_ITEM ( '' )  SURFACE ( )  );
#11322=CARTESIAN_POINT ( 'NONE',  ( -0.2821522309711278487, -0.5511811023622048555, -0.09757992244046775898 ) ) ;
#11324=CARTESIAN_POINT ( 'NONE',  ( 0.7414698162729663755, 0.2952755905511811885, 0.1292274648535926551 ) ) ;
#11326=CARTESIAN_POINT ( 'NONE',  ( 1.213910761154856299, -0.5511811023622048555, -0.09757992244046775898 ) ) ;
#11327=CARTESIAN_POINT ( 'NONE',  ( -1.069553805774277722, 0.2952755905511811885, 0.1292274648535926551 ) ) ;
#11328=CARTESIAN_POINT ( 'NONE',  ( -0.3543307086614165824, 0.1771653543307087630, 0.000000000000000000 ) ) ;
#11330=CARTESIAN_POINT ( 'NONE',  ( 0.03280839895013198948, 0.1771653543307087630, 0.09757992244046791164 ) ) ;
#11331=CARTESIAN_POINT ( 'NONE',  ( -0.4265091863517051496, -0.6692913385826771977, 0.1292274648535927661 ) ) ;
#11335=CARTESIAN_POINT ( 'NONE',  ( 0.8005249343832027131, -0.004921259842519576551, 0.3153832671262227771 ) ) ;
#11336=CARTESIAN_POINT ( 'NONE',  ( -0.3871391076115476282, -0.05778040916215522460, 0.4822834645669289988 ) ) ;
#11337=CARTESIAN_POINT ( 'NONE',  ( -0.6299212598425188991, -0.1870078740157480879, -0.4822834645669291653 ) ) ;
#11338=CARTESIAN_POINT ( 'NONE',  ( -0.6233595800524928121, -0.2845877964562161244, -0.3641732283464567121 ) ) ;
#11340=CARTESIAN_POINT ( 'NONE',  ( 0.06561679790026316017, -0.4281496062992124485, 0.4176697321401328655 ) ) ;
#11342=CARTESIAN_POINT ( 'NONE',  ( -1.161417322834644716, -0.4536011799217368745, -0.2665933059059886201 ) ) ;
#11343=CARTESIAN_POINT ( 'NONE',  ( -1.469816272965878357, 0.2306618581243848609, 0.2411417322834645549 ) ) ;
#11344=CARTESIAN_POINT ( 'NONE',  ( 2.795275590551181466, 1.968503937007874960, 0.000000000000000000 ) ) ;
#11346=VERTEX_POINT ( 'NONE', #64607 ) ;
#11348=CARTESIAN_POINT ( 'NONE',  ( -1.397637795275589623, 0.07958543189024085140, 0.2665933059059887866 ) ) ;
#11349=CARTESIAN_POINT ( 'NONE',  ( -1.561679790026246017, 0.05413385826771666132, 0.4176697321401328100 ) ) ;
#11350=CARTESIAN_POINT ( 'NONE',  ( -0.9448818897637790704, -0.1870078740157479769, 0.4822834645669291653 ) ) ;
#11351=CARTESIAN_POINT ( 'NONE',  ( -1.627296587926508442, 0.2306618581243848609, 0.2411417322834645549 ) ) ;
#11354=CARTESIAN_POINT ( 'NONE',  ( 0.9973753280839902091, -0.6046776061558807314, 0.2411417322834647770 ) ) ;
#11355=CARTESIAN_POINT ( 'NONE',  ( 0.3477690288713918276, -0.6692913385826773087, -0.1292274648535924053 ) ) ;
#11358=CARTESIAN_POINT ( 'NONE',  ( 1.338582677165355062, -0.1870078740157480601, -0.3641732283464567677 ) ) ;
#11361=CARTESIAN_POINT ( 'NONE',  ( -1.043307086614172041, -0.4536011799217367080, 0.2665933059059888421 ) ) ;
#11365=CARTESIAN_POINT ( 'NONE',  ( 0.2690288713910767848, -0.6692913385826773087, -0.1292274648535924053 ) ) ;
#11366=CARTESIAN_POINT ( 'NONE',  ( -0.4199475065616791736, 0.2306618581243847221, -0.2411417322834647770 ) ) ;
#11367=CARTESIAN_POINT ( 'NONE',  ( -1.272965879265091305, 0.05413385826771626580, -0.4176697321401330321 ) ) ;
#11368=CARTESIAN_POINT ( 'NONE',  ( 0.9186351706036752773, 0.2306618581243847221, -0.2411417322834647770 ) ) ;
#11369=CARTESIAN_POINT ( 'NONE',  ( 1.640419947506562393, -0.4281496062992124485, 0.4176697321401328655 ) ) ;
#11371=CARTESIAN_POINT ( 'NONE',  ( 0.02624671916010564918, -0.6046776061558809534, -0.2411417322834644161 ) ) ;
#11372=CARTESIAN_POINT ( 'NONE',  ( -1.141732283464566011, 0.2952755905511811885, 0.000000000000000000 ) ) ;
#11373=CARTESIAN_POINT ( 'NONE',  ( -1.614173228346455824, 0.2952755905511811885, 0.000000000000000000 ) ) ;
#11376=CARTESIAN_POINT ( 'NONE',  ( 0.6758530183727039509, -0.5511811023622046335, 0.09757992244046803654 ) ) ;
#11377=VERTEX_POINT ( 'NONE', #56624 ) ;
#11379=CARTESIAN_POINT ( 'NONE',  ( -0.7939632545931750718, -0.05778040916215560624, -0.4822834645669293319 ) ) ;
#11380=VERTEX_POINT ( 'NONE', #18350 ) ;
#11381=CARTESIAN_POINT ( 'NONE',  ( -0.03937007874015669567, -0.5511811023622047445, 6.969142054262312111E-17 ) ) ;
#11383=CARTESIAN_POINT ( 'NONE',  ( 0.6430446194225728496, 0.05413385826771666132, 0.4176697321401328100 ) ) ;
#11384=CARTESIAN_POINT ( 'NONE',  ( 0.3937007874015754361, -0.1870078740157480879, -0.4822834645669291653 ) ) ;
#11385=CARTESIAN_POINT ( 'NONE',  ( -0.4199475065616791736, 0.2306618581243847221, -0.2411417322834647770 ) ) ;
#11387=CARTESIAN_POINT ( 'NONE',  ( -1.371391076115484609, -0.6692913385826771977, 0.1292274648535927661 ) ) ;
#11389=CARTESIAN_POINT ( 'NONE',  ( 1.489501312335958172, -0.08942795157528024563, -0.3641732283464568787 ) ) ;
#11390=CARTESIAN_POINT ( 'NONE',  ( -1.213910761154854745, -0.6692913385826771977, 0.1292274648535927661 ) ) ;
#11391=CARTESIAN_POINT ( 'NONE',  ( 0.7020997375328090762, -0.3162353388693405765, 0.4822834645669290543 ) ) ;
#11392=CARTESIAN_POINT ( 'NONE',  ( 1.102362204724410155, -0.1870078740157480879, -0.4822834645669291653 ) ) ;
#11394=CARTESIAN_POINT ( 'NONE',  ( -1.351706036745406347, 0.05413385826771626580, -0.4176697321401330321 ) ) ;
#11396=CARTESIAN_POINT ( 'NONE',  ( 0.1377952755905518800, -0.5400638737290844871, 0.3530559997133364547 ) ) ;
#11399=CARTESIAN_POINT ( 'NONE',  ( -1.469816272965878357, 0.1283753931104748280, 0.1820866141732283561 ) ) ;
#11400=CARTESIAN_POINT ( 'NONE',  ( 0.6102362204724416372, 0.07958543189024071263, -0.2665933059059888421 ) ) ;
#11401=CARTESIAN_POINT ( 'NONE',  ( 1.069553805774278610, -0.6692913385826771977, 0.1292274648535927661 ) ) ;
#11403=CARTESIAN_POINT ( 'NONE',  ( 0.7611548556430454138, 0.1283753931104746893, -0.1820866141732285504 ) ) ;
#11404=CARTESIAN_POINT ( 'NONE',  ( 0.2887139107611556010, -0.6046776061558807314, 0.2411417322834647770 ) ) ;
#11407=CARTESIAN_POINT ( 'NONE',  ( -0.7808398950131225646, -0.05778040916215522460, 0.4822834645669289988 ) ) ;
#11408=CARTESIAN_POINT ( 'NONE',  ( -0.2034120734908128059, 0.2952755905511811885, 0.1292274648535926551 ) ) ;
#11410=CARTESIAN_POINT ( 'NONE',  ( 1.062992125984252745, -0.5511811023622047445, 6.969142054262312111E-17 ) ) ;
#11411=CARTESIAN_POINT ( 'NONE',  ( -0.1246719160104980823, 0.2952755905511811885, 0.1292274648535926551 ) ) ;
#11413=CARTESIAN_POINT ( 'NONE',  ( -0.3018372703412066094, 0.05413385826771666132, 0.4176697321401328100 ) ) ;
#11414=CARTESIAN_POINT ( 'NONE',  ( -0.07217847769028787330, -0.08942795157527998196, 0.3641732283464567121 ) ) ;
#11416=CARTESIAN_POINT ( 'NONE',  ( -0.3740157480314953431, -0.5400638737290845981, -0.3530559997133363437 ) ) ;
#11417=CARTESIAN_POINT ( 'NONE',  ( 0.8858267716535438430, -0.4536011799217368745, -0.2665933059059886201 ) ) ;
#11420=CARTESIAN_POINT ( 'NONE',  ( 0.4790026246719168435, -0.3162353388693409650, -0.4822834645669289433 ) ) ;
#11422=CARTESIAN_POINT ( 'NONE',  ( 1.299212598425197429, -0.5511811023622047445, 6.969142054262312111E-17 ) ) ;
#11423=CARTESIAN_POINT ( 'NONE',  ( 0.3826031302655975019, 1.809133623825372073E-16, -0.3954985857520062487 ) ) ;
#11424=CARTESIAN_POINT ( 'NONE',  ( -0.4330708661417315697, 0.1771653543307087630, 0.000000000000000000 ) ) ;
#11426=CARTESIAN_POINT ( 'NONE',  ( -0.9186351706036736120, 0.1283753931104748280, 0.1820866141732283561 ) ) ;
#11427=CARTESIAN_POINT ( 'NONE',  ( -0.2165354330708654795, 0.1660481256975885056, 0.3530559997133364547 ) ) ;
#11428=CARTESIAN_POINT ( 'NONE',  ( 0.5183727034120741983, 0.2952755905511810774, -0.1292274648535930714 ) ) ;
#11429=CARTESIAN_POINT ( 'NONE',  ( 1.010498687664042716, -0.3690944881889763329, 0.3153832671262228327 ) ) ;
#11431=CARTESIAN_POINT ( 'NONE',  ( -1.719160104986876103, 0.05413385826771666132, 0.4176697321401328100 ) ) ;
#11432=CARTESIAN_POINT ( 'NONE',  ( 0.8923884514435703741, 0.2306618581243848609, 0.2411417322834645549 ) ) ;
#11434=CARTESIAN_POINT ( 'NONE',  ( 0.2362204724409456558, -0.1870078740157480879, -0.4822834645669291653 ) ) ;
#11436=CARTESIAN_POINT ( 'NONE',  ( 0.8070866141732289112, -0.5400638737290845981, -0.3530559997133363437 ) ) ;
#11437=CARTESIAN_POINT ( 'NONE',  ( 0.6955380577427828781, -0.4281496062992124485, 0.4176697321401328655 ) ) ;
#11439=CARTESIAN_POINT ( 'NONE',  ( 0.5380577427821529035, -0.3690944881889763329, 0.3153832671262228327 ) ) ;
#11440=CARTESIAN_POINT ( 'NONE',  ( 1.299212598425197429, -0.6692913385826771977, 8.415575281601705876E-17 ) ) ;
#11441=CARTESIAN_POINT ( 'NONE',  ( -0.07874015748031421014, -0.1870078740157480601, -0.3641732283464567677 ) ) ;
#11442=CARTESIAN_POINT ( 'NONE',  ( -0.1706036745406816491, 0.05413385826771626580, -0.4176697321401330321 ) ) ;
#11443=CARTESIAN_POINT ( 'NONE',  ( 0.2887139107611556010, -0.6046776061558807314, 0.2411417322834647770 ) ) ;
#11444=CARTESIAN_POINT ( 'NONE',  ( -0.7874015748031489847, -0.1870078740157480879, -0.4822834645669291653 ) ) ;
#11445=CARTESIAN_POINT ( 'NONE',  ( -0.4724409448818890911, -0.1870078740157479769, 0.3641732283464567677 ) ) ;
#11446=CARTESIAN_POINT ( 'NONE',  ( 0.3215223097112867578, -0.05778040916215522460, 0.4822834645669289988 ) ) ;
#11447=CARTESIAN_POINT ( 'NONE',  ( 0.9842519685039378130, -0.5511811023622047445, 6.969142054262312111E-17 ) ) ;
#11448=CARTESIAN_POINT ( 'NONE',  ( 0.08530183727034192087, -0.05778040916215522460, 0.4822834645669289988 ) ) ;
#11449=CARTESIAN_POINT ( 'NONE',  ( 1.122047244094488860, 0.1012011053420777407, 0.2882089793578257453 ) ) ;
#11450=CARTESIAN_POINT ( 'NONE',  ( -0.6155095129759579065, 1.955395699586848224, 0.5046436704918912941 ) ) ;
#11452=CARTESIAN_POINT ( 'NONE',  ( 1.555118110236221041, 0.1660481256975883668, -0.3530559997133364547 ) ) ;
#11454=CARTESIAN_POINT ( 'NONE',  ( -1.181102362204723644, -0.1870078740157479769, 0.4822834645669291653 ) ) ;
#11455=CARTESIAN_POINT ( 'NONE',  ( -0.8661417322834640276, -0.1870078740157480879, -0.4822834645669291653 ) ) ;
#11459=CARTESIAN_POINT ( 'NONE',  ( 0.4527559055118117182, 0.07958543189024071263, -0.2665933059059888421 ) ) ;
#11461=CARTESIAN_POINT ( 'NONE',  ( 0.4790026246719167324, -0.05778040916215522460, 0.4822834645669289988 ) ) ;
#11464=CARTESIAN_POINT ( 'NONE',  ( -0.3033747635708576307, 0.02791078216816064370, 0.4328096321851915285 ) ) ;
#11465=CARTESIAN_POINT ( 'NONE',  ( 1.246719160104987623, 0.05413385826771626580, -0.4176697321401330321 ) ) ;
#11466=EDGE_CURVE ( 'NONE', #54098, #80968, #19914, .T. ) ;
#11467=CARTESIAN_POINT ( 'NONE',  ( 1.148293963254593653, 0.1771653543307087075, -0.09757992244046823083 ) ) ;
#11468=CARTESIAN_POINT ( 'NONE',  ( 0.2099737532808405305, -0.6046776061558807314, 0.2411417322834647770 ) ) ;
#11470=CARTESIAN_POINT ( 'NONE',  ( -0.4199475065616791736, -0.6046776061558807314, 0.2411417322834647770 ) ) ;
#11471=CARTESIAN_POINT ( 'NONE',  ( -1.489501312335957062, -0.2845877964562161244, -0.3641732283464567121 ) ) ;
#11472=CARTESIAN_POINT ( 'NONE',  ( 0.2362204724409456558, -0.1870078740157480879, -0.4822834645669291653 ) ) ;
#11473=CARTESIAN_POINT ( 'NONE',  ( -0.4921259842519677963, -0.5400638737290844871, 0.3530559997133364547 ) ) ;
#11475=CARTESIAN_POINT ( 'NONE',  ( 1.627296587926509996, -0.6046776061558807314, 0.2411417322834647770 ) ) ;
#11479=CARTESIAN_POINT ( 'NONE',  ( 0.2427821522309719648, -0.05778040916215522460, 0.4822834645669289988 ) ) ;
#11481=CARTESIAN_POINT ( 'NONE',  ( -0.5249343832020990641, -0.6046776061558809534, -0.2411417322834644161 ) ) ;
#11482=CARTESIAN_POINT ( 'NONE',  ( -1.640419947506561060, 0.05413385826771666132, 0.4176697321401328100 ) ) ;
#11484=CARTESIAN_POINT ( 'NONE',  ( 0.7283464566929140904, -0.5400638737290845981, -0.3530559997133363437 ) ) ;
#11485=CARTESIAN_POINT ( 'NONE',  ( 0.2887139107611556010, 0.2306618581243847221, -0.2411417322834647770 ) ) ;
#11487=CARTESIAN_POINT ( 'NONE',  ( -0.9711286089238838626, -0.6046776061558807314, 0.2411417322834647770 ) ) ;
#11488=CARTESIAN_POINT ( 'NONE',  ( 0.06561679790026316017, -0.4281496062992124485, 0.4176697321401328655 ) ) ;
#11489=CARTESIAN_POINT ( 'NONE',  ( -0.4724409448818890911, -0.1870078740157480879, -0.4822834645669291653 ) ) ;
#11490=CARTESIAN_POINT ( 'NONE',  ( 0.3018372703412079971, -0.004921259842519870586, -0.3153832671262229437 ) ) ;
#11491=CARTESIAN_POINT ( 'NONE',  ( -1.607611548556429737, -0.6692913385826771977, 0.1292274648535927661 ) ) ;
#11493=CARTESIAN_POINT ( 'NONE',  ( 5.463695987328526437E-16, -0.1870078740157479769, 0.4822834645669291653 ) ) ;
#11494=CARTESIAN_POINT ( 'NONE',  ( 0.4935044252197983150, 1.488513638086841118, -0.5309055118110237448 ) ) ;
#11495=CARTESIAN_POINT ( 'NONE',  ( 1.456692913385827515, 0.2952755905511811885, 0.000000000000000000 ) ) ;
#11497=ORIENTED_EDGE ( 'NONE', *, *, #50269, .F. ) ;
#11498=ADVANCED_FACE ( 'NONE', ( #33033 ), #65362, .F. ) ;
#11499=VERTEX_POINT ( 'NONE', #60370 ) ;
#11500=CARTESIAN_POINT ( 'NONE',  ( 0.7611548556430454138, 0.2306618581243847221, -0.2411417322834647770 ) ) ;
#11501=CARTESIAN_POINT ( 'NONE',  ( 0.1509186351706042484, -0.2845877964562159024, 0.3641732283464567677 ) ) ;
#11502=CARTESIAN_POINT ( 'NONE',  ( 1.692913385826772421, 0.1771653543307087630, 0.000000000000000000 ) ) ;
#11503=CARTESIAN_POINT ( 'NONE',  ( 1.306827173596999403, 0.000000000000000000, -0.4445507791589060620 ) ) ;
#11508=CARTESIAN_POINT ( 'NONE',  ( 0.3018372703412079971, -0.4281496062992124485, 0.4176697321401328655 ) ) ;
#11509=CARTESIAN_POINT ( 'NONE',  ( -1.122047244094487306, 0.1660481256975883668, -0.3530559997133364547 ) ) ;
#11510=CARTESIAN_POINT ( 'NONE',  ( -1.076115485564303809, 0.2306618581243848609, 0.2411417322834645549 ) ) ;
#11511=CARTESIAN_POINT ( 'NONE',  ( 0.3805774278215230400, 0.05413385826771626580, -0.4176697321401330321 ) ) ;
#11512=CARTESIAN_POINT ( 'NONE',  ( 1.122047244094488860, 0.1660481256975885056, 0.3530559997133364547 ) ) ;
#11513=CARTESIAN_POINT ( 'NONE',  ( 1.535433070866142558, 0.1771653543307087630, 0.000000000000000000 ) ) ;
#11514=CARTESIAN_POINT ( 'NONE',  ( 1.437007874015748810, -0.4536011799217368745, -0.2665933059059886201 ) ) ;
#11515=CARTESIAN_POINT ( 'NONE',  ( -1.017060367454067249, -0.05778040916215522460, 0.4822834645669289988 ) ) ;
#11517=CARTESIAN_POINT ( 'NONE',  ( 1.601049868766404982, -0.6046776061558809534, -0.2411417322834644161 ) ) ;
#11519=CARTESIAN_POINT ( 'NONE',  ( -0.3412073490813641308, 0.2306618581243847221, -0.2411417322834647770 ) ) ;
#11520=CARTESIAN_POINT ( 'NONE',  ( 1.076115485564305141, 0.2306618581243847221, -0.2411417322834647770 ) ) ;
#11522=CARTESIAN_POINT ( 'NONE',  ( -1.607611548556429737, -0.5511811023622046335, 0.09757992244046803654 ) ) ;
#11523=CARTESIAN_POINT ( 'NONE',  ( 0.5446194225721792126, -0.3162353388693405765, 0.4822834645669290543 ) ) ;
#11524=CARTESIAN_POINT ( 'NONE',  ( 0.9776902887139113929, 0.1771653543307087630, 0.09757992244046791164 ) ) ;
#11525=CARTESIAN_POINT ( 'NONE',  ( -1.581364829396324945, -0.2845877964562159024, 0.3641732283464567677 ) ) ;
#11526=CARTESIAN_POINT ( 'NONE',  ( 0.7480314960629927956, 0.2952755905511811885, 0.000000000000000000 ) ) ;
#11528=CARTESIAN_POINT ( 'NONE',  ( -0.6364829396325453192, -0.2845877964562159024, 0.3641732283464567677 ) ) ;
#11529=CARTESIAN_POINT ( 'NONE',  ( -0.7020997375328076329, -0.3162353388693409650, -0.4822834645669289433 ) ) ;
#11530=CARTESIAN_POINT ( 'NONE',  ( 1.456692913385827515, -0.6692913385826771977, 8.415575281601705876E-17 ) ) ;
#11531=CARTESIAN_POINT ( 'NONE',  ( -0.7086614173228339419, -0.1870078740157480879, -0.4822834645669291653 ) ) ;
#11532=CARTESIAN_POINT ( 'NONE',  ( 1.528871391076116026, 0.2952755905511811885, 0.1292274648535926551 ) ) ;
#11534=CARTESIAN_POINT ( 'NONE',  ( -0.9448818897637790704, -0.1870078740157480601, -0.3641732283464567677 ) ) ;
#11536=CARTESIAN_POINT ( 'NONE',  ( 1.528871391076116026, -0.6692913385826773087, -0.1292274648535924053 ) ) ;
#11539=CARTESIAN_POINT ( 'NONE',  ( -0.09067318884954536640, -4.069555009745408348E-17, -0.3627989612356148363 ) ) ;
#11540=CARTESIAN_POINT ( 'NONE',  ( 1.646981627296588035, -0.3162353388693405765, 0.4822834645669290543 ) ) ;
#11541=CARTESIAN_POINT ( 'NONE',  ( -1.200787401574802349, 0.07958543189024071263, -0.2665933059059888421 ) ) ;
#11542=DIRECTION ( 'NONE',  ( 1.000000000000000000, -0.000000000000000000, -0.000000000000000000 ) ) ;
#11543=CARTESIAN_POINT ( 'NONE',  ( -0.2230971128608915943, 0.05413385826771666132, 0.4176697321401328100 ) ) ;
#11544=CARTESIAN_POINT ( 'NONE',  ( 0.1181102362204730916, 0.1771653543307087630, 0.000000000000000000 ) ) ;
#11545=CARTESIAN_POINT ( 'NONE',  ( -1.135170603674539924, -0.5511811023622046335, 0.09757992244046803654 ) ) ;
#11546=CARTESIAN_POINT ( 'NONE',  ( 1.305774278215223960, 0.1771653543307087075, -0.09757992244046823083 ) ) ;
#11547=CARTESIAN_POINT ( 'NONE',  ( 0.8398950131233602345, -0.6046776061558807314, 0.2411417322834647770 ) ) ;
#11548=CARTESIAN_POINT ( 'NONE',  ( 1.607611548556431069, 0.2952755905511811885, 0.1292274648535926551 ) ) ;
#11549=CARTESIAN_POINT ( 'NONE',  ( 0.4002624671916016896, -0.08942795157527998196, 0.3641732283464567121 ) ) ;
#11551=CARTESIAN_POINT ( 'NONE',  ( 0.4068241469816281097, 0.05413385826771666132, 0.4176697321401328100 ) ) ;
#11552=CARTESIAN_POINT ( 'NONE',  ( 0.8070866141732288002, 0.07958543189024085140, 0.2665933059059887866 ) ) ;
#11554=CARTESIAN_POINT ( 'NONE',  ( -1.338582677165353729, -0.1870078740157479769, 0.4822834645669291653 ) ) ;
#11556=CARTESIAN_POINT ( 'NONE',  ( -1.167979002624671470, 0.05413385826771666132, 0.4176697321401328100 ) ) ;
#11557=CARTESIAN_POINT ( 'NONE',  ( 0.03937007874015806264, 0.2952755905511811885, 0.000000000000000000 ) ) ;
#11560=CARTESIAN_POINT ( 'NONE',  ( 0.6036745406824153282, -0.6046776061558807314, 0.2411417322834647770 ) ) ;
#11561=CARTESIAN_POINT ( 'NONE',  ( 1.358267716535433323, -0.4536011799217368745, -0.2665933059059886201 ) ) ;
#11562=CARTESIAN_POINT ( 'NONE',  ( 0.03937007874015833325, -0.6692913385826771977, 8.415575281601705876E-17 ) ) ;
#11563=CARTESIAN_POINT ( 'NONE',  ( 0.3740157480314966754, 0.1660481256975883668, -0.3530559997133364547 ) ) ;
#11569=CARTESIAN_POINT ( 'NONE',  ( -0.5052493438320203589, -0.5511811023622046335, 0.09757992244046803654 ) ) ;
#11570=CARTESIAN_POINT ( 'NONE',  ( -0.6627296587926503335, -0.6692913385826771977, 0.1292274648535927661 ) ) ;
#11571=CARTESIAN_POINT ( 'NONE',  ( 0.5971128608923890191, -0.6692913385826771977, 0.1292274648535927661 ) ) ;
#11573=CARTESIAN_POINT ( 'NONE',  ( 0.7217847769028878924, 0.05413385826771666132, 0.4176697321401328100 ) ) ;
#11574=CARTESIAN_POINT ( 'NONE',  ( -1.568241469816272105, -0.3162353388693409650, -0.4822834645669289433 ) ) ;
#11575=CARTESIAN_POINT ( 'NONE',  ( 0.6824146981627303710, 0.2306618581243847221, -0.2411417322834647770 ) ) ;
#11579=CARTESIAN_POINT ( 'NONE',  ( 1.555118110236221041, 0.1660481256975883668, -0.3530559997133364547 ) ) ;
#11581=CARTESIAN_POINT ( 'NONE',  ( 1.062992125984252745, -0.6692913385826771977, 8.415575281601705876E-17 ) ) ;
#11582=CARTESIAN_POINT ( 'NONE',  ( 0.5380577427821529035, 0.05413385826771626580, -0.4176697321401330321 ) ) ;
#11583=CARTESIAN_POINT ( 'NONE',  ( 1.240157480314961314, -0.4536011799217367080, 0.2665933059059888421 ) ) ;
#11584=CARTESIAN_POINT ( 'NONE',  ( -1.423884514435694859, -0.08942795157528024563, -0.3641732283464568787 ) ) ;
#11585=CARTESIAN_POINT ( 'NONE',  ( -1.614173228346455824, 0.2952755905511811885, 0.000000000000000000 ) ) ;
#11587=CYLINDRICAL_SURFACE ( 'NONE', #13077, 1.181102362204724310 ) ;
#11588=CARTESIAN_POINT ( 'NONE',  ( 0.7939632545931766261, -0.3162353388693409650, -0.4822834645669289433 ) ) ;
#11589=FACE_OUTER_BOUND ( 'NONE', #50870, .T. ) ;
#11590=CARTESIAN_POINT ( 'NONE',  ( -0.3346456692913377662, -0.5400638737290844871, 0.3530559997133364547 ) ) ;
#11591=CARTESIAN_POINT ( 'NONE',  ( -0.9776902887139098386, -0.6692913385826771977, 0.1292274648535927661 ) ) ;
#11592=CARTESIAN_POINT ( 'NONE',  ( 1.023622047244095112, -0.1870078740157480879, -0.4822834645669291653 ) ) ;
#11596=CARTESIAN_POINT ( 'NONE',  ( 1.548556430446194954, 0.2306618581243847221, -0.2411417322834647770 ) ) ;
#11602=CARTESIAN_POINT ( 'NONE',  ( 1.450131233595801428, 0.1771653543307087630, 0.09757992244046791164 ) ) ;
#11604=CARTESIAN_POINT ( 'NONE',  ( 1.614173228346457378, -0.5511811023622047445, 6.969142054262312111E-17 ) ) ;
#11609=CARTESIAN_POINT ( 'NONE',  ( -0.9120734908136475250, -0.5511811023622048555, -0.09757992244046775898 ) ) ;
#11610=CARTESIAN_POINT ( 'NONE',  ( -1.266404199475064773, -0.2845877964562159024, 0.3641732283464567677 ) ) ;
#11611=CARTESIAN_POINT ( 'NONE',  ( -1.089238845144356427, -0.4281496062992127816, -0.4176697321401328100 ) ) ;
#11612=CARTESIAN_POINT ( 'NONE',  ( 0.3083989501312343062, -0.3162353388693405765, 0.4822834645669290543 ) ) ;
#11613=CARTESIAN_POINT ( 'NONE',  ( -1.404199475065615932, -0.4281496062992127816, -0.4176697321401328100 ) ) ;
#11614=VERTEX_POINT ( 'NONE', #54039 ) ;
#11615=CARTESIAN_POINT ( 'NONE',  ( 1.469816272965879911, 0.2306618581243847221, -0.2411417322834647770 ) ) ;
#11618=CARTESIAN_POINT ( 'NONE',  ( -0.6299212598425188991, -0.1870078740157480601, -0.3641732283464567677 ) ) ;
#11619=CARTESIAN_POINT ( 'NONE',  ( -1.122047244094487306, 0.1660481256975883668, -0.3530559997133364547 ) ) ;
#11620=CARTESIAN_POINT ( 'NONE',  ( 0.9448818897637802916, -0.1870078740157480879, -0.4822834645669291653 ) ) ;
#11626=CARTESIAN_POINT ( 'NONE',  ( -1.069553805774277722, 0.2952755905511811885, 0.1292274648535926551 ) ) ;
#11628=CARTESIAN_POINT ( 'NONE',  ( 0.1837270341207354329, 0.1283753931104748280, 0.1820866141732283561 ) ) ;
#11631=CARTESIAN_POINT ( 'NONE',  ( 0.05905511811023709395, -0.4536011799217367080, 0.2665933059059888421 ) ) ;
#11632=CARTESIAN_POINT ( 'NONE',  ( 0.5183727034120741983, 0.1771653543307087075, -0.09757992244046823083 ) ) ;
#11633=CARTESIAN_POINT ( 'NONE',  ( 0.5446194225721792126, -0.05778040916215560624, -0.4822834645669293319 ) ) ;
#11634=CARTESIAN_POINT ( 'NONE',  ( -0.8202099737532799750, 0.1771653543307087075, -0.09757992244046823083 ) ) ;
#11636=CARTESIAN_POINT ( 'NONE',  ( 1.062992125984252745, -0.6692913385826771977, 8.415575281601705876E-17 ) ) ;
#11638=CARTESIAN_POINT ( 'NONE',  ( -1.167979002624671470, 0.05413385826771666132, 0.4176697321401328100 ) ) ;
#11641=AXIS2_PLACEMENT_3D ( 'NONE', #61675, #4016, #29270 ) ;
#11642=CARTESIAN_POINT ( 'NONE',  ( 0.02624671916010564918, 0.2306618581243848609, 0.2411417322834645549 ) ) ;
#11643=CARTESIAN_POINT ( 'NONE',  ( -0.4265091863517051496, -0.6692913385826771977, 0.1292274648535927661 ) ) ;
#11644=CARTESIAN_POINT ( 'NONE',  ( 1.391076115485564868, 0.1283753931104746893, -0.1820866141732285504 ) ) ;
#11645=CARTESIAN_POINT ( 'NONE',  ( 0.2427821522309716595, -0.2845877964562161244, -0.3641732283464567121 ) ) ;
#11646=CARTESIAN_POINT ( 'NONE',  ( -0.1509186351706028884, -0.05778040916215522460, 0.4822834645669289988 ) ) ;
#11647=CARTESIAN_POINT ( 'NONE',  ( -1.161417322834644716, 0.1660481256975885056, 0.3530559997133364547 ) ) ;
#11650=CARTESIAN_POINT ( 'NONE',  ( -0.2099737532808391705, 0.2306618581243848609, 0.2411417322834645549 ) ) ;
#11651=CARTESIAN_POINT ( 'NONE',  ( -1.194225721784776262, 0.05413385826771626580, -0.4176697321401330321 ) ) ;
#11652=ORIENTED_EDGE ( 'NONE', *, *, #66673, .F. ) ;
#11654=CARTESIAN_POINT ( 'NONE',  ( 1.154855643044620184, 0.2306618581243847221, -0.2411417322834647770 ) ) ;
#11655=CARTESIAN_POINT ( 'NONE',  ( -0.6627296587926503335, -0.5511811023622046335, 0.09757992244046803654 ) ) ;
#11657=CARTESIAN_POINT ( 'NONE',  ( -0.6496062992125976043, -0.5400638737290844871, 0.3530559997133364547 ) ) ;
#11658=CARTESIAN_POINT ( 'NONE',  ( 1.227034120734908917, 0.2952755905511810774, -0.1292274648535930714 ) ) ;
#11659=CARTESIAN_POINT ( 'NONE',  ( 0.8989501312335964611, 0.2952755905511811885, 0.1292274648535926551 ) ) ;
#11661=CARTESIAN_POINT ( 'NONE',  ( -1.233595800524933894, 0.1283753931104748280, 0.1820866141732283561 ) ) ;
#11664=ADVANCED_FACE ( 'NONE', ( #65869 ), #34465, .F. ) ;
#11667=CARTESIAN_POINT ( 'NONE',  ( 1.181102362204725198, -0.1870078740157479769, 0.3641732283464567677 ) ) ;
#11668=CARTESIAN_POINT ( 'NONE',  ( 0.6036745406824153282, -0.5023911411419708095, 0.1820866141732285504 ) ) ;
#11669=CARTESIAN_POINT ( 'NONE',  ( 0.6758530183727039509, 0.2952755905511810774, -0.1292274648535930714 ) ) ;
#11672=CARTESIAN_POINT ( 'NONE',  ( 0.8398950131233602345, -0.5023911411419708095, 0.1820866141732285504 ) ) ;
#11673=CARTESIAN_POINT ( 'NONE',  ( -0.3149606299212590610, -0.1870078740157480879, -0.4822834645669291653 ) ) ;
#11674=CARTESIAN_POINT ( 'NONE',  ( -1.423884514435694859, -0.05778040916215560624, -0.4822834645669293319 ) ) ;
#11675=CARTESIAN_POINT ( 'NONE',  ( 1.076115485564305141, 0.2306618581243847221, -0.2411417322834647770 ) ) ;
#11678=CARTESIAN_POINT ( 'NONE',  ( -0.1771653543307080136, -0.4536011799217367080, 0.2665933059059888421 ) ) ;
#11680=ORIENTED_EDGE ( 'NONE', *, *, #16612, .F. ) ;
#11682=CARTESIAN_POINT ( 'NONE',  ( -0.9186351706036736120, 0.2306618581243848609, 0.2411417322834645549 ) ) ;
#11683=CARTESIAN_POINT ( 'NONE',  ( -0.6167979002624665030, -0.4281496062992127816, -0.4176697321401328100 ) ) ;
#11684=CARTESIAN_POINT ( 'NONE',  ( -0.4133858267716528645, -0.5400638737290844871, 0.3530559997133364547 ) ) ;
#11685=CARTESIAN_POINT ( 'NONE',  ( 0.2887139107611556010, 0.2306618581243847221, -0.2411417322834647770 ) ) ;
#11686=CARTESIAN_POINT ( 'NONE',  ( -0.5839895013123351797, -0.6692913385826771977, 0.1292274648535927661 ) ) ;
#11687=CARTESIAN_POINT ( 'NONE',  ( -1.509186351706035767, -0.4281496062992124485, 0.4176697321401328655 ) ) ;
#11688=CARTESIAN_POINT ( 'NONE',  ( -0.9711286089238838626, -0.6046776061558807314, 0.2411417322834647770 ) ) ;
#11689=CARTESIAN_POINT ( 'NONE',  ( 0.5511811023622054106, -0.1870078740157480879, -0.4822834645669291653 ) ) ;
#11692=CARTESIAN_POINT ( 'NONE',  ( -0.3412073490813641308, 0.1283753931104746893, -0.1820866141732285504 ) ) ;
#11693=ORIENTED_EDGE ( 'NONE', *, *, #70646, .F. ) ;
#11695=AXIS2_PLACEMENT_3D ( 'NONE', #73945, #54559, #17122 ) ;
#11697=CARTESIAN_POINT ( 'NONE',  ( -1.161417322834644716, -0.4536011799217368745, -0.2665933059059886201 ) ) ;
#11699=VECTOR ( 'NONE', #52150, 39.37007874015748854 ) ;
#11700=CARTESIAN_POINT ( 'NONE',  ( -0.9383202099737524282, -0.3162353388693409650, -0.4822834645669289433 ) ) ;
#11701=CARTESIAN_POINT ( 'NONE',  ( -1.023622047244093558, -0.1870078740157479769, 0.4822834645669291653 ) ) ;
#11703=CARTESIAN_POINT ( 'NONE',  ( -0.7874015748031489847, -0.1870078740157479769, 0.4822834645669291653 ) ) ;
#11704=CARTESIAN_POINT ( 'NONE',  ( -0.6955380577427815458, -0.4281496062992127816, -0.4176697321401328100 ) ) ;
#11705=CARTESIAN_POINT ( 'NONE',  ( -1.548556430446193399, -0.6046776061558809534, -0.2411417322834644161 ) ) ;
#11707=CARTESIAN_POINT ( 'NONE',  ( 0.4986876640419954376, -0.5023911411419708095, -0.1820866141732282451 ) ) ;
#11708=DIRECTION ( 'NONE',  ( -3.096699300667737957E-16, 1.000000000000000000, -0.000000000000000000 ) ) ;
#11710=CARTESIAN_POINT ( 'NONE',  ( 0.07874015748031558404, -0.1870078740157480601, -0.3641732283464567677 ) ) ;
#11711=CARTESIAN_POINT ( 'NONE',  ( -0.2427821522309703550, -0.3162353388693405765, 0.4822834645669290543 ) ) ;
#11712=CARTESIAN_POINT ( 'NONE',  ( 1.332020997375328974, -0.05778040916215560624, -0.4822834645669293319 ) ) ;
#11713=CARTESIAN_POINT ( 'NONE',  ( -0.05905511811023545637, 0.1660481256975885056, 0.3530559997133364547 ) ) ;
#11719=LINE ( 'NONE', #5384, #3256 ) ;
#11720=CARTESIAN_POINT ( 'NONE',  ( -1.240157480314959759, 0.07958543189024085140, 0.2665933059059887866 ) ) ;
#11721=CARTESIAN_POINT ( 'NONE',  ( -1.555118110236219930, 0.1660481256975885056, 0.3530559997133364547 ) ) ;
#11725=CARTESIAN_POINT ( 'NONE',  ( 1.332020997375329197, -0.3162353388693405765, 0.4822834645669290543 ) ) ;
#11726=CARTESIAN_POINT ( 'NONE',  ( 0.5577427821522314977, -0.3162353388693409650, -0.4822834645669289433 ) ) ;
#11727=CARTESIAN_POINT ( 'NONE',  ( -0.1115485564304453947, -0.6692913385826771977, 0.1292274648535927661 ) ) ;
#11728=CARTESIAN_POINT ( 'NONE',  ( -0.8792650918635160906, -0.3690944881889763329, 0.3153832671262228327 ) ) ;
#11729=CARTESIAN_POINT ( 'NONE',  ( -0.1574803149606292529, -0.1870078740157479769, 0.4822834645669291653 ) ) ;
#11731=CARTESIAN_POINT ( 'NONE',  ( -1.003937007874015297, -0.5400638737290845981, -0.3530559997133363437 ) ) ;
#11734=CARTESIAN_POINT ( 'NONE',  ( 1.351706036745407458, -0.3690944881889765550, -0.3153832671262227771 ) ) ;
#11735=CARTESIAN_POINT ( 'NONE',  ( -0.2034120734908131112, -0.5511811023622048555, -0.09757992244046775898 ) ) ;
#11736=CARTESIAN_POINT ( 'NONE',  ( 1.167979002624672580, -0.3690944881889763329, 0.3153832671262228327 ) ) ;
#11737=CARTESIAN_POINT ( 'NONE',  ( -1.384514435695537005, 0.2952755905511811885, 0.1292274648535926551 ) ) ;
#11738=CARTESIAN_POINT ( 'NONE',  ( -0.9645669291338575535, 0.07958543189024071263, -0.2665933059059888421 ) ) ;
#11739=CARTESIAN_POINT ( 'NONE',  ( 0.4768059346183038394, 1.738380701482456381, 0.5050996235782295729 ) ) ;
#11740=CARTESIAN_POINT ( 'NONE',  ( 0.5577427821522316087, -0.08942795157527998196, 0.3641732283464567121 ) ) ;
#11741=CARTESIAN_POINT ( 'NONE',  ( -0.8989501312335946848, -0.6692913385826771977, 0.1292274648535927661 ) ) ;
#11742=CARTESIAN_POINT ( 'NONE',  ( 0.2559055118110243887, 0.1660481256975885056, 0.3530559997133364547 ) ) ;
#11743=CARTESIAN_POINT ( 'NONE',  ( 0.1115485564304470323, 0.1771653543307087630, 0.09757992244046791164 ) ) ;
#11744=CARTESIAN_POINT ( 'NONE',  ( -1.482939632545930975, -0.3690944881889765550, -0.3153832671262227771 ) ) ;
#11745=CARTESIAN_POINT ( 'NONE',  ( 0.6561679790026253567, -0.6046776061558809534, -0.2411417322834644161 ) ) ;
#11747=CARTESIAN_POINT ( 'NONE',  ( 1.200787401574803681, -0.4536011799217368745, -0.2665933059059886201 ) ) ;
#11748=CARTESIAN_POINT ( 'NONE',  ( -0.8661417322834640276, -0.1870078740157480879, -0.4822834645669291653 ) ) ;
#11749=CARTESIAN_POINT ( 'NONE',  ( -0.3871391076115476282, -0.08942795157527998196, 0.3641732283464567121 ) ) ;
#11751=CARTESIAN_POINT ( 'NONE',  ( 0.4133858267716541968, -0.4536011799217368745, -0.2665933059059886201 ) ) ;
#11752=CARTESIAN_POINT ( 'NONE',  ( -0.9842519685039365918, -0.6692913385826771977, 8.415575281601705876E-17 ) ) ;
#11753=CARTESIAN_POINT ( 'NONE',  ( -0.4724409448818890911, -0.1870078740157480879, -0.4822834645669291653 ) ) ;
#11757=CARTESIAN_POINT ( 'NONE',  ( 0.8136482939632553313, 0.1283753931104748280, 0.1820866141732283561 ) ) ;
#11758=CARTESIAN_POINT ( 'NONE',  ( -0.1837270341207340729, 0.2306618581243847221, -0.2411417322834647770 ) ) ;
#11759=CIRCLE ( 'NONE', #41320, 0.4822834645669291653 ) ;
#11760=CARTESIAN_POINT ( 'NONE',  ( -0.7545931758530176614, -0.6692913385826773087, -0.1292274648535924053 ) ) ;
#11761=CARTESIAN_POINT ( 'NONE',  ( -0.8202099737532799750, 0.1771653543307087075, -0.09757992244046823083 ) ) ;
#11763=CARTESIAN_POINT ( 'NONE',  ( 0.09186351706036827158, 0.05413385826771666132, 0.4176697321401328100 ) ) ;
#11764=CARTESIAN_POINT ( 'NONE',  ( -1.627296587926508442, -0.5023911411419708095, -0.1820866141732282451 ) ) ;
#11765=CARTESIAN_POINT ( 'NONE',  ( -1.574803149606298192, -0.1870078740157480879, -0.4822834645669291653 ) ) ;
#11769=CARTESIAN_POINT ( 'NONE',  ( -1.437007874015747477, -0.5400638737290844871, 0.3530559997133364547 ) ) ;
#11770=CARTESIAN_POINT ( 'NONE',  ( -0.9645669291338575535, -0.5400638737290844871, 0.3530559997133364547 ) ) ;
#11772=CARTESIAN_POINT ( 'NONE',  ( 1.528871391076116026, -0.6692913385826773087, -0.1292274648535924053 ) ) ;
#11775=CARTESIAN_POINT ( 'NONE',  ( 0.9055118110236227702, 0.2952755905511811885, 0.000000000000000000 ) ) ;
#11776=CARTESIAN_POINT ( 'NONE',  ( 0.4986876640419954376, -0.6046776061558809534, -0.2411417322834644161 ) ) ;
#11779=CARTESIAN_POINT ( 'NONE',  ( 1.213910761154856299, -0.5511811023622048555, -0.09757992244046775898 ) ) ;
#11784=CARTESIAN_POINT ( 'NONE',  ( 0.4068241469816279987, -0.4281496062992127816, -0.4176697321401328100 ) ) ;
#11785=CARTESIAN_POINT ( 'NONE',  ( -0.7808398950131225646, -0.05778040916215522460, 0.4822834645669289988 ) ) ;
#11786=CARTESIAN_POINT ( 'NONE',  ( 1.607611548556431069, 0.2952755905511811885, 0.1292274648535926551 ) ) ;
#11787=CARTESIAN_POINT ( 'NONE',  ( 1.200787401574803681, 0.1660481256975885056, 0.3530559997133364547 ) ) ;
#11788=CARTESIAN_POINT ( 'NONE',  ( -1.601049868766403650, 0.1283753931104746893, -0.1820866141732285504 ) ) ;
#11790=CARTESIAN_POINT ( 'NONE',  ( -0.1771653543307080136, 0.1660481256975883668, -0.3530559997133364547 ) ) ;
#11791=CARTESIAN_POINT ( 'NONE',  ( -1.417322834645668772, -0.1870078740157480879, -0.4822834645669291653 ) ) ;
#11792=CARTESIAN_POINT ( 'NONE',  ( -1.568241469816272105, -0.3162353388693409650, -0.4822834645669289433 ) ) ;
#11793=CARTESIAN_POINT ( 'NONE',  ( 1.391076115485564868, 0.2306618581243847221, -0.2411417322834647770 ) ) ;
#11795=CARTESIAN_POINT ( 'NONE',  ( 0.8727034120734913358, -0.08942795157527998196, 0.3641732283464567121 ) ) ;
#11799=CARTESIAN_POINT ( 'NONE',  ( -0.1443569553805768291, -0.004921259842519576551, 0.3153832671262227771 ) ) ;
#11800=CARTESIAN_POINT ( 'NONE',  ( 0.7677165354330716118, -0.5400638737290844871, 0.3530559997133364547 ) ) ;
#11801=CARTESIAN_POINT ( 'NONE',  ( 0.4330708661417329575, -0.6692913385826771977, 8.415575281601705876E-17 ) ) ;
#11802=CARTESIAN_POINT ( 'NONE',  ( -0.6692913385826764205, -0.6692913385826771977, 8.415575281601705876E-17 ) ) ;
#11804=CARTESIAN_POINT ( 'NONE',  ( -1.377952755905511140, -0.6692913385826771977, 8.415575281601705876E-17 ) ) ;
#11806=CARTESIAN_POINT ( 'NONE',  ( 1.345144356955381593, -0.2845877964562161244, -0.3641732283464567121 ) ) ;
#11807=CARTESIAN_POINT ( 'NONE',  ( -1.522309711286088607, -0.6046776061558807314, 0.2411417322834647770 ) ) ;
#11808=CARTESIAN_POINT ( 'NONE',  ( 0.9448818897637802916, -0.1870078740157480879, -0.4822834645669291653 ) ) ;
#11809=CARTESIAN_POINT ( 'NONE',  ( 0.9908136482939640111, -0.6692913385826771977, 0.1292274648535927661 ) ) ;
#11811=CARTESIAN_POINT ( 'NONE',  ( -1.371391076115484831, 0.2952755905511810774, -0.1292274648535930714 ) ) ;
#11813=CARTESIAN_POINT ( 'NONE',  ( -0.1968503937007867743, -0.6692913385826771977, 8.415575281601705876E-17 ) ) ;
#11819=CARTESIAN_POINT ( 'NONE',  ( 1.299212598425197429, -0.6692913385826771977, 8.415575281601705876E-17 ) ) ;
#11820=CARTESIAN_POINT ( 'NONE',  ( 0.09842519685039434474, 0.07958543189024085140, 0.2665933059059887866 ) ) ;
#11821=CARTESIAN_POINT ( 'NONE',  ( 0.8070866141732288002, 0.1660481256975885056, 0.3530559997133364547 ) ) ;
#11823=CARTESIAN_POINT ( 'NONE',  ( 0.8202099737532814183, -0.5511811023622048555, -0.09757992244046775898 ) ) ;
#11824=CARTESIAN_POINT ( 'NONE',  ( 0.3740157480314966754, 0.1660481256975883668, -0.3530559997133364547 ) ) ;
#11826=CARTESIAN_POINT ( 'NONE',  ( -0.6889763779527552368, -0.5400638737290845981, -0.3530559997133363437 ) ) ;
#11827=CARTESIAN_POINT ( 'NONE',  ( -0.2099737532808391705, 0.2306618581243848609, 0.2411417322834645549 ) ) ;
#11828=CARTESIAN_POINT ( 'NONE',  ( 1.115485564304462551, -0.004921259842519576551, 0.3153832671262227771 ) ) ;
#11830=CARTESIAN_POINT ( 'NONE',  ( -0.2230971128608915943, -0.4281496062992127816, -0.4176697321401328100 ) ) ;
#11831=CARTESIAN_POINT ( 'NONE',  ( 0.2493438320209980519, -0.004921259842519576551, 0.3153832671262227771 ) ) ;
#11833=CARTESIAN_POINT ( 'NONE',  ( -0.4790026246719154557, -0.3162353388693405765, 0.4822834645669290543 ) ) ;
#11834=CARTESIAN_POINT ( 'NONE',  ( 0.5380577427821529035, -0.004921259842519870586, -0.3153832671262229437 ) ) ;
#11836=CARTESIAN_POINT ( 'NONE',  ( 0.1509186351706045259, -0.05778040916215560624, -0.4822834645669293319 ) ) ;
#11837=CARTESIAN_POINT ( 'NONE',  ( 1.384514435695538559, 0.1771653543307087075, -0.09757992244046823083 ) ) ;
#11838=CARTESIAN_POINT ( 'NONE',  ( 0.4839371108951637801, 2.606013654608237919E-15, 0.3791475997938224540 ) ) ;
#11839=CARTESIAN_POINT ( 'NONE',  ( -0.3608923884514428360, -0.5511811023622048555, -0.09757992244046775898 ) ) ;
#11840=CARTESIAN_POINT ( 'NONE',  ( -0.5380577427821514602, -0.3690944881889765550, -0.3153832671262227771 ) ) ;
#11841=CARTESIAN_POINT ( 'NONE',  ( -0.2230971128608915943, 0.05413385826771666132, 0.4176697321401328100 ) ) ;
#11842=CARTESIAN_POINT ( 'NONE',  ( 0.1377952755905518800, -0.5400638737290844871, 0.3530559997133364547 ) ) ;
#11843=CARTESIAN_POINT ( 'NONE',  ( 0.8792650918635177559, -0.004921259842519576551, 0.3153832671262227771 ) ) ;
#11845=CARTESIAN_POINT ( 'NONE',  ( -1.679790026246718693, 0.2306618581243847221, -0.2411417322834647770 ) ) ;
#11846=CARTESIAN_POINT ( 'NONE',  ( 0.7480314960629927956, 0.2952755905511811885, 0.000000000000000000 ) ) ;
#11848=CARTESIAN_POINT ( 'NONE',  ( -0.3149606299212590610, -0.1870078740157479769, 0.4822834645669291653 ) ) ;
#11850=CARTESIAN_POINT ( 'NONE',  ( 0.8005249343832028242, -0.4281496062992127816, -0.4176697321401328100 ) ) ;
#11851=CARTESIAN_POINT ( 'NONE',  ( 0.5643044619422579178, 0.05413385826771666132, 0.4176697321401328100 ) ) ;
#11853=CARTESIAN_POINT ( 'NONE',  ( 0.5643044619422579178, -0.004921259842519576551, 0.3153832671262227771 ) ) ;
#11854=CARTESIAN_POINT ( 'NONE',  ( 0.9973753280839902091, -0.6046776061558807314, 0.2411417322834647770 ) ) ;
#11855=CARTESIAN_POINT ( 'NONE',  ( 0.01968503937007930540, 0.07958543189024085140, 0.2665933059059887866 ) ) ;
#11856=CARTESIAN_POINT ( 'NONE',  ( -0.3280839895013117347, 0.05413385826771626580, -0.4176697321401330321 ) ) ;
#11858=CARTESIAN_POINT ( 'NONE',  ( 0.4724409448818904789, -0.1870078740157479769, 0.4822834645669291653 ) ) ;
#11859=CARTESIAN_POINT ( 'NONE',  ( -0.9580052493438311334, 0.05413385826771626580, -0.4176697321401330321 ) ) ;
#11860=CARTESIAN_POINT ( 'NONE',  ( -0.4133858267716528645, 0.07958543189024071263, -0.2665933059059888421 ) ) ;
#11861=CARTESIAN_POINT ( 'NONE',  ( 0.2755905511811031494, -0.6692913385826771977, 8.415575281601705876E-17 ) ) ;
#11862=CARTESIAN_POINT ( 'NONE',  ( 0.8530183727034128527, -0.3690944881889763329, 0.3153832671262228327 ) ) ;
#11863=CARTESIAN_POINT ( 'NONE',  ( -0.3871391076115476282, -0.05778040916215522460, 0.4822834645669289988 ) ) ;
#11866=CARTESIAN_POINT ( 'NONE',  ( 1.502624671916010790, -0.3162353388693409650, -0.4822834645669289433 ) ) ;
#11870=CARTESIAN_POINT ( 'NONE',  ( -1.463254593175852492, 0.2952755905511811885, 0.1292274648535926551 ) ) ;
#11871=CARTESIAN_POINT ( 'NONE',  ( -0.7480314960629914633, 0.2952755905511811885, 0.000000000000000000 ) ) ;
#11874=VERTEX_POINT ( 'NONE', #39341 ) ;
#11875=CARTESIAN_POINT ( 'NONE',  ( 0.5183727034120741983, -0.5511811023622046335, 0.09757992244046803654 ) ) ;
#11877=CARTESIAN_POINT ( 'NONE',  ( 0.8464566929133865436, 0.1660481256975883668, -0.3530559997133364547 ) ) ;
#11879=CARTESIAN_POINT ( 'NONE',  ( -1.614173228346457378, 1.818966223839196372, 0.1372047244094476981 ) ) ;
#11880=CARTESIAN_POINT ( 'NONE',  ( -0.2624671916010490880, -0.5023911411419708095, 0.1820866141732285504 ) ) ;
#11881=CARTESIAN_POINT ( 'NONE',  ( -1.646981627296586703, -0.2845877964562161244, -0.3641732283464567121 ) ) ;
#11882=CARTESIAN_POINT ( 'NONE',  ( 1.187664041994751285, -0.05778040916215522460, 0.4822834645669289988 ) ) ;
#11883=CARTESIAN_POINT ( 'NONE',  ( 1.377952755905512472, -0.5511811023622047445, 6.969142054262312111E-17 ) ) ;
#11884=CARTESIAN_POINT ( 'NONE',  ( 0.03280839895013198948, -0.6692913385826773087, -0.1292274648535924053 ) ) ;
#11886=CARTESIAN_POINT ( 'NONE',  ( -0.2230971128608915943, 0.05413385826771666132, 0.4176697321401328100 ) ) ;
#11887=CARTESIAN_POINT ( 'NONE',  ( -1.502624671916009680, -0.08942795157528024563, -0.3641732283464568787 ) ) ;
#11888=CARTESIAN_POINT ( 'NONE',  ( -0.3937007874015740483, -0.1870078740157480879, -0.4822834645669291653 ) ) ;
#11891=ORIENTED_EDGE ( 'NONE', *, *, #3865, .T. ) ;
#11893=CARTESIAN_POINT ( 'NONE',  ( 0.2952755905511819101, 0.1660481256975883668, -0.3530559997133364547 ) ) ;
#11894=ORIENTED_EDGE ( 'NONE', *, *, #57231, .F. ) ;
#11895=CARTESIAN_POINT ( 'NONE',  ( -0.3871391076115479057, -0.3162353388693409650, -0.4822834645669289433 ) ) ;
#11896=CARTESIAN_POINT ( 'NONE',  ( -1.587926509186350810, 0.05413385826771626580, -0.4176697321401330321 ) ) ;
#11897=CARTESIAN_POINT ( 'NONE',  ( 0.7414698162729663755, -0.6692913385826773087, -0.1292274648535924053 ) ) ;
#11898=CARTESIAN_POINT ( 'NONE',  ( 0.1509186351706045259, -0.05778040916215560624, -0.4822834645669293319 ) ) ;
#11900=CARTESIAN_POINT ( 'NONE',  ( -0.7545931758530177724, 0.2952755905511811885, 0.1292274648535926551 ) ) ;
#11901=CARTESIAN_POINT ( 'NONE',  ( 0.3543307086614181922, -0.6692913385826771977, 8.415575281601705876E-17 ) ) ;
#11902=CARTESIAN_POINT ( 'NONE',  ( -0.3346456692913377662, 0.1660481256975883668, -0.3530559997133364547 ) ) ;
#11903=CARTESIAN_POINT ( 'NONE',  ( 0.3346456692913393205, -0.4536011799217368745, -0.2665933059059886201 ) ) ;
#11905=CARTESIAN_POINT ( 'NONE',  ( -0.1509186351706028884, -0.05778040916215522460, 0.4822834645669289988 ) ) ;
#11907=CARTESIAN_POINT ( 'NONE',  ( 1.515748031496063186, -0.5400638737290845981, -0.3530559997133363437 ) ) ;
#11911=CARTESIAN_POINT ( 'NONE',  ( 0.5905511811023629321, 0.2952755905511811885, 0.000000000000000000 ) ) ;
#11912=CARTESIAN_POINT ( 'NONE',  ( 0.06561679790026316017, -0.004921259842519870586, -0.3153832671262229437 ) ) ;
#11913=CARTESIAN_POINT ( 'NONE',  ( 1.272965879265092637, -0.3690944881889765550, -0.3153832671262227771 ) ) ;
#11919=CARTESIAN_POINT ( 'NONE',  ( 0.3083989501312343062, -0.3162353388693405765, 0.4822834645669290543 ) ) ;
#11920=CARTESIAN_POINT ( 'NONE',  ( -1.417322834645668772, -0.1870078740157480879, -0.4822834645669291653 ) ) ;
#11921=CARTESIAN_POINT ( 'NONE',  ( -1.220472440944881054, 0.2952755905511811885, 0.000000000000000000 ) ) ;
#11922=CARTESIAN_POINT ( 'NONE',  ( 0.2887139107611556010, -0.6046776061558807314, 0.2411417322834647770 ) ) ;
#11923=CARTESIAN_POINT ( 'NONE',  ( 0.9842519685039375910, 0.2952755905511811885, 0.000000000000000000 ) ) ;
#11924=CARTESIAN_POINT ( 'NONE',  ( 1.305774278215223960, -0.5511811023622046335, 0.09757992244046803654 ) ) ;
#11925=CARTESIAN_POINT ( 'NONE',  ( 0.8070866141732289112, -0.4536011799217368745, -0.2665933059059886201 ) ) ;
#11926=CARTESIAN_POINT ( 'NONE',  ( -0.6889763779527552368, 0.1660481256975885056, 0.3530559997133364547 ) ) ;
#11928=CARTESIAN_POINT ( 'NONE',  ( 1.489501312335958172, -0.3162353388693405765, 0.4822834645669290543 ) ) ;
#11930=CARTESIAN_POINT ( 'NONE',  ( 1.161417322834646493, -0.5400638737290844871, 0.3530559997133364547 ) ) ;
#11932=CARTESIAN_POINT ( 'NONE',  ( -1.627296587926508442, -0.5023911411419708095, -0.1820866141732282451 ) ) ;
#11933=CARTESIAN_POINT ( 'NONE',  ( 0.1706036745406830368, -0.4281496062992127816, -0.4176697321401328100 ) ) ;
#11934=CARTESIAN_POINT ( 'NONE',  ( 0.9251968503937015864, -0.4536011799217367080, 0.2665933059059888421 ) ) ;
#11935=CARTESIAN_POINT ( 'NONE',  ( -1.673228346456691717, 0.07958543189024071263, -0.2665933059059888421 ) ) ;
#11936=CARTESIAN_POINT ( 'NONE',  ( 0.8989501312335964611, 0.2952755905511811885, 0.1292274648535926551 ) ) ;
#11937=CARTESIAN_POINT ( 'NONE',  ( -0.5052493438320202479, 0.2952755905511810219, -0.1292274648535930437 ) ) ;
#11938=CARTESIAN_POINT ( 'NONE',  ( -0.4002624671916004129, -0.08942795157528024563, -0.3641732283464568787 ) ) ;
#11939=CARTESIAN_POINT ( 'NONE',  ( -0.4002624671916004129, -0.05778040916215560624, -0.4822834645669293319 ) ) ;
#11940=CARTESIAN_POINT ( 'NONE',  ( 1.489501312335958172, -0.3162353388693405765, 0.4822834645669290543 ) ) ;
#11942=CARTESIAN_POINT ( 'NONE',  ( -1.062992125984250968, 0.2952755905511811885, 0.000000000000000000 ) ) ;
#11943=CARTESIAN_POINT ( 'NONE',  ( 1.194225721784777594, 0.05413385826771666132, 0.4176697321401328100 ) ) ;
#11945=CARTESIAN_POINT ( 'NONE',  ( -1.141732283464566011, 0.1771653543307087630, 0.000000000000000000 ) ) ;
#11947=CARTESIAN_POINT ( 'NONE',  ( 1.607611548556431069, 0.2952755905511811885, 0.1292274648535926551 ) ) ;
#11949=CARTESIAN_POINT ( 'NONE',  ( -1.456692913385826182, -0.6692913385826771977, 8.415575281601705876E-17 ) ) ;
#11950=CARTESIAN_POINT ( 'NONE',  ( -1.568241469816272105, -0.2845877964562161244, -0.3641732283464567121 ) ) ;
#11951=CARTESIAN_POINT ( 'NONE',  ( -1.069553805774277722, 0.1771653543307087630, 0.09757992244046791164 ) ) ;
#11952=CARTESIAN_POINT ( 'NONE',  ( 1.640419947506562393, -0.3690944881889763329, 0.3153832671262228327 ) ) ;
#11953=CARTESIAN_POINT ( 'NONE',  ( -0.5052493438320203589, 0.2952755905511810774, -0.1292274648535930714 ) ) ;
#11954=CARTESIAN_POINT ( 'NONE',  ( 0.1377952755905518800, 0.07958543189024071263, -0.2665933059059888421 ) ) ;
#11955=CARTESIAN_POINT ( 'NONE',  ( -1.371391076115484831, 0.1771653543307087075, -0.09757992244046823083 ) ) ;
#11956=CARTESIAN_POINT ( 'NONE',  ( 1.299212598425197429, 0.1771653543307087630, 0.000000000000000000 ) ) ;
#11957=CARTESIAN_POINT ( 'NONE',  ( 0.9448818897637802916, -0.1870078740157480879, -0.4822834645669291653 ) ) ;
#11958=CARTESIAN_POINT ( 'NONE',  ( 1.443569553805774897, 0.2306618581243848609, 0.2411417322834645549 ) ) ;
#11959=CARTESIAN_POINT ( 'NONE',  ( 0.03937007874015833325, -0.5511811023622047445, 6.969142054262312111E-17 ) ) ;
#11960=CARTESIAN_POINT ( 'NONE',  ( 0.5446194225721792126, -0.3162353388693405765, 0.4822834645669290543 ) ) ;
#11961=CARTESIAN_POINT ( 'NONE',  ( 1.141732283464567566, 0.1771653543307087630, 0.000000000000000000 ) ) ;
#11962=VERTEX_POINT ( 'NONE', #65028 ) ;
#11963=CARTESIAN_POINT ( 'NONE',  ( 1.594488188976378673, 0.1660481256975885056, 0.3530559997133364547 ) ) ;
#11965=CARTESIAN_POINT ( 'NONE',  ( -1.154855643044618851, 0.2306618581243848609, 0.2411417322834645549 ) ) ;
#11966=CARTESIAN_POINT ( 'NONE',  ( -0.2952755905511804668, 0.1660481256975885056, 0.3530559997133364547 ) ) ;
#11969=CARTESIAN_POINT ( 'NONE',  ( 0.3149606299212603933, -0.1870078740157479769, 0.4822834645669291653 ) ) ;
#11970=CARTESIAN_POINT ( 'NONE',  ( 1.036745406824147508, -0.3690944881889765550, -0.3153832671262227771 ) ) ;
#11971=CARTESIAN_POINT ( 'NONE',  ( 0.1312335958005257930, 0.2306618581243847221, -0.2411417322834647770 ) ) ;
#11972=CARTESIAN_POINT ( 'NONE',  ( 0.2230971128608929543, 0.05413385826771626580, -0.4176697321401330321 ) ) ;
#11978=CARTESIAN_POINT ( 'NONE',  ( -0.3412073490813641308, -0.5023911411419708095, 0.1820866141732285504 ) ) ;
#11979=CARTESIAN_POINT ( 'NONE',  ( -0.6167979002624665030, 0.05413385826771666132, 0.4176697321401328100 ) ) ;
#11980=EDGE_CURVE ( 'NONE', #54857, #36796, #42578, .T. ) ;
#11982=CARTESIAN_POINT ( 'NONE',  ( 0.9580052493438327987, -0.4281496062992127816, -0.4176697321401328100 ) ) ;
#11983=CARTESIAN_POINT ( 'NONE',  ( -1.528871391076114250, -0.6692913385826771977, 0.1292274648535927661 ) ) ;
#11984=CARTESIAN_POINT ( 'NONE',  ( 0.7939632545931766261, -0.05778040916215522460, 0.4822834645669289988 ) ) ;
#11985=DIRECTION ( 'NONE',  ( 0.000000000000000000, 0.000000000000000000, 1.000000000000000000 ) ) ;
#11987=CARTESIAN_POINT ( 'NONE',  ( 1.574803149606299746, -0.1870078740157480879, -0.4822834645669291653 ) ) ;
#11988=CARTESIAN_POINT ( 'NONE',  ( 1.036745406824147508, -0.4281496062992127816, -0.4176697321401328100 ) ) ;
#11989=CARTESIAN_POINT ( 'NONE',  ( 0.7808398950131240079, -0.3162353388693405765, 0.4822834645669290543 ) ) ;
#11990=CARTESIAN_POINT ( 'NONE',  ( 0.9842519685039375910, 0.1771653543307087630, 0.000000000000000000 ) ) ;
#11991=CARTESIAN_POINT ( 'NONE',  ( 1.253280839895013710, -0.05778040916215560624, -0.4822834645669293319 ) ) ;
#11994=CARTESIAN_POINT ( 'NONE',  ( 0.8202099737532814183, -0.6692913385826773087, -0.1292274648535924053 ) ) ;
#11995=CARTESIAN_POINT ( 'NONE',  ( 1.686351706036745890, 0.1771653543307087630, 0.09757992244046791164 ) ) ;
#11996=CARTESIAN_POINT ( 'NONE',  ( -0.3280839895013117347, -0.4281496062992124485, 0.4176697321401328655 ) ) ;
#11997=CARTESIAN_POINT ( 'NONE',  ( -0.9514435695538050464, -0.3162353388693405765, 0.4822834645669290543 ) ) ;
#11998=CARTESIAN_POINT ( 'NONE',  ( 1.364829396325459854, -0.6046776061558809534, -0.2411417322834644161 ) ) ;
#12002=CARTESIAN_POINT ( 'NONE',  ( 1.443569553805774897, -0.6046776061558809534, -0.2411417322834644161 ) ) ;
#12005=ORIENTED_EDGE ( 'NONE', *, *, #76979, .F. ) ;
#12007=CARTESIAN_POINT ( 'NONE',  ( 1.410761154855643795, -0.2845877964562159024, 0.3641732283464567677 ) ) ;
#12009=CARTESIAN_POINT ( 'NONE',  ( 1.391076115485564868, 0.1283753931104746893, -0.1820866141732285504 ) ) ;
#12010=CARTESIAN_POINT ( 'NONE',  ( -0.7754685323813622633, -1.146068349578384814E-15, 0.3627985898453520153 ) ) ;
#12011=DIRECTION ( 'NONE',  ( -1.000000000000000000, -3.083952846180989294E-16, 0.000000000000000000 ) ) ;
#12014=CARTESIAN_POINT ( 'NONE',  ( -0.7611548556430438595, -0.5023911411419708095, -0.1820866141732282451 ) ) ;
#12015=CARTESIAN_POINT ( 'NONE',  ( -1.391076115485563758, 0.1283753931104748280, 0.1820866141732283561 ) ) ;
#12016=CARTESIAN_POINT ( 'NONE',  ( -1.371391076115484609, -0.6692913385826771977, 0.1292274648535927661 ) ) ;
#12017=CARTESIAN_POINT ( 'NONE',  ( 0.1049868766404206816, -0.6046776061558809534, -0.2411417322834644161 ) ) ;
#12018=CARTESIAN_POINT ( 'NONE',  ( 1.502624671916010790, -0.3162353388693409650, -0.4822834645669289433 ) ) ;
#12019=ORIENTED_EDGE ( 'NONE', *, *, #62545, .T. ) ;
#12020=CARTESIAN_POINT ( 'NONE',  ( -1.620734908136482577, 0.2952755905511811885, 0.1292274648535926551 ) ) ;
#12021=CARTESIAN_POINT ( 'NONE',  ( -1.607539944893438655, 0.2919301301068724097, 0.05787806847778405317 ) ) ;
#12025=CARTESIAN_POINT ( 'NONE',  ( -0.5774278215223089816, -0.5023911411419708095, 0.1820866141732285504 ) ) ;
#12026=CARTESIAN_POINT ( 'NONE',  ( -1.358267716535432434, -0.5400638737290844871, 0.3530559997133364547 ) ) ;
#12027=CARTESIAN_POINT ( 'NONE',  ( 1.115485564304462551, -0.4281496062992127816, -0.4176697321401328100 ) ) ;
#12028=ORIENTED_EDGE ( 'NONE', *, *, #43363, .T. ) ;
#12030=DIRECTION ( 'NONE',  ( 0.000000000000000000, 0.000000000000000000, -1.000000000000000000 ) ) ;
#12031=CARTESIAN_POINT ( 'NONE',  ( 1.174540682414699111, -0.3162353388693405765, 0.4822834645669290543 ) ) ;
#12032=CARTESIAN_POINT ( 'NONE',  ( -1.102362204724408601, -0.1870078740157479769, 0.4822834645669291653 ) ) ;
#12034=CARTESIAN_POINT ( 'NONE',  ( -0.3871391076115479057, -0.2845877964562161244, -0.3641732283464567121 ) ) ;
#12036=CARTESIAN_POINT ( 'NONE',  ( -0.6627296587926501115, 0.1771653543307087075, -0.09757992244046823083 ) ) ;
#12037=CARTESIAN_POINT ( 'NONE',  ( 0.6889763779527563470, 0.07958543189024071263, -0.2665933059059888421 ) ) ;
#12038=CARTESIAN_POINT ( 'NONE',  ( 0.07874015748031558404, -0.1870078740157480879, -0.4822834645669291653 ) ) ;
#12040=CARTESIAN_POINT ( 'NONE',  ( -0.6758530183727028406, 0.1771653543307087630, 0.09757992244046791164 ) ) ;
#12042=CARTESIAN_POINT ( 'NONE',  ( 0.9580052493438326877, 0.05413385826771666132, 0.4176697321401328100 ) ) ;
#12043=CARTESIAN_POINT ( 'NONE',  ( -0.8530183727034112984, 0.05413385826771666132, 0.4176697321401328100 ) ) ;
#12045=CARTESIAN_POINT ( 'NONE',  ( -0.3149606299212590610, -0.1870078740157479769, 0.4822834645669291653 ) ) ;
#12046=CARTESIAN_POINT ( 'NONE',  ( -0.8398950131233585692, 0.2306618581243848609, 0.2411417322834645549 ) ) ;
#12047=CARTESIAN_POINT ( 'NONE',  ( 1.148293963254593875, -0.5511811023622046335, 0.09757992244046803654 ) ) ;
#12048=CARTESIAN_POINT ( 'NONE',  ( 0.3149606299212603933, -0.1870078740157479769, 0.3641732283464567677 ) ) ;
#12049=CARTESIAN_POINT ( 'NONE',  ( -0.5774278215223089816, 0.2306618581243847221, -0.2411417322834647770 ) ) ;
#12051=CARTESIAN_POINT ( 'NONE',  ( -1.220472440944881054, -0.6692913385826771977, 8.415575281601705876E-17 ) ) ;
#12053=CARTESIAN_POINT ( 'NONE',  ( 1.646981627296588035, -0.2845877964562159024, 0.3641732283464567677 ) ) ;
#12054=CARTESIAN_POINT ( 'NONE',  ( -0.4068241469816264999, -0.4281496062992124485, 0.4176697321401328655 ) ) ;
#12055=CARTESIAN_POINT ( 'NONE',  ( -1.056430446194224881, 0.2952755905511810774, -0.1292274648535930714 ) ) ;
#12056=EDGE_LOOP ( 'NONE', ( #55436, #10363, #21935, #2965 ) ) ;
#12058=CARTESIAN_POINT ( 'NONE',  ( 1.036745406824147508, -0.4281496062992127816, -0.4176697321401328100 ) ) ;
#12059=CARTESIAN_POINT ( 'NONE',  ( -0.5249343832020990641, -0.5023911411419708095, -0.1820866141732282451 ) ) ;
#12060=CARTESIAN_POINT ( 'NONE',  ( -0.8267716535433065062, -0.6692913385826771977, 8.415575281601705876E-17 ) ) ;
#12061=CARTESIAN_POINT ( 'NONE',  ( 1.089238845144357759, 0.05413385826771626580, -0.4176697321401330321 ) ) ;
#12062=CARTESIAN_POINT ( 'NONE',  ( 0.7152230971128616943, -0.05778040916215522460, 0.4822834645669289988 ) ) ;
#12064=CARTESIAN_POINT ( 'NONE',  ( -1.240157480314959759, 0.07958543189024085140, 0.2665933059059887866 ) ) ;
#12070=CARTESIAN_POINT ( 'NONE',  ( 1.017060367454068803, -0.2845877964562159024, 0.3641732283464567677 ) ) ;
#12071=CARTESIAN_POINT ( 'NONE',  ( 0.6692913385826777528, 0.1771653543307087630, 0.000000000000000000 ) ) ;
#12072=CARTESIAN_POINT ( 'NONE',  ( 0.6955380577427828781, 0.05413385826771626580, -0.4176697321401330321 ) ) ;
#12075=CARTESIAN_POINT ( 'NONE',  ( 0.8661417322834653598, -0.1870078740157479769, 0.3641732283464567677 ) ) ;
#12076=CARTESIAN_POINT ( 'NONE',  ( -0.1640419947506553400, -0.05778040916215560624, -0.4822834645669293319 ) ) ;
#12077=CARTESIAN_POINT ( 'NONE',  ( -1.181102362204723644, -0.1870078740157479769, 0.4822834645669291653 ) ) ;
#12078=CARTESIAN_POINT ( 'NONE',  ( 1.351706036745407680, 0.05413385826771666132, 0.4176697321401328100 ) ) ;
#12081=CARTESIAN_POINT ( 'NONE',  ( -0.1902887139107604098, -0.5511811023622046335, 0.09757992244046803654 ) ) ;
#12082=EDGE_CURVE ( 'NONE', #46955, #61268, #20535, .T. ) ;
#12085=CARTESIAN_POINT ( 'NONE',  ( -1.003937007874015297, -0.5400638737290845981, -0.3530559997133363437 ) ) ;
#12086=CARTESIAN_POINT ( 'NONE',  ( -0.4790026246719152336, -0.05778040916215560624, -0.4822834645669293319 ) ) ;
#12087=CARTESIAN_POINT ( 'NONE',  ( -0.7152230971128602510, -0.3162353388693405765, 0.4822834645669290543 ) ) ;
#12088=CARTESIAN_POINT ( 'NONE',  ( 0.3805774278215230400, -0.4281496062992124485, 0.4176697321401328655 ) ) ;
#12089=EDGE_CURVE ( 'NONE', #62837, #21784, #71758, .T. ) ;
#12090=CARTESIAN_POINT ( 'NONE',  ( -0.4855643044619415427, 0.05413385826771626580, -0.4176697321401330321 ) ) ;
#12091=CARTESIAN_POINT ( 'NONE',  ( -1.279527559055116948, 0.1660481256975883668, -0.3530559997133364547 ) ) ;
#12092=CARTESIAN_POINT ( 'NONE',  ( -1.023622047244094002, -0.1870078740157480879, -0.4822834645669291653 ) ) ;
#12093=CARTESIAN_POINT ( 'NONE',  ( 0.8727034120734912248, -0.3162353388693409650, -0.4822834645669289433 ) ) ;
#12095=CARTESIAN_POINT ( 'NONE',  ( -0.4527559055118102749, -0.4536011799217368745, -0.2665933059059886201 ) ) ;
#12099=CARTESIAN_POINT ( 'NONE',  ( -1.174540682414697335, -0.2845877964562161244, -0.3641732283464567121 ) ) ;
#12100=CARTESIAN_POINT ( 'NONE',  ( -1.076115485564303809, -0.6046776061558809534, -0.2411417322834644161 ) ) ;
#12101=CARTESIAN_POINT ( 'NONE',  ( -1.043307086614172041, -0.5400638737290844871, 0.3530559997133364547 ) ) ;
#12103=CARTESIAN_POINT ( 'NONE',  ( -1.312335958005248715, -0.6046776061558809534, -0.2411417322834644161 ) ) ;
#12104=CARTESIAN_POINT ( 'NONE',  ( -0.9514435695538050464, -0.3162353388693405765, 0.4822834645669290543 ) ) ;
#12107=CARTESIAN_POINT ( 'NONE',  ( 0.3871391076115493490, -0.2845877964562159024, 0.3641732283464567677 ) ) ;
#12108=CYLINDRICAL_SURFACE ( 'NONE', #72, 0.3937007874015748254 ) ;
#12110=CARTESIAN_POINT ( 'NONE',  ( 0.05905511811023681640, 0.07958543189024071263, -0.2665933059059888421 ) ) ;
#12111=CARTESIAN_POINT ( 'NONE',  ( -0.5314960629921250401, 0.1660481256975885056, 0.3530559997133364547 ) ) ;
#12112=CARTESIAN_POINT ( 'NONE',  ( 1.227034120734908917, -0.6692913385826771977, 0.1292274648535927661 ) ) ;
#12113=CARTESIAN_POINT ( 'NONE',  ( -0.4265091863517051496, -0.6692913385826771977, 0.1292274648535927661 ) ) ;
#12116=CARTESIAN_POINT ( 'NONE',  ( -0.8537221893815262197, -2.294479370626195693E-15, 0.3464511005275217603 ) ) ;
#12119=CARTESIAN_POINT ( 'NONE',  ( -0.3871391076115476282, -0.05778040916215522460, 0.4822834645669289988 ) ) ;
#12120=CARTESIAN_POINT ( 'NONE',  ( 1.299212598425197429, 0.2952755905511811885, 0.000000000000000000 ) ) ;
#12121=CARTESIAN_POINT ( 'NONE',  ( -1.023622047244094002, -0.1870078740157480601, -0.3641732283464567677 ) ) ;
#12122=CARTESIAN_POINT ( 'NONE',  ( -1.410761154855642463, -0.05778040916215522460, 0.4822834645669289988 ) ) ;
#12125=CARTESIAN_POINT ( 'NONE',  ( -0.7137454485294948414, 2.165354330708661124, 0.4917280318828577412 ) ) ;
#12127=CARTESIAN_POINT ( 'NONE',  ( 1.272965879265092637, -0.4281496062992127816, -0.4176697321401328100 ) ) ;
#12129=CARTESIAN_POINT ( 'NONE',  ( 0.09186351706036827158, 0.05413385826771666132, 0.4176697321401328100 ) ) ;
#12130=CARTESIAN_POINT ( 'NONE',  ( -1.122047244094487306, 0.07958543189024071263, -0.2665933059059888421 ) ) ;
#12131=CARTESIAN_POINT ( 'NONE',  ( -0.3149606299212590610, -0.1870078740157479769, 0.4822834645669291653 ) ) ;
#12133=CARTESIAN_POINT ( 'NONE',  ( -0.8136482939632537770, -0.6046776061558807314, 0.2411417322834647770 ) ) ;
#12136=CARTESIAN_POINT ( 'NONE',  ( 0.7217847769028878924, -0.3690944881889765550, -0.3153832671262227771 ) ) ;
#12137=CARTESIAN_POINT ( 'NONE',  ( -0.2493438320209966919, -0.004921259842519870586, -0.3153832671262229437 ) ) ;
#12138=CARTESIAN_POINT ( 'NONE',  ( 0.8398950131233602345, -0.5023911411419708095, 0.1820866141732285504 ) ) ;
#12139=CARTESIAN_POINT ( 'NONE',  ( -1.404199475065615932, 0.05413385826771666132, 0.4176697321401328100 ) ) ;
#12141=CARTESIAN_POINT ( 'NONE',  ( 0.7414698162729663755, 0.1771653543307087630, 0.09757992244046791164 ) ) ;
#12142=CARTESIAN_POINT ( 'NONE',  ( -0.8070866141732276899, 0.1660481256975883668, -0.3530559997133364547 ) ) ;
#12145=CARTESIAN_POINT ( 'NONE',  ( 0.04593175853018440641, -0.5511811023622046335, 0.09757992244046803654 ) ) ;
#12146=CARTESIAN_POINT ( 'NONE',  ( -1.719160104986876103, -0.004921259842519576551, 0.3153832671262227771 ) ) ;
#12147=CARTESIAN_POINT ( 'NONE',  ( 0.5643044619422579178, 0.05413385826771666132, 0.4176697321401328100 ) ) ;
#12149=CARTESIAN_POINT ( 'NONE',  ( 1.541994750656168645, -0.5511811023622046335, 0.09757992244046803654 ) ) ;
#12151=CARTESIAN_POINT ( 'NONE',  ( -1.456692913385826182, -0.6692913385826771977, 8.415575281601705876E-17 ) ) ;
#12152=CARTESIAN_POINT ( 'NONE',  ( -0.4330708661417315697, -0.5511811023622047445, 6.969142054262312111E-17 ) ) ;
#12153=CARTESIAN_POINT ( 'NONE',  ( 0.4606732211678789546, 1.763126522798926343, 0.5309055118110234117 ) ) ;
#12154=CARTESIAN_POINT ( 'NONE',  ( 0.1902887139107617975, 0.1771653543307087630, 0.09757992244046791164 ) ) ;
#12155=CARTESIAN_POINT ( 'NONE',  ( -0.9580052493438311334, -0.4281496062992124485, 0.4176697321401328655 ) ) ;
#12157=CARTESIAN_POINT ( 'NONE',  ( -0.6955380577427815458, 0.05413385826771666132, 0.4176697321401328100 ) ) ;
#12160=CARTESIAN_POINT ( 'NONE',  ( 0.5905511811023629321, -0.5511811023622047445, 6.969142054262312111E-17 ) ) ;
#12161=CARTESIAN_POINT ( 'NONE',  ( -0.3346456692913377662, 0.1660481256975883668, -0.3530559997133364547 ) ) ;
#12162=CARTESIAN_POINT ( 'NONE',  ( -0.6561679790026240244, 0.2306618581243847221, -0.2411417322834647770 ) ) ;
#12163=CARTESIAN_POINT ( 'NONE',  ( -1.017060367454067249, -0.08942795157527998196, 0.3641732283464567121 ) ) ;
#12165=CARTESIAN_POINT ( 'NONE',  ( -0.05249343832020911260, 0.2306618581243848609, 0.2411417322834645549 ) ) ;
#12166=CARTESIAN_POINT ( 'NONE',  ( -1.410761154855642463, -0.08942795157527998196, 0.3641732283464567121 ) ) ;
#12167=CARTESIAN_POINT ( 'NONE',  ( 1.154855643044620184, 0.2306618581243847221, -0.2411417322834647770 ) ) ;
#12172=CARTESIAN_POINT ( 'NONE',  ( -1.325459317585300889, -0.4281496062992127816, -0.4176697321401328100 ) ) ;
#12173=CARTESIAN_POINT ( 'NONE',  ( -1.076115485564303809, 0.2306618581243848609, 0.2411417322834645549 ) ) ;
#12174=CARTESIAN_POINT ( 'NONE',  ( 1.482939632545932307, 0.05413385826771626580, -0.4176697321401330321 ) ) ;
#12177=CARTESIAN_POINT ( 'NONE',  ( 0.8267716535433078384, -0.6692913385826771977, 8.415575281601705876E-17 ) ) ;
#12178=CARTESIAN_POINT ( 'NONE',  ( 0.1312335958005257930, 0.2306618581243847221, -0.2411417322834647770 ) ) ;
#12180=CARTESIAN_POINT ( 'NONE',  ( 1.614173228346456712, 0.000000000000000000, -0.5309055118110239668 ) ) ;
#12181=CARTESIAN_POINT ( 'NONE',  ( 1.095800524934383846, -0.2845877964562159024, 0.3641732283464567677 ) ) ;
#12187=CARTESIAN_POINT ( 'NONE',  ( 0.2034120734908142214, 0.2952755905511810774, -0.1292274648535930714 ) ) ;
#12188=CARTESIAN_POINT ( 'NONE',  ( -0.8661417322834640276, -0.1870078740157480879, -0.4822834645669291653 ) ) ;
#12189=CARTESIAN_POINT ( 'NONE',  ( -1.607611548556429737, 0.2952755905511810774, -0.1292274648535930714 ) ) ;
#12190=CARTESIAN_POINT ( 'NONE',  ( 0.8136482939632553313, -0.6046776061558809534, -0.2411417322834644161 ) ) ;
#12191=CARTESIAN_POINT ( 'NONE',  ( -1.548556430446193399, -0.5023911411419708095, -0.1820866141732282451 ) ) ;
#12192=CARTESIAN_POINT ( 'NONE',  ( 1.240157480314961314, -0.5400638737290844871, 0.3530559997133364547 ) ) ;
#12193=CARTESIAN_POINT ( 'NONE',  ( -0.1509186351706028884, -0.3162353388693409650, -0.4822834645669289433 ) ) ;
#12194=CARTESIAN_POINT ( 'NONE',  ( -1.384514435695537005, -0.6692913385826773087, -0.1292274648535924053 ) ) ;
#12195=CARTESIAN_POINT ( 'NONE',  ( -1.463254593175852492, 0.2952755905511811885, 0.1292274648535926551 ) ) ;
#12197=CARTESIAN_POINT ( 'NONE',  ( 1.555118110236221041, 0.1660481256975883668, -0.3530559997133364547 ) ) ;
#12199=CARTESIAN_POINT ( 'NONE',  ( 0.9711286089238851948, -0.5023911411419708095, -0.1820866141732282451 ) ) ;
#12203=CARTESIAN_POINT ( 'NONE',  ( -0.1771653543307080136, -0.4536011799217367080, 0.2665933059059888421 ) ) ;
#12205=CARTESIAN_POINT ( 'NONE',  ( 0.01312335958005323398, 0.05413385826771666132, 0.4176697321401328100 ) ) ;
#12206=CARTESIAN_POINT ( 'NONE',  ( 0.6036745406824153282, -0.6046776061558807314, 0.2411417322834647770 ) ) ;
#12207=CARTESIAN_POINT ( 'NONE',  ( -0.4396325459317579898, 0.2952755905511811885, 0.1292274648535926551 ) ) ;
#12210=CARTESIAN_POINT ( 'NONE',  ( -1.417322834645668772, -0.1870078740157480879, -0.4822834645669291653 ) ) ;
#12212=CARTESIAN_POINT ( 'NONE',  ( 1.240157480314961314, -0.4536011799217367080, 0.2665933059059888421 ) ) ;
#12213=CARTESIAN_POINT ( 'NONE',  ( -1.581364829396324945, -0.05778040916215560624, -0.4822834645669293319 ) ) ;
#12214=CARTESIAN_POINT ( 'NONE',  ( 0.7283464566929143125, 0.1660481256975885056, 0.3530559997133364547 ) ) ;
#12215=CARTESIAN_POINT ( 'NONE',  ( 1.115485564304462551, -0.4281496062992127816, -0.4176697321401328100 ) ) ;
#12216=AXIS2_PLACEMENT_3D ( 'NONE', #58794, #43044, #67922 ) ;
#12218=CARTESIAN_POINT ( 'NONE',  ( -1.246719160104986512, 0.05413385826771666132, 0.4176697321401328100 ) ) ;
#12221=CARTESIAN_POINT ( 'NONE',  ( -0.2887139107611542133, 0.2306618581243848609, 0.2411417322834645549 ) ) ;
#12224=CARTESIAN_POINT ( 'NONE',  ( 1.102362204724410155, -0.1870078740157479769, 0.4822834645669291653 ) ) ;
#12225=CARTESIAN_POINT ( 'NONE',  ( 1.496062992125985147, -0.1870078740157479769, 0.4822834645669291653 ) ) ;
#12226=CARTESIAN_POINT ( 'NONE',  ( 0.1246719160104994284, 0.1771653543307087075, -0.09757992244046823083 ) ) ;
#12227=CARTESIAN_POINT ( 'NONE',  ( 0.7020997375328090762, -0.05778040916215560624, -0.4822834645669293319 ) ) ;
#12229=CARTESIAN_POINT ( 'NONE',  ( 0.4068241469816281097, -0.004921259842519576551, 0.3153832671262227771 ) ) ;
#12230=CARTESIAN_POINT ( 'NONE',  ( 0.3543307086614179147, 0.2952755905511811885, 0.000000000000000000 ) ) ;
#12232=CARTESIAN_POINT ( 'NONE',  ( -0.8267716535433065062, -0.6692913385826771977, 8.415575281601705876E-17 ) ) ;
#12233=CARTESIAN_POINT ( 'NONE',  ( 0.7283464566929140904, -0.4536011799217368745, -0.2665933059059886201 ) ) ;
#12234=VECTOR ( 'NONE', #9699, 39.37007874015748143 ) ;
#12236=CARTESIAN_POINT ( 'NONE',  ( -0.1968503937007867743, -0.6692913385826771977, 8.415575281601705876E-17 ) ) ;
#12237=CARTESIAN_POINT ( 'NONE',  ( 0.2427821522309719648, -0.08942795157527998196, 0.3641732283464567121 ) ) ;
#12239=CARTESIAN_POINT ( 'NONE',  ( -0.2034120734908131112, -0.6692913385826773087, -0.1292274648535924053 ) ) ;
#12240=CARTESIAN_POINT ( 'NONE',  ( 0.3215223097112867578, -0.08942795157527998196, 0.3641732283464567121 ) ) ;
#12242=CARTESIAN_POINT ( 'NONE',  ( 0.3805774278215230400, -0.4281496062992124485, 0.4176697321401328655 ) ) ;
#12243=CARTESIAN_POINT ( 'NONE',  ( 0.9711286089238851948, -0.5023911411419708095, -0.1820866141732282451 ) ) ;
#12244=CARTESIAN_POINT ( 'NONE',  ( -0.1681795077207344780, 5.625543525484885637E-15, -0.4118477457932931962 ) ) ;
#12245=CARTESIAN_POINT ( 'NONE',  ( -0.5183727034120726440, -0.5511811023622048555, -0.09757992244046775898 ) ) ;
#12246=CARTESIAN_POINT ( 'NONE',  ( -0.5774278215223089816, 0.1283753931104746893, -0.1820866141732285504 ) ) ;
#12247=CARTESIAN_POINT ( 'NONE',  ( -0.2952755905511803003, -0.5400638737290845981, -0.3530559997133363437 ) ) ;
#12248=CARTESIAN_POINT ( 'NONE',  ( 5.463695987328526437E-16, -0.1870078740157479769, 0.4822834645669291653 ) ) ;
#12249=CARTESIAN_POINT ( 'NONE',  ( 1.069553805774278832, 0.1771653543307087075, -0.09757992244046823083 ) ) ;
#12250=CARTESIAN_POINT ( 'NONE',  ( -1.568241469816272105, -0.08942795157527998196, 0.3641732283464567121 ) ) ;
#12251=CARTESIAN_POINT ( 'NONE',  ( 1.561679790026247350, -0.3690944881889763329, 0.3153832671262228327 ) ) ;
#12252=CARTESIAN_POINT ( 'NONE',  ( 0.5643044619422579178, 0.05413385826771666132, 0.4176697321401328100 ) ) ;
#12254=CARTESIAN_POINT ( 'NONE',  ( -0.1509186351706028884, -0.05778040916215522460, 0.4822834645669289988 ) ) ;
#12256=CARTESIAN_POINT ( 'NONE',  ( 1.062992125984252745, 0.2952755905511811885, 0.000000000000000000 ) ) ;
#12257=CARTESIAN_POINT ( 'NONE',  ( 0.6102362204724416372, 0.1660481256975883668, -0.3530559997133364547 ) ) ;
#12258=CARTESIAN_POINT ( 'NONE',  ( -1.600415083108464254, 2.375314266909943406, -0.1324231768467337145 ) ) ;
#12259=CARTESIAN_POINT ( 'NONE',  ( 0.3018372703412079971, -0.004921259842519870586, -0.3153832671262229437 ) ) ;
#12260=CARTESIAN_POINT ( 'NONE',  ( 1.240157480314961314, 0.1660481256975883668, -0.3530559997133364547 ) ) ;
#12261=CARTESIAN_POINT ( 'NONE',  ( -0.1443569553805768291, -0.004921259842519576551, 0.3153832671262227771 ) ) ;
#12262=CARTESIAN_POINT ( 'NONE',  ( -0.1246719160104980823, -0.6692913385826773087, -0.1292274648535924053 ) ) ;
#12264=CARTESIAN_POINT ( 'NONE',  ( 0.4068241469816279987, -0.4281496062992127816, -0.4176697321401328100 ) ) ;
#12265=CARTESIAN_POINT ( 'NONE',  ( -0.8464566929133852113, 0.1660481256975885056, 0.3530559997133364547 ) ) ;
#12266=CARTESIAN_POINT ( 'NONE',  ( -0.4986876640419942164, -0.5023911411419708095, 0.1820866141732285504 ) ) ;
#12267=CARTESIAN_POINT ( 'NONE',  ( 0.3477690288713918276, 0.2952755905511811885, 0.1292274648535926551 ) ) ;
#12268=CARTESIAN_POINT ( 'NONE',  ( -1.351706036745406347, 0.05413385826771626580, -0.4176697321401330321 ) ) ;
#12269=CARTESIAN_POINT ( 'NONE',  ( -0.1706036745406816491, 0.05413385826771626580, -0.4176697321401330321 ) ) ;
#12272=CARTESIAN_POINT ( 'NONE',  ( 1.305774278215223960, 0.2952755905511810774, -0.1292274648535930714 ) ) ;
#12273=CARTESIAN_POINT ( 'NONE',  ( 1.364829396325460076, 0.2306618581243848609, 0.2411417322834645549 ) ) ;
#12275=CARTESIAN_POINT ( 'NONE',  ( -1.594488188976377119, 0.1660481256975883668, -0.3530559997133364547 ) ) ;
#12277=CARTESIAN_POINT ( 'NONE',  ( -0.7611548556430438595, 0.2306618581243848609, 0.2411417322834645549 ) ) ;
#12279=ADVANCED_FACE ( 'NONE', ( #81819 ), #15777, .F. ) ;
#12282=CARTESIAN_POINT ( 'NONE',  ( -0.2952755905511803003, -0.4536011799217368745, -0.2665933059059886201 ) ) ;
#12284=CARTESIAN_POINT ( 'NONE',  ( 0.6299212598425204535, -0.1870078740157479769, 0.4822834645669291653 ) ) ;
#12286=DIRECTION ( 'NONE',  ( 0.000000000000000000, 0.000000000000000000, -1.000000000000000000 ) ) ;
#12287=CARTESIAN_POINT ( 'NONE',  ( -0.6364829396325453192, -0.08942795157528024563, -0.3641732283464568787 ) ) ;
#12289=CARTESIAN_POINT ( 'NONE',  ( 1.023622047244095334, -0.1870078740157479769, 0.4822834645669291653 ) ) ;
#12290=CARTESIAN_POINT ( 'NONE',  ( 0.9383202099737536495, -0.2845877964562159024, 0.3641732283464567677 ) ) ;
#12291=CARTESIAN_POINT ( 'NONE',  ( 0.1968503937007881344, -0.6692913385826771977, 8.415575281601705876E-17 ) ) ;
#12293=CARTESIAN_POINT ( 'NONE',  ( -0.4068241469816264999, -0.4281496062992124485, 0.4176697321401328655 ) ) ;
#12294=CARTESIAN_POINT ( 'NONE',  ( -1.456692913385826182, -0.5511811023622047445, 6.969142054262312111E-17 ) ) ;
#12295=CARTESIAN_POINT ( 'NONE',  ( -0.5971128608923877978, 0.2952755905511811885, 0.1292274648535926551 ) ) ;
#12296=CARTESIAN_POINT ( 'NONE',  ( 1.653543307086614789, -0.1870078740157479769, 0.4822834645669291653 ) ) ;
#12300=CARTESIAN_POINT ( 'NONE',  ( 0.5577427821522316087, -0.05778040916215522460, 0.4822834645669289988 ) ) ;
#12301=ORIENTED_EDGE ( 'NONE', *, *, #22171, .T. ) ;
#12302=CARTESIAN_POINT ( 'NONE',  ( -0.9055118110236215490, 0.2952755905511811885, 0.000000000000000000 ) ) ;
#12303=CARTESIAN_POINT ( 'NONE',  ( -1.463254593175852492, 0.2952755905511811885, 0.1292274648535926551 ) ) ;
#12304=CARTESIAN_POINT ( 'NONE',  ( 0.8398950131233602345, 0.2306618581243847221, -0.2411417322834647770 ) ) ;
#12305=CARTESIAN_POINT ( 'NONE',  ( 0.2559055118110243332, 0.1660481256975885056, 0.3530559997133364547 ) ) ;
#12307=CARTESIAN_POINT ( 'NONE',  ( -0.7677165354330699465, 0.1660481256975885056, 0.3530559997133364547 ) ) ;
#12308=CARTESIAN_POINT ( 'NONE',  ( -0.2952755905511803003, -0.5400638737290845981, -0.3530559997133363437 ) ) ;
#12309=CARTESIAN_POINT ( 'NONE',  ( -1.017060367454067249, -0.05778040916215522460, 0.4822834645669289988 ) ) ;
#12310=CARTESIAN_POINT ( 'NONE',  ( -0.1902887139107604098, 0.1771653543307087075, -0.09757992244046823083 ) ) ;
#12312=CARTESIAN_POINT ( 'NONE',  ( -0.05905511811023545637, -0.5400638737290845981, -0.3530559997133363437 ) ) ;
#12313=FACE_OUTER_BOUND ( 'NONE', #81380, .T. ) ;
#12314=CARTESIAN_POINT ( 'NONE',  ( 1.299212598425197429, 0.2952755905511811885, 0.000000000000000000 ) ) ;
#12316=ORIENTED_EDGE ( 'NONE', *, *, #31050, .T. ) ;
#12318=CARTESIAN_POINT ( 'NONE',  ( 0.1771653543307093182, -0.5400638737290845981, -0.3530559997133363437 ) ) ;
#12319=CARTESIAN_POINT ( 'NONE',  ( -0.08530183727034056085, -0.08942795157528024563, -0.3641732283464568787 ) ) ;
#12320=CARTESIAN_POINT ( 'NONE',  ( 1.502624671916010790, -0.08942795157527998196, 0.3641732283464567121 ) ) ;
#12321=CARTESIAN_POINT ( 'NONE',  ( -1.646051170424378096, 0.000000000000000000, 0.3464511005275205946 ) ) ;
#12323=CARTESIAN_POINT ( 'NONE',  ( -0.9548908091195642545, -2.567464376874931580E-15, -0.4445507791589072832 ) ) ;
#12324=CARTESIAN_POINT ( 'NONE',  ( 0.7210809602247731931, 4.888820689338890882E-16, 0.3464511005275202615 ) ) ;
#12325=CARTESIAN_POINT ( 'NONE',  ( -1.548556430446193399, -0.6046776061558809534, -0.2411417322834644161 ) ) ;
#12327=CARTESIAN_POINT ( 'NONE',  ( 0.3477690288713918276, 0.2952755905511811885, 0.1292274648535926551 ) ) ;
#12328=CARTESIAN_POINT ( 'NONE',  ( -1.325459317585300889, 0.05413385826771666132, 0.4176697321401328100 ) ) ;
#12329=CARTESIAN_POINT ( 'NONE',  ( -1.174540682414697335, -0.3162353388693409650, -0.4822834645669289433 ) ) ;
#12330=CARTESIAN_POINT ( 'NONE',  ( 0.05249343832021075018, 0.2306618581243847221, -0.2411417322834647770 ) ) ;
#12332=CARTESIAN_POINT ( 'NONE',  ( 0.9645669291338588858, 0.1660481256975885056, 0.3530559997133364547 ) ) ;
#12333=CARTESIAN_POINT ( 'NONE',  ( 1.423884514435696413, -0.2845877964562161244, -0.3641732283464567121 ) ) ;
#12335=CARTESIAN_POINT ( 'NONE',  ( 0.8923884514435703741, 0.1283753931104748280, 0.1820866141732283561 ) ) ;
#12336=CARTESIAN_POINT ( 'NONE',  ( -0.8923884514435688198, -0.6046776061558807314, 0.2411417322834647770 ) ) ;
#12338=CARTESIAN_POINT ( 'NONE',  ( 1.653543307086614789, -0.1870078740157479769, 0.4822834645669291653 ) ) ;
#12340=CARTESIAN_POINT ( 'NONE',  ( 0.8005249343832028242, -0.4281496062992127816, -0.4176697321401328100 ) ) ;
#12342=CARTESIAN_POINT ( 'NONE',  ( -1.732283464566928277, -0.1870078740157479769, 0.3641732283464567677 ) ) ;
#12343=CARTESIAN_POINT ( 'NONE',  ( -0.05249343832020911260, 0.2306618581243848609, 0.2411417322834645549 ) ) ;
#12344=CARTESIAN_POINT ( 'NONE',  ( 1.017060367454068581, -0.08942795157528024563, -0.3641732283464568787 ) ) ;
#12345=CARTESIAN_POINT ( 'NONE',  ( -1.561679790026246017, -0.004921259842519576551, 0.3153832671262227771 ) ) ;
#12346=CARTESIAN_POINT ( 'NONE',  ( 0.8267716535433078384, -0.6692913385826771977, 8.415575281601705876E-17 ) ) ;
#12347=CARTESIAN_POINT ( 'NONE',  ( 1.614173228346456712, 2.401574803149606474, -0.1372047244094476703 ) ) ;
#12348=CARTESIAN_POINT ( 'NONE',  ( -0.3477690288713905509, -0.5511811023622046335, 0.09757992244046803654 ) ) ;
#12349=CARTESIAN_POINT ( 'NONE',  ( -0.5446194225721777693, -0.3162353388693409650, -0.4822834645669289433 ) ) ;
#12350=CARTESIAN_POINT ( 'NONE',  ( -1.561679790026246017, -0.3690944881889765550, -0.3153832671262227771 ) ) ;
#12351=CARTESIAN_POINT ( 'NONE',  ( -1.345144356955379816, -0.05778040916215560624, -0.4822834645669293319 ) ) ;
#12352=CARTESIAN_POINT ( 'NONE',  ( 1.240157480314961314, 0.1660481256975883668, -0.3530559997133364547 ) ) ;
#12354=CARTESIAN_POINT ( 'NONE',  ( -1.417322834645668772, -0.1870078740157480601, -0.3641732283464567677 ) ) ;
#12356=CARTESIAN_POINT ( 'NONE',  ( 0.8267716535433077274, 0.2952755905511811885, 0.000000000000000000 ) ) ;
#12358=CARTESIAN_POINT ( 'NONE',  ( -1.607611548556429737, -0.6692913385826771977, 0.1292274648535927661 ) ) ;
#12359=CARTESIAN_POINT ( 'NONE',  ( -1.410761154855641575, -0.2845877964562161244, -0.3641732283464567121 ) ) ;
#12360=CARTESIAN_POINT ( 'NONE',  ( -0.8333333333333323711, -0.5511811023622048555, -0.09757992244046775898 ) ) ;
#12361=CARTESIAN_POINT ( 'NONE',  ( 1.673228346456693494, 0.07958543189024085140, 0.2665933059059887866 ) ) ;
#12362=CARTESIAN_POINT ( 'NONE',  ( -0.3149606299212590610, -0.1870078740157480879, -0.4822834645669291653 ) ) ;
#12363=CARTESIAN_POINT ( 'NONE',  ( -0.1640419947506553400, -0.08942795157528024563, -0.3641732283464568787 ) ) ;
#12364=CARTESIAN_POINT ( 'NONE',  ( -1.712598425196849572, 0.07958543189024085140, 0.2665933059059887866 ) ) ;
#12365=CARTESIAN_POINT ( 'NONE',  ( 1.135170603674541256, 0.1771653543307087630, 0.09757992244046791164 ) ) ;
#12366=CARTESIAN_POINT ( 'NONE',  ( 1.135170603674541256, -0.6692913385826773087, -0.1292274648535924053 ) ) ;
#12367=CARTESIAN_POINT ( 'NONE',  ( 1.476377952755906220, 0.1660481256975883668, -0.3530559997133364547 ) ) ;
#12368=CARTESIAN_POINT ( 'NONE',  ( 0.1640419947506569498, -0.2845877964562161244, -0.3641732283464567121 ) ) ;
#12369=CARTESIAN_POINT ( 'NONE',  ( 0.4790026246719168435, -0.3162353388693409650, -0.4822834645669289433 ) ) ;
#12370=CARTESIAN_POINT ( 'NONE',  ( 0.3871391076115492380, -0.08942795157528024563, -0.3641732283464568787 ) ) ;
#12371=CARTESIAN_POINT ( 'NONE',  ( -1.640419947506561060, 0.05413385826771666132, 0.4176697321401328100 ) ) ;
#12373=CARTESIAN_POINT ( 'NONE',  ( -1.220472440944881054, -0.6692913385826771977, 8.415575281601705876E-17 ) ) ;
#12374=CARTESIAN_POINT ( 'NONE',  ( -0.3346456692913377662, -0.5400638737290844871, 0.3530559997133364547 ) ) ;
#12377=CARTESIAN_POINT ( 'NONE',  ( 0.3018372703412079971, -0.4281496062992124485, 0.4176697321401328655 ) ) ;
#12378=CARTESIAN_POINT ( 'NONE',  ( 0.9908136482939640111, 0.1771653543307087075, -0.09757992244046823083 ) ) ;
#12379=CARTESIAN_POINT ( 'NONE',  ( -0.4068241469816264999, -0.4281496062992124485, 0.4176697321401328655 ) ) ;
#12380=CARTESIAN_POINT ( 'NONE',  ( 0.2690288713910767848, -0.6692913385826773087, -0.1292274648535924053 ) ) ;
#12386=CARTESIAN_POINT ( 'NONE',  ( -0.6889763779527552368, -0.4536011799217368745, -0.2665933059059886201 ) ) ;
#12387=CARTESIAN_POINT ( 'NONE',  ( -1.003937007874015297, -0.5400638737290845981, -0.3530559997133363437 ) ) ;
#12390=CARTESIAN_POINT ( 'NONE',  ( 0.6561679790026253567, -0.6046776061558809534, -0.2411417322834644161 ) ) ;
#12391=CARTESIAN_POINT ( 'NONE',  ( 1.220472440944882386, -0.6692913385826771977, 8.415575281601705876E-17 ) ) ;
#12392=CARTESIAN_POINT ( 'NONE',  ( 0.9645669291338588858, 0.1660481256975885056, 0.3530559997133364547 ) ) ;
#12395=CARTESIAN_POINT ( 'NONE',  ( 1.601049868766404982, -0.6046776061558809534, -0.2411417322834644161 ) ) ;
#12396=CARTESIAN_POINT ( 'NONE',  ( 0.9776902887139113929, 0.2952755905511811885, 0.1292274648535926551 ) ) ;
#12397=CARTESIAN_POINT ( 'NONE',  ( 0.7480314960629927956, -0.6692913385826771977, 8.415575281601705876E-17 ) ) ;
#12398=CARTESIAN_POINT ( 'NONE',  ( 0.7086614173228352742, -0.1870078740157480601, -0.3641732283464567677 ) ) ;
#12399=CARTESIAN_POINT ( 'NONE',  ( 1.122047244094488860, -0.5400638737290845981, -0.3530559997133363437 ) ) ;
#12401=CARTESIAN_POINT ( 'NONE',  ( 0.5183727034120741983, 0.2952755905511810774, -0.1292274648535930714 ) ) ;
#12402=CARTESIAN_POINT ( 'NONE',  ( 1.135170603674541256, -0.6692913385826773087, -0.1292274648535924053 ) ) ;
#12403=CARTESIAN_POINT ( 'NONE',  ( 0.4068241469816281097, 0.05413385826771666132, 0.4176697321401328100 ) ) ;
#12404=CARTESIAN_POINT ( 'NONE',  ( 1.410761154855643795, -0.08942795157528024563, -0.3641732283464568787 ) ) ;
#12405=CARTESIAN_POINT ( 'NONE',  ( -0.8005249343832013809, -0.4281496062992124485, 0.4176697321401328655 ) ) ;
#12406=CARTESIAN_POINT ( 'NONE',  ( -1.187664041994750175, -0.05778040916215560624, -0.4822834645669293319 ) ) ;
#12407=CARTESIAN_POINT ( 'NONE',  ( 1.246719160104987623, -0.4281496062992124485, 0.4176697321401328655 ) ) ;
#12413=ORIENTED_EDGE ( 'NONE', *, *, #12082, .F. ) ;
#12414=CARTESIAN_POINT ( 'NONE',  ( 1.614173228346457378, -0.6692913385826771977, 8.415575281601705876E-17 ) ) ;
#12415=CARTESIAN_POINT ( 'NONE',  ( 1.541994750656168645, -0.5511811023622046335, 0.09757992244046803654 ) ) ;
#12417=CARTESIAN_POINT ( 'NONE',  ( 1.404199475065617708, -0.004921259842519870586, -0.3153832671262229437 ) ) ;
#12419=CONICAL_SURFACE ( 'NONE', #22562, 1.220472440944881942, 0.7853981633974621568 ) ;
#12423=CARTESIAN_POINT ( 'NONE',  ( -0.9448818897637790704, -0.1870078740157480601, -0.3641732283464567677 ) ) ;
#12424=CARTESIAN_POINT ( 'NONE',  ( -1.679790026246718693, 0.1283753931104746893, -0.1820866141732285504 ) ) ;
#12425=CARTESIAN_POINT ( 'NONE',  ( -1.358267716535432434, -0.5400638737290844871, 0.3530559997133364547 ) ) ;
#12426=CARTESIAN_POINT ( 'NONE',  ( 0.07217847769028949700, -0.05778040916215560624, -0.4822834645669293319 ) ) ;
#12427=CARTESIAN_POINT ( 'NONE',  ( 1.338582677165355062, -0.1870078740157480879, -0.4822834645669291653 ) ) ;
#12429=CARTESIAN_POINT ( 'NONE',  ( -1.168682819302786058, -2.294479370626195693E-15, 0.3464511005275217603 ) ) ;
#12432=CARTESIAN_POINT ( 'NONE',  ( -0.6036745406824141069, -0.5023911411419708095, -0.1820866141732282451 ) ) ;
#12433=CARTESIAN_POINT ( 'NONE',  ( -0.9973753280839886548, 0.2306618581243848609, 0.2411417322834645549 ) ) ;
#12434=CARTESIAN_POINT ( 'NONE',  ( 0.9973753280839902091, -0.6046776061558807314, 0.2411417322834647770 ) ) ;
#12437=CARTESIAN_POINT ( 'NONE',  ( -1.604771003085130543, 0.7690346235818137366, 0.1466069496707740338 ) ) ;
#12438=CARTESIAN_POINT ( 'NONE',  ( 1.259842519685040019, -0.1870078740157480879, -0.4822834645669291653 ) ) ;
#12439=CARTESIAN_POINT ( 'NONE',  ( -1.253280839895012377, -0.05778040916215522460, 0.4822834645669289988 ) ) ;
#12442=CARTESIAN_POINT ( 'NONE',  ( -0.4855643044619415427, -0.3690944881889763329, 0.3153832671262228327 ) ) ;
#12444=CARTESIAN_POINT ( 'NONE',  ( -0.5971128608923877978, -0.5511811023622048555, -0.09757992244046775898 ) ) ;
#12445=CARTESIAN_POINT ( 'NONE',  ( 0.4461942257217855201, -0.5023911411419708095, 0.1820866141732285504 ) ) ;
#12446=CARTESIAN_POINT ( 'NONE',  ( 0.2362204724409456558, -0.1870078740157480879, -0.4822834645669291653 ) ) ;
#12447=CARTESIAN_POINT ( 'NONE',  ( -0.8136482939632537770, 0.1283753931104746893, -0.1820866141732285504 ) ) ;
#12449=CARTESIAN_POINT ( 'NONE',  ( 0.9514435695538062676, -0.05778040916215522460, 0.4822834645669289988 ) ) ;
#12450=CARTESIAN_POINT ( 'NONE',  ( -1.325459317585300889, 0.05413385826771666132, 0.4176697321401328100 ) ) ;
#12452=CARTESIAN_POINT ( 'NONE',  ( -0.2755905511811018171, 0.2952755905511811885, 0.000000000000000000 ) ) ;
#12453=CARTESIAN_POINT ( 'NONE',  ( -0.7414698162729651543, -0.6692913385826771977, 0.1292274648535927661 ) ) ;
#12454=CARTESIAN_POINT ( 'NONE',  ( 1.423884514435696413, -0.2845877964562161244, -0.3641732283464567121 ) ) ;
#12455=CARTESIAN_POINT ( 'NONE',  ( -0.1574803149606292529, -0.1870078740157479769, 0.3641732283464567677 ) ) ;
#12456=CARTESIAN_POINT ( 'NONE',  ( -0.7939632545931754048, -0.3162353388693405765, 0.4822834645669290543 ) ) ;
#12457=CARTESIAN_POINT ( 'NONE',  ( -1.076115485564303809, -0.6046776061558809534, -0.2411417322834644161 ) ) ;
#12459=CARTESIAN_POINT ( 'NONE',  ( 1.364829396325460076, 0.1283753931104748280, 0.1820866141732283561 ) ) ;
#12460=CARTESIAN_POINT ( 'NONE',  ( -0.3018372703412066094, -0.4281496062992127816, -0.4176697321401328100 ) ) ;
#12461=CARTESIAN_POINT ( 'NONE',  ( -1.023622047244094002, -0.1870078740157480879, -0.4822834645669291653 ) ) ;
#12462=ORIENTED_EDGE ( 'NONE', *, *, #47715, .T. ) ;
#12464=CARTESIAN_POINT ( 'NONE',  ( -0.6824146981627288167, 0.1283753931104748280, 0.1820866141732283561 ) ) ;
#12465=CARTESIAN_POINT ( 'NONE',  ( 1.194225721784777594, -0.4281496062992127816, -0.4176697321401328100 ) ) ;
#12466=CARTESIAN_POINT ( 'NONE',  ( -0.8792650918635160906, -0.004921259842519870586, -0.3153832671262229437 ) ) ;
#12468=CARTESIAN_POINT ( 'NONE',  ( -0.9514435695538050464, -0.3162353388693405765, 0.4822834645669290543 ) ) ;
#12469=CARTESIAN_POINT ( 'NONE',  ( 1.049868766404200349, 0.2306618581243848609, 0.2411417322834645549 ) ) ;
#12470=CARTESIAN_POINT ( 'NONE',  ( 0.9842519685039378130, -0.6692913385826771977, 8.415575281601705876E-17 ) ) ;
#12472=CARTESIAN_POINT ( 'NONE',  ( -1.397637795275589623, 0.07958543189024085140, 0.2665933059059887866 ) ) ;
#12477=CARTESIAN_POINT ( 'NONE',  ( 1.253280839895013710, -0.08942795157528024563, -0.3641732283464568787 ) ) ;
#12478=CARTESIAN_POINT ( 'NONE',  ( 0.6824146981627303710, 0.1283753931104746893, -0.1820866141732285504 ) ) ;
#12479=CARTESIAN_POINT ( 'NONE',  ( 0.6561679790026253567, 0.2306618581243848609, 0.2411417322834645549 ) ) ;
#12480=CARTESIAN_POINT ( 'NONE',  ( 1.607611548556431069, 0.2952755905511811885, 0.1292274648535926551 ) ) ;
#12482=CARTESIAN_POINT ( 'NONE',  ( 0.6627296587926517768, -0.5511811023622048555, -0.09757992244046775898 ) ) ;
#12483=CARTESIAN_POINT ( 'NONE',  ( -0.4724409448818890911, -0.1870078740157480879, -0.4822834645669291653 ) ) ;
#12484=CARTESIAN_POINT ( 'NONE',  ( -1.030183727034119867, -0.3162353388693405765, 0.4822834645669290543 ) ) ;
#12485=CARTESIAN_POINT ( 'NONE',  ( 0.8267716535433078384, -0.6692913385826771977, 8.415575281601705876E-17 ) ) ;
#12488=ORIENTED_EDGE ( 'NONE', *, *, #73660, .F. ) ;
#12490=VECTOR ( 'NONE', #60809, 39.37007874015748143 ) ;
#12491=CARTESIAN_POINT ( 'NONE',  ( -1.207349081364828880, 0.2306618581243847221, -0.2411417322834647770 ) ) ;
#12492=CARTESIAN_POINT ( 'NONE',  ( -0.7020997375328074108, -0.05778040916215522460, 0.4822834645669289988 ) ) ;
#12493=CARTESIAN_POINT ( 'NONE',  ( -0.8136482939632537770, 0.1283753931104746893, -0.1820866141732285504 ) ) ;
#12494=CARTESIAN_POINT ( 'NONE',  ( -0.8858267716535425107, -0.5400638737290844871, 0.3530559997133364547 ) ) ;
#12496=CARTESIAN_POINT ( 'NONE',  ( 0.5314960629921267055, -0.5400638737290844871, 0.3530559997133364547 ) ) ;
#12497=CARTESIAN_POINT ( 'NONE',  ( -0.3674540682414689785, 0.2306618581243848609, 0.2411417322834645549 ) ) ;
#12498=CARTESIAN_POINT ( 'NONE',  ( 1.587926509186352142, 0.05413385826771666132, 0.4176697321401328100 ) ) ;
#12499=CARTESIAN_POINT ( 'NONE',  ( -0.8136482939632537770, -0.6046776061558807314, 0.2411417322834647770 ) ) ;
#12500=CARTESIAN_POINT ( 'NONE',  ( 0.3608923884514443348, 0.2952755905511810774, -0.1292274648535930714 ) ) ;
#12501=ADVANCED_FACE ( 'NONE', ( #23720 ), #74259, .T. ) ;
#12504=CARTESIAN_POINT ( 'NONE',  ( -0.9842519685039360366, 0.1771653543307087630, 0.000000000000000000 ) ) ;
#12505=EDGE_LOOP ( 'NONE', ( #52785, #23977, #23496, #42750 ) ) ;
#12508=CARTESIAN_POINT ( 'NONE',  ( -1.135170603674539924, -0.5511811023622046335, 0.09757992244046803654 ) ) ;
#12509=CARTESIAN_POINT ( 'NONE',  ( -1.122047244094487306, 0.1660481256975883668, -0.3530559997133364547 ) ) ;
#12510=CARTESIAN_POINT ( 'NONE',  ( -0.7545931758530176614, -0.6692913385826773087, -0.1292274648535924053 ) ) ;
#12512=CARTESIAN_POINT ( 'NONE',  ( -1.036745406824146176, 0.05413385826771626580, -0.4176697321401330321 ) ) ;
#12513=CARTESIAN_POINT ( 'NONE',  ( -1.227034120734907585, 0.2952755905511811885, 0.1292274648535926551 ) ) ;
#12514=CARTESIAN_POINT ( 'NONE',  ( -1.568241469816272105, -0.3162353388693409650, -0.4822834645669289433 ) ) ;
#12516=CARTESIAN_POINT ( 'NONE',  ( 0.6955380577427828781, -0.3690944881889763329, 0.3153832671262228327 ) ) ;
#12519=CARTESIAN_POINT ( 'NONE',  ( -0.4658792650918627265, -0.08942795157527998196, 0.3641732283464567121 ) ) ;
#12520=CARTESIAN_POINT ( 'NONE',  ( -0.1837270341207340729, 0.2306618581243847221, -0.2411417322834647770 ) ) ;
#12521=CARTESIAN_POINT ( 'NONE',  ( 1.509186351706037543, -0.4281496062992127816, -0.4176697321401328100 ) ) ;
#12522=CARTESIAN_POINT ( 'NONE',  ( -0.4986876640419939388, 0.2306618581243847221, -0.2411417322834647770 ) ) ;
#12526=CARTESIAN_POINT ( 'NONE',  ( -0.4724409448818890911, -0.1870078740157480879, -0.4822834645669291653 ) ) ;
#12527=CARTESIAN_POINT ( 'NONE',  ( 1.456692913385827515, 0.2952755905511811885, 0.000000000000000000 ) ) ;
#12528=CARTESIAN_POINT ( 'NONE',  ( -1.108923884514435132, -0.2845877964562159024, 0.3641732283464567677 ) ) ;
#12529=CARTESIAN_POINT ( 'NONE',  ( -1.312335958005248715, -0.6046776061558809534, -0.2411417322834644161 ) ) ;
#12532=EDGE_CURVE ( 'NONE', #12831, #11346, #16600, .T. ) ;
#12534=CARTESIAN_POINT ( 'NONE',  ( 1.581364829396326277, -0.05778040916215522460, 0.4822834645669289988 ) ) ;
#12536=CARTESIAN_POINT ( 'NONE',  ( -0.01968503937007793844, 0.1660481256975883668, -0.3530559997133364547 ) ) ;
#12537=CARTESIAN_POINT ( 'NONE',  ( -1.161417322834644716, 0.07958543189024085140, 0.2665933059059887866 ) ) ;
#12538=CARTESIAN_POINT ( 'NONE',  ( -0.3871391076115479057, -0.3162353388693409650, -0.4822834645669289433 ) ) ;
#12541=CARTESIAN_POINT ( 'NONE',  ( -0.7939632545931754048, -0.3162353388693405765, 0.4822834645669290543 ) ) ;
#12542=CARTESIAN_POINT ( 'NONE',  ( -0.9251968503937002541, 0.1660481256975885056, 0.3530559997133364547 ) ) ;
#12544=CARTESIAN_POINT ( 'NONE',  ( 1.049868766404200127, -0.5023911411419708095, -0.1820866141732282451 ) ) ;
#12545=CARTESIAN_POINT ( 'NONE',  ( -0.8923884514435688198, 0.1283753931104746893, -0.1820866141732285504 ) ) ;
#12547=CARTESIAN_POINT ( 'NONE',  ( 0.8989501312335964611, 0.1771653543307087630, 0.09757992244046791164 ) ) ;
#12548=CARTESIAN_POINT ( 'NONE',  ( -1.620734908136482577, -0.6692913385826773087, -0.1292274648535924053 ) ) ;
#12549=CARTESIAN_POINT ( 'NONE',  ( 1.417322834645670104, -0.1870078740157479769, 0.4822834645669291653 ) ) ;
#12550=CARTESIAN_POINT ( 'NONE',  ( 0.7086614173228353852, -0.1870078740157479769, 0.3641732283464567677 ) ) ;
#12551=CARTESIAN_POINT ( 'NONE',  ( -0.7152230971128602510, -0.3162353388693405765, 0.4822834645669290543 ) ) ;
#12552=CARTESIAN_POINT ( 'NONE',  ( 1.154855643044620184, 0.2306618581243847221, -0.2411417322834647770 ) ) ;
#12554=CARTESIAN_POINT ( 'NONE',  ( -0.2296587926509179312, -0.08942795157527998196, 0.3641732283464567121 ) ) ;
#12556=CARTESIAN_POINT ( 'NONE',  ( 0.3018372703412079971, 0.05413385826771626580, -0.4176697321401330321 ) ) ;
#12557=CARTESIAN_POINT ( 'NONE',  ( 0.6889763779527563470, 0.1660481256975883391, -0.3530559997133364547 ) ) ;
#12559=CARTESIAN_POINT ( 'NONE',  ( 0.9448818897637802916, -0.1870078740157479769, 0.3641732283464567677 ) ) ;
#12560=CARTESIAN_POINT ( 'NONE',  ( 0.2690288713910767848, -0.5511811023622048555, -0.09757992244046775898 ) ) ;
#12561=CARTESIAN_POINT ( 'NONE',  ( -0.05249343832020911260, 0.2306618581243848609, 0.2411417322834645549 ) ) ;
#12562=CARTESIAN_POINT ( 'NONE',  ( -1.555118110236219930, 0.1660481256975885056, 0.3530559997133364547 ) ) ;
#12563=CARTESIAN_POINT ( 'NONE',  ( -0.6430446194225712953, -0.004921259842519870586, -0.3153832671262229437 ) ) ;
#12565=CARTESIAN_POINT ( 'NONE',  ( -0.6692913385826764205, 0.2952755905511811885, 0.000000000000000000 ) ) ;
#12568=CARTESIAN_POINT ( 'NONE',  ( 0.1312335958005255154, -0.5023911411419708095, 0.1820866141732285504 ) ) ;
#12569=CARTESIAN_POINT ( 'NONE',  ( -0.4396325459317577122, -0.6692913385826773087, -0.1292274648535924053 ) ) ;
#12570=CARTESIAN_POINT ( 'NONE',  ( -0.9514435695538050464, -0.05778040916215560624, -0.4822834645669293319 ) ) ;
#12571=CARTESIAN_POINT ( 'NONE',  ( -0.9383202099737524282, -0.2845877964562161244, -0.3641732283464567121 ) ) ;
#12573=EDGE_CURVE ( 'NONE', #23460, #58699, #31796, .T. ) ;
#12574=CARTESIAN_POINT ( 'NONE',  ( -0.1246719160104980823, -0.6692913385826773087, -0.1292274648535924053 ) ) ;
#12575=CARTESIAN_POINT ( 'NONE',  ( -1.502624671916009680, -0.08942795157528024563, -0.3641732283464568787 ) ) ;
#12576=CARTESIAN_POINT ( 'NONE',  ( 1.292650918635171564, 0.2952755905511811885, 0.1292274648535926551 ) ) ;
#12581=CARTESIAN_POINT ( 'NONE',  ( -1.456692913385826182, -0.6692913385826771977, 8.415575281601705876E-17 ) ) ;
#12582=CARTESIAN_POINT ( 'NONE',  ( -0.9908136482939626788, -0.6692913385826773087, -0.1292274648535924053 ) ) ;
#12583=EDGE_CURVE ( 'NONE', #36535, #11377, #52713, .T. ) ;
#12584=CARTESIAN_POINT ( 'NONE',  ( -1.541994750656167090, -0.6692913385826773087, -0.1292274648535924053 ) ) ;
#12587=CARTESIAN_POINT ( 'NONE',  ( 0.8398950131233602345, -0.6046776061558807314, 0.2411417322834647770 ) ) ;
#12588=CARTESIAN_POINT ( 'NONE',  ( 0.04593175853018440641, -0.6692913385826771977, 0.1292274648535927661 ) ) ;
#12589=CARTESIAN_POINT ( 'NONE',  ( 0.4600214019799526155, 2.784432375088962958E-17, -0.3464511005275205946 ) ) ;
#12591=CARTESIAN_POINT ( 'NONE',  ( 1.325459317585302665, -0.004921259842519870586, -0.3153832671262229437 ) ) ;
#12596=CARTESIAN_POINT ( 'NONE',  ( -0.1640419947506555343, -0.3162353388693405765, 0.4822834645669290543 ) ) ;
#12597=CARTESIAN_POINT ( 'NONE',  ( -0.7020997375328076329, -0.3162353388693409650, -0.4822834645669289433 ) ) ;
#12598=CARTESIAN_POINT ( 'NONE',  ( -1.633858267716534529, 0.1660481256975885056, 0.3530559997133364547 ) ) ;
#12599=CARTESIAN_POINT ( 'NONE',  ( 0.4658792650918641698, -0.05778040916215560624, -0.4822834645669293319 ) ) ;
#12601=CARTESIAN_POINT ( 'NONE',  ( 1.607611548556431069, -0.6692913385826773087, -0.1292274648535924053 ) ) ;
#12602=CARTESIAN_POINT ( 'NONE',  ( 1.509186351706037543, -0.4281496062992127816, -0.4176697321401328100 ) ) ;
#12603=CARTESIAN_POINT ( 'NONE',  ( -0.05905511811023545637, 0.1660481256975885056, 0.3530559997133364547 ) ) ;
#12604=CARTESIAN_POINT ( 'NONE',  ( -1.318897637795274802, 0.1660481256975885056, 0.3530559997133364547 ) ) ;
#12605=CARTESIAN_POINT ( 'NONE',  ( 1.135170603674541256, 0.2952755905511811885, 0.1292274648535926551 ) ) ;
#12606=CARTESIAN_POINT ( 'NONE',  ( 1.594488188976378673, -0.5400638737290845981, -0.3530559997133363437 ) ) ;
#12607=CARTESIAN_POINT ( 'NONE',  ( -0.04593175853018302557, -0.6692913385826773087, -0.1292274648535924053 ) ) ;
#12609=CARTESIAN_POINT ( 'NONE',  ( 0.4199475065616805614, 0.1283753931104748280, 0.1820866141732283561 ) ) ;
#12612=EDGE_LOOP ( 'NONE', ( #10729, #35292, #78563, #68792, #17278, #4126, #53409, #82299 ) ) ;
#12613=CARTESIAN_POINT ( 'NONE',  ( -0.02624671916010428221, -0.5023911411419708095, 0.1820866141732285504 ) ) ;
#12615=CARTESIAN_POINT ( 'NONE',  ( -0.01312335958005186876, -0.4281496062992124485, 0.4176697321401328655 ) ) ;
#12616=CARTESIAN_POINT ( 'NONE',  ( -0.1246719160104980823, 0.2952755905511811885, 0.1292274648535926551 ) ) ;
#12617=CARTESIAN_POINT ( 'NONE',  ( -0.7611548556430438595, 0.2306618581243848609, 0.2411417322834645549 ) ) ;
#12620=CARTESIAN_POINT ( 'NONE',  ( -1.148293963254592542, 0.2952755905511811885, 0.1292274648535926551 ) ) ;
#12622=CARTESIAN_POINT ( 'NONE',  ( 1.423884514435696191, -0.08942795157527998196, 0.3641732283464567121 ) ) ;
#12623=CARTESIAN_POINT ( 'NONE',  ( 1.030183727034121421, -0.05778040916215522460, 0.4822834645669289988 ) ) ;
#12624=CARTESIAN_POINT ( 'NONE',  ( 0.9383202099737538715, -0.05778040916215560624, -0.4822834645669293319 ) ) ;
#12626=CARTESIAN_POINT ( 'NONE',  ( -1.233595800524933894, 0.2306618581243848609, 0.2411417322834645549 ) ) ;
#12629=CARTESIAN_POINT ( 'NONE',  ( -0.2821522309711278487, 0.2952755905511811885, 0.1292274648535926551 ) ) ;
#12632=CARTESIAN_POINT ( 'NONE',  ( 1.456692913385827515, 0.2952755905511811885, 0.000000000000000000 ) ) ;
#12633=CARTESIAN_POINT ( 'NONE',  ( 1.318897637795276356, -0.5400638737290844871, 0.3530559997133364547 ) ) ;
#12634=CARTESIAN_POINT ( 'NONE',  ( 0.3477690288713918276, -0.5511811023622048555, -0.09757992244046775898 ) ) ;
#12635=CARTESIAN_POINT ( 'NONE',  ( 1.108923884514436242, -0.05778040916215522460, 0.4822834645669289988 ) ) ;
#12637=CARTESIAN_POINT ( 'NONE',  ( 0.5446194225721792126, -0.2845877964562159024, 0.3641732283464567677 ) ) ;
#12638=CARTESIAN_POINT ( 'NONE',  ( 0.5643044619422579178, -0.4281496062992127816, -0.4176697321401328100 ) ) ;
#12640=CARTESIAN_POINT ( 'NONE',  ( -1.036745406824146176, 0.05413385826771626580, -0.4176697321401330321 ) ) ;
#12641=CARTESIAN_POINT ( 'NONE',  ( 1.010498687664042716, -0.004921259842519870586, -0.3153832671262229437 ) ) ;
#12643=CARTESIAN_POINT ( 'NONE',  ( -0.4396325459317579898, 0.2952755905511811885, 0.1292274648535926551 ) ) ;
#12644=CARTESIAN_POINT ( 'NONE',  ( -0.1246719160104980823, -0.5511811023622048555, -0.09757992244046775898 ) ) ;
#12645=CARTESIAN_POINT ( 'NONE',  ( 0.4581548244795011215, 1.775897344681688805, 0.5309055118110234117 ) ) ;
#12646=CARTESIAN_POINT ( 'NONE',  ( -0.2690288713910754526, 0.2952755905511810774, -0.1292274648535930714 ) ) ;
#12647=CARTESIAN_POINT ( 'NONE',  ( 0.5183727034120741983, 0.1771653543307087075, -0.09757992244046823083 ) ) ;
#12648=B_SPLINE_CURVE_WITH_KNOTS ( 'NONE', 3,
 ( #3173, #80214, #28837, #67569 ),
 .UNSPECIFIED., .F., .F.,
 ( 4, 4 ),
 ( 3.210432057656183116E-07, 0.001287787053612039377 ),
 .UNSPECIFIED. ) ;
#12650=CARTESIAN_POINT ( 'NONE',  ( 0.1246719160104994284, 0.2952755905511810774, -0.1292274648535930714 ) ) ;
#12652=CARTESIAN_POINT ( 'NONE',  ( 1.279527559055118724, -0.4536011799217368745, -0.2665933059059886201 ) ) ;
#12653=CARTESIAN_POINT ( 'NONE',  ( 0.3830016109920622025, 1.809133623825372073E-16, -0.4118484887281974038 ) ) ;
#12654=CARTESIAN_POINT ( 'NONE',  ( -0.9580052493438311334, -0.3690944881889763329, 0.3153832671262228327 ) ) ;
#12656=CARTESIAN_POINT ( 'NONE',  ( -0.7152230971128602510, -0.08942795157528024563, -0.3641732283464568787 ) ) ;
#12657=CARTESIAN_POINT ( 'NONE',  ( -0.1181102362204717315, -0.6692913385826771977, 8.415575281601705876E-17 ) ) ;
#12658=CARTESIAN_POINT ( 'NONE',  ( -0.2755905511811018171, 0.2952755905511811885, 0.000000000000000000 ) ) ;
#12659=CARTESIAN_POINT ( 'NONE',  ( 0.4068241469816281097, -0.004921259842519576551, 0.3153832671262227771 ) ) ;
#12660=CARTESIAN_POINT ( 'NONE',  ( -1.587926509186350810, -0.3690944881889763329, 0.3153832671262228327 ) ) ;
#12661=CARTESIAN_POINT ( 'NONE',  ( -1.725721784776902190, -0.05778040916215522460, 0.4822834645669289988 ) ) ;
#12664=CARTESIAN_POINT ( 'NONE',  ( 0.7545931758530189937, 0.2952755905511810774, -0.1292274648535930714 ) ) ;
#12666=CARTESIAN_POINT ( 'NONE',  ( -0.1181102362204717315, 0.2952755905511811885, 0.000000000000000000 ) ) ;
#12668=CARTESIAN_POINT ( 'NONE',  ( -1.469816272965878357, -0.6046776061558809534, -0.2411417322834644161 ) ) ;
#12669=CARTESIAN_POINT ( 'NONE',  ( 1.076115485564305141, 0.2306618581243847221, -0.2411417322834647770 ) ) ;
#12670=CARTESIAN_POINT ( 'NONE',  ( 0.7480314960629927956, 0.2952755905511811885, 0.000000000000000000 ) ) ;
#12671=DIRECTION ( 'NONE',  ( 0.000000000000000000, 0.000000000000000000, 1.000000000000000000 ) ) ;
#12672=CARTESIAN_POINT ( 'NONE',  ( 0.1902887139107617975, -0.5511811023622048555, -0.09757992244046775898 ) ) ;
#12673=CARTESIAN_POINT ( 'NONE',  ( 1.371391076115485941, 0.2952755905511811885, 0.1292274648535926551 ) ) ;
#12674=CARTESIAN_POINT ( 'NONE',  ( -0.2099737532808391705, -0.5023911411419708095, -0.1820866141732282451 ) ) ;
#12676=CARTESIAN_POINT ( 'NONE',  ( -0.5446194225721777693, -0.05778040916215522460, 0.4822834645669289988 ) ) ;
#12678=CARTESIAN_POINT ( 'NONE',  ( 0.09186351706036799403, -0.4281496062992127816, -0.4176697321401328100 ) ) ;
#12680=CARTESIAN_POINT ( 'NONE',  ( -0.8661417322834640276, -0.1870078740157479769, 0.4822834645669291653 ) ) ;
#12681=CARTESIAN_POINT ( 'NONE',  ( -0.6889763779527552368, -0.4536011799217368745, -0.2665933059059886201 ) ) ;
#12682=CARTESIAN_POINT ( 'NONE',  ( 0.4396325459317590445, -0.6692913385826771977, 0.1292274648535927661 ) ) ;
#12683=CARTESIAN_POINT ( 'NONE',  ( -1.089238845144356427, 0.05413385826771666132, 0.4176697321401328100 ) ) ;
#12684=CARTESIAN_POINT ( 'NONE',  ( -0.2821522309711278487, -0.6692913385826773087, -0.1292274648535924053 ) ) ;
#12686=LINE ( 'NONE', #13107, #35232 ) ;
#12687=CARTESIAN_POINT ( 'NONE',  ( 1.213910761154856299, -0.6692913385826773087, -0.1292274648535924053 ) ) ;
#12688=CARTESIAN_POINT ( 'NONE',  ( 1.253280839895013710, -0.05778040916215560624, -0.4822834645669293319 ) ) ;
#12690=DIRECTION ( 'NONE',  ( 0.7071067811865477948, 0.000000000000000000, -0.7071067811865473507 ) ) ;
#12691=CARTESIAN_POINT ( 'NONE',  ( -1.043307086614172707, 0.1660481256975883668, -0.3530559997133364547 ) ) ;
#12695=CARTESIAN_POINT ( 'NONE',  ( -0.1377952755905504645, -0.4536011799217368745, -0.2665933059059886201 ) ) ;
#12697=CARTESIAN_POINT ( 'NONE',  ( 0.7152230971128614723, -0.3162353388693409650, -0.4822834645669289433 ) ) ;
#12699=CARTESIAN_POINT ( 'NONE',  ( -1.614173228346457378, 1.881821177735609085, -0.1372047244094477536 ) ) ;
#12700=CARTESIAN_POINT ( 'NONE',  ( -0.3805774278215216522, -0.004921259842519576551, 0.3153832671262227771 ) ) ;
#12701=CARTESIAN_POINT ( 'NONE',  ( 0.3836918680457899744, 8.471767977567108961E-16, -0.4445507791589058955 ) ) ;
#12702=CARTESIAN_POINT ( 'NONE',  ( 1.332020997375329197, -0.3162353388693405765, 0.4822834645669290543 ) ) ;
#12703=CARTESIAN_POINT ( 'NONE',  ( 0.7611548556430451917, -0.5023911411419708095, 0.1820866141732285504 ) ) ;
#12704=CARTESIAN_POINT ( 'NONE',  ( -0.2034120734908128059, 0.2952755905511811885, 0.1292274648535926551 ) ) ;
#12706=CARTESIAN_POINT ( 'NONE',  ( -1.003937007874014853, 0.1660481256975885056, 0.3530559997133364547 ) ) ;
#12707=CARTESIAN_POINT ( 'NONE',  ( -1.194225721784776262, -0.004921259842519870586, -0.3153832671262229437 ) ) ;
#12708=CARTESIAN_POINT ( 'NONE',  ( -0.4724409448818890911, -0.1870078740157479769, 0.4822834645669291653 ) ) ;
#12710=CARTESIAN_POINT ( 'NONE',  ( 0.4531182788721080934, 1.771653543307086354, -0.5309055118110237448 ) ) ;
#12713=CARTESIAN_POINT ( 'NONE',  ( 0.5511811023622055217, -0.1870078740157479769, 0.4822834645669291653 ) ) ;
#12715=CARTESIAN_POINT ( 'NONE',  ( -0.9514435695538050464, -0.3162353388693405765, 0.4822834645669290543 ) ) ;
#12716=CARTESIAN_POINT ( 'NONE',  ( 1.456692913385827515, 0.2952755905511811885, 0.000000000000000000 ) ) ;
#12717=CARTESIAN_POINT ( 'NONE',  ( 0.8858267716535438430, -0.5400638737290845981, -0.3530559997133363437 ) ) ;
#12718=CARTESIAN_POINT ( 'NONE',  ( 0.01968503937007957949, -0.5400638737290845981, -0.3530559997133363437 ) ) ;
#12720=CARTESIAN_POINT ( 'NONE',  ( -0.6102362204724400829, 0.1660481256975885056, 0.3530559997133364547 ) ) ;
#12721=CARTESIAN_POINT ( 'NONE',  ( -0.05905511811023545637, 0.1660481256975885056, 0.3530559997133364547 ) ) ;
#12723=CARTESIAN_POINT ( 'NONE',  ( -0.09842519685039295696, -0.4536011799217367080, 0.2665933059059888421 ) ) ;
#12725=CARTESIAN_POINT ( 'NONE',  ( 0.1181102362204730916, -0.6692913385826771977, 8.415575281601705876E-17 ) ) ;
#12727=CARTESIAN_POINT ( 'NONE',  ( 0.9580052493438326877, 0.05413385826771666132, 0.4176697321401328100 ) ) ;
#12728=CARTESIAN_POINT ( 'NONE',  ( 0.4852136692201463597, 0.004960608223778677044, 0.3437734562760191293 ) ) ;
#12731=CARTESIAN_POINT ( 'NONE',  ( 0.09186351706036827158, 0.05413385826771666132, 0.4176697321401328100 ) ) ;
#12732=CARTESIAN_POINT ( 'NONE',  ( -0.3608923884514428360, -0.5511811023622048555, -0.09757992244046775898 ) ) ;
#12733=CARTESIAN_POINT ( 'NONE',  ( 1.299212598425197429, -0.5511811023622047445, 6.969142054262312111E-17 ) ) ;
#12737=CARTESIAN_POINT ( 'NONE',  ( 1.620734908136483465, -0.5511811023622046335, 0.09757992244046803654 ) ) ;
#12738=CARTESIAN_POINT ( 'NONE',  ( 1.463254593175853824, 0.2952755905511810774, -0.1292274648535930714 ) ) ;
#12741=CARTESIAN_POINT ( 'NONE',  ( -0.09842519685039295696, 0.1660481256975883668, -0.3530559997133364547 ) ) ;
#12742=CARTESIAN_POINT ( 'NONE',  ( -1.332020997375327642, -0.05778040916215522460, 0.4822834645669289988 ) ) ;
#12743=CARTESIAN_POINT ( 'NONE',  ( -1.135170603674539924, -0.6692913385826771977, 0.1292274648535927661 ) ) ;
#12744=CARTESIAN_POINT ( 'NONE',  ( 0.07217847769028949700, -0.05778040916215560624, -0.4822834645669293319 ) ) ;
#12746=CARTESIAN_POINT ( 'NONE',  ( 1.515748031496063408, 0.1660481256975885056, 0.3530559997133364547 ) ) ;
#12747=CARTESIAN_POINT ( 'NONE',  ( 0.7874015748031503170, -0.1870078740157479769, 0.4822834645669291653 ) ) ;
#12748=CARTESIAN_POINT ( 'NONE',  ( 1.259842519685040019, -0.1870078740157480601, -0.3641732283464567677 ) ) ;
#12751=CARTESIAN_POINT ( 'NONE',  ( 0.6561679790026253567, -0.5023911411419708095, -0.1820866141732282451 ) ) ;
#12752=CARTESIAN_POINT ( 'NONE',  ( -1.115485564304461219, 0.05413385826771626580, -0.4176697321401330321 ) ) ;
#12754=CARTESIAN_POINT ( 'NONE',  ( 1.082677165354331228, 0.1660481256975883668, -0.3530559997133364547 ) ) ;
#12756=CARTESIAN_POINT ( 'NONE',  ( 0.5643044619422579178, 0.05413385826771666132, 0.4176697321401328100 ) ) ;
#12758=CARTESIAN_POINT ( 'NONE',  ( -1.725721784776902190, -0.08942795157527998196, 0.3641732283464567121 ) ) ;
#12759=CARTESIAN_POINT ( 'NONE',  ( 0.1574803149606306130, -0.1870078740157480879, -0.4822834645669291653 ) ) ;
#12760=CARTESIAN_POINT ( 'NONE',  ( 0.7217847769028878924, -0.3690944881889765550, -0.3153832671262227771 ) ) ;
#12762=CARTESIAN_POINT ( 'NONE',  ( 0.9514435695538062676, -0.3162353388693409650, -0.4822834645669289433 ) ) ;
#12764=CARTESIAN_POINT ( 'NONE',  ( -0.3805774278215216522, -0.3690944881889765550, -0.3153832671262227771 ) ) ;
#12765=CARTESIAN_POINT ( 'NONE',  ( -0.4921259842519677963, -0.5400638737290844871, 0.3530559997133364547 ) ) ;
#12766=CARTESIAN_POINT ( 'NONE',  ( -1.607611548556429737, 0.1771653543307087075, -0.09757992244046823083 ) ) ;
#12767=CARTESIAN_POINT ( 'NONE',  ( -0.9908136482939626788, -0.6692913385826773087, -0.1292274648535924053 ) ) ;
#12768=CARTESIAN_POINT ( 'NONE',  ( 1.056430446194226658, 0.2952755905511811885, 0.1292274648535926551 ) ) ;
#12770=CARTESIAN_POINT ( 'NONE',  ( -1.541994750656167090, -0.5511811023622048555, -0.09757992244046775898 ) ) ;
#12772=CARTESIAN_POINT ( 'NONE',  ( 1.089238845144357537, -0.4281496062992124485, 0.4176697321401328655 ) ) ;
#12774=CARTESIAN_POINT ( 'NONE',  ( -1.620734908136482577, -0.6692913385826773087, -0.1292274648535924053 ) ) ;
#12775=CARTESIAN_POINT ( 'NONE',  ( -1.548556430446193399, -0.5023911411419708095, -0.1820866141732282451 ) ) ;
#12776=CARTESIAN_POINT ( 'NONE',  ( -0.9842519685039365918, -0.5511811023622047445, 6.969142054262312111E-17 ) ) ;
#12778=CARTESIAN_POINT ( 'NONE',  ( -0.3740157480314953431, 0.1660481256975885056, 0.3530559997133364547 ) ) ;
#12779=CARTESIAN_POINT ( 'NONE',  ( -0.4133858267716528645, -0.4536011799217367080, 0.2665933059059888421 ) ) ;
#12781=CARTESIAN_POINT ( 'NONE',  ( 1.122047244094488860, 0.07958543189024085140, 0.2665933059059887866 ) ) ;
#12782=CARTESIAN_POINT ( 'NONE',  ( 0.3937007874015754361, -0.1870078740157479769, 0.4822834645669291653 ) ) ;
#12783=CARTESIAN_POINT ( 'NONE',  ( 1.358267716535433323, -0.5400638737290845981, -0.3530559997133363437 ) ) ;
#12784=CARTESIAN_POINT ( 'NONE',  ( -0.03280839895013062252, 0.1771653543307087075, -0.09757992244046823083 ) ) ;
#12786=CARTESIAN_POINT ( 'NONE',  ( 0.6496062992125991586, -0.5400638737290845981, -0.3530559997133363437 ) ) ;
#12787=CARTESIAN_POINT ( 'NONE',  ( 0.7742782152230978099, -0.3690944881889763329, 0.3153832671262228327 ) ) ;
#12788=CARTESIAN_POINT ( 'NONE',  ( -1.437007874015747477, 0.1660481256975883668, -0.3530559997133364547 ) ) ;
#12789=CARTESIAN_POINT ( 'NONE',  ( -1.141732283464566011, 0.2952755905511811885, 0.000000000000000000 ) ) ;
#12790=CARTESIAN_POINT ( 'NONE',  ( -0.3543307086614165824, -0.6692913385826771977, 8.415575281601705876E-17 ) ) ;
#12793=CARTESIAN_POINT ( 'NONE',  ( 0.4724409448818904789, -0.1870078740157479769, 0.4822834645669291653 ) ) ;
#12794=CARTESIAN_POINT ( 'NONE',  ( 1.049868766404200127, -0.5023911411419708095, -0.1820866141732282451 ) ) ;
#12795=CARTESIAN_POINT ( 'NONE',  ( -0.4658792650918627265, -0.3162353388693409650, -0.4822834645669289433 ) ) ;
#12796=CARTESIAN_POINT ( 'NONE',  ( 0.4790026246719167324, -0.05778040916215522460, 0.4822834645669289988 ) ) ;
#12803=CARTESIAN_POINT ( 'NONE',  ( -1.141732283464566011, -0.5511811023622047445, 6.969142054262312111E-17 ) ) ;
#12804=CARTESIAN_POINT ( 'NONE',  ( -1.062992125984250968, 0.2952755905511811885, 0.000000000000000000 ) ) ;
#12805=B_SPLINE_CURVE_WITH_KNOTS ( 'NONE', 3,
 ( #67798, #61466, #10549, #36207, #81673, #56379, #23984 ),
 .UNSPECIFIED., .F., .F.,
 ( 4, 3, 4 ),
 ( 1.734723475976807094E-18, 0.001246232571205268744, 0.002492492258783275856 ),
 .UNSPECIFIED. ) ;
#12807=CARTESIAN_POINT ( 'NONE',  ( 0.6692913385826778638, -0.6692913385826771977, 8.415575281601705876E-17 ) ) ;
#12808=CARTESIAN_POINT ( 'NONE',  ( 1.292650918635171564, 0.2952755905511811885, 0.1292274648535926551 ) ) ;
#12809=CARTESIAN_POINT ( 'NONE',  ( 0.8070866141732288002, 0.1660481256975885056, 0.3530559997133364547 ) ) ;
#12810=CARTESIAN_POINT ( 'NONE',  ( -2.787279214012418738, 0.000000000000000000, 0.000000000000000000 ) ) ;
#12814=CARTESIAN_POINT ( 'NONE',  ( 0.5118110236220478892, 0.2952755905511811885, 0.000000000000000000 ) ) ;
#12815=CARTESIAN_POINT ( 'NONE',  ( 0.4921259842519691285, 0.1660481256975885056, 0.3530559997133364547 ) ) ;
#12816=CARTESIAN_POINT ( 'NONE',  ( 0.8267716535433077274, 0.1771653543307087630, 0.000000000000000000 ) ) ;
#12817=CARTESIAN_POINT ( 'NONE',  ( 1.423884514435696413, -0.3162353388693409650, -0.4822834645669289433 ) ) ;
#12819=CARTESIAN_POINT ( 'NONE',  ( 0.4330708661417329575, -0.6692913385826771977, 8.415575281601705876E-17 ) ) ;
#12820=CARTESIAN_POINT ( 'NONE',  ( 0.9711286089238851948, -0.6046776061558809534, -0.2411417322834644161 ) ) ;
#12821=CARTESIAN_POINT ( 'NONE',  ( 0.5314960629921267055, -0.5400638737290844871, 0.3530559997133364547 ) ) ;
#12822=CARTESIAN_POINT ( 'NONE',  ( 1.089238845144357759, -0.004921259842519870586, -0.3153832671262229437 ) ) ;
#12823=CARTESIAN_POINT ( 'NONE',  ( -0.9776902887139098386, -0.6692913385826771977, 0.1292274648535927661 ) ) ;
#12824=CARTESIAN_POINT ( 'NONE',  ( -0.8136482939632537770, -0.6046776061558807314, 0.2411417322834647770 ) ) ;
#12825=CARTESIAN_POINT ( 'NONE',  ( 1.358267716535433323, -0.5400638737290845981, -0.3530559997133363437 ) ) ;
#12831=VERTEX_POINT ( 'NONE', #50209 ) ;
#12832=CARTESIAN_POINT ( 'NONE',  ( 1.673228346456693494, 0.1660481256975885056, 0.3530559997133364547 ) ) ;
#12833=CARTESIAN_POINT ( 'NONE',  ( 0.9186351706036751663, -0.5023911411419708095, 0.1820866141732285504 ) ) ;
#12835=CARTESIAN_POINT ( 'NONE',  ( 1.272965879265092637, -0.3690944881889765550, -0.3153832671262227771 ) ) ;
#12838=CARTESIAN_POINT ( 'NONE',  ( -1.473278426072732739, 0.2335363939278404244, -0.2780995266831706170 ) ) ;
#12840=CARTESIAN_POINT ( 'NONE',  ( -0.6364829396325453192, -0.08942795157528024563, -0.3641732283464568787 ) ) ;
#12841=CARTESIAN_POINT ( 'NONE',  ( -1.489501312335957062, -0.2845877964562161244, -0.3641732283464567121 ) ) ;
#12842=CARTESIAN_POINT ( 'NONE',  ( -1.476377952755905110, 0.1660481256975885056, 0.3530559997133364547 ) ) ;
#12843=CARTESIAN_POINT ( 'NONE',  ( -0.03937007874015669567, -0.6692913385826771977, 8.415575281601705876E-17 ) ) ;
#12844=CARTESIAN_POINT ( 'NONE',  ( -1.561679790026246017, -0.4281496062992127816, -0.4176697321401328100 ) ) ;
#12850=CARTESIAN_POINT ( 'NONE',  ( -0.6955380577427815458, -0.004921259842519576551, 0.3153832671262227771 ) ) ;
#12851=EDGE_CURVE ( 'NONE', #38184, #69360, #39606, .T. ) ;
#12852=CARTESIAN_POINT ( 'NONE',  ( -1.089238845144356427, -0.4281496062992127816, -0.4176697321401328100 ) ) ;
#12853=CARTESIAN_POINT ( 'NONE',  ( 1.220472440944882608, 0.2952755905511811885, 0.000000000000000000 ) ) ;
#12857=CARTESIAN_POINT ( 'NONE',  ( 1.030183727034121421, -0.05778040916215522460, 0.4822834645669289988 ) ) ;
#12858=CARTESIAN_POINT ( 'NONE',  ( -1.161417322834644716, -0.5400638737290845981, -0.3530559997133363437 ) ) ;
#12861=CARTESIAN_POINT ( 'NONE',  ( -0.2493438320209966919, -0.004921259842519870586, -0.3153832671262229437 ) ) ;
#12863=CARTESIAN_POINT ( 'NONE',  ( -0.6102362204724400829, -0.4536011799217368745, -0.2665933059059886201 ) ) ;
#12864=CARTESIAN_POINT ( 'NONE',  ( -0.05249343832020938322, -0.5023911411419708095, -0.1820866141732282451 ) ) ;
#12865=CARTESIAN_POINT ( 'NONE',  ( 0.1509186351706042484, -0.3162353388693405765, 0.4822834645669290543 ) ) ;
#12866=CARTESIAN_POINT ( 'NONE',  ( -0.9776902887139098386, 0.1771653543307087075, -0.09757992244046823083 ) ) ;
#12868=CARTESIAN_POINT ( 'NONE',  ( 1.030183727034121421, -0.3162353388693409650, -0.4822834645669289433 ) ) ;
#12869=CARTESIAN_POINT ( 'NONE',  ( -1.377952755905511140, -0.6692913385826771977, 8.415575281601705876E-17 ) ) ;
#12871=CARTESIAN_POINT ( 'NONE',  ( -0.4068241469816267775, 0.05413385826771626580, -0.4176697321401330321 ) ) ;
#12872=CARTESIAN_POINT ( 'NONE',  ( -0.9317585301837263412, -0.4281496062992127816, -0.4176697321401328100 ) ) ;
#12873=CARTESIAN_POINT ( 'NONE',  ( 0.6430446194225729606, -0.3690944881889765550, -0.3153832671262227771 ) ) ;
#12874=CARTESIAN_POINT ( 'NONE',  ( -0.4855643044619415427, -0.3690944881889763329, 0.3153832671262228327 ) ) ;
#12875=CARTESIAN_POINT ( 'NONE',  ( -0.5249343832020990641, -0.6046776061558809534, -0.2411417322834644161 ) ) ;
#12876=CARTESIAN_POINT ( 'NONE',  ( -1.338582677165353729, -0.1870078740157479769, 0.4822834645669291653 ) ) ;
#12877=PLANE ( 'NONE',  #40726 ) ;
#12878=CARTESIAN_POINT ( 'NONE',  ( 1.272965879265092637, -0.3690944881889765550, -0.3153832671262227771 ) ) ;
#12879=CARTESIAN_POINT ( 'NONE',  ( -0.3543307086614165824, 0.2952755905511811885, 0.000000000000000000 ) ) ;
#12880=CARTESIAN_POINT ( 'NONE',  ( -1.535433070866141225, 0.2952755905511811885, 0.000000000000000000 ) ) ;
#12881=ORIENTED_EDGE ( 'NONE', *, *, #13568, .F. ) ;
#12883=CARTESIAN_POINT ( 'NONE',  ( -0.8727034120734901146, -0.2845877964562159024, 0.3641732283464567677 ) ) ;
#12884=CARTESIAN_POINT ( 'NONE',  ( 0.7152230971128614723, -0.3162353388693409650, -0.4822834645669289433 ) ) ;
#12885=CARTESIAN_POINT ( 'NONE',  ( -1.194225721784776262, -0.004921259842519870586, -0.3153832671262229437 ) ) ;
#12887=CARTESIAN_POINT ( 'NONE',  ( -1.069553805774277722, 0.2952755905511811885, 0.1292274648535926551 ) ) ;
#12888=AXIS2_PLACEMENT_3D ( 'NONE', #46599, #52068, #60067 ) ;
#12889=CARTESIAN_POINT ( 'NONE',  ( 0.7349081364829403995, 0.2306618581243848609, 0.2411417322834645549 ) ) ;
#12890=CARTESIAN_POINT ( 'NONE',  ( 0.2821522309711292364, 0.2952755905511810774, -0.1292274648535930714 ) ) ;
#12891=CARTESIAN_POINT ( 'NONE',  ( 1.587926509186352142, 0.05413385826771666132, 0.4176697321401328100 ) ) ;
#12892=CARTESIAN_POINT ( 'NONE',  ( -1.463254593175852492, -0.5511811023622048555, -0.09757992244046775898 ) ) ;
#12897=CARTESIAN_POINT ( 'NONE',  ( 1.279527559055118724, -0.4536011799217368745, -0.2665933059059886201 ) ) ;
#12898=CARTESIAN_POINT ( 'NONE',  ( 0.1049868766404206816, -0.5023911411419708095, -0.1820866141732282451 ) ) ;
#12899=CARTESIAN_POINT ( 'NONE',  ( 0.09186351706036799403, -0.4281496062992127816, -0.4176697321401328100 ) ) ;
#12900=CARTESIAN_POINT ( 'NONE',  ( 1.417322834645670104, -0.1870078740157479769, 0.4822834645669291653 ) ) ;
#12902=CARTESIAN_POINT ( 'NONE',  ( 0.4265091863517067594, 0.1771653543307087630, 0.09757992244046791164 ) ) ;
#12903=CARTESIAN_POINT ( 'NONE',  ( -0.5708661417322825615, -0.5400638737290844871, 0.3530559997133364547 ) ) ;
#12904=CARTESIAN_POINT ( 'NONE',  ( -1.122047244094487306, 0.1660481256975883668, -0.3530559997133364547 ) ) ;
#12905=CARTESIAN_POINT ( 'NONE',  ( 0.6758530183727039509, -0.6692913385826771977, 0.1292274648535927661 ) ) ;
#12911=CARTESIAN_POINT ( 'NONE',  ( -1.108923884514435132, -0.3162353388693405765, 0.4822834645669290543 ) ) ;
#12912=EDGE_CURVE ( 'NONE', #66112, #199, #51440, .T. ) ;
#12913=CARTESIAN_POINT ( 'NONE',  ( -0.5380577427821514602, 0.05413385826771666132, 0.4176697321401328100 ) ) ;
#12914=CARTESIAN_POINT ( 'NONE',  ( -0.6627296587926501115, 0.1771653543307087075, -0.09757992244046823083 ) ) ;
#12915=CARTESIAN_POINT ( 'NONE',  ( -0.5446194225721777693, -0.05778040916215522460, 0.4822834645669289988 ) ) ;
#12918=CARTESIAN_POINT ( 'NONE',  ( -1.555118110236219930, -0.4536011799217368745, -0.2665933059059886201 ) ) ;
#12919=CARTESIAN_POINT ( 'NONE',  ( -1.305774278215222184, -0.6692913385826773087, -0.1292274648535924053 ) ) ;
#12920=CARTESIAN_POINT ( 'NONE',  ( 0.4921259842519691285, 0.1660481256975885056, 0.3530559997133364547 ) ) ;
#12921=CARTESIAN_POINT ( 'NONE',  ( -0.9448818897637790704, -0.1870078740157480879, -0.4822834645669291653 ) ) ;
#12923=CARTESIAN_POINT ( 'NONE',  ( -0.8661417322834640276, -0.1870078740157479769, 0.3641732283464567677 ) ) ;
#12926=VERTEX_POINT ( 'NONE', #69585 ) ;
#12927=CARTESIAN_POINT ( 'NONE',  ( -1.614173228346456268, -0.5511811023622047445, 6.969142054262312111E-17 ) ) ;
#12928=CARTESIAN_POINT ( 'NONE',  ( -1.023622047244093558, -0.1870078740157479769, 0.4822834645669291653 ) ) ;
#12929=CARTESIAN_POINT ( 'NONE',  ( -0.8267716535433065062, 0.2952755905511811885, 0.000000000000000000 ) ) ;
#12931=CARTESIAN_POINT ( 'NONE',  ( -1.266404199475064773, -0.3162353388693405765, 0.4822834645669290543 ) ) ;
#12932=CARTESIAN_POINT ( 'NONE',  ( -1.082677165354329896, 0.1660481256975885056, 0.3530559997133364547 ) ) ;
#12934=CARTESIAN_POINT ( 'NONE',  ( -0.8267716535433065062, 0.2952755905511811885, 0.000000000000000000 ) ) ;
#12936=CARTESIAN_POINT ( 'NONE',  ( 0.4133858267716541968, 0.07958543189024085140, 0.2665933059059887866 ) ) ;
#12937=DIRECTION ( 'NONE',  ( -1.000000000000000000, -3.469446951953613696E-16, 0.000000000000000000 ) ) ;
#12939=CARTESIAN_POINT ( 'NONE',  ( -0.3018372703412066094, -0.004921259842519576551, 0.3153832671262227771 ) ) ;
#12940=CARTESIAN_POINT ( 'NONE',  ( -0.9317585301837263412, -0.4281496062992127816, -0.4176697321401328100 ) ) ;
#12941=CARTESIAN_POINT ( 'NONE',  ( 1.259842519685040019, -0.1870078740157479769, 0.4822834645669291653 ) ) ;
#12942=CARTESIAN_POINT ( 'NONE',  ( -0.5971128608923877978, -0.6692913385826773087, -0.1292274648535924053 ) ) ;
#12946=CARTESIAN_POINT ( 'NONE',  ( -0.7939632545931750718, -0.05778040916215560624, -0.4822834645669293319 ) ) ;
#12947=CARTESIAN_POINT ( 'NONE',  ( 1.325459317585302665, 0.05413385826771626580, -0.4176697321401330321 ) ) ;
#12948=CARTESIAN_POINT ( 'NONE',  ( -1.082677165354329896, 0.07958543189024085140, 0.2665933059059887866 ) ) ;
#12949=CARTESIAN_POINT ( 'NONE',  ( -1.568241469816272105, -0.05778040916215522460, 0.4822834645669289988 ) ) ;
#12954=CARTESIAN_POINT ( 'NONE',  ( 0.1246719160104994284, 0.2952755905511810774, -0.1292274648535930714 ) ) ;
#12955=CARTESIAN_POINT ( 'NONE',  ( -1.076115485564303809, -0.5023911411419708095, -0.1820866141732282451 ) ) ;
#12957=CARTESIAN_POINT ( 'NONE',  ( -0.6627296587926503335, -0.6692913385826771977, 0.1292274648535927661 ) ) ;
#12959=CARTESIAN_POINT ( 'NONE',  ( -1.233595800524933894, 0.2306618581243848609, 0.2411417322834645549 ) ) ;
#12960=CARTESIAN_POINT ( 'NONE',  ( -1.043307086614172707, 0.1660481256975883668, -0.3530559997133364547 ) ) ;
#12961=CARTESIAN_POINT ( 'NONE',  ( 0.006561679790026889343, -0.05778040916215522460, 0.4822834645669289988 ) ) ;
#12963=CARTESIAN_POINT ( 'NONE',  ( 0.8792650918635177559, -0.3690944881889765550, -0.3153832671262227771 ) ) ;
#12964=CARTESIAN_POINT ( 'NONE',  ( -0.5708661417322828946, 0.07958543189024071263, -0.2665933059059888421 ) ) ;
#12966=CARTESIAN_POINT ( 'NONE',  ( 0.6955380577427828781, -0.3690944881889763329, 0.3153832671262228327 ) ) ;
#12967=CARTESIAN_POINT ( 'NONE',  ( 1.174540682414699111, -0.08942795157528024563, -0.3641732283464568787 ) ) ;
#12968=CARTESIAN_POINT ( 'NONE',  ( 1.404199475065617264, -0.4281496062992124485, 0.4176697321401328655 ) ) ;
#12969=CARTESIAN_POINT ( 'NONE',  ( 0.3608923884514443348, -0.5511811023622046335, 0.09757992244046803654 ) ) ;
#12971=CARTESIAN_POINT ( 'NONE',  ( -0.9383202099737524282, -0.3162353388693409650, -0.4822834645669289433 ) ) ;
#12972=CARTESIAN_POINT ( 'NONE',  ( 1.292650918635171564, 0.2952755905511811885, 0.1292274648535926551 ) ) ;
#12973=AXIS2_PLACEMENT_3D ( 'NONE', #74771, #5290, #56213 ) ;
#12975=CARTESIAN_POINT ( 'NONE',  ( -0.6430446194225712953, -0.004921259842519870586, -0.3153832671262229437 ) ) ;
#12976=CARTESIAN_POINT ( 'NONE',  ( 0.02624671916010564918, 0.2306618581243848609, 0.2411417322834645549 ) ) ;
#12977=CARTESIAN_POINT ( 'NONE',  ( 0.4921259842519691285, -0.5400638737290845981, -0.3530559997133363437 ) ) ;
#12978=DIRECTION ( 'NONE',  ( 0.000000000000000000, -1.000000000000000000, -0.000000000000000000 ) ) ;
#12979=CARTESIAN_POINT ( 'NONE',  ( 1.095800524934383846, -0.2845877964562159024, 0.3641732283464567677 ) ) ;
#12980=CARTESIAN_POINT ( 'NONE',  ( 0.03280839895013198948, 0.1771653543307087630, 0.09757992244046791164 ) ) ;
#12981=CARTESIAN_POINT ( 'NONE',  ( 0.07217847769028949700, -0.3162353388693405765, 0.4822834645669290543 ) ) ;
#12982=CARTESIAN_POINT ( 'NONE',  ( -1.489501312335957062, -0.3162353388693409650, -0.4822834645669289433 ) ) ;
#12983=CARTESIAN_POINT ( 'NONE',  ( -0.6627296587926501115, 0.1771653543307087075, -0.09757992244046823083 ) ) ;
#12984=FACE_OUTER_BOUND ( 'NONE', #29777, .T. ) ;
#12986=CARTESIAN_POINT ( 'NONE',  ( -0.4921259842519677963, 0.1660481256975883668, -0.3530559997133364547 ) ) ;
#12989=CARTESIAN_POINT ( 'NONE',  ( 0.3477690288713918276, 0.1771653543307087630, 0.09757992244046791164 ) ) ;
#12990=CARTESIAN_POINT ( 'NONE',  ( -0.8727034120734901146, -0.3162353388693405765, 0.4822834645669290543 ) ) ;
#12991=CARTESIAN_POINT ( 'NONE',  ( -1.056430446194224881, -0.6692913385826771977, 0.1292274648535927661 ) ) ;
#12992=CARTESIAN_POINT ( 'NONE',  ( -1.194225721784776262, -0.3690944881889763329, 0.3153832671262228327 ) ) ;
#12993=LINE ( 'NONE', #52516, #6447 ) ;
#12994=CARTESIAN_POINT ( 'NONE',  ( -0.5511811023622038563, -0.1870078740157479769, 0.4822834645669291653 ) ) ;
#12995=CARTESIAN_POINT ( 'NONE',  ( -0.7611548556430438595, -0.5023911411419708095, -0.1820866141732282451 ) ) ;
#12996=CARTESIAN_POINT ( 'NONE',  ( -1.699475065616797398, 0.1771653543307087630, 0.09757992244046791164 ) ) ;
#12997=CARTESIAN_POINT ( 'NONE',  ( 1.384514435695538337, -0.6692913385826771977, 0.1292274648535927661 ) ) ;
#13001=DIRECTION ( 'NONE',  ( 0.000000000000000000, -1.000000000000000000, -0.000000000000000000 ) ) ;
#13002=CARTESIAN_POINT ( 'NONE',  ( -1.404199475065615932, 0.05413385826771666132, 0.4176697321401328100 ) ) ;
#13003=CARTESIAN_POINT ( 'NONE',  ( -0.8070866141732276899, -0.5400638737290844871, 0.3530559997133364547 ) ) ;
#13004=CARTESIAN_POINT ( 'NONE',  ( -1.528871391076114250, -0.6692913385826771977, 0.1292274648535927661 ) ) ;
#13006=CARTESIAN_POINT ( 'NONE',  ( 1.607611548556431069, -0.5511811023622048555, -0.09757992244046775898 ) ) ;
#13008=CARTESIAN_POINT ( 'NONE',  ( 0.4855643044619430415, -0.4281496062992127816, -0.4176697321401328100 ) ) ;
#13009=CARTESIAN_POINT ( 'NONE',  ( 0.07217847769028949700, -0.3162353388693405765, 0.4822834645669290543 ) ) ;
#13013=CARTESIAN_POINT ( 'NONE',  ( 0.7480314960629927956, -0.5511811023622047445, 6.969142054262312111E-17 ) ) ;
#13018=CARTESIAN_POINT ( 'NONE',  ( -0.07217847769028813698, -0.3162353388693409650, -0.4822834645669289433 ) ) ;
#13019=CARTESIAN_POINT ( 'NONE',  ( -0.6364829396325453192, -0.3162353388693405765, 0.4822834645669290543 ) ) ;
#13020=CARTESIAN_POINT ( 'NONE',  ( -1.482939632545930975, 0.05413385826771666132, 0.4176697321401328100 ) ) ;
#13021=CARTESIAN_POINT ( 'NONE',  ( 0.6561679790026253567, -0.6046776061558809534, -0.2411417322834644161 ) ) ;
#13022=CARTESIAN_POINT ( 'NONE',  ( -1.633858267716534529, 0.07958543189024085140, 0.2665933059059887866 ) ) ;
#13023=CARTESIAN_POINT ( 'NONE',  ( 1.227034120734908917, -0.6692913385826771977, 0.1292274648535927661 ) ) ;
#13024=CARTESIAN_POINT ( 'NONE',  ( -0.4658792650918627265, -0.3162353388693409650, -0.4822834645669289433 ) ) ;
#13025=CARTESIAN_POINT ( 'NONE',  ( 0.4790026246719167324, -0.05778040916215522460, 0.4822834645669289988 ) ) ;
#13026=CARTESIAN_POINT ( 'NONE',  ( 1.541994750656168645, -0.6692913385826771977, 0.1292274648535927661 ) ) ;
#13027=CARTESIAN_POINT ( 'NONE',  ( 1.122047244094488860, 0.1660481256975885056, 0.3530559997133364547 ) ) ;
#13028=CARTESIAN_POINT ( 'NONE',  ( 1.607611548556431069, -0.6692913385826773087, -0.1292274648535924053 ) ) ;
#13030=CARTESIAN_POINT ( 'NONE',  ( -0.1181102362204717315, 0.2952755905511811885, 0.000000000000000000 ) ) ;
#13032=CARTESIAN_POINT ( 'NONE',  ( 0.3412073490813655186, -0.5023911411419708095, -0.1820866141732282451 ) ) ;
#13035=EDGE_LOOP ( 'NONE', ( #30710, #49518, #14708, #38124 ) ) ;
#13036=CARTESIAN_POINT ( 'NONE',  ( -0.4921259842519677963, -0.4536011799217367080, 0.2665933059059888421 ) ) ;
#13037=PLANE ( 'NONE',  #81130 ) ;
#13038=CARTESIAN_POINT ( 'NONE',  ( 0.05249343832021075018, 0.2306618581243847221, -0.2411417322834647770 ) ) ;
#13039=CARTESIAN_POINT ( 'NONE',  ( -0.1574803149606292529, -0.1870078740157479769, 0.4822834645669291653 ) ) ;
#13040=CARTESIAN_POINT ( 'NONE',  ( -0.9186351706036736120, 0.2306618581243848609, 0.2411417322834645549 ) ) ;
#13042=CARTESIAN_POINT ( 'NONE',  ( -1.154855643044618851, 0.2306618581243848609, 0.2411417322834645549 ) ) ;
#13044=CARTESIAN_POINT ( 'NONE',  ( 0.9973753280839902091, 0.1283753931104746893, -0.1820866141732285504 ) ) ;
#13045=CARTESIAN_POINT ( 'NONE',  ( 0.5708661417322842269, 0.1660481256975885056, 0.3530559997133364547 ) ) ;
#13046=CARTESIAN_POINT ( 'NONE',  ( 0.8267716535433078384, -0.6692913385826771977, 8.415575281601705876E-17 ) ) ;
#13048=CARTESIAN_POINT ( 'NONE',  ( -1.706036745406823485, 0.2306618581243848609, 0.2411417322834645549 ) ) ;
#13051=CARTESIAN_POINT ( 'NONE',  ( -0.1640419947506555343, -0.3162353388693405765, 0.4822834645669290543 ) ) ;
#13054=CARTESIAN_POINT ( 'NONE',  ( -1.279527559055116948, 0.07958543189024071263, -0.2665933059059888421 ) ) ;
#13055=CARTESIAN_POINT ( 'NONE',  ( 1.194225721784777594, -0.4281496062992127816, -0.4176697321401328100 ) ) ;
#13056=CARTESIAN_POINT ( 'NONE',  ( 1.482939632545932307, -0.4281496062992124485, 0.4176697321401328655 ) ) ;
#13057=CARTESIAN_POINT ( 'NONE',  ( -0.006561679790025524116, -0.08942795157528024563, -0.3641732283464568787 ) ) ;
#13058=CARTESIAN_POINT ( 'NONE',  ( 0.4199475065616803948, -0.6046776061558809534, -0.2411417322834644161 ) ) ;
#13060=CARTESIAN_POINT ( 'NONE',  ( 0.4658792650918641698, -0.08942795157528024563, -0.3641732283464568787 ) ) ;
#13061=CARTESIAN_POINT ( 'NONE',  ( 0.2952755905511816326, -0.5400638737290844871, 0.3530559997133364547 ) ) ;
#13063=CARTESIAN_POINT ( 'NONE',  ( -1.371391076115484831, 0.2952755905511810774, -0.1292274648535930714 ) ) ;
#13064=CARTESIAN_POINT ( 'NONE',  ( 0.6299212598425204535, -0.1870078740157479769, 0.3641732283464567677 ) ) ;
#13065=CARTESIAN_POINT ( 'NONE',  ( 0.4768132735438208591, 1.796500554427756802, 0.5050878842330650542 ) ) ;
#13066=CARTESIAN_POINT ( 'NONE',  ( -0.6102362204724400829, 0.1660481256975885056, 0.3530559997133364547 ) ) ;
#13067=CARTESIAN_POINT ( 'NONE',  ( -0.3018372703412066094, -0.3690944881889765550, -0.3153832671262227771 ) ) ;
#13068=CARTESIAN_POINT ( 'NONE',  ( -0.7080320533160963103, 1.900312960331933976, -0.5309055118110235227 ) ) ;
#13069=CARTESIAN_POINT ( 'NONE',  ( -0.2296587926509179312, -0.3162353388693409650, -0.4822834645669289433 ) ) ;
#13070=CARTESIAN_POINT ( 'NONE',  ( -0.1771653543307080136, 0.1660481256975883668, -0.3530559997133364547 ) ) ;
#13071=CARTESIAN_POINT ( 'NONE',  ( 0.2427821522309716595, -0.2845877964562161244, -0.3641732283464567121 ) ) ;
#13074=CARTESIAN_POINT ( 'NONE',  ( -0.06561679790026180015, 0.05413385826771666132, 0.4176697321401328100 ) ) ;
#13077=AXIS2_PLACEMENT_3D ( 'NONE', #69239, #4842, #37247 ) ;
#13078=CARTESIAN_POINT ( 'NONE',  ( 1.220472440944882608, 0.1771653543307087630, 0.000000000000000000 ) ) ;
#13079=CARTESIAN_POINT ( 'NONE',  ( 1.351706036745407458, -0.4281496062992127816, -0.4176697321401328100 ) ) ;
#13080=CARTESIAN_POINT ( 'NONE',  ( -0.6692913385826764205, -0.5511811023622047445, 6.969142054262312111E-17 ) ) ;
#13081=CARTESIAN_POINT ( 'NONE',  ( -0.5314960629921254842, -0.4536011799217368745, -0.2665933059059886201 ) ) ;
#13082=CARTESIAN_POINT ( 'NONE',  ( -0.6561679790026240244, 0.2306618581243847221, -0.2411417322834647770 ) ) ;
#13083=CARTESIAN_POINT ( 'NONE',  ( 0.006561679790026889343, -0.05778040916215522460, 0.4822834645669289988 ) ) ;
#13084=CARTESIAN_POINT ( 'NONE',  ( 0.5183727034120741983, -0.5511811023622046335, 0.09757992244046803654 ) ) ;
#13086=CARTESIAN_POINT ( 'NONE',  ( 1.115485564304462551, -0.004921259842519576551, 0.3153832671262227771 ) ) ;
#13088=CARTESIAN_POINT ( 'NONE',  ( 0.7939632545931766261, -0.3162353388693409650, -0.4822834645669289433 ) ) ;
#13090=CARTESIAN_POINT ( 'NONE',  ( -0.1246719160104980823, 0.2952755905511811885, 0.1292274648535926551 ) ) ;
#13092=CARTESIAN_POINT ( 'NONE',  ( 1.482939632545932307, -0.004921259842519870586, -0.3153832671262229437 ) ) ;
#13093=CARTESIAN_POINT ( 'NONE',  ( 0.7349081364829403995, 0.2306618581243848609, 0.2411417322834645549 ) ) ;
#13094=CARTESIAN_POINT ( 'NONE',  ( -0.07217847769028787330, -0.05778040916215522460, 0.4822834645669289988 ) ) ;
#13096=CARTESIAN_POINT ( 'NONE',  ( 0.4724409448818904789, -0.1870078740157480601, -0.3641732283464567677 ) ) ;
#13097=CARTESIAN_POINT ( 'NONE',  ( 0.7152230971128616943, -0.05778040916215522460, 0.4822834645669289988 ) ) ;
#13098=CARTESIAN_POINT ( 'NONE',  ( -0.5183727034120726440, -0.5511811023622048555, -0.09757992244046775898 ) ) ;
#13099=CARTESIAN_POINT ( 'NONE',  ( -0.9251968503937002541, -0.5400638737290845981, -0.3530559997133363437 ) ) ;
#13100=CARTESIAN_POINT ( 'NONE',  ( 0.4658792650918640033, -0.3162353388693405765, 0.4822834645669290543 ) ) ;
#13101=CARTESIAN_POINT ( 'NONE',  ( -1.391076115485563314, -0.6046776061558809534, -0.2411417322834644161 ) ) ;
#13102=CARTESIAN_POINT ( 'NONE',  ( -0.5577427821522301654, -0.08942795157528024563, -0.3641732283464568787 ) ) ;
#13103=CARTESIAN_POINT ( 'NONE',  ( 0.2362204724409456558, -0.1870078740157480879, -0.4822834645669291653 ) ) ;
#13104=CARTESIAN_POINT ( 'NONE',  ( -1.332020997375327642, -0.3162353388693409650, -0.4822834645669289433 ) ) ;
#13105=CARTESIAN_POINT ( 'NONE',  ( -0.3477690288713902178, 0.2952755905511810774, -0.1292274648535930714 ) ) ;
#13106=CARTESIAN_POINT ( 'NONE',  ( 1.115485564304462551, 0.009842519685039463617, 0.3409548833797002576 ) ) ;
#13107=CARTESIAN_POINT ( 'NONE',  ( -0.8478501267249380913, 2.401574803149606474, 0.8478501267249375362 ) ) ;
#13108=CARTESIAN_POINT ( 'NONE',  ( 1.410761154855643795, -0.3162353388693405765, 0.4822834645669290543 ) ) ;
#13109=CARTESIAN_POINT ( 'NONE',  ( 1.450131233595801428, -0.6692913385826773087, -0.1292274648535924053 ) ) ;
#13111=CARTESIAN_POINT ( 'NONE',  ( -1.220472440944881054, 2.401574803149606474, 0.5309055118110237448 ) ) ;
#13112=CARTESIAN_POINT ( 'NONE',  ( -1.076115485564303809, 0.2306618581243848609, 0.2411417322834645549 ) ) ;
#13116=ORIENTED_EDGE ( 'NONE', *, *, #50670, .T. ) ;
#13117=CARTESIAN_POINT ( 'NONE',  ( -0.2165354330708654795, 0.07958543189024085140, 0.2665933059059887866 ) ) ;
#13119=ORIENTED_EDGE ( 'NONE', *, *, #58308, .F. ) ;
#13120=CARTESIAN_POINT ( 'NONE',  ( 0.1377952755905518800, -0.5400638737290844871, 0.3530559997133364547 ) ) ;
#13122=CARTESIAN_POINT ( 'NONE',  ( 0.5905511811023629321, -0.6692913385826771977, 8.415575281601705876E-17 ) ) ;
#13125=CARTESIAN_POINT ( 'NONE',  ( -0.5052493438320203589, 0.1771653543307087075, -0.09757992244046823083 ) ) ;
#13127=CARTESIAN_POINT ( 'NONE',  ( 0.6824146981627303710, -0.6046776061558807314, 0.2411417322834647770 ) ) ;
#13128=CARTESIAN_POINT ( 'NONE',  ( 1.023622047244095112, -0.1870078740157480601, -0.3641732283464567677 ) ) ;
#13129=CARTESIAN_POINT ( 'NONE',  ( -0.5905511811023613777, -0.6692913385826771977, 8.415575281601705876E-17 ) ) ;
#13131=CARTESIAN_POINT ( 'NONE',  ( -0.8136482939632537770, 0.2306618581243847221, -0.2411417322834647770 ) ) ;
#13132=CARTESIAN_POINT ( 'NONE',  ( -1.332020997375327642, -0.2845877964562161244, -0.3641732283464567121 ) ) ;
#13133=CARTESIAN_POINT ( 'NONE',  ( -0.8005249343832013809, -0.4281496062992124485, 0.4176697321401328655 ) ) ;
#13134=CARTESIAN_POINT ( 'NONE',  ( 1.679790026246720025, 0.2306618581243848609, 0.2411417322834645549 ) ) ;
#13138=CARTESIAN_POINT ( 'NONE',  ( -0.1706036745406816491, 0.05413385826771626580, -0.4176697321401330321 ) ) ;
#13140=CARTESIAN_POINT ( 'NONE',  ( -0.7939632545931754048, -0.3162353388693405765, 0.4822834645669290543 ) ) ;
#13141=CARTESIAN_POINT ( 'NONE',  ( 1.482939632545932307, 0.05413385826771626580, -0.4176697321401330321 ) ) ;
#13142=CARTESIAN_POINT ( 'NONE',  ( 1.167979002624672580, 0.05413385826771626580, -0.4176697321401330321 ) ) ;
#13143=ADVANCED_FACE ( 'NONE', ( #77989 ), #21561, .F. ) ;
#13144=CARTESIAN_POINT ( 'NONE',  ( 0.6758530183727039509, 0.2952755905511810774, -0.1292274648535930714 ) ) ;
#13145=CARTESIAN_POINT ( 'NONE',  ( 0.2493438320209980519, 0.05413385826771666132, 0.4176697321401328100 ) ) ;
#13147=CARTESIAN_POINT ( 'NONE',  ( -1.036745406824146176, 0.05413385826771626580, -0.4176697321401330321 ) ) ;
#13148=CARTESIAN_POINT ( 'NONE',  ( -0.08530183727034056085, -0.3162353388693405765, 0.4822834645669290543 ) ) ;
#13149=EDGE_CURVE ( 'NONE', #79410, #57515, #8614, .T. ) ;
#13150=CARTESIAN_POINT ( 'NONE',  ( 0.09186351706036827158, -0.004921259842519576551, 0.3153832671262227771 ) ) ;
#13151=LINE ( 'NONE', #40481, #79919 ) ;
#13152=CARTESIAN_POINT ( 'NONE',  ( -0.2099737532808391705, -0.6046776061558809534, -0.2411417322834644161 ) ) ;
#13154=CARTESIAN_POINT ( 'NONE',  ( 0.9251968503937015864, -0.5400638737290844871, 0.3530559997133364547 ) ) ;
#13156=ORIENTED_EDGE ( 'NONE', *, *, #74163, .F. ) ;
#13158=CARTESIAN_POINT ( 'NONE',  ( 0.3608923884514443348, -0.6692913385826771977, 0.1292274648535927661 ) ) ;
#13159=CARTESIAN_POINT ( 'NONE',  ( -0.2427821522309703550, -0.08942795157528024563, -0.3641732283464568787 ) ) ;
#13160=CARTESIAN_POINT ( 'NONE',  ( 1.443569553805774897, -0.5023911411419708095, -0.1820866141732282451 ) ) ;
#13161=CARTESIAN_POINT ( 'NONE',  ( 1.614173228346457378, 0.5038684218300975015, 0.1372047244094478369 ) ) ;
#13164=CARTESIAN_POINT ( 'NONE',  ( -1.476377952755905110, 0.1660481256975885056, 0.3530559997133364547 ) ) ;
#13166=CARTESIAN_POINT ( 'NONE',  ( -0.1443569553805768291, 0.05413385826771666132, 0.4176697321401328100 ) ) ;
#13167=CARTESIAN_POINT ( 'NONE',  ( -1.646051170424378096, 0.000000000000000000, 0.3464511005275205946 ) ) ;
#13168=CARTESIAN_POINT ( 'NONE',  ( -1.561679790026246017, 0.05413385826771666132, 0.4176697321401328100 ) ) ;
#13169=CARTESIAN_POINT ( 'NONE',  ( 0.3280839895013130669, 0.05413385826771666132, 0.4176697321401328100 ) ) ;
#13171=CARTESIAN_POINT ( 'NONE',  ( 1.555118110236221041, 0.1660481256975883668, -0.3530559997133364547 ) ) ;
#13172=CARTESIAN_POINT ( 'NONE',  ( 0.8530183727034126306, 0.05413385826771626580, -0.4176697321401330321 ) ) ;
#13173=CARTESIAN_POINT ( 'NONE',  ( 1.102362204724410155, -0.1870078740157480601, -0.3641732283464567677 ) ) ;
#13175=CARTESIAN_POINT ( 'NONE',  ( 0.7939632545931766261, -0.2845877964562161244, -0.3641732283464567121 ) ) ;
#13176=CARTESIAN_POINT ( 'NONE',  ( -1.292650918635170010, 0.2952755905511810774, -0.1292274648535930714 ) ) ;
#13179=CARTESIAN_POINT ( 'NONE',  ( 1.364829396325460076, 0.2306618581243848609, 0.2411417322834645549 ) ) ;
#13181=CARTESIAN_POINT ( 'NONE',  ( 0.7217847769028878924, 0.05413385826771666132, 0.4176697321401328100 ) ) ;
#13183=CARTESIAN_POINT ( 'NONE',  ( -1.377952755905511140, 0.1771653543307087630, 0.000000000000000000 ) ) ;
#13184=CARTESIAN_POINT ( 'NONE',  ( 0.4133858267716541968, -0.4536011799217368745, -0.2665933059059886201 ) ) ;
#13186=CARTESIAN_POINT ( 'NONE',  ( 0.6102362204724416372, 0.1660481256975883668, -0.3530559997133364547 ) ) ;
#13187=CARTESIAN_POINT ( 'NONE',  ( 0.7480314960629927956, 0.2066929133858268208, 0.000000000000000000 ) ) ;
#13188=CARTESIAN_POINT ( 'NONE',  ( -0.8398950131233589023, -0.5023911411419708095, -0.1820866141732282451 ) ) ;
#13189=CARTESIAN_POINT ( 'NONE',  ( -0.5839895013123351797, 0.2952755905511810774, -0.1292274648535930714 ) ) ;
#13190=CARTESIAN_POINT ( 'NONE',  ( 1.568241469816273659, -0.05778040916215560624, -0.4822834645669293319 ) ) ;
#13191=CARTESIAN_POINT ( 'NONE',  ( -1.148293963254592542, -0.6692913385826773087, -0.1292274648535924053 ) ) ;
#13192=CARTESIAN_POINT ( 'NONE',  ( 0.7939632545931766261, -0.3162353388693409650, -0.4822834645669289433 ) ) ;
#13193=CARTESIAN_POINT ( 'NONE',  ( -1.200787401574802349, -0.4536011799217367080, 0.2665933059059888421 ) ) ;
#13196=CARTESIAN_POINT ( 'NONE',  ( 0.9448818897637802916, -0.1870078740157479769, 0.4822834645669291653 ) ) ;
#13199=CARTESIAN_POINT ( 'NONE',  ( -1.653543307086613234, -0.1870078740157480879, -0.4822834645669291653 ) ) ;
#13200=CARTESIAN_POINT ( 'NONE',  ( 1.423884514435696413, -0.3162353388693409650, -0.4822834645669289433 ) ) ;
#13201=CARTESIAN_POINT ( 'NONE',  ( -1.089238845144356427, -0.004921259842519576551, 0.3153832671262227771 ) ) ;
#13202=CARTESIAN_POINT ( 'NONE',  ( 1.574803149606299746, -0.1870078740157480601, -0.3641732283464567677 ) ) ;
#13203=CARTESIAN_POINT ( 'NONE',  ( -0.3674540682414689785, 0.2306618581243848609, 0.2411417322834645549 ) ) ;
#13204=CARTESIAN_POINT ( 'NONE',  ( -0.4527559055118102749, -0.4536011799217368745, -0.2665933059059886201 ) ) ;
#13205=CARTESIAN_POINT ( 'NONE',  ( -1.719160104986876103, -0.004921259842519576551, 0.3153832671262227771 ) ) ;
#13206=CARTESIAN_POINT ( 'NONE',  ( 0.7874015748031503170, -0.1870078740157479769, 0.3641732283464567677 ) ) ;
#13207=CARTESIAN_POINT ( 'NONE',  ( 0.7217847769028878924, 0.05413385826771666132, 0.4176697321401328100 ) ) ;
#13208=CARTESIAN_POINT ( 'NONE',  ( 1.332020997375328974, -0.05778040916215560624, -0.4822834645669293319 ) ) ;
#13209=CARTESIAN_POINT ( 'NONE',  ( 0.5774278215223104249, 0.2306618581243848609, 0.2411417322834645549 ) ) ;
#13210=CARTESIAN_POINT ( 'NONE',  ( 0.3674540682414705883, 0.1283753931104746893, -0.1820866141732285504 ) ) ;
#13212=CARTESIAN_POINT ( 'NONE',  ( -1.535433070866141225, -0.6692913385826771977, 8.415575281601705876E-17 ) ) ;
#13213=CARTESIAN_POINT ( 'NONE',  ( -1.272965879265091305, 0.05413385826771626580, -0.4176697321401330321 ) ) ;
#13214=CARTESIAN_POINT ( 'NONE',  ( -0.6496062992125976043, -0.5400638737290844871, 0.3530559997133364547 ) ) ;
#13217=CARTESIAN_POINT ( 'NONE',  ( 0.1181102362204730916, -0.6692913385826771977, 8.415575281601705876E-17 ) ) ;
#13218=CARTESIAN_POINT ( 'NONE',  ( 1.240157480314961314, -0.4536011799217367080, 0.2665933059059888421 ) ) ;
#13219=CARTESIAN_POINT ( 'NONE',  ( -0.2821522309711278487, -0.6692913385826773087, -0.1292274648535924053 ) ) ;
#13220=CARTESIAN_POINT ( 'NONE',  ( 0.4068241469816279987, -0.4281496062992127816, -0.4176697321401328100 ) ) ;
#13226=CARTESIAN_POINT ( 'NONE',  ( -0.9711286089238838626, -0.5023911411419708095, 0.1820866141732285504 ) ) ;
#13227=CARTESIAN_POINT ( 'NONE',  ( -1.246719160104986512, 0.05413385826771666132, 0.4176697321401328100 ) ) ;
#13229=CARTESIAN_POINT ( 'NONE',  ( 0.3674540682414705883, -0.6046776061558807314, 0.2411417322834647770 ) ) ;
#13230=CARTESIAN_POINT ( 'NONE',  ( 1.345144356955381593, -0.3162353388693409650, -0.4822834645669289433 ) ) ;
#13231=CARTESIAN_POINT ( 'NONE',  ( 0.9120734908136489683, -0.6692913385826771977, 0.1292274648535927661 ) ) ;
#13235=CARTESIAN_POINT ( 'NONE',  ( 1.502624671916010790, -0.05778040916215522460, 0.4822834645669289988 ) ) ;
#13236=CARTESIAN_POINT ( 'NONE',  ( 0.4002624671916016896, -0.3162353388693409650, -0.4822834645669289433 ) ) ;
#13238=CARTESIAN_POINT ( 'NONE',  ( 0.3149606299212603933, -0.1870078740157479769, 0.4822834645669291653 ) ) ;
#13239=CARTESIAN_POINT ( 'NONE',  ( 0.7939632545931766261, -0.08942795157527998196, 0.3641732283464567121 ) ) ;
#13240=CARTESIAN_POINT ( 'NONE',  ( 1.167979002624672580, -0.4281496062992124485, 0.4176697321401328655 ) ) ;
#13242=CARTESIAN_POINT ( 'NONE',  ( 0.2559055118110243332, -0.5400638737290845981, -0.3530559997133363437 ) ) ;
#13243=CARTESIAN_POINT ( 'NONE',  ( 0.9383202099737538715, -0.05778040916215560624, -0.4822834645669293319 ) ) ;
#13244=CARTESIAN_POINT ( 'NONE',  ( 0.4199475065616805614, 0.2306618581243848609, 0.2411417322834645549 ) ) ;
#13245=CARTESIAN_POINT ( 'NONE',  ( 1.069553805774278832, 0.1771653543307087075, -0.09757992244046823083 ) ) ;
#13246=CARTESIAN_POINT ( 'NONE',  ( -0.9055118110236215490, 0.2952755905511811885, 0.000000000000000000 ) ) ;
#13247=CARTESIAN_POINT ( 'NONE',  ( -1.069553805774277722, 0.2952755905511811885, 0.1292274648535926551 ) ) ;
#13248=CARTESIAN_POINT ( 'NONE',  ( 1.036745406824147508, -0.4281496062992127816, -0.4176697321401328100 ) ) ;
#13255=CARTESIAN_POINT ( 'NONE',  ( 1.679790026246720025, 0.2306618581243848609, 0.2411417322834645549 ) ) ;
#13256=CARTESIAN_POINT ( 'NONE',  ( 0.9645669291338588858, 0.07958543189024085140, 0.2665933059059887866 ) ) ;
#13258=CARTESIAN_POINT ( 'NONE',  ( 1.489501312335958172, -0.2845877964562159024, 0.3641732283464567677 ) ) ;
#13260=CARTESIAN_POINT ( 'NONE',  ( -0.1246719160104980684, 0.2952755905511811885, 0.1292274648535926551 ) ) ;
#13262=CARTESIAN_POINT ( 'NONE',  ( -1.220472440944881054, -0.5511811023622047445, 6.969142054262312111E-17 ) ) ;
#13263=CARTESIAN_POINT ( 'NONE',  ( -1.541994750656167090, 0.1771653543307087630, 0.09757992244046791164 ) ) ;
#13264=CARTESIAN_POINT ( 'NONE',  ( -1.266404199475064773, -0.05778040916215560624, -0.4822834645669293319 ) ) ;
#13265=CARTESIAN_POINT ( 'NONE',  ( 0.1574803149606306130, -0.1870078740157479769, 0.4822834645669291653 ) ) ;
#13266=CARTESIAN_POINT ( 'NONE',  ( 1.345144356955381593, -0.3162353388693409650, -0.4822834645669289433 ) ) ;
#13267=ORIENTED_EDGE ( 'NONE', *, *, #31580, .F. ) ;
#13270=CARTESIAN_POINT ( 'NONE',  ( -0.9580052493438311334, -0.004921259842519870586, -0.3153832671262229437 ) ) ;
#13271=LINE ( 'NONE', #7359, #79940 ) ;
#13272=CARTESIAN_POINT ( 'NONE',  ( 0.7611548556430454138, 0.2306618581243847221, -0.2411417322834647770 ) ) ;
#13276=CARTESIAN_POINT ( 'NONE',  ( 1.430446194225722500, -0.4281496062992127816, -0.4176697321401328100 ) ) ;
#13277=CARTESIAN_POINT ( 'NONE',  ( 1.522309711286089939, -0.5023911411419708095, -0.1820866141732282451 ) ) ;
#13279=CARTESIAN_POINT ( 'NONE',  ( -0.2624671916010490880, 0.1283753931104746893, -0.1820866141732285504 ) ) ;
#13280=CARTESIAN_POINT ( 'NONE',  ( -1.299212598425196097, 0.1771653543307087630, 0.000000000000000000 ) ) ;
#13282=CARTESIAN_POINT ( 'NONE',  ( -0.4527559055118102749, -0.4536011799217368745, -0.2665933059059886201 ) ) ;
#13283=CARTESIAN_POINT ( 'NONE',  ( 0.2559055118110243332, -0.4536011799217368745, -0.2665933059059886201 ) ) ;
#13284=CARTESIAN_POINT ( 'NONE',  ( 0.2427821522309716595, -0.3162353388693409650, -0.4822834645669289433 ) ) ;
#13285=CARTESIAN_POINT ( 'NONE',  ( -0.9908136482939626788, 0.1771653543307087630, 0.09757992244046791164 ) ) ;
#13287=CARTESIAN_POINT ( 'NONE',  ( 1.174540682414699111, -0.05778040916215560624, -0.4822834645669293319 ) ) ;
#13288=CARTESIAN_POINT ( 'NONE',  ( -1.227034120734907141, -0.6692913385826773087, -0.1292274648535924053 ) ) ;
#13290=CARTESIAN_POINT ( 'NONE',  ( -0.4527559055118102749, 0.1660481256975885056, 0.3530559997133364547 ) ) ;
#13291=CARTESIAN_POINT ( 'NONE',  ( -0.8792650918635160906, -0.4281496062992124485, 0.4176697321401328655 ) ) ;
#13292=CARTESIAN_POINT ( 'NONE',  ( 0.8464566929133866546, -0.4536011799217367080, 0.2665933059059888421 ) ) ;
#13293=CARTESIAN_POINT ( 'NONE',  ( -0.2952755905511804668, 0.07958543189024085140, 0.2665933059059887866 ) ) ;
#13294=CARTESIAN_POINT ( 'NONE',  ( -0.7874015748031489847, -0.1870078740157479769, 0.4822834645669291653 ) ) ;
#13295=CARTESIAN_POINT ( 'NONE',  ( -1.469816272965878357, 0.2306618581243848609, 0.2411417322834645549 ) ) ;
#13296=CARTESIAN_POINT ( 'NONE',  ( 0.4330708661417329575, 1.488513638086841118, 0.000000000000000000 ) ) ;
#13297=CARTESIAN_POINT ( 'NONE',  ( 1.233595800524935227, 0.1283753931104746893, -0.1820866141732285504 ) ) ;
#13298=CARTESIAN_POINT ( 'NONE',  ( -1.509186351706035767, -0.4281496062992124485, 0.4176697321401328655 ) ) ;
#13299=CARTESIAN_POINT ( 'NONE',  ( -1.522309711286088607, 0.2306618581243847221, -0.2411417322834647770 ) ) ;
#13300=VERTEX_POINT ( 'NONE', #59032 ) ;
#13302=CARTESIAN_POINT ( 'NONE',  ( -0.9317585301837263412, -0.3690944881889765550, -0.3153832671262227771 ) ) ;
#13303=CARTESIAN_POINT ( 'NONE',  ( 0.6167979002624678353, -0.4281496062992124485, 0.4176697321401328655 ) ) ;
#13304=CARTESIAN_POINT ( 'NONE',  ( -0.9645669291338575535, -0.4536011799217367080, 0.2665933059059888421 ) ) ;
#13306=CARTESIAN_POINT ( 'NONE',  ( -0.9645669291338575535, -0.5400638737290844871, 0.3530559997133364547 ) ) ;
#13307=CARTESIAN_POINT ( 'NONE',  ( 0.6692913385826778638, -0.6692913385826771977, 8.415575281601705876E-17 ) ) ;
#13308=CARTESIAN_POINT ( 'NONE',  ( 0.4593175853018380828, 0.05413385826771626580, -0.4176697321401330321 ) ) ;
#13309=CARTESIAN_POINT ( 'NONE',  ( 1.574803149606299746, -0.1870078740157479769, 0.4822834645669291653 ) ) ;
#13310=CARTESIAN_POINT ( 'NONE',  ( -1.614173228346456268, -0.5511811023622047445, 6.969142054262312111E-17 ) ) ;
#13315=CARTESIAN_POINT ( 'NONE',  ( 1.003937007874016407, -0.4536011799217367080, 0.2665933059059888421 ) ) ;
#13316=CARTESIAN_POINT ( 'NONE',  ( 0.2493438320209980519, -0.3690944881889765550, -0.3153832671262227771 ) ) ;
#13317=CARTESIAN_POINT ( 'NONE',  ( 0.2493438320209980519, -0.4281496062992127816, -0.4176697321401328100 ) ) ;
#13318=CARTESIAN_POINT ( 'NONE',  ( 1.345144356955381593, -0.3162353388693409650, -0.4822834645669289433 ) ) ;
#13320=CARTESIAN_POINT ( 'NONE',  ( 0.3083989501312343062, -0.08942795157528024563, -0.3641732283464568787 ) ) ;
#13321=CARTESIAN_POINT ( 'NONE',  ( -0.6561679790026240244, 0.2306618581243847221, -0.2411417322834647770 ) ) ;
#13322=CARTESIAN_POINT ( 'NONE',  ( -1.286089238845143479, 0.2306618581243847221, -0.2411417322834647770 ) ) ;
#13323=CARTESIAN_POINT ( 'NONE',  ( 0.8070866141732289112, -0.5400638737290845981, -0.3530559997133363437 ) ) ;
#13325=CARTESIAN_POINT ( 'NONE',  ( -0.7545931758530176614, 0.2952755905511811885, 0.1292274648535926551 ) ) ;
#13328=CARTESIAN_POINT ( 'NONE',  ( -1.161417322834644716, -0.5400638737290845981, -0.3530559997133363437 ) ) ;
#13329=CARTESIAN_POINT ( 'NONE',  ( -0.4855643044619415427, 0.05413385826771626580, -0.4176697321401330321 ) ) ;
#13330=CARTESIAN_POINT ( 'NONE',  ( -0.8070866141732276899, 0.07958543189024071263, -0.2665933059059888421 ) ) ;
#13331=CARTESIAN_POINT ( 'NONE',  ( -0.9120734908136475250, -0.6692913385826773087, -0.1292274648535924053 ) ) ;
#13334=CARTESIAN_POINT ( 'NONE',  ( 1.614173228346457378, -0.6692913385826771977, 8.415575281601705876E-17 ) ) ;
#13335=CARTESIAN_POINT ( 'NONE',  ( -1.030183727034119867, -0.05778040916215560624, -0.4822834645669293319 ) ) ;
#13336=CARTESIAN_POINT ( 'NONE',  ( 0.1837270341207354329, 0.2306618581243848609, 0.2411417322834645549 ) ) ;
#13337=CARTESIAN_POINT ( 'NONE',  ( -0.6496062992125976043, 0.1660481256975883668, -0.3530559997133364547 ) ) ;
#13339=CARTESIAN_POINT ( 'NONE',  ( -0.8727034120734901146, -0.2845877964562159024, 0.3641732283464567677 ) ) ;
#13340=ORIENTED_EDGE ( 'NONE', *, *, #49331, .F. ) ;
#13344=CARTESIAN_POINT ( 'NONE',  ( -0.9317585301837263412, 0.05413385826771666132, 0.4176697321401328100 ) ) ;
#13345=CARTESIAN_POINT ( 'NONE',  ( -1.358267716535432434, -0.5400638737290844871, 0.3530559997133364547 ) ) ;
#13347=CARTESIAN_POINT ( 'NONE',  ( -1.174540682414697335, -0.3162353388693409650, -0.4822834645669289433 ) ) ;
#13348=CARTESIAN_POINT ( 'NONE',  ( -1.246719160104986512, 0.05413385826771666132, 0.4176697321401328100 ) ) ;
#13351=CARTESIAN_POINT ( 'NONE',  ( 1.595398199321655275, 1.288687073698532526, -0.1559797534342494130 ) ) ;
#13352=CARTESIAN_POINT ( 'NONE',  ( 0.07874015748031558404, -0.1870078740157479769, 0.3641732283464567677 ) ) ;
#13355=CARTESIAN_POINT ( 'NONE',  ( -0.2099737532808391705, -0.5023911411419708095, -0.1820866141732282451 ) ) ;
#13356=CARTESIAN_POINT ( 'NONE',  ( -0.8202099737532799750, 0.2952755905511810774, -0.1292274648535930714 ) ) ;
#13357=CARTESIAN_POINT ( 'NONE',  ( 1.154855643044620184, 0.2306618581243847221, -0.2411417322834647770 ) ) ;
#13358=CARTESIAN_POINT ( 'NONE',  ( -0.6167979002624665030, -0.4281496062992127816, -0.4176697321401328100 ) ) ;
#13359=ORIENTED_EDGE ( 'NONE', *, *, #70319, .T. ) ;
#13362=CARTESIAN_POINT ( 'NONE',  ( -1.161417322834644716, 0.1660481256975885056, 0.3530559997133364547 ) ) ;
#13363=CARTESIAN_POINT ( 'NONE',  ( 1.220472440944882386, -0.6692913385826771977, 8.415575281601705876E-17 ) ) ;
#13364=CARTESIAN_POINT ( 'NONE',  ( -1.292650918635170010, -0.5511811023622046335, 0.09757992244046803654 ) ) ;
#13365=CARTESIAN_POINT ( 'NONE',  ( -1.476377952755905110, -0.5400638737290845981, -0.3530559997133363437 ) ) ;
#13370=CARTESIAN_POINT ( 'NONE',  ( 0.1771653543307093182, -0.5400638737290845981, -0.3530559997133363437 ) ) ;
#13371=CARTESIAN_POINT ( 'NONE',  ( -1.515748031496062076, -0.4536011799217367080, 0.2665933059059888421 ) ) ;
#13372=CARTESIAN_POINT ( 'NONE',  ( -0.7349081364829390672, 0.2306618581243847221, -0.2411417322834647770 ) ) ;
#13374=CARTESIAN_POINT ( 'NONE',  ( -1.200787401574802349, 0.1660481256975883668, -0.3530559997133364547 ) ) ;
#13375=CARTESIAN_POINT ( 'NONE',  ( -0.2230971128608915943, 0.05413385826771666132, 0.4176697321401328100 ) ) ;
#13376=CARTESIAN_POINT ( 'NONE',  ( -0.8136482939632537770, -0.6046776061558807314, 0.2411417322834647770 ) ) ;
#13377=CARTESIAN_POINT ( 'NONE',  ( -0.4855643044619415427, -0.4281496062992124485, 0.4176697321401328655 ) ) ;
#13379=CARTESIAN_POINT ( 'NONE',  ( 1.062992125984252745, -0.5511811023622047445, 6.969142054262312111E-17 ) ) ;
#13380=CARTESIAN_POINT ( 'NONE',  ( -0.8464566929133852113, -0.4536011799217368745, -0.2665933059059886201 ) ) ;
#13382=CARTESIAN_POINT ( 'NONE',  ( 0.9186351706036752773, 0.1283753931104746893, -0.1820866141732285504 ) ) ;
#13383=CARTESIAN_POINT ( 'NONE',  ( 1.318897637795276356, 0.07958543189024071263, -0.2665933059059888421 ) ) ;
#13384=CARTESIAN_POINT ( 'NONE',  ( 1.555118110236221041, -0.5400638737290844871, 0.3530559997133364547 ) ) ;
#13386=CARTESIAN_POINT ( 'NONE',  ( 0.2952755905511819101, 0.07958543189024071263, -0.2665933059059888421 ) ) ;
#13388=CARTESIAN_POINT ( 'NONE',  ( -0.8136482939632537770, 0.2306618581243847221, -0.2411417322834647770 ) ) ;
#13389=CARTESIAN_POINT ( 'NONE',  ( 1.332020997375328974, -0.05778040916215560624, -0.4822834645669293319 ) ) ;
#13391=CARTESIAN_POINT ( 'NONE',  ( -0.4133858267716528645, -0.4536011799217367080, 0.2665933059059888421 ) ) ;
#13393=CARTESIAN_POINT ( 'NONE',  ( 0.4199475065616805614, 0.2306618581243848609, 0.2411417322834645549 ) ) ;
#13394=DIRECTION ( 'NONE',  ( 1.000000000000000000, -0.000000000000000000, -0.000000000000000000 ) ) ;
#13395=CARTESIAN_POINT ( 'NONE',  ( 0.9514435695538062676, -0.08942795157527998196, 0.3641732283464567121 ) ) ;
#13396=CARTESIAN_POINT ( 'NONE',  ( 0.3674540682414705883, 0.1283753931104746893, -0.1820866141732285504 ) ) ;
#13397=CARTESIAN_POINT ( 'NONE',  ( -0.2034120734908128059, 0.2952755905511811885, 0.1292274648535926551 ) ) ;
#13398=CARTESIAN_POINT ( 'NONE',  ( -1.482939632545930975, -0.4281496062992127816, -0.4176697321401328100 ) ) ;
#13399=CARTESIAN_POINT ( 'NONE',  ( -0.6692913385826764205, 0.1771653543307087630, 0.000000000000000000 ) ) ;
#13401=CARTESIAN_POINT ( 'NONE',  ( -0.7874015748031489847, -0.1870078740157480879, -0.4822834645669291653 ) ) ;
#13404=CARTESIAN_POINT ( 'NONE',  ( 0.006561679790026889343, -0.08942795157527998196, 0.3641732283464567121 ) ) ;
#13405=CARTESIAN_POINT ( 'NONE',  ( -0.8530183727034112984, 0.05413385826771666132, 0.4176697321401328100 ) ) ;
#13406=CARTESIAN_POINT ( 'NONE',  ( -1.141732283464566011, 0.2952755905511811885, 0.000000000000000000 ) ) ;
#13407=CARTESIAN_POINT ( 'NONE',  ( -1.154855643044618851, 0.1283753931104748280, 0.1820866141732283561 ) ) ;
#13409=CARTESIAN_POINT ( 'NONE',  ( -0.9711286089238838626, 0.1283753931104746893, -0.1820866141732285504 ) ) ;
#13410=CARTESIAN_POINT ( 'NONE',  ( -1.469816272965878357, -0.5023911411419708095, -0.1820866141732282451 ) ) ;
#13411=CARTESIAN_POINT ( 'NONE',  ( 1.207349081364829990, -0.6046776061558809534, -0.2411417322834644161 ) ) ;
#13415=CARTESIAN_POINT ( 'NONE',  ( 1.603475055217291612, 1.054977578535739369, -0.04573490813648244807 ) ) ;
#13416=CARTESIAN_POINT ( 'NONE',  ( -1.614173228346456268, -0.6692913385826771977, 8.415575281601705876E-17 ) ) ;
#13417=CARTESIAN_POINT ( 'NONE',  ( -1.469816272965878357, -0.6046776061558809534, -0.2411417322834644161 ) ) ;
#13418=CARTESIAN_POINT ( 'NONE',  ( 1.227034120734908917, -0.6692913385826771977, 0.1292274648535927661 ) ) ;
#13420=CARTESIAN_POINT ( 'NONE',  ( 1.673228346456693494, 0.07958543189024085140, 0.2665933059059887866 ) ) ;
#13422=CARTESIAN_POINT ( 'NONE',  ( 0.5052493438320218022, -0.6692913385826773087, -0.1292274648535924053 ) ) ;
#13423=CARTESIAN_POINT ( 'NONE',  ( -0.1640419947506553400, -0.05778040916215560624, -0.4822834645669293319 ) ) ;
#13424=CARTESIAN_POINT ( 'NONE',  ( -0.6983222978630787559, 2.320010949979154579E-15, 0.4281993546915509041 ) ) ;
#13426=CARTESIAN_POINT ( 'NONE',  ( 0.9711286089238851948, 0.1283753931104748280, 0.1820866141732283561 ) ) ;
#13431=CARTESIAN_POINT ( 'NONE',  ( -0.1968503937007867743, -0.6692913385826771977, 8.415575281601705876E-17 ) ) ;
#13432=CARTESIAN_POINT ( 'NONE',  ( -1.476377952755905110, 0.1660481256975885056, 0.3530559997133364547 ) ) ;
#13433=CARTESIAN_POINT ( 'NONE',  ( 0.4461942257217856311, 0.2306618581243847221, -0.2411417322834647770 ) ) ;
#13434=CARTESIAN_POINT ( 'NONE',  ( 1.377952755905512472, 0.2952755905511811885, 0.000000000000000000 ) ) ;
#13435=CARTESIAN_POINT ( 'NONE',  ( 1.443569553805774897, 0.2306618581243848609, 0.2411417322834645549 ) ) ;
#13436=CARTESIAN_POINT ( 'NONE',  ( -0.6627296587926501115, 0.2952755905511810774, -0.1292274648535930714 ) ) ;
#13437=CARTESIAN_POINT ( 'NONE',  ( 0.1377952755905518800, -0.5400638737290844871, 0.3530559997133364547 ) ) ;
#13438=CARTESIAN_POINT ( 'NONE',  ( 1.410761154855643795, -0.3162353388693405765, 0.4822834645669290543 ) ) ;
#13439=CARTESIAN_POINT ( 'NONE',  ( 1.528871391076116026, -0.6692913385826773087, -0.1292274648535924053 ) ) ;
#13440=CARTESIAN_POINT ( 'NONE',  ( 1.017060367454068803, -0.3162353388693405765, 0.4822834645669290543 ) ) ;
#13441=CARTESIAN_POINT ( 'NONE',  ( -0.1377952755905504645, 0.1660481256975885056, 0.3530559997133364547 ) ) ;
#13443=CARTESIAN_POINT ( 'NONE',  ( 0.2559055118110243332, 0.07958543189024085140, 0.2665933059059887866 ) ) ;
#13444=ORIENTED_EDGE ( 'NONE', *, *, #61281, .F. ) ;
#13447=CARTESIAN_POINT ( 'NONE',  ( -0.6299212598425188991, -0.1870078740157479769, 0.3641732283464567677 ) ) ;
#13449=CARTESIAN_POINT ( 'NONE',  ( 0.1312335958005255154, -0.6046776061558807314, 0.2411417322834647770 ) ) ;
#13450=CARTESIAN_POINT ( 'NONE',  ( -0.2034120734908131112, -0.6692913385826773087, -0.1292274648535924053 ) ) ;
#13451=CARTESIAN_POINT ( 'NONE',  ( -1.076115485564303809, 0.2306618581243848609, 0.2411417322834645549 ) ) ;
#13453=CARTESIAN_POINT ( 'NONE',  ( -1.522309711286088607, -0.6046776061558807314, 0.2411417322834647770 ) ) ;
#13454=CARTESIAN_POINT ( 'NONE',  ( -0.1459841489473561460, -2.624320362099288585E-15, 0.3791475997938241749 ) ) ;
#13455=CARTESIAN_POINT ( 'NONE',  ( 0.9908136482939640111, 0.1771653543307087075, -0.09757992244046823083 ) ) ;
#13456=CARTESIAN_POINT ( 'NONE',  ( 0.3937007874015754361, -0.1870078740157479769, 0.4822834645669291653 ) ) ;
#13457=CARTESIAN_POINT ( 'NONE',  ( 0.8661417322834653598, -0.1870078740157479769, 0.4822834645669291653 ) ) ;
#13462=CARTESIAN_POINT ( 'NONE',  ( -0.09186351706036689768, 0.05413385826771626580, -0.4176697321401330321 ) ) ;
#13465=CARTESIAN_POINT ( 'NONE',  ( -1.299212598425196097, 0.1771653543307087630, 0.000000000000000000 ) ) ;
#13466=CARTESIAN_POINT ( 'NONE',  ( 1.332020997375328974, -0.05778040916215560624, -0.4822834645669293319 ) ) ;
#13467=CARTESIAN_POINT ( 'NONE',  ( 1.154855643044620184, -0.6046776061558807314, 0.2411417322834647770 ) ) ;
#13468=CARTESIAN_POINT ( 'NONE',  ( 0.2493438320209980519, -0.004921259842519576551, 0.3153832671262227771 ) ) ;
#13469=CARTESIAN_POINT ( 'NONE',  ( 0.5774278215223103139, -0.6046776061558809534, -0.2411417322834644161 ) ) ;
#13471=CARTESIAN_POINT ( 'NONE',  ( 0.3805774278215230400, -0.3690944881889763329, 0.3153832671262228327 ) ) ;
#13472=CARTESIAN_POINT ( 'NONE',  ( -0.006561679790025524116, -0.3162353388693405765, 0.4822834645669290543 ) ) ;
#13474=CARTESIAN_POINT ( 'NONE',  ( -1.410761154855642463, -0.05778040916215522460, 0.4822834645669289988 ) ) ;
#13475=CARTESIAN_POINT ( 'NONE',  ( 0.4658792650918640033, -0.2845877964562159024, 0.3641732283464567677 ) ) ;
#13477=CARTESIAN_POINT ( 'NONE',  ( -0.6167979002624665030, 0.05413385826771666132, 0.4176697321401328100 ) ) ;
#13478=CARTESIAN_POINT ( 'NONE',  ( -0.2034120734908128059, 0.1771653543307087630, 0.09757992244046791164 ) ) ;
#13480=CARTESIAN_POINT ( 'NONE',  ( -0.9251968503937002541, 0.1660481256975885056, 0.3530559997133364547 ) ) ;
#13481=CARTESIAN_POINT ( 'NONE',  ( -0.1968503937007867743, 0.2952755905511811885, 0.000000000000000000 ) ) ;
#13482=CARTESIAN_POINT ( 'NONE',  ( 0.1640419947506569498, -0.08942795157527998196, 0.3641732283464567121 ) ) ;
#13484=CARTESIAN_POINT ( 'NONE',  ( 0.07217847769028949700, -0.3162353388693405765, 0.4822834645669290543 ) ) ;
#13487=CARTESIAN_POINT ( 'NONE',  ( 0.7545931758530189937, 0.1771653543307087075, -0.09757992244046823083 ) ) ;
#13488=CARTESIAN_POINT ( 'NONE',  ( 1.259842519685040019, -0.1870078740157479769, 0.4822834645669291653 ) ) ;
#13489=CARTESIAN_POINT ( 'NONE',  ( -0.8333333333333323711, -0.5511811023622048555, -0.09757992244046775898 ) ) ;
#13490=CARTESIAN_POINT ( 'NONE',  ( -1.332020997375327642, -0.2845877964562161244, -0.3641732283464567121 ) ) ;
#13491=CARTESIAN_POINT ( 'NONE',  ( -0.6299212598425188991, -0.1870078740157480879, -0.4822834645669291653 ) ) ;
#13492=CARTESIAN_POINT ( 'NONE',  ( -0.01312335958005186876, -0.4281496062992124485, 0.4176697321401328655 ) ) ;
#13493=CARTESIAN_POINT ( 'NONE',  ( 0.3740157480314966754, -0.4536011799217367080, 0.2665933059059888421 ) ) ;
#13495=CARTESIAN_POINT ( 'NONE',  ( 1.017060367454068581, -0.08942795157528024563, -0.3641732283464568787 ) ) ;
#13496=CARTESIAN_POINT ( 'NONE',  ( 0.4461942257217856311, 0.2306618581243847221, -0.2411417322834647770 ) ) ;
#13498=CARTESIAN_POINT ( 'NONE',  ( -0.2887139107611542133, 0.2306618581243848609, 0.2411417322834645549 ) ) ;
#13500=CARTESIAN_POINT ( 'NONE',  ( -1.699475065616797398, 0.2952755905511811885, 0.1292274648535926551 ) ) ;
#13501=CARTESIAN_POINT ( 'NONE',  ( 0.4593175853018380828, 0.05413385826771626580, -0.4176697321401330321 ) ) ;
#13502=CARTESIAN_POINT ( 'NONE',  ( 0.2165354330708668673, -0.5400638737290844871, 0.3530559997133364547 ) ) ;
#13504=CARTESIAN_POINT ( 'NONE',  ( 0.1640419947506569498, -0.2845877964562161244, -0.3641732283464567121 ) ) ;
#13505=CARTESIAN_POINT ( 'NONE',  ( 0.6496062992125991586, -0.5400638737290845981, -0.3530559997133363437 ) ) ;
#13506=CARTESIAN_POINT ( 'NONE',  ( -0.3871391076115479057, -0.2845877964562161244, -0.3641732283464567121 ) ) ;
#13507=CARTESIAN_POINT ( 'NONE',  ( -0.7020997375328074108, -0.05778040916215522460, 0.4822834645669289988 ) ) ;
#13509=CARTESIAN_POINT ( 'NONE',  ( 0.04593175853018440641, 0.2952755905511810774, -0.1292274648535930714 ) ) ;
#13510=VERTEX_POINT ( 'NONE', #46810 ) ;
#13511=CARTESIAN_POINT ( 'NONE',  ( -1.010498687664041384, 0.05413385826771666132, 0.4176697321401328100 ) ) ;
#13512=CARTESIAN_POINT ( 'NONE',  ( -0.5708661417322828946, 0.07958543189024071263, -0.2665933059059888421 ) ) ;
#13513=CARTESIAN_POINT ( 'NONE',  ( 0.01312335958005323398, 0.05413385826771666132, 0.4176697321401328100 ) ) ;
#13514=CARTESIAN_POINT ( 'NONE',  ( -1.325459317585300889, -0.4281496062992127816, -0.4176697321401328100 ) ) ;
#13515=CARTESIAN_POINT ( 'NONE',  ( -0.8792650918635160906, -0.4281496062992124485, 0.4176697321401328655 ) ) ;
#13516=( BOUNDED_CURVE ( )  B_SPLINE_CURVE ( 2, ( #76210, #49282, #23201, #43361, #68258, #18139, #69062, #10594, #82118, #56824, #69476, #35844, #74572 ),
 .UNSPECIFIED., .F., .F. ) 
 B_SPLINE_CURVE_WITH_KNOTS ( ( 3, 2, 2, 2, 2, 2, 3 ),
 ( 0.4467605387524145044, 0.4469696969696969613, 0.4507575757575757458, 0.4545454545454545303, 0.4583333333333333148, 0.4621212121212120993, 0.4623303703384945562 ),
 .UNSPECIFIED. ) 
 CURVE ( )  GEOMETRIC_REPRESENTATION_ITEM ( )  RATIONAL_B_SPLINE_CURVE ( ( 0.9964447847208428577, 0.9981185001348096275, 1.000000000000000000, 0.9659258262890683122, 1.000000000000000000, 0.9659258262890683122, 1.000000000000000000, 0.9659258262890683122, 1.000000000000000000, 0.9659258262890683122, 1.000000000000000000, 0.9981185001348097385, 0.9964447847208430797 ) ) 
 REPRESENTATION_ITEM ( '' )  );
#13518=CARTESIAN_POINT ( 'NONE',  ( 1.035207913594496709, 0.02791078216816225699, 0.4328096321851905293 ) ) ;
#13519=CARTESIAN_POINT ( 'NONE',  ( 1.555118110236221041, -0.5400638737290844871, 0.3530559997133364547 ) ) ;
#13520=CARTESIAN_POINT ( 'NONE',  ( 1.207349081364829990, 0.2306618581243848609, 0.2411417322834645549 ) ) ;
#13523=CARTESIAN_POINT ( 'NONE',  ( -1.174540682414697335, -0.3162353388693409650, -0.4822834645669289433 ) ) ;
#13526=ORIENTED_EDGE ( 'NONE', *, *, #32799, .T. ) ;
#13527=CARTESIAN_POINT ( 'NONE',  ( -0.1706036745406816491, -0.004921259842519870586, -0.3153832671262229437 ) ) ;
#13529=ORIENTED_EDGE ( 'NONE', *, *, #12532, .T. ) ;
#13530=CARTESIAN_POINT ( 'NONE',  ( 0.3477690288713918276, 0.2952755905511811885, 0.1292274648535926551 ) ) ;
#13531=CARTESIAN_POINT ( 'NONE',  ( 0.3477690288713918276, 0.2952755905511811885, 0.1292274648535926551 ) ) ;
#13533=CARTESIAN_POINT ( 'NONE',  ( -0.5387615594602663815, -2.294479370626195693E-15, 0.3464511005275217603 ) ) ;
#13534=CARTESIAN_POINT ( 'NONE',  ( -0.7939632545931750718, -0.08942795157528024563, -0.3641732283464568787 ) ) ;
#13536=CARTESIAN_POINT ( 'NONE',  ( 0.8398950131233602345, -0.6046776061558807314, 0.2411417322834647770 ) ) ;
#13537=CARTESIAN_POINT ( 'NONE',  ( 0.8530183727034126306, -0.004921259842519870586, -0.3153832671262229437 ) ) ;
#13538=CIRCLE ( 'NONE', #39054, 3.543307086614174484 ) ;
#13539=CARTESIAN_POINT ( 'NONE',  ( -0.2165354330708654795, 0.1660481256975885056, 0.3530559997133364547 ) ) ;
#13541=CARTESIAN_POINT ( 'NONE',  ( -0.9383202099737524282, -0.3162353388693409650, -0.4822834645669289433 ) ) ;
#13542=CARTESIAN_POINT ( 'NONE',  ( -1.614173228346456268, -0.5511811023622047445, 6.969142054262312111E-17 ) ) ;
#13543=CARTESIAN_POINT ( 'NONE',  ( -0.8595800524934373854, -0.3162353388693409650, -0.4822834645669289433 ) ) ;
#13544=CARTESIAN_POINT ( 'NONE',  ( 1.377952755905512472, 0.2952755905511811885, 0.000000000000000000 ) ) ;
#13545=CARTESIAN_POINT ( 'NONE',  ( 1.692913385826772421, 0.1771653543307087630, 0.000000000000000000 ) ) ;
#13548=CARTESIAN_POINT ( 'NONE',  ( -0.01968503937007793844, 0.1660481256975883668, -0.3530559997133364547 ) ) ;
#13550=CARTESIAN_POINT ( 'NONE',  ( -0.7414698162729651543, 0.2952755905511810774, -0.1292274648535930714 ) ) ;
#13551=CARTESIAN_POINT ( 'NONE',  ( 1.450131233595801428, 0.2952755905511811885, 0.1292274648535926551 ) ) ;
#13552=CARTESIAN_POINT ( 'NONE',  ( 1.200787401574803681, -0.5400638737290845981, -0.3530559997133363437 ) ) ;
#13553=CARTESIAN_POINT ( 'NONE',  ( 0.4593175853018379162, -0.4281496062992124485, 0.4176697321401328655 ) ) ;
#13554=CARTESIAN_POINT ( 'NONE',  ( -0.06561679790026180015, 0.05413385826771666132, 0.4176697321401328100 ) ) ;
#13556=CARTESIAN_POINT ( 'NONE',  ( -1.325459317585300889, -0.4281496062992127816, -0.4176697321401328100 ) ) ;
#13557=CARTESIAN_POINT ( 'NONE',  ( -0.2690288713910754526, -0.6692913385826771977, 0.1292274648535927661 ) ) ;
#13558=CARTESIAN_POINT ( 'NONE',  ( -0.2296587926509179312, -0.08942795157527998196, 0.3641732283464567121 ) ) ;
#13559=CARTESIAN_POINT ( 'NONE',  ( 1.627296587926509996, -0.6046776061558807314, 0.2411417322834647770 ) ) ;
#13562=CARTESIAN_POINT ( 'NONE',  ( 1.469816272965879911, -0.6046776061558807314, 0.2411417322834647770 ) ) ;
#13563=CARTESIAN_POINT ( 'NONE',  ( -0.3018372703412066094, 0.05413385826771666132, 0.4176697321401328100 ) ) ;
#13565=CARTESIAN_POINT ( 'NONE',  ( 1.161417322834646271, 0.1660481256975883668, -0.3530559997133364547 ) ) ;
#13568=EDGE_CURVE ( 'NONE', #82899, #22644, #18587, .T. ) ;
#13570=CARTESIAN_POINT ( 'NONE',  ( 0.2755905511811031494, 0.2952755905511811885, 0.000000000000000000 ) ) ;
#13571=CARTESIAN_POINT ( 'NONE',  ( -0.1640419947506555343, -0.2845877964562159024, 0.3641732283464567677 ) ) ;
#13572=CARTESIAN_POINT ( 'NONE',  ( 1.358267716535433323, 0.07958543189024085140, 0.2665933059059887866 ) ) ;
#13573=CARTESIAN_POINT ( 'NONE',  ( -0.7535225988626923499, 2.401574803149606474, -0.4915354330708644470 ) ) ;
#13575=CARTESIAN_POINT ( 'NONE',  ( 1.548556430446194954, 0.1283753931104746893, -0.1820866141732285504 ) ) ;
#13576=CARTESIAN_POINT ( 'NONE',  ( 1.181102362204724976, -0.1870078740157480879, -0.4822834645669291653 ) ) ;
#13578=CARTESIAN_POINT ( 'NONE',  ( 0.1181102362204730916, -0.6692913385826771977, 8.415575281601705876E-17 ) ) ;
#13579=CARTESIAN_POINT ( 'NONE',  ( -1.476377952755905110, 0.1660481256975885056, 0.3530559997133364547 ) ) ;
#13580=CARTESIAN_POINT ( 'NONE',  ( -1.692913385826770645, 0.2952755905511811885, 0.000000000000000000 ) ) ;
#13581=CARTESIAN_POINT ( 'NONE',  ( -0.2296587926509179312, -0.3162353388693409650, -0.4822834645669289433 ) ) ;
#13583=CARTESIAN_POINT ( 'NONE',  ( -1.502624671916009680, -0.2845877964562159024, 0.3641732283464567677 ) ) ;
#13584=CARTESIAN_POINT ( 'NONE',  ( 0.3215223097112867578, -0.05778040916215522460, 0.4822834645669289988 ) ) ;
#13585=CARTESIAN_POINT ( 'NONE',  ( 0.9711286089238851948, -0.5023911411419708095, -0.1820866141732282451 ) ) ;
#13586=CARTESIAN_POINT ( 'NONE',  ( -0.06715429112991272431, 0.02791078216816064370, 0.4328096321851915285 ) ) ;
#13587=CARTESIAN_POINT ( 'NONE',  ( 0.7414698162729663755, 0.1771653543307087630, 0.09757992244046791164 ) ) ;
#13588=CARTESIAN_POINT ( 'NONE',  ( -1.174540682414697335, -0.05778040916215522460, 0.4822834645669289988 ) ) ;
#13590=CARTESIAN_POINT ( 'NONE',  ( 1.108923884514436686, -0.3162353388693409650, -0.4822834645669289433 ) ) ;
#13594=CARTESIAN_POINT ( 'NONE',  ( 0.6889763779527566800, -0.5400638737290844871, 0.3530559997133364547 ) ) ;
#13595=CARTESIAN_POINT ( 'NONE',  ( 0.9055118110236227702, 0.2952755905511811885, 0.000000000000000000 ) ) ;
#13596=CARTESIAN_POINT ( 'NONE',  ( -0.3346456692913378217, 0.1012011053420775880, -0.2882089793578256898 ) ) ;
#13597=CARTESIAN_POINT ( 'NONE',  ( 0.5314960629921264834, 0.07958543189024071263, -0.2665933059059888421 ) ) ;
#13598=CARTESIAN_POINT ( 'NONE',  ( 0.4133858267716541968, 0.1660481256975885056, 0.3530559997133364547 ) ) ;
#13600=CARTESIAN_POINT ( 'NONE',  ( -1.122047244094487306, -0.4536011799217367080, 0.2665933059059888421 ) ) ;
#13601=CARTESIAN_POINT ( 'NONE',  ( -0.8136482939632537770, -0.6046776061558807314, 0.2411417322834647770 ) ) ;
#13602=CARTESIAN_POINT ( 'NONE',  ( 1.135170603674541256, -0.6692913385826773087, -0.1292274648535924053 ) ) ;
#13603=CARTESIAN_POINT ( 'NONE',  ( -1.076115485564303809, 0.2306618581243848609, 0.2411417322834645549 ) ) ;
#13604=CARTESIAN_POINT ( 'NONE',  ( 0.8398950131233602345, -0.6046776061558807314, 0.2411417322834647770 ) ) ;
#13605=CARTESIAN_POINT ( 'NONE',  ( -1.167979002624671470, -0.004921259842519576551, 0.3153832671262227771 ) ) ;
#13606=DIRECTION ( 'NONE',  ( 1.000000000000000000, -0.000000000000000000, -0.000000000000000000 ) ) ;
#13607=CARTESIAN_POINT ( 'NONE',  ( 1.076115485564305141, -0.6046776061558807314, 0.2411417322834647770 ) ) ;
#13609=CARTESIAN_POINT ( 'NONE',  ( 1.633858267716535639, -0.5400638737290844871, 0.3530559997133364547 ) ) ;
#13610=CARTESIAN_POINT ( 'NONE',  ( 1.509186351706037543, 0.05413385826771666132, 0.4176697321401328100 ) ) ;
#13611=CARTESIAN_POINT ( 'NONE',  ( -1.620734908136482577, -0.5511811023622048555, -0.09757992244046775898 ) ) ;
#13612=CARTESIAN_POINT ( 'NONE',  ( 1.450131233595801428, -0.5511811023622048555, -0.09757992244046775898 ) ) ;
#13613=CARTESIAN_POINT ( 'NONE',  ( -1.108923884514435132, -0.08942795157528024563, -0.3641732283464568787 ) ) ;
#13614=CARTESIAN_POINT ( 'NONE',  ( -0.4724409448818890911, -0.1870078740157480601, -0.3641732283464567677 ) ) ;
#13615=CARTESIAN_POINT ( 'NONE',  ( -1.423884514435694859, -0.2845877964562159024, 0.3641732283464567677 ) ) ;
#13616=CARTESIAN_POINT ( 'NONE',  ( 0.9186351706036751663, -0.5023911411419708095, 0.1820866141732285504 ) ) ;
#13617=CARTESIAN_POINT ( 'NONE',  ( 0.6627296587926517768, -0.6692913385826773087, -0.1292274648535924053 ) ) ;
#13618=CARTESIAN_POINT ( 'NONE',  ( 1.049868766404200127, -0.6046776061558809534, -0.2411417322834644161 ) ) ;
#13619=CARTESIAN_POINT ( 'NONE',  ( 0.1706036745406830368, -0.4281496062992127816, -0.4176697321401328100 ) ) ;
#13620=ADVANCED_FACE ( 'NONE', ( #17340 ), #42995, .F. ) ;
#13622=CARTESIAN_POINT ( 'NONE',  ( 0.7020997375328090762, -0.08942795157528024563, -0.3641732283464568787 ) ) ;
#13623=CARTESIAN_POINT ( 'NONE',  ( 1.528871391076116026, -0.6692913385826773087, -0.1292274648535924053 ) ) ;
#13624=CARTESIAN_POINT ( 'NONE',  ( -1.541994750656167090, -0.6692913385826773087, -0.1292274648535924053 ) ) ;
#13625=CARTESIAN_POINT ( 'NONE',  ( -0.5314960629921254842, -0.5400638737290845981, -0.3530559997133363437 ) ) ;
#13628=CARTESIAN_POINT ( 'NONE',  ( 0.1574803149606306130, -0.1870078740157479769, 0.4822834645669291653 ) ) ;
#13629=CARTESIAN_POINT ( 'NONE',  ( -0.4330708661417315697, -0.6692913385826771977, 8.415575281601705876E-17 ) ) ;
#13630=CARTESIAN_POINT ( 'NONE',  ( -0.04593175853018302557, -0.6692913385826773087, -0.1292274648535924053 ) ) ;
#13634=CARTESIAN_POINT ( 'NONE',  ( 2.795275590551181466, 2.001539355558160871, 0.000000000000000000 ) ) ;
#13636=CARTESIAN_POINT ( 'NONE',  ( -0.7545931758530177724, 0.1771653543307087630, 0.09757992244046791164 ) ) ;
#13638=CARTESIAN_POINT ( 'NONE',  ( -1.128608923884513837, -0.6046776061558807314, 0.2411417322834647770 ) ) ;
#13641=CARTESIAN_POINT ( 'NONE',  ( 0.2427821522309719648, -0.05778040916215522460, 0.4822834645669289988 ) ) ;
#13642=CARTESIAN_POINT ( 'NONE',  ( -0.2099737532808391705, -0.5023911411419708095, -0.1820866141732282451 ) ) ;
#13643=CARTESIAN_POINT ( 'NONE',  ( 1.207349081364829990, -0.6046776061558809534, -0.2411417322834644161 ) ) ;
#13644=CARTESIAN_POINT ( 'NONE',  ( 0.2559055118110243332, -0.5400638737290845981, -0.3530559997133363437 ) ) ;
#13648=CARTESIAN_POINT ( 'NONE',  ( 1.108923884514436686, -0.3162353388693409650, -0.4822834645669289433 ) ) ;
#13649=CARTESIAN_POINT ( 'NONE',  ( 0.3608923884514443348, 0.2952755905511810774, -0.1292274648535930714 ) ) ;
#13650=CARTESIAN_POINT ( 'NONE',  ( 0.1377952755905518800, -0.5400638737290844871, 0.3530559997133364547 ) ) ;
#13651=CARTESIAN_POINT ( 'NONE',  ( 1.489501312335958172, -0.3162353388693405765, 0.4822834645669290543 ) ) ;
#13653=CARTESIAN_POINT ( 'NONE',  ( 0.06561679790026316017, 0.05413385826771626580, -0.4176697321401330321 ) ) ;
#13654=CARTESIAN_POINT ( 'NONE',  ( 1.279527559055118724, -0.5400638737290845981, -0.3530559997133363437 ) ) ;
#13655=CARTESIAN_POINT ( 'NONE',  ( 0.2493438320209980519, 0.05413385826771666132, 0.4176697321401328100 ) ) ;
#13656=CARTESIAN_POINT ( 'NONE',  ( 1.181102362204725198, -0.1870078740157479769, 0.3641732283464567677 ) ) ;
#13657=CARTESIAN_POINT ( 'NONE',  ( -0.9186351706036736120, 0.2306618581243848609, 0.2411417322834645549 ) ) ;
#13658=CARTESIAN_POINT ( 'NONE',  ( -1.318897637795274802, -0.5400638737290845981, -0.3530559997133363437 ) ) ;
#13660=CARTESIAN_POINT ( 'NONE',  ( 0.8202099737532813073, 0.2952755905511811885, 0.1292274648535926551 ) ) ;
#13663=CARTESIAN_POINT ( 'NONE',  ( 1.660104986876641320, -0.05778040916215522460, 0.4822834645669289988 ) ) ;
#13668=CARTESIAN_POINT ( 'NONE',  ( 1.633858267716535639, -0.5400638737290844871, 0.3530559997133364547 ) ) ;
#13669=CARTESIAN_POINT ( 'NONE',  ( 0.9711286089238851948, 0.1283753931104748280, 0.1820866141732283561 ) ) ;
#13671=LINE ( 'NONE', #26701, #75950 ) ;
#13674=CARTESIAN_POINT ( 'NONE',  ( -1.299212598425196097, 0.1771653543307087630, 0.000000000000000000 ) ) ;
#13675=CARTESIAN_POINT ( 'NONE',  ( 1.614173228346457378, 0.2952755905511811885, 0.000000000000000000 ) ) ;
#13676=CARTESIAN_POINT ( 'NONE',  ( -1.515748031496062076, -0.5400638737290844871, 0.3530559997133364547 ) ) ;
#13677=CARTESIAN_POINT ( 'NONE',  ( -0.1640419947506555343, -0.3162353388693405765, 0.4822834645669290543 ) ) ;
#13678=CARTESIAN_POINT ( 'NONE',  ( 1.391076115485564868, -0.6046776061558807314, 0.2411417322834647770 ) ) ;
#13679=EDGE_LOOP ( 'NONE', ( #75350, #26159, #68618, #27998 ) ) ;
#13683=CARTESIAN_POINT ( 'NONE',  ( -0.7939632545931750718, -0.08942795157528024563, -0.3641732283464568787 ) ) ;
#13684=CARTESIAN_POINT ( 'NONE',  ( -1.456692913385826182, 0.2952755905511811885, 0.000000000000000000 ) ) ;
#13685=CARTESIAN_POINT ( 'NONE',  ( 0.6102362204724416372, 0.1660481256975883668, -0.3530559997133364547 ) ) ;
#13686=ORIENTED_EDGE ( 'NONE', *, *, #54850, .T. ) ;
#13687=CARTESIAN_POINT ( 'NONE',  ( -1.646051170424378096, 0.000000000000000000, -0.3464511005275205946 ) ) ;
#13688=CARTESIAN_POINT ( 'NONE',  ( 0.6962418744208975774, 2.409604939980833412E-17, -0.3464511005275205946 ) ) ;
#13689=CARTESIAN_POINT ( 'NONE',  ( 1.122047244094488860, -0.5400638737290845981, -0.3530559997133363437 ) ) ;
#13690=CARTESIAN_POINT ( 'NONE',  ( -1.627296587926508442, -0.6046776061558809534, -0.2411417322834644161 ) ) ;
#13692=CARTESIAN_POINT ( 'NONE',  ( -0.4199475065616791736, 0.1283753931104746893, -0.1820866141732285504 ) ) ;
#13693=CARTESIAN_POINT ( 'NONE',  ( -1.397637795275589623, -0.4536011799217368745, -0.2665933059059886201 ) ) ;
#13695=CARTESIAN_POINT ( 'NONE',  ( 0.3083989501312343062, -0.3162353388693405765, 0.4822834645669290543 ) ) ;
#13696=CARTESIAN_POINT ( 'NONE',  ( -0.8858267716535425107, -0.4536011799217367080, 0.2665933059059888421 ) ) ;
#13697=CARTESIAN_POINT ( 'NONE',  ( 0.01968503937007930540, 0.07958543189024085140, 0.2665933059059887866 ) ) ;
#13698=CARTESIAN_POINT ( 'NONE',  ( 0.1771653543307093182, 0.1660481256975885056, 0.3530559997133364547 ) ) ;
#13699=CARTESIAN_POINT ( 'NONE',  ( -0.9383202099737524282, -0.2845877964562161244, -0.3641732283464567121 ) ) ;
#13701=CARTESIAN_POINT ( 'NONE',  ( 0.7939632545931766261, -0.05778040916215522460, 0.4822834645669289988 ) ) ;
#13703=CARTESIAN_POINT ( 'NONE',  ( -1.614173228346455824, 0.2952755905511811885, 0.000000000000000000 ) ) ;
#13705=CARTESIAN_POINT ( 'NONE',  ( -0.4724409448818890911, -0.1870078740157479769, 0.4822834645669291653 ) ) ;
#13706=CARTESIAN_POINT ( 'NONE',  ( 0.2755905511811031494, -0.5511811023622047445, 6.969142054262312111E-17 ) ) ;
#13708=CARTESIAN_POINT ( 'NONE',  ( -1.036745406824146176, -0.4281496062992124485, 0.4176697321401328655 ) ) ;
#13709=CARTESIAN_POINT ( 'NONE',  ( 0.7217847769028878924, -0.004921259842519576551, 0.3153832671262227771 ) ) ;
#13710=CARTESIAN_POINT ( 'NONE',  ( -0.1049868766404193215, 0.1283753931104746893, -0.1820866141732285504 ) ) ;
#13711=CARTESIAN_POINT ( 'NONE',  ( -0.8464566929133852113, -0.5400638737290845981, -0.3530559997133363437 ) ) ;
#13712=CARTESIAN_POINT ( 'NONE',  ( -1.305774278215222184, -0.6692913385826773087, -0.1292274648535924053 ) ) ;
#13713=CARTESIAN_POINT ( 'NONE',  ( -1.410761154855641575, -0.3162353388693409650, -0.4822834645669289433 ) ) ;
#13715=CARTESIAN_POINT ( 'NONE',  ( 1.200787401574803681, 0.07958543189024085140, 0.2665933059059887866 ) ) ;
#13716=CARTESIAN_POINT ( 'NONE',  ( 0.3346456692913393205, -0.5400638737290845981, -0.3530559997133363437 ) ) ;
#13718=CARTESIAN_POINT ( 'NONE',  ( -1.351706036745406347, -0.4281496062992124485, 0.4176697321401328655 ) ) ;
#13719=CARTESIAN_POINT ( 'NONE',  ( -1.646981627296586703, -0.3162353388693409650, -0.4822834645669289433 ) ) ;
#13720=ORIENTED_EDGE ( 'NONE', *, *, #8454, .T. ) ;
#13722=CARTESIAN_POINT ( 'NONE',  ( -0.6758530183727028406, 0.1771653543307087630, 0.09757992244046791164 ) ) ;
#13723=CARTESIAN_POINT ( 'NONE',  ( 0.7677165354330716118, -0.5400638737290844871, 0.3530559997133364547 ) ) ;
#13724=CARTESIAN_POINT ( 'NONE',  ( -1.174540682414697335, -0.2845877964562161244, -0.3641732283464567121 ) ) ;
#13726=CARTESIAN_POINT ( 'NONE',  ( -0.9120734908136475250, 0.2952755905511811885, 0.1292274648535926551 ) ) ;
#13727=CARTESIAN_POINT ( 'NONE',  ( 0.8792650918635177559, 0.05413385826771666132, 0.4176697321401328100 ) ) ;
#13728=CARTESIAN_POINT ( 'NONE',  ( 0.6233595800524942554, -0.05778040916215560624, -0.4822834645669293319 ) ) ;
#13730=CARTESIAN_POINT ( 'NONE',  ( -1.541994750656167090, 0.1771653543307087630, 0.09757992244046791164 ) ) ;
#13735=CARTESIAN_POINT ( 'NONE',  ( 0.6430446194225729606, -0.3690944881889765550, -0.3153832671262227771 ) ) ;
#13736=CARTESIAN_POINT ( 'NONE',  ( 0.4593175853018379162, -0.3690944881889763329, 0.3153832671262228327 ) ) ;
#13737=CARTESIAN_POINT ( 'NONE',  ( -0.05249343832020938322, -0.6046776061558809534, -0.2411417322834644161 ) ) ;
#13738=CARTESIAN_POINT ( 'NONE',  ( 1.240157480314961314, -0.5400638737290844871, 0.3530559997133364547 ) ) ;
#13740=CARTESIAN_POINT ( 'NONE',  ( 0.5774278215223104249, 0.1283753931104748280, 0.1820866141732283561 ) ) ;
#13741=CARTESIAN_POINT ( 'NONE',  ( -0.9251968503937002541, -0.5400638737290845981, -0.3530559997133363437 ) ) ;
#13742=CARTESIAN_POINT ( 'NONE',  ( 1.450131233595801428, 0.2952755905511811885, 0.1292274648535926551 ) ) ;
#13743=CARTESIAN_POINT ( 'NONE',  ( 0.8136482939632553313, -0.6046776061558809534, -0.2411417322834644161 ) ) ;
#13745=DIRECTION ( 'NONE',  ( 3.114085624724525612E-16, -1.000000000000000000, -5.270319453084425600E-32 ) ) ;
#13748=CARTESIAN_POINT ( 'NONE',  ( -1.069553805774277722, 0.2952755905511811885, 0.1292274648535926551 ) ) ;
#13749=CARTESIAN_POINT ( 'NONE',  ( -1.213910761154854745, -0.6692913385826771977, 0.1292274648535927661 ) ) ;
#13750=CARTESIAN_POINT ( 'NONE',  ( -0.6496062992125976043, 0.07958543189024071263, -0.2665933059059888421 ) ) ;
#13751=CARTESIAN_POINT ( 'NONE',  ( -0.8333333333333323711, 0.2952755905511811885, 0.1292274648535926551 ) ) ;
#13753=CARTESIAN_POINT ( 'NONE',  ( -0.4609447788686161229, -1.429000049448402363E-15, 0.3791475997938249520 ) ) ;
#13754=CARTESIAN_POINT ( 'NONE',  ( 1.581364829396326277, -0.3162353388693409650, -0.4822834645669289433 ) ) ;
#13755=CARTESIAN_POINT ( 'NONE',  ( -1.108923884514435132, -0.3162353388693405765, 0.4822834645669290543 ) ) ;
#13756=CARTESIAN_POINT ( 'NONE',  ( 0.5446194225721792126, -0.05778040916215560624, -0.4822834645669293319 ) ) ;
#13757=CARTESIAN_POINT ( 'NONE',  ( -0.7677165354330699465, -0.5400638737290845981, -0.3530559997133363437 ) ) ;
#13759=CARTESIAN_POINT ( 'NONE',  ( 0.5446194225721792126, -0.05778040916215560624, -0.4822834645669293319 ) ) ;
#13761=CARTESIAN_POINT ( 'NONE',  ( -0.7874015748031489847, -0.1870078740157480601, -0.3641732283464567677 ) ) ;
#13762=ORIENTED_EDGE ( 'NONE', *, *, #20862, .F. ) ;
#13764=VERTEX_POINT ( 'NONE', #7778 ) ;
#13765=CARTESIAN_POINT ( 'NONE',  ( -1.601049868766403650, -0.5023911411419708095, 0.1820866141732285504 ) ) ;
#13766=CARTESIAN_POINT ( 'NONE',  ( -1.141732283464566011, -0.6692913385826771977, 8.415575281601705876E-17 ) ) ;
#13767=CARTESIAN_POINT ( 'NONE',  ( -1.410761154855641575, -0.3162353388693409650, -0.4822834645669289433 ) ) ;
#13769=CARTESIAN_POINT ( 'NONE',  ( -1.049868766404198794, 0.2306618581243847221, -0.2411417322834647770 ) ) ;
#13770=CARTESIAN_POINT ( 'NONE',  ( -1.351706036745406347, 0.05413385826771626580, -0.4176697321401330321 ) ) ;
#13771=CARTESIAN_POINT ( 'NONE',  ( -1.528871391076114250, -0.6692913385826771977, 0.1292274648535927661 ) ) ;
#13772=CARTESIAN_POINT ( 'NONE',  ( 1.586052503253845281, 1.299212598425198095, -0.1653254495020587411 ) ) ;
#13773=CARTESIAN_POINT ( 'NONE',  ( 0.2230971128608932319, -0.3690944881889763329, 0.3153832671262228327 ) ) ;
#13776=CARTESIAN_POINT ( 'NONE',  ( -0.2755905511811018171, 0.1771653543307087630, 0.000000000000000000 ) ) ;
#13777=CARTESIAN_POINT ( 'NONE',  ( -0.9973753280839886548, 0.2306618581243848609, 0.2411417322834645549 ) ) ;
#13778=CARTESIAN_POINT ( 'NONE',  ( 1.003937007874016185, 0.1660481256975883668, -0.3530559997133364547 ) ) ;
#13779=CARTESIAN_POINT ( 'NONE',  ( -0.4593175853018364174, -0.4281496062992127816, -0.4176697321401328100 ) ) ;
#13783=CARTESIAN_POINT ( 'NONE',  ( -0.9645669291338575535, 0.1660481256975883668, -0.3530559997133364547 ) ) ;
#13785=CARTESIAN_POINT ( 'NONE',  ( 1.312335958005249825, 0.2306618581243847221, -0.2411417322834647770 ) ) ;
#13786=CARTESIAN_POINT ( 'NONE',  ( -1.673228346456691717, 0.07958543189024071263, -0.2665933059059888421 ) ) ;
#13791=CARTESIAN_POINT ( 'NONE',  ( -0.3805774278215216522, 0.05413385826771666132, 0.4176697321401328100 ) ) ;
#13792=CARTESIAN_POINT ( 'NONE',  ( -1.640419947506561060, -0.004921259842519576551, 0.3153832671262227771 ) ) ;
#13793=CARTESIAN_POINT ( 'NONE',  ( -0.8333333333333323711, -0.6692913385826773087, -0.1292274648535924053 ) ) ;
#13795=CARTESIAN_POINT ( 'NONE',  ( -1.299212598425196097, -0.6692913385826771977, 8.415575281601705876E-17 ) ) ;
#13797=CARTESIAN_POINT ( 'NONE',  ( -1.003937007874015297, -0.5400638737290845981, -0.3530559997133363437 ) ) ;
#13798=CARTESIAN_POINT ( 'NONE',  ( -0.3083989501312330295, -0.05778040916215522460, 0.4822834645669289988 ) ) ;
#13800=CARTESIAN_POINT ( 'NONE',  ( 0.8398950131233602345, 0.1283753931104746893, -0.1820866141732285504 ) ) ;
#13803=CARTESIAN_POINT ( 'NONE',  ( 0.7480314960629927956, 0.1771653543307087630, 0.000000000000000000 ) ) ;
#13804=CARTESIAN_POINT ( 'NONE',  ( 1.181102362204724976, -0.1870078740157480601, -0.3641732283464567677 ) ) ;
#13805=CARTESIAN_POINT ( 'NONE',  ( 1.463254593175853824, 0.2952755905511810774, -0.1292274648535930714 ) ) ;
#13806=CARTESIAN_POINT ( 'NONE',  ( 0.03937007874015833325, -0.5511811023622047445, 6.969142054262312111E-17 ) ) ;
#13808=CARTESIAN_POINT ( 'NONE',  ( -1.259842519685038686, -0.1870078740157480879, -0.4822834645669291653 ) ) ;
#13809=CARTESIAN_POINT ( 'NONE',  ( 1.056430446194226436, -0.6692913385826773087, -0.1292274648535924053 ) ) ;
#13811=CARTESIAN_POINT ( 'NONE',  ( -0.3937007874015740483, -0.1870078740157479769, 0.3641732283464567677 ) ) ;
#13812=CARTESIAN_POINT ( 'NONE',  ( 0.05249343832021075018, 0.2306618581243847221, -0.2411417322834647770 ) ) ;
#13814=CARTESIAN_POINT ( 'NONE',  ( 0.3149606299212606708, -0.1870078740157480879, -0.4822834645669291653 ) ) ;
#13816=CARTESIAN_POINT ( 'NONE',  ( 1.036745406824147508, -0.3690944881889765550, -0.3153832671262227771 ) ) ;
#13817=CARTESIAN_POINT ( 'NONE',  ( 0.2624671916010504757, -0.5023911411419708095, -0.1820866141732282451 ) ) ;
#13818=CARTESIAN_POINT ( 'NONE',  ( -0.2690288713910754526, -0.6692913385826771977, 0.1292274648535927661 ) ) ;
#13819=CARTESIAN_POINT ( 'NONE',  ( -1.496062992125983815, -0.1870078740157480879, -0.4822834645669291653 ) ) ;
#13820=CARTESIAN_POINT ( 'NONE',  ( -0.8136482939632537770, 0.1283753931104746893, -0.1820866141732285504 ) ) ;
#13822=CARTESIAN_POINT ( 'NONE',  ( 0.6036745406824154392, 0.2306618581243847221, -0.2411417322834647770 ) ) ;
#13823=CARTESIAN_POINT ( 'NONE',  ( -0.8595800524934373854, -0.05778040916215522460, 0.4822834645669289988 ) ) ;
#13826=CARTESIAN_POINT ( 'NONE',  ( 0.2887139107611556010, -0.5023911411419708095, 0.1820866141732285504 ) ) ;
#13827=CARTESIAN_POINT ( 'NONE',  ( -0.9383202099737524282, -0.3162353388693409650, -0.4822834645669289433 ) ) ;
#13828=CARTESIAN_POINT ( 'NONE',  ( -1.135170603674539924, 0.2952755905511810774, -0.1292274648535930714 ) ) ;
#13829=CARTESIAN_POINT ( 'NONE',  ( -1.030183727034119867, -0.2845877964562159024, 0.3641732283464567677 ) ) ;
#13831=CARTESIAN_POINT ( 'NONE',  ( -0.6889763779527552368, 0.07958543189024085140, 0.2665933059059887866 ) ) ;
#13832=CARTESIAN_POINT ( 'NONE',  ( -0.7480314960629914633, 0.2066929133858268208, 0.000000000000000000 ) ) ;
#13833=CARTESIAN_POINT ( 'NONE',  ( 1.437007874015748810, 0.1660481256975885056, 0.3530559997133364547 ) ) ;
#13839=CARTESIAN_POINT ( 'NONE',  ( 1.364829396325459854, -0.5023911411419708095, -0.1820866141732282451 ) ) ;
#13840=CARTESIAN_POINT ( 'NONE',  ( -1.456692913385826182, -0.6692913385826771977, 8.415575281601705876E-17 ) ) ;
#13841=CARTESIAN_POINT ( 'NONE',  ( 1.089238845144357537, -0.4281496062992124485, 0.4176697321401328655 ) ) ;
#13843=CARTESIAN_POINT ( 'NONE',  ( 1.541994750656168645, 0.1771653543307087075, -0.09757992244046823083 ) ) ;
#13844=CARTESIAN_POINT ( 'NONE',  ( 0.3740157480314966754, -0.5400638737290844871, 0.3530559997133364547 ) ) ;
#13845=CARTESIAN_POINT ( 'NONE',  ( 0.09842519685039434474, 0.1660481256975885056, 0.3530559997133364547 ) ) ;
#13848=CARTESIAN_POINT ( 'NONE',  ( 0.8858267716535438430, -0.4536011799217368745, -0.2665933059059886201 ) ) ;
#13853=CARTESIAN_POINT ( 'NONE',  ( 0.03937007874015806264, 0.2952755905511811885, 0.000000000000000000 ) ) ;
#13854=CARTESIAN_POINT ( 'NONE',  ( 1.122047244094488860, 0.1660481256975885056, 0.3530559997133364547 ) ) ;
#13855=CARTESIAN_POINT ( 'NONE',  ( 0.7414698162729663755, 0.2952755905511811885, 0.1292274648535926551 ) ) ;
#13856=CARTESIAN_POINT ( 'NONE',  ( 1.417322834645670104, -0.1870078740157480879, -0.4822834645669291653 ) ) ;
#13857=CARTESIAN_POINT ( 'NONE',  ( -0.4199475065616791736, -0.6046776061558807314, 0.2411417322834647770 ) ) ;
#13858=CARTESIAN_POINT ( 'NONE',  ( 0.01312335958005323398, 0.05413385826771666132, 0.4176697321401328100 ) ) ;
#13859=CARTESIAN_POINT ( 'NONE',  ( 1.430446194225722500, 0.05413385826771666132, 0.4176697321401328100 ) ) ;
#13860=CARTESIAN_POINT ( 'NONE',  ( 1.161417322834646271, 0.1660481256975883668, -0.3530559997133364547 ) ) ;
#13861=CARTESIAN_POINT ( 'NONE',  ( 0.9908136482939640111, -0.6692913385826771977, 0.1292274648535927661 ) ) ;
#13863=CARTESIAN_POINT ( 'NONE',  ( 0.5380577427821529035, -0.3690944881889763329, 0.3153832671262228327 ) ) ;
#13864=ORIENTED_EDGE ( 'NONE', *, *, #9579, .F. ) ;
#13867=CARTESIAN_POINT ( 'NONE',  ( -0.4855643044619415427, -0.3690944881889763329, 0.3153832671262228327 ) ) ;
#13868=CARTESIAN_POINT ( 'NONE',  ( -0.07217847769028787330, -0.05778040916215522460, 0.4822834645669289988 ) ) ;
#13870=CARTESIAN_POINT ( 'NONE',  ( 0.07217847769028949700, -0.05778040916215560624, -0.4822834645669293319 ) ) ;
#13871=CARTESIAN_POINT ( 'NONE',  ( 0.09186351706036799403, -0.4281496062992127816, -0.4176697321401328100 ) ) ;
#13872=CARTESIAN_POINT ( 'NONE',  ( -0.8923884514435688198, -0.6046776061558807314, 0.2411417322834647770 ) ) ;
#13873=CARTESIAN_POINT ( 'NONE',  ( -0.8595800524934373854, -0.3162353388693409650, -0.4822834645669289433 ) ) ;
#13874=CARTESIAN_POINT ( 'NONE',  ( 1.423884514435696413, -0.2845877964562161244, -0.3641732283464567121 ) ) ;
#13877=CARTESIAN_POINT ( 'NONE',  ( 0.7611548556430451917, -0.5023911411419708095, 0.1820866141732285504 ) ) ;
#13879=CARTESIAN_POINT ( 'NONE',  ( 0.3083989501312343062, -0.05778040916215560624, -0.4822834645669293319 ) ) ;
#13880=CARTESIAN_POINT ( 'NONE',  ( 0.8202099737532814183, -0.6692913385826773087, -0.1292274648535924053 ) ) ;
#13885=CARTESIAN_POINT ( 'NONE',  ( -0.6627296587926503335, -0.6692913385826771977, 0.1292274648535927661 ) ) ;
#13888=CARTESIAN_POINT ( 'NONE',  ( -1.240157480314959759, -0.4536011799217368745, -0.2665933059059886201 ) ) ;
#13889=CARTESIAN_POINT ( 'NONE',  ( 1.384514435695538337, -0.6692913385826771977, 0.1292274648535927661 ) ) ;
#13890=CARTESIAN_POINT ( 'NONE',  ( 0.9645669291338591078, -0.5400638737290845981, -0.3530559997133363437 ) ) ;
#13891=CARTESIAN_POINT ( 'NONE',  ( -0.1509186351706028884, -0.2845877964562161244, -0.3641732283464567121 ) ) ;
#13892=CARTESIAN_POINT ( 'NONE',  ( 0.6627296587926515548, 0.2952755905511811885, 0.1292274648535926551 ) ) ;
#13894=CARTESIAN_POINT ( 'NONE',  ( 0.2165354330708668673, -0.4536011799217367080, 0.2665933059059888421 ) ) ;
#13896=CARTESIAN_POINT ( 'NONE',  ( -0.03937007874015669567, -0.6692913385826771977, 8.415575281601705876E-17 ) ) ;
#13899=CARTESIAN_POINT ( 'NONE',  ( -1.292650918635170010, -0.6692913385826771977, 0.1292274648535927661 ) ) ;
#13900=CARTESIAN_POINT ( 'NONE',  ( 0.3412073490813655186, 0.1283753931104748280, 0.1820866141732283561 ) ) ;
#13902=CARTESIAN_POINT ( 'NONE',  ( -0.7414698162729651543, 0.2952755905511810774, -0.1292274648535930714 ) ) ;
#13903=CARTESIAN_POINT ( 'NONE',  ( -0.2296587926509179312, -0.08942795157527998196, 0.3641732283464567121 ) ) ;
#13905=CARTESIAN_POINT ( 'NONE',  ( -0.6430446194225716283, -0.4281496062992124485, 0.4176697321401328655 ) ) ;
#13906=CARTESIAN_POINT ( 'NONE',  ( -0.5774278215223089816, -0.6046776061558807314, 0.2411417322834647770 ) ) ;
#13907=CARTESIAN_POINT ( 'NONE',  ( 0.3740157480314966754, 0.07958543189024071263, -0.2665933059059888421 ) ) ;
#13909=CARTESIAN_POINT ( 'NONE',  ( 0.1115485564304470323, 0.2952755905511811885, 0.1292274648535926551 ) ) ;
#13913=CARTESIAN_POINT ( 'NONE',  ( 0.9514435695538062676, -0.2845877964562161244, -0.3641732283464567121 ) ) ;
#13914=CARTESIAN_POINT ( 'NONE',  ( 1.410761154855643795, -0.3162353388693405765, 0.4822834645669290543 ) ) ;
#13915=CARTESIAN_POINT ( 'NONE',  ( -0.8398950131233589023, -0.5023911411419708095, -0.1820866141732282451 ) ) ;
#13916=CARTESIAN_POINT ( 'NONE',  ( -1.266404199475064773, -0.2845877964562159024, 0.3641732283464567677 ) ) ;
#13917=EDGE_CURVE ( 'NONE', #48718, #35380, #44901, .T. ) ;
#13918=CARTESIAN_POINT ( 'NONE',  ( -0.5314960629921250401, 0.1660481256975885056, 0.3530559997133364547 ) ) ;
#13919=CARTESIAN_POINT ( 'NONE',  ( -0.1246719160104980823, 0.2952755905511811885, 0.1292274648535926551 ) ) ;
#13920=CARTESIAN_POINT ( 'NONE',  ( 0.3543307086614181922, -0.5511811023622047445, 6.969142054262312111E-17 ) ) ;
#13922=CARTESIAN_POINT ( 'NONE',  ( 1.227034120734908917, -0.5511811023622046335, 0.09757992244046803654 ) ) ;
#13923=CARTESIAN_POINT ( 'NONE',  ( 0.5380577427821529035, -0.4281496062992124485, 0.4176697321401328655 ) ) ;
#13925=CARTESIAN_POINT ( 'NONE',  ( -0.7020997375328076329, -0.3162353388693409650, -0.4822834645669289433 ) ) ;
#13927=CARTESIAN_POINT ( 'NONE',  ( 1.594488188976378673, 0.07958543189024085140, 0.2665933059059887866 ) ) ;
#13928=CARTESIAN_POINT ( 'NONE',  ( 0.3805774278215230400, -0.4281496062992124485, 0.4176697321401328655 ) ) ;
#13929=CARTESIAN_POINT ( 'NONE',  ( 0.1902887139107617975, -0.6692913385826773087, -0.1292274648535924053 ) ) ;
#13930=DIRECTION ( 'NONE',  ( 0.000000000000000000, 0.000000000000000000, 1.000000000000000000 ) ) ;
#13931=CARTESIAN_POINT ( 'NONE',  ( 0.06561679790026316017, -0.3690944881889763329, 0.3153832671262228327 ) ) ;
#13932=CARTESIAN_POINT ( 'NONE',  ( 0.9055118110236227702, 0.2952755905511811885, 0.000000000000000000 ) ) ;
#13933=CARTESIAN_POINT ( 'NONE',  ( -0.2755905511811018171, 0.1771653543307087630, 0.000000000000000000 ) ) ;
#13934=CARTESIAN_POINT ( 'NONE',  ( -0.8595800524934373854, -0.05778040916215522460, 0.4822834645669289988 ) ) ;
#13936=CARTESIAN_POINT ( 'NONE',  ( 0.03937007874015806264, 0.2952755905511811885, 0.000000000000000000 ) ) ;
#13937=EDGE_LOOP ( 'NONE', ( #70644, #22928, #59626, #57301 ) ) ;
#13938=CARTESIAN_POINT ( 'NONE',  ( -1.069553805774277722, -0.6692913385826773087, -0.1292274648535924053 ) ) ;
#13939=CIRCLE ( 'NONE', #81117, 3.582677165354331450 ) ;
#13940=CARTESIAN_POINT ( 'NONE',  ( -0.6496062992125976043, -0.4536011799217367080, 0.2665933059059888421 ) ) ;
#13941=CARTESIAN_POINT ( 'NONE',  ( -0.08530183727034056085, -0.05778040916215560624, -0.4822834645669293319 ) ) ;
#13942=CARTESIAN_POINT ( 'NONE',  ( -1.371391076115484831, 0.2952755905511810774, -0.1292274648535930714 ) ) ;
#13943=CARTESIAN_POINT ( 'NONE',  ( -0.5905511811023613777, -0.6692913385826771977, 8.415575281601705876E-17 ) ) ;
#13945=CARTESIAN_POINT ( 'NONE',  ( -0.8858267716535425107, 0.1660481256975883391, -0.3530559997133364547 ) ) ;
#13946=CARTESIAN_POINT ( 'NONE',  ( 0.7480314960629927956, -0.6692913385826771977, 8.415575281601705876E-17 ) ) ;
#13947=CARTESIAN_POINT ( 'NONE',  ( 1.076115485564305141, 0.2306618581243847221, -0.2411417322834647770 ) ) ;
#13949=CARTESIAN_POINT ( 'NONE',  ( 1.476377952755906220, 0.1660481256975883668, -0.3530559997133364547 ) ) ;
#13950=CARTESIAN_POINT ( 'NONE',  ( -1.272965879265091305, -0.4281496062992124485, 0.4176697321401328655 ) ) ;
#13954=CARTESIAN_POINT ( 'NONE',  ( 0.02624671916010564918, -0.5023911411419708095, -0.1820866141732282451 ) ) ;
#13958=CARTESIAN_POINT ( 'NONE',  ( 0.2755905511811031494, -0.6692913385826771977, 8.415575281601705876E-17 ) ) ;
#13959=CARTESIAN_POINT ( 'NONE',  ( -0.1312335958005241554, 0.2306618581243848609, 0.2411417322834645549 ) ) ;
#13960=CARTESIAN_POINT ( 'NONE',  ( -0.7677165354330699465, -0.5400638737290845981, -0.3530559997133363437 ) ) ;
#13962=CARTESIAN_POINT ( 'NONE',  ( -0.9186351706036736120, -0.5023911411419708095, -0.1820866141732282451 ) ) ;
#13963=CARTESIAN_POINT ( 'NONE',  ( 0.3412073490813655186, 0.2306618581243848609, 0.2411417322834645549 ) ) ;
#13964=CARTESIAN_POINT ( 'NONE',  ( 0.6430446194225729606, -0.4281496062992127816, -0.4176697321401328100 ) ) ;
#13965=CARTESIAN_POINT ( 'NONE',  ( 1.108923884514436242, -0.08942795157527998196, 0.3641732283464567121 ) ) ;
#13966=CARTESIAN_POINT ( 'NONE',  ( -0.3674540682414689785, 0.2306618581243848609, 0.2411417322834645549 ) ) ;
#13968=CARTESIAN_POINT ( 'NONE',  ( -0.7217847769028863381, -0.4281496062992124485, 0.4176697321401328655 ) ) ;
#13969=CARTESIAN_POINT ( 'NONE',  ( 1.586052503253845503, 0.7480314960629931287, 0.1653254495020587966 ) ) ;
#13970=CARTESIAN_POINT ( 'NONE',  ( 1.482939632545932307, -0.4281496062992124485, 0.4176697321401328655 ) ) ;
#13971=CARTESIAN_POINT ( 'NONE',  ( 1.496062992125985147, -0.1870078740157479769, 0.3641732283464567677 ) ) ;
#13974=CARTESIAN_POINT ( 'NONE',  ( -0.1312335958005241554, -0.6046776061558809534, -0.2411417322834644161 ) ) ;
#13976=CARTESIAN_POINT ( 'NONE',  ( -0.7611548556430438595, 0.2306618581243848609, 0.2411417322834645549 ) ) ;
#13977=CARTESIAN_POINT ( 'NONE',  ( 1.561679790026247350, -0.4281496062992124485, 0.4176697321401328655 ) ) ;
#13978=CARTESIAN_POINT ( 'NONE',  ( 1.404199475065617264, -0.4281496062992124485, 0.4176697321401328655 ) ) ;
#13979=CARTESIAN_POINT ( 'NONE',  ( 0.2165354330708668673, 0.1660481256975883668, -0.3530559997133364547 ) ) ;
#13981=CARTESIAN_POINT ( 'NONE',  ( -0.4986876640419939388, 0.2306618581243847221, -0.2411417322834647770 ) ) ;
#13983=CARTESIAN_POINT ( 'NONE',  ( -1.181102362204723644, -0.1870078740157480879, -0.4822834645669291653 ) ) ;
#13984=CARTESIAN_POINT ( 'NONE',  ( -0.1771653543307080136, 0.1660481256975883668, -0.3530559997133364547 ) ) ;
#13985=CARTESIAN_POINT ( 'NONE',  ( -0.1640419947506553400, -0.08942795157528024563, -0.3641732283464568787 ) ) ;
#13986=CARTESIAN_POINT ( 'NONE',  ( 1.555118110236221041, 0.1660481256975883668, -0.3530559997133364547 ) ) ;
#13987=CARTESIAN_POINT ( 'NONE',  ( 1.397637795275591177, 0.1660481256975883668, -0.3530559997133364547 ) ) ;
#13988=CARTESIAN_POINT ( 'NONE',  ( -0.4330708661417315697, 0.2952755905511811885, 0.000000000000000000 ) ) ;
#13990=CARTESIAN_POINT ( 'NONE',  ( 0.9776902887139113929, 0.2952755905511811885, 0.1292274648535926551 ) ) ;
#13993=CARTESIAN_POINT ( 'NONE',  ( 0.3346456692913393205, -0.5400638737290845981, -0.3530559997133363437 ) ) ;
#13994=CARTESIAN_POINT ( 'NONE',  ( -0.1377952755905504645, 0.07958543189024085140, 0.2665933059059887866 ) ) ;
#13995=CARTESIAN_POINT ( 'NONE',  ( 0.8989501312335964611, 0.1771653543307087630, 0.09757992244046791164 ) ) ;
#13998=CARTESIAN_POINT ( 'NONE',  ( 1.574803149606299746, -0.1870078740157480601, -0.3641732283464567677 ) ) ;
#13999=CARTESIAN_POINT ( 'NONE',  ( 1.049868766404200127, -0.6046776061558809534, -0.2411417322834644161 ) ) ;
#14001=CARTESIAN_POINT ( 'NONE',  ( -0.05249343832020938322, -0.6046776061558809534, -0.2411417322834644161 ) ) ;
#14002=CARTESIAN_POINT ( 'NONE',  ( -1.482939632545930975, 0.05413385826771666132, 0.4176697321401328100 ) ) ;
#14004=CARTESIAN_POINT ( 'NONE',  ( -1.384514435695537005, 0.2952755905511811885, 0.1292274648535926551 ) ) ;
#14005=CARTESIAN_POINT ( 'NONE',  ( -0.2755905511811018171, 0.2952755905511811885, 0.000000000000000000 ) ) ;
#14007=CARTESIAN_POINT ( 'NONE',  ( 1.601049868766404982, -0.6046776061558809534, -0.2411417322834644161 ) ) ;
#14008=CARTESIAN_POINT ( 'NONE',  ( 0.7349081364829402885, -0.6046776061558809534, -0.2411417322834644161 ) ) ;
#14009=CARTESIAN_POINT ( 'NONE',  ( 0.9317585301837276734, -0.004921259842519870586, -0.3153832671262229437 ) ) ;
#14010=CARTESIAN_POINT ( 'NONE',  ( -0.04593175853018303251, 0.2952755905511811885, 0.1292274648535926551 ) ) ;
#14011=CARTESIAN_POINT ( 'NONE',  ( 0.2362204724409456558, -0.1870078740157479769, 0.3641732283464567677 ) ) ;
#14012=CARTESIAN_POINT ( 'NONE',  ( -1.095800524934382292, -0.3162353388693409650, -0.4822834645669289433 ) ) ;
#14014=CARTESIAN_POINT ( 'NONE',  ( 1.069553805774278832, 0.2952755905511810774, -0.1292274648535930714 ) ) ;
#14016=CARTESIAN_POINT ( 'NONE',  ( 0.8333333333333340365, -0.6692913385826771977, 0.1292274648535927661 ) ) ;
#14019=CARTESIAN_POINT ( 'NONE',  ( 0.3805774278215230400, -0.004921259842519870586, -0.3153832671262229437 ) ) ;
#14021=CARTESIAN_POINT ( 'NONE',  ( 0.5971128608923891301, 0.2952755905511810774, -0.1292274648535930714 ) ) ;
#14022=CARTESIAN_POINT ( 'NONE',  ( 0.7414698162729664865, 0.2066929133858267931, 0.1054918080437490802 ) ) ;
#14023=CARTESIAN_POINT ( 'NONE',  ( -1.049868766404198794, 0.1283753931104746893, -0.1820866141732285504 ) ) ;
#14024=CARTESIAN_POINT ( 'NONE',  ( -0.8923884514435688198, 0.2306618581243847221, -0.2411417322834647770 ) ) ;
#14025=CARTESIAN_POINT ( 'NONE',  ( -1.568241469816272105, -0.05778040916215522460, 0.4822834645669289988 ) ) ;
#14026=CARTESIAN_POINT ( 'NONE',  ( 0.8005249343832028242, -0.4281496062992127816, -0.4176697321401328100 ) ) ;
#14027=CARTESIAN_POINT ( 'NONE',  ( -1.601049868766403650, 0.1283753931104746893, -0.1820866141732285504 ) ) ;
#14028=( BOUNDED_CURVE ( )  B_SPLINE_CURVE ( 2, ( #20660, #73255, #58953, #27376, #78750, #46733, #72425, #14775, #10111, #75319, #62682, #36584, #74086 ),
 .UNSPECIFIED., .F., .F. ) 
 B_SPLINE_CURVE_WITH_KNOTS ( ( 3, 2, 2, 2, 2, 2, 3 ),
 ( 0.5490332660251417973, 0.5492424242424243097, 0.5530303030303029832, 0.5568181818181818787, 0.5606060606060606633, 0.5643939393939394478, 0.5646030976112219602 ),
 .UNSPECIFIED. ) 
 CURVE ( )  GEOMETRIC_REPRESENTATION_ITEM ( )  RATIONAL_B_SPLINE_CURVE ( ( 0.9964447847208420805, 0.9981185001348091834, 1.000000000000000000, 0.9659258262890683122, 1.000000000000000000, 0.9659258262890683122, 1.000000000000000000, 0.9659258262890683122, 1.000000000000000000, 0.9659258262890683122, 1.000000000000000000, 0.9981185001348091834, 0.9964447847208420805 ) ) 
 REPRESENTATION_ITEM ( '' )  );
#14030=CARTESIAN_POINT ( 'NONE',  ( 0.5446194225721792126, -0.05778040916215560624, -0.4822834645669293319 ) ) ;
#14032=CARTESIAN_POINT ( 'NONE',  ( 1.666666666666667185, 0.05413385826771666132, 0.4176697321401328100 ) ) ;
#14033=CARTESIAN_POINT ( 'NONE',  ( 1.404199475065617708, 0.05413385826771626580, -0.4176697321401330321 ) ) ;
#14034=CARTESIAN_POINT ( 'NONE',  ( -1.502624671916009680, -0.08942795157528024563, -0.3641732283464568787 ) ) ;
#14035=CARTESIAN_POINT ( 'NONE',  ( 1.023622047244095334, -0.1870078740157479769, 0.3641732283464567677 ) ) ;
#14036=CARTESIAN_POINT ( 'NONE',  ( -1.391076115485563314, -0.5023911411419708095, -0.1820866141732282451 ) ) ;
#14037=CARTESIAN_POINT ( 'NONE',  ( -0.3149606299212590610, -0.1870078740157480601, -0.3641732283464567677 ) ) ;
#14039=CARTESIAN_POINT ( 'NONE',  ( 0.7283464566929140904, -0.4536011799217368745, -0.2665933059059886201 ) ) ;
#14040=CARTESIAN_POINT ( 'NONE',  ( 0.6496062992125991586, -0.5400638737290845981, -0.3530559997133363437 ) ) ;
#14041=CARTESIAN_POINT ( 'NONE',  ( 0.9448818897637802916, -0.1870078740157479769, 0.4822834645669291653 ) ) ;
#14042=CARTESIAN_POINT ( 'NONE',  ( 0.1968503937007881344, -0.6692913385826771977, 8.415575281601705876E-17 ) ) ;
#14044=CARTESIAN_POINT ( 'NONE',  ( 0.7152230971128614723, -0.2845877964562161244, -0.3641732283464567121 ) ) ;
#14045=CARTESIAN_POINT ( 'NONE',  ( 1.187664041994751285, -0.3162353388693409650, -0.4822834645669289433 ) ) ;
#14048=CARTESIAN_POINT ( 'NONE',  ( -1.594488188976377119, 0.1660481256975883668, -0.3530559997133364547 ) ) ;
#14049=CARTESIAN_POINT ( 'NONE',  ( -0.5577427821522301654, -0.05778040916215560624, -0.4822834645669293319 ) ) ;
#14052=CARTESIAN_POINT ( 'NONE',  ( 0.2165354330708668673, 0.1660481256975883668, -0.3530559997133364547 ) ) ;
#14053=CARTESIAN_POINT ( 'NONE',  ( -0.2887139107611542133, -0.6046776061558809534, -0.2411417322834644161 ) ) ;
#14054=CARTESIAN_POINT ( 'NONE',  ( -0.2230971128608915943, -0.4281496062992127816, -0.4176697321401328100 ) ) ;
#14060=CARTESIAN_POINT ( 'NONE',  ( -0.8858267716535425107, 0.07958543189024071263, -0.2665933059059888421 ) ) ;
#14062=CARTESIAN_POINT ( 'NONE',  ( -1.364829396325458521, 0.2306618581243847221, -0.2411417322834647770 ) ) ;
#14064=CARTESIAN_POINT ( 'NONE',  ( 0.4068241469816281097, 0.05413385826771666132, 0.4176697321401328100 ) ) ;
#14065=CARTESIAN_POINT ( 'NONE',  ( -0.3543307086614165824, -0.5511811023622047445, 6.969142054262312111E-17 ) ) ;
#14066=EDGE_CURVE ( 'NONE', #43230, #24616, #3649, .T. ) ;
#14067=CARTESIAN_POINT ( 'NONE',  ( 1.082677165354331228, -0.5400638737290844871, 0.3530559997133364547 ) ) ;
#14068=CARTESIAN_POINT ( 'NONE',  ( 0.1902887139107617975, 0.2952755905511811885, 0.1292274648535926551 ) ) ;
#14072=CARTESIAN_POINT ( 'NONE',  ( 1.128608923884515169, -0.6046776061558809534, -0.2411417322834644161 ) ) ;
#14073=CARTESIAN_POINT ( 'NONE',  ( 0.6233595800524939223, -0.3162353388693405765, 0.4822834645669290543 ) ) ;
#14074=CARTESIAN_POINT ( 'NONE',  ( 0.1706036745406830368, 0.05413385826771666132, 0.4176697321401328100 ) ) ;
#14075=VECTOR ( 'NONE', #67520, 39.37007874015748854 ) ;
#14076=CARTESIAN_POINT ( 'NONE',  ( -1.601049868766403650, 0.2306618581243847221, -0.2411417322834647770 ) ) ;
#14077=CARTESIAN_POINT ( 'NONE',  ( 1.076115485564305141, 0.2306618581243847221, -0.2411417322834647770 ) ) ;
#14079=CARTESIAN_POINT ( 'NONE',  ( -0.1246719160104980823, 0.2952755905511811885, 0.1292274648535926551 ) ) ;
#14080=CARTESIAN_POINT ( 'NONE',  ( 1.023622047244095334, -0.1870078740157479769, 0.4822834645669291653 ) ) ;
#14081=CARTESIAN_POINT ( 'NONE',  ( 0.3346456692913393205, -0.5400638737290845981, -0.3530559997133363437 ) ) ;
#14082=CARTESIAN_POINT ( 'NONE',  ( 1.259842519685040019, -0.1870078740157480601, -0.3641732283464567677 ) ) ;
#14083=CARTESIAN_POINT ( 'NONE',  ( -0.9514435695538050464, -0.3162353388693405765, 0.4822834645669290543 ) ) ;
#14084=CARTESIAN_POINT ( 'NONE',  ( -1.292650918635170010, -0.6692913385826771977, 0.1292274648535927661 ) ) ;
#14085=CARTESIAN_POINT ( 'NONE',  ( 0.7480314960629927956, -0.6692913385826771977, 8.415575281601705876E-17 ) ) ;
#14088=ORIENTED_EDGE ( 'NONE', *, *, #80532, .F. ) ;
#14091=CARTESIAN_POINT ( 'NONE',  ( 1.450131233595801428, -0.6692913385826773087, -0.1292274648535924053 ) ) ;
#14092=CARTESIAN_POINT ( 'NONE',  ( 1.167979002624672580, -0.004921259842519870586, -0.3153832671262229437 ) ) ;
#14093=CARTESIAN_POINT ( 'NONE',  ( -0.7773926554473638006, -2.191421614605370878E-15, 0.4445507791589071167 ) ) ;
#14097=CARTESIAN_POINT ( 'NONE',  ( 1.555118110236221041, -0.5400638737290844871, 0.3530559997133364547 ) ) ;
#14098=CARTESIAN_POINT ( 'NONE',  ( -1.633858267716534529, 0.1660481256975885056, 0.3530559997133364547 ) ) ;
#14099=CARTESIAN_POINT ( 'NONE',  ( -0.3871391076115479057, -0.3162353388693409650, -0.4822834645669289433 ) ) ;
#14100=CARTESIAN_POINT ( 'NONE',  ( 1.003937007874016185, 0.1660481256975883668, -0.3530559997133364547 ) ) ;
#14102=CARTESIAN_POINT ( 'NONE',  ( -1.646981627296586703, -0.3162353388693409650, -0.4822834645669289433 ) ) ;
#14107=CARTESIAN_POINT ( 'NONE',  ( -0.9317585301837263412, -0.3690944881889765550, -0.3153832671262227771 ) ) ;
#14108=CARTESIAN_POINT ( 'NONE',  ( 0.9321091654255241332, 0.004960608223779158429, -0.3437734562760187962 ) ) ;
#14109=CARTESIAN_POINT ( 'NONE',  ( 0.6036745406824154392, 0.2306618581243847221, -0.2411417322834647770 ) ) ;
#14110=EDGE_LOOP ( 'NONE', ( #25948, #34968, #42110, #36183, #36919 ) ) ;
#14112=CARTESIAN_POINT ( 'NONE',  ( -0.4133858267716528090, 0.1012011053420775880, -0.2882089793578257453 ) ) ;
#14113=CARTESIAN_POINT ( 'NONE',  ( 0.6758530183727039509, -0.6692913385826771977, 0.1292274648535927661 ) ) ;
#14114=CARTESIAN_POINT ( 'NONE',  ( -1.469816272965878357, -0.6046776061558809534, -0.2411417322834644161 ) ) ;
#14116=CARTESIAN_POINT ( 'NONE',  ( -0.6824146981627291497, -0.5023911411419708095, -0.1820866141732282451 ) ) ;
#14117=CARTESIAN_POINT ( 'NONE',  ( -1.496062992125983815, -0.1870078740157479769, 0.3641732283464567677 ) ) ;
#14118=CARTESIAN_POINT ( 'NONE',  ( -1.646051170424378096, 0.000000000000000000, 0.3464511005275205946 ) ) ;
#14119=( GEOMETRIC_REPRESENTATION_CONTEXT ( 3 ) GLOBAL_UNCERTAINTY_ASSIGNED_CONTEXT ( ( #73958 ) ) GLOBAL_UNIT_ASSIGNED_CONTEXT ( ( #215, #25038, #6522 ) ) REPRESENTATION_CONTEXT ( 'NONE', 'WORKASPACE' ) );
#14120=CARTESIAN_POINT ( 'NONE',  ( 0.4658792650918640033, -0.3162353388693405765, 0.4822834645669290543 ) ) ;
#14121=CARTESIAN_POINT ( 'NONE',  ( -0.8398950131233585692, 0.1283753931104748280, 0.1820866141732283561 ) ) ;
#14122=CARTESIAN_POINT ( 'NONE',  ( 0.01312335958005323398, -0.004921259842519576551, 0.3153832671262227771 ) ) ;
#14123=CARTESIAN_POINT ( 'NONE',  ( -0.3608923884514428360, -0.6692913385826773087, -0.1292274648535924053 ) ) ;
#14124=CARTESIAN_POINT ( 'NONE',  ( -1.286089238845143479, 0.1283753931104746893, -0.1820866141732285504 ) ) ;
#14126=CARTESIAN_POINT ( 'NONE',  ( 0.6430446194225728496, 0.05413385826771666132, 0.4176697321401328100 ) ) ;
#14127=ADVANCED_FACE ( 'NONE', ( #9961 ), #23406, .F. ) ;
#14128=CARTESIAN_POINT ( 'NONE',  ( -1.312335958005248715, 0.2306618581243848609, 0.2411417322834645549 ) ) ;
#14130=CARTESIAN_POINT ( 'NONE',  ( -0.7086614173228339419, -0.1870078740157480879, -0.4822834645669291653 ) ) ;
#14131=CARTESIAN_POINT ( 'NONE',  ( -0.01312335958005186876, -0.3690944881889763329, 0.3153832671262228327 ) ) ;
#14132=CARTESIAN_POINT ( 'NONE',  ( -1.299212598425196097, 0.2952755905511811885, 0.000000000000000000 ) ) ;
#14133=CARTESIAN_POINT ( 'NONE',  ( 1.036745406824147731, -0.004921259842519576551, 0.3153832671262227771 ) ) ;
#14135=CARTESIAN_POINT ( 'NONE',  ( -0.3805774278215216522, -0.3690944881889765550, -0.3153832671262227771 ) ) ;
#14136=CARTESIAN_POINT ( 'NONE',  ( -1.122047244094487306, -0.5400638737290844871, 0.3530559997133364547 ) ) ;
#14137=CARTESIAN_POINT ( 'NONE',  ( -1.154855643044618851, -0.6046776061558809534, -0.2411417322834644161 ) ) ;
#14138=CARTESIAN_POINT ( 'NONE',  ( -1.627296587926508442, 0.2306618581243848609, 0.2411417322834645549 ) ) ;
#14139=CARTESIAN_POINT ( 'NONE',  ( 1.089238845144357759, 0.009842519685039147898, -0.3409548833797004797 ) ) ;
#14140=CARTESIAN_POINT ( 'NONE',  ( 1.115485564304462551, -0.3690944881889765550, -0.3153832671262227771 ) ) ;
#14141=CARTESIAN_POINT ( 'NONE',  ( 0.2230971128608932319, -0.4281496062992124485, 0.4176697321401328655 ) ) ;
#14142=CARTESIAN_POINT ( 'NONE',  ( -1.555118110236219930, -0.5400638737290845981, -0.3530559997133363437 ) ) ;
#14143=CARTESIAN_POINT ( 'NONE',  ( -1.345144356955379816, -0.05778040916215560624, -0.4822834645669293319 ) ) ;
#14146=CARTESIAN_POINT ( 'NONE',  ( -1.089238845144356427, -0.3690944881889765550, -0.3153832671262227771 ) ) ;
#14147=CARTESIAN_POINT ( 'NONE',  ( 0.7808398950131240079, -0.3162353388693405765, 0.4822834645669290543 ) ) ;
#14148=CARTESIAN_POINT ( 'NONE',  ( -1.246719160104986512, -0.004921259842519576551, 0.3153832671262227771 ) ) ;
#14150=CARTESIAN_POINT ( 'NONE',  ( -1.561679790026246017, 0.05413385826771666132, 0.4176697321401328100 ) ) ;
#14151=CARTESIAN_POINT ( 'NONE',  ( 1.023622047244095334, -0.1870078740157479769, 0.4822834645669291653 ) ) ;
#14152=CARTESIAN_POINT ( 'NONE',  ( 0.5249343832021005074, -0.6046776061558807314, 0.2411417322834647770 ) ) ;
#14153=CARTESIAN_POINT ( 'NONE',  ( 1.095800524934383846, -0.3162353388693405765, 0.4822834645669290543 ) ) ;
#14154=CARTESIAN_POINT ( 'NONE',  ( -1.364829396325458521, 0.1283753931104746893, -0.1820866141732285504 ) ) ;
#14159=CARTESIAN_POINT ( 'NONE',  ( 0.5708661417322842269, 0.07958543189024085140, 0.2665933059059887866 ) ) ;
#14160=CARTESIAN_POINT ( 'NONE',  ( 0.3215223097112867578, -0.08942795157527998196, 0.3641732283464567121 ) ) ;
#14161=CARTESIAN_POINT ( 'NONE',  ( 0.1574803149606306130, -0.1870078740157479769, 0.4822834645669291653 ) ) ;
#14162=CARTESIAN_POINT ( 'NONE',  ( 1.430446194225722500, 0.05413385826771666132, 0.4176697321401328100 ) ) ;
#14164=CARTESIAN_POINT ( 'NONE',  ( 0.5380577427821529035, -0.3690944881889763329, 0.3153832671262228327 ) ) ;
#14165=CARTESIAN_POINT ( 'NONE',  ( -0.5314960629921250401, 0.1660481256975885056, 0.3530559997133364547 ) ) ;
#14166=CARTESIAN_POINT ( 'NONE',  ( -1.548556430446193399, -0.6046776061558809534, -0.2411417322834644161 ) ) ;
#14167=CARTESIAN_POINT ( 'NONE',  ( 0.8923884514435703741, 0.2306618581243848609, 0.2411417322834645549 ) ) ;
#14169=CARTESIAN_POINT ( 'NONE',  ( 1.220472440944882386, 0.2952755905511811885, 0.000000000000000000 ) ) ;
#14171=VERTEX_POINT ( 'NONE', #4466 ) ;
#14172=CARTESIAN_POINT ( 'NONE',  ( -1.115485564304461219, -0.4281496062992124485, 0.4176697321401328655 ) ) ;
#14173=CARTESIAN_POINT ( 'NONE',  ( -0.6430446194225712953, -0.004921259842519870586, -0.3153832671262229437 ) ) ;
#14174=CARTESIAN_POINT ( 'NONE',  ( -1.246719160104985846, -0.4281496062992127816, -0.4176697321401328100 ) ) ;
#14177=CARTESIAN_POINT ( 'NONE',  ( -1.535433070866141225, -0.5511811023622047445, 6.969142054262312111E-17 ) ) ;
#14178=CARTESIAN_POINT ( 'NONE',  ( -1.089238845144356427, 0.05413385826771666132, 0.4176697321401328100 ) ) ;
#14179=CARTESIAN_POINT ( 'NONE',  ( 0.1509186351706042484, -0.3162353388693405765, 0.4822834645669290543 ) ) ;
#14180=CARTESIAN_POINT ( 'NONE',  ( -1.286089238845143479, 0.2306618581243847221, -0.2411417322834647770 ) ) ;
#14182=CARTESIAN_POINT ( 'NONE',  ( 0.5905511811023629321, -0.6692913385826771977, 8.415575281601705876E-17 ) ) ;
#14184=CARTESIAN_POINT ( 'NONE',  ( -0.7677165354330699465, -0.4536011799217368745, -0.2665933059059886201 ) ) ;
#14185=ORIENTED_EDGE ( 'NONE', *, *, #3063, .T. ) ;
#14188=CARTESIAN_POINT ( 'NONE',  ( -0.6410189441372351471, -3.721645946415733147E-15, -0.3954974714151476278 ) ) ;
#14190=CARTESIAN_POINT ( 'NONE',  ( -1.115485564304461219, -0.4281496062992124485, 0.4176697321401328655 ) ) ;
#14191=CARTESIAN_POINT ( 'NONE',  ( -1.482939632545930975, 0.05413385826771666132, 0.4176697321401328100 ) ) ;
#14193=CARTESIAN_POINT ( 'NONE',  ( -1.679790026246718693, 0.2306618581243847221, -0.2411417322834647770 ) ) ;
#14194=CARTESIAN_POINT ( 'NONE',  ( -1.364829396325458521, 0.2306618581243847221, -0.2411417322834647770 ) ) ;
#14195=CARTESIAN_POINT ( 'NONE',  ( -1.548556430446193399, -0.6046776061558809534, -0.2411417322834644161 ) ) ;
#14196=ADVANCED_FACE ( 'NONE', ( #42756 ), #74773, .F. ) ;
#14198=CARTESIAN_POINT ( 'NONE',  ( -0.01312335958005186876, -0.004921259842519870586, -0.3153832671262229437 ) ) ;
#14201=CARTESIAN_POINT ( 'NONE',  ( -0.1902887139107604098, -0.5511811023622046335, 0.09757992244046803654 ) ) ;
#14202=CARTESIAN_POINT ( 'NONE',  ( -0.8005249343832011588, 0.05413385826771626580, -0.4176697321401330321 ) ) ;
#14204=CARTESIAN_POINT ( 'NONE',  ( 0.9580052493438326877, 0.05413385826771666132, 0.4176697321401328100 ) ) ;
#14205=CARTESIAN_POINT ( 'NONE',  ( -1.089238845144356427, -0.4281496062992127816, -0.4176697321401328100 ) ) ;
#14208=CARTESIAN_POINT ( 'NONE',  ( -1.036745406824146176, -0.4281496062992124485, 0.4176697321401328655 ) ) ;
#14209=CARTESIAN_POINT ( 'NONE',  ( 0.8792650918635177559, -0.4281496062992127816, -0.4176697321401328100 ) ) ;
#14210=CARTESIAN_POINT ( 'NONE',  ( -1.509186351706035767, -0.004921259842519870586, -0.3153832671262229437 ) ) ;
#14215=CARTESIAN_POINT ( 'NONE',  ( -0.2099737532808391705, 0.2306618581243848609, 0.2411417322834645549 ) ) ;
#14216=CARTESIAN_POINT ( 'NONE',  ( 1.666666666666667185, 0.05413385826771666132, 0.4176697321401328100 ) ) ;
#14217=CARTESIAN_POINT ( 'NONE',  ( -0.9055118110236215490, 0.2952755905511811885, 0.000000000000000000 ) ) ;
#14219=CARTESIAN_POINT ( 'NONE',  ( -1.410761154855642463, -0.05778040916215522460, 0.4822834645669289988 ) ) ;
#14221=CARTESIAN_POINT ( 'NONE',  ( -1.089238845144356427, 0.05413385826771666132, 0.4176697321401328100 ) ) ;
#14222=CARTESIAN_POINT ( 'NONE',  ( -0.3937007874015740483, -0.1870078740157480879, -0.4822834645669291653 ) ) ;
#14224=CARTESIAN_POINT ( 'NONE',  ( 0.5905511811023629321, -0.5511811023622047445, 6.969142054262312111E-17 ) ) ;
#14225=CYLINDRICAL_SURFACE ( 'NONE', #12888, 2.362204724409449064 ) ;
#14226=CARTESIAN_POINT ( 'NONE',  ( 0.3871391076115493490, -0.2845877964562159024, 0.3641732283464567677 ) ) ;
#14227=CARTESIAN_POINT ( 'NONE',  ( 1.233595800524935227, -0.5023911411419708095, 0.1820866141732285504 ) ) ;
#14228=CARTESIAN_POINT ( 'NONE',  ( 1.338582677165355062, -0.1870078740157480879, -0.4822834645669291653 ) ) ;
#14229=CARTESIAN_POINT ( 'NONE',  ( 0.2034120734908144990, -0.5511811023622046335, 0.09757992244046803654 ) ) ;
#14231=CARTESIAN_POINT ( 'NONE',  ( -1.450131233595799651, 0.2952755905511810774, -0.1292274648535930714 ) ) ;
#14232=CARTESIAN_POINT ( 'NONE',  ( -0.1377952755905504645, 0.07958543189024085140, 0.2665933059059887866 ) ) ;
#14233=EDGE_CURVE ( 'NONE', #199, #57945, #17558, .T. ) ;
#14235=CARTESIAN_POINT ( 'NONE',  ( -0.4527559055118102749, -0.4536011799217368745, -0.2665933059059886201 ) ) ;
#14236=CARTESIAN_POINT ( 'NONE',  ( 0.05905511811023682334, 0.1660481256975883391, -0.3530559997133364547 ) ) ;
#14237=CARTESIAN_POINT ( 'NONE',  ( 0.4986876640419954376, -0.6046776061558809534, -0.2411417322834644161 ) ) ;
#14239=EDGE_CURVE ( 'NONE', #69836, #13510, #51018, .T. ) ;
#14240=CARTESIAN_POINT ( 'NONE',  ( 0.8792650918635177559, -0.3690944881889765550, -0.3153832671262227771 ) ) ;
#14241=CARTESIAN_POINT ( 'NONE',  ( 0.1902887139107617975, 0.1771653543307087630, 0.09757992244046791164 ) ) ;
#14242=CARTESIAN_POINT ( 'NONE',  ( -0.1771653543307080136, 0.1660481256975883668, -0.3530559997133364547 ) ) ;
#14244=CARTESIAN_POINT ( 'NONE',  ( -0.5380577427821514602, -0.004921259842519576551, 0.3153832671262227771 ) ) ;
#14246=CARTESIAN_POINT ( 'NONE',  ( 0.3740157480314966754, -0.5400638737290844871, 0.3530559997133364547 ) ) ;
#14247=CARTESIAN_POINT ( 'NONE',  ( -0.8005249343832011588, 0.05413385826771626580, -0.4176697321401330321 ) ) ;
#14250=CARTESIAN_POINT ( 'NONE',  ( 0.1640419947506569498, -0.08942795157527998196, 0.3641732283464567121 ) ) ;
#14251=CARTESIAN_POINT ( 'NONE',  ( -0.9448818897637790704, -0.1870078740157480879, -0.4822834645669291653 ) ) ;
#14253=CARTESIAN_POINT ( 'NONE',  ( -1.115485564304461219, 0.05413385826771626580, -0.4176697321401330321 ) ) ;
#14254=CARTESIAN_POINT ( 'NONE',  ( -1.227034120734907141, -0.5511811023622048555, -0.09757992244046775898 ) ) ;
#14255=CARTESIAN_POINT ( 'NONE',  ( 1.614173228346457378, 0.5038684218300978346, -0.1372047244094476148 ) ) ;
#14256=CARTESIAN_POINT ( 'NONE',  ( -0.6955380577427815458, -0.004921259842519576551, 0.3153832671262227771 ) ) ;
#14257=CARTESIAN_POINT ( 'NONE',  ( 2.795275590551181466, 0.7480314960629931287, -2.695814348275282069E-16 ) ) ;
#14258=CARTESIAN_POINT ( 'NONE',  ( 1.017060367454068581, -0.05778040916215560624, -0.4822834645669293319 ) ) ;
#14263=CARTESIAN_POINT ( 'NONE',  ( 1.522309711286089939, -0.5023911411419708095, -0.1820866141732282451 ) ) ;
#14264=CARTESIAN_POINT ( 'NONE',  ( -1.259842519685038686, -0.1870078740157479769, 0.4822834645669291653 ) ) ;
#14265=CARTESIAN_POINT ( 'NONE',  ( 1.049868766404200127, -0.6046776061558809534, -0.2411417322834644161 ) ) ;
#14267=DIRECTION ( 'NONE',  ( 0.7071067811865495711, -0.000000000000000000, -0.7071067811865454633 ) ) ;
#14268=CARTESIAN_POINT ( 'NONE',  ( 0.7349081364829403995, 0.2306618581243848609, 0.2411417322834645549 ) ) ;
#14269=CARTESIAN_POINT ( 'NONE',  ( -0.5314960629921250401, 0.1660481256975885056, 0.3530559997133364547 ) ) ;
#14272=CARTESIAN_POINT ( 'NONE',  ( 0.6824146981627303710, 0.1283753931104746893, -0.1820866141732285504 ) ) ;
#14274=EDGE_LOOP ( 'NONE', ( #68479, #34347, #75062, #12005 ) ) ;
#14277=CARTESIAN_POINT ( 'NONE',  ( -0.02624671916010428221, -0.6046776061558807314, 0.2411417322834647770 ) ) ;
#14278=CARTESIAN_POINT ( 'NONE',  ( 1.338582677165355062, -0.1870078740157480879, -0.4822834645669291653 ) ) ;
#14279=CARTESIAN_POINT ( 'NONE',  ( 0.2755905511811031494, 0.2952755905511811885, 0.000000000000000000 ) ) ;
#14280=CARTESIAN_POINT ( 'NONE',  ( 1.148293963254593875, -0.6692913385826771977, 0.1292274648535927661 ) ) ;
#14281=CARTESIAN_POINT ( 'NONE',  ( -0.6955380577427815458, 0.05413385826771666132, 0.4176697321401328100 ) ) ;
#14282=CARTESIAN_POINT ( 'NONE',  ( 0.09186351706036799403, -0.4281496062992127816, -0.4176697321401328100 ) ) ;
#14283=CARTESIAN_POINT ( 'NONE',  ( 1.463254593175853824, 0.2952755905511810774, -0.1292274648535930714 ) ) ;
#14284=CARTESIAN_POINT ( 'NONE',  ( 1.181102362204724976, -0.1870078740157480879, -0.4822834645669291653 ) ) ;
#14285=CARTESIAN_POINT ( 'NONE',  ( 0.9711286089238851948, -0.6046776061558809534, -0.2411417322834644161 ) ) ;
#14287=CARTESIAN_POINT ( 'NONE',  ( 0.5314960629921267055, -0.4536011799217367080, 0.2665933059059888421 ) ) ;
#14292=CARTESIAN_POINT ( 'NONE',  ( -0.5183727034120726440, -0.5511811023622048555, -0.09757992244046775898 ) ) ;
#14295=CARTESIAN_POINT ( 'NONE',  ( -0.2099737532808391705, 0.2306618581243848609, 0.2411417322834645549 ) ) ;
#14297=CARTESIAN_POINT ( 'NONE',  ( -0.4855643044619415427, -0.4281496062992124485, 0.4176697321401328655 ) ) ;
#14298=CARTESIAN_POINT ( 'NONE',  ( 5.463695987328526437E-16, -0.1870078740157479769, 0.4822834645669291653 ) ) ;
#14299=CARTESIAN_POINT ( 'NONE',  ( -0.7414698162729651543, -0.6692913385826771977, 0.1292274648535927661 ) ) ;
#14301=CARTESIAN_POINT ( 'NONE',  ( -1.102362204724408601, -0.1870078740157479769, 0.4822834645669291653 ) ) ;
#14302=CARTESIAN_POINT ( 'NONE',  ( 1.259842519685040019, -0.1870078740157480601, -0.3641732283464567677 ) ) ;
#14305=CARTESIAN_POINT ( 'NONE',  ( 1.036745406824147508, -0.3690944881889765550, -0.3153832671262227771 ) ) ;
#14306=CARTESIAN_POINT ( 'NONE',  ( 0.5314960629921267055, -0.5400638737290844871, 0.3530559997133364547 ) ) ;
#14307=CARTESIAN_POINT ( 'NONE',  ( 0.6102362204724416372, 0.1660481256975883668, -0.3530559997133364547 ) ) ;
#14309=CARTESIAN_POINT ( 'NONE',  ( -1.732283464566928277, -0.1870078740157479769, 0.4822834645669291653 ) ) ;
#14312=CARTESIAN_POINT ( 'NONE',  ( -0.4921259842519677963, -0.5400638737290844871, 0.3530559997133364547 ) ) ;
#14316=CARTESIAN_POINT ( 'NONE',  ( -1.148293963254592542, 0.1771653543307087630, 0.09757992244046791164 ) ) ;
#14317=CARTESIAN_POINT ( 'NONE',  ( 1.062992125984252745, -0.6692913385826771977, 8.415575281601705876E-17 ) ) ;
#14319=CARTESIAN_POINT ( 'NONE',  ( 1.076115485564305141, 0.2306618581243847221, -0.2411417322834647770 ) ) ;
#14320=CARTESIAN_POINT ( 'NONE',  ( -0.3740157480314953431, 0.07958543189024085140, 0.2665933059059887866 ) ) ;
#14321=CARTESIAN_POINT ( 'NONE',  ( 0.6824146981627303710, 0.2306618581243847221, -0.2411417322834647770 ) ) ;
#14323=CARTESIAN_POINT ( 'NONE',  ( -0.1837270341207340729, 0.1283753931104746893, -0.1820866141732285504 ) ) ;
#14324=CARTESIAN_POINT ( 'NONE',  ( 0.1181102362204730916, -0.6692913385826771977, 8.415575281601705876E-17 ) ) ;
#14326=CARTESIAN_POINT ( 'NONE',  ( -1.194225721784776262, 0.05413385826771626580, -0.4176697321401330321 ) ) ;
#14327=CARTESIAN_POINT ( 'NONE',  ( 0.4724409448818904789, -0.1870078740157479769, 0.3641732283464567677 ) ) ;
#14328=CARTESIAN_POINT ( 'NONE',  ( 1.417322834645670104, -0.1870078740157480601, -0.3641732283464567677 ) ) ;
#14329=CARTESIAN_POINT ( 'NONE',  ( -0.7349081364829390672, 0.2306618581243847221, -0.2411417322834647770 ) ) ;
#14330=CARTESIAN_POINT ( 'NONE',  ( -0.2493438320209966919, -0.3690944881889763329, 0.3153832671262228327 ) ) ;
#14331=CARTESIAN_POINT ( 'NONE',  ( -0.7478466213799872531, 1.968503937007873850, -0.5309055118110235227 ) ) ;
#14332=CARTESIAN_POINT ( 'NONE',  ( -0.7152230971128602510, -0.05778040916215560624, -0.4822834645669293319 ) ) ;
#14333=CARTESIAN_POINT ( 'NONE',  ( -0.5708661417322825615, -0.5400638737290844871, 0.3530559997133364547 ) ) ;
#14334=CARTESIAN_POINT ( 'NONE',  ( -0.03280839895013062252, 0.2952755905511810774, -0.1292274648535930714 ) ) ;
#14337=CARTESIAN_POINT ( 'NONE',  ( -1.489501312335957062, -0.2845877964562161244, -0.3641732283464567121 ) ) ;
#14338=CARTESIAN_POINT ( 'NONE',  ( 0.6036745406824154392, 0.1283753931104746893, -0.1820866141732285504 ) ) ;
#14339=CARTESIAN_POINT ( 'NONE',  ( 1.220472440944882386, -0.6692913385826771977, 8.415575281601705876E-17 ) ) ;
#14340=CARTESIAN_POINT ( 'NONE',  ( -0.6102362204724400829, 0.07958543189024085140, 0.2665933059059887866 ) ) ;
#14341=CARTESIAN_POINT ( 'NONE',  ( -1.128608923884513837, -0.5023911411419708095, 0.1820866141732285504 ) ) ;
#14342=CARTESIAN_POINT ( 'NONE',  ( -0.6692913385826764205, 0.2952755905511811885, 0.000000000000000000 ) ) ;
#14343=CARTESIAN_POINT ( 'NONE',  ( -0.6692913385826764205, -0.6692913385826771977, 8.415575281601705876E-17 ) ) ;
#14344=CARTESIAN_POINT ( 'NONE',  ( 0.6036745406824154392, 0.1283753931104746893, -0.1820866141732285504 ) ) ;
#14346=CARTESIAN_POINT ( 'NONE',  ( 1.043307086614173818, -0.4536011799217368745, -0.2665933059059886201 ) ) ;
#14347=CARTESIAN_POINT ( 'NONE',  ( 0.3674540682414705883, -0.6046776061558807314, 0.2411417322834647770 ) ) ;
#14349=CARTESIAN_POINT ( 'NONE',  ( -0.7283464566929126471, 0.1660481256975883668, -0.3530559997133364547 ) ) ;
#14352=CARTESIAN_POINT ( 'NONE',  ( 1.246719160104987623, -0.3690944881889763329, 0.3153832671262228327 ) ) ;
#14354=CARTESIAN_POINT ( 'NONE',  ( 0.4068241469816281097, 0.05413385826771666132, 0.4176697321401328100 ) ) ;
#14355=VECTOR ( 'NONE', #69831, 39.37007874015748143 ) ;
#14356=CARTESIAN_POINT ( 'NONE',  ( 0.2690288713910767848, 0.2952755905511811885, 0.1292274648535926551 ) ) ;
#14357=CARTESIAN_POINT ( 'NONE',  ( -0.1443569553805765515, -0.3690944881889765550, -0.3153832671262227771 ) ) ;
#14358=CARTESIAN_POINT ( 'NONE',  ( 0.6102362204724415262, 0.1012011053420775880, -0.2882089793578256898 ) ) ;
#14359=CARTESIAN_POINT ( 'NONE',  ( -0.07217847769028787330, -0.08942795157527998196, 0.3641732283464567121 ) ) ;
#14360=CARTESIAN_POINT ( 'NONE',  ( 0.5905511811023629321, 0.2952755905511811885, 0.000000000000000000 ) ) ;
#14361=CARTESIAN_POINT ( 'NONE',  ( -0.5577427821522301654, -0.08942795157528024563, -0.3641732283464568787 ) ) ;
#14362=CARTESIAN_POINT ( 'NONE',  ( -0.6167979002624665030, -0.4281496062992127816, -0.4176697321401328100 ) ) ;
#14363=CARTESIAN_POINT ( 'NONE',  ( -1.112371124080194340, -2.567464376874931580E-15, -0.4445507791589072832 ) ) ;
#14365=CARTESIAN_POINT ( 'NONE',  ( -1.299212598425196097, 0.2952755905511811885, 0.000000000000000000 ) ) ;
#14366=CARTESIAN_POINT ( 'NONE',  ( -1.017060367454067249, -0.2845877964562161244, -0.3641732283464567121 ) ) ;
#14367=CARTESIAN_POINT ( 'NONE',  ( -0.05905511811023545637, -0.5400638737290845981, -0.3530559997133363437 ) ) ;
#14368=CARTESIAN_POINT ( 'NONE',  ( -1.686351706036744558, 0.2952755905511810774, -0.1292274648535930714 ) ) ;
#14369=CARTESIAN_POINT ( 'NONE',  ( -0.7677165354330699465, -0.5400638737290845981, -0.3530559997133363437 ) ) ;
#14372=CARTESIAN_POINT ( 'NONE',  ( 0.8661417322834652488, -0.1870078740157480879, -0.4822834645669291653 ) ) ;
#14373=CARTESIAN_POINT ( 'NONE',  ( 0.9317585301837276734, 0.05413385826771626580, -0.4176697321401330321 ) ) ;
#14375=CARTESIAN_POINT ( 'NONE',  ( 1.555118110236221041, -0.5400638737290844871, 0.3530559997133364547 ) ) ;
#14376=CARTESIAN_POINT ( 'NONE',  ( -1.207349081364828880, 0.2306618581243847221, -0.2411417322834647770 ) ) ;
#14379=CARTESIAN_POINT ( 'NONE',  ( -0.4396325459317577122, -0.5511811023622048555, -0.09757992244046775898 ) ) ;
#14381=ORIENTED_EDGE ( 'NONE', *, *, #14233, .F. ) ;
#14382=CARTESIAN_POINT ( 'NONE',  ( 0.4724409448818904789, -0.1870078740157479769, 0.4822834645669291653 ) ) ;
#14383=CARTESIAN_POINT ( 'NONE',  ( -0.1640419947506555343, -0.3162353388693405765, 0.4822834645669290543 ) ) ;
#14384=CARTESIAN_POINT ( 'NONE',  ( -0.4986876640419939388, 0.2306618581243847221, -0.2411417322834647770 ) ) ;
#14385=CARTESIAN_POINT ( 'NONE',  ( 1.528871391076116026, 0.2952755905511811885, 0.1292274648535926551 ) ) ;
#14386=CARTESIAN_POINT ( 'NONE',  ( -0.9776902887139098386, 0.1771653543307087075, -0.09757992244046823083 ) ) ;
#14388=CARTESIAN_POINT ( 'NONE',  ( 0.9711286089238851948, -0.6046776061558809534, -0.2411417322834644161 ) ) ;
#14389=CARTESIAN_POINT ( 'NONE',  ( 0.6102362204724416372, -0.4536011799217367080, 0.2665933059059888421 ) ) ;
#14390=CARTESIAN_POINT ( 'NONE',  ( -0.3805774278215216522, 0.05413385826771666132, 0.4176697321401328100 ) ) ;
#14392=CARTESIAN_POINT ( 'NONE',  ( -0.8267716535433065062, 0.2952755905511811885, 0.000000000000000000 ) ) ;
#14395=CARTESIAN_POINT ( 'NONE',  ( 1.410761154855643795, -0.05778040916215560624, -0.4822834645669293319 ) ) ;
#14399=CARTESIAN_POINT ( 'NONE',  ( -0.1049868766404193215, -0.6046776061558807314, 0.2411417322834647770 ) ) ;
#14401=CARTESIAN_POINT ( 'NONE',  ( -1.272965879265091305, -0.4281496062992124485, 0.4176697321401328655 ) ) ;
#14402=B_SPLINE_CURVE_WITH_KNOTS ( 'NONE', 3,
 ( #80054, #75681, #40899, #22373 ),
 .UNSPECIFIED., .F., .F.,
 ( 4, 4 ),
 ( 3.593986969204291827E-07, 0.001287825409103293597 ),
 .UNSPECIFIED. ) ;
#14403=CARTESIAN_POINT ( 'NONE',  ( 1.476377952755906220, 0.1660481256975883668, -0.3530559997133364547 ) ) ;
#14404=CARTESIAN_POINT ( 'NONE',  ( 1.122047244094488860, 0.1660481256975885056, 0.3530559997133364547 ) ) ;
#14405=( BOUNDED_CURVE ( )  B_SPLINE_CURVE ( 2, ( #61553, #15294, #40955, #16955, #10633, #48911, #60311 ),
 .UNSPECIFIED., .F., .F. ) 
 B_SPLINE_CURVE_WITH_KNOTS ( ( 3, 2, 2, 3 ),
 ( 0.1477272727272727071, 0.1515151515151514916, 0.1553030303030303871, 0.1555121885203128163 ),
 .UNSPECIFIED. ) 
 CURVE ( )  GEOMETRIC_REPRESENTATION_ITEM ( )  RATIONAL_B_SPLINE_CURVE ( ( 1.000000000000000000, 0.9659258262890683122, 1.000000000000000000, 0.9659258262890683122, 1.000000000000000000, 0.9981185001348099606, 0.9964447847208435238 ) ) 
 REPRESENTATION_ITEM ( '' )  );
#14406=CARTESIAN_POINT ( 'NONE',  ( 0.2952755905511816326, -0.5400638737290844871, 0.3530559997133364547 ) ) ;
#14407=CARTESIAN_POINT ( 'NONE',  ( -0.3346456692913377662, 0.1660481256975883668, -0.3530559997133364547 ) ) ;
#14409=CARTESIAN_POINT ( 'NONE',  ( -1.082677165354329896, 0.1660481256975885056, 0.3530559997133364547 ) ) ;
#14410=CARTESIAN_POINT ( 'NONE',  ( -0.4068241469816264999, -0.4281496062992124485, 0.4176697321401328655 ) ) ;
#14411=CARTESIAN_POINT ( 'NONE',  ( -0.5446194225721777693, -0.08942795157527998196, 0.3641732283464567121 ) ) ;
#14413=CARTESIAN_POINT ( 'NONE',  ( -0.4855643044619415427, -0.4281496062992124485, 0.4176697321401328655 ) ) ;
#14415=AXIS2_PLACEMENT_3D ( 'NONE', #36493, #24273, #49944 ) ;
#14416=CARTESIAN_POINT ( 'NONE',  ( 0.8530183727034126306, 0.05413385826771626580, -0.4176697321401330321 ) ) ;
#14419=CARTESIAN_POINT ( 'NONE',  ( -0.2559055118110227234, -0.5400638737290844871, 0.3530559997133364547 ) ) ;
#14420=CARTESIAN_POINT ( 'NONE',  ( -0.2952755905511804668, 0.07958543189024085140, 0.2665933059059887866 ) ) ;
#14422=CARTESIAN_POINT ( 'NONE',  ( 0.8792650918635177559, -0.004921259842519576551, 0.3153832671262227771 ) ) ;
#14423=CARTESIAN_POINT ( 'NONE',  ( -0.9186351706036736120, 0.1539470093639523085, 0.1968503937007873850 ) ) ;
#14425=CARTESIAN_POINT ( 'NONE',  ( 1.128608923884515169, -0.5023911411419708095, -0.1820866141732282451 ) ) ;
#14426=CARTESIAN_POINT ( 'NONE',  ( 1.253280839895013710, -0.3162353388693405765, 0.4822834645669290543 ) ) ;
#14428=CARTESIAN_POINT ( 'NONE',  ( 0.1837270341207354329, 0.2306618581243848609, 0.2411417322834645549 ) ) ;
#14429=DIRECTION ( 'NONE',  ( 1.000000000000000000, 0.000000000000000000, -1.692413147294446216E-16 ) ) ;
#14430=CARTESIAN_POINT ( 'NONE',  ( 1.614173228346457378, 0.1771653543307087630, 0.000000000000000000 ) ) ;
#14431=CARTESIAN_POINT ( 'NONE',  ( -0.3674540682414692561, -0.6046776061558809534, -0.2411417322834644161 ) ) ;
#14433=CARTESIAN_POINT ( 'NONE',  ( 1.574803149606299746, -0.1870078740157480879, -0.4822834645669291653 ) ) ;
#14434=CARTESIAN_POINT ( 'NONE',  ( 0.6102362204724416372, -0.5400638737290844871, 0.3530559997133364547 ) ) ;
#14435=CARTESIAN_POINT ( 'NONE',  ( 0.8398950131233602345, -0.5023911411419708095, 0.1820866141732285504 ) ) ;
#14436=DIRECTION ( 'NONE',  ( -0.7071067811865463515, -2.189697074797793155E-16, -0.7071067811865486830 ) ) ;
#14437=CARTESIAN_POINT ( 'NONE',  ( 0.2690288713910767848, 0.1771653543307087630, 0.09757992244046791164 ) ) ;
#14438=CARTESIAN_POINT ( 'NONE',  ( -1.135170603674539924, 0.2952755905511810774, -0.1292274648535930714 ) ) ;
#14440=CARTESIAN_POINT ( 'NONE',  ( 1.305774278215223960, -0.6692913385826771977, 0.1292274648535927661 ) ) ;
#14442=CARTESIAN_POINT ( 'NONE',  ( 0.3149606299212606708, -0.1870078740157480879, -0.4822834645669291653 ) ) ;
#14445=CARTESIAN_POINT ( 'NONE',  ( 0.5905511811023629321, -0.5511811023622047445, 6.969142054262312111E-17 ) ) ;
#14446=CARTESIAN_POINT ( 'NONE',  ( 0.4593175853018380828, 0.05413385826771626580, -0.4176697321401330321 ) ) ;
#14448=CARTESIAN_POINT ( 'NONE',  ( -0.7480314960629914633, 0.1771653543307087630, 0.000000000000000000 ) ) ;
#14449=CARTESIAN_POINT ( 'NONE',  ( -1.069553805774277722, 0.2952755905511811885, 0.1292274648535926551 ) ) ;
#14450=CARTESIAN_POINT ( 'NONE',  ( -1.725721784776902190, -0.05778040916215522460, 0.4822834645669289988 ) ) ;
#14451=CARTESIAN_POINT ( 'NONE',  ( 0.8333333333333340365, -0.6692913385826771977, 0.1292274648535927661 ) ) ;
#14452=CARTESIAN_POINT ( 'NONE',  ( 1.614173228346457378, -0.6692913385826771977, 8.415575281601705876E-17 ) ) ;
#14454=CARTESIAN_POINT ( 'NONE',  ( 0.6889763779527563470, 0.1660481256975883668, -0.3530559997133364547 ) ) ;
#14456=CARTESIAN_POINT ( 'NONE',  ( 1.581364829396326277, -0.3162353388693409650, -0.4822834645669289433 ) ) ;
#14457=CARTESIAN_POINT ( 'NONE',  ( 1.601049868766404982, -0.6046776061558809534, -0.2411417322834644161 ) ) ;
#14458=CARTESIAN_POINT ( 'NONE',  ( -1.574803149606298636, -0.1870078740157479769, 0.3641732283464567677 ) ) ;
#14459=CARTESIAN_POINT ( 'NONE',  ( 1.417322834645670104, -0.1870078740157480601, -0.3641732283464567677 ) ) ;
#14460=CARTESIAN_POINT ( 'NONE',  ( -1.312335958005248715, 0.1283753931104748280, 0.1820866141732283561 ) ) ;
#14461=CARTESIAN_POINT ( 'NONE',  ( -0.4593175853018364174, -0.3690944881889765550, -0.3153832671262227771 ) ) ;
#14463=CARTESIAN_POINT ( 'NONE',  ( 0.3215223097112867578, -0.08942795157527998196, 0.3641732283464567121 ) ) ;
#14464=CARTESIAN_POINT ( 'NONE',  ( 0.5249343832021005074, -0.6046776061558807314, 0.2411417322834647770 ) ) ;
#14465=CARTESIAN_POINT ( 'NONE',  ( 0.9055118110236227702, -0.6692913385826771977, 8.415575281601705876E-17 ) ) ;
#14466=CARTESIAN_POINT ( 'NONE',  ( -0.03280839895013062252, 0.2952755905511810774, -0.1292274648535930714 ) ) ;
#14467=CARTESIAN_POINT ( 'NONE',  ( 0.05905511811023681640, 0.07958543189024071263, -0.2665933059059888421 ) ) ;
#14468=CARTESIAN_POINT ( 'NONE',  ( 1.030183727034121421, -0.3162353388693409650, -0.4822834645669289433 ) ) ;
#14469=CARTESIAN_POINT ( 'NONE',  ( -1.436417322834644850, 2.401574803149606474, 0.3149606299212598381 ) ) ;
#14470=CARTESIAN_POINT ( 'NONE',  ( -1.148293963254592542, -0.6692913385826773087, -0.1292274648535924053 ) ) ;
#14473=CARTESIAN_POINT ( 'NONE',  ( 0.01312335958005323398, 0.05413385826771666132, 0.4176697321401328100 ) ) ;
#14475=CARTESIAN_POINT ( 'NONE',  ( -0.8530183727034112984, 0.05413385826771666132, 0.4176697321401328100 ) ) ;
#14476=CARTESIAN_POINT ( 'NONE',  ( -0.09186351706036689768, 0.05413385826771626580, -0.4176697321401330321 ) ) ;
#14481=CARTESIAN_POINT ( 'NONE',  ( -0.9973753280839886548, -0.5023911411419708095, -0.1820866141732282451 ) ) ;
#14483=CARTESIAN_POINT ( 'NONE',  ( -1.528871391076114250, 0.2952755905511810774, -0.1292274648535930714 ) ) ;
#14485=CARTESIAN_POINT ( 'NONE',  ( 0.4855643044619430415, -0.4281496062992127816, -0.4176697321401328100 ) ) ;
#14486=CARTESIAN_POINT ( 'NONE',  ( -0.6955380577427815458, -0.3690944881889765550, -0.3153832671262227771 ) ) ;
#14487=CARTESIAN_POINT ( 'NONE',  ( 0.7283464566929140904, -0.5400638737290845981, -0.3530559997133363437 ) ) ;
#14488=EDGE_CURVE ( 'NONE', #38370, #39166, #63901, .T. ) ;
#14489=CARTESIAN_POINT ( 'NONE',  ( 0.4330708661417329575, -0.6692913385826771977, 8.415575281601705876E-17 ) ) ;
#14493=CARTESIAN_POINT ( 'NONE',  ( 1.246719160104987623, 0.05413385826771626580, -0.4176697321401330321 ) ) ;
#14494=CARTESIAN_POINT ( 'NONE',  ( 0.2099737532808405305, 0.2306618581243847221, -0.2411417322834647770 ) ) ;
#14495=CARTESIAN_POINT ( 'NONE',  ( 0.1115485564304467270, -0.6692913385826773087, -0.1292274648535924053 ) ) ;
#14496=CARTESIAN_POINT ( 'NONE',  ( 1.561679790026247350, -0.4281496062992124485, 0.4176697321401328655 ) ) ;
#14497=CARTESIAN_POINT ( 'NONE',  ( 0.9842519685039378130, -0.6692913385826771977, 8.415575281601705876E-17 ) ) ;
#14499=CARTESIAN_POINT ( 'NONE',  ( 0.03937007874015806264, 0.2952755905511811885, 0.000000000000000000 ) ) ;
#14500=CARTESIAN_POINT ( 'NONE',  ( 0.5446194225721792126, -0.3162353388693405765, 0.4822834645669290543 ) ) ;
#14501=CARTESIAN_POINT ( 'NONE',  ( -0.1968503937007867743, 0.2952755905511811885, 0.000000000000000000 ) ) ;
#14502=CARTESIAN_POINT ( 'NONE',  ( 1.213910761154856299, 0.1771653543307087630, 0.09757992244046791164 ) ) ;
#14503=CARTESIAN_POINT ( 'NONE',  ( -1.161417322834644716, -0.5400638737290845981, -0.3530559997133363437 ) ) ;
#14504=CARTESIAN_POINT ( 'NONE',  ( -1.345144356955379816, -0.05778040916215560624, -0.4822834645669293319 ) ) ;
#14505=CARTESIAN_POINT ( 'NONE',  ( 0.8333333333333340365, 0.2952755905511810774, -0.1292274648535930714 ) ) ;
#14508=EDGE_LOOP ( 'NONE', ( #38270, #18187, #75997, #81159 ) ) ;
#14510=EDGE_LOOP ( 'NONE', ( #52032, #79912, #31299, #1158 ) ) ;
#14511=CARTESIAN_POINT ( 'NONE',  ( 1.030183727034121421, -0.05778040916215522460, 0.4822834645669289988 ) ) ;
#14512=CARTESIAN_POINT ( 'NONE',  ( 0.9842519685039375910, 0.1771653543307087630, 0.000000000000000000 ) ) ;
#14517=CARTESIAN_POINT ( 'NONE',  ( 1.509186351706037543, -0.4281496062992127816, -0.4176697321401328100 ) ) ;
#14518=CARTESIAN_POINT ( 'NONE',  ( -1.581364829396324945, -0.05778040916215560624, -0.4822834645669293319 ) ) ;
#14519=CARTESIAN_POINT ( 'NONE',  ( -0.1443569553805768291, 0.05413385826771666132, 0.4176697321401328100 ) ) ;
#14520=CARTESIAN_POINT ( 'NONE',  ( 0.9842519685039375910, 0.2952755905511811885, 0.000000000000000000 ) ) ;
#14521=EDGE_LOOP ( 'NONE', ( #64583, #50377, #65608, #7823 ) ) ;
#14522=ADVANCED_FACE ( 'NONE', ( #1789 ), #72077, .F. ) ;
#14523=CARTESIAN_POINT ( 'NONE',  ( -1.443569553805773564, -0.6046776061558807314, 0.2411417322834647770 ) ) ;
#14524=CARTESIAN_POINT ( 'NONE',  ( 0.5419760673063066525, 1.535433070866141447, 0.4915354330708653907 ) ) ;
#14526=CARTESIAN_POINT ( 'NONE',  ( -1.604771003085130543, 0.7690346235818137366, -0.1466069496707740616 ) ) ;
#14527=DIRECTION ( 'NONE',  ( 0.000000000000000000, 1.000000000000000000, 0.000000000000000000 ) ) ;
#14528=CARTESIAN_POINT ( 'NONE',  ( -0.7349081364829387342, -0.5023911411419708095, 0.1820866141732285504 ) ) ;
#14529=( BOUNDED_SURFACE ( )  B_SPLINE_SURFACE ( 1, 2, ( 
 ( #8611, #33862, #1471, #40590, #41422, #78913, #8196, #54033, #22481, #15771, #60364, #41010, #35108, #3125, #16180, #27959, #2711, #22062, #72996, #21234, #59943, #72170, #67517, #72583, #67106, #27125, #52789, #59526, #20821, #1883, #53200, #53618, #46890, #14931, #21646, #47306, #30851, #55688, #35942, #11514, #17425, #30441, #61612, #61186, #42239, #80987, #17832, #43466, #82218, #80580, #23300, #10691, #16594, #69163, #56106, #67934, #18239, #37170, #74252, #68351, #62850, #5186, #29208, #23712, #54874, #49383, #3954, #56515, #17014, #10275, #29616, #75078, #11095, #55277, #48970, #74670, #24537, #50202, #22888, #42654, #75899, #36346, #43880, #69578, #62021, #36753, #4357, #48555, #30025, #81396, #35524, #43056, #68753, #62428, #4766, #3541, #81811, #24122, #49791, #75493, #45963, #7264, #6426, #32512, #37991, #56927, #77137, #57756, #51434, #25773, #64926, #63667, #45545, #6008, #64503, #32095, #45120, #58174, #71243, #76315, #118, #58601, #12335, #44698, #70828, #970, #26624, #52278, #25357, #82622, #19470, #18645, #77564, #77982, #32936, #11925, #31677, #13175, #38825, #20312, #57337, #70395, #51020, #6841, #37580, #13587, #63253, #24937, #31260, #50608, #19051, #39243, #69980, #543, #5594, #83033, #26196, #76719, #12751, #51857, #19898, #44289, #38408, #64089, #40918, #28282, #9350, #27450, #41337, #53944, #65776, #21149, #14844, #53533, #8108, #33363, #59026, #3035, #15676, #59436, #72495, #22391, #21556, #40504, #52695, #2626, #78402, #59853, #80074, #33774, #79241, #35021, #60276, #2205, #47635, #46804, #66186, #46385, #8521, #60685, #20734, #78820, #79657, #21973, #15259, #73329, #71660, #72907, #66600, #1790, #47217, #67017, #72078, #28700, #34189, #34611, #8934, #14437, #40089, #53111, #54362, #27873, #14011, #39668, #65358, #7696, #1381, #27033, #29928, #74989, #62331, #73752, #17334, #16921, #54782, #48876, #42558, #61517, #3862, #10996, #4668, #68658, #4266, #61924, #67427, #30341, #9761, #36656, #68262, #55591, #23205, #81718, #48051, #24028, #56007, #16088, #67844, #10598, #36254, #41733, #10183, #74576, #80892, #81303, #35432, #49696, #61097, #22799, #80485, #16506, #23617, #75392, #35848, #49286, #3448, #42964, #29112, #48458, #74158, #42149, #29522, #55184, #15521, #33621, #9199, #79918, #60942, #79090, #9610, #22235, #34035, #72754, #66443, #21814, #59696, #1641, #27299, #54622, #67277, #27716, #40759, #74004, #73170, #8780, #20993, #54202, #46655, #28132, #48307, #2052, #47478, #3292, #28546, #53787, #15940, #15103, #34453, #14696, #60122, #28957, #72348, #47062, #47890, #73598, #66869, #41587, #39942, #41179, #34872, #53383, #60533, #35279, #40352, #80333, #2473, #2883, #22648, #66031, #8369, #21408, #65628, #79499, #7959, #59284, #52957, #78672, #70558, #51596, #38571, #50777, #78143, #76880, #20053, #7428, #64666, #18804, #14173, #13750, #77298, #12914, #45290, #33098, #19629, #7005, #58764, #282, #63829, #39407, #70986, #58339, #6167, #5755, #70141, #25517, #45706, #71402, #26777, #25104, #51182, #64252, #44449, #13330, #12493, #77724, #1127, #6586, #38156, #63418, #44859, #65090, #83195, #31842, #701, #52433, #20475, #38983, #32673, #46129, #71823, #31425, #32257, #26358, #19211, #57918, #52018, #25937, #76477, #57087, #82783, #57504, #67179, #41078, #78566, #73909, #73496, #53686, #46958, #21713, #9508, #79394, #66767, #35181, #60016, #40245, #15844, #47377, #34773, #65928, #65520, #46545, #1950, #22134, #47792, #3194, #1537, #27612, #15000, #20892, #41493, #60432, #72243, #22551, #60842, #14592, #72650, #28858, #54520, #33517, #28028, #59180, #73068, #8265, #80235, #21305, #33930, #59595, #15417, #9100, #53275, #78985, #40657, #48213, #39831, #27192, #66342, #7851, #8680, #52856, #34350, #2371, #2783, #28443, #54102, #79818, #29275, #11584, #68003, #30096, #3609, #49037, #16249, #67590, #41896, #75560, #74319, #50272, #37244, #10755, #36828, #42305, #61255, #81465, #62088, #55759, #23783, #69236, #10348, #49860, #36009, #68822, #36415, #49454, #62501, #17900, #80645, #4430, #62920, #16666, #74734, #43537, #61679 ),
 ( #4020, #75148, #30514, #22958, #81879, #17493, #4839, #43124, #48624, #29684, #55347, #56176, #81053, #23369, #5253, #24603, #24191, #11167, #17082, #30917, #56584, #82285, #9921, #35592, #54939, #42719, #68415, #32161, #25420, #51085, #77627, #13651, #51922, #45187, #19530, #37645, #39304, #63322, #45610, #57817, #70890, #12817, #32995, #75969, #64991, #7327, #58665, #6072, #5660, #184, #56992, #58239, #1030, #71303, #26683, #70045, #6491, #25837, #18310, #76379, #76782, #31746, #51496, #43951, #26261, #69647, #31327, #11991, #82689, #83100, #19959, #50681, #70460, #25008, #38056, #38474, #57408, #19114, #77200, #64158, #13240, #38889, #18713, #64568, #32576, #44354, #44763, #12399, #605, #63733, #6905, #78885, #34253, #46448, #14077, #39729, #67077, #79718, #40150, #53170, #3097, #2269, #21206, #33424, #66663, #59085, #40562, #60745, #14497, #59914, #15741, #65834, #59499, #22035, #52339, #72967, #14902, #1440, #41395, #34674, #47695, #78046, #60337, #66243, #27097, #8581, #27932, #1852, #27514, #54006, #73390, #28345, #21617, #79299, #65424, #9409, #7758, #35079, #53590, #47277, #72555, #20375, #46027, #71721, #52759, #78467, #8167, #20792, #15318, #72141, #2685, #33832, #46861, #40983, #9002, #42626, #10661, #37139, #29178, #3926, #67908, #68323, #17802, #62398, #62824, #73812, #48114, #67487, #35915, #30410, #3509, #23270, #69133, #74222, #48939, #10244, #29585, #29994, #74641, #16983, #4328, #22455, #81367, #68723, #49763, #61581, #81783, #11064, #22861, #55248, #80955, #36316, #48522, #16149, #41796, #43436, #56078, #16567, #61991, #28761, #55657, #23680, #9823, #43028, #35493, #49354, #54424, #42212, #75051, #75463, #17398, #36722, #4737, #24094, #11485, #54845, #80134, #61158, #80549, #12305, #13145, #70793, #32064, #38796, #39210, #6394, #57725, #24911, #38378, #19438, #69550, #64472, #50988, #51404, #88, #11898, #31231, #50579, #77106, #45089, #32480, #25741, #43847, #5159, #6809, #19020, #37962, #70363, #58143, #44668, #512, #26165, #25324, #5566, #51826, #12718, #77531, #56898, #30823, #37552, #76286, #19866, #45515, #71211, #50174, #18617, #63638, #63226, #13554, #56488, #82592, #82190, #24507, #44260, #5976, #75869, #18212, #69951, #76686, #31647, #64054, #57305, #83003, #46356, #39637, #20281, #53080, #40476, #65328, #1353, #7665, #53914, #34579, #52247, #27004, #21945, #40061, #8903, #28253, #33336, #66154, #58997, #26595, #8081, #77952, #60247, #52666, #78793, #45930, #14407, #64895, #32905, #7232, #40887, #78373, #15647, #2595, #59405, #2176, #20704, #71629, #46777, #27419, #21117, #72468, #79627, #72050, #15228, #65748, #34160, #1762, #14817, #27843, #66569, #13981, #8493, #47604, #33744, #59821, #53504, #79212, #21528, #73298, #47187, #72879, #58572, #937, #23587, #61069, #48021, #36225, #36627, #81271, #74547, #23176, #74960, #17306, #62304, #10154, #61894, #3420, #48431, #29494, #16475, #28672, #55980, #54753, #16060, #80043, #55153, #16892, #41707, #29083, #67399, #30312, #10968, #54333, #80459, #81691, #42122, #68628, #4641, #9734, #42531, #35405, #3005, #67817, #22362, #24002, #22768, #80864, #73721, #74130, #41303, #9321, #66989, #42933, #35820, #75360, #49670, #61485, #4235, #3834, #48846, #68233, #10567, #29899, #55563, #34991, #49258, #60656, #69454, #70265, #37868, #50894, #38278, #77007, #82094, #63543, #64373, #18115, #50482, #76594, #56396, #31967, #70689, #76186, #75774, #17708, #82499, #45012, #37459, #24408, #12620, #13042, #57628, #18924, #82908, #51305, #19340, #38695, #69859, #63955, #63132, #24815, #5876, #18523, #5064, #32379, #31133, #25642, #44990, #44573, #50078, #51724, #6710, #31550, #44166, #25229, #58043, #57207, #6292, #408, #26065, #43748, #43336, #69037, #11387, #11804, #37044, #5471, #56799, #62726, #30733, #12210, #39109, #39535, #52562, #58470, #2074, #14718, #834, #60143, #27739, #32803, #26903, #53404, #47085, #71110, #65650, #13453, #7979, #45829, #79112, #58895, #33643, #64791, #78271, #77426, #45414, #19761, #21430, #52144, #28154, #72775, #71950, #40372, #20179, #7129, #59305, #39963 ) ),
 .UNSPECIFIED., .F., .F., .F. ) 
 B_SPLINE_SURFACE_WITH_KNOTS ( ( 2, 2 ),
 ( 3, 2, 2, 2, 2, 2, 2, 2, 2, 2, 2, 2, 2, 2, 2, 2, 2, 2, 2, 2, 2, 2, 2, 2, 2, 2, 2, 2, 2, 2, 2, 2, 2, 2, 2, 2, 2, 2, 2, 2, 2, 2, 2, 2, 2, 2, 2, 2, 2, 2, 2, 2, 2, 2, 2, 2, 2, 2, 2, 2, 2, 2, 2, 2, 2, 2, 2, 2, 2, 2, 2, 2, 2, 2, 2, 2, 2, 2, 2, 2, 2, 2, 2, 2, 2, 2, 2, 2, 2, 2, 2, 2, 2, 2, 2, 2, 2, 2, 2, 2, 2, 2, 2, 2, 2, 2, 2, 2, 2, 2, 2, 2, 2, 2, 2, 2, 2, 2, 2, 2, 2, 2, 2, 2, 2, 2, 2, 2, 2, 2, 2, 2, 2, 2, 2, 2, 2, 2, 2, 2, 2, 2, 2, 2, 2, 2, 2, 2, 2, 2, 2, 2, 2, 2, 2, 2, 2, 2, 2, 2, 2, 2, 2, 2, 2, 2, 2, 2, 2, 2, 2, 2, 2, 2, 2, 2, 2, 2, 2, 2, 2, 2, 2, 2, 2, 2, 2, 2, 2, 2, 2, 2, 2, 2, 2, 2, 2, 2, 2, 2, 2, 2, 2, 2, 2, 2, 2, 2, 2, 2, 2, 2, 2, 2, 2, 2, 2, 2, 2, 2, 2, 2, 2, 2, 2, 2, 2, 2, 2, 2, 2, 2, 2, 2, 2, 2, 2, 2, 2, 2, 2, 2, 2, 2, 2, 2, 2, 2, 2, 2, 2, 2, 2, 2, 2, 3 ),
 ( 0.000000000000000000, 1.000000000000000000 ),
 ( 0.000000000000000000, 0.003787878787878787984, 0.007575757575757575968, 0.01136363636363636395, 0.01515151515151515194, 0.01893939393939393992, 0.02272727272727272790, 0.02651515151515151589, 0.03030303030303030387, 0.03409090909090908839, 0.03787878787878787984, 0.04166666666666666435, 0.04545454545454545581, 0.04924242424242424032, 0.05303030303030303177, 0.05681818181818181629, 0.06060606060606060774, 0.06439393939393939226, 0.06818181818181817677, 0.07196969696969697516, 0.07575757575757575968, 0.07954545454545454419, 0.08333333333333332871, 0.08712121212121212710, 0.09090909090909091161, 0.09469696969696969613, 0.09848484848484848064, 0.1022727272727272790, 0.1060606060606060635, 0.1098484848484848481, 0.1136363636363636326, 0.1174242424242424310, 0.1212121212121212155, 0.1250000000000000000, 0.1287878787878787845, 0.1325757575757575690, 0.1363636363636363535, 0.1401515151515151381, 0.1439393939393939503, 0.1477272727272727348, 0.1515151515151515194, 0.1553030303030303039, 0.1590909090909090884, 0.1628787878787878729, 0.1666666666666666574, 0.1704545454545454419, 0.1742424242424242542, 0.1780303030303030387, 0.1818181818181818232, 0.1856060606060606077, 0.1893939393939393923, 0.1931818181818181768, 0.1969696969696969613, 0.2007575757575757458, 0.2045454545454545581, 0.2083333333333333426, 0.2121212121212121271, 0.2159090909090909116, 0.2196969696969696961, 0.2234848484848484806, 0.2272727272727272652, 0.2310606060606060497, 0.2348484848484848619, 0.2386363636363636465, 0.2424242424242424310, 0.2462121212121212155, 0.2500000000000000000, 0.2537878787878787845, 0.2575757575757575690, 0.2613636363636363535, 0.2651515151515151381, 0.2689393939393939226, 0.2727272727272727071, 0.2765151515151514916, 0.2803030303030302761, 0.2840909090909091161, 0.2878787878787879007, 0.2916666666666666852, 0.2954545454545454697, 0.2992424242424242542, 0.3030303030303030387, 0.3068181818181818232, 0.3106060606060606077, 0.3143939393939393923, 0.3181818181818181768, 0.3219696969696969613, 0.3257575757575757458, 0.3295454545454545303, 0.3333333333333333148, 0.3371212121212120993, 0.3409090909090908839, 0.3446969696969697239, 0.3484848484848485084, 0.3522727272727272929, 0.3560606060606060774, 0.3598484848484848619, 0.3636363636363636465, 0.3674242424242424310, 0.3712121212121212155, 0.3750000000000000000, 0.3787878787878787845, 0.3825757575757575690, 0.3863636363636363535, 0.3901515151515151381, 0.3939393939393939226, 0.3977272727272727071, 0.4015151515151514916, 0.4053030303030302761, 0.4090909090909091161, 0.4128787878787879007, 0.4166666666666666852, 0.4204545454545454697, 0.4242424242424242542, 0.4280303030303030387, 0.4318181818181818232, 0.4356060606060606077, 0.4393939393939393923, 0.4431818181818181768, 0.4469696969696969613, 0.4507575757575757458, 0.4545454545454545303, 0.4583333333333333148, 0.4621212121212120993, 0.4659090909090908839, 0.4696969696969697239, 0.4734848484848485084, 0.4772727272727272929, 0.4810606060606060774, 0.4848484848484848619, 0.4886363636363636465, 0.4924242424242424310, 0.4962121212121212155, 0.5000000000000000000, 0.5037878787878787845, 0.5075757575757575690, 0.5113636363636363535, 0.5151515151515151381, 0.5189393939393939226, 0.5227272727272727071, 0.5265151515151514916, 0.5303030303030302761, 0.5340909090909090606, 0.5378787878787878451, 0.5416666666666666297, 0.5454545454545454142, 0.5492424242424241987, 0.5530303030303029832, 0.5568181818181817677, 0.5606060606060605522, 0.5643939393939394478, 0.5681818181818182323, 0.5719696969696970168, 0.5757575757575758013, 0.5795454545454545858, 0.5833333333333333703, 0.5871212121212121549, 0.5909090909090909394, 0.5946969696969697239, 0.5984848484848485084, 0.6022727272727272929, 0.6060606060606060774, 0.6098484848484848619, 0.6136363636363636465, 0.6174242424242424310, 0.6212121212121212155, 0.6250000000000000000, 0.6287878787878787845, 0.6325757575757575690, 0.6363636363636363535, 0.6401515151515151381, 0.6439393939393939226, 0.6477272727272727071, 0.6515151515151514916, 0.6553030303030302761, 0.6590909090909090606, 0.6628787878787878451, 0.6666666666666666297, 0.6704545454545454142, 0.6742424242424241987, 0.6780303030303029832, 0.6818181818181817677, 0.6856060606060605522, 0.6893939393939394478, 0.6931818181818182323, 0.6969696969696970168, 0.7007575757575758013, 0.7045454545454545858, 0.7083333333333333703, 0.7121212121212121549, 0.7159090909090909394, 0.7196969696969697239, 0.7234848484848485084, 0.7272727272727272929, 0.7310606060606060774, 0.7348484848484848619, 0.7386363636363636465, 0.7424242424242424310, 0.7462121212121212155, 0.7500000000000000000, 0.7537878787878787845, 0.7575757575757575690, 0.7613636363636363535, 0.7651515151515151381, 0.7689393939393939226, 0.7727272727272727071, 0.7765151515151514916, 0.7803030303030302761, 0.7840909090909090606, 0.7878787878787878451, 0.7916666666666666297, 0.7954545454545454142, 0.7992424242424241987, 0.8030303030303029832, 0.8068181818181817677, 0.8106060606060605522, 0.8143939393939394478, 0.8181818181818182323, 0.8219696969696970168, 0.8257575757575758013, 0.8295454545454545858, 0.8333333333333333703, 0.8371212121212121549, 0.8409090909090909394, 0.8446969696969697239, 0.8484848484848485084, 0.8522727272727272929, 0.8560606060606060774, 0.8598484848484848619, 0.8636363636363636465, 0.8674242424242424310, 0.8712121212121212155, 0.8750000000000000000, 0.8787878787878787845, 0.8825757575757575690, 0.8863636363636363535, 0.8901515151515151381, 0.8939393939393939226, 0.8977272727272727071, 0.9015151515151514916, 0.9053030303030302761, 0.9090909090909090606, 0.9128787878787878451, 0.9166666666666666297, 0.9204545454545454142, 0.9242424242424241987, 0.9280303030303029832, 0.9318181818181817677, 0.9356060606060605522, 0.9393939393939394478, 0.9431818181818182323, 0.9469696969696970168, 0.9507575757575758013, 0.9545454545454545858, 0.9583333333333333703, 0.9621212121212121549, 0.9659090909090909394 ),
 .UNSPECIFIED. ) 
 GEOMETRIC_REPRESENTATION_ITEM ( )  RATIONAL_B_SPLINE_SURFACE ( (
 ( 1.000000000000000000, 0.9659258262890683122, 1.000000000000000000, 0.9659258262890683122, 1.000000000000000000, 0.9659258262890683122, 1.000000000000000000, 0.9659258262890683122, 1.000000000000000000, 0.9659258262890683122, 1.000000000000000000, 0.9659258262890683122, 1.000000000000000000, 0.9659258262890683122, 1.000000000000000000, 0.9659258262890683122, 1.000000000000000000, 0.9659258262890683122, 1.000000000000000000, 0.9659258262890683122, 1.000000000000000000, 0.9659258262890683122, 1.000000000000000000, 0.9659258262890683122, 1.000000000000000000, 0.9659258262890683122, 1.000000000000000000, 0.9659258262890683122, 1.000000000000000000, 0.9659258262890683122, 1.000000000000000000, 0.9659258262890683122, 1.000000000000000000, 0.9659258262890683122, 1.000000000000000000, 0.9659258262890683122, 1.000000000000000000, 0.9659258262890683122, 1.000000000000000000, 0.9659258262890683122, 1.000000000000000000, 0.9659258262890683122, 1.000000000000000000, 0.9659258262890683122, 1.000000000000000000, 0.9659258262890683122, 1.000000000000000000, 0.9659258262890683122, 1.000000000000000000, 0.9659258262890683122, 1.000000000000000000, 0.9659258262890683122, 1.000000000000000000, 0.9659258262890683122, 1.000000000000000000, 0.9659258262890683122, 1.000000000000000000, 0.9659258262890683122, 1.000000000000000000, 0.9659258262890683122, 1.000000000000000000, 0.9659258262890683122, 1.000000000000000000, 0.9659258262890683122, 1.000000000000000000, 0.9659258262890683122, 1.000000000000000000, 0.9659258262890683122, 1.000000000000000000, 0.9659258262890683122, 1.000000000000000000, 0.9659258262890683122, 1.000000000000000000, 0.9659258262890683122, 1.000000000000000000, 0.9659258262890683122, 1.000000000000000000, 0.9659258262890683122, 1.000000000000000000, 0.9659258262890683122, 1.000000000000000000, 0.9659258262890683122, 1.000000000000000000, 0.9659258262890683122, 1.000000000000000000, 0.9659258262890683122, 1.000000000000000000, 0.9659258262890683122, 1.000000000000000000, 0.9659258262890683122, 1.000000000000000000, 0.9659258262890683122, 1.000000000000000000, 0.9659258262890683122, 1.000000000000000000, 0.9659258262890683122, 1.000000000000000000, 0.9659258262890683122, 1.000000000000000000, 0.9659258262890683122, 1.000000000000000000, 0.9659258262890683122, 1.000000000000000000, 0.9659258262890683122, 1.000000000000000000, 0.9659258262890683122, 1.000000000000000000, 0.9659258262890683122, 1.000000000000000000, 0.9659258262890683122, 1.000000000000000000, 0.9659258262890683122, 1.000000000000000000, 0.9659258262890683122, 1.000000000000000000, 0.9659258262890683122, 1.000000000000000000, 0.9659258262890683122, 1.000000000000000000, 0.9659258262890683122, 1.000000000000000000, 0.9659258262890683122, 1.000000000000000000, 0.9659258262890683122, 1.000000000000000000, 0.9659258262890683122, 1.000000000000000000, 0.9659258262890683122, 1.000000000000000000, 0.9659258262890683122, 1.000000000000000000, 0.9659258262890683122, 1.000000000000000000, 0.9659258262890683122, 1.000000000000000000, 0.9659258262890683122, 1.000000000000000000, 0.9659258262890683122, 1.000000000000000000, 0.9659258262890683122, 1.000000000000000000, 0.9659258262890683122, 1.000000000000000000, 0.9659258262890683122, 1.000000000000000000, 0.9659258262890683122, 1.000000000000000000, 0.9659258262890683122, 1.000000000000000000, 0.9659258262890683122, 1.000000000000000000, 0.9659258262890683122, 1.000000000000000000, 0.9659258262890683122, 1.000000000000000000, 0.9659258262890683122, 1.000000000000000000, 0.9659258262890683122, 1.000000000000000000, 0.9659258262890683122, 1.000000000000000000, 0.9659258262890683122, 1.000000000000000000, 0.9659258262890683122, 1.000000000000000000, 0.9659258262890683122, 1.000000000000000000, 0.9659258262890683122, 1.000000000000000000, 0.9659258262890683122, 1.000000000000000000, 0.9659258262890683122, 1.000000000000000000, 0.9659258262890683122, 1.000000000000000000, 0.9659258262890683122, 1.000000000000000000, 0.9659258262890683122, 1.000000000000000000, 0.9659258262890683122, 1.000000000000000000, 0.9659258262890683122, 1.000000000000000000, 0.9659258262890683122, 1.000000000000000000, 0.9659258262890683122, 1.000000000000000000, 0.9659258262890683122, 1.000000000000000000, 0.9659258262890683122, 1.000000000000000000, 0.9659258262890683122, 1.000000000000000000, 0.9659258262890683122, 1.000000000000000000, 0.9659258262890683122, 1.000000000000000000, 0.9659258262890683122, 1.000000000000000000, 0.9659258262890683122, 1.000000000000000000, 0.9659258262890683122, 1.000000000000000000, 0.9659258262890683122, 1.000000000000000000, 0.9659258262890683122, 1.000000000000000000, 0.9659258262890683122, 1.000000000000000000, 0.9659258262890683122, 1.000000000000000000, 0.9659258262890683122, 1.000000000000000000, 0.9659258262890683122, 1.000000000000000000, 0.9659258262890683122, 1.000000000000000000, 0.9659258262890683122, 1.000000000000000000, 0.9659258262890683122, 1.000000000000000000, 0.9659258262890683122, 1.000000000000000000, 0.9659258262890683122, 1.000000000000000000, 0.9659258262890683122, 1.000000000000000000, 0.9659258262890683122, 1.000000000000000000, 0.9659258262890683122, 1.000000000000000000, 0.9659258262890683122, 1.000000000000000000, 0.9659258262890683122, 1.000000000000000000, 0.9659258262890683122, 1.000000000000000000, 0.9659258262890683122, 1.000000000000000000, 0.9659258262890683122, 1.000000000000000000, 0.9659258262890683122, 1.000000000000000000, 0.9659258262890683122, 1.000000000000000000, 0.9659258262890683122, 1.000000000000000000, 0.9659258262890683122, 1.000000000000000000, 0.9659258262890683122, 1.000000000000000000, 0.9659258262890683122, 1.000000000000000000, 0.9659258262890683122, 1.000000000000000000, 0.9659258262890683122, 1.000000000000000000, 0.9659258262890683122, 1.000000000000000000, 0.9659258262890683122, 1.000000000000000000, 0.9659258262890683122, 1.000000000000000000, 0.9659258262890683122, 1.000000000000000000, 0.9659258262890683122, 1.000000000000000000, 0.9659258262890683122, 1.000000000000000000, 0.9659258262890683122, 1.000000000000000000, 0.9659258262890683122, 1.000000000000000000, 0.9659258262890683122, 1.000000000000000000, 0.9659258262890683122, 1.000000000000000000, 0.9659258262890683122, 1.000000000000000000, 0.9659258262890683122, 1.000000000000000000, 0.9659258262890683122, 1.000000000000000000, 0.9659258262890683122, 1.000000000000000000, 0.9659258262890683122, 1.000000000000000000, 0.9659258262890683122, 1.000000000000000000, 0.9659258262890683122, 1.000000000000000000, 0.9659258262890683122, 1.000000000000000000, 0.9659258262890683122, 1.000000000000000000, 0.9659258262890683122, 1.000000000000000000, 0.9659258262890683122, 1.000000000000000000, 0.9659258262890683122, 1.000000000000000000, 0.9659258262890683122, 1.000000000000000000, 0.9659258262890683122, 1.000000000000000000, 0.9659258262890683122, 1.000000000000000000, 0.9659258262890683122, 1.000000000000000000, 0.9659258262890683122, 1.000000000000000000, 0.9659258262890683122, 1.000000000000000000, 0.9659258262890683122, 1.000000000000000000, 0.9659258262890683122, 1.000000000000000000, 0.9659258262890683122, 1.000000000000000000, 0.9659258262890683122, 1.000000000000000000, 0.9659258262890683122, 1.000000000000000000, 0.9659258262890683122, 1.000000000000000000, 0.9659258262890683122, 1.000000000000000000, 0.9659258262890683122, 1.000000000000000000, 0.9659258262890683122, 1.000000000000000000, 0.9659258262890683122, 1.000000000000000000, 0.9659258262890683122, 1.000000000000000000, 0.9659258262890683122, 1.000000000000000000, 0.9659258262890683122, 1.000000000000000000, 0.9659258262890683122, 1.000000000000000000, 0.9659258262890683122, 1.000000000000000000, 0.9659258262890683122, 1.000000000000000000, 0.9659258262890683122, 1.000000000000000000, 0.9659258262890683122, 1.000000000000000000, 0.9659258262890683122, 1.000000000000000000, 0.9659258262890683122, 1.000000000000000000, 0.9659258262890683122, 1.000000000000000000, 0.9659258262890683122, 1.000000000000000000, 0.9659258262890683122, 1.000000000000000000, 0.9659258262890683122, 1.000000000000000000, 0.9659258262890683122, 1.000000000000000000, 0.9659258262890683122, 1.000000000000000000, 0.9659258262890683122, 1.000000000000000000, 0.9659258262890683122, 1.000000000000000000, 0.9659258262890683122, 1.000000000000000000, 0.9659258262890683122, 1.000000000000000000, 0.9659258262890683122, 1.000000000000000000, 0.9659258262890683122, 1.000000000000000000, 0.9659258262890683122, 1.000000000000000000, 0.9659258262890683122, 1.000000000000000000, 0.9659258262890683122, 1.000000000000000000, 0.9659258262890683122, 1.000000000000000000, 0.9659258262890683122, 1.000000000000000000, 0.9659258262890683122, 1.000000000000000000, 0.9659258262890683122, 1.000000000000000000, 0.9659258262890683122, 1.000000000000000000, 0.9659258262890683122, 1.000000000000000000, 0.9659258262890683122, 1.000000000000000000, 0.9659258262890683122, 1.000000000000000000, 0.9659258262890683122, 1.000000000000000000, 0.9659258262890683122, 1.000000000000000000, 0.9659258262890683122, 1.000000000000000000, 0.9659258262890683122, 1.000000000000000000, 0.9659258262890683122, 1.000000000000000000, 0.9659258262890683122, 1.000000000000000000, 0.9659258262890683122, 1.000000000000000000, 0.9659258262890683122, 1.000000000000000000, 0.9659258262890683122, 1.000000000000000000, 0.9659258262890683122, 1.000000000000000000, 0.9659258262890683122, 1.000000000000000000, 0.9659258262890683122, 1.000000000000000000, 0.9659258262890683122, 1.000000000000000000, 0.9659258262890683122, 1.000000000000000000, 0.9659258262890683122, 1.000000000000000000, 0.9659258262890683122, 1.000000000000000000, 0.9659258262890683122, 1.000000000000000000, 0.9659258262890683122, 1.000000000000000000, 0.9659258262890683122, 1.000000000000000000, 0.9659258262890683122, 1.000000000000000000, 0.9659258262890683122, 1.000000000000000000, 0.9659258262890683122, 1.000000000000000000, 0.9659258262890683122, 1.000000000000000000, 0.9659258262890683122, 1.000000000000000000, 0.9659258262890683122, 1.000000000000000000, 0.9659258262890683122, 1.000000000000000000, 0.9659258262890683122, 1.000000000000000000, 0.9659258262890683122, 1.000000000000000000, 0.9659258262890683122, 1.000000000000000000, 0.9659258262890683122, 1.000000000000000000, 0.9659258262890683122, 1.000000000000000000, 0.9659258262890683122, 1.000000000000000000, 0.9659258262890683122, 1.000000000000000000, 0.9659258262890683122, 1.000000000000000000, 0.9659258262890683122, 1.000000000000000000, 0.9659258262890683122, 1.000000000000000000, 0.9659258262890683122, 1.000000000000000000, 0.9659258262890683122, 1.000000000000000000, 0.9659258262890683122, 1.000000000000000000, 0.9659258262890683122, 1.000000000000000000, 0.9659258262890683122, 1.000000000000000000, 0.9659258262890683122, 1.000000000000000000, 0.9659258262890683122, 1.000000000000000000, 0.9659258262890683122, 1.000000000000000000, 0.9659258262890683122, 1.000000000000000000, 0.9659258262890683122, 1.000000000000000000, 0.9659258262890683122, 1.000000000000000000, 0.9659258262890683122, 1.000000000000000000, 0.9659258262890683122, 1.000000000000000000, 0.9659258262890683122, 1.000000000000000000, 0.9659258262890683122, 1.000000000000000000, 0.9659258262890683122, 1.000000000000000000, 0.9659258262890683122, 1.000000000000000000, 0.9659258262890683122, 1.000000000000000000, 0.9659258262890683122, 1.000000000000000000, 0.9659258262890683122, 1.000000000000000000),
 ( 1.000000000000000000, 0.9659258262890683122, 1.000000000000000000, 0.9659258262890683122, 1.000000000000000000, 0.9659258262890683122, 1.000000000000000000, 0.9659258262890683122, 1.000000000000000000, 0.9659258262890683122, 1.000000000000000000, 0.9659258262890683122, 1.000000000000000000, 0.9659258262890683122, 1.000000000000000000, 0.9659258262890683122, 1.000000000000000000, 0.9659258262890683122, 1.000000000000000000, 0.9659258262890683122, 1.000000000000000000, 0.9659258262890683122, 1.000000000000000000, 0.9659258262890683122, 1.000000000000000000, 0.9659258262890683122, 1.000000000000000000, 0.9659258262890683122, 1.000000000000000000, 0.9659258262890683122, 1.000000000000000000, 0.9659258262890683122, 1.000000000000000000, 0.9659258262890683122, 1.000000000000000000, 0.9659258262890683122, 1.000000000000000000, 0.9659258262890683122, 1.000000000000000000, 0.9659258262890683122, 1.000000000000000000, 0.9659258262890683122, 1.000000000000000000, 0.9659258262890683122, 1.000000000000000000, 0.9659258262890683122, 1.000000000000000000, 0.9659258262890683122, 1.000000000000000000, 0.9659258262890683122, 1.000000000000000000, 0.9659258262890683122, 1.000000000000000000, 0.9659258262890683122, 1.000000000000000000, 0.9659258262890683122, 1.000000000000000000, 0.9659258262890683122, 1.000000000000000000, 0.9659258262890683122, 1.000000000000000000, 0.9659258262890683122, 1.000000000000000000, 0.9659258262890683122, 1.000000000000000000, 0.9659258262890683122, 1.000000000000000000, 0.9659258262890683122, 1.000000000000000000, 0.9659258262890683122, 1.000000000000000000, 0.9659258262890683122, 1.000000000000000000, 0.9659258262890683122, 1.000000000000000000, 0.9659258262890683122, 1.000000000000000000, 0.9659258262890683122, 1.000000000000000000, 0.9659258262890683122, 1.000000000000000000, 0.9659258262890683122, 1.000000000000000000, 0.9659258262890683122, 1.000000000000000000, 0.9659258262890683122, 1.000000000000000000, 0.9659258262890683122, 1.000000000000000000, 0.9659258262890683122, 1.000000000000000000, 0.9659258262890683122, 1.000000000000000000, 0.9659258262890683122, 1.000000000000000000, 0.9659258262890683122, 1.000000000000000000, 0.9659258262890683122, 1.000000000000000000, 0.9659258262890683122, 1.000000000000000000, 0.9659258262890683122, 1.000000000000000000, 0.9659258262890683122, 1.000000000000000000, 0.9659258262890683122, 1.000000000000000000, 0.9659258262890683122, 1.000000000000000000, 0.9659258262890683122, 1.000000000000000000, 0.9659258262890683122, 1.000000000000000000, 0.9659258262890683122, 1.000000000000000000, 0.9659258262890683122, 1.000000000000000000, 0.9659258262890683122, 1.000000000000000000, 0.9659258262890683122, 1.000000000000000000, 0.9659258262890683122, 1.000000000000000000, 0.9659258262890683122, 1.000000000000000000, 0.9659258262890683122, 1.000000000000000000, 0.9659258262890683122, 1.000000000000000000, 0.9659258262890683122, 1.000000000000000000, 0.9659258262890683122, 1.000000000000000000, 0.9659258262890683122, 1.000000000000000000, 0.9659258262890683122, 1.000000000000000000, 0.9659258262890683122, 1.000000000000000000, 0.9659258262890683122, 1.000000000000000000, 0.9659258262890683122, 1.000000000000000000, 0.9659258262890683122, 1.000000000000000000, 0.9659258262890683122, 1.000000000000000000, 0.9659258262890683122, 1.000000000000000000, 0.9659258262890683122, 1.000000000000000000, 0.9659258262890683122, 1.000000000000000000, 0.9659258262890683122, 1.000000000000000000, 0.9659258262890683122, 1.000000000000000000, 0.9659258262890683122, 1.000000000000000000, 0.9659258262890683122, 1.000000000000000000, 0.9659258262890683122, 1.000000000000000000, 0.9659258262890683122, 1.000000000000000000, 0.9659258262890683122, 1.000000000000000000, 0.9659258262890683122, 1.000000000000000000, 0.9659258262890683122, 1.000000000000000000, 0.9659258262890683122, 1.000000000000000000, 0.9659258262890683122, 1.000000000000000000, 0.9659258262890683122, 1.000000000000000000, 0.9659258262890683122, 1.000000000000000000, 0.9659258262890683122, 1.000000000000000000, 0.9659258262890683122, 1.000000000000000000, 0.9659258262890683122, 1.000000000000000000, 0.9659258262890683122, 1.000000000000000000, 0.9659258262890683122, 1.000000000000000000, 0.9659258262890683122, 1.000000000000000000, 0.9659258262890683122, 1.000000000000000000, 0.9659258262890683122, 1.000000000000000000, 0.9659258262890683122, 1.000000000000000000, 0.9659258262890683122, 1.000000000000000000, 0.9659258262890683122, 1.000000000000000000, 0.9659258262890683122, 1.000000000000000000, 0.9659258262890683122, 1.000000000000000000, 0.9659258262890683122, 1.000000000000000000, 0.9659258262890683122, 1.000000000000000000, 0.9659258262890683122, 1.000000000000000000, 0.9659258262890683122, 1.000000000000000000, 0.9659258262890683122, 1.000000000000000000, 0.9659258262890683122, 1.000000000000000000, 0.9659258262890683122, 1.000000000000000000, 0.9659258262890683122, 1.000000000000000000, 0.9659258262890683122, 1.000000000000000000, 0.9659258262890683122, 1.000000000000000000, 0.9659258262890683122, 1.000000000000000000, 0.9659258262890683122, 1.000000000000000000, 0.9659258262890683122, 1.000000000000000000, 0.9659258262890683122, 1.000000000000000000, 0.9659258262890683122, 1.000000000000000000, 0.9659258262890683122, 1.000000000000000000, 0.9659258262890683122, 1.000000000000000000, 0.9659258262890683122, 1.000000000000000000, 0.9659258262890683122, 1.000000000000000000, 0.9659258262890683122, 1.000000000000000000, 0.9659258262890683122, 1.000000000000000000, 0.9659258262890683122, 1.000000000000000000, 0.9659258262890683122, 1.000000000000000000, 0.9659258262890683122, 1.000000000000000000, 0.9659258262890683122, 1.000000000000000000, 0.9659258262890683122, 1.000000000000000000, 0.9659258262890683122, 1.000000000000000000, 0.9659258262890683122, 1.000000000000000000, 0.9659258262890683122, 1.000000000000000000, 0.9659258262890683122, 1.000000000000000000, 0.9659258262890683122, 1.000000000000000000, 0.9659258262890683122, 1.000000000000000000, 0.9659258262890683122, 1.000000000000000000, 0.9659258262890683122, 1.000000000000000000, 0.9659258262890683122, 1.000000000000000000, 0.9659258262890683122, 1.000000000000000000, 0.9659258262890683122, 1.000000000000000000, 0.9659258262890683122, 1.000000000000000000, 0.9659258262890683122, 1.000000000000000000, 0.9659258262890683122, 1.000000000000000000, 0.9659258262890683122, 1.000000000000000000, 0.9659258262890683122, 1.000000000000000000, 0.9659258262890683122, 1.000000000000000000, 0.9659258262890683122, 1.000000000000000000, 0.9659258262890683122, 1.000000000000000000, 0.9659258262890683122, 1.000000000000000000, 0.9659258262890683122, 1.000000000000000000, 0.9659258262890683122, 1.000000000000000000, 0.9659258262890683122, 1.000000000000000000, 0.9659258262890683122, 1.000000000000000000, 0.9659258262890683122, 1.000000000000000000, 0.9659258262890683122, 1.000000000000000000, 0.9659258262890683122, 1.000000000000000000, 0.9659258262890683122, 1.000000000000000000, 0.9659258262890683122, 1.000000000000000000, 0.9659258262890683122, 1.000000000000000000, 0.9659258262890683122, 1.000000000000000000, 0.9659258262890683122, 1.000000000000000000, 0.9659258262890683122, 1.000000000000000000, 0.9659258262890683122, 1.000000000000000000, 0.9659258262890683122, 1.000000000000000000, 0.9659258262890683122, 1.000000000000000000, 0.9659258262890683122, 1.000000000000000000, 0.9659258262890683122, 1.000000000000000000, 0.9659258262890683122, 1.000000000000000000, 0.9659258262890683122, 1.000000000000000000, 0.9659258262890683122, 1.000000000000000000, 0.9659258262890683122, 1.000000000000000000, 0.9659258262890683122, 1.000000000000000000, 0.9659258262890683122, 1.000000000000000000, 0.9659258262890683122, 1.000000000000000000, 0.9659258262890683122, 1.000000000000000000, 0.9659258262890683122, 1.000000000000000000, 0.9659258262890683122, 1.000000000000000000, 0.9659258262890683122, 1.000000000000000000, 0.9659258262890683122, 1.000000000000000000, 0.9659258262890683122, 1.000000000000000000, 0.9659258262890683122, 1.000000000000000000, 0.9659258262890683122, 1.000000000000000000, 0.9659258262890683122, 1.000000000000000000, 0.9659258262890683122, 1.000000000000000000, 0.9659258262890683122, 1.000000000000000000, 0.9659258262890683122, 1.000000000000000000, 0.9659258262890683122, 1.000000000000000000, 0.9659258262890683122, 1.000000000000000000, 0.9659258262890683122, 1.000000000000000000, 0.9659258262890683122, 1.000000000000000000, 0.9659258262890683122, 1.000000000000000000, 0.9659258262890683122, 1.000000000000000000, 0.9659258262890683122, 1.000000000000000000, 0.9659258262890683122, 1.000000000000000000, 0.9659258262890683122, 1.000000000000000000, 0.9659258262890683122, 1.000000000000000000, 0.9659258262890683122, 1.000000000000000000, 0.9659258262890683122, 1.000000000000000000, 0.9659258262890683122, 1.000000000000000000, 0.9659258262890683122, 1.000000000000000000, 0.9659258262890683122, 1.000000000000000000, 0.9659258262890683122, 1.000000000000000000, 0.9659258262890683122, 1.000000000000000000, 0.9659258262890683122, 1.000000000000000000, 0.9659258262890683122, 1.000000000000000000, 0.9659258262890683122, 1.000000000000000000, 0.9659258262890683122, 1.000000000000000000, 0.9659258262890683122, 1.000000000000000000, 0.9659258262890683122, 1.000000000000000000, 0.9659258262890683122, 1.000000000000000000, 0.9659258262890683122, 1.000000000000000000, 0.9659258262890683122, 1.000000000000000000, 0.9659258262890683122, 1.000000000000000000, 0.9659258262890683122, 1.000000000000000000, 0.9659258262890683122, 1.000000000000000000, 0.9659258262890683122, 1.000000000000000000, 0.9659258262890683122, 1.000000000000000000, 0.9659258262890683122, 1.000000000000000000, 0.9659258262890683122, 1.000000000000000000, 0.9659258262890683122, 1.000000000000000000, 0.9659258262890683122, 1.000000000000000000, 0.9659258262890683122, 1.000000000000000000, 0.9659258262890683122, 1.000000000000000000, 0.9659258262890683122, 1.000000000000000000, 0.9659258262890683122, 1.000000000000000000, 0.9659258262890683122, 1.000000000000000000, 0.9659258262890683122, 1.000000000000000000, 0.9659258262890683122, 1.000000000000000000, 0.9659258262890683122, 1.000000000000000000, 0.9659258262890683122, 1.000000000000000000, 0.9659258262890683122, 1.000000000000000000, 0.9659258262890683122, 1.000000000000000000, 0.9659258262890683122, 1.000000000000000000, 0.9659258262890683122, 1.000000000000000000, 0.9659258262890683122, 1.000000000000000000, 0.9659258262890683122, 1.000000000000000000, 0.9659258262890683122, 1.000000000000000000, 0.9659258262890683122, 1.000000000000000000, 0.9659258262890683122, 1.000000000000000000, 0.9659258262890683122, 1.000000000000000000, 0.9659258262890683122, 1.000000000000000000, 0.9659258262890683122, 1.000000000000000000, 0.9659258262890683122, 1.000000000000000000, 0.9659258262890683122, 1.000000000000000000, 0.9659258262890683122, 1.000000000000000000, 0.9659258262890683122, 1.000000000000000000, 0.9659258262890683122, 1.000000000000000000, 0.9659258262890683122, 1.000000000000000000, 0.9659258262890683122, 1.000000000000000000, 0.9659258262890683122, 1.000000000000000000, 0.9659258262890683122, 1.000000000000000000, 0.9659258262890683122, 1.000000000000000000, 0.9659258262890683122, 1.000000000000000000, 0.9659258262890683122, 1.000000000000000000, 0.9659258262890683122, 1.000000000000000000, 0.9659258262890683122, 1.000000000000000000) ) ) 
 REPRESENTATION_ITEM ( '' )  SURFACE ( )  );
#14530=CARTESIAN_POINT ( 'NONE',  ( -1.469816272965878357, 0.2306618581243848609, 0.2411417322834645549 ) ) ;
#14531=CARTESIAN_POINT ( 'NONE',  ( 0.3937007874015754361, -0.1870078740157479769, 0.4822834645669291653 ) ) ;
#14533=ORIENTED_EDGE ( 'NONE', *, *, #23671, .F. ) ;
#14534=CARTESIAN_POINT ( 'NONE',  ( -1.614173228346457378, 0.5038684218300931716, 0.1372047244094476981 ) ) ;
#14535=DIRECTION ( 'NONE',  ( 0.000000000000000000, 0.000000000000000000, 1.000000000000000000 ) ) ;
#14536=CARTESIAN_POINT ( 'NONE',  ( 0.6627296587926517768, -0.6692913385826773087, -0.1292274648535924053 ) ) ;
#14537=CARTESIAN_POINT ( 'NONE',  ( -1.502624671916009680, -0.05778040916215560624, -0.4822834645669293319 ) ) ;
#14539=CARTESIAN_POINT ( 'NONE',  ( -0.9120734908136475250, 0.1771653543307087630, 0.09757992244046791164 ) ) ;
#14540=CARTESIAN_POINT ( 'NONE',  ( 1.620734908136483465, -0.6692913385826771977, 0.1292274648535927661 ) ) ;
#14542=CARTESIAN_POINT ( 'NONE',  ( 0.3871391076115492380, -0.05778040916215560624, -0.4822834645669293319 ) ) ;
#14543=CARTESIAN_POINT ( 'NONE',  ( -0.8333333333333323711, 0.1771653543307087630, 0.09757992244046791164 ) ) ;
#14544=CARTESIAN_POINT ( 'NONE',  ( -0.3215223097112853146, -0.2845877964562159024, 0.3641732283464567677 ) ) ;
#14545=CARTESIAN_POINT ( 'NONE',  ( -0.1640419947506555343, -0.3162353388693405765, 0.4822834645669290543 ) ) ;
#14546=CARTESIAN_POINT ( 'NONE',  ( -1.259842519685038686, -0.1870078740157480601, -0.3641732283464567677 ) ) ;
#14548=CARTESIAN_POINT ( 'NONE',  ( 0.9251968503937015864, -0.5400638737290844871, 0.3530559997133364547 ) ) ;
#14552=CARTESIAN_POINT ( 'NONE',  ( -0.6627296587926503335, -0.6692913385826771977, 0.1292274648535927661 ) ) ;
#14553=CARTESIAN_POINT ( 'NONE',  ( -0.006561679790025524116, -0.2845877964562159024, 0.3641732283464567677 ) ) ;
#14554=CARTESIAN_POINT ( 'NONE',  ( -1.318897637795274802, 0.1660481256975885056, 0.3530559997133364547 ) ) ;
#14555=CARTESIAN_POINT ( 'NONE',  ( 0.6955380577427828781, -0.3690944881889763329, 0.3153832671262228327 ) ) ;
#14556=CARTESIAN_POINT ( 'NONE',  ( -0.6299212598425188991, -0.1870078740157479769, 0.3641732283464567677 ) ) ;
#14557=CARTESIAN_POINT ( 'NONE',  ( -0.8595800524934373854, -0.3162353388693409650, -0.4822834645669289433 ) ) ;
#14558=CARTESIAN_POINT ( 'NONE',  ( -1.200787401574802349, 0.1660481256975883668, -0.3530559997133364547 ) ) ;
#14559=CARTESIAN_POINT ( 'NONE',  ( 1.620734908136483465, -0.6692913385826771977, 0.1292274648535927661 ) ) ;
#14561=CARTESIAN_POINT ( 'NONE',  ( 1.043307086614173818, 0.07958543189024085140, 0.2665933059059887866 ) ) ;
#14562=CARTESIAN_POINT ( 'NONE',  ( 0.3608923884514443348, -0.6692913385826771977, 0.1292274648535927661 ) ) ;
#14564=CARTESIAN_POINT ( 'NONE',  ( -1.351706036745406347, 0.05413385826771626580, -0.4176697321401330321 ) ) ;
#14567=CARTESIAN_POINT ( 'NONE',  ( -1.312335958005248715, 0.1283753931104748280, 0.1820866141732283561 ) ) ;
#14568=CARTESIAN_POINT ( 'NONE',  ( -0.6692913385826764205, 0.2952755905511811885, 0.000000000000000000 ) ) ;
#14569=CARTESIAN_POINT ( 'NONE',  ( 0.7480314960629927956, -0.6692913385826771977, 8.415575281601705876E-17 ) ) ;
#14570=CARTESIAN_POINT ( 'NONE',  ( -1.437007874015747477, -0.4536011799217367080, 0.2665933059059888421 ) ) ;
#14572=CARTESIAN_POINT ( 'NONE',  ( -1.607611548556429737, -0.6692913385826771977, 0.1292274648535927661 ) ) ;
#14573=CARTESIAN_POINT ( 'NONE',  ( 0.6496062992125991586, -0.5400638737290845981, -0.3530559997133363437 ) ) ;
#14574=CARTESIAN_POINT ( 'NONE',  ( 0.5774278215223104249, 0.2306618581243848609, 0.2411417322834645549 ) ) ;
#14575=CARTESIAN_POINT ( 'NONE',  ( 1.102362204724410155, -0.1870078740157479769, 0.4822834645669291653 ) ) ;
#14579=CARTESIAN_POINT ( 'NONE',  ( 0.1902887139107617975, 0.1771653543307087630, 0.09757992244046791164 ) ) ;
#14580=CARTESIAN_POINT ( 'NONE',  ( -0.3608923884514428360, -0.6692913385826773087, -0.1292274648535924053 ) ) ;
#14581=CARTESIAN_POINT ( 'NONE',  ( 1.377952755905512472, -0.6692913385826771977, 8.415575281601705876E-17 ) ) ;
#14583=CARTESIAN_POINT ( 'NONE',  ( 0.4330708661417329575, 0.1771653543307087630, 0.000000000000000000 ) ) ;
#14584=CARTESIAN_POINT ( 'NONE',  ( -0.6167979002624665030, -0.4281496062992127816, -0.4176697321401328100 ) ) ;
#14585=CARTESIAN_POINT ( 'NONE',  ( 1.476377952755906220, 0.1660481256975883668, -0.3530559997133364547 ) ) ;
#14586=CARTESIAN_POINT ( 'NONE',  ( 0.4265091863517067594, 0.2952755905511811885, 0.1292274648535926551 ) ) ;
#14590=ORIENTED_EDGE ( 'NONE', *, *, #54812, .T. ) ;
#14591=CARTESIAN_POINT ( 'NONE',  ( 1.456692913385827515, 0.1771653543307087630, 0.000000000000000000 ) ) ;
#14592=CARTESIAN_POINT ( 'NONE',  ( -1.213910761154854745, -0.5511811023622046335, 0.09757992244046803654 ) ) ;
#14593=CARTESIAN_POINT ( 'NONE',  ( -0.9842519685039360366, 0.2952755905511811885, 0.000000000000000000 ) ) ;
#14596=CARTESIAN_POINT ( 'NONE',  ( -1.653543307086613234, -0.1870078740157479769, 0.3641732283464567677 ) ) ;
#14597=CARTESIAN_POINT ( 'NONE',  ( -1.358267716535432434, 0.1660481256975883668, -0.3530559997133364547 ) ) ;
#14598=CARTESIAN_POINT ( 'NONE',  ( -0.07874015748031421014, -0.1870078740157480879, -0.4822834645669291653 ) ) ;
#14599=CARTESIAN_POINT ( 'NONE',  ( -1.371391076115484609, -0.6692913385826771977, 0.1292274648535927661 ) ) ;
#14601=CARTESIAN_POINT ( 'NONE',  ( 0.7414698162729663755, -0.6692913385826773087, -0.1292274648535924053 ) ) ;
#14603=CARTESIAN_POINT ( 'NONE',  ( -1.220472440944881054, -0.5511811023622047445, 6.969142054262312111E-17 ) ) ;
#14608=CARTESIAN_POINT ( 'NONE',  ( -1.338582677165353729, -0.1870078740157480879, -0.4822834645669291653 ) ) ;
#14609=CARTESIAN_POINT ( 'NONE',  ( -1.437007874015747477, 0.1660481256975883668, -0.3530559997133364547 ) ) ;
#14611=CARTESIAN_POINT ( 'NONE',  ( -1.646981627296586703, -0.3162353388693409650, -0.4822834645669289433 ) ) ;
#14612=CARTESIAN_POINT ( 'NONE',  ( -1.732283464566928277, -0.1870078740157479769, 0.4822834645669291653 ) ) ;
#14613=CARTESIAN_POINT ( 'NONE',  ( -1.482939632545930975, 0.05413385826771666132, 0.4176697321401328100 ) ) ;
#14614=CARTESIAN_POINT ( 'NONE',  ( -0.6199123404867337150, -2.191421614605370878E-15, 0.4445507791589071167 ) ) ;
#14616=CARTESIAN_POINT ( 'NONE',  ( 0.04593175853018440641, -0.5511811023622046335, 0.09757992244046803654 ) ) ;
#14618=CARTESIAN_POINT ( 'NONE',  ( -0.5971128608923877978, 0.1771653543307087630, 0.09757992244046791164 ) ) ;
#14619=CARTESIAN_POINT ( 'NONE',  ( -1.010498687664041384, 0.05413385826771666132, 0.4176697321401328100 ) ) ;
#14620=CARTESIAN_POINT ( 'NONE',  ( 0.7349081364829402885, -0.6046776061558809534, -0.2411417322834644161 ) ) ;
#14621=CARTESIAN_POINT ( 'NONE',  ( -0.8923884514435688198, -0.6046776061558807314, 0.2411417322834647770 ) ) ;
#14624=CARTESIAN_POINT ( 'NONE',  ( -0.8661417322834640276, -0.1870078740157479769, 0.4822834645669291653 ) ) ;
#14625=CARTESIAN_POINT ( 'NONE',  ( 1.003937007874016185, 0.1660481256975883668, -0.3530559997133364547 ) ) ;
#14626=CARTESIAN_POINT ( 'NONE',  ( -1.646981627296586703, -0.2845877964562161244, -0.3641732283464567121 ) ) ;
#14627=CARTESIAN_POINT ( 'NONE',  ( -1.692913385826770645, 0.2952755905511811885, 0.000000000000000000 ) ) ;
#14632=CARTESIAN_POINT ( 'NONE',  ( -0.2952755905511803003, -0.5400638737290845981, -0.3530559997133363437 ) ) ;
#14633=CARTESIAN_POINT ( 'NONE',  ( -1.423884514435694859, -0.08942795157528024563, -0.3641732283464568787 ) ) ;
#14635=CARTESIAN_POINT ( 'NONE',  ( -1.141732283464566011, -0.6692913385826771977, 8.415575281601705876E-17 ) ) ;
#14636=CARTESIAN_POINT ( 'NONE',  ( -0.6758530183727027296, 0.2066929133858267931, 0.1054918080437490802 ) ) ;
#14637=CARTESIAN_POINT ( 'NONE',  ( -1.509186351706035767, 0.05413385826771626580, -0.4176697321401330321 ) ) ;
#14638=CARTESIAN_POINT ( 'NONE',  ( -0.5511811023622041894, -0.1870078740157480879, -0.4822834645669291653 ) ) ;
#14640=CARTESIAN_POINT ( 'NONE',  ( 0.4593175853018379162, -0.3690944881889763329, 0.3153832671262228327 ) ) ;
#14642=CARTESIAN_POINT ( 'NONE',  ( 0.3083989501312343062, -0.08942795157528024563, -0.3641732283464568787 ) ) ;
#14643=CARTESIAN_POINT ( 'NONE',  ( 1.450131233595801428, 0.1771653543307087630, 0.09757992244046791164 ) ) ;
#14644=CARTESIAN_POINT ( 'NONE',  ( 1.069553805774278610, -0.6692913385826771977, 0.1292274648535927661 ) ) ;
#14645=CARTESIAN_POINT ( 'NONE',  ( -0.02624671916010428221, 0.1283753931104746893, -0.1820866141732285504 ) ) ;
#14647=CARTESIAN_POINT ( 'NONE',  ( -1.108923884514435132, -0.05778040916215560624, -0.4822834645669293319 ) ) ;
#14648=CARTESIAN_POINT ( 'NONE',  ( -0.09842519685039295696, 0.07958543189024071263, -0.2665933059059888421 ) ) ;
#14649=CARTESIAN_POINT ( 'NONE',  ( -1.482939632545930975, -0.004921259842519576551, 0.3153832671262227771 ) ) ;
#14651=CARTESIAN_POINT ( 'NONE',  ( -0.6167979002624665030, -0.3690944881889765550, -0.3153832671262227771 ) ) ;
#14652=EDGE_CURVE ( 'NONE', #72992, #38903, #26195, .T. ) ;
#14654=CARTESIAN_POINT ( 'NONE',  ( -0.1312335958005241554, -0.6046776061558809534, -0.2411417322834644161 ) ) ;
#14655=LINE ( 'NONE', #33995, #55897 ) ;
#14656=CARTESIAN_POINT ( 'NONE',  ( 0.4133858267716541968, -0.4536011799217368745, -0.2665933059059886201 ) ) ;
#14657=CARTESIAN_POINT ( 'NONE',  ( -0.2690288713910754526, 0.1771653543307087075, -0.09757992244046823083 ) ) ;
#14658=CARTESIAN_POINT ( 'NONE',  ( -0.3018372703412066094, -0.4281496062992127816, -0.4176697321401328100 ) ) ;
#14659=CARTESIAN_POINT ( 'NONE',  ( -1.732283464566928277, -0.1870078740157479769, 0.4822834645669291653 ) ) ;
#14660=CARTESIAN_POINT ( 'NONE',  ( -0.9645669291338575535, 0.07958543189024071263, -0.2665933059059888421 ) ) ;
#14662=CARTESIAN_POINT ( 'NONE',  ( 0.6561679790026253567, -0.6046776061558809534, -0.2411417322834644161 ) ) ;
#14663=CARTESIAN_POINT ( 'NONE',  ( -0.8727034120734901146, -0.3162353388693405765, 0.4822834645669290543 ) ) ;
#14666=CARTESIAN_POINT ( 'NONE',  ( -0.3608923884514428360, -0.5511811023622048555, -0.09757992244046775898 ) ) ;
#14667=DIRECTION ( 'NONE',  ( -2.956072690630991733E-16, 1.000000000000000000, 5.002896285981958034E-32 ) ) ;
#14668=CARTESIAN_POINT ( 'NONE',  ( -1.049868766404198794, -0.5023911411419708095, 0.1820866141732285504 ) ) ;
#14669=CARTESIAN_POINT ( 'NONE',  ( 1.574803149606299746, -0.1870078740157480879, -0.4822834645669291653 ) ) ;
#14670=EDGE_CURVE ( 'NONE', #11874, #32456, #72529, .T. ) ;
#14671=CARTESIAN_POINT ( 'NONE',  ( -0.8464566929133852113, 0.07958543189024085140, 0.2665933059059887866 ) ) ;
#14673=CARTESIAN_POINT ( 'NONE',  ( 0.9514435695538062676, -0.05778040916215522460, 0.4822834645669289988 ) ) ;
#14678=CARTESIAN_POINT ( 'NONE',  ( 1.574803149606299746, -0.1870078740157479769, 0.3641732283464567677 ) ) ;
#14679=CARTESIAN_POINT ( 'NONE',  ( -1.377952755905511140, 0.2952755905511811885, 0.000000000000000000 ) ) ;
#14680=CARTESIAN_POINT ( 'NONE',  ( 1.305774278215223960, 0.2952755905511810774, -0.1292274648535930714 ) ) ;
#14683=CARTESIAN_POINT ( 'NONE',  ( 0.3215223097112867578, -0.3162353388693409650, -0.4822834645669289433 ) ) ;
#14684=CARTESIAN_POINT ( 'NONE',  ( -0.5839895013123351797, -0.6692913385826771977, 0.1292274648535927661 ) ) ;
#14685=CARTESIAN_POINT ( 'NONE',  ( 1.535433070866142558, 0.2952755905511811885, 0.000000000000000000 ) ) ;
#14687=CARTESIAN_POINT ( 'NONE',  ( 0.5774278215223103139, -0.5023911411419708095, -0.1820866141732282451 ) ) ;
#14692=ORIENTED_EDGE ( 'NONE', *, *, #37239, .F. ) ;
#14693=CARTESIAN_POINT ( 'NONE',  ( -0.4527559055118102749, 0.1660481256975885056, 0.3530559997133364547 ) ) ;
#14694=CARTESIAN_POINT ( 'NONE',  ( 1.371391076115485719, -0.6692913385826773087, -0.1292274648535924053 ) ) ;
#14695=CARTESIAN_POINT ( 'NONE',  ( 0.3346456692913393205, -0.5400638737290845981, -0.3530559997133363437 ) ) ;
#14696=CARTESIAN_POINT ( 'NONE',  ( -0.3871391076115476282, -0.08942795157527998196, 0.3641732283464567121 ) ) ;
#14697=CARTESIAN_POINT ( 'NONE',  ( 1.410761154855643795, -0.05778040916215560624, -0.4822834645669293319 ) ) ;
#14698=CARTESIAN_POINT ( 'NONE',  ( -0.6299212598425188991, -0.1870078740157480879, -0.4822834645669291653 ) ) ;
#14699=CARTESIAN_POINT ( 'NONE',  ( 0.1312335958005255154, -0.6046776061558807314, 0.2411417322834647770 ) ) ;
#14700=CARTESIAN_POINT ( 'NONE',  ( -1.601049868766403650, 0.2306618581243847221, -0.2411417322834647770 ) ) ;
#14701=CARTESIAN_POINT ( 'NONE',  ( 0.7086614173228352742, -0.1870078740157480879, -0.4822834645669291653 ) ) ;
#14702=ADVANCED_FACE ( 'NONE', ( #23204 ), #9349, .F. ) ;
#14703=CARTESIAN_POINT ( 'NONE',  ( 1.036745406824147731, 0.05413385826771666132, 0.4176697321401328100 ) ) ;
#14705=CARTESIAN_POINT ( 'NONE',  ( 8.195543980992789655E-16, -0.1870078740157480601, -0.3641732283464567677 ) ) ;
#14708=ORIENTED_EDGE ( 'NONE', *, *, #20551, .F. ) ;
#14709=CARTESIAN_POINT ( 'NONE',  ( -0.4002624671916004129, -0.08942795157528024563, -0.3641732283464568787 ) ) ;
#14710=CARTESIAN_POINT ( 'NONE',  ( 0.1115485564304470323, 0.2952755905511811885, 0.1292274648535926551 ) ) ;
#14712=CARTESIAN_POINT ( 'NONE',  ( -0.2690288713910754526, 0.2952755905511810774, -0.1292274648535930714 ) ) ;
#14713=CARTESIAN_POINT ( 'NONE',  ( -0.3018372703412066094, 0.05413385826771666132, 0.4176697321401328100 ) ) ;
#14714=CARTESIAN_POINT ( 'NONE',  ( -0.9514435695538050464, -0.05778040916215560624, -0.4822834645669293319 ) ) ;
#14715=CARTESIAN_POINT ( 'NONE',  ( -0.8727034120734901146, -0.05778040916215560624, -0.4822834645669293319 ) ) ;
#14717=CARTESIAN_POINT ( 'NONE',  ( 1.318897637795276356, -0.4536011799217367080, 0.2665933059059888421 ) ) ;
#14718=CARTESIAN_POINT ( 'NONE',  ( -1.456692913385826182, 0.2952755905511811885, 0.000000000000000000 ) ) ;
#14720=CARTESIAN_POINT ( 'NONE',  ( 0.5446194225721792126, -0.08942795157528024563, -0.3641732283464568787 ) ) ;
#14721=CARTESIAN_POINT ( 'NONE',  ( 0.4461942257217856311, 0.2306618581243847221, -0.2411417322834647770 ) ) ;
#14722=CARTESIAN_POINT ( 'NONE',  ( 0.4199475065616805614, 0.2306618581243848609, 0.2411417322834645549 ) ) ;
#14724=CARTESIAN_POINT ( 'NONE',  ( -0.5611900217179893735, -2.567464376874931580E-15, -0.4445507791589072832 ) ) ;
#14727=CARTESIAN_POINT ( 'NONE',  ( -0.4002624671916004129, -0.05778040916215560624, -0.4822834645669293319 ) ) ;
#14731=CARTESIAN_POINT ( 'NONE',  ( -1.305774278215222184, 0.1771653543307087630, 0.09757992244046791164 ) ) ;
#14732=CARTESIAN_POINT ( 'NONE',  ( 0.8595800524934390507, -0.05778040916215560624, -0.4822834645669293319 ) ) ;
#14733=CARTESIAN_POINT ( 'NONE',  ( 0.8989501312335964611, 0.2952755905511811885, 0.1292274648535926551 ) ) ;
#14734=CARTESIAN_POINT ( 'NONE',  ( -0.07874015748031421014, -0.1870078740157479769, 0.3641732283464567677 ) ) ;
#14735=CARTESIAN_POINT ( 'NONE',  ( 0.4855643044619428750, 0.05413385826771666132, 0.4176697321401328100 ) ) ;
#14737=CARTESIAN_POINT ( 'NONE',  ( 0.05249343832021075018, -0.5023911411419708095, 0.1820866141732285504 ) ) ;
#14738=CARTESIAN_POINT ( 'NONE',  ( -0.1181102362204717315, 0.2952755905511811885, 0.000000000000000000 ) ) ;
#14740=CARTESIAN_POINT ( 'NONE',  ( -1.535433070866141225, 0.2952755905511811885, 0.000000000000000000 ) ) ;
#14741=CARTESIAN_POINT ( 'NONE',  ( 0.4265091863517067039, -0.5511811023622048555, -0.09757992244046775898 ) ) ;
#14743=CARTESIAN_POINT ( 'NONE',  ( -0.6561679790026240244, -0.6046776061558807314, 0.2411417322834647770 ) ) ;
#14744=CARTESIAN_POINT ( 'NONE',  ( -0.5314960629921250401, 0.07958543189024085140, 0.2665933059059887866 ) ) ;
#14745=CARTESIAN_POINT ( 'NONE',  ( 1.572991167713778227, 1.535433070866141447, -0.1227090857360983167 ) ) ;
#14746=CARTESIAN_POINT ( 'NONE',  ( -0.7808398950131225646, -0.05778040916215522460, 0.4822834645669289988 ) ) ;
#14747=CARTESIAN_POINT ( 'NONE',  ( -0.6627296587926501115, 0.2952755905511810774, -0.1292274648535930714 ) ) ;
#14748=CARTESIAN_POINT ( 'NONE',  ( 0.03280839895013198948, -0.6692913385826773087, -0.1292274648535924053 ) ) ;
#14752=CARTESIAN_POINT ( 'NONE',  ( 0.6955380577427828781, -0.3690944881889763329, 0.3153832671262228327 ) ) ;
#14753=CARTESIAN_POINT ( 'NONE',  ( 1.371391076115485719, -0.6692913385826773087, -0.1292274648535924053 ) ) ;
#14754=CARTESIAN_POINT ( 'NONE',  ( -1.115485564304461219, -0.3690944881889763329, 0.3153832671262228327 ) ) ;
#14755=CARTESIAN_POINT ( 'NONE',  ( -1.174540682414697335, -0.2845877964562161244, -0.3641732283464567121 ) ) ;
#14756=CARTESIAN_POINT ( 'NONE',  ( -0.5774278215223089816, 0.2306618581243847221, -0.2411417322834647770 ) ) ;
#14757=CARTESIAN_POINT ( 'NONE',  ( 0.006561679790026889343, -0.2845877964562161244, -0.3641732283464567121 ) ) ;
#14759=CARTESIAN_POINT ( 'NONE',  ( 0.9251968503937015864, -0.4536011799217367080, 0.2665933059059888421 ) ) ;
#14760=CARTESIAN_POINT ( 'NONE',  ( 0.4133858267716541968, 0.1660481256975885056, 0.3530559997133364547 ) ) ;
#14762=CARTESIAN_POINT ( 'NONE',  ( -0.6102362204724400829, 0.1660481256975885056, 0.3530559997133364547 ) ) ;
#14764=CARTESIAN_POINT ( 'NONE',  ( -1.719160104986876103, 0.05413385826771666132, 0.4176697321401328100 ) ) ;
#14765=CARTESIAN_POINT ( 'NONE',  ( 0.5249343832021005074, -0.6046776061558807314, 0.2411417322834647770 ) ) ;
#14766=CARTESIAN_POINT ( 'NONE',  ( -0.01312335958005186876, 0.05413385826771626580, -0.4176697321401330321 ) ) ;
#14767=CARTESIAN_POINT ( 'NONE',  ( -0.1246719160104980823, -0.5511811023622048555, -0.09757992244046775898 ) ) ;
#14768=CARTESIAN_POINT ( 'NONE',  ( 2.795275590551181466, 1.299212598425198095, -1.617488608965169241E-16 ) ) ;
#14769=CARTESIAN_POINT ( 'NONE',  ( -0.09842519685039295696, -0.4536011799217367080, 0.2665933059059888421 ) ) ;
#14770=CARTESIAN_POINT ( 'NONE',  ( 0.7480314960629927956, 0.2952755905511811885, 0.000000000000000000 ) ) ;
#14772=CARTESIAN_POINT ( 'NONE',  ( -0.6824146981627291497, -0.5023911411419708095, -0.1820866141732282451 ) ) ;
#14774=CARTESIAN_POINT ( 'NONE',  ( -1.148293963254592542, 0.2952755905511811885, 0.1292274648535926551 ) ) ;
#14775=CARTESIAN_POINT ( 'NONE',  ( 0.2034120734908141659, 0.2066929133858267098, -0.1054918080437494132 ) ) ;
#14777=CARTESIAN_POINT ( 'NONE',  ( -1.135170603674539924, 0.2952755905511810774, -0.1292274648535930714 ) ) ;
#14778=CARTESIAN_POINT ( 'NONE',  ( -1.161417322834644716, -0.4536011799217368745, -0.2665933059059886201 ) ) ;
#14779=CARTESIAN_POINT ( 'NONE',  ( 0.1509186351706042484, -0.3162353388693405765, 0.4822834645669290543 ) ) ;
#14781=CARTESIAN_POINT ( 'NONE',  ( -0.9383202099737524282, -0.3162353388693409650, -0.4822834645669289433 ) ) ;
#14782=CARTESIAN_POINT ( 'NONE',  ( -1.646051170424378096, 0.000000000000000000, 0.3464511005275205946 ) ) ;
#14783=CARTESIAN_POINT ( 'NONE',  ( 1.614173228346457378, -0.6692913385826771977, 8.415575281601705876E-17 ) ) ;
#14784=CARTESIAN_POINT ( 'NONE',  ( 0.9186351706036751663, -0.6046776061558807314, 0.2411417322834647770 ) ) ;
#14785=CARTESIAN_POINT ( 'NONE',  ( 0.7217847769028878924, 0.05413385826771666132, 0.4176697321401328100 ) ) ;
#14787=CARTESIAN_POINT ( 'NONE',  ( 1.594488188976378673, 0.1660481256975885056, 0.3530559997133364547 ) ) ;
#14788=CARTESIAN_POINT ( 'NONE',  ( -1.443569553805773564, -0.6046776061558807314, 0.2411417322834647770 ) ) ;
#14791=CARTESIAN_POINT ( 'NONE',  ( -0.4986876640419939388, 0.1283753931104746893, -0.1820866141732285504 ) ) ;
#14794=CARTESIAN_POINT ( 'NONE',  ( 0.4461942257217855201, -0.6046776061558807314, 0.2411417322834647770 ) ) ;
#14795=CARTESIAN_POINT ( 'NONE',  ( -0.07217847769028813698, -0.3162353388693409650, -0.4822834645669289433 ) ) ;
#14796=CARTESIAN_POINT ( 'NONE',  ( -0.8202099737532799750, 0.2952755905511810774, -0.1292274648535930714 ) ) ;
#14797=CARTESIAN_POINT ( 'NONE',  ( 1.345144356955381593, -0.05778040916215522460, 0.4822834645669289988 ) ) ;
#14798=CARTESIAN_POINT ( 'NONE',  ( -1.036745406824146176, -0.3690944881889763329, 0.3153832671262228327 ) ) ;
#14800=CARTESIAN_POINT ( 'NONE',  ( 0.6955380577427828781, -0.4281496062992124485, 0.4176697321401328655 ) ) ;
#14801=CARTESIAN_POINT ( 'NONE',  ( 0.4199475065616803948, -0.5023911411419708095, -0.1820866141732282451 ) ) ;
#14802=CARTESIAN_POINT ( 'NONE',  ( -0.4986876640419939388, 0.2306618581243847221, -0.2411417322834647770 ) ) ;
#14804=CARTESIAN_POINT ( 'NONE',  ( -1.272965879265091305, 0.05413385826771626580, -0.4176697321401330321 ) ) ;
#14805=CARTESIAN_POINT ( 'NONE',  ( -1.706036745406823485, 0.1283753931104748280, 0.1820866141732283561 ) ) ;
#14806=CARTESIAN_POINT ( 'NONE',  ( 1.522309711286089939, 0.2306618581243848609, 0.2411417322834645549 ) ) ;
#14807=CARTESIAN_POINT ( 'NONE',  ( 1.653543307086614789, -0.1870078740157479769, 0.3641732283464567677 ) ) ;
#14808=ORIENTED_EDGE ( 'NONE', *, *, #8454, .F. ) ;
#14810=CARTESIAN_POINT ( 'NONE',  ( -0.09186351706036663400, -0.4281496062992124485, 0.4176697321401328655 ) ) ;
#14812=CARTESIAN_POINT ( 'NONE',  ( 0.6627296587926515548, 0.1771653543307087630, 0.09757992244046791164 ) ) ;
#14813=CARTESIAN_POINT ( 'NONE',  ( -1.154855643044618851, -0.6046776061558809534, -0.2411417322834644161 ) ) ;
#14814=CARTESIAN_POINT ( 'NONE',  ( 1.056430446194226436, -0.6692913385826773087, -0.1292274648535924053 ) ) ;
#14815=CARTESIAN_POINT ( 'NONE',  ( 1.154855643044620184, 0.2306618581243847221, -0.2411417322834647770 ) ) ;
#14816=CARTESIAN_POINT ( 'NONE',  ( 0.4002624671916016896, -0.3162353388693409650, -0.4822834645669289433 ) ) ;
#14817=CARTESIAN_POINT ( 'NONE',  ( -0.4790026246719152336, -0.05778040916215560624, -0.4822834645669293319 ) ) ;
#14819=CARTESIAN_POINT ( 'NONE',  ( -1.128608923884513837, -0.6046776061558807314, 0.2411417322834647770 ) ) ;
#14820=CARTESIAN_POINT ( 'NONE',  ( -0.7349081364829387342, -0.6046776061558807314, 0.2411417322834647770 ) ) ;
#14821=CARTESIAN_POINT ( 'NONE',  ( -0.5774278215223089816, -0.5023911411419708095, 0.1820866141732285504 ) ) ;
#14822=CARTESIAN_POINT ( 'NONE',  ( 1.633858267716535639, -0.5400638737290844871, 0.3530559997133364547 ) ) ;
#14823=CARTESIAN_POINT ( 'NONE',  ( -0.4396325459317579898, 0.2952755905511811885, 0.1292274648535926551 ) ) ;
#14824=CARTESIAN_POINT ( 'NONE',  ( -1.646051170424378096, 0.000000000000000000, -0.3464511005275205946 ) ) ;
#14825=CARTESIAN_POINT ( 'NONE',  ( 0.5249343832021003964, 0.2306618581243847221, -0.2411417322834647770 ) ) ;
#14828=CARTESIAN_POINT ( 'NONE',  ( -0.1574803149606292529, -0.1870078740157480879, -0.4822834645669291653 ) ) ;
#14829=CARTESIAN_POINT ( 'NONE',  ( 0.8202099737532814183, -0.5511811023622048555, -0.09757992244046775898 ) ) ;
#14832=CARTESIAN_POINT ( 'NONE',  ( 1.082677165354331228, 0.07958543189024071263, -0.2665933059059888421 ) ) ;
#14833=CARTESIAN_POINT ( 'NONE',  ( 1.069553805774278610, -0.6692913385826771977, 0.1292274648535927661 ) ) ;
#14835=CARTESIAN_POINT ( 'NONE',  ( -0.3937007874015740483, -0.1870078740157480879, -0.4822834645669291653 ) ) ;
#14836=CARTESIAN_POINT ( 'NONE',  ( -0.4037097067573596210, -2.567464376874931580E-15, -0.4445507791589072832 ) ) ;
#14837=CARTESIAN_POINT ( 'NONE',  ( -1.712598425196849572, 0.1660481256975885056, 0.3530559997133364547 ) ) ;
#14838=CARTESIAN_POINT ( 'NONE',  ( -0.09186351706036689768, 0.05413385826771626580, -0.4176697321401330321 ) ) ;
#14840=CARTESIAN_POINT ( 'NONE',  ( 1.351706036745407680, 0.05413385826771666132, 0.4176697321401328100 ) ) ;
#14841=CARTESIAN_POINT ( 'NONE',  ( 0.6561679790026253567, 0.2306618581243848609, 0.2411417322834645549 ) ) ;
#14842=CARTESIAN_POINT ( 'NONE',  ( 0.7874015748031503170, -0.1870078740157480601, -0.3641732283464567677 ) ) ;
#14844=CARTESIAN_POINT ( 'NONE',  ( 0.5643044619422579178, -0.004921259842519576551, 0.3153832671262227771 ) ) ;
#14845=CARTESIAN_POINT ( 'NONE',  ( -1.056430446194224881, 0.2066929133858267098, -0.1054918080437494132 ) ) ;
#14847=CARTESIAN_POINT ( 'NONE',  ( 0.5971128608923891301, 0.2952755905511810774, -0.1292274648535930714 ) ) ;
#14849=CARTESIAN_POINT ( 'NONE',  ( 0.3412073490813655186, -0.6046776061558809534, -0.2411417322834644161 ) ) ;
#14851=CARTESIAN_POINT ( 'NONE',  ( -0.3674540682414689785, 0.1539470093639523085, 0.1968503937007873850 ) ) ;
#14852=CARTESIAN_POINT ( 'NONE',  ( 0.1837270341207354329, 0.1283753931104748280, 0.1820866141732283561 ) ) ;
#14853=CARTESIAN_POINT ( 'NONE',  ( 0.5708661417322842269, 0.1660481256975885056, 0.3530559997133364547 ) ) ;
#14854=FACE_OUTER_BOUND ( 'NONE', #6781, .T. ) ;
#14855=CARTESIAN_POINT ( 'NONE',  ( -1.043307086614172707, 0.07958543189024071263, -0.2665933059059888421 ) ) ;
#14856=CARTESIAN_POINT ( 'NONE',  ( -0.9514435695538050464, -0.3162353388693405765, 0.4822834645669290543 ) ) ;
#14857=CARTESIAN_POINT ( 'NONE',  ( -1.496062992125983815, -0.1870078740157480879, -0.4822834645669291653 ) ) ;
#14858=CARTESIAN_POINT ( 'NONE',  ( 0.6102362204724416372, 0.1660481256975883668, -0.3530559997133364547 ) ) ;
#14859=CARTESIAN_POINT ( 'NONE',  ( -1.594488188976377119, 0.07958543189024071263, -0.2665933059059888421 ) ) ;
#14861=CARTESIAN_POINT ( 'NONE',  ( 0.4790026246719167324, -0.05778040916215522460, 0.4822834645669289988 ) ) ;
#14863=CARTESIAN_POINT ( 'NONE',  ( 1.686351706036745890, 0.2952755905511811885, 0.1292274648535926551 ) ) ;
#14864=CARTESIAN_POINT ( 'NONE',  ( 1.325459317585302665, -0.4281496062992124485, 0.4176697321401328655 ) ) ;
#14865=CARTESIAN_POINT ( 'NONE',  ( -1.469816272965878357, -0.5023911411419708095, -0.1820866141732282451 ) ) ;
#14866=CARTESIAN_POINT ( 'NONE',  ( 1.318897637795276356, -0.4536011799217367080, 0.2665933059059888421 ) ) ;
#14867=CARTESIAN_POINT ( 'NONE',  ( -1.509186351706035767, -0.3690944881889763329, 0.3153832671262228327 ) ) ;
#14868=CARTESIAN_POINT ( 'NONE',  ( -0.7283464566929126471, -0.4536011799217367080, 0.2665933059059888421 ) ) ;
#14870=CARTESIAN_POINT ( 'NONE',  ( 1.548556430446194954, -0.6046776061558807314, 0.2411417322834647770 ) ) ;
#14871=CARTESIAN_POINT ( 'NONE',  ( 0.4461942257217855201, -0.5023911411419708095, 0.1820866141732285504 ) ) ;
#14872=CARTESIAN_POINT ( 'NONE',  ( -0.04593175853018302557, 0.2952755905511811885, 0.1292274648535926551 ) ) ;
#14873=CARTESIAN_POINT ( 'NONE',  ( 0.9908136482939640111, 0.2952755905511810774, -0.1292274648535930714 ) ) ;
#14874=CARTESIAN_POINT ( 'NONE',  ( 8.195543980992789655E-16, -0.1870078740157480879, -0.4822834645669291653 ) ) ;
#14875=CARTESIAN_POINT ( 'NONE',  ( 0.1377952755905518800, -0.4536011799217367080, 0.2665933059059888421 ) ) ;
#14877=CARTESIAN_POINT ( 'NONE',  ( 1.181102362204724976, -0.1870078740157480879, -0.4822834645669291653 ) ) ;
#14878=CARTESIAN_POINT ( 'NONE',  ( -1.653543307086613234, -0.1870078740157479769, 0.4822834645669291653 ) ) ;
#14879=CARTESIAN_POINT ( 'NONE',  ( -0.9383202099737524282, -0.05778040916215522460, 0.4822834645669289988 ) ) ;
#14881=CARTESIAN_POINT ( 'NONE',  ( 0.01968503937007930540, 0.1012011053420777407, 0.2882089793578257453 ) ) ;
#14882=CARTESIAN_POINT ( 'NONE',  ( -0.8136482939632537770, 0.2306618581243847221, -0.2411417322834647770 ) ) ;
#14883=CARTESIAN_POINT ( 'NONE',  ( -0.1312335958005241554, 0.2306618581243848609, 0.2411417322834645549 ) ) ;
#14888=CARTESIAN_POINT ( 'NONE',  ( -1.463254593175852492, -0.5511811023622048555, -0.09757992244046775898 ) ) ;
#14890=CARTESIAN_POINT ( 'NONE',  ( -1.686351706036744558, 0.2952755905511810774, -0.1292274648535930714 ) ) ;
#14892=CARTESIAN_POINT ( 'NONE',  ( 0.3805774278215230400, -0.4281496062992124485, 0.4176697321401328655 ) ) ;
#14893=CARTESIAN_POINT ( 'NONE',  ( -0.4330708661417315697, 0.1771653543307087630, 0.000000000000000000 ) ) ;
#14894=CARTESIAN_POINT ( 'NONE',  ( 0.8923884514435701520, -0.6046776061558809534, -0.2411417322834644161 ) ) ;
#14895=CARTESIAN_POINT ( 'NONE',  ( 0.1509186351706042484, -0.3162353388693405765, 0.4822834645669290543 ) ) ;
#14899=CARTESIAN_POINT ( 'NONE',  ( 1.404199475065617708, 0.05413385826771626580, -0.4176697321401330321 ) ) ;
#14900=CARTESIAN_POINT ( 'NONE',  ( 0.05905511811023681640, 0.1660481256975883668, -0.3530559997133364547 ) ) ;
#14901=CARTESIAN_POINT ( 'NONE',  ( 1.574803149606299746, -0.1870078740157479769, 0.4822834645669291653 ) ) ;
#14902=CARTESIAN_POINT ( 'NONE',  ( 0.9317585301837276734, 0.05413385826771626580, -0.4176697321401330321 ) ) ;
#14904=CARTESIAN_POINT ( 'NONE',  ( 0.05905511811023681640, 0.1660481256975883668, -0.3530559997133364547 ) ) ;
#14905=CARTESIAN_POINT ( 'NONE',  ( 0.5249343832021005074, -0.6046776061558807314, 0.2411417322834647770 ) ) ;
#14906=CARTESIAN_POINT ( 'NONE',  ( 0.09186351706036827158, 0.05413385826771666132, 0.4176697321401328100 ) ) ;
#14907=CARTESIAN_POINT ( 'NONE',  ( 0.9186351706036752773, 0.1283753931104746893, -0.1820866141732285504 ) ) ;
#14908=CARTESIAN_POINT ( 'NONE',  ( -1.338582677165353729, -0.1870078740157480879, -0.4822834645669291653 ) ) ;
#14909=CARTESIAN_POINT ( 'NONE',  ( -1.253280839895012377, -0.05778040916215522460, 0.4822834645669289988 ) ) ;
#14910=CARTESIAN_POINT ( 'NONE',  ( 0.6627296587926515548, 0.2952755905511811885, 0.1292274648535926551 ) ) ;
#14916=CARTESIAN_POINT ( 'NONE',  ( 1.240157480314961314, 0.1660481256975883668, -0.3530559997133364547 ) ) ;
#14917=CARTESIAN_POINT ( 'NONE',  ( 0.3674540682414705883, 0.1283753931104746893, -0.1820866141732285504 ) ) ;
#14918=CARTESIAN_POINT ( 'NONE',  ( 0.6167979002624679463, 0.05413385826771626580, -0.4176697321401330321 ) ) ;
#14919=CARTESIAN_POINT ( 'NONE',  ( 0.4531182788721080934, 1.771653543307086354, -0.5309055118110237448 ) ) ;
#14922=CARTESIAN_POINT ( 'NONE',  ( 1.417322834645670104, -0.1870078740157479769, 0.4822834645669291653 ) ) ;
#14924=CARTESIAN_POINT ( 'NONE',  ( -0.2821522309711278487, 0.2952755905511811885, 0.1292274648535926551 ) ) ;
#14925=CARTESIAN_POINT ( 'NONE',  ( 1.115485564304462551, 0.05413385826771666132, 0.4176697321401328100 ) ) ;
#14928=CARTESIAN_POINT ( 'NONE',  ( -1.587926509186350810, -0.4281496062992124485, 0.4176697321401328655 ) ) ;
#14931=CARTESIAN_POINT ( 'NONE',  ( 1.476377952755906442, -0.4536011799217367080, 0.2665933059059888421 ) ) ;
#14933=CARTESIAN_POINT ( 'NONE',  ( -0.8333333333333323711, 0.1771653543307087630, 0.09757992244046791164 ) ) ;
#14934=CARTESIAN_POINT ( 'NONE',  ( -1.620734908136482577, 0.2952755905511811885, 0.1292274648535926551 ) ) ;
#14935=CARTESIAN_POINT ( 'NONE',  ( 0.7349081364829403995, 0.2306618581243848609, 0.2411417322834645549 ) ) ;
#14937=CARTESIAN_POINT ( 'NONE',  ( 1.646981627296588035, -0.3162353388693405765, 0.4822834645669290543 ) ) ;
#14939=CARTESIAN_POINT ( 'NONE',  ( -0.5577427821522301654, -0.08942795157528024563, -0.3641732283464568787 ) ) ;
#14940=CARTESIAN_POINT ( 'NONE',  ( 0.6889763779527566800, -0.5400638737290844871, 0.3530559997133364547 ) ) ;
#14941=CARTESIAN_POINT ( 'NONE',  ( -1.443569553805773564, -0.6046776061558807314, 0.2411417322834647770 ) ) ;
#14943=CARTESIAN_POINT ( 'NONE',  ( -0.6167979002624665030, -0.004921259842519576551, 0.3153832671262227771 ) ) ;
#14944=CARTESIAN_POINT ( 'NONE',  ( -1.417322834645668772, -0.1870078740157480601, -0.3641732283464567677 ) ) ;
#14946=CARTESIAN_POINT ( 'NONE',  ( 0.4527559055118117182, -0.5400638737290844871, 0.3530559997133364547 ) ) ;
#14947=CARTESIAN_POINT ( 'NONE',  ( -1.023622047244093558, -0.1870078740157479769, 0.3641732283464567677 ) ) ;
#14948=CARTESIAN_POINT ( 'NONE',  ( -0.1771653543307080136, -0.4536011799217367080, 0.2665933059059888421 ) ) ;
#14950=CARTESIAN_POINT ( 'NONE',  ( -0.4265091863517051496, 0.2952755905511810774, -0.1292274648535930714 ) ) ;
#14951=CARTESIAN_POINT ( 'NONE',  ( 1.614173228346457378, -0.6692913385826771977, 8.415575281601705876E-17 ) ) ;
#14953=CARTESIAN_POINT ( 'NONE',  ( 0.8989501312335963501, -0.6692913385826773087, -0.1292274648535924053 ) ) ;
#14955=DIRECTION ( 'NONE',  ( -1.000000000000000000, -3.083952846180990774E-16, 0.000000000000000000 ) ) ;
#14957=CARTESIAN_POINT ( 'NONE',  ( -0.8989501312335946848, 0.2952755905511810774, -0.1292274648535930714 ) ) ;
#14958=CARTESIAN_POINT ( 'NONE',  ( -0.3280839895013117347, -0.3690944881889763329, 0.3153832671262228327 ) ) ;
#14959=CARTESIAN_POINT ( 'NONE',  ( -1.423884514435694859, -0.05778040916215560624, -0.4822834645669293319 ) ) ;
#14960=CARTESIAN_POINT ( 'NONE',  ( 0.5446194225721792126, -0.2845877964562159024, 0.3641732283464567677 ) ) ;
#14961=CARTESIAN_POINT ( 'NONE',  ( -0.8595800524934373854, -0.2845877964562161244, -0.3641732283464567121 ) ) ;
#14962=CARTESIAN_POINT ( 'NONE',  ( -1.246719160104986512, 0.05413385826771666132, 0.4176697321401328100 ) ) ;
#14963=CARTESIAN_POINT ( 'NONE',  ( -1.594488188976377563, -0.5400638737290844871, 0.3530559997133364547 ) ) ;
#14964=CARTESIAN_POINT ( 'NONE',  ( -1.548556430446193399, -0.6046776061558809534, -0.2411417322834644161 ) ) ;
#14965=CARTESIAN_POINT ( 'NONE',  ( 1.049868766404200349, 0.1539470093639523085, 0.1968503937007873850 ) ) ;
#14966=CARTESIAN_POINT ( 'NONE',  ( 0.7939632545931766261, -0.2845877964562161244, -0.3641732283464567121 ) ) ;
#14967=CARTESIAN_POINT ( 'NONE',  ( 0.2952755905511819101, 0.1660481256975883668, -0.3530559997133364547 ) ) ;
#14968=CARTESIAN_POINT ( 'NONE',  ( -1.318897637795274802, 0.1660481256975885056, 0.3530559997133364547 ) ) ;
#14969=CARTESIAN_POINT ( 'NONE',  ( 1.607611548556431069, 0.1771653543307087630, 0.09757992244046791164 ) ) ;
#14972=CARTESIAN_POINT ( 'NONE',  ( -1.279527559055116948, 0.07958543189024071263, -0.2665933059059888421 ) ) ;
#14973=CARTESIAN_POINT ( 'NONE',  ( -0.4724409448818890911, -0.1870078740157480879, -0.4822834645669291653 ) ) ;
#14974=CARTESIAN_POINT ( 'NONE',  ( 0.5052493438320215802, 0.2952755905511811885, 0.1292274648535926551 ) ) ;
#14975=CARTESIAN_POINT ( 'NONE',  ( -1.410761154855642463, -0.08942795157527998196, 0.3641732283464567121 ) ) ;
#14977=CARTESIAN_POINT ( 'NONE',  ( -1.482939632545930975, -0.4281496062992127816, -0.4176697321401328100 ) ) ;
#14978=CARTESIAN_POINT ( 'NONE',  ( 0.5708661417322842269, 0.1660481256975885056, 0.3530559997133364547 ) ) ;
#14979=CARTESIAN_POINT ( 'NONE',  ( 0.07217847769028949700, -0.3162353388693405765, 0.4822834645669290543 ) ) ;
#14980=CARTESIAN_POINT ( 'NONE',  ( 1.332020997375328974, -0.05778040916215560624, -0.4822834645669293319 ) ) ;
#14985=CARTESIAN_POINT ( 'NONE',  ( -0.3083989501312330295, -0.08942795157527998196, 0.3641732283464567121 ) ) ;
#14987=CARTESIAN_POINT ( 'NONE',  ( -0.2427821522309703550, -0.05778040916215560624, -0.4822834645669293319 ) ) ;
#14988=CARTESIAN_POINT ( 'NONE',  ( 0.8727034120734912248, -0.3162353388693409650, -0.4822834645669289433 ) ) ;
#14991=CARTESIAN_POINT ( 'NONE',  ( -0.03280839895013062252, 0.1771653543307087075, -0.09757992244046823083 ) ) ;
#14992=CARTESIAN_POINT ( 'NONE',  ( -0.9973753280839886548, 0.2306618581243848609, 0.2411417322834645549 ) ) ;
#14993=CARTESIAN_POINT ( 'NONE',  ( -1.528871391076114250, -0.6692913385826771977, 0.1292274648535927661 ) ) ;
#14996=VERTEX_POINT ( 'NONE', #82121 ) ;
#14998=CARTESIAN_POINT ( 'NONE',  ( 1.450131233595801428, 0.2952755905511811885, 0.1292274648535926551 ) ) ;
#14999=CARTESIAN_POINT ( 'NONE',  ( -1.620734908136482577, -0.6692913385826773087, -0.1292274648535924053 ) ) ;
#15000=CARTESIAN_POINT ( 'NONE',  ( -1.167979002624671470, -0.004921259842519576551, 0.3153832671262227771 ) ) ;
#15001=CARTESIAN_POINT ( 'NONE',  ( -1.148293963254592542, 0.2952755905511811885, 0.1292274648535926551 ) ) ;
#15003=CARTESIAN_POINT ( 'NONE',  ( -1.010498687664041384, 0.009842519685039467087, 0.3409548833797002021 ) ) ;
#15004=CARTESIAN_POINT ( 'NONE',  ( 1.148293963254593875, -0.6692913385826771977, 0.1292274648535927661 ) ) ;
#15005=CARTESIAN_POINT ( 'NONE',  ( -1.646981627296586703, -0.3162353388693409650, -0.4822834645669289433 ) ) ;
#15006=CARTESIAN_POINT ( 'NONE',  ( -0.2296587926509179312, -0.3162353388693409650, -0.4822834645669289433 ) ) ;
#15007=CARTESIAN_POINT ( 'NONE',  ( -0.05249343832020938322, -0.6046776061558809534, -0.2411417322834644161 ) ) ;
#15008=CARTESIAN_POINT ( 'NONE',  ( -1.437007874015747477, 0.1660481256975883668, -0.3530559997133364547 ) ) ;
#15010=CARTESIAN_POINT ( 'NONE',  ( 0.5052493438320215802, 0.2952755905511811885, 0.1292274648535926551 ) ) ;
#15013=CARTESIAN_POINT ( 'NONE',  ( -1.318897637795274802, 0.07958543189024085140, 0.2665933059059887866 ) ) ;
#15014=ORIENTED_EDGE ( 'NONE', *, *, #1342, .F. ) ;
#15018=CARTESIAN_POINT ( 'NONE',  ( -1.148293963254592542, -0.6692913385826773087, -0.1292274648535924053 ) ) ;
#15019=CARTESIAN_POINT ( 'NONE',  ( -1.200787401574802349, -0.5400638737290844871, 0.3530559997133364547 ) ) ;
#15021=CARTESIAN_POINT ( 'NONE',  ( -1.594488188976377563, -0.5400638737290844871, 0.3530559997133364547 ) ) ;
#15023=CARTESIAN_POINT ( 'NONE',  ( -0.9711286089238838626, 0.2306618581243847221, -0.2411417322834647770 ) ) ;
#15026=CARTESIAN_POINT ( 'NONE',  ( -0.06561679790026180015, -0.004921259842519576551, 0.3153832671262227771 ) ) ;
#15027=CARTESIAN_POINT ( 'NONE',  ( -0.7152230971128602510, -0.08942795157528024563, -0.3641732283464568787 ) ) ;
#15028=CARTESIAN_POINT ( 'NONE',  ( -1.325459317585300889, 0.05413385826771666132, 0.4176697321401328100 ) ) ;
#15029=CARTESIAN_POINT ( 'NONE',  ( 1.115485564304462551, 0.05413385826771666132, 0.4176697321401328100 ) ) ;
#15030=CARTESIAN_POINT ( 'NONE',  ( -0.8070866141732276899, 0.1660481256975883668, -0.3530559997133364547 ) ) ;
#15033=CARTESIAN_POINT ( 'NONE',  ( -1.522309711286088607, -0.6046776061558807314, 0.2411417322834647770 ) ) ;
#15034=CARTESIAN_POINT ( 'NONE',  ( 0.7742782152230978099, -0.4281496062992124485, 0.4176697321401328655 ) ) ;
#15035=CARTESIAN_POINT ( 'NONE',  ( -1.666666666666665853, -0.004921259842519870586, -0.3153832671262229437 ) ) ;
#15041=CARTESIAN_POINT ( 'NONE',  ( -0.4790026246719152336, -0.05778040916215560624, -0.4822834645669293319 ) ) ;
#15042=CARTESIAN_POINT ( 'NONE',  ( -1.377952755905511140, -0.5511811023622047445, 6.969142054262312111E-17 ) ) ;
#15044=LINE ( 'NONE', #79860, #38237 ) ;
#15045=CARTESIAN_POINT ( 'NONE',  ( -0.6955380577427815458, 0.009842519685039467087, 0.3409548833797002021 ) ) ;
#15046=CARTESIAN_POINT ( 'NONE',  ( -1.318897637795274802, -0.5400638737290845981, -0.3530559997133363437 ) ) ;
#15047=CARTESIAN_POINT ( 'NONE',  ( -0.3018372703412066094, 0.05413385826771666132, 0.4176697321401328100 ) ) ;
#15049=CARTESIAN_POINT ( 'NONE',  ( 0.3871391076115492380, -0.08942795157528024563, -0.3641732283464568787 ) ) ;
#15051=CARTESIAN_POINT ( 'NONE',  ( 0.3805774278215230400, -0.3690944881889763329, 0.3153832671262228327 ) ) ;
#15052=CARTESIAN_POINT ( 'NONE',  ( 0.8727034120734912248, -0.2845877964562161244, -0.3641732283464567121 ) ) ;
#15053=CARTESIAN_POINT ( 'NONE',  ( 1.161417322834646271, 0.1660481256975883668, -0.3530559997133364547 ) ) ;
#15054=CARTESIAN_POINT ( 'NONE',  ( 0.2493438320209980519, -0.004921259842519576551, 0.3153832671262227771 ) ) ;
#15056=CARTESIAN_POINT ( 'NONE',  ( -1.148293963254592542, 0.2952755905511811885, 0.1292274648535926551 ) ) ;
#15057=CARTESIAN_POINT ( 'NONE',  ( -0.03280839895013062252, -0.5511811023622046335, 0.09757992244046803654 ) ) ;
#15058=CARTESIAN_POINT ( 'NONE',  ( -1.437007874015747477, 0.07958543189024071263, -0.2665933059059888421 ) ) ;
#15060=CARTESIAN_POINT ( 'NONE',  ( -1.122047244094487306, 0.07958543189024071263, -0.2665933059059888421 ) ) ;
#15062=CARTESIAN_POINT ( 'NONE',  ( 0.006561679790026889343, -0.3162353388693409650, -0.4822834645669289433 ) ) ;
#15064=CARTESIAN_POINT ( 'NONE',  ( 0.4068241469816279987, -0.3690944881889765550, -0.3153832671262227771 ) ) ;
#15065=CARTESIAN_POINT ( 'NONE',  ( -0.2165354330708654795, -0.4536011799217368745, -0.2665933059059886201 ) ) ;
#15066=CARTESIAN_POINT ( 'NONE',  ( -0.3871391076115476282, -0.05778040916215522460, 0.4822834645669289988 ) ) ;
#15067=CARTESIAN_POINT ( 'NONE',  ( -1.204164820379010514, 2.401574803149606474, 0.4915354330708645580 ) ) ;
#15068=CARTESIAN_POINT ( 'NONE',  ( -1.181102362204723644, -0.1870078740157479769, 0.3641732283464567677 ) ) ;
#15070=CARTESIAN_POINT ( 'NONE',  ( 0.4330708661417329575, 0.2952755905511811885, 0.000000000000000000 ) ) ;
#15071=ORIENTED_EDGE ( 'NONE', *, *, #3063, .F. ) ;
#15073=CARTESIAN_POINT ( 'NONE',  ( 2.795275590551181910, 1.771653543307087242, 0.000000000000000000 ) ) ;
#15074=CARTESIAN_POINT ( 'NONE',  ( -0.1509186351706028884, -0.08942795157527998196, 0.3641732283464567121 ) ) ;
#15075=CARTESIAN_POINT ( 'NONE',  ( -1.463254593175852492, 0.2952755905511811885, 0.1292274648535926551 ) ) ;
#15076=CARTESIAN_POINT ( 'NONE',  ( -1.469816272965878357, 0.1283753931104748280, 0.1820866141732283561 ) ) ;
#15077=CARTESIAN_POINT ( 'NONE',  ( 1.496062992125985147, -0.1870078740157479769, 0.4822834645669291653 ) ) ;
#15078=CARTESIAN_POINT ( 'NONE',  ( -0.5971128608923877978, 0.1771653543307087630, 0.09757992244046791164 ) ) ;
#15080=CARTESIAN_POINT ( 'NONE',  ( 0.8202099737532813073, 0.2952755905511811885, 0.1292274648535926551 ) ) ;
#15085=CARTESIAN_POINT ( 'NONE',  ( 1.482939632545932307, -0.004921259842519870586, -0.3153832671262229437 ) ) ;
#15086=CARTESIAN_POINT ( 'NONE',  ( -1.318897637795274802, -0.5400638737290845981, -0.3530559997133363437 ) ) ;
#15087=CARTESIAN_POINT ( 'NONE',  ( 1.312335958005249825, 0.2306618581243847221, -0.2411417322834647770 ) ) ;
#15089=CARTESIAN_POINT ( 'NONE',  ( 1.279527559055118724, -0.4536011799217368745, -0.2665933059059886201 ) ) ;
#15091=CARTESIAN_POINT ( 'NONE',  ( -0.01312335958005186876, 0.05413385826771626580, -0.4176697321401330321 ) ) ;
#15092=CARTESIAN_POINT ( 'NONE',  ( -0.3871391076115476282, -0.05778040916215522460, 0.4822834645669289988 ) ) ;
#15094=CARTESIAN_POINT ( 'NONE',  ( 1.586052503253845281, 0.7480314960629931287, -0.1653254495020588799 ) ) ;
#15095=CARTESIAN_POINT ( 'NONE',  ( 0.3346456692913390985, 0.07958543189024085140, 0.2665933059059887866 ) ) ;
#15099=CARTESIAN_POINT ( 'NONE',  ( -0.4133858267716528645, 0.1660481256975883668, -0.3530559997133364547 ) ) ;
#15101=CARTESIAN_POINT ( 'NONE',  ( 1.502624671916010790, -0.3162353388693409650, -0.4822834645669289433 ) ) ;
#15102=CARTESIAN_POINT ( 'NONE',  ( 0.1181102362204730916, 0.2952755905511811885, 0.000000000000000000 ) ) ;
#15103=CARTESIAN_POINT ( 'NONE',  ( -0.3740157480314953431, 0.07958543189024085140, 0.2665933059059887866 ) ) ;
#15104=CARTESIAN_POINT ( 'NONE',  ( 1.213910761154856299, 0.2952755905511811885, 0.1292274648535926551 ) ) ;
#15105=CARTESIAN_POINT ( 'NONE',  ( -1.108923884514435132, -0.05778040916215560624, -0.4822834645669293319 ) ) ;
#15106=CARTESIAN_POINT ( 'NONE',  ( 0.1968503937007881344, 0.2952755905511811885, 0.000000000000000000 ) ) ;
#15107=CARTESIAN_POINT ( 'NONE',  ( -0.9973753280839886548, -0.6046776061558809534, -0.2411417322834644161 ) ) ;
#15108=CARTESIAN_POINT ( 'NONE',  ( 1.128608923884514947, 0.2306618581243848609, 0.2411417322834645549 ) ) ;
#15110=CARTESIAN_POINT ( 'NONE',  ( 0.9973753280839902091, 0.2306618581243847221, -0.2411417322834647770 ) ) ;
#15111=CARTESIAN_POINT ( 'NONE',  ( 1.227034120734908917, 0.2952755905511810774, -0.1292274648535930714 ) ) ;
#15114=CARTESIAN_POINT ( 'NONE',  ( 0.06561679790026316017, -0.3690944881889763329, 0.3153832671262228327 ) ) ;
#15117=ORIENTED_EDGE ( 'NONE', *, *, #73492, .T. ) ;
#15118=CARTESIAN_POINT ( 'NONE',  ( -0.9776902887139098386, -0.5511811023622046335, 0.09757992244046803654 ) ) ;
#15119=CARTESIAN_POINT ( 'NONE',  ( -0.07874015748031421014, -0.1870078740157479769, 0.4822834645669291653 ) ) ;
#15120=CARTESIAN_POINT ( 'NONE',  ( 1.614173228346457378, 0.5038684218300978346, -0.1372047244094476148 ) ) ;
#15121=CARTESIAN_POINT ( 'NONE',  ( -0.07874015748031421014, -0.1870078740157480879, -0.4822834645669291653 ) ) ;
#15122=CARTESIAN_POINT ( 'NONE',  ( -0.4790026246719154557, -0.3162353388693405765, 0.4822834645669290543 ) ) ;
#15123=CARTESIAN_POINT ( 'NONE',  ( -0.9448818897637790704, -0.1870078740157480879, -0.4822834645669291653 ) ) ;
#15124=CARTESIAN_POINT ( 'NONE',  ( -1.614173228346456268, -0.6692913385826771977, 8.415575281601705876E-17 ) ) ;
#15125=CARTESIAN_POINT ( 'NONE',  ( 1.351706036745407680, -0.004921259842519576551, 0.3153832671262227771 ) ) ;
#15127=CARTESIAN_POINT ( 'NONE',  ( 0.3412073490813655186, 0.1283753931104748280, 0.1820866141732283561 ) ) ;
#15128=CARTESIAN_POINT ( 'NONE',  ( 0.006561679790026889343, -0.3162353388693409650, -0.4822834645669289433 ) ) ;
#15129=CARTESIAN_POINT ( 'NONE',  ( 0.4068241469816281097, 0.05413385826771666132, 0.4176697321401328100 ) ) ;
#15130=ORIENTED_EDGE ( 'NONE', *, *, #15427, .T. ) ;
#15132=CARTESIAN_POINT ( 'NONE',  ( -0.6102362204724400829, 0.1012011053420777407, 0.2882089793578257453 ) ) ;
#15135=CARTESIAN_POINT ( 'NONE',  ( -0.7414698162729651543, 0.2952755905511810774, -0.1292274648535930714 ) ) ;
#15138=CARTESIAN_POINT ( 'NONE',  ( -1.469816272965878357, 0.1283753931104748280, 0.1820866141732283561 ) ) ;
#15139=CARTESIAN_POINT ( 'NONE',  ( 0.7414698162729663755, -0.6692913385826773087, -0.1292274648535924053 ) ) ;
#15140=CARTESIAN_POINT ( 'NONE',  ( 1.023622047244095334, -0.1870078740157479769, 0.4822834645669291653 ) ) ;
#15141=CARTESIAN_POINT ( 'NONE',  ( -0.05249343832020911260, 0.1283753931104748280, 0.1820866141732283561 ) ) ;
#15142=CARTESIAN_POINT ( 'NONE',  ( -0.1115485564304456306, 0.2952755905511810774, -0.1292274648535930714 ) ) ;
#15144=CARTESIAN_POINT ( 'NONE',  ( -0.03937007874015669567, 0.1771653543307087630, 0.000000000000000000 ) ) ;
#15145=CARTESIAN_POINT ( 'NONE',  ( -0.01312335958005186876, -0.4281496062992124485, 0.4176697321401328655 ) ) ;
#15147=CARTESIAN_POINT ( 'NONE',  ( 1.555118110236221041, -0.4536011799217367080, 0.2665933059059888421 ) ) ;
#15148=CARTESIAN_POINT ( 'NONE',  ( 0.1115485564304467270, -0.5511811023622048555, -0.09757992244046775898 ) ) ;
#15149=CARTESIAN_POINT ( 'NONE',  ( 1.397637795275591177, 0.07958543189024071263, -0.2665933059059888421 ) ) ;
#15150=CARTESIAN_POINT ( 'NONE',  ( -1.358267716535432434, 0.1660481256975883668, -0.3530559997133364547 ) ) ;
#15151=CARTESIAN_POINT ( 'NONE',  ( -0.5774278215223089816, -0.5023911411419708095, 0.1820866141732285504 ) ) ;
#15152=CARTESIAN_POINT ( 'NONE',  ( -1.035555078613324964, 4.688555745438257773E-15, -0.3627989612356130045 ) ) ;
#15153=CARTESIAN_POINT ( 'NONE',  ( -0.5577427821522301654, -0.05778040916215560624, -0.4822834645669293319 ) ) ;
#15154=CARTESIAN_POINT ( 'NONE',  ( -0.7611548556430438595, -0.6046776061558809534, -0.2411417322834644161 ) ) ;
#15155=CARTESIAN_POINT ( 'NONE',  ( 0.05249343832021075018, -0.6046776061558807314, 0.2411417322834647770 ) ) ;
#15159=CARTESIAN_POINT ( 'NONE',  ( 0.9317585301837276734, -0.004921259842519870586, -0.3153832671262229437 ) ) ;
#15161=CARTESIAN_POINT ( 'NONE',  ( 0.9514435695538062676, -0.05778040916215522460, 0.4822834645669289988 ) ) ;
#15162=CARTESIAN_POINT ( 'NONE',  ( -1.443569553805773564, -0.5023911411419708095, 0.1820866141732285504 ) ) ;
#15163=CARTESIAN_POINT ( 'NONE',  ( 1.207349081364829990, 0.2306618581243848609, 0.2411417322834645549 ) ) ;
#15164=CARTESIAN_POINT ( 'NONE',  ( -1.154855643044618851, -0.5023911411419708095, -0.1820866141732282451 ) ) ;
#15166=CARTESIAN_POINT ( 'NONE',  ( -0.7020997375328076329, -0.3162353388693409650, -0.4822834645669289433 ) ) ;
#15167=CARTESIAN_POINT ( 'NONE',  ( -0.06561679790026180015, -0.004921259842519576551, 0.3153832671262227771 ) ) ;
#15168=CARTESIAN_POINT ( 'NONE',  ( -0.8772393894194419062, 5.410171027439680070E-15, -0.3954985857520040282 ) ) ;
#15169=CARTESIAN_POINT ( 'NONE',  ( 0.8333333333333340365, 0.1771653543307087075, -0.09757992244046823083 ) ) ;
#15170=EDGE_CURVE ( 'NONE', #18898, #60349, #399, .T. ) ;
#15171=CARTESIAN_POINT ( 'NONE',  ( 0.4068241469816281097, 0.05413385826771666132, 0.4176697321401328100 ) ) ;
#15173=CARTESIAN_POINT ( 'NONE',  ( -0.8136482939632537770, -0.6046776061558807314, 0.2411417322834647770 ) ) ;
#15175=CARTESIAN_POINT ( 'NONE',  ( 1.227034120734908917, -0.5511811023622046335, 0.09757992244046803654 ) ) ;
#15176=CARTESIAN_POINT ( 'NONE',  ( 0.6233595800524942554, -0.05778040916215560624, -0.4822834645669293319 ) ) ;
#15177=CARTESIAN_POINT ( 'NONE',  ( -0.09842519685039295696, -0.5400638737290844871, 0.3530559997133364547 ) ) ;
#15178=CARTESIAN_POINT ( 'NONE',  ( -0.1837270341207340729, 0.1283753931104746893, -0.1820866141732285504 ) ) ;
#15179=LINE ( 'NONE', #27370, #61554 ) ;
#15180=CARTESIAN_POINT ( 'NONE',  ( 0.08530183727034192087, -0.08942795157527998196, 0.3641732283464567121 ) ) ;
#15181=CARTESIAN_POINT ( 'NONE',  ( 0.4527559055118117182, 0.1660481256975883668, -0.3530559997133364547 ) ) ;
#15182=CARTESIAN_POINT ( 'NONE',  ( -0.6496062992125976043, -0.4536011799217367080, 0.2665933059059888421 ) ) ;
#15184=CARTESIAN_POINT ( 'NONE',  ( -1.220472440944881054, -0.6692913385826771977, 8.415575281601705876E-17 ) ) ;
#15185=CARTESIAN_POINT ( 'NONE',  ( 0.8554425558739519042, 1.722984403643211298E-16, -0.4118484887281974594 ) ) ;
#15187=CARTESIAN_POINT ( 'NONE',  ( -1.082677165354329896, 0.07958543189024085140, 0.2665933059059887866 ) ) ;
#15188=CARTESIAN_POINT ( 'NONE',  ( -0.2230971128608915943, -0.4281496062992127816, -0.4176697321401328100 ) ) ;
#15190=CARTESIAN_POINT ( 'NONE',  ( -0.8727034120734901146, -0.3162353388693405765, 0.4822834645669290543 ) ) ;
#15192=CARTESIAN_POINT ( 'NONE',  ( 0.4935044252197983150, 1.488513638086841118, -0.5309055118110237448 ) ) ;
#15193=CARTESIAN_POINT ( 'NONE',  ( 0.6824146981627303710, -0.6046776061558807314, 0.2411417322834647770 ) ) ;
#15194=CARTESIAN_POINT ( 'NONE',  ( -0.2493438320209966919, 0.009842519685039144428, -0.3409548833797004797 ) ) ;
#15195=CARTESIAN_POINT ( 'NONE',  ( 1.601049868766404982, 0.2306618581243848609, 0.2411417322834645549 ) ) ;
#15197=CARTESIAN_POINT ( 'NONE',  ( -1.358267716535432434, 0.1660481256975883668, -0.3530559997133364547 ) ) ;
#15199=ORIENTED_EDGE ( 'NONE', *, *, #30053, .T. ) ;
#15200=CARTESIAN_POINT ( 'NONE',  ( -0.4265091863517051496, -0.5511811023622046335, 0.09757992244046803654 ) ) ;
#15202=ORIENTED_EDGE ( 'NONE', *, *, #15589, .T. ) ;
#15203=CARTESIAN_POINT ( 'NONE',  ( 0.9120734908136489683, -0.6692913385826771977, 0.1292274648535927661 ) ) ;
#15204=CARTESIAN_POINT ( 'NONE',  ( 0.1837270341207354329, 0.2306618581243848609, 0.2411417322834645549 ) ) ;
#15205=CARTESIAN_POINT ( 'NONE',  ( -0.8661417322834640276, -0.1870078740157479769, 0.4822834645669291653 ) ) ;
#15206=CARTESIAN_POINT ( 'NONE',  ( 1.653543307086614789, -0.1870078740157479769, 0.4822834645669291653 ) ) ;
#15208=CARTESIAN_POINT ( 'NONE',  ( -0.6824146981627288167, 0.1283753931104748280, 0.1820866141732283561 ) ) ;
#15210=CARTESIAN_POINT ( 'NONE',  ( 0.5052493438320218022, -0.6692913385826773087, -0.1292274648535924053 ) ) ;
#15211=CARTESIAN_POINT ( 'NONE',  ( 0.5052493438320215802, 0.1771653543307087630, 0.09757992244046791164 ) ) ;
#15212=CARTESIAN_POINT ( 'NONE',  ( -1.017060367454067249, -0.05778040916215522460, 0.4822834645669289988 ) ) ;
#15214=CARTESIAN_POINT ( 'NONE',  ( -1.404199475065615932, -0.4281496062992127816, -0.4176697321401328100 ) ) ;
#15215=CARTESIAN_POINT ( 'NONE',  ( -1.686351706036744558, 0.1771653543307087075, -0.09757992244046823083 ) ) ;
#15216=CARTESIAN_POINT ( 'NONE',  ( 1.489501312335958172, -0.3162353388693405765, 0.4822834645669290543 ) ) ;
#15217=CARTESIAN_POINT ( 'NONE',  ( 1.220472440944882608, 0.1771653543307087630, 0.000000000000000000 ) ) ;
#15220=CARTESIAN_POINT ( 'NONE',  ( -0.4658792650918627265, -0.3162353388693409650, -0.4822834645669289433 ) ) ;
#15222=CARTESIAN_POINT ( 'NONE',  ( 0.3937007874015754361, -0.1870078740157480601, -0.3641732283464567677 ) ) ;
#15223=CARTESIAN_POINT ( 'NONE',  ( -1.305774278215222184, -0.6692913385826773087, -0.1292274648535924053 ) ) ;
#15224=CARTESIAN_POINT ( 'NONE',  ( 0.8595800524934390507, -0.05778040916215560624, -0.4822834645669293319 ) ) ;
#15225=CARTESIAN_POINT ( 'NONE',  ( 0.7480314960629927956, -0.6692913385826771977, 8.415575281601705876E-17 ) ) ;
#15226=CARTESIAN_POINT ( 'NONE',  ( 0.3280839895013130669, 0.05413385826771666132, 0.4176697321401328100 ) ) ;
#15228=CARTESIAN_POINT ( 'NONE',  ( -0.4527559055118102749, -0.5400638737290845981, -0.3530559997133363437 ) ) ;
#15230=CARTESIAN_POINT ( 'NONE',  ( 1.535433070866142335, -0.5511811023622047445, 6.969142054262312111E-17 ) ) ;
#15231=CARTESIAN_POINT ( 'NONE',  ( -0.7414698162729651543, -0.6692913385826771977, 0.1292274648535927661 ) ) ;
#15232=CARTESIAN_POINT ( 'NONE',  ( -0.3346456692913377662, 0.07958543189024071263, -0.2665933059059888421 ) ) ;
#15233=CARTESIAN_POINT ( 'NONE',  ( 1.167979002624672580, -0.4281496062992124485, 0.4176697321401328655 ) ) ;
#15234=CARTESIAN_POINT ( 'NONE',  ( 1.463254593175853824, -0.6692913385826771977, 0.1292274648535927661 ) ) ;
#15235=CARTESIAN_POINT ( 'NONE',  ( -0.3477690288713905509, -0.6692913385826771977, 0.1292274648535927661 ) ) ;
#15237=CARTESIAN_POINT ( 'NONE',  ( 0.7874015748031503170, -0.1870078740157479769, 0.4822834645669291653 ) ) ;
#15239=DIRECTION ( 'NONE',  ( 1.000000000000000000, 3.096699300667737464E-16, -1.692413147294446216E-16 ) ) ;
#15240=CARTESIAN_POINT ( 'NONE',  ( -0.1181102362204717315, -0.6692913385826771977, 8.415575281601705876E-17 ) ) ;
#15241=CARTESIAN_POINT ( 'NONE',  ( -1.279527559055116948, 0.07958543189024071263, -0.2665933059059888421 ) ) ;
#15242=CARTESIAN_POINT ( 'NONE',  ( 1.017060367454068803, -0.2845877964562159024, 0.3641732283464567677 ) ) ;
#15243=CARTESIAN_POINT ( 'NONE',  ( 0.4848199769444413998, 1.968301573707852192, -0.4917377963708869926 ) ) ;
#15245=CARTESIAN_POINT ( 'NONE',  ( 1.279527559055118724, -0.4536011799217368745, -0.2665933059059886201 ) ) ;
#15247=CARTESIAN_POINT ( 'NONE',  ( 1.338582677165355062, -0.1870078740157480879, -0.4822834645669291653 ) ) ;
#15249=CARTESIAN_POINT ( 'NONE',  ( -0.3280839895013117347, -0.4281496062992124485, 0.4176697321401328655 ) ) ;
#15251=CARTESIAN_POINT ( 'NONE',  ( 1.423884514435696191, -0.08942795157527998196, 0.3641732283464567121 ) ) ;
#15252=CARTESIAN_POINT ( 'NONE',  ( -0.05905511811023545637, -0.5400638737290845981, -0.3530559997133363437 ) ) ;
#15255=CARTESIAN_POINT ( 'NONE',  ( 1.135170603674541256, -0.6692913385826773087, -0.1292274648535924053 ) ) ;
#15256=CARTESIAN_POINT ( 'NONE',  ( 0.3805774278215230400, 0.05413385826771626580, -0.4176697321401330321 ) ) ;
#15257=CARTESIAN_POINT ( 'NONE',  ( 0.6824146981627303710, -0.5023911411419708095, 0.1820866141732285504 ) ) ;
#15259=CARTESIAN_POINT ( 'NONE',  ( 0.3543307086614181922, -0.5511811023622047445, 6.969142054262312111E-17 ) ) ;
#15262=CARTESIAN_POINT ( 'NONE',  ( 0.6627296587926517768, -0.6692913385826773087, -0.1292274648535924053 ) ) ;
#15264=CARTESIAN_POINT ( 'NONE',  ( 0.9332960234133783617, 0.02791078216816427274, -0.4328096321851894190 ) ) ;
#15266=CARTESIAN_POINT ( 'NONE',  ( 0.2296587926509192634, -0.08942795157528024563, -0.3641732283464568787 ) ) ;
#15267=CARTESIAN_POINT ( 'NONE',  ( -0.08530183727034056085, -0.3162353388693405765, 0.4822834645669290543 ) ) ;
#15268=CARTESIAN_POINT ( 'NONE',  ( 1.541994750656168645, 0.1771653543307087075, -0.09757992244046823083 ) ) ;
#15269=CARTESIAN_POINT ( 'NONE',  ( -1.450131233595799651, -0.5511811023622046335, 0.09757992244046803654 ) ) ;
#15270=CARTESIAN_POINT ( 'NONE',  ( -1.036745406824146176, 0.05413385826771626580, -0.4176697321401330321 ) ) ;
#15272=CARTESIAN_POINT ( 'NONE',  ( 0.6824146981627303710, -0.6046776061558807314, 0.2411417322834647770 ) ) ;
#15273=CARTESIAN_POINT ( 'NONE',  ( 1.509186351706037543, 0.05413385826771666132, 0.4176697321401328100 ) ) ;
#15275=CARTESIAN_POINT ( 'NONE',  ( 0.6102362204724416372, -0.5400638737290844871, 0.3530559997133364547 ) ) ;
#15278=CARTESIAN_POINT ( 'NONE',  ( 1.003937007874016407, -0.5400638737290844871, 0.3530559997133364547 ) ) ;
#15279=CARTESIAN_POINT ( 'NONE',  ( -1.437007874015747477, -0.4536011799217367080, 0.2665933059059888421 ) ) ;
#15280=CARTESIAN_POINT ( 'NONE',  ( 1.272965879265092637, -0.3690944881889765550, -0.3153832671262227771 ) ) ;
#15281=CARTESIAN_POINT ( 'NONE',  ( 1.515748031496063408, 0.1660481256975885056, 0.3530559997133364547 ) ) ;
#15282=CARTESIAN_POINT ( 'NONE',  ( -0.8267716535433065062, 0.1771653543307087630, 0.000000000000000000 ) ) ;
#15283=CARTESIAN_POINT ( 'NONE',  ( 1.515748031496063186, -0.5400638737290845981, -0.3530559997133363437 ) ) ;
#15284=CARTESIAN_POINT ( 'NONE',  ( 0.7020997375328090762, -0.08942795157528024563, -0.3641732283464568787 ) ) ;
#15286=CARTESIAN_POINT ( 'NONE',  ( 0.1968503937007881344, -0.6692913385826771977, 8.415575281601705876E-17 ) ) ;
#15287=CARTESIAN_POINT ( 'NONE',  ( 1.010498687664042716, 0.05413385826771626580, -0.4176697321401330321 ) ) ;
#15288=CARTESIAN_POINT ( 'NONE',  ( -0.04593175853018302557, 0.2952755905511811885, 0.1292274648535926551 ) ) ;
#15289=CARTESIAN_POINT ( 'NONE',  ( -0.05905511811023545637, -0.4536011799217368745, -0.2665933059059886201 ) ) ;
#15290=CARTESIAN_POINT ( 'NONE',  ( 1.246719160104987623, -0.4281496062992124485, 0.4176697321401328655 ) ) ;
#15291=CARTESIAN_POINT ( 'NONE',  ( -1.581364829396324945, -0.05778040916215560624, -0.4822834645669293319 ) ) ;
#15292=CARTESIAN_POINT ( 'NONE',  ( -1.122047244094487306, -0.5400638737290844871, 0.3530559997133364547 ) ) ;
#15294=CARTESIAN_POINT ( 'NONE',  ( -1.213910761154854967, 0.2066929133858267098, -0.1054918080437494132 ) ) ;
#15295=CARTESIAN_POINT ( 'NONE',  ( -0.9251968503937002541, -0.5400638737290845981, -0.3530559997133363437 ) ) ;
#15296=CARTESIAN_POINT ( 'NONE',  ( -0.03280839895013062252, -0.6692913385826771977, 0.1292274648535927661 ) ) ;
#15299=ORIENTED_EDGE ( 'NONE', *, *, #45555, .T. ) ;
#15301=CARTESIAN_POINT ( 'NONE',  ( 1.227034120734908917, -0.6692913385826771977, 0.1292274648535927661 ) ) ;
#15303=CARTESIAN_POINT ( 'NONE',  ( -1.509186351706035767, -0.004921259842519870586, -0.3153832671262229437 ) ) ;
#15304=CARTESIAN_POINT ( 'NONE',  ( 1.614173228346457378, -0.6692913385826771977, 8.415575281601705876E-17 ) ) ;
#15305=CARTESIAN_POINT ( 'NONE',  ( 1.561679790026247350, -0.3690944881889763329, 0.3153832671262228327 ) ) ;
#15307=CARTESIAN_POINT ( 'NONE',  ( 0.2099737532808405305, -0.6046776061558807314, 0.2411417322834647770 ) ) ;
#15308=CARTESIAN_POINT ( 'NONE',  ( -0.5774278215223089816, 0.1283753931104746893, -0.1820866141732285504 ) ) ;
#15309=CARTESIAN_POINT ( 'NONE',  ( 0.6692913385826777528, 0.2952755905511811885, 0.000000000000000000 ) ) ;
#15310=CARTESIAN_POINT ( 'NONE',  ( 0.5183727034120741983, 0.2952755905511810774, -0.1292274648535930714 ) ) ;
#15314=CARTESIAN_POINT ( 'NONE',  ( 1.410761154855643795, -0.05778040916215560624, -0.4822834645669293319 ) ) ;
#15315=CARTESIAN_POINT ( 'NONE',  ( -0.02624671916010428221, -0.6046776061558807314, 0.2411417322834647770 ) ) ;
#15316=CARTESIAN_POINT ( 'NONE',  ( -0.8858267716535425107, -0.5400638737290844871, 0.3530559997133364547 ) ) ;
#15317=CARTESIAN_POINT ( 'NONE',  ( -1.587926509186350810, 0.05413385826771626580, -0.4176697321401330321 ) ) ;
#15318=CARTESIAN_POINT ( 'NONE',  ( 0.7217847769028878924, 0.05413385826771666132, 0.4176697321401328100 ) ) ;
#15320=CARTESIAN_POINT ( 'NONE',  ( -0.3477690288713905509, -0.6692913385826771977, 0.1292274648535927661 ) ) ;
#15321=CARTESIAN_POINT ( 'NONE',  ( 0.4790026246719168435, -0.3162353388693409650, -0.4822834645669289433 ) ) ;
#15322=CARTESIAN_POINT ( 'NONE',  ( -0.03280839895013062252, 0.2952755905511810774, -0.1292274648535930714 ) ) ;
#15324=CARTESIAN_POINT ( 'NONE',  ( 0.7152230971128616943, -0.08942795157527998196, 0.3641732283464567121 ) ) ;
#15325=CARTESIAN_POINT ( 'NONE',  ( -1.535433070866141225, 0.2952755905511811885, 0.000000000000000000 ) ) ;
#15326=CARTESIAN_POINT ( 'NONE',  ( -1.299212598425196097, -0.6692913385826771977, 8.415575281601705876E-17 ) ) ;
#15327=CARTESIAN_POINT ( 'NONE',  ( 0.8464566929133865436, 0.1660481256975883668, -0.3530559997133364547 ) ) ;
#15333=CARTESIAN_POINT ( 'NONE',  ( 1.233595800524935227, 0.2306618581243847221, -0.2411417322834647770 ) ) ;
#15334=CARTESIAN_POINT ( 'NONE',  ( 0.5577427821522314977, -0.2845877964562161244, -0.3641732283464567121 ) ) ;
#15340=AXIS2_PLACEMENT_3D ( 'NONE', #1828, #77602, #27488 ) ;
#15343=CARTESIAN_POINT ( 'NONE',  ( -0.2165354330708654795, -0.5400638737290845981, -0.3530559997133363437 ) ) ;
#15344=CARTESIAN_POINT ( 'NONE',  ( 1.286089238845145033, 0.2306618581243848609, 0.2411417322834645549 ) ) ;
#15346=CARTESIAN_POINT ( 'NONE',  ( -1.706036745406823485, 0.2306618581243848609, 0.2411417322834645549 ) ) ;
#15347=CARTESIAN_POINT ( 'NONE',  ( 1.679790026246720025, 0.1283753931104748280, 0.1820866141732283561 ) ) ;
#15350=CARTESIAN_POINT ( 'NONE',  ( -1.443569553805773564, 0.1283753931104746893, -0.1820866141732285504 ) ) ;
#15352=CARTESIAN_POINT ( 'NONE',  ( 0.2230971128608932319, -0.4281496062992124485, 0.4176697321401328655 ) ) ;
#15353=ORIENTED_EDGE ( 'NONE', *, *, #42934, .T. ) ;
#15354=CARTESIAN_POINT ( 'NONE',  ( 1.541994750656168645, 0.2952755905511810774, -0.1292274648535930714 ) ) ;
#15356=CARTESIAN_POINT ( 'NONE',  ( -0.6824146981627291497, -0.5023911411419708095, -0.1820866141732282451 ) ) ;
#15357=CARTESIAN_POINT ( 'NONE',  ( 0.7742782152230979209, 0.05413385826771626580, -0.4176697321401330321 ) ) ;
#15358=CARTESIAN_POINT ( 'NONE',  ( 1.358267716535433323, -0.4536011799217368745, -0.2665933059059886201 ) ) ;
#15360=CARTESIAN_POINT ( 'NONE',  ( -0.8202099737532801971, -0.5511811023622046335, 0.09757992244046803654 ) ) ;
#15361=CARTESIAN_POINT ( 'NONE',  ( -1.555118110236219930, -0.4536011799217368745, -0.2665933059059886201 ) ) ;
#15363=CARTESIAN_POINT ( 'NONE',  ( 0.4199475065616803948, -0.6046776061558809534, -0.2411417322834644161 ) ) ;
#15364=CARTESIAN_POINT ( 'NONE',  ( -0.8530183727034112984, -0.004921259842519576551, 0.3153832671262227771 ) ) ;
#15365=CARTESIAN_POINT ( 'NONE',  ( -0.3805774278215216522, -0.3690944881889765550, -0.3153832671262227771 ) ) ;
#15366=CARTESIAN_POINT ( 'NONE',  ( -0.3937007874015740483, -0.1870078740157480879, -0.4822834645669291653 ) ) ;
#15367=CARTESIAN_POINT ( 'NONE',  ( -1.627296587926508442, 0.1283753931104748280, 0.1820866141732283561 ) ) ;
#15369=CARTESIAN_POINT ( 'NONE',  ( 0.7611548556430451917, -0.6046776061558807314, 0.2411417322834647770 ) ) ;
#15372=CARTESIAN_POINT ( 'NONE',  ( -0.8858267716535425107, 0.1660481256975883668, -0.3530559997133364547 ) ) ;
#15373=CARTESIAN_POINT ( 'NONE',  ( -0.2296587926509179312, -0.2845877964562161244, -0.3641732283464567121 ) ) ;
#15374=CARTESIAN_POINT ( 'NONE',  ( -1.509186351706035767, -0.4281496062992124485, 0.4176697321401328655 ) ) ;
#15375=CARTESIAN_POINT ( 'NONE',  ( 0.4790026246719168435, -0.2845877964562161244, -0.3641732283464567121 ) ) ;
#15376=CARTESIAN_POINT ( 'NONE',  ( -0.6889763779527552368, -0.4536011799217368745, -0.2665933059059886201 ) ) ;
#15377=CARTESIAN_POINT ( 'NONE',  ( -0.8727034120734901146, -0.05778040916215560624, -0.4822834645669293319 ) ) ;
#15378=CARTESIAN_POINT ( 'NONE',  ( -1.541994750656167090, 0.2952755905511811885, 0.1292274648535926551 ) ) ;
#15379=CARTESIAN_POINT ( 'NONE',  ( 1.213910761154856299, 0.2952755905511811885, 0.1292274648535926551 ) ) ;
#15381=CARTESIAN_POINT ( 'NONE',  ( 0.9251968503937015864, 0.07958543189024071263, -0.2665933059059888421 ) ) ;
#15382=CARTESIAN_POINT ( 'NONE',  ( 0.5183727034120741983, -0.6692913385826771977, 0.1292274648535927661 ) ) ;
#15384=CARTESIAN_POINT ( 'NONE',  ( 1.601049868766404982, 0.1283753931104748280, 0.1820866141732283561 ) ) ;
#15387=CARTESIAN_POINT ( 'NONE',  ( -1.292650918635170010, 0.1771653543307087075, -0.09757992244046823083 ) ) ;
#15388=CARTESIAN_POINT ( 'NONE',  ( -0.2755905511811015396, -0.6692913385826771977, 8.415575281601705876E-17 ) ) ;
#15389=CARTESIAN_POINT ( 'NONE',  ( 0.4265091863517067039, -0.6692913385826773087, -0.1292274648535924053 ) ) ;
#15390=CARTESIAN_POINT ( 'NONE',  ( -1.325459317585300889, -0.3690944881889765550, -0.3153832671262227771 ) ) ;
#15392=CARTESIAN_POINT ( 'NONE',  ( -1.502624671916009680, -0.05778040916215560624, -0.4822834645669293319 ) ) ;
#15393=CARTESIAN_POINT ( 'NONE',  ( 0.2690288713910767848, 0.2952755905511811885, 0.1292274648535926551 ) ) ;
#15394=CARTESIAN_POINT ( 'NONE',  ( -0.09842519685039295696, -0.5400638737290844871, 0.3530559997133364547 ) ) ;
#15395=CARTESIAN_POINT ( 'NONE',  ( 1.325459317585302665, 0.05413385826771626580, -0.4176697321401330321 ) ) ;
#15404=CARTESIAN_POINT ( 'NONE',  ( -0.1115485564304456306, 0.1771653543307087075, -0.09757992244046823083 ) ) ;
#15405=CARTESIAN_POINT ( 'NONE',  ( -0.2493438320209966919, 0.05413385826771626580, -0.4176697321401330321 ) ) ;
#15406=CARTESIAN_POINT ( 'NONE',  ( 1.010498687664042716, 0.05413385826771626580, -0.4176697321401330321 ) ) ;
#15408=CARTESIAN_POINT ( 'NONE',  ( -0.1049868766404193215, -0.5023911411419708095, 0.1820866141732285504 ) ) ;
#15409=CARTESIAN_POINT ( 'NONE',  ( -1.148293963254592542, 0.2952755905511811885, 0.1292274648535926551 ) ) ;
#15410=CARTESIAN_POINT ( 'NONE',  ( -1.561679790026246017, -0.4281496062992127816, -0.4176697321401328100 ) ) ;
#15412=CARTESIAN_POINT ( 'NONE',  ( -0.01000891935578489267, 8.471767977567108961E-16, -0.4445507791589058955 ) ) ;
#15415=CARTESIAN_POINT ( 'NONE',  ( 0.9973753280839902091, 0.2306618581243847221, -0.2411417322834647770 ) ) ;
#15416=CARTESIAN_POINT ( 'NONE',  ( -1.692913385826770645, 0.2952755905511811885, 0.000000000000000000 ) ) ;
#15417=CARTESIAN_POINT ( 'NONE',  ( -1.299212598425196097, 0.1771653543307087630, 0.000000000000000000 ) ) ;
#15418=CARTESIAN_POINT ( 'NONE',  ( -1.154855643044618851, 0.2306618581243848609, 0.2411417322834645549 ) ) ;
#15420=CARTESIAN_POINT ( 'NONE',  ( -1.114781747626346187, -2.609869883881465018E-15, -0.3464511005275220379 ) ) ;
#15421=CARTESIAN_POINT ( 'NONE',  ( 1.371391076115485941, 0.2952755905511811885, 0.1292274648535926551 ) ) ;
#15422=CARTESIAN_POINT ( 'NONE',  ( -1.574803149606298636, -0.1870078740157479769, 0.4822834645669291653 ) ) ;
#15423=CARTESIAN_POINT ( 'NONE',  ( -0.1968503937007867743, -0.6692913385826771977, 8.415575281601705876E-17 ) ) ;
#15424=CARTESIAN_POINT ( 'NONE',  ( -0.3608923884514428360, -0.6692913385826773087, -0.1292274648535924053 ) ) ;
#15425=CARTESIAN_POINT ( 'NONE',  ( -1.338582677165353729, -0.1870078740157479769, 0.4822834645669291653 ) ) ;
#15427=EDGE_CURVE ( 'NONE', #72166, #6582, #4423, .T. ) ;
#15428=CARTESIAN_POINT ( 'NONE',  ( 0.5314960629921264834, 0.1660481256975883668, -0.3530559997133364547 ) ) ;
#15430=CARTESIAN_POINT ( 'NONE',  ( -1.069553805774277722, -0.5511811023622048555, -0.09757992244046775898 ) ) ;
#15431=ORIENTED_EDGE ( 'NONE', *, *, #3865, .F. ) ;
#15433=ORIENTED_EDGE ( 'NONE', *, *, #17984, .F. ) ;
#15434=DIRECTION ( 'NONE',  ( 0.000000000000000000, -1.000000000000000000, -0.000000000000000000 ) ) ;
#15435=CARTESIAN_POINT ( 'NONE',  ( -1.640419947506561060, -0.4281496062992127816, -0.4176697321401328100 ) ) ;
#15436=CARTESIAN_POINT ( 'NONE',  ( 1.397637795275591177, -0.5400638737290844871, 0.3530559997133364547 ) ) ;
#15438=CARTESIAN_POINT ( 'NONE',  ( -1.568241469816272105, -0.05778040916215522460, 0.4822834645669289988 ) ) ;
#15440=CARTESIAN_POINT ( 'NONE',  ( 0.4461942257217856311, 0.2306618581243847221, -0.2411417322834647770 ) ) ;
#15441=CARTESIAN_POINT ( 'NONE',  ( -2.795275590551184575, 0.7480314960629931287, -3.317813449798768424E-16 ) ) ;
#15444=CARTESIAN_POINT ( 'NONE',  ( -0.2099737532808391705, 0.1283753931104748280, 0.1820866141732283561 ) ) ;
#15445=CARTESIAN_POINT ( 'NONE',  ( -0.9186351706036736120, 0.1283753931104748280, 0.1820866141732283561 ) ) ;
#15447=CARTESIAN_POINT ( 'NONE',  ( -1.266404199475064773, -0.05778040916215560624, -0.4822834645669293319 ) ) ;
#15448=CARTESIAN_POINT ( 'NONE',  ( 1.043307086614173818, -0.5400638737290845981, -0.3530559997133363437 ) ) ;
#15449=CARTESIAN_POINT ( 'NONE',  ( -0.7874015748031489847, -0.1870078740157480879, -0.4822834645669291653 ) ) ;
#15451=ORIENTED_EDGE ( 'NONE', *, *, #52110, .T. ) ;
#15452=CARTESIAN_POINT ( 'NONE',  ( -1.266404199475064773, -0.05778040916215560624, -0.4822834645669293319 ) ) ;
#15453=CARTESIAN_POINT ( 'NONE',  ( -1.608952832271129729, 0.2885925887579551818, -0.09257012520105759035 ) ) ;
#15459=CARTESIAN_POINT ( 'NONE',  ( -0.1902887139107604098, 0.2952755905511810774, -0.1292274648535930714 ) ) ;
#15460=CARTESIAN_POINT ( 'NONE',  ( 1.312335958005250269, -0.6046776061558807314, 0.2411417322834647770 ) ) ;
#15462=CARTESIAN_POINT ( 'NONE',  ( -1.541994750656167090, 0.2952755905511811885, 0.1292274648535926551 ) ) ;
#15464=CARTESIAN_POINT ( 'NONE',  ( -1.240157480314959759, 0.1660481256975885056, 0.3530559997133364547 ) ) ;
#15465=CARTESIAN_POINT ( 'NONE',  ( -0.7283464566929126471, 0.1660481256975883668, -0.3530559997133364547 ) ) ;
#15468=CARTESIAN_POINT ( 'NONE',  ( 0.6496062992125991586, 0.07958543189024085140, 0.2665933059059887866 ) ) ;
#15470=CARTESIAN_POINT ( 'NONE',  ( 0.5249343832021005074, -0.5023911411419708095, 0.1820866141732285504 ) ) ;
#15471=CARTESIAN_POINT ( 'NONE',  ( 1.102362204724410155, -0.1870078740157479769, 0.3641732283464567677 ) ) ;
#15472=CARTESIAN_POINT ( 'NONE',  ( 1.049868766404200127, -0.6046776061558809534, -0.2411417322834644161 ) ) ;
#15473=CARTESIAN_POINT ( 'NONE',  ( -0.4593175853018364174, -0.3690944881889765550, -0.3153832671262227771 ) ) ;
#15475=CARTESIAN_POINT ( 'NONE',  ( -1.135170603674539924, 0.2952755905511810774, -0.1292274648535930714 ) ) ;
#15476=CARTESIAN_POINT ( 'NONE',  ( -0.02624671916010428221, -0.5023911411419708095, 0.1820866141732285504 ) ) ;
#15478=CARTESIAN_POINT ( 'NONE',  ( -1.141732283464566011, 0.1771653543307087630, 0.000000000000000000 ) ) ;
#15480=CARTESIAN_POINT ( 'NONE',  ( -0.8333333333333323711, 0.1771653543307087630, 0.09757992244046791164 ) ) ;
#15481=CARTESIAN_POINT ( 'NONE',  ( -0.2099737532808391705, 0.2306618581243848609, 0.2411417322834645549 ) ) ;
#15482=CARTESIAN_POINT ( 'NONE',  ( 1.666666666666667185, -0.004921259842519576551, 0.3153832671262227771 ) ) ;
#15483=CARTESIAN_POINT ( 'NONE',  ( 0.5249343832021003964, 0.1283753931104746893, -0.1820866141732285504 ) ) ;
#15484=CARTESIAN_POINT ( 'NONE',  ( -0.1706036745406816491, -0.3690944881889763329, 0.3153832671262228327 ) ) ;
#15485=CARTESIAN_POINT ( 'NONE',  ( -0.8530183727034112984, 0.05413385826771666132, 0.4176697321401328100 ) ) ;
#15487=CARTESIAN_POINT ( 'NONE',  ( -0.9711286089238838626, 0.1283753931104746893, -0.1820866141732285504 ) ) ;
#15489=CARTESIAN_POINT ( 'NONE',  ( 0.6692913385826778638, -0.6692913385826771977, 8.415575281601705876E-17 ) ) ;
#15491=CARTESIAN_POINT ( 'NONE',  ( 1.515748031496063186, -0.5400638737290845981, -0.3530559997133363437 ) ) ;
#15492=CARTESIAN_POINT ( 'NONE',  ( -0.3280839895013117347, -0.3690944881889763329, 0.3153832671262228327 ) ) ;
#15493=CARTESIAN_POINT ( 'NONE',  ( -0.02624671916010428221, -0.6046776061558807314, 0.2411417322834647770 ) ) ;
#15494=CARTESIAN_POINT ( 'NONE',  ( -1.430446194225720724, 0.05413385826771626580, -0.4176697321401330321 ) ) ;
#15495=CARTESIAN_POINT ( 'NONE',  ( -1.561679790026246017, -0.3690944881889765550, -0.3153832671262227771 ) ) ;
#15496=CARTESIAN_POINT ( 'NONE',  ( 1.200787401574803681, 0.1660481256975885056, 0.3530559997133364547 ) ) ;
#15497=CARTESIAN_POINT ( 'NONE',  ( -0.8661417322834640276, -0.1870078740157480601, -0.3641732283464567677 ) ) ;
#15502=CARTESIAN_POINT ( 'NONE',  ( 1.043307086614173818, -0.4536011799217368745, -0.2665933059059886201 ) ) ;
#15503=CARTESIAN_POINT ( 'NONE',  ( -1.528871391076114250, 0.2952755905511810774, -0.1292274648535930714 ) ) ;
#15504=CARTESIAN_POINT ( 'NONE',  ( 0.8333333333333340365, 0.2952755905511810774, -0.1292274648535930714 ) ) ;
#15506=CARTESIAN_POINT ( 'NONE',  ( 1.345144356955381593, -0.08942795157527998196, 0.3641732283464567121 ) ) ;
#15507=CARTESIAN_POINT ( 'NONE',  ( 0.04593175853018440641, -0.6692913385826771977, 0.1292274648535927661 ) ) ;
#15508=CARTESIAN_POINT ( 'NONE',  ( -0.2690288713910754526, -0.6692913385826771977, 0.1292274648535927661 ) ) ;
#15509=CARTESIAN_POINT ( 'NONE',  ( 1.509186351706037543, 0.05413385826771666132, 0.4176697321401328100 ) ) ;
#15511=CARTESIAN_POINT ( 'NONE',  ( 0.06873123812453012238, 8.471767977567108961E-16, -0.4445507791589058955 ) ) ;
#15513=CARTESIAN_POINT ( 'NONE',  ( 0.2559055118110243332, -0.4536011799217368745, -0.2665933059059886201 ) ) ;
#15515=AXIS2_PLACEMENT_3D ( 'NONE', #80238, #73499, #79821 ) ;
#15518=CARTESIAN_POINT ( 'NONE',  ( -0.6102362204724400829, 0.1660481256975885056, 0.3530559997133364547 ) ) ;
#15519=CARTESIAN_POINT ( 'NONE',  ( 1.174540682414699111, -0.05778040916215560624, -0.4822834645669293319 ) ) ;
#15520=CARTESIAN_POINT ( 'NONE',  ( 0.03937007874015833325, -0.6692913385826771977, 8.415575281601705876E-17 ) ) ;
#15521=CARTESIAN_POINT ( 'NONE',  ( -0.1574803149606292529, -0.1870078740157480601, -0.3641732283464567677 ) ) ;
#15522=CARTESIAN_POINT ( 'NONE',  ( 1.003937007874016407, -0.5400638737290844871, 0.3530559997133364547 ) ) ;
#15523=CARTESIAN_POINT ( 'NONE',  ( -0.8727034120734901146, -0.3162353388693405765, 0.4822834645669290543 ) ) ;
#15524=CARTESIAN_POINT ( 'NONE',  ( -0.4068241469816267775, 0.05413385826771626580, -0.4176697321401330321 ) ) ;
#15525=CARTESIAN_POINT ( 'NONE',  ( -0.7677165354330699465, 0.1660481256975885056, 0.3530559997133364547 ) ) ;
#15526=CARTESIAN_POINT ( 'NONE',  ( 1.056430446194226436, -0.6692913385826773087, -0.1292274648535924053 ) ) ;
#15527=CARTESIAN_POINT ( 'NONE',  ( 1.076115485564305141, -0.6046776061558807314, 0.2411417322834647770 ) ) ;
#15528=CARTESIAN_POINT ( 'NONE',  ( 0.7939632545931766261, -0.3162353388693409650, -0.4822834645669289433 ) ) ;
#15530=CARTESIAN_POINT ( 'NONE',  ( -0.01312335958005186876, -0.004921259842519870586, -0.3153832671262229437 ) ) ;
#15531=ORIENTED_EDGE ( 'NONE', *, *, #57864, .F. ) ;
#15534=CARTESIAN_POINT ( 'NONE',  ( -0.7874015748031489847, -0.1870078740157479769, 0.3641732283464567677 ) ) ;
#15535=CARTESIAN_POINT ( 'NONE',  ( 0.1312335958005257930, 0.2306618581243847221, -0.2411417322834647770 ) ) ;
#15537=CARTESIAN_POINT ( 'NONE',  ( -0.2099737532808391705, -0.6046776061558809534, -0.2411417322834644161 ) ) ;
#15538=CARTESIAN_POINT ( 'NONE',  ( -0.3543307086614165824, -0.6692913385826771977, 8.415575281601705876E-17 ) ) ;
#15539=B_SPLINE_CURVE_WITH_KNOTS ( 'NONE', 3,
 ( #29858, #81229, #55521, #62263, #23546, #74919, #4599 ),
 .UNSPECIFIED., .F., .F.,
 ( 4, 3, 4 ),
 ( 1.734723475976807094E-18, 0.001246230184515548971, 0.002492489877932635954 ),
 .UNSPECIFIED. ) ;
#15540=CARTESIAN_POINT ( 'NONE',  ( -1.154855643044618851, 0.2306618581243848609, 0.2411417322834645549 ) ) ;
#15541=CARTESIAN_POINT ( 'NONE',  ( -1.279527559055116948, -0.5400638737290844871, 0.3530559997133364547 ) ) ;
#15542=CARTESIAN_POINT ( 'NONE',  ( 1.213910761154856299, 0.1771653543307087630, 0.09757992244046791164 ) ) ;
#15545=CARTESIAN_POINT ( 'NONE',  ( 0.4133858267716541968, -0.4536011799217368745, -0.2665933059059886201 ) ) ;
#15546=CARTESIAN_POINT ( 'NONE',  ( 0.1837270341207357105, -0.6046776061558809534, -0.2411417322834644161 ) ) ;
#15547=CARTESIAN_POINT ( 'NONE',  ( 0.2362204724409456558, -0.1870078740157479769, 0.4822834645669291653 ) ) ;
#15554=CARTESIAN_POINT ( 'NONE',  ( -0.4986876640419942164, -0.6046776061558807314, 0.2411417322834647770 ) ) ;
#15557=CARTESIAN_POINT ( 'NONE',  ( -1.555118110236219930, -0.4536011799217368745, -0.2665933059059886201 ) ) ;
#15558=CARTESIAN_POINT ( 'NONE',  ( 0.7677165354330716118, -0.5400638737290844871, 0.3530559997133364547 ) ) ;
#15559=CARTESIAN_POINT ( 'NONE',  ( 0.8202099737532814183, -0.6692913385826773087, -0.1292274648535924053 ) ) ;
#15560=CARTESIAN_POINT ( 'NONE',  ( -0.4002624671916004129, -0.2845877964562159024, 0.3641732283464567677 ) ) ;
#15561=CARTESIAN_POINT ( 'NONE',  ( -0.04593175853018302557, -0.6692913385826773087, -0.1292274648535924053 ) ) ;
#15563=CARTESIAN_POINT ( 'NONE',  ( 0.05905511811023709395, -0.4536011799217367080, 0.2665933059059888421 ) ) ;
#15564=CARTESIAN_POINT ( 'NONE',  ( -0.4593175853018366950, 0.05413385826771666132, 0.4176697321401328100 ) ) ;
#15566=CARTESIAN_POINT ( 'NONE',  ( -1.660104986876639543, -0.05778040916215560624, -0.4822834645669293319 ) ) ;
#15567=CARTESIAN_POINT ( 'NONE',  ( 5.463695987328526437E-16, -0.1870078740157479769, 0.3641732283464567677 ) ) ;
#15568=CARTESIAN_POINT ( 'NONE',  ( 1.528871391076116026, 0.1771653543307087630, 0.09757992244046791164 ) ) ;
#15569=CARTESIAN_POINT ( 'NONE',  ( -1.181102362204723644, -0.1870078740157480879, -0.4822834645669291653 ) ) ;
#15571=CARTESIAN_POINT ( 'NONE',  ( -0.6561679790026240244, 0.1283753931104746893, -0.1820866141732285504 ) ) ;
#15573=CARTESIAN_POINT ( 'NONE',  ( -1.358267716535432434, 0.1660481256975883668, -0.3530559997133364547 ) ) ;
#15574=CARTESIAN_POINT ( 'NONE',  ( -0.7217847769028863381, -0.4281496062992124485, 0.4176697321401328655 ) ) ;
#15575=CARTESIAN_POINT ( 'NONE',  ( 0.1771653543307093182, -0.5400638737290845981, -0.3530559997133363437 ) ) ;
#15579=CARTESIAN_POINT ( 'NONE',  ( 0.4790026246719168435, -0.2845877964562161244, -0.3641732283464567121 ) ) ;
#15580=CARTESIAN_POINT ( 'NONE',  ( 1.056430446194226436, -0.6692913385826773087, -0.1292274648535924053 ) ) ;
#15581=CARTESIAN_POINT ( 'NONE',  ( -1.194225721784776262, -0.004921259842519870586, -0.3153832671262229437 ) ) ;
#15582=CARTESIAN_POINT ( 'NONE',  ( 1.371391076115485941, 0.2952755905511811885, 0.1292274648535926551 ) ) ;
#15583=CARTESIAN_POINT ( 'NONE',  ( -1.469816272965878357, -0.5023911411419708095, -0.1820866141732282451 ) ) ;
#15584=CARTESIAN_POINT ( 'NONE',  ( -0.4658792650918627265, -0.05778040916215522460, 0.4822834645669289988 ) ) ;
#15585=CARTESIAN_POINT ( 'NONE',  ( 0.3215223097112867578, -0.2845877964562161244, -0.3641732283464567121 ) ) ;
#15587=CARTESIAN_POINT ( 'NONE',  ( 0.5183727034120741983, 0.1771653543307087075, -0.09757992244046823083 ) ) ;
#15588=CARTESIAN_POINT ( 'NONE',  ( 0.07217847769028949700, -0.3162353388693405765, 0.4822834645669290543 ) ) ;
#15589=EDGE_CURVE ( 'NONE', #30707, #8650, #32196, .T. ) ;
#15591=CARTESIAN_POINT ( 'NONE',  ( -0.4986876640419942164, -0.6046776061558807314, 0.2411417322834647770 ) ) ;
#15593=CARTESIAN_POINT ( 'NONE',  ( 0.9973753280839902091, 0.1283753931104746893, -0.1820866141732285504 ) ) ;
#15594=CARTESIAN_POINT ( 'NONE',  ( 0.07217847769028949700, -0.3162353388693405765, 0.4822834645669290543 ) ) ;
#15595=CARTESIAN_POINT ( 'NONE',  ( -0.1181102362204717315, -0.6692913385826771977, 8.415575281601705876E-17 ) ) ;
#15596=CARTESIAN_POINT ( 'NONE',  ( -0.3018372703412066094, -0.3690944881889765550, -0.3153832671262227771 ) ) ;
#15598=CARTESIAN_POINT ( 'NONE',  ( -0.6233595800524928121, -0.2845877964562161244, -0.3641732283464567121 ) ) ;
#15599=CARTESIAN_POINT ( 'NONE',  ( 0.5183727034120741983, -0.6692913385826771977, 0.1292274648535927661 ) ) ;
#15600=CARTESIAN_POINT ( 'NONE',  ( -0.8727034120734901146, -0.08942795157528024563, -0.3641732283464568787 ) ) ;
#15602=CARTESIAN_POINT ( 'NONE',  ( -1.286089238845143479, 0.2306618581243847221, -0.2411417322834647770 ) ) ;
#15603=CARTESIAN_POINT ( 'NONE',  ( 0.8550440751474870371, 1.722984403643211298E-16, -0.3954985857520063597 ) ) ;
#15605=CARTESIAN_POINT ( 'NONE',  ( -1.102362204724408601, -0.1870078740157479769, 0.3641732283464567677 ) ) ;
#15606=CARTESIAN_POINT ( 'NONE',  ( -0.4002624671916004129, -0.05778040916215560624, -0.4822834645669293319 ) ) ;
#15608=CARTESIAN_POINT ( 'NONE',  ( -1.699475065616797398, 0.2952755905511811885, 0.1292274648535926551 ) ) ;
#15609=CARTESIAN_POINT ( 'NONE',  ( -1.174540682414697335, -0.05778040916215522460, 0.4822834645669289988 ) ) ;
#15610=FACE_OUTER_BOUND ( 'NONE', #42637, .T. ) ;
#15611=CARTESIAN_POINT ( 'NONE',  ( 1.332020997375329197, -0.3162353388693405765, 0.4822834645669290543 ) ) ;
#15612=CARTESIAN_POINT ( 'NONE',  ( 0.7414698162729663755, 0.2952755905511811885, 0.1292274648535926551 ) ) ;
#15613=CARTESIAN_POINT ( 'NONE',  ( -0.2887139107611542133, 0.1539470093639523085, 0.1968503937007873850 ) ) ;
#15617=CARTESIAN_POINT ( 'NONE',  ( 1.574803149606299746, -0.1870078740157479769, 0.3641732283464567677 ) ) ;
#15619=ORIENTED_EDGE ( 'NONE', *, *, #36782, .T. ) ;
#15620=CARTESIAN_POINT ( 'NONE',  ( -0.6430446194225712953, -0.004921259842519870586, -0.3153832671262229437 ) ) ;
#15622=ORIENTED_EDGE ( 'NONE', *, *, #72813, .T. ) ;
#15623=CARTESIAN_POINT ( 'NONE',  ( 1.010498687664042716, 0.05413385826771626580, -0.4176697321401330321 ) ) ;
#15624=CARTESIAN_POINT ( 'NONE',  ( 0.1902887139107617975, 0.2952755905511811885, 0.1292274648535926551 ) ) ;
#15625=CARTESIAN_POINT ( 'NONE',  ( -0.7611548556430438595, -0.6046776061558809534, -0.2411417322834644161 ) ) ;
#15626=CARTESIAN_POINT ( 'NONE',  ( 1.332020997375329197, -0.3162353388693405765, 0.4822834645669290543 ) ) ;
#15627=CARTESIAN_POINT ( 'NONE',  ( -1.122047244094487306, 0.07958543189024071263, -0.2665933059059888421 ) ) ;
#15628=CARTESIAN_POINT ( 'NONE',  ( -0.6299212598425204535, 1.968503937007873628, -0.4915354330708654462 ) ) ;
#15629=CARTESIAN_POINT ( 'NONE',  ( 0.3477690288713918276, -0.6692913385826773087, -0.1292274648535924053 ) ) ;
#15630=CARTESIAN_POINT ( 'NONE',  ( 0.6430446194225728496, -0.004921259842519576551, 0.3153832671262227771 ) ) ;
#15631=CARTESIAN_POINT ( 'NONE',  ( -0.7020997375328074108, -0.05778040916215522460, 0.4822834645669289988 ) ) ;
#15633=CARTESIAN_POINT ( 'NONE',  ( -1.318897637795274802, 0.1660481256975885056, 0.3530559997133364547 ) ) ;
#15635=CARTESIAN_POINT ( 'NONE',  ( 1.082677165354331228, 0.1660481256975883668, -0.3530559997133364547 ) ) ;
#15636=CARTESIAN_POINT ( 'NONE',  ( 1.154855643044620184, -0.5023911411419708095, 0.1820866141732285504 ) ) ;
#15639=CARTESIAN_POINT ( 'NONE',  ( -0.5708661417322825615, -0.5400638737290844871, 0.3530559997133364547 ) ) ;
#15641=CARTESIAN_POINT ( 'NONE',  ( 0.2755905511811031494, -0.5511811023622047445, 6.969142054262312111E-17 ) ) ;
#15643=CARTESIAN_POINT ( 'NONE',  ( -1.161417322834644716, -0.5400638737290845981, -0.3530559997133363437 ) ) ;
#15644=CARTESIAN_POINT ( 'NONE',  ( 0.8989501312335963501, -0.6692913385826773087, -0.1292274648535924053 ) ) ;
#15645=CARTESIAN_POINT ( 'NONE',  ( 0.7808398950131240079, -0.3162353388693405765, 0.4822834645669290543 ) ) ;
#15646=CARTESIAN_POINT ( 'NONE',  ( -0.05905511811023545637, -0.5400638737290845981, -0.3530559997133363437 ) ) ;
#15647=CARTESIAN_POINT ( 'NONE',  ( -0.3740157480314953431, 0.1660481256975885056, 0.3530559997133364547 ) ) ;
#15649=CARTESIAN_POINT ( 'NONE',  ( -1.653543307086613234, -0.1870078740157480879, -0.4822834645669291653 ) ) ;
#15650=CARTESIAN_POINT ( 'NONE',  ( -0.6036745406824141069, -0.6046776061558809534, -0.2411417322834644161 ) ) ;
#15651=CARTESIAN_POINT ( 'NONE',  ( -0.6299212598425188991, -0.1870078740157480601, -0.3641732283464567677 ) ) ;
#15652=CARTESIAN_POINT ( 'NONE',  ( 1.489501312335958172, -0.3162353388693405765, 0.4822834645669290543 ) ) ;
#15653=DIRECTION ( 'NONE',  ( -0.000000000000000000, 1.000000000000000000, -0.000000000000000000 ) ) ;
#15654=CARTESIAN_POINT ( 'NONE',  ( -1.023622047244094002, -0.1870078740157480879, -0.4822834645669291653 ) ) ;
#15656=CARTESIAN_POINT ( 'NONE',  ( 0.5118110236220478892, 0.2952755905511811885, 0.000000000000000000 ) ) ;
#15658=LINE ( 'NONE', #75269, #30821 ) ;
#15659=CARTESIAN_POINT ( 'NONE',  ( -0.1837270341207340729, 0.2306618581243847221, -0.2411417322834647770 ) ) ;
#15660=CARTESIAN_POINT ( 'NONE',  ( -1.364829396325458521, -0.5023911411419708095, 0.1820866141732285504 ) ) ;
#15661=CARTESIAN_POINT ( 'NONE',  ( 1.102362204724410155, -0.1870078740157480601, -0.3641732283464567677 ) ) ;
#15663=CARTESIAN_POINT ( 'NONE',  ( 1.272965879265092637, -0.3690944881889765550, -0.3153832671262227771 ) ) ;
#15664=CARTESIAN_POINT ( 'NONE',  ( 0.7152230971128614723, -0.3162353388693409650, -0.4822834645669289433 ) ) ;
#15666=CARTESIAN_POINT ( 'NONE',  ( -0.4855643044619415427, -0.4281496062992124485, 0.4176697321401328655 ) ) ;
#15668=CARTESIAN_POINT ( 'NONE',  ( 1.384514435695538337, -0.5511811023622046335, 0.09757992244046803654 ) ) ;
#15669=CARTESIAN_POINT ( 'NONE',  ( -0.5249343832020990641, -0.6046776061558809534, -0.2411417322834644161 ) ) ;
#15672=CARTESIAN_POINT ( 'NONE',  ( 1.391076115485564868, 0.2306618581243847221, -0.2411417322834647770 ) ) ;
#15673=CARTESIAN_POINT ( 'NONE',  ( 0.3149606299212603933, -0.1870078740157479769, 0.4822834645669291653 ) ) ;
#15674=CARTESIAN_POINT ( 'NONE',  ( 0.5905511811023629321, 0.1771653543307087630, 0.000000000000000000 ) ) ;
#15676=CARTESIAN_POINT ( 'NONE',  ( 0.5249343832021005074, -0.5023911411419708095, 0.1820866141732285504 ) ) ;
#15677=CARTESIAN_POINT ( 'NONE',  ( -0.06632061457837669372, -2.294479370626195693E-15, 0.3464511005275217603 ) ) ;
#15679=CARTESIAN_POINT ( 'NONE',  ( 0.5708661417322842269, 0.1660481256975885056, 0.3530559997133364547 ) ) ;
#15680=AXIS2_PLACEMENT_3D ( 'NONE', #72290, #9145, #40292 ) ;
#15682=VECTOR ( 'NONE', #81678, 39.37007874015748143 ) ;
#15683=AXIS2_PLACEMENT_3D ( 'NONE', #66003, #14527, #64190 ) ;
#15684=CARTESIAN_POINT ( 'NONE',  ( 0.2262115530851599166, 8.471767977567108961E-16, -0.4445507791589058955 ) ) ;
#15686=CARTESIAN_POINT ( 'NONE',  ( 0.2230971128608929543, -0.004921259842519870586, -0.3153832671262229437 ) ) ;
#15687=CARTESIAN_POINT ( 'NONE',  ( 0.09186351706036827158, 0.05413385826771666132, 0.4176697321401328100 ) ) ;
#15688=CARTESIAN_POINT ( 'NONE',  ( 1.489501312335958172, -0.2845877964562159024, 0.3641732283464567677 ) ) ;
#15689=CARTESIAN_POINT ( 'NONE',  ( -1.240157480314959759, 0.07958543189024085140, 0.2665933059059887866 ) ) ;
#15690=CARTESIAN_POINT ( 'NONE',  ( -1.279527559055116948, -0.5400638737290844871, 0.3530559997133364547 ) ) ;
#15691=CARTESIAN_POINT ( 'NONE',  ( 0.6692913385826778638, -0.6692913385826771977, 8.415575281601705876E-17 ) ) ;
#15692=CARTESIAN_POINT ( 'NONE',  ( 1.561679790026247350, 0.05413385826771626580, -0.4176697321401330321 ) ) ;
#15694=CARTESIAN_POINT ( 'NONE',  ( 0.5249343832021003964, 0.2306618581243847221, -0.2411417322834647770 ) ) ;
#15696=CARTESIAN_POINT ( 'NONE',  ( 1.443569553805774897, -0.6046776061558809534, -0.2411417322834644161 ) ) ;
#15697=CARTESIAN_POINT ( 'NONE',  ( 0.8333333333333340365, -0.6692913385826771977, 0.1292274648535927661 ) ) ;
#15698=CARTESIAN_POINT ( 'NONE',  ( -1.679790026246718693, 0.1283753931104746893, -0.1820866141732285504 ) ) ;
#15699=CARTESIAN_POINT ( 'NONE',  ( 1.200787401574803681, 0.07958543189024085140, 0.2665933059059887866 ) ) ;
#15700=CARTESIAN_POINT ( 'NONE',  ( -1.646981627296586703, -0.08942795157527998196, 0.3641732283464567121 ) ) ;
#15701=CARTESIAN_POINT ( 'NONE',  ( -0.9448818897637790704, -0.1870078740157480601, -0.3641732283464567677 ) ) ;
#15702=CARTESIAN_POINT ( 'NONE',  ( 0.6955380577427828781, -0.004921259842519870586, -0.3153832671262229437 ) ) ;
#15703=CARTESIAN_POINT ( 'NONE',  ( 0.2690288713910767848, 0.2952755905511811885, 0.1292274648535926551 ) ) ;
#15704=CARTESIAN_POINT ( 'NONE',  ( 0.7545931758530188826, -0.6692913385826771977, 0.1292274648535927661 ) ) ;
#15705=CARTESIAN_POINT ( 'NONE',  ( -0.2034120734908128059, 0.2952755905511811885, 0.1292274648535926551 ) ) ;
#15706=CARTESIAN_POINT ( 'NONE',  ( 0.1181102362204730916, -0.5511811023622047445, 6.969142054262312111E-17 ) ) ;
#15707=CARTESIAN_POINT ( 'NONE',  ( 1.332020997375328974, -0.05778040916215560624, -0.4822834645669293319 ) ) ;
#15708=DIRECTION ( 'NONE',  ( 0.000000000000000000, 0.000000000000000000, 1.000000000000000000 ) ) ;
#15709=CARTESIAN_POINT ( 'NONE',  ( -0.8070866141732276899, -0.5400638737290844871, 0.3530559997133364547 ) ) ;
#15713=CARTESIAN_POINT ( 'NONE',  ( -0.6561679790026240244, 0.2306618581243847221, -0.2411417322834647770 ) ) ;
#15714=CARTESIAN_POINT ( 'NONE',  ( -0.5905511811023615998, 0.2952755905511811885, 0.000000000000000000 ) ) ;
#15719=CARTESIAN_POINT ( 'NONE',  ( 0.6102362204724416372, 0.07958543189024071263, -0.2665933059059888421 ) ) ;
#15721=CARTESIAN_POINT ( 'NONE',  ( 1.115485564304462551, 0.05413385826771666132, 0.4176697321401328100 ) ) ;
#15723=EDGE_CURVE ( 'NONE', #41461, #76146, #71219, .T. ) ;
#15724=CARTESIAN_POINT ( 'NONE',  ( -1.181102362204723644, -0.1870078740157480601, -0.3641732283464567677 ) ) ;
#15725=DIRECTION ( 'NONE',  ( 0.000000000000000000, 1.000000000000000000, 0.000000000000000000 ) ) ;
#15726=CARTESIAN_POINT ( 'NONE',  ( -1.712598425196849572, 0.1660481256975885056, 0.3530559997133364547 ) ) ;
#15728=CARTESIAN_POINT ( 'NONE',  ( 0.1312335958005257930, 0.2306618581243847221, -0.2411417322834647770 ) ) ;
#15729=CARTESIAN_POINT ( 'NONE',  ( -0.6167979002624665030, -0.004921259842519576551, 0.3153832671262227771 ) ) ;
#15730=CARTESIAN_POINT ( 'NONE',  ( 0.9055118110236227702, -0.6692913385826771977, 8.415575281601705876E-17 ) ) ;
#15731=CARTESIAN_POINT ( 'NONE',  ( -0.1902887139107604098, -0.6692913385826771977, 0.1292274648535927661 ) ) ;
#15732=CARTESIAN_POINT ( 'NONE',  ( 2.795275590551181466, 2.362204724409448620, 0.000000000000000000 ) ) ;
#15736=CARTESIAN_POINT ( 'NONE',  ( 0.9645669291338591078, -0.5400638737290845981, -0.3530559997133363437 ) ) ;
#15738=CARTESIAN_POINT ( 'NONE',  ( 0.2034120734908142214, 0.2952755905511810774, -0.1292274648535930714 ) ) ;
#15739=CARTESIAN_POINT ( 'NONE',  ( -0.9448818897637790704, -0.1870078740157480879, -0.4822834645669291653 ) ) ;
#15740=CARTESIAN_POINT ( 'NONE',  ( 1.115485564304462551, 0.05413385826771666132, 0.4176697321401328100 ) ) ;
#15741=CARTESIAN_POINT ( 'NONE',  ( 0.9711286089238851948, -0.6046776061558809534, -0.2411417322834644161 ) ) ;
#15743=CARTESIAN_POINT ( 'NONE',  ( -0.3083989501312330295, -0.05778040916215522460, 0.4822834645669289988 ) ) ;
#15744=CARTESIAN_POINT ( 'NONE',  ( 0.5905511811023629321, 0.2952755905511811885, 0.000000000000000000 ) ) ;
#15745=CARTESIAN_POINT ( 'NONE',  ( 0.03280839895013198948, -0.6692913385826773087, -0.1292274648535924053 ) ) ;
#15746=CARTESIAN_POINT ( 'NONE',  ( 0.7808398950131241190, -0.08942795157528024563, -0.3641732283464568787 ) ) ;
#15747=CARTESIAN_POINT ( 'NONE',  ( -1.397637795275589623, 0.1660481256975885056, 0.3530559997133364547 ) ) ;
#15749=CARTESIAN_POINT ( 'NONE',  ( 0.3215223097112867578, -0.05778040916215522460, 0.4822834645669289988 ) ) ;
#15751=ADVANCED_FACE ( 'NONE', ( #1281 ), #26930, .F. ) ;
#15755=CARTESIAN_POINT ( 'NONE',  ( 0.9842519685039378130, -0.6692913385826771977, 8.415575281601705876E-17 ) ) ;
#15756=CARTESIAN_POINT ( 'NONE',  ( 0.5249343832021003964, 0.1283753931104746893, -0.1820866141732285504 ) ) ;
#15757=CARTESIAN_POINT ( 'NONE',  ( -1.614173228346456712, 2.401574803149606474, 0.1372047244094477536 ) ) ;
#15758=CARTESIAN_POINT ( 'NONE',  ( 0.6183353934921186346, 0.02791078216816508459, -0.4328096321851889194 ) ) ;
#15764=CARTESIAN_POINT ( 'NONE',  ( -0.9842519685039360366, 0.2952755905511811885, 0.000000000000000000 ) ) ;
#15765=CARTESIAN_POINT ( 'NONE',  ( -0.6102362204724400829, 0.1660481256975885056, 0.3530559997133364547 ) ) ;
#15766=CARTESIAN_POINT ( 'NONE',  ( 1.095800524934383846, -0.3162353388693405765, 0.4822834645669290543 ) ) ;
#15768=CARTESIAN_POINT ( 'NONE',  ( 1.167979002624672580, 0.05413385826771626580, -0.4176697321401330321 ) ) ;
#15769=DIRECTION ( 'NONE',  ( 0.000000000000000000, -1.000000000000000000, 0.000000000000000000 ) ) ;
#15771=CARTESIAN_POINT ( 'NONE',  ( 1.633858267716535639, -0.4536011799217367080, 0.2665933059059888421 ) ) ;
#15773=CARTESIAN_POINT ( 'NONE',  ( -1.148293963254592542, 0.1771653543307087630, 0.09757992244046791164 ) ) ;
#15774=EDGE_CURVE ( 'NONE', #36844, #72992, #36037, .T. ) ;
#15776=CARTESIAN_POINT ( 'NONE',  ( 0.3871391076115493490, -0.3162353388693405765, 0.4822834645669290543 ) ) ;
#15777=PLANE ( 'NONE',  #25058 ) ;
#15778=CARTESIAN_POINT ( 'NONE',  ( -1.259842519685038686, -0.1870078740157479769, 0.3641732283464567677 ) ) ;
#15779=CARTESIAN_POINT ( 'NONE',  ( 0.9711286089238851948, -0.6046776061558809534, -0.2411417322834644161 ) ) ;
#15780=CARTESIAN_POINT ( 'NONE',  ( 1.286089238845145033, 0.1283753931104748280, 0.1820866141732283561 ) ) ;
#15782=CARTESIAN_POINT ( 'NONE',  ( -0.8398950131233589023, -0.5023911411419708095, -0.1820866141732282451 ) ) ;
#15783=CARTESIAN_POINT ( 'NONE',  ( 1.443569553805774897, -0.6046776061558809534, -0.2411417322834644161 ) ) ;
#15785=CARTESIAN_POINT ( 'NONE',  ( -0.04593175853018302557, -0.6692913385826773087, -0.1292274648535924053 ) ) ;
#15786=CARTESIAN_POINT ( 'NONE',  ( -1.541994750656167090, -0.5511811023622048555, -0.09757992244046775898 ) ) ;
#15787=CARTESIAN_POINT ( 'NONE',  ( -0.1706036745406816491, -0.3690944881889763329, 0.3153832671262228327 ) ) ;
#15788=CARTESIAN_POINT ( 'NONE',  ( -0.3543307086614165824, -0.6692913385826771977, 8.415575281601705876E-17 ) ) ;
#15789=CARTESIAN_POINT ( 'NONE',  ( -1.594488188976377119, 0.07958543189024071263, -0.2665933059059888421 ) ) ;
#15791=CARTESIAN_POINT ( 'NONE',  ( 0.3412073490813655186, 0.2306618581243848609, 0.2411417322834645549 ) ) ;
#15792=CIRCLE ( 'NONE', #43925, 2.362204724409449064 ) ;
#15796=CARTESIAN_POINT ( 'NONE',  ( -0.8333333333333323711, -0.6692913385826773087, -0.1292274648535924053 ) ) ;
#15797=CARTESIAN_POINT ( 'NONE',  ( -0.2230971128608915943, -0.3690944881889765550, -0.3153832671262227771 ) ) ;
#15798=CARTESIAN_POINT ( 'NONE',  ( -1.548556430446193399, -0.6046776061558809534, -0.2411417322834644161 ) ) ;
#15799=CARTESIAN_POINT ( 'NONE',  ( -0.1181102362204717315, -0.6692913385826771977, 8.415575281601705876E-17 ) ) ;
#15800=CARTESIAN_POINT ( 'NONE',  ( 0.6102362204724416372, 0.07958543189024071263, -0.2665933059059888421 ) ) ;
#15801=CARTESIAN_POINT ( 'NONE',  ( -0.8398950131233589023, -0.5023911411419708095, -0.1820866141732282451 ) ) ;
#15802=CARTESIAN_POINT ( 'NONE',  ( -0.8530183727034112984, -0.4281496062992127816, -0.4176697321401328100 ) ) ;
#15803=CARTESIAN_POINT ( 'NONE',  ( -1.692913385826770645, 0.2952755905511811885, 0.000000000000000000 ) ) ;
#15804=CARTESIAN_POINT ( 'NONE',  ( 1.515748031496063408, 0.1660481256975885056, 0.3530559997133364547 ) ) ;
#15806=CARTESIAN_POINT ( 'NONE',  ( 0.6758530183727039509, -0.5511811023622046335, 0.09757992244046803654 ) ) ;
#15808=CARTESIAN_POINT ( 'NONE',  ( 0.6955380577427828781, -0.4281496062992124485, 0.4176697321401328655 ) ) ;
#15810=CARTESIAN_POINT ( 'NONE',  ( 1.207349081364829990, -0.5023911411419708095, -0.1820866141732282451 ) ) ;
#15811=ORIENTED_EDGE ( 'NONE', *, *, #67121, .T. ) ;
#15812=CARTESIAN_POINT ( 'NONE',  ( -0.7874015748031489847, -0.1870078740157480879, -0.4822834645669291653 ) ) ;
#15813=B_SPLINE_CURVE_WITH_KNOTS ( 'NONE', 3,
 ( #81739, #45042, #12258, #57259 ),
 .UNSPECIFIED., .F., .F.,
 ( 4, 4 ),
 ( 0.000000000000000000, 0.001493228121701170282 ),
 .UNSPECIFIED. ) ;
#15815=CARTESIAN_POINT ( 'NONE',  ( -1.102362204724408601, -0.1870078740157480601, -0.3641732283464567677 ) ) ;
#15816=CARTESIAN_POINT ( 'NONE',  ( -0.4068241469816264999, -0.4281496062992124485, 0.4176697321401328655 ) ) ;
#15817=CARTESIAN_POINT ( 'NONE',  ( 0.2165354330708668673, 0.1660481256975883668, -0.3530559997133364547 ) ) ;
#15818=CARTESIAN_POINT ( 'NONE',  ( -1.640419947506561060, -0.3690944881889765550, -0.3153832671262227771 ) ) ;
#15820=CARTESIAN_POINT ( 'NONE',  ( -1.463254593175852492, -0.6692913385826773087, -0.1292274648535924053 ) ) ;
#15821=CARTESIAN_POINT ( 'NONE',  ( 0.2952755905511819101, 0.1660481256975883668, -0.3530559997133364547 ) ) ;
#15822=CARTESIAN_POINT ( 'NONE',  ( 0.1706036745406830368, -0.4281496062992127816, -0.4176697321401328100 ) ) ;
#15823=CARTESIAN_POINT ( 'NONE',  ( 1.338582677165355062, -0.1870078740157480879, -0.4822834645669291653 ) ) ;
#15824=CARTESIAN_POINT ( 'NONE',  ( 1.686351706036745890, 0.2952755905511811885, 0.1292274648535926551 ) ) ;
#15829=DIRECTION ( 'NONE',  ( 0.000000000000000000, 1.000000000000000000, 0.000000000000000000 ) ) ;
#15831=CARTESIAN_POINT ( 'NONE',  ( -0.1706036745406816491, -0.3690944881889763329, 0.3153832671262228327 ) ) ;
#15832=CARTESIAN_POINT ( 'NONE',  ( -0.1443569553805768291, 0.05413385826771666132, 0.4176697321401328100 ) ) ;
#15833=CARTESIAN_POINT ( 'NONE',  ( 0.7874015748031503170, -0.1870078740157479769, 0.4822834645669291653 ) ) ;
#15835=CARTESIAN_POINT ( 'NONE',  ( 0.1443569553805781891, -0.004921259842519870586, -0.3153832671262229437 ) ) ;
#15836=CARTESIAN_POINT ( 'NONE',  ( -1.082677165354329896, -0.5400638737290845981, -0.3530559997133363437 ) ) ;
#15837=CARTESIAN_POINT ( 'NONE',  ( 1.049868766404200127, -0.6046776061558809534, -0.2411417322834644161 ) ) ;
#15839=DIRECTION ( 'NONE',  ( -0.8050726085550603539, -2.493067783899206833E-16, -0.5931762764594944448 ) ) ;
#15840=VERTEX_POINT ( 'NONE', #41231 ) ;
#15841=ORIENTED_EDGE ( 'NONE', *, *, #73907, .T. ) ;
#15842=CARTESIAN_POINT ( 'NONE',  ( 1.135170603674541256, 0.2952755905511811885, 0.1292274648535926551 ) ) ;
#15843=CARTESIAN_POINT ( 'NONE',  ( -1.496062992125983815, -0.1870078740157480879, -0.4822834645669291653 ) ) ;
#15844=CARTESIAN_POINT ( 'NONE',  ( -1.089238845144356427, -0.3690944881889765550, -0.3153832671262227771 ) ) ;
#15845=CARTESIAN_POINT ( 'NONE',  ( -0.9973753280839886548, 0.2306618581243848609, 0.2411417322834645549 ) ) ;
#15847=CARTESIAN_POINT ( 'NONE',  ( 1.193521905106662784, 3.421639014772782816E-16, 0.3464511005275203726 ) ) ;
#15848=CARTESIAN_POINT ( 'NONE',  ( 1.076115485564305141, 0.2306618581243847221, -0.2411417322834647770 ) ) ;
#15850=CARTESIAN_POINT ( 'NONE',  ( 0.02624671916010564918, 0.2306618581243848609, 0.2411417322834645549 ) ) ;
#15851=CARTESIAN_POINT ( 'NONE',  ( -0.6430446194225716283, -0.4281496062992124485, 0.4176697321401328655 ) ) ;
#15852=CARTESIAN_POINT ( 'NONE',  ( -1.450131233595799651, 0.2952755905511810774, -0.1292274648535930714 ) ) ;
#15854=CARTESIAN_POINT ( 'NONE',  ( 0.05249343832021075018, 0.2306618581243847221, -0.2411417322834647770 ) ) ;
#15856=CARTESIAN_POINT ( 'NONE',  ( -1.332020997375327642, -0.08942795157527998196, 0.3641732283464567121 ) ) ;
#15859=ORIENTED_EDGE ( 'NONE', *, *, #70225, .F. ) ;
#15862=CARTESIAN_POINT ( 'NONE',  ( 1.601049868766404982, 0.1283753931104748280, 0.1820866141732283561 ) ) ;
#15864=CARTESIAN_POINT ( 'NONE',  ( -1.653543307086613234, -0.1870078740157480879, -0.4822834645669291653 ) ) ;
#15865=CARTESIAN_POINT ( 'NONE',  ( -1.489501312335957062, -0.3162353388693409650, -0.4822834645669289433 ) ) ;
#15866=CARTESIAN_POINT ( 'NONE',  ( -0.9908136482939625678, 0.2952755905511811885, 0.1292274648535926551 ) ) ;
#15867=CARTESIAN_POINT ( 'NONE',  ( -0.3836918680457887532, -2.191421614605370878E-15, 0.4445507791589071167 ) ) ;
#15869=CARTESIAN_POINT ( 'NONE',  ( -0.2493438320209966919, -0.3690944881889763329, 0.3153832671262228327 ) ) ;
#15870=CARTESIAN_POINT ( 'NONE',  ( -0.7217847769028863381, -0.004921259842519870586, -0.3153832671262229437 ) ) ;
#15871=CARTESIAN_POINT ( 'NONE',  ( -1.167979002624671470, 0.05413385826771666132, 0.4176697321401328100 ) ) ;
#15872=CARTESIAN_POINT ( 'NONE',  ( 0.4199475065616803948, -0.6046776061558809534, -0.2411417322834644161 ) ) ;
#15873=CARTESIAN_POINT ( 'NONE',  ( -0.7414698162729651543, -0.6692913385826771977, 0.1292274648535927661 ) ) ;
#15876=CARTESIAN_POINT ( 'NONE',  ( -1.594488188976377119, 0.1660481256975883668, -0.3530559997133364547 ) ) ;
#15877=DIRECTION ( 'NONE',  ( 0.000000000000000000, -1.000000000000000000, 0.000000000000000000 ) ) ;
#15879=PLANE ( 'NONE',  #4915 ) ;
#15882=CARTESIAN_POINT ( 'NONE',  ( -0.5774278215223089816, -0.6046776061558807314, 0.2411417322834647770 ) ) ;
#15883=CARTESIAN_POINT ( 'NONE',  ( 1.443569553805774897, -0.6046776061558809534, -0.2411417322834644161 ) ) ;
#15886=CARTESIAN_POINT ( 'NONE',  ( -1.325459317585300889, -0.4281496062992127816, -0.4176697321401328100 ) ) ;
#15887=CARTESIAN_POINT ( 'NONE',  ( -0.6430446194225716283, -0.4281496062992124485, 0.4176697321401328655 ) ) ;
#15889=CARTESIAN_POINT ( 'NONE',  ( 0.3215223097112867578, -0.08942795157527998196, 0.3641732283464567121 ) ) ;
#15891=CARTESIAN_POINT ( 'NONE',  ( 0.1509186351706045259, -0.08942795157528024563, -0.3641732283464568787 ) ) ;
#15892=CARTESIAN_POINT ( 'NONE',  ( 1.082677165354331228, -0.4536011799217367080, 0.2665933059059888421 ) ) ;
#15893=CARTESIAN_POINT ( 'NONE',  ( 0.8005249343832027131, 0.05413385826771666132, 0.4176697321401328100 ) ) ;
#15894=UNCERTAINTY_MEASURE_WITH_UNIT (LENGTH_MEASURE( 1.000000000000000082E-05 ), #28354, 'distance_accuracy_value', 'NONE');
#15895=CARTESIAN_POINT ( 'NONE',  ( -0.1837270341207340729, 0.1283753931104746893, -0.1820866141732285504 ) ) ;
#15897=CARTESIAN_POINT ( 'NONE',  ( 1.397637795275591177, -0.5400638737290844871, 0.3530559997133364547 ) ) ;
#15898=CARTESIAN_POINT ( 'NONE',  ( -1.351706036745406347, -0.3690944881889763329, 0.3153832671262228327 ) ) ;
#15900=CARTESIAN_POINT ( 'NONE',  ( -0.7874015748031489847, -0.1870078740157480601, -0.3641732283464567677 ) ) ;
#15901=CARTESIAN_POINT ( 'NONE',  ( -0.006561679790025524116, -0.05778040916215560624, -0.4822834645669293319 ) ) ;
#15903=CARTESIAN_POINT ( 'NONE',  ( 0.3937007874015754361, -0.1870078740157480601, -0.3641732283464567677 ) ) ;
#15904=CARTESIAN_POINT ( 'NONE',  ( -0.4658792650918627265, -0.08942795157527998196, 0.3641732283464567121 ) ) ;
#15905=CARTESIAN_POINT ( 'NONE',  ( -0.9055118110236215490, -0.6692913385826771977, 8.415575281601705876E-17 ) ) ;
#15908=CARTESIAN_POINT ( 'NONE',  ( 0.3018372703412079971, 0.05413385826771626580, -0.4176697321401330321 ) ) ;
#15910=CARTESIAN_POINT ( 'NONE',  ( 1.377952755905512472, -0.6692913385826771977, 8.415575281601705876E-17 ) ) ;
#15911=CARTESIAN_POINT ( 'NONE',  ( -0.2755905511811018171, 0.1771653543307087630, 0.000000000000000000 ) ) ;
#15912=VECTOR ( 'NONE', #1400, 39.37007874015748143 ) ;
#15913=CARTESIAN_POINT ( 'NONE',  ( -0.1509186351706028884, -0.05778040916215522460, 0.4822834645669289988 ) ) ;
#15914=CARTESIAN_POINT ( 'NONE',  ( -1.601049868766403650, 0.2306618581243847221, -0.2411417322834647770 ) ) ;
#15915=CARTESIAN_POINT ( 'NONE',  ( 1.601049868766404982, -0.6046776061558809534, -0.2411417322834644161 ) ) ;
#15916=CARTESIAN_POINT ( 'NONE',  ( 1.469816272965879911, -0.6046776061558807314, 0.2411417322834647770 ) ) ;
#15917=CARTESIAN_POINT ( 'NONE',  ( -0.7480314960629914633, 0.1771653543307087630, 0.000000000000000000 ) ) ;
#15922=CARTESIAN_POINT ( 'NONE',  ( 1.627296587926509996, -0.5023911411419708095, 0.1820866141732285504 ) ) ;
#15923=CARTESIAN_POINT ( 'NONE',  ( 1.200787401574803681, -0.4536011799217368745, -0.2665933059059886201 ) ) ;
#15924=CARTESIAN_POINT ( 'NONE',  ( -1.614173228346456268, -0.6692913385826771977, 8.415575281601705876E-17 ) ) ;
#15925=CARTESIAN_POINT ( 'NONE',  ( 0.7874015748031503170, -0.1870078740157479769, 0.4822834645669291653 ) ) ;
#15927=CARTESIAN_POINT ( 'NONE',  ( 1.154855643044620184, -0.5023911411419708095, 0.1820866141732285504 ) ) ;
#15928=CARTESIAN_POINT ( 'NONE',  ( -0.08530183727034056085, -0.3162353388693405765, 0.4822834645669290543 ) ) ;
#15929=CARTESIAN_POINT ( 'NONE',  ( -0.4986876640419939388, 0.2306618581243847221, -0.2411417322834647770 ) ) ;
#15933=CARTESIAN_POINT ( 'NONE',  ( 0.4461942257217855201, -0.5023911411419708095, 0.1820866141732285504 ) ) ;
#15937=CARTESIAN_POINT ( 'NONE',  ( -0.5183727034120726440, -0.6692913385826773087, -0.1292274648535924053 ) ) ;
#15938=CARTESIAN_POINT ( 'NONE',  ( 0.8333333333333340365, 0.2952755905511810774, -0.1292274648535930714 ) ) ;
#15939=CARTESIAN_POINT ( 'NONE',  ( 0.1968503937007881344, -0.6692913385826771977, 8.415575281601705876E-17 ) ) ;
#15940=CARTESIAN_POINT ( 'NONE',  ( -0.3674540682414689785, 0.1283753931104748280, 0.1820866141732283561 ) ) ;
#15941=CARTESIAN_POINT ( 'NONE',  ( 0.8858267716535438430, 0.1660481256975885056, 0.3530559997133364547 ) ) ;
#15942=CARTESIAN_POINT ( 'NONE',  ( -0.9973753280839886548, 0.2306618581243848609, 0.2411417322834645549 ) ) ;
#15943=CARTESIAN_POINT ( 'NONE',  ( -0.4265091863517051496, 0.2952755905511810774, -0.1292274648535930714 ) ) ;
#15944=CARTESIAN_POINT ( 'NONE',  ( -0.7611548556430438595, 0.2306618581243848609, 0.2411417322834645549 ) ) ;
#15945=CARTESIAN_POINT ( 'NONE',  ( 1.377952755905512472, -0.6692913385826771977, 8.415575281601705876E-17 ) ) ;
#15946=CARTESIAN_POINT ( 'NONE',  ( 0.7808398950131240079, -0.3162353388693405765, 0.4822834645669290543 ) ) ;
#15947=CARTESIAN_POINT ( 'NONE',  ( 0.7152230971128616943, -0.05778040916215522460, 0.4822834645669289988 ) ) ;
#15949=CARTESIAN_POINT ( 'NONE',  ( 0.08530183727034192087, -0.08942795157527998196, 0.3641732283464567121 ) ) ;
#15950=ORIENTED_EDGE ( 'NONE', *, *, #21903, .T. ) ;
#15952=ORIENTED_EDGE ( 'NONE', *, *, #38343, .F. ) ;
#15953=CARTESIAN_POINT ( 'NONE',  ( -0.7283464566929126471, 0.07958543189024071263, -0.2665933059059888421 ) ) ;
#15954=CARTESIAN_POINT ( 'NONE',  ( -0.5446194225721777693, -0.05778040916215522460, 0.4822834645669289988 ) ) ;
#15956=CARTESIAN_POINT ( 'NONE',  ( -0.3740157480314953431, -0.5400638737290845981, -0.3530559997133363437 ) ) ;
#15957=CARTESIAN_POINT ( 'NONE',  ( -0.4265091863517051496, 0.2952755905511810774, -0.1292274648535930714 ) ) ;
#15958=CARTESIAN_POINT ( 'NONE',  ( -1.082677165354329896, -0.5400638737290845981, -0.3530559997133363437 ) ) ;
#15959=CARTESIAN_POINT ( 'NONE',  ( -1.213910761154854745, 0.2952755905511810774, -0.1292274648535930714 ) ) ;
#15960=CARTESIAN_POINT ( 'NONE',  ( 1.115485564304462551, -0.3690944881889765550, -0.3153832671262227771 ) ) ;
#15963=CARTESIAN_POINT ( 'NONE',  ( 0.5314960629921264834, 0.07958543189024071263, -0.2665933059059888421 ) ) ;
#15964=CARTESIAN_POINT ( 'NONE',  ( -0.1509186351706028884, -0.3162353388693409650, -0.4822834645669289433 ) ) ;
#15965=CARTESIAN_POINT ( 'NONE',  ( 0.1377952755905518800, 0.1660481256975883668, -0.3530559997133364547 ) ) ;
#15968=CARTESIAN_POINT ( 'NONE',  ( -0.6199123404867337150, -2.191421614605370878E-15, 0.4445507791589071167 ) ) ;
#15972=CARTESIAN_POINT ( 'NONE',  ( -0.6233595800524928121, -0.08942795157527998196, 0.3641732283464567121 ) ) ;
#15973=CARTESIAN_POINT ( 'NONE',  ( -0.8333333333333323711, -0.6692913385826773087, -0.1292274648535924053 ) ) ;
#15976=CARTESIAN_POINT ( 'NONE',  ( 1.561679790026247350, 0.05413385826771626580, -0.4176697321401330321 ) ) ;
#15977=CARTESIAN_POINT ( 'NONE',  ( 0.6758530183727039509, 0.2952755905511810774, -0.1292274648535930714 ) ) ;
#15978=CARTESIAN_POINT ( 'NONE',  ( 0.3346456692913393205, -0.5400638737290845981, -0.3530559997133363437 ) ) ;
#15979=CARTESIAN_POINT ( 'NONE',  ( -0.5118110236220466680, 0.1771653543307087630, 0.000000000000000000 ) ) ;
#15980=CARTESIAN_POINT ( 'NONE',  ( 0.01968503937007930540, 0.1660481256975885056, 0.3530559997133364547 ) ) ;
#15982=CARTESIAN_POINT ( 'NONE',  ( -0.1640419947506553400, -0.08942795157528024563, -0.3641732283464568787 ) ) ;
#15983=CARTESIAN_POINT ( 'NONE',  ( -0.4658792650918627265, -0.05778040916215522460, 0.4822834645669289988 ) ) ;
#15985=CARTESIAN_POINT ( 'NONE',  ( 1.541994750656168645, -0.5511811023622046335, 0.09757992244046803654 ) ) ;
#15986=CARTESIAN_POINT ( 'NONE',  ( 0.2230971128608929543, -0.004921259842519870586, -0.3153832671262229437 ) ) ;
#15988=CARTESIAN_POINT ( 'NONE',  ( -0.9776902887139098386, -0.6692913385826771977, 0.1292274648535927661 ) ) ;
#15989=CARTESIAN_POINT ( 'NONE',  ( -0.7414698162729651543, -0.5511811023622046335, 0.09757992244046803654 ) ) ;
#15990=CARTESIAN_POINT ( 'NONE',  ( -1.034719704380071992, 5.987370802660155681E-15, -0.3954985857520046388 ) ) ;
#15991=CARTESIAN_POINT ( 'NONE',  ( -1.325459317585300889, -0.4281496062992127816, -0.4176697321401328100 ) ) ;
#15992=CARTESIAN_POINT ( 'NONE',  ( -0.1246719160104980823, -0.6692913385826773087, -0.1292274648535924053 ) ) ;
#15997=CARTESIAN_POINT ( 'NONE',  ( 0.2690288713910767848, 0.1771653543307087630, 0.09757992244046791164 ) ) ;
#15998=CARTESIAN_POINT ( 'NONE',  ( 0.9842519685039375910, 0.2952755905511811885, 0.000000000000000000 ) ) ;
#15999=CARTESIAN_POINT ( 'NONE',  ( -1.371391076115484831, 0.1771653543307087075, -0.09757992244046823083 ) ) ;
#16000=CARTESIAN_POINT ( 'NONE',  ( 1.200787401574803681, 0.1660481256975885056, 0.3530559997133364547 ) ) ;
#16001=CARTESIAN_POINT ( 'NONE',  ( -1.666666666666665853, -0.004921259842519870586, -0.3153832671262229437 ) ) ;
#16002=CARTESIAN_POINT ( 'NONE',  ( -0.5314960629921254842, -0.5400638737290845981, -0.3530559997133363437 ) ) ;
#16003=CARTESIAN_POINT ( 'NONE',  ( 0.1115485564304470323, 0.1771653543307087630, 0.09757992244046791164 ) ) ;
#16005=CARTESIAN_POINT ( 'NONE',  ( 0.7349081364829402885, -0.5023911411419708095, -0.1820866141732282451 ) ) ;
#16006=CARTESIAN_POINT ( 'NONE',  ( 0.006561679790026889343, -0.3162353388693409650, -0.4822834645669289433 ) ) ;
#16009=CARTESIAN_POINT ( 'NONE',  ( -1.266404199475064773, -0.3162353388693405765, 0.4822834645669290543 ) ) ;
#16011=CARTESIAN_POINT ( 'NONE',  ( 0.9645669291338588858, 0.07958543189024085140, 0.2665933059059887866 ) ) ;
#16012=CARTESIAN_POINT ( 'NONE',  ( -0.1312335958005241554, -0.6046776061558809534, -0.2411417322834644161 ) ) ;
#16013=CARTESIAN_POINT ( 'NONE',  ( -0.1246719160104980823, -0.6692913385826773087, -0.1292274648535924053 ) ) ;
#16014=CARTESIAN_POINT ( 'NONE',  ( -0.4199475065616791736, -0.5023911411419708095, 0.1820866141732285504 ) ) ;
#16015=CARTESIAN_POINT ( 'NONE',  ( 0.9776902887139113929, 0.2066929133858267931, 0.1054918080437490802 ) ) ;
#16016=CARTESIAN_POINT ( 'NONE',  ( -0.5643044619422565855, -0.3690944881889763329, 0.3153832671262228327 ) ) ;
#16017=CARTESIAN_POINT ( 'NONE',  ( 0.1771653543307093182, -0.5400638737290845981, -0.3530559997133363437 ) ) ;
#16018=CARTESIAN_POINT ( 'NONE',  ( -0.6036745406824141069, 0.1283753931104748280, 0.1820866141732283561 ) ) ;
#16020=CARTESIAN_POINT ( 'NONE',  ( -1.272965879265091305, 0.05413385826771626580, -0.4176697321401330321 ) ) ;
#16021=ORIENTED_EDGE ( 'NONE', *, *, #1687, .F. ) ;
#16022=CARTESIAN_POINT ( 'NONE',  ( -1.279527559055116948, -0.4536011799217367080, 0.2665933059059888421 ) ) ;
#16023=CARTESIAN_POINT ( 'NONE',  ( -0.5380577427821514602, -0.4281496062992127816, -0.4176697321401328100 ) ) ;
#16025=CARTESIAN_POINT ( 'NONE',  ( -1.227034120734907141, -0.6692913385826773087, -0.1292274648535924053 ) ) ;
#16027=CARTESIAN_POINT ( 'NONE',  ( 1.181102362204725198, -0.1870078740157479769, 0.4822834645669291653 ) ) ;
#16028=CARTESIAN_POINT ( 'NONE',  ( 0.7480314960629927956, 0.2952755905511811885, 0.000000000000000000 ) ) ;
#16029=CARTESIAN_POINT ( 'NONE',  ( -0.2486400153428821869, 2.660739321503277841E-15, -0.3464511005275191513 ) ) ;
#16031=CARTESIAN_POINT ( 'NONE',  ( -1.692913385826770645, 0.2952755905511811885, 0.000000000000000000 ) ) ;
#16034=CARTESIAN_POINT ( 'NONE',  ( -0.3477690288713902178, 0.1771653543307087075, -0.09757992244046823083 ) ) ;
#16037=CARTESIAN_POINT ( 'NONE',  ( 0.9055118110236227702, -0.6692913385826771977, 8.415575281601705876E-17 ) ) ;
#16038=CARTESIAN_POINT ( 'NONE',  ( -0.5052493438320203589, -0.6692913385826771977, 0.1292274648535927661 ) ) ;
#16039=CARTESIAN_POINT ( 'NONE',  ( -0.9186351706036736120, -0.6046776061558809534, -0.2411417322834644161 ) ) ;
#16040=CARTESIAN_POINT ( 'NONE',  ( 1.620734908136483465, -0.6692913385826771977, 0.1292274648535927661 ) ) ;
#16041=CARTESIAN_POINT ( 'NONE',  ( -1.240157480314959759, -0.4536011799217368745, -0.2665933059059886201 ) ) ;
#16043=CARTESIAN_POINT ( 'NONE',  ( 0.2230971128608932319, -0.4281496062992124485, 0.4176697321401328655 ) ) ;
#16044=CARTESIAN_POINT ( 'NONE',  ( -0.8792650918635160906, -0.4281496062992124485, 0.4176697321401328655 ) ) ;
#16046=CARTESIAN_POINT ( 'NONE',  ( -1.213910761154854745, -0.6692913385826771977, 0.1292274648535927661 ) ) ;
#16048=CARTESIAN_POINT ( 'NONE',  ( 0.9448818897637802916, -0.1870078740157480879, -0.4822834645669291653 ) ) ;
#16049=CARTESIAN_POINT ( 'NONE',  ( 1.076115485564305141, 0.1283753931104746893, -0.1820866141732285504 ) ) ;
#16050=ORIENTED_EDGE ( 'NONE', *, *, #42486, .F. ) ;
#16052=CARTESIAN_POINT ( 'NONE',  ( -0.2755905511811015396, -0.6692913385826771977, 8.415575281601705876E-17 ) ) ;
#16053=ORIENTED_EDGE ( 'NONE', *, *, #38721, .T. ) ;
#16054=CARTESIAN_POINT ( 'NONE',  ( 0.1902887139107617975, 0.1771653543307087630, 0.09757992244046791164 ) ) ;
#16055=CARTESIAN_POINT ( 'NONE',  ( -1.200787401574802349, 0.1660481256975883668, -0.3530559997133364547 ) ) ;
#16056=CARTESIAN_POINT ( 'NONE',  ( 0.7874015748031503170, -0.1870078740157479769, 0.4822834645669291653 ) ) ;
#16057=CARTESIAN_POINT ( 'NONE',  ( 1.043307086614173818, -0.5400638737290845981, -0.3530559997133363437 ) ) ;
#16058=CARTESIAN_POINT ( 'NONE',  ( -0.3018372703412066094, 0.05413385826771666132, 0.4176697321401328100 ) ) ;
#16060=CARTESIAN_POINT ( 'NONE',  ( -0.7152230971128602510, -0.3162353388693405765, 0.4822834645669290543 ) ) ;
#16062=CARTESIAN_POINT ( 'NONE',  ( -1.496062992125983815, -0.1870078740157480879, -0.4822834645669291653 ) ) ;
#16063=CARTESIAN_POINT ( 'NONE',  ( -0.6364829396325453192, -0.05778040916215560624, -0.4822834645669293319 ) ) ;
#16064=CARTESIAN_POINT ( 'NONE',  ( -0.3805774278215216522, -0.004921259842519576551, 0.3153832671262227771 ) ) ;
#16065=CARTESIAN_POINT ( 'NONE',  ( 1.364829396325460076, 0.2306618581243848609, 0.2411417322834645549 ) ) ;
#16066=CARTESIAN_POINT ( 'NONE',  ( 1.423884514435696413, -0.3162353388693409650, -0.4822834645669289433 ) ) ;
#16067=CARTESIAN_POINT ( 'NONE',  ( -0.8661417322834640276, -0.1870078740157480879, -0.4822834645669291653 ) ) ;
#16069=CARTESIAN_POINT ( 'NONE',  ( 0.7742782152230978099, -0.4281496062992124485, 0.4176697321401328655 ) ) ;
#16071=CARTESIAN_POINT ( 'NONE',  ( -0.5380577427821514602, 0.05413385826771666132, 0.4176697321401328100 ) ) ;
#16072=CARTESIAN_POINT ( 'NONE',  ( -1.069553805774277722, -0.5511811023622048555, -0.09757992244046775898 ) ) ;
#16073=CARTESIAN_POINT ( 'NONE',  ( 0.8005249343832028242, -0.3690944881889765550, -0.3153832671262227771 ) ) ;
#16075=CARTESIAN_POINT ( 'NONE',  ( 1.187664041994751285, -0.08942795157527998196, 0.3641732283464567121 ) ) ;
#16076=VECTOR ( 'NONE', #3016, 39.37007874015748143 ) ;
#16077=CARTESIAN_POINT ( 'NONE',  ( 0.8858267716535438430, -0.5400638737290845981, -0.3530559997133363437 ) ) ;
#16079=CARTESIAN_POINT ( 'NONE',  ( -0.4133858267716528645, 0.1660481256975883668, -0.3530559997133364547 ) ) ;
#16081=CARTESIAN_POINT ( 'NONE',  ( 1.174540682414699111, -0.08942795157528024563, -0.3641732283464568787 ) ) ;
#16082=CARTESIAN_POINT ( 'NONE',  ( -0.5905511811023615998, 0.2952755905511811885, 0.000000000000000000 ) ) ;
#16084=CARTESIAN_POINT ( 'NONE',  ( 1.469816272965879911, -0.6046776061558807314, 0.2411417322834647770 ) ) ;
#16085=CARTESIAN_POINT ( 'NONE',  ( -0.03937007874015669567, -0.6692913385826771977, 8.415575281601705876E-17 ) ) ;
#16086=CARTESIAN_POINT ( 'NONE',  ( 0.6036745406824154392, 0.1283753931104746893, -0.1820866141732285504 ) ) ;
#16088=CARTESIAN_POINT ( 'NONE',  ( 0.01968503937007957949, -0.4536011799217368745, -0.2665933059059886201 ) ) ;
#16091=CARTESIAN_POINT ( 'NONE',  ( 0.5643044619422579178, 0.05413385826771666132, 0.4176697321401328100 ) ) ;
#16093=CARTESIAN_POINT ( 'NONE',  ( 1.555118110236221041, 0.07958543189024071263, -0.2665933059059888421 ) ) ;
#16095=CARTESIAN_POINT ( 'NONE',  ( -0.04593175853018302557, -0.5511811023622048555, -0.09757992244046775898 ) ) ;
#16096=CARTESIAN_POINT ( 'NONE',  ( -0.03280839895013062252, 0.2952755905511810774, -0.1292274648535930714 ) ) ;
#16097=CARTESIAN_POINT ( 'NONE',  ( 1.338582677165355062, -0.1870078740157479769, 0.3641732283464567677 ) ) ;
#16098=CARTESIAN_POINT ( 'NONE',  ( -1.555118110236219930, 0.07958543189024085140, 0.2665933059059887866 ) ) ;
#16099=CARTESIAN_POINT ( 'NONE',  ( -1.581364829396324945, -0.3162353388693405765, 0.4822834645669290543 ) ) ;
#16100=CARTESIAN_POINT ( 'NONE',  ( 0.7217847769028878924, 0.05413385826771666132, 0.4176697321401328100 ) ) ;
#16101=CARTESIAN_POINT ( 'NONE',  ( 1.082677165354331228, 0.1660481256975883668, -0.3530559997133364547 ) ) ;
#16103=CARTESIAN_POINT ( 'NONE',  ( 0.3149606299212603933, -0.1870078740157479769, 0.4822834645669291653 ) ) ;
#16104=CARTESIAN_POINT ( 'NONE',  ( 1.338582677165355062, -0.1870078740157479769, 0.4822834645669291653 ) ) ;
#16105=CARTESIAN_POINT ( 'NONE',  ( 0.9448818897637802916, -0.1870078740157480879, -0.4822834645669291653 ) ) ;
#16107=B_SPLINE_CURVE_WITH_KNOTS ( 'NONE', 3,
 ( #66111, #66949, #41263, #2553, #21486, #53038, #1311 ),
 .UNSPECIFIED., .F., .F.,
 ( 4, 3, 4 ),
 ( 1.734723475976806902E-18, 0.001246232571205225376, 0.002492492258783241162 ),
 .UNSPECIFIED. ) ;
#16108=CARTESIAN_POINT ( 'NONE',  ( 0.9383202099737538715, -0.08942795157528024563, -0.3641732283464568787 ) ) ;
#16109=CARTESIAN_POINT ( 'NONE',  ( 1.456692913385827515, -0.6692913385826771977, 8.415575281601705876E-17 ) ) ;
#16110=CARTESIAN_POINT ( 'NONE',  ( -0.8595800524934373854, -0.08942795157527998196, 0.3641732283464567121 ) ) ;
#16111=CARTESIAN_POINT ( 'NONE',  ( 0.3740157480314966754, 0.07958543189024071263, -0.2665933059059888421 ) ) ;
#16112=CARTESIAN_POINT ( 'NONE',  ( 0.1377952755905518800, 0.1660481256975883668, -0.3530559997133364547 ) ) ;
#16113=CARTESIAN_POINT ( 'NONE',  ( 0.7742782152230978099, -0.4281496062992124485, 0.4176697321401328655 ) ) ;
#16114=CARTESIAN_POINT ( 'NONE',  ( -0.5118110236220466680, 0.2952755905511811885, 0.000000000000000000 ) ) ;
#16115=CARTESIAN_POINT ( 'NONE',  ( 0.07217847769028949700, -0.08942795157528024563, -0.3641732283464568787 ) ) ;
#16116=CARTESIAN_POINT ( 'NONE',  ( 0.8267716535433077274, 0.2952755905511811885, 0.000000000000000000 ) ) ;
#16118=CARTESIAN_POINT ( 'NONE',  ( -0.8136482939632537770, -0.6046776061558807314, 0.2411417322834647770 ) ) ;
#16122=CARTESIAN_POINT ( 'NONE',  ( -0.9776902887139098386, 0.2952755905511810774, -0.1292274648535930714 ) ) ;
#16123=CARTESIAN_POINT ( 'NONE',  ( -0.6299212598425188991, -0.1870078740157479769, 0.4822834645669291653 ) ) ;
#16126=VERTEX_POINT ( 'NONE', #28599 ) ;
#16127=CARTESIAN_POINT ( 'NONE',  ( 0.5643044619422579178, -0.004921259842519576551, 0.3153832671262227771 ) ) ;
#16129=CARTESIAN_POINT ( 'NONE',  ( 0.9251968503937015864, -0.5400638737290844871, 0.3530559997133364547 ) ) ;
#16131=CARTESIAN_POINT ( 'NONE',  ( -1.194225721784776262, -0.004921259842519870586, -0.3153832671262229437 ) ) ;
#16132=CARTESIAN_POINT ( 'NONE',  ( 1.555118110236221041, 0.1660481256975883668, -0.3530559997133364547 ) ) ;
#16134=CARTESIAN_POINT ( 'NONE',  ( -1.417322834645668772, -0.1870078740157479769, 0.4822834645669291653 ) ) ;
#16135=CARTESIAN_POINT ( 'NONE',  ( 0.5118110236220480003, -0.6692913385826771977, 8.415575281601705876E-17 ) ) ;
#16137=CARTESIAN_POINT ( 'NONE',  ( 0.07874015748031558404, -0.1870078740157479769, 0.4822834645669291653 ) ) ;
#16138=CARTESIAN_POINT ( 'NONE',  ( -0.7742782152230965886, -0.004921259842519576551, 0.3153832671262227771 ) ) ;
#16139=CARTESIAN_POINT ( 'NONE',  ( 0.8267716535433077274, 0.2952755905511811885, 0.000000000000000000 ) ) ;
#16140=CARTESIAN_POINT ( 'NONE',  ( -0.1968503937007867743, -0.6692913385826771977, 8.415575281601705876E-17 ) ) ;
#16142=CARTESIAN_POINT ( 'NONE',  ( -1.191111281560509383, -2.567464376874931580E-15, -0.4445507791589072832 ) ) ;
#16145=CARTESIAN_POINT ( 'NONE',  ( 1.043307086614173818, 0.1660481256975885056, 0.3530559997133364547 ) ) ;
#16146=CARTESIAN_POINT ( 'NONE',  ( 0.1706036745406830368, 0.05413385826771666132, 0.4176697321401328100 ) ) ;
#16147=CARTESIAN_POINT ( 'NONE',  ( -0.9580052493438311334, 0.05413385826771626580, -0.4176697321401330321 ) ) ;
#16148=CARTESIAN_POINT ( 'NONE',  ( 1.154855643044620184, 0.2306618581243847221, -0.2411417322834647770 ) ) ;
#16149=CARTESIAN_POINT ( 'NONE',  ( 0.4265091863517067594, 0.2952755905511811885, 0.1292274648535926551 ) ) ;
#16151=CARTESIAN_POINT ( 'NONE',  ( -0.4461942257217840213, 0.2306618581243848609, 0.2411417322834645549 ) ) ;
#16152=CARTESIAN_POINT ( 'NONE',  ( 0.7283464566929143125, 0.1660481256975885056, 0.3530559997133364547 ) ) ;
#16153=CARTESIAN_POINT ( 'NONE',  ( -0.07217847769028787330, -0.05778040916215522460, 0.4822834645669289988 ) ) ;
#16154=CARTESIAN_POINT ( 'NONE',  ( 0.7086614173228353852, -0.1870078740157479769, 0.3641732283464567677 ) ) ;
#16155=CARTESIAN_POINT ( 'NONE',  ( -1.318897637795274802, -0.5400638737290845981, -0.3530559997133363437 ) ) ;
#16157=CARTESIAN_POINT ( 'NONE',  ( 0.5183727034120741983, 0.2952755905511810774, -0.1292274648535930714 ) ) ;
#16161=EDGE_CURVE ( 'NONE', #72462, #23065, #72276, .T. ) ;
#16163=CARTESIAN_POINT ( 'NONE',  ( 1.102362204724410155, -0.1870078740157480879, -0.4822834645669291653 ) ) ;
#16164=CARTESIAN_POINT ( 'NONE',  ( 0.5839895013123367340, -0.5511811023622048555, -0.09757992244046775898 ) ) ;
#16173=CARTESIAN_POINT ( 'NONE',  ( -0.8398950131233585692, 0.2306618581243848609, 0.2411417322834645549 ) ) ;
#16174=CARTESIAN_POINT ( 'NONE',  ( -0.8267716535433065062, -0.6692913385826771977, 8.415575281601705876E-17 ) ) ;
#16175=CARTESIAN_POINT ( 'NONE',  ( 0.5774278215223103139, -0.6046776061558809534, -0.2411417322834644161 ) ) ;
#16177=CARTESIAN_POINT ( 'NONE',  ( 1.286089238845145033, 0.2306618581243848609, 0.2411417322834645549 ) ) ;
#16180=CARTESIAN_POINT ( 'NONE',  ( 1.601049868766404982, -0.5023911411419708095, -0.1820866141732282451 ) ) ;
#16182=CARTESIAN_POINT ( 'NONE',  ( -1.364829396325458521, -0.5023911411419708095, 0.1820866141732285504 ) ) ;
#16184=CARTESIAN_POINT ( 'NONE',  ( 0.1246719160104994284, 0.2952755905511810774, -0.1292274648535930714 ) ) ;
#16185=CARTESIAN_POINT ( 'NONE',  ( 1.653543307086614789, -0.1870078740157479769, 0.4822834645669291653 ) ) ;
#16187=CARTESIAN_POINT ( 'NONE',  ( -1.141732283464566011, -0.5511811023622047445, 6.969142054262312111E-17 ) ) ;
#16188=CARTESIAN_POINT ( 'NONE',  ( 0.2296587926509192634, -0.3162353388693405765, 0.4822834645669290543 ) ) ;
#16189=CARTESIAN_POINT ( 'NONE',  ( 1.246719160104987623, -0.3690944881889763329, 0.3153832671262228327 ) ) ;
#16191=VECTOR ( 'NONE', #6634, 39.37007874015748854 ) ;
#16192=CARTESIAN_POINT ( 'NONE',  ( -1.174540682414697335, -0.2845877964562161244, -0.3641732283464567121 ) ) ;
#16193=CARTESIAN_POINT ( 'NONE',  ( 1.332020997375329197, -0.3162353388693405765, 0.4822834645669290543 ) ) ;
#16195=CARTESIAN_POINT ( 'NONE',  ( -0.3280839895013117347, -0.4281496062992124485, 0.4176697321401328655 ) ) ;
#16196=CARTESIAN_POINT ( 'NONE',  ( -1.351706036745406347, -0.3690944881889763329, 0.3153832671262228327 ) ) ;
#16197=CARTESIAN_POINT ( 'NONE',  ( -0.1377952755905504645, 0.07958543189024085140, 0.2665933059059887866 ) ) ;
#16198=CARTESIAN_POINT ( 'NONE',  ( -0.5511811023622041894, -0.1870078740157480879, -0.4822834645669291653 ) ) ;
#16199=CARTESIAN_POINT ( 'NONE',  ( -1.489501312335957062, -0.08942795157527998196, 0.3641732283464567121 ) ) ;
#16201=CARTESIAN_POINT ( 'NONE',  ( 0.4527559055118117182, -0.5400638737290844871, 0.3530559997133364547 ) ) ;
#16202=CARTESIAN_POINT ( 'NONE',  ( 0.4043999638110887807, 7.699586553780600482E-16, 0.4118484887281971263 ) ) ;
#16204=CARTESIAN_POINT ( 'NONE',  ( -1.194225721784776262, 0.05413385826771626580, -0.4176697321401330321 ) ) ;
#16205=CARTESIAN_POINT ( 'NONE',  ( -0.6627296587926503335, -0.5511811023622046335, 0.09757992244046803654 ) ) ;
#16206=DIRECTION ( 'NONE',  ( -1.000000000000000000, 0.000000000000000000, 0.000000000000000000 ) ) ;
#16207=CARTESIAN_POINT ( 'NONE',  ( 0.03937007874015833325, -0.6692913385826771977, 8.415575281601705876E-17 ) ) ;
#16208=CARTESIAN_POINT ( 'NONE',  ( 0.3346456692913393205, -0.4536011799217368745, -0.2665933059059886201 ) ) ;
#16209=CARTESIAN_POINT ( 'NONE',  ( -0.9251968503937002541, 0.07958543189024085140, 0.2665933059059887866 ) ) ;
#16210=CARTESIAN_POINT ( 'NONE',  ( -1.640419947506561060, -0.4281496062992127816, -0.4176697321401328100 ) ) ;
#16211=CARTESIAN_POINT ( 'NONE',  ( -1.522309711286088607, 0.2306618581243847221, -0.2411417322834647770 ) ) ;
#16212=CARTESIAN_POINT ( 'NONE',  ( 1.325459317585302665, -0.4281496062992124485, 0.4176697321401328655 ) ) ;
#16213=CARTESIAN_POINT ( 'NONE',  ( -1.604771003085130765, 0.4934440724007108092, -0.1466069496707737840 ) ) ;
#16214=CARTESIAN_POINT ( 'NONE',  ( 0.9842519685039378130, -0.5511811023622047445, 6.969142054262312111E-17 ) ) ;
#16215=CARTESIAN_POINT ( 'NONE',  ( 0.6824146981627303710, -0.6046776061558807314, 0.2411417322834647770 ) ) ;
#16217=CARTESIAN_POINT ( 'NONE',  ( 1.397637795275591177, -0.4536011799217367080, 0.2665933059059888421 ) ) ;
#16219=CARTESIAN_POINT ( 'NONE',  ( -1.332020997375327642, -0.05778040916215522460, 0.4822834645669289988 ) ) ;
#16220=ADVANCED_FACE ( 'NONE', ( #40809 ), #8828, .F. ) ;
#16221=CARTESIAN_POINT ( 'NONE',  ( -0.9842519685039360366, 0.2952755905511811885, 0.000000000000000000 ) ) ;
#16222=CARTESIAN_POINT ( 'NONE',  ( 0.3346456692913390985, 0.1660481256975885056, 0.3530559997133364547 ) ) ;
#16223=CARTESIAN_POINT ( 'NONE',  ( -1.312335958005248715, -0.5023911411419708095, -0.1820866141732282451 ) ) ;
#16225=CARTESIAN_POINT ( 'NONE',  ( -1.646981627296586703, -0.3162353388693409650, -0.4822834645669289433 ) ) ;
#16226=CARTESIAN_POINT ( 'NONE',  ( 0.3674540682414705883, -0.6046776061558807314, 0.2411417322834647770 ) ) ;
#16227=CARTESIAN_POINT ( 'NONE',  ( 0.7545931758530188826, -0.6692913385826771977, 0.1292274648535927661 ) ) ;
#16228=CARTESIAN_POINT ( 'NONE',  ( 1.568241469816273659, -0.05778040916215560624, -0.4822834645669293319 ) ) ;
#16232=CARTESIAN_POINT ( 'NONE',  ( -0.7461015445742957830, 1.969952063615671101, -0.5309055118110235227 ) ) ;
#16234=CARTESIAN_POINT ( 'NONE',  ( -0.1049868766404193215, 0.1283753931104746893, -0.1820866141732285504 ) ) ;
#16235=CARTESIAN_POINT ( 'NONE',  ( -0.4855643044619415427, -0.4281496062992124485, 0.4176697321401328655 ) ) ;
#16236=CARTESIAN_POINT ( 'NONE',  ( 0.9514435695538062676, -0.05778040916215522460, 0.4822834645669289988 ) ) ;
#16238=CARTESIAN_POINT ( 'NONE',  ( -0.07217847769028787330, -0.08942795157527998196, 0.3641732283464567121 ) ) ;
#16239=( BOUNDED_CURVE ( )  B_SPLINE_CURVE ( 3, ( #77222, #58683, #12838, #45629 ),
 .UNSPECIFIED., .F., .F. ) 
 B_SPLINE_CURVE_WITH_KNOTS ( ( 4, 4 ),
 ( 3.539787554096436306, 4.423914789137159076 ),
 .UNSPECIFIED. ) 
 CURVE ( )  GEOMETRIC_REPRESENTATION_ITEM ( )  RATIONAL_B_SPLINE_CURVE ( ( 1.000000000000000000, 0.9359138408343250504, 0.9359138408343250504, 1.000000000000000000 ) ) 
 REPRESENTATION_ITEM ( '' )  );
#16240=CARTESIAN_POINT ( 'NONE',  ( -1.069553805774277722, -0.6692913385826773087, -0.1292274648535924053 ) ) ;
#16241=CARTESIAN_POINT ( 'NONE',  ( 1.108923884514436242, -0.05778040916215522460, 0.4822834645669289988 ) ) ;
#16244=CYLINDRICAL_SURFACE ( 'NONE', #11641, 1.181102362204724310 ) ;
#16247=CARTESIAN_POINT ( 'NONE',  ( 1.102362204724410155, -0.1870078740157479769, 0.4822834645669291653 ) ) ;
#16248=CARTESIAN_POINT ( 'NONE',  ( -1.522309711286088607, 0.2306618581243847221, -0.2411417322834647770 ) ) ;
#16249=CARTESIAN_POINT ( 'NONE',  ( -1.456692913385826182, 0.1771653543307087630, 0.000000000000000000 ) ) ;
#16250=CARTESIAN_POINT ( 'NONE',  ( -1.607611548556429737, 0.2952755905511810774, -0.1292274648535930714 ) ) ;
#16252=CARTESIAN_POINT ( 'NONE',  ( -0.9973753280839886548, 0.1539470093639523085, 0.1968503937007873850 ) ) ;
#16253=CARTESIAN_POINT ( 'NONE',  ( 1.345144356955381593, -0.05778040916215522460, 0.4822834645669289988 ) ) ;
#16255=CARTESIAN_POINT ( 'NONE',  ( 0.1049868766404206816, -0.6046776061558809534, -0.2411417322834644161 ) ) ;
#16256=CARTESIAN_POINT ( 'NONE',  ( -0.6824146981627291497, -0.6046776061558809534, -0.2411417322834644161 ) ) ;
#16258=CARTESIAN_POINT ( 'NONE',  ( 1.601049868766404982, 0.2306618581243848609, 0.2411417322834645549 ) ) ;
#16260=CARTESIAN_POINT ( 'NONE',  ( 0.2887139107611556010, -0.6046776061558807314, 0.2411417322834647770 ) ) ;
#16263=CARTESIAN_POINT ( 'NONE',  ( -1.036745406824146176, -0.3690944881889763329, 0.3153832671262228327 ) ) ;
#16266=EDGE_LOOP ( 'NONE', ( #32776, #18914, #6670, #52539 ) ) ;
#16268=CARTESIAN_POINT ( 'NONE',  ( -1.528871391076114250, 0.2952755905511810774, -0.1292274648535930714 ) ) ;
#16270=CARTESIAN_POINT ( 'NONE',  ( 1.686351706036745890, 0.1771653543307087630, 0.09757992244046791164 ) ) ;
#16271=CARTESIAN_POINT ( 'NONE',  ( -1.640419947506561060, -0.4281496062992127816, -0.4176697321401328100 ) ) ;
#16272=CARTESIAN_POINT ( 'NONE',  ( 0.4330708661417329575, 0.2952755905511811885, 0.000000000000000000 ) ) ;
#16274=DIRECTION ( 'NONE',  ( 0.000000000000000000, 0.000000000000000000, -1.000000000000000000 ) ) ;
#16276=CARTESIAN_POINT ( 'NONE',  ( -0.4265091863517051496, -0.5511811023622046335, 0.09757992244046803654 ) ) ;
#16277=CARTESIAN_POINT ( 'NONE',  ( -0.7677165354330699465, 0.07958543189024085140, 0.2665933059059887866 ) ) ;
#16278=CARTESIAN_POINT ( 'NONE',  ( -1.279527559055116948, 0.1660481256975883668, -0.3530559997133364547 ) ) ;
#16279=CARTESIAN_POINT ( 'NONE',  ( 0.3937007874015754361, -0.1870078740157480879, -0.4822834645669291653 ) ) ;
#16280=CARTESIAN_POINT ( 'NONE',  ( -1.417322834645668772, -0.1870078740157480879, -0.4822834645669291653 ) ) ;
#16283=ORIENTED_EDGE ( 'NONE', *, *, #45519, .F. ) ;
#16284=CARTESIAN_POINT ( 'NONE',  ( -1.299212598425196097, 0.2952755905511811885, 0.000000000000000000 ) ) ;
#16288=CYLINDRICAL_SURFACE ( 'NONE', #82842, 0.3937007874015748254 ) ;
#16291=CARTESIAN_POINT ( 'NONE',  ( -0.9055118110236215490, -0.6692913385826771977, 8.415575281601705876E-17 ) ) ;
#16292=CARTESIAN_POINT ( 'NONE',  ( 1.620734908136483465, -0.6692913385826771977, 0.1292274648535927661 ) ) ;
#16293=CARTESIAN_POINT ( 'NONE',  ( -0.7426113562967729953, 2.199547029020892275, -0.5309055118110235227 ) ) ;
#16296=CARTESIAN_POINT ( 'NONE',  ( -1.535433070866141225, 0.2952755905511811885, 0.000000000000000000 ) ) ;
#16297=CARTESIAN_POINT ( 'NONE',  ( -0.7611548556430438595, 0.2306618581243848609, 0.2411417322834645549 ) ) ;
#16299=CARTESIAN_POINT ( 'NONE',  ( -0.1706036745406816491, -0.3690944881889763329, 0.3153832671262228327 ) ) ;
#16302=CARTESIAN_POINT ( 'NONE',  ( -0.2755905511811015396, -0.5511811023622047445, 6.969142054262312111E-17 ) ) ;
#16303=CARTESIAN_POINT ( 'NONE',  ( 0.9645669291338588858, 0.07958543189024085140, 0.2665933059059887866 ) ) ;
#16304=CARTESIAN_POINT ( 'NONE',  ( 0.4855643044619428750, 0.05413385826771666132, 0.4176697321401328100 ) ) ;
#16305=CARTESIAN_POINT ( 'NONE',  ( -0.3346456692913377662, 0.07958543189024071263, -0.2665933059059888421 ) ) ;
#16307=CARTESIAN_POINT ( 'NONE',  ( 1.377952755905512472, -0.6692913385826771977, 8.415575281601705876E-17 ) ) ;
#16308=CARTESIAN_POINT ( 'NONE',  ( -1.181102362204723644, -0.1870078740157479769, 0.3641732283464567677 ) ) ;
#16310=CARTESIAN_POINT ( 'NONE',  ( 0.2099737532808405305, 0.2306618581243847221, -0.2411417322834647770 ) ) ;
#16311=CARTESIAN_POINT ( 'NONE',  ( -0.6167979002624665030, -0.4281496062992127816, -0.4176697321401328100 ) ) ;
#16313=CARTESIAN_POINT ( 'NONE',  ( 0.5905511811023629321, -0.5511811023622047445, 6.969142054262312111E-17 ) ) ;
#16314=CARTESIAN_POINT ( 'NONE',  ( -0.2755905511811018171, 0.1771653543307087630, 0.000000000000000000 ) ) ;
#16315=CARTESIAN_POINT ( 'NONE',  ( -0.6824146981627288167, 0.2306618581243848609, 0.2411417322834645549 ) ) ;
#16317=DIRECTION ( 'NONE',  ( -3.096699300667737957E-16, 1.000000000000000000, -0.000000000000000000 ) ) ;
#16318=CARTESIAN_POINT ( 'NONE',  ( 0.3280839895013130669, -0.4281496062992127816, -0.4176697321401328100 ) ) ;
#16319=CIRCLE ( 'NONE', #2850, 3.425196850393701808 ) ;
#16321=CARTESIAN_POINT ( 'NONE',  ( 1.594488188976378673, 0.1660481256975885056, 0.3530559997133364547 ) ) ;
#16322=CARTESIAN_POINT ( 'NONE',  ( -0.1640419947506555343, -0.2845877964562159024, 0.3641732283464567677 ) ) ;
#16323=CARTESIAN_POINT ( 'NONE',  ( -0.5314960629921254842, -0.5400638737290845981, -0.3530559997133363437 ) ) ;
#16324=CARTESIAN_POINT ( 'NONE',  ( 0.4606732211678792877, 2.401574803149606030, 0.5309055118110234117 ) ) ;
#16325=CARTESIAN_POINT ( 'NONE',  ( 1.633858267716535639, -0.5400638737290844871, 0.3530559997133364547 ) ) ;
#16326=CARTESIAN_POINT ( 'NONE',  ( 1.318897637795276356, -0.5400638737290844871, 0.3530559997133364547 ) ) ;
#16328=CARTESIAN_POINT ( 'NONE',  ( -0.7414698162729651543, 0.1771653543307087075, -0.09757992244046823083 ) ) ;
#16333=CARTESIAN_POINT ( 'NONE',  ( 1.417322834645670104, -0.1870078740157480601, -0.3641732283464567677 ) ) ;
#16334=CARTESIAN_POINT ( 'NONE',  ( 1.312335958005249825, 0.1283753931104746893, -0.1820866141732285504 ) ) ;
#16335=CARTESIAN_POINT ( 'NONE',  ( 0.9514435695538062676, -0.05778040916215522460, 0.4822834645669289988 ) ) ;
#16336=CARTESIAN_POINT ( 'NONE',  ( -1.719160104986876103, 0.05413385826771666132, 0.4176697321401328100 ) ) ;
#16337=CARTESIAN_POINT ( 'NONE',  ( 1.030183727034121421, -0.3162353388693409650, -0.4822834645669289433 ) ) ;
#16339=CARTESIAN_POINT ( 'NONE',  ( 1.135170603674541256, -0.5511811023622048555, -0.09757992244046775898 ) ) ;
#16340=CARTESIAN_POINT ( 'NONE',  ( -0.05905511811023545637, 0.1660481256975885056, 0.3530559997133364547 ) ) ;
#16341=CARTESIAN_POINT ( 'NONE',  ( -0.6233595800524928121, -0.3162353388693409650, -0.4822834645669289433 ) ) ;
#16342=CARTESIAN_POINT ( 'NONE',  ( 1.627296587926509996, -0.6046776061558807314, 0.2411417322834647770 ) ) ;
#16345=CARTESIAN_POINT ( 'NONE',  ( 0.4986876640419954376, 0.1283753931104748280, 0.1820866141732283561 ) ) ;
#16348=ORIENTED_EDGE ( 'NONE', *, *, #72224, .F. ) ;
#16349=CARTESIAN_POINT ( 'NONE',  ( -0.4986876640419942164, -0.6046776061558807314, 0.2411417322834647770 ) ) ;
#16350=CARTESIAN_POINT ( 'NONE',  ( -0.2821522309711278487, -0.6692913385826773087, -0.1292274648535924053 ) ) ;
#16351=CARTESIAN_POINT ( 'NONE',  ( -0.3608923884514428360, 0.2952755905511811885, 0.1292274648535926551 ) ) ;
#16352=CARTESIAN_POINT ( 'NONE',  ( 0.5971128608923891301, 0.2952755905511810774, -0.1292274648535930714 ) ) ;
#16353=CARTESIAN_POINT ( 'NONE',  ( -1.076115485564303809, -0.6046776061558809534, -0.2411417322834644161 ) ) ;
#16354=CARTESIAN_POINT ( 'NONE',  ( -0.3280839895013117347, -0.4281496062992124485, 0.4176697321401328655 ) ) ;
#16355=CARTESIAN_POINT ( 'NONE',  ( 1.272965879265092637, 0.05413385826771666132, 0.4176697321401328100 ) ) ;
#16356=CARTESIAN_POINT ( 'NONE',  ( 1.017060367454068581, -0.05778040916215560624, -0.4822834645669293319 ) ) ;
#16357=CARTESIAN_POINT ( 'NONE',  ( 0.6889763779527566800, -0.5400638737290844871, 0.3530559997133364547 ) ) ;
#16359=CARTESIAN_POINT ( 'NONE',  ( 0.1640419947506569498, -0.2845877964562161244, -0.3641732283464567121 ) ) ;
#16360=ORIENTED_EDGE ( 'NONE', *, *, #6655, .T. ) ;
#16363=CARTESIAN_POINT ( 'NONE',  ( -1.036745406824146176, -0.004921259842519870586, -0.3153832671262229437 ) ) ;
#16364=CARTESIAN_POINT ( 'NONE',  ( -0.6561679790026240244, 0.2306618581243847221, -0.2411417322834647770 ) ) ;
#16365=CARTESIAN_POINT ( 'NONE',  ( -0.6299212598425188991, -0.1870078740157479769, 0.4822834645669291653 ) ) ;
#16366=CARTESIAN_POINT ( 'NONE',  ( -0.4855643044619415427, -0.4281496062992124485, 0.4176697321401328655 ) ) ;
#16367=CARTESIAN_POINT ( 'NONE',  ( -1.318897637795274802, 0.1660481256975885056, 0.3530559997133364547 ) ) ;
#16368=CARTESIAN_POINT ( 'NONE',  ( -1.627296587926508442, -0.6046776061558809534, -0.2411417322834644161 ) ) ;
#16369=CARTESIAN_POINT ( 'NONE',  ( 0.9842519685039378130, -0.5511811023622047445, 6.969142054262312111E-17 ) ) ;
#16372=CARTESIAN_POINT ( 'NONE',  ( 0.2821522309711292364, -0.5511811023622046335, 0.09757992244046803654 ) ) ;
#16373=CARTESIAN_POINT ( 'NONE',  ( 0.2230971128608932319, -0.4281496062992124485, 0.4176697321401328655 ) ) ;
#16374=CARTESIAN_POINT ( 'NONE',  ( 0.3412073490813655186, -0.6046776061558809534, -0.2411417322834644161 ) ) ;
#16378=CARTESIAN_POINT ( 'NONE',  ( -0.5708661417322828946, 0.1660481256975883391, -0.3530559997133364547 ) ) ;
#16381=CARTESIAN_POINT ( 'NONE',  ( 1.528871391076116026, -0.6692913385826773087, -0.1292274648535924053 ) ) ;
#16382=CARTESIAN_POINT ( 'NONE',  ( -0.8530183727034112984, -0.3690944881889765550, -0.3153832671262227771 ) ) ;
#16383=CARTESIAN_POINT ( 'NONE',  ( -0.9908136482939626788, -0.6692913385826773087, -0.1292274648535924053 ) ) ;
#16386=CARTESIAN_POINT ( 'NONE',  ( 1.673228346456693494, 0.1660481256975885056, 0.3530559997133364547 ) ) ;
#16387=CARTESIAN_POINT ( 'NONE',  ( 0.4658792650918640033, -0.3162353388693405765, 0.4822834645669290543 ) ) ;
#16388=CARTESIAN_POINT ( 'NONE',  ( 0.6627296587926517768, -0.6692913385826773087, -0.1292274648535924053 ) ) ;
#16389=CARTESIAN_POINT ( 'NONE',  ( -0.7020997375328074108, -0.08942795157527998196, 0.3641732283464567121 ) ) ;
#16390=CARTESIAN_POINT ( 'NONE',  ( 0.05905511811023681640, 0.1660481256975883668, -0.3530559997133364547 ) ) ;
#16392=CARTESIAN_POINT ( 'NONE',  ( -0.4855643044619415427, -0.004921259842519870586, -0.3153832671262229437 ) ) ;
#16393=CARTESIAN_POINT ( 'NONE',  ( -0.4855643044619415427, -0.4281496062992124485, 0.4176697321401328655 ) ) ;
#16396=CARTESIAN_POINT ( 'NONE',  ( -1.502624671916009680, -0.05778040916215560624, -0.4822834645669293319 ) ) ;
#16397=CARTESIAN_POINT ( 'NONE',  ( 0.1049868766404206816, -0.5023911411419708095, -0.1820866141732282451 ) ) ;
#16398=CARTESIAN_POINT ( 'NONE',  ( 1.010498687664042716, -0.3690944881889763329, 0.3153832671262228327 ) ) ;
#16399=CARTESIAN_POINT ( 'NONE',  ( -1.292650918635170010, -0.6692913385826771977, 0.1292274648535927661 ) ) ;
#16400=CARTESIAN_POINT ( 'NONE',  ( -0.9251968503937002541, -0.4536011799217368745, -0.2665933059059886201 ) ) ;
#16401=DIRECTION ( 'NONE',  ( -1.692413147294446216E-16, 0.000000000000000000, -1.000000000000000000 ) ) ;
#16402=CARTESIAN_POINT ( 'NONE',  ( -1.122047244094487306, -0.5400638737290844871, 0.3530559997133364547 ) ) ;
#16403=CARTESIAN_POINT ( 'NONE',  ( -0.5643044619422565855, -0.4281496062992124485, 0.4176697321401328655 ) ) ;
#16404=CARTESIAN_POINT ( 'NONE',  ( 0.4790026246719168435, -0.3162353388693409650, -0.4822834645669289433 ) ) ;
#16407=CARTESIAN_POINT ( 'NONE',  ( 0.1837270341207357105, -0.5023911411419708095, -0.1820866141732282451 ) ) ;
#16408=CARTESIAN_POINT ( 'NONE',  ( 1.154855643044620184, 0.2306618581243847221, -0.2411417322834647770 ) ) ;
#16409=CARTESIAN_POINT ( 'NONE',  ( -1.095800524934382292, -0.08942795157527998196, 0.3641732283464567121 ) ) ;
#16410=CARTESIAN_POINT ( 'NONE',  ( 1.161417322834646493, -0.5400638737290844871, 0.3530559997133364547 ) ) ;
#16411=CARTESIAN_POINT ( 'NONE',  ( -1.732283464566928277, -0.1870078740157479769, 0.3641732283464567677 ) ) ;
#16412=CARTESIAN_POINT ( 'NONE',  ( 1.607611548556431069, 0.1771653543307087630, 0.09757992244046791164 ) ) ;
#16413=CARTESIAN_POINT ( 'NONE',  ( -0.9645669291338575535, -0.5400638737290844871, 0.3530559997133364547 ) ) ;
#16414=CARTESIAN_POINT ( 'NONE',  ( 0.09842519685039434474, 0.07958543189024085140, 0.2665933059059887866 ) ) ;
#16415=CARTESIAN_POINT ( 'NONE',  ( -0.8780747636526944344, -4.654285808514094606E-15, -0.3627989612356153915 ) ) ;
#16416=CARTESIAN_POINT ( 'NONE',  ( 0.8595800524934390507, -0.08942795157528024563, -0.3641732283464568787 ) ) ;
#16417=CARTESIAN_POINT ( 'NONE',  ( -0.04593175853018302557, 0.2952755905511811885, 0.1292274648535926551 ) ) ;
#16418=( BOUNDED_SURFACE ( )  B_SPLINE_SURFACE ( 1, 2, ( 
 ( #73558, #9986, #3255, #40719, #15482, #21776, #60081, #74797, #9569, #66404, #10408, #2843, #23017, #28507, #79878, #29334, #23428, #34413, #36065, #48269, #61737, #2435, #80703, #35240, #4074, #29741, #22196, #55405, #49093, #80295, #22609, #28917, #54585, #73967, #28092, #53749, #51143, #50738, #30973, #24247, #36886, #12454, #76025, #49920, #69295, #50327, #11644, #6128, #63378, #37302, #5714, #68472, #82341, #75618, #49511, #25064, #56640, #76436, #17144, #62145, #36470, #30154, #62563, #43180, #44408, #38115, #4902, #18370, #17956, #30573, #62976, #56239, #5315, #18765, #63789, #23844, #44010, #75204, #69704, #17548, #57049, #68877, #11226, #12047, #42776, #81936, #43593, #24659, #70102, #37705, #31384, #31803, #82743, #57463, #83157, #25476, #10810, #4486, #55816, #81524, #14133, #1910, #33479, #46502, #7385, #44819, #58724, #6963, #39786, #51555, #51979, #65890, #57876, #77258, #19588, #45250, #25895, #243, #70947, #7813, #1087, #65481, #65048, #70516, #39363, #59141, #33053, #1499, #20433, #13292, #52393, #27151, #52815, #32634, #662, #78526, #58297, #26318, #45665, #77684, #46087, #20014, #71779, #32218, #38944, #59555, #19171, #20849, #13709, #71361, #26739, #72202, #14555, #64627, #78102, #40207, #8225, #33889, #27572, #76837, #12873, #38532, #64213, #6547, #79355, #15800, #61641, #67135, #9464, #54900, #22916, #34310, #47751, #35138, #72612, #14960, #40617, #79775, #29236, #61214, #73868, #28402, #73450, #59972, #66722, #15375, #41451, #21674, #8639, #41036, #60800, #53230, #80193, #3154, #46919, #21264, #2331, #67963, #28817, #35971, #66300, #27987, #53647, #47335, #73025, #9059, #54482, #16208, #80606, #34731, #2742, #22511, #48172, #78946, #60391, #54060, #22091, #3982, #41855, #67547, #48583, #9882, #35551, #3569, #74280, #16624, #10305, #42266, #24967, #37200, #82652, #74698, #5216, #4796, #56955, #37609, #30057, #11954, #30880, #69195, #11544, #4389, #56137, #49823, #81016, #43086, #63697, #63284, #43497, #36785, #49416, #50639, #56547, #62461, #81842, #62881, #24153, #18673, #75929, #75523, #18270, #23329, #82248, #30473, #62051, #5624, #43910, #48999, #31290, #17862, #24566, #50233, #11127, #69608, #17043, #42683, #76343, #44318, #68783, #70008, #68381, #10720, #36377, #12363, #81428, #38021, #29646, #55308, #55718, #23743, #75110, #17456, #146, #51047, #46409, #77164, #20759, #44726, #51885, #51462, #32124, #6454, #45150, #25384, #70423, #83063, #14037, #65385, #39694, #78431, #20337, #25801, #76748, #57368, #19078, #77590, #57782, #7720, #19924, #45574, #70853, #12779, #40113, #71267, #19496, #38436, #72103, #13204, #14461, #64119, #13614, #38851, #64531, #6868, #32537, #58201, #569, #26222, #33388, #59051, #1405, #6036, #45989, #39268, #64950, #7290, #32960, #58627, #994, #26649, #52303, #31708, #78009, #71685, #27061, #52720, #46828, #73774, #53967, #41754, #33799, #53135, #72520, #59464, #1815, #21173, #28305, #73353, #3056, #14868, #79264, #79679, #40943, #65800, #40530, #78846, #27477, #8134, #21996, #66209, #8548, #47241, #34214, #2648, #15282, #67449, #59877, #27896, #2231, #16110, #53556, #66622, #9783, #60707, #21579, #72931, #41358, #8960, #34634, #60298, #47657, #22415, #15701, #67039, #28722, #9371, #35042, #54385, #80095, #48072, #77439, #52991, #33246, #7142, #26504, #7573, #52157, #46688, #20615, #77862, #46267, #25655, #39547, #32815, #6722, #65664, #71962, #51317, #7991, #847, #45842, #20191, #39122, #14316, #77020, #19353, #58907, #71541, #71122, #72381, #65236, #58482, #32392, #33655, #39975, #45002, #59318, #13888, #1267, #26915, #64803, #1674, #70701, #13054, #52575, #78284, #13465, #14731, #38707, #64386, #58055, #27331, #26077, #78704, #21028, #40383, #66066, #421, #8402, #57640, #51737, #19773, #3, #45426, #48758, #72788, #79958, #79538, #60156, #34490, #73207, #53416, #15138, #27752, #42033, #10062, #67727, #23091, #48342, #53824, #47515, #21851, #54241, #2508, #40794, #15557, #22271, #34069, #60979, #73634, #79125, #2087, #66479, #74457, #9647, #16804, #21442, #47099, #8814, #28167, #41216 ),
 ( #68140, #35725, #66904, #16386, #9235, #34907, #28993, #42440, #59733, #29408, #41623, #3744, #60570, #35316, #2921, #61395, #55067, #28585, #80775, #3329, #15976, #67312, #47930, #54659, #80370, #22683, #74039, #44490, #44088, #24327, #17625, #30231, #5795, #69371, #43257, #62640, #43669, #4984, #82821, #56721, #30651, #82418, #61811, #42852, #18446, #24737, #4151, #69782, #36963, #82013, #56315, #75282, #50405, #29816, #55477, #11725, #49997, #23921, #25146, #81187, #23504, #49171, #75694, #62222, #12127, #18035, #37381, #68954, #74876, #10485, #63052, #4560, #17220, #50814, #81605, #76515, #68545, #5390, #55893, #36546, #10886, #49587, #11304, #31052, #76102, #37784, #63461, #31465, #18844, #57127, #36139, #10313, #68790, #22924, #80613, #17463, #61648, #3989, #11135, #36793, #35559, #3576, #48590, #42273, #49006, #62469, #68388, #81435, #67970, #79783, #35978, #41862, #74705, #3161, #29243, #43093, #9471, #28825, #54489, #80200, #60808, #35145, #22518, #42691, #29653, #17050, #16631, #22099, #74287, #10727, #55315, #36384, #81024, #48179, #23336, #62058, #4396, #67554, #61222, #30064, #9889, #54907, #55726, #23750, #49423, #75118, #28409, #67142, #73875, #54068, #47759, #73457, #15808, #41458, #16215, #6460, #25806, #37206, #5223, #12786, #5630, #70015, #25390, #32129, #51467, #18276, #57787, #83069, #30886, #50645, #13209, #38028, #63703, #45155, #38856, #11960, #63290, #82659, #18679, #51053, #4803, #44733, #151, #44324, #56146, #12369, #43917, #76754, #62887, #31297, #77169, #69202, #56553, #82254, #24573, #50240, #11551, #75936, #19085, #6043, #70429, #76349, #81849, #31715, #38442, #57374, #64124, #19501, #69614, #70858, #30480, #24161, #37616, #56961, #49829, #24973, #75529, #17869, #43503, #8139, #45994, #59469, #19929, #7295, #47247, #6873, #46833, #1411, #14042, #39699, #66214, #2236, #13619, #64957, #72525, #65390, #46414, #1822, #8553, #27900, #78015, #34220, #27482, #32965, #27066, #72936, #78437, #20764, #59882, #53561, #45579, #59056, #72108, #574, #26227, #51891, #7725, #40535, #14874, #53140, #33394, #52725, #71272, #14466, #79269, #15288, #77595, #39273, #58632, #1000, #26654, #21584, #64536, #52308, #65806, #40118, #20342, #33804, #71691, #78851, #32542, #58207, #21178, #16532, #73357, #42177, #41362, #80918, #67043, #15705, #10209, #75015, #29141, #9375, #22826, #81329, #35458, #9787, #29954, #48902, #55210, #8965, #74603, #67453, #54807, #61123, #22419, #23231, #60303, #34639, #67871, #3474, #54389, #55619, #2653, #28311, #53972, #80511, #35046, #16946, #48484, #74185, #48076, #79685, #40948, #35877, #60711, #22002, #23643, #28728, #49314, #47662, #61544, #3060, #80100, #73778, #16114, #41758, #3888, #29548, #42588, #68288, #10624, #66627, #36280, #61952, #4292, #18979, #37512, #43396, #56037, #5119, #63187, #17361, #44221, #56856, #11027, #68684, #24055, #32025, #76244, #47, #36683, #30370, #75422, #62359, #4696, #49725, #50540, #37923, #76648, #81745, #50132, #18578, #5526, #42990, #17765, #69096, #11444, #51361, #75832, #37100, #44628, #62785, #82965, #30786, #56449, #12265, #57685, #82151, #12680, #24872, #70324, #24467, #69911, #18173, #38338, #25283, #43806, #50951, #63599, #82554, #5936, #69510, #11859, #31191, #31606, #57267, #64013, #6354, #25700, #896, #13511, #72427, #52626, #26553, #45889, #26962, #71587, #66113, #40022, #13938, #65710, #45049, #58955, #52206, #26123, #6767, #39167, #19823, #21077, #14777, #64852, #78332, #77910, #7189, #39596, #32862, #65285, #78752, #40432, #466, #20662, #51784, #46316, #77488, #33703, #45473, #71170, #72009, #28931, #7623, #58530, #1313, #35255, #33295, #14365, #9586, #8040, #59363, #60919, #3270, #20241, #1722, #27378, #53040, #46735, #77064, #19398, #70750, #13101, #38755, #64432, #32438, #58101, #29349, #29756, #43608, #35666, #55008, #80716, #23031, #3684, #61330, #48697, #68891, #36485, #75218, #42791, #48284, #17158, #36901, #68486, #17563, #81539, #74395, #30168, #43196, #4919, #10422, #61751, #56253, #36080, #4088, #23443, #55419, #23858, #81126, #49525, #10001, #16739 ) ),
 .UNSPECIFIED., .F., .F., .F. ) 
 B_SPLINE_SURFACE_WITH_KNOTS ( ( 2, 2 ),
 ( 3, 2, 2, 2, 2, 2, 2, 2, 2, 2, 2, 2, 2, 2, 2, 2, 2, 2, 2, 2, 2, 2, 2, 2, 2, 2, 2, 2, 2, 2, 2, 2, 2, 2, 2, 2, 2, 2, 2, 2, 2, 2, 2, 2, 2, 2, 2, 2, 2, 2, 2, 2, 2, 2, 2, 2, 2, 2, 2, 2, 2, 2, 2, 2, 2, 2, 2, 2, 2, 2, 2, 2, 2, 2, 2, 2, 2, 2, 2, 2, 2, 2, 2, 2, 2, 2, 2, 2, 2, 2, 2, 2, 2, 2, 2, 2, 2, 2, 2, 2, 2, 2, 2, 2, 2, 2, 2, 2, 2, 2, 2, 2, 2, 2, 2, 2, 2, 2, 2, 2, 2, 2, 2, 2, 2, 2, 2, 2, 2, 2, 2, 2, 2, 2, 2, 2, 2, 2, 2, 2, 2, 2, 2, 2, 2, 2, 2, 2, 2, 2, 2, 2, 2, 2, 2, 2, 2, 2, 2, 2, 2, 2, 2, 2, 2, 2, 2, 2, 2, 2, 2, 2, 2, 2, 2, 2, 2, 2, 2, 2, 2, 2, 2, 2, 2, 2, 2, 2, 2, 2, 2, 2, 2, 2, 2, 2, 2, 2, 2, 2, 2, 2, 2, 2, 2, 2, 2, 2, 2, 2, 2, 2, 2, 2, 2, 2, 2, 2, 2, 2, 2, 2, 2, 2, 2, 2, 2, 2, 2, 2, 2, 2, 2, 2, 2, 2, 2, 2, 2, 2, 2, 2, 2, 2, 2, 2, 2, 2, 2, 2, 2, 2, 2, 2, 2, 3 ),
 ( 0.000000000000000000, 1.000000000000000000 ),
 ( 0.000000000000000000, 0.003787878787878787984, 0.007575757575757575968, 0.01136363636363636395, 0.01515151515151515194, 0.01893939393939393992, 0.02272727272727272790, 0.02651515151515151589, 0.03030303030303030387, 0.03409090909090908839, 0.03787878787878787984, 0.04166666666666666435, 0.04545454545454545581, 0.04924242424242424032, 0.05303030303030303177, 0.05681818181818181629, 0.06060606060606060774, 0.06439393939393939226, 0.06818181818181817677, 0.07196969696969697516, 0.07575757575757575968, 0.07954545454545454419, 0.08333333333333332871, 0.08712121212121212710, 0.09090909090909091161, 0.09469696969696969613, 0.09848484848484848064, 0.1022727272727272790, 0.1060606060606060635, 0.1098484848484848481, 0.1136363636363636326, 0.1174242424242424310, 0.1212121212121212155, 0.1250000000000000000, 0.1287878787878787845, 0.1325757575757575690, 0.1363636363636363535, 0.1401515151515151381, 0.1439393939393939503, 0.1477272727272727348, 0.1515151515151515194, 0.1553030303030303039, 0.1590909090909090884, 0.1628787878787878729, 0.1666666666666666574, 0.1704545454545454419, 0.1742424242424242542, 0.1780303030303030387, 0.1818181818181818232, 0.1856060606060606077, 0.1893939393939393923, 0.1931818181818181768, 0.1969696969696969613, 0.2007575757575757458, 0.2045454545454545581, 0.2083333333333333426, 0.2121212121212121271, 0.2159090909090909116, 0.2196969696969696961, 0.2234848484848484806, 0.2272727272727272652, 0.2310606060606060497, 0.2348484848484848619, 0.2386363636363636465, 0.2424242424242424310, 0.2462121212121212155, 0.2500000000000000000, 0.2537878787878787845, 0.2575757575757575690, 0.2613636363636363535, 0.2651515151515151381, 0.2689393939393939226, 0.2727272727272727071, 0.2765151515151514916, 0.2803030303030302761, 0.2840909090909091161, 0.2878787878787879007, 0.2916666666666666852, 0.2954545454545454697, 0.2992424242424242542, 0.3030303030303030387, 0.3068181818181818232, 0.3106060606060606077, 0.3143939393939393923, 0.3181818181818181768, 0.3219696969696969613, 0.3257575757575757458, 0.3295454545454545303, 0.3333333333333333148, 0.3371212121212120993, 0.3409090909090908839, 0.3446969696969697239, 0.3484848484848485084, 0.3522727272727272929, 0.3560606060606060774, 0.3598484848484848619, 0.3636363636363636465, 0.3674242424242424310, 0.3712121212121212155, 0.3750000000000000000, 0.3787878787878787845, 0.3825757575757575690, 0.3863636363636363535, 0.3901515151515151381, 0.3939393939393939226, 0.3977272727272727071, 0.4015151515151514916, 0.4053030303030302761, 0.4090909090909091161, 0.4128787878787879007, 0.4166666666666666852, 0.4204545454545454697, 0.4242424242424242542, 0.4280303030303030387, 0.4318181818181818232, 0.4356060606060606077, 0.4393939393939393923, 0.4431818181818181768, 0.4469696969696969613, 0.4507575757575757458, 0.4545454545454545303, 0.4583333333333333148, 0.4621212121212120993, 0.4659090909090908839, 0.4696969696969697239, 0.4734848484848485084, 0.4772727272727272929, 0.4810606060606060774, 0.4848484848484848619, 0.4886363636363636465, 0.4924242424242424310, 0.4962121212121212155, 0.5000000000000000000, 0.5037878787878787845, 0.5075757575757575690, 0.5113636363636363535, 0.5151515151515151381, 0.5189393939393939226, 0.5227272727272727071, 0.5265151515151514916, 0.5303030303030302761, 0.5340909090909090606, 0.5378787878787878451, 0.5416666666666666297, 0.5454545454545454142, 0.5492424242424241987, 0.5530303030303029832, 0.5568181818181817677, 0.5606060606060605522, 0.5643939393939394478, 0.5681818181818182323, 0.5719696969696970168, 0.5757575757575758013, 0.5795454545454545858, 0.5833333333333333703, 0.5871212121212121549, 0.5909090909090909394, 0.5946969696969697239, 0.5984848484848485084, 0.6022727272727272929, 0.6060606060606060774, 0.6098484848484848619, 0.6136363636363636465, 0.6174242424242424310, 0.6212121212121212155, 0.6250000000000000000, 0.6287878787878787845, 0.6325757575757575690, 0.6363636363636363535, 0.6401515151515151381, 0.6439393939393939226, 0.6477272727272727071, 0.6515151515151514916, 0.6553030303030302761, 0.6590909090909090606, 0.6628787878787878451, 0.6666666666666666297, 0.6704545454545454142, 0.6742424242424241987, 0.6780303030303029832, 0.6818181818181817677, 0.6856060606060605522, 0.6893939393939394478, 0.6931818181818182323, 0.6969696969696970168, 0.7007575757575758013, 0.7045454545454545858, 0.7083333333333333703, 0.7121212121212121549, 0.7159090909090909394, 0.7196969696969697239, 0.7234848484848485084, 0.7272727272727272929, 0.7310606060606060774, 0.7348484848484848619, 0.7386363636363636465, 0.7424242424242424310, 0.7462121212121212155, 0.7500000000000000000, 0.7537878787878787845, 0.7575757575757575690, 0.7613636363636363535, 0.7651515151515151381, 0.7689393939393939226, 0.7727272727272727071, 0.7765151515151514916, 0.7803030303030302761, 0.7840909090909090606, 0.7878787878787878451, 0.7916666666666666297, 0.7954545454545454142, 0.7992424242424241987, 0.8030303030303029832, 0.8068181818181817677, 0.8106060606060605522, 0.8143939393939394478, 0.8181818181818182323, 0.8219696969696970168, 0.8257575757575758013, 0.8295454545454545858, 0.8333333333333333703, 0.8371212121212121549, 0.8409090909090909394, 0.8446969696969697239, 0.8484848484848485084, 0.8522727272727272929, 0.8560606060606060774, 0.8598484848484848619, 0.8636363636363636465, 0.8674242424242424310, 0.8712121212121212155, 0.8750000000000000000, 0.8787878787878787845, 0.8825757575757575690, 0.8863636363636363535, 0.8901515151515151381, 0.8939393939393939226, 0.8977272727272727071, 0.9015151515151514916, 0.9053030303030302761, 0.9090909090909090606, 0.9128787878787878451, 0.9166666666666666297, 0.9204545454545454142, 0.9242424242424241987, 0.9280303030303029832, 0.9318181818181817677, 0.9356060606060605522, 0.9393939393939394478, 0.9431818181818182323, 0.9469696969696970168, 0.9507575757575758013, 0.9545454545454545858, 0.9583333333333333703, 0.9621212121212121549, 0.9659090909090909394 ),
 .UNSPECIFIED. ) 
 GEOMETRIC_REPRESENTATION_ITEM ( )  RATIONAL_B_SPLINE_SURFACE ( (
 ( 1.000000000000000000, 0.9659258262890683122, 1.000000000000000000, 0.9659258262890683122, 1.000000000000000000, 0.9659258262890683122, 1.000000000000000000, 0.9659258262890683122, 1.000000000000000000, 0.9659258262890683122, 1.000000000000000000, 0.9659258262890683122, 1.000000000000000000, 0.9659258262890683122, 1.000000000000000000, 0.9659258262890683122, 1.000000000000000000, 0.9659258262890683122, 1.000000000000000000, 0.9659258262890683122, 1.000000000000000000, 0.9659258262890683122, 1.000000000000000000, 0.9659258262890683122, 1.000000000000000000, 0.9659258262890683122, 1.000000000000000000, 0.9659258262890683122, 1.000000000000000000, 0.9659258262890683122, 1.000000000000000000, 0.9659258262890683122, 1.000000000000000000, 0.9659258262890683122, 1.000000000000000000, 0.9659258262890683122, 1.000000000000000000, 0.9659258262890683122, 1.000000000000000000, 0.9659258262890683122, 1.000000000000000000, 0.9659258262890683122, 1.000000000000000000, 0.9659258262890683122, 1.000000000000000000, 0.9659258262890683122, 1.000000000000000000, 0.9659258262890683122, 1.000000000000000000, 0.9659258262890683122, 1.000000000000000000, 0.9659258262890683122, 1.000000000000000000, 0.9659258262890683122, 1.000000000000000000, 0.9659258262890683122, 1.000000000000000000, 0.9659258262890683122, 1.000000000000000000, 0.9659258262890683122, 1.000000000000000000, 0.9659258262890683122, 1.000000000000000000, 0.9659258262890683122, 1.000000000000000000, 0.9659258262890683122, 1.000000000000000000, 0.9659258262890683122, 1.000000000000000000, 0.9659258262890683122, 1.000000000000000000, 0.9659258262890683122, 1.000000000000000000, 0.9659258262890683122, 1.000000000000000000, 0.9659258262890683122, 1.000000000000000000, 0.9659258262890683122, 1.000000000000000000, 0.9659258262890683122, 1.000000000000000000, 0.9659258262890683122, 1.000000000000000000, 0.9659258262890683122, 1.000000000000000000, 0.9659258262890683122, 1.000000000000000000, 0.9659258262890683122, 1.000000000000000000, 0.9659258262890683122, 1.000000000000000000, 0.9659258262890683122, 1.000000000000000000, 0.9659258262890683122, 1.000000000000000000, 0.9659258262890683122, 1.000000000000000000, 0.9659258262890683122, 1.000000000000000000, 0.9659258262890683122, 1.000000000000000000, 0.9659258262890683122, 1.000000000000000000, 0.9659258262890683122, 1.000000000000000000, 0.9659258262890683122, 1.000000000000000000, 0.9659258262890683122, 1.000000000000000000, 0.9659258262890683122, 1.000000000000000000, 0.9659258262890683122, 1.000000000000000000, 0.9659258262890683122, 1.000000000000000000, 0.9659258262890683122, 1.000000000000000000, 0.9659258262890683122, 1.000000000000000000, 0.9659258262890683122, 1.000000000000000000, 0.9659258262890683122, 1.000000000000000000, 0.9659258262890683122, 1.000000000000000000, 0.9659258262890683122, 1.000000000000000000, 0.9659258262890683122, 1.000000000000000000, 0.9659258262890683122, 1.000000000000000000, 0.9659258262890683122, 1.000000000000000000, 0.9659258262890683122, 1.000000000000000000, 0.9659258262890683122, 1.000000000000000000, 0.9659258262890683122, 1.000000000000000000, 0.9659258262890683122, 1.000000000000000000, 0.9659258262890683122, 1.000000000000000000, 0.9659258262890683122, 1.000000000000000000, 0.9659258262890683122, 1.000000000000000000, 0.9659258262890683122, 1.000000000000000000, 0.9659258262890683122, 1.000000000000000000, 0.9659258262890683122, 1.000000000000000000, 0.9659258262890683122, 1.000000000000000000, 0.9659258262890683122, 1.000000000000000000, 0.9659258262890683122, 1.000000000000000000, 0.9659258262890683122, 1.000000000000000000, 0.9659258262890683122, 1.000000000000000000, 0.9659258262890683122, 1.000000000000000000, 0.9659258262890683122, 1.000000000000000000, 0.9659258262890683122, 1.000000000000000000, 0.9659258262890683122, 1.000000000000000000, 0.9659258262890683122, 1.000000000000000000, 0.9659258262890683122, 1.000000000000000000, 0.9659258262890683122, 1.000000000000000000, 0.9659258262890683122, 1.000000000000000000, 0.9659258262890683122, 1.000000000000000000, 0.9659258262890683122, 1.000000000000000000, 0.9659258262890683122, 1.000000000000000000, 0.9659258262890683122, 1.000000000000000000, 0.9659258262890683122, 1.000000000000000000, 0.9659258262890683122, 1.000000000000000000, 0.9659258262890683122, 1.000000000000000000, 0.9659258262890683122, 1.000000000000000000, 0.9659258262890683122, 1.000000000000000000, 0.9659258262890683122, 1.000000000000000000, 0.9659258262890683122, 1.000000000000000000, 0.9659258262890683122, 1.000000000000000000, 0.9659258262890683122, 1.000000000000000000, 0.9659258262890683122, 1.000000000000000000, 0.9659258262890683122, 1.000000000000000000, 0.9659258262890683122, 1.000000000000000000, 0.9659258262890683122, 1.000000000000000000, 0.9659258262890683122, 1.000000000000000000, 0.9659258262890683122, 1.000000000000000000, 0.9659258262890683122, 1.000000000000000000, 0.9659258262890683122, 1.000000000000000000, 0.9659258262890683122, 1.000000000000000000, 0.9659258262890683122, 1.000000000000000000, 0.9659258262890683122, 1.000000000000000000, 0.9659258262890683122, 1.000000000000000000, 0.9659258262890683122, 1.000000000000000000, 0.9659258262890683122, 1.000000000000000000, 0.9659258262890683122, 1.000000000000000000, 0.9659258262890683122, 1.000000000000000000, 0.9659258262890683122, 1.000000000000000000, 0.9659258262890683122, 1.000000000000000000, 0.9659258262890683122, 1.000000000000000000, 0.9659258262890683122, 1.000000000000000000, 0.9659258262890683122, 1.000000000000000000, 0.9659258262890683122, 1.000000000000000000, 0.9659258262890683122, 1.000000000000000000, 0.9659258262890683122, 1.000000000000000000, 0.9659258262890683122, 1.000000000000000000, 0.9659258262890683122, 1.000000000000000000, 0.9659258262890683122, 1.000000000000000000, 0.9659258262890683122, 1.000000000000000000, 0.9659258262890683122, 1.000000000000000000, 0.9659258262890683122, 1.000000000000000000, 0.9659258262890683122, 1.000000000000000000, 0.9659258262890683122, 1.000000000000000000, 0.9659258262890683122, 1.000000000000000000, 0.9659258262890683122, 1.000000000000000000, 0.9659258262890683122, 1.000000000000000000, 0.9659258262890683122, 1.000000000000000000, 0.9659258262890683122, 1.000000000000000000, 0.9659258262890683122, 1.000000000000000000, 0.9659258262890683122, 1.000000000000000000, 0.9659258262890683122, 1.000000000000000000, 0.9659258262890683122, 1.000000000000000000, 0.9659258262890683122, 1.000000000000000000, 0.9659258262890683122, 1.000000000000000000, 0.9659258262890683122, 1.000000000000000000, 0.9659258262890683122, 1.000000000000000000, 0.9659258262890683122, 1.000000000000000000, 0.9659258262890683122, 1.000000000000000000, 0.9659258262890683122, 1.000000000000000000, 0.9659258262890683122, 1.000000000000000000, 0.9659258262890683122, 1.000000000000000000, 0.9659258262890683122, 1.000000000000000000, 0.9659258262890683122, 1.000000000000000000, 0.9659258262890683122, 1.000000000000000000, 0.9659258262890683122, 1.000000000000000000, 0.9659258262890683122, 1.000000000000000000, 0.9659258262890683122, 1.000000000000000000, 0.9659258262890683122, 1.000000000000000000, 0.9659258262890683122, 1.000000000000000000, 0.9659258262890683122, 1.000000000000000000, 0.9659258262890683122, 1.000000000000000000, 0.9659258262890683122, 1.000000000000000000, 0.9659258262890683122, 1.000000000000000000, 0.9659258262890683122, 1.000000000000000000, 0.9659258262890683122, 1.000000000000000000, 0.9659258262890683122, 1.000000000000000000, 0.9659258262890683122, 1.000000000000000000, 0.9659258262890683122, 1.000000000000000000, 0.9659258262890683122, 1.000000000000000000, 0.9659258262890683122, 1.000000000000000000, 0.9659258262890683122, 1.000000000000000000, 0.9659258262890683122, 1.000000000000000000, 0.9659258262890683122, 1.000000000000000000, 0.9659258262890683122, 1.000000000000000000, 0.9659258262890683122, 1.000000000000000000, 0.9659258262890683122, 1.000000000000000000, 0.9659258262890683122, 1.000000000000000000, 0.9659258262890683122, 1.000000000000000000, 0.9659258262890683122, 1.000000000000000000, 0.9659258262890683122, 1.000000000000000000, 0.9659258262890683122, 1.000000000000000000, 0.9659258262890683122, 1.000000000000000000, 0.9659258262890683122, 1.000000000000000000, 0.9659258262890683122, 1.000000000000000000, 0.9659258262890683122, 1.000000000000000000, 0.9659258262890683122, 1.000000000000000000, 0.9659258262890683122, 1.000000000000000000, 0.9659258262890683122, 1.000000000000000000, 0.9659258262890683122, 1.000000000000000000, 0.9659258262890683122, 1.000000000000000000, 0.9659258262890683122, 1.000000000000000000, 0.9659258262890683122, 1.000000000000000000, 0.9659258262890683122, 1.000000000000000000, 0.9659258262890683122, 1.000000000000000000, 0.9659258262890683122, 1.000000000000000000, 0.9659258262890683122, 1.000000000000000000, 0.9659258262890683122, 1.000000000000000000, 0.9659258262890683122, 1.000000000000000000, 0.9659258262890683122, 1.000000000000000000, 0.9659258262890683122, 1.000000000000000000, 0.9659258262890683122, 1.000000000000000000, 0.9659258262890683122, 1.000000000000000000, 0.9659258262890683122, 1.000000000000000000, 0.9659258262890683122, 1.000000000000000000, 0.9659258262890683122, 1.000000000000000000, 0.9659258262890683122, 1.000000000000000000, 0.9659258262890683122, 1.000000000000000000, 0.9659258262890683122, 1.000000000000000000, 0.9659258262890683122, 1.000000000000000000, 0.9659258262890683122, 1.000000000000000000, 0.9659258262890683122, 1.000000000000000000, 0.9659258262890683122, 1.000000000000000000, 0.9659258262890683122, 1.000000000000000000, 0.9659258262890683122, 1.000000000000000000, 0.9659258262890683122, 1.000000000000000000, 0.9659258262890683122, 1.000000000000000000, 0.9659258262890683122, 1.000000000000000000, 0.9659258262890683122, 1.000000000000000000, 0.9659258262890683122, 1.000000000000000000, 0.9659258262890683122, 1.000000000000000000, 0.9659258262890683122, 1.000000000000000000, 0.9659258262890683122, 1.000000000000000000, 0.9659258262890683122, 1.000000000000000000, 0.9659258262890683122, 1.000000000000000000, 0.9659258262890683122, 1.000000000000000000, 0.9659258262890683122, 1.000000000000000000, 0.9659258262890683122, 1.000000000000000000, 0.9659258262890683122, 1.000000000000000000, 0.9659258262890683122, 1.000000000000000000, 0.9659258262890683122, 1.000000000000000000, 0.9659258262890683122, 1.000000000000000000, 0.9659258262890683122, 1.000000000000000000, 0.9659258262890683122, 1.000000000000000000, 0.9659258262890683122, 1.000000000000000000, 0.9659258262890683122, 1.000000000000000000, 0.9659258262890683122, 1.000000000000000000, 0.9659258262890683122, 1.000000000000000000, 0.9659258262890683122, 1.000000000000000000, 0.9659258262890683122, 1.000000000000000000, 0.9659258262890683122, 1.000000000000000000, 0.9659258262890683122, 1.000000000000000000, 0.9659258262890683122, 1.000000000000000000, 0.9659258262890683122, 1.000000000000000000, 0.9659258262890683122, 1.000000000000000000, 0.9659258262890683122, 1.000000000000000000, 0.9659258262890683122, 1.000000000000000000, 0.9659258262890683122, 1.000000000000000000, 0.9659258262890683122, 1.000000000000000000, 0.9659258262890683122, 1.000000000000000000, 0.9659258262890683122, 1.000000000000000000, 0.9659258262890683122, 1.000000000000000000, 0.9659258262890683122, 1.000000000000000000, 0.9659258262890683122, 1.000000000000000000, 0.9659258262890683122, 1.000000000000000000),
 ( 1.000000000000000000, 0.9659258262890683122, 1.000000000000000000, 0.9659258262890683122, 1.000000000000000000, 0.9659258262890683122, 1.000000000000000000, 0.9659258262890683122, 1.000000000000000000, 0.9659258262890683122, 1.000000000000000000, 0.9659258262890683122, 1.000000000000000000, 0.9659258262890683122, 1.000000000000000000, 0.9659258262890683122, 1.000000000000000000, 0.9659258262890683122, 1.000000000000000000, 0.9659258262890683122, 1.000000000000000000, 0.9659258262890683122, 1.000000000000000000, 0.9659258262890683122, 1.000000000000000000, 0.9659258262890683122, 1.000000000000000000, 0.9659258262890683122, 1.000000000000000000, 0.9659258262890683122, 1.000000000000000000, 0.9659258262890683122, 1.000000000000000000, 0.9659258262890683122, 1.000000000000000000, 0.9659258262890683122, 1.000000000000000000, 0.9659258262890683122, 1.000000000000000000, 0.9659258262890683122, 1.000000000000000000, 0.9659258262890683122, 1.000000000000000000, 0.9659258262890683122, 1.000000000000000000, 0.9659258262890683122, 1.000000000000000000, 0.9659258262890683122, 1.000000000000000000, 0.9659258262890683122, 1.000000000000000000, 0.9659258262890683122, 1.000000000000000000, 0.9659258262890683122, 1.000000000000000000, 0.9659258262890683122, 1.000000000000000000, 0.9659258262890683122, 1.000000000000000000, 0.9659258262890683122, 1.000000000000000000, 0.9659258262890683122, 1.000000000000000000, 0.9659258262890683122, 1.000000000000000000, 0.9659258262890683122, 1.000000000000000000, 0.9659258262890683122, 1.000000000000000000, 0.9659258262890683122, 1.000000000000000000, 0.9659258262890683122, 1.000000000000000000, 0.9659258262890683122, 1.000000000000000000, 0.9659258262890683122, 1.000000000000000000, 0.9659258262890683122, 1.000000000000000000, 0.9659258262890683122, 1.000000000000000000, 0.9659258262890683122, 1.000000000000000000, 0.9659258262890683122, 1.000000000000000000, 0.9659258262890683122, 1.000000000000000000, 0.9659258262890683122, 1.000000000000000000, 0.9659258262890683122, 1.000000000000000000, 0.9659258262890683122, 1.000000000000000000, 0.9659258262890683122, 1.000000000000000000, 0.9659258262890683122, 1.000000000000000000, 0.9659258262890683122, 1.000000000000000000, 0.9659258262890683122, 1.000000000000000000, 0.9659258262890683122, 1.000000000000000000, 0.9659258262890683122, 1.000000000000000000, 0.9659258262890683122, 1.000000000000000000, 0.9659258262890683122, 1.000000000000000000, 0.9659258262890683122, 1.000000000000000000, 0.9659258262890683122, 1.000000000000000000, 0.9659258262890683122, 1.000000000000000000, 0.9659258262890683122, 1.000000000000000000, 0.9659258262890683122, 1.000000000000000000, 0.9659258262890683122, 1.000000000000000000, 0.9659258262890683122, 1.000000000000000000, 0.9659258262890683122, 1.000000000000000000, 0.9659258262890683122, 1.000000000000000000, 0.9659258262890683122, 1.000000000000000000, 0.9659258262890683122, 1.000000000000000000, 0.9659258262890683122, 1.000000000000000000, 0.9659258262890683122, 1.000000000000000000, 0.9659258262890683122, 1.000000000000000000, 0.9659258262890683122, 1.000000000000000000, 0.9659258262890683122, 1.000000000000000000, 0.9659258262890683122, 1.000000000000000000, 0.9659258262890683122, 1.000000000000000000, 0.9659258262890683122, 1.000000000000000000, 0.9659258262890683122, 1.000000000000000000, 0.9659258262890683122, 1.000000000000000000, 0.9659258262890683122, 1.000000000000000000, 0.9659258262890683122, 1.000000000000000000, 0.9659258262890683122, 1.000000000000000000, 0.9659258262890683122, 1.000000000000000000, 0.9659258262890683122, 1.000000000000000000, 0.9659258262890683122, 1.000000000000000000, 0.9659258262890683122, 1.000000000000000000, 0.9659258262890683122, 1.000000000000000000, 0.9659258262890683122, 1.000000000000000000, 0.9659258262890683122, 1.000000000000000000, 0.9659258262890683122, 1.000000000000000000, 0.9659258262890683122, 1.000000000000000000, 0.9659258262890683122, 1.000000000000000000, 0.9659258262890683122, 1.000000000000000000, 0.9659258262890683122, 1.000000000000000000, 0.9659258262890683122, 1.000000000000000000, 0.9659258262890683122, 1.000000000000000000, 0.9659258262890683122, 1.000000000000000000, 0.9659258262890683122, 1.000000000000000000, 0.9659258262890683122, 1.000000000000000000, 0.9659258262890683122, 1.000000000000000000, 0.9659258262890683122, 1.000000000000000000, 0.9659258262890683122, 1.000000000000000000, 0.9659258262890683122, 1.000000000000000000, 0.9659258262890683122, 1.000000000000000000, 0.9659258262890683122, 1.000000000000000000, 0.9659258262890683122, 1.000000000000000000, 0.9659258262890683122, 1.000000000000000000, 0.9659258262890683122, 1.000000000000000000, 0.9659258262890683122, 1.000000000000000000, 0.9659258262890683122, 1.000000000000000000, 0.9659258262890683122, 1.000000000000000000, 0.9659258262890683122, 1.000000000000000000, 0.9659258262890683122, 1.000000000000000000, 0.9659258262890683122, 1.000000000000000000, 0.9659258262890683122, 1.000000000000000000, 0.9659258262890683122, 1.000000000000000000, 0.9659258262890683122, 1.000000000000000000, 0.9659258262890683122, 1.000000000000000000, 0.9659258262890683122, 1.000000000000000000, 0.9659258262890683122, 1.000000000000000000, 0.9659258262890683122, 1.000000000000000000, 0.9659258262890683122, 1.000000000000000000, 0.9659258262890683122, 1.000000000000000000, 0.9659258262890683122, 1.000000000000000000, 0.9659258262890683122, 1.000000000000000000, 0.9659258262890683122, 1.000000000000000000, 0.9659258262890683122, 1.000000000000000000, 0.9659258262890683122, 1.000000000000000000, 0.9659258262890683122, 1.000000000000000000, 0.9659258262890683122, 1.000000000000000000, 0.9659258262890683122, 1.000000000000000000, 0.9659258262890683122, 1.000000000000000000, 0.9659258262890683122, 1.000000000000000000, 0.9659258262890683122, 1.000000000000000000, 0.9659258262890683122, 1.000000000000000000, 0.9659258262890683122, 1.000000000000000000, 0.9659258262890683122, 1.000000000000000000, 0.9659258262890683122, 1.000000000000000000, 0.9659258262890683122, 1.000000000000000000, 0.9659258262890683122, 1.000000000000000000, 0.9659258262890683122, 1.000000000000000000, 0.9659258262890683122, 1.000000000000000000, 0.9659258262890683122, 1.000000000000000000, 0.9659258262890683122, 1.000000000000000000, 0.9659258262890683122, 1.000000000000000000, 0.9659258262890683122, 1.000000000000000000, 0.9659258262890683122, 1.000000000000000000, 0.9659258262890683122, 1.000000000000000000, 0.9659258262890683122, 1.000000000000000000, 0.9659258262890683122, 1.000000000000000000, 0.9659258262890683122, 1.000000000000000000, 0.9659258262890683122, 1.000000000000000000, 0.9659258262890683122, 1.000000000000000000, 0.9659258262890683122, 1.000000000000000000, 0.9659258262890683122, 1.000000000000000000, 0.9659258262890683122, 1.000000000000000000, 0.9659258262890683122, 1.000000000000000000, 0.9659258262890683122, 1.000000000000000000, 0.9659258262890683122, 1.000000000000000000, 0.9659258262890683122, 1.000000000000000000, 0.9659258262890683122, 1.000000000000000000, 0.9659258262890683122, 1.000000000000000000, 0.9659258262890683122, 1.000000000000000000, 0.9659258262890683122, 1.000000000000000000, 0.9659258262890683122, 1.000000000000000000, 0.9659258262890683122, 1.000000000000000000, 0.9659258262890683122, 1.000000000000000000, 0.9659258262890683122, 1.000000000000000000, 0.9659258262890683122, 1.000000000000000000, 0.9659258262890683122, 1.000000000000000000, 0.9659258262890683122, 1.000000000000000000, 0.9659258262890683122, 1.000000000000000000, 0.9659258262890683122, 1.000000000000000000, 0.9659258262890683122, 1.000000000000000000, 0.9659258262890683122, 1.000000000000000000, 0.9659258262890683122, 1.000000000000000000, 0.9659258262890683122, 1.000000000000000000, 0.9659258262890683122, 1.000000000000000000, 0.9659258262890683122, 1.000000000000000000, 0.9659258262890683122, 1.000000000000000000, 0.9659258262890683122, 1.000000000000000000, 0.9659258262890683122, 1.000000000000000000, 0.9659258262890683122, 1.000000000000000000, 0.9659258262890683122, 1.000000000000000000, 0.9659258262890683122, 1.000000000000000000, 0.9659258262890683122, 1.000000000000000000, 0.9659258262890683122, 1.000000000000000000, 0.9659258262890683122, 1.000000000000000000, 0.9659258262890683122, 1.000000000000000000, 0.9659258262890683122, 1.000000000000000000, 0.9659258262890683122, 1.000000000000000000, 0.9659258262890683122, 1.000000000000000000, 0.9659258262890683122, 1.000000000000000000, 0.9659258262890683122, 1.000000000000000000, 0.9659258262890683122, 1.000000000000000000, 0.9659258262890683122, 1.000000000000000000, 0.9659258262890683122, 1.000000000000000000, 0.9659258262890683122, 1.000000000000000000, 0.9659258262890683122, 1.000000000000000000, 0.9659258262890683122, 1.000000000000000000, 0.9659258262890683122, 1.000000000000000000, 0.9659258262890683122, 1.000000000000000000, 0.9659258262890683122, 1.000000000000000000, 0.9659258262890683122, 1.000000000000000000, 0.9659258262890683122, 1.000000000000000000, 0.9659258262890683122, 1.000000000000000000, 0.9659258262890683122, 1.000000000000000000, 0.9659258262890683122, 1.000000000000000000, 0.9659258262890683122, 1.000000000000000000, 0.9659258262890683122, 1.000000000000000000, 0.9659258262890683122, 1.000000000000000000, 0.9659258262890683122, 1.000000000000000000, 0.9659258262890683122, 1.000000000000000000, 0.9659258262890683122, 1.000000000000000000, 0.9659258262890683122, 1.000000000000000000, 0.9659258262890683122, 1.000000000000000000, 0.9659258262890683122, 1.000000000000000000, 0.9659258262890683122, 1.000000000000000000, 0.9659258262890683122, 1.000000000000000000, 0.9659258262890683122, 1.000000000000000000, 0.9659258262890683122, 1.000000000000000000, 0.9659258262890683122, 1.000000000000000000, 0.9659258262890683122, 1.000000000000000000, 0.9659258262890683122, 1.000000000000000000, 0.9659258262890683122, 1.000000000000000000, 0.9659258262890683122, 1.000000000000000000, 0.9659258262890683122, 1.000000000000000000, 0.9659258262890683122, 1.000000000000000000, 0.9659258262890683122, 1.000000000000000000, 0.9659258262890683122, 1.000000000000000000, 0.9659258262890683122, 1.000000000000000000, 0.9659258262890683122, 1.000000000000000000, 0.9659258262890683122, 1.000000000000000000, 0.9659258262890683122, 1.000000000000000000, 0.9659258262890683122, 1.000000000000000000, 0.9659258262890683122, 1.000000000000000000, 0.9659258262890683122, 1.000000000000000000, 0.9659258262890683122, 1.000000000000000000, 0.9659258262890683122, 1.000000000000000000, 0.9659258262890683122, 1.000000000000000000, 0.9659258262890683122, 1.000000000000000000, 0.9659258262890683122, 1.000000000000000000, 0.9659258262890683122, 1.000000000000000000, 0.9659258262890683122, 1.000000000000000000, 0.9659258262890683122, 1.000000000000000000, 0.9659258262890683122, 1.000000000000000000, 0.9659258262890683122, 1.000000000000000000, 0.9659258262890683122, 1.000000000000000000, 0.9659258262890683122, 1.000000000000000000, 0.9659258262890683122, 1.000000000000000000, 0.9659258262890683122, 1.000000000000000000, 0.9659258262890683122, 1.000000000000000000, 0.9659258262890683122, 1.000000000000000000, 0.9659258262890683122, 1.000000000000000000, 0.9659258262890683122, 1.000000000000000000, 0.9659258262890683122, 1.000000000000000000, 0.9659258262890683122, 1.000000000000000000, 0.9659258262890683122, 1.000000000000000000, 0.9659258262890683122, 1.000000000000000000) ) ) 
 REPRESENTATION_ITEM ( '' )  SURFACE ( )  );
#16420=CARTESIAN_POINT ( 'NONE',  ( -1.167979002624671470, -0.4281496062992127816, -0.4176697321401328100 ) ) ;
#16422=CARTESIAN_POINT ( 'NONE',  ( 1.174540682414699111, -0.08942795157528024563, -0.3641732283464568787 ) ) ;
#16423=CARTESIAN_POINT ( 'NONE',  ( -0.01312335958005186876, 0.05413385826771626580, -0.4176697321401330321 ) ) ;
#16424=CARTESIAN_POINT ( 'NONE',  ( -0.4593175853018364174, -0.4281496062992127816, -0.4176697321401328100 ) ) ;
#16425=CARTESIAN_POINT ( 'NONE',  ( -0.3149606299212590610, -0.1870078740157480601, -0.3641732283464567677 ) ) ;
#16427=CARTESIAN_POINT ( 'NONE',  ( -0.5052493438320203589, 0.1771653543307087075, -0.09757992244046823083 ) ) ;
#16428=CARTESIAN_POINT ( 'NONE',  ( 0.4593175853018380828, 0.05413385826771626580, -0.4176697321401330321 ) ) ;
#16429=CARTESIAN_POINT ( 'NONE',  ( -1.227034120734907585, 0.1771653543307087630, 0.09757992244046791164 ) ) ;
#16431=CARTESIAN_POINT ( 'NONE',  ( -1.122047244094487306, 0.1660481256975883668, -0.3530559997133364547 ) ) ;
#16434=CARTESIAN_POINT ( 'NONE',  ( -1.587926509186350810, -0.3690944881889763329, 0.3153832671262228327 ) ) ;
#16436=CARTESIAN_POINT ( 'NONE',  ( -0.6167979002624665030, 0.05413385826771666132, 0.4176697321401328100 ) ) ;
#16438=CARTESIAN_POINT ( 'NONE',  ( -1.200787401574802349, -0.5400638737290844871, 0.3530559997133364547 ) ) ;
#16441=CARTESIAN_POINT ( 'NONE',  ( 1.489501312335958172, -0.3162353388693405765, 0.4822834645669290543 ) ) ;
#16442=CARTESIAN_POINT ( 'NONE',  ( 0.4002624671916016896, -0.05778040916215522460, 0.4822834645669289988 ) ) ;
#16443=CARTESIAN_POINT ( 'NONE',  ( -1.646051170424378096, 0.8346805926620876059, -0.3149606299212598381 ) ) ;
#16445=CARTESIAN_POINT ( 'NONE',  ( -1.712598425196849572, 0.1660481256975885056, 0.3530559997133364547 ) ) ;
#16448=CARTESIAN_POINT ( 'NONE',  ( -0.8661417322834640276, -0.1870078740157479769, 0.3641732283464567677 ) ) ;
#16451=CARTESIAN_POINT ( 'NONE',  ( 0.8070866141732288002, 0.1660481256975885056, 0.3530559997133364547 ) ) ;
#16452=CARTESIAN_POINT ( 'NONE',  ( -0.4986876640419942164, -0.6046776061558807314, 0.2411417322834647770 ) ) ;
#16453=CARTESIAN_POINT ( 'NONE',  ( -1.049868766404198794, -0.6046776061558807314, 0.2411417322834647770 ) ) ;
#16454=CARTESIAN_POINT ( 'NONE',  ( 1.181102362204725198, -0.1870078740157479769, 0.4822834645669291653 ) ) ;
#16455=CARTESIAN_POINT ( 'NONE',  ( -1.384514435695537005, -0.5511811023622048555, -0.09757992244046775898 ) ) ;
#16456=CARTESIAN_POINT ( 'NONE',  ( 0.6867064689427456736, 2.290696638571109833, -0.1693427315076261597 ) ) ;
#16457=CARTESIAN_POINT ( 'NONE',  ( 0.3412073490813655186, -0.6046776061558809534, -0.2411417322834644161 ) ) ;
#16458=CARTESIAN_POINT ( 'NONE',  ( -0.8267716535433065062, 0.2952755905511811885, 0.000000000000000000 ) ) ;
#16460=CARTESIAN_POINT ( 'NONE',  ( -1.082677165354329896, -0.5400638737290845981, -0.3530559997133363437 ) ) ;
#16461=DIRECTION ( 'NONE',  ( 0.000000000000000000, 0.000000000000000000, 1.000000000000000000 ) ) ;
#16462=CARTESIAN_POINT ( 'NONE',  ( 0.7874015748031503170, -0.1870078740157480879, -0.4822834645669291653 ) ) ;
#16464=CARTESIAN_POINT ( 'NONE',  ( 1.318897637795276356, -0.4536011799217367080, 0.2665933059059888421 ) ) ;
#16467=CARTESIAN_POINT ( 'NONE',  ( -0.3740157480314953431, 0.1660481256975885056, 0.3530559997133364547 ) ) ;
#16469=CARTESIAN_POINT ( 'NONE',  ( 0.3412073490813655186, 0.1283753931104748280, 0.1820866141732283561 ) ) ;
#16470=CARTESIAN_POINT ( 'NONE',  ( -1.535433070866141225, 0.2952755905511811885, 0.000000000000000000 ) ) ;
#16471=CARTESIAN_POINT ( 'NONE',  ( 0.9842519685039375910, 0.2952755905511811885, 0.000000000000000000 ) ) ;
#16472=CARTESIAN_POINT ( 'NONE',  ( 0.9186351706036751663, -0.6046776061558807314, 0.2411417322834647770 ) ) ;
#16473=CARTESIAN_POINT ( 'NONE',  ( 0.01312335958005323398, 0.05413385826771666132, 0.4176697321401328100 ) ) ;
#16475=CARTESIAN_POINT ( 'NONE',  ( -0.6889763779527552368, 0.1660481256975885056, 0.3530559997133364547 ) ) ;
#16477=CARTESIAN_POINT ( 'NONE',  ( -1.627296587926508442, -0.6046776061558809534, -0.2411417322834644161 ) ) ;
#16478=CARTESIAN_POINT ( 'NONE',  ( -1.089238845144356427, -0.4281496062992127816, -0.4176697321401328100 ) ) ;
#16479=CARTESIAN_POINT ( 'NONE',  ( 1.246719160104987623, 0.05413385826771626580, -0.4176697321401330321 ) ) ;
#16481=CARTESIAN_POINT ( 'NONE',  ( -0.8398950131233589023, -0.6046776061558809534, -0.2411417322834644161 ) ) ;
#16483=CARTESIAN_POINT ( 'NONE',  ( 0.3018372703412079971, -0.4281496062992124485, 0.4176697321401328655 ) ) ;
#16486=CARTESIAN_POINT ( 'NONE',  ( -0.6496062992125976043, 0.1660481256975883668, -0.3530559997133364547 ) ) ;
#16487=CARTESIAN_POINT ( 'NONE',  ( -1.502624671916009680, -0.2845877964562159024, 0.3641732283464567677 ) ) ;
#16488=CARTESIAN_POINT ( 'NONE',  ( 0.6299212598425204535, -0.1870078740157480601, -0.3641732283464567677 ) ) ;
#16489=CARTESIAN_POINT ( 'NONE',  ( 1.430446194225722500, 0.05413385826771666132, 0.4176697321401328100 ) ) ;
#16491=CARTESIAN_POINT ( 'NONE',  ( 0.8792650918635177559, -0.004921259842519576551, 0.3153832671262227771 ) ) ;
#16492=CARTESIAN_POINT ( 'NONE',  ( 0.5971128608923890191, -0.6692913385826771977, 0.1292274648535927661 ) ) ;
#16494=EDGE_CURVE ( 'NONE', #21005, #64347, #10386, .T. ) ;
#16496=CARTESIAN_POINT ( 'NONE',  ( -0.2296587926509179312, -0.3162353388693409650, -0.4822834645669289433 ) ) ;
#16498=CARTESIAN_POINT ( 'NONE',  ( 1.463254593175853824, 0.1771653543307087075, -0.09757992244046823083 ) ) ;
#16499=CARTESIAN_POINT ( 'NONE',  ( -0.7152230971128602510, -0.05778040916215560624, -0.4822834645669293319 ) ) ;
#16501=CARTESIAN_POINT ( 'NONE',  ( 1.253280839895013710, -0.05778040916215560624, -0.4822834645669293319 ) ) ;
#16502=CARTESIAN_POINT ( 'NONE',  ( 0.1509186351706042484, -0.3162353388693405765, 0.4822834645669290543 ) ) ;
#16504=CARTESIAN_POINT ( 'NONE',  ( 0.3608923884514443348, -0.5511811023622046335, 0.09757992244046803654 ) ) ;
#16506=CARTESIAN_POINT ( 'NONE',  ( -0.07217847769028787330, -0.08942795157527998196, 0.3641732283464567121 ) ) ;
#16507=CARTESIAN_POINT ( 'NONE',  ( 0.8070866141732288002, 0.07958543189024085140, 0.2665933059059887866 ) ) ;
#16508=CARTESIAN_POINT ( 'NONE',  ( -1.633858267716534529, 0.1660481256975885056, 0.3530559997133364547 ) ) ;
#16510=CARTESIAN_POINT ( 'NONE',  ( 0.9514435695538062676, -0.3162353388693409650, -0.4822834645669289433 ) ) ;
#16512=CARTESIAN_POINT ( 'NONE',  ( 1.646981627296588035, -0.2845877964562159024, 0.3641732283464567677 ) ) ;
#16514=CARTESIAN_POINT ( 'NONE',  ( 0.006561679790026889343, -0.08942795157527998196, 0.3641732283464567121 ) ) ;
#16515=CARTESIAN_POINT ( 'NONE',  ( 0.04593175853018440641, -0.6692913385826771977, 0.1292274648535927661 ) ) ;
#16516=CARTESIAN_POINT ( 'NONE',  ( 1.463254593175853824, -0.5511811023622046335, 0.09757992244046803654 ) ) ;
#16517=CARTESIAN_POINT ( 'NONE',  ( -1.213910761154854745, 0.1771653543307087075, -0.09757992244046823083 ) ) ;
#16518=CARTESIAN_POINT ( 'NONE',  ( -1.371391076115484831, 0.2952755905511810774, -0.1292274648535930714 ) ) ;
#16519=CARTESIAN_POINT ( 'NONE',  ( 0.7283464566929143125, 0.1660481256975885056, 0.3530559997133364547 ) ) ;
#16520=CARTESIAN_POINT ( 'NONE',  ( 1.181102362204725198, -0.1870078740157479769, 0.4822834645669291653 ) ) ;
#16522=CARTESIAN_POINT ( 'NONE',  ( -0.02624671916010428221, -0.6046776061558807314, 0.2411417322834647770 ) ) ;
#16523=CARTESIAN_POINT ( 'NONE',  ( 1.391076115485564868, 0.2306618581243847221, -0.2411417322834647770 ) ) ;
#16524=CARTESIAN_POINT ( 'NONE',  ( 0.9776902887139113929, -0.6692913385826773087, -0.1292274648535924053 ) ) ;
#16525=CIRCLE ( 'NONE', #45589, 2.401574803149606474 ) ;
#16527=CARTESIAN_POINT ( 'NONE',  ( 0.9448818897637802916, -0.1870078740157480601, -0.3641732283464567677 ) ) ;
#16528=CARTESIAN_POINT ( 'NONE',  ( 1.666666666666667185, 0.05413385826771666132, 0.4176697321401328100 ) ) ;
#16529=CARTESIAN_POINT ( 'NONE',  ( 0.03280839895013198948, 0.1771653543307087630, 0.09757992244046791164 ) ) ;
#16530=CARTESIAN_POINT ( 'NONE',  ( 0.05249343832021075018, -0.6046776061558807314, 0.2411417322834647770 ) ) ;
#16531=CARTESIAN_POINT ( 'NONE',  ( 0.7414698162729663755, -0.6692913385826773087, -0.1292274648535924053 ) ) ;
#16532=CARTESIAN_POINT ( 'NONE',  ( -0.1640419947506553400, -0.05778040916215560624, -0.4822834645669293319 ) ) ;
#16533=CARTESIAN_POINT ( 'NONE',  ( -0.1312335958005241554, 0.1283753931104748280, 0.1820866141732283561 ) ) ;
#16534=CARTESIAN_POINT ( 'NONE',  ( 0.6627296587926515548, 0.2952755905511811885, 0.1292274648535926551 ) ) ;
#16535=CARTESIAN_POINT ( 'NONE',  ( 0.7611548556430454138, 0.1283753931104746893, -0.1820866141732285504 ) ) ;
#16540=CARTESIAN_POINT ( 'NONE',  ( -1.128608923884513837, 0.2306618581243847221, -0.2411417322834647770 ) ) ;
#16541=CARTESIAN_POINT ( 'NONE',  ( -0.4396325459317579898, 0.2952755905511811885, 0.1292274648535926551 ) ) ;
#16545=CARTESIAN_POINT ( 'NONE',  ( 0.5577427821522316087, -0.08942795157527998196, 0.3641732283464567121 ) ) ;
#16547=CARTESIAN_POINT ( 'NONE',  ( 1.299212598425197429, 0.2952755905511811885, 0.000000000000000000 ) ) ;
#16550=DIRECTION ( 'NONE',  ( 0.000000000000000000, 1.000000000000000000, 0.000000000000000000 ) ) ;
#16551=CARTESIAN_POINT ( 'NONE',  ( -1.213910761154854745, 0.1771653543307087075, -0.09757992244046823083 ) ) ;
#16553=CARTESIAN_POINT ( 'NONE',  ( 1.397637795275591177, -0.4536011799217367080, 0.2665933059059888421 ) ) ;
#16554=CARTESIAN_POINT ( 'NONE',  ( 0.2493438320209980519, 0.05413385826771666132, 0.4176697321401328100 ) ) ;
#16556=CARTESIAN_POINT ( 'NONE',  ( 0.1246719160104994284, 0.2952755905511810774, -0.1292274648535930714 ) ) ;
#16557=CARTESIAN_POINT ( 'NONE',  ( -0.9645669291338575535, -0.4536011799217367080, 0.2665933059059888421 ) ) ;
#16558=CARTESIAN_POINT ( 'NONE',  ( 0.3149606299212603933, -0.1870078740157479769, 0.4822834645669291653 ) ) ;
#16559=CARTESIAN_POINT ( 'NONE',  ( -0.2427821522309703550, -0.05778040916215560624, -0.4822834645669293319 ) ) ;
#16563=CARTESIAN_POINT ( 'NONE',  ( 0.9055118110236227702, 0.2952755905511811885, 0.000000000000000000 ) ) ;
#16564=CARTESIAN_POINT ( 'NONE',  ( -0.4593175853018366950, 0.05413385826771666132, 0.4176697321401328100 ) ) ;
#16565=CARTESIAN_POINT ( 'NONE',  ( -1.082677165354329896, -0.5400638737290845981, -0.3530559997133363437 ) ) ;
#16566=CARTESIAN_POINT ( 'NONE',  ( 1.279527559055118724, 0.1660481256975885056, 0.3530559997133364547 ) ) ;
#16567=CARTESIAN_POINT ( 'NONE',  ( 0.4002624671916016896, -0.05778040916215522460, 0.4822834645669289988 ) ) ;
#16569=CARTESIAN_POINT ( 'NONE',  ( -0.5249343832020990641, -0.6046776061558809534, -0.2411417322834644161 ) ) ;
#16570=CARTESIAN_POINT ( 'NONE',  ( 0.4199475065616805614, 0.2306618581243848609, 0.2411417322834645549 ) ) ;
#16571=CARTESIAN_POINT ( 'NONE',  ( -0.4593175853018364174, -0.4281496062992127816, -0.4176697321401328100 ) ) ;
#16572=CARTESIAN_POINT ( 'NONE',  ( 0.7677165354330716118, 0.07958543189024071263, -0.2665933059059888421 ) ) ;
#16573=CARTESIAN_POINT ( 'NONE',  ( -1.666666666666665853, 0.05413385826771626580, -0.4176697321401330321 ) ) ;
#16575=CARTESIAN_POINT ( 'NONE',  ( 0.2624671916010504757, -0.6046776061558809534, -0.2411417322834644161 ) ) ;
#16578=ORIENTED_EDGE ( 'NONE', *, *, #43922, .F. ) ;
#16580=CARTESIAN_POINT ( 'NONE',  ( 0.5380577427821529035, -0.4281496062992124485, 0.4176697321401328655 ) ) ;
#16581=CARTESIAN_POINT ( 'NONE',  ( 0.3871391076115492380, -0.08942795157528024563, -0.3641732283464568787 ) ) ;
#16582=CARTESIAN_POINT ( 'NONE',  ( 0.9555810825238854056, -8.614921172258640174E-17, 0.4118477457932991359 ) ) ;
#16587=CARTESIAN_POINT ( 'NONE',  ( 0.8923884514435701520, -0.6046776061558809534, -0.2411417322834644161 ) ) ;
#16588=CARTESIAN_POINT ( 'NONE',  ( -0.7152230971128602510, -0.3162353388693405765, 0.4822834645669290543 ) ) ;
#16590=CARTESIAN_POINT ( 'NONE',  ( -0.6233595800524928121, -0.05778040916215522460, 0.4822834645669289988 ) ) ;
#16591=CARTESIAN_POINT ( 'NONE',  ( 0.6496062992125991586, 0.1660481256975885056, 0.3530559997133364547 ) ) ;
#16592=CARTESIAN_POINT ( 'NONE',  ( 1.351706036745407458, -0.4281496062992127816, -0.4176697321401328100 ) ) ;
#16594=CARTESIAN_POINT ( 'NONE',  ( 1.351706036745407680, -0.004921259842519576551, 0.3153832671262227771 ) ) ;
#16596=CARTESIAN_POINT ( 'NONE',  ( -1.272965879265091305, -0.004921259842519870586, -0.3153832671262229437 ) ) ;
#16598=CARTESIAN_POINT ( 'NONE',  ( -0.01968503937007793844, 0.1660481256975883668, -0.3530559997133364547 ) ) ;
#16600=LINE ( 'NONE', #67523, #2260 ) ;
#16601=CARTESIAN_POINT ( 'NONE',  ( -1.345144356955379816, -0.08942795157528024563, -0.3641732283464568787 ) ) ;
#16602=( BOUNDED_CURVE ( )  B_SPLINE_CURVE ( 2, ( #79476, #77807, #27695, #79069, #20138, #71485, #13832, #7935, #20970, #65178, #33596, #27274, #66008 ),
 .UNSPECIFIED., .F., .F. ) 
 B_SPLINE_CURVE_WITH_KNOTS ( ( 3, 2, 2, 2, 2, 2, 3 ),
 ( 0.2763059932978689792, 0.2765151515151514916, 0.2803030303030303871, 0.2840909090909091717, 0.2878787878787879562, 0.2916666666666667407, 0.2918758248839492531 ),
 .UNSPECIFIED. ) 
 CURVE ( )  GEOMETRIC_REPRESENTATION_ITEM ( )  RATIONAL_B_SPLINE_CURVE ( ( 0.9964447847208419695, 0.9981185001348091834, 1.000000000000000000, 0.9659258262890683122, 1.000000000000000000, 0.9659258262890683122, 1.000000000000000000, 0.9659258262890683122, 1.000000000000000000, 0.9659258262890683122, 1.000000000000000000, 0.9981185001348091834, 0.9964447847208420805 ) ) 
 REPRESENTATION_ITEM ( '' )  );
#16603=CARTESIAN_POINT ( 'NONE',  ( 0.1902887139107617975, -0.6692913385826773087, -0.1292274648535924053 ) ) ;
#16604=CARTESIAN_POINT ( 'NONE',  ( 1.141732283464567566, 0.1771653543307087630, 0.000000000000000000 ) ) ;
#16607=CARTESIAN_POINT ( 'NONE',  ( -1.220472440944881054, 0.1771653543307087630, 0.000000000000000000 ) ) ;
#16608=CARTESIAN_POINT ( 'NONE',  ( 1.246719160104987623, 0.05413385826771626580, -0.4176697321401330321 ) ) ;
#16610=CARTESIAN_POINT ( 'NONE',  ( -0.03937007874015669567, -0.6692913385826771977, 8.415575281601705876E-17 ) ) ;
#16611=CARTESIAN_POINT ( 'NONE',  ( -1.443569553805773564, 0.1283753931104746893, -0.1820866141732285504 ) ) ;
#16612=EDGE_CURVE ( 'NONE', #79410, #37352, #40814, .T. ) ;
#16613=CARTESIAN_POINT ( 'NONE',  ( -0.7677165354330699465, 0.1660481256975885056, 0.3530559997133364547 ) ) ;
#16614=CARTESIAN_POINT ( 'NONE',  ( -1.384514435695537005, -0.5511811023622048555, -0.09757992244046775898 ) ) ;
#16616=CARTESIAN_POINT ( 'NONE',  ( 0.3608923884514443348, 0.2952755905511810774, -0.1292274648535930714 ) ) ;
#16618=CARTESIAN_POINT ( 'NONE',  ( 1.246719160104987623, -0.4281496062992124485, 0.4176697321401328655 ) ) ;
#16620=CARTESIAN_POINT ( 'NONE',  ( -1.259842519685038686, -0.1870078740157479769, 0.4822834645669291653 ) ) ;
#16621=CARTESIAN_POINT ( 'NONE',  ( -0.4527559055118102749, 0.07958543189024085140, 0.2665933059059887866 ) ) ;
#16622=CARTESIAN_POINT ( 'NONE',  ( -0.5183727034120726440, 0.2066929133858267931, 0.1054918080437490802 ) ) ;
#16623=CARTESIAN_POINT ( 'NONE',  ( 0.09186351706036827158, 0.05413385826771666132, 0.4176697321401328100 ) ) ;
#16624=CARTESIAN_POINT ( 'NONE',  ( 0.2165354330708668673, -0.4536011799217367080, 0.2665933059059888421 ) ) ;
#16625=CARTESIAN_POINT ( 'NONE',  ( -1.095800524934382292, -0.08942795157527998196, 0.3641732283464567121 ) ) ;
#16626=CARTESIAN_POINT ( 'NONE',  ( -1.515748031496062076, 0.1660481256975883668, -0.3530559997133364547 ) ) ;
#16627=CARTESIAN_POINT ( 'NONE',  ( 1.555118110236221041, -0.4536011799217367080, 0.2665933059059888421 ) ) ;
#16628=CARTESIAN_POINT ( 'NONE',  ( 1.430446194225722500, -0.4281496062992127816, -0.4176697321401328100 ) ) ;
#16630=CARTESIAN_POINT ( 'NONE',  ( 0.3280839895013130669, -0.3690944881889765550, -0.3153832671262227771 ) ) ;
#16631=CARTESIAN_POINT ( 'NONE',  ( 0.8661417322834653598, -0.1870078740157479769, 0.4822834645669291653 ) ) ;
#16633=CARTESIAN_POINT ( 'NONE',  ( 1.023622047244095112, -0.1870078740157480601, -0.3641732283464567677 ) ) ;
#16634=ORIENTED_EDGE ( 'NONE', *, *, #41785, .F. ) ;
#16635=EDGE_CURVE ( 'NONE', #23493, #43326, #68968, .T. ) ;
#16636=CARTESIAN_POINT ( 'NONE',  ( -1.272965879265091305, 0.05413385826771626580, -0.4176697321401330321 ) ) ;
#16637=EDGE_CURVE ( 'NONE', #8180, #8792, #60187, .T. ) ;
#16638=CARTESIAN_POINT ( 'NONE',  ( -0.8727034120734901146, -0.3162353388693405765, 0.4822834645669290543 ) ) ;
#16639=CARTESIAN_POINT ( 'NONE',  ( 0.2493438320209980519, -0.4281496062992127816, -0.4176697321401328100 ) ) ;
#16642=CARTESIAN_POINT ( 'NONE',  ( 0.8005249343832027131, 0.05413385826771666132, 0.4176697321401328100 ) ) ;
#16643=CARTESIAN_POINT ( 'NONE',  ( 1.502624671916010790, -0.2845877964562161244, -0.3641732283464567121 ) ) ;
#16644=CARTESIAN_POINT ( 'NONE',  ( 0.02624671916010564918, -0.6046776061558809534, -0.2411417322834644161 ) ) ;
#16645=CARTESIAN_POINT ( 'NONE',  ( 0.8661417322834652488, -0.1870078740157480879, -0.4822834645669291653 ) ) ;
#16652=CARTESIAN_POINT ( 'NONE',  ( -0.2165354330708654795, -0.4536011799217368745, -0.2665933059059886201 ) ) ;
#16653=CARTESIAN_POINT ( 'NONE',  ( -0.5380577427821514602, -0.4281496062992127816, -0.4176697321401328100 ) ) ;
#16654=CARTESIAN_POINT ( 'NONE',  ( 1.003937007874016185, 0.1660481256975883668, -0.3530559997133364547 ) ) ;
#16656=CARTESIAN_POINT ( 'NONE',  ( 0.06561679790026316017, -0.3690944881889763329, 0.3153832671262228327 ) ) ;
#16657=CARTESIAN_POINT ( 'NONE',  ( -1.272965879265091305, 0.05413385826771626580, -0.4176697321401330321 ) ) ;
#16658=CARTESIAN_POINT ( 'NONE',  ( 1.253280839895013710, -0.3162353388693405765, 0.4822834645669290543 ) ) ;
#16662=VERTEX_POINT ( 'NONE', #29422 ) ;
#16663=CARTESIAN_POINT ( 'NONE',  ( 1.213910761154856299, -0.6692913385826773087, -0.1292274648535924053 ) ) ;
#16665=CARTESIAN_POINT ( 'NONE',  ( 1.233595800524935227, -0.5023911411419708095, 0.1820866141732285504 ) ) ;
#16666=CARTESIAN_POINT ( 'NONE',  ( -1.633858267716534529, 0.07958543189024085140, 0.2665933059059887866 ) ) ;
#16667=CARTESIAN_POINT ( 'NONE',  ( 1.476377952755906220, 0.1660481256975883668, -0.3530559997133364547 ) ) ;
#16669=CARTESIAN_POINT ( 'NONE',  ( -0.9573014326657163231, -2.609869883881465018E-15, -0.3464511005275220379 ) ) ;
#16670=CARTESIAN_POINT ( 'NONE',  ( 1.174540682414699111, -0.3162353388693405765, 0.4822834645669290543 ) ) ;
#16671=CARTESIAN_POINT ( 'NONE',  ( -1.535433070866141225, 0.2952755905511811885, 0.000000000000000000 ) ) ;
#16672=CARTESIAN_POINT ( 'NONE',  ( -0.6430446194225716283, -0.4281496062992124485, 0.4176697321401328655 ) ) ;
#16673=CARTESIAN_POINT ( 'NONE',  ( -0.7611548556430438595, 0.2306618581243848609, 0.2411417322834645549 ) ) ;
#16674=CARTESIAN_POINT ( 'NONE',  ( 1.489501312335958172, -0.05778040916215560624, -0.4822834645669293319 ) ) ;
#16676=CARTESIAN_POINT ( 'NONE',  ( 0.04593175853018440641, 0.2952755905511810774, -0.1292274648535930714 ) ) ;
#16678=CARTESIAN_POINT ( 'NONE',  ( -1.594488188976377119, 0.07958543189024071263, -0.2665933059059888421 ) ) ;
#16682=CARTESIAN_POINT ( 'NONE',  ( 0.3937007874015751585, 1.535433070866141447, 0.000000000000000000 ) ) ;
#16683=CARTESIAN_POINT ( 'NONE',  ( -1.614173228346456268, -0.6692913385826771977, 8.415575281601705876E-17 ) ) ;
#16685=CARTESIAN_POINT ( 'NONE',  ( 1.660104986876641320, -0.08942795157527998196, 0.3641732283464567121 ) ) ;
#16688=DIRECTION ( 'NONE',  ( -3.096699300667737957E-16, 1.000000000000000000, -0.000000000000000000 ) ) ;
#16690=CARTESIAN_POINT ( 'NONE',  ( -0.5118110236220466680, 0.1771653543307087630, 0.000000000000000000 ) ) ;
#16691=CARTESIAN_POINT ( 'NONE',  ( -1.095800524934382292, -0.08942795157527998196, 0.3641732283464567121 ) ) ;
#16692=CARTESIAN_POINT ( 'NONE',  ( 1.476377952755906220, 0.1660481256975883668, -0.3530559997133364547 ) ) ;
#16693=CARTESIAN_POINT ( 'NONE',  ( 0.3412073490813655186, 0.2306618581243848609, 0.2411417322834645549 ) ) ;
#16694=CARTESIAN_POINT ( 'NONE',  ( -1.253280839895012377, -0.3162353388693409650, -0.4822834645669289433 ) ) ;
#16696=EDGE_LOOP ( 'NONE', ( #13116, #29716, #38808, #56286 ) ) ;
#16697=CARTESIAN_POINT ( 'NONE',  ( -1.312335958005248715, 0.2306618581243848609, 0.2411417322834645549 ) ) ;
#16702=DIRECTION ( 'NONE',  ( 1.000000000000000000, -0.000000000000000000, -0.000000000000000000 ) ) ;
#16703=CARTESIAN_POINT ( 'NONE',  ( -0.6561679790026240244, 0.2306618581243847221, -0.2411417322834647770 ) ) ;
#16704=CARTESIAN_POINT ( 'NONE',  ( 1.404199475065617708, 0.05413385826771626580, -0.4176697321401330321 ) ) ;
#16705=CARTESIAN_POINT ( 'NONE',  ( -1.640419947506561060, -0.4281496062992127816, -0.4176697321401328100 ) ) ;
#16706=FACE_OUTER_BOUND ( 'NONE', #35608, .T. ) ;
#16707=CARTESIAN_POINT ( 'NONE',  ( 1.633858267716535639, -0.5400638737290844871, 0.3530559997133364547 ) ) ;
#16708=CARTESIAN_POINT ( 'NONE',  ( -0.6299212598425188991, -0.1870078740157479769, 0.4822834645669291653 ) ) ;
#16710=CARTESIAN_POINT ( 'NONE',  ( -0.1181102362204717315, 0.1771653543307087630, 0.000000000000000000 ) ) ;
#16712=VECTOR ( 'NONE', #41094, 39.37007874015748854 ) ;
#16713=CARTESIAN_POINT ( 'NONE',  ( -0.2952755905511803003, -0.4536011799217368745, -0.2665933059059886201 ) ) ;
#16714=CARTESIAN_POINT ( 'NONE',  ( 0.8792650918635177559, -0.3690944881889765550, -0.3153832671262227771 ) ) ;
#16715=CARTESIAN_POINT ( 'NONE',  ( 0.5314960629921264834, 0.1660481256975883668, -0.3530559997133364547 ) ) ;
#16716=CARTESIAN_POINT ( 'NONE',  ( -0.09186351706036663400, -0.3690944881889763329, 0.3153832671262228327 ) ) ;
#16718=CARTESIAN_POINT ( 'NONE',  ( 1.607611548556431069, 0.2952755905511811885, 0.1292274648535926551 ) ) ;
#16719=CARTESIAN_POINT ( 'NONE',  ( -0.9908136482939626788, 0.2952755905511811885, 0.1292274648535926551 ) ) ;
#16721=CARTESIAN_POINT ( 'NONE',  ( 0.09186351706036799403, -0.4281496062992127816, -0.4176697321401328100 ) ) ;
#16722=CARTESIAN_POINT ( 'NONE',  ( -0.6496062992125976043, 0.1660481256975883668, -0.3530559997133364547 ) ) ;
#16725=CARTESIAN_POINT ( 'NONE',  ( 0.1443569553805781891, -0.3690944881889763329, 0.3153832671262228327 ) ) ;
#16726=CARTESIAN_POINT ( 'NONE',  ( -0.2230971128608915943, -0.4281496062992127816, -0.4176697321401328100 ) ) ;
#16727=CARTESIAN_POINT ( 'NONE',  ( -0.7480314960629914633, -0.6692913385826771977, 8.415575281601705876E-17 ) ) ;
#16728=CARTESIAN_POINT ( 'NONE',  ( -1.646051170424378096, 0.4405861044731112508, -0.3149606299212598381 ) ) ;
#16729=CARTESIAN_POINT ( 'NONE',  ( 1.614173228346457378, -0.5511811023622047445, 6.969142054262312111E-17 ) ) ;
#16730=CARTESIAN_POINT ( 'NONE',  ( 0.2821522309711292364, 0.2952755905511810774, -0.1292274648535930714 ) ) ;
#16731=ORIENTED_EDGE ( 'NONE', *, *, #24704, .F. ) ;
#16733=( BOUNDED_SURFACE ( )  B_SPLINE_SURFACE ( 1, 2, ( 
 ( #65346, #46372, #19457, #32498, #64491, #7251, #20300, #1369, #63657, #45949, #51845, #12737, #530, #71231, #70813, #58162, #39655, #27021, #13998, #32923, #58589, #25345, #13575, #25760, #52264, #39229, #957, #77970, #20721, #37982, #52682, #5996, #31667, #51422, #51007, #57328, #70382, #76706, #38396, #64076, #6413, #32083, #57744, #106, #77124, #45108, #72895, #53521, #53932, #3436, #48038, #48446, #59422, #33760, #34599, #59840, #3021, #35008, #72483, #2193, #34176, #47620, #79228, #15245, #15663, #60264, #8922, #73316, #8096, #67005, #41324, #2613, #40905, #53098, #66586, #54349, #1778, #16075, #79644, #8510, #27436, #78808, #29098, #28688, #60673, #28270, #14425, #9337, #21961, #21137, #80060, #46792, #22378, #14832, #21544, #73740, #41721, #67414, #9748, #40492, #66170, #35420, #27861, #61085, #54770, #47205, #80474, #22786, #40076, #65763, #80880, #16909, #36241, #37060, #61911, #81289, #18132, #82515, #55579, #42950, #74977, #17726, #56412, #69470, #16491, #82111, #4656, #48863, #36643, #30329, #23605, #49274, #75790, #11823, #50094, #43352, #69054, #35836, #17322, #4253, #62744, #10983, #11403, #62319, #31150, #74146, #37475, #63148, #56816, #29915, #61503, #81707, #55171, #24424, #24017, #74563, #5080, #5489, #30749, #24831, #49685, #75377, #68644, #55995, #43765, #42137, #67832, #10171, #3850, #29510, #23192, #42547, #68250, #10584, #25247, #12637, #70284, #427, #6309, #25661, #51743, #70708, #45008, #26083, #44184, #19779, #77446, #13060, #51323, #5895, #77026, #7148, #69876, #52164, #32398, #44590, #12229, #37886, #39553, #64809, #13471, #19359, #1273, #45433, #38714, #31567, #64392, #63561, #71128, #57225, #58061, #18942, #65242, #39128, #6728, #26510, #32821, #58488, #50911, #853, #7580, #77868, #20197, #45848, #71547, #13894, #76612, #33252, #58914, #82926, #57646, #50500, #76203, #18541, #38296, #63973, #31986, #9, #46694, #60162, #41223, #7997, #9241, #72794, #73213, #53830, #33661, #52997, #72387, #15563, #14737, #34075, #54247, #35322, #8408, #79131, #27758, #79544, #34913, #22277, #52581, #60576, #40800, #1680, #15144, #66485, #59739, #2093, #28591, #47937, #2927, #21857, #47521, #71968, #53422, #40389, #66910, #47105, #79964, #8820, #67318, #26921, #73640, #15982, #9653, #66072, #14323, #34497, #59324, #41629, #2514, #27337, #60985, #78290, #20621, #46273, #28173, #39981, #21448, #65671, #78710, #21034, #38091, #38509, #48348, #22689, #24638, #49897, #76413, #25041, #62538, #75596, #24226, #37681, #43571, #62955, #5691, #50305, #82318, #63357, #80376, #57027, #31361, #76003, #5291, #42039, #30952, #44386, #74045, #6106, #69682, #81914, #16392, #67733, #76815, #18743, #50714, #56619, #3335, #82721, #18345, #10068, #43985, #35731, #70079, #4876, #12025, #56215, #19147, #30549, #12432, #17935, #63765, #54665, #11618, #31779, #69272, #57441, #37279, #44797, #83134, #70493, #25453, #51120, #12850, #28999, #39336, #8198, #27545, #71336, #14528, #20408, #65023, #45223, #59528, #1885, #7358, #78077, #51532, #13683, #64191, #33027, #58696, #1061, #20823, #14933, #53202, #26714, #1473, #6526, #52369, #219, #46059, #6938, #78915, #70924, #71753, #40180, #32610, #33454, #14107, #39759, #27127, #65864, #13270, #65455, #21236, #64603, #7787, #33864, #32195, #59115, #52791, #78500, #38922, #57852, #45641, #46476, #637, #58272, #72172, #46892, #72586, #25870, #77235, #19564, #26292, #51953, #77658, #19990, #48557, #41012, #22889, #15773, #27961, #55279, #54035, #80582, #67936, #41829, #79328, #74672, #74254, #54455, #47725, #22483, #10277, #80167, #67519, #28792, #2713, #66696, #16596, #48145, #35526, #9031, #66274, #47308, #28374, #42241, #35944, #3956, #2301, #79748, #41424, #73842, #16182, #53620, #9856, #60366, #72998, #21648, #61188, #61614, #29618, #34283, #3543, #29210, #15350, #67108, #22065, #54876, #60776, #80989, #3127, #23302, #40592, #48972, #8613, #59945, #73423, #34704, #9439, #35110, #82626, #24540, #75081, #63256, #37994, #43883, #57341, #50205, #18242, #75496, #56109, #56518, #6011, #50611, #51023, #62023, #36348 ),
 ( #63670, #24125, #76318, #82221, #17835, #81399, #12338, #31681, #43469, #30854, #4360, #49794, #17016, #69166, #11517, #37173, #56930, #42656, #83036, #62853, #37583, #68353, #5189, #30028, #75902, #43059, #25360, #23715, #69581, #18648, #68756, #11928, #5597, #31263, #24940, #44292, #49386, #69983, #10693, #17428, #55691, #11098, #36756, #62431, #4769, #30444, #81814, #76722, #58177, #59029, #13179, #121, #71663, #72081, #33366, #26627, #58604, #27037, #52698, #14440, #45549, #20737, #1384, #77140, #78406, #51860, #64093, #8111, #6845, #46388, #40092, #77986, #32098, #27453, #65779, #7267, #546, #973, #33777, #77567, #57759, #59440, #1793, #19901, #32939, #6429, #26199, #19054, #71246, #13590, #39246, #44701, #70398, #12754, #64929, #14014, #38411, #52281, #25776, #20315, #19473, #51437, #45123, #45966, #70831, #38828, #39671, #65361, #7699, #64506, #32515, #34192, #73333, #16510, #53536, #2629, #22804, #53114, #28285, #3038, #53947, #27876, #78823, #34614, #35435, #72910, #59856, #48054, #48462, #9764, #28703, #35024, #3451, #29115, #74162, #21976, #80489, #61100, #79244, #54786, #79660, #40507, #67848, #66603, #42153, #10187, #54365, #8525, #3867, #35852, #67020, #60279, #60688, #61521, #9353, #80077, #41340, #15262, #21559, #21152, #22395, #73755, #47221, #46807, #2208, #40922, #72498, #14847, #66189, #8936, #47638, #15679, #16091, #41736, #67430, #17742, #49290, #36259, #10602, #43370, #5502, #82529, #23209, #69070, #48880, #11420, #81307, #37489, #80896, #36660, #37075, #74580, #24846, #61928, #69888, #55595, #18553, #50513, #16925, #74993, #12242, #4672, #56831, #76218, #62335, #63164, #62761, #5096, #75396, #30345, #68266, #56011, #69484, #42562, #31164, #30764, #23621, #4270, #29932, #44198, #43781, #75805, #81722, #63574, #56426, #24031, #17338, #82126, #42968, #24441, #68663, #50109, #11001, #37898, #18147, #11836, #29526, #49700, #55188, #12650, #45021, #13909, #44602, #77039, #58502, #866, #45446, #13484, #57237, #6323, #45862, #31999, #51756, #7163, #18955, #26523, #6741, #39141, #19795, #70297, #63986, #57659, #64823, #21, #19371, #52178, #7593, #51335, #13074, #70721, #71142, #32834, #20212, #31582, #77881, #58075, #38311, #32412, #441, #38728, #64405, #71560, #39567, #65256, #33265, #5909, #25675, #26096, #77459, #82939, #25260, #50924, #76624, #38159, #81152, #44454, #70145, #63833, #11268, #68510, #5354, #62187, #63421, #31013, #55856, #44052, #18808, #24700, #6170, #56682, #82383, #56278, #36927, #37344, #12497, #31428, #31845, #42816, #17183, #17999, #43220, #69744, #18409, #81566, #68918, #17588, #50369, #62604, #81975, #76067, #43633, #75658, #12090, #74839, #37746, #4945, #30615, #25107, #23468, #24289, #49961, #69336, #5758, #57090, #76481, #49135, #82786, #11686, #23884, #63017, #50780, #10850, #36511, #4524, #30194, #49549, #75244, #83034, #5187, #62429, #43057, #50609, #82219, #11926, #17426, #42655, #23713, #4767, #82623, #24938, #63668, #62022, #30442, #75494, #24538, #56516, #30026, #30852, #36754, #49384, #81397, #50203, #76316, #69981, #10692, #75900, #36347, #18240, #68754, #18646, #68352, #24123, #43881, #4358, #12336, #75079, #57338, #11096, #6009, #37992, #55689, #56107, #25358, #17833, #44290, #31678, #49792, #51021, #69579, #43467, #81812, #17015, #69164, #11515, #37581, #37171, #62851, #63254, #5595, #31261, #56928, #33364, #27451, #72079, #71244, #14012, #76720, #26197, #12752, #64927, #19471, #14438, #57757, #7265, #27034, #45121, #45964, #13588, #26625, #39669, #52696, #119, #39244, #40090, #77138, #51858, #46386, #19052, #77565, #52279, #19899, #51435, #44699, #58175, #59027, #13176, #25774, #71661, #65777, #1382, #77983, #58602, #78403, #70829, #65359, #32937, #20313, #7697, #20735, #38826, #971, #8109, #64504, #45546, #33775, #70396, #59437, #1791, #38409, #6843, #64090, #544, #6427, #32513, #32096, #48052, #48460, #9762, #3036, #35022, #3449, #29113, #74160, #21974, #80487, #61098, #53534, #35433, #28283, #40505, #67846, #66601, #54783, #22802, #54363, #8522, #3864, #16508, #67018, #60277, #41338 ) ),
 .UNSPECIFIED., .F., .F., .F. ) 
 B_SPLINE_SURFACE_WITH_KNOTS ( ( 2, 2 ),
 ( 3, 2, 2, 2, 2, 2, 2, 2, 2, 2, 2, 2, 2, 2, 2, 2, 2, 2, 2, 2, 2, 2, 2, 2, 2, 2, 2, 2, 2, 2, 2, 2, 2, 2, 2, 2, 2, 2, 2, 2, 2, 2, 2, 2, 2, 2, 2, 2, 2, 2, 2, 2, 2, 2, 2, 2, 2, 2, 2, 2, 2, 2, 2, 2, 2, 2, 2, 2, 2, 2, 2, 2, 2, 2, 2, 2, 2, 2, 2, 2, 2, 2, 2, 2, 2, 2, 2, 2, 2, 2, 2, 2, 2, 2, 2, 2, 2, 2, 2, 2, 2, 2, 2, 2, 2, 2, 2, 2, 2, 2, 2, 2, 2, 2, 2, 2, 2, 2, 2, 2, 2, 2, 2, 2, 2, 2, 2, 2, 2, 2, 2, 2, 2, 2, 2, 2, 2, 2, 2, 2, 2, 2, 2, 2, 2, 2, 2, 2, 2, 2, 2, 2, 2, 2, 2, 2, 2, 2, 2, 2, 2, 2, 2, 2, 2, 2, 2, 2, 2, 2, 2, 2, 2, 2, 2, 2, 2, 2, 2, 2, 2, 2, 2, 2, 2, 2, 2, 2, 2, 2, 2, 2, 2, 2, 2, 2, 2, 2, 2, 2, 2, 2, 2, 2, 2, 2, 2, 2, 2, 2, 2, 2, 2, 2, 2, 2, 2, 2, 2, 2, 2, 2, 2, 2, 2, 2, 2, 2, 2, 2, 2, 2, 2, 2, 2, 2, 2, 2, 2, 2, 2, 2, 2, 2, 2, 2, 2, 2, 2, 2, 2, 2, 2, 2, 2, 3 ),
 ( 0.000000000000000000, 1.000000000000000000 ),
 ( 0.000000000000000000, 0.003787878787878787984, 0.007575757575757575968, 0.01136363636363636395, 0.01515151515151515194, 0.01893939393939393992, 0.02272727272727272790, 0.02651515151515151589, 0.03030303030303030387, 0.03409090909090908839, 0.03787878787878787984, 0.04166666666666666435, 0.04545454545454545581, 0.04924242424242424032, 0.05303030303030303177, 0.05681818181818181629, 0.06060606060606060774, 0.06439393939393939226, 0.06818181818181817677, 0.07196969696969697516, 0.07575757575757575968, 0.07954545454545454419, 0.08333333333333332871, 0.08712121212121212710, 0.09090909090909091161, 0.09469696969696969613, 0.09848484848484848064, 0.1022727272727272790, 0.1060606060606060635, 0.1098484848484848481, 0.1136363636363636326, 0.1174242424242424310, 0.1212121212121212155, 0.1250000000000000000, 0.1287878787878787845, 0.1325757575757575690, 0.1363636363636363535, 0.1401515151515151381, 0.1439393939393939503, 0.1477272727272727348, 0.1515151515151515194, 0.1553030303030303039, 0.1590909090909090884, 0.1628787878787878729, 0.1666666666666666574, 0.1704545454545454419, 0.1742424242424242542, 0.1780303030303030387, 0.1818181818181818232, 0.1856060606060606077, 0.1893939393939393923, 0.1931818181818181768, 0.1969696969696969613, 0.2007575757575757458, 0.2045454545454545581, 0.2083333333333333426, 0.2121212121212121271, 0.2159090909090909116, 0.2196969696969696961, 0.2234848484848484806, 0.2272727272727272652, 0.2310606060606060497, 0.2348484848484848619, 0.2386363636363636465, 0.2424242424242424310, 0.2462121212121212155, 0.2500000000000000000, 0.2537878787878787845, 0.2575757575757575690, 0.2613636363636363535, 0.2651515151515151381, 0.2689393939393939226, 0.2727272727272727071, 0.2765151515151514916, 0.2803030303030302761, 0.2840909090909091161, 0.2878787878787879007, 0.2916666666666666852, 0.2954545454545454697, 0.2992424242424242542, 0.3030303030303030387, 0.3068181818181818232, 0.3106060606060606077, 0.3143939393939393923, 0.3181818181818181768, 0.3219696969696969613, 0.3257575757575757458, 0.3295454545454545303, 0.3333333333333333148, 0.3371212121212120993, 0.3409090909090908839, 0.3446969696969697239, 0.3484848484848485084, 0.3522727272727272929, 0.3560606060606060774, 0.3598484848484848619, 0.3636363636363636465, 0.3674242424242424310, 0.3712121212121212155, 0.3750000000000000000, 0.3787878787878787845, 0.3825757575757575690, 0.3863636363636363535, 0.3901515151515151381, 0.3939393939393939226, 0.3977272727272727071, 0.4015151515151514916, 0.4053030303030302761, 0.4090909090909091161, 0.4128787878787879007, 0.4166666666666666852, 0.4204545454545454697, 0.4242424242424242542, 0.4280303030303030387, 0.4318181818181818232, 0.4356060606060606077, 0.4393939393939393923, 0.4431818181818181768, 0.4469696969696969613, 0.4507575757575757458, 0.4545454545454545303, 0.4583333333333333148, 0.4621212121212120993, 0.4659090909090908839, 0.4696969696969697239, 0.4734848484848485084, 0.4772727272727272929, 0.4810606060606060774, 0.4848484848484848619, 0.4886363636363636465, 0.4924242424242424310, 0.4962121212121212155, 0.5000000000000000000, 0.5037878787878787845, 0.5075757575757575690, 0.5113636363636363535, 0.5151515151515151381, 0.5189393939393939226, 0.5227272727272727071, 0.5265151515151514916, 0.5303030303030302761, 0.5340909090909090606, 0.5378787878787878451, 0.5416666666666666297, 0.5454545454545454142, 0.5492424242424241987, 0.5530303030303029832, 0.5568181818181817677, 0.5606060606060605522, 0.5643939393939394478, 0.5681818181818182323, 0.5719696969696970168, 0.5757575757575758013, 0.5795454545454545858, 0.5833333333333333703, 0.5871212121212121549, 0.5909090909090909394, 0.5946969696969697239, 0.5984848484848485084, 0.6022727272727272929, 0.6060606060606060774, 0.6098484848484848619, 0.6136363636363636465, 0.6174242424242424310, 0.6212121212121212155, 0.6250000000000000000, 0.6287878787878787845, 0.6325757575757575690, 0.6363636363636363535, 0.6401515151515151381, 0.6439393939393939226, 0.6477272727272727071, 0.6515151515151514916, 0.6553030303030302761, 0.6590909090909090606, 0.6628787878787878451, 0.6666666666666666297, 0.6704545454545454142, 0.6742424242424241987, 0.6780303030303029832, 0.6818181818181817677, 0.6856060606060605522, 0.6893939393939394478, 0.6931818181818182323, 0.6969696969696970168, 0.7007575757575758013, 0.7045454545454545858, 0.7083333333333333703, 0.7121212121212121549, 0.7159090909090909394, 0.7196969696969697239, 0.7234848484848485084, 0.7272727272727272929, 0.7310606060606060774, 0.7348484848484848619, 0.7386363636363636465, 0.7424242424242424310, 0.7462121212121212155, 0.7500000000000000000, 0.7537878787878787845, 0.7575757575757575690, 0.7613636363636363535, 0.7651515151515151381, 0.7689393939393939226, 0.7727272727272727071, 0.7765151515151514916, 0.7803030303030302761, 0.7840909090909090606, 0.7878787878787878451, 0.7916666666666666297, 0.7954545454545454142, 0.7992424242424241987, 0.8030303030303029832, 0.8068181818181817677, 0.8106060606060605522, 0.8143939393939394478, 0.8181818181818182323, 0.8219696969696970168, 0.8257575757575758013, 0.8295454545454545858, 0.8333333333333333703, 0.8371212121212121549, 0.8409090909090909394, 0.8446969696969697239, 0.8484848484848485084, 0.8522727272727272929, 0.8560606060606060774, 0.8598484848484848619, 0.8636363636363636465, 0.8674242424242424310, 0.8712121212121212155, 0.8750000000000000000, 0.8787878787878787845, 0.8825757575757575690, 0.8863636363636363535, 0.8901515151515151381, 0.8939393939393939226, 0.8977272727272727071, 0.9015151515151514916, 0.9053030303030302761, 0.9090909090909090606, 0.9128787878787878451, 0.9166666666666666297, 0.9204545454545454142, 0.9242424242424241987, 0.9280303030303029832, 0.9318181818181817677, 0.9356060606060605522, 0.9393939393939394478, 0.9431818181818182323, 0.9469696969696970168, 0.9507575757575758013, 0.9545454545454545858, 0.9583333333333333703, 0.9621212121212121549, 0.9659090909090909394 ),
 .UNSPECIFIED. ) 
 GEOMETRIC_REPRESENTATION_ITEM ( )  RATIONAL_B_SPLINE_SURFACE ( (
 ( 1.000000000000000000, 0.9659258262890683122, 1.000000000000000000, 0.9659258262890683122, 1.000000000000000000, 0.9659258262890683122, 1.000000000000000000, 0.9659258262890683122, 1.000000000000000000, 0.9659258262890683122, 1.000000000000000000, 0.9659258262890683122, 1.000000000000000000, 0.9659258262890683122, 1.000000000000000000, 0.9659258262890683122, 1.000000000000000000, 0.9659258262890683122, 1.000000000000000000, 0.9659258262890683122, 1.000000000000000000, 0.9659258262890683122, 1.000000000000000000, 0.9659258262890683122, 1.000000000000000000, 0.9659258262890683122, 1.000000000000000000, 0.9659258262890683122, 1.000000000000000000, 0.9659258262890683122, 1.000000000000000000, 0.9659258262890683122, 1.000000000000000000, 0.9659258262890683122, 1.000000000000000000, 0.9659258262890683122, 1.000000000000000000, 0.9659258262890683122, 1.000000000000000000, 0.9659258262890683122, 1.000000000000000000, 0.9659258262890683122, 1.000000000000000000, 0.9659258262890683122, 1.000000000000000000, 0.9659258262890683122, 1.000000000000000000, 0.9659258262890683122, 1.000000000000000000, 0.9659258262890683122, 1.000000000000000000, 0.9659258262890683122, 1.000000000000000000, 0.9659258262890683122, 1.000000000000000000, 0.9659258262890683122, 1.000000000000000000, 0.9659258262890683122, 1.000000000000000000, 0.9659258262890683122, 1.000000000000000000, 0.9659258262890683122, 1.000000000000000000, 0.9659258262890683122, 1.000000000000000000, 0.9659258262890683122, 1.000000000000000000, 0.9659258262890683122, 1.000000000000000000, 0.9659258262890683122, 1.000000000000000000, 0.9659258262890683122, 1.000000000000000000, 0.9659258262890683122, 1.000000000000000000, 0.9659258262890683122, 1.000000000000000000, 0.9659258262890683122, 1.000000000000000000, 0.9659258262890683122, 1.000000000000000000, 0.9659258262890683122, 1.000000000000000000, 0.9659258262890683122, 1.000000000000000000, 0.9659258262890683122, 1.000000000000000000, 0.9659258262890683122, 1.000000000000000000, 0.9659258262890683122, 1.000000000000000000, 0.9659258262890683122, 1.000000000000000000, 0.9659258262890683122, 1.000000000000000000, 0.9659258262890683122, 1.000000000000000000, 0.9659258262890683122, 1.000000000000000000, 0.9659258262890683122, 1.000000000000000000, 0.9659258262890683122, 1.000000000000000000, 0.9659258262890683122, 1.000000000000000000, 0.9659258262890683122, 1.000000000000000000, 0.9659258262890683122, 1.000000000000000000, 0.9659258262890683122, 1.000000000000000000, 0.9659258262890683122, 1.000000000000000000, 0.9659258262890683122, 1.000000000000000000, 0.9659258262890683122, 1.000000000000000000, 0.9659258262890683122, 1.000000000000000000, 0.9659258262890683122, 1.000000000000000000, 0.9659258262890683122, 1.000000000000000000, 0.9659258262890683122, 1.000000000000000000, 0.9659258262890683122, 1.000000000000000000, 0.9659258262890683122, 1.000000000000000000, 0.9659258262890683122, 1.000000000000000000, 0.9659258262890683122, 1.000000000000000000, 0.9659258262890683122, 1.000000000000000000, 0.9659258262890683122, 1.000000000000000000, 0.9659258262890683122, 1.000000000000000000, 0.9659258262890683122, 1.000000000000000000, 0.9659258262890683122, 1.000000000000000000, 0.9659258262890683122, 1.000000000000000000, 0.9659258262890683122, 1.000000000000000000, 0.9659258262890683122, 1.000000000000000000, 0.9659258262890683122, 1.000000000000000000, 0.9659258262890683122, 1.000000000000000000, 0.9659258262890683122, 1.000000000000000000, 0.9659258262890683122, 1.000000000000000000, 0.9659258262890683122, 1.000000000000000000, 0.9659258262890683122, 1.000000000000000000, 0.9659258262890683122, 1.000000000000000000, 0.9659258262890683122, 1.000000000000000000, 0.9659258262890683122, 1.000000000000000000, 0.9659258262890683122, 1.000000000000000000, 0.9659258262890683122, 1.000000000000000000, 0.9659258262890683122, 1.000000000000000000, 0.9659258262890683122, 1.000000000000000000, 0.9659258262890683122, 1.000000000000000000, 0.9659258262890683122, 1.000000000000000000, 0.9659258262890683122, 1.000000000000000000, 0.9659258262890683122, 1.000000000000000000, 0.9659258262890683122, 1.000000000000000000, 0.9659258262890683122, 1.000000000000000000, 0.9659258262890683122, 1.000000000000000000, 0.9659258262890683122, 1.000000000000000000, 0.9659258262890683122, 1.000000000000000000, 0.9659258262890683122, 1.000000000000000000, 0.9659258262890683122, 1.000000000000000000, 0.9659258262890683122, 1.000000000000000000, 0.9659258262890683122, 1.000000000000000000, 0.9659258262890683122, 1.000000000000000000, 0.9659258262890683122, 1.000000000000000000, 0.9659258262890683122, 1.000000000000000000, 0.9659258262890683122, 1.000000000000000000, 0.9659258262890683122, 1.000000000000000000, 0.9659258262890683122, 1.000000000000000000, 0.9659258262890683122, 1.000000000000000000, 0.9659258262890683122, 1.000000000000000000, 0.9659258262890683122, 1.000000000000000000, 0.9659258262890683122, 1.000000000000000000, 0.9659258262890683122, 1.000000000000000000, 0.9659258262890683122, 1.000000000000000000, 0.9659258262890683122, 1.000000000000000000, 0.9659258262890683122, 1.000000000000000000, 0.9659258262890683122, 1.000000000000000000, 0.9659258262890683122, 1.000000000000000000, 0.9659258262890683122, 1.000000000000000000, 0.9659258262890683122, 1.000000000000000000, 0.9659258262890683122, 1.000000000000000000, 0.9659258262890683122, 1.000000000000000000, 0.9659258262890683122, 1.000000000000000000, 0.9659258262890683122, 1.000000000000000000, 0.9659258262890683122, 1.000000000000000000, 0.9659258262890683122, 1.000000000000000000, 0.9659258262890683122, 1.000000000000000000, 0.9659258262890683122, 1.000000000000000000, 0.9659258262890683122, 1.000000000000000000, 0.9659258262890683122, 1.000000000000000000, 0.9659258262890683122, 1.000000000000000000, 0.9659258262890683122, 1.000000000000000000, 0.9659258262890683122, 1.000000000000000000, 0.9659258262890683122, 1.000000000000000000, 0.9659258262890683122, 1.000000000000000000, 0.9659258262890683122, 1.000000000000000000, 0.9659258262890683122, 1.000000000000000000, 0.9659258262890683122, 1.000000000000000000, 0.9659258262890683122, 1.000000000000000000, 0.9659258262890683122, 1.000000000000000000, 0.9659258262890683122, 1.000000000000000000, 0.9659258262890683122, 1.000000000000000000, 0.9659258262890683122, 1.000000000000000000, 0.9659258262890683122, 1.000000000000000000, 0.9659258262890683122, 1.000000000000000000, 0.9659258262890683122, 1.000000000000000000, 0.9659258262890683122, 1.000000000000000000, 0.9659258262890683122, 1.000000000000000000, 0.9659258262890683122, 1.000000000000000000, 0.9659258262890683122, 1.000000000000000000, 0.9659258262890683122, 1.000000000000000000, 0.9659258262890683122, 1.000000000000000000, 0.9659258262890683122, 1.000000000000000000, 0.9659258262890683122, 1.000000000000000000, 0.9659258262890683122, 1.000000000000000000, 0.9659258262890683122, 1.000000000000000000, 0.9659258262890683122, 1.000000000000000000, 0.9659258262890683122, 1.000000000000000000, 0.9659258262890683122, 1.000000000000000000, 0.9659258262890683122, 1.000000000000000000, 0.9659258262890683122, 1.000000000000000000, 0.9659258262890683122, 1.000000000000000000, 0.9659258262890683122, 1.000000000000000000, 0.9659258262890683122, 1.000000000000000000, 0.9659258262890683122, 1.000000000000000000, 0.9659258262890683122, 1.000000000000000000, 0.9659258262890683122, 1.000000000000000000, 0.9659258262890683122, 1.000000000000000000, 0.9659258262890683122, 1.000000000000000000, 0.9659258262890683122, 1.000000000000000000, 0.9659258262890683122, 1.000000000000000000, 0.9659258262890683122, 1.000000000000000000, 0.9659258262890683122, 1.000000000000000000, 0.9659258262890683122, 1.000000000000000000, 0.9659258262890683122, 1.000000000000000000, 0.9659258262890683122, 1.000000000000000000, 0.9659258262890683122, 1.000000000000000000, 0.9659258262890683122, 1.000000000000000000, 0.9659258262890683122, 1.000000000000000000, 0.9659258262890683122, 1.000000000000000000, 0.9659258262890683122, 1.000000000000000000, 0.9659258262890683122, 1.000000000000000000, 0.9659258262890683122, 1.000000000000000000, 0.9659258262890683122, 1.000000000000000000, 0.9659258262890683122, 1.000000000000000000, 0.9659258262890683122, 1.000000000000000000, 0.9659258262890683122, 1.000000000000000000, 0.9659258262890683122, 1.000000000000000000, 0.9659258262890683122, 1.000000000000000000, 0.9659258262890683122, 1.000000000000000000, 0.9659258262890683122, 1.000000000000000000, 0.9659258262890683122, 1.000000000000000000, 0.9659258262890683122, 1.000000000000000000, 0.9659258262890683122, 1.000000000000000000, 0.9659258262890683122, 1.000000000000000000, 0.9659258262890683122, 1.000000000000000000, 0.9659258262890683122, 1.000000000000000000, 0.9659258262890683122, 1.000000000000000000, 0.9659258262890683122, 1.000000000000000000, 0.9659258262890683122, 1.000000000000000000, 0.9659258262890683122, 1.000000000000000000, 0.9659258262890683122, 1.000000000000000000, 0.9659258262890683122, 1.000000000000000000, 0.9659258262890683122, 1.000000000000000000, 0.9659258262890683122, 1.000000000000000000, 0.9659258262890683122, 1.000000000000000000, 0.9659258262890683122, 1.000000000000000000, 0.9659258262890683122, 1.000000000000000000, 0.9659258262890683122, 1.000000000000000000, 0.9659258262890683122, 1.000000000000000000, 0.9659258262890683122, 1.000000000000000000, 0.9659258262890683122, 1.000000000000000000, 0.9659258262890683122, 1.000000000000000000, 0.9659258262890683122, 1.000000000000000000, 0.9659258262890683122, 1.000000000000000000, 0.9659258262890683122, 1.000000000000000000, 0.9659258262890683122, 1.000000000000000000, 0.9659258262890683122, 1.000000000000000000, 0.9659258262890683122, 1.000000000000000000, 0.9659258262890683122, 1.000000000000000000, 0.9659258262890683122, 1.000000000000000000, 0.9659258262890683122, 1.000000000000000000, 0.9659258262890683122, 1.000000000000000000, 0.9659258262890683122, 1.000000000000000000, 0.9659258262890683122, 1.000000000000000000, 0.9659258262890683122, 1.000000000000000000, 0.9659258262890683122, 1.000000000000000000, 0.9659258262890683122, 1.000000000000000000, 0.9659258262890683122, 1.000000000000000000, 0.9659258262890683122, 1.000000000000000000, 0.9659258262890683122, 1.000000000000000000, 0.9659258262890683122, 1.000000000000000000, 0.9659258262890683122, 1.000000000000000000, 0.9659258262890683122, 1.000000000000000000, 0.9659258262890683122, 1.000000000000000000, 0.9659258262890683122, 1.000000000000000000, 0.9659258262890683122, 1.000000000000000000, 0.9659258262890683122, 1.000000000000000000, 0.9659258262890683122, 1.000000000000000000, 0.9659258262890683122, 1.000000000000000000, 0.9659258262890683122, 1.000000000000000000, 0.9659258262890683122, 1.000000000000000000, 0.9659258262890683122, 1.000000000000000000, 0.9659258262890683122, 1.000000000000000000, 0.9659258262890683122, 1.000000000000000000, 0.9659258262890683122, 1.000000000000000000, 0.9659258262890683122, 1.000000000000000000, 0.9659258262890683122, 1.000000000000000000, 0.9659258262890683122, 1.000000000000000000, 0.9659258262890683122, 1.000000000000000000, 0.9659258262890683122, 1.000000000000000000, 0.9659258262890683122, 1.000000000000000000, 0.9659258262890683122, 1.000000000000000000, 0.9659258262890683122, 1.000000000000000000, 0.9659258262890683122, 1.000000000000000000, 0.9659258262890683122, 1.000000000000000000, 0.9659258262890683122, 1.000000000000000000),
 ( 1.000000000000000000, 0.9659258262890683122, 1.000000000000000000, 0.9659258262890683122, 1.000000000000000000, 0.9659258262890683122, 1.000000000000000000, 0.9659258262890683122, 1.000000000000000000, 0.9659258262890683122, 1.000000000000000000, 0.9659258262890683122, 1.000000000000000000, 0.9659258262890683122, 1.000000000000000000, 0.9659258262890683122, 1.000000000000000000, 0.9659258262890683122, 1.000000000000000000, 0.9659258262890683122, 1.000000000000000000, 0.9659258262890683122, 1.000000000000000000, 0.9659258262890683122, 1.000000000000000000, 0.9659258262890683122, 1.000000000000000000, 0.9659258262890683122, 1.000000000000000000, 0.9659258262890683122, 1.000000000000000000, 0.9659258262890683122, 1.000000000000000000, 0.9659258262890683122, 1.000000000000000000, 0.9659258262890683122, 1.000000000000000000, 0.9659258262890683122, 1.000000000000000000, 0.9659258262890683122, 1.000000000000000000, 0.9659258262890683122, 1.000000000000000000, 0.9659258262890683122, 1.000000000000000000, 0.9659258262890683122, 1.000000000000000000, 0.9659258262890683122, 1.000000000000000000, 0.9659258262890683122, 1.000000000000000000, 0.9659258262890683122, 1.000000000000000000, 0.9659258262890683122, 1.000000000000000000, 0.9659258262890683122, 1.000000000000000000, 0.9659258262890683122, 1.000000000000000000, 0.9659258262890683122, 1.000000000000000000, 0.9659258262890683122, 1.000000000000000000, 0.9659258262890683122, 1.000000000000000000, 0.9659258262890683122, 1.000000000000000000, 0.9659258262890683122, 1.000000000000000000, 0.9659258262890683122, 1.000000000000000000, 0.9659258262890683122, 1.000000000000000000, 0.9659258262890683122, 1.000000000000000000, 0.9659258262890683122, 1.000000000000000000, 0.9659258262890683122, 1.000000000000000000, 0.9659258262890683122, 1.000000000000000000, 0.9659258262890683122, 1.000000000000000000, 0.9659258262890683122, 1.000000000000000000, 0.9659258262890683122, 1.000000000000000000, 0.9659258262890683122, 1.000000000000000000, 0.9659258262890683122, 1.000000000000000000, 0.9659258262890683122, 1.000000000000000000, 0.9659258262890683122, 1.000000000000000000, 0.9659258262890683122, 1.000000000000000000, 0.9659258262890683122, 1.000000000000000000, 0.9659258262890683122, 1.000000000000000000, 0.9659258262890683122, 1.000000000000000000, 0.9659258262890683122, 1.000000000000000000, 0.9659258262890683122, 1.000000000000000000, 0.9659258262890683122, 1.000000000000000000, 0.9659258262890683122, 1.000000000000000000, 0.9659258262890683122, 1.000000000000000000, 0.9659258262890683122, 1.000000000000000000, 0.9659258262890683122, 1.000000000000000000, 0.9659258262890683122, 1.000000000000000000, 0.9659258262890683122, 1.000000000000000000, 0.9659258262890683122, 1.000000000000000000, 0.9659258262890683122, 1.000000000000000000, 0.9659258262890683122, 1.000000000000000000, 0.9659258262890683122, 1.000000000000000000, 0.9659258262890683122, 1.000000000000000000, 0.9659258262890683122, 1.000000000000000000, 0.9659258262890683122, 1.000000000000000000, 0.9659258262890683122, 1.000000000000000000, 0.9659258262890683122, 1.000000000000000000, 0.9659258262890683122, 1.000000000000000000, 0.9659258262890683122, 1.000000000000000000, 0.9659258262890683122, 1.000000000000000000, 0.9659258262890683122, 1.000000000000000000, 0.9659258262890683122, 1.000000000000000000, 0.9659258262890683122, 1.000000000000000000, 0.9659258262890683122, 1.000000000000000000, 0.9659258262890683122, 1.000000000000000000, 0.9659258262890683122, 1.000000000000000000, 0.9659258262890683122, 1.000000000000000000, 0.9659258262890683122, 1.000000000000000000, 0.9659258262890683122, 1.000000000000000000, 0.9659258262890683122, 1.000000000000000000, 0.9659258262890683122, 1.000000000000000000, 0.9659258262890683122, 1.000000000000000000, 0.9659258262890683122, 1.000000000000000000, 0.9659258262890683122, 1.000000000000000000, 0.9659258262890683122, 1.000000000000000000, 0.9659258262890683122, 1.000000000000000000, 0.9659258262890683122, 1.000000000000000000, 0.9659258262890683122, 1.000000000000000000, 0.9659258262890683122, 1.000000000000000000, 0.9659258262890683122, 1.000000000000000000, 0.9659258262890683122, 1.000000000000000000, 0.9659258262890683122, 1.000000000000000000, 0.9659258262890683122, 1.000000000000000000, 0.9659258262890683122, 1.000000000000000000, 0.9659258262890683122, 1.000000000000000000, 0.9659258262890683122, 1.000000000000000000, 0.9659258262890683122, 1.000000000000000000, 0.9659258262890683122, 1.000000000000000000, 0.9659258262890683122, 1.000000000000000000, 0.9659258262890683122, 1.000000000000000000, 0.9659258262890683122, 1.000000000000000000, 0.9659258262890683122, 1.000000000000000000, 0.9659258262890683122, 1.000000000000000000, 0.9659258262890683122, 1.000000000000000000, 0.9659258262890683122, 1.000000000000000000, 0.9659258262890683122, 1.000000000000000000, 0.9659258262890683122, 1.000000000000000000, 0.9659258262890683122, 1.000000000000000000, 0.9659258262890683122, 1.000000000000000000, 0.9659258262890683122, 1.000000000000000000, 0.9659258262890683122, 1.000000000000000000, 0.9659258262890683122, 1.000000000000000000, 0.9659258262890683122, 1.000000000000000000, 0.9659258262890683122, 1.000000000000000000, 0.9659258262890683122, 1.000000000000000000, 0.9659258262890683122, 1.000000000000000000, 0.9659258262890683122, 1.000000000000000000, 0.9659258262890683122, 1.000000000000000000, 0.9659258262890683122, 1.000000000000000000, 0.9659258262890683122, 1.000000000000000000, 0.9659258262890683122, 1.000000000000000000, 0.9659258262890683122, 1.000000000000000000, 0.9659258262890683122, 1.000000000000000000, 0.9659258262890683122, 1.000000000000000000, 0.9659258262890683122, 1.000000000000000000, 0.9659258262890683122, 1.000000000000000000, 0.9659258262890683122, 1.000000000000000000, 0.9659258262890683122, 1.000000000000000000, 0.9659258262890683122, 1.000000000000000000, 0.9659258262890683122, 1.000000000000000000, 0.9659258262890683122, 1.000000000000000000, 0.9659258262890683122, 1.000000000000000000, 0.9659258262890683122, 1.000000000000000000, 0.9659258262890683122, 1.000000000000000000, 0.9659258262890683122, 1.000000000000000000, 0.9659258262890683122, 1.000000000000000000, 0.9659258262890683122, 1.000000000000000000, 0.9659258262890683122, 1.000000000000000000, 0.9659258262890683122, 1.000000000000000000, 0.9659258262890683122, 1.000000000000000000, 0.9659258262890683122, 1.000000000000000000, 0.9659258262890683122, 1.000000000000000000, 0.9659258262890683122, 1.000000000000000000, 0.9659258262890683122, 1.000000000000000000, 0.9659258262890683122, 1.000000000000000000, 0.9659258262890683122, 1.000000000000000000, 0.9659258262890683122, 1.000000000000000000, 0.9659258262890683122, 1.000000000000000000, 0.9659258262890683122, 1.000000000000000000, 0.9659258262890683122, 1.000000000000000000, 0.9659258262890683122, 1.000000000000000000, 0.9659258262890683122, 1.000000000000000000, 0.9659258262890683122, 1.000000000000000000, 0.9659258262890683122, 1.000000000000000000, 0.9659258262890683122, 1.000000000000000000, 0.9659258262890683122, 1.000000000000000000, 0.9659258262890683122, 1.000000000000000000, 0.9659258262890683122, 1.000000000000000000, 0.9659258262890683122, 1.000000000000000000, 0.9659258262890683122, 1.000000000000000000, 0.9659258262890683122, 1.000000000000000000, 0.9659258262890683122, 1.000000000000000000, 0.9659258262890683122, 1.000000000000000000, 0.9659258262890683122, 1.000000000000000000, 0.9659258262890683122, 1.000000000000000000, 0.9659258262890683122, 1.000000000000000000, 0.9659258262890683122, 1.000000000000000000, 0.9659258262890683122, 1.000000000000000000, 0.9659258262890683122, 1.000000000000000000, 0.9659258262890683122, 1.000000000000000000, 0.9659258262890683122, 1.000000000000000000, 0.9659258262890683122, 1.000000000000000000, 0.9659258262890683122, 1.000000000000000000, 0.9659258262890683122, 1.000000000000000000, 0.9659258262890683122, 1.000000000000000000, 0.9659258262890683122, 1.000000000000000000, 0.9659258262890683122, 1.000000000000000000, 0.9659258262890683122, 1.000000000000000000, 0.9659258262890683122, 1.000000000000000000, 0.9659258262890683122, 1.000000000000000000, 0.9659258262890683122, 1.000000000000000000, 0.9659258262890683122, 1.000000000000000000, 0.9659258262890683122, 1.000000000000000000, 0.9659258262890683122, 1.000000000000000000, 0.9659258262890683122, 1.000000000000000000, 0.9659258262890683122, 1.000000000000000000, 0.9659258262890683122, 1.000000000000000000, 0.9659258262890683122, 1.000000000000000000, 0.9659258262890683122, 1.000000000000000000, 0.9659258262890683122, 1.000000000000000000, 0.9659258262890683122, 1.000000000000000000, 0.9659258262890683122, 1.000000000000000000, 0.9659258262890683122, 1.000000000000000000, 0.9659258262890683122, 1.000000000000000000, 0.9659258262890683122, 1.000000000000000000, 0.9659258262890683122, 1.000000000000000000, 0.9659258262890683122, 1.000000000000000000, 0.9659258262890683122, 1.000000000000000000, 0.9659258262890683122, 1.000000000000000000, 0.9659258262890683122, 1.000000000000000000, 0.9659258262890683122, 1.000000000000000000, 0.9659258262890683122, 1.000000000000000000, 0.9659258262890683122, 1.000000000000000000, 0.9659258262890683122, 1.000000000000000000, 0.9659258262890683122, 1.000000000000000000, 0.9659258262890683122, 1.000000000000000000, 0.9659258262890683122, 1.000000000000000000, 0.9659258262890683122, 1.000000000000000000, 0.9659258262890683122, 1.000000000000000000, 0.9659258262890683122, 1.000000000000000000, 0.9659258262890683122, 1.000000000000000000, 0.9659258262890683122, 1.000000000000000000, 0.9659258262890683122, 1.000000000000000000, 0.9659258262890683122, 1.000000000000000000, 0.9659258262890683122, 1.000000000000000000, 0.9659258262890683122, 1.000000000000000000, 0.9659258262890683122, 1.000000000000000000, 0.9659258262890683122, 1.000000000000000000, 0.9659258262890683122, 1.000000000000000000, 0.9659258262890683122, 1.000000000000000000, 0.9659258262890683122, 1.000000000000000000, 0.9659258262890683122, 1.000000000000000000, 0.9659258262890683122, 1.000000000000000000, 0.9659258262890683122, 1.000000000000000000, 0.9659258262890683122, 1.000000000000000000, 0.9659258262890683122, 1.000000000000000000, 0.9659258262890683122, 1.000000000000000000, 0.9659258262890683122, 1.000000000000000000, 0.9659258262890683122, 1.000000000000000000, 0.9659258262890683122, 1.000000000000000000, 0.9659258262890683122, 1.000000000000000000, 0.9659258262890683122, 1.000000000000000000, 0.9659258262890683122, 1.000000000000000000, 0.9659258262890683122, 1.000000000000000000, 0.9659258262890683122, 1.000000000000000000, 0.9659258262890683122, 1.000000000000000000, 0.9659258262890683122, 1.000000000000000000, 0.9659258262890683122, 1.000000000000000000, 0.9659258262890683122, 1.000000000000000000, 0.9659258262890683122, 1.000000000000000000, 0.9659258262890683122, 1.000000000000000000, 0.9659258262890683122, 1.000000000000000000, 0.9659258262890683122, 1.000000000000000000, 0.9659258262890683122, 1.000000000000000000, 0.9659258262890683122, 1.000000000000000000, 0.9659258262890683122, 1.000000000000000000, 0.9659258262890683122, 1.000000000000000000, 0.9659258262890683122, 1.000000000000000000, 0.9659258262890683122, 1.000000000000000000, 0.9659258262890683122, 1.000000000000000000, 0.9659258262890683122, 1.000000000000000000, 0.9659258262890683122, 1.000000000000000000, 0.9659258262890683122, 1.000000000000000000) ) ) 
 REPRESENTATION_ITEM ( '' )  SURFACE ( )  );
#16734=CARTESIAN_POINT ( 'NONE',  ( 1.450131233595801428, 0.2952755905511811885, 0.1292274648535926551 ) ) ;
#16735=CARTESIAN_POINT ( 'NONE',  ( -0.7020997375328076329, -0.2845877964562161244, -0.3641732283464567121 ) ) ;
#16736=CARTESIAN_POINT ( 'NONE',  ( -0.6692913385826764205, -0.6692913385826771977, 8.415575281601705876E-17 ) ) ;
#16737=CARTESIAN_POINT ( 'NONE',  ( 1.548556430446194954, 0.2306618581243847221, -0.2411417322834647770 ) ) ;
#16738=CARTESIAN_POINT ( 'NONE',  ( 1.443569553805774897, -0.6046776061558809534, -0.2411417322834644161 ) ) ;
#16739=CARTESIAN_POINT ( 'NONE',  ( -1.653543307086613234, -0.1870078740157479769, 0.4822834645669291653 ) ) ;
#16740=CARTESIAN_POINT ( 'NONE',  ( -1.299212598425196097, -0.5511811023622047445, 6.969142054262312111E-17 ) ) ;
#16746=CARTESIAN_POINT ( 'NONE',  ( 1.279527559055118724, 0.07958543189024085140, 0.2665933059059887866 ) ) ;
#16747=CARTESIAN_POINT ( 'NONE',  ( 0.8792650918635177559, -0.4281496062992127816, -0.4176697321401328100 ) ) ;
#16748=CARTESIAN_POINT ( 'NONE',  ( 0.01241954290193841674, 0.000000000000000000, 0.3464511005275205946 ) ) ;
#16749=CARTESIAN_POINT ( 'NONE',  ( 0.7086614173228352742, -0.1870078740157480879, -0.4822834645669291653 ) ) ;
#16751=CARTESIAN_POINT ( 'NONE',  ( 1.069553805774278832, 0.1771653543307087075, -0.09757992244046823083 ) ) ;
#16752=CARTESIAN_POINT ( 'NONE',  ( 0.2821522309711292364, 0.2952755905511810774, -0.1292274648535930714 ) ) ;
#16753=CARTESIAN_POINT ( 'NONE',  ( -0.8464566929133852113, 0.1660481256975885056, 0.3530559997133364547 ) ) ;
#16754=CARTESIAN_POINT ( 'NONE',  ( 1.397637795275591177, 0.1660481256975883668, -0.3530559997133364547 ) ) ;
#16757=CARTESIAN_POINT ( 'NONE',  ( 0.2034120734908142214, 0.1771653543307087075, -0.09757992244046823083 ) ) ;
#16758=EDGE_CURVE ( 'NONE', #76877, #22642, #53157, .T. ) ;
#16761=VERTEX_POINT ( 'NONE', #23104 ) ;
#16762=CARTESIAN_POINT ( 'NONE',  ( -0.8989501312335946848, 0.2952755905511810774, -0.1292274648535930714 ) ) ;
#16763=CARTESIAN_POINT ( 'NONE',  ( -0.1509186351706028884, -0.3162353388693409650, -0.4822834645669289433 ) ) ;
#16764=CARTESIAN_POINT ( 'NONE',  ( -0.4396325459317577122, -0.6692913385826773087, -0.1292274648535924053 ) ) ;
#16766=CARTESIAN_POINT ( 'NONE',  ( 0.6692913385826778638, -0.6692913385826771977, 8.415575281601705876E-17 ) ) ;
#16768=CARTESIAN_POINT ( 'NONE',  ( -1.437007874015747477, 0.1660481256975883668, -0.3530559997133364547 ) ) ;
#16769=CARTESIAN_POINT ( 'NONE',  ( -0.2821522309711278487, 0.2952755905511811885, 0.1292274648535926551 ) ) ;
#16770=CARTESIAN_POINT ( 'NONE',  ( 1.246719160104987623, -0.4281496062992124485, 0.4176697321401328655 ) ) ;
#16771=CARTESIAN_POINT ( 'NONE',  ( 0.5905511811023629321, -0.6692913385826771977, 8.415575281601705876E-17 ) ) ;
#16772=CARTESIAN_POINT ( 'NONE',  ( 0.6233595800524942554, -0.05778040916215560624, -0.4822834645669293319 ) ) ;
#16774=CARTESIAN_POINT ( 'NONE',  ( -0.5905511811023613777, -0.5511811023622047445, 6.969142054262312111E-17 ) ) ;
#16778=CARTESIAN_POINT ( 'NONE',  ( -0.8989501312335946848, 0.1771653543307087075, -0.09757992244046823083 ) ) ;
#16779=CARTESIAN_POINT ( 'NONE',  ( -0.2624671916010490880, -0.6046776061558807314, 0.2411417322834647770 ) ) ;
#16781=CARTESIAN_POINT ( 'NONE',  ( -0.8530183727034112984, -0.4281496062992127816, -0.4176697321401328100 ) ) ;
#16782=CARTESIAN_POINT ( 'NONE',  ( -0.9580052493438311334, -0.4281496062992124485, 0.4176697321401328655 ) ) ;
#16783=CARTESIAN_POINT ( 'NONE',  ( -1.391076115485563314, -0.6046776061558809534, -0.2411417322834644161 ) ) ;
#16784=CARTESIAN_POINT ( 'NONE',  ( -1.240157480314959759, 0.1660481256975885056, 0.3530559997133364547 ) ) ;
#16786=CARTESIAN_POINT ( 'NONE',  ( 0.7480314960629927956, 0.1771653543307087630, 0.000000000000000000 ) ) ;
#16789=CARTESIAN_POINT ( 'NONE',  ( 0.07217847769028949700, -0.08942795157528024563, -0.3641732283464568787 ) ) ;
#16790=CARTESIAN_POINT ( 'NONE',  ( -0.05905511811023545637, 0.1660481256975885056, 0.3530559997133364547 ) ) ;
#16791=CARTESIAN_POINT ( 'NONE',  ( 0.07217847769028949700, -0.3162353388693405765, 0.4822834645669290543 ) ) ;
#16792=ORIENTED_EDGE ( 'NONE', *, *, #56212, .T. ) ;
#16795=ORIENTED_EDGE ( 'NONE', *, *, #80522, .T. ) ;
#16797=CARTESIAN_POINT ( 'NONE',  ( 1.594488188976378673, 0.1660481256975885056, 0.3530559997133364547 ) ) ;
#16798=CARTESIAN_POINT ( 'NONE',  ( -0.8136482939632537770, -0.5023911411419708095, 0.1820866141732285504 ) ) ;
#16799=CARTESIAN_POINT ( 'NONE',  ( -0.7874015748031489847, -0.1870078740157479769, 0.4822834645669291653 ) ) ;
#16801=ADVANCED_FACE ( 'NONE', ( #49186 ), #20409, .F. ) ;
#16802=CARTESIAN_POINT ( 'NONE',  ( -1.646051170424378096, 0.4405861044731112508, 0.5309055118110234117 ) ) ;
#16804=CARTESIAN_POINT ( 'NONE',  ( -1.620734908136482577, 0.1771653543307087630, 0.09757992244046791164 ) ) ;
#16805=CARTESIAN_POINT ( 'NONE',  ( 0.3871391076115492380, -0.05778040916215560624, -0.4822834645669293319 ) ) ;
#16806=CARTESIAN_POINT ( 'NONE',  ( 0.4790026246719168435, -0.3162353388693409650, -0.4822834645669289433 ) ) ;
#16807=CARTESIAN_POINT ( 'NONE',  ( -0.7545931758530176614, -0.5511811023622048555, -0.09757992244046775898 ) ) ;
#16808=CARTESIAN_POINT ( 'NONE',  ( 0.03280839895013198948, 0.2952755905511811885, 0.1292274648535926551 ) ) ;
#16810=CARTESIAN_POINT ( 'NONE',  ( -0.6364829396325453192, -0.3162353388693405765, 0.4822834645669290543 ) ) ;
#16813=CARTESIAN_POINT ( 'NONE',  ( 1.496062992125984703, -0.1870078740157480601, -0.3641732283464567677 ) ) ;
#16814=CARTESIAN_POINT ( 'NONE',  ( 0.1377952755905518800, -0.4536011799217367080, 0.2665933059059888421 ) ) ;
#16815=CARTESIAN_POINT ( 'NONE',  ( 1.030183727034121421, -0.08942795157527998196, 0.3641732283464567121 ) ) ;
#16816=CARTESIAN_POINT ( 'NONE',  ( -1.227034120734907585, 0.2952755905511811885, 0.1292274648535926551 ) ) ;
#16817=CARTESIAN_POINT ( 'NONE',  ( -1.345144356955379816, -0.2845877964562159024, 0.3641732283464567677 ) ) ;
#16818=CARTESIAN_POINT ( 'NONE',  ( -1.220472440944878834, 2.401574803149606474, -0.4915354330708643360 ) ) ;
#16819=CARTESIAN_POINT ( 'NONE',  ( -1.115485564304461219, -0.4281496062992124485, 0.4176697321401328655 ) ) ;
#16820=CARTESIAN_POINT ( 'NONE',  ( -0.3805774278215216522, 0.05413385826771666132, 0.4176697321401328100 ) ) ;
#16821=CARTESIAN_POINT ( 'NONE',  ( 0.3674540682414705883, -0.6046776061558807314, 0.2411417322834647770 ) ) ;
#16823=CARTESIAN_POINT ( 'NONE',  ( 1.091264520429693574, -3.876714527516387216E-16, -0.3954974714151466841 ) ) ;
#16824=CARTESIAN_POINT ( 'NONE',  ( 0.1443569553805781891, -0.004921259842519870586, -0.3153832671262229437 ) ) ;
#16825=CARTESIAN_POINT ( 'NONE',  ( 0.8464566929133865436, 0.1660481256975883668, -0.3530559997133364547 ) ) ;
#16826=CARTESIAN_POINT ( 'NONE',  ( -1.587926509186350810, -0.3690944881889763329, 0.3153832671262228327 ) ) ;
#16827=CARTESIAN_POINT ( 'NONE',  ( 0.8267716535433078384, -0.6692913385826771977, 8.415575281601705876E-17 ) ) ;
#16829=CARTESIAN_POINT ( 'NONE',  ( -1.476377952755905110, -0.5400638737290845981, -0.3530559997133363437 ) ) ;
#16830=CARTESIAN_POINT ( 'NONE',  ( -0.9448818897637790704, -0.1870078740157479769, 0.4822834645669291653 ) ) ;
#16831=CARTESIAN_POINT ( 'NONE',  ( -0.2034120734908128059, 0.1771653543307087630, 0.09757992244046791164 ) ) ;
#16833=CARTESIAN_POINT ( 'NONE',  ( 0.6167979002624678353, -0.3690944881889763329, 0.3153832671262228327 ) ) ;
#16835=CARTESIAN_POINT ( 'NONE',  ( 0.1049868766404206816, 0.2306618581243848609, 0.2411417322834645549 ) ) ;
#16837=CARTESIAN_POINT ( 'NONE',  ( -1.082677165354329896, 0.1660481256975885056, 0.3530559997133364547 ) ) ;
#16839=CARTESIAN_POINT ( 'NONE',  ( 0.8464566929133865436, 0.07958543189024071263, -0.2665933059059888421 ) ) ;
#16840=CARTESIAN_POINT ( 'NONE',  ( 0.1771653543307093182, -0.5400638737290845981, -0.3530559997133363437 ) ) ;
#16841=CARTESIAN_POINT ( 'NONE',  ( -0.4724409448818890911, -0.1870078740157480879, -0.4822834645669291653 ) ) ;
#16842=CARTESIAN_POINT ( 'NONE',  ( -0.2624671916010490880, -0.5023911411419708095, 0.1820866141732285504 ) ) ;
#16843=CARTESIAN_POINT ( 'NONE',  ( -1.646051170424378096, 0.000000000000000000, -0.3464511005275205946 ) ) ;
#16844=CARTESIAN_POINT ( 'NONE',  ( -0.3412073490813641308, 0.1283753931104746893, -0.1820866141732285504 ) ) ;
#16845=CARTESIAN_POINT ( 'NONE',  ( 0.4921259842519691285, -0.5400638737290845981, -0.3530559997133363437 ) ) ;
#16846=CARTESIAN_POINT ( 'NONE',  ( -1.017060367454067249, -0.2845877964562161244, -0.3641732283464567121 ) ) ;
#16849=CARTESIAN_POINT ( 'NONE',  ( 1.522309711286089939, -0.6046776061558809534, -0.2411417322834644161 ) ) ;
#16850=DIRECTION ( 'NONE',  ( -1.000000000000000000, -3.050063254464715288E-16, 0.000000000000000000 ) ) ;
#16852=CARTESIAN_POINT ( 'NONE',  ( -1.574803149606298636, -0.1870078740157479769, 0.3641732283464567677 ) ) ;
#16853=CARTESIAN_POINT ( 'NONE',  ( -0.4724409448818890911, -0.1870078740157479769, 0.4822834645669291653 ) ) ;
#16854=CARTESIAN_POINT ( 'NONE',  ( -1.272965879265091305, 0.05413385826771626580, -0.4176697321401330321 ) ) ;
#16857=CARTESIAN_POINT ( 'NONE',  ( 1.312335958005250269, -0.6046776061558807314, 0.2411417322834647770 ) ) ;
#16858=CARTESIAN_POINT ( 'NONE',  ( 0.6299212598425204535, -0.1870078740157480879, -0.4822834645669291653 ) ) ;
#16861=CARTESIAN_POINT ( 'NONE',  ( -1.548556430446193399, 0.2306618581243848609, 0.2411417322834645549 ) ) ;
#16865=CARTESIAN_POINT ( 'NONE',  ( -0.8727034120734901146, -0.2845877964562159024, 0.3641732283464567677 ) ) ;
#16868=CARTESIAN_POINT ( 'NONE',  ( 0.6824146981627303710, 0.2306618581243847221, -0.2411417322834647770 ) ) ;
#16869=CARTESIAN_POINT ( 'NONE',  ( -0.1771653543307080136, -0.5400638737290844871, 0.3530559997133364547 ) ) ;
#16870=CARTESIAN_POINT ( 'NONE',  ( -1.174540682414697335, -0.05778040916215522460, 0.4822834645669289988 ) ) ;
#16871=CARTESIAN_POINT ( 'NONE',  ( 1.030183727034121421, -0.05778040916215522460, 0.4822834645669289988 ) ) ;
#16872=CARTESIAN_POINT ( 'NONE',  ( -1.089238845144356427, -0.3690944881889765550, -0.3153832671262227771 ) ) ;
#16874=CARTESIAN_POINT ( 'NONE',  ( 0.4593175853018380828, 0.05413385826771626580, -0.4176697321401330321 ) ) ;
#16875=CARTESIAN_POINT ( 'NONE',  ( -0.9448818897637790704, -0.1870078740157480879, -0.4822834645669291653 ) ) ;
#16877=FACE_OUTER_BOUND ( 'NONE', #25206, .T. ) ;
#16879=CARTESIAN_POINT ( 'NONE',  ( 1.056430446194226658, 0.2952755905511811885, 0.1292274648535926551 ) ) ;
#16881=CARTESIAN_POINT ( 'NONE',  ( 1.358267716535433323, 0.07958543189024085140, 0.2665933059059887866 ) ) ;
#16882=EDGE_LOOP ( 'NONE', ( #4729, #20294, #8279, #30543, #23475 ) ) ;
#16884=CARTESIAN_POINT ( 'NONE',  ( -0.2296587926509179312, -0.05778040916215522460, 0.4822834645669289988 ) ) ;
#16885=VERTEX_POINT ( 'NONE', #21997 ) ;
#16886=CARTESIAN_POINT ( 'NONE',  ( 0.2427821522309716595, -0.2845877964562161244, -0.3641732283464567121 ) ) ;
#16887=CARTESIAN_POINT ( 'NONE',  ( -1.692913385826770645, 0.2952755905511811885, 0.000000000000000000 ) ) ;
#16888=CARTESIAN_POINT ( 'NONE',  ( 0.5708661417322841158, -0.5400638737290845981, -0.3530559997133363437 ) ) ;
#16889=CARTESIAN_POINT ( 'NONE',  ( 0.9251968503937015864, -0.5400638737290844871, 0.3530559997133364547 ) ) ;
#16890=CARTESIAN_POINT ( 'NONE',  ( 0.03280839895013198948, 0.2952755905511811885, 0.1292274648535926551 ) ) ;
#16892=CARTESIAN_POINT ( 'NONE',  ( -0.7349081364829387342, -0.6046776061558807314, 0.2411417322834647770 ) ) ;
#16894=CARTESIAN_POINT ( 'NONE',  ( 1.587926509186352142, -0.004921259842519576551, 0.3153832671262227771 ) ) ;
#16895=CARTESIAN_POINT ( 'NONE',  ( -0.8267716535433065062, 0.2952755905511811885, 0.000000000000000000 ) ) ;
#16896=CARTESIAN_POINT ( 'NONE',  ( 1.476377952755906442, -0.5400638737290844871, 0.3530559997133364547 ) ) ;
#16897=CARTESIAN_POINT ( 'NONE',  ( 1.305774278215223960, -0.6692913385826771977, 0.1292274648535927661 ) ) ;
#16899=CARTESIAN_POINT ( 'NONE',  ( -0.7217847769028863381, 0.05413385826771626580, -0.4176697321401330321 ) ) ;
#16901=CARTESIAN_POINT ( 'NONE',  ( 0.1049868766404206816, -0.6046776061558809534, -0.2411417322834644161 ) ) ;
#16903=CARTESIAN_POINT ( 'NONE',  ( -0.5905511811023613777, -0.6692913385826771977, 8.415575281601705876E-17 ) ) ;
#16904=CIRCLE ( 'NONE', #6109, 2.362204724409449064 ) ;
#16905=CARTESIAN_POINT ( 'NONE',  ( 1.620734908136483465, -0.6692913385826771977, 0.1292274648535927661 ) ) ;
#16906=CARTESIAN_POINT ( 'NONE',  ( 0.7480314960629927956, 0.1771653543307087630, 0.000000000000000000 ) ) ;
#16907=CARTESIAN_POINT ( 'NONE',  ( 1.220472440944882386, -0.6692913385826771977, 8.415575281601705876E-17 ) ) ;
#16909=CARTESIAN_POINT ( 'NONE',  ( 0.9645669291338591078, -0.4536011799217368745, -0.2665933059059886201 ) ) ;
#16910=CARTESIAN_POINT ( 'NONE',  ( 0.6758530183727039509, 0.2952755905511810774, -0.1292274648535930714 ) ) ;
#16912=CARTESIAN_POINT ( 'NONE',  ( -1.003937007874015297, -0.5400638737290845981, -0.3530559997133363437 ) ) ;
#16913=CARTESIAN_POINT ( 'NONE',  ( -1.603475055217291612, 2.157339783260149080, -0.04573490813648262154 ) ) ;
#16914=CARTESIAN_POINT ( 'NONE',  ( 1.154855643044620184, 0.1283753931104746893, -0.1820866141732285504 ) ) ;
#16915=CARTESIAN_POINT ( 'NONE',  ( -0.4593175853018366950, 0.05413385826771666132, 0.4176697321401328100 ) ) ;
#16916=CARTESIAN_POINT ( 'NONE',  ( 0.03937007874015806264, 0.2952755905511811885, 0.000000000000000000 ) ) ;
#16917=CARTESIAN_POINT ( 'NONE',  ( 0.1689764809739037477, -2.839693391405754848E-15, 0.3791475997938237308 ) ) ;
#16918=CARTESIAN_POINT ( 'NONE',  ( -0.09842519685039295696, 0.1660481256975883668, -0.3530559997133364547 ) ) ;
#16919=CARTESIAN_POINT ( 'NONE',  ( 0.01312335958005323398, -0.3690944881889765550, -0.3153832671262227771 ) ) ;
#16921=CARTESIAN_POINT ( 'NONE',  ( 0.1640419947506569498, -0.2845877964562161244, -0.3641732283464567121 ) ) ;
#16922=CARTESIAN_POINT ( 'NONE',  ( 0.6627296587926515548, 0.1771653543307087630, 0.09757992244046791164 ) ) ;
#16923=DIRECTION ( 'NONE',  ( 0.000000000000000000, 0.000000000000000000, 1.000000000000000000 ) ) ;
#16925=CARTESIAN_POINT ( 'NONE',  ( 0.3937007874015754361, -0.1870078740157479769, 0.4822834645669291653 ) ) ;
#16927=CARTESIAN_POINT ( 'NONE',  ( 1.410761154855643795, -0.08942795157528024563, -0.3641732283464568787 ) ) ;
#16928=DIRECTION ( 'NONE',  ( 0.000000000000000000, 0.000000000000000000, 1.000000000000000000 ) ) ;
#16929=CARTESIAN_POINT ( 'NONE',  ( -0.5380577427821514602, -0.3690944881889765550, -0.3153832671262227771 ) ) ;
#16930=CARTESIAN_POINT ( 'NONE',  ( 0.2690288713910767848, 0.2952755905511811885, 0.1292274648535926551 ) ) ;
#16931=CARTESIAN_POINT ( 'NONE',  ( 1.233595800524935227, 0.1283753931104746893, -0.1820866141732285504 ) ) ;
#16932=CARTESIAN_POINT ( 'NONE',  ( -1.437007874015747477, -0.4536011799217367080, 0.2665933059059888421 ) ) ;
#16933=CARTESIAN_POINT ( 'NONE',  ( -1.574803149606298636, -0.1870078740157479769, 0.4822834645669291653 ) ) ;
#16934=CARTESIAN_POINT ( 'NONE',  ( 0.2755905511811031494, 0.2952755905511811885, 0.000000000000000000 ) ) ;
#16935=CARTESIAN_POINT ( 'NONE',  ( 1.377952755905512472, 0.2952755905511811885, 0.000000000000000000 ) ) ;
#16937=CARTESIAN_POINT ( 'NONE',  ( 0.1640419947506569498, -0.05778040916215522460, 0.4822834645669289988 ) ) ;
#16938=CARTESIAN_POINT ( 'NONE',  ( 1.404199475065617708, 0.05413385826771626580, -0.4176697321401330321 ) ) ;
#16939=CARTESIAN_POINT ( 'NONE',  ( 0.8595800524934390507, -0.3162353388693405765, 0.4822834645669290543 ) ) ;
#16941=CARTESIAN_POINT ( 'NONE',  ( 0.9645669291338591078, -0.4536011799217368745, -0.2665933059059886201 ) ) ;
#16942=CARTESIAN_POINT ( 'NONE',  ( 1.476377952755906442, -0.5400638737290844871, 0.3530559997133364547 ) ) ;
#16943=CARTESIAN_POINT ( 'NONE',  ( -0.06561679790026180015, -0.3690944881889765550, -0.3153832671262227771 ) ) ;
#16944=CARTESIAN_POINT ( 'NONE',  ( -0.09186351706036663400, -0.4281496062992124485, 0.4176697321401328655 ) ) ;
#16945=CARTESIAN_POINT ( 'NONE',  ( 0.6561679790026253567, 0.2306618581243848609, 0.2411417322834645549 ) ) ;
#16946=CARTESIAN_POINT ( 'NONE',  ( -0.4002624671916004129, -0.3162353388693405765, 0.4822834645669290543 ) ) ;
#16948=CARTESIAN_POINT ( 'NONE',  ( -0.2165354330708654795, -0.4536011799217368745, -0.2665933059059886201 ) ) ;
#16949=CARTESIAN_POINT ( 'NONE',  ( 0.6824146981627303710, 0.2306618581243847221, -0.2411417322834647770 ) ) ;
#16950=CARTESIAN_POINT ( 'NONE',  ( 0.8595800524934390507, -0.2845877964562159024, 0.3641732283464567677 ) ) ;
#16954=FACE_OUTER_BOUND ( 'NONE', #65858, .T. ) ;
#16955=CARTESIAN_POINT ( 'NONE',  ( -1.200787401574802349, 0.1012011053420775880, -0.2882089793578257453 ) ) ;
#16956=CARTESIAN_POINT ( 'NONE',  ( -1.220472440944881054, -0.6692913385826771977, 8.415575281601705876E-17 ) ) ;
#16958=CARTESIAN_POINT ( 'NONE',  ( -0.3937007874015740483, -0.1870078740157480879, -0.4822834645669291653 ) ) ;
#16962=CARTESIAN_POINT ( 'NONE',  ( 0.3215223097112867578, -0.2845877964562161244, -0.3641732283464567121 ) ) ;
#16964=CARTESIAN_POINT ( 'NONE',  ( 1.213910761154856299, -0.6692913385826773087, -0.1292274648535924053 ) ) ;
#16966=CARTESIAN_POINT ( 'NONE',  ( -1.220472440944881054, 0.2952755905511811885, 0.000000000000000000 ) ) ;
#16968=CARTESIAN_POINT ( 'NONE',  ( 1.463254593175853824, -0.6692913385826771977, 0.1292274648535927661 ) ) ;
#16969=CARTESIAN_POINT ( 'NONE',  ( 1.404199475065617264, -0.3690944881889763329, 0.3153832671262228327 ) ) ;
#16970=CARTESIAN_POINT ( 'NONE',  ( 0.6036745406824154392, 0.2306618581243847221, -0.2411417322834647770 ) ) ;
#16972=CARTESIAN_POINT ( 'NONE',  ( -0.07874015748031421014, -0.1870078740157479769, 0.4822834645669291653 ) ) ;
#16973=CARTESIAN_POINT ( 'NONE',  ( -0.8398950131233589023, -0.5023911411419708095, -0.1820866141732282451 ) ) ;
#16974=CARTESIAN_POINT ( 'NONE',  ( 0.3871391076115492380, -0.05778040916215560624, -0.4822834645669293319 ) ) ;
#16975=CARTESIAN_POINT ( 'NONE',  ( 0.09186351706036799403, -0.4281496062992127816, -0.4176697321401328100 ) ) ;
#16977=CARTESIAN_POINT ( 'NONE',  ( -0.01109768429471590621, 1.490381362800744269E-15, -0.3954974714151453519 ) ) ;
#16979=CARTESIAN_POINT ( 'NONE',  ( 0.6955380577427828781, -0.4281496062992124485, 0.4176697321401328655 ) ) ;
#16980=CARTESIAN_POINT ( 'NONE',  ( -0.2296587926509179312, -0.3162353388693409650, -0.4822834645669289433 ) ) ;
#16981=CARTESIAN_POINT ( 'NONE',  ( -1.541994750656167090, -0.6692913385826773087, -0.1292274648535924053 ) ) ;
#16982=CARTESIAN_POINT ( 'NONE',  ( 1.010498687664042716, 0.05413385826771626580, -0.4176697321401330321 ) ) ;
#16983=CARTESIAN_POINT ( 'NONE',  ( 0.5183727034120741983, -0.6692913385826771977, 0.1292274648535927661 ) ) ;
#16985=CARTESIAN_POINT ( 'NONE',  ( -0.4068241469816267775, 0.05413385826771626580, -0.4176697321401330321 ) ) ;
#16986=CARTESIAN_POINT ( 'NONE',  ( 0.1312335958005257930, 0.2306618581243847221, -0.2411417322834647770 ) ) ;
#16987=CARTESIAN_POINT ( 'NONE',  ( -0.5052493438320203589, 0.2952755905511810774, -0.1292274648535930714 ) ) ;
#16988=CARTESIAN_POINT ( 'NONE',  ( 0.4527559055118117182, 0.07958543189024071263, -0.2665933059059888421 ) ) ;
#16989=CARTESIAN_POINT ( 'NONE',  ( 1.614173228346457378, -0.5511811023622047445, 6.969142054262312111E-17 ) ) ;
#16990=CARTESIAN_POINT ( 'NONE',  ( -1.725721784776902190, -0.05778040916215522460, 0.4822834645669289988 ) ) ;
#16991=CARTESIAN_POINT ( 'NONE',  ( 0.4330708661417329575, -0.6692913385826771977, 8.415575281601705876E-17 ) ) ;
#16992=CARTESIAN_POINT ( 'NONE',  ( 1.463254593175853824, 0.2952755905511810774, -0.1292274648535930714 ) ) ;
#16997=CARTESIAN_POINT ( 'NONE',  ( 0.7152230971128616943, -0.05778040916215522460, 0.4822834645669289988 ) ) ;
#16998=CARTESIAN_POINT ( 'NONE',  ( 0.1902887139107617975, 0.1771653543307087630, 0.09757992244046791164 ) ) ;
#17001=CARTESIAN_POINT ( 'NONE',  ( 1.660104986876641320, -0.08942795157527998196, 0.3641732283464567121 ) ) ;
#17002=DIRECTION ( 'NONE',  ( -3.096699300667737957E-16, 1.000000000000000000, -0.000000000000000000 ) ) ;
#17004=FACE_OUTER_BOUND ( 'NONE', #37860, .T. ) ;
#17007=CARTESIAN_POINT ( 'NONE',  ( 0.7217847769028878924, -0.4281496062992127816, -0.4176697321401328100 ) ) ;
#17008=CARTESIAN_POINT ( 'NONE',  ( -0.8070866141732276899, 0.1660481256975883668, -0.3530559997133364547 ) ) ;
#17009=CARTESIAN_POINT ( 'NONE',  ( -0.7939632545931754048, -0.3162353388693405765, 0.4822834645669290543 ) ) ;
#17010=CARTESIAN_POINT ( 'NONE',  ( 0.7742782152230978099, -0.4281496062992124485, 0.4176697321401328655 ) ) ;
#17011=CARTESIAN_POINT ( 'NONE',  ( 1.194225721784777594, -0.4281496062992127816, -0.4176697321401328100 ) ) ;
#17014=CARTESIAN_POINT ( 'NONE',  ( 1.246719160104987623, -0.004921259842519870586, -0.3153832671262229437 ) ) ;
#17015=CARTESIAN_POINT ( 'NONE',  ( -1.003937007874014853, 0.1660481256975885056, 0.3530559997133364547 ) ) ;
#17016=CARTESIAN_POINT ( 'NONE',  ( 1.614173228346457378, -0.6692913385826771977, 8.415575281601705876E-17 ) ) ;
#17018=CARTESIAN_POINT ( 'NONE',  ( 0.03937007874015833325, -0.6692913385826771977, 8.415575281601705876E-17 ) ) ;
#17019=VECTOR ( 'NONE', #33452, 39.37007874015748143 ) ;
#17020=CARTESIAN_POINT ( 'NONE',  ( 1.049868766404200349, 0.2306618581243848609, 0.2411417322834645549 ) ) ;
#17021=CARTESIAN_POINT ( 'NONE',  ( 0.4687358108553574265, 1.787282772535975672, -0.5180085934481405419 ) ) ;
#17022=CARTESIAN_POINT ( 'NONE',  ( -1.305774278215222184, -0.5511811023622048555, -0.09757992244046775898 ) ) ;
#17023=CARTESIAN_POINT ( 'NONE',  ( 0.3674540682414705883, -0.6046776061558807314, 0.2411417322834647770 ) ) ;
#17024=CARTESIAN_POINT ( 'NONE',  ( 1.220472440944882386, -0.5511811023622047445, 6.969142054262312111E-17 ) ) ;
#17026=CARTESIAN_POINT ( 'NONE',  ( -1.141732283464566011, -0.5511811023622047445, 6.969142054262312111E-17 ) ) ;
#17027=CARTESIAN_POINT ( 'NONE',  ( 1.469816272965879911, -0.6046776061558807314, 0.2411417322834647770 ) ) ;
#17029=CARTESIAN_POINT ( 'NONE',  ( -0.06561679790026180015, -0.3690944881889765550, -0.3153832671262227771 ) ) ;
#17030=CARTESIAN_POINT ( 'NONE',  ( -0.1902887139107604098, -0.6692913385826771977, 0.1292274648535927661 ) ) ;
#17031=CARTESIAN_POINT ( 'NONE',  ( -1.286089238845143479, 0.1283753931104746893, -0.1820866141732285504 ) ) ;
#17032=CARTESIAN_POINT ( 'NONE',  ( -0.9186351706036736120, 0.2306618581243848609, 0.2411417322834645549 ) ) ;
#17033=CARTESIAN_POINT ( 'NONE',  ( 1.509186351706037543, 0.05413385826771666132, 0.4176697321401328100 ) ) ;
#17036=CARTESIAN_POINT ( 'NONE',  ( 1.207349081364829990, -0.6046776061558809534, -0.2411417322834644161 ) ) ;
#17038=CARTESIAN_POINT ( 'NONE',  ( -1.299212598425196097, -0.6692913385826771977, 8.415575281601705876E-17 ) ) ;
#17039=CARTESIAN_POINT ( 'NONE',  ( -1.062992125984250968, -0.5511811023622047445, 6.969142054262312111E-17 ) ) ;
#17040=CARTESIAN_POINT ( 'NONE',  ( -0.7677165354330699465, 0.07958543189024085140, 0.2665933059059887866 ) ) ;
#17042=CARTESIAN_POINT ( 'NONE',  ( -0.1443569553805765515, -0.4281496062992127816, -0.4176697321401328100 ) ) ;
#17043=CARTESIAN_POINT ( 'NONE',  ( -0.1049868766404193215, -0.5023911411419708095, 0.1820866141732285504 ) ) ;
#17044=CARTESIAN_POINT ( 'NONE',  ( -0.9514435695538050464, -0.2845877964562159024, 0.3641732283464567677 ) ) ;
#17045=CARTESIAN_POINT ( 'NONE',  ( -1.660104986876639543, -0.05778040916215560624, -0.4822834645669293319 ) ) ;
#17046=CARTESIAN_POINT ( 'NONE',  ( 1.509186351706037543, -0.3690944881889765550, -0.3153832671262227771 ) ) ;
#17047=CARTESIAN_POINT ( 'NONE',  ( 1.332020997375329197, -0.3162353388693405765, 0.4822834645669290543 ) ) ;
#17049=CARTESIAN_POINT ( 'NONE',  ( 0.4068241469816281097, -0.004921259842519576551, 0.3153832671262227771 ) ) ;
#17050=CARTESIAN_POINT ( 'NONE',  ( 0.8727034120734913358, -0.05778040916215522460, 0.4822834645669289988 ) ) ;
#17051=CARTESIAN_POINT ( 'NONE',  ( 1.082677165354331228, -0.4536011799217367080, 0.2665933059059888421 ) ) ;
#17053=CARTESIAN_POINT ( 'NONE',  ( -1.043307086614172041, -0.5400638737290844871, 0.3530559997133364547 ) ) ;
#17055=CARTESIAN_POINT ( 'NONE',  ( -1.049868766404198794, -0.6046776061558807314, 0.2411417322834647770 ) ) ;
#17056=CARTESIAN_POINT ( 'NONE',  ( 0.006561679790026889343, -0.05778040916215522460, 0.4822834645669289988 ) ) ;
#17060=CARTESIAN_POINT ( 'NONE',  ( 1.030183727034121421, -0.3162353388693409650, -0.4822834645669289433 ) ) ;
#17061=CARTESIAN_POINT ( 'NONE',  ( 1.410761154855643795, -0.2845877964562159024, 0.3641732283464567677 ) ) ;
#17063=VECTOR ( 'NONE', #41062, 39.37007874015748143 ) ;
#17064=CARTESIAN_POINT ( 'NONE',  ( -0.03937007874015669567, 0.2952755905511811885, 0.000000000000000000 ) ) ;
#17065=CARTESIAN_POINT ( 'NONE',  ( 0.8005249343832027131, 0.05413385826771666132, 0.4176697321401328100 ) ) ;
#17071=CARTESIAN_POINT ( 'NONE',  ( -0.5971128608923877978, 0.1771653543307087630, 0.09757992244046791164 ) ) ;
#17072=CARTESIAN_POINT ( 'NONE',  ( -0.6889763779527552368, -0.5400638737290845981, -0.3530559997133363437 ) ) ;
#17073=CARTESIAN_POINT ( 'NONE',  ( 0.4199475065616803948, -0.6046776061558809534, -0.2411417322834644161 ) ) ;
#17075=CARTESIAN_POINT ( 'NONE',  ( 1.594488188976378673, 0.1660481256975885056, 0.3530559997133364547 ) ) ;
#17076=CARTESIAN_POINT ( 'NONE',  ( 1.318897637795276356, 0.1660481256975883668, -0.3530559997133364547 ) ) ;
#17080=CARTESIAN_POINT ( 'NONE',  ( 1.128608923884514947, 0.2306618581243848609, 0.2411417322834645549 ) ) ;
#17081=CARTESIAN_POINT ( 'NONE',  ( 1.227034120734908917, -0.5511811023622046335, 0.09757992244046803654 ) ) ;
#17082=CARTESIAN_POINT ( 'NONE',  ( 1.574803149606299746, -0.1870078740157480879, -0.4822834645669291653 ) ) ;
#17083=CARTESIAN_POINT ( 'NONE',  ( -1.541994750656167090, -0.6692913385826773087, -0.1292274648535924053 ) ) ;
#17086=CARTESIAN_POINT ( 'NONE',  ( 0.9711286089238851948, -0.6046776061558809534, -0.2411417322834644161 ) ) ;
#17087=CARTESIAN_POINT ( 'NONE',  ( 1.607611548556431069, -0.5511811023622048555, -0.09757992244046775898 ) ) ;
#17088=CARTESIAN_POINT ( 'NONE',  ( -0.6692913385826764205, -0.6692913385826771977, 8.415575281601705876E-17 ) ) ;
#17089=CARTESIAN_POINT ( 'NONE',  ( -0.5905511811023615998, 0.2952755905511811885, 0.000000000000000000 ) ) ;
#17091=CARTESIAN_POINT ( 'NONE',  ( -1.607611548556429737, 0.2952755905511810774, -0.1292274648535930714 ) ) ;
#17092=B_SPLINE_CURVE_WITH_KNOTS ( 'NONE', 3,
 ( #78498, #14526, #66272, #60774 ),
 .UNSPECIFIED., .F., .F.,
 ( 4, 4 ),
 ( 3.593986969197074577E-07, 0.001287825409103162408 ),
 .UNSPECIFIED. ) ;
#17094=CARTESIAN_POINT ( 'NONE',  ( 0.03280839895013198948, 0.2952755905511811885, 0.1292274648535926551 ) ) ;
#17096=CARTESIAN_POINT ( 'NONE',  ( 1.594488188976378673, -0.5400638737290845981, -0.3530559997133363437 ) ) ;
#17097=VERTEX_POINT ( 'NONE', #59052 ) ;
#17099=EDGE_LOOP ( 'NONE', ( #61475, #11680, #31244, #67774 ) ) ;
#17100=CARTESIAN_POINT ( 'NONE',  ( -0.06596743314205839870, 0.004960608223778821026, 0.3437734562760189072 ) ) ;
#17101=CARTESIAN_POINT ( 'NONE',  ( -1.351706036745406347, 0.05413385826771626580, -0.4176697321401330321 ) ) ;
#17103=FACE_OUTER_BOUND ( 'NONE', #28662, .T. ) ;
#17104=CARTESIAN_POINT ( 'NONE',  ( -0.7137454485294959516, 2.001539355558159983, 0.4917280318828578523 ) ) ;
#17109=CARTESIAN_POINT ( 'NONE',  ( -0.2821522309711278487, -0.5511811023622048555, -0.09757992244046775898 ) ) ;
#17110=CARTESIAN_POINT ( 'NONE',  ( -1.312335958005248715, -0.5023911411419708095, -0.1820866141732282451 ) ) ;
#17111=CARTESIAN_POINT ( 'NONE',  ( 1.581364829396326277, -0.05778040916215522460, 0.4822834645669289988 ) ) ;
#17112=CARTESIAN_POINT ( 'NONE',  ( 0.3543307086614179147, 0.2952755905511811885, 0.000000000000000000 ) ) ;
#17113=CARTESIAN_POINT ( 'NONE',  ( -1.220472440944881054, -0.6692913385826771977, 8.415575281601705876E-17 ) ) ;
#17116=CARTESIAN_POINT ( 'NONE',  ( 1.555118110236221041, -0.5400638737290844871, 0.3530559997133364547 ) ) ;
#17117=LINE ( 'NONE', #68447, #9801 ) ;
#17121=AXIS2_PLACEMENT_3D ( 'NONE', #33164, #50834, #83255 ) ;
#17122=DIRECTION ( 'NONE',  ( 1.000000000000000000, 0.000000000000000000, -1.692413147294446216E-16 ) ) ;
#17123=CARTESIAN_POINT ( 'NONE',  ( -0.9514435695538050464, -0.05778040916215560624, -0.4822834645669293319 ) ) ;
#17124=CARTESIAN_POINT ( 'NONE',  ( 1.627296587926509996, -0.6046776061558807314, 0.2411417322834647770 ) ) ;
#17127=CARTESIAN_POINT ( 'NONE',  ( 0.7202472836732369821, 0.02791078216816263863, 0.4328096321851903627 ) ) ;
#17128=CARTESIAN_POINT ( 'NONE',  ( 0.6430446194225728496, 0.009842519685039463617, 0.3409548833797002576 ) ) ;
#17129=CARTESIAN_POINT ( 'NONE',  ( 1.535433070866142558, 0.2952755905511811885, 0.000000000000000000 ) ) ;
#17130=CARTESIAN_POINT ( 'NONE',  ( -0.9186351706036736120, 0.2306618581243848609, 0.2411417322834645549 ) ) ;
#17132=CARTESIAN_POINT ( 'NONE',  ( -0.06561679790026180015, -0.3690944881889765550, -0.3153832671262227771 ) ) ;
#17134=CARTESIAN_POINT ( 'NONE',  ( 0.01312335958005323398, -0.3690944881889765550, -0.3153832671262227771 ) ) ;
#17135=CARTESIAN_POINT ( 'NONE',  ( 0.7152230971128614723, -0.2845877964562161244, -0.3641732283464567121 ) ) ;
#17136=CARTESIAN_POINT ( 'NONE',  ( 0.4527559055118117182, -0.5400638737290844871, 0.3530559997133364547 ) ) ;
#17137=CARTESIAN_POINT ( 'NONE',  ( -0.8530183727034112984, -0.004921259842519576551, 0.3153832671262227771 ) ) ;
#17139=CARTESIAN_POINT ( 'NONE',  ( -1.528871391076114250, -0.6692913385826771977, 0.1292274648535927661 ) ) ;
#17140=CARTESIAN_POINT ( 'NONE',  ( -1.220472440944881054, -0.6692913385826771977, 8.415575281601705876E-17 ) ) ;
#17142=CARTESIAN_POINT ( 'NONE',  ( 0.09842519685039434474, -0.5400638737290845981, -0.3530559997133363437 ) ) ;
#17143=CARTESIAN_POINT ( 'NONE',  ( -0.4790026246719152336, -0.05778040916215560624, -0.4822834645669293319 ) ) ;
#17144=CARTESIAN_POINT ( 'NONE',  ( 1.312335958005250269, -0.5023911411419708095, 0.1820866141732285504 ) ) ;
#17145=CARTESIAN_POINT ( 'NONE',  ( 0.3083989501312343062, -0.2845877964562159024, 0.3641732283464567677 ) ) ;
#17146=CARTESIAN_POINT ( 'NONE',  ( -0.3871391076115479057, -0.3162353388693409650, -0.4822834645669289433 ) ) ;
#17147=CARTESIAN_POINT ( 'NONE',  ( -0.7086614173228339419, -0.1870078740157479769, 0.4822834645669291653 ) ) ;
#17148=DIRECTION ( 'NONE',  ( 1.000000000000000000, -0.000000000000000000, -0.000000000000000000 ) ) ;
#17149=LINE ( 'NONE', #49925, #8646 ) ;
#17150=CARTESIAN_POINT ( 'NONE',  ( 0.2165354330708668673, -0.5400638737290844871, 0.3530559997133364547 ) ) ;
#17153=CARTESIAN_POINT ( 'NONE',  ( 1.141732283464567566, 0.2952755905511811885, 0.000000000000000000 ) ) ;
#17154=CARTESIAN_POINT ( 'NONE',  ( -0.4396325459317579898, 0.1771653543307087630, 0.09757992244046791164 ) ) ;
#17155=CARTESIAN_POINT ( 'NONE',  ( -0.6561679790026240244, -0.6046776061558807314, 0.2411417322834647770 ) ) ;
#17156=CARTESIAN_POINT ( 'NONE',  ( 1.456692913385827515, -0.6692913385826771977, 8.415575281601705876E-17 ) ) ;
#17157=CARTESIAN_POINT ( 'NONE',  ( 0.8727034120734913358, -0.05778040916215522460, 0.4822834645669289988 ) ) ;
#17158=CARTESIAN_POINT ( 'NONE',  ( -1.522309711286088607, -0.6046776061558807314, 0.2411417322834647770 ) ) ;
#17159=CARTESIAN_POINT ( 'NONE',  ( -1.017060367454067249, -0.2845877964562161244, -0.3641732283464567121 ) ) ;
#17163=CARTESIAN_POINT ( 'NONE',  ( 1.594488188976378673, -0.4536011799217368745, -0.2665933059059886201 ) ) ;
#17164=CARTESIAN_POINT ( 'NONE',  ( 1.017060367454068581, -0.08942795157528024563, -0.3641732283464568787 ) ) ;
#17165=CARTESIAN_POINT ( 'NONE',  ( 0.3674540682414705883, 0.2306618581243847221, -0.2411417322834647770 ) ) ;
#17166=CARTESIAN_POINT ( 'NONE',  ( -1.660104986876639543, -0.05778040916215560624, -0.4822834645669293319 ) ) ;
#17168=CARTESIAN_POINT ( 'NONE',  ( 0.7742782152230979209, -0.004921259842519870586, -0.3153832671262229437 ) ) ;
#17169=CARTESIAN_POINT ( 'NONE',  ( -0.3083989501312330295, -0.3162353388693409650, -0.4822834645669289433 ) ) ;
#17170=CARTESIAN_POINT ( 'NONE',  ( -0.7152230971128602510, -0.3162353388693405765, 0.4822834645669290543 ) ) ;
#17171=CARTESIAN_POINT ( 'NONE',  ( 1.286089238845145033, -0.6046776061558809534, -0.2411417322834644161 ) ) ;
#17175=CARTESIAN_POINT ( 'NONE',  ( 0.1115485564304467270, -0.5511811023622048555, -0.09757992244046775898 ) ) ;
#17179=CARTESIAN_POINT ( 'NONE',  ( -0.7283464566929126471, 0.1660481256975883668, -0.3530559997133364547 ) ) ;
#17180=CARTESIAN_POINT ( 'NONE',  ( -0.1049868766404193215, -0.6046776061558807314, 0.2411417322834647770 ) ) ;
#17181=CARTESIAN_POINT ( 'NONE',  ( -0.3280839895013117347, 0.05413385826771626580, -0.4176697321401330321 ) ) ;
#17182=CARTESIAN_POINT ( 'NONE',  ( 0.9580052493438327987, -0.4281496062992127816, -0.4176697321401328100 ) ) ;
#17183=CARTESIAN_POINT ( 'NONE',  ( -0.3937007874015740483, -0.1870078740157479769, 0.4822834645669291653 ) ) ;
#17184=CARTESIAN_POINT ( 'NONE',  ( -1.318897637795274802, 0.1660481256975885056, 0.3530559997133364547 ) ) ;
#17185=CARTESIAN_POINT ( 'NONE',  ( -0.4921259842519677963, -0.5400638737290844871, 0.3530559997133364547 ) ) ;
#17186=CARTESIAN_POINT ( 'NONE',  ( 0.7152230971128614723, -0.3162353388693409650, -0.4822834645669289433 ) ) ;
#17187=ADVANCED_FACE ( 'NONE', ( #34215 ), #49406, .F. ) ;
#17188=CARTESIAN_POINT ( 'NONE',  ( 0.4527559055118117182, -0.5400638737290844871, 0.3530559997133364547 ) ) ;
#17190=CARTESIAN_POINT ( 'NONE',  ( -0.5183727034120726440, 0.1771653543307087630, 0.09757992244046791164 ) ) ;
#17194=CARTESIAN_POINT ( 'NONE',  ( -1.476377952755905110, -0.4536011799217368745, -0.2665933059059886201 ) ) ;
#17195=CARTESIAN_POINT ( 'NONE',  ( -0.3674540682414689785, 0.2306618581243848609, 0.2411417322834645549 ) ) ;
#17197=CARTESIAN_POINT ( 'NONE',  ( -0.8070866141732276899, -0.5400638737290844871, 0.3530559997133364547 ) ) ;
#17198=CARTESIAN_POINT ( 'NONE',  ( -0.7611548556430438595, 0.2306618581243848609, 0.2411417322834645549 ) ) ;
#17199=CARTESIAN_POINT ( 'NONE',  ( -1.450131233595799651, 0.2952755905511810774, -0.1292274648535930714 ) ) ;
#17200=CYLINDRICAL_SURFACE ( 'NONE', #61721, 0.3937007874015748254 ) ;
#17201=CARTESIAN_POINT ( 'NONE',  ( 0.9055118110236227702, 0.1771653543307087630, 0.000000000000000000 ) ) ;
#17204=CARTESIAN_POINT ( 'NONE',  ( 0.1115485564304467270, -0.5511811023622048555, -0.09757992244046775898 ) ) ;
#17205=CARTESIAN_POINT ( 'NONE',  ( -0.4724409448818890911, -0.1870078740157480879, -0.4822834645669291653 ) ) ;
#17207=CARTESIAN_POINT ( 'NONE',  ( 0.02624671916010564918, -0.6046776061558809534, -0.2411417322834644161 ) ) ;
#17214=CARTESIAN_POINT ( 'NONE',  ( -0.6364829396325453192, -0.2845877964562159024, 0.3641732283464567677 ) ) ;
#17215=CARTESIAN_POINT ( 'NONE',  ( -0.9973753280839886548, -0.6046776061558809534, -0.2411417322834644161 ) ) ;
#17220=CARTESIAN_POINT ( 'NONE',  ( 1.220472440944882608, 0.2952755905511811885, 0.000000000000000000 ) ) ;
#17221=CARTESIAN_POINT ( 'NONE',  ( 0.3280839895013130669, 0.05413385826771666132, 0.4176697321401328100 ) ) ;
#17222=CARTESIAN_POINT ( 'NONE',  ( 0.5052493438320218022, -0.6692913385826773087, -0.1292274648535924053 ) ) ;
#17223=CARTESIAN_POINT ( 'NONE',  ( -0.4593175853018364174, -0.3690944881889765550, -0.3153832671262227771 ) ) ;
#17224=CARTESIAN_POINT ( 'NONE',  ( -0.4461942257217840213, 0.2306618581243848609, 0.2411417322834645549 ) ) ;
#17227=CARTESIAN_POINT ( 'NONE',  ( -0.8398950131233589023, -0.6046776061558809534, -0.2411417322834644161 ) ) ;
#17230=CARTESIAN_POINT ( 'NONE',  ( 1.417322834645670104, -0.1870078740157479769, 0.3641732283464567677 ) ) ;
#17231=CARTESIAN_POINT ( 'NONE',  ( -0.1574803149606292529, -0.1870078740157479769, 0.3641732283464567677 ) ) ;
#17232=CARTESIAN_POINT ( 'NONE',  ( 1.187664041994751285, -0.08942795157527998196, 0.3641732283464567121 ) ) ;
#17233=CARTESIAN_POINT ( 'NONE',  ( 1.614173228346457378, 0.1771653543307087630, 0.000000000000000000 ) ) ;
#17234=CARTESIAN_POINT ( 'NONE',  ( -1.181102362204723644, -0.1870078740157479769, 0.3641732283464567677 ) ) ;
#17235=DIRECTION ( 'NONE',  ( 0.000000000000000000, 0.000000000000000000, 1.000000000000000000 ) ) ;
#17236=CARTESIAN_POINT ( 'NONE',  ( -1.049868766404198794, 0.2306618581243847221, -0.2411417322834647770 ) ) ;
#17237=CARTESIAN_POINT ( 'NONE',  ( -0.4068241469816264999, -0.4281496062992124485, 0.4176697321401328655 ) ) ;
#17241=CARTESIAN_POINT ( 'NONE',  ( -0.1115485564304453947, -0.5511811023622046335, 0.09757992244046803654 ) ) ;
#17242=CARTESIAN_POINT ( 'NONE',  ( -1.666666666666665853, -0.004921259842519870586, -0.3153832671262229437 ) ) ;
#17243=CARTESIAN_POINT ( 'NONE',  ( 0.6102362204724416372, 0.1660481256975883668, -0.3530559997133364547 ) ) ;
#17245=CARTESIAN_POINT ( 'NONE',  ( 1.574803149606299746, -0.1870078740157479769, 0.3641732283464567677 ) ) ;
#17246=CARTESIAN_POINT ( 'NONE',  ( -1.089238845144356427, 0.05413385826771666132, 0.4176697321401328100 ) ) ;
#17247=CARTESIAN_POINT ( 'NONE',  ( -0.2493438320209966919, -0.3690944881889763329, 0.3153832671262228327 ) ) ;
#17249=CARTESIAN_POINT ( 'NONE',  ( 0.1443569553805781891, -0.3690944881889763329, 0.3153832671262228327 ) ) ;
#17251=CARTESIAN_POINT ( 'NONE',  ( -0.2690288713910754526, -0.6692913385826771977, 0.1292274648535927661 ) ) ;
#17254=CARTESIAN_POINT ( 'NONE',  ( 0.7545931758530188826, -0.5511811023622046335, 0.09757992244046803654 ) ) ;
#17255=CARTESIAN_POINT ( 'NONE',  ( 0.09186351706036827158, 0.05413385826771666132, 0.4176697321401328100 ) ) ;
#17256=CARTESIAN_POINT ( 'NONE',  ( -0.5774278215223089816, -0.6046776061558807314, 0.2411417322834647770 ) ) ;
#17257=CARTESIAN_POINT ( 'NONE',  ( -0.8267716535433065062, 0.1771653543307087630, 0.000000000000000000 ) ) ;
#17258=CARTESIAN_POINT ( 'NONE',  ( 0.9645669291338589968, 0.1012011053420777407, 0.2882089793578257453 ) ) ;
#17259=CARTESIAN_POINT ( 'NONE',  ( -0.3674540682414689785, 0.1283753931104748280, 0.1820866141732283561 ) ) ;
#17260=CARTESIAN_POINT ( 'NONE',  ( -0.1771653543307080136, 0.1660481256975883668, -0.3530559997133364547 ) ) ;
#17261=CARTESIAN_POINT ( 'NONE',  ( -1.207349081364828880, 0.1283753931104746893, -0.1820866141732285504 ) ) ;
#17263=CARTESIAN_POINT ( 'NONE',  ( -1.450131233595799651, 0.2952755905511810774, -0.1292274648535930714 ) ) ;
#17266=CARTESIAN_POINT ( 'NONE',  ( -1.358267716535432434, 0.07958543189024071263, -0.2665933059059888421 ) ) ;
#17267=CARTESIAN_POINT ( 'NONE',  ( -0.3477690288713905509, -0.6692913385826771977, 0.1292274648535927661 ) ) ;
#17269=CARTESIAN_POINT ( 'NONE',  ( -1.030183727034119867, -0.3162353388693405765, 0.4822834645669290543 ) ) ;
#17272=CARTESIAN_POINT ( 'NONE',  ( 1.555118110236221041, 0.1660481256975883668, -0.3530559997133364547 ) ) ;
#17273=CARTESIAN_POINT ( 'NONE',  ( 0.3149606299212606708, -0.1870078740157480879, -0.4822834645669291653 ) ) ;
#17276=CARTESIAN_POINT ( 'NONE',  ( 1.535433070866142335, -0.5511811023622047445, 6.969142054262312111E-17 ) ) ;
#17278=ORIENTED_EDGE ( 'NONE', *, *, #53641, .F. ) ;
#17279=CARTESIAN_POINT ( 'NONE',  ( -0.7808398950131222316, -0.2845877964562161244, -0.3641732283464567121 ) ) ;
#17282=CARTESIAN_POINT ( 'NONE',  ( 0.2887139107611556010, -0.6046776061558807314, 0.2411417322834647770 ) ) ;
#17283=CARTESIAN_POINT ( 'NONE',  ( -0.5774278215223089816, 0.2306618581243847221, -0.2411417322834647770 ) ) ;
#17284=CARTESIAN_POINT ( 'NONE',  ( -1.213910761154854745, -0.6692913385826771977, 0.1292274648535927661 ) ) ;
#17285=CARTESIAN_POINT ( 'NONE',  ( 1.246719160104987623, 0.05413385826771626580, -0.4176697321401330321 ) ) ;
#17286=CARTESIAN_POINT ( 'NONE',  ( -1.345144356955379816, -0.2845877964562159024, 0.3641732283464567677 ) ) ;
#17288=CARTESIAN_POINT ( 'NONE',  ( -0.05249343832020911260, 0.2306618581243848609, 0.2411417322834645549 ) ) ;
#17289=CARTESIAN_POINT ( 'NONE',  ( -1.128608923884513837, 0.2306618581243847221, -0.2411417322834647770 ) ) ;
#17291=CARTESIAN_POINT ( 'NONE',  ( -1.646051170424378096, -0.1870078740157480046, 1.254653134982923898E-17 ) ) ;
#17292=CYLINDRICAL_SURFACE ( 'NONE', #34528, 1.181102362204724310 ) ;
#17293=EDGE_CURVE ( 'NONE', #10560, #71339, #72038, .T. ) ;
#17295=CARTESIAN_POINT ( 'NONE',  ( 0.8858267716535438430, 0.07958543189024085140, 0.2665933059059887866 ) ) ;
#17298=CARTESIAN_POINT ( 'NONE',  ( -1.003937007874014853, 0.1660481256975885056, 0.3530559997133364547 ) ) ;
#17299=VERTEX_POINT ( 'NONE', #38632 ) ;
#17300=CARTESIAN_POINT ( 'NONE',  ( -0.1574803149606292529, -0.1870078740157479769, 0.3641732283464567677 ) ) ;
#17301=CARTESIAN_POINT ( 'NONE',  ( -1.725721784776902190, -0.05778040916215522460, 0.4822834645669289988 ) ) ;
#17302=CARTESIAN_POINT ( 'NONE',  ( 0.4527559055118117182, -0.5400638737290844871, 0.3530559997133364547 ) ) ;
#17303=CARTESIAN_POINT ( 'NONE',  ( 0.6167979002624678353, -0.4281496062992124485, 0.4176697321401328655 ) ) ;
#17304=CARTESIAN_POINT ( 'NONE',  ( -0.1640419947506555343, -0.3162353388693405765, 0.4822834645669290543 ) ) ;
#17306=CARTESIAN_POINT ( 'NONE',  ( -0.6430446194225712953, 0.05413385826771626580, -0.4176697321401330321 ) ) ;
#17308=CARTESIAN_POINT ( 'NONE',  ( 1.122047244094488860, 0.07958543189024085140, 0.2665933059059887866 ) ) ;
#17309=CARTESIAN_POINT ( 'NONE',  ( -0.9383202099737524282, -0.3162353388693409650, -0.4822834645669289433 ) ) ;
#17310=CARTESIAN_POINT ( 'NONE',  ( 0.8464566929133866546, -0.5400638737290844871, 0.3530559997133364547 ) ) ;
#17311=CARTESIAN_POINT ( 'NONE',  ( 1.089238845144357759, 0.05413385826771626580, -0.4176697321401330321 ) ) ;
#17313=CARTESIAN_POINT ( 'NONE',  ( -0.9383202099737524282, -0.05778040916215522460, 0.4822834645669289988 ) ) ;
#17315=CARTESIAN_POINT ( 'NONE',  ( 0.3740157480314966754, 0.1660481256975883668, -0.3530559997133364547 ) ) ;
#17317=CARTESIAN_POINT ( 'NONE',  ( -0.5971128608923877978, -0.6692913385826773087, -0.1292274648535924053 ) ) ;
#17318=CARTESIAN_POINT ( 'NONE',  ( -1.568241469816272105, -0.2845877964562161244, -0.3641732283464567121 ) ) ;
#17319=CARTESIAN_POINT ( 'NONE',  ( 0.4855643044619430415, -0.3690944881889765550, -0.3153832671262227771 ) ) ;
#17320=CARTESIAN_POINT ( 'NONE',  ( 0.8267716535433077274, 0.2952755905511811885, 0.000000000000000000 ) ) ;
#17322=CARTESIAN_POINT ( 'NONE',  ( 0.7874015748031503170, -0.1870078740157480601, -0.3641732283464567677 ) ) ;
#17323=CARTESIAN_POINT ( 'NONE',  ( 0.7808398950131240079, -0.3162353388693405765, 0.4822834645669290543 ) ) ;
#17325=CARTESIAN_POINT ( 'NONE',  ( -0.5971128608923877978, 0.2952755905511811885, 0.1292274648535926551 ) ) ;
#17326=CARTESIAN_POINT ( 'NONE',  ( -0.1706036745406816491, 0.05413385826771626580, -0.4176697321401330321 ) ) ;
#17327=CARTESIAN_POINT ( 'NONE',  ( 0.8202099737532813073, 0.1771653543307087630, 0.09757992244046791164 ) ) ;
#17328=CARTESIAN_POINT ( 'NONE',  ( -0.6430446194225716283, -0.4281496062992124485, 0.4176697321401328655 ) ) ;
#17329=CARTESIAN_POINT ( 'NONE',  ( -0.09186351706036689768, 0.05413385826771626580, -0.4176697321401330321 ) ) ;
#17331=CARTESIAN_POINT ( 'NONE',  ( -0.006561679790025524116, -0.3162353388693405765, 0.4822834645669290543 ) ) ;
#17332=CARTESIAN_POINT ( 'NONE',  ( 0.1771653543307093182, -0.4536011799217368745, -0.2665933059059886201 ) ) ;
#17334=CARTESIAN_POINT ( 'NONE',  ( 0.1706036745406830368, -0.3690944881889765550, -0.3153832671262227771 ) ) ;
#17335=CARTESIAN_POINT ( 'NONE',  ( 0.7414698162729663755, -0.5511811023622048555, -0.09757992244046775898 ) ) ;
#17338=CARTESIAN_POINT ( 'NONE',  ( 0.2099737532808405305, -0.6046776061558807314, 0.2411417322834647770 ) ) ;
#17340=FACE_OUTER_BOUND ( 'NONE', #68334, .T. ) ;
#17342=CARTESIAN_POINT ( 'NONE',  ( -0.3937007874015740483, -0.1870078740157480601, -0.3641732283464567677 ) ) ;
#17343=EDGE_CURVE ( 'NONE', #20923, #9917, #71539, .T. ) ;
#17344=CARTESIAN_POINT ( 'NONE',  ( -0.2493438320209966919, -0.4281496062992124485, 0.4176697321401328655 ) ) ;
#17345=CARTESIAN_POINT ( 'NONE',  ( 1.102362204724410155, -0.1870078740157480601, -0.3641732283464567677 ) ) ;
#17347=CARTESIAN_POINT ( 'NONE',  ( -1.325459317585300889, -0.4281496062992127816, -0.4176697321401328100 ) ) ;
#17349=CARTESIAN_POINT ( 'NONE',  ( 0.1706036745406830368, -0.4281496062992127816, -0.4176697321401328100 ) ) ;
#17350=CARTESIAN_POINT ( 'NONE',  ( 1.286089238845145033, -0.6046776061558809534, -0.2411417322834644161 ) ) ;
#17352=CARTESIAN_POINT ( 'NONE',  ( 0.09186351706036799403, -0.4281496062992127816, -0.4176697321401328100 ) ) ;
#17353=CARTESIAN_POINT ( 'NONE',  ( 1.266404199475066328, -0.3162353388693409650, -0.4822834645669289433 ) ) ;
#17354=CARTESIAN_POINT ( 'NONE',  ( 0.4461942257217856311, 0.2306618581243847221, -0.2411417322834647770 ) ) ;
#17355=CARTESIAN_POINT ( 'NONE',  ( -1.603475055217291612, 1.330568129716839909, -0.04573490813648262154 ) ) ;
#17356=CARTESIAN_POINT ( 'NONE',  ( 0.8202099737532814183, -0.5511811023622048555, -0.09757992244046775898 ) ) ;
#17357=CARTESIAN_POINT ( 'NONE',  ( 1.115485564304462551, -0.4281496062992127816, -0.4176697321401328100 ) ) ;
#17358=CARTESIAN_POINT ( 'NONE',  ( 0.2296587926509192634, -0.08942795157528024563, -0.3641732283464568787 ) ) ;
#17359=CARTESIAN_POINT ( 'NONE',  ( -0.3346456692913377662, 0.1660481256975883668, -0.3530559997133364547 ) ) ;
#17360=CARTESIAN_POINT ( 'NONE',  ( 0.7677165354330716118, -0.5400638737290844871, 0.3530559997133364547 ) ) ;
#17361=CARTESIAN_POINT ( 'NONE',  ( -0.6233595800524928121, -0.3162353388693409650, -0.4822834645669289433 ) ) ;
#17363=CARTESIAN_POINT ( 'NONE',  ( -0.08530183727034056085, -0.08942795157528024563, -0.3641732283464568787 ) ) ;
#17364=CARTESIAN_POINT ( 'NONE',  ( 0.6955380577427828781, 0.05413385826771626580, -0.4176697321401330321 ) ) ;
#17365=CARTESIAN_POINT ( 'NONE',  ( 1.003937007874016407, -0.4536011799217367080, 0.2665933059059888421 ) ) ;
#17366=CARTESIAN_POINT ( 'NONE',  ( 0.02624671916010564918, -0.6046776061558809534, -0.2411417322834644161 ) ) ;
#17367=DIRECTION ( 'NONE',  ( -0.000000000000000000, 1.000000000000000000, -0.000000000000000000 ) ) ;
#17369=CARTESIAN_POINT ( 'NONE',  ( 1.574803149606299746, -0.1870078740157479769, 0.4822834645669291653 ) ) ;
#17371=CARTESIAN_POINT ( 'NONE',  ( -1.430446194225720724, 0.05413385826771626580, -0.4176697321401330321 ) ) ;
#17372=CARTESIAN_POINT ( 'NONE',  ( -0.3412073490813641308, -0.6046776061558807314, 0.2411417322834647770 ) ) ;
#17376=CARTESIAN_POINT ( 'NONE',  ( 0.2296587926509192634, -0.2845877964562159024, 0.3641732283464567677 ) ) ;
#17378=CARTESIAN_POINT ( 'NONE',  ( 0.8923884514435701520, -0.6046776061558809534, -0.2411417322834644161 ) ) ;
#17380=CARTESIAN_POINT ( 'NONE',  ( 0.9580052493438326877, 0.05413385826771666132, 0.4176697321401328100 ) ) ;
#17381=CARTESIAN_POINT ( 'NONE',  ( -1.653543307086613234, -0.1870078740157480601, -0.3641732283464567677 ) ) ;
#17382=CARTESIAN_POINT ( 'NONE',  ( 1.167979002624672580, -0.4281496062992124485, 0.4176697321401328655 ) ) ;
#17383=CARTESIAN_POINT ( 'NONE',  ( 1.515748031496063186, -0.4536011799217368745, -0.2665933059059886201 ) ) ;
#17384=CARTESIAN_POINT ( 'NONE',  ( 0.3871391076115493490, -0.3162353388693405765, 0.4822834645669290543 ) ) ;
#17386=CARTESIAN_POINT ( 'NONE',  ( -0.3018372703412066094, -0.4281496062992127816, -0.4176697321401328100 ) ) ;
#17387=CARTESIAN_POINT ( 'NONE',  ( -1.036745406824146176, -0.004921259842519870586, -0.3153832671262229437 ) ) ;
#17388=CARTESIAN_POINT ( 'NONE',  ( 0.2559055118110243332, -0.5400638737290845981, -0.3530559997133363437 ) ) ;
#17389=CARTESIAN_POINT ( 'NONE',  ( 0.07874015748031558404, -0.1870078740157480879, -0.4822834645669291653 ) ) ;
#17391=CARTESIAN_POINT ( 'NONE',  ( 0.6418543022643073970, 2.377811541467197069E-16, 0.3627985898453514602 ) ) ;
#17393=CARTESIAN_POINT ( 'NONE',  ( 0.5905511811023629321, 0.2952755905511811885, 0.000000000000000000 ) ) ;
#17394=CARTESIAN_POINT ( 'NONE',  ( -0.4002624671916004129, -0.05778040916215560624, -0.4822834645669293319 ) ) ;
#17395=CARTESIAN_POINT ( 'NONE',  ( -1.410761154855641575, -0.3162353388693409650, -0.4822834645669289433 ) ) ;
#17396=VECTOR ( 'NONE', #66165, 39.37007874015748143 ) ;
#17397=CARTESIAN_POINT ( 'NONE',  ( 1.246719160104987623, -0.4281496062992124485, 0.4176697321401328655 ) ) ;
#17398=CARTESIAN_POINT ( 'NONE',  ( 0.3149606299212606708, -0.1870078740157480879, -0.4822834645669291653 ) ) ;
#17400=CARTESIAN_POINT ( 'NONE',  ( -0.9186351706036736120, 0.2306618581243848609, 0.2411417322834645549 ) ) ;
#17401=CARTESIAN_POINT ( 'NONE',  ( 0.03280839895013198948, -0.6692913385826773087, -0.1292274648535924053 ) ) ;
#17402=CARTESIAN_POINT ( 'NONE',  ( -0.3937007874015740483, -0.1870078740157479769, 0.4822834645669291653 ) ) ;
#17403=CARTESIAN_POINT ( 'NONE',  ( 0.1837270341207357105, -0.5023911411419708095, -0.1820866141732282451 ) ) ;
#17404=CARTESIAN_POINT ( 'NONE',  ( 1.581364829396326277, -0.2845877964562161244, -0.3641732283464567121 ) ) ;
#17406=CARTESIAN_POINT ( 'NONE',  ( 0.1968503937007881344, 0.2952755905511811885, 0.000000000000000000 ) ) ;
#17408=CARTESIAN_POINT ( 'NONE',  ( -1.581364829396324945, -0.05778040916215560624, -0.4822834645669293319 ) ) ;
#17410=EDGE_LOOP ( 'NONE', ( #8296, #46770, #252, #19312 ) ) ;
#17412=CARTESIAN_POINT ( 'NONE',  ( 0.8530183727034128527, -0.4281496062992124485, 0.4176697321401328655 ) ) ;
#17413=CARTESIAN_POINT ( 'NONE',  ( 0.006561679790026889343, -0.08942795157527998196, 0.3641732283464567121 ) ) ;
#17419=CARTESIAN_POINT ( 'NONE',  ( 0.5708661417322841158, -0.5400638737290845981, -0.3530559997133363437 ) ) ;
#17420=CARTESIAN_POINT ( 'NONE',  ( -0.7283464566929126471, -0.5400638737290844871, 0.3530559997133364547 ) ) ;
#17421=CARTESIAN_POINT ( 'NONE',  ( -0.8070866141732276899, -0.5400638737290844871, 0.3530559997133364547 ) ) ;
#17422=CARTESIAN_POINT ( 'NONE',  ( 0.6233595800524939223, -0.3162353388693405765, 0.4822834645669290543 ) ) ;
#17423=CARTESIAN_POINT ( 'NONE',  ( 1.476377952755906220, 0.1660481256975883668, -0.3530559997133364547 ) ) ;
#17424=CARTESIAN_POINT ( 'NONE',  ( 1.437007874015748810, -0.4536011799217368745, -0.2665933059059886201 ) ) ;
#17425=CARTESIAN_POINT ( 'NONE',  ( 1.430446194225722500, -0.3690944881889765550, -0.3153832671262227771 ) ) ;
#17426=CARTESIAN_POINT ( 'NONE',  ( -0.6955380577427815458, 0.05413385826771666132, 0.4176697321401328100 ) ) ;
#17428=CARTESIAN_POINT ( 'NONE',  ( 1.437007874015748810, -0.5400638737290845981, -0.3530559997133363437 ) ) ;
#17430=CARTESIAN_POINT ( 'NONE',  ( -0.04593175853018302557, 0.2952755905511811885, 0.1292274648535926551 ) ) ;
#17431=CARTESIAN_POINT ( 'NONE',  ( 0.9842519685039378130, -0.6692913385826771977, 8.415575281601705876E-17 ) ) ;
#17433=CARTESIAN_POINT ( 'NONE',  ( -1.312335958005248715, -0.5023911411419708095, -0.1820866141732282451 ) ) ;
#17434=CARTESIAN_POINT ( 'NONE',  ( 0.4133858267716541968, 0.1660481256975885056, 0.3530559997133364547 ) ) ;
#17435=CARTESIAN_POINT ( 'NONE',  ( 0.9842519685039375910, 0.1771653543307087630, 0.000000000000000000 ) ) ;
#17436=EDGE_CURVE ( 'NONE', #59949, #49068, #45766, .T. ) ;
#17438=CARTESIAN_POINT ( 'NONE',  ( -1.259842519685038686, -0.1870078740157479769, 0.3641732283464567677 ) ) ;
#17439=CARTESIAN_POINT ( 'NONE',  ( 1.233595800524935227, 0.2306618581243847221, -0.2411417322834647770 ) ) ;
#17441=CARTESIAN_POINT ( 'NONE',  ( -0.6758530183727028406, -0.5511811023622048555, -0.09757992244046775898 ) ) ;
#17442=CARTESIAN_POINT ( 'NONE',  ( -0.1771653543307080136, -0.5400638737290844871, 0.3530559997133364547 ) ) ;
#17443=CARTESIAN_POINT ( 'NONE',  ( -1.207349081364828436, -0.5023911411419708095, 0.1820866141732285504 ) ) ;
#17444=CARTESIAN_POINT ( 'NONE',  ( -0.6692913385826764205, -0.6692913385826771977, 8.415575281601705876E-17 ) ) ;
#17445=CARTESIAN_POINT ( 'NONE',  ( 1.246719160104987623, 0.05413385826771626580, -0.4176697321401330321 ) ) ;
#17447=CARTESIAN_POINT ( 'NONE',  ( -0.9580052493438311334, -0.004921259842519870586, -0.3153832671262229437 ) ) ;
#17449=CARTESIAN_POINT ( 'NONE',  ( 1.555118110236221041, -0.5400638737290844871, 0.3530559997133364547 ) ) ;
#17451=CARTESIAN_POINT ( 'NONE',  ( -1.076115485564303809, 0.2306618581243848609, 0.2411417322834645549 ) ) ;
#17452=CARTESIAN_POINT ( 'NONE',  ( -1.266404199475064773, -0.08942795157528024563, -0.3641732283464568787 ) ) ;
#17453=CARTESIAN_POINT ( 'NONE',  ( -0.4265091863517051496, 0.1771653543307087075, -0.09757992244046823083 ) ) ;
#17454=LINE ( 'NONE', #61212, #44667 ) ;
#17455=CARTESIAN_POINT ( 'NONE',  ( 0.006561679790026889343, -0.3162353388693409650, -0.4822834645669289433 ) ) ;
#17456=CARTESIAN_POINT ( 'NONE',  ( -0.2165354330708654795, 0.07958543189024085140, 0.2665933059059887866 ) ) ;
#17457=CARTESIAN_POINT ( 'NONE',  ( -1.174540682414697335, -0.2845877964562161244, -0.3641732283464567121 ) ) ;
#17458=CARTESIAN_POINT ( 'NONE',  ( -1.614173228346456268, -0.6692913385826771977, 8.415575281601705876E-17 ) ) ;
#17459=CARTESIAN_POINT ( 'NONE',  ( 1.345144356955381593, -0.2845877964562161244, -0.3641732283464567121 ) ) ;
#17460=CARTESIAN_POINT ( 'NONE',  ( 1.049868766404200349, 0.2306618581243848609, 0.2411417322834645549 ) ) ;
#17462=CARTESIAN_POINT ( 'NONE',  ( 0.5052493438320218022, -0.5511811023622048555, -0.09757992244046775898 ) ) ;
#17463=CARTESIAN_POINT ( 'NONE',  ( 1.069553805774278832, 0.2952755905511810774, -0.1292274648535930714 ) ) ;
#17464=CARTESIAN_POINT ( 'NONE',  ( 0.9580052493438326877, -0.004921259842519576551, 0.3153832671262227771 ) ) ;
#17466=CARTESIAN_POINT ( 'NONE',  ( -1.345144356955379816, -0.3162353388693405765, 0.4822834645669290543 ) ) ;
#17467=CARTESIAN_POINT ( 'NONE',  ( -1.010498687664041384, 0.05413385826771666132, 0.4176697321401328100 ) ) ;
#17468=CARTESIAN_POINT ( 'NONE',  ( -0.1181102362204717315, 0.2952755905511811885, 0.000000000000000000 ) ) ;
#17469=CARTESIAN_POINT ( 'NONE',  ( -1.706036745406823485, 0.1283753931104748280, 0.1820866141732283561 ) ) ;
#17471=CARTESIAN_POINT ( 'NONE',  ( 0.2690288713910767848, -0.6692913385826773087, -0.1292274648535924053 ) ) ;
#17472=CARTESIAN_POINT ( 'NONE',  ( 1.325459317585302665, -0.004921259842519870586, -0.3153832671262229437 ) ) ;
#17473=CARTESIAN_POINT ( 'NONE',  ( 0.03280839895013198948, -0.6692913385826773087, -0.1292274648535924053 ) ) ;
#17474=CARTESIAN_POINT ( 'NONE',  ( 0.5905511811023629321, -0.6692913385826771977, 8.415575281601705876E-17 ) ) ;
#17480=CARTESIAN_POINT ( 'NONE',  ( -0.3740157480314953431, -0.4536011799217368745, -0.2665933059059886201 ) ) ;
#17481=CARTESIAN_POINT ( 'NONE',  ( -0.7677165354330699465, 0.1660481256975885056, 0.3530559997133364547 ) ) ;
#17482=CARTESIAN_POINT ( 'NONE',  ( 0.5774278215223103139, -0.6046776061558809534, -0.2411417322834644161 ) ) ;
#17484=CARTESIAN_POINT ( 'NONE',  ( 0.9776902887139113929, -0.6692913385826773087, -0.1292274648535924053 ) ) ;
#17485=CARTESIAN_POINT ( 'NONE',  ( 1.601049868766404982, 0.2306618581243848609, 0.2411417322834645549 ) ) ;
#17486=CARTESIAN_POINT ( 'NONE',  ( 1.312335958005249825, 0.2306618581243847221, -0.2411417322834647770 ) ) ;
#17490=CARTESIAN_POINT ( 'NONE',  ( 1.003937007874016185, 0.1660481256975883668, -0.3530559997133364547 ) ) ;
#17491=CARTESIAN_POINT ( 'NONE',  ( 0.5052493438320215802, 0.2952755905511811885, 0.1292274648535926551 ) ) ;
#17492=CARTESIAN_POINT ( 'NONE',  ( 1.200787401574803681, -0.4536011799217368745, -0.2665933059059886201 ) ) ;
#17493=CARTESIAN_POINT ( 'NONE',  ( 1.660104986876641320, -0.05778040916215522460, 0.4822834645669289988 ) ) ;
#17494=CARTESIAN_POINT ( 'NONE',  ( 1.548556430446194954, -0.6046776061558807314, 0.2411417322834647770 ) ) ;
#17497=CARTESIAN_POINT ( 'NONE',  ( 0.7677165354330716118, 0.1660481256975883668, -0.3530559997133364547 ) ) ;
#17498=CARTESIAN_POINT ( 'NONE',  ( 1.614173228346457378, -0.5511811023622047445, 6.969142054262312111E-17 ) ) ;
#17499=CARTESIAN_POINT ( 'NONE',  ( -0.4265091863517051496, 0.2952755905511810774, -0.1292274648535930714 ) ) ;
#17500=CARTESIAN_POINT ( 'NONE',  ( -0.4068241469816267775, 0.05413385826771626580, -0.4176697321401330321 ) ) ;
#17501=CARTESIAN_POINT ( 'NONE',  ( -1.633858267716534529, 0.1660481256975885056, 0.3530559997133364547 ) ) ;
#17505=CARTESIAN_POINT ( 'NONE',  ( 1.660104986876641320, -0.05778040916215522460, 0.4822834645669289988 ) ) ;
#17508=ORIENTED_EDGE ( 'NONE', *, *, #42986, .F. ) ;
#17510=CARTESIAN_POINT ( 'NONE',  ( 1.364829396325459854, -0.5023911411419708095, -0.1820866141732282451 ) ) ;
#17512=CARTESIAN_POINT ( 'NONE',  ( 1.601049868766404982, -0.5023911411419708095, -0.1820866141732282451 ) ) ;
#17513=CARTESIAN_POINT ( 'NONE',  ( -0.09151288181857039628, 0.004960608223779798542, -0.3437734562760185186 ) ) ;
#17517=CARTESIAN_POINT ( 'NONE',  ( -0.5905511811023613777, -0.5511811023622047445, 6.969142054262312111E-17 ) ) ;
#17518=CARTESIAN_POINT ( 'NONE',  ( -1.286089238845143479, -0.5023911411419708095, 0.1820866141732285504 ) ) ;
#17519=CARTESIAN_POINT ( 'NONE',  ( 0.5446194225721792126, -0.05778040916215560624, -0.4822834645669293319 ) ) ;
#17520=CARTESIAN_POINT ( 'NONE',  ( -1.227034120734907141, -0.6692913385826773087, -0.1292274648535924053 ) ) ;
#17523=CARTESIAN_POINT ( 'NONE',  ( 1.371391076115485719, -0.6692913385826773087, -0.1292274648535924053 ) ) ;
#17528=ADVANCED_FACE ( 'NONE', ( #19270 ), #52498, .F. ) ;
#17530=CARTESIAN_POINT ( 'NONE',  ( -0.6889763779527552368, 0.1660481256975885056, 0.3530559997133364547 ) ) ;
#17531=CARTESIAN_POINT ( 'NONE',  ( 0.8267716535433078384, -0.6692913385826771977, 8.415575281601705876E-17 ) ) ;
#17532=DIRECTION ( 'NONE',  ( 0.000000000000000000, -0.000000000000000000, 1.000000000000000000 ) ) ;
#17533=CARTESIAN_POINT ( 'NONE',  ( 1.437007874015748810, -0.5400638737290845981, -0.3530559997133363437 ) ) ;
#17534=CARTESIAN_POINT ( 'NONE',  ( -1.305774278215222184, -0.6692913385826773087, -0.1292274648535924053 ) ) ;
#17536=CARTESIAN_POINT ( 'NONE',  ( 0.2362204724409456558, -0.1870078740157480601, -0.3641732283464567677 ) ) ;
#17538=CARTESIAN_POINT ( 'NONE',  ( 0.09186351706036827158, -0.004921259842519576551, 0.3153832671262227771 ) ) ;
#17539=CARTESIAN_POINT ( 'NONE',  ( 0.7283464566929140904, -0.4536011799217368745, -0.2665933059059886201 ) ) ;
#17540=CARTESIAN_POINT ( 'NONE',  ( 0.6758530183727039509, 0.2952755905511810774, -0.1292274648535930714 ) ) ;
#17541=CARTESIAN_POINT ( 'NONE',  ( -0.7545931758530176614, -0.5511811023622048555, -0.09757992244046775898 ) ) ;
#17543=CARTESIAN_POINT ( 'NONE',  ( 1.587926509186352142, 0.05413385826771666132, 0.4176697321401328100 ) ) ;
#17544=CARTESIAN_POINT ( 'NONE',  ( -1.161417322834644716, 0.1660481256975885056, 0.3530559997133364547 ) ) ;
#17546=CARTESIAN_POINT ( 'NONE',  ( -0.1312335958005241554, 0.2306618581243848609, 0.2411417322834645549 ) ) ;
#17547=CARTESIAN_POINT ( 'NONE',  ( -0.5183727034120726440, 0.2952755905511811885, 0.1292274648535926551 ) ) ;
#17548=CARTESIAN_POINT ( 'NONE',  ( 1.174540682414699111, -0.2845877964562159024, 0.3641732283464567677 ) ) ;
#17549=CARTESIAN_POINT ( 'NONE',  ( 0.2755905511811031494, -0.5511811023622047445, 6.969142054262312111E-17 ) ) ;
#17550=CARTESIAN_POINT ( 'NONE',  ( -0.01968503937007793844, -0.5400638737290844871, 0.3530559997133364547 ) ) ;
#17551=CARTESIAN_POINT ( 'NONE',  ( -0.9383202099737524282, -0.3162353388693409650, -0.4822834645669289433 ) ) ;
#17554=CARTESIAN_POINT ( 'NONE',  ( 0.01312335958005323398, -0.4281496062992127816, -0.4176697321401328100 ) ) ;
#17557=CARTESIAN_POINT ( 'NONE',  ( 0.9776902887139113929, 0.2952755905511811885, 0.1292274648535926551 ) ) ;
#17558=B_SPLINE_CURVE_WITH_KNOTS ( 'NONE', 3,
 ( #70394, #80274, #48249, #29314 ),
 .UNSPECIFIED., .F., .F.,
 ( 4, 4 ),
 ( 1.734723475976807094E-18, 0.001346657832036806226 ),
 .UNSPECIFIED. ) ;
#17559=CARTESIAN_POINT ( 'NONE',  ( -0.8398950131233589023, -0.5023911411419708095, -0.1820866141732282451 ) ) ;
#17560=CARTESIAN_POINT ( 'NONE',  ( -0.6299212598425188991, -0.1870078740157479769, 0.4822834645669291653 ) ) ;
#17561=CARTESIAN_POINT ( 'NONE',  ( 1.141732283464567788, -0.6692913385826771977, 8.415575281601705876E-17 ) ) ;
#17562=CARTESIAN_POINT ( 'NONE',  ( 0.8070866141732289112, -0.5400638737290845981, -0.3530559997133363437 ) ) ;
#17563=CARTESIAN_POINT ( 'NONE',  ( -1.541994750656167090, -0.6692913385826773087, -0.1292274648535924053 ) ) ;
#17564=CARTESIAN_POINT ( 'NONE',  ( -0.9842519685039365918, -0.5511811023622047445, 6.969142054262312111E-17 ) ) ;
#17569=CARTESIAN_POINT ( 'NONE',  ( 0.6430446194225728496, -0.004921259842519576551, 0.3153832671262227771 ) ) ;
#17570=CARTESIAN_POINT ( 'NONE',  ( 0.5380577427821529035, 0.05413385826771626580, -0.4176697321401330321 ) ) ;
#17573=CARTESIAN_POINT ( 'NONE',  ( 0.7020997375328090762, -0.2845877964562159024, 0.3641732283464567677 ) ) ;
#17574=CARTESIAN_POINT ( 'NONE',  ( -0.4921259842519677963, 0.1660481256975883668, -0.3530559997133364547 ) ) ;
#17575=CARTESIAN_POINT ( 'NONE',  ( -0.7545931758530176614, -0.6692913385826773087, -0.1292274648535924053 ) ) ;
#17576=CARTESIAN_POINT ( 'NONE',  ( 1.148293963254593875, -0.6692913385826771977, 0.1292274648535927661 ) ) ;
#17579=CARTESIAN_POINT ( 'NONE',  ( -0.2493438320209966919, -0.004921259842519870586, -0.3153832671262229437 ) ) ;
#17584=CARTESIAN_POINT ( 'NONE',  ( -0.8267716535433065062, -0.6692913385826771977, 8.415575281601705876E-17 ) ) ;
#17585=CARTESIAN_POINT ( 'NONE',  ( -0.1902887139107604098, 0.2952755905511810774, -0.1292274648535930714 ) ) ;
#17586=CARTESIAN_POINT ( 'NONE',  ( -0.3674540682414689785, 0.2306618581243848609, 0.2411417322834645549 ) ) ;
#17587=CARTESIAN_POINT ( 'NONE',  ( 0.3346456692913393205, -0.5400638737290845981, -0.3530559997133363437 ) ) ;
#17588=CARTESIAN_POINT ( 'NONE',  ( -0.4396325459317577122, -0.6692913385826773087, -0.1292274648535924053 ) ) ;
#17589=CARTESIAN_POINT ( 'NONE',  ( -1.227034120734907141, -0.6692913385826773087, -0.1292274648535924053 ) ) ;
#17591=CARTESIAN_POINT ( 'NONE',  ( -0.6167979002624665030, 0.05413385826771666132, 0.4176697321401328100 ) ) ;
#17592=CARTESIAN_POINT ( 'NONE',  ( 0.9383202099737536495, -0.3162353388693405765, 0.4822834645669290543 ) ) ;
#17593=CARTESIAN_POINT ( 'NONE',  ( 0.6299212598425204535, -0.1870078740157479769, 0.4822834645669291653 ) ) ;
#17595=CARTESIAN_POINT ( 'NONE',  ( -0.5577427821522301654, -0.2845877964562159024, 0.3641732283464567677 ) ) ;
#17596=VERTEX_POINT ( 'NONE', #25165 ) ;
#17598=ORIENTED_EDGE ( 'NONE', *, *, #18267, .F. ) ;
#17599=CARTESIAN_POINT ( 'NONE',  ( -1.318897637795274802, -0.4536011799217368745, -0.2665933059059886201 ) ) ;
#17600=CARTESIAN_POINT ( 'NONE',  ( -1.069553805774277722, -0.6692913385826773087, -0.1292274648535924053 ) ) ;
#17601=CARTESIAN_POINT ( 'NONE',  ( -0.3871391076115476282, -0.05778040916215522460, 0.4822834645669289988 ) ) ;
#17603=CARTESIAN_POINT ( 'NONE',  ( -0.8136482939632537770, -0.6046776061558807314, 0.2411417322834647770 ) ) ;
#17604=CARTESIAN_POINT ( 'NONE',  ( -1.017060367454067249, -0.3162353388693409650, -0.4822834645669289433 ) ) ;
#17605=DIRECTION ( 'NONE',  ( -3.096699300667737957E-16, 1.000000000000000000, -0.000000000000000000 ) ) ;
#17607=CARTESIAN_POINT ( 'NONE',  ( 0.7874015748031503170, -0.1870078740157480601, -0.3641732283464567677 ) ) ;
#17610=CARTESIAN_POINT ( 'NONE',  ( -0.02624671916010428221, -0.5023911411419708095, 0.1820866141732285504 ) ) ;
#17611=CARTESIAN_POINT ( 'NONE',  ( -0.4527559055118102749, -0.5400638737290845981, -0.3530559997133363437 ) ) ;
#17613=CARTESIAN_POINT ( 'NONE',  ( 0.05249343832021075018, -0.6046776061558807314, 0.2411417322834647770 ) ) ;
#17620=CARTESIAN_POINT ( 'NONE',  ( -0.7217847769028863381, -0.004921259842519870586, -0.3153832671262229437 ) ) ;
#17621=CARTESIAN_POINT ( 'NONE',  ( -0.8595800524934373854, -0.3162353388693409650, -0.4822834645669289433 ) ) ;
#17625=CARTESIAN_POINT ( 'NONE',  ( 1.496062992125985147, -0.1870078740157479769, 0.4822834645669291653 ) ) ;
#17626=CARTESIAN_POINT ( 'NONE',  ( 0.2624671916010504757, -0.6046776061558809534, -0.2411417322834644161 ) ) ;
#17627=CARTESIAN_POINT ( 'NONE',  ( 0.4002624671916016896, -0.05778040916215522460, 0.4822834645669289988 ) ) ;
#17628=CARTESIAN_POINT ( 'NONE',  ( -0.8136482939632537770, 0.1283753931104746893, -0.1820866141732285504 ) ) ;
#17629=CARTESIAN_POINT ( 'NONE',  ( -0.2362204724409442680, -0.1870078740157480879, -0.4822834645669291653 ) ) ;
#17631=CARTESIAN_POINT ( 'NONE',  ( -1.056430446194224881, 0.2952755905511810774, -0.1292274648535930714 ) ) ;
#17633=CARTESIAN_POINT ( 'NONE',  ( 1.200787401574803681, -0.4536011799217368745, -0.2665933059059886201 ) ) ;
#17634=CARTESIAN_POINT ( 'NONE',  ( -0.2952755905511804668, 0.07958543189024085140, 0.2665933059059887866 ) ) ;
#17635=CARTESIAN_POINT ( 'NONE',  ( 0.9842519685039378130, -0.5511811023622047445, 6.969142054262312111E-17 ) ) ;
#17636=CARTESIAN_POINT ( 'NONE',  ( -1.417322834645668772, -0.1870078740157479769, 0.4822834645669291653 ) ) ;
#17637=VECTOR ( 'NONE', #78588, 39.37007874015748143 ) ;
#17638=CARTESIAN_POINT ( 'NONE',  ( -1.023622047244093558, -0.1870078740157479769, 0.3641732283464567677 ) ) ;
#17640=CARTESIAN_POINT ( 'NONE',  ( 0.5971128608923891301, 0.1771653543307087075, -0.09757992244046823083 ) ) ;
#17641=CARTESIAN_POINT ( 'NONE',  ( -0.4855643044619415427, 0.05413385826771626580, -0.4176697321401330321 ) ) ;
#17643=CARTESIAN_POINT ( 'NONE',  ( -0.01312335958005186876, -0.004921259842519870586, -0.3153832671262229437 ) ) ;
#17645=CARTESIAN_POINT ( 'NONE',  ( 0.5774278215223104249, 0.2306618581243848609, 0.2411417322834645549 ) ) ;
#17647=CARTESIAN_POINT ( 'NONE',  ( 1.528871391076116026, -0.5511811023622048555, -0.09757992244046775898 ) ) ;
#17648=CARTESIAN_POINT ( 'NONE',  ( -0.9908136482939626788, -0.6692913385826773087, -0.1292274648535924053 ) ) ;
#17649=CARTESIAN_POINT ( 'NONE',  ( -0.2099737532808391705, 0.1283753931104748280, 0.1820866141732283561 ) ) ;
#17650=CARTESIAN_POINT ( 'NONE',  ( 1.036041590146032698, 3.421639014772782816E-16, 0.3464511005275203726 ) ) ;
#17651=CARTESIAN_POINT ( 'NONE',  ( 0.1181102362204730916, -0.5511811023622047445, 6.969142054262312111E-17 ) ) ;
#17654=CARTESIAN_POINT ( 'NONE',  ( -0.3674540682414689785, 0.2306618581243848609, 0.2411417322834645549 ) ) ;
#17658=CARTESIAN_POINT ( 'NONE',  ( 0.8070866141732288002, 0.07958543189024085140, 0.2665933059059887866 ) ) ;
#17659=CARTESIAN_POINT ( 'NONE',  ( -0.4068241469816264999, -0.4281496062992124485, 0.4176697321401328655 ) ) ;
#17660=CARTESIAN_POINT ( 'NONE',  ( -0.9120734908136475250, -0.6692913385826773087, -0.1292274648535924053 ) ) ;
#17661=CARTESIAN_POINT ( 'NONE',  ( -0.8923884514435688198, -0.5023911411419708095, 0.1820866141732285504 ) ) ;
#17663=CARTESIAN_POINT ( 'NONE',  ( -0.1115485564304453947, -0.6692913385826771977, 0.1292274648535927661 ) ) ;
#17664=CARTESIAN_POINT ( 'NONE',  ( -1.187664041994750175, -0.08942795157528024563, -0.3641732283464568787 ) ) ;
#17665=CARTESIAN_POINT ( 'NONE',  ( -1.522309711286088607, -0.6046776061558807314, 0.2411417322834647770 ) ) ;
#17668=CARTESIAN_POINT ( 'NONE',  ( -1.568241469816272105, -0.08942795157527998196, 0.3641732283464567121 ) ) ;
#17669=CARTESIAN_POINT ( 'NONE',  ( -1.246719160104986512, 0.05413385826771666132, 0.4176697321401328100 ) ) ;
#17670=CARTESIAN_POINT ( 'NONE',  ( -0.9055118110236215490, 0.2952755905511811885, 0.000000000000000000 ) ) ;
#17671=CARTESIAN_POINT ( 'NONE',  ( 1.568241469816273437, -0.3162353388693405765, 0.4822834645669290543 ) ) ;
#17675=CARTESIAN_POINT ( 'NONE',  ( 0.7939632545931766261, -0.3162353388693409650, -0.4822834645669289433 ) ) ;
#17676=CARTESIAN_POINT ( 'NONE',  ( 0.2755905511811031494, 0.2952755905511811885, 0.000000000000000000 ) ) ;
#17679=CARTESIAN_POINT ( 'NONE',  ( 1.345144356955381593, -0.2845877964562161244, -0.3641732283464567121 ) ) ;
#17681=ORIENTED_EDGE ( 'NONE', *, *, #39809, .F. ) ;
#17682=CARTESIAN_POINT ( 'NONE',  ( -0.9645669291338575535, 0.07958543189024071263, -0.2665933059059888421 ) ) ;
#17685=CARTESIAN_POINT ( 'NONE',  ( 0.4461942257217855201, -0.6046776061558807314, 0.2411417322834647770 ) ) ;
#17686=CARTESIAN_POINT ( 'NONE',  ( -0.2296587926509179312, -0.3162353388693409650, -0.4822834645669289433 ) ) ;
#17687=CARTESIAN_POINT ( 'NONE',  ( -1.030183727034119867, -0.3162353388693405765, 0.4822834645669290543 ) ) ;
#17688=CARTESIAN_POINT ( 'NONE',  ( 1.135170603674541256, -0.6692913385826773087, -0.1292274648535924053 ) ) ;
#17689=CARTESIAN_POINT ( 'NONE',  ( 1.555118110236221041, 0.1660481256975883668, -0.3530559997133364547 ) ) ;
#17691=CARTESIAN_POINT ( 'NONE',  ( -0.1181102362204717315, -0.6692913385826771977, 8.415575281601705876E-17 ) ) ;
#17693=CARTESIAN_POINT ( 'NONE',  ( -1.220472440944881054, -0.6692913385826771977, 8.415575281601705876E-17 ) ) ;
#17694=DIRECTION ( 'NONE',  ( 1.000000000000000000, -0.000000000000000000, -0.000000000000000000 ) ) ;
#17697=CARTESIAN_POINT ( 'NONE',  ( 0.9973753280839902091, -0.5023911411419708095, 0.1820866141732285504 ) ) ;
#17698=ORIENTED_EDGE ( 'NONE', *, *, #74163, .T. ) ;
#17700=CARTESIAN_POINT ( 'NONE',  ( -0.9317585301837263412, -0.4281496062992127816, -0.4176697321401328100 ) ) ;
#17702=CARTESIAN_POINT ( 'NONE',  ( 0.1443569553805781891, -0.3690944881889763329, 0.3153832671262228327 ) ) ;
#17703=CARTESIAN_POINT ( 'NONE',  ( -1.548556430446193399, 0.2306618581243848609, 0.2411417322834645549 ) ) ;
#17704=CARTESIAN_POINT ( 'NONE',  ( 0.3740157480314966754, 0.1660481256975883668, -0.3530559997133364547 ) ) ;
#17705=CARTESIAN_POINT ( 'NONE',  ( 0.5774278215223103139, -0.6046776061558809534, -0.2411417322834644161 ) ) ;
#17706=CARTESIAN_POINT ( 'NONE',  ( -0.6430446194225716283, -0.4281496062992124485, 0.4176697321401328655 ) ) ;
#17708=CARTESIAN_POINT ( 'NONE',  ( -1.115485564304461219, 0.05413385826771626580, -0.4176697321401330321 ) ) ;
#17710=CARTESIAN_POINT ( 'NONE',  ( 1.108923884514436242, -0.08942795157527998196, 0.3641732283464567121 ) ) ;
#17711=CARTESIAN_POINT ( 'NONE',  ( -1.049868766404198794, -0.6046776061558807314, 0.2411417322834647770 ) ) ;
#17712=CARTESIAN_POINT ( 'NONE',  ( 1.082677165354331228, 0.1660481256975883668, -0.3530559997133364547 ) ) ;
#17713=CARTESIAN_POINT ( 'NONE',  ( 1.351706036745407680, 0.05413385826771666132, 0.4176697321401328100 ) ) ;
#17715=CARTESIAN_POINT ( 'NONE',  ( -1.541994750656167090, 0.2952755905511811885, 0.1292274648535926551 ) ) ;
#17717=CARTESIAN_POINT ( 'NONE',  ( 0.2952755905511816326, -0.5400638737290844871, 0.3530559997133364547 ) ) ;
#17722=CARTESIAN_POINT ( 'NONE',  ( -1.601049868766403650, 0.1283753931104746893, -0.1820866141732285504 ) ) ;
#17723=CARTESIAN_POINT ( 'NONE',  ( 0.6824146981627303710, -0.5023911411419708095, 0.1820866141732285504 ) ) ;
#17724=CARTESIAN_POINT ( 'NONE',  ( 0.8727034120734912248, -0.3162353388693409650, -0.4822834645669289433 ) ) ;
#17726=CARTESIAN_POINT ( 'NONE',  ( 0.8989501312335964611, 0.1771653543307087630, 0.09757992244046791164 ) ) ;
#17727=CARTESIAN_POINT ( 'NONE',  ( 0.4593175853018379162, -0.4281496062992124485, 0.4176697321401328655 ) ) ;
#17729=CARTESIAN_POINT ( 'NONE',  ( -0.9514435695538050464, -0.3162353388693405765, 0.4822834645669290543 ) ) ;
#17731=CARTESIAN_POINT ( 'NONE',  ( 0.9383202099737536495, -0.2845877964562159024, 0.3641732283464567677 ) ) ;
#17732=CARTESIAN_POINT ( 'NONE',  ( -0.1312335958005241554, 0.2306618581243848609, 0.2411417322834645549 ) ) ;
#17734=CARTESIAN_POINT ( 'NONE',  ( -0.3215223097112853146, -0.3162353388693405765, 0.4822834645669290543 ) ) ;
#17735=CARTESIAN_POINT ( 'NONE',  ( -0.05249343832020911260, 0.1283753931104748280, 0.1820866141732283561 ) ) ;
#17737=CARTESIAN_POINT ( 'NONE',  ( -0.1902887139107604098, -0.6692913385826771977, 0.1292274648535927661 ) ) ;
#17738=CARTESIAN_POINT ( 'NONE',  ( 0.8464566929133865436, 0.07958543189024071263, -0.2665933059059888421 ) ) ;
#17739=LINE ( 'NONE', #43368, #62645 ) ;
#17740=EDGE_CURVE ( 'NONE', #11614, #30580, #77437, .T. ) ;
#17742=CARTESIAN_POINT ( 'NONE',  ( 0.5446194225721792126, -0.3162353388693405765, 0.4822834645669290543 ) ) ;
#17744=CARTESIAN_POINT ( 'NONE',  ( 1.174540682414699111, -0.2845877964562159024, 0.3641732283464567677 ) ) ;
#17745=CARTESIAN_POINT ( 'NONE',  ( 0.4827800718432856963, 2.459406111854941508E-15, 0.4281989832122449768 ) ) ;
#17746=CARTESIAN_POINT ( 'NONE',  ( -0.5839895013123351797, 0.1771653543307087075, -0.09757992244046823083 ) ) ;
#17747=CARTESIAN_POINT ( 'NONE',  ( -0.9055118110236215490, 0.1771653543307087630, 0.000000000000000000 ) ) ;
#17748=CARTESIAN_POINT ( 'NONE',  ( -0.4593175853018364174, -0.4281496062992127816, -0.4176697321401328100 ) ) ;
#17749=CARTESIAN_POINT ( 'NONE',  ( 1.056430446194226658, 0.1771653543307087630, 0.09757992244046791164 ) ) ;
#17750=CARTESIAN_POINT ( 'NONE',  ( -1.725721784776902190, -0.08942795157527998196, 0.3641732283464567121 ) ) ;
#17751=CARTESIAN_POINT ( 'NONE',  ( 1.614173228346457378, 0.1771653543307087630, 0.000000000000000000 ) ) ;
#17752=CARTESIAN_POINT ( 'NONE',  ( 0.3018372703412079971, 0.05413385826771626580, -0.4176697321401330321 ) ) ;
#17753=CARTESIAN_POINT ( 'NONE',  ( 1.161417322834646493, -0.5400638737290844871, 0.3530559997133364547 ) ) ;
#17755=CARTESIAN_POINT ( 'NONE',  ( 0.1181102362204730916, -0.6692913385826771977, 8.415575281601705876E-17 ) ) ;
#17757=CARTESIAN_POINT ( 'NONE',  ( 0.6955380577427828781, -0.4281496062992124485, 0.4176697321401328655 ) ) ;
#17758=CARTESIAN_POINT ( 'NONE',  ( 0.5118110236220480003, -0.6692913385826771977, 8.415575281601705876E-17 ) ) ;
#17760=CARTESIAN_POINT ( 'NONE',  ( 0.3215223097112867578, -0.2845877964562161244, -0.3641732283464567121 ) ) ;
#17761=CARTESIAN_POINT ( 'NONE',  ( 1.253280839895013710, -0.05778040916215560624, -0.4822834645669293319 ) ) ;
#17762=CARTESIAN_POINT ( 'NONE',  ( 0.1115485564304467270, -0.5511811023622048555, -0.09757992244046775898 ) ) ;
#17763=CARTESIAN_POINT ( 'NONE',  ( -0.3805774278215216522, 0.05413385826771666132, 0.4176697321401328100 ) ) ;
#17764=CARTESIAN_POINT ( 'NONE',  ( 0.1377952755905518800, -0.5400638737290844871, 0.3530559997133364547 ) ) ;
#17765=CARTESIAN_POINT ( 'NONE',  ( -0.7742782152230962556, -0.4281496062992127816, -0.4176697321401328100 ) ) ;
#17766=CARTESIAN_POINT ( 'NONE',  ( -0.4527559055118102749, 0.07958543189024085140, 0.2665933059059887866 ) ) ;
#17767=CARTESIAN_POINT ( 'NONE',  ( 0.9908136482939640111, 0.2952755905511810774, -0.1292274648535930714 ) ) ;
#17768=CARTESIAN_POINT ( 'NONE',  ( 1.010498687664042716, -0.3690944881889763329, 0.3153832671262228327 ) ) ;
#17769=CARTESIAN_POINT ( 'NONE',  ( 0.2099737532808405305, -0.6046776061558807314, 0.2411417322834647770 ) ) ;
#17771=CARTESIAN_POINT ( 'NONE',  ( 1.587926509186352142, 0.05413385826771666132, 0.4176697321401328100 ) ) ;
#17774=CARTESIAN_POINT ( 'NONE',  ( -1.292650918635170010, 0.2952755905511810774, -0.1292274648535930714 ) ) ;
#17775=CARTESIAN_POINT ( 'NONE',  ( -0.7808398950131225646, -0.05778040916215522460, 0.4822834645669289988 ) ) ;
#17779=CARTESIAN_POINT ( 'NONE',  ( 0.2952755905511819101, 0.07958543189024071263, -0.2665933059059888421 ) ) ;
#17781=CARTESIAN_POINT ( 'NONE',  ( 0.4986876640419954376, 0.2306618581243848609, 0.2411417322834645549 ) ) ;
#17783=CARTESIAN_POINT ( 'NONE',  ( 0.9973753280839902091, 0.2306618581243847221, -0.2411417322834647770 ) ) ;
#17785=CARTESIAN_POINT ( 'NONE',  ( 1.200787401574803681, 0.1660481256975885056, 0.3530559997133364547 ) ) ;
#17786=CARTESIAN_POINT ( 'NONE',  ( 1.410761154855643795, -0.2845877964562159024, 0.3641732283464567677 ) ) ;
#17787=CARTESIAN_POINT ( 'NONE',  ( 8.195543980992789655E-16, -0.1870078740157480879, -0.4822834645669291653 ) ) ;
#17789=CARTESIAN_POINT ( 'NONE',  ( -0.3083989501312330295, -0.3162353388693409650, -0.4822834645669289433 ) ) ;
#17790=CARTESIAN_POINT ( 'NONE',  ( -0.8464566929133852113, -0.4536011799217368745, -0.2665933059059886201 ) ) ;
#17791=CARTESIAN_POINT ( 'NONE',  ( 0.2821522309711292364, -0.6692913385826771977, 0.1292274648535927661 ) ) ;
#17792=CARTESIAN_POINT ( 'NONE',  ( -0.5905511811023615998, 0.2952755905511811885, 0.000000000000000000 ) ) ;
#17797=CARTESIAN_POINT ( 'NONE',  ( 0.4855643044619430415, -0.4281496062992127816, -0.4176697321401328100 ) ) ;
#17798=CARTESIAN_POINT ( 'NONE',  ( -0.5052493438320203589, -0.6692913385826771977, 0.1292274648535927661 ) ) ;
#17799=CARTESIAN_POINT ( 'NONE',  ( -1.522309711286088607, -0.6046776061558807314, 0.2411417322834647770 ) ) ;
#17800=EDGE_CURVE ( 'NONE', #59008, #81558, #66142, .T. ) ;
#17801=CARTESIAN_POINT ( 'NONE',  ( 0.6496062992125991586, 0.1660481256975885056, 0.3530559997133364547 ) ) ;
#17802=CARTESIAN_POINT ( 'NONE',  ( 0.6299212598425204535, -0.1870078740157480879, -0.4822834645669291653 ) ) ;
#17804=CARTESIAN_POINT ( 'NONE',  ( -0.8530183727034112984, -0.4281496062992127816, -0.4176697321401328100 ) ) ;
#17805=CARTESIAN_POINT ( 'NONE',  ( 0.1968503937007881344, -0.6692913385826771977, 8.415575281601705876E-17 ) ) ;
#17806=CARTESIAN_POINT ( 'NONE',  ( -0.4527559055118102749, -0.5400638737290845981, -0.3530559997133363437 ) ) ;
#17807=EDGE_CURVE ( 'NONE', #59927, #74430, #15792, .T. ) ;
#17808=CARTESIAN_POINT ( 'NONE',  ( 0.3543307086614181922, -0.5511811023622047445, 6.969142054262312111E-17 ) ) ;
#17809=CARTESIAN_POINT ( 'NONE',  ( 1.660104986876641320, -0.08942795157527998196, 0.3641732283464567121 ) ) ;
#17811=CARTESIAN_POINT ( 'NONE',  ( -0.1443569553805768291, 0.05413385826771666132, 0.4176697321401328100 ) ) ;
#17814=CARTESIAN_POINT ( 'NONE',  ( -1.627296587926508442, 0.2306618581243848609, 0.2411417322834645549 ) ) ;
#17816=ORIENTED_EDGE ( 'NONE', *, *, #10592, .F. ) ;
#17818=CARTESIAN_POINT ( 'NONE',  ( 0.4986876640419954376, -0.6046776061558809534, -0.2411417322834644161 ) ) ;
#17819=CARTESIAN_POINT ( 'NONE',  ( 0.05905511811023681640, 0.07958543189024071263, -0.2665933059059888421 ) ) ;
#17824=CARTESIAN_POINT ( 'NONE',  ( 0.3030275874994733387, -1.017388752436352087E-17, -0.3627985898453451874 ) ) ;
#17826=CARTESIAN_POINT ( 'NONE',  ( 0.3674540682414705883, 0.2306618581243847221, -0.2411417322834647770 ) ) ;
#17827=CARTESIAN_POINT ( 'NONE',  ( -1.043307086614172041, -0.5400638737290844871, 0.3530559997133364547 ) ) ;
#17828=CARTESIAN_POINT ( 'NONE',  ( -1.364829396325458521, 0.2306618581243847221, -0.2411417322834647770 ) ) ;
#17829=CARTESIAN_POINT ( 'NONE',  ( 0.7808398950131240079, -0.3162353388693405765, 0.4822834645669290543 ) ) ;
#17830=CARTESIAN_POINT ( 'NONE',  ( 0.7414698162729663755, -0.6692913385826773087, -0.1292274648535924053 ) ) ;
#17831=CARTESIAN_POINT ( 'NONE',  ( 1.279527559055118724, -0.4536011799217368745, -0.2665933059059886201 ) ) ;
#17832=CARTESIAN_POINT ( 'NONE',  ( 1.391076115485564868, 0.1283753931104746893, -0.1820866141732285504 ) ) ;
#17833=CARTESIAN_POINT ( 'NONE',  ( -0.9514435695538050464, -0.05778040916215560624, -0.4822834645669293319 ) ) ;
#17835=CARTESIAN_POINT ( 'NONE',  ( 1.666666666666667185, 0.05413385826771666132, 0.4176697321401328100 ) ) ;
#17837=CARTESIAN_POINT ( 'NONE',  ( -0.1246719160104980823, -0.6692913385826773087, -0.1292274648535924053 ) ) ;
#17838=CARTESIAN_POINT ( 'NONE',  ( 1.338582677165355062, -0.1870078740157479769, 0.4822834645669291653 ) ) ;
#17839=CARTESIAN_POINT ( 'NONE',  ( 0.4606732211678797317, 2.401574803149606030, -0.5309055118110237448 ) ) ;
#17840=CARTESIAN_POINT ( 'NONE',  ( -1.469816272965878357, -0.5023911411419708095, -0.1820866141732282451 ) ) ;
#17841=CARTESIAN_POINT ( 'NONE',  ( 0.4068241469816281097, 0.05413385826771666132, 0.4176697321401328100 ) ) ;
#17842=CARTESIAN_POINT ( 'NONE',  ( 0.9383202099737536495, -0.2845877964562159024, 0.3641732283464567677 ) ) ;
#17844=CARTESIAN_POINT ( 'NONE',  ( -1.325459317585300889, -0.3690944881889765550, -0.3153832671262227771 ) ) ;
#17845=CARTESIAN_POINT ( 'NONE',  ( 1.115485564304462551, -0.4281496062992127816, -0.4176697321401328100 ) ) ;
#17846=CARTESIAN_POINT ( 'NONE',  ( -0.5249343832020990641, 0.2306618581243848609, 0.2411417322834645549 ) ) ;
#17847=CARTESIAN_POINT ( 'NONE',  ( -0.6167979002624665030, -0.004921259842519576551, 0.3153832671262227771 ) ) ;
#17848=CARTESIAN_POINT ( 'NONE',  ( -0.6692913385826764205, -0.6692913385826771977, 8.415575281601705876E-17 ) ) ;
#17849=CARTESIAN_POINT ( 'NONE',  ( 1.476377952755906442, -0.5400638737290844871, 0.3530559997133364547 ) ) ;
#17850=CARTESIAN_POINT ( 'NONE',  ( -0.5380577427821514602, -0.4281496062992127816, -0.4176697321401328100 ) ) ;
#17851=CARTESIAN_POINT ( 'NONE',  ( 1.410761154855643795, -0.05778040916215560624, -0.4822834645669293319 ) ) ;
#17853=CARTESIAN_POINT ( 'NONE',  ( -1.102362204724408601, -0.1870078740157480601, -0.3641732283464567677 ) ) ;
#17855=CARTESIAN_POINT ( 'NONE',  ( 1.364829396325459854, -0.6046776061558809534, -0.2411417322834644161 ) ) ;
#17857=CARTESIAN_POINT ( 'NONE',  ( -1.082677165354329896, 0.1660481256975885056, 0.3530559997133364547 ) ) ;
#17858=CARTESIAN_POINT ( 'NONE',  ( -1.614173228346455824, 0.1771653543307087630, 0.000000000000000000 ) ) ;
#17859=CARTESIAN_POINT ( 'NONE',  ( -0.5183727034120726440, -0.5511811023622048555, -0.09757992244046775898 ) ) ;
#17860=CARTESIAN_POINT ( 'NONE',  ( -1.640419947506561060, 0.05413385826771666132, 0.4176697321401328100 ) ) ;
#17861=CARTESIAN_POINT ( 'NONE',  ( -0.2690288713910754526, -0.6692913385826771977, 0.1292274648535927661 ) ) ;
#17862=CARTESIAN_POINT ( 'NONE',  ( -0.07217847769028787330, -0.08942795157527998196, 0.3641732283464567121 ) ) ;
#17863=CARTESIAN_POINT ( 'NONE',  ( -1.082677165354329896, 0.07958543189024085140, 0.2665933059059887866 ) ) ;
#17864=CARTESIAN_POINT ( 'NONE',  ( 1.561679790026247350, -0.3690944881889763329, 0.3153832671262228327 ) ) ;
#17866=CARTESIAN_POINT ( 'NONE',  ( 0.8530183727034128527, -0.4281496062992124485, 0.4176697321401328655 ) ) ;
#17868=CARTESIAN_POINT ( 'NONE',  ( 0.3608923884514443348, -0.5511811023622046335, 0.09757992244046803654 ) ) ;
#17869=CARTESIAN_POINT ( 'NONE',  ( 0.2690288713910767848, 0.2952755905511811885, 0.1292274648535926551 ) ) ;
#17870=CARTESIAN_POINT ( 'NONE',  ( 1.089238845144357537, -0.3690944881889763329, 0.3153832671262228327 ) ) ;
#17872=CARTESIAN_POINT ( 'NONE',  ( -1.233595800524933894, -0.6046776061558809534, -0.2411417322834644161 ) ) ;
#17873=CARTESIAN_POINT ( 'NONE',  ( -1.515748031496062076, -0.5400638737290844871, 0.3530559997133364547 ) ) ;
#17874=CARTESIAN_POINT ( 'NONE',  ( -0.08530183727034056085, -0.05778040916215560624, -0.4822834645669293319 ) ) ;
#17877=CARTESIAN_POINT ( 'NONE',  ( 0.5249343832021003964, 0.2306618581243847221, -0.2411417322834647770 ) ) ;
#17878=CARTESIAN_POINT ( 'NONE',  ( 1.456692913385827515, 0.1771653543307087630, 0.000000000000000000 ) ) ;
#17879=CARTESIAN_POINT ( 'NONE',  ( -0.1377952755905504645, -0.5400638737290845981, -0.3530559997133363437 ) ) ;
#17880=CARTESIAN_POINT ( 'NONE',  ( 0.9842519685039375910, 0.2952755905511811885, 0.000000000000000000 ) ) ;
#17886=CARTESIAN_POINT ( 'NONE',  ( -0.7283464566929126471, 0.07958543189024071263, -0.2665933059059888421 ) ) ;
#17887=CARTESIAN_POINT ( 'NONE',  ( -0.6364829396325453192, -0.3162353388693405765, 0.4822834645669290543 ) ) ;
#17888=CARTESIAN_POINT ( 'NONE',  ( 0.5183727034120741983, 0.2952755905511810774, -0.1292274648535930714 ) ) ;
#17890=CARTESIAN_POINT ( 'NONE',  ( 1.023622047244095334, -0.1870078740157479769, 0.4822834645669291653 ) ) ;
#17891=CARTESIAN_POINT ( 'NONE',  ( -1.397637795275589623, -0.5400638737290845981, -0.3530559997133363437 ) ) ;
#17892=CARTESIAN_POINT ( 'NONE',  ( 0.8530183727034126306, 0.05413385826771626580, -0.4176697321401330321 ) ) ;
#17893=FACE_OUTER_BOUND ( 'NONE', #83208, .T. ) ;
#17895=CARTESIAN_POINT ( 'NONE',  ( 1.482939632545932307, -0.4281496062992124485, 0.4176697321401328655 ) ) ;
#17896=CARTESIAN_POINT ( 'NONE',  ( 0.9973753280839902091, 0.2306618581243847221, -0.2411417322834647770 ) ) ;
#17898=CARTESIAN_POINT ( 'NONE',  ( 0.5905511811023629321, -0.6692913385826771977, 8.415575281601705876E-17 ) ) ;
#17899=CARTESIAN_POINT ( 'NONE',  ( 1.187664041994751285, -0.2845877964562161244, -0.3641732283464567121 ) ) ;
#17900=CARTESIAN_POINT ( 'NONE',  ( -1.607611548556429737, 0.1771653543307087075, -0.09757992244046823083 ) ) ;
#17901=CARTESIAN_POINT ( 'NONE',  ( -1.430446194225720724, 0.05413385826771626580, -0.4176697321401330321 ) ) ;
#17904=CARTESIAN_POINT ( 'NONE',  ( 0.9186351706036752773, 0.2306618581243847221, -0.2411417322834647770 ) ) ;
#17906=CARTESIAN_POINT ( 'NONE',  ( 1.653543307086614789, -0.1870078740157479769, 0.3641732283464567677 ) ) ;
#17907=CARTESIAN_POINT ( 'NONE',  ( -0.2952755905511804668, 0.1660481256975885056, 0.3530559997133364547 ) ) ;
#17908=CARTESIAN_POINT ( 'NONE',  ( -0.8070866141732276899, -0.5400638737290844871, 0.3530559997133364547 ) ) ;
#17909=CARTESIAN_POINT ( 'NONE',  ( -1.482939632545930975, 0.05413385826771666132, 0.4176697321401328100 ) ) ;
#17913=CARTESIAN_POINT ( 'NONE',  ( 1.686351706036745890, 0.2952755905511811885, 0.1292274648535926551 ) ) ;
#17917=CARTESIAN_POINT ( 'NONE',  ( -0.01277272433825534827, 0.004960608223779807216, -0.3437734562760184631 ) ) ;
#17918=CARTESIAN_POINT ( 'NONE',  ( 1.535433070866142335, -0.5511811023622047445, 6.969142054262312111E-17 ) ) ;
#17925=CARTESIAN_POINT ( 'NONE',  ( -0.8923884514435688198, -0.5023911411419708095, 0.1820866141732285504 ) ) ;
#17926=CARTESIAN_POINT ( 'NONE',  ( -1.108923884514435132, -0.2845877964562159024, 0.3641732283464567677 ) ) ;
#17927=CARTESIAN_POINT ( 'NONE',  ( -1.364829396325458521, -0.6046776061558807314, 0.2411417322834647770 ) ) ;
#17928=CARTESIAN_POINT ( 'NONE',  ( 0.01312335958005323398, 0.05413385826771666132, 0.4176697321401328100 ) ) ;
#17929=CARTESIAN_POINT ( 'NONE',  ( -1.384514435695537005, -0.6692913385826773087, -0.1292274648535924053 ) ) ;
#17930=ORIENTED_EDGE ( 'NONE', *, *, #20551, .T. ) ;
#17931=CARTESIAN_POINT ( 'NONE',  ( -1.633858267716534529, 0.1660481256975885056, 0.3530559997133364547 ) ) ;
#17934=PLANE ( 'NONE',  #12973 ) ;
#17935=CARTESIAN_POINT ( 'NONE',  ( -0.6102362204724400829, -0.4536011799217368745, -0.2665933059059886201 ) ) ;
#17936=CARTESIAN_POINT ( 'NONE',  ( -1.095800524934382292, -0.3162353388693409650, -0.4822834645669289433 ) ) ;
#17937=CARTESIAN_POINT ( 'NONE',  ( 1.010498687664042716, -0.4281496062992124485, 0.4176697321401328655 ) ) ;
#17939=CARTESIAN_POINT ( 'NONE',  ( 0.000000000000000000, 0.000000000000000000, 0.000000000000000000 ) ) ;
#17941=CARTESIAN_POINT ( 'NONE',  ( 1.627296587926509996, -0.6046776061558807314, 0.2411417322834647770 ) ) ;
#17942=CARTESIAN_POINT ( 'NONE',  ( -1.391076115485563758, 0.2306618581243848609, 0.2411417322834645549 ) ) ;
#17944=CARTESIAN_POINT ( 'NONE',  ( 0.2034120734908142214, 0.1771653543307087075, -0.09757992244046823083 ) ) ;
#17946=CARTESIAN_POINT ( 'NONE',  ( -0.2230971128608915943, -0.004921259842519576551, 0.3153832671262227771 ) ) ;
#17947=CARTESIAN_POINT ( 'NONE',  ( 0.6036745406824153282, -0.5023911411419708095, 0.1820866141732285504 ) ) ;
#17948=CARTESIAN_POINT ( 'NONE',  ( 0.4921259842519691285, 0.1660481256975885056, 0.3530559997133364547 ) ) ;
#17949=CARTESIAN_POINT ( 'NONE',  ( -0.6561679790026240244, 0.1283753931104746893, -0.1820866141732285504 ) ) ;
#17951=CARTESIAN_POINT ( 'NONE',  ( 1.069553805774278610, -0.6692913385826771977, 0.1292274648535927661 ) ) ;
#17952=CARTESIAN_POINT ( 'NONE',  ( -0.8267716535433065062, 0.2952755905511811885, 0.000000000000000000 ) ) ;
#17954=CARTESIAN_POINT ( 'NONE',  ( 0.01968503937007930540, 0.1660481256975885056, 0.3530559997133364547 ) ) ;
#17955=CARTESIAN_POINT ( 'NONE',  ( -0.5380577427821514602, 0.05413385826771666132, 0.4176697321401328100 ) ) ;
#17956=CARTESIAN_POINT ( 'NONE',  ( 1.246719160104987623, -0.004921259842519870586, -0.3153832671262229437 ) ) ;
#17957=CARTESIAN_POINT ( 'NONE',  ( -0.07874015748031421014, -0.1870078740157480601, -0.3641732283464567677 ) ) ;
#17958=CARTESIAN_POINT ( 'NONE',  ( -0.1115485564304456306, 0.2952755905511810774, -0.1292274648535930714 ) ) ;
#17959=CARTESIAN_POINT ( 'NONE',  ( -1.017060367454067249, -0.05778040916215522460, 0.4822834645669289988 ) ) ;
#17961=CARTESIAN_POINT ( 'NONE',  ( 1.601049868766404982, -0.5023911411419708095, -0.1820866141732282451 ) ) ;
#17963=CARTESIAN_POINT ( 'NONE',  ( -0.1049868766404193215, -0.6046776061558807314, 0.2411417322834647770 ) ) ;
#17966=CARTESIAN_POINT ( 'NONE',  ( 1.174540682414699111, -0.05778040916215560624, -0.4822834645669293319 ) ) ;
#17967=CARTESIAN_POINT ( 'NONE',  ( -0.4527559055118102749, 0.07958543189024085140, 0.2665933059059887866 ) ) ;
#17968=CARTESIAN_POINT ( 'NONE',  ( -0.5052493438320203589, -0.6692913385826771977, 0.1292274648535927661 ) ) ;
#17969=CARTESIAN_POINT ( 'NONE',  ( 1.358267716535433323, 0.1660481256975885056, 0.3530559997133364547 ) ) ;
#17970=CARTESIAN_POINT ( 'NONE',  ( 0.9908136482939640111, -0.6692913385826771977, 0.1292274648535927661 ) ) ;
#17972=CARTESIAN_POINT ( 'NONE',  ( -1.076115485564303809, 0.1283753931104748280, 0.1820866141732283561 ) ) ;
#17978=CARTESIAN_POINT ( 'NONE',  ( 1.233595800524935227, 0.1283753931104746893, -0.1820866141732285504 ) ) ;
#17979=CARTESIAN_POINT ( 'NONE',  ( 0.8136482939632553313, 0.1283753931104748280, 0.1820866141732283561 ) ) ;
#17980=CARTESIAN_POINT ( 'NONE',  ( 0.5643044619422579178, -0.4281496062992127816, -0.4176697321401328100 ) ) ;
#17983=CARTESIAN_POINT ( 'NONE',  ( 0.6496062992125991586, -0.4536011799217368745, -0.2665933059059886201 ) ) ;
#17984=EDGE_CURVE ( 'NONE', #4208, #2914, #3974, .T. ) ;
#17985=CARTESIAN_POINT ( 'NONE',  ( -0.2493438320209966919, -0.4281496062992124485, 0.4176697321401328655 ) ) ;
#17986=CARTESIAN_POINT ( 'NONE',  ( -0.9186351706036736120, -0.6046776061558809534, -0.2411417322834644161 ) ) ;
#17987=CARTESIAN_POINT ( 'NONE',  ( 1.240157480314961314, 0.1660481256975883668, -0.3530559997133364547 ) ) ;
#17990=CARTESIAN_POINT ( 'NONE',  ( 0.05905511811023681640, 0.07958543189024071263, -0.2665933059059888421 ) ) ;
#17993=ORIENTED_EDGE ( 'NONE', *, *, #24157, .F. ) ;
#17994=CARTESIAN_POINT ( 'NONE',  ( -0.8923884514435688198, 0.2306618581243847221, -0.2411417322834647770 ) ) ;
#17995=CARTESIAN_POINT ( 'NONE',  ( -0.3149606299212590610, -0.1870078740157480879, -0.4822834645669291653 ) ) ;
#17996=CARTESIAN_POINT ( 'NONE',  ( -0.3805774278215216522, 0.05413385826771666132, 0.4176697321401328100 ) ) ;
#17998=CARTESIAN_POINT ( 'NONE',  ( 0.5183727034120741983, -0.6692913385826771977, 0.1292274648535927661 ) ) ;
#17999=CARTESIAN_POINT ( 'NONE',  ( -0.4002624671916004129, -0.3162353388693405765, 0.4822834645669290543 ) ) ;
#18000=CARTESIAN_POINT ( 'NONE',  ( -1.489501312335957062, -0.05778040916215522460, 0.4822834645669289988 ) ) ;
#18001=CARTESIAN_POINT ( 'NONE',  ( -0.8989501312335946848, 0.2952755905511810774, -0.1292274648535930714 ) ) ;
#18002=CARTESIAN_POINT ( 'NONE',  ( 0.5708661417322841158, -0.5400638737290845981, -0.3530559997133363437 ) ) ;
#18004=CARTESIAN_POINT ( 'NONE',  ( -0.4068241469816264999, -0.3690944881889763329, 0.3153832671262228327 ) ) ;
#18008=CARTESIAN_POINT ( 'NONE',  ( -1.128608923884513837, -0.5023911411419708095, 0.1820866141732285504 ) ) ;
#18009=CARTESIAN_POINT ( 'NONE',  ( -1.003937007874014853, 0.1660481256975885056, 0.3530559997133364547 ) ) ;
#18010=CARTESIAN_POINT ( 'NONE',  ( -0.7020997375328074108, -0.05778040916215522460, 0.4822834645669289988 ) ) ;
#18012=CARTESIAN_POINT ( 'NONE',  ( -0.6692913385826764205, -0.6692913385826771977, 8.415575281601705876E-17 ) ) ;
#18013=CARTESIAN_POINT ( 'NONE',  ( -0.8989501312335946848, 0.2952755905511810774, -0.1292274648535930714 ) ) ;
#18014=CARTESIAN_POINT ( 'NONE',  ( 1.436417322834644406, 0.8346805926620876059, 0.3149606299212598381 ) ) ;
#18016=CARTESIAN_POINT ( 'NONE',  ( 0.4527559055118117182, 0.07958543189024071263, -0.2665933059059888421 ) ) ;
#18019=CARTESIAN_POINT ( 'NONE',  ( -0.1181102362204717315, 0.1771653543307087630, 0.000000000000000000 ) ) ;
#18021=CARTESIAN_POINT ( 'NONE',  ( -0.1771653543307080136, 0.1660481256975883668, -0.3530559997133364547 ) ) ;
#18022=CARTESIAN_POINT ( 'NONE',  ( 1.601049868766404982, 0.2306618581243848609, 0.2411417322834645549 ) ) ;
#18023=CARTESIAN_POINT ( 'NONE',  ( -0.1771653543307080136, 0.1660481256975883668, -0.3530559997133364547 ) ) ;
#18030=CARTESIAN_POINT ( 'NONE',  ( -0.9842519685039365918, -0.5511811023622047445, 6.969142054262312111E-17 ) ) ;
#18031=CARTESIAN_POINT ( 'NONE',  ( -1.463254593175852492, -0.6692913385826773087, -0.1292274648535924053 ) ) ;
#18033=CARTESIAN_POINT ( 'NONE',  ( -0.7426113562971994320, 2.199547029021313715, 0.5309055118110236338 ) ) ;
#18035=CARTESIAN_POINT ( 'NONE',  ( 1.266404199475066328, -0.3162353388693409650, -0.4822834645669289433 ) ) ;
#18036=CARTESIAN_POINT ( 'NONE',  ( 0.4527559055118117182, -0.5400638737290844871, 0.3530559997133364547 ) ) ;
#18037=CARTESIAN_POINT ( 'NONE',  ( 0.2034120734908144990, -0.6692913385826771977, 0.1292274648535927661 ) ) ;
#18038=CARTESIAN_POINT ( 'NONE',  ( -1.272965879265091305, -0.004921259842519870586, -0.3153832671262229437 ) ) ;
#18039=CARTESIAN_POINT ( 'NONE',  ( -0.2493438320209966919, 0.05413385826771626580, -0.4176697321401330321 ) ) ;
#18041=CARTESIAN_POINT ( 'NONE',  ( -0.9842519685039365918, -0.6692913385826771977, 8.415575281601705876E-17 ) ) ;
#18044=CARTESIAN_POINT ( 'NONE',  ( 1.377952755905512472, -0.5511811023622047445, 6.969142054262312111E-17 ) ) ;
#18045=CARTESIAN_POINT ( 'NONE',  ( -0.1640419947506555343, -0.2845877964562159024, 0.3641732283464567677 ) ) ;
#18046=CARTESIAN_POINT ( 'NONE',  ( 1.345144356955381593, -0.08942795157527998196, 0.3641732283464567121 ) ) ;
#18047=CARTESIAN_POINT ( 'NONE',  ( -1.476377952755905110, -0.5400638737290845981, -0.3530559997133363437 ) ) ;
#18048=CARTESIAN_POINT ( 'NONE',  ( -0.9448818897637790704, -0.1870078740157480601, -0.3641732283464567677 ) ) ;
#18050=CARTESIAN_POINT ( 'NONE',  ( 0.6233595800524942554, -0.08942795157528024563, -0.3641732283464568787 ) ) ;
#18051=CARTESIAN_POINT ( 'NONE',  ( -0.3937007874015740483, -0.1870078740157479769, 0.4822834645669291653 ) ) ;
#18052=CARTESIAN_POINT ( 'NONE',  ( 0.2755905511811031494, 0.2952755905511811885, 0.000000000000000000 ) ) ;
#18053=CARTESIAN_POINT ( 'NONE',  ( -0.02624671916010428221, 0.1283753931104746893, -0.1820866141732285504 ) ) ;
#18055=CARTESIAN_POINT ( 'NONE',  ( 0.8136482939632553313, -0.6046776061558809534, -0.2411417322834644161 ) ) ;
#18057=CARTESIAN_POINT ( 'NONE',  ( 1.227034120734908917, -0.5511811023622046335, 0.09757992244046803654 ) ) ;
#18058=CARTESIAN_POINT ( 'NONE',  ( -1.122047244094487306, -0.5400638737290844871, 0.3530559997133364547 ) ) ;
#18059=CARTESIAN_POINT ( 'NONE',  ( -0.2296587926509179312, -0.08942795157527998196, 0.3641732283464567121 ) ) ;
#18061=CARTESIAN_POINT ( 'NONE',  ( 0.1640419947506569498, -0.08942795157527998196, 0.3641732283464567121 ) ) ;
#18062=CARTESIAN_POINT ( 'NONE',  ( -1.213910761154854745, 0.2952755905511810774, -0.1292274648535930714 ) ) ;
#18063=CARTESIAN_POINT ( 'NONE',  ( -0.3412073490813641308, 0.2306618581243847221, -0.2411417322834647770 ) ) ;
#18066=CARTESIAN_POINT ( 'NONE',  ( 0.6824146981627303710, 0.1283753931104746893, -0.1820866141732285504 ) ) ;
#18067=CARTESIAN_POINT ( 'NONE',  ( -0.3280839895013117347, 0.05413385826771626580, -0.4176697321401330321 ) ) ;
#18068=CARTESIAN_POINT ( 'NONE',  ( -0.6627296587926501115, 0.2952755905511810774, -0.1292274648535930714 ) ) ;
#18069=CARTESIAN_POINT ( 'NONE',  ( -0.9776902887139098386, 0.1771653543307087075, -0.09757992244046823083 ) ) ;
#18071=CARTESIAN_POINT ( 'NONE',  ( -0.1968503937007867743, 0.2952755905511811885, 0.000000000000000000 ) ) ;
#18072=CARTESIAN_POINT ( 'NONE',  ( -1.437007874015747477, -0.4536011799217367080, 0.2665933059059888421 ) ) ;
#18073=CARTESIAN_POINT ( 'NONE',  ( -1.358267716535432434, -0.5400638737290844871, 0.3530559997133364547 ) ) ;
#18077=LINE ( 'NONE', #24777, #6857 ) ;
#18078=CARTESIAN_POINT ( 'NONE',  ( -1.417322834645668772, -0.1870078740157479769, 0.4822834645669291653 ) ) ;
#18079=CARTESIAN_POINT ( 'NONE',  ( -0.8530183727034112984, -0.4281496062992127816, -0.4176697321401328100 ) ) ;
#18080=CARTESIAN_POINT ( 'NONE',  ( -1.646981627296586703, -0.05778040916215522460, 0.4822834645669289988 ) ) ;
#18083=CARTESIAN_POINT ( 'NONE',  ( 1.036745406824147731, 0.05413385826771666132, 0.4176697321401328100 ) ) ;
#18084=CARTESIAN_POINT ( 'NONE',  ( 0.4461942257217856311, 0.2306618581243847221, -0.2411417322834647770 ) ) ;
#18087=CARTESIAN_POINT ( 'NONE',  ( 1.102362204724410155, -0.1870078740157479769, 0.3641732283464567677 ) ) ;
#18090=CONICAL_SURFACE ( 'NONE', #81245, 2.401574803149606918, 0.7125723459225955514 ) ;
#18093=CARTESIAN_POINT ( 'NONE',  ( 0.4265091863517067039, -0.6692913385826773087, -0.1292274648535924053 ) ) ;
#18094=CARTESIAN_POINT ( 'NONE',  ( -0.7545931758530177724, 0.2952755905511811885, 0.1292274648535926551 ) ) ;
#18096=CARTESIAN_POINT ( 'NONE',  ( 1.555118110236221041, -0.5400638737290844871, 0.3530559997133364547 ) ) ;
#18097=CARTESIAN_POINT ( 'NONE',  ( 0.9645669291338591078, -0.5400638737290845981, -0.3530559997133363437 ) ) ;
#18098=CARTESIAN_POINT ( 'NONE',  ( 1.627296587926509996, -0.6046776061558807314, 0.2411417322834647770 ) ) ;
#18099=DIRECTION ( 'NONE',  ( -0.4999999999999955036, -0.7071067811865522357, -0.4999999999999977796 ) ) ;
#18100=CARTESIAN_POINT ( 'NONE',  ( -0.2296587926509179312, -0.05778040916215522460, 0.4822834645669289988 ) ) ;
#18101=CARTESIAN_POINT ( 'NONE',  ( -1.391076115485563314, -0.6046776061558809534, -0.2411417322834644161 ) ) ;
#18102=CARTESIAN_POINT ( 'NONE',  ( -1.574803149606298192, -0.1870078740157480879, -0.4822834645669291653 ) ) ;
#18103=CARTESIAN_POINT ( 'NONE',  ( 1.692913385826772421, 0.2952755905511811885, 0.000000000000000000 ) ) ;
#18105=CARTESIAN_POINT ( 'NONE',  ( 0.8530183727034128527, -0.3690944881889763329, 0.3153832671262228327 ) ) ;
#18106=ORIENTED_EDGE ( 'NONE', *, *, #30053, .F. ) ;
#18109=CARTESIAN_POINT ( 'NONE',  ( -0.1706036745406816491, -0.3690944881889763329, 0.3153832671262228327 ) ) ;
#18110=CARTESIAN_POINT ( 'NONE',  ( -1.633858267716534529, -0.5400638737290845981, -0.3530559997133363437 ) ) ;
#18111=CARTESIAN_POINT ( 'NONE',  ( 0.4855643044619428750, 0.05413385826771666132, 0.4176697321401328100 ) ) ;
#18112=CARTESIAN_POINT ( 'NONE',  ( 0.4461942257217855201, -0.6046776061558807314, 0.2411417322834647770 ) ) ;
#18113=CARTESIAN_POINT ( 'NONE',  ( -0.4068241469816267775, 0.05413385826771626580, -0.4176697321401330321 ) ) ;
#18115=CARTESIAN_POINT ( 'NONE',  ( -1.062992125984250968, -0.6692913385826771977, 8.415575281601705876E-17 ) ) ;
#18117=CARTESIAN_POINT ( 'NONE',  ( 1.404199475065617264, -0.3690944881889763329, 0.3153832671262228327 ) ) ;
#18118=CARTESIAN_POINT ( 'NONE',  ( -0.9055118110236215490, -0.6692913385826771977, 8.415575281601705876E-17 ) ) ;
#18119=CARTESIAN_POINT ( 'NONE',  ( 1.036745406824147731, 0.05413385826771666132, 0.4176697321401328100 ) ) ;
#18120=CARTESIAN_POINT ( 'NONE',  ( 1.141732283464567788, -0.6692913385826771977, 8.415575281601705876E-17 ) ) ;
#18123=CARTESIAN_POINT ( 'NONE',  ( -1.220472440944881054, 0.2952755905511811885, 0.000000000000000000 ) ) ;
#18125=CARTESIAN_POINT ( 'NONE',  ( 0.2362204724409456558, -0.1870078740157480879, -0.4822834645669291653 ) ) ;
#18128=CARTESIAN_POINT ( 'NONE',  ( 1.601049868766404982, -0.6046776061558809534, -0.2411417322834644161 ) ) ;
#18129=CARTESIAN_POINT ( 'NONE',  ( 0.2952755905511819101, 0.07958543189024071263, -0.2665933059059888421 ) ) ;
#18130=CARTESIAN_POINT ( 'NONE',  ( 0.8792650918635177559, -0.4281496062992127816, -0.4176697321401328100 ) ) ;
#18132=CARTESIAN_POINT ( 'NONE',  ( 0.9317585301837276734, -0.004921259842519870586, -0.3153832671262229437 ) ) ;
#18133=CARTESIAN_POINT ( 'NONE',  ( 0.4855643044619428750, 0.05413385826771666132, 0.4176697321401328100 ) ) ;
#18135=CARTESIAN_POINT ( 'NONE',  ( -0.9711286089238838626, -0.6046776061558807314, 0.2411417322834647770 ) ) ;
#18136=CARTESIAN_POINT ( 'NONE',  ( -0.1690661813110308498, 0.02791078216816347476, -0.4328096321851898631 ) ) ;
#18138=CARTESIAN_POINT ( 'NONE',  ( 0.7742782152230978099, -0.3690944881889763329, 0.3153832671262228327 ) ) ;
#18139=CARTESIAN_POINT ( 'NONE',  ( 0.1246719160104994284, 0.2066929133858267098, -0.1054918080437494132 ) ) ;
#18140=CARTESIAN_POINT ( 'NONE',  ( -0.3477690288713905509, -0.6692913385826771977, 0.1292274648535927661 ) ) ;
#18141=CARTESIAN_POINT ( 'NONE',  ( 0.3018372703412079971, -0.004921259842519870586, -0.3153832671262229437 ) ) ;
#18143=CARTESIAN_POINT ( 'NONE',  ( -0.1771653543307080136, -0.5400638737290844871, 0.3530559997133364547 ) ) ;
#18144=CARTESIAN_POINT ( 'NONE',  ( 0.8989501312335963501, -0.5511811023622048555, -0.09757992244046775898 ) ) ;
#18145=CARTESIAN_POINT ( 'NONE',  ( -1.113858370737681902, -4.850200619981615293E-15, -0.3791475997938227316 ) ) ;
#18147=CARTESIAN_POINT ( 'NONE',  ( 0.1574803149606306130, -0.1870078740157480879, -0.4822834645669291653 ) ) ;
#18149=CARTESIAN_POINT ( 'NONE',  ( 1.095800524934383846, -0.08942795157528024563, -0.3641732283464568787 ) ) ;
#18150=CARTESIAN_POINT ( 'NONE',  ( 0.1837270341207354329, 0.2306618581243848609, 0.2411417322834645549 ) ) ;
#18151=CARTESIAN_POINT ( 'NONE',  ( -0.4921259842519677963, -0.4536011799217367080, 0.2665933059059888421 ) ) ;
#18152=CIRCLE ( 'NONE', #7386, 3.543307086614174484 ) ;
#18153=CARTESIAN_POINT ( 'NONE',  ( -0.6364829396325453192, -0.2845877964562159024, 0.3641732283464567677 ) ) ;
#18154=CARTESIAN_POINT ( 'NONE',  ( -0.2034120734908128059, 0.2952755905511811885, 0.1292274648535926551 ) ) ;
#18155=CARTESIAN_POINT ( 'NONE',  ( 0.1574803149606306130, -0.1870078740157479769, 0.4822834645669291653 ) ) ;
#18156=CARTESIAN_POINT ( 'NONE',  ( 0.9514435695538062676, -0.2845877964562161244, -0.3641732283464567121 ) ) ;
#18158=CARTESIAN_POINT ( 'NONE',  ( 1.469816272965879911, 0.1283753931104746893, -0.1820866141732285504 ) ) ;
#18160=CARTESIAN_POINT ( 'NONE',  ( 0.8070866141732289112, -0.5400638737290845981, -0.3530559997133363437 ) ) ;
#18161=CARTESIAN_POINT ( 'NONE',  ( -1.603475055217291612, 1.819038169495759361, 0.04573490813648255215 ) ) ;
#18162=CARTESIAN_POINT ( 'NONE',  ( -0.3871391076115479057, -0.3162353388693409650, -0.4822834645669289433 ) ) ;
#18164=CARTESIAN_POINT ( 'NONE',  ( 0.9317585301837276734, 0.05413385826771626580, -0.4176697321401330321 ) ) ;
#18165=CARTESIAN_POINT ( 'NONE',  ( 0.4068241469816281097, 0.05413385826771666132, 0.4176697321401328100 ) ) ;
#18167=CARTESIAN_POINT ( 'NONE',  ( 0.3674540682414705883, -0.5023911411419708095, 0.1820866141732285504 ) ) ;
#18168=CARTESIAN_POINT ( 'NONE',  ( 1.010498687664042716, -0.4281496062992124485, 0.4176697321401328655 ) ) ;
#18169=CARTESIAN_POINT ( 'NONE',  ( 0.07217847769028949700, -0.08942795157528024563, -0.3641732283464568787 ) ) ;
#18170=CARTESIAN_POINT ( 'NONE',  ( -0.4658792650918627265, -0.3162353388693409650, -0.4822834645669289433 ) ) ;
#18172=CARTESIAN_POINT ( 'NONE',  ( 0.09842519685039434474, -0.5400638737290845981, -0.3530559997133363437 ) ) ;
#18173=CARTESIAN_POINT ( 'NONE',  ( -0.8989501312335946848, -0.6692913385826771977, 0.1292274648535927661 ) ) ;
#18174=CARTESIAN_POINT ( 'NONE',  ( -0.1181102362204717315, 0.1771653543307087630, 0.000000000000000000 ) ) ;
#18175=CARTESIAN_POINT ( 'NONE',  ( 0.3083989501312343062, -0.3162353388693405765, 0.4822834645669290543 ) ) ;
#18176=CARTESIAN_POINT ( 'NONE',  ( 1.076115485564305141, 0.1283753931104746893, -0.1820866141732285504 ) ) ;
#18177=CARTESIAN_POINT ( 'NONE',  ( -0.3543307086614165824, 0.2952755905511811885, 0.000000000000000000 ) ) ;
#18178=CARTESIAN_POINT ( 'NONE',  ( 1.161417322834646271, 0.1012011053420775880, -0.2882089793578257453 ) ) ;
#18179=CARTESIAN_POINT ( 'NONE',  ( -0.3836918680457887532, -2.191421614605370878E-15, 0.4445507791589071167 ) ) ;
#18180=CARTESIAN_POINT ( 'NONE',  ( 1.227034120734908917, -0.6692913385826771977, 0.1292274648535927661 ) ) ;
#18183=CARTESIAN_POINT ( 'NONE',  ( -1.332020997375327642, -0.05778040916215522460, 0.4822834645669289988 ) ) ;
#18184=CARTESIAN_POINT ( 'NONE',  ( -0.9251968503937002541, 0.1660481256975885056, 0.3530559997133364547 ) ) ;
#18187=ORIENTED_EDGE ( 'NONE', *, *, #77172, .T. ) ;
#18188=CARTESIAN_POINT ( 'NONE',  ( 0.4921259842519691285, -0.4536011799217368745, -0.2665933059059886201 ) ) ;
#18190=CARTESIAN_POINT ( 'NONE',  ( 0.7217847769028878924, -0.4281496062992127816, -0.4176697321401328100 ) ) ;
#18193=CARTESIAN_POINT ( 'NONE',  ( -0.4133858267716528645, -0.4536011799217367080, 0.2665933059059888421 ) ) ;
#18195=CARTESIAN_POINT ( 'NONE',  ( 1.056430446194226658, 0.2952755905511811885, 0.1292274648535926551 ) ) ;
#18196=CARTESIAN_POINT ( 'NONE',  ( 1.548556430446194954, -0.5023911411419708095, 0.1820866141732285504 ) ) ;
#18197=CARTESIAN_POINT ( 'NONE',  ( 0.08530183727034192087, -0.05778040916215522460, 0.4822834645669289988 ) ) ;
#18199=CARTESIAN_POINT ( 'NONE',  ( -0.5183727034120726440, 0.2952755905511811885, 0.1292274648535926551 ) ) ;
#18200=CARTESIAN_POINT ( 'NONE',  ( -1.279527559055116948, -0.4536011799217367080, 0.2665933059059888421 ) ) ;
#18201=CARTESIAN_POINT ( 'NONE',  ( -0.4068241469816267775, 0.05413385826771626580, -0.4176697321401330321 ) ) ;
#18206=CARTESIAN_POINT ( 'NONE',  ( 0.3215223097112867578, -0.3162353388693409650, -0.4822834645669289433 ) ) ;
#18207=ORIENTED_EDGE ( 'NONE', *, *, #82686, .F. ) ;
#18209=CARTESIAN_POINT ( 'NONE',  ( -0.5314960629921254842, -0.5400638737290845981, -0.3530559997133363437 ) ) ;
#18210=CARTESIAN_POINT ( 'NONE',  ( -1.469816272965878357, 0.2306618581243848609, 0.2411417322834645549 ) ) ;
#18211=CARTESIAN_POINT ( 'NONE',  ( 0.5839895013123367340, -0.6692913385826773087, -0.1292274648535924053 ) ) ;
#18212=CARTESIAN_POINT ( 'NONE',  ( -0.1181102362204717315, -0.6692913385826771977, 8.415575281601705876E-17 ) ) ;
#18214=CARTESIAN_POINT ( 'NONE',  ( -0.8989501312335946848, 0.2952755905511810774, -0.1292274648535930714 ) ) ;
#18215=CARTESIAN_POINT ( 'NONE',  ( 0.4068241469816281097, 0.05413385826771666132, 0.4176697321401328100 ) ) ;
#18216=CARTESIAN_POINT ( 'NONE',  ( -0.6167979002624665030, -0.4281496062992127816, -0.4176697321401328100 ) ) ;
#18217=CARTESIAN_POINT ( 'NONE',  ( 0.4461942257217856311, 0.1283753931104746893, -0.1820866141732285504 ) ) ;
#18219=CARTESIAN_POINT ( 'NONE',  ( -0.06561679790026180015, -0.4281496062992127816, -0.4176697321401328100 ) ) ;
#18221=CARTESIAN_POINT ( 'NONE',  ( 1.594488188976378673, 0.1660481256975885056, 0.3530559997133364547 ) ) ;
#18224=ORIENTED_EDGE ( 'NONE', *, *, #72350, .F. ) ;
#18225=CARTESIAN_POINT ( 'NONE',  ( 0.9120734908136490793, 0.2952755905511810774, -0.1292274648535930714 ) ) ;
#18226=CARTESIAN_POINT ( 'NONE',  ( 0.2493438320209980519, -0.3690944881889765550, -0.3153832671262227771 ) ) ;
#18231=CARTESIAN_POINT ( 'NONE',  ( 0.7205944486920661252, 7.754911898504981261E-16, 0.3627989612356142257 ) ) ;
#18233=CARTESIAN_POINT ( 'NONE',  ( 0.3608923884514443348, 0.2952755905511810774, -0.1292274648535930714 ) ) ;
#18234=CARTESIAN_POINT ( 'NONE',  ( -1.227034120734907141, -0.6692913385826773087, -0.1292274648535924053 ) ) ;
#18235=CARTESIAN_POINT ( 'NONE',  ( -1.272965879265091305, -0.4281496062992124485, 0.4176697321401328655 ) ) ;
#18236=CARTESIAN_POINT ( 'NONE',  ( 0.4527559055118117182, -0.5400638737290844871, 0.3530559997133364547 ) ) ;
#18237=CARTESIAN_POINT ( 'NONE',  ( 0.9055118110236227702, -0.6692913385826771977, 8.415575281601705876E-17 ) ) ;
#18238=CARTESIAN_POINT ( 'NONE',  ( 1.561679790026247350, -0.004921259842519870586, -0.3153832671262229437 ) ) ;
#18239=CARTESIAN_POINT ( 'NONE',  ( 1.325459317585302665, -0.3690944881889763329, 0.3153832671262228327 ) ) ;
#18240=CARTESIAN_POINT ( 'NONE',  ( -0.8464566929133852113, 0.1660481256975885056, 0.3530559997133364547 ) ) ;
#18242=CARTESIAN_POINT ( 'NONE',  ( -1.601049868766403650, 0.1283753931104746893, -0.1820866141732285504 ) ) ;
#18244=CARTESIAN_POINT ( 'NONE',  ( -0.2165354330708654795, 0.1660481256975885056, 0.3530559997133364547 ) ) ;
#18245=CARTESIAN_POINT ( 'NONE',  ( 0.9514435695538062676, -0.3162353388693409650, -0.4822834645669289433 ) ) ;
#18247=CARTESIAN_POINT ( 'NONE',  ( -1.463254593175852492, -0.5511811023622048555, -0.09757992244046775898 ) ) ;
#18248=CARTESIAN_POINT ( 'NONE',  ( 0.03937007874015833325, -0.6692913385826771977, 8.415575281601705876E-17 ) ) ;
#18249=CARTESIAN_POINT ( 'NONE',  ( 0.6955380577427828781, -0.004921259842519870586, -0.3153832671262229437 ) ) ;
#18250=CARTESIAN_POINT ( 'NONE',  ( -1.601049868766403650, -0.5023911411419708095, 0.1820866141732285504 ) ) ;
#18251=CARTESIAN_POINT ( 'NONE',  ( 1.089238845144357759, 0.05413385826771626580, -0.4176697321401330321 ) ) ;
#18253=CARTESIAN_POINT ( 'NONE',  ( -0.4855643044619415427, -0.3690944881889763329, 0.3153832671262228327 ) ) ;
#18254=CARTESIAN_POINT ( 'NONE',  ( -0.7152230971128602510, -0.05778040916215560624, -0.4822834645669293319 ) ) ;
#18255=CARTESIAN_POINT ( 'NONE',  ( -1.594488188976377119, 0.07958543189024071263, -0.2665933059059888421 ) ) ;
#18256=CARTESIAN_POINT ( 'NONE',  ( -1.141732283464566011, -0.6692913385826771977, 8.415575281601705876E-17 ) ) ;
#18257=CARTESIAN_POINT ( 'NONE',  ( 1.207349081364829990, 0.2306618581243848609, 0.2411417322834645549 ) ) ;
#18259=CARTESIAN_POINT ( 'NONE',  ( -1.312335958005248715, 0.1283753931104748280, 0.1820866141732283561 ) ) ;
#18261=CARTESIAN_POINT ( 'NONE',  ( 1.279527559055118724, 0.1660481256975885056, 0.3530559997133364547 ) ) ;
#18263=AXIS2_PLACEMENT_3D ( 'NONE', #61598, #17002, #3944 ) ;
#18264=CARTESIAN_POINT ( 'NONE',  ( -1.443569553805773564, -0.6046776061558807314, 0.2411417322834647770 ) ) ;
#18265=CARTESIAN_POINT ( 'NONE',  ( -1.489501312335957062, -0.08942795157527998196, 0.3641732283464567121 ) ) ;
#18266=CARTESIAN_POINT ( 'NONE',  ( -1.010498687664041384, -0.3690944881889765550, -0.3153832671262227771 ) ) ;
#18267=EDGE_CURVE ( 'NONE', #60047, #35589, #67954, .T. ) ;
#18269=CARTESIAN_POINT ( 'NONE',  ( -0.3018372703412066094, -0.4281496062992127816, -0.4176697321401328100 ) ) ;
#18270=CARTESIAN_POINT ( 'NONE',  ( -0.01312335958005186876, -0.004921259842519870586, -0.3153832671262229437 ) ) ;
#18271=CARTESIAN_POINT ( 'NONE',  ( -1.233595800524933894, 0.1283753931104748280, 0.1820866141732283561 ) ) ;
#18272=CARTESIAN_POINT ( 'NONE',  ( 1.325459317585302665, -0.004921259842519870586, -0.3153832671262229437 ) ) ;
#18273=CARTESIAN_POINT ( 'NONE',  ( 0.9580052493438327987, -0.4281496062992127816, -0.4176697321401328100 ) ) ;
#18274=FACE_OUTER_BOUND ( 'NONE', #49544, .T. ) ;
#18275=CARTESIAN_POINT ( 'NONE',  ( 0.08530183727034192087, -0.08942795157527998196, 0.3641732283464567121 ) ) ;
#18276=CARTESIAN_POINT ( 'NONE',  ( 0.6102362204724416372, 0.1660481256975883668, -0.3530559997133364547 ) ) ;
#18277=ADVANCED_FACE ( 'NONE', ( #47022 ), #62043, .F. ) ;
#18278=CARTESIAN_POINT ( 'NONE',  ( 0.8727034120734912248, -0.2845877964562161244, -0.3641732283464567121 ) ) ;
#18279=ORIENTED_EDGE ( 'NONE', *, *, #63984, .T. ) ;
#18280=CARTESIAN_POINT ( 'NONE',  ( 1.482939632545932307, 0.05413385826771626580, -0.4176697321401330321 ) ) ;
#18281=CARTESIAN_POINT ( 'NONE',  ( -1.377952755905511140, -0.6692913385826771977, 8.415575281601705876E-17 ) ) ;
#18282=CARTESIAN_POINT ( 'NONE',  ( -0.1574803149606292529, -0.1870078740157479769, 0.4822834645669291653 ) ) ;
#18285=CARTESIAN_POINT ( 'NONE',  ( 0.5971128608923890191, -0.6692913385826771977, 0.1292274648535927661 ) ) ;
#18286=CARTESIAN_POINT ( 'NONE',  ( 1.259842519685040019, -0.1870078740157479769, 0.3641732283464567677 ) ) ;
#18287=CARTESIAN_POINT ( 'NONE',  ( 0.1115485564304470323, 0.2952755905511811885, 0.1292274648535926551 ) ) ;
#18288=CARTESIAN_POINT ( 'NONE',  ( 0.3280839895013130669, 0.05413385826771666132, 0.4176697321401328100 ) ) ;
#18294=CARTESIAN_POINT ( 'NONE',  ( -0.3280839895013117347, -0.3690944881889763329, 0.3153832671262228327 ) ) ;
#18295=CARTESIAN_POINT ( 'NONE',  ( -0.6496062992125976043, -0.5400638737290844871, 0.3530559997133364547 ) ) ;
#18298=CARTESIAN_POINT ( 'NONE',  ( 0.8858267716535438430, 0.1660481256975885056, 0.3530559997133364547 ) ) ;
#18299=CARTESIAN_POINT ( 'NONE',  ( -1.456692913385826182, 0.2952755905511811885, 0.000000000000000000 ) ) ;
#18300=CARTESIAN_POINT ( 'NONE',  ( 0.8005249343832027131, 0.05413385826771666132, 0.4176697321401328100 ) ) ;
#18306=CARTESIAN_POINT ( 'NONE',  ( 0.7152230971128614723, -0.3162353388693409650, -0.4822834645669289433 ) ) ;
#18307=CARTESIAN_POINT ( 'NONE',  ( 0.6496062992125991586, 0.1660481256975885056, 0.3530559997133364547 ) ) ;
#18309=CARTESIAN_POINT ( 'NONE',  ( 1.332020997375328974, -0.08942795157528024563, -0.3641732283464568787 ) ) ;
#18310=CARTESIAN_POINT ( 'NONE',  ( 1.312335958005250269, -0.6046776061558807314, 0.2411417322834647770 ) ) ;
#18312=CARTESIAN_POINT ( 'NONE',  ( 0.9514435695538062676, -0.3162353388693409650, -0.4822834645669289433 ) ) ;
#18313=CARTESIAN_POINT ( 'NONE',  ( 1.437007874015748810, -0.4536011799217368745, -0.2665933059059886201 ) ) ;
#18314=CARTESIAN_POINT ( 'NONE',  ( -0.3018372703412066094, 0.05413385826771666132, 0.4176697321401328100 ) ) ;
#18315=CARTESIAN_POINT ( 'NONE',  ( -0.9055118110236215490, 0.2952755905511811885, 0.000000000000000000 ) ) ;
#18316=CARTESIAN_POINT ( 'NONE',  ( 1.259842519685040019, -0.1870078740157479769, 0.4822834645669291653 ) ) ;
#18321=CARTESIAN_POINT ( 'NONE',  ( -1.522309711286088607, -0.5023911411419708095, 0.1820866141732285504 ) ) ;
#18324=ORIENTED_EDGE ( 'NONE', *, *, #19808, .F. ) ;
#18326=CONICAL_SURFACE ( 'NONE', #19691, 2.362204724409449508, 0.8726646259971704289 ) ;
#18327=CARTESIAN_POINT ( 'NONE',  ( 1.463254593175853824, 0.1771653543307087075, -0.09757992244046823083 ) ) ;
#18329=CARTESIAN_POINT ( 'NONE',  ( 1.509186351706037543, -0.004921259842519576551, 0.3153832671262227771 ) ) ;
#18334=CARTESIAN_POINT ( 'NONE',  ( -0.9251968503937002541, -0.4536011799217368745, -0.2665933059059886201 ) ) ;
#18335=CARTESIAN_POINT ( 'NONE',  ( -1.194225721784776262, -0.004921259842519870586, -0.3153832671262229437 ) ) ;
#18336=CARTESIAN_POINT ( 'NONE',  ( -1.082677165354329896, -0.5400638737290845981, -0.3530559997133363437 ) ) ;
#18337=CARTESIAN_POINT ( 'NONE',  ( 0.2296587926509192634, -0.05778040916215560624, -0.4822834645669293319 ) ) ;
#18338=CARTESIAN_POINT ( 'NONE',  ( 1.614173228346457378, 0.2952755905511811885, 0.000000000000000000 ) ) ;
#18339=VERTEX_POINT ( 'NONE', #10297 ) ;
#18340=CARTESIAN_POINT ( 'NONE',  ( 1.384514435695538337, -0.6692913385826771977, 0.1292274648535927661 ) ) ;
#18341=CARTESIAN_POINT ( 'NONE',  ( -1.115485564304460997, 0.009842519685039147898, -0.3409548833797004797 ) ) ;
#18344=DIRECTION ( 'NONE',  ( -1.000000000000000000, -2.312964634635741971E-16, 0.000000000000000000 ) ) ;
#18345=CARTESIAN_POINT ( 'NONE',  ( -0.5380577427821514602, -0.004921259842519576551, 0.3153832671262227771 ) ) ;
#18346=CARTESIAN_POINT ( 'NONE',  ( -1.286089238845143479, 0.2306618581243847221, -0.2411417322834647770 ) ) ;
#18347=CARTESIAN_POINT ( 'NONE',  ( 0.8464566929133866546, -0.5400638737290844871, 0.3530559997133364547 ) ) ;
#18349=CARTESIAN_POINT ( 'NONE',  ( -1.586052503253847057, 1.574803149606300412, -0.1653254495020572423 ) ) ;
#18350=CARTESIAN_POINT ( 'NONE',  ( 1.614173228346456712, 0.4410134679336843999, 0.1372047244094478646 ) ) ;
#18351=CARTESIAN_POINT ( 'NONE',  ( 1.548556430446194954, 0.2306618581243847221, -0.2411417322834647770 ) ) ;
#18352=CARTESIAN_POINT ( 'NONE',  ( -1.423884514435694859, -0.3162353388693405765, 0.4822834645669290543 ) ) ;
#18354=CARTESIAN_POINT ( 'NONE',  ( -0.3740157480314953431, -0.4536011799217368745, -0.2665933059059886201 ) ) ;
#18356=CARTESIAN_POINT ( 'NONE',  ( -0.6561679790026240244, 0.1283753931104746893, -0.1820866141732285504 ) ) ;
#18357=CARTESIAN_POINT ( 'NONE',  ( 0.4002624671916016896, -0.2845877964562161244, -0.3641732283464567121 ) ) ;
#18358=CARTESIAN_POINT ( 'NONE',  ( 0.05905511811023681640, 0.1660481256975883668, -0.3530559997133364547 ) ) ;
#18359=CARTESIAN_POINT ( 'NONE',  ( -0.8005249343832011588, -0.004921259842519870586, -0.3153832671262229437 ) ) ;
#18361=CARTESIAN_POINT ( 'NONE',  ( 0.9776902887139113929, 0.2952755905511811885, 0.1292274648535926551 ) ) ;
#18363=CARTESIAN_POINT ( 'NONE',  ( -0.9120734908136475250, -0.6692913385826773087, -0.1292274648535924053 ) ) ;
#18367=CARTESIAN_POINT ( 'NONE',  ( -0.5314960629921254842, -0.5400638737290845981, -0.3530559997133363437 ) ) ;
#18369=CARTESIAN_POINT ( 'NONE',  ( -0.9973753280839886548, 0.2306618581243848609, 0.2411417322834645549 ) ) ;
#18370=CARTESIAN_POINT ( 'NONE',  ( 1.253280839895013710, -0.08942795157528024563, -0.3641732283464568787 ) ) ;
#18371=CARTESIAN_POINT ( 'NONE',  ( 0.2034120734908142214, 0.1771653543307087075, -0.09757992244046823083 ) ) ;
#18372=CARTESIAN_POINT ( 'NONE',  ( -0.3937007874015740483, -0.1870078740157480879, -0.4822834645669291653 ) ) ;
#18373=CARTESIAN_POINT ( 'NONE',  ( -1.115485564304461219, 0.05413385826771626580, -0.4176697321401330321 ) ) ;
#18376=CARTESIAN_POINT ( 'NONE',  ( -0.3608923884514428360, 0.2952755905511811885, 0.1292274648535926551 ) ) ;
#18377=CARTESIAN_POINT ( 'NONE',  ( -0.9383202099737524282, -0.05778040916215522460, 0.4822834645669289988 ) ) ;
#18380=CARTESIAN_POINT ( 'NONE',  ( 1.227034120734908917, -0.6692913385826771977, 0.1292274648535927661 ) ) ;
#18381=CARTESIAN_POINT ( 'NONE',  ( -0.7742782152230965886, -0.004921259842519576551, 0.3153832671262227771 ) ) ;
#18382=CARTESIAN_POINT ( 'NONE',  ( -0.9908136482939626788, -0.6692913385826773087, -0.1292274648535924053 ) ) ;
#18383=CARTESIAN_POINT ( 'NONE',  ( 1.115485564304462551, -0.4281496062992127816, -0.4176697321401328100 ) ) ;
#18384=CARTESIAN_POINT ( 'NONE',  ( 0.7480314960629927956, 0.2952755905511811885, 0.000000000000000000 ) ) ;
#18386=CARTESIAN_POINT ( 'NONE',  ( -1.213910761154854745, 0.1771653543307087075, -0.09757992244046823083 ) ) ;
#18391=CARTESIAN_POINT ( 'NONE',  ( 1.213910761154856299, 0.1771653543307087630, 0.09757992244046791164 ) ) ;
#18392=CARTESIAN_POINT ( 'NONE',  ( 0.7349081364829402885, -0.5023911411419708095, -0.1820866141732282451 ) ) ;
#18393=CARTESIAN_POINT ( 'NONE',  ( 0.7217847769028878924, -0.4281496062992127816, -0.4176697321401328100 ) ) ;
#18396=CARTESIAN_POINT ( 'NONE',  ( 0.8136482939632553313, -0.5023911411419708095, -0.1820866141732282451 ) ) ;
#18397=CARTESIAN_POINT ( 'NONE',  ( -0.1312335958005241554, -0.6046776061558809534, -0.2411417322834644161 ) ) ;
#18398=CARTESIAN_POINT ( 'NONE',  ( -1.207349081364828436, -0.6046776061558807314, 0.2411417322834647770 ) ) ;
#18399=CARTESIAN_POINT ( 'NONE',  ( 1.181102362204725198, -0.1870078740157479769, 0.4822834645669291653 ) ) ;
#18401=CARTESIAN_POINT ( 'NONE',  ( -0.7414698162729651543, 0.2952755905511810219, -0.1292274648535930437 ) ) ;
#18402=CARTESIAN_POINT ( 'NONE',  ( 0.07217847769028949700, -0.08942795157528024563, -0.3641732283464568787 ) ) ;
#18405=CARTESIAN_POINT ( 'NONE',  ( -0.7152230971128602510, -0.05778040916215560624, -0.4822834645669293319 ) ) ;
#18406=CARTESIAN_POINT ( 'NONE',  ( -0.5708661417322825615, -0.5400638737290844871, 0.3530559997133364547 ) ) ;
#18407=CARTESIAN_POINT ( 'NONE',  ( -0.6889763779527552368, 0.1660481256975885056, 0.3530559997133364547 ) ) ;
#18408=CARTESIAN_POINT ( 'NONE',  ( 0.4330708661417329575, 0.2952755905511811885, 0.000000000000000000 ) ) ;
#18409=CARTESIAN_POINT ( 'NONE',  ( -0.4199475065616791736, -0.6046776061558807314, 0.2411417322834647770 ) ) ;
#18410=CARTESIAN_POINT ( 'NONE',  ( -1.377952755905511140, -0.6692913385826771977, 8.415575281601705876E-17 ) ) ;
#18411=CARTESIAN_POINT ( 'NONE',  ( -1.017060367454067249, -0.3162353388693409650, -0.4822834645669289433 ) ) ;
#18412=CARTESIAN_POINT ( 'NONE',  ( 0.8989501312335963501, -0.6692913385826773087, -0.1292274648535924053 ) ) ;
#18414=CARTESIAN_POINT ( 'NONE',  ( -0.3674540682414689785, 0.1283753931104748280, 0.1820866141732283561 ) ) ;
#18419=CARTESIAN_POINT ( 'NONE',  ( -1.194225721784776262, -0.004921259842519870586, -0.3153832671262229437 ) ) ;
#18421=CARTESIAN_POINT ( 'NONE',  ( -1.187664041994749731, -0.3162353388693405765, 0.4822834645669290543 ) ) ;
#18422=CARTESIAN_POINT ( 'NONE',  ( -1.056430446194224881, -0.6692913385826771977, 0.1292274648535927661 ) ) ;
#18424=CARTESIAN_POINT ( 'NONE',  ( -1.194225721784776262, 0.05413385826771626580, -0.4176697321401330321 ) ) ;
#18425=CARTESIAN_POINT ( 'NONE',  ( -0.8727034120734901146, -0.05778040916215560624, -0.4822834645669293319 ) ) ;
#18426=DIRECTION ( 'NONE',  ( -1.000000000000000000, -3.190296047773437643E-16, 0.000000000000000000 ) ) ;
#18427=CARTESIAN_POINT ( 'NONE',  ( -1.692913385826770645, 0.2952755905511811885, 0.000000000000000000 ) ) ;
#18428=CARTESIAN_POINT ( 'NONE',  ( 0.6824146981627303710, -0.5023911411419708095, 0.1820866141732285504 ) ) ;
#18430=CARTESIAN_POINT ( 'NONE',  ( -1.614173228346457378, 2.157411728916712068, 0.1372047244094476981 ) ) ;
#18431=CARTESIAN_POINT ( 'NONE',  ( -0.1509186351706028884, -0.08942795157527998196, 0.3641732283464567121 ) ) ;
#18432=CARTESIAN_POINT ( 'NONE',  ( -0.3018372703412066094, -0.4281496062992127816, -0.4176697321401328100 ) ) ;
#18433=CARTESIAN_POINT ( 'NONE',  ( 1.305774278215223960, 0.2952755905511810774, -0.1292274648535930714 ) ) ;
#18434=CARTESIAN_POINT ( 'NONE',  ( -0.6430446194225712953, 0.05413385826771626580, -0.4176697321401330321 ) ) ;
#18440=CARTESIAN_POINT ( 'NONE',  ( 1.148293963254593653, 0.2952755905511810774, -0.1292274648535930714 ) ) ;
#18441=CARTESIAN_POINT ( 'NONE',  ( -1.056430446194224881, 0.1771653543307087075, -0.09757992244046823083 ) ) ;
#18442=CARTESIAN_POINT ( 'NONE',  ( -1.397637795275589623, 0.1660481256975885056, 0.3530559997133364547 ) ) ;
#18446=CARTESIAN_POINT ( 'NONE',  ( 1.404199475065617708, 0.05413385826771626580, -0.4176697321401330321 ) ) ;
#18448=CARTESIAN_POINT ( 'NONE',  ( 0.1377952755905518800, 0.1660481256975883668, -0.3530559997133364547 ) ) ;
#18449=CARTESIAN_POINT ( 'NONE',  ( -0.9580052493438311334, -0.004921259842519870586, -0.3153832671262229437 ) ) ;
#18450=CARTESIAN_POINT ( 'NONE',  ( -0.3346456692913377662, -0.5400638737290844871, 0.3530559997133364547 ) ) ;
#18452=CARTESIAN_POINT ( 'NONE',  ( -0.6692913385826764205, -0.6692913385826771977, 8.415575281601705876E-17 ) ) ;
#18454=CARTESIAN_POINT ( 'NONE',  ( 1.240157480314961314, -0.4536011799217367080, 0.2665933059059888421 ) ) ;
#18455=CARTESIAN_POINT ( 'NONE',  ( -0.2624671916010490880, 0.1283753931104746893, -0.1820866141732285504 ) ) ;
#18456=CARTESIAN_POINT ( 'NONE',  ( 0.7020997375328090762, -0.2845877964562159024, 0.3641732283464567677 ) ) ;
#18457=CARTESIAN_POINT ( 'NONE',  ( -1.489501312335957062, -0.3162353388693409650, -0.4822834645669289433 ) ) ;
#18459=CARTESIAN_POINT ( 'NONE',  ( 0.5905511811023629321, 0.1771653543307087630, 0.000000000000000000 ) ) ;
#18460=CARTESIAN_POINT ( 'NONE',  ( -0.8858267716535425107, -0.5400638737290844871, 0.3530559997133364547 ) ) ;
#18461=CARTESIAN_POINT ( 'NONE',  ( 1.089942661822472569, 9.906153642143428645E-17, -0.3464511005275205946 ) ) ;
#18462=CARTESIAN_POINT ( 'NONE',  ( 0.006561679790026889343, -0.2845877964562161244, -0.3641732283464567121 ) ) ;
#18463=CARTESIAN_POINT ( 'NONE',  ( -1.673228346456691717, 0.07958543189024071263, -0.2665933059059888421 ) ) ;
#18464=EDGE_CURVE ( 'NONE', #21784, #38952, #31993, .T. ) ;
#18465=CARTESIAN_POINT ( 'NONE',  ( 0.7283464566929143125, 0.1660481256975885056, 0.3530559997133364547 ) ) ;
#18467=CARTESIAN_POINT ( 'NONE',  ( 1.548556430446194954, -0.5023911411419708095, 0.1820866141732285504 ) ) ;
#18468=CARTESIAN_POINT ( 'NONE',  ( -1.220472440944881054, 0.2952755905511811885, 0.000000000000000000 ) ) ;
#18469=CARTESIAN_POINT ( 'NONE',  ( -0.1246719160104980823, -0.5511811023622048555, -0.09757992244046775898 ) ) ;
#18470=CARTESIAN_POINT ( 'NONE',  ( -1.614173228346456712, 0.9921945702958917535, -0.1372047244094478091 ) ) ;
#18471=CARTESIAN_POINT ( 'NONE',  ( 0.2559055118110243332, -0.4536011799217368745, -0.2665933059059886201 ) ) ;
#18472=CARTESIAN_POINT ( 'NONE',  ( -1.364829396325458521, 0.2306618581243847221, -0.2411417322834647770 ) ) ;
#18473=CARTESIAN_POINT ( 'NONE',  ( -0.6758530183727028406, 0.2952755905511811885, 0.1292274648535926551 ) ) ;
#18475=VECTOR ( 'NONE', #10712, 39.37007874015748143 ) ;
#18477=CARTESIAN_POINT ( 'NONE',  ( 0.4199475065616803948, -0.5023911411419708095, -0.1820866141732282451 ) ) ;
#18478=CARTESIAN_POINT ( 'NONE',  ( -0.5249343832020990641, 0.2306618581243848609, 0.2411417322834645549 ) ) ;
#18479=CARTESIAN_POINT ( 'NONE',  ( -0.9055118110236215490, -0.6692913385826771977, 8.415575281601705876E-17 ) ) ;
#18480=CARTESIAN_POINT ( 'NONE',  ( -0.9580052493438311334, -0.004921259842519870586, -0.3153832671262229437 ) ) ;
#18482=CARTESIAN_POINT ( 'NONE',  ( 0.03280839895013198948, -0.6692913385826773087, -0.1292274648535924053 ) ) ;
#18483=CARTESIAN_POINT ( 'NONE',  ( -1.555118110236219930, 0.07958543189024085140, 0.2665933059059887866 ) ) ;
#18484=CARTESIAN_POINT ( 'NONE',  ( 1.555118110236221041, -0.5400638737290844871, 0.3530559997133364547 ) ) ;
#18486=EDGE_LOOP ( 'NONE', ( #76033, #45701, #481, #9692 ) ) ;
#18488=CARTESIAN_POINT ( 'NONE',  ( -1.528871391076114250, 0.2952755905511810774, -0.1292274648535930714 ) ) ;
#18489=CARTESIAN_POINT ( 'NONE',  ( -0.8005249343832013809, -0.4281496062992124485, 0.4176697321401328655 ) ) ;
#18490=CARTESIAN_POINT ( 'NONE',  ( 1.496062992125984703, -0.1870078740157480879, -0.4822834645669291653 ) ) ;
#18493=CARTESIAN_POINT ( 'NONE',  ( 0.7545931758530189937, 0.2952755905511810774, -0.1292274648535930714 ) ) ;
#18494=CARTESIAN_POINT ( 'NONE',  ( 0.1837270341207357105, -0.6046776061558809534, -0.2411417322834644161 ) ) ;
#18497=CARTESIAN_POINT ( 'NONE',  ( 1.167979002624672580, -0.004921259842519870586, -0.3153832671262229437 ) ) ;
#18499=ORIENTED_EDGE ( 'NONE', *, *, #12912, .F. ) ;
#18502=CARTESIAN_POINT ( 'NONE',  ( 0.2952755905511816326, -0.5400638737290844871, 0.3530559997133364547 ) ) ;
#18503=CARTESIAN_POINT ( 'NONE',  ( -0.7217847769028863381, 0.05413385826771626580, -0.4176697321401330321 ) ) ;
#18504=CARTESIAN_POINT ( 'NONE',  ( 1.594488188976378673, 0.1660481256975885056, 0.3530559997133364547 ) ) ;
#18505=CARTESIAN_POINT ( 'NONE',  ( 0.6102362204724416372, 0.1660481256975883668, -0.3530559997133364547 ) ) ;
#18506=CARTESIAN_POINT ( 'NONE',  ( 1.469816272965879911, -0.6046776061558807314, 0.2411417322834647770 ) ) ;
#18507=CARTESIAN_POINT ( 'NONE',  ( 1.607611548556431069, 0.2952755905511811885, 0.1292274648535926551 ) ) ;
#18508=CARTESIAN_POINT ( 'NONE',  ( 0.04593175853018440641, -0.6692913385826771977, 0.1292274648535927661 ) ) ;
#18509=CARTESIAN_POINT ( 'NONE',  ( -1.213910761154854745, -0.6692913385826771977, 0.1292274648535927661 ) ) ;
#18510=CARTESIAN_POINT ( 'NONE',  ( 1.607611548556431069, 0.2952755905511811885, 0.1292274648535926551 ) ) ;
#18511=FACE_OUTER_BOUND ( 'NONE', #14521, .T. ) ;
#18513=CARTESIAN_POINT ( 'NONE',  ( 1.023622047244095334, -0.1870078740157479769, 0.3641732283464567677 ) ) ;
#18517=CARTESIAN_POINT ( 'NONE',  ( 0.1509186351706042484, -0.2845877964562159024, 0.3641732283464567677 ) ) ;
#18518=FACE_OUTER_BOUND ( 'NONE', #73790, .T. ) ;
#18519=CARTESIAN_POINT ( 'NONE',  ( 0.6364829396325465405, -0.05778040916215522460, 0.4822834645669289988 ) ) ;
#18520=CARTESIAN_POINT ( 'NONE',  ( 0.2230971128608929543, 0.05413385826771626580, -0.4176697321401330321 ) ) ;
#18521=CARTESIAN_POINT ( 'NONE',  ( -0.6102362204724400829, 0.1660481256975885056, 0.3530559997133364547 ) ) ;
#18523=CARTESIAN_POINT ( 'NONE',  ( -1.233595800524933894, -0.6046776061558809534, -0.2411417322834644161 ) ) ;
#18525=CARTESIAN_POINT ( 'NONE',  ( 1.456692913385827515, 0.1771653543307087630, 0.000000000000000000 ) ) ;
#18526=CARTESIAN_POINT ( 'NONE',  ( -1.351706036745406347, -0.4281496062992124485, 0.4176697321401328655 ) ) ;
#18527=CARTESIAN_POINT ( 'NONE',  ( 0.9973753280839902091, -0.6046776061558807314, 0.2411417322834647770 ) ) ;
#18528=CARTESIAN_POINT ( 'NONE',  ( 1.318897637795276356, -0.5400638737290844871, 0.3530559997133364547 ) ) ;
#18530=CARTESIAN_POINT ( 'NONE',  ( -1.174540682414697335, -0.3162353388693409650, -0.4822834645669289433 ) ) ;
#18533=CARTESIAN_POINT ( 'NONE',  ( -0.03937007874015669567, -0.6692913385826771977, 8.415575281601705876E-17 ) ) ;
#18536=VECTOR ( 'NONE', #60196, 39.37007874015748143 ) ;
#18537=CARTESIAN_POINT ( 'NONE',  ( 1.555118110236221041, 0.1660481256975883668, -0.3530559997133364547 ) ) ;
#18538=CARTESIAN_POINT ( 'NONE',  ( 0.03937007874015833325, -0.5511811023622047445, 6.969142054262312111E-17 ) ) ;
#18539=CARTESIAN_POINT ( 'NONE',  ( 1.076115485564305141, -0.6046776061558807314, 0.2411417322834647770 ) ) ;
#18541=CARTESIAN_POINT ( 'NONE',  ( 0.1640419947506569498, -0.2845877964562161244, -0.3641732283464567121 ) ) ;
#18542=CARTESIAN_POINT ( 'NONE',  ( 0.4330708661417329575, -0.6692913385826771977, 8.415575281601705876E-17 ) ) ;
#18544=CARTESIAN_POINT ( 'NONE',  ( -0.8070866141732276899, -0.5400638737290844871, 0.3530559997133364547 ) ) ;
#18545=CARTESIAN_POINT ( 'NONE',  ( -0.1837270341207340729, 0.2306618581243847221, -0.2411417322834647770 ) ) ;
#18546=CARTESIAN_POINT ( 'NONE',  ( 0.7414698162729663755, -0.5511811023622048555, -0.09757992244046775898 ) ) ;
#18547=CARTESIAN_POINT ( 'NONE',  ( -0.2821522309711278487, 0.2952755905511811885, 0.1292274648535926551 ) ) ;
#18548=CARTESIAN_POINT ( 'NONE',  ( 0.1377952755905518800, 0.07958543189024071263, -0.2665933059059888421 ) ) ;
#18550=CARTESIAN_POINT ( 'NONE',  ( -0.2165354330708654795, -0.5400638737290845981, -0.3530559997133363437 ) ) ;
#18551=CARTESIAN_POINT ( 'NONE',  ( 0.3346456692913390985, 0.07958543189024085140, 0.2665933059059887866 ) ) ;
#18553=CARTESIAN_POINT ( 'NONE',  ( 0.4068241469816281097, 0.05413385826771666132, 0.4176697321401328100 ) ) ;
#18555=CARTESIAN_POINT ( 'NONE',  ( 1.049868766404200349, 0.1283753931104748280, 0.1820866141732283561 ) ) ;
#18556=CARTESIAN_POINT ( 'NONE',  ( -0.1678194419220245537, 3.103433371374072050E-15, -0.4281989832122387041 ) ) ;
#18557=CARTESIAN_POINT ( 'NONE',  ( -0.5511811023622041894, -0.1870078740157480601, -0.3641732283464567677 ) ) ;
#18558=CARTESIAN_POINT ( 'NONE',  ( -0.8267716535433065062, -0.5511811023622047445, 6.969142054262312111E-17 ) ) ;
#18559=CARTESIAN_POINT ( 'NONE',  ( -0.4330708661417315697, -0.6692913385826771977, 8.415575281601705876E-17 ) ) ;
#18560=EDGE_CURVE ( 'NONE', #6101, #48718, #18665, .T. ) ;
#18561=CARTESIAN_POINT ( 'NONE',  ( 0.2952755905511816326, -0.5400638737290844871, 0.3530559997133364547 ) ) ;
#18562=CARTESIAN_POINT ( 'NONE',  ( 1.095800524934383846, -0.08942795157528024563, -0.3641732283464568787 ) ) ;
#18564=CARTESIAN_POINT ( 'NONE',  ( 1.377952755905512472, -0.5511811023622047445, 6.969142054262312111E-17 ) ) ;
#18565=CARTESIAN_POINT ( 'NONE',  ( 0.6627296587926517768, -0.6692913385826773087, -0.1292274648535924053 ) ) ;
#18566=CARTESIAN_POINT ( 'NONE',  ( -1.586052503253846169, 1.850393700787402729, -0.1653254495020583803 ) ) ;
#18567=CARTESIAN_POINT ( 'NONE',  ( -0.07217847769028813698, -0.3162353388693409650, -0.4822834645669289433 ) ) ;
#18569=CARTESIAN_POINT ( 'NONE',  ( 0.9186351706036752773, 0.2306618581243847221, -0.2411417322834647770 ) ) ;
#18570=CARTESIAN_POINT ( 'NONE',  ( 0.5774278215223104249, 0.2306618581243848609, 0.2411417322834645549 ) ) ;
#18572=CARTESIAN_POINT ( 'NONE',  ( 0.3740157480314966754, -0.4536011799217367080, 0.2665933059059888421 ) ) ;
#18573=CARTESIAN_POINT ( 'NONE',  ( 1.154855643044620184, -0.6046776061558807314, 0.2411417322834647770 ) ) ;
#18574=CARTESIAN_POINT ( 'NONE',  ( -0.4396325459317579898, 0.1771653543307087630, 0.09757992244046791164 ) ) ;
#18575=CARTESIAN_POINT ( 'NONE',  ( -0.5052493438320203589, 0.2952755905511810774, -0.1292274648535930714 ) ) ;
#18577=CARTESIAN_POINT ( 'NONE',  ( 0.2165354330708668673, 0.1660481256975883668, -0.3530559997133364547 ) ) ;
#18578=CARTESIAN_POINT ( 'NONE',  ( -0.7545931758530176614, -0.6692913385826773087, -0.1292274648535924053 ) ) ;
#18579=CARTESIAN_POINT ( 'NONE',  ( -0.8070866141732276899, -0.4536011799217367080, 0.2665933059059888421 ) ) ;
#18580=CARTESIAN_POINT ( 'NONE',  ( 0.5118110236220478892, 0.2952755905511811885, 0.000000000000000000 ) ) ;
#18581=CARTESIAN_POINT ( 'NONE',  ( -1.292650918635170010, -0.6692913385826771977, 0.1292274648535927661 ) ) ;
#18582=CARTESIAN_POINT ( 'NONE',  ( -0.5314960629921250401, 0.1660481256975885056, 0.3530559997133364547 ) ) ;
#18584=FACE_OUTER_BOUND ( 'NONE', #69127, .T. ) ;
#18585=CARTESIAN_POINT ( 'NONE',  ( 1.489501312335958172, -0.05778040916215560624, -0.4822834645669293319 ) ) ;
#18587=B_SPLINE_CURVE_WITH_KNOTS ( 'NONE', 3,
 ( #15684, #35857, #9355, #10604, #74995, #23623, #62337 ),
 .UNSPECIFIED., .F., .F.,
 ( 4, 3, 4 ),
 ( 0.000000000000000000, 0.001246232571205245976, 0.002492492258783242029 ),
 .UNSPECIFIED. ) ;
#18588=VECTOR ( 'NONE', #27915, 39.37007874015748143 ) ;
#18589=CARTESIAN_POINT ( 'NONE',  ( -1.469816272965878357, 0.2306618581243848609, 0.2411417322834645549 ) ) ;
#18590=CARTESIAN_POINT ( 'NONE',  ( -0.9186351706036736120, 0.2306618581243848609, 0.2411417322834645549 ) ) ;
#18593=VERTEX_POINT ( 'NONE', #25376 ) ;
#18594=CARTESIAN_POINT ( 'NONE',  ( 0.4986876640419954376, -0.5023911411419708095, -0.1820866141732282451 ) ) ;
#18596=CARTESIAN_POINT ( 'NONE',  ( 0.6496062992125991586, 0.1660481256975885056, 0.3530559997133364547 ) ) ;
#18599=CARTESIAN_POINT ( 'NONE',  ( -0.5183727034120726440, 0.1771653543307087630, 0.09757992244046791164 ) ) ;
#18601=CARTESIAN_POINT ( 'NONE',  ( 1.102362204724410155, -0.1870078740157480879, -0.4822834645669291653 ) ) ;
#18602=CARTESIAN_POINT ( 'NONE',  ( 0.7742782152230978099, -0.3690944881889763329, 0.3153832671262228327 ) ) ;
#18603=CARTESIAN_POINT ( 'NONE',  ( -0.05905511811023545637, 0.1660481256975885056, 0.3530559997133364547 ) ) ;
#18605=CARTESIAN_POINT ( 'NONE',  ( -0.2887139107611542133, -0.6046776061558809534, -0.2411417322834644161 ) ) ;
#18606=CARTESIAN_POINT ( 'NONE',  ( -1.384514435695537005, 0.1771653543307087630, 0.09757992244046791164 ) ) ;
#18607=CARTESIAN_POINT ( 'NONE',  ( -0.5052493438320203589, -0.6692913385826771977, 0.1292274648535927661 ) ) ;
#18608=DIRECTION ( 'NONE',  ( 1.000000000000000000, -0.000000000000000000, -0.000000000000000000 ) ) ;
#18612=CARTESIAN_POINT ( 'NONE',  ( 0.4330708661417329575, 0.2952755905511811885, 0.000000000000000000 ) ) ;
#18614=CARTESIAN_POINT ( 'NONE',  ( -0.9383202099737524282, -0.05778040916215522460, 0.4822834645669289988 ) ) ;
#18615=CARTESIAN_POINT ( 'NONE',  ( -1.555118110236219930, -0.5400638737290845981, -0.3530559997133363437 ) ) ;
#18616=CARTESIAN_POINT ( 'NONE',  ( 0.5249343832021003964, 0.2306618581243847221, -0.2411417322834647770 ) ) ;
#18617=CARTESIAN_POINT ( 'NONE',  ( -0.04593175853018302557, 0.2952755905511811885, 0.1292274648535926551 ) ) ;
#18619=CARTESIAN_POINT ( 'NONE',  ( -0.8398950131233589023, -0.6046776061558809534, -0.2411417322834644161 ) ) ;
#18620=CARTESIAN_POINT ( 'NONE',  ( -0.1443569553805765515, -0.4281496062992127816, -0.4176697321401328100 ) ) ;
#18621=CARTESIAN_POINT ( 'NONE',  ( -1.023622047244093558, -0.1870078740157479769, 0.4822834645669291653 ) ) ;
#18622=CARTESIAN_POINT ( 'NONE',  ( 0.3215223097112867578, -0.2845877964562161244, -0.3641732283464567121 ) ) ;
#18624=CARTESIAN_POINT ( 'NONE',  ( 0.08530183727034192087, -0.3162353388693409650, -0.4822834645669289433 ) ) ;
#18626=CARTESIAN_POINT ( 'NONE',  ( 1.305774278215223960, 0.2952755905511810774, -0.1292274648535930714 ) ) ;
#18630=CARTESIAN_POINT ( 'NONE',  ( 0.4527559055118117182, 0.1660481256975883668, -0.3530559997133364547 ) ) ;
#18631=CARTESIAN_POINT ( 'NONE',  ( 0.04593175853018440641, 0.1771653543307087075, -0.09757992244046823083 ) ) ;
#18632=CARTESIAN_POINT ( 'NONE',  ( 1.568241469816273659, -0.08942795157528024563, -0.3641732283464568787 ) ) ;
#18637=CARTESIAN_POINT ( 'NONE',  ( -1.574803149606298192, -0.1870078740157480879, -0.4822834645669291653 ) ) ;
#18639=CARTESIAN_POINT ( 'NONE',  ( 0.4790026246719167324, -0.05778040916215522460, 0.4822834645669289988 ) ) ;
#18640=CARTESIAN_POINT ( 'NONE',  ( -1.351706036745406347, -0.4281496062992124485, 0.4176697321401328655 ) ) ;
#18641=CARTESIAN_POINT ( 'NONE',  ( -1.207349081364828880, 0.2306618581243847221, -0.2411417322834647770 ) ) ;
#18642=CARTESIAN_POINT ( 'NONE',  ( 0.4002624671916016896, -0.3162353388693409650, -0.4822834645669289433 ) ) ;
#18643=CARTESIAN_POINT ( 'NONE',  ( 1.148293963254593653, 0.2952755905511810774, -0.1292274648535930714 ) ) ;
#18644=CARTESIAN_POINT ( 'NONE',  ( 1.286089238845145033, -0.5023911411419708095, -0.1820866141732282451 ) ) ;
#18645=CARTESIAN_POINT ( 'NONE',  ( 0.8333333333333340365, -0.5511811023622046335, 0.09757992244046803654 ) ) ;
#18646=CARTESIAN_POINT ( 'NONE',  ( -0.8595800524934373854, -0.05778040916215522460, 0.4822834645669289988 ) ) ;
#18648=CARTESIAN_POINT ( 'NONE',  ( 1.502624671916010790, -0.05778040916215522460, 0.4822834645669289988 ) ) ;
#18650=CARTESIAN_POINT ( 'NONE',  ( 0.8595800524934390507, -0.3162353388693405765, 0.4822834645669290543 ) ) ;
#18652=CARTESIAN_POINT ( 'NONE',  ( -1.574803149606298636, -0.1870078740157479769, 0.3641732283464567677 ) ) ;
#18653=CARTESIAN_POINT ( 'NONE',  ( 0.1246719160104994284, 0.2952755905511810774, -0.1292274648535930714 ) ) ;
#18654=CARTESIAN_POINT ( 'NONE',  ( 0.6561679790026253567, 0.1283753931104748280, 0.1820866141732283561 ) ) ;
#18655=CARTESIAN_POINT ( 'NONE',  ( -1.719160104986876103, -0.004921259842519576551, 0.3153832671262227771 ) ) ;
#18656=CARTESIAN_POINT ( 'NONE',  ( 0.9448818897637802916, -0.1870078740157480879, -0.4822834645669291653 ) ) ;
#18657=LINE ( 'NONE', #12347, #826 ) ;
#18658=CARTESIAN_POINT ( 'NONE',  ( -0.6233595800524928121, -0.08942795157527998196, 0.3641732283464567121 ) ) ;
#18659=CARTESIAN_POINT ( 'NONE',  ( -0.7808398950131225646, -0.05778040916215522460, 0.4822834645669289988 ) ) ;
#18660=CARTESIAN_POINT ( 'NONE',  ( 1.384514435695538559, 0.2952755905511810774, -0.1292274648535930714 ) ) ;
#18661=CARTESIAN_POINT ( 'NONE',  ( -1.240157480314959759, 0.1660481256975885056, 0.3530559997133364547 ) ) ;
#18662=CARTESIAN_POINT ( 'NONE',  ( 1.266404199475066328, -0.3162353388693409650, -0.4822834645669289433 ) ) ;
#18664=CARTESIAN_POINT ( 'NONE',  ( -1.397637795275589623, -0.4536011799217368745, -0.2665933059059886201 ) ) ;
#18665=LINE ( 'NONE', #43902, #3431 ) ;
#18666=CARTESIAN_POINT ( 'NONE',  ( 1.082677165354331228, -0.5400638737290844871, 0.3530559997133364547 ) ) ;
#18668=CARTESIAN_POINT ( 'NONE',  ( -1.423884514435694859, -0.3162353388693405765, 0.4822834645669290543 ) ) ;
#18669=CARTESIAN_POINT ( 'NONE',  ( -1.463254593175852492, 0.1771653543307087630, 0.09757992244046791164 ) ) ;
#18670=CARTESIAN_POINT ( 'NONE',  ( -0.9776902887139098386, -0.5511811023622046335, 0.09757992244046803654 ) ) ;
#18672=CARTESIAN_POINT ( 'NONE',  ( -0.5249343832020990641, 0.2306618581243848609, 0.2411417322834645549 ) ) ;
#18673=CARTESIAN_POINT ( 'NONE',  ( 0.006561679790026889343, -0.2845877964562161244, -0.3641732283464567121 ) ) ;
#18674=CARTESIAN_POINT ( 'NONE',  ( -1.581364829396324945, -0.2845877964562159024, 0.3641732283464567677 ) ) ;
#18675=CARTESIAN_POINT ( 'NONE',  ( 0.9514435695538062676, -0.08942795157527998196, 0.3641732283464567121 ) ) ;
#18676=CARTESIAN_POINT ( 'NONE',  ( 0.7874015748031503170, -0.1870078740157480879, -0.4822834645669291653 ) ) ;
#18677=CARTESIAN_POINT ( 'NONE',  ( 1.581364829396326277, -0.05778040916215522460, 0.4822834645669289988 ) ) ;
#18678=CARTESIAN_POINT ( 'NONE',  ( 0.1049868766404206816, 0.1283753931104748280, 0.1820866141732283561 ) ) ;
#18679=CARTESIAN_POINT ( 'NONE',  ( 0.5249343832021005074, -0.6046776061558807314, 0.2411417322834647770 ) ) ;
#18681=CARTESIAN_POINT ( 'NONE',  ( 0.5249343832021003964, 0.1283753931104746893, -0.1820866141732285504 ) ) ;
#18683=CARTESIAN_POINT ( 'NONE',  ( -1.561679790026246017, -0.4281496062992127816, -0.4176697321401328100 ) ) ;
#18685=( BOUNDED_CURVE ( )  B_SPLINE_CURVE ( 2, ( #5504, #25262, #62338, #50516, #5911, #82128, #51338, #77042, #18150, #69489, #82531, #24849, #30348 ),
 .UNSPECIFIED., .F., .F. ) 
 B_SPLINE_CURVE_WITH_KNOTS ( ( 3, 2, 2, 2, 2, 2, 3 ),
 ( 0.4006038219075281348, 0.4015151515151514916, 0.4053030303030302761, 0.4090909090909091161, 0.4128787878787879007, 0.4166666666666666852, 0.4175779962742901530 ),
 .UNSPECIFIED. ) 
 CURVE ( )  GEOMETRIC_REPRESENTATION_ITEM ( )  RATIONAL_B_SPLINE_CURVE ( ( 0.9875488213027530104, 0.9918020599134685922, 1.000000000000000000, 0.9659258262890683122, 1.000000000000000000, 0.9659258262890683122, 1.000000000000000000, 0.9659258262890683122, 1.000000000000000000, 0.9659258262890683122, 1.000000000000000000, 0.9918020599134675930, 0.9875488213027519002 ) ) 
 REPRESENTATION_ITEM ( '' )  );
#18686=CARTESIAN_POINT ( 'NONE',  ( -1.410761154855641575, -0.3162353388693409650, -0.4822834645669289433 ) ) ;
#18687=CARTESIAN_POINT ( 'NONE',  ( -0.03937007874015669567, -0.6692913385826771977, 8.415575281601705876E-17 ) ) ;
#18690=CARTESIAN_POINT ( 'NONE',  ( 0.4658792650918640033, -0.3162353388693405765, 0.4822834645669290543 ) ) ;
#18691=CARTESIAN_POINT ( 'NONE',  ( 1.069553805774278610, -0.5511811023622046335, 0.09757992244046803654 ) ) ;
#18692=CARTESIAN_POINT ( 'NONE',  ( -0.2362204724409440182, -0.1870078740157479769, 0.4822834645669291653 ) ) ;
#18693=CARTESIAN_POINT ( 'NONE',  ( 0.4133858267716541968, -0.5400638737290845981, -0.3530559997133363437 ) ) ;
#18694=AXIS2_PLACEMENT_3D ( 'NONE', #65783, #78412, #26203 ) ;
#18698=DIRECTION ( 'NONE',  ( 1.000000000000000000, 3.469446951953613203E-16, 0.000000000000000000 ) ) ;
#18700=CARTESIAN_POINT ( 'NONE',  ( -0.3346456692913377662, -0.4536011799217367080, 0.2665933059059888421 ) ) ;
#18701=CARTESIAN_POINT ( 'NONE',  ( -1.102362204724408601, -0.1870078740157479769, 0.4822834645669291653 ) ) ;
#18703=CARTESIAN_POINT ( 'NONE',  ( 0.8595800524934390507, -0.3162353388693405765, 0.4822834645669290543 ) ) ;
#18705=CARTESIAN_POINT ( 'NONE',  ( -1.614173228346455824, 0.2952755905511811885, 0.000000000000000000 ) ) ;
#18706=CARTESIAN_POINT ( 'NONE',  ( 0.7545931758530188826, -0.6692913385826771977, 0.1292274648535927661 ) ) ;
#18708=CARTESIAN_POINT ( 'NONE',  ( 1.646981627296588035, -0.3162353388693405765, 0.4822834645669290543 ) ) ;
#18710=CARTESIAN_POINT ( 'NONE',  ( 1.102362204724410155, -0.1870078740157479769, 0.4822834645669291653 ) ) ;
#18711=CARTESIAN_POINT ( 'NONE',  ( 0.5314960629921264834, 0.1660481256975883668, -0.3530559997133364547 ) ) ;
#18712=CARTESIAN_POINT ( 'NONE',  ( 0.7611548556430451917, -0.5023911411419708095, 0.1820866141732285504 ) ) ;
#18713=CARTESIAN_POINT ( 'NONE',  ( 1.154855643044620184, -0.6046776061558807314, 0.2411417322834647770 ) ) ;
#18715=CARTESIAN_POINT ( 'NONE',  ( -1.586052503253845503, 2.125984251968505045, 0.1653254495020588799 ) ) ;
#18716=CARTESIAN_POINT ( 'NONE',  ( 0.6167979002624679463, 0.05413385826771626580, -0.4176697321401330321 ) ) ;
#18717=CARTESIAN_POINT ( 'NONE',  ( -1.128608923884513837, -0.6046776061558807314, 0.2411417322834647770 ) ) ;
#18718=CARTESIAN_POINT ( 'NONE',  ( -0.8792650918635160906, 0.05413385826771626580, -0.4176697321401330321 ) ) ;
#18719=CARTESIAN_POINT ( 'NONE',  ( 1.266404199475066328, -0.05778040916215522460, 0.4822834645669289988 ) ) ;
#18726=FACE_OUTER_BOUND ( 'NONE', #12056, .T. ) ;
#18727=CARTESIAN_POINT ( 'NONE',  ( 1.417322834645670104, -0.1870078740157479769, 0.3641732283464567677 ) ) ;
#18729=CARTESIAN_POINT ( 'NONE',  ( 1.279527559055118724, -0.4536011799217368745, -0.2665933059059886201 ) ) ;
#18731=CARTESIAN_POINT ( 'NONE',  ( -1.646051170424378096, 0.000000000000000000, -0.3464511005275205946 ) ) ;
#18734=CARTESIAN_POINT ( 'NONE',  ( -0.9317585301837263412, -0.3690944881889765550, -0.3153832671262227771 ) ) ;
#18735=CARTESIAN_POINT ( 'NONE',  ( -1.456692913385826182, -0.5511811023622047445, 6.969142054262312111E-17 ) ) ;
#18736=CARTESIAN_POINT ( 'NONE',  ( -1.148293963254592542, 0.2952755905511811885, 0.1292274648535926551 ) ) ;
#18737=CARTESIAN_POINT ( 'NONE',  ( 0.1377952755905518800, -0.5400638737290844871, 0.3530559997133364547 ) ) ;
#18738=CARTESIAN_POINT ( 'NONE',  ( 1.371391076115485719, -0.6692913385826773087, -0.1292274648535924053 ) ) ;
#18742=CARTESIAN_POINT ( 'NONE',  ( 1.614173228346457156, 1.496062992125984037, 0.5309055118110233007 ) ) ;
#18743=CARTESIAN_POINT ( 'NONE',  ( -0.5052493438320203589, 0.1771653543307087075, -0.09757992244046823083 ) ) ;
#18744=CARTESIAN_POINT ( 'NONE',  ( -1.227034120734907141, -0.6692913385826773087, -0.1292274648535924053 ) ) ;
#18745=CARTESIAN_POINT ( 'NONE',  ( 1.036745406824147731, 0.05413385826771666132, 0.4176697321401328100 ) ) ;
#18746=ORIENTED_EDGE ( 'NONE', *, *, #4808, .T. ) ;
#18749=CARTESIAN_POINT ( 'NONE',  ( 1.266404199475066328, -0.3162353388693409650, -0.4822834645669289433 ) ) ;
#18750=CARTESIAN_POINT ( 'NONE',  ( -1.128608923884513837, -0.6046776061558807314, 0.2411417322834647770 ) ) ;
#18752=CARTESIAN_POINT ( 'NONE',  ( -0.4002624671916004129, -0.08942795157528024563, -0.3641732283464568787 ) ) ;
#18754=CARTESIAN_POINT ( 'NONE',  ( -0.5905511811023613777, -0.5511811023622047445, 6.969142054262312111E-17 ) ) ;
#18755=CARTESIAN_POINT ( 'NONE',  ( 0.3215223097112867578, -0.08942795157527998196, 0.3641732283464567121 ) ) ;
#18756=CARTESIAN_POINT ( 'NONE',  ( 0.01968503937007930540, 0.1660481256975885056, 0.3530559997133364547 ) ) ;
#18757=CARTESIAN_POINT ( 'NONE',  ( -0.7349081364829387342, -0.5023911411419708095, 0.1820866141732285504 ) ) ;
#18759=CARTESIAN_POINT ( 'NONE',  ( 1.148293963254593653, 0.2952755905511810774, -0.1292274648535930714 ) ) ;
#18761=CARTESIAN_POINT ( 'NONE',  ( -1.496062992125983815, -0.1870078740157479769, 0.4822834645669291653 ) ) ;
#18763=CARTESIAN_POINT ( 'NONE',  ( -0.5643044619422565855, 0.05413385826771626580, -0.4176697321401330321 ) ) ;
#18764=CARTESIAN_POINT ( 'NONE',  ( -0.8530183727034112984, 0.05413385826771666132, 0.4176697321401328100 ) ) ;
#18765=CARTESIAN_POINT ( 'NONE',  ( 1.213910761154856299, 0.1771653543307087630, 0.09757992244046791164 ) ) ;
#18766=CARTESIAN_POINT ( 'NONE',  ( -0.3937007874015740483, -0.1870078740157480601, -0.3641732283464567677 ) ) ;
#18767=CARTESIAN_POINT ( 'NONE',  ( -0.8005249343832013809, -0.4281496062992124485, 0.4176697321401328655 ) ) ;
#18768=CARTESIAN_POINT ( 'NONE',  ( -1.292650918635170010, 0.2952755905511810774, -0.1292274648535930714 ) ) ;
#18770=CARTESIAN_POINT ( 'NONE',  ( 1.135170603674541256, -0.5511811023622048555, -0.09757992244046775898 ) ) ;
#18771=CARTESIAN_POINT ( 'NONE',  ( -0.4461942257217840213, -0.6046776061558809534, -0.2411417322834644161 ) ) ;
#18772=CARTESIAN_POINT ( 'NONE',  ( -1.187664041994750175, -0.05778040916215560624, -0.4822834645669293319 ) ) ;
#18775=CARTESIAN_POINT ( 'NONE',  ( -0.6889763779527552368, 0.07958543189024085140, 0.2665933059059887866 ) ) ;
#18776=CARTESIAN_POINT ( 'NONE',  ( 1.240157480314961314, -0.5400638737290844871, 0.3530559997133364547 ) ) ;
#18777=CARTESIAN_POINT ( 'NONE',  ( -1.036745406824146176, -0.004921259842519870586, -0.3153832671262229437 ) ) ;
#18779=CARTESIAN_POINT ( 'NONE',  ( -0.9317585301837263412, 0.05413385826771666132, 0.4176697321401328100 ) ) ;
#18780=CARTESIAN_POINT ( 'NONE',  ( 1.417322834645670104, -0.1870078740157480879, -0.4822834645669291653 ) ) ;
#18781=CARTESIAN_POINT ( 'NONE',  ( 1.023622047244095334, -0.1870078740157479769, 0.4822834645669291653 ) ) ;
#18782=CARTESIAN_POINT ( 'NONE',  ( 1.456692913385827515, 0.2952755905511811885, 0.000000000000000000 ) ) ;
#18783=CARTESIAN_POINT ( 'NONE',  ( -1.325459317585300889, -0.3690944881889765550, -0.3153832671262227771 ) ) ;
#18788=CARTESIAN_POINT ( 'NONE',  ( 1.299212598425197429, -0.5511811023622047445, 6.969142054262312111E-17 ) ) ;
#18789=CARTESIAN_POINT ( 'NONE',  ( 0.6955380577427828781, -0.004921259842519870586, -0.3153832671262229437 ) ) ;
#18790=CARTESIAN_POINT ( 'NONE',  ( 0.5183727034120741983, 0.2952755905511810774, -0.1292274648535930714 ) ) ;
#18791=CARTESIAN_POINT ( 'NONE',  ( 1.509186351706037543, -0.4281496062992127816, -0.4176697321401328100 ) ) ;
#18793=CARTESIAN_POINT ( 'NONE',  ( 0.9842519685039378130, -0.5511811023622047445, 6.969142054262312111E-17 ) ) ;
#18795=CARTESIAN_POINT ( 'NONE',  ( -0.4068241469816264999, -0.4281496062992124485, 0.4176697321401328655 ) ) ;
#18796=CARTESIAN_POINT ( 'NONE',  ( -1.364829396325458521, -0.6046776061558807314, 0.2411417322834647770 ) ) ;
#18797=CARTESIAN_POINT ( 'NONE',  ( 0.9842519685039378130, -0.6692913385826771977, 8.415575281601705876E-17 ) ) ;
#18800=ORIENTED_EDGE ( 'NONE', *, *, #48192, .T. ) ;
#18801=ORIENTED_EDGE ( 'NONE', *, *, #73800, .T. ) ;
#18802=CARTESIAN_POINT ( 'NONE',  ( -1.082677165354329896, 0.1660481256975885056, 0.3530559997133364547 ) ) ;
#18803=CARTESIAN_POINT ( 'NONE',  ( -0.7808398950131222316, -0.3162353388693409650, -0.4822834645669289433 ) ) ;
#18804=CARTESIAN_POINT ( 'NONE',  ( -0.6364829396325453192, -0.08942795157528024563, -0.3641732283464568787 ) ) ;
#18805=CARTESIAN_POINT ( 'NONE',  ( -0.8923884514435688198, -0.6046776061558807314, 0.2411417322834647770 ) ) ;
#18807=CARTESIAN_POINT ( 'NONE',  ( 0.4986876640419954376, -0.6046776061558809534, -0.2411417322834644161 ) ) ;
#18808=CARTESIAN_POINT ( 'NONE',  ( -0.3149606299212590610, -0.1870078740157480879, -0.4822834645669291653 ) ) ;
#18809=CARTESIAN_POINT ( 'NONE',  ( 1.437007874015748810, 0.1660481256975885056, 0.3530559997133364547 ) ) ;
#18810=CARTESIAN_POINT ( 'NONE',  ( -0.6758530183727028406, -0.6692913385826773087, -0.1292274648535924053 ) ) ;
#18811=CARTESIAN_POINT ( 'NONE',  ( 0.6036745406824153282, -0.6046776061558807314, 0.2411417322834647770 ) ) ;
#18813=CARTESIAN_POINT ( 'NONE',  ( -0.8989501312335946848, -0.5511811023622046335, 0.09757992244046803654 ) ) ;
#18814=ORIENTED_EDGE ( 'NONE', *, *, #4808, .F. ) ;
#18817=CARTESIAN_POINT ( 'NONE',  ( -1.220472440944881054, 0.1771653543307087630, 0.000000000000000000 ) ) ;
#18818=CARTESIAN_POINT ( 'NONE',  ( -1.089238845144356427, -0.4281496062992127816, -0.4176697321401328100 ) ) ;
#18819=CARTESIAN_POINT ( 'NONE',  ( -1.069553805774277722, -0.6692913385826773087, -0.1292274648535924053 ) ) ;
#18821=CARTESIAN_POINT ( 'NONE',  ( -1.003937007874015297, -0.5400638737290845981, -0.3530559997133363437 ) ) ;
#18822=CARTESIAN_POINT ( 'NONE',  ( -1.148293963254592542, -0.6692913385826773087, -0.1292274648535924053 ) ) ;
#18823=CARTESIAN_POINT ( 'NONE',  ( -1.509186351706035767, -0.4281496062992124485, 0.4176697321401328655 ) ) ;
#18826=CARTESIAN_POINT ( 'NONE',  ( 0.3805774278215230400, -0.3690944881889763329, 0.3153832671262228327 ) ) ;
#18829=CARTESIAN_POINT ( 'NONE',  ( -0.5446194225721777693, -0.2845877964562161244, -0.3641732283464567121 ) ) ;
#18830=CARTESIAN_POINT ( 'NONE',  ( -0.2099737532808391705, 0.2306618581243848609, 0.2411417322834645549 ) ) ;
#18832=CARTESIAN_POINT ( 'NONE',  ( 1.167979002624672580, 0.05413385826771626580, -0.4176697321401330321 ) ) ;
#18833=CARTESIAN_POINT ( 'NONE',  ( -0.4724409448818890911, -0.1870078740157480879, -0.4822834645669291653 ) ) ;
#18835=ORIENTED_EDGE ( 'NONE', *, *, #58189, .F. ) ;
#18837=CARTESIAN_POINT ( 'NONE',  ( -0.3805774278215216522, 0.05413385826771666132, 0.4176697321401328100 ) ) ;
#18838=CARTESIAN_POINT ( 'NONE',  ( 1.174540682414699111, -0.05778040916215560624, -0.4822834645669293319 ) ) ;
#18839=CARTESIAN_POINT ( 'NONE',  ( -1.017060367454067249, -0.2845877964562161244, -0.3641732283464567121 ) ) ;
#18840=CARTESIAN_POINT ( 'NONE',  ( -1.266404199475064773, -0.3162353388693405765, 0.4822834645669290543 ) ) ;
#18842=CARTESIAN_POINT ( 'NONE',  ( -0.7426113562972000981, 2.362204724409448620, 0.5309055118110236338 ) ) ;
#18844=CARTESIAN_POINT ( 'NONE',  ( 1.115485564304462551, -0.4281496062992127816, -0.4176697321401328100 ) ) ;
#18846=CARTESIAN_POINT ( 'NONE',  ( -0.006561679790025524116, -0.05778040916215560624, -0.4822834645669293319 ) ) ;
#18847=CARTESIAN_POINT ( 'NONE',  ( -0.9120734908136475250, -0.5511811023622048555, -0.09757992244046775898 ) ) ;
#18848=CARTESIAN_POINT ( 'NONE',  ( -0.3740157480314953431, -0.5400638737290845981, -0.3530559997133363437 ) ) ;
#18850=CARTESIAN_POINT ( 'NONE',  ( -0.8070866141732276899, -0.5400638737290844871, 0.3530559997133364547 ) ) ;
#18851=CARTESIAN_POINT ( 'NONE',  ( -1.200787401574802349, 0.1660481256975883668, -0.3530559997133364547 ) ) ;
#18853=CARTESIAN_POINT ( 'NONE',  ( 0.8989501312335963501, -0.5511811023622048555, -0.09757992244046775898 ) ) ;
#18854=CARTESIAN_POINT ( 'NONE',  ( -0.4265091863517051496, 0.1771653543307087075, -0.09757992244046823083 ) ) ;
#18855=CARTESIAN_POINT ( 'NONE',  ( 0.7677165354330716118, 0.07958543189024071263, -0.2665933059059888421 ) ) ;
#18856=CARTESIAN_POINT ( 'NONE',  ( -1.614173228346456268, -0.6692913385826771977, 8.415575281601705876E-17 ) ) ;
#18857=CARTESIAN_POINT ( 'NONE',  ( 1.384514435695538337, -0.6692913385826771977, 0.1292274648535927661 ) ) ;
#18858=CARTESIAN_POINT ( 'NONE',  ( 0.7020997375328090762, -0.2845877964562159024, 0.3641732283464567677 ) ) ;
#18859=CARTESIAN_POINT ( 'NONE',  ( -0.9120734908136475250, -0.6692913385826773087, -0.1292274648535924053 ) ) ;
#18860=CARTESIAN_POINT ( 'NONE',  ( 1.194225721784777594, -0.4281496062992127816, -0.4176697321401328100 ) ) ;
#18862=CARTESIAN_POINT ( 'NONE',  ( -0.1706036745406816491, -0.004921259842519870586, -0.3153832671262229437 ) ) ;
#18863=DIRECTION ( 'NONE',  ( 0.000000000000000000, 1.000000000000000000, 0.000000000000000000 ) ) ;
#18864=CARTESIAN_POINT ( 'NONE',  ( 0.1640419947506569498, -0.3162353388693409650, -0.4822834645669289433 ) ) ;
#18865=CARTESIAN_POINT ( 'NONE',  ( 0.6824146981627303710, 0.2306618581243847221, -0.2411417322834647770 ) ) ;
#18866=CARTESIAN_POINT ( 'NONE',  ( 0.9908136482939640111, 0.1771653543307087075, -0.09757992244046823083 ) ) ;
#18867=CARTESIAN_POINT ( 'NONE',  ( 0.2821522309711292364, -0.5511811023622046335, 0.09757992244046803654 ) ) ;
#18868=CARTESIAN_POINT ( 'NONE',  ( -1.351706036745406347, 0.05413385826771626580, -0.4176697321401330321 ) ) ;
#18869=CARTESIAN_POINT ( 'NONE',  ( -0.6955380577427815458, -0.004921259842519576551, 0.3153832671262227771 ) ) ;
#18870=FACE_OUTER_BOUND ( 'NONE', #62194, .T. ) ;
#18871=CARTESIAN_POINT ( 'NONE',  ( -1.115485564304461219, -0.4281496062992124485, 0.4176697321401328655 ) ) ;
#18872=CARTESIAN_POINT ( 'NONE',  ( -0.5708661417322825615, -0.5400638737290844871, 0.3530559997133364547 ) ) ;
#18875=CARTESIAN_POINT ( 'NONE',  ( 0.5774278215223103139, -0.5023911411419708095, -0.1820866141732282451 ) ) ;
#18876=CARTESIAN_POINT ( 'NONE',  ( -0.1771653543307080136, 0.1660481256975883668, -0.3530559997133364547 ) ) ;
#18877=CARTESIAN_POINT ( 'NONE',  ( -0.6233595800524928121, -0.3162353388693409650, -0.4822834645669289433 ) ) ;
#18878=CARTESIAN_POINT ( 'NONE',  ( -0.7611548556430438595, -0.5023911411419708095, -0.1820866141732282451 ) ) ;
#18880=CARTESIAN_POINT ( 'NONE',  ( 8.195543980992789655E-16, -0.1870078740157480879, -0.4822834645669291653 ) ) ;
#18881=CARTESIAN_POINT ( 'NONE',  ( -1.712598425196849572, 0.07958543189024085140, 0.2665933059059887866 ) ) ;
#18882=CARTESIAN_POINT ( 'NONE',  ( 1.305774278215223960, 0.2952755905511810774, -0.1292274648535930714 ) ) ;
#18885=VERTEX_POINT ( 'NONE', #77156 ) ;
#18886=CARTESIAN_POINT ( 'NONE',  ( -0.7443564561544175895, 1.971400176368010237, 0.5309055118110236338 ) ) ;
#18887=CARTESIAN_POINT ( 'NONE',  ( -1.332020997375327642, -0.3162353388693409650, -0.4822834645669289433 ) ) ;
#18888=CARTESIAN_POINT ( 'NONE',  ( -0.9711286089238838626, -0.6046776061558807314, 0.2411417322834647770 ) ) ;
#18889=CARTESIAN_POINT ( 'NONE',  ( -1.653543307086613234, -0.1870078740157479769, 0.4822834645669291653 ) ) ;
#18892=CARTESIAN_POINT ( 'NONE',  ( 0.9514435695538062676, -0.3162353388693409650, -0.4822834645669289433 ) ) ;
#18893=CARTESIAN_POINT ( 'NONE',  ( 0.06561679790026316017, -0.4281496062992124485, 0.4176697321401328655 ) ) ;
#18894=DIRECTION ( 'NONE',  ( -3.096699300667737957E-16, 1.000000000000000000, -0.000000000000000000 ) ) ;
#18895=CARTESIAN_POINT ( 'NONE',  ( -0.6692913385826764205, 0.2952755905511811885, 0.000000000000000000 ) ) ;
#18896=CARTESIAN_POINT ( 'NONE',  ( 1.253280839895013710, -0.2845877964562159024, 0.3641732283464567677 ) ) ;
#18898=VERTEX_POINT ( 'NONE', #19488 ) ;
#18901=CARTESIAN_POINT ( 'NONE',  ( 0.6102362204724416372, -0.5400638737290844871, 0.3530559997133364547 ) ) ;
#18902=CARTESIAN_POINT ( 'NONE',  ( -0.6036745406824141069, 0.2306618581243848609, 0.2411417322834645549 ) ) ;
#18903=CARTESIAN_POINT ( 'NONE',  ( -1.574803149606298192, -0.1870078740157480879, -0.4822834645669291653 ) ) ;
#18904=CARTESIAN_POINT ( 'NONE',  ( 0.7611548556430454138, 0.2306618581243847221, -0.2411417322834647770 ) ) ;
#18905=CARTESIAN_POINT ( 'NONE',  ( 1.614173228346457378, -0.6692913385826771977, 8.415575281601705876E-17 ) ) ;
#18906=CARTESIAN_POINT ( 'NONE',  ( 1.364829396325459854, -0.6046776061558809534, -0.2411417322834644161 ) ) ;
#18907=CARTESIAN_POINT ( 'NONE',  ( -0.01312335958005186876, 0.05413385826771626580, -0.4176697321401330321 ) ) ;
#18908=CARTESIAN_POINT ( 'NONE',  ( -1.404199475065615932, -0.4281496062992127816, -0.4176697321401328100 ) ) ;
#18909=CARTESIAN_POINT ( 'NONE',  ( 1.437007874015748810, 0.1660481256975885056, 0.3530559997133364547 ) ) ;
#18910=CARTESIAN_POINT ( 'NONE',  ( 1.581364829396326277, -0.3162353388693409650, -0.4822834645669289433 ) ) ;
#18911=( BOUNDED_CURVE ( )  B_SPLINE_CURVE ( 2, ( #62863, #63681, #38003, #82636, #30456, #11937, #43480, #75507, #17846, #5606, #69992, #70407, #69176 ),
 .UNSPECIFIED., .F., .F. ) 
 B_SPLINE_CURVE_WITH_KNOTS ( ( 3, 2, 2, 2, 2, 2, 3 ),
 ( 0.6278765491802553722, 0.6287878787878787845, 0.6325757575757575690, 0.6363636363636363535, 0.6401515151515151381, 0.6439393939393939226, 0.6448507235470174459 ),
 .UNSPECIFIED. ) 
 CURVE ( )  GEOMETRIC_REPRESENTATION_ITEM ( )  RATIONAL_B_SPLINE_CURVE ( ( 0.9875488213027523443, 0.9918020599134680371, 1.000000000000000000, 0.9659258262890683122, 1.000000000000000000, 0.9659258262890683122, 1.000000000000000000, 0.9659258262890683122, 1.000000000000000000, 0.9659258262890683122, 1.000000000000000000, 0.9918020599134671489, 0.9875488213027514561 ) ) 
 REPRESENTATION_ITEM ( '' )  );
#18913=CARTESIAN_POINT ( 'NONE',  ( 0.8661417322834653598, -0.1870078740157479769, 0.3641732283464567677 ) ) ;
#18914=ORIENTED_EDGE ( 'NONE', *, *, #68203, .T. ) ;
#18917=CARTESIAN_POINT ( 'NONE',  ( 0.01968503937007930540, 0.07958543189024085140, 0.2665933059059887866 ) ) ;
#18919=CARTESIAN_POINT ( 'NONE',  ( 0.04593175853018440641, 0.2952755905511810774, -0.1292274648535930714 ) ) ;
#18920=CARTESIAN_POINT ( 'NONE',  ( -0.09842519685039295696, 0.1660481256975883668, -0.3530559997133364547 ) ) ;
#18922=CARTESIAN_POINT ( 'NONE',  ( -0.7545931758530177724, 0.2952755905511811885, 0.1292274648535926551 ) ) ;
#18924=CARTESIAN_POINT ( 'NONE',  ( -1.167979002624671470, 0.05413385826771666132, 0.4176697321401328100 ) ) ;
#18926=CARTESIAN_POINT ( 'NONE',  ( 1.154855643044620184, 0.1283753931104746893, -0.1820866141732285504 ) ) ;
#18927=CARTESIAN_POINT ( 'NONE',  ( 1.010498687664042716, -0.4281496062992124485, 0.4176697321401328655 ) ) ;
#18928=CARTESIAN_POINT ( 'NONE',  ( 0.5708661417322842269, 0.1660481256975885056, 0.3530559997133364547 ) ) ;
#18931=CARTESIAN_POINT ( 'NONE',  ( -1.148293963254592542, -0.6692913385826773087, -0.1292274648535924053 ) ) ;
#18934=CARTESIAN_POINT ( 'NONE',  ( -0.06561679790026180015, -0.4281496062992127816, -0.4176697321401328100 ) ) ;
#18937=CARTESIAN_POINT ( 'NONE',  ( 1.423884514435696191, -0.05778040916215522460, 0.4822834645669289988 ) ) ;
#18938=CARTESIAN_POINT ( 'NONE',  ( 1.371391076115485941, 0.2952755905511811885, 0.1292274648535926551 ) ) ;
#18939=CARTESIAN_POINT ( 'NONE',  ( 0.3543307086614181922, -0.5511811023622047445, 6.969142054262312111E-17 ) ) ;
#18940=CARTESIAN_POINT ( 'NONE',  ( 0.8923884514435701520, -0.6046776061558809534, -0.2411417322834644161 ) ) ;
#18942=CARTESIAN_POINT ( 'NONE',  ( 0.3083989501312343062, -0.08942795157528024563, -0.3641732283464568787 ) ) ;
#18943=CARTESIAN_POINT ( 'NONE',  ( 0.5249343832021003964, 0.2306618581243847221, -0.2411417322834647770 ) ) ;
#18945=CARTESIAN_POINT ( 'NONE',  ( -1.318897637795274802, -0.5400638737290845981, -0.3530559997133363437 ) ) ;
#18946=CARTESIAN_POINT ( 'NONE',  ( 0.9055118110236227702, -0.5511811023622047445, 6.969142054262312111E-17 ) ) ;
#18948=CARTESIAN_POINT ( 'NONE',  ( -1.161417322834644716, 0.1660481256975885056, 0.3530559997133364547 ) ) ;
#18949=CARTESIAN_POINT ( 'NONE',  ( -0.2559055118110230564, 0.1660481256975883668, -0.3530559997133364547 ) ) ;
#18950=CARTESIAN_POINT ( 'NONE',  ( -0.2362204724409440182, -0.1870078740157479769, 0.3641732283464567677 ) ) ;
#18952=CARTESIAN_POINT ( 'NONE',  ( -0.1509186351706028884, -0.05778040916215522460, 0.4822834645669289988 ) ) ;
#18953=CARTESIAN_POINT ( 'NONE',  ( 0.1443569553805781891, -0.3690944881889763329, 0.3153832671262228327 ) ) ;
#18955=CARTESIAN_POINT ( 'NONE',  ( 0.02624671916010564918, -0.6046776061558809534, -0.2411417322834644161 ) ) ;
#18956=CARTESIAN_POINT ( 'NONE',  ( 1.364829396325460076, 0.1283753931104748280, 0.1820866141732283561 ) ) ;
#18957=CARTESIAN_POINT ( 'NONE',  ( -0.1685779992553458895, 5.625543525484885637E-15, -0.3954974714151418547 ) ) ;
#18958=CARTESIAN_POINT ( 'NONE',  ( -0.9383202099737524282, -0.08942795157527998196, 0.3641732283464567121 ) ) ;
#18959=CARTESIAN_POINT ( 'NONE',  ( -0.6167979002624665030, -0.004921259842519576551, 0.3153832671262227771 ) ) ;
#18960=CARTESIAN_POINT ( 'NONE',  ( -0.1049868766404193215, -0.6046776061558807314, 0.2411417322834647770 ) ) ;
#18961=CARTESIAN_POINT ( 'NONE',  ( -0.2034120734908131112, -0.6692913385826773087, -0.1292274648535924053 ) ) ;
#18962=CARTESIAN_POINT ( 'NONE',  ( 0.9251968503937015864, 0.07958543189024071263, -0.2665933059059888421 ) ) ;
#18963=CARTESIAN_POINT ( 'NONE',  ( -1.732283464566928277, -0.1870078740157479769, 0.3641732283464567677 ) ) ;
#18964=CARTESIAN_POINT ( 'NONE',  ( -1.666666666666665853, 0.05413385826771626580, -0.4176697321401330321 ) ) ;
#18965=CARTESIAN_POINT ( 'NONE',  ( 0.8267716535433078384, -0.6692913385826771977, 8.415575281601705876E-17 ) ) ;
#18967=CARTESIAN_POINT ( 'NONE',  ( -0.4593175853018366950, 0.05413385826771666132, 0.4176697321401328100 ) ) ;
#18969=CARTESIAN_POINT ( 'NONE',  ( -1.325459317585300889, -0.4281496062992127816, -0.4176697321401328100 ) ) ;
#18970=CARTESIAN_POINT ( 'NONE',  ( 0.9120734908136490793, 0.2952755905511810774, -0.1292274648535930714 ) ) ;
#18971=CARTESIAN_POINT ( 'NONE',  ( 0.4593175853018380828, 0.05413385826771626580, -0.4176697321401330321 ) ) ;
#18973=CARTESIAN_POINT ( 'NONE',  ( 0.5708661417322842269, 0.07958543189024085140, 0.2665933059059887866 ) ) ;
#18974=CARTESIAN_POINT ( 'NONE',  ( 1.351706036745407680, 0.05413385826771666132, 0.4176697321401328100 ) ) ;
#18975=CARTESIAN_POINT ( 'NONE',  ( -0.4921259842519677963, -0.4536011799217367080, 0.2665933059059888421 ) ) ;
#18976=CARTESIAN_POINT ( 'NONE',  ( -0.6496062992125976043, 0.1660481256975883668, -0.3530559997133364547 ) ) ;
#18977=CARTESIAN_POINT ( 'NONE',  ( 0.8070866141732288002, 0.1660481256975885056, 0.3530559997133364547 ) ) ;
#18978=CARTESIAN_POINT ( 'NONE',  ( 0.3412073490813655186, 0.2306618581243848609, 0.2411417322834645549 ) ) ;
#18979=CARTESIAN_POINT ( 'NONE',  ( -0.5839895013123351797, -0.6692913385826771977, 0.1292274648535927661 ) ) ;
#18980=CARTESIAN_POINT ( 'NONE',  ( -0.5446194225721777693, -0.2845877964562161244, -0.3641732283464567121 ) ) ;
#18982=CARTESIAN_POINT ( 'NONE',  ( 0.2952755905511816326, -0.5400638737290844871, 0.3530559997133364547 ) ) ;
#18983=CARTESIAN_POINT ( 'NONE',  ( -1.062992125984250968, 0.2952755905511811885, 0.000000000000000000 ) ) ;
#18984=CARTESIAN_POINT ( 'NONE',  ( -0.5511811023622038563, -0.1870078740157479769, 0.4822834645669291653 ) ) ;
#18987=CARTESIAN_POINT ( 'NONE',  ( 1.181102362204724976, -0.1870078740157480879, -0.4822834645669291653 ) ) ;
#18988=CARTESIAN_POINT ( 'NONE',  ( 1.384514435695538559, 0.2952755905511810774, -0.1292274648535930714 ) ) ;
#18991=CARTESIAN_POINT ( 'NONE',  ( -0.8136482939632537770, -0.6046776061558807314, 0.2411417322834647770 ) ) ;
#18994=EDGE_LOOP ( 'NONE', ( #23083, #37151, #14185, #55885 ) ) ;
#18995=CARTESIAN_POINT ( 'NONE',  ( -0.1312335958005241554, -0.5023911411419708095, -0.1820866141732282451 ) ) ;
#18997=CARTESIAN_POINT ( 'NONE',  ( 0.8202099737532813073, 0.2952755905511811885, 0.1292274648535926551 ) ) ;
#18999=DIRECTION ( 'NONE',  ( -3.096699300667737957E-16, 1.000000000000000000, -0.000000000000000000 ) ) ;
#19000=CARTESIAN_POINT ( 'NONE',  ( -0.4199475065616791736, -0.5023911411419708095, 0.1820866141732285504 ) ) ;
#19002=CARTESIAN_POINT ( 'NONE',  ( 1.141732283464567788, -0.6692913385826771977, 8.415575281601705876E-17 ) ) ;
#19003=CARTESIAN_POINT ( 'NONE',  ( 0.9908136482939640111, 0.1771653543307087075, -0.09757992244046823083 ) ) ;
#19004=CARTESIAN_POINT ( 'NONE',  ( 0.1640419947506569498, -0.3162353388693409650, -0.4822834645669289433 ) ) ;
#19006=CARTESIAN_POINT ( 'NONE',  ( -0.3149606299212590610, -0.1870078740157480879, -0.4822834645669291653 ) ) ;
#19007=CARTESIAN_POINT ( 'NONE',  ( -1.122047244094487306, -0.4536011799217367080, 0.2665933059059888421 ) ) ;
#19008=EDGE_CURVE ( 'NONE', #27226, #34463, #561, .T. ) ;
#19009=CARTESIAN_POINT ( 'NONE',  ( -0.4986876640419942164, -0.6046776061558807314, 0.2411417322834647770 ) ) ;
#19010=FACE_OUTER_BOUND ( 'NONE', #56271, .T. ) ;
#19014=CARTESIAN_POINT ( 'NONE',  ( 0.4133858267716541968, 0.1660481256975885056, 0.3530559997133364547 ) ) ;
#19016=CARTESIAN_POINT ( 'NONE',  ( -0.6233595800524928121, -0.05778040916215522460, 0.4822834645669289988 ) ) ;
#19017=CARTESIAN_POINT ( 'NONE',  ( 1.509186351706037543, -0.4281496062992127816, -0.4176697321401328100 ) ) ;
#19018=CARTESIAN_POINT ( 'NONE',  ( 0.7086614173228352742, -0.1870078740157480879, -0.4822834645669291653 ) ) ;
#19019=EDGE_CURVE ( 'NONE', #16885, #38903, #42576, .T. ) ;
#19020=CARTESIAN_POINT ( 'NONE',  ( 0.08530183727034192087, -0.05778040916215522460, 0.4822834645669289988 ) ) ;
#19022=CARTESIAN_POINT ( 'NONE',  ( -0.8267716535433065062, -0.6692913385826771977, 8.415575281601705876E-17 ) ) ;
#19023=CARTESIAN_POINT ( 'NONE',  ( -0.09842519685039295696, -0.5400638737290844871, 0.3530559997133364547 ) ) ;
#19024=CARTESIAN_POINT ( 'NONE',  ( -1.076115485564303809, -0.6046776061558809534, -0.2411417322834644161 ) ) ;
#19025=CARTESIAN_POINT ( 'NONE',  ( 0.04593175853018440641, -0.5511811023622046335, 0.09757992244046803654 ) ) ;
#19027=CARTESIAN_POINT ( 'NONE',  ( -0.1968503937007867743, -0.6692913385826771977, 8.415575281601705876E-17 ) ) ;
#19028=CARTESIAN_POINT ( 'NONE',  ( 2.787279214012418738, 0.000000000000000000, 0.000000000000000000 ) ) ;
#19029=CARTESIAN_POINT ( 'NONE',  ( 1.292650918635171564, 0.2952755905511811885, 0.1292274648535926551 ) ) ;
#19032=EDGE_LOOP ( 'NONE', ( #25530, #80113, #52258, #80232 ) ) ;
#19033=CARTESIAN_POINT ( 'NONE',  ( 0.09842519685039434474, 0.1660481256975885056, 0.3530559997133364547 ) ) ;
#19034=CARTESIAN_POINT ( 'NONE',  ( -0.4658792650918627265, -0.08942795157527998196, 0.3641732283464567121 ) ) ;
#19035=CARTESIAN_POINT ( 'NONE',  ( 1.581364829396326277, -0.2845877964562161244, -0.3641732283464567121 ) ) ;
#19040=CARTESIAN_POINT ( 'NONE',  ( 1.555118110236221041, -0.5400638737290844871, 0.3530559997133364547 ) ) ;
#19042=CARTESIAN_POINT ( 'NONE',  ( 0.4724409448818904789, -0.1870078740157479769, 0.4822834645669291653 ) ) ;
#19043=CARTESIAN_POINT ( 'NONE',  ( -1.049868766404198794, -0.6046776061558807314, 0.2411417322834647770 ) ) ;
#19044=CARTESIAN_POINT ( 'NONE',  ( -0.9908136482939626788, -0.6692913385826773087, -0.1292274648535924053 ) ) ;
#19045=CARTESIAN_POINT ( 'NONE',  ( 0.2034120734908142214, 0.2952755905511810774, -0.1292274648535930714 ) ) ;
#19047=CARTESIAN_POINT ( 'NONE',  ( -1.496062992125983815, -0.1870078740157479769, 0.3641732283464567677 ) ) ;
#19048=CARTESIAN_POINT ( 'NONE',  ( 0.8464566929133865436, 0.1660481256975883668, -0.3530559997133364547 ) ) ;
#19049=CARTESIAN_POINT ( 'NONE',  ( 1.325459317585302665, -0.3690944881889763329, 0.3153832671262228327 ) ) ;
#19050=CARTESIAN_POINT ( 'NONE',  ( 1.220472440944881942, 2.401574803149606474, -0.5309055118110238558 ) ) ;
#19051=CARTESIAN_POINT ( 'NONE',  ( 0.7086614173228353852, -0.1870078740157479769, 0.3641732283464567677 ) ) ;
#19052=CARTESIAN_POINT ( 'NONE',  ( -1.240157480314959759, -0.5400638737290845981, -0.3530559997133363437 ) ) ;
#19054=CARTESIAN_POINT ( 'NONE',  ( 1.122047244094488860, -0.5400638737290845981, -0.3530559997133363437 ) ) ;
#19056=CARTESIAN_POINT ( 'NONE',  ( 0.5774278215223104249, 0.2306618581243848609, 0.2411417322834645549 ) ) ;
#19058=CARTESIAN_POINT ( 'NONE',  ( -1.640419947506561060, -0.3690944881889765550, -0.3153832671262227771 ) ) ;
#19059=CARTESIAN_POINT ( 'NONE',  ( 0.1049868766404206816, 0.2306618581243848609, 0.2411417322834645549 ) ) ;
#19060=CARTESIAN_POINT ( 'NONE',  ( 0.8398950131233602345, 0.1283753931104746893, -0.1820866141732285504 ) ) ;
#19061=CARTESIAN_POINT ( 'NONE',  ( 0.8595800524934390507, -0.3162353388693405765, 0.4822834645669290543 ) ) ;
#19063=CARTESIAN_POINT ( 'NONE',  ( -0.7086614173228339419, -0.1870078740157480601, -0.3641732283464567677 ) ) ;
#19064=CARTESIAN_POINT ( 'NONE',  ( -0.7545931758530177724, 0.2952755905511811885, 0.1292274648535926551 ) ) ;
#19065=CARTESIAN_POINT ( 'NONE',  ( 1.561679790026247350, 0.05413385826771626580, -0.4176697321401330321 ) ) ;
#19066=CARTESIAN_POINT ( 'NONE',  ( -1.102362204724408601, -0.1870078740157479769, 0.4822834645669291653 ) ) ;
#19067=CARTESIAN_POINT ( 'NONE',  ( 1.023622047244095334, -0.1870078740157479769, 0.4822834645669291653 ) ) ;
#19069=CARTESIAN_POINT ( 'NONE',  ( -1.535433070866141225, -0.5511811023622047445, 6.969142054262312111E-17 ) ) ;
#19071=CARTESIAN_POINT ( 'NONE',  ( 0.9251968503937015864, -0.5400638737290844871, 0.3530559997133364547 ) ) ;
#19073=CARTESIAN_POINT ( 'NONE',  ( -1.555118110236219930, 0.1660481256975885056, 0.3530559997133364547 ) ) ;
#19074=CARTESIAN_POINT ( 'NONE',  ( -1.345144356955379816, -0.2845877964562159024, 0.3641732283464567677 ) ) ;
#19075=CARTESIAN_POINT ( 'NONE',  ( -1.220472440944881054, 0.1771653543307087630, 0.000000000000000000 ) ) ;
#19076=CARTESIAN_POINT ( 'NONE',  ( 1.620734908136483465, -0.5511811023622046335, 0.09757992244046803654 ) ) ;
#19077=CARTESIAN_POINT ( 'NONE',  ( -0.4658792650918627265, -0.3162353388693409650, -0.4822834645669289433 ) ) ;
#19078=CARTESIAN_POINT ( 'NONE',  ( -0.3674540682414689785, 0.1283753931104748280, 0.1820866141732283561 ) ) ;
#19079=CARTESIAN_POINT ( 'NONE',  ( -1.535433070866141225, 0.1771653543307087630, 0.000000000000000000 ) ) ;
#19080=CARTESIAN_POINT ( 'NONE',  ( 1.115485564304462551, -0.004921259842519576551, 0.3153832671262227771 ) ) ;
#19081=CARTESIAN_POINT ( 'NONE',  ( 1.003937007874016407, -0.5400638737290844871, 0.3530559997133364547 ) ) ;
#19082=CARTESIAN_POINT ( 'NONE',  ( 1.371391076115485719, -0.6692913385826773087, -0.1292274648535924053 ) ) ;
#19083=CARTESIAN_POINT ( 'NONE',  ( -0.1115485564304453947, -0.5511811023622046335, 0.09757992244046803654 ) ) ;
#19084=EDGE_CURVE ( 'NONE', #17596, #69360, #65097, .T. ) ;
#19085=CARTESIAN_POINT ( 'NONE',  ( 0.3937007874015754361, -0.1870078740157479769, 0.4822834645669291653 ) ) ;
#19086=CARTESIAN_POINT ( 'NONE',  ( 0.5577427821522314977, -0.2845877964562161244, -0.3641732283464567121 ) ) ;
#19087=CARTESIAN_POINT ( 'NONE',  ( 1.443569553805774897, 0.2306618581243848609, 0.2411417322834645549 ) ) ;
#19088=CARTESIAN_POINT ( 'NONE',  ( -1.496062992125983815, -0.1870078740157479769, 0.4822834645669291653 ) ) ;
#19089=CARTESIAN_POINT ( 'NONE',  ( -0.4921259842519677963, -0.5400638737290844871, 0.3530559997133364547 ) ) ;
#19092=CARTESIAN_POINT ( 'NONE',  ( 0.3805774278215230400, 0.05413385826771626580, -0.4176697321401330321 ) ) ;
#19093=CARTESIAN_POINT ( 'NONE',  ( 1.167979002624672580, -0.004921259842519870586, -0.3153832671262229437 ) ) ;
#19094=CARTESIAN_POINT ( 'NONE',  ( -0.5643044619422565855, -0.4281496062992124485, 0.4176697321401328655 ) ) ;
#19095=CARTESIAN_POINT ( 'NONE',  ( 0.5118110236220478892, 0.2952755905511811885, 0.000000000000000000 ) ) ;
#19099=CARTESIAN_POINT ( 'NONE',  ( -0.4848604877838266214, -2.609869883881465018E-15, -0.3464511005275220379 ) ) ;
#19101=CARTESIAN_POINT ( 'NONE',  ( -1.056430446194224881, 0.1771653543307087075, -0.09757992244046823083 ) ) ;
#19102=CARTESIAN_POINT ( 'NONE',  ( -1.141732283464566011, -0.6692913385826771977, 8.415575281601705876E-17 ) ) ;
#19105=CARTESIAN_POINT ( 'NONE',  ( 0.9120734908136490793, 0.2952755905511810774, -0.1292274648535930714 ) ) ;
#19106=CARTESIAN_POINT ( 'NONE',  ( 1.430446194225722500, 0.05413385826771666132, 0.4176697321401328100 ) ) ;
#19107=CARTESIAN_POINT ( 'NONE',  ( 0.9055118110236227702, -0.6692913385826771977, 8.415575281601705876E-17 ) ) ;
#19110=CARTESIAN_POINT ( 'NONE',  ( 1.522309711286089939, 0.2306618581243848609, 0.2411417322834645549 ) ) ;
#19111=CARTESIAN_POINT ( 'NONE',  ( 0.5380577427821529035, 0.05413385826771626580, -0.4176697321401330321 ) ) ;
#19112=CARTESIAN_POINT ( 'NONE',  ( 0.5511811023622054106, -0.1870078740157480879, -0.4822834645669291653 ) ) ;
#19113=CARTESIAN_POINT ( 'NONE',  ( 0.7152230971128614723, -0.2845877964562161244, -0.3641732283464567121 ) ) ;
#19114=CARTESIAN_POINT ( 'NONE',  ( 1.187664041994751285, -0.05778040916215522460, 0.4822834645669289988 ) ) ;
#19116=CARTESIAN_POINT ( 'NONE',  ( 0.5052493438320215802, 0.2952755905511811885, 0.1292274648535926551 ) ) ;
#19117=CARTESIAN_POINT ( 'NONE',  ( 1.154855643044620184, -0.6046776061558807314, 0.2411417322834647770 ) ) ;
#19118=CARTESIAN_POINT ( 'NONE',  ( 0.2034120734908144990, -0.6692913385826771977, 0.1292274648535927661 ) ) ;
#19119=CARTESIAN_POINT ( 'NONE',  ( 1.272965879265092637, -0.3690944881889765550, -0.3153832671262227771 ) ) ;
#19120=CARTESIAN_POINT ( 'NONE',  ( -0.7217847769028863381, 0.05413385826771626580, -0.4176697321401330321 ) ) ;
#19121=CARTESIAN_POINT ( 'NONE',  ( -1.128608923884513837, -0.6046776061558807314, 0.2411417322834647770 ) ) ;
#19122=CARTESIAN_POINT ( 'NONE',  ( 1.135170603674541256, 0.2952755905511811885, 0.1292274648535926551 ) ) ;
#19126=ORIENTED_EDGE ( 'NONE', *, *, #73907, .F. ) ;
#19129=CARTESIAN_POINT ( 'NONE',  ( 1.666666666666667185, 0.05413385826771666132, 0.4176697321401328100 ) ) ;
#19130=CARTESIAN_POINT ( 'NONE',  ( 1.233595800524935227, -0.5023911411419708095, 0.1820866141732285504 ) ) ;
#19132=CARTESIAN_POINT ( 'NONE',  ( 1.286089238845145033, -0.5023911411419708095, -0.1820866141732282451 ) ) ;
#19137=CARTESIAN_POINT ( 'NONE',  ( -0.7349081364829387342, -0.5023911411419708095, 0.1820866141732285504 ) ) ;
#19138=CARTESIAN_POINT ( 'NONE',  ( 1.607611548556431069, 0.2952755905511811885, 0.1292274648535926551 ) ) ;
#19139=CARTESIAN_POINT ( 'NONE',  ( -1.213910761154854745, -0.6692913385826771977, 0.1292274648535927661 ) ) ;
#19140=CARTESIAN_POINT ( 'NONE',  ( 0.1312335958005255154, -0.6046776061558807314, 0.2411417322834647770 ) ) ;
#19141=CARTESIAN_POINT ( 'NONE',  ( 1.318897637795276356, 0.1660481256975883668, -0.3530559997133364547 ) ) ;
#19147=CARTESIAN_POINT ( 'NONE',  ( -0.5905511811023613777, -0.5511811023622047445, 6.969142054262312111E-17 ) ) ;
#19148=CARTESIAN_POINT ( 'NONE',  ( -1.194225721784776262, -0.4281496062992124485, 0.4176697321401328655 ) ) ;
#19149=CARTESIAN_POINT ( 'NONE',  ( 1.017060367454068803, -0.3162353388693405765, 0.4822834645669290543 ) ) ;
#19153=CARTESIAN_POINT ( 'NONE',  ( 1.135170603674541256, -0.6692913385826773087, -0.1292274648535924053 ) ) ;
#19154=CARTESIAN_POINT ( 'NONE',  ( -1.154855643044618851, -0.6046776061558809534, -0.2411417322834644161 ) ) ;
#19157=CARTESIAN_POINT ( 'NONE',  ( -0.5774278215223089816, 0.1283753931104746893, -0.1820866141732285504 ) ) ;
#19159=CARTESIAN_POINT ( 'NONE',  ( -0.4724409448818890911, -0.1870078740157480601, -0.3641732283464567677 ) ) ;
#19160=CARTESIAN_POINT ( 'NONE',  ( 0.05905511811023681640, 0.07958543189024071263, -0.2665933059059888421 ) ) ;
#19161=CARTESIAN_POINT ( 'NONE',  ( -0.03280839895013062252, -0.6692913385826771977, 0.1292274648535927661 ) ) ;
#19162=CARTESIAN_POINT ( 'NONE',  ( -1.318897637795274802, 0.07958543189024085140, 0.2665933059059887866 ) ) ;
#19164=CARTESIAN_POINT ( 'NONE',  ( 1.332020997375328974, -0.05778040916215560624, -0.4822834645669293319 ) ) ;
#19167=CARTESIAN_POINT ( 'NONE',  ( -1.364829396325458521, -0.6046776061558807314, 0.2411417322834647770 ) ) ;
#19169=CARTESIAN_POINT ( 'NONE',  ( -0.2559055118110230564, 0.1660481256975883668, -0.3530559997133364547 ) ) ;
#19170=CARTESIAN_POINT ( 'NONE',  ( -0.7742782152230962556, -0.4281496062992127816, -0.4176697321401328100 ) ) ;
#19171=CARTESIAN_POINT ( 'NONE',  ( 0.7349081364829403995, 0.1283753931104748280, 0.1820866141732283561 ) ) ;
#19172=CARTESIAN_POINT ( 'NONE',  ( -0.1968503937007867743, -0.5511811023622047445, 6.969142054262312111E-17 ) ) ;
#19173=CARTESIAN_POINT ( 'NONE',  ( -0.7545931758530177724, 0.2952755905511811885, 0.1292274648535926551 ) ) ;
#19174=CARTESIAN_POINT ( 'NONE',  ( -1.036745406824146176, -0.4281496062992124485, 0.4176697321401328655 ) ) ;
#19176=CARTESIAN_POINT ( 'NONE',  ( 1.332020997375329197, -0.2845877964562159024, 0.3641732283464567677 ) ) ;
#19177=CARTESIAN_POINT ( 'NONE',  ( -0.2821522309711278487, -0.6692913385826773087, -0.1292274648535924053 ) ) ;
#19178=CARTESIAN_POINT ( 'NONE',  ( -1.371391076115484831, 0.2952755905511810774, -0.1292274648535930714 ) ) ;
#19181=CARTESIAN_POINT ( 'NONE',  ( -0.8595800524934373854, -0.08942795157527998196, 0.3641732283464567121 ) ) ;
#19182=CARTESIAN_POINT ( 'NONE',  ( 0.6430446194225728496, 0.05413385826771666132, 0.4176697321401328100 ) ) ;
#19183=CARTESIAN_POINT ( 'NONE',  ( -0.8858267716535425107, 0.07958543189024071263, -0.2665933059059888421 ) ) ;
#19185=CARTESIAN_POINT ( 'NONE',  ( -0.8005249343832013809, -0.4281496062992124485, 0.4176697321401328655 ) ) ;
#19186=CARTESIAN_POINT ( 'NONE',  ( 0.7677165354330716118, 0.1660481256975883668, -0.3530559997133364547 ) ) ;
#19187=CARTESIAN_POINT ( 'NONE',  ( 0.6824146981627303710, -0.6046776061558807314, 0.2411417322834647770 ) ) ;
#19189=CARTESIAN_POINT ( 'NONE',  ( -1.450131233595799651, -0.5511811023622046335, 0.09757992244046803654 ) ) ;
#19195=CARTESIAN_POINT ( 'NONE',  ( 1.128608923884515169, -0.5023911411419708095, -0.1820866141732282451 ) ) ;
#19196=CARTESIAN_POINT ( 'NONE',  ( 0.8398950131233602345, 0.1283753931104746893, -0.1820866141732285504 ) ) ;
#19197=CARTESIAN_POINT ( 'NONE',  ( 0.2296587926509192634, -0.05778040916215560624, -0.4822834645669293319 ) ) ;
#19200=CARTESIAN_POINT ( 'NONE',  ( 0.3477690288713918276, -0.5511811023622048555, -0.09757992244046775898 ) ) ;
#19201=CARTESIAN_POINT ( 'NONE',  ( -0.8070866141732276899, 0.1660481256975883668, -0.3530559997133364547 ) ) ;
#19202=CARTESIAN_POINT ( 'NONE',  ( -1.391076115485563314, -0.6046776061558809534, -0.2411417322834644161 ) ) ;
#19203=CARTESIAN_POINT ( 'NONE',  ( 0.6955380577427828781, -0.4281496062992124485, 0.4176697321401328655 ) ) ;
#19205=CARTESIAN_POINT ( 'NONE',  ( -0.7283464566929126471, 0.1660481256975883391, -0.3530559997133364547 ) ) ;
#19208=AXIS2_PLACEMENT_3D ( 'NONE', #53461, #80004, #52624 ) ;
#19209=CARTESIAN_POINT ( 'NONE',  ( -1.450131233595799651, -0.6692913385826771977, 0.1292274648535927661 ) ) ;
#19210=CARTESIAN_POINT ( 'NONE',  ( -0.6627296587926501115, 0.2952755905511810774, -0.1292274648535930714 ) ) ;
#19211=CARTESIAN_POINT ( 'NONE',  ( -0.9448818897637790704, -0.1870078740157480601, -0.3641732283464567677 ) ) ;
#19212=CARTESIAN_POINT ( 'NONE',  ( -0.8530183727034112984, 0.05413385826771666132, 0.4176697321401328100 ) ) ;
#19215=CARTESIAN_POINT ( 'NONE',  ( 1.443569553805774897, -0.6046776061558809534, -0.2411417322834644161 ) ) ;
#19216=CARTESIAN_POINT ( 'NONE',  ( -0.7480314960629914633, 0.2952755905511811885, 0.000000000000000000 ) ) ;
#19217=CARTESIAN_POINT ( 'NONE',  ( 0.4855643044619428750, 0.05413385826771666132, 0.4176697321401328100 ) ) ;
#19218=CARTESIAN_POINT ( 'NONE',  ( -0.8595800524934373854, -0.05778040916215522460, 0.4822834645669289988 ) ) ;
#19220=CARTESIAN_POINT ( 'NONE',  ( -0.7152230971128602510, -0.2845877964562159024, 0.3641732283464567677 ) ) ;
#19221=ORIENTED_EDGE ( 'NONE', *, *, #79585, .F. ) ;
#19223=ORIENTED_EDGE ( 'NONE', *, *, #54463, .F. ) ;
#19224=CARTESIAN_POINT ( 'NONE',  ( -1.561679790026246017, -0.004921259842519576551, 0.3153832671262227771 ) ) ;
#19225=CARTESIAN_POINT ( 'NONE',  ( -0.9055118110236215490, -0.6692913385826771977, 8.415575281601705876E-17 ) ) ;
#19226=CARTESIAN_POINT ( 'NONE',  ( -0.9711286089238838626, 0.2306618581243847221, -0.2411417322834647770 ) ) ;
#19228=CARTESIAN_POINT ( 'NONE',  ( -1.108923884514435132, -0.3162353388693405765, 0.4822834645669290543 ) ) ;
#19229=CARTESIAN_POINT ( 'NONE',  ( -1.299212598425196097, -0.6692913385826771977, 8.415575281601705876E-17 ) ) ;
#19232=CARTESIAN_POINT ( 'NONE',  ( 0.6561679790026253567, -0.5023911411419708095, -0.1820866141732282451 ) ) ;
#19233=CARTESIAN_POINT ( 'NONE',  ( 1.604771003085129433, 1.002618919725272617, -0.1466069496707750053 ) ) ;
#19235=CARTESIAN_POINT ( 'NONE',  ( -0.3280839895013117347, -0.3690944881889763329, 0.3153832671262228327 ) ) ;
#19236=CARTESIAN_POINT ( 'NONE',  ( -0.8333333333333323711, 0.2952755905511811885, 0.1292274648535926551 ) ) ;
#19237=CARTESIAN_POINT ( 'NONE',  ( 1.364829396325459854, -0.6046776061558809534, -0.2411417322834644161 ) ) ;
#19238=CARTESIAN_POINT ( 'NONE',  ( -0.5511811023622038563, -0.1870078740157479769, 0.4822834645669291653 ) ) ;
#19240=ORIENTED_EDGE ( 'NONE', *, *, #69643, .F. ) ;
#19242=CARTESIAN_POINT ( 'NONE',  ( -1.056430446194224881, -0.6692913385826771977, 0.1292274648535927661 ) ) ;
#19243=CARTESIAN_POINT ( 'NONE',  ( 1.187664041994751285, -0.3162353388693409650, -0.4822834645669289433 ) ) ;
#19244=CARTESIAN_POINT ( 'NONE',  ( -1.345144356955379816, -0.08942795157528024563, -0.3641732283464568787 ) ) ;
#19245=CARTESIAN_POINT ( 'NONE',  ( -1.391076115485563758, 0.2306618581243848609, 0.2411417322834645549 ) ) ;
#19250=CARTESIAN_POINT ( 'NONE',  ( -0.01312335958005186876, 0.05413385826771626580, -0.4176697321401330321 ) ) ;
#19251=CARTESIAN_POINT ( 'NONE',  ( -0.8858267716535425107, -0.4536011799217367080, 0.2665933059059888421 ) ) ;
#19252=CARTESIAN_POINT ( 'NONE',  ( -0.6561679790026240244, -0.6046776061558807314, 0.2411417322834647770 ) ) ;
#19254=CARTESIAN_POINT ( 'NONE',  ( -1.253280839895012377, -0.05778040916215522460, 0.4822834645669289988 ) ) ;
#19255=CARTESIAN_POINT ( 'NONE',  ( -1.069553805774277722, 0.2952755905511811885, 0.1292274648535926551 ) ) ;
#19256=CARTESIAN_POINT ( 'NONE',  ( -0.08530183727034056085, -0.05778040916215560624, -0.4822834645669293319 ) ) ;
#19258=CARTESIAN_POINT ( 'NONE',  ( 0.9251968503937015864, -0.4536011799217367080, 0.2665933059059888421 ) ) ;
#19259=CARTESIAN_POINT ( 'NONE',  ( -0.6889763779527552368, -0.4536011799217368745, -0.2665933059059886201 ) ) ;
#19261=CARTESIAN_POINT ( 'NONE',  ( 0.7874015748031503170, -0.1870078740157480601, -0.3641732283464567677 ) ) ;
#19262=CARTESIAN_POINT ( 'NONE',  ( 1.220472440944882386, -0.5511811023622047445, 6.969142054262312111E-17 ) ) ;
#19263=CARTESIAN_POINT ( 'NONE',  ( 1.568241469816273437, -0.3162353388693405765, 0.4822834645669290543 ) ) ;
#19264=CARTESIAN_POINT ( 'NONE',  ( 0.6167979002624679463, -0.004921259842519870586, -0.3153832671262229437 ) ) ;
#19266=CARTESIAN_POINT ( 'NONE',  ( -0.9317585301837263412, -0.4281496062992127816, -0.4176697321401328100 ) ) ;
#19267=CARTESIAN_POINT ( 'NONE',  ( 1.240157480314961314, -0.5400638737290844871, 0.3530559997133364547 ) ) ;
#19269=CARTESIAN_POINT ( 'NONE',  ( -0.6692913385826764205, 0.1771653543307087630, 0.000000000000000000 ) ) ;
#19270=FACE_OUTER_BOUND ( 'NONE', #14110, .T. ) ;
#19271=CARTESIAN_POINT ( 'NONE',  ( 0.1312335958005257930, 0.2306618581243847221, -0.2411417322834647770 ) ) ;
#19274=CARTESIAN_POINT ( 'NONE',  ( 1.069553805774278610, -0.5511811023622046335, 0.09757992244046803654 ) ) ;
#19275=CARTESIAN_POINT ( 'NONE',  ( 0.1246719160104994284, -0.5511811023622046335, 0.09757992244046803654 ) ) ;
#19276=CARTESIAN_POINT ( 'NONE',  ( 0.2362204724409456558, -0.1870078740157479769, 0.4822834645669291653 ) ) ;
#19277=CARTESIAN_POINT ( 'NONE',  ( -1.397637795275589623, 0.1660481256975885056, 0.3530559997133364547 ) ) ;
#19279=CARTESIAN_POINT ( 'NONE',  ( -0.7152230971128602510, -0.2845877964562159024, 0.3641732283464567677 ) ) ;
#19281=CARTESIAN_POINT ( 'NONE',  ( -0.3608923884514428360, 0.2952755905511811885, 0.1292274648535926551 ) ) ;
#19284=CARTESIAN_POINT ( 'NONE',  ( 0.1574803149606306130, -0.1870078740157479769, 0.3641732283464567677 ) ) ;
#19285=CARTESIAN_POINT ( 'NONE',  ( -0.5643044619422565855, -0.4281496062992124485, 0.4176697321401328655 ) ) ;
#19286=CARTESIAN_POINT ( 'NONE',  ( -0.9776902887139098386, 0.2952755905511810774, -0.1292274648535930714 ) ) ;
#19287=CARTESIAN_POINT ( 'NONE',  ( -1.299212598425196097, 0.1771653543307087630, 0.000000000000000000 ) ) ;
#19289=CARTESIAN_POINT ( 'NONE',  ( -0.3674540682414689785, 0.2306618581243848609, 0.2411417322834645549 ) ) ;
#19291=CARTESIAN_POINT ( 'NONE',  ( -0.8070866141732276899, 0.07958543189024071263, -0.2665933059059888421 ) ) ;
#19292=CARTESIAN_POINT ( 'NONE',  ( -1.476377952755905110, -0.4536011799217368745, -0.2665933059059886201 ) ) ;
#19293=CARTESIAN_POINT ( 'NONE',  ( 1.135170603674541256, 0.2952755905511811885, 0.1292274648535926551 ) ) ;
#19297=EDGE_CURVE ( 'NONE', #4124, #34136, #61076, .T. ) ;
#19298=CARTESIAN_POINT ( 'NONE',  ( -0.7478466213799878082, 1.968503937007873850, 0.5309055118110236338 ) ) ;
#19299=CARTESIAN_POINT ( 'NONE',  ( -1.548556430446193399, 0.2306618581243848609, 0.2411417322834645549 ) ) ;
#19300=CARTESIAN_POINT ( 'NONE',  ( -0.7677165354330699465, 0.1660481256975885056, 0.3530559997133364547 ) ) ;
#19301=CARTESIAN_POINT ( 'NONE',  ( -1.430446194225720724, 0.05413385826771626580, -0.4176697321401330321 ) ) ;
#19303=CARTESIAN_POINT ( 'NONE',  ( 1.450131233595801428, -0.5511811023622048555, -0.09757992244046775898 ) ) ;
#19304=CARTESIAN_POINT ( 'NONE',  ( 0.5446194225721792126, -0.3162353388693405765, 0.4822834645669290543 ) ) ;
#19305=CARTESIAN_POINT ( 'NONE',  ( 0.1443569553805781891, 0.05413385826771626580, -0.4176697321401330321 ) ) ;
#19306=CARTESIAN_POINT ( 'NONE',  ( -0.3264567959345324177, -3.773335473449285555E-15, -0.3791475997938234532 ) ) ;
#19308=CARTESIAN_POINT ( 'NONE',  ( 1.154855643044620184, 0.1283753931104746893, -0.1820866141732285504 ) ) ;
#19312=ORIENTED_EDGE ( 'NONE', *, *, #2159, .F. ) ;
#19313=CARTESIAN_POINT ( 'NONE',  ( -0.06561679790026180015, -0.4281496062992127816, -0.4176697321401328100 ) ) ;
#19314=CARTESIAN_POINT ( 'NONE',  ( -0.9448818897637790704, -0.1870078740157479769, 0.4822834645669291653 ) ) ;
#19315=CARTESIAN_POINT ( 'NONE',  ( -1.443569553805773564, 0.2306618581243847221, -0.2411417322834647770 ) ) ;
#19316=CARTESIAN_POINT ( 'NONE',  ( 0.7020997375328090762, -0.3162353388693405765, 0.4822834645669290543 ) ) ;
#19318=CARTESIAN_POINT ( 'NONE',  ( 1.686351706036745890, 0.2952755905511811885, 0.1292274648535926551 ) ) ;
#19319=CARTESIAN_POINT ( 'NONE',  ( 1.279527559055118724, 0.1660481256975885056, 0.3530559997133364547 ) ) ;
#19320=CARTESIAN_POINT ( 'NONE',  ( -0.3477690288713902178, 0.2952755905511810774, -0.1292274648535930714 ) ) ;
#19321=CARTESIAN_POINT ( 'NONE',  ( 0.6233595800524939223, -0.3162353388693405765, 0.4822834645669290543 ) ) ;
#19322=CARTESIAN_POINT ( 'NONE',  ( -1.555118110236219930, -0.5400638737290845981, -0.3530559997133363437 ) ) ;
#19323=CARTESIAN_POINT ( 'NONE',  ( 1.259842519685040019, -0.1870078740157479769, 0.4822834645669291653 ) ) ;
#19325=CARTESIAN_POINT ( 'NONE',  ( 1.463254593175853824, -0.6692913385826771977, 0.1292274648535927661 ) ) ;
#19326=CARTESIAN_POINT ( 'NONE',  ( -0.2362204724409442680, -0.1870078740157480879, -0.4822834645669291653 ) ) ;
#19328=CARTESIAN_POINT ( 'NONE',  ( 0.6233595800524942554, -0.08942795157528024563, -0.3641732283464568787 ) ) ;
#19329=ORIENTED_EDGE ( 'NONE', *, *, #41924, .T. ) ;
#19331=ORIENTED_EDGE ( 'NONE', *, *, #69939, .T. ) ;
#19332=CARTESIAN_POINT ( 'NONE',  ( -0.4724409448818890911, -0.1870078740157479769, 0.3641732283464567677 ) ) ;
#19334=CARTESIAN_POINT ( 'NONE',  ( 0.3083989501312343062, -0.3162353388693405765, 0.4822834645669290543 ) ) ;
#19335=CARTESIAN_POINT ( 'NONE',  ( 0.02624671916010564918, 0.2306618581243848609, 0.2411417322834645549 ) ) ;
#19336=CARTESIAN_POINT ( 'NONE',  ( -1.161417322834644716, -0.5400638737290845981, -0.3530559997133363437 ) ) ;
#19340=CARTESIAN_POINT ( 'NONE',  ( -1.187664041994749731, -0.3162353388693405765, 0.4822834645669290543 ) ) ;
#19341=CARTESIAN_POINT ( 'NONE',  ( -0.1474713956048439301, -2.191421614605370878E-15, 0.4445507791589071167 ) ) ;
#19342=CARTESIAN_POINT ( 'NONE',  ( 0.9776902887139113929, 0.1771653543307087630, 0.09757992244046791164 ) ) ;
#19343=CARTESIAN_POINT ( 'NONE',  ( 0.5380577427821529035, -0.4281496062992124485, 0.4176697321401328655 ) ) ;
#19344=CARTESIAN_POINT ( 'NONE',  ( 0.8989501312335964611, 0.2952755905511811885, 0.1292274648535926551 ) ) ;
#19346=CARTESIAN_POINT ( 'NONE',  ( -1.404199475065615932, 0.05413385826771666132, 0.4176697321401328100 ) ) ;
#19349=CARTESIAN_POINT ( 'NONE',  ( -0.1443569553805768291, 0.05413385826771666132, 0.4176697321401328100 ) ) ;
#19353=CARTESIAN_POINT ( 'NONE',  ( -1.161417322834644716, 0.07958543189024085140, 0.2665933059059887866 ) ) ;
#19354=CARTESIAN_POINT ( 'NONE',  ( 1.391076115485564868, -0.6046776061558807314, 0.2411417322834647770 ) ) ;
#19355=CARTESIAN_POINT ( 'NONE',  ( 1.528871391076116026, 0.2952755905511811885, 0.1292274648535926551 ) ) ;
#19356=CARTESIAN_POINT ( 'NONE',  ( 0.01312335958005323398, -0.3690944881889765550, -0.3153832671262227771 ) ) ;
#19357=CARTESIAN_POINT ( 'NONE',  ( 0.3543307086614179147, 0.2952755905511811885, 0.000000000000000000 ) ) ;
#19359=CARTESIAN_POINT ( 'NONE',  ( 0.3740157480314966754, -0.4536011799217367080, 0.2665933059059888421 ) ) ;
#19360=CARTESIAN_POINT ( 'NONE',  ( 0.4790026246719167324, -0.05778040916215522460, 0.4822834645669289988 ) ) ;
#19362=CARTESIAN_POINT ( 'NONE',  ( -1.141732283464566011, -0.6692913385826771977, 8.415575281601705876E-17 ) ) ;
#19363=CARTESIAN_POINT ( 'NONE',  ( 0.3083989501312343062, -0.2845877964562159024, 0.3641732283464567677 ) ) ;
#19364=CARTESIAN_POINT ( 'NONE',  ( 0.3273801728231982566, 0.000000000000000000, 0.3464511005275205946 ) ) ;
#19365=CARTESIAN_POINT ( 'NONE',  ( -0.4790026246719154557, -0.3162353388693405765, 0.4822834645669290543 ) ) ;
#19366=CARTESIAN_POINT ( 'NONE',  ( -0.1968503937007867743, 0.1771653543307087630, 0.000000000000000000 ) ) ;
#19368=CARTESIAN_POINT ( 'NONE',  ( -0.2230971128608915943, -0.4281496062992127816, -0.4176697321401328100 ) ) ;
#19369=CARTESIAN_POINT ( 'NONE',  ( 0.1902887139107617975, 0.1771653543307087630, 0.09757992244046791164 ) ) ;
#19371=CARTESIAN_POINT ( 'NONE',  ( -0.03937007874015669567, 0.2952755905511811885, 0.000000000000000000 ) ) ;
#19373=CARTESIAN_POINT ( 'NONE',  ( 1.332020997375329197, -0.2845877964562159024, 0.3641732283464567677 ) ) ;
#19374=CARTESIAN_POINT ( 'NONE',  ( 0.4848604877838280647, 0.000000000000000000, 0.3464511005275205946 ) ) ;
#19375=CARTESIAN_POINT ( 'NONE',  ( -0.9120734908136475250, 0.1771653543307087630, 0.09757992244046791164 ) ) ;
#19376=CARTESIAN_POINT ( 'NONE',  ( -0.8989501312335946848, 0.1771653543307087075, -0.09757992244046823083 ) ) ;
#19377=CARTESIAN_POINT ( 'NONE',  ( -0.8267716535433065062, 0.2952755905511811885, 0.000000000000000000 ) ) ;
#19378=CARTESIAN_POINT ( 'NONE',  ( -0.1115485564304456306, 0.2952755905511810774, -0.1292274648535930714 ) ) ;
#19379=CARTESIAN_POINT ( 'NONE',  ( 0.7611548556430454138, 0.1283753931104746893, -0.1820866141732285504 ) ) ;
#19381=CARTESIAN_POINT ( 'NONE',  ( 1.049868766404200127, -0.5023911411419708095, -0.1820866141732282451 ) ) ;
#19382=AXIS2_PLACEMENT_3D ( 'NONE', #10391, #73948, #67633 ) ;
#19383=CARTESIAN_POINT ( 'NONE',  ( 0.8792650918635177559, 0.05413385826771666132, 0.4176697321401328100 ) ) ;
#19385=CARTESIAN_POINT ( 'NONE',  ( -0.3018372703412066094, 0.05413385826771666132, 0.4176697321401328100 ) ) ;
#19387=CARTESIAN_POINT ( 'NONE',  ( -1.732283464566928277, -0.1870078740157479769, 0.4822834645669291653 ) ) ;
#19388=CARTESIAN_POINT ( 'NONE',  ( 0.7742782152230979209, 0.05413385826771626580, -0.4176697321401330321 ) ) ;
#19389=CARTESIAN_POINT ( 'NONE',  ( -0.05249343832020911260, 0.2306618581243848609, 0.2411417322834645549 ) ) ;
#19391=CARTESIAN_POINT ( 'NONE',  ( 0.3871391076115493490, -0.2845877964562159024, 0.3641732283464567677 ) ) ;
#19392=CARTESIAN_POINT ( 'NONE',  ( 0.7677165354330716118, 0.1660481256975883668, -0.3530559997133364547 ) ) ;
#19394=CARTESIAN_POINT ( 'NONE',  ( -0.3018372703412066094, -0.004921259842519576551, 0.3153832671262227771 ) ) ;
#19395=CARTESIAN_POINT ( 'NONE',  ( -0.7742782152230962556, -0.4281496062992127816, -0.4176697321401328100 ) ) ;
#19397=CARTESIAN_POINT ( 'NONE',  ( 0.1837270341207354329, 0.2306618581243848609, 0.2411417322834645549 ) ) ;
#19398=CARTESIAN_POINT ( 'NONE',  ( -1.377952755905511140, -0.6692913385826771977, 8.415575281601705876E-17 ) ) ;
#19399=CARTESIAN_POINT ( 'NONE',  ( -0.8464566929133852113, -0.4536011799217368745, -0.2665933059059886201 ) ) ;
#19400=CARTESIAN_POINT ( 'NONE',  ( 0.3805774278215230400, 0.05413385826771626580, -0.4176697321401330321 ) ) ;
#19401=CARTESIAN_POINT ( 'NONE',  ( -1.082677165354329896, 0.1660481256975885056, 0.3530559997133364547 ) ) ;
#19402=CARTESIAN_POINT ( 'NONE',  ( -0.4396325459317577122, -0.6692913385826773087, -0.1292274648535924053 ) ) ;
#19403=( BOUNDED_SURFACE ( )  B_SPLINE_SURFACE ( 1, 2, ( 
 ( #13675, #19138, #38913, #64593, #71327, #65013, #7348, #20398, #1051, #14097, #26705, #46050, #71744, #53192, #10169, #49272, #14517, #1875, #59518, #74144, #72575, #40582, #36239, #7777, #67830, #27535, #27117, #78905, #16489, #3434, #14922, #78490, #40170, #29508, #35418, #39749, #22784, #33854, #1461, #52781, #29913, #68248, #48861, #65854, #23190, #42135, #80472, #48444, #8187, #80878, #10582, #35834, #20813, #74975, #74561, #54768, #46881, #21226, #61501, #66263, #16907, #29096, #8603, #61083, #42545, #59105, #4251, #81287, #61909, #46468, #3848, #55577, #23603, #55169, #72162, #65445, #33445, #12635, #49683, #68642, #37058, #82109, #18539, #11401, #57644, #76610, #70282, #10981, #5487, #36641, #31148, #69052, #25245, #7, #24015, #24422, #25659, #38294, #81705, #51321, #43350, #37473, #75375, #50909, #6307, #37884, #42948, #5893, #63971, #50092, #18940, #56814, #18130, #17724, #30327, #44588, #62742, #82513, #4654, #75788, #17320, #43763, #69468, #11821, #57223, #24829, #62317, #55993, #5078, #30747, #63146, #56410, #50498, #76201, #31984, #44182, #69874, #63559, #82924, #12227, #31565, #26919, #14321, #52995, #58059, #13892, #40387, #77444, #26508, #52579, #52162, #58486, #78288, #77866, #51741, #77024, #851, #59322, #13469, #425, #71966, #72385, #33659, #20619, #58912, #66070, #65669, #39551, #46692, #64390, #59737, #45006, #14735, #26081, #70706, #39126, #20195, #46271, #71126, #34073, #78708, #8406, #13058, #65240, #38712, #7578, #45431, #1678, #2091, #19777, #45846, #27756, #19357, #64807, #6726, #7146, #33250, #32819, #27335, #32396, #39979, #71545, #7995, #1271, #21032, #3748, #9651, #54245, #53828, #66483, #55071, #73211, #67316, #40798, #2925, #53420, #79962, #22275, #28589, #10066, #41627, #36143, #21446, #47103, #4155, #47935, #72792, #35320, #79542, #48762, #34495, #60983, #74043, #35729, #3333, #60574, #28997, #16390, #29412, #60160, #73638, #16808, #21855, #15980, #54663, #80374, #34911, #22687, #48346, #28171, #79129, #42037, #61399, #15561, #2512, #67731, #74461, #80779, #23095, #42445, #68144, #10489, #61815, #15142, #8818, #47519, #41221, #66908, #9239, #69376, #11729, #4564, #69786, #57131, #31056, #68549, #63872, #63465, #43673, #36967, #75286, #37385, #17629, #5799, #18039, #43261, #55899, #31469, #49176, #76519, #70185, #25150, #36550, #68958, #12131, #37788, #81610, #18450, #50001, #10890, #24741, #50818, #44092, #18848, #44494, #12538, #11308, #82828, #62646, #38197, #5394, #63056, #29820, #62226, #17224, #55482, #81191, #30235, #56725, #4988, #30655, #82422, #23508, #74880, #42856, #23925, #49591, #50409, #56319, #76109, #82017, #24331, #75698, #32298, #52061, #19674, #71028, #46171, #31887, #20099, #57958, #51226, #326, #77767, #7049, #45333, #19252, #12957, #65138, #39025, #6211, #45750, #25980, #76924, #44904, #65564, #58814, #7474, #13372, #70602, #71867, #57547, #38614, #746, #64292, #33145, #6626, #71445, #51638, #33559, #1171, #20519, #26822, #13793, #39877, #77343, #64709, #7898, #32718, #58385, #52480, #78188, #39450, #26407, #14217, #83238, #25559, #59611, #13344, #45722, #65945, #20070, #7020, #78582, #79003, #40262, #33533, #65538, #72669, #72260, #46145, #53291, #27629, #8281, #717, #33947, #59196, #39847, #7869, #58355, #1966, #21322, #1555, #38998, #34368, #46975, #14190, #7445, #71419, #27209, #13766, #15018, #71840, #39423, #33115, #65107, #52872, #58785, #40674, #20908, #1143, #26375, #66359, #19645, #8697, #296, #25952, #32688, #26793, #51610, #77315, #52035, #71001, #45306, #64681, #77739, #52450, #78160, #20491, #46561, #14608, #54121, #17101, #36025, #29702, #53703, #48230, #79412, #73926, #28460, #68022, #42736, #66784, #67195, #68432, #55365, #41096, #10772, #2801, #80253, #9119, #10365, #49054, #80663, #2389, #48642, #81070, #9526, #61697, #16268, #60859, #60449, #73085, #4037, #79835, #41913, #47394, #35198, #60033, #3213, #28875, #54538, #16683, #67607, #28045, #21731, #15435, #34790, #22570, #22152, #9938, #47811, #23386, #73513, #35610, #22975, #42322, #61273, #3626, #29294, #74336 ),
 ( #74753, #54956, #15862, #41510, #43142, #62518, #81896, #82704, #75985, #82301, #4857, #12415, #17918, #5270, #37261, #63339, #43554, #31342, #75165, #30531, #50287, #11185, #24620, #18327, #69255, #11602, #38073, #63749, #44369, #36846, #18727, #12007, #43967, #69664, #56195, #76395, #6088, #37661, #17510, #70476, #70061, #5674, #62937, #24207, #57008, #49878, #31763, #25024, #75578, #30934, #57424, #55775, #83118, #76799, #25436, #68839, #56601, #51102, #19130, #50697, #23799, #44779, #4448, #36432, #62105, #30113, #81483, #49472, #14092, #6922, #53185, #72157, #65849, #6508, #1045, #32178, #26699, #64585, #20807, #78900, #19546, #19975, #21221, #8182, #77217, #46876, #38905, #33010, #45205, #46463, #1868, #33440, #38491, #1455, #33848, #45626, #14512, #52354, #13669, #13256, #25853, #40165, #32593, #78061, #201, #71320, #12833, #39321, #65006, #7342, #52775, #20391, #64174, #57833, #51513, #70905, #58680, #58256, #46043, #621, #59514, #26277, #71737, #59100, #78483, #39744, #65440, #7773, #27112, #27530, #51939, #77643, #35929, #72982, #22049, #48129, #47709, #54021, #73826, #21633, #48537, #2285, #34689, #54859, #9016, #79314, #67502, #67921, #29192, #22469, #54438, #61596, #61172, #35093, #42226, #41409, #73405, #16164, #79732, #9837, #27947, #15334, #3111, #47293, #60760, #28776, #15756, #67093, #74237, #10259, #53606, #28359, #80149, #34269, #9424, #60352, #3524, #41810, #40999, #35508, #3942, #80564, #29601, #55262, #80972, #2699, #22875, #16581, #23285, #72570, #14917, #40577, #66679, #59929, #66258, #8597, #4343, #50188, #24109, #4752, #5173, #37977, #82608, #83017, #10676, #68337, #37155, #62414, #18226, #57321, #23696, #11081, #68739, #82204, #81798, #49778, #44275, #16998, #75885, #36738, #36332, #30426, #24522, #11501, #75478, #30010, #49369, #37566, #43452, #48955, #30837, #43043, #62007, #55673, #63652, #63240, #11912, #17819, #81382, #18631, #74656, #42640, #62839, #75065, #43863, #17413, #56502, #56093, #5991, #5580, #24926, #31246, #69564, #69965, #69150, #56912, #31662, #50593, #76302, #12319, #7677, #52260, #71227, #19452, #51002, #8092, #26608, #13994, #32078, #25755, #33348, #13571, #71643, #77966, #57739, #51417, #70807, #39651, #64910, #39225, #77119, #1365, #6825, #13159, #65342, #45529, #6408, #20296, #20717, #59010, #72062, #14420, #65759, #38810, #27017, #32494, #78386, #952, #58585, #52678, #101, #12732, #46368, #25340, #64069, #45945, #526, #64487, #7247, #40072, #33756, #60566, #70377, #44681, #32919, #58158, #76701, #19034, #45103, #26179, #51841, #38391, #77546, #19880, #81599, #54237, #29811, #22679, #73630, #48338, #36133, #48753, #61391, #41619, #3325, #74871, #80771, #2917, #68135, #80366, #47925, #15972, #75277, #17214, #49165, #3740, #67308, #55888, #28580, #79954, #74452, #9643, #81182, #35312, #10480, #54655, #17620, #42847, #62217, #68540, #61806, #23916, #60974, #29404, #43252, #28989, #10058, #10880, #36541, #55472, #16798, #74035, #22267, #68949, #4146, #4555, #16382, #42028, #30225, #42435, #49581, #23499, #67722, #35721, #55063, #11299, #36958, #23086, #5385, #38606, #44083, #31460, #63455, #6201, #69777, #57539, #18030, #31046, #76510, #37376, #25140, #18839, #12121, #37779, #64284, #318, #43664, #18441, #44484, #24321, #5790, #12948, #70176, #57122, #24732, #12528, #50400, #6619, #50809, #76097, #56715, #32290, #82007, #25971, #19663, #57950, #69366, #82816, #44895, #70594, #82413, #49992, #45325, #30645, #51630, #11720, #56310, #38189, #63864, #31879, #83230, #71020, #77334, #13364, #75689, #25551, #63046, #51218, #76915, #62635, #4979, #19244, #46164, #21747, #8713, #20092, #79428, #65130, #59214, #71438, #46994, #28063, #59629, #64701, #27647, #34384, #71860, #72687, #78602, #39866, #39442, #52054, #40690, #58805, #52890, #26396, #14210, #39017, #65557, #7889, #33552, #79022, #27230, #47412, #7041, #32710, #73101, #1575, #58376, #20926, #7465, #60049, #45742, #46581, #1984, #21341, #72279, #14626, #40281, #53309, #15035, #13786, #65963, #2405, #33135, #8299, #33967, #66376, #20511, #53720, #1163 ) ),
 .UNSPECIFIED., .F., .F., .F. ) 
 B_SPLINE_SURFACE_WITH_KNOTS ( ( 2, 2 ),
 ( 3, 2, 2, 2, 2, 2, 2, 2, 2, 2, 2, 2, 2, 2, 2, 2, 2, 2, 2, 2, 2, 2, 2, 2, 2, 2, 2, 2, 2, 2, 2, 2, 2, 2, 2, 2, 2, 2, 2, 2, 2, 2, 2, 2, 2, 2, 2, 2, 2, 2, 2, 2, 2, 2, 2, 2, 2, 2, 2, 2, 2, 2, 2, 2, 2, 2, 2, 2, 2, 2, 2, 2, 2, 2, 2, 2, 2, 2, 2, 2, 2, 2, 2, 2, 2, 2, 2, 2, 2, 2, 2, 2, 2, 2, 2, 2, 2, 2, 2, 2, 2, 2, 2, 2, 2, 2, 2, 2, 2, 2, 2, 2, 2, 2, 2, 2, 2, 2, 2, 2, 2, 2, 2, 2, 2, 2, 2, 2, 2, 2, 2, 2, 2, 2, 2, 2, 2, 2, 2, 2, 2, 2, 2, 2, 2, 2, 2, 2, 2, 2, 2, 2, 2, 2, 2, 2, 2, 2, 2, 2, 2, 2, 2, 2, 2, 2, 2, 2, 2, 2, 2, 2, 2, 2, 2, 2, 2, 2, 2, 2, 2, 2, 2, 2, 2, 2, 2, 2, 2, 2, 2, 2, 2, 2, 2, 2, 2, 2, 2, 2, 2, 2, 2, 2, 2, 2, 2, 2, 2, 2, 2, 2, 2, 2, 2, 2, 2, 2, 2, 2, 2, 2, 2, 2, 2, 2, 2, 2, 2, 2, 2, 2, 2, 2, 2, 2, 2, 2, 2, 2, 2, 2, 2, 2, 2, 2, 2, 2, 2, 2, 2, 2, 2, 2, 2, 3 ),
 ( 0.000000000000000000, 1.000000000000000000 ),
 ( 0.000000000000000000, 0.003787878787878787984, 0.007575757575757575968, 0.01136363636363636395, 0.01515151515151515194, 0.01893939393939393992, 0.02272727272727272790, 0.02651515151515151589, 0.03030303030303030387, 0.03409090909090908839, 0.03787878787878787984, 0.04166666666666666435, 0.04545454545454545581, 0.04924242424242424032, 0.05303030303030303177, 0.05681818181818181629, 0.06060606060606060774, 0.06439393939393939226, 0.06818181818181817677, 0.07196969696969697516, 0.07575757575757575968, 0.07954545454545454419, 0.08333333333333332871, 0.08712121212121212710, 0.09090909090909091161, 0.09469696969696969613, 0.09848484848484848064, 0.1022727272727272790, 0.1060606060606060635, 0.1098484848484848481, 0.1136363636363636326, 0.1174242424242424310, 0.1212121212121212155, 0.1250000000000000000, 0.1287878787878787845, 0.1325757575757575690, 0.1363636363636363535, 0.1401515151515151381, 0.1439393939393939503, 0.1477272727272727348, 0.1515151515151515194, 0.1553030303030303039, 0.1590909090909090884, 0.1628787878787878729, 0.1666666666666666574, 0.1704545454545454419, 0.1742424242424242542, 0.1780303030303030387, 0.1818181818181818232, 0.1856060606060606077, 0.1893939393939393923, 0.1931818181818181768, 0.1969696969696969613, 0.2007575757575757458, 0.2045454545454545581, 0.2083333333333333426, 0.2121212121212121271, 0.2159090909090909116, 0.2196969696969696961, 0.2234848484848484806, 0.2272727272727272652, 0.2310606060606060497, 0.2348484848484848619, 0.2386363636363636465, 0.2424242424242424310, 0.2462121212121212155, 0.2500000000000000000, 0.2537878787878787845, 0.2575757575757575690, 0.2613636363636363535, 0.2651515151515151381, 0.2689393939393939226, 0.2727272727272727071, 0.2765151515151514916, 0.2803030303030302761, 0.2840909090909091161, 0.2878787878787879007, 0.2916666666666666852, 0.2954545454545454697, 0.2992424242424242542, 0.3030303030303030387, 0.3068181818181818232, 0.3106060606060606077, 0.3143939393939393923, 0.3181818181818181768, 0.3219696969696969613, 0.3257575757575757458, 0.3295454545454545303, 0.3333333333333333148, 0.3371212121212120993, 0.3409090909090908839, 0.3446969696969697239, 0.3484848484848485084, 0.3522727272727272929, 0.3560606060606060774, 0.3598484848484848619, 0.3636363636363636465, 0.3674242424242424310, 0.3712121212121212155, 0.3750000000000000000, 0.3787878787878787845, 0.3825757575757575690, 0.3863636363636363535, 0.3901515151515151381, 0.3939393939393939226, 0.3977272727272727071, 0.4015151515151514916, 0.4053030303030302761, 0.4090909090909091161, 0.4128787878787879007, 0.4166666666666666852, 0.4204545454545454697, 0.4242424242424242542, 0.4280303030303030387, 0.4318181818181818232, 0.4356060606060606077, 0.4393939393939393923, 0.4431818181818181768, 0.4469696969696969613, 0.4507575757575757458, 0.4545454545454545303, 0.4583333333333333148, 0.4621212121212120993, 0.4659090909090908839, 0.4696969696969697239, 0.4734848484848485084, 0.4772727272727272929, 0.4810606060606060774, 0.4848484848484848619, 0.4886363636363636465, 0.4924242424242424310, 0.4962121212121212155, 0.5000000000000000000, 0.5037878787878787845, 0.5075757575757575690, 0.5113636363636363535, 0.5151515151515151381, 0.5189393939393939226, 0.5227272727272727071, 0.5265151515151514916, 0.5303030303030302761, 0.5340909090909090606, 0.5378787878787878451, 0.5416666666666666297, 0.5454545454545454142, 0.5492424242424241987, 0.5530303030303029832, 0.5568181818181817677, 0.5606060606060605522, 0.5643939393939394478, 0.5681818181818182323, 0.5719696969696970168, 0.5757575757575758013, 0.5795454545454545858, 0.5833333333333333703, 0.5871212121212121549, 0.5909090909090909394, 0.5946969696969697239, 0.5984848484848485084, 0.6022727272727272929, 0.6060606060606060774, 0.6098484848484848619, 0.6136363636363636465, 0.6174242424242424310, 0.6212121212121212155, 0.6250000000000000000, 0.6287878787878787845, 0.6325757575757575690, 0.6363636363636363535, 0.6401515151515151381, 0.6439393939393939226, 0.6477272727272727071, 0.6515151515151514916, 0.6553030303030302761, 0.6590909090909090606, 0.6628787878787878451, 0.6666666666666666297, 0.6704545454545454142, 0.6742424242424241987, 0.6780303030303029832, 0.6818181818181817677, 0.6856060606060605522, 0.6893939393939394478, 0.6931818181818182323, 0.6969696969696970168, 0.7007575757575758013, 0.7045454545454545858, 0.7083333333333333703, 0.7121212121212121549, 0.7159090909090909394, 0.7196969696969697239, 0.7234848484848485084, 0.7272727272727272929, 0.7310606060606060774, 0.7348484848484848619, 0.7386363636363636465, 0.7424242424242424310, 0.7462121212121212155, 0.7500000000000000000, 0.7537878787878787845, 0.7575757575757575690, 0.7613636363636363535, 0.7651515151515151381, 0.7689393939393939226, 0.7727272727272727071, 0.7765151515151514916, 0.7803030303030302761, 0.7840909090909090606, 0.7878787878787878451, 0.7916666666666666297, 0.7954545454545454142, 0.7992424242424241987, 0.8030303030303029832, 0.8068181818181817677, 0.8106060606060605522, 0.8143939393939394478, 0.8181818181818182323, 0.8219696969696970168, 0.8257575757575758013, 0.8295454545454545858, 0.8333333333333333703, 0.8371212121212121549, 0.8409090909090909394, 0.8446969696969697239, 0.8484848484848485084, 0.8522727272727272929, 0.8560606060606060774, 0.8598484848484848619, 0.8636363636363636465, 0.8674242424242424310, 0.8712121212121212155, 0.8750000000000000000, 0.8787878787878787845, 0.8825757575757575690, 0.8863636363636363535, 0.8901515151515151381, 0.8939393939393939226, 0.8977272727272727071, 0.9015151515151514916, 0.9053030303030302761, 0.9090909090909090606, 0.9128787878787878451, 0.9166666666666666297, 0.9204545454545454142, 0.9242424242424241987, 0.9280303030303029832, 0.9318181818181817677, 0.9356060606060605522, 0.9393939393939394478, 0.9431818181818182323, 0.9469696969696970168, 0.9507575757575758013, 0.9545454545454545858, 0.9583333333333333703, 0.9621212121212121549, 0.9659090909090909394 ),
 .UNSPECIFIED. ) 
 GEOMETRIC_REPRESENTATION_ITEM ( )  RATIONAL_B_SPLINE_SURFACE ( (
 ( 1.000000000000000000, 0.9659258262890683122, 1.000000000000000000, 0.9659258262890683122, 1.000000000000000000, 0.9659258262890683122, 1.000000000000000000, 0.9659258262890683122, 1.000000000000000000, 0.9659258262890683122, 1.000000000000000000, 0.9659258262890683122, 1.000000000000000000, 0.9659258262890683122, 1.000000000000000000, 0.9659258262890683122, 1.000000000000000000, 0.9659258262890683122, 1.000000000000000000, 0.9659258262890683122, 1.000000000000000000, 0.9659258262890683122, 1.000000000000000000, 0.9659258262890683122, 1.000000000000000000, 0.9659258262890683122, 1.000000000000000000, 0.9659258262890683122, 1.000000000000000000, 0.9659258262890683122, 1.000000000000000000, 0.9659258262890683122, 1.000000000000000000, 0.9659258262890683122, 1.000000000000000000, 0.9659258262890683122, 1.000000000000000000, 0.9659258262890683122, 1.000000000000000000, 0.9659258262890683122, 1.000000000000000000, 0.9659258262890683122, 1.000000000000000000, 0.9659258262890683122, 1.000000000000000000, 0.9659258262890683122, 1.000000000000000000, 0.9659258262890683122, 1.000000000000000000, 0.9659258262890683122, 1.000000000000000000, 0.9659258262890683122, 1.000000000000000000, 0.9659258262890683122, 1.000000000000000000, 0.9659258262890683122, 1.000000000000000000, 0.9659258262890683122, 1.000000000000000000, 0.9659258262890683122, 1.000000000000000000, 0.9659258262890683122, 1.000000000000000000, 0.9659258262890683122, 1.000000000000000000, 0.9659258262890683122, 1.000000000000000000, 0.9659258262890683122, 1.000000000000000000, 0.9659258262890683122, 1.000000000000000000, 0.9659258262890683122, 1.000000000000000000, 0.9659258262890683122, 1.000000000000000000, 0.9659258262890683122, 1.000000000000000000, 0.9659258262890683122, 1.000000000000000000, 0.9659258262890683122, 1.000000000000000000, 0.9659258262890683122, 1.000000000000000000, 0.9659258262890683122, 1.000000000000000000, 0.9659258262890683122, 1.000000000000000000, 0.9659258262890683122, 1.000000000000000000, 0.9659258262890683122, 1.000000000000000000, 0.9659258262890683122, 1.000000000000000000, 0.9659258262890683122, 1.000000000000000000, 0.9659258262890683122, 1.000000000000000000, 0.9659258262890683122, 1.000000000000000000, 0.9659258262890683122, 1.000000000000000000, 0.9659258262890683122, 1.000000000000000000, 0.9659258262890683122, 1.000000000000000000, 0.9659258262890683122, 1.000000000000000000, 0.9659258262890683122, 1.000000000000000000, 0.9659258262890683122, 1.000000000000000000, 0.9659258262890683122, 1.000000000000000000, 0.9659258262890683122, 1.000000000000000000, 0.9659258262890683122, 1.000000000000000000, 0.9659258262890683122, 1.000000000000000000, 0.9659258262890683122, 1.000000000000000000, 0.9659258262890683122, 1.000000000000000000, 0.9659258262890683122, 1.000000000000000000, 0.9659258262890683122, 1.000000000000000000, 0.9659258262890683122, 1.000000000000000000, 0.9659258262890683122, 1.000000000000000000, 0.9659258262890683122, 1.000000000000000000, 0.9659258262890683122, 1.000000000000000000, 0.9659258262890683122, 1.000000000000000000, 0.9659258262890683122, 1.000000000000000000, 0.9659258262890683122, 1.000000000000000000, 0.9659258262890683122, 1.000000000000000000, 0.9659258262890683122, 1.000000000000000000, 0.9659258262890683122, 1.000000000000000000, 0.9659258262890683122, 1.000000000000000000, 0.9659258262890683122, 1.000000000000000000, 0.9659258262890683122, 1.000000000000000000, 0.9659258262890683122, 1.000000000000000000, 0.9659258262890683122, 1.000000000000000000, 0.9659258262890683122, 1.000000000000000000, 0.9659258262890683122, 1.000000000000000000, 0.9659258262890683122, 1.000000000000000000, 0.9659258262890683122, 1.000000000000000000, 0.9659258262890683122, 1.000000000000000000, 0.9659258262890683122, 1.000000000000000000, 0.9659258262890683122, 1.000000000000000000, 0.9659258262890683122, 1.000000000000000000, 0.9659258262890683122, 1.000000000000000000, 0.9659258262890683122, 1.000000000000000000, 0.9659258262890683122, 1.000000000000000000, 0.9659258262890683122, 1.000000000000000000, 0.9659258262890683122, 1.000000000000000000, 0.9659258262890683122, 1.000000000000000000, 0.9659258262890683122, 1.000000000000000000, 0.9659258262890683122, 1.000000000000000000, 0.9659258262890683122, 1.000000000000000000, 0.9659258262890683122, 1.000000000000000000, 0.9659258262890683122, 1.000000000000000000, 0.9659258262890683122, 1.000000000000000000, 0.9659258262890683122, 1.000000000000000000, 0.9659258262890683122, 1.000000000000000000, 0.9659258262890683122, 1.000000000000000000, 0.9659258262890683122, 1.000000000000000000, 0.9659258262890683122, 1.000000000000000000, 0.9659258262890683122, 1.000000000000000000, 0.9659258262890683122, 1.000000000000000000, 0.9659258262890683122, 1.000000000000000000, 0.9659258262890683122, 1.000000000000000000, 0.9659258262890683122, 1.000000000000000000, 0.9659258262890683122, 1.000000000000000000, 0.9659258262890683122, 1.000000000000000000, 0.9659258262890683122, 1.000000000000000000, 0.9659258262890683122, 1.000000000000000000, 0.9659258262890683122, 1.000000000000000000, 0.9659258262890683122, 1.000000000000000000, 0.9659258262890683122, 1.000000000000000000, 0.9659258262890683122, 1.000000000000000000, 0.9659258262890683122, 1.000000000000000000, 0.9659258262890683122, 1.000000000000000000, 0.9659258262890683122, 1.000000000000000000, 0.9659258262890683122, 1.000000000000000000, 0.9659258262890683122, 1.000000000000000000, 0.9659258262890683122, 1.000000000000000000, 0.9659258262890683122, 1.000000000000000000, 0.9659258262890683122, 1.000000000000000000, 0.9659258262890683122, 1.000000000000000000, 0.9659258262890683122, 1.000000000000000000, 0.9659258262890683122, 1.000000000000000000, 0.9659258262890683122, 1.000000000000000000, 0.9659258262890683122, 1.000000000000000000, 0.9659258262890683122, 1.000000000000000000, 0.9659258262890683122, 1.000000000000000000, 0.9659258262890683122, 1.000000000000000000, 0.9659258262890683122, 1.000000000000000000, 0.9659258262890683122, 1.000000000000000000, 0.9659258262890683122, 1.000000000000000000, 0.9659258262890683122, 1.000000000000000000, 0.9659258262890683122, 1.000000000000000000, 0.9659258262890683122, 1.000000000000000000, 0.9659258262890683122, 1.000000000000000000, 0.9659258262890683122, 1.000000000000000000, 0.9659258262890683122, 1.000000000000000000, 0.9659258262890683122, 1.000000000000000000, 0.9659258262890683122, 1.000000000000000000, 0.9659258262890683122, 1.000000000000000000, 0.9659258262890683122, 1.000000000000000000, 0.9659258262890683122, 1.000000000000000000, 0.9659258262890683122, 1.000000000000000000, 0.9659258262890683122, 1.000000000000000000, 0.9659258262890683122, 1.000000000000000000, 0.9659258262890683122, 1.000000000000000000, 0.9659258262890683122, 1.000000000000000000, 0.9659258262890683122, 1.000000000000000000, 0.9659258262890683122, 1.000000000000000000, 0.9659258262890683122, 1.000000000000000000, 0.9659258262890683122, 1.000000000000000000, 0.9659258262890683122, 1.000000000000000000, 0.9659258262890683122, 1.000000000000000000, 0.9659258262890683122, 1.000000000000000000, 0.9659258262890683122, 1.000000000000000000, 0.9659258262890683122, 1.000000000000000000, 0.9659258262890683122, 1.000000000000000000, 0.9659258262890683122, 1.000000000000000000, 0.9659258262890683122, 1.000000000000000000, 0.9659258262890683122, 1.000000000000000000, 0.9659258262890683122, 1.000000000000000000, 0.9659258262890683122, 1.000000000000000000, 0.9659258262890683122, 1.000000000000000000, 0.9659258262890683122, 1.000000000000000000, 0.9659258262890683122, 1.000000000000000000, 0.9659258262890683122, 1.000000000000000000, 0.9659258262890683122, 1.000000000000000000, 0.9659258262890683122, 1.000000000000000000, 0.9659258262890683122, 1.000000000000000000, 0.9659258262890683122, 1.000000000000000000, 0.9659258262890683122, 1.000000000000000000, 0.9659258262890683122, 1.000000000000000000, 0.9659258262890683122, 1.000000000000000000, 0.9659258262890683122, 1.000000000000000000, 0.9659258262890683122, 1.000000000000000000, 0.9659258262890683122, 1.000000000000000000, 0.9659258262890683122, 1.000000000000000000, 0.9659258262890683122, 1.000000000000000000, 0.9659258262890683122, 1.000000000000000000, 0.9659258262890683122, 1.000000000000000000, 0.9659258262890683122, 1.000000000000000000, 0.9659258262890683122, 1.000000000000000000, 0.9659258262890683122, 1.000000000000000000, 0.9659258262890683122, 1.000000000000000000, 0.9659258262890683122, 1.000000000000000000, 0.9659258262890683122, 1.000000000000000000, 0.9659258262890683122, 1.000000000000000000, 0.9659258262890683122, 1.000000000000000000, 0.9659258262890683122, 1.000000000000000000, 0.9659258262890683122, 1.000000000000000000, 0.9659258262890683122, 1.000000000000000000, 0.9659258262890683122, 1.000000000000000000, 0.9659258262890683122, 1.000000000000000000, 0.9659258262890683122, 1.000000000000000000, 0.9659258262890683122, 1.000000000000000000, 0.9659258262890683122, 1.000000000000000000, 0.9659258262890683122, 1.000000000000000000, 0.9659258262890683122, 1.000000000000000000, 0.9659258262890683122, 1.000000000000000000, 0.9659258262890683122, 1.000000000000000000, 0.9659258262890683122, 1.000000000000000000, 0.9659258262890683122, 1.000000000000000000, 0.9659258262890683122, 1.000000000000000000, 0.9659258262890683122, 1.000000000000000000, 0.9659258262890683122, 1.000000000000000000, 0.9659258262890683122, 1.000000000000000000, 0.9659258262890683122, 1.000000000000000000, 0.9659258262890683122, 1.000000000000000000, 0.9659258262890683122, 1.000000000000000000, 0.9659258262890683122, 1.000000000000000000, 0.9659258262890683122, 1.000000000000000000, 0.9659258262890683122, 1.000000000000000000, 0.9659258262890683122, 1.000000000000000000, 0.9659258262890683122, 1.000000000000000000, 0.9659258262890683122, 1.000000000000000000, 0.9659258262890683122, 1.000000000000000000, 0.9659258262890683122, 1.000000000000000000, 0.9659258262890683122, 1.000000000000000000, 0.9659258262890683122, 1.000000000000000000, 0.9659258262890683122, 1.000000000000000000, 0.9659258262890683122, 1.000000000000000000, 0.9659258262890683122, 1.000000000000000000, 0.9659258262890683122, 1.000000000000000000, 0.9659258262890683122, 1.000000000000000000, 0.9659258262890683122, 1.000000000000000000, 0.9659258262890683122, 1.000000000000000000, 0.9659258262890683122, 1.000000000000000000, 0.9659258262890683122, 1.000000000000000000, 0.9659258262890683122, 1.000000000000000000, 0.9659258262890683122, 1.000000000000000000, 0.9659258262890683122, 1.000000000000000000, 0.9659258262890683122, 1.000000000000000000, 0.9659258262890683122, 1.000000000000000000, 0.9659258262890683122, 1.000000000000000000, 0.9659258262890683122, 1.000000000000000000, 0.9659258262890683122, 1.000000000000000000, 0.9659258262890683122, 1.000000000000000000, 0.9659258262890683122, 1.000000000000000000, 0.9659258262890683122, 1.000000000000000000, 0.9659258262890683122, 1.000000000000000000, 0.9659258262890683122, 1.000000000000000000, 0.9659258262890683122, 1.000000000000000000, 0.9659258262890683122, 1.000000000000000000, 0.9659258262890683122, 1.000000000000000000, 0.9659258262890683122, 1.000000000000000000, 0.9659258262890683122, 1.000000000000000000, 0.9659258262890683122, 1.000000000000000000, 0.9659258262890683122, 1.000000000000000000, 0.9659258262890683122, 1.000000000000000000, 0.9659258262890683122, 1.000000000000000000, 0.9659258262890683122, 1.000000000000000000),
 ( 1.000000000000000000, 0.9659258262890683122, 1.000000000000000000, 0.9659258262890683122, 1.000000000000000000, 0.9659258262890683122, 1.000000000000000000, 0.9659258262890683122, 1.000000000000000000, 0.9659258262890683122, 1.000000000000000000, 0.9659258262890683122, 1.000000000000000000, 0.9659258262890683122, 1.000000000000000000, 0.9659258262890683122, 1.000000000000000000, 0.9659258262890683122, 1.000000000000000000, 0.9659258262890683122, 1.000000000000000000, 0.9659258262890683122, 1.000000000000000000, 0.9659258262890683122, 1.000000000000000000, 0.9659258262890683122, 1.000000000000000000, 0.9659258262890683122, 1.000000000000000000, 0.9659258262890683122, 1.000000000000000000, 0.9659258262890683122, 1.000000000000000000, 0.9659258262890683122, 1.000000000000000000, 0.9659258262890683122, 1.000000000000000000, 0.9659258262890683122, 1.000000000000000000, 0.9659258262890683122, 1.000000000000000000, 0.9659258262890683122, 1.000000000000000000, 0.9659258262890683122, 1.000000000000000000, 0.9659258262890683122, 1.000000000000000000, 0.9659258262890683122, 1.000000000000000000, 0.9659258262890683122, 1.000000000000000000, 0.9659258262890683122, 1.000000000000000000, 0.9659258262890683122, 1.000000000000000000, 0.9659258262890683122, 1.000000000000000000, 0.9659258262890683122, 1.000000000000000000, 0.9659258262890683122, 1.000000000000000000, 0.9659258262890683122, 1.000000000000000000, 0.9659258262890683122, 1.000000000000000000, 0.9659258262890683122, 1.000000000000000000, 0.9659258262890683122, 1.000000000000000000, 0.9659258262890683122, 1.000000000000000000, 0.9659258262890683122, 1.000000000000000000, 0.9659258262890683122, 1.000000000000000000, 0.9659258262890683122, 1.000000000000000000, 0.9659258262890683122, 1.000000000000000000, 0.9659258262890683122, 1.000000000000000000, 0.9659258262890683122, 1.000000000000000000, 0.9659258262890683122, 1.000000000000000000, 0.9659258262890683122, 1.000000000000000000, 0.9659258262890683122, 1.000000000000000000, 0.9659258262890683122, 1.000000000000000000, 0.9659258262890683122, 1.000000000000000000, 0.9659258262890683122, 1.000000000000000000, 0.9659258262890683122, 1.000000000000000000, 0.9659258262890683122, 1.000000000000000000, 0.9659258262890683122, 1.000000000000000000, 0.9659258262890683122, 1.000000000000000000, 0.9659258262890683122, 1.000000000000000000, 0.9659258262890683122, 1.000000000000000000, 0.9659258262890683122, 1.000000000000000000, 0.9659258262890683122, 1.000000000000000000, 0.9659258262890683122, 1.000000000000000000, 0.9659258262890683122, 1.000000000000000000, 0.9659258262890683122, 1.000000000000000000, 0.9659258262890683122, 1.000000000000000000, 0.9659258262890683122, 1.000000000000000000, 0.9659258262890683122, 1.000000000000000000, 0.9659258262890683122, 1.000000000000000000, 0.9659258262890683122, 1.000000000000000000, 0.9659258262890683122, 1.000000000000000000, 0.9659258262890683122, 1.000000000000000000, 0.9659258262890683122, 1.000000000000000000, 0.9659258262890683122, 1.000000000000000000, 0.9659258262890683122, 1.000000000000000000, 0.9659258262890683122, 1.000000000000000000, 0.9659258262890683122, 1.000000000000000000, 0.9659258262890683122, 1.000000000000000000, 0.9659258262890683122, 1.000000000000000000, 0.9659258262890683122, 1.000000000000000000, 0.9659258262890683122, 1.000000000000000000, 0.9659258262890683122, 1.000000000000000000, 0.9659258262890683122, 1.000000000000000000, 0.9659258262890683122, 1.000000000000000000, 0.9659258262890683122, 1.000000000000000000, 0.9659258262890683122, 1.000000000000000000, 0.9659258262890683122, 1.000000000000000000, 0.9659258262890683122, 1.000000000000000000, 0.9659258262890683122, 1.000000000000000000, 0.9659258262890683122, 1.000000000000000000, 0.9659258262890683122, 1.000000000000000000, 0.9659258262890683122, 1.000000000000000000, 0.9659258262890683122, 1.000000000000000000, 0.9659258262890683122, 1.000000000000000000, 0.9659258262890683122, 1.000000000000000000, 0.9659258262890683122, 1.000000000000000000, 0.9659258262890683122, 1.000000000000000000, 0.9659258262890683122, 1.000000000000000000, 0.9659258262890683122, 1.000000000000000000, 0.9659258262890683122, 1.000000000000000000, 0.9659258262890683122, 1.000000000000000000, 0.9659258262890683122, 1.000000000000000000, 0.9659258262890683122, 1.000000000000000000, 0.9659258262890683122, 1.000000000000000000, 0.9659258262890683122, 1.000000000000000000, 0.9659258262890683122, 1.000000000000000000, 0.9659258262890683122, 1.000000000000000000, 0.9659258262890683122, 1.000000000000000000, 0.9659258262890683122, 1.000000000000000000, 0.9659258262890683122, 1.000000000000000000, 0.9659258262890683122, 1.000000000000000000, 0.9659258262890683122, 1.000000000000000000, 0.9659258262890683122, 1.000000000000000000, 0.9659258262890683122, 1.000000000000000000, 0.9659258262890683122, 1.000000000000000000, 0.9659258262890683122, 1.000000000000000000, 0.9659258262890683122, 1.000000000000000000, 0.9659258262890683122, 1.000000000000000000, 0.9659258262890683122, 1.000000000000000000, 0.9659258262890683122, 1.000000000000000000, 0.9659258262890683122, 1.000000000000000000, 0.9659258262890683122, 1.000000000000000000, 0.9659258262890683122, 1.000000000000000000, 0.9659258262890683122, 1.000000000000000000, 0.9659258262890683122, 1.000000000000000000, 0.9659258262890683122, 1.000000000000000000, 0.9659258262890683122, 1.000000000000000000, 0.9659258262890683122, 1.000000000000000000, 0.9659258262890683122, 1.000000000000000000, 0.9659258262890683122, 1.000000000000000000, 0.9659258262890683122, 1.000000000000000000, 0.9659258262890683122, 1.000000000000000000, 0.9659258262890683122, 1.000000000000000000, 0.9659258262890683122, 1.000000000000000000, 0.9659258262890683122, 1.000000000000000000, 0.9659258262890683122, 1.000000000000000000, 0.9659258262890683122, 1.000000000000000000, 0.9659258262890683122, 1.000000000000000000, 0.9659258262890683122, 1.000000000000000000, 0.9659258262890683122, 1.000000000000000000, 0.9659258262890683122, 1.000000000000000000, 0.9659258262890683122, 1.000000000000000000, 0.9659258262890683122, 1.000000000000000000, 0.9659258262890683122, 1.000000000000000000, 0.9659258262890683122, 1.000000000000000000, 0.9659258262890683122, 1.000000000000000000, 0.9659258262890683122, 1.000000000000000000, 0.9659258262890683122, 1.000000000000000000, 0.9659258262890683122, 1.000000000000000000, 0.9659258262890683122, 1.000000000000000000, 0.9659258262890683122, 1.000000000000000000, 0.9659258262890683122, 1.000000000000000000, 0.9659258262890683122, 1.000000000000000000, 0.9659258262890683122, 1.000000000000000000, 0.9659258262890683122, 1.000000000000000000, 0.9659258262890683122, 1.000000000000000000, 0.9659258262890683122, 1.000000000000000000, 0.9659258262890683122, 1.000000000000000000, 0.9659258262890683122, 1.000000000000000000, 0.9659258262890683122, 1.000000000000000000, 0.9659258262890683122, 1.000000000000000000, 0.9659258262890683122, 1.000000000000000000, 0.9659258262890683122, 1.000000000000000000, 0.9659258262890683122, 1.000000000000000000, 0.9659258262890683122, 1.000000000000000000, 0.9659258262890683122, 1.000000000000000000, 0.9659258262890683122, 1.000000000000000000, 0.9659258262890683122, 1.000000000000000000, 0.9659258262890683122, 1.000000000000000000, 0.9659258262890683122, 1.000000000000000000, 0.9659258262890683122, 1.000000000000000000, 0.9659258262890683122, 1.000000000000000000, 0.9659258262890683122, 1.000000000000000000, 0.9659258262890683122, 1.000000000000000000, 0.9659258262890683122, 1.000000000000000000, 0.9659258262890683122, 1.000000000000000000, 0.9659258262890683122, 1.000000000000000000, 0.9659258262890683122, 1.000000000000000000, 0.9659258262890683122, 1.000000000000000000, 0.9659258262890683122, 1.000000000000000000, 0.9659258262890683122, 1.000000000000000000, 0.9659258262890683122, 1.000000000000000000, 0.9659258262890683122, 1.000000000000000000, 0.9659258262890683122, 1.000000000000000000, 0.9659258262890683122, 1.000000000000000000, 0.9659258262890683122, 1.000000000000000000, 0.9659258262890683122, 1.000000000000000000, 0.9659258262890683122, 1.000000000000000000, 0.9659258262890683122, 1.000000000000000000, 0.9659258262890683122, 1.000000000000000000, 0.9659258262890683122, 1.000000000000000000, 0.9659258262890683122, 1.000000000000000000, 0.9659258262890683122, 1.000000000000000000, 0.9659258262890683122, 1.000000000000000000, 0.9659258262890683122, 1.000000000000000000, 0.9659258262890683122, 1.000000000000000000, 0.9659258262890683122, 1.000000000000000000, 0.9659258262890683122, 1.000000000000000000, 0.9659258262890683122, 1.000000000000000000, 0.9659258262890683122, 1.000000000000000000, 0.9659258262890683122, 1.000000000000000000, 0.9659258262890683122, 1.000000000000000000, 0.9659258262890683122, 1.000000000000000000, 0.9659258262890683122, 1.000000000000000000, 0.9659258262890683122, 1.000000000000000000, 0.9659258262890683122, 1.000000000000000000, 0.9659258262890683122, 1.000000000000000000, 0.9659258262890683122, 1.000000000000000000, 0.9659258262890683122, 1.000000000000000000, 0.9659258262890683122, 1.000000000000000000, 0.9659258262890683122, 1.000000000000000000, 0.9659258262890683122, 1.000000000000000000, 0.9659258262890683122, 1.000000000000000000, 0.9659258262890683122, 1.000000000000000000, 0.9659258262890683122, 1.000000000000000000, 0.9659258262890683122, 1.000000000000000000, 0.9659258262890683122, 1.000000000000000000, 0.9659258262890683122, 1.000000000000000000, 0.9659258262890683122, 1.000000000000000000, 0.9659258262890683122, 1.000000000000000000, 0.9659258262890683122, 1.000000000000000000, 0.9659258262890683122, 1.000000000000000000, 0.9659258262890683122, 1.000000000000000000, 0.9659258262890683122, 1.000000000000000000, 0.9659258262890683122, 1.000000000000000000, 0.9659258262890683122, 1.000000000000000000, 0.9659258262890683122, 1.000000000000000000, 0.9659258262890683122, 1.000000000000000000, 0.9659258262890683122, 1.000000000000000000, 0.9659258262890683122, 1.000000000000000000, 0.9659258262890683122, 1.000000000000000000, 0.9659258262890683122, 1.000000000000000000, 0.9659258262890683122, 1.000000000000000000, 0.9659258262890683122, 1.000000000000000000, 0.9659258262890683122, 1.000000000000000000, 0.9659258262890683122, 1.000000000000000000, 0.9659258262890683122, 1.000000000000000000, 0.9659258262890683122, 1.000000000000000000, 0.9659258262890683122, 1.000000000000000000, 0.9659258262890683122, 1.000000000000000000, 0.9659258262890683122, 1.000000000000000000, 0.9659258262890683122, 1.000000000000000000, 0.9659258262890683122, 1.000000000000000000, 0.9659258262890683122, 1.000000000000000000, 0.9659258262890683122, 1.000000000000000000, 0.9659258262890683122, 1.000000000000000000, 0.9659258262890683122, 1.000000000000000000, 0.9659258262890683122, 1.000000000000000000, 0.9659258262890683122, 1.000000000000000000, 0.9659258262890683122, 1.000000000000000000, 0.9659258262890683122, 1.000000000000000000, 0.9659258262890683122, 1.000000000000000000, 0.9659258262890683122, 1.000000000000000000, 0.9659258262890683122, 1.000000000000000000, 0.9659258262890683122, 1.000000000000000000, 0.9659258262890683122, 1.000000000000000000, 0.9659258262890683122, 1.000000000000000000, 0.9659258262890683122, 1.000000000000000000, 0.9659258262890683122, 1.000000000000000000, 0.9659258262890683122, 1.000000000000000000, 0.9659258262890683122, 1.000000000000000000, 0.9659258262890683122, 1.000000000000000000) ) ) 
 REPRESENTATION_ITEM ( '' )  SURFACE ( )  );
#19404=DIRECTION ( 'NONE',  ( 0.7071067811865472397, 0.000000000000000000, 0.7071067811865476838 ) ) ;
#19405=CARTESIAN_POINT ( 'NONE',  ( 1.476377952755906220, 0.1660481256975883668, -0.3530559997133364547 ) ) ;
#19406=CARTESIAN_POINT ( 'NONE',  ( 1.377952755905512472, 0.2952755905511811885, 0.000000000000000000 ) ) ;
#19408=CARTESIAN_POINT ( 'NONE',  ( -1.568241469816272105, -0.3162353388693409650, -0.4822834645669289433 ) ) ;
#19409=CARTESIAN_POINT ( 'NONE',  ( -1.017060367454067249, -0.3162353388693409650, -0.4822834645669289433 ) ) ;
#19413=CARTESIAN_POINT ( 'NONE',  ( -0.09186351706036663400, -0.3690944881889763329, 0.3153832671262228327 ) ) ;
#19416=CARTESIAN_POINT ( 'NONE',  ( 0.1771653543307093182, 0.1660481256975885056, 0.3530559997133364547 ) ) ;
#19417=CARTESIAN_POINT ( 'NONE',  ( 0.5052493438320215802, 0.2952755905511811885, 0.1292274648535926551 ) ) ;
#19420=CARTESIAN_POINT ( 'NONE',  ( -0.2559055118110227234, -0.4536011799217367080, 0.2665933059059888421 ) ) ;
#19421=CARTESIAN_POINT ( 'NONE',  ( 0.7152230971128616943, -0.05778040916215522460, 0.4822834645669289988 ) ) ;
#19422=CARTESIAN_POINT ( 'NONE',  ( 1.017060367454068581, -0.08942795157528024563, -0.3641732283464568787 ) ) ;
#19423=CARTESIAN_POINT ( 'NONE',  ( 0.1574803149606306130, -0.1870078740157480879, -0.4822834645669291653 ) ) ;
#19425=CARTESIAN_POINT ( 'NONE',  ( -0.7742782152230962556, -0.4281496062992127816, -0.4176697321401328100 ) ) ;
#19426=CARTESIAN_POINT ( 'NONE',  ( -1.443569553805773564, -0.5023911411419708095, 0.1820866141732285504 ) ) ;
#19427=CARTESIAN_POINT ( 'NONE',  ( -0.6430446194225716283, -0.4281496062992124485, 0.4176697321401328655 ) ) ;
#19430=ORIENTED_EDGE ( 'NONE', *, *, #9579, .T. ) ;
#19432=CARTESIAN_POINT ( 'NONE',  ( -0.1574803149606292529, -0.1870078740157480879, -0.4822834645669291653 ) ) ;
#19434=CARTESIAN_POINT ( 'NONE',  ( -0.5839895013123351797, 0.2952755905511810774, -0.1292274648535930714 ) ) ;
#19435=CARTESIAN_POINT ( 'NONE',  ( 1.305774278215223960, 0.2952755905511810774, -0.1292274648535930714 ) ) ;
#19436=CARTESIAN_POINT ( 'NONE',  ( 1.082677165354331228, -0.5400638737290844871, 0.3530559997133364547 ) ) ;
#19437=CARTESIAN_POINT ( 'NONE',  ( 0.6364829396325465405, -0.05778040916215522460, 0.4822834645669289988 ) ) ;
#19438=CARTESIAN_POINT ( 'NONE',  ( 0.1902887139107617975, -0.6692913385826773087, -0.1292274648535924053 ) ) ;
#19440=CARTESIAN_POINT ( 'NONE',  ( -1.174540682414697335, -0.3162353388693409650, -0.4822834645669289433 ) ) ;
#19441=CARTESIAN_POINT ( 'NONE',  ( -0.2755905511811015396, -0.6692913385826771977, 8.415575281601705876E-17 ) ) ;
#19443=CARTESIAN_POINT ( 'NONE',  ( 0.08530183727034192087, -0.08942795157527998196, 0.3641732283464567121 ) ) ;
#19445=CARTESIAN_POINT ( 'NONE',  ( -0.1377952755905504645, 0.1660481256975885056, 0.3530559997133364547 ) ) ;
#19447=CARTESIAN_POINT ( 'NONE',  ( 1.030183727034121421, -0.3162353388693409650, -0.4822834645669289433 ) ) ;
#19448=CARTESIAN_POINT ( 'NONE',  ( 0.5183727034120741983, 0.2066929133858267098, -0.1054918080437494132 ) ) ;
#19450=VERTEX_POINT ( 'NONE', #72922 ) ;
#19451=CARTESIAN_POINT ( 'NONE',  ( 0.3740157480314966754, -0.5400638737290844871, 0.3530559997133364547 ) ) ;
#19452=CARTESIAN_POINT ( 'NONE',  ( -0.1115485564304456306, 0.1771653543307087075, -0.09757992244046823083 ) ) ;
#19453=CARTESIAN_POINT ( 'NONE',  ( 1.318897637795276356, -0.4536011799217367080, 0.2665933059059888421 ) ) ;
#19454=CARTESIAN_POINT ( 'NONE',  ( -0.06680712611108347021, -4.070224344450961593E-15, 0.3627989612356168347 ) ) ;
#19457=CARTESIAN_POINT ( 'NONE',  ( 1.679790026246720025, 0.1283753931104748280, 0.1820866141732283561 ) ) ;
#19458=CARTESIAN_POINT ( 'NONE',  ( -1.437007874015747477, 0.1660481256975883668, -0.3530559997133364547 ) ) ;
#19459=CONICAL_SURFACE ( 'NONE', #6055, 3.543307086614173151, 0.7853981633974691512 ) ;
#19461=CARTESIAN_POINT ( 'NONE',  ( 0.1312335958005255154, -0.6046776061558807314, 0.2411417322834647770 ) ) ;
#19462=CARTESIAN_POINT ( 'NONE',  ( -1.174540682414697335, -0.05778040916215522460, 0.4822834645669289988 ) ) ;
#19463=CARTESIAN_POINT ( 'NONE',  ( -1.187664041994750175, -0.05778040916215560624, -0.4822834645669293319 ) ) ;
#19464=CARTESIAN_POINT ( 'NONE',  ( 0.2427821522309716595, -0.3162353388693409650, -0.4822834645669289433 ) ) ;
#19466=CARTESIAN_POINT ( 'NONE',  ( 1.660104986876641320, -0.05778040916215522460, 0.4822834645669289988 ) ) ;
#19467=CARTESIAN_POINT ( 'NONE',  ( 0.7611548556430451917, -0.6046776061558807314, 0.2411417322834647770 ) ) ;
#19468=CARTESIAN_POINT ( 'NONE',  ( 1.010498687664042716, -0.3690944881889763329, 0.3153832671262228327 ) ) ;
#19469=CARTESIAN_POINT ( 'NONE',  ( 0.7998211177050879028, 0.000000000000000000, 0.3464511005275205946 ) ) ;
#19470=CARTESIAN_POINT ( 'NONE',  ( 0.8398950131233602345, -0.5023911411419708095, 0.1820866141732285504 ) ) ;
#19471=CARTESIAN_POINT ( 'NONE',  ( -1.128608923884513837, 0.2306618581243847221, -0.2411417322834647770 ) ) ;
#19473=CARTESIAN_POINT ( 'NONE',  ( 1.036745406824147731, 0.05413385826771666132, 0.4176697321401328100 ) ) ;
#19475=CARTESIAN_POINT ( 'NONE',  ( 0.5314960629921267055, -0.5400638737290844871, 0.3530559997133364547 ) ) ;
#19477=CARTESIAN_POINT ( 'NONE',  ( -1.646981627296586703, -0.2845877964562161244, -0.3641732283464567121 ) ) ;
#19478=CARTESIAN_POINT ( 'NONE',  ( 0.09186351706036827158, 0.05413385826771666132, 0.4176697321401328100 ) ) ;
#19479=CARTESIAN_POINT ( 'NONE',  ( 0.5839895013123367340, -0.5511811023622048555, -0.09757992244046775898 ) ) ;
#19480=CARTESIAN_POINT ( 'NONE',  ( 0.6627296587926517768, -0.6692913385826773087, -0.1292274648535924053 ) ) ;
#19481=CARTESIAN_POINT ( 'NONE',  ( 0.7611548556430454138, 0.1539470093639521697, -0.1968503937007875793 ) ) ;
#19482=CARTESIAN_POINT ( 'NONE',  ( -0.9908136482939626788, -0.5511811023622048555, -0.09757992244046775898 ) ) ;
#19483=CARTESIAN_POINT ( 'NONE',  ( -0.5511811023622041894, -0.1870078740157480879, -0.4822834645669291653 ) ) ;
#19484=CARTESIAN_POINT ( 'NONE',  ( 1.633858267716535639, -0.5400638737290844871, 0.3530559997133364547 ) ) ;
#19485=CARTESIAN_POINT ( 'NONE',  ( -1.194225721784776262, 0.05413385826771626580, -0.4176697321401330321 ) ) ;
#19486=CARTESIAN_POINT ( 'NONE',  ( 1.135170603674541256, -0.6692913385826773087, -0.1292274648535924053 ) ) ;
#19487=CARTESIAN_POINT ( 'NONE',  ( -1.384514435695537005, -0.5511811023622048555, -0.09757992244046775898 ) ) ;
#19488=CARTESIAN_POINT ( 'NONE',  ( -0.7478466213799872531, 1.968503937007873850, -0.5309055118110235227 ) ) ;
#19489=CARTESIAN_POINT ( 'NONE',  ( 1.161417322834646271, 0.1660481256975883668, -0.3530559997133364547 ) ) ;
#19491=CARTESIAN_POINT ( 'NONE',  ( -1.594488188976377563, -0.5400638737290844871, 0.3530559997133364547 ) ) ;
#19492=CARTESIAN_POINT ( 'NONE',  ( -1.561679790026246017, -0.3690944881889765550, -0.3153832671262227771 ) ) ;
#19493=CARTESIAN_POINT ( 'NONE',  ( -0.9580052493438311334, -0.3690944881889763329, 0.3153832671262228327 ) ) ;
#19495=CARTESIAN_POINT ( 'NONE',  ( -0.2296587926509179312, -0.05778040916215522460, 0.4822834645669289988 ) ) ;
#19496=CARTESIAN_POINT ( 'NONE',  ( -0.4330708661417315697, -0.5511811023622047445, 6.969142054262312111E-17 ) ) ;
#19497=CARTESIAN_POINT ( 'NONE',  ( -1.607611548556429737, -0.5511811023622046335, 0.09757992244046803654 ) ) ;
#19498=CARTESIAN_POINT ( 'NONE',  ( 0.8070866141732288002, 0.07958543189024085140, 0.2665933059059887866 ) ) ;
#19499=CARTESIAN_POINT ( 'NONE',  ( 0.3674540682414705883, -0.6046776061558807314, 0.2411417322834647770 ) ) ;
#19500=CARTESIAN_POINT ( 'NONE',  ( 1.338582677165355062, -0.1870078740157480879, -0.4822834645669291653 ) ) ;
#19501=CARTESIAN_POINT ( 'NONE',  ( 0.3346456692913393205, -0.5400638737290845981, -0.3530559997133363437 ) ) ;
#19502=CARTESIAN_POINT ( 'NONE',  ( 0.4396325459317590445, -0.5511811023622046335, 0.09757992244046803654 ) ) ;
#19503=CARTESIAN_POINT ( 'NONE',  ( 1.476377952755906220, 0.1660481256975883668, -0.3530559997133364547 ) ) ;
#19504=CARTESIAN_POINT ( 'NONE',  ( -1.148293963254592542, 0.2952755905511811885, 0.1292274648535926551 ) ) ;
#19505=CARTESIAN_POINT ( 'NONE',  ( -0.6167979002624665030, 0.05413385826771666132, 0.4176697321401328100 ) ) ;
#19508=CARTESIAN_POINT ( 'NONE',  ( -0.05905511811023545637, -0.5400638737290845981, -0.3530559997133363437 ) ) ;
#19509=CARTESIAN_POINT ( 'NONE',  ( 1.135170603674541256, 0.1771653543307087630, 0.09757992244046791164 ) ) ;
#19510=CARTESIAN_POINT ( 'NONE',  ( -0.5971128608923877978, -0.6692913385826773087, -0.1292274648535924053 ) ) ;
#19511=CARTESIAN_POINT ( 'NONE',  ( 0.2165354330708668673, 0.1660481256975883668, -0.3530559997133364547 ) ) ;
#19513=CIRCLE ( 'NONE', #15515, 0.3937007874015748254 ) ;
#19518=CARTESIAN_POINT ( 'NONE',  ( -0.9120734908136475250, 0.1771653543307087630, 0.09757992244046791164 ) ) ;
#19519=CARTESIAN_POINT ( 'NONE',  ( -1.318897637795274802, -0.5400638737290845981, -0.3530559997133363437 ) ) ;
#19521=CARTESIAN_POINT ( 'NONE',  ( 0.2952755905511819101, 0.1660481256975883668, -0.3530559997133364547 ) ) ;
#19522=CARTESIAN_POINT ( 'NONE',  ( 1.161417322834646271, 0.1660481256975883668, -0.3530559997133364547 ) ) ;
#19523=CARTESIAN_POINT ( 'NONE',  ( 0.6364829396325465405, -0.05778040916215522460, 0.4822834645669289988 ) ) ;
#19527=CARTESIAN_POINT ( 'NONE',  ( 0.3215223097112867578, -0.05778040916215522460, 0.4822834645669289988 ) ) ;
#19528=CARTESIAN_POINT ( 'NONE',  ( 0.03937007874015806264, 0.2952755905511811885, 0.000000000000000000 ) ) ;
#19529=CARTESIAN_POINT ( 'NONE',  ( 0.9448818897637802916, -0.1870078740157479769, 0.3641732283464567677 ) ) ;
#19530=CARTESIAN_POINT ( 'NONE',  ( 1.469816272965879911, -0.6046776061558807314, 0.2411417322834647770 ) ) ;
#19532=CARTESIAN_POINT ( 'NONE',  ( 0.3412073490813655186, 0.2306618581243848609, 0.2411417322834645549 ) ) ;
#19533=CARTESIAN_POINT ( 'NONE',  ( 1.174540682414699111, -0.3162353388693405765, 0.4822834645669290543 ) ) ;
#19534=CARTESIAN_POINT ( 'NONE',  ( 0.5708661417322842269, 0.1660481256975885056, 0.3530559997133364547 ) ) ;
#19535=CARTESIAN_POINT ( 'NONE',  ( 1.095800524934383846, -0.08942795157528024563, -0.3641732283464568787 ) ) ;
#19536=CARTESIAN_POINT ( 'NONE',  ( -1.082677165354329896, 0.1660481256975885056, 0.3530559997133364547 ) ) ;
#19537=CARTESIAN_POINT ( 'NONE',  ( -0.9186351706036736120, 0.2306618581243848609, 0.2411417322834645549 ) ) ;
#19538=CARTESIAN_POINT ( 'NONE',  ( 1.332020997375328974, -0.05778040916215560624, -0.4822834645669293319 ) ) ;
#19545=CARTESIAN_POINT ( 'NONE',  ( 1.437007874015748810, -0.5400638737290845981, -0.3530559997133363437 ) ) ;
#19546=CARTESIAN_POINT ( 'NONE',  ( 1.089238845144357537, -0.3690944881889763329, 0.3153832671262228327 ) ) ;
#19548=CARTESIAN_POINT ( 'NONE',  ( 1.187664041994751285, -0.08942795157527998196, 0.3641732283464567121 ) ) ;
#19553=CARTESIAN_POINT ( 'NONE',  ( -1.154855643044618851, 0.1283753931104748280, 0.1820866141732283561 ) ) ;
#19554=CARTESIAN_POINT ( 'NONE',  ( -1.673228346456691717, 0.07958543189024071263, -0.2665933059059888421 ) ) ;
#19555=CARTESIAN_POINT ( 'NONE',  ( -1.246719160104985846, -0.4281496062992127816, -0.4176697321401328100 ) ) ;
#19556=CARTESIAN_POINT ( 'NONE',  ( -0.09842519685039295696, 0.1660481256975883668, -0.3530559997133364547 ) ) ;
#19557=CARTESIAN_POINT ( 'NONE',  ( 1.509186351706037543, -0.4281496062992127816, -0.4176697321401328100 ) ) ;
#19563=CARTESIAN_POINT ( 'NONE',  ( -0.3049517105654738214, -2.191421614605370878E-15, 0.4445507791589071167 ) ) ;
#19564=CARTESIAN_POINT ( 'NONE',  ( -1.095800524934382292, -0.2845877964562161244, -0.3641732283464567121 ) ) ;
#19565=CARTESIAN_POINT ( 'NONE',  ( -1.325459317585300889, 0.05413385826771666132, 0.4176697321401328100 ) ) ;
#19566=CARTESIAN_POINT ( 'NONE',  ( 0.7808398950131241190, -0.05778040916215560624, -0.4822834645669293319 ) ) ;
#19567=AXIS2_PLACEMENT_3D ( 'NONE', #70735, #26539, #78737 ) ;
#19571=CARTESIAN_POINT ( 'NONE',  ( 1.233595800524935227, 0.2306618581243847221, -0.2411417322834647770 ) ) ;
#19572=CARTESIAN_POINT ( 'NONE',  ( -1.456692913385826182, -0.6692913385826771977, 8.415575281601705876E-17 ) ) ;
#19574=CARTESIAN_POINT ( 'NONE',  ( -0.3937007874015740483, -0.1870078740157480601, -0.3641732283464567677 ) ) ;
#19575=CARTESIAN_POINT ( 'NONE',  ( -1.272965879265091305, -0.004921259842519870586, -0.3153832671262229437 ) ) ;
#19577=CARTESIAN_POINT ( 'NONE',  ( -0.4002624671916004129, -0.2845877964562159024, 0.3641732283464567677 ) ) ;
#19578=CARTESIAN_POINT ( 'NONE',  ( 0.2887139107611556010, -0.5023911411419708095, 0.1820866141732285504 ) ) ;
#19579=CARTESIAN_POINT ( 'NONE',  ( 0.03937007874015806264, 0.2952755905511811885, 0.000000000000000000 ) ) ;
#19580=CARTESIAN_POINT ( 'NONE',  ( -0.9973753280839886548, 0.1283753931104748280, 0.1820866141732283561 ) ) ;
#19582=CARTESIAN_POINT ( 'NONE',  ( 1.154855643044620184, 0.2306618581243847221, -0.2411417322834647770 ) ) ;
#19583=EDGE_CURVE ( 'NONE', #32176, #44890, #16904, .T. ) ;
#19584=CARTESIAN_POINT ( 'NONE',  ( -1.482939632545930975, 0.05413385826771666132, 0.4176697321401328100 ) ) ;
#19586=CARTESIAN_POINT ( 'NONE',  ( -0.2362204724409442680, -0.1870078740157480879, -0.4822834645669291653 ) ) ;
#19587=CARTESIAN_POINT ( 'NONE',  ( -1.056430446194224881, -0.6692913385826771977, 0.1292274648535927661 ) ) ;
#19588=CARTESIAN_POINT ( 'NONE',  ( 0.9448818897637802916, -0.1870078740157480601, -0.3641732283464567677 ) ) ;
#19589=CARTESIAN_POINT ( 'NONE',  ( -0.5118110236220466680, -0.5511811023622047445, 6.969142054262312111E-17 ) ) ;
#19590=CARTESIAN_POINT ( 'NONE',  ( -0.5839895013123351797, 0.2952755905511810774, -0.1292274648535930714 ) ) ;
#19591=CARTESIAN_POINT ( 'NONE',  ( -1.522309711286088607, -0.6046776061558807314, 0.2411417322834647770 ) ) ;
#19593=CARTESIAN_POINT ( 'NONE',  ( 1.469816272965879911, -0.5023911411419708095, 0.1820866141732285504 ) ) ;
#19594=CARTESIAN_POINT ( 'NONE',  ( -0.4593175853018364174, -0.4281496062992127816, -0.4176697321401328100 ) ) ;
#19595=CARTESIAN_POINT ( 'NONE',  ( -1.325459317585300889, -0.4281496062992127816, -0.4176697321401328100 ) ) ;
#19598=CARTESIAN_POINT ( 'NONE',  ( -0.7742782152230962556, -0.3690944881889765550, -0.3153832671262227771 ) ) ;
#19599=CARTESIAN_POINT ( 'NONE',  ( 0.6889763779527563470, 0.1660481256975883668, -0.3530559997133364547 ) ) ;
#19600=CARTESIAN_POINT ( 'NONE',  ( -1.043307086614172707, 0.07958543189024071263, -0.2665933059059888421 ) ) ;
#19602=CARTESIAN_POINT ( 'NONE',  ( -1.056430446194224881, 0.2952755905511810774, -0.1292274648535930714 ) ) ;
#19604=CARTESIAN_POINT ( 'NONE',  ( 0.8136482939632553313, -0.6046776061558809534, -0.2411417322834644161 ) ) ;
#19605=CARTESIAN_POINT ( 'NONE',  ( 0.5314960629921267055, -0.5400638737290844871, 0.3530559997133364547 ) ) ;
#19607=CARTESIAN_POINT ( 'NONE',  ( -1.384514435695537005, 0.1771653543307087630, 0.09757992244046791164 ) ) ;
#19612=CARTESIAN_POINT ( 'NONE',  ( 1.082677165354331228, 0.07958543189024071263, -0.2665933059059888421 ) ) ;
#19613=EDGE_CURVE ( 'NONE', #38994, #33309, #69185, .T. ) ;
#19614=CARTESIAN_POINT ( 'NONE',  ( 0.2952755905511816326, -0.4536011799217367080, 0.2665933059059888421 ) ) ;
#19615=CARTESIAN_POINT ( 'NONE',  ( -0.01968503937007793844, -0.5400638737290844871, 0.3530559997133364547 ) ) ;
#19616=CARTESIAN_POINT ( 'NONE',  ( 1.371391076115485719, -0.6692913385826773087, -0.1292274648535924053 ) ) ;
#19618=CARTESIAN_POINT ( 'NONE',  ( 0.3871391076115493490, -0.2845877964562159024, 0.3641732283464567677 ) ) ;
#19619=CARTESIAN_POINT ( 'NONE',  ( -0.5577427821522301654, -0.3162353388693405765, 0.4822834645669290543 ) ) ;
#19620=CARTESIAN_POINT ( 'NONE',  ( -1.220472440944881054, -0.6692913385826771977, 8.415575281601705876E-17 ) ) ;
#19621=CARTESIAN_POINT ( 'NONE',  ( 0.8989501312335964611, 0.2952755905511811885, 0.1292274648535926551 ) ) ;
#19624=AXIS2_PLACEMENT_3D ( 'NONE', #38908, #65007, #64588 ) ;
#19627=CARTESIAN_POINT ( 'NONE',  ( -1.371391076115484831, 0.2952755905511810774, -0.1292274648535930714 ) ) ;
#19628=CARTESIAN_POINT ( 'NONE',  ( -0.4396325459317577122, -0.6692913385826773087, -0.1292274648535924053 ) ) ;
#19629=CARTESIAN_POINT ( 'NONE',  ( -0.6824146981627288167, 0.1283753931104748280, 0.1820866141732283561 ) ) ;
#19630=CARTESIAN_POINT ( 'NONE',  ( -0.8792650918635160906, -0.4281496062992124485, 0.4176697321401328655 ) ) ;
#19633=CARTESIAN_POINT ( 'NONE',  ( -1.646981627296586703, -0.08942795157527998196, 0.3641732283464567121 ) ) ;
#19634=CARTESIAN_POINT ( 'NONE',  ( -1.364829396325458521, 0.2306618581243847221, -0.2411417322834647770 ) ) ;
#19635=CARTESIAN_POINT ( 'NONE',  ( 0.2165354330708668673, 0.1660481256975883668, -0.3530559997133364547 ) ) ;
#19636=CARTESIAN_POINT ( 'NONE',  ( -0.7611548556430438595, -0.6046776061558809534, -0.2411417322834644161 ) ) ;
#19640=CARTESIAN_POINT ( 'NONE',  ( -1.010498687664041384, -0.004921259842519576551, 0.3153832671262227771 ) ) ;
#19643=VERTEX_POINT ( 'NONE', #29944 ) ;
#19644=DIRECTION ( 'NONE',  ( -0.8050726085550657940, -2.493067783899223597E-16, -0.5931762764594871173 ) ) ;
#19645=CARTESIAN_POINT ( 'NONE',  ( -1.227034120734907585, 0.2952755905511811885, 0.1292274648535926551 ) ) ;
#19646=CARTESIAN_POINT ( 'NONE',  ( -0.7086614173228339419, -0.1870078740157479769, 0.4822834645669291653 ) ) ;
#19648=CARTESIAN_POINT ( 'NONE',  ( -1.056430446194224881, 0.2952755905511810774, -0.1292274648535930714 ) ) ;
#19649=CARTESIAN_POINT ( 'NONE',  ( -1.049868766404198794, 0.2306618581243847221, -0.2411417322834647770 ) ) ;
#19651=CARTESIAN_POINT ( 'NONE',  ( -0.006561679790025524116, -0.08942795157528024563, -0.3641732283464568787 ) ) ;
#19654=CARTESIAN_POINT ( 'NONE',  ( -0.3477690288713905509, -0.5511811023622046335, 0.09757992244046803654 ) ) ;
#19655=CARTESIAN_POINT ( 'NONE',  ( -0.7349081364829387342, -0.6046776061558807314, 0.2411417322834647770 ) ) ;
#19656=CARTESIAN_POINT ( 'NONE',  ( 1.377952755905512472, -0.6692913385826771977, 8.415575281601705876E-17 ) ) ;
#19657=CARTESIAN_POINT ( 'NONE',  ( -0.5774278215223089816, -0.6046776061558807314, 0.2411417322834647770 ) ) ;
#19661=CARTESIAN_POINT ( 'NONE',  ( -1.141732283464566011, 0.2952755905511811885, 0.000000000000000000 ) ) ;
#19662=CARTESIAN_POINT ( 'NONE',  ( 1.292650918635171564, 0.2952755905511811885, 0.1292274648535926551 ) ) ;
#19663=CARTESIAN_POINT ( 'NONE',  ( -1.167979002624671470, -0.3690944881889765550, -0.3153832671262227771 ) ) ;
#19664=CARTESIAN_POINT ( 'NONE',  ( -1.272965879265091305, -0.4281496062992124485, 0.4176697321401328655 ) ) ;
#19670=CARTESIAN_POINT ( 'NONE',  ( -0.05249343832020911260, 0.2306618581243848609, 0.2411417322834645549 ) ) ;
#19671=CARTESIAN_POINT ( 'NONE',  ( -1.174540682414697335, -0.08942795157527998196, 0.3641732283464567121 ) ) ;
#19674=CARTESIAN_POINT ( 'NONE',  ( -0.5839895013123351797, 0.2952755905511810774, -0.1292274648535930714 ) ) ;
#19676=CARTESIAN_POINT ( 'NONE',  ( -1.161417322834644716, -0.5400638737290845981, -0.3530559997133363437 ) ) ;
#19677=CARTESIAN_POINT ( 'NONE',  ( -1.036745406824146176, 0.05413385826771626580, -0.4176697321401330321 ) ) ;
#19678=CARTESIAN_POINT ( 'NONE',  ( -0.1706036745406816491, -0.4281496062992124485, 0.4176697321401328655 ) ) ;
#19680=CARTESIAN_POINT ( 'NONE',  ( 0.7677165354330716118, -0.4536011799217367080, 0.2665933059059888421 ) ) ;
#19682=CARTESIAN_POINT ( 'NONE',  ( -0.8530183727034112984, -0.3690944881889765550, -0.3153832671262227771 ) ) ;
#19684=CARTESIAN_POINT ( 'NONE',  ( 0.6824146981627303710, -0.5023911411419708095, 0.1820866141732285504 ) ) ;
#19685=CARTESIAN_POINT ( 'NONE',  ( 1.476377952755906220, 0.07958543189024071263, -0.2665933059059888421 ) ) ;
#19686=CARTESIAN_POINT ( 'NONE',  ( 1.391076115485564868, -0.6046776061558807314, 0.2411417322834647770 ) ) ;
#19687=CARTESIAN_POINT ( 'NONE',  ( -0.08530183727034056085, -0.2845877964562159024, 0.3641732283464567677 ) ) ;
#19689=CARTESIAN_POINT ( 'NONE',  ( -0.6758530183727028406, 0.2952755905511811885, 0.1292274648535926551 ) ) ;
#19690=CARTESIAN_POINT ( 'NONE',  ( 1.423884514435696191, -0.05778040916215522460, 0.4822834645669289988 ) ) ;
#19691=AXIS2_PLACEMENT_3D ( 'NONE', #73943, #28479, #41527 ) ;
#19693=CARTESIAN_POINT ( 'NONE',  ( -0.3871391076115476282, -0.08942795157527998196, 0.3641732283464567121 ) ) ;
#19694=CARTESIAN_POINT ( 'NONE',  ( -0.4068241469816267775, 0.05413385826771626580, -0.4176697321401330321 ) ) ;
#19695=CARTESIAN_POINT ( 'NONE',  ( 0.5314960629921267055, -0.5400638737290844871, 0.3530559997133364547 ) ) ;
#19697=CARTESIAN_POINT ( 'NONE',  ( 0.7874015748031503170, -0.1870078740157479769, 0.3641732283464567677 ) ) ;
#19698=CARTESIAN_POINT ( 'NONE',  ( -0.01312335958005186876, -0.3690944881889763329, 0.3153832671262228327 ) ) ;
#19699=CARTESIAN_POINT ( 'NONE',  ( -0.5052493438320203589, 0.2952755905511810774, -0.1292274648535930714 ) ) ;
#19700=CARTESIAN_POINT ( 'NONE',  ( -1.437007874015747477, -0.5400638737290844871, 0.3530559997133364547 ) ) ;
#19701=CARTESIAN_POINT ( 'NONE',  ( -0.5314960629921250401, 0.07958543189024085140, 0.2665933059059887866 ) ) ;
#19703=CARTESIAN_POINT ( 'NONE',  ( -1.023622047244093558, -0.1870078740157479769, 0.4822834645669291653 ) ) ;
#19706=CARTESIAN_POINT ( 'NONE',  ( 0.02624671916010564918, 0.1283753931104748280, 0.1820866141732283561 ) ) ;
#19707=CARTESIAN_POINT ( 'NONE',  ( -0.6627296587926501115, 0.2952755905511810774, -0.1292274648535930714 ) ) ;
#19708=CARTESIAN_POINT ( 'NONE',  ( -1.233595800524933894, -0.6046776061558809534, -0.2411417322834644161 ) ) ;
#19709=CARTESIAN_POINT ( 'NONE',  ( -1.410761154855641575, -0.2845877964562161244, -0.3641732283464567121 ) ) ;
#19711=CARTESIAN_POINT ( 'NONE',  ( -0.8333333333333323711, 0.1771653543307087630, 0.09757992244046791164 ) ) ;
#19712=CARTESIAN_POINT ( 'NONE',  ( -1.732283464566928277, -0.1870078740157479769, 0.3641732283464567677 ) ) ;
#19713=CARTESIAN_POINT ( 'NONE',  ( 1.338582677165355062, -0.1870078740157480879, -0.4822834645669291653 ) ) ;
#19719=CARTESIAN_POINT ( 'NONE',  ( 1.528871391076116026, -0.5511811023622048555, -0.09757992244046775898 ) ) ;
#19720=CARTESIAN_POINT ( 'NONE',  ( -1.325459317585300889, -0.4281496062992127816, -0.4176697321401328100 ) ) ;
#19721=CARTESIAN_POINT ( 'NONE',  ( 1.410761154855643795, -0.3162353388693405765, 0.4822834645669290543 ) ) ;
#19723=CARTESIAN_POINT ( 'NONE',  ( 1.535433070866142558, 0.1771653543307087630, 0.000000000000000000 ) ) ;
#19725=CARTESIAN_POINT ( 'NONE',  ( 0.7086614173228353852, -0.1870078740157479769, 0.4822834645669291653 ) ) ;
#19726=CARTESIAN_POINT ( 'NONE',  ( -0.1443569553805765515, -0.4281496062992127816, -0.4176697321401328100 ) ) ;
#19727=DIRECTION ( 'NONE',  ( -1.000000000000000000, -3.050063254464715781E-16, 0.000000000000000000 ) ) ;
#19729=AXIS2_PLACEMENT_3D ( 'NONE', #30080, #15829, #9905 ) ;
#19731=CARTESIAN_POINT ( 'NONE',  ( 0.6627296587926515548, 0.1771653543307087630, 0.09757992244046791164 ) ) ;
#19736=CARTESIAN_POINT ( 'NONE',  ( -0.1377952755905504645, 0.1660481256975885056, 0.3530559997133364547 ) ) ;
#19738=CARTESIAN_POINT ( 'NONE',  ( -1.450131233595799651, 0.2952755905511810774, -0.1292274648535930714 ) ) ;
#19739=CARTESIAN_POINT ( 'NONE',  ( 0.4527559055118117182, 0.1660481256975883668, -0.3530559997133364547 ) ) ;
#19740=CARTESIAN_POINT ( 'NONE',  ( 1.135170603674541256, -0.6692913385826773087, -0.1292274648535924053 ) ) ;
#19741=CARTESIAN_POINT ( 'NONE',  ( 1.482939632545932307, 0.05413385826771626580, -0.4176697321401330321 ) ) ;
#19742=CARTESIAN_POINT ( 'NONE',  ( -0.4527559055118102749, -0.5400638737290845981, -0.3530559997133363437 ) ) ;
#19743=CARTESIAN_POINT ( 'NONE',  ( -0.1312335958005241554, 0.2306618581243848609, 0.2411417322834645549 ) ) ;
#19744=CARTESIAN_POINT ( 'NONE',  ( 1.502624671916010790, -0.3162353388693409650, -0.4822834645669289433 ) ) ;
#19745=CARTESIAN_POINT ( 'NONE',  ( 1.345144356955381593, -0.3162353388693409650, -0.4822834645669289433 ) ) ;
#19746=CARTESIAN_POINT ( 'NONE',  ( 1.056430446194226658, 0.2952755905511811885, 0.1292274648535926551 ) ) ;
#19747=CARTESIAN_POINT ( 'NONE',  ( -0.07874015748031421014, -0.1870078740157480879, -0.4822834645669291653 ) ) ;
#19750=CARTESIAN_POINT ( 'NONE',  ( 0.5446194225721792126, -0.2845877964562159024, 0.3641732283464567677 ) ) ;
#19754=CARTESIAN_POINT ( 'NONE',  ( -0.2493438320209966919, -0.004921259842519870586, -0.3153832671262229437 ) ) ;
#19756=CARTESIAN_POINT ( 'NONE',  ( 0.08530183727034192087, -0.3162353388693409650, -0.4822834645669289433 ) ) ;
#19757=CARTESIAN_POINT ( 'NONE',  ( -0.05249343832020938322, -0.6046776061558809534, -0.2411417322834644161 ) ) ;
#19759=CARTESIAN_POINT ( 'NONE',  ( -0.9776902887139098386, -0.6692913385826771977, 0.1292274648535927661 ) ) ;
#19761=CARTESIAN_POINT ( 'NONE',  ( -1.587926509186350810, 0.05413385826771626580, -0.4176697321401330321 ) ) ;
#19762=CARTESIAN_POINT ( 'NONE',  ( -1.595398199321656385, 1.564277624879635509, -0.1559797534342483583 ) ) ;
#19763=CARTESIAN_POINT ( 'NONE',  ( 0.8136482939632553313, 0.1283753931104748280, 0.1820866141732283561 ) ) ;
#19764=CARTESIAN_POINT ( 'NONE',  ( 0.4396325459317593221, 0.2952755905511810774, -0.1292274648535930714 ) ) ;
#19765=CARTESIAN_POINT ( 'NONE',  ( 0.8595800524934390507, -0.3162353388693405765, 0.4822834645669290543 ) ) ;
#19767=CARTESIAN_POINT ( 'NONE',  ( -1.660104986876639543, -0.05778040916215560624, -0.4822834645669293319 ) ) ;
#19770=CARTESIAN_POINT ( 'NONE',  ( 0.01968503937007930540, 0.1660481256975885056, 0.3530559997133364547 ) ) ;
#19773=CARTESIAN_POINT ( 'NONE',  ( -1.397637795275589623, -0.4536011799217368745, -0.2665933059059886201 ) ) ;
#19774=CARTESIAN_POINT ( 'NONE',  ( 1.174540682414699111, -0.05778040916215560624, -0.4822834645669293319 ) ) ;
#19775=CARTESIAN_POINT ( 'NONE',  ( 1.502624671916010790, -0.05778040916215522460, 0.4822834645669289988 ) ) ;
#19776=CARTESIAN_POINT ( 'NONE',  ( 0.2887139107611556010, 0.1283753931104746893, -0.1820866141732285504 ) ) ;
#19777=CARTESIAN_POINT ( 'NONE',  ( 0.3740157480314966754, 0.1660481256975883668, -0.3530559997133364547 ) ) ;
#19779=CARTESIAN_POINT ( 'NONE',  ( 0.4790026246719168435, -0.2845877964562161244, -0.3641732283464567121 ) ) ;
#19781=CARTESIAN_POINT ( 'NONE',  ( -0.02624671916010428221, -0.6046776061558807314, 0.2411417322834647770 ) ) ;
#19783=CARTESIAN_POINT ( 'NONE',  ( -1.391076115485563758, 0.2306618581243848609, 0.2411417322834645549 ) ) ;
#19784=CARTESIAN_POINT ( 'NONE',  ( 0.5905511811023629321, -0.5511811023622047445, 6.969142054262312111E-17 ) ) ;
#19787=CARTESIAN_POINT ( 'NONE',  ( -0.5577427821522301654, -0.05778040916215560624, -0.4822834645669293319 ) ) ;
#19788=CARTESIAN_POINT ( 'NONE',  ( -0.3346456692913377662, 0.07958543189024071263, -0.2665933059059888421 ) ) ;
#19790=CARTESIAN_POINT ( 'NONE',  ( -0.7611548556430438595, 0.2306618581243848609, 0.2411417322834645549 ) ) ;
#19791=CARTESIAN_POINT ( 'NONE',  ( -0.1640419947506553400, -0.05778040916215560624, -0.4822834645669293319 ) ) ;
#19792=CARTESIAN_POINT ( 'NONE',  ( 0.1968503937007881344, 0.1771653543307087630, 0.000000000000000000 ) ) ;
#19795=CARTESIAN_POINT ( 'NONE',  ( 8.195543980992789655E-16, -0.1870078740157480879, -0.4822834645669291653 ) ) ;
#19799=CARTESIAN_POINT ( 'NONE',  ( 0.9055118110236227702, 0.1771653543307087630, 0.000000000000000000 ) ) ;
#19800=CARTESIAN_POINT ( 'NONE',  ( 1.279527559055118724, 0.1660481256975885056, 0.3530559997133364547 ) ) ;
#19801=CARTESIAN_POINT ( 'NONE',  ( -0.6299212598425188991, -0.1870078740157479769, 0.3641732283464567677 ) ) ;
#19802=CARTESIAN_POINT ( 'NONE',  ( -1.318897637795274802, -0.4536011799217368745, -0.2665933059059886201 ) ) ;
#19803=CARTESIAN_POINT ( 'NONE',  ( -0.7020997375328074108, -0.05778040916215522460, 0.4822834645669289988 ) ) ;
#19804=CARTESIAN_POINT ( 'NONE',  ( -0.02624671916010428221, -0.6046776061558807314, 0.2411417322834647770 ) ) ;
#19805=CARTESIAN_POINT ( 'NONE',  ( 0.6364829396325465405, -0.2845877964562161244, -0.3641732283464567121 ) ) ;
#19807=CARTESIAN_POINT ( 'NONE',  ( 1.030183727034121421, -0.2845877964562161244, -0.3641732283464567121 ) ) ;
#19808=EDGE_CURVE ( 'NONE', #33309, #68837, #66219, .T. ) ;
#19809=CARTESIAN_POINT ( 'NONE',  ( 0.1312335958005257930, 0.2306618581243847221, -0.2411417322834647770 ) ) ;
#19811=CARTESIAN_POINT ( 'NONE',  ( -0.3346456692913377662, -0.5400638737290844871, 0.3530559997133364547 ) ) ;
#19813=CARTESIAN_POINT ( 'NONE',  ( 1.581364829396326277, -0.08942795157527998196, 0.3641732283464567121 ) ) ;
#19814=CARTESIAN_POINT ( 'NONE',  ( 0.2755905511811031494, 0.2952755905511811885, 0.000000000000000000 ) ) ;
#19815=CARTESIAN_POINT ( 'NONE',  ( 0.2887139107611556010, 0.2306618581243847221, -0.2411417322834647770 ) ) ;
#19816=CARTESIAN_POINT ( 'NONE',  ( 0.5905511811023628210, 0.2066929133858268208, 0.000000000000000000 ) ) ;
#19817=CARTESIAN_POINT ( 'NONE',  ( -0.09186351706036663400, -0.3690944881889763329, 0.3153832671262228327 ) ) ;
#19818=CARTESIAN_POINT ( 'NONE',  ( 0.6364829396325465405, -0.3162353388693409650, -0.4822834645669289433 ) ) ;
#19819=CARTESIAN_POINT ( 'NONE',  ( -0.5249343832020990641, -0.5023911411419708095, -0.1820866141732282451 ) ) ;
#19820=CARTESIAN_POINT ( 'NONE',  ( -0.7283464566929126471, -0.5400638737290844871, 0.3530559997133364547 ) ) ;
#19822=CARTESIAN_POINT ( 'NONE',  ( 0.02624671916010564918, 0.2306618581243848609, 0.2411417322834645549 ) ) ;
#19823=CARTESIAN_POINT ( 'NONE',  ( -1.122047244094487306, 0.1660481256975883668, -0.3530559997133364547 ) ) ;
#19824=CARTESIAN_POINT ( 'NONE',  ( -0.8989501312335946848, 0.1771653543307087075, -0.09757992244046823083 ) ) ;
#19825=CARTESIAN_POINT ( 'NONE',  ( 0.3346456692913390985, 0.1660481256975885056, 0.3530559997133364547 ) ) ;
#19826=CARTESIAN_POINT ( 'NONE',  ( -1.200787401574802349, 0.1660481256975883668, -0.3530559997133364547 ) ) ;
#19827=CARTESIAN_POINT ( 'NONE',  ( -0.2887139107611542133, -0.6046776061558809534, -0.2411417322834644161 ) ) ;
#19830=CARTESIAN_POINT ( 'NONE',  ( -0.9055118110236215490, 0.2952755905511811885, 0.000000000000000000 ) ) ;
#19831=CARTESIAN_POINT ( 'NONE',  ( 1.496062992125984703, -0.1870078740157480879, -0.4822834645669291653 ) ) ;
#19832=CARTESIAN_POINT ( 'NONE',  ( 1.463254593175853824, -0.6692913385826771977, 0.1292274648535927661 ) ) ;
#19835=CARTESIAN_POINT ( 'NONE',  ( -1.397637795275589623, 0.1660481256975885056, 0.3530559997133364547 ) ) ;
#19838=VERTEX_POINT ( 'NONE', #71157 ) ;
#19839=CARTESIAN_POINT ( 'NONE',  ( -0.1443569553805765515, -0.3690944881889765550, -0.3153832671262227771 ) ) ;
#19842=CARTESIAN_POINT ( 'NONE',  ( 0.4330708661417329575, -0.6692913385826771977, 8.415575281601705876E-17 ) ) ;
#19843=CARTESIAN_POINT ( 'NONE',  ( 0.4724409448818904789, -0.1870078740157479769, 0.4822834645669291653 ) ) ;
#19845=CARTESIAN_POINT ( 'NONE',  ( -0.5396849562100385356, -4.992347309556208597E-15, 0.3791483426435189319 ) ) ;
#19846=CARTESIAN_POINT ( 'NONE',  ( -0.3346456692913377662, 0.07958543189024071263, -0.2665933059059888421 ) ) ;
#19847=CARTESIAN_POINT ( 'NONE',  ( 0.4965823425844641537, 1.491030243332470917, -0.5309055118110237448 ) ) ;
#19848=CARTESIAN_POINT ( 'NONE',  ( 0.7217847769028878924, 0.05413385826771666132, 0.4176697321401328100 ) ) ;
#19849=CARTESIAN_POINT ( 'NONE',  ( 0.9317585301837276734, -0.3690944881889763329, 0.3153832671262228327 ) ) ;
#19850=CARTESIAN_POINT ( 'NONE',  ( -0.2362204724409440182, -0.1870078740157479769, 0.4822834645669291653 ) ) ;
#19852=CARTESIAN_POINT ( 'NONE',  ( -0.8858267716535425107, -0.5400638737290844871, 0.3530559997133364547 ) ) ;
#19853=CARTESIAN_POINT ( 'NONE',  ( -1.482939632545930975, -0.3690944881889765550, -0.3153832671262227771 ) ) ;
#19854=CARTESIAN_POINT ( 'NONE',  ( -0.8333333333333323711, -0.6692913385826773087, -0.1292274648535924053 ) ) ;
#19855=CARTESIAN_POINT ( 'NONE',  ( 1.384514435695538559, 0.2952755905511810774, -0.1292274648535930714 ) ) ;
#19856=CARTESIAN_POINT ( 'NONE',  ( 1.679790026246720025, 0.1283753931104748280, 0.1820866141732283561 ) ) ;
#19859=CARTESIAN_POINT ( 'NONE',  ( -0.07874015748031421014, -0.1870078740157479769, 0.4822834645669291653 ) ) ;
#19860=VERTEX_POINT ( 'NONE', #64838 ) ;
#19862=CARTESIAN_POINT ( 'NONE',  ( -0.6299212598425188991, -0.1870078740157479769, 0.4822834645669291653 ) ) ;
#19863=CARTESIAN_POINT ( 'NONE',  ( 1.253280839895013710, -0.3162353388693405765, 0.4822834645669290543 ) ) ;
#19864=CARTESIAN_POINT ( 'NONE',  ( 1.437007874015748810, 0.1660481256975885056, 0.3530559997133364547 ) ) ;
#19865=CARTESIAN_POINT ( 'NONE',  ( 0.2296587926509192634, -0.05778040916215560624, -0.4822834645669293319 ) ) ;
#19866=CARTESIAN_POINT ( 'NONE',  ( -0.01968503937007793844, 0.1660481256975883668, -0.3530559997133364547 ) ) ;
#19868=CARTESIAN_POINT ( 'NONE',  ( -1.108923884514435132, -0.3162353388693405765, 0.4822834645669290543 ) ) ;
#19869=CARTESIAN_POINT ( 'NONE',  ( -0.3805774278215216522, 0.05413385826771666132, 0.4176697321401328100 ) ) ;
#19870=CARTESIAN_POINT ( 'NONE',  ( -0.02624671916010428221, 0.1283753931104746893, -0.1820866141732285504 ) ) ;
#19872=CARTESIAN_POINT ( 'NONE',  ( 1.312335958005250269, -0.6046776061558807314, 0.2411417322834647770 ) ) ;
#19873=CARTESIAN_POINT ( 'NONE',  ( -0.5511811023622041894, -0.1870078740157480879, -0.4822834645669291653 ) ) ;
#19874=CARTESIAN_POINT ( 'NONE',  ( 0.2821522309711291809, 0.2066929133858267098, -0.1054918080437494132 ) ) ;
#19875=CARTESIAN_POINT ( 'NONE',  ( 1.062992125984252745, -0.6692913385826771977, 8.415575281601705876E-17 ) ) ;
#19877=ORIENTED_EDGE ( 'NONE', *, *, #47629, .F. ) ;
#19878=VERTEX_POINT ( 'NONE', #32425 ) ;
#19879=CARTESIAN_POINT ( 'NONE',  ( 0.2362204724409456558, -0.1870078740157479769, 0.4822834645669291653 ) ) ;
#19880=CARTESIAN_POINT ( 'NONE',  ( -0.5052493438320203589, -0.5511811023622046335, 0.09757992244046803654 ) ) ;
#19881=CARTESIAN_POINT ( 'NONE',  ( 1.587926509186352586, -0.3690944881889765550, -0.3153832671262227771 ) ) ;
#19885=ADVANCED_FACE ( 'NONE', ( #7606 ), #65695, .F. ) ;
#19886=CARTESIAN_POINT ( 'NONE',  ( 1.200787401574803681, -0.5400638737290845981, -0.3530559997133363437 ) ) ;
#19888=CARTESIAN_POINT ( 'NONE',  ( 0.03280839895013198948, 0.2952755905511811885, 0.1292274648535926551 ) ) ;
#19889=CARTESIAN_POINT ( 'NONE',  ( -1.306827173596998737, 0.000000000000000000, 0.4445507791589060065 ) ) ;
#19890=CARTESIAN_POINT ( 'NONE',  ( -1.614173228346456268, -0.6692913385826771977, 8.415575281601705876E-17 ) ) ;
#19891=CARTESIAN_POINT ( 'NONE',  ( -0.3215223097112853146, -0.3162353388693405765, 0.4822834645669290543 ) ) ;
#19894=CARTESIAN_POINT ( 'NONE',  ( -1.574803149606298192, -0.1870078740157480601, -0.3641732283464567677 ) ) ;
#19895=CARTESIAN_POINT ( 'NONE',  ( 0.3412073490813655186, 0.2306618581243848609, 0.2411417322834645549 ) ) ;
#19896=CARTESIAN_POINT ( 'NONE',  ( 0.9383202099737538715, -0.08942795157528024563, -0.3641732283464568787 ) ) ;
#19897=CARTESIAN_POINT ( 'NONE',  ( -0.03937007874015669567, 0.2952755905511811885, 0.000000000000000000 ) ) ;
#19898=CARTESIAN_POINT ( 'NONE',  ( 0.6430446194225729606, -0.3690944881889765550, -0.3153832671262227771 ) ) ;
#19899=CARTESIAN_POINT ( 'NONE',  ( -1.259842519685038686, -0.1870078740157480879, -0.4822834645669291653 ) ) ;
#19901=CARTESIAN_POINT ( 'NONE',  ( 1.148293963254593875, -0.6692913385826771977, 0.1292274648535927661 ) ) ;
#19903=CARTESIAN_POINT ( 'NONE',  ( 0.8792650918635177559, 0.05413385826771666132, 0.4176697321401328100 ) ) ;
#19905=CARTESIAN_POINT ( 'NONE',  ( 0.4790026246719167324, -0.08942795157527998196, 0.3641732283464567121 ) ) ;
#19906=CARTESIAN_POINT ( 'NONE',  ( 0.7020997375328090762, -0.3162353388693405765, 0.4822834645669290543 ) ) ;
#19908=CARTESIAN_POINT ( 'NONE',  ( -0.9448818897637790704, -0.1870078740157479769, 0.3641732283464567677 ) ) ;
#19909=CARTESIAN_POINT ( 'NONE',  ( -1.161417322834644716, -0.5400638737290845981, -0.3530559997133363437 ) ) ;
#19910=CARTESIAN_POINT ( 'NONE',  ( 1.220472440944882608, 0.2952755905511811885, 0.000000000000000000 ) ) ;
#19911=CARTESIAN_POINT ( 'NONE',  ( -0.9711286089238838626, -0.6046776061558807314, 0.2411417322834647770 ) ) ;
#19912=CARTESIAN_POINT ( 'NONE',  ( 0.7480314960629927956, 0.2952755905511811885, 0.000000000000000000 ) ) ;
#19913=CARTESIAN_POINT ( 'NONE',  ( -1.299212598425196097, 0.1771653543307087630, 0.000000000000000000 ) ) ;
#19914=( BOUNDED_CURVE ( )  B_SPLINE_CURVE ( 2, ( #21653, #59121, #46065, #34289, #34709, #79333, #72591, #21242, #52796, #14112, #33869, #78506, #8204 ),
 .UNSPECIFIED., .F., .F. ) 
 B_SPLINE_CURVE_WITH_KNOTS ( ( 3, 2, 2, 2, 2, 2, 3 ),
 ( 0.3672150842069599186, 0.3674242424242424310, 0.3712121212121212155, 0.3750000000000000000, 0.3787878787878787845, 0.3825757575757575690, 0.3827849157930400814 ),
 .UNSPECIFIED. ) 
 CURVE ( )  GEOMETRIC_REPRESENTATION_ITEM ( )  RATIONAL_B_SPLINE_CURVE ( ( 0.9964447847208419695, 0.9981185001348091834, 1.000000000000000000, 0.9659258262890683122, 1.000000000000000000, 0.9659258262890683122, 1.000000000000000000, 0.9659258262890683122, 1.000000000000000000, 0.9659258262890683122, 1.000000000000000000, 0.9981185001348091834, 0.9964447847208420805 ) ) 
 REPRESENTATION_ITEM ( '' )  );
#19916=CARTESIAN_POINT ( 'NONE',  ( 1.122047244094488860, 0.1660481256975885056, 0.3530559997133364547 ) ) ;
#19920=CARTESIAN_POINT ( 'NONE',  ( 1.200787401574803681, 0.1660481256975885056, 0.3530559997133364547 ) ) ;
#19921=CARTESIAN_POINT ( 'NONE',  ( -1.141732283464566011, -0.5511811023622047445, 6.969142054262312111E-17 ) ) ;
#19922=CARTESIAN_POINT ( 'NONE',  ( 1.463254593175853824, -0.5511811023622046335, 0.09757992244046803654 ) ) ;
#19923=CARTESIAN_POINT ( 'NONE',  ( -1.410761154855641575, -0.2845877964562161244, -0.3641732283464567121 ) ) ;
#19924=CARTESIAN_POINT ( 'NONE',  ( -0.3937007874015740483, -0.1870078740157479769, 0.3641732283464567677 ) ) ;
#19925=CARTESIAN_POINT ( 'NONE',  ( -1.476377952755905110, -0.4536011799217368745, -0.2665933059059886201 ) ) ;
#19926=CARTESIAN_POINT ( 'NONE',  ( 1.056430446194226436, -0.5511811023622048555, -0.09757992244046775898 ) ) ;
#19927=CARTESIAN_POINT ( 'NONE',  ( 0.6430446194225729606, -0.4281496062992127816, -0.4176697321401328100 ) ) ;
#19928=CARTESIAN_POINT ( 'NONE',  ( 1.207349081364829990, -0.6046776061558809534, -0.2411417322834644161 ) ) ;
#19929=CARTESIAN_POINT ( 'NONE',  ( 0.2362204724409456558, -0.1870078740157479769, 0.4822834645669291653 ) ) ;
#19930=CARTESIAN_POINT ( 'NONE',  ( 0.5774278215223103139, -0.5023911411419708095, -0.1820866141732282451 ) ) ;
#19932=CARTESIAN_POINT ( 'NONE',  ( 1.522309711286089939, -0.6046776061558809534, -0.2411417322834644161 ) ) ;
#19933=FACE_OUTER_BOUND ( 'NONE', #16882, .T. ) ;
#19934=CARTESIAN_POINT ( 'NONE',  ( -0.6299212598425188991, -0.1870078740157479769, 0.4822834645669291653 ) ) ;
#19936=CARTESIAN_POINT ( 'NONE',  ( 0.01277272433825663370, 0.004960608223778963273, 0.3437734562760189072 ) ) ;
#19937=CARTESIAN_POINT ( 'NONE',  ( 0.1837270341207354329, 0.2306618581243848609, 0.2411417322834645549 ) ) ;
#19938=CARTESIAN_POINT ( 'NONE',  ( -0.2559055118110227234, -0.5400638737290844871, 0.3530559997133364547 ) ) ;
#19939=CARTESIAN_POINT ( 'NONE',  ( 0.09186351706036799403, -0.4281496062992127816, -0.4176697321401328100 ) ) ;
#19943=CARTESIAN_POINT ( 'NONE',  ( 0.1698998578625684763, 0.000000000000000000, 0.3464511005275205946 ) ) ;
#19945=CARTESIAN_POINT ( 'NONE',  ( -1.102362204724408601, -0.1870078740157479769, 0.3641732283464567677 ) ) ;
#19947=CARTESIAN_POINT ( 'NONE',  ( -1.181102362204723644, -0.1870078740157480879, -0.4822834645669291653 ) ) ;
#19949=CARTESIAN_POINT ( 'NONE',  ( 0.2821522309711292364, 0.2952755905511810774, -0.1292274648535930714 ) ) ;
#19950=CARTESIAN_POINT ( 'NONE',  ( 0.02624671916010564918, 0.1283753931104748280, 0.1820866141732283561 ) ) ;
#19951=CARTESIAN_POINT ( 'NONE',  ( 1.108923884514436242, -0.05778040916215522460, 0.4822834645669289988 ) ) ;
#19952=CARTESIAN_POINT ( 'NONE',  ( 0.2887139107611556010, -0.6046776061558807314, 0.2411417322834647770 ) ) ;
#19956=CARTESIAN_POINT ( 'NONE',  ( 1.417322834645670104, -0.1870078740157480879, -0.4822834645669291653 ) ) ;
#19957=CARTESIAN_POINT ( 'NONE',  ( 0.6955380577427828781, 0.05413385826771626580, -0.4176697321401330321 ) ) ;
#19958=CARTESIAN_POINT ( 'NONE',  ( 0.1509186351706042484, -0.3162353388693405765, 0.4822834645669290543 ) ) ;
#19959=CARTESIAN_POINT ( 'NONE',  ( 1.233595800524935227, 0.2306618581243847221, -0.2411417322834647770 ) ) ;
#19961=CARTESIAN_POINT ( 'NONE',  ( 0.006561679790026889343, -0.05778040916215522460, 0.4822834645669289988 ) ) ;
#19962=CARTESIAN_POINT ( 'NONE',  ( 0.9055118110236227702, 0.2952755905511811885, 0.000000000000000000 ) ) ;
#19963=CARTESIAN_POINT ( 'NONE',  ( 0.4986876640419954376, -0.6046776061558809534, -0.2411417322834644161 ) ) ;
#19964=CARTESIAN_POINT ( 'NONE',  ( 1.023622047244095334, -0.1870078740157479769, 0.3641732283464567677 ) ) ;
#19965=CARTESIAN_POINT ( 'NONE',  ( -0.8727034120734901146, -0.05778040916215560624, -0.4822834645669293319 ) ) ;
#19966=CARTESIAN_POINT ( 'NONE',  ( -1.266404199475064773, -0.3162353388693405765, 0.4822834645669290543 ) ) ;
#19967=CARTESIAN_POINT ( 'NONE',  ( 0.7611548556430451917, -0.6046776061558807314, 0.2411417322834647770 ) ) ;
#19970=CARTESIAN_POINT ( 'NONE',  ( 1.541994750656168645, 0.2952755905511810774, -0.1292274648535930714 ) ) ;
#19973=VERTEX_POINT ( 'NONE', #72370 ) ;
#19974=CARTESIAN_POINT ( 'NONE',  ( 1.391076115485564868, 0.2306618581243847221, -0.2411417322834647770 ) ) ;
#19975=CARTESIAN_POINT ( 'NONE',  ( 1.082677165354331228, -0.4536011799217367080, 0.2665933059059888421 ) ) ;
#19976=CARTESIAN_POINT ( 'NONE',  ( 0.7974104941589355011, -4.927456884911482678E-16, 0.4445507791589062840 ) ) ;
#19981=CARTESIAN_POINT ( 'NONE',  ( -1.266404199475064773, -0.08942795157528024563, -0.3641732283464568787 ) ) ;
#19982=CARTESIAN_POINT ( 'NONE',  ( -1.719160104986876103, -0.004921259842519576551, 0.3153832671262227771 ) ) ;
#19984=CARTESIAN_POINT ( 'NONE',  ( -0.3018372703412066094, 0.05413385826771666132, 0.4176697321401328100 ) ) ;
#19985=CARTESIAN_POINT ( 'NONE',  ( -1.601049868766403650, 0.2306618581243847221, -0.2411417322834647770 ) ) ;
#19989=CARTESIAN_POINT ( 'NONE',  ( 0.8561328129276796206, 8.471767977567108961E-16, -0.4445507791589058955 ) ) ;
#19990=CARTESIAN_POINT ( 'NONE',  ( -1.122047244094487306, 0.07958543189024071263, -0.2665933059059888421 ) ) ;
#19991=CARTESIAN_POINT ( 'NONE',  ( -1.482939632545930975, 0.05413385826771666132, 0.4176697321401328100 ) ) ;
#19992=CARTESIAN_POINT ( 'NONE',  ( 0.5249343832021005074, -0.6046776061558807314, 0.2411417322834647770 ) ) ;
#19996=CARTESIAN_POINT ( 'NONE',  ( 1.213910761154856299, 0.2952755905511811885, 0.1292274648535926551 ) ) ;
#19997=CARTESIAN_POINT ( 'NONE',  ( 1.581364829396326277, -0.08942795157527998196, 0.3641732283464567121 ) ) ;
#19999=CARTESIAN_POINT ( 'NONE',  ( -0.2755905511811018171, 0.1771653543307087630, 0.000000000000000000 ) ) ;
#20000=CARTESIAN_POINT ( 'NONE',  ( -1.528871391076114250, -0.5511811023622046335, 0.09757992244046803654 ) ) ;
#20001=CARTESIAN_POINT ( 'NONE',  ( 1.614173228346457156, 1.929133858267716661, 0.5309055118110233007 ) ) ;
#20002=CARTESIAN_POINT ( 'NONE',  ( 0.3215223097112867578, -0.05778040916215522460, 0.4822834645669289988 ) ) ;
#20003=CARTESIAN_POINT ( 'NONE',  ( -0.3280839895013117347, -0.004921259842519870586, -0.3153832671262229437 ) ) ;
#20004=CARTESIAN_POINT ( 'NONE',  ( 0.1509186351706042484, -0.2845877964562159024, 0.3641732283464567677 ) ) ;
#20005=CARTESIAN_POINT ( 'NONE',  ( -0.08530183727034056085, -0.05778040916215560624, -0.4822834645669293319 ) ) ;
#20006=CARTESIAN_POINT ( 'NONE',  ( -1.213910761154854745, -0.5511811023622046335, 0.09757992244046803654 ) ) ;
#20008=CARTESIAN_POINT ( 'NONE',  ( 0.8530183727034126306, 0.05413385826771626580, -0.4176697321401330321 ) ) ;
#20009=CARTESIAN_POINT ( 'NONE',  ( -1.574803149606298192, -0.1870078740157480879, -0.4822834645669291653 ) ) ;
#20011=CARTESIAN_POINT ( 'NONE',  ( -0.4461942257217840213, 0.2306618581243848609, 0.2411417322834645549 ) ) ;
#20012=CARTESIAN_POINT ( 'NONE',  ( 0.2821522309711292364, -0.5511811023622046335, 0.09757992244046803654 ) ) ;
#20013=CARTESIAN_POINT ( 'NONE',  ( -1.043307086614172041, -0.5400638737290844871, 0.3530559997133364547 ) ) ;
#20014=CARTESIAN_POINT ( 'NONE',  ( 0.7677165354330716118, 0.07958543189024071263, -0.2665933059059888421 ) ) ;
#20015=CARTESIAN_POINT ( 'NONE',  ( -0.1509186351706028884, -0.08942795157527998196, 0.3641732283464567121 ) ) ;
#20016=CARTESIAN_POINT ( 'NONE',  ( -0.7283464566929126471, 0.1660481256975883668, -0.3530559997133364547 ) ) ;
#20017=CARTESIAN_POINT ( 'NONE',  ( -1.456692913385826182, 0.2952755905511811885, 0.000000000000000000 ) ) ;
#20019=CARTESIAN_POINT ( 'NONE',  ( 1.194225721784777594, -0.004921259842519576551, 0.3153832671262227771 ) ) ;
#20020=CARTESIAN_POINT ( 'NONE',  ( 0.3805774278215230400, -0.4281496062992124485, 0.4176697321401328655 ) ) ;
#20021=CARTESIAN_POINT ( 'NONE',  ( -1.601049868766403650, 0.2306618581243847221, -0.2411417322834647770 ) ) ;
#20022=CARTESIAN_POINT ( 'NONE',  ( -1.332020997375327642, -0.3162353388693409650, -0.4822834645669289433 ) ) ;
#20023=ORIENTED_EDGE ( 'NONE', *, *, #35324, .T. ) ;
#20025=CARTESIAN_POINT ( 'NONE',  ( -0.9120734908136475250, -0.5511811023622048555, -0.09757992244046775898 ) ) ;
#20026=CARTESIAN_POINT ( 'NONE',  ( 0.5839895013123367340, -0.6692913385826773087, -0.1292274648535924053 ) ) ;
#20027=CARTESIAN_POINT ( 'NONE',  ( -0.9514435695538050464, -0.2845877964562159024, 0.3641732283464567677 ) ) ;
#20029=CARTESIAN_POINT ( 'NONE',  ( -1.194225721784776262, 0.05413385826771626580, -0.4176697321401330321 ) ) ;
#20030=CARTESIAN_POINT ( 'NONE',  ( 0.9120734908136490793, 0.2952755905511810774, -0.1292274648535930714 ) ) ;
#20031=CARTESIAN_POINT ( 'NONE',  ( 0.3280839895013130669, -0.4281496062992127816, -0.4176697321401328100 ) ) ;
#20032=CARTESIAN_POINT ( 'NONE',  ( 1.469816272965879911, 0.2306618581243847221, -0.2411417322834647770 ) ) ;
#20033=CARTESIAN_POINT ( 'NONE',  ( -1.679790026246718693, 0.1283753931104746893, -0.1820866141732285504 ) ) ;
#20038=CARTESIAN_POINT ( 'NONE',  ( 0.6692913385826778638, -0.5511811023622047445, 6.969142054262312111E-17 ) ) ;
#20039=CARTESIAN_POINT ( 'NONE',  ( 0.3477690288713918276, 0.1771653543307087630, 0.09757992244046791164 ) ) ;
#20040=CARTESIAN_POINT ( 'NONE',  ( -0.09842519685039295696, 0.1660481256975883668, -0.3530559997133364547 ) ) ;
#20041=CARTESIAN_POINT ( 'NONE',  ( 1.148293963254593653, 0.2952755905511810774, -0.1292274648535930714 ) ) ;
#20043=CARTESIAN_POINT ( 'NONE',  ( 0.2559055118110243332, 0.07958543189024085140, 0.2665933059059887866 ) ) ;
#20044=CARTESIAN_POINT ( 'NONE',  ( -0.7086614173228339419, -0.1870078740157479769, 0.4822834645669291653 ) ) ;
#20045=CARTESIAN_POINT ( 'NONE',  ( -1.358267716535432434, -0.5400638737290844871, 0.3530559997133364547 ) ) ;
#20046=CARTESIAN_POINT ( 'NONE',  ( 1.017060367454068803, -0.3162353388693405765, 0.4822834645669290543 ) ) ;
#20051=CARTESIAN_POINT ( 'NONE',  ( -1.410761154855642463, -0.05778040916215522460, 0.4822834645669289988 ) ) ;
#20052=CARTESIAN_POINT ( 'NONE',  ( -0.4461942257217840213, -0.6046776061558809534, -0.2411417322834644161 ) ) ;
#20053=CARTESIAN_POINT ( 'NONE',  ( -0.6167979002624665030, -0.3690944881889765550, -0.3153832671262227771 ) ) ;
#20054=CARTESIAN_POINT ( 'NONE',  ( -0.9580052493438311334, 0.05413385826771626580, -0.4176697321401330321 ) ) ;
#20056=CARTESIAN_POINT ( 'NONE',  ( -0.4613432605871728986, -1.429000049448402363E-15, 0.3954974714151491821 ) ) ;
#20057=CARTESIAN_POINT ( 'NONE',  ( 1.633858267716535639, -0.5400638737290844871, 0.3530559997133364547 ) ) ;
#20058=CARTESIAN_POINT ( 'NONE',  ( -1.325459317585300889, -0.4281496062992127816, -0.4176697321401328100 ) ) ;
#20059=CARTESIAN_POINT ( 'NONE',  ( 0.4265091863517067039, -0.6692913385826773087, -0.1292274648535924053 ) ) ;
#20060=CARTESIAN_POINT ( 'NONE',  ( -0.8989501312335946848, -0.6692913385826771977, 0.1292274648535927661 ) ) ;
#20062=EDGE_CURVE ( 'NONE', #82183, #54857, #62175, .T. ) ;
#20063=CARTESIAN_POINT ( 'NONE',  ( 0.6561679790026253567, 0.2306618581243848609, 0.2411417322834645549 ) ) ;
#20065=CARTESIAN_POINT ( 'NONE',  ( -0.7611548556430438595, -0.5023911411419708095, -0.1820866141732282451 ) ) ;
#20069=CARTESIAN_POINT ( 'NONE',  ( -1.660104986876639543, -0.08942795157528024563, -0.3641732283464568787 ) ) ;
#20070=CARTESIAN_POINT ( 'NONE',  ( -0.9514435695538050464, -0.3162353388693405765, 0.4822834645669290543 ) ) ;
#20071=CARTESIAN_POINT ( 'NONE',  ( -1.227034120734907141, -0.6692913385826773087, -0.1292274648535924053 ) ) ;
#20073=CARTESIAN_POINT ( 'NONE',  ( -1.141732283464566011, -0.6692913385826771977, 8.415575281601705876E-17 ) ) ;
#20074=CARTESIAN_POINT ( 'NONE',  ( -1.456692913385826182, -0.6692913385826771977, 8.415575281601705876E-17 ) ) ;
#20076=CARTESIAN_POINT ( 'NONE',  ( -1.358267716535432434, -0.5400638737290844871, 0.3530559997133364547 ) ) ;
#20078=CARTESIAN_POINT ( 'NONE',  ( 0.1698998578625684763, 0.000000000000000000, 0.3464511005275205946 ) ) ;
#20080=CARTESIAN_POINT ( 'NONE',  ( 0.2559055118110243332, 0.07958543189024085140, 0.2665933059059887866 ) ) ;
#20081=DIRECTION ( 'NONE',  ( 0.000000000000000000, 1.000000000000000000, 0.000000000000000000 ) ) ;
#20083=CARTESIAN_POINT ( 'NONE',  ( -0.3608923884514428360, -0.5511811023622048555, -0.09757992244046775898 ) ) ;
#20084=CARTESIAN_POINT ( 'NONE',  ( -0.8398950131233585692, 0.2306618581243848609, 0.2411417322834645549 ) ) ;
#20085=CARTESIAN_POINT ( 'NONE',  ( 0.7545931758530188826, -0.6692913385826771977, 0.1292274648535927661 ) ) ;
#20086=CARTESIAN_POINT ( 'NONE',  ( -0.3018372703412066094, -0.4281496062992127816, -0.4176697321401328100 ) ) ;
#20088=ORIENTED_EDGE ( 'NONE', *, *, #48534, .T. ) ;
#20090=CARTESIAN_POINT ( 'NONE',  ( -1.115485564304461219, 0.05413385826771626580, -0.4176697321401330321 ) ) ;
#20091=CARTESIAN_POINT ( 'NONE',  ( 1.266404199475066328, -0.05778040916215522460, 0.4822834645669289988 ) ) ;
#20092=CARTESIAN_POINT ( 'NONE',  ( -1.371391076115484831, 0.1771653543307087075, -0.09757992244046823083 ) ) ;
#20097=CARTESIAN_POINT ( 'NONE',  ( -0.3215223097112853146, -0.05778040916215560624, -0.4822834645669293319 ) ) ;
#20098=CARTESIAN_POINT ( 'NONE',  ( -1.601049868766403650, 0.1283753931104746893, -0.1820866141732285504 ) ) ;
#20099=CARTESIAN_POINT ( 'NONE',  ( -0.6102362204724400829, 0.1660481256975885056, 0.3530559997133364547 ) ) ;
#20101=CARTESIAN_POINT ( 'NONE',  ( -1.397637795275589623, 0.1660481256975885056, 0.3530559997133364547 ) ) ;
#20103=CARTESIAN_POINT ( 'NONE',  ( -1.115485564304461219, -0.4281496062992124485, 0.4176697321401328655 ) ) ;
#20104=CARTESIAN_POINT ( 'NONE',  ( -0.3477690288713905509, -0.6692913385826771977, 0.1292274648535927661 ) ) ;
#20107=CARTESIAN_POINT ( 'NONE',  ( 0.8858267716535438430, -0.4536011799217368745, -0.2665933059059886201 ) ) ;
#20109=CARTESIAN_POINT ( 'NONE',  ( 0.8661417322834653598, -0.1870078740157479769, 0.3641732283464567677 ) ) ;
#20110=CARTESIAN_POINT ( 'NONE',  ( 1.561679790026247350, -0.3690944881889763329, 0.3153832671262228327 ) ) ;
#20111=CARTESIAN_POINT ( 'NONE',  ( 1.233595800524935227, -0.6046776061558807314, 0.2411417322834647770 ) ) ;
#20113=CARTESIAN_POINT ( 'NONE',  ( 0.05249343832021075018, -0.5023911411419708095, 0.1820866141732285504 ) ) ;
#20115=CARTESIAN_POINT ( 'NONE',  ( -0.7742782152230962556, -0.4281496062992127816, -0.4176697321401328100 ) ) ;
#20116=CARTESIAN_POINT ( 'NONE',  ( 1.108923884514436242, -0.05778040916215522460, 0.4822834645669289988 ) ) ;
#20118=CARTESIAN_POINT ( 'NONE',  ( -0.6758530183727028406, 0.1771653543307087630, 0.09757992244046791164 ) ) ;
#20120=CARTESIAN_POINT ( 'NONE',  ( 0.2821522309711292364, 0.2952755905511810774, -0.1292274648535930714 ) ) ;
#20122=CARTESIAN_POINT ( 'NONE',  ( 0.9251968503937015864, -0.4536011799217367080, 0.2665933059059888421 ) ) ;
#20123=CARTESIAN_POINT ( 'NONE',  ( -0.03280839895013062252, -0.5511811023622046335, 0.09757992244046803654 ) ) ;
#20124=CARTESIAN_POINT ( 'NONE',  ( -0.2755905511811015396, -0.6692913385826771977, 8.415575281601705876E-17 ) ) ;
#20125=CARTESIAN_POINT ( 'NONE',  ( -1.187664041994750175, -0.05778040916215560624, -0.4822834645669293319 ) ) ;
#20126=CARTESIAN_POINT ( 'NONE',  ( -0.6167979002624665030, -0.3690944881889765550, -0.3153832671262227771 ) ) ;
#20128=CARTESIAN_POINT ( 'NONE',  ( 0.7217847769028878924, 0.05413385826771666132, 0.4176697321401328100 ) ) ;
#20129=CARTESIAN_POINT ( 'NONE',  ( -1.049868766404198794, -0.6046776061558807314, 0.2411417322834647770 ) ) ;
#20132=CARTESIAN_POINT ( 'NONE',  ( 0.2427821522309716595, -0.2845877964562161244, -0.3641732283464567121 ) ) ;
#20133=CARTESIAN_POINT ( 'NONE',  ( -0.8989501312335946848, -0.6692913385826771977, 0.1292274648535927661 ) ) ;
#20134=CARTESIAN_POINT ( 'NONE',  ( -1.010498687664041384, 0.05413385826771666132, 0.4176697321401328100 ) ) ;
#20135=CARTESIAN_POINT ( 'NONE',  ( -1.240157480314959759, -0.4536011799217368745, -0.2665933059059886201 ) ) ;
#20136=CARTESIAN_POINT ( 'NONE',  ( 1.660104986876641320, -0.05778040916215522460, 0.4822834645669289988 ) ) ;
#20137=CARTESIAN_POINT ( 'NONE',  ( -1.030183727034119867, -0.2845877964562159024, 0.3641732283464567677 ) ) ;
#20138=CARTESIAN_POINT ( 'NONE',  ( -0.7611548556430438595, 0.1539470093639523085, 0.1968503937007873850 ) ) ;
#20139=CARTESIAN_POINT ( 'NONE',  ( 1.332020997375328974, -0.05778040916215560624, -0.4822834645669293319 ) ) ;
#20141=EDGE_CURVE ( 'NONE', #69851, #50773, #38013, .T. ) ;
#20144=CARTESIAN_POINT ( 'NONE',  ( 1.561679790026247350, -0.3690944881889763329, 0.3153832671262228327 ) ) ;
#20145=CARTESIAN_POINT ( 'NONE',  ( -1.095800524934382292, -0.05778040916215522460, 0.4822834645669289988 ) ) ;
#20146=CARTESIAN_POINT ( 'NONE',  ( 1.148293963254593653, 0.2952755905511810774, -0.1292274648535930714 ) ) ;
#20148=CARTESIAN_POINT ( 'NONE',  ( 1.646981627296588035, -0.2845877964562159024, 0.3641732283464567677 ) ) ;
#20149=CARTESIAN_POINT ( 'NONE',  ( 0.6233595800524942554, -0.05778040916215560624, -0.4822834645669293319 ) ) ;
#20150=CARTESIAN_POINT ( 'NONE',  ( 0.1049868766404206816, 0.2306618581243848609, 0.2411417322834645549 ) ) ;
#20153=CARTESIAN_POINT ( 'NONE',  ( 0.6496062992125991586, 0.07958543189024085140, 0.2665933059059887866 ) ) ;
#20155=ORIENTED_EDGE ( 'NONE', *, *, #76274, .F. ) ;
#20158=CARTESIAN_POINT ( 'NONE',  ( 0.06561679790026316017, 0.05413385826771626580, -0.4176697321401330321 ) ) ;
#20159=CARTESIAN_POINT ( 'NONE',  ( 1.528871391076116026, -0.6692913385826773087, -0.1292274648535924053 ) ) ;
#20160=CARTESIAN_POINT ( 'NONE',  ( 0.5774278215223104249, 0.2306618581243848609, 0.2411417322834645549 ) ) ;
#20161=CARTESIAN_POINT ( 'NONE',  ( 1.069553805774278832, 0.2952755905511810774, -0.1292274648535930714 ) ) ;
#20162=CARTESIAN_POINT ( 'NONE',  ( -0.3608923884514428360, 0.2952755905511811885, 0.1292274648535926551 ) ) ;
#20163=CARTESIAN_POINT ( 'NONE',  ( 0.02624671916010564918, 0.2306618581243848609, 0.2411417322834645549 ) ) ;
#20164=CARTESIAN_POINT ( 'NONE',  ( 1.561679790026247350, -0.4281496062992124485, 0.4176697321401328655 ) ) ;
#20165=CARTESIAN_POINT ( 'NONE',  ( 1.397637795275591177, -0.5400638737290844871, 0.3530559997133364547 ) ) ;
#20166=CARTESIAN_POINT ( 'NONE',  ( 1.128608923884515169, -0.6046776061558809534, -0.2411417322834644161 ) ) ;
#20168=CARTESIAN_POINT ( 'NONE',  ( 0.6430446194225729606, -0.3690944881889765550, -0.3153832671262227771 ) ) ;
#20169=ORIENTED_EDGE ( 'NONE', *, *, #15774, .F. ) ;
#20172=CARTESIAN_POINT ( 'NONE',  ( -0.3083989501312330295, -0.08942795157527998196, 0.3641732283464567121 ) ) ;
#20173=CARTESIAN_POINT ( 'NONE',  ( -0.03280839895013062252, 0.2952755905511810774, -0.1292274648535930714 ) ) ;
#20175=CARTESIAN_POINT ( 'NONE',  ( 0.2034120734908142214, 0.2952755905511810774, -0.1292274648535930714 ) ) ;
#20176=CARTESIAN_POINT ( 'NONE',  ( 0.1509186351706042484, -0.3162353388693405765, 0.4822834645669290543 ) ) ;
#20177=CARTESIAN_POINT ( 'NONE',  ( -0.8202099737532801971, -0.6692913385826771977, 0.1292274648535927661 ) ) ;
#20178=CARTESIAN_POINT ( 'NONE',  ( 1.450131233595801428, -0.5511811023622048555, -0.09757992244046775898 ) ) ;
#20179=CARTESIAN_POINT ( 'NONE',  ( -1.633858267716534529, 0.1660481256975885056, 0.3530559997133364547 ) ) ;
#20180=DIRECTION ( 'NONE',  ( -0.000000000000000000, 1.000000000000000000, -0.000000000000000000 ) ) ;
#20181=CARTESIAN_POINT ( 'NONE',  ( 0.8398950131233602345, 0.1283753931104746893, -0.1820866141732285504 ) ) ;
#20182=CARTESIAN_POINT ( 'NONE',  ( 0.6233595800524942554, -0.05778040916215560624, -0.4822834645669293319 ) ) ;
#20183=CARTESIAN_POINT ( 'NONE',  ( 0.7086614173228353852, -0.1870078740157479769, 0.4822834645669291653 ) ) ;
#20185=CARTESIAN_POINT ( 'NONE',  ( -1.581364829396324945, -0.3162353388693405765, 0.4822834645669290543 ) ) ;
#20188=CARTESIAN_POINT ( 'NONE',  ( -0.07874015748031421014, -0.1870078740157480879, -0.4822834645669291653 ) ) ;
#20191=CARTESIAN_POINT ( 'NONE',  ( -1.135170603674539924, 0.1771653543307087075, -0.09757992244046823083 ) ) ;
#20192=CARTESIAN_POINT ( 'NONE',  ( 1.450131233595801428, 0.2952755905511811885, 0.1292274648535926551 ) ) ;
#20193=CARTESIAN_POINT ( 'NONE',  ( 1.443569553805774897, -0.6046776061558809534, -0.2411417322834644161 ) ) ;
#20194=CARTESIAN_POINT ( 'NONE',  ( -0.09842519685039295696, -0.4536011799217367080, 0.2665933059059888421 ) ) ;
#20195=CARTESIAN_POINT ( 'NONE',  ( 0.4593175853018379162, -0.4281496062992124485, 0.4176697321401328655 ) ) ;
#20197=CARTESIAN_POINT ( 'NONE',  ( 0.2362204724409456558, -0.1870078740157479769, 0.3641732283464567677 ) ) ;
#20198=CARTESIAN_POINT ( 'NONE',  ( 5.463695987328526437E-16, -0.1870078740157479769, 0.4822834645669291653 ) ) ;
#20200=CONICAL_SURFACE ( 'NONE', #79528, 1.220472440944881942, 0.7853981633974621568 ) ;
#20201=CARTESIAN_POINT ( 'NONE',  ( -1.135170603674539924, -0.6692913385826771977, 0.1292274648535927661 ) ) ;
#20202=CARTESIAN_POINT ( 'NONE',  ( 0.4068241469816279987, -0.3690944881889765550, -0.3153832671262227771 ) ) ;
#20203=CARTESIAN_POINT ( 'NONE',  ( 0.3740157480314966754, 0.1012011053420775880, -0.2882089793578257453 ) ) ;
#20204=CARTESIAN_POINT ( 'NONE',  ( -0.8464566929133852113, -0.5400638737290845981, -0.3530559997133363437 ) ) ;
#20206=CARTESIAN_POINT ( 'NONE',  ( -0.4855643044619415427, -0.004921259842519870586, -0.3153832671262229437 ) ) ;
#20208=CARTESIAN_POINT ( 'NONE',  ( -0.6364829396325453192, -0.3162353388693405765, 0.4822834645669290543 ) ) ;
#20209=CARTESIAN_POINT ( 'NONE',  ( -0.3871391076115476282, -0.05778040916215522460, 0.4822834645669289988 ) ) ;
#20210=CARTESIAN_POINT ( 'NONE',  ( 0.3543307086614179147, 0.1771653543307087630, 0.000000000000000000 ) ) ;
#20212=CARTESIAN_POINT ( 'NONE',  ( -0.09186351706036663400, -0.4281496062992124485, 0.4176697321401328655 ) ) ;
#20215=CARTESIAN_POINT ( 'NONE',  ( -1.660104986876639543, -0.08942795157528024563, -0.3641732283464568787 ) ) ;
#20216=CARTESIAN_POINT ( 'NONE',  ( 0.6167979002624679463, -0.004921259842519870586, -0.3153832671262229437 ) ) ;
#20217=CARTESIAN_POINT ( 'NONE',  ( 1.463254593175853824, 0.2952755905511810774, -0.1292274648535930714 ) ) ;
#20218=CARTESIAN_POINT ( 'NONE',  ( -0.6627296587926503335, -0.5511811023622046335, 0.09757992244046803654 ) ) ;
#20219=CARTESIAN_POINT ( 'NONE',  ( -0.9514435695538050464, -0.2845877964562159024, 0.3641732283464567677 ) ) ;
#20220=CARTESIAN_POINT ( 'NONE',  ( -0.7283464566929126471, -0.5400638737290844871, 0.3530559997133364547 ) ) ;
#20221=CARTESIAN_POINT ( 'NONE',  ( 0.01968503937007930540, 0.1660481256975885056, 0.3530559997133364547 ) ) ;
#20222=CARTESIAN_POINT ( 'NONE',  ( 0.4724409448818904789, -0.1870078740157480601, -0.3641732283464567677 ) ) ;
#20224=CARTESIAN_POINT ( 'NONE',  ( 0.8923884514435701520, -0.5023911411419708095, -0.1820866141732282451 ) ) ;
#20225=CARTESIAN_POINT ( 'NONE',  ( 0.2099737532808405305, -0.6046776061558807314, 0.2411417322834647770 ) ) ;
#20226=EDGE_CURVE ( 'NONE', #69770, #31420, #77851, .T. ) ;
#20228=CARTESIAN_POINT ( 'NONE',  ( -0.6233595800524928121, -0.05778040916215522460, 0.4822834645669289988 ) ) ;
#20230=CARTESIAN_POINT ( 'NONE',  ( 1.404199475065617264, -0.3690944881889763329, 0.3153832671262228327 ) ) ;
#20231=CARTESIAN_POINT ( 'NONE',  ( 0.4330708661417329575, 0.2952755905511811885, 0.000000000000000000 ) ) ;
#20232=CARTESIAN_POINT ( 'NONE',  ( 0.05905511811023709395, -0.5400638737290844871, 0.3530559997133364547 ) ) ;
#20233=CARTESIAN_POINT ( 'NONE',  ( 1.604771003085129211, 1.002618919725273061, 0.1466069496707753106 ) ) ;
#20234=CARTESIAN_POINT ( 'NONE',  ( -0.06561679790026180015, -0.004921259842519576551, 0.3153832671262227771 ) ) ;
#20235=CARTESIAN_POINT ( 'NONE',  ( 0.8202099737532814183, -0.6692913385826773087, -0.1292274648535924053 ) ) ;
#20236=CARTESIAN_POINT ( 'NONE',  ( -0.2559055118110230564, 0.07958543189024071263, -0.2665933059059888421 ) ) ;
#20237=CARTESIAN_POINT ( 'NONE',  ( -0.8398950131233585692, 0.2306618581243848609, 0.2411417322834645549 ) ) ;
#20239=CARTESIAN_POINT ( 'NONE',  ( -0.2952755905511804668, 0.1660481256975885056, 0.3530559997133364547 ) ) ;
#20241=CARTESIAN_POINT ( 'NONE',  ( -1.338582677165353729, -0.1870078740157479769, 0.4822834645669291653 ) ) ;
#20242=CARTESIAN_POINT ( 'NONE',  ( -0.5774278215223089816, 0.1283753931104746893, -0.1820866141732285504 ) ) ;
#20243=CARTESIAN_POINT ( 'NONE',  ( -0.01968503937007793844, -0.5400638737290844871, 0.3530559997133364547 ) ) ;
#20244=CARTESIAN_POINT ( 'NONE',  ( -1.174540682414697335, -0.3162353388693409650, -0.4822834645669289433 ) ) ;
#20245=CARTESIAN_POINT ( 'NONE',  ( -0.8661417322834640276, -0.1870078740157479769, 0.4822834645669291653 ) ) ;
#20247=CARTESIAN_POINT ( 'NONE',  ( 0.4531182788721080934, 1.535433070866141447, -0.5309055118110237448 ) ) ;
#20248=CARTESIAN_POINT ( 'NONE',  ( 0.7677165354330716118, -0.5400638737290844871, 0.3530559997133364547 ) ) ;
#20249=CARTESIAN_POINT ( 'NONE',  ( 1.095800524934383846, -0.05778040916215560624, -0.4822834645669293319 ) ) ;
#20251=CARTESIAN_POINT ( 'NONE',  ( -1.509186351706035767, -0.4281496062992124485, 0.4176697321401328655 ) ) ;
#20252=CARTESIAN_POINT ( 'NONE',  ( -1.430446194225721390, -0.4281496062992124485, 0.4176697321401328655 ) ) ;
#20256=CARTESIAN_POINT ( 'NONE',  ( -0.01312335958005186876, -0.004921259842519870586, -0.3153832671262229437 ) ) ;
#20258=EDGE_LOOP ( 'NONE', ( #24520, #62297, #2814, #24886 ) ) ;
#20259=CARTESIAN_POINT ( 'NONE',  ( 0.09186351706036799403, -0.4281496062992127816, -0.4176697321401328100 ) ) ;
#20260=CARTESIAN_POINT ( 'NONE',  ( -0.1049868766404193215, 0.2306618581243847221, -0.2411417322834647770 ) ) ;
#20262=CARTESIAN_POINT ( 'NONE',  ( -0.9055118110236215490, -0.5511811023622047445, 6.969142054262312111E-17 ) ) ;
#20264=CARTESIAN_POINT ( 'NONE',  ( 0.8923884514435703741, 0.2306618581243848609, 0.2411417322834645549 ) ) ;
#20265=CARTESIAN_POINT ( 'NONE',  ( 0.9711286089238851948, 0.1283753931104748280, 0.1820866141732283561 ) ) ;
#20266=CARTESIAN_POINT ( 'NONE',  ( -0.4396325459317577122, -0.6692913385826773087, -0.1292274648535924053 ) ) ;
#20268=CARTESIAN_POINT ( 'NONE',  ( -0.7611548556430438595, -0.6046776061558809534, -0.2411417322834644161 ) ) ;
#20269=CARTESIAN_POINT ( 'NONE',  ( -1.620734908136482577, -0.5511811023622048555, -0.09757992244046775898 ) ) ;
#20270=CARTESIAN_POINT ( 'NONE',  ( 1.148293963254593875, -0.6692913385826771977, 0.1292274648535927661 ) ) ;
#20271=CARTESIAN_POINT ( 'NONE',  ( 1.568241469816273659, -0.08942795157528024563, -0.3641732283464568787 ) ) ;
#20274=CARTESIAN_POINT ( 'NONE',  ( 0.05249343832021075018, -0.6046776061558807314, 0.2411417322834647770 ) ) ;
#20276=CARTESIAN_POINT ( 'NONE',  ( -0.8005249343832013809, -0.4281496062992124485, 0.4176697321401328655 ) ) ;
#20277=CARTESIAN_POINT ( 'NONE',  ( 1.371391076115485719, -0.6692913385826773087, -0.1292274648535924053 ) ) ;
#20278=CARTESIAN_POINT ( 'NONE',  ( 1.397637795275591177, -0.5400638737290844871, 0.3530559997133364547 ) ) ;
#20279=( BOUNDED_CURVE ( )  B_SPLINE_CURVE ( 2, ( #75878, #77961, #20711, #65336, #45096, #19874, #520, #64480, #79220, #77539, #21124, #58151, #7240 ),
 .UNSPECIFIED., .F., .F. ) 
 B_SPLINE_CURVE_WITH_KNOTS ( ( 3, 2, 2, 2, 2, 2, 3 ),
 ( 0.4013059932978690347, 0.4015151515151514916, 0.4053030303030302761, 0.4090909090909091161, 0.4128787878787879007, 0.4166666666666666852, 0.4168758248839491420 ),
 .UNSPECIFIED. ) 
 CURVE ( )  GEOMETRIC_REPRESENTATION_ITEM ( )  RATIONAL_B_SPLINE_CURVE ( ( 0.9964447847208428577, 0.9981185001348096275, 1.000000000000000000, 0.9659258262890683122, 1.000000000000000000, 0.9659258262890683122, 1.000000000000000000, 0.9659258262890683122, 1.000000000000000000, 0.9659258262890683122, 1.000000000000000000, 0.9981185001348097385, 0.9964447847208430797 ) ) 
 REPRESENTATION_ITEM ( '' )  );
#20280=CARTESIAN_POINT ( 'NONE',  ( 0.2362204724409456558, -0.1870078740157480879, -0.4822834645669291653 ) ) ;
#20281=CARTESIAN_POINT ( 'NONE',  ( -0.1771653543307080136, 0.1660481256975883668, -0.3530559997133364547 ) ) ;
#20283=CARTESIAN_POINT ( 'NONE',  ( -1.089238845144356427, 0.05413385826771666132, 0.4176697321401328100 ) ) ;
#20284=CARTESIAN_POINT ( 'NONE',  ( -0.1312335958005241554, -0.6046776061558809534, -0.2411417322834644161 ) ) ;
#20285=CARTESIAN_POINT ( 'NONE',  ( -0.3083989501312330295, -0.2845877964562161244, -0.3641732283464567121 ) ) ;
#20288=CARTESIAN_POINT ( 'NONE',  ( 1.305774278215223960, -0.6692913385826771977, 0.1292274648535927661 ) ) ;
#20289=CARTESIAN_POINT ( 'NONE',  ( -0.5118110236220466680, -0.6692913385826771977, 8.415575281601705876E-17 ) ) ;
#20292=CARTESIAN_POINT ( 'NONE',  ( 1.272965879265092637, 0.05413385826771666132, 0.4176697321401328100 ) ) ;
#20294=ORIENTED_EDGE ( 'NONE', *, *, #60874, .T. ) ;
#20295=CARTESIAN_POINT ( 'NONE',  ( 0.1902887139107617975, -0.6692913385826773087, -0.1292274648535924053 ) ) ;
#20296=CARTESIAN_POINT ( 'NONE',  ( -0.2690288713910754526, 0.1771653543307087075, -0.09757992244046823083 ) ) ;
#20297=CARTESIAN_POINT ( 'NONE',  ( 0.9580052493438327987, -0.3690944881889765550, -0.3153832671262227771 ) ) ;
#20298=DIRECTION ( 'NONE',  ( 1.000000000000000000, -0.000000000000000000, -0.000000000000000000 ) ) ;
#20300=CARTESIAN_POINT ( 'NONE',  ( 1.653543307086614789, -0.1870078740157479769, 0.3641732283464567677 ) ) ;
#20301=CARTESIAN_POINT ( 'NONE',  ( 1.430446194225722500, 0.05413385826771666132, 0.4176697321401328100 ) ) ;
#20303=CARTESIAN_POINT ( 'NONE',  ( 0.1509186351706042484, -0.3162353388693405765, 0.4822834645669290543 ) ) ;
#20304=CARTESIAN_POINT ( 'NONE',  ( -1.607611548556429737, 0.2952755905511810774, -0.1292274648535930714 ) ) ;
#20305=CARTESIAN_POINT ( 'NONE',  ( 1.581364829396326277, -0.08942795157527998196, 0.3641732283464567121 ) ) ;
#20306=CARTESIAN_POINT ( 'NONE',  ( -0.07217847769028813698, -0.3162353388693409650, -0.4822834645669289433 ) ) ;
#20308=CARTESIAN_POINT ( 'NONE',  ( -1.601049868766403650, 0.1283753931104746893, -0.1820866141732285504 ) ) ;
#20309=CARTESIAN_POINT ( 'NONE',  ( 0.5905511811023629321, -0.6692913385826771977, 8.415575281601705876E-17 ) ) ;
#20310=CARTESIAN_POINT ( 'NONE',  ( 1.076115485564305141, 0.1283753931104746893, -0.1820866141732285504 ) ) ;
#20311=CARTESIAN_POINT ( 'NONE',  ( -0.01312335958005186876, 0.05413385826771626580, -0.4176697321401330321 ) ) ;
#20312=CARTESIAN_POINT ( 'NONE',  ( 0.7808398950131241190, -0.08942795157528024563, -0.3641732283464568787 ) ) ;
#20313=CARTESIAN_POINT ( 'NONE',  ( -1.364829396325458521, -0.6046776061558807314, 0.2411417322834647770 ) ) ;
#20315=CARTESIAN_POINT ( 'NONE',  ( 1.043307086614173818, 0.1660481256975885056, 0.3530559997133364547 ) ) ;
#20317=CARTESIAN_POINT ( 'NONE',  ( 0.8989501312335964611, 0.2952755905511811885, 0.1292274648535926551 ) ) ;
#20318=CARTESIAN_POINT ( 'NONE',  ( 0.9251968503937014754, 0.1660481256975883391, -0.3530559997133364547 ) ) ;
#20319=CARTESIAN_POINT ( 'NONE',  ( -0.3477690288713902178, 0.2066929133858267098, -0.1054918080437494132 ) ) ;
#20320=CARTESIAN_POINT ( 'NONE',  ( 0.4658792650918640033, -0.2845877964562159024, 0.3641732283464567677 ) ) ;
#20321=CARTESIAN_POINT ( 'NONE',  ( 0.6430446194225729606, -0.4281496062992127816, -0.4176697321401328100 ) ) ;
#20323=CARTESIAN_POINT ( 'NONE',  ( -0.8923884514435688198, 0.1283753931104746893, -0.1820866141732285504 ) ) ;
#20324=CARTESIAN_POINT ( 'NONE',  ( -1.167979002624671470, -0.4281496062992127816, -0.4176697321401328100 ) ) ;
#20325=CARTESIAN_POINT ( 'NONE',  ( -1.561679790026246017, 0.05413385826771666132, 0.4176697321401328100 ) ) ;
#20326=VECTOR ( 'NONE', #13001, 39.37007874015748143 ) ;
#20327=CARTESIAN_POINT ( 'NONE',  ( 1.148293963254593875, -0.6692913385826771977, 0.1292274648535927661 ) ) ;
#20328=CARTESIAN_POINT ( 'NONE',  ( -1.646981627296586703, -0.08942795157527998196, 0.3641732283464567121 ) ) ;
#20330=CARTESIAN_POINT ( 'NONE',  ( 0.8202099737532813073, 0.2952755905511811885, 0.1292274648535926551 ) ) ;
#20332=CARTESIAN_POINT ( 'NONE',  ( 1.692913385826772421, 0.2952755905511811885, 0.000000000000000000 ) ) ;
#20333=CARTESIAN_POINT ( 'NONE',  ( 1.417322834645670104, -0.1870078740157480879, -0.4822834645669291653 ) ) ;
#20334=CARTESIAN_POINT ( 'NONE',  ( -1.312335958005248715, -0.5023911411419708095, -0.1820866141732282451 ) ) ;
#20335=CARTESIAN_POINT ( 'NONE',  ( 1.207349081364829990, 0.1283753931104748280, 0.1820866141732283561 ) ) ;
#20336=CARTESIAN_POINT ( 'NONE',  ( -1.194225721784776262, -0.3690944881889763329, 0.3153832671262228327 ) ) ;
#20337=CARTESIAN_POINT ( 'NONE',  ( -0.3412073490813641308, 0.1283753931104746893, -0.1820866141732285504 ) ) ;
#20339=CARTESIAN_POINT ( 'NONE',  ( 1.108923884514436242, -0.08942795157527998196, 0.3641732283464567121 ) ) ;
#20340=CARTESIAN_POINT ( 'NONE',  ( 0.7152230971128616943, -0.05778040916215522460, 0.4822834645669289988 ) ) ;
#20341=CARTESIAN_POINT ( 'NONE',  ( 1.154855643044620184, 0.2306618581243847221, -0.2411417322834647770 ) ) ;
#20342=CARTESIAN_POINT ( 'NONE',  ( -0.1181102362204717315, -0.6692913385826771977, 8.415575281601705876E-17 ) ) ;
#20344=CARTESIAN_POINT ( 'NONE',  ( 0.6430446194225728496, -0.004921259842519576551, 0.3153832671262227771 ) ) ;
#20345=CARTESIAN_POINT ( 'NONE',  ( 1.240157480314961314, -0.5400638737290844871, 0.3530559997133364547 ) ) ;
#20346=CARTESIAN_POINT ( 'NONE',  ( -1.640419947506561060, 0.05413385826771666132, 0.4176697321401328100 ) ) ;
#20347=CARTESIAN_POINT ( 'NONE',  ( -0.5052493438320203589, -0.6692913385826771977, 0.1292274648535927661 ) ) ;
#20350=CARTESIAN_POINT ( 'NONE',  ( 0.02624671916010564918, 0.2306618581243848609, 0.2411417322834645549 ) ) ;
#20351=CARTESIAN_POINT ( 'NONE',  ( -0.4461942257217840213, -0.6046776061558809534, -0.2411417322834644161 ) ) ;
#20352=CARTESIAN_POINT ( 'NONE',  ( 0.1115485564304467270, -0.6692913385826773087, -0.1292274648535924053 ) ) ;
#20360=CARTESIAN_POINT ( 'NONE',  ( -0.7611548556430438595, 0.1283753931104748280, 0.1820866141732283561 ) ) ;
#20362=CARTESIAN_POINT ( 'NONE',  ( -1.345144356955379816, -0.05778040916215560624, -0.4822834645669293319 ) ) ;
#20364=CARTESIAN_POINT ( 'NONE',  ( 0.4527559055118117182, 0.1660481256975883668, -0.3530559997133364547 ) ) ;
#20365=CARTESIAN_POINT ( 'NONE',  ( -0.5905511811023615998, 0.1771653543307087630, 0.000000000000000000 ) ) ;
#20366=CARTESIAN_POINT ( 'NONE',  ( 1.102362204724410155, -0.1870078740157479769, 0.4822834645669291653 ) ) ;
#20367=CARTESIAN_POINT ( 'NONE',  ( 0.3608923884514443348, 0.2952755905511810774, -0.1292274648535930714 ) ) ;
#20371=CARTESIAN_POINT ( 'NONE',  ( 1.266404199475066328, -0.3162353388693409650, -0.4822834645669289433 ) ) ;
#20372=CARTESIAN_POINT ( 'NONE',  ( 0.2887139107611556010, -0.6046776061558807314, 0.2411417322834647770 ) ) ;
#20373=CARTESIAN_POINT ( 'NONE',  ( 0.05905511811023681640, 0.1660481256975883668, -0.3530559997133364547 ) ) ;
#20374=CARTESIAN_POINT ( 'NONE',  ( -1.646981627296586703, -0.05778040916215522460, 0.4822834645669289988 ) ) ;
#20375=CARTESIAN_POINT ( 'NONE',  ( 0.7677165354330716118, 0.1660481256975883668, -0.3530559997133364547 ) ) ;
#20377=CARTESIAN_POINT ( 'NONE',  ( -0.01968503937007793844, -0.5400638737290844871, 0.3530559997133364547 ) ) ;
#20378=CARTESIAN_POINT ( 'NONE',  ( 1.089238845144357759, 0.05413385826771626580, -0.4176697321401330321 ) ) ;
#20379=CARTESIAN_POINT ( 'NONE',  ( 0.5249343832021005074, -0.6046776061558807314, 0.2411417322834647770 ) ) ;
#20380=CARTESIAN_POINT ( 'NONE',  ( 0.9711286089238851948, -0.5023911411419708095, -0.1820866141732282451 ) ) ;
#20381=CARTESIAN_POINT ( 'NONE',  ( -0.9317585301837263412, 0.05413385826771666132, 0.4176697321401328100 ) ) ;
#20382=CARTESIAN_POINT ( 'NONE',  ( -1.437007874015747477, -0.5400638737290844871, 0.3530559997133364547 ) ) ;
#20384=CARTESIAN_POINT ( 'NONE',  ( 0.7808398950131240079, -0.3162353388693405765, 0.4822834645669290543 ) ) ;
#20389=ORIENTED_EDGE ( 'NONE', *, *, #53708, .T. ) ;
#20390=CARTESIAN_POINT ( 'NONE',  ( 1.568241469816273659, -0.05778040916215560624, -0.4822834645669293319 ) ) ;
#20391=CARTESIAN_POINT ( 'NONE',  ( 0.8858267716535438430, -0.4536011799217368745, -0.2665933059059886201 ) ) ;
#20397=CARTESIAN_POINT ( 'NONE',  ( -1.036745406824146176, -0.3690944881889763329, 0.3153832671262228327 ) ) ;
#20398=CARTESIAN_POINT ( 'NONE',  ( 1.568241469816273437, -0.3162353388693405765, 0.4822834645669290543 ) ) ;
#20399=CARTESIAN_POINT ( 'NONE',  ( -1.541994750656167090, -0.6692913385826773087, -0.1292274648535924053 ) ) ;
#20400=CARTESIAN_POINT ( 'NONE',  ( -0.3083989501312330295, -0.05778040916215522460, 0.4822834645669289988 ) ) ;
#20401=CARTESIAN_POINT ( 'NONE',  ( 1.122047244094488860, 0.1660481256975885056, 0.3530559997133364547 ) ) ;
#20402=VERTEX_POINT ( 'NONE', #58896 ) ;
#20403=CARTESIAN_POINT ( 'NONE',  ( -1.410761154855642463, -0.05778040916215522460, 0.4822834645669289988 ) ) ;
#20404=CARTESIAN_POINT ( 'NONE',  ( 0.4849061582275022153, 1.568468489416427580, 0.4921425059946342717 ) ) ;
#20407=CARTESIAN_POINT ( 'NONE',  ( 1.603475055217291612, 1.267857067133554061, -0.04573490813648243419 ) ) ;
#20408=CARTESIAN_POINT ( 'NONE',  ( -0.7414698162729651543, -0.5511811023622046335, 0.09757992244046803654 ) ) ;
#20409=( BOUNDED_SURFACE ( )  B_SPLINE_SURFACE ( 1, 2, ( 
 ( #74889, #36559, #10901, #62236, #31479, #76529, #71457, #19263, #26833, #13384, #1182, #39463, #57140, #52491, #39037, #63881, #83248, #38207, #78200, #33156, #50827, #25571, #757, #13805, #77354, #32730, #6220, #64721, #31896, #25159, #12549, #26418, #12968, #58397, #19686, #18857, #38625, #63474, #52071, #82837, #20530, #5809, #14228, #58825, #57971, #77778, #44505, #46182, #337, #71879, #70194, #57557, #51236, #7061, #76935, #44916, #70613, #64303, #20111, #45759, #65150, #6637, #32309, #71040, #25992, #51650, #45344, #7486, #41542, #15053, #60070, #52907, #33570, #2425, #22187, #59647, #46602, #34826, #35231, #79870, #73121, #21766, #53331, #14644, #34402, #79040, #15472, #47429, #53739, #2003, #40709, #27248, #54573, #21359, #60483, #47012, #65575, #41129, #66820, #28081, #33985, #7909, #2834, #54155, #47844, #60895, #72706, #9561, #3246, #80287, #67231, #28495, #9153, #27665, #1593, #78621, #66394, #8732, #48261, #28910, #73957, #73550, #79447, #20944, #15893, #22600, #39888, #59232, #72298, #40300, #65981, #8319, #3663, #82333, #75609, #69286, #74371, #74785, #5306, #80695, #9975, #24651, #4476, #17540, #37293, #30146, #81102, #4890, #55807, #50319, #30965, #29326, #81928, #62136, #62555, #43172, #23008, #42355, #61729, #30565, #48675, #49503, #56230, #11633, #24239, #16715, #4066, #11217, #49912, #62968, #41946, #17948, #16304, #68053, #54987, #42768, #49085, #17136, #43585, #56632, #81514, #23835, #67642, #75196, #10400, #68464, #35645, #68868, #36877, #36462, #61305, #36057, #29733, #55395, #23419, #10802, #63370, #234, #57041, #58287, #39354, #45656, #26730, #70092, #6539, #57868, #1077, #76428, #652, #13284, #12446, #5704, #82735, #58712, #25054, #32209, #25886, #44400, #51546, #13698, #70507, #33043, #38105, #12865, #31792, #51134, #38522, #38936, #31376, #71352, #64205, #65038, #76016, #69695, #12038, #77250, #50729, #18358, #44002, #37695, #19579, #64617, #51967, #18756, #63781, #45239, #6120, #57455, #76829, #7375, #77675, #19161, #70939, #83148, #25468, #6954, #26309, #44811, #32624, #20005, #47740, #9046, #2318, #34301, #65880, #27142, #46908, #8216, #27978, #59962, #66291, #14545, #27562, #39776, #67124, #33880, #47324, #59546, #78093, #53637, #3144, #2730, #8630, #1901, #46077, #53221, #66713, #78931, #35127, #54050, #52806, #9454, #79344, #73015, #78516, #20424, #59131, #40197, #34721, #60381, #15788, #14123, #21254, #72603, #33469, #28391, #15366, #1489, #60791, #79764, #7804, #14950, #20840, #22081, #71770, #65470, #73438, #40608, #41440, #21665, #52384, #46492, #72188, #41027, #4376, #29224, #48572, #3559, #17850, #81830, #16198, #74269, #49402, #62448, #42671, #81415, #54891, #30044, #80596, #73857, #61202, #75096, #61629, #23731, #68370, #41845, #3971, #28807, #17444, #80184, #75511, #54471, #62868, #24140, #11531, #9872, #10708, #62039, #22904, #55706, #49810, #23318, #69180, #16613, #48988, #67950, #29634, #43074, #74686, #42255, #22499, #68771, #11115, #36772, #43484, #10293, #37188, #48162, #67535, #30461, #4784, #36364, #35960, #35541, #55295, #81004, #17032, #56124, #51873, #39257, #38424, #57353, #69595, #83049, #19911, #76331, #57771, #12767, #70842, #63269, #25372, #75917, #71257, #64519, #58190, #5610, #63685, #77579, #11942, #82236, #13603, #76735, #6441, #26211, #19066, #69996, #77153, #44714, #5204, #45561, #18256, #13191, #51035, #51450, #32113, #37596, #31278, #50626, #19485, #56943, #64106, #45138, #558, #38840, #82640, #18661, #133, #6856, #30868, #56533, #32526, #24555, #24953, #43898, #31694, #38007, #6023, #50221, #44306, #70411, #25789, #12351, #46817, #65374, #65789, #35753, #78835, #34203, #1804, #23117, #64939, #29433, #55091, #48785, #78420, #52292, #72508, #45978, #48367, #80800, #61419, #16829, #59040, #21161, #14857, #74482, #7709, #74066, #2219, #1394, #77997, #71674, #27885, #27048, #20325, #14025, #7279, #39682, #40518, #66198, #33376, #8536, #3769, #59451, #32949, #52708, #27466, #20748, #40101, #59866, #53124, #46398, #58615, #53545, #79253, #21568, #982, #72091, #26638, #14450, #8122 ),
 ( #33787, #16412, #42059, #67754, #10088, #24757, #17245, #62665, #29839, #25169, #18467, #12149, #42874, #17647, #31488, #23526, #36161, #50838, #30675, #43690, #63484, #56336, #23941, #31074, #82035, #76538, #57149, #55503, #50425, #5005, #5412, #69395, #49196, #68567, #4582, #56742, #74897, #75717, #82440, #37806, #76125, #10909, #30253, #37403, #44110, #5818, #68165, #69802, #42465, #36567, #81211, #68978, #75303, #43279, #82848, #10508, #24349, #50018, #61835, #18057, #62245, #11326, #4175, #11747, #63075, #55917, #81630, #49608, #36986, #7919, #59243, #32320, #6230, #26429, #83259, #1193, #65586, #71889, #52918, #12979, #32741, #767, #27258, #19274, #26842, #33580, #1602, #20542, #13816, #52080, #38635, #63892, #31906, #26004, #57982, #18866, #44515, #70202, #77789, #71051, #25581, #13395, #12559, #6647, #71468, #20122, #52501, #76947, #39048, #57567, #38217, #78210, #14240, #44926, #77365, #51245, #70623, #64313, #347, #7071, #45769, #39898, #58408, #51661, #7498, #39475, #19697, #45354, #64733, #46194, #65162, #33167, #58835, #2014, #21370, #40720, #41552, #59658, #28508, #67240, #48270, #3257, #27678, #66406, #73559, #60905, #73968, #20956, #28918, #78632, #47025, #8330, #21777, #28094, #53750, #80296, #16313, #34835, #60495, #9571, #2844, #79053, #79460, #41958, #9163, #47854, #15483, #35654, #46614, #67651, #9988, #61317, #8743, #65992, #54165, #53343, #54586, #3672, #29335, #72309, #72717, #79880, #22197, #14656, #15064, #22610, #15903, #34414, #33996, #60082, #40313, #2436, #35241, #47439, #73133, #41140, #66830, #49512, #12048, #17145, #75205, #10811, #30155, #56240, #17549, #49094, #80704, #49921, #69296, #11645, #76026, #36471, #24660, #37303, #62977, #18371, #62146, #50329, #44011, #37706, #56641, #75619, #36888, #74798, #16725, #42366, #4487, #68473, #63379, #69705, #5715, #4903, #23845, #36066, #43181, #54996, #42777, #24248, #62564, #5316, #29742, #68878, #68065, #23018, #30974, #48685, #55406, #55817, #74382, #61738, #10409, #4075, #11227, #81937, #81112, #30574, #81525, #43594, #17957, #23430, #82342, #44409, #13710, #77260, #77685, #58298, #38116, #57464, #76838, #20015, #12455, #64628, #45666, #1088, #39364, #63791, #19172, #26319, #65049, #26740, #57051, #7387, #31385, #83158, #70103, #57877, #64214, #6548, #33054, #52394, #70948, #13293, #71362, #38945, #31804, #32219, #78103, #45251, #664, #51556, #71780, #82744, #20434, #46088, #14135, #44820, #18766, #6964, #6129, #58725, #39787, #65482, #25065, #25477, #32635, #51980, #50739, #51144, #76437, #70518, #12874, #38533, #244, #25896, #19589, #21675, #41038, #59556, #66723, #28818, #2332, #48173, #53231, #27988, #46920, #66301, #9060, #53648, #1911, #33480, #2743, #34732, #14556, #7814, #41856, #52816, #60392, #28403, #67136, #72203, #27574, #15376, #40208, #46503, #8640, #22512, #9465, #34312, #79356, #20851, #1500, #47336, #73451, #78947, #65891, #54061, #3155, #47753, #79776, #73026, #21265, #8226, #22092, #72613, #15801, #41452, #35139, #14961, #59973, #78527, #73869, #40618, #60801, #54483, #59142, #80194, #27152, #16209, #33890, #74699, #61215, #17044, #81843, #10721, #50234, #69196, #67964, #82249, #49417, #62462, #10306, #9883, #74281, #29647, #49824, #75524, #30881, #29237, #55309, #42684, #48584, #17863, #4797, #16625, #75930, #43498, #22917, #68382, #42267, #11545, #35552, #80607, #37201, #23330, #56548, #17457, #5217, #62882, #3570, #24567, #43087, #35972, #3983, #61642, #18271, #67548, #54901, #81017, #30474, #49000, #81429, #36786, #36378, #68784, #62052, #4390, #30058, #56138, #55719, #24154, #23744, #75111, #11128, #43911, #64532, #11955, #7291, #69609, #78010, #39269, #38437, #6869, #82653, #13615, #64120, #64951, #37610, #63285, #5625, #77165, #32538, #19925, #24968, #38022, #51463, #50640, #76344, #44727, #58628, #45575, #19079, #6455, #56956, #31291, #32125, #26223, #63698, #18674, #38852, #32961, #570, #19497, #25802, #57369, #44319, #57783, #83064, #45151, #70854, #147, #6037, #70424, #70009, #996, #25385, #58202, #51048, #12364, #13205, #31709, #77591 ) ),
 .UNSPECIFIED., .F., .F., .F. ) 
 B_SPLINE_SURFACE_WITH_KNOTS ( ( 2, 2 ),
 ( 3, 2, 2, 2, 2, 2, 2, 2, 2, 2, 2, 2, 2, 2, 2, 2, 2, 2, 2, 2, 2, 2, 2, 2, 2, 2, 2, 2, 2, 2, 2, 2, 2, 2, 2, 2, 2, 2, 2, 2, 2, 2, 2, 2, 2, 2, 2, 2, 2, 2, 2, 2, 2, 2, 2, 2, 2, 2, 2, 2, 2, 2, 2, 2, 2, 2, 2, 2, 2, 2, 2, 2, 2, 2, 2, 2, 2, 2, 2, 2, 2, 2, 2, 2, 2, 2, 2, 2, 2, 2, 2, 2, 2, 2, 2, 2, 2, 2, 2, 2, 2, 2, 2, 2, 2, 2, 2, 2, 2, 2, 2, 2, 2, 2, 2, 2, 2, 2, 2, 2, 2, 2, 2, 2, 2, 2, 2, 2, 2, 2, 2, 2, 2, 2, 2, 2, 2, 2, 2, 2, 2, 2, 2, 2, 2, 2, 2, 2, 2, 2, 2, 2, 2, 2, 2, 2, 2, 2, 2, 2, 2, 2, 2, 2, 2, 2, 2, 2, 2, 2, 2, 2, 2, 2, 2, 2, 2, 2, 2, 2, 2, 2, 2, 2, 2, 2, 2, 2, 2, 2, 2, 2, 2, 2, 2, 2, 2, 2, 2, 2, 2, 2, 2, 2, 2, 2, 2, 2, 2, 2, 2, 2, 2, 2, 2, 2, 2, 2, 2, 2, 2, 2, 2, 2, 2, 2, 2, 2, 2, 2, 2, 2, 2, 2, 2, 2, 2, 2, 2, 2, 2, 2, 2, 2, 2, 2, 2, 2, 2, 2, 2, 2, 2, 2, 2, 3 ),
 ( 0.000000000000000000, 1.000000000000000000 ),
 ( 0.000000000000000000, 0.003787878787878787984, 0.007575757575757575968, 0.01136363636363636395, 0.01515151515151515194, 0.01893939393939393992, 0.02272727272727272790, 0.02651515151515151589, 0.03030303030303030387, 0.03409090909090908839, 0.03787878787878787984, 0.04166666666666666435, 0.04545454545454545581, 0.04924242424242424032, 0.05303030303030303177, 0.05681818181818181629, 0.06060606060606060774, 0.06439393939393939226, 0.06818181818181817677, 0.07196969696969697516, 0.07575757575757575968, 0.07954545454545454419, 0.08333333333333332871, 0.08712121212121212710, 0.09090909090909091161, 0.09469696969696969613, 0.09848484848484848064, 0.1022727272727272790, 0.1060606060606060635, 0.1098484848484848481, 0.1136363636363636326, 0.1174242424242424310, 0.1212121212121212155, 0.1250000000000000000, 0.1287878787878787845, 0.1325757575757575690, 0.1363636363636363535, 0.1401515151515151381, 0.1439393939393939503, 0.1477272727272727348, 0.1515151515151515194, 0.1553030303030303039, 0.1590909090909090884, 0.1628787878787878729, 0.1666666666666666574, 0.1704545454545454419, 0.1742424242424242542, 0.1780303030303030387, 0.1818181818181818232, 0.1856060606060606077, 0.1893939393939393923, 0.1931818181818181768, 0.1969696969696969613, 0.2007575757575757458, 0.2045454545454545581, 0.2083333333333333426, 0.2121212121212121271, 0.2159090909090909116, 0.2196969696969696961, 0.2234848484848484806, 0.2272727272727272652, 0.2310606060606060497, 0.2348484848484848619, 0.2386363636363636465, 0.2424242424242424310, 0.2462121212121212155, 0.2500000000000000000, 0.2537878787878787845, 0.2575757575757575690, 0.2613636363636363535, 0.2651515151515151381, 0.2689393939393939226, 0.2727272727272727071, 0.2765151515151514916, 0.2803030303030302761, 0.2840909090909091161, 0.2878787878787879007, 0.2916666666666666852, 0.2954545454545454697, 0.2992424242424242542, 0.3030303030303030387, 0.3068181818181818232, 0.3106060606060606077, 0.3143939393939393923, 0.3181818181818181768, 0.3219696969696969613, 0.3257575757575757458, 0.3295454545454545303, 0.3333333333333333148, 0.3371212121212120993, 0.3409090909090908839, 0.3446969696969697239, 0.3484848484848485084, 0.3522727272727272929, 0.3560606060606060774, 0.3598484848484848619, 0.3636363636363636465, 0.3674242424242424310, 0.3712121212121212155, 0.3750000000000000000, 0.3787878787878787845, 0.3825757575757575690, 0.3863636363636363535, 0.3901515151515151381, 0.3939393939393939226, 0.3977272727272727071, 0.4015151515151514916, 0.4053030303030302761, 0.4090909090909091161, 0.4128787878787879007, 0.4166666666666666852, 0.4204545454545454697, 0.4242424242424242542, 0.4280303030303030387, 0.4318181818181818232, 0.4356060606060606077, 0.4393939393939393923, 0.4431818181818181768, 0.4469696969696969613, 0.4507575757575757458, 0.4545454545454545303, 0.4583333333333333148, 0.4621212121212120993, 0.4659090909090908839, 0.4696969696969697239, 0.4734848484848485084, 0.4772727272727272929, 0.4810606060606060774, 0.4848484848484848619, 0.4886363636363636465, 0.4924242424242424310, 0.4962121212121212155, 0.5000000000000000000, 0.5037878787878787845, 0.5075757575757575690, 0.5113636363636363535, 0.5151515151515151381, 0.5189393939393939226, 0.5227272727272727071, 0.5265151515151514916, 0.5303030303030302761, 0.5340909090909090606, 0.5378787878787878451, 0.5416666666666666297, 0.5454545454545454142, 0.5492424242424241987, 0.5530303030303029832, 0.5568181818181817677, 0.5606060606060605522, 0.5643939393939394478, 0.5681818181818182323, 0.5719696969696970168, 0.5757575757575758013, 0.5795454545454545858, 0.5833333333333333703, 0.5871212121212121549, 0.5909090909090909394, 0.5946969696969697239, 0.5984848484848485084, 0.6022727272727272929, 0.6060606060606060774, 0.6098484848484848619, 0.6136363636363636465, 0.6174242424242424310, 0.6212121212121212155, 0.6250000000000000000, 0.6287878787878787845, 0.6325757575757575690, 0.6363636363636363535, 0.6401515151515151381, 0.6439393939393939226, 0.6477272727272727071, 0.6515151515151514916, 0.6553030303030302761, 0.6590909090909090606, 0.6628787878787878451, 0.6666666666666666297, 0.6704545454545454142, 0.6742424242424241987, 0.6780303030303029832, 0.6818181818181817677, 0.6856060606060605522, 0.6893939393939394478, 0.6931818181818182323, 0.6969696969696970168, 0.7007575757575758013, 0.7045454545454545858, 0.7083333333333333703, 0.7121212121212121549, 0.7159090909090909394, 0.7196969696969697239, 0.7234848484848485084, 0.7272727272727272929, 0.7310606060606060774, 0.7348484848484848619, 0.7386363636363636465, 0.7424242424242424310, 0.7462121212121212155, 0.7500000000000000000, 0.7537878787878787845, 0.7575757575757575690, 0.7613636363636363535, 0.7651515151515151381, 0.7689393939393939226, 0.7727272727272727071, 0.7765151515151514916, 0.7803030303030302761, 0.7840909090909090606, 0.7878787878787878451, 0.7916666666666666297, 0.7954545454545454142, 0.7992424242424241987, 0.8030303030303029832, 0.8068181818181817677, 0.8106060606060605522, 0.8143939393939394478, 0.8181818181818182323, 0.8219696969696970168, 0.8257575757575758013, 0.8295454545454545858, 0.8333333333333333703, 0.8371212121212121549, 0.8409090909090909394, 0.8446969696969697239, 0.8484848484848485084, 0.8522727272727272929, 0.8560606060606060774, 0.8598484848484848619, 0.8636363636363636465, 0.8674242424242424310, 0.8712121212121212155, 0.8750000000000000000, 0.8787878787878787845, 0.8825757575757575690, 0.8863636363636363535, 0.8901515151515151381, 0.8939393939393939226, 0.8977272727272727071, 0.9015151515151514916, 0.9053030303030302761, 0.9090909090909090606, 0.9128787878787878451, 0.9166666666666666297, 0.9204545454545454142, 0.9242424242424241987, 0.9280303030303029832, 0.9318181818181817677, 0.9356060606060605522, 0.9393939393939394478, 0.9431818181818182323, 0.9469696969696970168, 0.9507575757575758013, 0.9545454545454545858, 0.9583333333333333703, 0.9621212121212121549, 0.9659090909090909394 ),
 .UNSPECIFIED. ) 
 GEOMETRIC_REPRESENTATION_ITEM ( )  RATIONAL_B_SPLINE_SURFACE ( (
 ( 1.000000000000000000, 0.9659258262890683122, 1.000000000000000000, 0.9659258262890683122, 1.000000000000000000, 0.9659258262890683122, 1.000000000000000000, 0.9659258262890683122, 1.000000000000000000, 0.9659258262890683122, 1.000000000000000000, 0.9659258262890683122, 1.000000000000000000, 0.9659258262890683122, 1.000000000000000000, 0.9659258262890683122, 1.000000000000000000, 0.9659258262890683122, 1.000000000000000000, 0.9659258262890683122, 1.000000000000000000, 0.9659258262890683122, 1.000000000000000000, 0.9659258262890683122, 1.000000000000000000, 0.9659258262890683122, 1.000000000000000000, 0.9659258262890683122, 1.000000000000000000, 0.9659258262890683122, 1.000000000000000000, 0.9659258262890683122, 1.000000000000000000, 0.9659258262890683122, 1.000000000000000000, 0.9659258262890683122, 1.000000000000000000, 0.9659258262890683122, 1.000000000000000000, 0.9659258262890683122, 1.000000000000000000, 0.9659258262890683122, 1.000000000000000000, 0.9659258262890683122, 1.000000000000000000, 0.9659258262890683122, 1.000000000000000000, 0.9659258262890683122, 1.000000000000000000, 0.9659258262890683122, 1.000000000000000000, 0.9659258262890683122, 1.000000000000000000, 0.9659258262890683122, 1.000000000000000000, 0.9659258262890683122, 1.000000000000000000, 0.9659258262890683122, 1.000000000000000000, 0.9659258262890683122, 1.000000000000000000, 0.9659258262890683122, 1.000000000000000000, 0.9659258262890683122, 1.000000000000000000, 0.9659258262890683122, 1.000000000000000000, 0.9659258262890683122, 1.000000000000000000, 0.9659258262890683122, 1.000000000000000000, 0.9659258262890683122, 1.000000000000000000, 0.9659258262890683122, 1.000000000000000000, 0.9659258262890683122, 1.000000000000000000, 0.9659258262890683122, 1.000000000000000000, 0.9659258262890683122, 1.000000000000000000, 0.9659258262890683122, 1.000000000000000000, 0.9659258262890683122, 1.000000000000000000, 0.9659258262890683122, 1.000000000000000000, 0.9659258262890683122, 1.000000000000000000, 0.9659258262890683122, 1.000000000000000000, 0.9659258262890683122, 1.000000000000000000, 0.9659258262890683122, 1.000000000000000000, 0.9659258262890683122, 1.000000000000000000, 0.9659258262890683122, 1.000000000000000000, 0.9659258262890683122, 1.000000000000000000, 0.9659258262890683122, 1.000000000000000000, 0.9659258262890683122, 1.000000000000000000, 0.9659258262890683122, 1.000000000000000000, 0.9659258262890683122, 1.000000000000000000, 0.9659258262890683122, 1.000000000000000000, 0.9659258262890683122, 1.000000000000000000, 0.9659258262890683122, 1.000000000000000000, 0.9659258262890683122, 1.000000000000000000, 0.9659258262890683122, 1.000000000000000000, 0.9659258262890683122, 1.000000000000000000, 0.9659258262890683122, 1.000000000000000000, 0.9659258262890683122, 1.000000000000000000, 0.9659258262890683122, 1.000000000000000000, 0.9659258262890683122, 1.000000000000000000, 0.9659258262890683122, 1.000000000000000000, 0.9659258262890683122, 1.000000000000000000, 0.9659258262890683122, 1.000000000000000000, 0.9659258262890683122, 1.000000000000000000, 0.9659258262890683122, 1.000000000000000000, 0.9659258262890683122, 1.000000000000000000, 0.9659258262890683122, 1.000000000000000000, 0.9659258262890683122, 1.000000000000000000, 0.9659258262890683122, 1.000000000000000000, 0.9659258262890683122, 1.000000000000000000, 0.9659258262890683122, 1.000000000000000000, 0.9659258262890683122, 1.000000000000000000, 0.9659258262890683122, 1.000000000000000000, 0.9659258262890683122, 1.000000000000000000, 0.9659258262890683122, 1.000000000000000000, 0.9659258262890683122, 1.000000000000000000, 0.9659258262890683122, 1.000000000000000000, 0.9659258262890683122, 1.000000000000000000, 0.9659258262890683122, 1.000000000000000000, 0.9659258262890683122, 1.000000000000000000, 0.9659258262890683122, 1.000000000000000000, 0.9659258262890683122, 1.000000000000000000, 0.9659258262890683122, 1.000000000000000000, 0.9659258262890683122, 1.000000000000000000, 0.9659258262890683122, 1.000000000000000000, 0.9659258262890683122, 1.000000000000000000, 0.9659258262890683122, 1.000000000000000000, 0.9659258262890683122, 1.000000000000000000, 0.9659258262890683122, 1.000000000000000000, 0.9659258262890683122, 1.000000000000000000, 0.9659258262890683122, 1.000000000000000000, 0.9659258262890683122, 1.000000000000000000, 0.9659258262890683122, 1.000000000000000000, 0.9659258262890683122, 1.000000000000000000, 0.9659258262890683122, 1.000000000000000000, 0.9659258262890683122, 1.000000000000000000, 0.9659258262890683122, 1.000000000000000000, 0.9659258262890683122, 1.000000000000000000, 0.9659258262890683122, 1.000000000000000000, 0.9659258262890683122, 1.000000000000000000, 0.9659258262890683122, 1.000000000000000000, 0.9659258262890683122, 1.000000000000000000, 0.9659258262890683122, 1.000000000000000000, 0.9659258262890683122, 1.000000000000000000, 0.9659258262890683122, 1.000000000000000000, 0.9659258262890683122, 1.000000000000000000, 0.9659258262890683122, 1.000000000000000000, 0.9659258262890683122, 1.000000000000000000, 0.9659258262890683122, 1.000000000000000000, 0.9659258262890683122, 1.000000000000000000, 0.9659258262890683122, 1.000000000000000000, 0.9659258262890683122, 1.000000000000000000, 0.9659258262890683122, 1.000000000000000000, 0.9659258262890683122, 1.000000000000000000, 0.9659258262890683122, 1.000000000000000000, 0.9659258262890683122, 1.000000000000000000, 0.9659258262890683122, 1.000000000000000000, 0.9659258262890683122, 1.000000000000000000, 0.9659258262890683122, 1.000000000000000000, 0.9659258262890683122, 1.000000000000000000, 0.9659258262890683122, 1.000000000000000000, 0.9659258262890683122, 1.000000000000000000, 0.9659258262890683122, 1.000000000000000000, 0.9659258262890683122, 1.000000000000000000, 0.9659258262890683122, 1.000000000000000000, 0.9659258262890683122, 1.000000000000000000, 0.9659258262890683122, 1.000000000000000000, 0.9659258262890683122, 1.000000000000000000, 0.9659258262890683122, 1.000000000000000000, 0.9659258262890683122, 1.000000000000000000, 0.9659258262890683122, 1.000000000000000000, 0.9659258262890683122, 1.000000000000000000, 0.9659258262890683122, 1.000000000000000000, 0.9659258262890683122, 1.000000000000000000, 0.9659258262890683122, 1.000000000000000000, 0.9659258262890683122, 1.000000000000000000, 0.9659258262890683122, 1.000000000000000000, 0.9659258262890683122, 1.000000000000000000, 0.9659258262890683122, 1.000000000000000000, 0.9659258262890683122, 1.000000000000000000, 0.9659258262890683122, 1.000000000000000000, 0.9659258262890683122, 1.000000000000000000, 0.9659258262890683122, 1.000000000000000000, 0.9659258262890683122, 1.000000000000000000, 0.9659258262890683122, 1.000000000000000000, 0.9659258262890683122, 1.000000000000000000, 0.9659258262890683122, 1.000000000000000000, 0.9659258262890683122, 1.000000000000000000, 0.9659258262890683122, 1.000000000000000000, 0.9659258262890683122, 1.000000000000000000, 0.9659258262890683122, 1.000000000000000000, 0.9659258262890683122, 1.000000000000000000, 0.9659258262890683122, 1.000000000000000000, 0.9659258262890683122, 1.000000000000000000, 0.9659258262890683122, 1.000000000000000000, 0.9659258262890683122, 1.000000000000000000, 0.9659258262890683122, 1.000000000000000000, 0.9659258262890683122, 1.000000000000000000, 0.9659258262890683122, 1.000000000000000000, 0.9659258262890683122, 1.000000000000000000, 0.9659258262890683122, 1.000000000000000000, 0.9659258262890683122, 1.000000000000000000, 0.9659258262890683122, 1.000000000000000000, 0.9659258262890683122, 1.000000000000000000, 0.9659258262890683122, 1.000000000000000000, 0.9659258262890683122, 1.000000000000000000, 0.9659258262890683122, 1.000000000000000000, 0.9659258262890683122, 1.000000000000000000, 0.9659258262890683122, 1.000000000000000000, 0.9659258262890683122, 1.000000000000000000, 0.9659258262890683122, 1.000000000000000000, 0.9659258262890683122, 1.000000000000000000, 0.9659258262890683122, 1.000000000000000000, 0.9659258262890683122, 1.000000000000000000, 0.9659258262890683122, 1.000000000000000000, 0.9659258262890683122, 1.000000000000000000, 0.9659258262890683122, 1.000000000000000000, 0.9659258262890683122, 1.000000000000000000, 0.9659258262890683122, 1.000000000000000000, 0.9659258262890683122, 1.000000000000000000, 0.9659258262890683122, 1.000000000000000000, 0.9659258262890683122, 1.000000000000000000, 0.9659258262890683122, 1.000000000000000000, 0.9659258262890683122, 1.000000000000000000, 0.9659258262890683122, 1.000000000000000000, 0.9659258262890683122, 1.000000000000000000, 0.9659258262890683122, 1.000000000000000000, 0.9659258262890683122, 1.000000000000000000, 0.9659258262890683122, 1.000000000000000000, 0.9659258262890683122, 1.000000000000000000, 0.9659258262890683122, 1.000000000000000000, 0.9659258262890683122, 1.000000000000000000, 0.9659258262890683122, 1.000000000000000000, 0.9659258262890683122, 1.000000000000000000, 0.9659258262890683122, 1.000000000000000000, 0.9659258262890683122, 1.000000000000000000, 0.9659258262890683122, 1.000000000000000000, 0.9659258262890683122, 1.000000000000000000, 0.9659258262890683122, 1.000000000000000000, 0.9659258262890683122, 1.000000000000000000, 0.9659258262890683122, 1.000000000000000000, 0.9659258262890683122, 1.000000000000000000, 0.9659258262890683122, 1.000000000000000000, 0.9659258262890683122, 1.000000000000000000, 0.9659258262890683122, 1.000000000000000000, 0.9659258262890683122, 1.000000000000000000, 0.9659258262890683122, 1.000000000000000000, 0.9659258262890683122, 1.000000000000000000, 0.9659258262890683122, 1.000000000000000000, 0.9659258262890683122, 1.000000000000000000, 0.9659258262890683122, 1.000000000000000000, 0.9659258262890683122, 1.000000000000000000, 0.9659258262890683122, 1.000000000000000000, 0.9659258262890683122, 1.000000000000000000, 0.9659258262890683122, 1.000000000000000000, 0.9659258262890683122, 1.000000000000000000, 0.9659258262890683122, 1.000000000000000000, 0.9659258262890683122, 1.000000000000000000, 0.9659258262890683122, 1.000000000000000000, 0.9659258262890683122, 1.000000000000000000, 0.9659258262890683122, 1.000000000000000000, 0.9659258262890683122, 1.000000000000000000, 0.9659258262890683122, 1.000000000000000000, 0.9659258262890683122, 1.000000000000000000, 0.9659258262890683122, 1.000000000000000000, 0.9659258262890683122, 1.000000000000000000, 0.9659258262890683122, 1.000000000000000000, 0.9659258262890683122, 1.000000000000000000, 0.9659258262890683122, 1.000000000000000000, 0.9659258262890683122, 1.000000000000000000, 0.9659258262890683122, 1.000000000000000000, 0.9659258262890683122, 1.000000000000000000, 0.9659258262890683122, 1.000000000000000000, 0.9659258262890683122, 1.000000000000000000, 0.9659258262890683122, 1.000000000000000000, 0.9659258262890683122, 1.000000000000000000, 0.9659258262890683122, 1.000000000000000000, 0.9659258262890683122, 1.000000000000000000, 0.9659258262890683122, 1.000000000000000000, 0.9659258262890683122, 1.000000000000000000, 0.9659258262890683122, 1.000000000000000000, 0.9659258262890683122, 1.000000000000000000, 0.9659258262890683122, 1.000000000000000000, 0.9659258262890683122, 1.000000000000000000, 0.9659258262890683122, 1.000000000000000000, 0.9659258262890683122, 1.000000000000000000, 0.9659258262890683122, 1.000000000000000000, 0.9659258262890683122, 1.000000000000000000, 0.9659258262890683122, 1.000000000000000000, 0.9659258262890683122, 1.000000000000000000, 0.9659258262890683122, 1.000000000000000000),
 ( 1.000000000000000000, 0.9659258262890683122, 1.000000000000000000, 0.9659258262890683122, 1.000000000000000000, 0.9659258262890683122, 1.000000000000000000, 0.9659258262890683122, 1.000000000000000000, 0.9659258262890683122, 1.000000000000000000, 0.9659258262890683122, 1.000000000000000000, 0.9659258262890683122, 1.000000000000000000, 0.9659258262890683122, 1.000000000000000000, 0.9659258262890683122, 1.000000000000000000, 0.9659258262890683122, 1.000000000000000000, 0.9659258262890683122, 1.000000000000000000, 0.9659258262890683122, 1.000000000000000000, 0.9659258262890683122, 1.000000000000000000, 0.9659258262890683122, 1.000000000000000000, 0.9659258262890683122, 1.000000000000000000, 0.9659258262890683122, 1.000000000000000000, 0.9659258262890683122, 1.000000000000000000, 0.9659258262890683122, 1.000000000000000000, 0.9659258262890683122, 1.000000000000000000, 0.9659258262890683122, 1.000000000000000000, 0.9659258262890683122, 1.000000000000000000, 0.9659258262890683122, 1.000000000000000000, 0.9659258262890683122, 1.000000000000000000, 0.9659258262890683122, 1.000000000000000000, 0.9659258262890683122, 1.000000000000000000, 0.9659258262890683122, 1.000000000000000000, 0.9659258262890683122, 1.000000000000000000, 0.9659258262890683122, 1.000000000000000000, 0.9659258262890683122, 1.000000000000000000, 0.9659258262890683122, 1.000000000000000000, 0.9659258262890683122, 1.000000000000000000, 0.9659258262890683122, 1.000000000000000000, 0.9659258262890683122, 1.000000000000000000, 0.9659258262890683122, 1.000000000000000000, 0.9659258262890683122, 1.000000000000000000, 0.9659258262890683122, 1.000000000000000000, 0.9659258262890683122, 1.000000000000000000, 0.9659258262890683122, 1.000000000000000000, 0.9659258262890683122, 1.000000000000000000, 0.9659258262890683122, 1.000000000000000000, 0.9659258262890683122, 1.000000000000000000, 0.9659258262890683122, 1.000000000000000000, 0.9659258262890683122, 1.000000000000000000, 0.9659258262890683122, 1.000000000000000000, 0.9659258262890683122, 1.000000000000000000, 0.9659258262890683122, 1.000000000000000000, 0.9659258262890683122, 1.000000000000000000, 0.9659258262890683122, 1.000000000000000000, 0.9659258262890683122, 1.000000000000000000, 0.9659258262890683122, 1.000000000000000000, 0.9659258262890683122, 1.000000000000000000, 0.9659258262890683122, 1.000000000000000000, 0.9659258262890683122, 1.000000000000000000, 0.9659258262890683122, 1.000000000000000000, 0.9659258262890683122, 1.000000000000000000, 0.9659258262890683122, 1.000000000000000000, 0.9659258262890683122, 1.000000000000000000, 0.9659258262890683122, 1.000000000000000000, 0.9659258262890683122, 1.000000000000000000, 0.9659258262890683122, 1.000000000000000000, 0.9659258262890683122, 1.000000000000000000, 0.9659258262890683122, 1.000000000000000000, 0.9659258262890683122, 1.000000000000000000, 0.9659258262890683122, 1.000000000000000000, 0.9659258262890683122, 1.000000000000000000, 0.9659258262890683122, 1.000000000000000000, 0.9659258262890683122, 1.000000000000000000, 0.9659258262890683122, 1.000000000000000000, 0.9659258262890683122, 1.000000000000000000, 0.9659258262890683122, 1.000000000000000000, 0.9659258262890683122, 1.000000000000000000, 0.9659258262890683122, 1.000000000000000000, 0.9659258262890683122, 1.000000000000000000, 0.9659258262890683122, 1.000000000000000000, 0.9659258262890683122, 1.000000000000000000, 0.9659258262890683122, 1.000000000000000000, 0.9659258262890683122, 1.000000000000000000, 0.9659258262890683122, 1.000000000000000000, 0.9659258262890683122, 1.000000000000000000, 0.9659258262890683122, 1.000000000000000000, 0.9659258262890683122, 1.000000000000000000, 0.9659258262890683122, 1.000000000000000000, 0.9659258262890683122, 1.000000000000000000, 0.9659258262890683122, 1.000000000000000000, 0.9659258262890683122, 1.000000000000000000, 0.9659258262890683122, 1.000000000000000000, 0.9659258262890683122, 1.000000000000000000, 0.9659258262890683122, 1.000000000000000000, 0.9659258262890683122, 1.000000000000000000, 0.9659258262890683122, 1.000000000000000000, 0.9659258262890683122, 1.000000000000000000, 0.9659258262890683122, 1.000000000000000000, 0.9659258262890683122, 1.000000000000000000, 0.9659258262890683122, 1.000000000000000000, 0.9659258262890683122, 1.000000000000000000, 0.9659258262890683122, 1.000000000000000000, 0.9659258262890683122, 1.000000000000000000, 0.9659258262890683122, 1.000000000000000000, 0.9659258262890683122, 1.000000000000000000, 0.9659258262890683122, 1.000000000000000000, 0.9659258262890683122, 1.000000000000000000, 0.9659258262890683122, 1.000000000000000000, 0.9659258262890683122, 1.000000000000000000, 0.9659258262890683122, 1.000000000000000000, 0.9659258262890683122, 1.000000000000000000, 0.9659258262890683122, 1.000000000000000000, 0.9659258262890683122, 1.000000000000000000, 0.9659258262890683122, 1.000000000000000000, 0.9659258262890683122, 1.000000000000000000, 0.9659258262890683122, 1.000000000000000000, 0.9659258262890683122, 1.000000000000000000, 0.9659258262890683122, 1.000000000000000000, 0.9659258262890683122, 1.000000000000000000, 0.9659258262890683122, 1.000000000000000000, 0.9659258262890683122, 1.000000000000000000, 0.9659258262890683122, 1.000000000000000000, 0.9659258262890683122, 1.000000000000000000, 0.9659258262890683122, 1.000000000000000000, 0.9659258262890683122, 1.000000000000000000, 0.9659258262890683122, 1.000000000000000000, 0.9659258262890683122, 1.000000000000000000, 0.9659258262890683122, 1.000000000000000000, 0.9659258262890683122, 1.000000000000000000, 0.9659258262890683122, 1.000000000000000000, 0.9659258262890683122, 1.000000000000000000, 0.9659258262890683122, 1.000000000000000000, 0.9659258262890683122, 1.000000000000000000, 0.9659258262890683122, 1.000000000000000000, 0.9659258262890683122, 1.000000000000000000, 0.9659258262890683122, 1.000000000000000000, 0.9659258262890683122, 1.000000000000000000, 0.9659258262890683122, 1.000000000000000000, 0.9659258262890683122, 1.000000000000000000, 0.9659258262890683122, 1.000000000000000000, 0.9659258262890683122, 1.000000000000000000, 0.9659258262890683122, 1.000000000000000000, 0.9659258262890683122, 1.000000000000000000, 0.9659258262890683122, 1.000000000000000000, 0.9659258262890683122, 1.000000000000000000, 0.9659258262890683122, 1.000000000000000000, 0.9659258262890683122, 1.000000000000000000, 0.9659258262890683122, 1.000000000000000000, 0.9659258262890683122, 1.000000000000000000, 0.9659258262890683122, 1.000000000000000000, 0.9659258262890683122, 1.000000000000000000, 0.9659258262890683122, 1.000000000000000000, 0.9659258262890683122, 1.000000000000000000, 0.9659258262890683122, 1.000000000000000000, 0.9659258262890683122, 1.000000000000000000, 0.9659258262890683122, 1.000000000000000000, 0.9659258262890683122, 1.000000000000000000, 0.9659258262890683122, 1.000000000000000000, 0.9659258262890683122, 1.000000000000000000, 0.9659258262890683122, 1.000000000000000000, 0.9659258262890683122, 1.000000000000000000, 0.9659258262890683122, 1.000000000000000000, 0.9659258262890683122, 1.000000000000000000, 0.9659258262890683122, 1.000000000000000000, 0.9659258262890683122, 1.000000000000000000, 0.9659258262890683122, 1.000000000000000000, 0.9659258262890683122, 1.000000000000000000, 0.9659258262890683122, 1.000000000000000000, 0.9659258262890683122, 1.000000000000000000, 0.9659258262890683122, 1.000000000000000000, 0.9659258262890683122, 1.000000000000000000, 0.9659258262890683122, 1.000000000000000000, 0.9659258262890683122, 1.000000000000000000, 0.9659258262890683122, 1.000000000000000000, 0.9659258262890683122, 1.000000000000000000, 0.9659258262890683122, 1.000000000000000000, 0.9659258262890683122, 1.000000000000000000, 0.9659258262890683122, 1.000000000000000000, 0.9659258262890683122, 1.000000000000000000, 0.9659258262890683122, 1.000000000000000000, 0.9659258262890683122, 1.000000000000000000, 0.9659258262890683122, 1.000000000000000000, 0.9659258262890683122, 1.000000000000000000, 0.9659258262890683122, 1.000000000000000000, 0.9659258262890683122, 1.000000000000000000, 0.9659258262890683122, 1.000000000000000000, 0.9659258262890683122, 1.000000000000000000, 0.9659258262890683122, 1.000000000000000000, 0.9659258262890683122, 1.000000000000000000, 0.9659258262890683122, 1.000000000000000000, 0.9659258262890683122, 1.000000000000000000, 0.9659258262890683122, 1.000000000000000000, 0.9659258262890683122, 1.000000000000000000, 0.9659258262890683122, 1.000000000000000000, 0.9659258262890683122, 1.000000000000000000, 0.9659258262890683122, 1.000000000000000000, 0.9659258262890683122, 1.000000000000000000, 0.9659258262890683122, 1.000000000000000000, 0.9659258262890683122, 1.000000000000000000, 0.9659258262890683122, 1.000000000000000000, 0.9659258262890683122, 1.000000000000000000, 0.9659258262890683122, 1.000000000000000000, 0.9659258262890683122, 1.000000000000000000, 0.9659258262890683122, 1.000000000000000000, 0.9659258262890683122, 1.000000000000000000, 0.9659258262890683122, 1.000000000000000000, 0.9659258262890683122, 1.000000000000000000, 0.9659258262890683122, 1.000000000000000000, 0.9659258262890683122, 1.000000000000000000, 0.9659258262890683122, 1.000000000000000000, 0.9659258262890683122, 1.000000000000000000, 0.9659258262890683122, 1.000000000000000000, 0.9659258262890683122, 1.000000000000000000, 0.9659258262890683122, 1.000000000000000000, 0.9659258262890683122, 1.000000000000000000, 0.9659258262890683122, 1.000000000000000000, 0.9659258262890683122, 1.000000000000000000, 0.9659258262890683122, 1.000000000000000000, 0.9659258262890683122, 1.000000000000000000, 0.9659258262890683122, 1.000000000000000000, 0.9659258262890683122, 1.000000000000000000, 0.9659258262890683122, 1.000000000000000000, 0.9659258262890683122, 1.000000000000000000, 0.9659258262890683122, 1.000000000000000000, 0.9659258262890683122, 1.000000000000000000, 0.9659258262890683122, 1.000000000000000000, 0.9659258262890683122, 1.000000000000000000, 0.9659258262890683122, 1.000000000000000000, 0.9659258262890683122, 1.000000000000000000, 0.9659258262890683122, 1.000000000000000000, 0.9659258262890683122, 1.000000000000000000, 0.9659258262890683122, 1.000000000000000000, 0.9659258262890683122, 1.000000000000000000, 0.9659258262890683122, 1.000000000000000000, 0.9659258262890683122, 1.000000000000000000, 0.9659258262890683122, 1.000000000000000000, 0.9659258262890683122, 1.000000000000000000, 0.9659258262890683122, 1.000000000000000000, 0.9659258262890683122, 1.000000000000000000, 0.9659258262890683122, 1.000000000000000000, 0.9659258262890683122, 1.000000000000000000, 0.9659258262890683122, 1.000000000000000000, 0.9659258262890683122, 1.000000000000000000, 0.9659258262890683122, 1.000000000000000000, 0.9659258262890683122, 1.000000000000000000, 0.9659258262890683122, 1.000000000000000000, 0.9659258262890683122, 1.000000000000000000, 0.9659258262890683122, 1.000000000000000000, 0.9659258262890683122, 1.000000000000000000, 0.9659258262890683122, 1.000000000000000000, 0.9659258262890683122, 1.000000000000000000, 0.9659258262890683122, 1.000000000000000000, 0.9659258262890683122, 1.000000000000000000, 0.9659258262890683122, 1.000000000000000000, 0.9659258262890683122, 1.000000000000000000, 0.9659258262890683122, 1.000000000000000000, 0.9659258262890683122, 1.000000000000000000, 0.9659258262890683122, 1.000000000000000000, 0.9659258262890683122, 1.000000000000000000, 0.9659258262890683122, 1.000000000000000000, 0.9659258262890683122, 1.000000000000000000) ) ) 
 REPRESENTATION_ITEM ( '' )  SURFACE ( )  );
#20410=CARTESIAN_POINT ( 'NONE',  ( 0.9251968503937013644, 0.1012011053420775880, -0.2882089793578256898 ) ) ;
#20411=CARTESIAN_POINT ( 'NONE',  ( 0.5183727034120741983, -0.6692913385826771977, 0.1292274648535927661 ) ) ;
#20412=ORIENTED_EDGE ( 'NONE', *, *, #60997, .T. ) ;
#20413=CARTESIAN_POINT ( 'NONE',  ( 1.614173228346457378, 0.9921945702958886448, -0.1372047244094476148 ) ) ;
#20415=CARTESIAN_POINT ( 'NONE',  ( 1.115485564304462551, -0.4281496062992127816, -0.4176697321401328100 ) ) ;
#20416=CARTESIAN_POINT ( 'NONE',  ( 1.515748031496063186, -0.4536011799217368745, -0.2665933059059886201 ) ) ;
#20418=CARTESIAN_POINT ( 'NONE',  ( -0.9711286089238838626, -0.5023911411419708095, 0.1820866141732285504 ) ) ;
#20419=CARTESIAN_POINT ( 'NONE',  ( -1.601049868766403650, 0.1283753931104746893, -0.1820866141732285504 ) ) ;
#20421=CARTESIAN_POINT ( 'NONE',  ( 0.6561679790026253567, 0.2306618581243848609, 0.2411417322834645549 ) ) ;
#20422=CARTESIAN_POINT ( 'NONE',  ( -0.9842519685039360366, 0.1771653543307087630, 0.000000000000000000 ) ) ;
#20423=CARTESIAN_POINT ( 'NONE',  ( 0.2165354330708668673, 0.07958543189024071263, -0.2665933059059888421 ) ) ;
#20424=CARTESIAN_POINT ( 'NONE',  ( -0.3215223097112853146, -0.3162353388693405765, 0.4822834645669290543 ) ) ;
#20425=CARTESIAN_POINT ( 'NONE',  ( -1.279527559055116948, 0.07958543189024071263, -0.2665933059059888421 ) ) ;
#20427=CARTESIAN_POINT ( 'NONE',  ( 0.7283464566929140904, -0.5400638737290845981, -0.3530559997133363437 ) ) ;
#20428=CARTESIAN_POINT ( 'NONE',  ( -1.404199475065615932, -0.4281496062992127816, -0.4176697321401328100 ) ) ;
#20430=CARTESIAN_POINT ( 'NONE',  ( -0.8398950131233589023, -0.6046776061558809534, -0.2411417322834644161 ) ) ;
#20431=CARTESIAN_POINT ( 'NONE',  ( -0.2165354330708654795, -0.4536011799217368745, -0.2665933059059886201 ) ) ;
#20432=CARTESIAN_POINT ( 'NONE',  ( -1.384514435695537005, -0.6692913385826773087, -0.1292274648535924053 ) ) ;
#20433=CARTESIAN_POINT ( 'NONE',  ( 0.8530183727034128527, -0.3690944881889763329, 0.3153832671262228327 ) ) ;
#20434=CARTESIAN_POINT ( 'NONE',  ( -0.3674540682414692561, -0.5023911411419708095, -0.1820866141732282451 ) ) ;
#20435=CARTESIAN_POINT ( 'NONE',  ( -0.9842519685039365918, -0.6692913385826771977, 8.415575281601705876E-17 ) ) ;
#20436=CARTESIAN_POINT ( 'NONE',  ( -1.286089238845143479, -0.6046776061558807314, 0.2411417322834647770 ) ) ;
#20437=CARTESIAN_POINT ( 'NONE',  ( -1.377952755905511140, -0.6692913385826771977, 8.415575281601705876E-17 ) ) ;
#20439=CARTESIAN_POINT ( 'NONE',  ( 1.207349081364829990, 0.1283753931104748280, 0.1820866141732283561 ) ) ;
#20441=CARTESIAN_POINT ( 'NONE',  ( 0.6102362204724416372, 0.1660481256975883668, -0.3530559997133364547 ) ) ;
#20442=CARTESIAN_POINT ( 'NONE',  ( -1.535433070866141225, -0.6692913385826771977, 8.415575281601705876E-17 ) ) ;
#20443=CARTESIAN_POINT ( 'NONE',  ( -1.725721784776902190, -0.05778040916215522460, 0.4822834645669289988 ) ) ;
#20447=CARTESIAN_POINT ( 'NONE',  ( -0.7414698162729651543, -0.5511811023622046335, 0.09757992244046803654 ) ) ;
#20448=CARTESIAN_POINT ( 'NONE',  ( 0.5774278215223103139, -0.6046776061558809534, -0.2411417322834644161 ) ) ;
#20449=CARTESIAN_POINT ( 'NONE',  ( -1.187664041994750175, -0.08942795157528024563, -0.3641732283464568787 ) ) ;
#20451=CARTESIAN_POINT ( 'NONE',  ( -1.469816272965878357, -0.6046776061558809534, -0.2411417322834644161 ) ) ;
#20452=CARTESIAN_POINT ( 'NONE',  ( 0.8202099737532814183, -0.6692913385826773087, -0.1292274648535924053 ) ) ;
#20453=CARTESIAN_POINT ( 'NONE',  ( 0.3740157480314966754, -0.5400638737290844871, 0.3530559997133364547 ) ) ;
#20454=CARTESIAN_POINT ( 'NONE',  ( 1.154855643044620184, 0.2306618581243847221, -0.2411417322834647770 ) ) ;
#20455=CARTESIAN_POINT ( 'NONE',  ( -1.686351706036744558, 0.1771653543307087075, -0.09757992244046823083 ) ) ;
#20461=CARTESIAN_POINT ( 'NONE',  ( 0.6758530183727039509, -0.5511811023622046335, 0.09757992244046803654 ) ) ;
#20462=CARTESIAN_POINT ( 'NONE',  ( 0.1246719160104994284, -0.5511811023622046335, 0.09757992244046803654 ) ) ;
#20463=CARTESIAN_POINT ( 'NONE',  ( -0.09186351706036689768, 0.05413385826771626580, -0.4176697321401330321 ) ) ;
#20464=CARTESIAN_POINT ( 'NONE',  ( 1.312335958005249825, 0.2306618581243847221, -0.2411417322834647770 ) ) ;
#20466=CARTESIAN_POINT ( 'NONE',  ( 0.1968503937007881344, -0.5511811023622047445, 6.969142054262312111E-17 ) ) ;
#20467=CARTESIAN_POINT ( 'NONE',  ( -0.8136482939632537770, 0.2306618581243847221, -0.2411417322834647770 ) ) ;
#20468=CARTESIAN_POINT ( 'NONE',  ( -1.522309711286088607, -0.6046776061558807314, 0.2411417322834647770 ) ) ;
#20469=CARTESIAN_POINT ( 'NONE',  ( 1.036745406824147731, 0.05413385826771666132, 0.4176697321401328100 ) ) ;
#20471=LINE ( 'NONE', #28022, #30428 ) ;
#20473=EDGE_LOOP ( 'NONE', ( #16050, #3704, #48420, #36430 ) ) ;
#20474=CARTESIAN_POINT ( 'NONE',  ( -1.213910761154854745, 0.2952755905511810774, -0.1292274648535930714 ) ) ;
#20475=CARTESIAN_POINT ( 'NONE',  ( -0.8923884514435688198, -0.5023911411419708095, 0.1820866141732285504 ) ) ;
#20476=CARTESIAN_POINT ( 'NONE',  ( -1.266404199475064773, -0.05778040916215560624, -0.4822834645669293319 ) ) ;
#20478=CARTESIAN_POINT ( 'NONE',  ( -0.4605079024601024251, -1.150887559458346504E-15, 0.3627985898453527924 ) ) ;
#20479=CARTESIAN_POINT ( 'NONE',  ( 1.476377952755906442, -0.5400638737290844871, 0.3530559997133364547 ) ) ;
#20480=CARTESIAN_POINT ( 'NONE',  ( -1.279527559055116948, -0.5400638737290844871, 0.3530559997133364547 ) ) ;
#20481=CARTESIAN_POINT ( 'NONE',  ( 0.2099737532808405305, 0.2306618581243847221, -0.2411417322834647770 ) ) ;
#20482=CARTESIAN_POINT ( 'NONE',  ( -1.463254593175852492, 0.2952755905511811885, 0.1292274648535926551 ) ) ;
#20484=CARTESIAN_POINT ( 'NONE',  ( 0.7086614173228352742, -0.1870078740157480879, -0.4822834645669291653 ) ) ;
#20486=CARTESIAN_POINT ( 'NONE',  ( -0.9251968503937002541, -0.4536011799217368745, -0.2665933059059886201 ) ) ;
#20487=ORIENTED_EDGE ( 'NONE', *, *, #26568, .F. ) ;
#20490=CARTESIAN_POINT ( 'NONE',  ( -1.568241469816272105, -0.08942795157527998196, 0.3641732283464567121 ) ) ;
#20491=CARTESIAN_POINT ( 'NONE',  ( -1.325459317585300889, -0.4281496062992127816, -0.4176697321401328100 ) ) ;
#20492=CARTESIAN_POINT ( 'NONE',  ( -1.463254593175852492, 0.2952755905511811885, 0.1292274648535926551 ) ) ;
#20494=CARTESIAN_POINT ( 'NONE',  ( -1.620734908136482577, -0.6692913385826773087, -0.1292274648535924053 ) ) ;
#20495=CARTESIAN_POINT ( 'NONE',  ( -1.135170603674539924, -0.6692913385826771977, 0.1292274648535927661 ) ) ;
#20496=CARTESIAN_POINT ( 'NONE',  ( -1.555118110236219930, -0.5400638737290845981, -0.3530559997133363437 ) ) ;
#20498=CARTESIAN_POINT ( 'NONE',  ( -0.7974104941589342799, -2.567464376874931580E-15, -0.4445507791589072832 ) ) ;
#20499=CARTESIAN_POINT ( 'NONE',  ( 0.1181102362204730916, 0.1771653543307087630, 0.000000000000000000 ) ) ;
#20502=CARTESIAN_POINT ( 'NONE',  ( -0.4921259842519677963, -0.4536011799217367080, 0.2665933059059888421 ) ) ;
#20503=CARTESIAN_POINT ( 'NONE',  ( -0.9383202099737524282, -0.3162353388693409650, -0.4822834645669289433 ) ) ;
#20504=CARTESIAN_POINT ( 'NONE',  ( 0.8202099737532813073, 0.2952755905511811885, 0.1292274648535926551 ) ) ;
#20505=CARTESIAN_POINT ( 'NONE',  ( -1.076115485564303809, -0.6046776061558809534, -0.2411417322834644161 ) ) ;
#20508=CARTESIAN_POINT ( 'NONE',  ( -1.069553805774277722, -0.6692913385826773087, -0.1292274648535924053 ) ) ;
#20510=CARTESIAN_POINT ( 'NONE',  ( 1.030183727034121421, -0.3162353388693409650, -0.4822834645669289433 ) ) ;
#20511=CARTESIAN_POINT ( 'NONE',  ( -1.719160104986876103, -0.004921259842519576551, 0.3153832671262227771 ) ) ;
#20512=CARTESIAN_POINT ( 'NONE',  ( -1.640419947506561060, -0.4281496062992127816, -0.4176697321401328100 ) ) ;
#20517=CARTESIAN_POINT ( 'NONE',  ( -0.1377952755905504645, -0.5400638737290845981, -0.3530559997133363437 ) ) ;
#20518=CARTESIAN_POINT ( 'NONE',  ( -1.292650918635170010, 0.1771653543307087075, -0.09757992244046823083 ) ) ;
#20519=CARTESIAN_POINT ( 'NONE',  ( -0.8202099737532801971, -0.6692913385826771977, 0.1292274648535927661 ) ) ;
#20521=CARTESIAN_POINT ( 'NONE',  ( -1.312335958005248715, -0.6046776061558809534, -0.2411417322834644161 ) ) ;
#20522=CARTESIAN_POINT ( 'NONE',  ( -0.6824146981627288167, 0.1539470093639523085, 0.1968503937007873850 ) ) ;
#20523=CARTESIAN_POINT ( 'NONE',  ( -0.8989501312335946848, 0.2952755905511810774, -0.1292274648535930714 ) ) ;
#20524=CARTESIAN_POINT ( 'NONE',  ( -0.2624671916010490880, 0.2306618581243847221, -0.2411417322834647770 ) ) ;
#20526=CARTESIAN_POINT ( 'NONE',  ( 0.7414698162729663755, -0.5511811023622048555, -0.09757992244046775898 ) ) ;
#20528=CARTESIAN_POINT ( 'NONE',  ( 0.3215223097112867578, -0.2845877964562161244, -0.3641732283464567121 ) ) ;
#20529=CARTESIAN_POINT ( 'NONE',  ( 1.443569553805774897, 0.1283753931104748280, 0.1820866141732283561 ) ) ;
#20530=CARTESIAN_POINT ( 'NONE',  ( 1.351706036745407458, -0.4281496062992127816, -0.4176697321401328100 ) ) ;
#20531=CARTESIAN_POINT ( 'NONE',  ( 0.1181102362204730916, 0.1771653543307087630, 0.000000000000000000 ) ) ;
#20533=CARTESIAN_POINT ( 'NONE',  ( -1.174540682414697335, -0.05778040916215522460, 0.4822834645669289988 ) ) ;
#20534=CARTESIAN_POINT ( 'NONE',  ( 1.325459317585302665, 0.05413385826771626580, -0.4176697321401330321 ) ) ;
#20535=B_SPLINE_CURVE_WITH_KNOTS ( 'NONE', 3,
 ( #3960, #17021, #36760, #29623 ),
 .UNSPECIFIED., .F., .F.,
 ( 4, 4 ),
 ( 1.734723475976806902E-18, 0.001357026659661017542 ),
 .UNSPECIFIED. ) ;
#20537=CARTESIAN_POINT ( 'NONE',  ( -0.5314960629921250401, 0.07958543189024085140, 0.2665933059059887866 ) ) ;
#20539=CARTESIAN_POINT ( 'NONE',  ( -0.4608550785314876053, 0.02791078216816064370, 0.4328096321851915285 ) ) ;
#20540=CARTESIAN_POINT ( 'NONE',  ( 0.2165354330708668673, -0.5400638737290844871, 0.3530559997133364547 ) ) ;
#20542=CARTESIAN_POINT ( 'NONE',  ( 1.043307086614173818, -0.4536011799217368745, -0.2665933059059886201 ) ) ;
#20543=CARTESIAN_POINT ( 'NONE',  ( 0.3018372703412079971, -0.3690944881889763329, 0.3153832671262228327 ) ) ;
#20544=CARTESIAN_POINT ( 'NONE',  ( -0.3477690288713902178, 0.2952755905511810774, -0.1292274648535930714 ) ) ;
#20545=CARTESIAN_POINT ( 'NONE',  ( -1.706036745406823485, 0.2306618581243848609, 0.2411417322834645549 ) ) ;
#20546=CARTESIAN_POINT ( 'NONE',  ( -0.5511811023622038563, -0.1870078740157479769, 0.3641732283464567677 ) ) ;
#20548=CARTESIAN_POINT ( 'NONE',  ( 0.4068241469816281097, 0.05413385826771666132, 0.4176697321401328100 ) ) ;
#20549=CARTESIAN_POINT ( 'NONE',  ( -0.8858267716535425107, -0.5400638737290844871, 0.3530559997133364547 ) ) ;
#20551=EDGE_CURVE ( 'NONE', #31839, #19838, #40124, .T. ) ;
#20553=CARTESIAN_POINT ( 'NONE',  ( 0.05905511811023681640, 0.07958543189024071263, -0.2665933059059888421 ) ) ;
#20554=CARTESIAN_POINT ( 'NONE',  ( -0.6102362204724400829, -0.5400638737290845981, -0.3530559997133363437 ) ) ;
#20555=CARTESIAN_POINT ( 'NONE',  ( -1.049868766404198794, -0.6046776061558807314, 0.2411417322834647770 ) ) ;
#20556=CARTESIAN_POINT ( 'NONE',  ( -1.233595800524933894, -0.5023911411419708095, -0.1820866141732282451 ) ) ;
#20558=CARTESIAN_POINT ( 'NONE',  ( -0.9448818897637790704, -0.1870078740157480601, -0.3641732283464567677 ) ) ;
#20560=CARTESIAN_POINT ( 'NONE',  ( 1.325459317585302665, 0.05413385826771626580, -0.4176697321401330321 ) ) ;
#20566=CARTESIAN_POINT ( 'NONE',  ( 1.456692913385827515, 0.1771653543307087630, 0.000000000000000000 ) ) ;
#20567=CARTESIAN_POINT ( 'NONE',  ( -1.410761154855642463, -0.05778040916215522460, 0.4822834645669289988 ) ) ;
#20568=CARTESIAN_POINT ( 'NONE',  ( 1.253280839895013710, -0.3162353388693405765, 0.4822834645669290543 ) ) ;
#20570=CARTESIAN_POINT ( 'NONE',  ( 1.555118110236221041, 0.07958543189024071263, -0.2665933059059888421 ) ) ;
#20571=CARTESIAN_POINT ( 'NONE',  ( 0.5774278215223104249, 0.2306618581243848609, 0.2411417322834645549 ) ) ;
#20572=CARTESIAN_POINT ( 'NONE',  ( -0.5249343832020990641, 0.2306618581243848609, 0.2411417322834645549 ) ) ;
#20575=CARTESIAN_POINT ( 'NONE',  ( 0.7545931758530188826, -0.5511811023622046335, 0.09757992244046803654 ) ) ;
#20580=CARTESIAN_POINT ( 'NONE',  ( 0.05249343832021075018, 0.2306618581243847221, -0.2411417322834647770 ) ) ;
#20581=CARTESIAN_POINT ( 'NONE',  ( 1.384514435695538337, -0.6692913385826771977, 0.1292274648535927661 ) ) ;
#20582=CARTESIAN_POINT ( 'NONE',  ( 0.3740157480314966754, -0.5400638737290844871, 0.3530559997133364547 ) ) ;
#20583=CARTESIAN_POINT ( 'NONE',  ( 1.325459317585302665, -0.4281496062992124485, 0.4176697321401328655 ) ) ;
#20584=CARTESIAN_POINT ( 'NONE',  ( -0.4133858267716528645, -0.5400638737290844871, 0.3530559997133364547 ) ) ;
#20585=CARTESIAN_POINT ( 'NONE',  ( -0.1246719160104980823, 0.2952755905511811885, 0.1292274648535926551 ) ) ;
#20586=CARTESIAN_POINT ( 'NONE',  ( 1.594488188976378673, 0.1660481256975885056, 0.3530559997133364547 ) ) ;
#20587=CARTESIAN_POINT ( 'NONE',  ( 1.240157480314961314, -0.5400638737290844871, 0.3530559997133364547 ) ) ;
#20588=CARTESIAN_POINT ( 'NONE',  ( 1.043307086614173818, 0.1660481256975885056, 0.3530559997133364547 ) ) ;
#20590=CARTESIAN_POINT ( 'NONE',  ( 0.6167979002624679463, -0.004921259842519870586, -0.3153832671262229437 ) ) ;
#20594=CARTESIAN_POINT ( 'NONE',  ( -0.4330708661417315697, 0.1771653543307087630, 0.000000000000000000 ) ) ;
#20595=CARTESIAN_POINT ( 'NONE',  ( -0.2034120734908128059, 0.2952755905511811885, 0.1292274648535926551 ) ) ;
#20597=CARTESIAN_POINT ( 'NONE',  ( 0.01968503937007930540, 0.1660481256975885056, 0.3530559997133364547 ) ) ;
#20598=CARTESIAN_POINT ( 'NONE',  ( 0.03280839895013198948, 0.2952755905511811885, 0.1292274648535926551 ) ) ;
#20599=CARTESIAN_POINT ( 'NONE',  ( -0.8398950131233585692, 0.2306618581243848609, 0.2411417322834645549 ) ) ;
#20600=CARTESIAN_POINT ( 'NONE',  ( -1.148293963254592542, -0.6692913385826773087, -0.1292274648535924053 ) ) ;
#20601=CARTESIAN_POINT ( 'NONE',  ( 1.187664041994751285, -0.08942795157527998196, 0.3641732283464567121 ) ) ;
#20604=CARTESIAN_POINT ( 'NONE',  ( 0.9580052493438326877, -0.004921259842519576551, 0.3153832671262227771 ) ) ;
#20606=CARTESIAN_POINT ( 'NONE',  ( 0.2821522309711292364, 0.2952755905511810774, -0.1292274648535930714 ) ) ;
#20607=CARTESIAN_POINT ( 'NONE',  ( 0.8333333333333340365, -0.6692913385826771977, 0.1292274648535927661 ) ) ;
#20609=CARTESIAN_POINT ( 'NONE',  ( -1.719160104986876103, 0.05413385826771666132, 0.4176697321401328100 ) ) ;
#20612=CARTESIAN_POINT ( 'NONE',  ( -0.6758530183727028406, -0.6692913385826773087, -0.1292274648535924053 ) ) ;
#20615=CARTESIAN_POINT ( 'NONE',  ( -1.049868766404198794, -0.5023911411419708095, 0.1820866141732285504 ) ) ;
#20616=CARTESIAN_POINT ( 'NONE',  ( 1.463254593175853824, 0.2952755905511810774, -0.1292274648535930714 ) ) ;
#20617=CARTESIAN_POINT ( 'NONE',  ( 1.108923884514436686, -0.3162353388693409650, -0.4822834645669289433 ) ) ;
#20618=CARTESIAN_POINT ( 'NONE',  ( -0.1181102362204717315, -0.5511811023622047445, 6.969142054262312111E-17 ) ) ;
#20619=CARTESIAN_POINT ( 'NONE',  ( 0.5446194225721792126, -0.05778040916215560624, -0.4822834645669293319 ) ) ;
#20621=CARTESIAN_POINT ( 'NONE',  ( -0.2362204724409440182, -0.1870078740157479769, 0.3641732283464567677 ) ) ;
#20622=CARTESIAN_POINT ( 'NONE',  ( -0.1115485564304456306, 0.2952755905511810774, -0.1292274648535930714 ) ) ;
#20625=CARTESIAN_POINT ( 'NONE',  ( -1.181102362204723644, -0.1870078740157480879, -0.4822834645669291653 ) ) ;
#20626=CARTESIAN_POINT ( 'NONE',  ( 0.6758530183727039509, 0.1771653543307087075, -0.09757992244046823083 ) ) ;
#20628=CARTESIAN_POINT ( 'NONE',  ( -0.7152230971128602510, -0.05778040916215560624, -0.4822834645669293319 ) ) ;
#20629=CARTESIAN_POINT ( 'NONE',  ( -0.2952755905511803003, -0.4536011799217368745, -0.2665933059059886201 ) ) ;
#20630=CARTESIAN_POINT ( 'NONE',  ( -1.595398199321657717, 0.4619154201552267414, -0.1559797534342468872 ) ) ;
#20631=CARTESIAN_POINT ( 'NONE',  ( -0.8398950131233589023, -0.6046776061558809534, -0.2411417322834644161 ) ) ;
#20632=CARTESIAN_POINT ( 'NONE',  ( -0.4527559055118102749, -0.5400638737290845981, -0.3530559997133363437 ) ) ;
#20633=CARTESIAN_POINT ( 'NONE',  ( 0.01312335958005323398, -0.4281496062992127816, -0.4176697321401328100 ) ) ;
#20637=CARTESIAN_POINT ( 'NONE',  ( 0.8464566929133866546, -0.4536011799217367080, 0.2665933059059888421 ) ) ;
#20638=CARTESIAN_POINT ( 'NONE',  ( 1.574803149606299746, -0.1870078740157479769, 0.4822834645669291653 ) ) ;
#20639=CARTESIAN_POINT ( 'NONE',  ( -0.7152230971128602510, -0.08942795157528024563, -0.3641732283464568787 ) ) ;
#20640=CARTESIAN_POINT ( 'NONE',  ( -1.010498687664041384, -0.3690944881889765550, -0.3153832671262227771 ) ) ;
#20641=CARTESIAN_POINT ( 'NONE',  ( -0.7217847769028863381, -0.4281496062992124485, 0.4176697321401328655 ) ) ;
#20642=CARTESIAN_POINT ( 'NONE',  ( -0.06561679790026180015, -0.4281496062992127816, -0.4176697321401328100 ) ) ;
#20643=CARTESIAN_POINT ( 'NONE',  ( 0.6102362204724416372, 0.07958543189024071263, -0.2665933059059888421 ) ) ;
#20645=CARTESIAN_POINT ( 'NONE',  ( 1.102362204724410155, -0.1870078740157479769, 0.3641732283464567677 ) ) ;
#20646=CARTESIAN_POINT ( 'NONE',  ( 0.4855643044619430415, -0.4281496062992127816, -0.4176697321401328100 ) ) ;
#20649=CARTESIAN_POINT ( 'NONE',  ( -0.6692913385826764205, -0.6692913385826771977, 8.415575281601705876E-17 ) ) ;
#20651=CARTESIAN_POINT ( 'NONE',  ( 1.259842519685040019, -0.1870078740157479769, 0.3641732283464567677 ) ) ;
#20652=CARTESIAN_POINT ( 'NONE',  ( 0.3149606299212606708, -0.1870078740157480879, -0.4822834645669291653 ) ) ;
#20653=CARTESIAN_POINT ( 'NONE',  ( 0.01968503937007957949, -0.5400638737290845981, -0.3530559997133363437 ) ) ;
#20654=CARTESIAN_POINT ( 'NONE',  ( -0.05905511811023545637, 0.07958543189024085140, 0.2665933059059887866 ) ) ;
#20655=CARTESIAN_POINT ( 'NONE',  ( 1.114781747626347963, 3.405574981839577511E-16, 0.3464511005275203726 ) ) ;
#20656=CARTESIAN_POINT ( 'NONE',  ( -0.1640419947506553400, -0.08942795157528024563, -0.3641732283464568787 ) ) ;
#20657=CARTESIAN_POINT ( 'NONE',  ( 0.6430446194225729606, -0.4281496062992127816, -0.4176697321401328100 ) ) ;
#20658=CARTESIAN_POINT ( 'NONE',  ( -0.9514435695538050464, -0.2845877964562159024, 0.3641732283464567677 ) ) ;
#20659=CARTESIAN_POINT ( 'NONE',  ( -0.8792650918635160906, -0.4281496062992124485, 0.4176697321401328655 ) ) ;
#20660=CARTESIAN_POINT ( 'NONE',  ( 0.1698998578625684763, 0.000000000000000000, 0.3464511005275205946 ) ) ;
#20661=ORIENTED_EDGE ( 'NONE', *, *, #13568, .T. ) ;
#20662=CARTESIAN_POINT ( 'NONE',  ( -1.207349081364828436, -0.6046776061558807314, 0.2411417322834647770 ) ) ;
#20664=CARTESIAN_POINT ( 'NONE',  ( -1.318897637795274802, -0.4536011799217368745, -0.2665933059059886201 ) ) ;
#20665=CARTESIAN_POINT ( 'NONE',  ( 0.03280839895013198948, 0.2952755905511811885, 0.1292274648535926551 ) ) ;
#20666=CARTESIAN_POINT ( 'NONE',  ( -1.587926509186350810, -0.4281496062992124485, 0.4176697321401328655 ) ) ;
#20667=CARTESIAN_POINT ( 'NONE',  ( -0.6167979002624665030, -0.4281496062992127816, -0.4176697321401328100 ) ) ;
#20669=CARTESIAN_POINT ( 'NONE',  ( 1.692913385826772421, 0.2952755905511811885, 0.000000000000000000 ) ) ;
#20670=CARTESIAN_POINT ( 'NONE',  ( 0.9383202099737536495, -0.3162353388693405765, 0.4822834645669290543 ) ) ;
#20671=CARTESIAN_POINT ( 'NONE',  ( 0.8398950131233602345, -0.6046776061558807314, 0.2411417322834647770 ) ) ;
#20673=CARTESIAN_POINT ( 'NONE',  ( -1.614173228346457378, 1.330640075373402897, 0.1372047244094476981 ) ) ;
#20674=CARTESIAN_POINT ( 'NONE',  ( -1.502624671916009680, -0.05778040916215560624, -0.4822834645669293319 ) ) ;
#20676=VERTEX_POINT ( 'NONE', #10470 ) ;
#20677=CARTESIAN_POINT ( 'NONE',  ( -0.3805774278215216522, -0.004921259842519576551, 0.3153832671262227771 ) ) ;
#20681=CARTESIAN_POINT ( 'NONE',  ( 0.4002624671916016896, -0.3162353388693409650, -0.4822834645669289433 ) ) ;
#20682=CARTESIAN_POINT ( 'NONE',  ( -0.03280839895013062252, -0.6692913385826771977, 0.1292274648535927661 ) ) ;
#20683=CARTESIAN_POINT ( 'NONE',  ( -0.5971128608923877978, -0.6692913385826773087, -0.1292274648535924053 ) ) ;
#20684=CARTESIAN_POINT ( 'NONE',  ( 1.305774278215223960, -0.6692913385826771977, 0.1292274648535927661 ) ) ;
#20685=CARTESIAN_POINT ( 'NONE',  ( -0.7480314960629914633, -0.5511811023622047445, 6.969142054262312111E-17 ) ) ;
#20686=CARTESIAN_POINT ( 'NONE',  ( 0.5643044619422579178, 0.05413385826771666132, 0.4176697321401328100 ) ) ;
#20688=CARTESIAN_POINT ( 'NONE',  ( 0.5774278215223103139, -0.5023911411419708095, -0.1820866141732282451 ) ) ;
#20689=CARTESIAN_POINT ( 'NONE',  ( -0.5118110236220466680, 0.2952755905511811885, 0.000000000000000000 ) ) ;
#20691=CARTESIAN_POINT ( 'NONE',  ( -0.7808398950131222316, -0.3162353388693409650, -0.4822834645669289433 ) ) ;
#20693=CARTESIAN_POINT ( 'NONE',  ( 1.515748031496063408, 0.1660481256975885056, 0.3530559997133364547 ) ) ;
#20694=CARTESIAN_POINT ( 'NONE',  ( 1.541994750656168645, 0.1771653543307087075, -0.09757992244046823083 ) ) ;
#20697=CARTESIAN_POINT ( 'NONE',  ( 0.01312335958005323398, -0.4281496062992127816, -0.4176697321401328100 ) ) ;
#20700=CARTESIAN_POINT ( 'NONE',  ( -1.338582677165353729, -0.1870078740157480879, -0.4822834645669291653 ) ) ;
#20701=CARTESIAN_POINT ( 'NONE',  ( 1.240157480314961314, -0.5400638737290844871, 0.3530559997133364547 ) ) ;
#20702=CARTESIAN_POINT ( 'NONE',  ( 1.135170603674541256, 0.2952755905511811885, 0.1292274648535926551 ) ) ;
#20703=CARTESIAN_POINT ( 'NONE',  ( 0.2559055118110243332, -0.5400638737290845981, -0.3530559997133363437 ) ) ;
#20704=CARTESIAN_POINT ( 'NONE',  ( -0.4002624671916004129, -0.3162353388693405765, 0.4822834645669290543 ) ) ;
#20706=CARTESIAN_POINT ( 'NONE',  ( -1.194225721784776262, 0.05413385826771626580, -0.4176697321401330321 ) ) ;
#20707=CARTESIAN_POINT ( 'NONE',  ( -0.7545931758530176614, -0.6692913385826773087, -0.1292274648535924053 ) ) ;
#20708=CARTESIAN_POINT ( 'NONE',  ( -0.1115485564304453947, -0.5511811023622046335, 0.09757992244046803654 ) ) ;
#20709=CARTESIAN_POINT ( 'NONE',  ( 1.541994750656168645, 0.2952755905511810774, -0.1292274648535930714 ) ) ;
#20710=CARTESIAN_POINT ( 'NONE',  ( -0.5052493438320203589, -0.6692913385826771977, 0.1292274648535927661 ) ) ;
#20711=CARTESIAN_POINT ( 'NONE',  ( 0.3018372703412079971, 0.009842519685039147898, -0.3409548833797004797 ) ) ;
#20712=B_SPLINE_CURVE_WITH_KNOTS ( 'NONE', 3,
 ( #26859, #1209, #52518, #8757 ),
 .UNSPECIFIED., .F., .F.,
 ( 4, 4 ),
 ( 3.210432057665806998E-07, 0.001287787053612119391 ),
 .UNSPECIFIED. ) ;
#20713=CARTESIAN_POINT ( 'NONE',  ( 0.6233595800524939223, -0.3162353388693405765, 0.4822834645669290543 ) ) ;
#20716=CARTESIAN_POINT ( 'NONE',  ( 0.03280839895013198948, -0.6692913385826773087, -0.1292274648535924053 ) ) ;
#20717=CARTESIAN_POINT ( 'NONE',  ( -0.2755905511811018171, 0.1771653543307087630, 0.000000000000000000 ) ) ;
#20718=CARTESIAN_POINT ( 'NONE',  ( 0.9120734908136490793, 0.1771653543307087075, -0.09757992244046823083 ) ) ;
#20719=CARTESIAN_POINT ( 'NONE',  ( -1.614173228346457378, 0.7794589730111968207, -0.1372047244094477536 ) ) ;
#20721=CARTESIAN_POINT ( 'NONE',  ( 1.509186351706037543, -0.004921259842519576551, 0.3153832671262227771 ) ) ;
#20722=CARTESIAN_POINT ( 'NONE',  ( 1.345144356955381593, -0.3162353388693409650, -0.4822834645669289433 ) ) ;
#20724=CARTESIAN_POINT ( 'NONE',  ( -0.03280839895013062252, -0.6692913385826771977, 0.1292274648535927661 ) ) ;
#20725=CARTESIAN_POINT ( 'NONE',  ( -1.469816272965878357, 0.2306618581243848609, 0.2411417322834645549 ) ) ;
#20727=CARTESIAN_POINT ( 'NONE',  ( -1.568241469816272105, -0.05778040916215522460, 0.4822834645669289988 ) ) ;
#20728=CARTESIAN_POINT ( 'NONE',  ( -0.1574803149606292529, -0.1870078740157479769, 0.4822834645669291653 ) ) ;
#20730=CARTESIAN_POINT ( 'NONE',  ( -1.620734908136482577, 0.1771653543307087630, 0.09757992244046791164 ) ) ;
#20731=CARTESIAN_POINT ( 'NONE',  ( 0.4658792650918640033, -0.3162353388693405765, 0.4822834645669290543 ) ) ;
#20732=CARTESIAN_POINT ( 'NONE',  ( 0.9055118110236227702, 0.1771653543307087630, 0.000000000000000000 ) ) ;
#20734=CARTESIAN_POINT ( 'NONE',  ( 0.3805774278215230400, -0.3690944881889763329, 0.3153832671262228327 ) ) ;
#20735=CARTESIAN_POINT ( 'NONE',  ( -1.377952755905511140, -0.6692913385826771977, 8.415575281601705876E-17 ) ) ;
#20737=CARTESIAN_POINT ( 'NONE',  ( 1.292650918635171564, -0.6692913385826773087, -0.1292274648535924053 ) ) ;
#20739=CARTESIAN_POINT ( 'NONE',  ( 0.2296587926509192634, -0.3162353388693405765, 0.4822834645669290543 ) ) ;
#20741=PLANE ( 'NONE',  #18694 ) ;
#20742=CARTESIAN_POINT ( 'NONE',  ( 0.4396325459317590445, -0.5511811023622046335, 0.09757992244046803654 ) ) ;
#20744=CARTESIAN_POINT ( 'NONE',  ( 0.4724409448818904789, -0.1870078740157480879, -0.4822834645669291653 ) ) ;
#20746=CARTESIAN_POINT ( 'NONE',  ( -0.9186351706036736120, 0.1283753931104748280, 0.1820866141732283561 ) ) ;
#20747=CARTESIAN_POINT ( 'NONE',  ( -1.227034120734907585, 0.2952755905511811885, 0.1292274648535926551 ) ) ;
#20748=CARTESIAN_POINT ( 'NONE',  ( -1.646981627296586703, -0.3162353388693409650, -0.4822834645669289433 ) ) ;
#20749=CARTESIAN_POINT ( 'NONE',  ( 1.049868766404200349, 0.2306618581243848609, 0.2411417322834645549 ) ) ;
#20750=CARTESIAN_POINT ( 'NONE',  ( 1.666666666666667185, 0.05413385826771666132, 0.4176697321401328100 ) ) ;
#20752=CARTESIAN_POINT ( 'NONE',  ( 0.4855643044619428750, 0.05413385826771666132, 0.4176697321401328100 ) ) ;
#20754=CARTESIAN_POINT ( 'NONE',  ( 1.627296587926509996, -0.6046776061558807314, 0.2411417322834647770 ) ) ;
#20755=CARTESIAN_POINT ( 'NONE',  ( 1.561679790026247350, 0.05413385826771626580, -0.4176697321401330321 ) ) ;
#20756=CARTESIAN_POINT ( 'NONE',  ( -1.568241469816272105, -0.08942795157527998196, 0.3641732283464567121 ) ) ;
#20757=CARTESIAN_POINT ( 'NONE',  ( 1.076115485564305141, 0.1283753931104746893, -0.1820866141732285504 ) ) ;
#20758=CARTESIAN_POINT ( 'NONE',  ( -1.148293963254592542, 0.1771653543307087630, 0.09757992244046791164 ) ) ;
#20759=CARTESIAN_POINT ( 'NONE',  ( -0.2493438320209966919, -0.3690944881889763329, 0.3153832671262228327 ) ) ;
#20761=CARTESIAN_POINT ( 'NONE',  ( 0.4790026246719167324, -0.08942795157527998196, 0.3641732283464567121 ) ) ;
#20762=CARTESIAN_POINT ( 'NONE',  ( 0.5511811023622055217, -0.1870078740157479769, 0.4822834645669291653 ) ) ;
#20763=CARTESIAN_POINT ( 'NONE',  ( 1.056430446194226436, -0.6692913385826773087, -0.1292274648535924053 ) ) ;
#20764=CARTESIAN_POINT ( 'NONE',  ( 0.07217847769028949700, -0.3162353388693405765, 0.4822834645669290543 ) ) ;
#20765=CARTESIAN_POINT ( 'NONE',  ( -0.03280839895013062252, -0.5511811023622046335, 0.09757992244046803654 ) ) ;
#20766=CARTESIAN_POINT ( 'NONE',  ( 1.135170603674541256, 0.2952755905511811885, 0.1292274648535926551 ) ) ;
#20767=CARTESIAN_POINT ( 'NONE',  ( -0.9448818897637790704, -0.1870078740157479769, 0.4822834645669291653 ) ) ;
#20770=CARTESIAN_POINT ( 'NONE',  ( 0.03937007874015806264, 0.2952755905511811885, 0.000000000000000000 ) ) ;
#20771=CARTESIAN_POINT ( 'NONE',  ( -0.6102362204724400829, -0.5400638737290845981, -0.3530559997133363437 ) ) ;
#20772=CARTESIAN_POINT ( 'NONE',  ( -0.07874015748031421014, -0.1870078740157480879, -0.4822834645669291653 ) ) ;
#20777=CARTESIAN_POINT ( 'NONE',  ( -0.9645669291338575535, -0.4536011799217367080, 0.2665933059059888421 ) ) ;
#20779=CARTESIAN_POINT ( 'NONE',  ( -1.679790026246718693, 0.2306618581243847221, -0.2411417322834647770 ) ) ;
#20781=CARTESIAN_POINT ( 'NONE',  ( 0.2887139107611556010, 0.2306618581243847221, -0.2411417322834647770 ) ) ;
#20782=CARTESIAN_POINT ( 'NONE',  ( -0.6889763779527552368, -0.4536011799217368745, -0.2665933059059886201 ) ) ;
#20783=CARTESIAN_POINT ( 'NONE',  ( 1.056430446194226436, -0.6692913385826773087, -0.1292274648535924053 ) ) ;
#20784=CARTESIAN_POINT ( 'NONE',  ( 0.4790026246719167324, -0.05778040916215522460, 0.4822834645669289988 ) ) ;
#20788=CARTESIAN_POINT ( 'NONE',  ( 1.358267716535433323, 0.1660481256975885056, 0.3530559997133364547 ) ) ;
#20789=CARTESIAN_POINT ( 'NONE',  ( 0.5708661417322841158, -0.5400638737290845981, -0.3530559997133363437 ) ) ;
#20790=CARTESIAN_POINT ( 'NONE',  ( 0.2296587926509192634, -0.05778040916215560624, -0.4822834645669293319 ) ) ;
#20791=CARTESIAN_POINT ( 'NONE',  ( 1.469816272965879911, 0.2306618581243847221, -0.2411417322834647770 ) ) ;
#20792=CARTESIAN_POINT ( 'NONE',  ( 0.7283464566929143125, 0.1660481256975885056, 0.3530559997133364547 ) ) ;
#20794=CARTESIAN_POINT ( 'NONE',  ( 0.1443569553805781891, -0.4281496062992124485, 0.4176697321401328655 ) ) ;
#20795=CARTESIAN_POINT ( 'NONE',  ( 1.003937007874016407, -0.5400638737290844871, 0.3530559997133364547 ) ) ;
#20796=CARTESIAN_POINT ( 'NONE',  ( 0.5774278215223104249, 0.2306618581243848609, 0.2411417322834645549 ) ) ;
#20797=CARTESIAN_POINT ( 'NONE',  ( 1.305774278215223960, -0.5511811023622046335, 0.09757992244046803654 ) ) ;
#20798=CARTESIAN_POINT ( 'NONE',  ( -1.423884514435694859, -0.3162353388693405765, 0.4822834645669290543 ) ) ;
#20799=CARTESIAN_POINT ( 'NONE',  ( -1.555118110236219930, 0.1660481256975885056, 0.3530559997133364547 ) ) ;
#20800=CARTESIAN_POINT ( 'NONE',  ( 0.8530183727034126306, 0.05413385826771626580, -0.4176697321401330321 ) ) ;
#20801=CARTESIAN_POINT ( 'NONE',  ( -0.7270051398050848546, 2.375327444609086402, -0.4916655823645590950 ) ) ;
#20803=VERTEX_POINT ( 'NONE', #18430 ) ;
#20805=ORIENTED_EDGE ( 'NONE', *, *, #24322, .T. ) ;
#20806=CARTESIAN_POINT ( 'NONE',  ( 1.095800524934383846, -0.05778040916215560624, -0.4822834645669293319 ) ) ;
#20807=CARTESIAN_POINT ( 'NONE',  ( 1.102362204724410155, -0.1870078740157479769, 0.3641732283464567677 ) ) ;
#20808=CARTESIAN_POINT ( 'NONE',  ( 1.586052503253845281, 0.4724409448818907564, -0.1653254495020589354 ) ) ;
#20813=CARTESIAN_POINT ( 'NONE',  ( 1.272965879265092637, 0.05413385826771666132, 0.4176697321401328100 ) ) ;
#20814=CARTESIAN_POINT ( 'NONE',  ( -1.509186351706035767, -0.4281496062992124485, 0.4176697321401328655 ) ) ;
#20815=CARTESIAN_POINT ( 'NONE',  ( -0.3937007874015740483, -0.1870078740157480879, -0.4822834645669291653 ) ) ;
#20816=CARTESIAN_POINT ( 'NONE',  ( 1.128608923884514947, 0.2306618581243848609, 0.2411417322834645549 ) ) ;
#20818=CARTESIAN_POINT ( 'NONE',  ( -1.699475065616797398, 0.2952755905511811885, 0.1292274648535926551 ) ) ;
#20821=CARTESIAN_POINT ( 'NONE',  ( 1.509186351706037543, -0.004921259842519576551, 0.3153832671262227771 ) ) ;
#20823=CARTESIAN_POINT ( 'NONE',  ( -0.8267716535433065062, 0.1771653543307087630, 0.000000000000000000 ) ) ;
#20824=CARTESIAN_POINT ( 'NONE',  ( -1.423884514435694859, -0.05778040916215560624, -0.4822834645669293319 ) ) ;
#20825=CARTESIAN_POINT ( 'NONE',  ( 0.6430446194225729606, -0.4281496062992127816, -0.4176697321401328100 ) ) ;
#20830=CARTESIAN_POINT ( 'NONE',  ( 0.8530183727034128527, -0.4281496062992124485, 0.4176697321401328655 ) ) ;
#20831=CARTESIAN_POINT ( 'NONE',  ( -1.633858267716534529, -0.5400638737290845981, -0.3530559997133363437 ) ) ;
#20833=CARTESIAN_POINT ( 'NONE',  ( -0.6036745406824141069, 0.1283753931104748280, 0.1820866141732283561 ) ) ;
#20834=CARTESIAN_POINT ( 'NONE',  ( -1.535433070866141225, -0.5511811023622047445, 6.969142054262312111E-17 ) ) ;
#20836=CARTESIAN_POINT ( 'NONE',  ( 0.4265091863517067039, -0.6692913385826773087, -0.1292274648535924053 ) ) ;
#20838=CARTESIAN_POINT ( 'NONE',  ( -0.8136482939632537770, 0.1283753931104746893, -0.1820866141732285504 ) ) ;
#20839=CARTESIAN_POINT ( 'NONE',  ( 0.2296587926509192634, -0.08942795157528024563, -0.3641732283464568787 ) ) ;
#20840=CARTESIAN_POINT ( 'NONE',  ( -0.4330708661417315697, 0.2952755905511811885, 0.000000000000000000 ) ) ;
#20841=CARTESIAN_POINT ( 'NONE',  ( -1.003937007874014853, 0.07958543189024085140, 0.2665933059059887866 ) ) ;
#20843=CARTESIAN_POINT ( 'NONE',  ( 0.8070866141732288002, 0.1660481256975885056, 0.3530559997133364547 ) ) ;
#20846=CARTESIAN_POINT ( 'NONE',  ( -0.9448818897637790704, -0.1870078740157479769, 0.4822834645669291653 ) ) ;
#20847=CARTESIAN_POINT ( 'NONE',  ( -0.3215223097112853146, -0.2845877964562159024, 0.3641732283464567677 ) ) ;
#20848=CARTESIAN_POINT ( 'NONE',  ( -1.443569553805773564, 0.2306618581243847221, -0.2411417322834647770 ) ) ;
#20849=CARTESIAN_POINT ( 'NONE',  ( 0.7283464566929143125, 0.07958543189024085140, 0.2665933059059887866 ) ) ;
#20851=CARTESIAN_POINT ( 'NONE',  ( -0.7414698162729651543, 0.1771653543307087075, -0.09757992244046823083 ) ) ;
#20852=CARTESIAN_POINT ( 'NONE',  ( -0.8989501312335946848, 0.2952755905511810774, -0.1292274648535930714 ) ) ;
#20853=CARTESIAN_POINT ( 'NONE',  ( -1.076115485564303809, 0.2306618581243848609, 0.2411417322834645549 ) ) ;
#20854=CARTESIAN_POINT ( 'NONE',  ( 1.633858267716535639, -0.5400638737290844871, 0.3530559997133364547 ) ) ;
#20856=CARTESIAN_POINT ( 'NONE',  ( 0.7742782152230979209, -0.004921259842519870586, -0.3153832671262229437 ) ) ;
#20857=CARTESIAN_POINT ( 'NONE',  ( 0.5249343832021005074, -0.6046776061558807314, 0.2411417322834647770 ) ) ;
#20858=CARTESIAN_POINT ( 'NONE',  ( -1.607611548556429737, 0.2952755905511810774, -0.1292274648535930714 ) ) ;
#20859=CARTESIAN_POINT ( 'NONE',  ( -1.404199475065615932, 0.05413385826771666132, 0.4176697321401328100 ) ) ;
#20862=EDGE_CURVE ( 'NONE', #38184, #24792, #42396, .T. ) ;
#20864=CARTESIAN_POINT ( 'NONE',  ( -1.187664041994749731, -0.2845877964562159024, 0.3641732283464567677 ) ) ;
#20865=CARTESIAN_POINT ( 'NONE',  ( -0.5183727034120726440, 0.2952755905511811885, 0.1292274648535926551 ) ) ;
#20866=CARTESIAN_POINT ( 'NONE',  ( 0.8661417322834652488, -0.1870078740157480879, -0.4822834645669291653 ) ) ;
#20867=CARTESIAN_POINT ( 'NONE',  ( -1.364829396325458521, 0.1283753931104746893, -0.1820866141732285504 ) ) ;
#20869=CARTESIAN_POINT ( 'NONE',  ( -1.259842519685038686, -0.1870078740157479769, 0.4822834645669291653 ) ) ;
#20870=CARTESIAN_POINT ( 'NONE',  ( 0.4921259842519691285, -0.5400638737290845981, -0.3530559997133363437 ) ) ;
#20871=CARTESIAN_POINT ( 'NONE',  ( 0.3477690288713918276, -0.6692913385826773087, -0.1292274648535924053 ) ) ;
#20872=CARTESIAN_POINT ( 'NONE',  ( 1.167979002624672580, 0.05413385826771626580, -0.4176697321401330321 ) ) ;
#20873=CARTESIAN_POINT ( 'NONE',  ( 1.092343761084413556, 1.535433070866141447, -0.6033564923654646250 ) ) ;
#20878=CARTESIAN_POINT ( 'NONE',  ( 0.2296587926509192634, -0.08942795157528024563, -0.3641732283464568787 ) ) ;
#20879=CARTESIAN_POINT ( 'NONE',  ( 0.2362204724409456558, -0.1870078740157480879, -0.4822834645669291653 ) ) ;
#20880=CARTESIAN_POINT ( 'NONE',  ( 1.469816272965879911, 0.2306618581243847221, -0.2411417322834647770 ) ) ;
#20882=CARTESIAN_POINT ( 'NONE',  ( 0.3412073490813655186, -0.5023911411419708095, -0.1820866141732282451 ) ) ;
#20883=ADVANCED_FACE ( 'NONE', ( #34585 ), #57493, .F. ) ;
#20884=CARTESIAN_POINT ( 'NONE',  ( -0.6102362204724400829, -0.5400638737290845981, -0.3530559997133363437 ) ) ;
#20885=CARTESIAN_POINT ( 'NONE',  ( -1.620734908136482577, 0.2952755905511811885, 0.1292274648535926551 ) ) ;
#20886=CARTESIAN_POINT ( 'NONE',  ( 0.3937007874015754361, -0.1870078740157479769, 0.4822834645669291653 ) ) ;
#20889=ORIENTED_EDGE ( 'NONE', *, *, #69043, .F. ) ;
#20890=ORIENTED_EDGE ( 'NONE', *, *, #1215, .T. ) ;
#20891=CARTESIAN_POINT ( 'NONE',  ( 1.489501312335958172, -0.08942795157528024563, -0.3641732283464568787 ) ) ;
#20892=CARTESIAN_POINT ( 'NONE',  ( -1.174540682414697335, -0.08942795157527998196, 0.3641732283464567121 ) ) ;
#20893=CARTESIAN_POINT ( 'NONE',  ( -1.305774278215222184, 0.2952755905511811885, 0.1292274648535926551 ) ) ;
#20896=CARTESIAN_POINT ( 'NONE',  ( 1.594488188976378673, -0.5400638737290845981, -0.3530559997133363437 ) ) ;
#20897=CARTESIAN_POINT ( 'NONE',  ( -1.351706036745406347, 0.05413385826771626580, -0.4176697321401330321 ) ) ;
#20898=CARTESIAN_POINT ( 'NONE',  ( 0.4724409448818904789, -0.1870078740157479769, 0.4822834645669291653 ) ) ;
#20899=CARTESIAN_POINT ( 'NONE',  ( -1.332020997375327642, -0.05778040916215522460, 0.4822834645669289988 ) ) ;
#20901=CARTESIAN_POINT ( 'NONE',  ( 0.7217847769028878924, -0.4281496062992127816, -0.4176697321401328100 ) ) ;
#20903=CARTESIAN_POINT ( 'NONE',  ( -1.089238845144356427, -0.3690944881889765550, -0.3153832671262227771 ) ) ;
#20904=ORIENTED_EDGE ( 'NONE', *, *, #22304, .T. ) ;
#20907=CARTESIAN_POINT ( 'NONE',  ( -1.692913385826770645, 0.1771653543307087630, 0.000000000000000000 ) ) ;
#20908=CARTESIAN_POINT ( 'NONE',  ( -1.200787401574802349, 0.1660481256975883668, -0.3530559997133364547 ) ) ;
#20909=CARTESIAN_POINT ( 'NONE',  ( -1.397637795275589623, -0.5400638737290845981, -0.3530559997133363437 ) ) ;
#20911=CARTESIAN_POINT ( 'NONE',  ( -1.719160104986876103, 0.05413385826771666132, 0.4176697321401328100 ) ) ;
#20912=CARTESIAN_POINT ( 'NONE',  ( -1.633858267716534529, -0.5400638737290845981, -0.3530559997133363437 ) ) ;
#20913=CARTESIAN_POINT ( 'NONE',  ( -1.338582677165353729, -0.1870078740157479769, 0.4822834645669291653 ) ) ;
#20914=CARTESIAN_POINT ( 'NONE',  ( -0.3830016109920609813, -4.992347309556208597E-15, 0.4118484887281982920 ) ) ;
#20915=CARTESIAN_POINT ( 'NONE',  ( 0.2362204724409456558, -0.1870078740157479769, 0.3641732283464567677 ) ) ;
#20918=CARTESIAN_POINT ( 'NONE',  ( -0.9842519685039365918, -0.5511811023622047445, 6.969142054262312111E-17 ) ) ;
#20919=CARTESIAN_POINT ( 'NONE',  ( -0.8923884514435688198, -0.6046776061558807314, 0.2411417322834647770 ) ) ;
#20920=CARTESIAN_POINT ( 'NONE',  ( 0.7808398950131240079, -0.3162353388693405765, 0.4822834645669290543 ) ) ;
#20921=CARTESIAN_POINT ( 'NONE',  ( -0.7480314960629914633, -0.6692913385826771977, 8.415575281601705876E-17 ) ) ;
#20922=ORIENTED_EDGE ( 'NONE', *, *, #2281, .T. ) ;
#20923=VERTEX_POINT ( 'NONE', #48667 ) ;
#20924=CARTESIAN_POINT ( 'NONE',  ( -1.148293963254592542, 0.2952755905511811885, 0.1292274648535926551 ) ) ;
#20925=CARTESIAN_POINT ( 'NONE',  ( 0.6824146981627303710, 0.2306618581243847221, -0.2411417322834647770 ) ) ;
#20926=CARTESIAN_POINT ( 'NONE',  ( -1.594488188976377563, -0.4536011799217367080, 0.2665933059059888421 ) ) ;
#20931=CARTESIAN_POINT ( 'NONE',  ( -0.4724409448818890911, -0.1870078740157480879, -0.4822834645669291653 ) ) ;
#20932=CARTESIAN_POINT ( 'NONE',  ( -1.568241469816272105, -0.2845877964562161244, -0.3641732283464567121 ) ) ;
#20934=CARTESIAN_POINT ( 'NONE',  ( -1.502624671916009680, -0.05778040916215560624, -0.4822834645669293319 ) ) ;
#20935=LINE ( 'NONE', #33562, #61310 ) ;
#20937=CARTESIAN_POINT ( 'NONE',  ( -1.305774278215222184, -0.6692913385826773087, -0.1292274648535924053 ) ) ;
#20938=CARTESIAN_POINT ( 'NONE',  ( -0.4527559055118102749, 0.1660481256975885056, 0.3530559997133364547 ) ) ;
#20940=CARTESIAN_POINT ( 'NONE',  ( 0.6364829396325465405, -0.08942795157527998196, 0.3641732283464567121 ) ) ;
#20942=CARTESIAN_POINT ( 'NONE',  ( 0.5380577427821529035, -0.3690944881889763329, 0.3153832671262228327 ) ) ;
#20943=CARTESIAN_POINT ( 'NONE',  ( 1.358267716535433323, -0.4536011799217368745, -0.2665933059059886201 ) ) ;
#20944=CARTESIAN_POINT ( 'NONE',  ( 0.8070866141732288002, 0.1660481256975885056, 0.3530559997133364547 ) ) ;
#20946=CARTESIAN_POINT ( 'NONE',  ( 0.2755905511811031494, 0.1771653543307087630, 0.000000000000000000 ) ) ;
#20948=CARTESIAN_POINT ( 'NONE',  ( -1.181102362204723644, -0.1870078740157479769, 0.4822834645669291653 ) ) ;
#20949=CARTESIAN_POINT ( 'NONE',  ( -0.04593175853018302557, -0.5511811023622048555, -0.09757992244046775898 ) ) ;
#20951=VECTOR ( 'NONE', #14667, 39.37007874015748143 ) ;
#20952=CARTESIAN_POINT ( 'NONE',  ( -0.7086614173228339419, -0.1870078740157479769, 0.3641732283464567677 ) ) ;
#20953=DIRECTION ( 'NONE',  ( -1.000000000000000000, -3.469446951953613696E-16, 0.000000000000000000 ) ) ;
#20954=CARTESIAN_POINT ( 'NONE',  ( -0.01312335958005186876, 0.05413385826771626580, -0.4176697321401330321 ) ) ;
#20955=CARTESIAN_POINT ( 'NONE',  ( -1.586052503253845503, 2.125984251968505045, -0.1653254495020588799 ) ) ;
#20956=CARTESIAN_POINT ( 'NONE',  ( 0.6496062992125991586, 0.07958543189024085140, 0.2665933059059887866 ) ) ;
#20957=CARTESIAN_POINT ( 'NONE',  ( -0.3608923884514428360, -0.5511811023622048555, -0.09757992244046775898 ) ) ;
#20958=CARTESIAN_POINT ( 'NONE',  ( -0.2099737532808391705, 0.2306618581243848609, 0.2411417322834645549 ) ) ;
#20960=CARTESIAN_POINT ( 'NONE',  ( -0.9514435695538050464, -0.08942795157528024563, -0.3641732283464568787 ) ) ;
#20961=CARTESIAN_POINT ( 'NONE',  ( 0.6758530183727039509, -0.6692913385826771977, 0.1292274648535927661 ) ) ;
#20962=CARTESIAN_POINT ( 'NONE',  ( -0.7349081364829387342, -0.6046776061558807314, 0.2411417322834647770 ) ) ;
#20965=CARTESIAN_POINT ( 'NONE',  ( 0.3280839895013130669, -0.004921259842519576551, 0.3153832671262227771 ) ) ;
#20966=CARTESIAN_POINT ( 'NONE',  ( -1.325459317585300889, 0.05413385826771666132, 0.4176697321401328100 ) ) ;
#20967=CARTESIAN_POINT ( 'NONE',  ( -1.187664041994749731, -0.2845877964562159024, 0.3641732283464567677 ) ) ;
#20968=CARTESIAN_POINT ( 'NONE',  ( 1.627296587926509996, -0.6046776061558807314, 0.2411417322834647770 ) ) ;
#20969=CARTESIAN_POINT ( 'NONE',  ( -0.7677165354330699465, -0.4536011799217368745, -0.2665933059059886201 ) ) ;
#20970=CARTESIAN_POINT ( 'NONE',  ( -0.7349081364829390672, 0.1539470093639521697, -0.1968503937007875793 ) ) ;
#20971=CARTESIAN_POINT ( 'NONE',  ( 0.9908136482939640111, 0.2952755905511810774, -0.1292274648535930714 ) ) ;
#20975=CARTESIAN_POINT ( 'NONE',  ( 1.555118110236221041, -0.4536011799217367080, 0.2665933059059888421 ) ) ;
#20976=CARTESIAN_POINT ( 'NONE',  ( -1.489501312335957062, -0.3162353388693409650, -0.4822834645669289433 ) ) ;
#20977=CARTESIAN_POINT ( 'NONE',  ( 1.450131233595801428, 0.2952755905511811885, 0.1292274648535926551 ) ) ;
#20980=CARTESIAN_POINT ( 'NONE',  ( 0.3477690288713918276, -0.6692913385826773087, -0.1292274648535924053 ) ) ;
#20981=CARTESIAN_POINT ( 'NONE',  ( -0.4527559055118102749, -0.5400638737290845981, -0.3530559997133363437 ) ) ;
#20982=CARTESIAN_POINT ( 'NONE',  ( 1.548556430446194954, 0.2306618581243847221, -0.2411417322834647770 ) ) ;
#20984=CARTESIAN_POINT ( 'NONE',  ( 0.5708661417322841158, -0.4536011799217368745, -0.2665933059059886201 ) ) ;
#20986=ORIENTED_EDGE ( 'NONE', *, *, #58958, .T. ) ;
#20990=CARTESIAN_POINT ( 'NONE',  ( 0.02624671916010564918, 0.2306618581243848609, 0.2411417322834645549 ) ) ;
#20991=CARTESIAN_POINT ( 'NONE',  ( 1.213910761154856299, -0.6692913385826773087, -0.1292274648535924053 ) ) ;
#20992=CARTESIAN_POINT ( 'NONE',  ( 0.1706036745406830368, -0.4281496062992127816, -0.4176697321401328100 ) ) ;
#20993=CARTESIAN_POINT ( 'NONE',  ( -0.3018372703412066094, -0.3690944881889765550, -0.3153832671262227771 ) ) ;
#20994=CARTESIAN_POINT ( 'NONE',  ( 1.062992125984252745, 0.2952755905511811885, 0.000000000000000000 ) ) ;
#20995=CARTESIAN_POINT ( 'NONE',  ( -0.6102362204724400829, -0.5400638737290845981, -0.3530559997133363437 ) ) ;
#20996=CARTESIAN_POINT ( 'NONE',  ( 0.1706036745406830368, 0.05413385826771666132, 0.4176697321401328100 ) ) ;
#20997=CARTESIAN_POINT ( 'NONE',  ( 1.587926509186352142, 0.05413385826771666132, 0.4176697321401328100 ) ) ;
#20998=CARTESIAN_POINT ( 'NONE',  ( 0.6955380577427828781, 0.05413385826771626580, -0.4176697321401330321 ) ) ;
#20999=CARTESIAN_POINT ( 'NONE',  ( 1.384514435695538559, 0.2952755905511810774, -0.1292274648535930714 ) ) ;
#21001=CARTESIAN_POINT ( 'NONE',  ( 0.07874015748031558404, -0.1870078740157479769, 0.3641732283464567677 ) ) ;
#21005=VERTEX_POINT ( 'NONE', #43994 ) ;
#21006=CARTESIAN_POINT ( 'NONE',  ( -0.4199475065616791736, 0.1283753931104746893, -0.1820866141732285504 ) ) ;
#21008=CARTESIAN_POINT ( 'NONE',  ( 0.09842519685039434474, 0.1660481256975885056, 0.3530559997133364547 ) ) ;
#21010=CARTESIAN_POINT ( 'NONE',  ( -0.2952755905511804668, 0.1660481256975885056, 0.3530559997133364547 ) ) ;
#21011=CARTESIAN_POINT ( 'NONE',  ( -0.3871391076115479057, -0.3162353388693409650, -0.4822834645669289433 ) ) ;
#21012=CARTESIAN_POINT ( 'NONE',  ( -0.8464566929133852113, 0.1660481256975885056, 0.3530559997133364547 ) ) ;
#21013=CARTESIAN_POINT ( 'NONE',  ( -0.9711286089238838626, -0.6046776061558807314, 0.2411417322834647770 ) ) ;
#21014=CARTESIAN_POINT ( 'NONE',  ( 1.266404199475066328, -0.2845877964562161244, -0.3641732283464567121 ) ) ;
#21015=CARTESIAN_POINT ( 'NONE',  ( -0.8478501267249328732, 2.401574803149606474, -0.8478501267249377582 ) ) ;
#21017=CARTESIAN_POINT ( 'NONE',  ( 0.7480314960629927956, -0.5511811023622047445, 6.969142054262312111E-17 ) ) ;
#21018=CARTESIAN_POINT ( 'NONE',  ( 0.4330708661417329575, 0.2952755905511811885, 0.000000000000000000 ) ) ;
#21019=CARTESIAN_POINT ( 'NONE',  ( 0.3149606299212606708, -0.1870078740157480879, -0.4822834645669291653 ) ) ;
#21021=CARTESIAN_POINT ( 'NONE',  ( -2.795275590551181466, 2.125984251968505045, 0.000000000000000000 ) ) ;
#21024=CARTESIAN_POINT ( 'NONE',  ( -0.6102362204724400829, 0.1660481256975885056, 0.3530559997133364547 ) ) ;
#21028=CARTESIAN_POINT ( 'NONE',  ( -1.351706036745406347, -0.3690944881889763329, 0.3153832671262228327 ) ) ;
#21029=CARTESIAN_POINT ( 'NONE',  ( 0.9120734908136489683, -0.6692913385826771977, 0.1292274648535927661 ) ) ;
#21030=CARTESIAN_POINT ( 'NONE',  ( 1.102362204724410155, -0.1870078740157480879, -0.4822834645669291653 ) ) ;
#21031=CARTESIAN_POINT ( 'NONE',  ( -0.3477690288713902178, 0.1771653543307087075, -0.09757992244046823083 ) ) ;
#21032=CARTESIAN_POINT ( 'NONE',  ( 0.2755905511811031494, -0.6692913385826771977, 8.415575281601705876E-17 ) ) ;
#21034=CARTESIAN_POINT ( 'NONE',  ( -0.2821522309711278487, -0.5511811023622048555, -0.09757992244046775898 ) ) ;
#21035=CARTESIAN_POINT ( 'NONE',  ( 0.05249343832021075018, 0.2306618581243847221, -0.2411417322834647770 ) ) ;
#21036=ADVANCED_FACE ( 'NONE', ( #30958 ), #28516, .F. ) ;
#21038=CARTESIAN_POINT ( 'NONE',  ( -1.666666666666665853, 0.05413385826771626580, -0.4176697321401330321 ) ) ;
#21039=CARTESIAN_POINT ( 'NONE',  ( 0.3543307086614179147, 0.1771653543307087630, 0.000000000000000000 ) ) ;
#21040=CARTESIAN_POINT ( 'NONE',  ( 1.404199475065617708, -0.004921259842519870586, -0.3153832671262229437 ) ) ;
#21041=CARTESIAN_POINT ( 'NONE',  ( -0.7545931758530177724, 0.2952755905511811885, 0.1292274648535926551 ) ) ;
#21042=CARTESIAN_POINT ( 'NONE',  ( -0.6167979002624665030, -0.3690944881889765550, -0.3153832671262227771 ) ) ;
#21044=CARTESIAN_POINT ( 'NONE',  ( -0.6167979002624665030, 0.05413385826771666132, 0.4176697321401328100 ) ) ;
#21045=CARTESIAN_POINT ( 'NONE',  ( -0.6824146981627288167, 0.2306618581243848609, 0.2411417322834645549 ) ) ;
#21046=CARTESIAN_POINT ( 'NONE',  ( -0.1181102362204717315, -0.6692913385826771977, 8.415575281601705876E-17 ) ) ;
#21050=CARTESIAN_POINT ( 'NONE',  ( -1.620734908136482577, -0.5511811023622048555, -0.09757992244046775898 ) ) ;
#21051=CARTESIAN_POINT ( 'NONE',  ( 0.9645669291338591078, -0.4536011799217368745, -0.2665933059059886201 ) ) ;
#21052=CARTESIAN_POINT ( 'NONE',  ( 1.430446194225722500, 0.05413385826771666132, 0.4176697321401328100 ) ) ;
#21053=CARTESIAN_POINT ( 'NONE',  ( -1.187664041994750175, -0.08942795157528024563, -0.3641732283464568787 ) ) ;
#21054=CARTESIAN_POINT ( 'NONE',  ( -1.272965879265091305, -0.3690944881889763329, 0.3153832671262228327 ) ) ;
#21055=CARTESIAN_POINT ( 'NONE',  ( -0.5708661417322828946, 0.1660481256975883668, -0.3530559997133364547 ) ) ;
#21056=CARTESIAN_POINT ( 'NONE',  ( -0.02624671916010428221, 0.1283753931104746893, -0.1820866141732285504 ) ) ;
#21058=CARTESIAN_POINT ( 'NONE',  ( 1.246719160104987623, -0.3690944881889763329, 0.3153832671262228327 ) ) ;
#21059=CARTESIAN_POINT ( 'NONE',  ( 0.3543307086614181922, -0.6692913385826771977, 8.415575281601705876E-17 ) ) ;
#21060=CARTESIAN_POINT ( 'NONE',  ( -0.5577427821522301654, -0.05778040916215560624, -0.4822834645669293319 ) ) ;
#21063=CARTESIAN_POINT ( 'NONE',  ( 1.601049868766404982, 0.1283753931104748280, 0.1820866141732283561 ) ) ;
#21065=CARTESIAN_POINT ( 'NONE',  ( 0.3937007874015754361, -0.1870078740157479769, 0.4822834645669291653 ) ) ;
#21067=CARTESIAN_POINT ( 'NONE',  ( 0.07874015748031558404, -0.1870078740157479769, 0.4822834645669291653 ) ) ;
#21068=CARTESIAN_POINT ( 'NONE',  ( 0.02624671916010564918, -0.5023911411419708095, -0.1820866141732282451 ) ) ;
#21069=CARTESIAN_POINT ( 'NONE',  ( 1.220472440944879722, 1.496062992125984037, 0.5309055118110233007 ) ) ;
#21070=CARTESIAN_POINT ( 'NONE',  ( -0.2165354330708654795, 0.07958543189024085140, 0.2665933059059887866 ) ) ;
#21071=CARTESIAN_POINT ( 'NONE',  ( 0.6167979002624679463, 0.05413385826771626580, -0.4176697321401330321 ) ) ;
#21072=CARTESIAN_POINT ( 'NONE',  ( -0.8202099737532801971, -0.5511811023622046335, 0.09757992244046803654 ) ) ;
#21074=CARTESIAN_POINT ( 'NONE',  ( -1.128608923884513837, 0.2306618581243847221, -0.2411417322834647770 ) ) ;
#21077=CARTESIAN_POINT ( 'NONE',  ( -1.128608923884513837, 0.2306618581243847221, -0.2411417322834647770 ) ) ;
#21078=CARTESIAN_POINT ( 'NONE',  ( -1.194225721784776262, -0.004921259842519870586, -0.3153832671262229437 ) ) ;
#21079=CARTESIAN_POINT ( 'NONE',  ( 0.07217847769028949700, -0.05778040916215560624, -0.4822834645669293319 ) ) ;
#21080=CARTESIAN_POINT ( 'NONE',  ( -1.673228346456691717, 0.1660481256975883668, -0.3530559997133364547 ) ) ;
#21081=CARTESIAN_POINT ( 'NONE',  ( -0.9055118110236215490, -0.6692913385826771977, 8.415575281601705876E-17 ) ) ;
#21083=CARTESIAN_POINT ( 'NONE',  ( 0.7414698162729663755, -0.6692913385826773087, -0.1292274648535924053 ) ) ;
#21084=CARTESIAN_POINT ( 'NONE',  ( 0.9580052493438327987, -0.4281496062992127816, -0.4176697321401328100 ) ) ;
#21087=CARTESIAN_POINT ( 'NONE',  ( -1.463254593175852492, -0.6692913385826773087, -0.1292274648535924053 ) ) ;
#21090=CARTESIAN_POINT ( 'NONE',  ( -0.5577427821522301654, -0.2845877964562159024, 0.3641732283464567677 ) ) ;
#21093=CARTESIAN_POINT ( 'NONE',  ( 0.3871391076115492380, -0.05778040916215560624, -0.4822834645669293319 ) ) ;
#21094=CARTESIAN_POINT ( 'NONE',  ( 0.01968503937007930540, 0.1660481256975885056, 0.3530559997133364547 ) ) ;
#21095=CARTESIAN_POINT ( 'NONE',  ( -0.4790026246719152336, -0.05778040916215560624, -0.4822834645669293319 ) ) ;
#21096=CARTESIAN_POINT ( 'NONE',  ( 1.358267716535433323, 0.1660481256975885056, 0.3530559997133364547 ) ) ;
#21097=CARTESIAN_POINT ( 'NONE',  ( -0.9973753280839886548, 0.1283753931104748280, 0.1820866141732283561 ) ) ;
#21099=CARTESIAN_POINT ( 'NONE',  ( 0.5577427821522316087, -0.05778040916215522460, 0.4822834645669289988 ) ) ;
#21100=CARTESIAN_POINT ( 'NONE',  ( 0.6758530183727039509, 0.1771653543307087075, -0.09757992244046823083 ) ) ;
#21101=CARTESIAN_POINT ( 'NONE',  ( -0.3543307086614165824, 0.2952755905511811885, 0.000000000000000000 ) ) ;
#21104=CARTESIAN_POINT ( 'NONE',  ( -0.9711286089238838626, 0.2306618581243847221, -0.2411417322834647770 ) ) ;
#21106=CARTESIAN_POINT ( 'NONE',  ( 1.272965879265092637, -0.4281496062992127816, -0.4176697321401328100 ) ) ;
#21110=CARTESIAN_POINT ( 'NONE',  ( -0.04593175853018302557, 0.2952755905511811885, 0.1292274648535926551 ) ) ;
#21112=CARTESIAN_POINT ( 'NONE',  ( 0.9383202099737536495, -0.2845877964562159024, 0.3641732283464567677 ) ) ;
#21113=CARTESIAN_POINT ( 'NONE',  ( -1.128608923884513837, -0.6046776061558807314, 0.2411417322834647770 ) ) ;
#21114=CARTESIAN_POINT ( 'NONE',  ( 1.128608923884514947, 0.2306618581243848609, 0.2411417322834645549 ) ) ;
#21115=CARTESIAN_POINT ( 'NONE',  ( 1.371391076115485719, -0.6692913385826773087, -0.1292274648535924053 ) ) ;
#21116=CARTESIAN_POINT ( 'NONE',  ( 0.2230971128608929543, 0.05413385826771626580, -0.4176697321401330321 ) ) ;
#21117=CARTESIAN_POINT ( 'NONE',  ( -0.4265091863517051496, -0.6692913385826771977, 0.1292274648535927661 ) ) ;
#21119=CARTESIAN_POINT ( 'NONE',  ( -1.010498687664041384, -0.4281496062992127816, -0.4176697321401328100 ) ) ;
#21120=CARTESIAN_POINT ( 'NONE',  ( -0.5839895013123351797, -0.6692913385826771977, 0.1292274648535927661 ) ) ;
#21121=CARTESIAN_POINT ( 'NONE',  ( -0.6561679790026240244, 0.1283753931104746893, -0.1820866141732285504 ) ) ;
#21123=CARTESIAN_POINT ( 'NONE',  ( -0.7086614173228339419, -0.1870078740157480879, -0.4822834645669291653 ) ) ;
#21124=CARTESIAN_POINT ( 'NONE',  ( 0.2493438320209980519, 0.009842519685039467087, 0.3409548833797002021 ) ) ;
#21126=CARTESIAN_POINT ( 'NONE',  ( 0.5577427821522314977, -0.3162353388693409650, -0.4822834645669289433 ) ) ;
#21128=DIRECTION ( 'NONE',  ( 1.000000000000000000, -0.000000000000000000, -0.000000000000000000 ) ) ;
#21129=EDGE_CURVE ( 'NONE', #24575, #62837, #73089, .T. ) ;
#21131=CARTESIAN_POINT ( 'NONE',  ( -0.1968503937007867743, 0.2952755905511811885, 0.000000000000000000 ) ) ;
#21134=CARTESIAN_POINT ( 'NONE',  ( 0.8464566929133866546, -0.4536011799217367080, 0.2665933059059888421 ) ) ;
#21135=CARTESIAN_POINT ( 'NONE',  ( -0.8785612751854012803, -2.613618158232546091E-15, -0.3464511005275220379 ) ) ;
#21137=CARTESIAN_POINT ( 'NONE',  ( 1.108923884514436686, -0.2845877964562161244, -0.3641732283464567121 ) ) ;
#21138=CARTESIAN_POINT ( 'NONE',  ( 1.305774278215223960, 0.2952755905511810774, -0.1292274648535930714 ) ) ;
#21140=CARTESIAN_POINT ( 'NONE',  ( -0.3871391076115479057, -0.3162353388693409650, -0.4822834645669289433 ) ) ;
#21141=DIRECTION ( 'NONE',  ( 1.000000000000000000, -0.000000000000000000, -0.000000000000000000 ) ) ;
#21142=CARTESIAN_POINT ( 'NONE',  ( -1.627296587926508442, -0.6046776061558809534, -0.2411417322834644161 ) ) ;
#21143=CARTESIAN_POINT ( 'NONE',  ( 0.006561679790026889343, -0.05778040916215522460, 0.4822834645669289988 ) ) ;
#21145=CARTESIAN_POINT ( 'NONE',  ( 1.207349081364829990, 0.2306618581243848609, 0.2411417322834645549 ) ) ;
#21146=CARTESIAN_POINT ( 'NONE',  ( 0.7283464566929140904, -0.5400638737290845981, -0.3530559997133363437 ) ) ;
#21147=CARTESIAN_POINT ( 'NONE',  ( 0.8530183727034128527, -0.3690944881889763329, 0.3153832671262228327 ) ) ;
#21149=CARTESIAN_POINT ( 'NONE',  ( 0.5708661417322842269, 0.07958543189024085140, 0.2665933059059887866 ) ) ;
#21152=CARTESIAN_POINT ( 'NONE',  ( 0.6496062992125991586, -0.5400638737290845981, -0.3530559997133363437 ) ) ;
#21154=CARTESIAN_POINT ( 'NONE',  ( 0.3871391076115493490, -0.3162353388693405765, 0.4822834645669290543 ) ) ;
#21155=CARTESIAN_POINT ( 'NONE',  ( -0.3608923884514428360, 0.2066929133858267931, 0.1054918080437490802 ) ) ;
#21156=CARTESIAN_POINT ( 'NONE',  ( 0.5118110236220478892, 0.1771653543307087630, 0.000000000000000000 ) ) ;
#21157=CARTESIAN_POINT ( 'NONE',  ( 0.4461942257217856311, 0.2306618581243847221, -0.2411417322834647770 ) ) ;
#21159=CARTESIAN_POINT ( 'NONE',  ( -0.7349081364829390672, 0.1283753931104746893, -0.1820866141732285504 ) ) ;
#21160=CARTESIAN_POINT ( 'NONE',  ( -1.010498687664041384, -0.4281496062992127816, -0.4176697321401328100 ) ) ;
#21161=CARTESIAN_POINT ( 'NONE',  ( -1.489501312335957062, -0.3162353388693409650, -0.4822834645669289433 ) ) ;
#21162=CARTESIAN_POINT ( 'NONE',  ( 0.5446194225721792126, -0.3162353388693405765, 0.4822834645669290543 ) ) ;
#21163=CARTESIAN_POINT ( 'NONE',  ( 1.620734908136483465, -0.6692913385826771977, 0.1292274648535927661 ) ) ;
#21165=CARTESIAN_POINT ( 'NONE',  ( 0.4396325459317590445, -0.6692913385826771977, 0.1292274648535927661 ) ) ;
#21168=CARTESIAN_POINT ( 'NONE',  ( 1.391076115485564868, 0.2306618581243847221, -0.2411417322834647770 ) ) ;
#21169=CARTESIAN_POINT ( 'NONE',  ( -1.259842519685038686, -0.1870078740157479769, 0.3641732283464567677 ) ) ;
#21170=B_SPLINE_CURVE_WITH_KNOTS ( 'NONE', 1,
 ( #33062, #58733 ),
 .UNSPECIFIED., .F., .F.,
 ( 2, 2 ),
 ( 0.000000000000000000, 0.002250000000000000264 ),
 .UNSPECIFIED. ) ;
#21171=CARTESIAN_POINT ( 'NONE',  ( 1.246719160104987623, -0.004921259842519870586, -0.3153832671262229437 ) ) ;
#21172=CARTESIAN_POINT ( 'NONE',  ( -1.417322834645668772, -0.1870078740157480601, -0.3641732283464567677 ) ) ;
#21173=CARTESIAN_POINT ( 'NONE',  ( -0.7020997375328074108, -0.08942795157527998196, 0.3641732283464567121 ) ) ;
#21175=CARTESIAN_POINT ( 'NONE',  ( 0.6824146981627303710, 0.1283753931104746893, -0.1820866141732285504 ) ) ;
#21176=CARTESIAN_POINT ( 'NONE',  ( 0.06561679790026316017, -0.4281496062992124485, 0.4176697321401328655 ) ) ;
#21177=CARTESIAN_POINT ( 'NONE',  ( 1.069553805774278610, -0.6692913385826771977, 0.1292274648535927661 ) ) ;
#21178=CARTESIAN_POINT ( 'NONE',  ( -0.1574803149606292529, -0.1870078740157480879, -0.4822834645669291653 ) ) ;
#21179=CARTESIAN_POINT ( 'NONE',  ( 0.1049868766404206816, -0.5023911411419708095, -0.1820866141732282451 ) ) ;
#21180=CARTESIAN_POINT ( 'NONE',  ( 1.220472440944882386, -0.6692913385826771977, 8.415575281601705876E-17 ) ) ;
#21181=CARTESIAN_POINT ( 'NONE',  ( -0.2099737532808391427, 0.1539470093639523085, 0.1968503937007873850 ) ) ;
#21182=CARTESIAN_POINT ( 'NONE',  ( -0.8792650918635160906, 0.05413385826771626580, -0.4176697321401330321 ) ) ;
#21184=CARTESIAN_POINT ( 'NONE',  ( 0.06596743314205978648, 0.004960608223778357855, -0.3437734562760192958 ) ) ;
#21185=VECTOR ( 'NONE', #42101, 39.37007874015748854 ) ;
#21186=CARTESIAN_POINT ( 'NONE',  ( -1.010498687664041384, 0.05413385826771666132, 0.4176697321401328100 ) ) ;
#21187=CARTESIAN_POINT ( 'NONE',  ( 0.01312335958005323398, 0.05413385826771666132, 0.4176697321401328100 ) ) ;
#21191=LINE ( 'NONE', #41378, #7846 ) ;
#21192=CARTESIAN_POINT ( 'NONE',  ( -1.240157480314959759, 0.07958543189024085140, 0.2665933059059887866 ) ) ;
#21194=CARTESIAN_POINT ( 'NONE',  ( -1.574803149606298636, -0.1870078740157479769, 0.4822834645669291653 ) ) ;
#21196=CARTESIAN_POINT ( 'NONE',  ( 0.5905511811023629321, 0.2952755905511811885, 0.000000000000000000 ) ) ;
#21197=CARTESIAN_POINT ( 'NONE',  ( -0.6692913385826764205, -0.5511811023622047445, 6.969142054262312111E-17 ) ) ;
#21198=CARTESIAN_POINT ( 'NONE',  ( 1.069553805774278610, -0.6692913385826771977, 0.1292274648535927661 ) ) ;
#21199=CARTESIAN_POINT ( 'NONE',  ( 0.2690288713910767848, -0.6692913385826773087, -0.1292274648535924053 ) ) ;
#21203=CARTESIAN_POINT ( 'NONE',  ( 1.437007874015748810, -0.5400638737290845981, -0.3530559997133363437 ) ) ;
#21204=CARTESIAN_POINT ( 'NONE',  ( 0.1377952755905518800, -0.5400638737290844871, 0.3530559997133364547 ) ) ;
#21205=CARTESIAN_POINT ( 'NONE',  ( 1.594488188976378673, 0.1660481256975885056, 0.3530559997133364547 ) ) ;
#21206=CARTESIAN_POINT ( 'NONE',  ( 1.023622047244095334, -0.1870078740157479769, 0.4822834645669291653 ) ) ;
#21208=CARTESIAN_POINT ( 'NONE',  ( 0.09842519685039434474, -0.5400638737290845981, -0.3530559997133363437 ) ) ;
#21209=CARTESIAN_POINT ( 'NONE',  ( 0.8530183727034128527, -0.4281496062992124485, 0.4176697321401328655 ) ) ;
#21210=CARTESIAN_POINT ( 'NONE',  ( 0.1574803149606306130, -0.1870078740157480879, -0.4822834645669291653 ) ) ;
#21211=CARTESIAN_POINT ( 'NONE',  ( 0.6233595800524942554, -0.08942795157528024563, -0.3641732283464568787 ) ) ;
#21212=CARTESIAN_POINT ( 'NONE',  ( -1.266404199475064773, -0.3162353388693405765, 0.4822834645669290543 ) ) ;
#21213=CARTESIAN_POINT ( 'NONE',  ( -1.594488188976377563, -0.5400638737290844871, 0.3530559997133364547 ) ) ;
#21214=CARTESIAN_POINT ( 'NONE',  ( 0.8070866141732288002, 0.1660481256975885056, 0.3530559997133364547 ) ) ;
#21220=CARTESIAN_POINT ( 'NONE',  ( 1.154855643044620184, -0.6046776061558807314, 0.2411417322834647770 ) ) ;
#21221=CARTESIAN_POINT ( 'NONE',  ( 1.076115485564305141, -0.5023911411419708095, 0.1820866141732285504 ) ) ;
#21226=CARTESIAN_POINT ( 'NONE',  ( 1.240157480314961314, -0.5400638737290844871, 0.3530559997133364547 ) ) ;
#21228=CARTESIAN_POINT ( 'NONE',  ( -0.1837270341207343505, -0.6046776061558807314, 0.2411417322834647770 ) ) ;
#21229=CARTESIAN_POINT ( 'NONE',  ( 1.279527559055118724, 0.1660481256975885056, 0.3530559997133364547 ) ) ;
#21231=CARTESIAN_POINT ( 'NONE',  ( -1.712598425196849572, 0.1660481256975885056, 0.3530559997133364547 ) ) ;
#21234=CARTESIAN_POINT ( 'NONE',  ( 1.568241469816273659, -0.08942795157528024563, -0.3641732283464568787 ) ) ;
#21236=CARTESIAN_POINT ( 'NONE',  ( -0.9711286089238838626, 0.1283753931104746893, -0.1820866141732285504 ) ) ;
#21237=CARTESIAN_POINT ( 'NONE',  ( -1.430446194225720724, 0.05413385826771626580, -0.4176697321401330321 ) ) ;
#21238=CARTESIAN_POINT ( 'NONE',  ( 0.7217847769028878924, 0.05413385826771666132, 0.4176697321401328100 ) ) ;
#21241=CARTESIAN_POINT ( 'NONE',  ( 1.443569553805774897, -0.6046776061558809534, -0.2411417322834644161 ) ) ;
#21242=CARTESIAN_POINT ( 'NONE',  ( -0.4265091863517051496, 0.2066929133858267098, -0.1054918080437494132 ) ) ;
#21243=CARTESIAN_POINT ( 'NONE',  ( -0.6036745406824141069, 0.1283753931104748280, 0.1820866141732283561 ) ) ;
#21244=CARTESIAN_POINT ( 'NONE',  ( 0.9251968503937015864, 0.1660481256975883668, -0.3530559997133364547 ) ) ;
#21245=CARTESIAN_POINT ( 'NONE',  ( -1.646981627296586703, -0.3162353388693409650, -0.4822834645669289433 ) ) ;
#21247=CARTESIAN_POINT ( 'NONE',  ( -0.6233595800524928121, -0.08942795157527998196, 0.3641732283464567121 ) ) ;
#21248=CARTESIAN_POINT ( 'NONE',  ( 1.607611548556431069, -0.6692913385826773087, -0.1292274648535924053 ) ) ;
#21250=CARTESIAN_POINT ( 'NONE',  ( 0.5708661417322841158, -0.5400638737290845981, -0.3530559997133363437 ) ) ;
#21251=CARTESIAN_POINT ( 'NONE',  ( -0.9645669291338575535, 0.07958543189024071263, -0.2665933059059888421 ) ) ;
#21252=CARTESIAN_POINT ( 'NONE',  ( -0.1509186351706028884, -0.08942795157527998196, 0.3641732283464567121 ) ) ;
#21254=CARTESIAN_POINT ( 'NONE',  ( -0.3674540682414692561, -0.6046776061558809534, -0.2411417322834644161 ) ) ;
#21255=CARTESIAN_POINT ( 'NONE',  ( -1.469816272965878357, 0.1283753931104748280, 0.1820866141732283561 ) ) ;
#21257=CARTESIAN_POINT ( 'NONE',  ( 0.6889763779527563470, 0.1660481256975883668, -0.3530559997133364547 ) ) ;
#21259=CARTESIAN_POINT ( 'NONE',  ( 0.8776378784356307916, 4.512065407040659715E-16, 0.3791483426435169335 ) ) ;
#21261=CARTESIAN_POINT ( 'NONE',  ( -0.8661417322834640276, -0.1870078740157480879, -0.4822834645669291653 ) ) ;
#21262=CARTESIAN_POINT ( 'NONE',  ( -0.1902887139107604098, -0.5511811023622046335, 0.09757992244046803654 ) ) ;
#21263=CARTESIAN_POINT ( 'NONE',  ( -1.482939632545930975, 0.05413385826771666132, 0.4176697321401328100 ) ) ;
#21264=CARTESIAN_POINT ( 'NONE',  ( 0.4133858267716541968, 0.07958543189024085140, 0.2665933059059887866 ) ) ;
#21265=CARTESIAN_POINT ( 'NONE',  ( -0.8136482939632537770, -0.5023911411419708095, 0.1820866141732285504 ) ) ;
#21266=CARTESIAN_POINT ( 'NONE',  ( -1.233595800524933894, 0.2306618581243848609, 0.2411417322834645549 ) ) ;
#21267=CARTESIAN_POINT ( 'NONE',  ( -1.410761154855642463, -0.05778040916215522460, 0.4822834645669289988 ) ) ;
#21268=CARTESIAN_POINT ( 'NONE',  ( -1.437007874015747477, 0.1660481256975883668, -0.3530559997133364547 ) ) ;
#21269=CARTESIAN_POINT ( 'NONE',  ( 1.036745406824147508, 0.009842519685039467087, 0.3409548833797002021 ) ) ;
#21270=CARTESIAN_POINT ( 'NONE',  ( 0.7086614173228353852, -0.1870078740157479769, 0.3641732283464567677 ) ) ;
#21271=CARTESIAN_POINT ( 'NONE',  ( 0.4855643044619430415, -0.4281496062992127816, -0.4176697321401328100 ) ) ;
#21272=CARTESIAN_POINT ( 'NONE',  ( -1.312335958005248715, 0.2306618581243848609, 0.2411417322834645549 ) ) ;
#21273=CARTESIAN_POINT ( 'NONE',  ( 1.587926509186352142, -0.004921259842519576551, 0.3153832671262227771 ) ) ;
#21277=CARTESIAN_POINT ( 'NONE',  ( -1.299212598425196097, 0.1771653543307087630, 0.000000000000000000 ) ) ;
#21278=CARTESIAN_POINT ( 'NONE',  ( -0.3477690288713902178, 0.2952755905511810774, -0.1292274648535930714 ) ) ;
#21279=CARTESIAN_POINT ( 'NONE',  ( 0.1246719160104994284, -0.6692913385826771977, 0.1292274648535927661 ) ) ;
#21280=CARTESIAN_POINT ( 'NONE',  ( -1.338582677165353729, -0.1870078740157480601, -0.3641732283464567677 ) ) ;
#21282=CARTESIAN_POINT ( 'NONE',  ( -1.312335958005248715, -0.6046776061558809534, -0.2411417322834644161 ) ) ;
#21283=CARTESIAN_POINT ( 'NONE',  ( 0.5118110236220480003, -0.6692913385826771977, 8.415575281601705876E-17 ) ) ;
#21284=CARTESIAN_POINT ( 'NONE',  ( 0.1574803149606306130, -0.1870078740157480879, -0.4822834645669291653 ) ) ;
#21286=CARTESIAN_POINT ( 'NONE',  ( 1.135170603674541256, 0.2952755905511811885, 0.1292274648535926551 ) ) ;
#21292=CARTESIAN_POINT ( 'NONE',  ( 0.2099737532808405305, 0.1283753931104746893, -0.1820866141732285504 ) ) ;
#21293=CARTESIAN_POINT ( 'NONE',  ( -0.4265091863517051496, 0.2952755905511810774, -0.1292274648535930714 ) ) ;
#21294=CARTESIAN_POINT ( 'NONE',  ( 1.181102362204724976, -0.1870078740157480879, -0.4822834645669291653 ) ) ;
#21296=CARTESIAN_POINT ( 'NONE',  ( 0.1377952755905518800, 0.07958543189024071263, -0.2665933059059888421 ) ) ;
#21297=CARTESIAN_POINT ( 'NONE',  ( -0.9645669291338575535, 0.1660481256975883668, -0.3530559997133364547 ) ) ;
#21298=CARTESIAN_POINT ( 'NONE',  ( -1.482939632545930975, 0.05413385826771666132, 0.4176697321401328100 ) ) ;
#21303=CARTESIAN_POINT ( 'NONE',  ( 1.476377952755906220, 0.1660481256975883668, -0.3530559997133364547 ) ) ;
#21304=CARTESIAN_POINT ( 'NONE',  ( -1.535433070866141225, 0.2952755905511811885, 0.000000000000000000 ) ) ;
#21305=CARTESIAN_POINT ( 'NONE',  ( -1.279527559055116948, 0.07958543189024071263, -0.2665933059059888421 ) ) ;
#21306=CARTESIAN_POINT ( 'NONE',  ( -1.351706036745406347, -0.4281496062992124485, 0.4176697321401328655 ) ) ;
#21308=FACE_OUTER_BOUND ( 'NONE', #64249, .T. ) ;
#21309=CARTESIAN_POINT ( 'NONE',  ( 1.161417322834646493, -0.5400638737290844871, 0.3530559997133364547 ) ) ;
#21310=CARTESIAN_POINT ( 'NONE',  ( -1.076115485564303809, 0.2306618581243848609, 0.2411417322834645549 ) ) ;
#21311=CARTESIAN_POINT ( 'NONE',  ( -0.1902887139107604098, -0.6692913385826771977, 0.1292274648535927661 ) ) ;
#21312=CARTESIAN_POINT ( 'NONE',  ( -0.1443569553805768291, 0.05413385826771666132, 0.4176697321401328100 ) ) ;
#21313=CARTESIAN_POINT ( 'NONE',  ( -1.384514435695537005, -0.6692913385826773087, -0.1292274648535924053 ) ) ;
#21315=CARTESIAN_POINT ( 'NONE',  ( 0.7480314960629927956, -0.6692913385826771977, 8.415575281601705876E-17 ) ) ;
#21317=CARTESIAN_POINT ( 'NONE',  ( -1.272965879265091305, -0.004921259842519870586, -0.3153832671262229437 ) ) ;
#21322=CARTESIAN_POINT ( 'NONE',  ( -1.082677165354329896, 0.1660481256975885056, 0.3530559997133364547 ) ) ;
#21323=CARTESIAN_POINT ( 'NONE',  ( -1.450131233595799651, 0.2952755905511810774, -0.1292274648535930714 ) ) ;
#21325=CARTESIAN_POINT ( 'NONE',  ( -1.437007874015747477, -0.5400638737290844871, 0.3530559997133364547 ) ) ;
#21326=CARTESIAN_POINT ( 'NONE',  ( -1.646981627296586703, -0.3162353388693409650, -0.4822834645669289433 ) ) ;
#21328=CARTESIAN_POINT ( 'NONE',  ( -1.364829396325458521, -0.6046776061558807314, 0.2411417322834647770 ) ) ;
#21331=CARTESIAN_POINT ( 'NONE',  ( 0.1115485564304470323, 0.1771653543307087630, 0.09757992244046791164 ) ) ;
#21333=CARTESIAN_POINT ( 'NONE',  ( -0.9908136482939626788, -0.5511811023622048555, -0.09757992244046775898 ) ) ;
#21334=CARTESIAN_POINT ( 'NONE',  ( -1.305774278215222184, 0.2952755905511811885, 0.1292274648535926551 ) ) ;
#21335=CARTESIAN_POINT ( 'NONE',  ( 0.9055118110236227702, -0.6692913385826771977, 8.415575281601705876E-17 ) ) ;
#21336=CARTESIAN_POINT ( 'NONE',  ( -1.010498687664041384, 0.05413385826771666132, 0.4176697321401328100 ) ) ;
#21339=CARTESIAN_POINT ( 'NONE',  ( -1.213910761154854745, -0.6692913385826771977, 0.1292274648535927661 ) ) ;
#21340=CARTESIAN_POINT ( 'NONE',  ( 1.010498687664042716, 0.05413385826771626580, -0.4176697321401330321 ) ) ;
#21341=CARTESIAN_POINT ( 'NONE',  ( -1.633858267716534529, -0.4536011799217368745, -0.2665933059059886201 ) ) ;
#21347=CARTESIAN_POINT ( 'NONE',  ( -0.3477690288713902178, 0.2952755905511810774, -0.1292274648535930714 ) ) ;
#21348=CARTESIAN_POINT ( 'NONE',  ( -1.581364829396324945, -0.08942795157528024563, -0.3641732283464568787 ) ) ;
#21350=CARTESIAN_POINT ( 'NONE',  ( -1.666666666666665853, 0.05413385826771626580, -0.4176697321401330321 ) ) ;
#21352=CARTESIAN_POINT ( 'NONE',  ( -1.463254593175852492, -0.6692913385826773087, -0.1292274648535924053 ) ) ;
#21353=CARTESIAN_POINT ( 'NONE',  ( -0.3674540682414692561, -0.6046776061558809534, -0.2411417322834644161 ) ) ;
#21355=CARTESIAN_POINT ( 'NONE',  ( 0.5446194225721792126, -0.08942795157528024563, -0.3641732283464568787 ) ) ;
#21357=CARTESIAN_POINT ( 'NONE',  ( 0.2427821522309719648, -0.08942795157527998196, 0.3641732283464567121 ) ) ;
#21358=CARTESIAN_POINT ( 'NONE',  ( 0.9580052493438326877, -0.004921259842519576551, 0.3153832671262227771 ) ) ;
#21359=CARTESIAN_POINT ( 'NONE',  ( 1.003937007874016185, 0.1660481256975883668, -0.3530559997133364547 ) ) ;
#21360=CARTESIAN_POINT ( 'NONE',  ( 0.1837270341207357105, -0.5023911411419708095, -0.1820866141732282451 ) ) ;
#21362=CARTESIAN_POINT ( 'NONE',  ( -1.246719160104985846, -0.4281496062992127816, -0.4176697321401328100 ) ) ;
#21363=CARTESIAN_POINT ( 'NONE',  ( -0.2165354330708654795, -0.4536011799217368745, -0.2665933059059886201 ) ) ;
#21364=CARTESIAN_POINT ( 'NONE',  ( -1.325459317585300889, -0.004921259842519576551, 0.3153832671262227771 ) ) ;
#21366=CARTESIAN_POINT ( 'NONE',  ( -1.082677165354329896, -0.4536011799217368745, -0.2665933059059886201 ) ) ;
#21368=CARTESIAN_POINT ( 'NONE',  ( -0.1115485564304453947, -0.6692913385826771977, 0.1292274648535927661 ) ) ;
#21370=CARTESIAN_POINT ( 'NONE',  ( 0.7349081364829402885, -0.5023911411419708095, -0.1820866141732282451 ) ) ;
#21371=CARTESIAN_POINT ( 'NONE',  ( -0.1574803149606292529, -0.1870078740157479769, 0.3641732283464567677 ) ) ;
#21372=CARTESIAN_POINT ( 'NONE',  ( -0.4855643044619415427, 0.05413385826771626580, -0.4176697321401330321 ) ) ;
#21373=CARTESIAN_POINT ( 'NONE',  ( 2.795275590551181466, 1.968503937007874738, 0.000000000000000000 ) ) ;
#21374=CARTESIAN_POINT ( 'NONE',  ( -1.089238845144356427, -0.3690944881889765550, -0.3153832671262227771 ) ) ;
#21376=CARTESIAN_POINT ( 'NONE',  ( 0.5446194225721792126, -0.3162353388693405765, 0.4822834645669290543 ) ) ;
#21379=DIRECTION ( 'NONE',  ( 0.000000000000000000, 0.000000000000000000, -1.000000000000000000 ) ) ;
#21380=CARTESIAN_POINT ( 'NONE',  ( -0.3477690288713905509, -0.5511811023622046335, 0.09757992244046803654 ) ) ;
#21381=CARTESIAN_POINT ( 'NONE',  ( -1.509186351706035767, -0.4281496062992124485, 0.4176697321401328655 ) ) ;
#21382=CARTESIAN_POINT ( 'NONE',  ( 1.574803149606299746, -0.1870078740157480879, -0.4822834645669291653 ) ) ;
#21384=CARTESIAN_POINT ( 'NONE',  ( -0.6889763779527552368, -0.4536011799217368745, -0.2665933059059886201 ) ) ;
#21386=CARTESIAN_POINT ( 'NONE',  ( 1.069553805774278610, -0.6692913385826771977, 0.1292274648535927661 ) ) ;
#21390=CARTESIAN_POINT ( 'NONE',  ( -1.725721784776902190, -0.05778040916215522460, 0.4822834645669289988 ) ) ;
#21391=CARTESIAN_POINT ( 'NONE',  ( -1.279527559055116948, -0.5400638737290844871, 0.3530559997133364547 ) ) ;
#21392=CARTESIAN_POINT ( 'NONE',  ( 1.338582677165355062, -0.1870078740157480879, -0.4822834645669291653 ) ) ;
#21394=CARTESIAN_POINT ( 'NONE',  ( 1.108923884514436686, -0.2845877964562161244, -0.3641732283464567121 ) ) ;
#21395=( BOUNDED_CURVE ( )  B_SPLINE_CURVE ( 1, ( #38176, #36943 ),
 .UNSPECIFIED., .F., .F. ) 
 B_SPLINE_CURVE_WITH_KNOTS ( ( 2, 2 ),
 ( 6.938893903907228378E-18, 0.002000000000000008715 ),
 .UNSPECIFIED. ) 
 CURVE ( )  GEOMETRIC_REPRESENTATION_ITEM ( )  RATIONAL_B_SPLINE_CURVE ( ( 0.9875488213027530104, 0.9875488213027530104 ) ) 
 REPRESENTATION_ITEM ( '' )  );
#21396=CARTESIAN_POINT ( 'NONE',  ( 0.03280839895013198948, -0.6692913385826773087, -0.1292274648535924053 ) ) ;
#21397=CARTESIAN_POINT ( 'NONE',  ( -0.4133858267716528645, -0.5400638737290844871, 0.3530559997133364547 ) ) ;
#21400=CARTESIAN_POINT ( 'NONE',  ( 0.2952755905511816326, -0.4536011799217367080, 0.2665933059059888421 ) ) ;
#21404=VERTEX_POINT ( 'NONE', #68842 ) ;
#21405=CARTESIAN_POINT ( 'NONE',  ( -0.3674540682414692561, -0.6046776061558809534, -0.2411417322834644161 ) ) ;
#21406=CARTESIAN_POINT ( 'NONE',  ( 1.246719160104987623, -0.4281496062992124485, 0.4176697321401328655 ) ) ;
#21407=CARTESIAN_POINT ( 'NONE',  ( 0.3674540682414705883, -0.6046776061558807314, 0.2411417322834647770 ) ) ;
#21408=CARTESIAN_POINT ( 'NONE',  ( -0.5314960629921250401, 0.07958543189024085140, 0.2665933059059887866 ) ) ;
#21409=CARTESIAN_POINT ( 'NONE',  ( 1.076115485564305141, 0.2306618581243847221, -0.2411417322834647770 ) ) ;
#21411=CARTESIAN_POINT ( 'NONE',  ( -0.9711286089238838626, 0.2306618581243847221, -0.2411417322834647770 ) ) ;
#21412=CARTESIAN_POINT ( 'NONE',  ( -0.07874015748031421014, -0.1870078740157480879, -0.4822834645669291653 ) ) ;
#21413=CARTESIAN_POINT ( 'NONE',  ( -0.7414698162729651543, 0.2952755905511810774, -0.1292274648535930714 ) ) ;
#21414=CARTESIAN_POINT ( 'NONE',  ( 1.259842519685040019, -0.1870078740157479769, 0.4822834645669291653 ) ) ;
#21415=CARTESIAN_POINT ( 'NONE',  ( 1.082677165354331228, -0.5400638737290844871, 0.3530559997133364547 ) ) ;
#21416=CARTESIAN_POINT ( 'NONE',  ( 1.207349081364829990, 0.2306618581243848609, 0.2411417322834645549 ) ) ;
#21418=CARTESIAN_POINT ( 'NONE',  ( -0.1049868766404193215, -0.5023911411419708095, 0.1820866141732285504 ) ) ;
#21422=CARTESIAN_POINT ( 'NONE',  ( -0.8858267716535425107, 0.07958543189024071263, -0.2665933059059888421 ) ) ;
#21423=CARTESIAN_POINT ( 'NONE',  ( -0.1377952755905504645, -0.5400638737290845981, -0.3530559997133363437 ) ) ;
#21425=CARTESIAN_POINT ( 'NONE',  ( -0.3477690288713905509, -0.6692913385826771977, 0.1292274648535927661 ) ) ;
#21426=CARTESIAN_POINT ( 'NONE',  ( -0.3608923884514428360, -0.6692913385826773087, -0.1292274648535924053 ) ) ;
#21427=CARTESIAN_POINT ( 'NONE',  ( -0.7874015748031489847, -0.1870078740157480879, -0.4822834645669291653 ) ) ;
#21428=CARTESIAN_POINT ( 'NONE',  ( -1.594488188976377563, -0.5400638737290844871, 0.3530559997133364547 ) ) ;
#21429=CARTESIAN_POINT ( 'NONE',  ( 1.240157480314961314, 0.07958543189024071263, -0.2665933059059888421 ) ) ;
#21430=CARTESIAN_POINT ( 'NONE',  ( -1.594488188976377119, 0.1660481256975883668, -0.3530559997133364547 ) ) ;
#21432=CARTESIAN_POINT ( 'NONE',  ( 0.5643044619422579178, -0.3690944881889765550, -0.3153832671262227771 ) ) ;
#21433=CARTESIAN_POINT ( 'NONE',  ( 0.1443569553805781891, 0.05413385826771626580, -0.4176697321401330321 ) ) ;
#21434=CARTESIAN_POINT ( 'NONE',  ( 0.1771653543307093182, -0.5400638737290845981, -0.3530559997133363437 ) ) ;
#21439=CARTESIAN_POINT ( 'NONE',  ( -0.7217847769028863381, 0.05413385826771626580, -0.4176697321401330321 ) ) ;
#21442=CARTESIAN_POINT ( 'NONE',  ( -1.627296587926508442, 0.1283753931104748280, 0.1820866141732283561 ) ) ;
#21443=CARTESIAN_POINT ( 'NONE',  ( 0.7086614173228352742, -0.1870078740157480879, -0.4822834645669291653 ) ) ;
#21444=CARTESIAN_POINT ( 'NONE',  ( 0.7939632545931766261, -0.3162353388693409650, -0.4822834645669289433 ) ) ;
#21445=CARTESIAN_POINT ( 'NONE',  ( -0.2034120734908128059, 0.1771653543307087630, 0.09757992244046791164 ) ) ;
#21446=CARTESIAN_POINT ( 'NONE',  ( 0.1574803149606306130, -0.1870078740157479769, 0.4822834645669291653 ) ) ;
#21448=CARTESIAN_POINT ( 'NONE',  ( -0.2624671916010490880, -0.5023911411419708095, 0.1820866141732285504 ) ) ;
#21449=CARTESIAN_POINT ( 'NONE',  ( -0.04593175853018302557, -0.6692913385826773087, -0.1292274648535924053 ) ) ;
#21451=CARTESIAN_POINT ( 'NONE',  ( 1.581364829396326277, -0.08942795157527998196, 0.3641732283464567121 ) ) ;
#21452=CARTESIAN_POINT ( 'NONE',  ( 0.1706036745406830368, -0.004921259842519576551, 0.3153832671262227771 ) ) ;
#21453=FACE_OUTER_BOUND ( 'NONE', #6801, .T. ) ;
#21454=CARTESIAN_POINT ( 'NONE',  ( -0.9383202099737524282, -0.05778040916215522460, 0.4822834645669289988 ) ) ;
#21455=CARTESIAN_POINT ( 'NONE',  ( -0.8136482939632537770, 0.1283753931104746893, -0.1820866141732285504 ) ) ;
#21456=CARTESIAN_POINT ( 'NONE',  ( -1.033630966599879297, -2.567464376874931580E-15, -0.4445507791589072832 ) ) ;
#21457=CARTESIAN_POINT ( 'NONE',  ( -0.6496062992125976043, -0.5400638737290844871, 0.3530559997133364547 ) ) ;
#21458=CARTESIAN_POINT ( 'NONE',  ( -0.6102362204724400829, -0.5400638737290845981, -0.3530559997133363437 ) ) ;
#21459=CARTESIAN_POINT ( 'NONE',  ( 0.04593175853018440641, -0.6692913385826771977, 0.1292274648535927661 ) ) ;
#21463=CARTESIAN_POINT ( 'NONE',  ( 0.6102362204724416372, 0.07958543189024071263, -0.2665933059059888421 ) ) ;
#21464=CARTESIAN_POINT ( 'NONE',  ( 1.437007874015748810, 0.1660481256975885056, 0.3530559997133364547 ) ) ;
#21465=CARTESIAN_POINT ( 'NONE',  ( -1.437007874015747477, -0.4536011799217367080, 0.2665933059059888421 ) ) ;
#21466=CARTESIAN_POINT ( 'NONE',  ( 1.351706036745407680, 0.05413385826771666132, 0.4176697321401328100 ) ) ;
#21467=CARTESIAN_POINT ( 'NONE',  ( -1.148293963254592542, -0.5511811023622048555, -0.09757992244046775898 ) ) ;
#21468=CARTESIAN_POINT ( 'NONE',  ( -0.6364829396325453192, -0.3162353388693405765, 0.4822834645669290543 ) ) ;
#21469=CARTESIAN_POINT ( 'NONE',  ( 0.2624671916010504757, 0.1283753931104748280, 0.1820866141732283561 ) ) ;
#21471=CARTESIAN_POINT ( 'NONE',  ( 0.5839895013123367340, -0.5511811023622048555, -0.09757992244046775898 ) ) ;
#21472=CARTESIAN_POINT ( 'NONE',  ( 0.4724409448818904789, -0.1870078740157480879, -0.4822834645669291653 ) ) ;
#21474=CARTESIAN_POINT ( 'NONE',  ( -0.7808398950131225646, -0.05778040916215522460, 0.4822834645669289988 ) ) ;
#21476=CARTESIAN_POINT ( 'NONE',  ( 0.9580052493438326877, -0.004921259842519576551, 0.3153832671262227771 ) ) ;
#21477=CARTESIAN_POINT ( 'NONE',  ( 0.6102362204724416372, 0.1660481256975883668, -0.3530559997133364547 ) ) ;
#21478=CARTESIAN_POINT ( 'NONE',  ( -0.1509186351706028884, -0.3162353388693409650, -0.4822834645669289433 ) ) ;
#21479=CARTESIAN_POINT ( 'NONE',  ( -0.3412073490813641308, 0.1283753931104746893, -0.1820866141732285504 ) ) ;
#21481=CARTESIAN_POINT ( 'NONE',  ( -0.1312335958005241554, -0.5023911411419708095, -0.1820866141732282451 ) ) ;
#21482=CARTESIAN_POINT ( 'NONE',  ( 0.3805774278215230400, -0.4281496062992124485, 0.4176697321401328655 ) ) ;
#21483=CARTESIAN_POINT ( 'NONE',  ( -0.7349081364829390672, 0.1283753931104746893, -0.1820866141732285504 ) ) ;
#21485=CARTESIAN_POINT ( 'NONE',  ( -1.030183727034119867, -0.3162353388693405765, 0.4822834645669290543 ) ) ;
#21486=CARTESIAN_POINT ( 'NONE',  ( -0.8546455861312985958, -4.966502543501560364E-15, 0.3791483426435189319 ) ) ;
#21487=VERTEX_POINT ( 'NONE', #17104 ) ;
#21488=CARTESIAN_POINT ( 'NONE',  ( -1.187664041994750175, -0.08942795157528024563, -0.3641732283464568787 ) ) ;
#21489=CARTESIAN_POINT ( 'NONE',  ( -0.1509186351706028884, -0.05778040916215522460, 0.4822834645669289988 ) ) ;
#21490=CARTESIAN_POINT ( 'NONE',  ( -1.646981627296586703, -0.3162353388693409650, -0.4822834645669289433 ) ) ;
#21491=CARTESIAN_POINT ( 'NONE',  ( -0.8530183727034112984, 0.05413385826771666132, 0.4176697321401328100 ) ) ;
#21492=LINE ( 'NONE', #14782, #80805 ) ;
#21493=CARTESIAN_POINT ( 'NONE',  ( 1.043307086614173818, 0.1660481256975885056, 0.3530559997133364547 ) ) ;
#21494=CARTESIAN_POINT ( 'NONE',  ( 0.9448818897637802916, -0.1870078740157479769, 0.4822834645669291653 ) ) ;
#21495=CARTESIAN_POINT ( 'NONE',  ( 0.8727034120734913358, -0.05778040916215522460, 0.4822834645669289988 ) ) ;
#21496=CARTESIAN_POINT ( 'NONE',  ( -0.2952755905511805223, 0.1012011053420777407, 0.2882089793578257453 ) ) ;
#21498=CARTESIAN_POINT ( 'NONE',  ( -1.482939632545930975, -0.4281496062992127816, -0.4176697321401328100 ) ) ;
#21502=CARTESIAN_POINT ( 'NONE',  ( -0.3280839895013117347, -0.004921259842519870586, -0.3153832671262229437 ) ) ;
#21505=CARTESIAN_POINT ( 'NONE',  ( 0.6889763779527563470, 0.1660481256975883668, -0.3530559997133364547 ) ) ;
#21506=CARTESIAN_POINT ( 'NONE',  ( 0.2230971128608929543, 0.05413385826771626580, -0.4176697321401330321 ) ) ;
#21507=CARTESIAN_POINT ( 'NONE',  ( -0.8464566929133852113, 0.1660481256975885056, 0.3530559997133364547 ) ) ;
#21508=CARTESIAN_POINT ( 'NONE',  ( 1.686351706036745890, 0.2952755905511811885, 0.1292274648535926551 ) ) ;
#21509=CARTESIAN_POINT ( 'NONE',  ( -0.8398950131233585692, 0.1283753931104748280, 0.1820866141732283561 ) ) ;
#21511=CARTESIAN_POINT ( 'NONE',  ( 0.3674540682414705883, -0.6046776061558807314, 0.2411417322834647770 ) ) ;
#21512=CARTESIAN_POINT ( 'NONE',  ( 0.6824146981627303710, 0.1283753931104746893, -0.1820866141732285504 ) ) ;
#21513=CARTESIAN_POINT ( 'NONE',  ( -0.9973753280839886548, 0.2306618581243848609, 0.2411417322834645549 ) ) ;
#21515=CARTESIAN_POINT ( 'NONE',  ( -1.227034120734907141, -0.6692913385826773087, -0.1292274648535924053 ) ) ;
#21516=CARTESIAN_POINT ( 'NONE',  ( -1.033630966599879297, -2.567464376874931580E-15, -0.4445507791589072832 ) ) ;
#21517=CARTESIAN_POINT ( 'NONE',  ( 1.227034120734908917, 0.2952755905511810774, -0.1292274648535930714 ) ) ;
#21518=CARTESIAN_POINT ( 'NONE',  ( 1.279527559055118724, -0.4536011799217368745, -0.2665933059059886201 ) ) ;
#21521=CARTESIAN_POINT ( 'NONE',  ( -0.4461942257217840213, -0.6046776061558809534, -0.2411417322834644161 ) ) ;
#21523=CARTESIAN_POINT ( 'NONE',  ( 0.9514435695538062676, -0.08942795157527998196, 0.3641732283464567121 ) ) ;
#21524=CARTESIAN_POINT ( 'NONE',  ( -1.148293963254592542, -0.6692913385826773087, -0.1292274648535924053 ) ) ;
#21525=CARTESIAN_POINT ( 'NONE',  ( 0.9186351706036751663, -0.6046776061558807314, 0.2411417322834647770 ) ) ;
#21526=CARTESIAN_POINT ( 'NONE',  ( 0.9317585301837276734, -0.4281496062992124485, 0.4176697321401328655 ) ) ;
#21527=CARTESIAN_POINT ( 'NONE',  ( 0.1049868766404206816, -0.6046776061558809534, -0.2411417322834644161 ) ) ;
#21528=CARTESIAN_POINT ( 'NONE',  ( -0.5446194225721777693, -0.05778040916215522460, 0.4822834645669289988 ) ) ;
#21530=CARTESIAN_POINT ( 'NONE',  ( 1.541994750656168645, -0.5511811023622046335, 0.09757992244046803654 ) ) ;
#21531=CARTESIAN_POINT ( 'NONE',  ( -0.7874015748031489847, -0.1870078740157480879, -0.4822834645669291653 ) ) ;
#21532=CARTESIAN_POINT ( 'NONE',  ( -0.5643044619422565855, -0.3690944881889763329, 0.3153832671262228327 ) ) ;
#21534=CARTESIAN_POINT ( 'NONE',  ( 1.561679790026247350, 0.05413385826771626580, -0.4176697321401330321 ) ) ;
#21535=CARTESIAN_POINT ( 'NONE',  ( -0.3412073490813641308, -0.6046776061558807314, 0.2411417322834647770 ) ) ;
#21537=CARTESIAN_POINT ( 'NONE',  ( 0.6299212598425204535, -0.1870078740157479769, 0.4822834645669291653 ) ) ;
#21540=CARTESIAN_POINT ( 'NONE',  ( -0.02624671916010428221, 0.2306618581243847221, -0.2411417322834647770 ) ) ;
#21541=CARTESIAN_POINT ( 'NONE',  ( 0.8595800524934390507, -0.2845877964562159024, 0.3641732283464567677 ) ) ;
#21542=CARTESIAN_POINT ( 'NONE',  ( -1.603475055217291612, 0.4410854135902511630, -0.04573490813648263542 ) ) ;
#21544=CARTESIAN_POINT ( 'NONE',  ( 1.076115485564305141, 0.1283753931104746893, -0.1820866141732285504 ) ) ;
#21545=CARTESIAN_POINT ( 'NONE',  ( 1.318897637795276356, 0.1660481256975883668, -0.3530559997133364547 ) ) ;
#21547=CARTESIAN_POINT ( 'NONE',  ( -0.3018372703412066094, 0.05413385826771666132, 0.4176697321401328100 ) ) ;
#21548=CARTESIAN_POINT ( 'NONE',  ( -1.646981627296586703, -0.05778040916215522460, 0.4822834645669289988 ) ) ;
#21549=CARTESIAN_POINT ( 'NONE',  ( 1.482939632545932307, -0.004921259842519870586, -0.3153832671262229437 ) ) ;
#21550=CARTESIAN_POINT ( 'NONE',  ( -0.1706036745406816491, -0.4281496062992124485, 0.4176697321401328655 ) ) ;
#21552=CARTESIAN_POINT ( 'NONE',  ( 1.286089238845145033, -0.6046776061558809534, -0.2411417322834644161 ) ) ;
#21553=CARTESIAN_POINT ( 'NONE',  ( 0.4396325459317590445, -0.6692913385826771977, 0.1292274648535927661 ) ) ;
#21554=CARTESIAN_POINT ( 'NONE',  ( 0.5314960629921267055, -0.4536011799217367080, 0.2665933059059888421 ) ) ;
#21556=CARTESIAN_POINT ( 'NONE',  ( 0.4986876640419954376, -0.5023911411419708095, -0.1820866141732282451 ) ) ;
#21557=CARTESIAN_POINT ( 'NONE',  ( -1.089238845144356427, 0.009842519685039463617, 0.3409548833797002576 ) ) ;
#21559=CARTESIAN_POINT ( 'NONE',  ( 0.6561679790026253567, -0.6046776061558809534, -0.2411417322834644161 ) ) ;
#21561=PLANE ( 'NONE',  #23756 ) ;
#21563=CARTESIAN_POINT ( 'NONE',  ( 0.04593175853018440641, 0.1771653543307087075, -0.09757992244046823083 ) ) ;
#21564=CARTESIAN_POINT ( 'NONE',  ( 0.1968503937007881344, -0.6692913385826771977, 8.415575281601705876E-17 ) ) ;
#21565=CARTESIAN_POINT ( 'NONE',  ( 1.253280839895013710, -0.08942795157528024563, -0.3641732283464568787 ) ) ;
#21566=CARTESIAN_POINT ( 'NONE',  ( -1.364829396325458521, 0.1283753931104746893, -0.1820866141732285504 ) ) ;
#21567=CARTESIAN_POINT ( 'NONE',  ( -1.017060367454067249, -0.3162353388693409650, -0.4822834645669289433 ) ) ;
#21568=CARTESIAN_POINT ( 'NONE',  ( -1.699475065616797398, 0.2952755905511811885, 0.1292274648535926551 ) ) ;
#21569=CARTESIAN_POINT ( 'NONE',  ( 0.4593175853018380828, 0.05413385826771626580, -0.4176697321401330321 ) ) ;
#21570=CARTESIAN_POINT ( 'NONE',  ( 1.594488188976378673, -0.5400638737290845981, -0.3530559997133363437 ) ) ;
#21572=CARTESIAN_POINT ( 'NONE',  ( 0.5643044619422579178, -0.4281496062992127816, -0.4176697321401328100 ) ) ;
#21575=CARTESIAN_POINT ( 'NONE',  ( 1.305774278215223960, -0.6692913385826771977, 0.1292274648535927661 ) ) ;
#21576=CARTESIAN_POINT ( 'NONE',  ( -1.272965879265091305, -0.3690944881889763329, 0.3153832671262228327 ) ) ;
#21577=CARTESIAN_POINT ( 'NONE',  ( 1.325459317585302665, -0.3690944881889763329, 0.3153832671262228327 ) ) ;
#21578=CARTESIAN_POINT ( 'NONE',  ( -1.259842519685038686, -0.1870078740157480601, -0.3641732283464567677 ) ) ;
#21579=CARTESIAN_POINT ( 'NONE',  ( -0.8923884514435688198, -0.5023911411419708095, 0.1820866141732285504 ) ) ;
#21580=CARTESIAN_POINT ( 'NONE',  ( 1.601049868766404982, 0.2306618581243848609, 0.2411417322834645549 ) ) ;
#21581=CARTESIAN_POINT ( 'NONE',  ( 0.6233595800524939223, -0.2845877964562159024, 0.3641732283464567677 ) ) ;
#21582=CARTESIAN_POINT ( 'NONE',  ( 0.2821522309711292364, 0.2952755905511810774, -0.1292274648535930714 ) ) ;
#21583=CARTESIAN_POINT ( 'NONE',  ( 1.240157480314961314, -0.5400638737290844871, 0.3530559997133364547 ) ) ;
#21584=CARTESIAN_POINT ( 'NONE',  ( -0.08530183727034056085, -0.3162353388693405765, 0.4822834645669290543 ) ) ;
#21585=CARTESIAN_POINT ( 'NONE',  ( 0.2821522309711292364, -0.5511811023622046335, 0.09757992244046803654 ) ) ;
#21586=CARTESIAN_POINT ( 'NONE',  ( 1.312335958005249825, 0.2306618581243847221, -0.2411417322834647770 ) ) ;
#21589=CARTESIAN_POINT ( 'NONE',  ( -1.082677165354329896, 0.1660481256975885056, 0.3530559997133364547 ) ) ;
#21591=CARTESIAN_POINT ( 'NONE',  ( 1.013613127888309595, -4.408777212815537393E-16, -0.4445507791589063395 ) ) ;
#21592=CARTESIAN_POINT ( 'NONE',  ( -0.8989501312335946848, -0.6692913385826771977, 0.1292274648535927661 ) ) ;
#21593=CARTESIAN_POINT ( 'NONE',  ( 0.03280839895013198948, 0.2952755905511811885, 0.1292274648535926551 ) ) ;
#21596=EDGE_LOOP ( 'NONE', ( #28774, #51280, #75457, #33719 ) ) ;
#21598=EDGE_CURVE ( 'NONE', #69851, #44891, #2714, .T. ) ;
#21599=CARTESIAN_POINT ( 'NONE',  ( 1.148293963254593653, 0.2952755905511810774, -0.1292274648535930714 ) ) ;
#21600=CARTESIAN_POINT ( 'NONE',  ( -0.2462293917967295909, -2.567464376874931580E-15, -0.4445507791589072832 ) ) ;
#21601=CARTESIAN_POINT ( 'NONE',  ( -1.496062992125983815, -0.1870078740157480601, -0.3641732283464567677 ) ) ;
#21604=CARTESIAN_POINT ( 'NONE',  ( 1.581364829396326277, -0.08942795157527998196, 0.3641732283464567121 ) ) ;
#21606=CARTESIAN_POINT ( 'NONE',  ( -0.1574803149606292529, -0.1870078740157480879, -0.4822834645669291653 ) ) ;
#21607=CARTESIAN_POINT ( 'NONE',  ( -0.4790026246719154557, -0.2845877964562159024, 0.3641732283464567677 ) ) ;
#21608=CARTESIAN_POINT ( 'NONE',  ( 0.9317585301837276734, -0.4281496062992124485, 0.4176697321401328655 ) ) ;
#21609=CARTESIAN_POINT ( 'NONE',  ( 0.3018372703412079971, -0.4281496062992124485, 0.4176697321401328655 ) ) ;
#21613=CARTESIAN_POINT ( 'NONE',  ( 1.161417322834646493, -0.5400638737290844871, 0.3530559997133364547 ) ) ;
#21614=CARTESIAN_POINT ( 'NONE',  ( 0.2624671916010504757, -0.6046776061558809534, -0.2411417322834644161 ) ) ;
#21615=CARTESIAN_POINT ( 'NONE',  ( -0.8398950131233585692, 0.2306618581243848609, 0.2411417322834645549 ) ) ;
#21616=CARTESIAN_POINT ( 'NONE',  ( 1.345144356955381593, -0.3162353388693409650, -0.4822834645669289433 ) ) ;
#21617=CARTESIAN_POINT ( 'NONE',  ( 0.8267716535433078384, -0.6692913385826771977, 8.415575281601705876E-17 ) ) ;
#21619=CARTESIAN_POINT ( 'NONE',  ( -0.07217847769028813698, -0.3162353388693409650, -0.4822834645669289433 ) ) ;
#21620=CARTESIAN_POINT ( 'NONE',  ( 0.5971128608923891301, 0.2952755905511810774, -0.1292274648535930714 ) ) ;
#21621=CARTESIAN_POINT ( 'NONE',  ( 0.1706036745406830368, -0.4281496062992127816, -0.4176697321401328100 ) ) ;
#21622=CARTESIAN_POINT ( 'NONE',  ( 0.9317585301837276734, -0.004921259842519870586, -0.3153832671262229437 ) ) ;
#21623=CARTESIAN_POINT ( 'NONE',  ( -1.515748031496062076, 0.1660481256975883668, -0.3530559997133364547 ) ) ;
#21624=CARTESIAN_POINT ( 'NONE',  ( -1.397637795275589623, 0.1660481256975885056, 0.3530559997133364547 ) ) ;
#21625=CARTESIAN_POINT ( 'NONE',  ( 0.5905511811023629321, -0.6692913385826771977, 8.415575281601705876E-17 ) ) ;
#21628=( BOUNDED_CURVE ( )  B_SPLINE_CURVE ( 1, ( #79549, #46699 ),
 .UNSPECIFIED., .F., .F. ) 
 B_SPLINE_CURVE_WITH_KNOTS ( ( 2, 2 ),
 ( 0.000000000000000000, 0.002000000000000005246 ),
 .UNSPECIFIED. ) 
 CURVE ( )  GEOMETRIC_REPRESENTATION_ITEM ( )  RATIONAL_B_SPLINE_CURVE ( ( 0.9875488213027527884, 0.9875488213027527884 ) ) 
 REPRESENTATION_ITEM ( '' )  );
#21632=CARTESIAN_POINT ( 'NONE',  ( 1.056430446194226658, 0.2952755905511811885, 0.1292274648535926551 ) ) ;
#21633=CARTESIAN_POINT ( 'NONE',  ( 0.7020997375328090762, -0.08942795157528024563, -0.3641732283464568787 ) ) ;
#21635=DIRECTION ( 'NONE',  ( -1.000000000000000000, -3.050063254464715781E-16, 0.000000000000000000 ) ) ;
#21636=CARTESIAN_POINT ( 'NONE',  ( -1.614173228346456712, 1.818966223839196816, -0.1372047244094478091 ) ) ;
#21640=CARTESIAN_POINT ( 'NONE',  ( -0.2952755905511804668, 0.1660481256975885056, 0.3530559997133364547 ) ) ;
#21641=CARTESIAN_POINT ( 'NONE',  ( 0.9055118110236227702, -0.6692913385826771977, 8.415575281601705876E-17 ) ) ;
#21642=ORIENTED_EDGE ( 'NONE', *, *, #74375, .F. ) ;
#21643=CARTESIAN_POINT ( 'NONE',  ( -1.437007874015747477, -0.5400638737290844871, 0.3530559997133364547 ) ) ;
#21644=CARTESIAN_POINT ( 'NONE',  ( -1.170004705068745876, -4.983732387537991731E-15, 0.3954985857520076920 ) ) ;
#21646=CARTESIAN_POINT ( 'NONE',  ( 1.469816272965879911, -0.5023911411419708095, 0.1820866141732285504 ) ) ;
#21648=CARTESIAN_POINT ( 'NONE',  ( -1.397637795275589623, -0.4536011799217368745, -0.2665933059059886201 ) ) ;
#21650=CARTESIAN_POINT ( 'NONE',  ( 0.3215223097112867578, -0.3162353388693409650, -0.4822834645669289433 ) ) ;
#21652=CARTESIAN_POINT ( 'NONE',  ( 1.620734908136483465, -0.6692913385826771977, 0.1292274648535927661 ) ) ;
#21653=CARTESIAN_POINT ( 'NONE',  ( -0.4600214019799515053, 0.000000000000000000, 0.3464511005275205946 ) ) ;
#21654=CARTESIAN_POINT ( 'NONE',  ( -0.9186351706036736120, 0.1283753931104748280, 0.1820866141732283561 ) ) ;
#21655=CARTESIAN_POINT ( 'NONE',  ( 0.7874015748031503170, -0.1870078740157480879, -0.4822834645669291653 ) ) ;
#21656=CARTESIAN_POINT ( 'NONE',  ( 1.154855643044620184, 0.1283753931104746893, -0.1820866141732285504 ) ) ;
#21658=CARTESIAN_POINT ( 'NONE',  ( -0.6102362204724400829, 0.07958543189024085140, 0.2665933059059887866 ) ) ;
#21659=CARTESIAN_POINT ( 'NONE',  ( -1.581364829396324945, -0.08942795157528024563, -0.3641732283464568787 ) ) ;
#21661=CARTESIAN_POINT ( 'NONE',  ( 0.5183727034120741983, 0.2952755905511810774, -0.1292274648535930714 ) ) ;
#21662=CARTESIAN_POINT ( 'NONE',  ( -0.7742782152230962556, -0.3690944881889765550, -0.3153832671262227771 ) ) ;
#21663=CARTESIAN_POINT ( 'NONE',  ( -0.2887139107611542133, 0.1283753931104748280, 0.1820866141732283561 ) ) ;
#21665=CARTESIAN_POINT ( 'NONE',  ( -0.4790026246719154557, -0.3162353388693405765, 0.4822834645669290543 ) ) ;
#21666=CARTESIAN_POINT ( 'NONE',  ( -1.528871391076114250, -0.5511811023622046335, 0.09757992244046803654 ) ) ;
#21668=CARTESIAN_POINT ( 'NONE',  ( 0.6496062992125991586, 0.1660481256975885056, 0.3530559997133364547 ) ) ;
#21671=CARTESIAN_POINT ( 'NONE',  ( -0.8727034120734901146, -0.05778040916215560624, -0.4822834645669293319 ) ) ;
#21672=CARTESIAN_POINT ( 'NONE',  ( -0.3805774278215216522, -0.3690944881889765550, -0.3153832671262227771 ) ) ;
#21673=CARTESIAN_POINT ( 'NONE',  ( -1.391076115485563314, -0.6046776061558809534, -0.2411417322834644161 ) ) ;
#21674=CARTESIAN_POINT ( 'NONE',  ( 0.4658792650918641698, -0.08942795157528024563, -0.3641732283464568787 ) ) ;
#21675=CARTESIAN_POINT ( 'NONE',  ( -0.5183727034120726440, -0.5511811023622048555, -0.09757992244046775898 ) ) ;
#21676=CARTESIAN_POINT ( 'NONE',  ( -1.030183727034119867, -0.05778040916215560624, -0.4822834645669293319 ) ) ;
#21677=CARTESIAN_POINT ( 'NONE',  ( 1.594488188976378673, 0.07958543189024085140, 0.2665933059059887866 ) ) ;
#21678=CARTESIAN_POINT ( 'NONE',  ( 1.220472440944882608, 0.2952755905511811885, 0.000000000000000000 ) ) ;
#21679=CARTESIAN_POINT ( 'NONE',  ( -1.614173228346456712, 2.362204724409448620, -0.1372047244094478091 ) ) ;
#21680=CARTESIAN_POINT ( 'NONE',  ( 0.9908136482939640111, -0.5511811023622046335, 0.09757992244046803654 ) ) ;
#21681=CARTESIAN_POINT ( 'NONE',  ( 0.4986876640419954376, -0.6046776061558809534, -0.2411417322834644161 ) ) ;
#21683=CARTESIAN_POINT ( 'NONE',  ( 1.213910761154856299, -0.5511811023622048555, -0.09757992244046775898 ) ) ;
#21686=CARTESIAN_POINT ( 'NONE',  ( -1.213910761154854745, -0.5511811023622046335, 0.09757992244046803654 ) ) ;
#21687=CARTESIAN_POINT ( 'NONE',  ( -0.3871391076115476282, -0.05778040916215522460, 0.4822834645669289988 ) ) ;
#21688=CARTESIAN_POINT ( 'NONE',  ( 0.1181102362204730916, -0.6692913385826771977, 8.415575281601705876E-17 ) ) ;
#21689=CARTESIAN_POINT ( 'NONE',  ( -1.515748031496062076, 0.07958543189024071263, -0.2665933059059888421 ) ) ;
#21691=CARTESIAN_POINT ( 'NONE',  ( -1.358267716535432434, 0.1660481256975883668, -0.3530559997133364547 ) ) ;
#21692=CARTESIAN_POINT ( 'NONE',  ( 0.3083989501312343062, -0.05778040916215560624, -0.4822834645669293319 ) ) ;
#21693=CARTESIAN_POINT ( 'NONE',  ( -0.06561679790026180015, 0.05413385826771666132, 0.4176697321401328100 ) ) ;
#21694=CARTESIAN_POINT ( 'NONE',  ( 1.036745406824147508, -0.4281496062992127816, -0.4176697321401328100 ) ) ;
#21700=CARTESIAN_POINT ( 'NONE',  ( -0.006561679790025524116, -0.2845877964562159024, 0.3641732283464567677 ) ) ;
#21701=CARTESIAN_POINT ( 'NONE',  ( -0.3740157480314953431, -0.5400638737290845981, -0.3530559997133363437 ) ) ;
#21702=CARTESIAN_POINT ( 'NONE',  ( 0.9186351706036751663, -0.6046776061558807314, 0.2411417322834647770 ) ) ;
#21704=CARTESIAN_POINT ( 'NONE',  ( 0.1509186351706045259, -0.08942795157528024563, -0.3641732283464568787 ) ) ;
#21705=CARTESIAN_POINT ( 'NONE',  ( -1.286089238845143479, 0.2306618581243847221, -0.2411417322834647770 ) ) ;
#21706=CARTESIAN_POINT ( 'NONE',  ( 1.528871391076116026, -0.6692913385826773087, -0.1292274648535924053 ) ) ;
#21710=ORIENTED_EDGE ( 'NONE', *, *, #23233, .T. ) ;
#21711=CARTESIAN_POINT ( 'NONE',  ( 1.122047244094488860, 0.1660481256975885056, 0.3530559997133364547 ) ) ;
#21712=CARTESIAN_POINT ( 'NONE',  ( 1.502624671916010790, -0.2845877964562161244, -0.3641732283464567121 ) ) ;
#21713=CARTESIAN_POINT ( 'NONE',  ( -1.043307086614172041, -0.4536011799217367080, 0.2665933059059888421 ) ) ;
#21714=CARTESIAN_POINT ( 'NONE',  ( -0.9776902887139098386, 0.2952755905511810774, -0.1292274648535930714 ) ) ;
#21716=CARTESIAN_POINT ( 'NONE',  ( -1.603475055217291612, 1.267857067133556281, 0.04573490813648255215 ) ) ;
#21717=CARTESIAN_POINT ( 'NONE',  ( 1.397637795275591177, 0.1660481256975883668, -0.3530559997133364547 ) ) ;
#21718=CARTESIAN_POINT ( 'NONE',  ( -1.673228346456691717, 0.1660481256975883668, -0.3530559997133364547 ) ) ;
#21719=CARTESIAN_POINT ( 'NONE',  ( -0.02624671916010428221, -0.6046776061558807314, 0.2411417322834647770 ) ) ;
#21720=CARTESIAN_POINT ( 'NONE',  ( -0.3543307086614165824, -0.6692913385826771977, 8.415575281601705876E-17 ) ) ;
#21722=CARTESIAN_POINT ( 'NONE',  ( -1.279527559055116948, 0.1660481256975883668, -0.3530559997133364547 ) ) ;
#21724=CARTESIAN_POINT ( 'NONE',  ( 0.5380577427821529035, 0.05413385826771626580, -0.4176697321401330321 ) ) ;
#21726=CARTESIAN_POINT ( 'NONE',  ( -1.213910761154854745, -0.5511811023622046335, 0.09757992244046803654 ) ) ;
#21727=ORIENTED_EDGE ( 'NONE', *, *, #31689, .T. ) ;
#21729=ORIENTED_EDGE ( 'NONE', *, *, #20862, .T. ) ;
#21731=CARTESIAN_POINT ( 'NONE',  ( -1.633858267716534529, -0.5400638737290845981, -0.3530559997133363437 ) ) ;
#21732=CARTESIAN_POINT ( 'NONE',  ( 1.443569553805774897, 0.2306618581243848609, 0.2411417322834645549 ) ) ;
#21734=CARTESIAN_POINT ( 'NONE',  ( -1.502624671916009680, -0.05778040916215560624, -0.4822834645669293319 ) ) ;
#21735=CARTESIAN_POINT ( 'NONE',  ( -1.515748031496062076, 0.1660481256975883668, -0.3530559997133364547 ) ) ;
#21739=CARTESIAN_POINT ( 'NONE',  ( -0.3740157480314953431, 0.07958543189024085140, 0.2665933059059887866 ) ) ;
#21740=CARTESIAN_POINT ( 'NONE',  ( -0.8727034120734901146, -0.08942795157528024563, -0.3641732283464568787 ) ) ;
#21741=CARTESIAN_POINT ( 'NONE',  ( -1.187664041994749731, -0.3162353388693405765, 0.4822834645669290543 ) ) ;
#21742=CARTESIAN_POINT ( 'NONE',  ( 0.9317585301837276734, -0.4281496062992124485, 0.4176697321401328655 ) ) ;
#21743=CARTESIAN_POINT ( 'NONE',  ( -0.9645669291338575535, 0.1660481256975883668, -0.3530559997133364547 ) ) ;
#21746=CARTESIAN_POINT ( 'NONE',  ( -1.371391076115484609, -0.6692913385826771977, 0.1292274648535927661 ) ) ;
#21747=CARTESIAN_POINT ( 'NONE',  ( -1.358267716535432434, 0.07958543189024071263, -0.2665933059059888421 ) ) ;
#21754=CARTESIAN_POINT ( 'NONE',  ( -0.1771653543307080136, 0.1660481256975883668, -0.3530559997133364547 ) ) ;
#21755=CARTESIAN_POINT ( 'NONE',  ( 1.607611548556431069, -0.6692913385826773087, -0.1292274648535924053 ) ) ;
#21757=CARTESIAN_POINT ( 'NONE',  ( -1.555118110236219930, 0.1660481256975885056, 0.3530559997133364547 ) ) ;
#21758=CARTESIAN_POINT ( 'NONE',  ( -0.6430446194225712953, 0.009842519685039147898, -0.3409548833797004797 ) ) ;
#21759=CARTESIAN_POINT ( 'NONE',  ( -1.581364829396324945, -0.3162353388693405765, 0.4822834645669290543 ) ) ;
#21760=CARTESIAN_POINT ( 'NONE',  ( -0.4330708661417315697, 0.2952755905511811885, 0.000000000000000000 ) ) ;
#21762=CARTESIAN_POINT ( 'NONE',  ( 0.5577427821522314977, -0.2845877964562161244, -0.3641732283464567121 ) ) ;
#21764=CARTESIAN_POINT ( 'NONE',  ( 0.2165354330708668673, -0.4536011799217367080, 0.2665933059059888421 ) ) ;
#21765=CARTESIAN_POINT ( 'NONE',  ( 1.069553805774278610, -0.5511811023622046335, 0.09757992244046803654 ) ) ;
#21766=CARTESIAN_POINT ( 'NONE',  ( 1.082677165354331228, -0.5400638737290844871, 0.3530559997133364547 ) ) ;
#21768=CARTESIAN_POINT ( 'NONE',  ( -0.3215223097112853146, -0.08942795157528024563, -0.3641732283464568787 ) ) ;
#21770=CARTESIAN_POINT ( 'NONE',  ( -1.364829396325458521, -0.6046776061558807314, 0.2411417322834647770 ) ) ;
#21771=CARTESIAN_POINT ( 'NONE',  ( -0.1312335958005241554, 0.1283753931104748280, 0.1820866141732283561 ) ) ;
#21772=CARTESIAN_POINT ( 'NONE',  ( -1.135170603674539924, 0.1771653543307087075, -0.09757992244046823083 ) ) ;
#21774=CARTESIAN_POINT ( 'NONE',  ( -1.076115485564303809, -0.5023911411419708095, -0.1820866141732282451 ) ) ;
#21775=CARTESIAN_POINT ( 'NONE',  ( 8.195543980992789655E-16, -0.1870078740157480879, -0.4822834645669291653 ) ) ;
#21776=CARTESIAN_POINT ( 'NONE',  ( 1.660104986876641320, -0.08942795157527998196, 0.3641732283464567121 ) ) ;
#21777=CARTESIAN_POINT ( 'NONE',  ( 0.6167979002624678353, -0.3690944881889763329, 0.3153832671262228327 ) ) ;
#21778=CARTESIAN_POINT ( 'NONE',  ( -0.1049868766404193215, 0.1283753931104746893, -0.1820866141732285504 ) ) ;
#21779=CARTESIAN_POINT ( 'NONE',  ( -0.6692913385826764205, 0.2952755905511811885, 0.000000000000000000 ) ) ;
#21780=CARTESIAN_POINT ( 'NONE',  ( -1.640419947506561060, -0.4281496062992127816, -0.4176697321401328100 ) ) ;
#21781=CARTESIAN_POINT ( 'NONE',  ( -1.135170603674539924, 0.1771653543307087075, -0.09757992244046823083 ) ) ;
#21783=CARTESIAN_POINT ( 'NONE',  ( 0.5643044619422579178, 0.05413385826771666132, 0.4176697321401328100 ) ) ;
#21784=VERTEX_POINT ( 'NONE', #31345 ) ;
#21786=CARTESIAN_POINT ( 'NONE',  ( -0.3083989501312330295, -0.08942795157527998196, 0.3641732283464567121 ) ) ;
#21787=CARTESIAN_POINT ( 'NONE',  ( -0.08530183727034056085, -0.05778040916215560624, -0.4822834645669293319 ) ) ;
#21788=CARTESIAN_POINT ( 'NONE',  ( -1.640419947506561060, 0.05413385826771666132, 0.4176697321401328100 ) ) ;
#21789=CARTESIAN_POINT ( 'NONE',  ( -1.502624671916009680, -0.2845877964562159024, 0.3641732283464567677 ) ) ;
#21790=CARTESIAN_POINT ( 'NONE',  ( 1.515748031496063408, 0.1660481256975885056, 0.3530559997133364547 ) ) ;
#21791=CARTESIAN_POINT ( 'NONE',  ( -0.7808398950131225646, -0.08942795157527998196, 0.3641732283464567121 ) ) ;
#21792=CARTESIAN_POINT ( 'NONE',  ( -1.092023077763013772, -4.378520898609941727E-15, 0.4281989832122466977 ) ) ;
#21796=CARTESIAN_POINT ( 'NONE',  ( 0.9514435695538062676, -0.08942795157527998196, 0.3641732283464567121 ) ) ;
#21798=CARTESIAN_POINT ( 'NONE',  ( 0.8398950131233602345, 0.2306618581243847221, -0.2411417322834647770 ) ) ;
#21800=CARTESIAN_POINT ( 'NONE',  ( 1.358267716535433323, 0.07958543189024085140, 0.2665933059059887866 ) ) ;
#21802=CARTESIAN_POINT ( 'NONE',  ( 0.1968503937007881344, -0.6692913385826771977, 8.415575281601705876E-17 ) ) ;
#21803=CARTESIAN_POINT ( 'NONE',  ( -0.3280839895013117347, 0.05413385826771626580, -0.4176697321401330321 ) ) ;
#21804=CARTESIAN_POINT ( 'NONE',  ( 1.568241469816273659, -0.05778040916215560624, -0.4822834645669293319 ) ) ;
#21807=CARTESIAN_POINT ( 'NONE',  ( 0.1706036745406830368, -0.004921259842519576551, 0.3153832671262227771 ) ) ;
#21811=CARTESIAN_POINT ( 'NONE',  ( -0.5971128608923877978, 0.2952755905511811885, 0.1292274648535926551 ) ) ;
#21812=CARTESIAN_POINT ( 'NONE',  ( 1.489501312335958172, -0.05778040916215560624, -0.4822834645669293319 ) ) ;
#21813=CARTESIAN_POINT ( 'NONE',  ( 0.04593175853018440641, -0.6692913385826771977, 0.1292274648535927661 ) ) ;
#21814=CARTESIAN_POINT ( 'NONE',  ( -0.2296587926509179312, -0.08942795157527998196, 0.3641732283464567121 ) ) ;
#21815=CARTESIAN_POINT ( 'NONE',  ( 0.7283464566929143125, 0.1660481256975885056, 0.3530559997133364547 ) ) ;
#21816=CARTESIAN_POINT ( 'NONE',  ( -0.7611548556430438595, -0.6046776061558809534, -0.2411417322834644161 ) ) ;
#21818=CARTESIAN_POINT ( 'NONE',  ( -0.4658792650918627265, -0.05778040916215522460, 0.4822834645669289988 ) ) ;
#21819=CARTESIAN_POINT ( 'NONE',  ( -0.9383202099737524282, -0.05778040916215522460, 0.4822834645669289988 ) ) ;
#21820=CARTESIAN_POINT ( 'NONE',  ( 1.161417322834646271, 0.1660481256975883668, -0.3530559997133364547 ) ) ;
#21821=CIRCLE ( 'NONE', #28552, 2.362204724409449064 ) ;
#21822=CARTESIAN_POINT ( 'NONE',  ( 0.8202099737532813073, 0.2952755905511811885, 0.1292274648535926551 ) ) ;
#21823=CARTESIAN_POINT ( 'NONE',  ( 0.8923884514435703741, 0.2306618581243848609, 0.2411417322834645549 ) ) ;
#21825=CARTESIAN_POINT ( 'NONE',  ( 0.1706036745406830368, -0.3690944881889765550, -0.3153832671262227771 ) ) ;
#21829=CARTESIAN_POINT ( 'NONE',  ( -0.9908136482939626788, -0.5511811023622048555, -0.09757992244046775898 ) ) ;
#21830=CARTESIAN_POINT ( 'NONE',  ( -0.2362204724409440182, -0.1870078740157479769, 0.4822834645669291653 ) ) ;
#21831=DIRECTION ( 'NONE',  ( 0.7071067811865495711, -0.000000000000000000, -0.7071067811865454633 ) ) ;
#21832=CARTESIAN_POINT ( 'NONE',  ( -0.4265091863517051496, 0.2952755905511810774, -0.1292274648535930714 ) ) ;
#21833=CARTESIAN_POINT ( 'NONE',  ( -0.5774278215223089816, 0.2306618581243847221, -0.2411417322834647770 ) ) ;
#21834=CARTESIAN_POINT ( 'NONE',  ( -1.200787401574802349, -0.5400638737290844871, 0.3530559997133364547 ) ) ;
#21835=CARTESIAN_POINT ( 'NONE',  ( -1.325459317585300889, -0.4281496062992127816, -0.4176697321401328100 ) ) ;
#21836=CARTESIAN_POINT ( 'NONE',  ( 1.227034120734908917, 0.1771653543307087075, -0.09757992244046823083 ) ) ;
#21839=CARTESIAN_POINT ( 'NONE',  ( 0.5971128608923890191, -0.5511811023622046335, 0.09757992244046803654 ) ) ;
#21840=CARTESIAN_POINT ( 'NONE',  ( 0.1771653543307093182, -0.5400638737290845981, -0.3530559997133363437 ) ) ;
#21841=CARTESIAN_POINT ( 'NONE',  ( 0.2887139107611556010, 0.2306618581243847221, -0.2411417322834647770 ) ) ;
#21848=CARTESIAN_POINT ( 'NONE',  ( -0.3608923884514428360, -0.6692913385826773087, -0.1292274648535924053 ) ) ;
#21851=CARTESIAN_POINT ( 'NONE',  ( -1.528871391076114250, -0.5511811023622046335, 0.09757992244046803654 ) ) ;
#21852=CARTESIAN_POINT ( 'NONE',  ( 0.9514435695538062676, -0.05778040916215522460, 0.4822834645669289988 ) ) ;
#21853=CARTESIAN_POINT ( 'NONE',  ( 0.9973753280839902091, -0.6046776061558807314, 0.2411417322834647770 ) ) ;
#21854=CARTESIAN_POINT ( 'NONE',  ( -0.2493438320209966919, -0.3690944881889763329, 0.3153832671262228327 ) ) ;
#21855=CARTESIAN_POINT ( 'NONE',  ( 0.02624671916010564918, 0.2306618581243848609, 0.2411417322834645549 ) ) ;
#21857=CARTESIAN_POINT ( 'NONE',  ( -0.08530183727034056085, -0.2845877964562159024, 0.3641732283464567677 ) ) ;
#21858=CARTESIAN_POINT ( 'NONE',  ( -0.4790026246719154557, -0.3162353388693405765, 0.4822834645669290543 ) ) ;
#21860=CARTESIAN_POINT ( 'NONE',  ( -1.469816272965878357, -0.6046776061558809534, -0.2411417322834644161 ) ) ;
#21861=CARTESIAN_POINT ( 'NONE',  ( 0.1771653543307093182, 0.07958543189024085140, 0.2665933059059887866 ) ) ;
#21862=CARTESIAN_POINT ( 'NONE',  ( 1.653543307086614789, -0.1870078740157479769, 0.3641732283464567677 ) ) ;
#21863=CARTESIAN_POINT ( 'NONE',  ( -0.9448818897637790704, -0.1870078740157479769, 0.4822834645669291653 ) ) ;
#21864=CARTESIAN_POINT ( 'NONE',  ( -0.8661417322834640276, -0.1870078740157479769, 0.3641732283464567677 ) ) ;
#21865=CARTESIAN_POINT ( 'NONE',  ( -1.646051170424378096, -0.1870078740157480046, 1.254653134982923898E-17 ) ) ;
#21866=CARTESIAN_POINT ( 'NONE',  ( -1.128608923884513837, -0.6046776061558807314, 0.2411417322834647770 ) ) ;
#21867=CARTESIAN_POINT ( 'NONE',  ( -0.6496062992125976043, 0.1660481256975883668, -0.3530559997133364547 ) ) ;
#21868=CARTESIAN_POINT ( 'NONE',  ( 0.1837270341207357105, -0.6046776061558809534, -0.2411417322834644161 ) ) ;
#21872=CARTESIAN_POINT ( 'NONE',  ( 0.3215223097112867578, -0.2845877964562161244, -0.3641732283464567121 ) ) ;
#21873=CARTESIAN_POINT ( 'NONE',  ( 0.9383202099737536495, -0.3162353388693405765, 0.4822834645669290543 ) ) ;
#21874=CARTESIAN_POINT ( 'NONE',  ( -1.266404199475064773, -0.2845877964562159024, 0.3641732283464567677 ) ) ;
#21875=EDGE_CURVE ( 'NONE', #7209, #47808, #46707, .T. ) ;
#21876=CARTESIAN_POINT ( 'NONE',  ( 1.213910761154856299, 0.2952755905511811885, 0.1292274648535926551 ) ) ;
#21877=CARTESIAN_POINT ( 'NONE',  ( -1.653543307086613234, -0.1870078740157480601, -0.3641732283464567677 ) ) ;
#21879=CARTESIAN_POINT ( 'NONE',  ( -0.4396325459317579898, 0.2952755905511811885, 0.1292274648535926551 ) ) ;
#21880=CARTESIAN_POINT ( 'NONE',  ( 0.3083989501312343062, -0.08942795157528024563, -0.3641732283464568787 ) ) ;
#21882=CARTESIAN_POINT ( 'NONE',  ( 0.7677165354330716118, -0.4536011799217367080, 0.2665933059059888421 ) ) ;
#21884=CARTESIAN_POINT ( 'NONE',  ( 0.05249343832021075018, -0.6046776061558807314, 0.2411417322834647770 ) ) ;
#21886=CARTESIAN_POINT ( 'NONE',  ( -0.8530183727034112984, -0.4281496062992127816, -0.4176697321401328100 ) ) ;
#21888=CARTESIAN_POINT ( 'NONE',  ( 1.030183727034121421, -0.2845877964562161244, -0.3641732283464567121 ) ) ;
#21889=CARTESIAN_POINT ( 'NONE',  ( -0.03280839895013062252, 0.2952755905511810774, -0.1292274648535930714 ) ) ;
#21890=CARTESIAN_POINT ( 'NONE',  ( -0.1706036745406816491, 0.05413385826771626580, -0.4176697321401330321 ) ) ;
#21891=CARTESIAN_POINT ( 'NONE',  ( -0.2821522309711278487, -0.5511811023622048555, -0.09757992244046775898 ) ) ;
#21893=CARTESIAN_POINT ( 'NONE',  ( -0.6102362204724400829, -0.4536011799217368745, -0.2665933059059886201 ) ) ;
#21894=CARTESIAN_POINT ( 'NONE',  ( 0.3871391076115493490, -0.3162353388693405765, 0.4822834645669290543 ) ) ;
#21895=CARTESIAN_POINT ( 'NONE',  ( -0.5774278215223089816, 0.1283753931104746893, -0.1820866141732285504 ) ) ;
#21897=CARTESIAN_POINT ( 'NONE',  ( -1.207349081364828436, -0.6046776061558807314, 0.2411417322834647770 ) ) ;
#21900=CARTESIAN_POINT ( 'NONE',  ( -1.148293963254592542, -0.5511811023622048555, -0.09757992244046775898 ) ) ;
#21901=CARTESIAN_POINT ( 'NONE',  ( -0.01312335958005186876, -0.4281496062992124485, 0.4176697321401328655 ) ) ;
#21903=EDGE_CURVE ( 'NONE', #199, #35363, #5967, .T. ) ;
#21904=CARTESIAN_POINT ( 'NONE',  ( -1.482939632545930975, -0.4281496062992127816, -0.4176697321401328100 ) ) ;
#21905=CARTESIAN_POINT ( 'NONE',  ( -0.8136482939632537770, 0.2306618581243847221, -0.2411417322834647770 ) ) ;
#21907=CARTESIAN_POINT ( 'NONE',  ( 1.404199475065617708, 0.05413385826771626580, -0.4176697321401330321 ) ) ;
#21908=CARTESIAN_POINT ( 'NONE',  ( 0.8530183727034128527, -0.4281496062992124485, 0.4176697321401328655 ) ) ;
#21912=CARTESIAN_POINT ( 'NONE',  ( -1.653543307086613234, -0.1870078740157480879, -0.4822834645669291653 ) ) ;
#21915=EDGE_CURVE ( 'NONE', #37974, #57515, #34926, .T. ) ;
#21916=CARTESIAN_POINT ( 'NONE',  ( -0.5905511811023613777, -0.5511811023622047445, 6.969142054262312111E-17 ) ) ;
#21919=CARTESIAN_POINT ( 'NONE',  ( 1.003937007874016185, 0.1660481256975883668, -0.3530559997133364547 ) ) ;
#21920=CARTESIAN_POINT ( 'NONE',  ( 0.2034120734908142214, 0.2952755905511810774, -0.1292274648535930714 ) ) ;
#21921=CARTESIAN_POINT ( 'NONE',  ( -0.5052493438320203589, 0.2952755905511810774, -0.1292274648535930714 ) ) ;
#21922=CARTESIAN_POINT ( 'NONE',  ( 1.522309711286089939, 0.2306618581243848609, 0.2411417322834645549 ) ) ;
#21924=CARTESIAN_POINT ( 'NONE',  ( -1.482939632545930975, -0.004921259842519576551, 0.3153832671262227771 ) ) ;
#21926=CARTESIAN_POINT ( 'NONE',  ( 0.3740157480314966754, -0.5400638737290844871, 0.3530559997133364547 ) ) ;
#21927=CARTESIAN_POINT ( 'NONE',  ( 0.7020997375328090762, -0.08942795157528024563, -0.3641732283464568787 ) ) ;
#21928=CARTESIAN_POINT ( 'NONE',  ( -0.6692913385826764205, 0.2952755905511811885, 0.000000000000000000 ) ) ;
#21930=CARTESIAN_POINT ( 'NONE',  ( -1.148293963254592542, 0.2952755905511811885, 0.1292274648535926551 ) ) ;
#21931=CARTESIAN_POINT ( 'NONE',  ( -1.673228346456691717, 0.07958543189024071263, -0.2665933059059888421 ) ) ;
#21933=CARTESIAN_POINT ( 'NONE',  ( 0.9842519685039378130, -0.6692913385826771977, 8.415575281601705876E-17 ) ) ;
#21934=CARTESIAN_POINT ( 'NONE',  ( 1.371391076115485941, 0.1771653543307087630, 0.09757992244046791164 ) ) ;
#21935=ORIENTED_EDGE ( 'NONE', *, *, #55786, .T. ) ;
#21937=CARTESIAN_POINT ( 'NONE',  ( -0.5511811023622038563, -0.1870078740157479769, 0.4822834645669291653 ) ) ;
#21938=ORIENTED_EDGE ( 'NONE', *, *, #45519, .T. ) ;
#21939=CARTESIAN_POINT ( 'NONE',  ( 0.2887139107611556010, -0.5023911411419708095, 0.1820866141732285504 ) ) ;
#21940=CARTESIAN_POINT ( 'NONE',  ( -1.049868766404198794, 0.2306618581243847221, -0.2411417322834647770 ) ) ;
#21941=CARTESIAN_POINT ( 'NONE',  ( 0.9448818897637802916, -0.1870078740157479769, 0.4822834645669291653 ) ) ;
#21942=CARTESIAN_POINT ( 'NONE',  ( 1.010498687664042716, 0.05413385826771626580, -0.4176697321401330321 ) ) ;
#21943=CARTESIAN_POINT ( 'NONE',  ( -0.1049868766404193215, 0.2306618581243847221, -0.2411417322834647770 ) ) ;
#21945=CARTESIAN_POINT ( 'NONE',  ( -0.2427821522309703550, -0.3162353388693405765, 0.4822834645669290543 ) ) ;
#21947=CARTESIAN_POINT ( 'NONE',  ( 1.601049868766404982, 0.1283753931104748280, 0.1820866141732283561 ) ) ;
#21948=CARTESIAN_POINT ( 'NONE',  ( -0.5774278215223089816, -0.6046776061558807314, 0.2411417322834647770 ) ) ;
#21949=CARTESIAN_POINT ( 'NONE',  ( -0.4133858267716528645, -0.4536011799217367080, 0.2665933059059888421 ) ) ;
#21950=CARTESIAN_POINT ( 'NONE',  ( 1.496062992125985147, -0.1870078740157479769, 0.4822834645669291653 ) ) ;
#21951=CARTESIAN_POINT ( 'NONE',  ( 1.450131233595801428, -0.6692913385826773087, -0.1292274648535924053 ) ) ;
#21952=CARTESIAN_POINT ( 'NONE',  ( -0.7677165354330699465, 0.1660481256975885056, 0.3530559997133364547 ) ) ;
#21954=CARTESIAN_POINT ( 'NONE',  ( 0.7283464566929140904, -0.5400638737290845981, -0.3530559997133363437 ) ) ;
#21957=CARTESIAN_POINT ( 'NONE',  ( -0.3018372703412066094, -0.4281496062992127816, -0.4176697321401328100 ) ) ;
#21958=CARTESIAN_POINT ( 'NONE',  ( -1.161417322834644716, 0.07958543189024085140, 0.2665933059059887866 ) ) ;
#21959=CARTESIAN_POINT ( 'NONE',  ( 1.043307086614173818, 0.07958543189024085140, 0.2665933059059887866 ) ) ;
#21961=CARTESIAN_POINT ( 'NONE',  ( 1.115485564304462551, -0.3690944881889765550, -0.3153832671262227771 ) ) ;
#21962=CARTESIAN_POINT ( 'NONE',  ( 0.8530183727034126306, 0.05413385826771626580, -0.4176697321401330321 ) ) ;
#21964=CARTESIAN_POINT ( 'NONE',  ( -0.2230971128608915943, -0.4281496062992127816, -0.4176697321401328100 ) ) ;
#21966=CARTESIAN_POINT ( 'NONE',  ( 1.266404199475066328, -0.08942795157527998196, 0.3641732283464567121 ) ) ;
#21967=CARTESIAN_POINT ( 'NONE',  ( -0.3871391076115479057, -0.3162353388693409650, -0.4822834645669289433 ) ) ;
#21969=CARTESIAN_POINT ( 'NONE',  ( 1.437007874015748810, -0.5400638737290845981, -0.3530559997133363437 ) ) ;
#21970=CARTESIAN_POINT ( 'NONE',  ( 0.1049868766404206816, -0.6046776061558809534, -0.2411417322834644161 ) ) ;
#21971=CARTESIAN_POINT ( 'NONE',  ( 0.4265091863517067594, 0.1771653543307087630, 0.09757992244046791164 ) ) ;
#21973=CARTESIAN_POINT ( 'NONE',  ( 0.3608923884514443348, -0.5511811023622046335, 0.09757992244046803654 ) ) ;
#21974=CARTESIAN_POINT ( 'NONE',  ( -1.541994750656167090, -0.6692913385826773087, -0.1292274648535924053 ) ) ;
#21976=CARTESIAN_POINT ( 'NONE',  ( 0.8070866141732289112, -0.5400638737290845981, -0.3530559997133363437 ) ) ;
#21978=CARTESIAN_POINT ( 'NONE',  ( 1.574803149606299746, -0.1870078740157480601, -0.3641732283464567677 ) ) ;
#21980=CARTESIAN_POINT ( 'NONE',  ( 0.01312335958005323398, -0.004921259842519576551, 0.3153832671262227771 ) ) ;
#21982=CARTESIAN_POINT ( 'NONE',  ( 0.1246719160104994284, 0.2952755905511810774, -0.1292274648535930714 ) ) ;
#21983=CARTESIAN_POINT ( 'NONE',  ( 1.528871391076116026, 0.1771653543307087630, 0.09757992244046791164 ) ) ;
#21984=CARTESIAN_POINT ( 'NONE',  ( -1.345144356955379816, -0.08942795157528024563, -0.3641732283464568787 ) ) ;
#21985=CARTESIAN_POINT ( 'NONE',  ( -1.646981627296586703, -0.3162353388693409650, -0.4822834645669289433 ) ) ;
#21987=CARTESIAN_POINT ( 'NONE',  ( 0.5643044619422579178, 0.05413385826771666132, 0.4176697321401328100 ) ) ;
#21988=CARTESIAN_POINT ( 'NONE',  ( -1.620734908136482577, 0.1771653543307087630, 0.09757992244046791164 ) ) ;
#21989=CARTESIAN_POINT ( 'NONE',  ( 1.586052503253845281, 1.299212598425198095, -0.1653254495020587411 ) ) ;
#21990=CARTESIAN_POINT ( 'NONE',  ( 0.7283464566929140904, -0.5400638737290845981, -0.3530559997133363437 ) ) ;
#21991=CARTESIAN_POINT ( 'NONE',  ( 1.194225721784777594, 0.05413385826771666132, 0.4176697321401328100 ) ) ;
#21992=CARTESIAN_POINT ( 'NONE',  ( 1.174540682414699111, -0.3162353388693405765, 0.4822834645669290543 ) ) ;
#21994=CARTESIAN_POINT ( 'NONE',  ( 1.115485564304462551, -0.3690944881889765550, -0.3153832671262227771 ) ) ;
#21995=CARTESIAN_POINT ( 'NONE',  ( -1.568241469816272105, -0.2845877964562161244, -0.3641732283464567121 ) ) ;
#21996=CARTESIAN_POINT ( 'NONE',  ( -0.7874015748031489847, -0.1870078740157480601, -0.3641732283464567677 ) ) ;
#21997=CARTESIAN_POINT ( 'NONE',  ( 1.220472440944881942, 1.496062992125984037, -0.5309055118110238558 ) ) ;
#21998=CARTESIAN_POINT ( 'NONE',  ( 0.6102362204724416372, -0.4536011799217367080, 0.2665933059059888421 ) ) ;
#21999=CIRCLE ( 'NONE', #75772, 3.543307086614173151 ) ;
#22000=CARTESIAN_POINT ( 'NONE',  ( 0.2952755905511819101, 0.1660481256975883668, -0.3530559997133364547 ) ) ;
#22001=CARTESIAN_POINT ( 'NONE',  ( 0.8005249343832027131, 0.05413385826771666132, 0.4176697321401328100 ) ) ;
#22002=CARTESIAN_POINT ( 'NONE',  ( -0.4527559055118102749, -0.5400638737290845981, -0.3530559997133363437 ) ) ;
#22003=CARTESIAN_POINT ( 'NONE',  ( 0.1509186351706042484, -0.2845877964562159024, 0.3641732283464567677 ) ) ;
#22004=CARTESIAN_POINT ( 'NONE',  ( 1.338582677165355062, -0.1870078740157480879, -0.4822834645669291653 ) ) ;
#22005=CARTESIAN_POINT ( 'NONE',  ( -1.614173228346456712, 2.401574803149606474, -0.1372047244094478091 ) ) ;
#22006=CARTESIAN_POINT ( 'NONE',  ( -0.9842519685039365918, -0.6692913385826771977, 8.415575281601705876E-17 ) ) ;
#22010=CARTESIAN_POINT ( 'NONE',  ( -0.6496062992125976043, 0.1660481256975883668, -0.3530559997133364547 ) ) ;
#22011=CARTESIAN_POINT ( 'NONE',  ( -0.5839895013123351797, 0.2952755905511810774, -0.1292274648535930714 ) ) ;
#22015=CARTESIAN_POINT ( 'NONE',  ( 0.9186351706036752773, 0.1283753931104746893, -0.1820866141732285504 ) ) ;
#22017=CARTESIAN_POINT ( 'NONE',  ( 1.017060367454068581, -0.05778040916215560624, -0.4822834645669293319 ) ) ;
#22018=CARTESIAN_POINT ( 'NONE',  ( 0.5027385518326215053, 1.496062992125283708, 0.5309055118110234117 ) ) ;
#22019=CARTESIAN_POINT ( 'NONE',  ( -1.233595800524933894, 0.1283753931104748280, 0.1820866141732283561 ) ) ;
#22020=CARTESIAN_POINT ( 'NONE',  ( 1.417322834645670104, -0.1870078740157480879, -0.4822834645669291653 ) ) ;
#22021=CARTESIAN_POINT ( 'NONE',  ( -1.482939632545930975, -0.4281496062992127816, -0.4176697321401328100 ) ) ;
#22023=CARTESIAN_POINT ( 'NONE',  ( 0.1574803149606306130, -0.1870078740157480879, -0.4822834645669291653 ) ) ;
#22024=CARTESIAN_POINT ( 'NONE',  ( -0.3740157480314953431, -0.4536011799217368745, -0.2665933059059886201 ) ) ;
#22025=CARTESIAN_POINT ( 'NONE',  ( 0.9448818897637802916, -0.1870078740157479769, 0.4822834645669291653 ) ) ;
#22026=CARTESIAN_POINT ( 'NONE',  ( -0.1771653543307080136, -0.5400638737290844871, 0.3530559997133364547 ) ) ;
#22030=CARTESIAN_POINT ( 'NONE',  ( 0.7808398950131241190, -0.05778040916215560624, -0.4822834645669293319 ) ) ;
#22031=CARTESIAN_POINT ( 'NONE',  ( 0.03280839895013198948, 0.2952755905511811885, 0.1292274648535926551 ) ) ;
#22032=CARTESIAN_POINT ( 'NONE',  ( -1.023622047244093558, -0.1870078740157479769, 0.4822834645669291653 ) ) ;
#22033=CARTESIAN_POINT ( 'NONE',  ( 1.089238845144357537, -0.4281496062992124485, 0.4176697321401328655 ) ) ;
#22035=CARTESIAN_POINT ( 'NONE',  ( 0.9514435695538062676, -0.3162353388693409650, -0.4822834645669289433 ) ) ;
#22037=CARTESIAN_POINT ( 'NONE',  ( -0.1640419947506555343, -0.3162353388693405765, 0.4822834645669290543 ) ) ;
#22038=CARTESIAN_POINT ( 'NONE',  ( 0.6955380577427828781, -0.4281496062992124485, 0.4176697321401328655 ) ) ;
#22039=CARTESIAN_POINT ( 'NONE',  ( -0.1771653543307080136, 0.1660481256975883668, -0.3530559997133364547 ) ) ;
#22040=CARTESIAN_POINT ( 'NONE',  ( 0.7480314960629927956, 0.1771653543307087630, 0.000000000000000000 ) ) ;
#22041=CARTESIAN_POINT ( 'NONE',  ( -1.259842519685038686, -0.1870078740157479769, 0.4822834645669291653 ) ) ;
#22042=CARTESIAN_POINT ( 'NONE',  ( -1.640419947506561060, -0.4281496062992127816, -0.4176697321401328100 ) ) ;
#22043=CARTESIAN_POINT ( 'NONE',  ( 0.1640419947506569498, -0.05778040916215522460, 0.4822834645669289988 ) ) ;
#22046=ORIENTED_EDGE ( 'NONE', *, *, #64557, .F. ) ;
#22048=CARTESIAN_POINT ( 'NONE',  ( 1.069553805774278832, 0.2952755905511810774, -0.1292274648535930714 ) ) ;
#22049=CARTESIAN_POINT ( 'NONE',  ( 0.7349081364829402885, -0.5023911411419708095, -0.1820866141732282451 ) ) ;
#22055=CARTESIAN_POINT ( 'NONE',  ( -0.8727034120734901146, -0.3162353388693405765, 0.4822834645669290543 ) ) ;
#22056=CARTESIAN_POINT ( 'NONE',  ( -0.6561679790026240244, -0.6046776061558807314, 0.2411417322834647770 ) ) ;
#22057=CARTESIAN_POINT ( 'NONE',  ( 1.141732283464567566, 0.2952755905511811885, 0.000000000000000000 ) ) ;
#22059=CARTESIAN_POINT ( 'NONE',  ( 1.594488188976378673, 0.1660481256975885056, 0.3530559997133364547 ) ) ;
#22062=CARTESIAN_POINT ( 'NONE',  ( 1.581364829396326277, -0.2845877964562161244, -0.3641732283464567121 ) ) ;
#22063=B_SPLINE_CURVE_WITH_KNOTS ( 'NONE', 3,
 ( #28446, #47795, #54523, #42308, #73912, #3612, #15847 ),
 .UNSPECIFIED., .F., .F.,
 ( 4, 3, 4 ),
 ( 7.703719777548943412E-34, 0.001246232571205256601, 0.002492492258783256774 ),
 .UNSPECIFIED. ) ;
#22065=CARTESIAN_POINT ( 'NONE',  ( -1.456692913385826182, 0.1771653543307087630, 0.000000000000000000 ) ) ;
#22067=CARTESIAN_POINT ( 'NONE',  ( 0.2362204724409456558, -0.1870078740157479769, 0.4822834645669291653 ) ) ;
#22068=CARTESIAN_POINT ( 'NONE',  ( -0.4824498642376744417, -2.567464376874931580E-15, -0.4445507791589072832 ) ) ;
#22070=CARTESIAN_POINT ( 'NONE',  ( -0.9514435695538050464, -0.2845877964562159024, 0.3641732283464567677 ) ) ;
#22071=CARTESIAN_POINT ( 'NONE',  ( 0.6036745406824154392, 0.2306618581243847221, -0.2411417322834647770 ) ) ;
#22072=CARTESIAN_POINT ( 'NONE',  ( 1.456692913385827515, 0.1771653543307087630, 0.000000000000000000 ) ) ;
#22075=CARTESIAN_POINT ( 'NONE',  ( -0.8267716535433065062, -0.5511811023622047445, 6.969142054262312111E-17 ) ) ;
#22076=CARTESIAN_POINT ( 'NONE',  ( 1.161417322834646493, -0.5400638737290844871, 0.3530559997133364547 ) ) ;
#22078=CARTESIAN_POINT ( 'NONE',  ( -0.3412073490813641308, -0.6046776061558807314, 0.2411417322834647770 ) ) ;
#22079=CARTESIAN_POINT ( 'NONE',  ( -1.128608923884513837, 0.1283753931104746893, -0.1820866141732285504 ) ) ;
#22080=CARTESIAN_POINT ( 'NONE',  ( -0.4658792650918627265, -0.08942795157527998196, 0.3641732283464567121 ) ) ;
#22081=CARTESIAN_POINT ( 'NONE',  ( -0.4396325459317579898, 0.2952755905511811885, 0.1292274648535926551 ) ) ;
#22082=CARTESIAN_POINT ( 'NONE',  ( 1.640419947506562393, -0.4281496062992124485, 0.4176697321401328655 ) ) ;
#22084=CARTESIAN_POINT ( 'NONE',  ( 0.4002624671916016896, -0.3162353388693409650, -0.4822834645669289433 ) ) ;
#22087=CARTESIAN_POINT ( 'NONE',  ( -0.8202099737532801971, -0.6692913385826771977, 0.1292274648535927661 ) ) ;
#22088=CARTESIAN_POINT ( 'NONE',  ( -0.1049868766404193215, 0.1283753931104746893, -0.1820866141732285504 ) ) ;
#22089=CARTESIAN_POINT ( 'NONE',  ( -1.528871391076114250, -0.6692913385826771977, 0.1292274648535927661 ) ) ;
#22090=CARTESIAN_POINT ( 'NONE',  ( 0.2165354330708668673, -0.5400638737290844871, 0.3530559997133364547 ) ) ;
#22091=CARTESIAN_POINT ( 'NONE',  ( 0.2755905511811031494, 0.1771653543307087630, 0.000000000000000000 ) ) ;
#22092=CARTESIAN_POINT ( 'NONE',  ( -0.8267716535433065062, -0.5511811023622047445, 6.969142054262312111E-17 ) ) ;
#22093=CARTESIAN_POINT ( 'NONE',  ( -0.9973753280839886548, -0.6046776061558809534, -0.2411417322834644161 ) ) ;
#22094=CARTESIAN_POINT ( 'NONE',  ( -1.384514435695537005, 0.2952755905511811885, 0.1292274648535926551 ) ) ;
#22095=CARTESIAN_POINT ( 'NONE',  ( 1.174540682414699111, -0.3162353388693405765, 0.4822834645669290543 ) ) ;
#22097=CARTESIAN_POINT ( 'NONE',  ( 0.8661417322834653598, -0.1870078740157479769, 0.3641732283464567677 ) ) ;
#22098=AXIS2_PLACEMENT_3D ( 'NONE', #9136, #2406, #28064 ) ;
#22099=CARTESIAN_POINT ( 'NONE',  ( 0.8595800524934390507, -0.3162353388693405765, 0.4822834645669290543 ) ) ;
#22101=CARTESIAN_POINT ( 'NONE',  ( 1.351706036745407458, -0.3690944881889765550, -0.3153832671262227771 ) ) ;
#22103=CARTESIAN_POINT ( 'NONE',  ( -0.6233595800524928121, -0.3162353388693409650, -0.4822834645669289433 ) ) ;
#22105=CARTESIAN_POINT ( 'NONE',  ( -1.358267716535432434, -0.4536011799217367080, 0.2665933059059888421 ) ) ;
#22106=CARTESIAN_POINT ( 'NONE',  ( -0.5708661417322825615, -0.5400638737290844871, 0.3530559997133364547 ) ) ;
#22107=CARTESIAN_POINT ( 'NONE',  ( 0.2362204724409456558, -0.1870078740157480879, -0.4822834645669291653 ) ) ;
#22108=CARTESIAN_POINT ( 'NONE',  ( -1.627296587926508442, -0.5023911411419708095, -0.1820866141732282451 ) ) ;
#22110=CARTESIAN_POINT ( 'NONE',  ( -1.345144356955379816, -0.05778040916215560624, -0.4822834645669293319 ) ) ;
#22111=CARTESIAN_POINT ( 'NONE',  ( 0.4133858267716541968, 0.1660481256975885056, 0.3530559997133364547 ) ) ;
#22112=CARTESIAN_POINT ( 'NONE',  ( -0.1246719160104980823, -0.6692913385826773087, -0.1292274648535924053 ) ) ;
#22113=CARTESIAN_POINT ( 'NONE',  ( 1.161417322834646271, 0.1660481256975883668, -0.3530559997133364547 ) ) ;
#22120=CARTESIAN_POINT ( 'NONE',  ( -0.1902887139107604098, -0.5511811023622046335, 0.09757992244046803654 ) ) ;
#22121=CARTESIAN_POINT ( 'NONE',  ( -0.1968503937007867743, -0.6692913385826771977, 8.415575281601705876E-17 ) ) ;
#22122=CARTESIAN_POINT ( 'NONE',  ( 0.7939632545931766261, -0.05778040916215522460, 0.4822834645669289988 ) ) ;
#22124=CARTESIAN_POINT ( 'NONE',  ( 0.03937007874015833325, -0.5511811023622047445, 6.969142054262312111E-17 ) ) ;
#22125=( BOUNDED_CURVE ( )  B_SPLINE_CURVE ( 2, ( #39081, #64344, #378, #5846, #82471, #37838, #18895, #45385, #32771, #24786, #50455, #44544, #6680 ),
 .UNSPECIFIED., .F., .F. ) 
 B_SPLINE_CURVE_WITH_KNOTS ( ( 3, 2, 2, 2, 2, 2, 3 ),
 ( 0.6733310946348007864, 0.6742424242424241987, 0.6780303030303029832, 0.6818181818181817677, 0.6856060606060605522, 0.6893939393939394478, 0.6903052690015629711 ),
 .UNSPECIFIED. ) 
 CURVE ( )  GEOMETRIC_REPRESENTATION_ITEM ( )  RATIONAL_B_SPLINE_CURVE ( ( 0.9875488213027523443, 0.9918020599134680371, 1.000000000000000000, 0.9659258262890683122, 1.000000000000000000, 0.9659258262890683122, 1.000000000000000000, 0.9659258262890683122, 1.000000000000000000, 0.9659258262890683122, 1.000000000000000000, 0.9918020599134671489, 0.9875488213027514561 ) ) 
 REPRESENTATION_ITEM ( '' )  );
#22126=CARTESIAN_POINT ( 'NONE',  ( -1.187664041994749731, -0.3162353388693405765, 0.4822834645669290543 ) ) ;
#22127=CARTESIAN_POINT ( 'NONE',  ( 1.122047244094488860, 0.1660481256975885056, 0.3530559997133364547 ) ) ;
#22129=CARTESIAN_POINT ( 'NONE',  ( 0.4848199769444405671, 1.968301573707853303, 0.4917377963708856048 ) ) ;
#22130=ORIENTED_EDGE ( 'NONE', *, *, #37699, .T. ) ;
#22132=CARTESIAN_POINT ( 'NONE',  ( 1.056430446194226436, -0.6692913385826773087, -0.1292274648535924053 ) ) ;
#22133=CARTESIAN_POINT ( 'NONE',  ( -1.568241469816272105, -0.05778040916215522460, 0.4822834645669289988 ) ) ;
#22134=CARTESIAN_POINT ( 'NONE',  ( -1.135170603674539924, 0.1771653543307087075, -0.09757992244046823083 ) ) ;
#22135=CARTESIAN_POINT ( 'NONE',  ( -1.207349081364828436, -0.6046776061558807314, 0.2411417322834647770 ) ) ;
#22138=CARTESIAN_POINT ( 'NONE',  ( 1.207349081364829990, 0.2306618581243848609, 0.2411417322834645549 ) ) ;
#22139=CARTESIAN_POINT ( 'NONE',  ( -1.601049868766403650, -0.6046776061558807314, 0.2411417322834647770 ) ) ;
#22140=CARTESIAN_POINT ( 'NONE',  ( -0.1181102362204717315, 0.2952755905511811885, 0.000000000000000000 ) ) ;
#22141=CARTESIAN_POINT ( 'NONE',  ( 0.03937007874015806264, 0.2952755905511811885, 0.000000000000000000 ) ) ;
#22142=CARTESIAN_POINT ( 'NONE',  ( -1.417322834645668772, -0.1870078740157480879, -0.4822834645669291653 ) ) ;
#22143=B_SPLINE_CURVE_WITH_KNOTS ( 'NONE', 3,
 ( #25452, #25040, #6105, #70492 ),
 .UNSPECIFIED., .F., .F.,
 ( 4, 4 ),
 ( 3.593986969187450165E-07, 0.001287825409103224641 ),
 .UNSPECIFIED. ) ;
#22145=CARTESIAN_POINT ( 'NONE',  ( 0.1574803149606306130, -0.1870078740157479769, 0.4822834645669291653 ) ) ;
#22147=CARTESIAN_POINT ( 'NONE',  ( -1.312335958005248715, 0.1283753931104748280, 0.1820866141732283561 ) ) ;
#22150=ORIENTED_EDGE ( 'NONE', *, *, #34100, .F. ) ;
#22152=CARTESIAN_POINT ( 'NONE',  ( -1.660104986876639543, -0.05778040916215560624, -0.4822834645669293319 ) ) ;
#22154=CARTESIAN_POINT ( 'NONE',  ( -1.463254593175852492, -0.6692913385826773087, -0.1292274648535924053 ) ) ;
#22157=CARTESIAN_POINT ( 'NONE',  ( -1.572991167713776672, 2.401574803149606474, 0.1227090857360981641 ) ) ;
#22159=CARTESIAN_POINT ( 'NONE',  ( -0.4330708661417315697, -0.5511811023622047445, 6.969142054262312111E-17 ) ) ;
#22160=CARTESIAN_POINT ( 'NONE',  ( -0.7414698162729651543, 0.1771653543307087075, -0.09757992244046823083 ) ) ;
#22162=CARTESIAN_POINT ( 'NONE',  ( -1.181102362204723644, -0.1870078740157479769, 0.4822834645669291653 ) ) ;
#22163=CARTESIAN_POINT ( 'NONE',  ( 0.4658792650918640033, -0.3162353388693405765, 0.4822834645669290543 ) ) ;
#22164=CARTESIAN_POINT ( 'NONE',  ( -0.7611548556430438595, -0.6046776061558809534, -0.2411417322834644161 ) ) ;
#22167=CARTESIAN_POINT ( 'NONE',  ( -1.568241469816272105, -0.3162353388693409650, -0.4822834645669289433 ) ) ;
#22171=EDGE_CURVE ( 'NONE', #949, #30946, #50495, .T. ) ;
#22174=CARTESIAN_POINT ( 'NONE',  ( -0.7939632545931750718, -0.05778040916215560624, -0.4822834645669293319 ) ) ;
#22175=CARTESIAN_POINT ( 'NONE',  ( 1.489501312335958172, -0.3162353388693405765, 0.4822834645669290543 ) ) ;
#22179=CARTESIAN_POINT ( 'NONE',  ( -1.437007874015747477, -0.5400638737290844871, 0.3530559997133364547 ) ) ;
#22180=CARTESIAN_POINT ( 'NONE',  ( -0.6955380577427815458, -0.4281496062992127816, -0.4176697321401328100 ) ) ;
#22183=CARTESIAN_POINT ( 'NONE',  ( 0.3805774278215230400, -0.004921259842519870586, -0.3153832671262229437 ) ) ;
#22185=CARTESIAN_POINT ( 'NONE',  ( 0.1968503937007881344, -0.5511811023622047445, 6.969142054262312111E-17 ) ) ;
#22186=CARTESIAN_POINT ( 'NONE',  ( 1.115485564304462551, -0.004921259842519576551, 0.3153832671262227771 ) ) ;
#22187=CARTESIAN_POINT ( 'NONE',  ( 1.128608923884514947, 0.2306618581243848609, 0.2411417322834645549 ) ) ;
#22188=CARTESIAN_POINT ( 'NONE',  ( -0.09842519685039295696, -0.4536011799217367080, 0.2665933059059888421 ) ) ;
#22190=CARTESIAN_POINT ( 'NONE',  ( 1.437007874015748810, 0.1660481256975885056, 0.3530559997133364547 ) ) ;
#22192=CARTESIAN_POINT ( 'NONE',  ( -1.095800524934382292, -0.2845877964562161244, -0.3641732283464567121 ) ) ;
#22194=CARTESIAN_POINT ( 'NONE',  ( -1.017060367454067249, -0.08942795157527998196, 0.3641732283464567121 ) ) ;
#22195=CARTESIAN_POINT ( 'NONE',  ( 0.03937007874015833325, -0.6692913385826771977, 8.415575281601705876E-17 ) ) ;
#22196=CARTESIAN_POINT ( 'NONE',  ( 1.522309711286089939, 0.1283753931104748280, 0.1820866141732283561 ) ) ;
#22197=CARTESIAN_POINT ( 'NONE',  ( 0.4199475065616803948, -0.5023911411419708095, -0.1820866141732282451 ) ) ;
#22198=CARTESIAN_POINT ( 'NONE',  ( -0.3937007874015740483, -0.1870078740157480601, -0.3641732283464567677 ) ) ;
#22200=CARTESIAN_POINT ( 'NONE',  ( -0.5971128608923877978, -0.6692913385826773087, -0.1292274648535924053 ) ) ;
#22202=CARTESIAN_POINT ( 'NONE',  ( 2.795275590551181466, 1.968503937007874960, 0.000000000000000000 ) ) ;
#22203=CARTESIAN_POINT ( 'NONE',  ( 0.2296587926509192634, -0.3162353388693405765, 0.4822834645669290543 ) ) ;
#22205=CARTESIAN_POINT ( 'NONE',  ( 1.528871391076116026, -0.6692913385826773087, -0.1292274648535924053 ) ) ;
#22206=CARTESIAN_POINT ( 'NONE',  ( -0.07874015748031421014, -0.1870078740157480601, -0.3641732283464567677 ) ) ;
#22207=CARTESIAN_POINT ( 'NONE',  ( -0.1706036745406816491, -0.4281496062992124485, 0.4176697321401328655 ) ) ;
#22208=CARTESIAN_POINT ( 'NONE',  ( -1.391076115485563314, -0.6046776061558809534, -0.2411417322834644161 ) ) ;
#22209=CARTESIAN_POINT ( 'NONE',  ( -1.443569553805773564, 0.1283753931104746893, -0.1820866141732285504 ) ) ;
#22210=CARTESIAN_POINT ( 'NONE',  ( 1.128608923884515169, -0.6046776061558809534, -0.2411417322834644161 ) ) ;
#22211=CARTESIAN_POINT ( 'NONE',  ( -0.7545931758530177724, 0.1771653543307087630, 0.09757992244046791164 ) ) ;
#22215=CARTESIAN_POINT ( 'NONE',  ( -1.456692913385826182, -0.6692913385826771977, 8.415575281601705876E-17 ) ) ;
#22216=CARTESIAN_POINT ( 'NONE',  ( 1.555118110236221041, 0.07958543189024071263, -0.2665933059059888421 ) ) ;
#22217=CARTESIAN_POINT ( 'NONE',  ( 1.246719160104987623, -0.3690944881889763329, 0.3153832671262228327 ) ) ;
#22218=CARTESIAN_POINT ( 'NONE',  ( -1.594488188976377563, -0.5400638737290844871, 0.3530559997133364547 ) ) ;
#22219=CARTESIAN_POINT ( 'NONE',  ( 0.7808398950131240079, -0.3162353388693405765, 0.4822834645669290543 ) ) ;
#22221=CARTESIAN_POINT ( 'NONE',  ( 1.391076115485564868, 0.1283753931104746893, -0.1820866141732285504 ) ) ;
#22222=CARTESIAN_POINT ( 'NONE',  ( 0.05905511811023709395, -0.5400638737290844871, 0.3530559997133364547 ) ) ;
#22223=CARTESIAN_POINT ( 'NONE',  ( -0.3215223097112853146, -0.05778040916215560624, -0.4822834645669293319 ) ) ;
#22224=CARTESIAN_POINT ( 'NONE',  ( 1.653543307086614789, -0.1870078740157479769, 0.4822834645669291653 ) ) ;
#22228=CARTESIAN_POINT ( 'NONE',  ( 0.1574803149606306130, -0.1870078740157479769, 0.3641732283464567677 ) ) ;
#22231=EDGE_LOOP ( 'NONE', ( #15841, #21729, #58267, #83206 ) ) ;
#22232=CARTESIAN_POINT ( 'NONE',  ( -0.3740157480314953431, -0.5400638737290845981, -0.3530559997133363437 ) ) ;
#22233=CARTESIAN_POINT ( 'NONE',  ( 0.9711286089238851948, 0.2306618581243848609, 0.2411417322834645549 ) ) ;
#22234=CARTESIAN_POINT ( 'NONE',  ( 0.3083989501312343062, -0.05778040916215560624, -0.4822834645669293319 ) ) ;
#22235=CARTESIAN_POINT ( 'NONE',  ( -0.2034120734908128059, 0.1771653543307087630, 0.09757992244046791164 ) ) ;
#22236=CARTESIAN_POINT ( 'NONE',  ( 0.9383202099737538715, -0.05778040916215560624, -0.4822834645669293319 ) ) ;
#22237=CARTESIAN_POINT ( 'NONE',  ( -0.9317585301837263412, -0.4281496062992127816, -0.4176697321401328100 ) ) ;
#22238=CARTESIAN_POINT ( 'NONE',  ( -0.5511811023622041894, -0.1870078740157480879, -0.4822834645669291653 ) ) ;
#22239=CARTESIAN_POINT ( 'NONE',  ( -1.003937007874015297, -0.5400638737290845981, -0.3530559997133363437 ) ) ;
#22240=CARTESIAN_POINT ( 'NONE',  ( 1.003937007874016185, 0.1660481256975883668, -0.3530559997133364547 ) ) ;
#22241=CARTESIAN_POINT ( 'NONE',  ( 0.8727034120734912248, -0.3162353388693409650, -0.4822834645669289433 ) ) ;
#22242=CARTESIAN_POINT ( 'NONE',  ( 0.9580052493438327987, -0.4281496062992127816, -0.4176697321401328100 ) ) ;
#22244=CARTESIAN_POINT ( 'NONE',  ( -0.1377952755905504645, -0.4536011799217368745, -0.2665933059059886201 ) ) ;
#22247=ORIENTED_EDGE ( 'NONE', *, *, #9984, .T. ) ;
#22248=CARTESIAN_POINT ( 'NONE',  ( -0.9383202099737524282, -0.08942795157527998196, 0.3641732283464567121 ) ) ;
#22249=CARTESIAN_POINT ( 'NONE',  ( -0.5380577427821514602, 0.05413385826771666132, 0.4176697321401328100 ) ) ;
#22251=CARTESIAN_POINT ( 'NONE',  ( -0.3083989501312330295, -0.05778040916215522460, 0.4822834645669289988 ) ) ;
#22252=CARTESIAN_POINT ( 'NONE',  ( -0.5577427821522301654, -0.05778040916215560624, -0.4822834645669293319 ) ) ;
#22253=CARTESIAN_POINT ( 'NONE',  ( -1.292650918635170010, 0.2952755905511810774, -0.1292274648535930714 ) ) ;
#22254=CARTESIAN_POINT ( 'NONE',  ( -1.561679790026246017, 0.05413385826771666132, 0.4176697321401328100 ) ) ;
#22255=CARTESIAN_POINT ( 'NONE',  ( 0.9317585301837276734, -0.004921259842519870586, -0.3153832671262229437 ) ) ;
#22257=CARTESIAN_POINT ( 'NONE',  ( -1.586688153636163001, 2.388437996263389707, 0.1275903502784764276 ) ) ;
#22258=CARTESIAN_POINT ( 'NONE',  ( 0.3149606299212603933, -0.1870078740157479769, 0.3641732283464567677 ) ) ;
#22259=CARTESIAN_POINT ( 'NONE',  ( 0.07874015748031558404, -0.1870078740157479769, 0.4822834645669291653 ) ) ;
#22260=CARTESIAN_POINT ( 'NONE',  ( 0.1706036745406830368, -0.4281496062992127816, -0.4176697321401328100 ) ) ;
#22261=VERTEX_POINT ( 'NONE', #52355 ) ;
#22267=CARTESIAN_POINT ( 'NONE',  ( -0.8267716535433065062, -0.5511811023622047445, 6.969142054262312111E-17 ) ) ;
#22268=CARTESIAN_POINT ( 'NONE',  ( -0.4593175853018366950, 0.05413385826771666132, 0.4176697321401328100 ) ) ;
#22271=CARTESIAN_POINT ( 'NONE',  ( -1.561679790026246017, -0.3690944881889765550, -0.3153832671262227771 ) ) ;
#22272=CARTESIAN_POINT ( 'NONE',  ( 0.6824146981627303710, 0.2306618581243847221, -0.2411417322834647770 ) ) ;
#22273=CARTESIAN_POINT ( 'NONE',  ( 0.3543307086614181922, -0.6692913385826771977, 8.415575281601705876E-17 ) ) ;
#22274=CARTESIAN_POINT ( 'NONE',  ( -0.7217847769028863381, -0.3690944881889763329, 0.3153832671262228327 ) ) ;
#22275=CARTESIAN_POINT ( 'NONE',  ( 0.1902887139107617975, 0.2952755905511811885, 0.1292274648535926551 ) ) ;
#22277=CARTESIAN_POINT ( 'NONE',  ( -0.006561679790025524116, -0.08942795157528024563, -0.3641732283464568787 ) ) ;
#22278=CARTESIAN_POINT ( 'NONE',  ( -0.4396325459317579898, 0.2952755905511811885, 0.1292274648535926551 ) ) ;
#22280=CARTESIAN_POINT ( 'NONE',  ( -1.594488188976377563, -0.5400638737290844871, 0.3530559997133364547 ) ) ;
#22281=CARTESIAN_POINT ( 'NONE',  ( -0.03937007874015669567, -0.5511811023622047445, 6.969142054262312111E-17 ) ) ;
#22282=CARTESIAN_POINT ( 'NONE',  ( 1.633858267716535639, -0.4536011799217367080, 0.2665933059059888421 ) ) ;
#22283=CARTESIAN_POINT ( 'NONE',  ( -1.213910761154854745, 0.2952755905511810774, -0.1292274648535930714 ) ) ;
#22284=CARTESIAN_POINT ( 'NONE',  ( -0.5577427821522301654, -0.2845877964562159024, 0.3641732283464567677 ) ) ;
#22286=CARTESIAN_POINT ( 'NONE',  ( -1.095800524934382292, -0.05778040916215522460, 0.4822834645669289988 ) ) ;
#22287=CARTESIAN_POINT ( 'NONE',  ( -0.2230971128608915943, 0.05413385826771666132, 0.4176697321401328100 ) ) ;
#22291=CARTESIAN_POINT ( 'NONE',  ( 0.1902887139107617975, -0.5511811023622048555, -0.09757992244046775898 ) ) ;
#22292=CARTESIAN_POINT ( 'NONE',  ( 1.108923884514436242, -0.05778040916215522460, 0.4822834645669289988 ) ) ;
#22293=CARTESIAN_POINT ( 'NONE',  ( -1.220472440944881054, 0.1771653543307087630, 0.000000000000000000 ) ) ;
#22294=CARTESIAN_POINT ( 'NONE',  ( 1.312335958005250269, -0.6046776061558807314, 0.2411417322834647770 ) ) ;
#22295=CARTESIAN_POINT ( 'NONE',  ( -1.601049868766403650, -0.5023911411419708095, 0.1820866141732285504 ) ) ;
#22296=CARTESIAN_POINT ( 'NONE',  ( -0.4527559055118102749, 0.1660481256975885056, 0.3530559997133364547 ) ) ;
#22297=CARTESIAN_POINT ( 'NONE',  ( 0.04593175853018440641, -0.5511811023622046335, 0.09757992244046803654 ) ) ;
#22299=CARTESIAN_POINT ( 'NONE',  ( 0.4855643044619428750, -0.004921259842519576551, 0.3153832671262227771 ) ) ;
#22300=EDGE_CURVE ( 'NONE', #29190, #64851, #81283, .T. ) ;
#22301=CARTESIAN_POINT ( 'NONE',  ( -0.1312335958005241554, -0.6046776061558809534, -0.2411417322834644161 ) ) ;
#22302=( BOUNDED_CURVE ( )  B_SPLINE_CURVE ( 1, ( #22068, #22892 ),
 .UNSPECIFIED., .F., .F. ) 
 B_SPLINE_CURVE_WITH_KNOTS ( ( 2, 2 ),
 ( 1.734723475976807094E-18, 0.002000000000000001776 ),
 .UNSPECIFIED. ) 
 CURVE ( )  GEOMETRIC_REPRESENTATION_ITEM ( )  RATIONAL_B_SPLINE_CURVE ( ( 0.9875488213027523443, 0.9875488213027523443 ) ) 
 REPRESENTATION_ITEM ( '' )  );
#22304=EDGE_CURVE ( 'NONE', #59607, #5541, #6511, .T. ) ;
#22305=CARTESIAN_POINT ( 'NONE',  ( -1.259842519685038686, -0.1870078740157479769, 0.4822834645669291653 ) ) ;
#22307=CARTESIAN_POINT ( 'NONE',  ( 0.9317585301837276734, -0.3690944881889763329, 0.3153832671262228327 ) ) ;
#22308=CARTESIAN_POINT ( 'NONE',  ( -0.1115485564304453947, -0.6692913385826771977, 0.1292274648535927661 ) ) ;
#22309=CARTESIAN_POINT ( 'NONE',  ( -0.3149606299212590610, -0.1870078740157480879, -0.4822834645669291653 ) ) ;
#22310=CARTESIAN_POINT ( 'NONE',  ( -0.5183727034120726440, 0.1771653543307087630, 0.09757992244046791164 ) ) ;
#22311=CARTESIAN_POINT ( 'NONE',  ( 1.191111281560510715, -4.927456884911482678E-16, 0.4445507791589062840 ) ) ;
#22312=CARTESIAN_POINT ( 'NONE',  ( -0.3871391076115476282, -0.08942795157527998196, 0.3641732283464567121 ) ) ;
#22313=CARTESIAN_POINT ( 'NONE',  ( 0.4265091863517067594, 0.2952755905511811885, 0.1292274648535926551 ) ) ;
#22314=CARTESIAN_POINT ( 'NONE',  ( -0.6692913385826764205, -0.5511811023622047445, 6.969142054262312111E-17 ) ) ;
#22316=CARTESIAN_POINT ( 'NONE',  ( -1.332020997375327642, -0.05778040916215522460, 0.4822834645669289988 ) ) ;
#22319=CARTESIAN_POINT ( 'NONE',  ( -1.227034120734907585, 0.1771653543307087630, 0.09757992244046791164 ) ) ;
#22320=CARTESIAN_POINT ( 'NONE',  ( -0.5249343832020990641, -0.6046776061558809534, -0.2411417322834644161 ) ) ;
#22321=CARTESIAN_POINT ( 'NONE',  ( -1.620734908136482577, -0.6692913385826773087, -0.1292274648535924053 ) ) ;
#22322=CARTESIAN_POINT ( 'NONE',  ( -1.240157480314959759, -0.5400638737290845981, -0.3530559997133363437 ) ) ;
#22324=EDGE_CURVE ( 'NONE', #44273, #44157, #65392, .T. ) ;
#22325=CARTESIAN_POINT ( 'NONE',  ( 1.443569553805774897, -0.6046776061558809534, -0.2411417322834644161 ) ) ;
#22326=CARTESIAN_POINT ( 'NONE',  ( 0.9120734908136490793, 0.2952755905511810774, -0.1292274648535930714 ) ) ;
#22328=CARTESIAN_POINT ( 'NONE',  ( 1.614173228346457378, 0.2753471884572478157, 0.1372047244094478646 ) ) ;
#22330=EDGE_CURVE ( 'NONE', #64851, #35306, #60714, .T. ) ;
#22331=CARTESIAN_POINT ( 'NONE',  ( -1.627296587926508442, -0.6046776061558809534, -0.2411417322834644161 ) ) ;
#22334=CARTESIAN_POINT ( 'NONE',  ( -0.4921259842519677963, 0.07958543189024071263, -0.2665933059059888421 ) ) ;
#22337=CARTESIAN_POINT ( 'NONE',  ( 0.7480314960629927956, -0.6692913385826771977, 8.415575281601705876E-17 ) ) ;
#22339=CARTESIAN_POINT ( 'NONE',  ( -0.2887139107611542133, 0.2306618581243848609, 0.2411417322834645549 ) ) ;
#22340=CARTESIAN_POINT ( 'NONE',  ( -0.7152230971128602510, -0.3162353388693405765, 0.4822834645669290543 ) ) ;
#22341=CARTESIAN_POINT ( 'NONE',  ( 1.325459317585302665, -0.4281496062992124485, 0.4176697321401328655 ) ) ;
#22342=CARTESIAN_POINT ( 'NONE',  ( -1.187664041994749731, -0.2845877964562159024, 0.3641732283464567677 ) ) ;
#22344=CARTESIAN_POINT ( 'NONE',  ( 0.2624671916010504757, 0.2306618581243848609, 0.2411417322834645549 ) ) ;
#22345=CARTESIAN_POINT ( 'NONE',  ( -0.8070866141732276899, 0.1660481256975883668, -0.3530559997133364547 ) ) ;
#22347=CARTESIAN_POINT ( 'NONE',  ( -1.089238845144356427, -0.4281496062992127816, -0.4176697321401328100 ) ) ;
#22349=CARTESIAN_POINT ( 'NONE',  ( 0.8464566929133866546, -0.5400638737290844871, 0.3530559997133364547 ) ) ;
#22350=CARTESIAN_POINT ( 'NONE',  ( 1.227034120734908917, 0.1771653543307087075, -0.09757992244046823083 ) ) ;
#22353=CARTESIAN_POINT ( 'NONE',  ( -0.5971128608923877978, -0.6692913385826773087, -0.1292274648535924053 ) ) ;
#22355=CARTESIAN_POINT ( 'NONE',  ( 0.2034120734908142214, 0.1771653543307087075, -0.09757992244046823083 ) ) ;
#22357=CARTESIAN_POINT ( 'NONE',  ( -0.9842519685039365918, -0.6692913385826771977, 8.415575281601705876E-17 ) ) ;
#22358=CARTESIAN_POINT ( 'NONE',  ( 0.8005249343832027131, 0.05413385826771666132, 0.4176697321401328100 ) ) ;
#22359=CARTESIAN_POINT ( 'NONE',  ( 0.9120734908136489683, -0.6692913385826771977, 0.1292274648535927661 ) ) ;
#22360=CARTESIAN_POINT ( 'NONE',  ( -0.1968503937007867743, -0.6692913385826771977, 8.415575281601705876E-17 ) ) ;
#22362=CARTESIAN_POINT ( 'NONE',  ( -0.8464566929133852113, 0.1660481256975885056, 0.3530559997133364547 ) ) ;
#22364=CARTESIAN_POINT ( 'NONE',  ( -1.601049868766403650, -0.6046776061558807314, 0.2411417322834647770 ) ) ;
#22365=CARTESIAN_POINT ( 'NONE',  ( -0.6824146981627288167, 0.2306618581243848609, 0.2411417322834645549 ) ) ;
#22366=CARTESIAN_POINT ( 'NONE',  ( -0.4855643044619415427, -0.004921259842519870586, -0.3153832671262229437 ) ) ;
#22367=CARTESIAN_POINT ( 'NONE',  ( 1.391076115485564868, 0.2306618581243847221, -0.2411417322834647770 ) ) ;
#22368=CARTESIAN_POINT ( 'NONE',  ( 1.673228346456693494, 0.1660481256975885056, 0.3530559997133364547 ) ) ;
#22369=CARTESIAN_POINT ( 'NONE',  ( -1.095800524934382292, -0.05778040916215522460, 0.4822834645669289988 ) ) ;
#22371=CARTESIAN_POINT ( 'NONE',  ( 0.8333333333333340365, 0.2952755905511810774, -0.1292274648535930714 ) ) ;
#22373=CARTESIAN_POINT ( 'NONE',  ( 1.586052503253845503, 1.023622047244095556, 0.1653254495020588799 ) ) ;
#22374=CARTESIAN_POINT ( 'NONE',  ( -0.1246719160104980823, -0.6692913385826773087, -0.1292274648535924053 ) ) ;
#22375=CARTESIAN_POINT ( 'NONE',  ( -0.9514435695538050464, -0.08942795157528024563, -0.3641732283464568787 ) ) ;
#22376=CARTESIAN_POINT ( 'NONE',  ( 0.4068241469816281097, -0.004921259842519576551, 0.3153832671262227771 ) ) ;
#22378=CARTESIAN_POINT ( 'NONE',  ( 1.089238845144357759, -0.004921259842519870586, -0.3153832671262229437 ) ) ;
#22380=CARTESIAN_POINT ( 'NONE',  ( 0.9055118110236227702, -0.6692913385826771977, 8.415575281601705876E-17 ) ) ;
#22382=CARTESIAN_POINT ( 'NONE',  ( -0.5314960629921254842, -0.5400638737290845981, -0.3530559997133363437 ) ) ;
#22384=CARTESIAN_POINT ( 'NONE',  ( 1.233595800524935227, -0.5023911411419708095, 0.1820866141732285504 ) ) ;
#22385=CARTESIAN_POINT ( 'NONE',  ( -0.5643044619422565855, 0.05413385826771626580, -0.4176697321401330321 ) ) ;
#22387=CARTESIAN_POINT ( 'NONE',  ( 1.108923884514436686, -0.3162353388693409650, -0.4822834645669289433 ) ) ;
#22388=CARTESIAN_POINT ( 'NONE',  ( 5.463695987328526437E-16, -0.1870078740157479769, 0.4822834645669291653 ) ) ;
#22389=CARTESIAN_POINT ( 'NONE',  ( 0.5511811023622055217, -0.1870078740157479769, 0.3641732283464567677 ) ) ;
#22391=CARTESIAN_POINT ( 'NONE',  ( 0.5052493438320218022, -0.5511811023622048555, -0.09757992244046775898 ) ) ;
#22395=CARTESIAN_POINT ( 'NONE',  ( 0.6430446194225729606, -0.4281496062992127816, -0.4176697321401328100 ) ) ;
#22401=CARTESIAN_POINT ( 'NONE',  ( 0.1443569553805781891, -0.3690944881889763329, 0.3153832671262228327 ) ) ;
#22402=CARTESIAN_POINT ( 'NONE',  ( 8.195543980992789655E-16, -0.1870078740157480879, -0.4822834645669291653 ) ) ;
#22403=CARTESIAN_POINT ( 'NONE',  ( 1.502624671916010790, -0.08942795157527998196, 0.3641732283464567121 ) ) ;
#22404=CARTESIAN_POINT ( 'NONE',  ( -1.207349081364828880, 0.1283753931104746893, -0.1820866141732285504 ) ) ;
#22405=CARTESIAN_POINT ( 'NONE',  ( -1.541994750656167090, 0.2952755905511811885, 0.1292274648535926551 ) ) ;
#22406=CARTESIAN_POINT ( 'NONE',  ( 0.4068241469816281097, 0.05413385826771666132, 0.4176697321401328100 ) ) ;
#22407=CARTESIAN_POINT ( 'NONE',  ( 1.135170603674541256, -0.6692913385826773087, -0.1292274648535924053 ) ) ;
#22410=CARTESIAN_POINT ( 'NONE',  ( 0.3937007874015754361, -0.1870078740157480879, -0.4822834645669291653 ) ) ;
#22411=CARTESIAN_POINT ( 'NONE',  ( 1.332020997375329197, -0.3162353388693405765, 0.4822834645669290543 ) ) ;
#22412=CARTESIAN_POINT ( 'NONE',  ( 1.128608923884515169, -0.6046776061558809534, -0.2411417322834644161 ) ) ;
#22413=CARTESIAN_POINT ( 'NONE',  ( 1.003937007874016407, -0.4536011799217367080, 0.2665933059059888421 ) ) ;
#22414=CARTESIAN_POINT ( 'NONE',  ( 1.535433070866142558, 0.2952755905511811885, 0.000000000000000000 ) ) ;
#22415=CARTESIAN_POINT ( 'NONE',  ( -0.9383202099737524282, -0.2845877964562161244, -0.3641732283464567121 ) ) ;
#22416=CARTESIAN_POINT ( 'NONE',  ( 0.5118110236220478892, 0.1771653543307087630, 0.000000000000000000 ) ) ;
#22417=CARTESIAN_POINT ( 'NONE',  ( 0.2165354330708668673, -0.5400638737290844871, 0.3530559997133364547 ) ) ;
#22418=CARTESIAN_POINT ( 'NONE',  ( 0.6299212598425204535, -0.1870078740157479769, 0.4822834645669291653 ) ) ;
#22419=CARTESIAN_POINT ( 'NONE',  ( -0.3149606299212590610, -0.1870078740157480879, -0.4822834645669291653 ) ) ;
#22420=CARTESIAN_POINT ( 'NONE',  ( 0.1640419947506569498, -0.08942795157527998196, 0.3641732283464567121 ) ) ;
#22421=CARTESIAN_POINT ( 'NONE',  ( 0.7611548556430451917, -0.6046776061558807314, 0.2411417322834647770 ) ) ;
#22423=CARTESIAN_POINT ( 'NONE',  ( -0.9514435695538050464, -0.3162353388693405765, 0.4822834645669290543 ) ) ;
#22424=CARTESIAN_POINT ( 'NONE',  ( -1.069553805774277722, 0.2952755905511811885, 0.1292274648535926551 ) ) ;
#22427=CARTESIAN_POINT ( 'NONE',  ( -0.8464566929133852113, 0.1660481256975885056, 0.3530559997133364547 ) ) ;
#22428=CARTESIAN_POINT ( 'NONE',  ( -0.6496062992125976043, -0.5400638737290844871, 0.3530559997133364547 ) ) ;
#22432=CARTESIAN_POINT ( 'NONE',  ( 0.5774278215223104249, 0.1283753931104748280, 0.1820866141732283561 ) ) ;
#22434=CARTESIAN_POINT ( 'NONE',  ( 1.082677165354331228, -0.5400638737290844871, 0.3530559997133364547 ) ) ;
#22435=CARTESIAN_POINT ( 'NONE',  ( -0.2477166185931099773, 5.952911114587291371E-15, -0.3791483426435156012 ) ) ;
#22436=CARTESIAN_POINT ( 'NONE',  ( -1.410761154855642463, -0.08942795157527998196, 0.3641732283464567121 ) ) ;
#22437=CARTESIAN_POINT ( 'NONE',  ( 1.502624671916010790, -0.05778040916215522460, 0.4822834645669289988 ) ) ;
#22438=CARTESIAN_POINT ( 'NONE',  ( -1.561679790026246017, 0.05413385826771666132, 0.4176697321401328100 ) ) ;
#22439=CARTESIAN_POINT ( 'NONE',  ( 0.2887139107611556010, 0.2306618581243847221, -0.2411417322834647770 ) ) ;
#22442=CARTESIAN_POINT ( 'NONE',  ( -0.05905511811023545637, 0.1660481256975885056, 0.3530559997133364547 ) ) ;
#22443=CARTESIAN_POINT ( 'NONE',  ( -0.8858267716535425107, 0.07958543189024071263, -0.2665933059059888421 ) ) ;
#22444=CARTESIAN_POINT ( 'NONE',  ( 0.9776902887139113929, 0.2952755905511811885, 0.1292274648535926551 ) ) ;
#22445=CARTESIAN_POINT ( 'NONE',  ( -0.03937007874015669567, -0.6692913385826771977, 8.415575281601705876E-17 ) ) ;
#22449=CARTESIAN_POINT ( 'NONE',  ( 0.6561679790026253567, -0.6046776061558809534, -0.2411417322834644161 ) ) ;
#22451=CARTESIAN_POINT ( 'NONE',  ( 0.1509186351706042484, -0.3162353388693405765, 0.4822834645669290543 ) ) ;
#22452=CARTESIAN_POINT ( 'NONE',  ( -0.8923884514435688198, -0.6046776061558807314, 0.2411417322834647770 ) ) ;
#22454=CARTESIAN_POINT ( 'NONE',  ( 1.220472440944882386, -0.6692913385826771977, 8.415575281601705876E-17 ) ) ;
#22455=CARTESIAN_POINT ( 'NONE',  ( 0.5052493438320218022, -0.6692913385826773087, -0.1292274648535924053 ) ) ;
#22457=CARTESIAN_POINT ( 'NONE',  ( -0.3674540682414692561, -0.6046776061558809534, -0.2411417322834644161 ) ) ;
#22458=CARTESIAN_POINT ( 'NONE',  ( 0.8202099737532814183, -0.6692913385826773087, -0.1292274648535924053 ) ) ;
#22459=CARTESIAN_POINT ( 'NONE',  ( 0.1771653543307093182, -0.5400638737290845981, -0.3530559997133363437 ) ) ;
#22461=CARTESIAN_POINT ( 'NONE',  ( 0.7414698162729663755, 0.1771653543307087630, 0.09757992244046791164 ) ) ;
#22462=CARTESIAN_POINT ( 'NONE',  ( -1.305774278215222184, -0.6692913385826773087, -0.1292274648535924053 ) ) ;
#22464=CARTESIAN_POINT ( 'NONE',  ( 0.4593175853018379162, -0.4281496062992124485, 0.4176697321401328655 ) ) ;
#22466=ORIENTED_EDGE ( 'NONE', *, *, #39648, .T. ) ;
#22468=CARTESIAN_POINT ( 'NONE',  ( 1.010498687664042716, -0.4281496062992124485, 0.4176697321401328655 ) ) ;
#22469=CARTESIAN_POINT ( 'NONE',  ( 0.6364829396325465405, -0.08942795157527998196, 0.3641732283464567121 ) ) ;
#22475=CARTESIAN_POINT ( 'NONE',  ( -0.6561679790026240244, 0.2306618581243847221, -0.2411417322834647770 ) ) ;
#22476=CARTESIAN_POINT ( 'NONE',  ( -0.7677165354330699465, 0.1660481256975885056, 0.3530559997133364547 ) ) ;
#22477=CARTESIAN_POINT ( 'NONE',  ( 0.5118110236220478892, 0.2952755905511811885, 0.000000000000000000 ) ) ;
#22479=CARTESIAN_POINT ( 'NONE',  ( 1.299212598425197429, 0.2952755905511811885, 0.000000000000000000 ) ) ;
#22480=CARTESIAN_POINT ( 'NONE',  ( 1.653543307086614789, -0.1870078740157479769, 0.3641732283464567677 ) ) ;
#22481=CARTESIAN_POINT ( 'NONE',  ( 1.640419947506562393, -0.3690944881889763329, 0.3153832671262228327 ) ) ;
#22483=CARTESIAN_POINT ( 'NONE',  ( -1.227034120734907141, -0.5511811023622048555, -0.09757992244046775898 ) ) ;
#22485=CARTESIAN_POINT ( 'NONE',  ( 0.3674540682414705883, -0.6046776061558807314, 0.2411417322834647770 ) ) ;
#22486=CARTESIAN_POINT ( 'NONE',  ( 1.364829396325460076, 0.2306618581243848609, 0.2411417322834645549 ) ) ;
#22487=DIRECTION ( 'NONE',  ( 0.000000000000000000, -0.000000000000000000, 1.000000000000000000 ) ) ;
#22488=CARTESIAN_POINT ( 'NONE',  ( -1.325459317585300889, -0.3690944881889765550, -0.3153832671262227771 ) ) ;
#22489=( BOUNDED_CURVE ( )  B_SPLINE_CURVE ( 2, ( #72475, #53088, #71220, #27427, #46364, #1360, #27012 ),
 .UNSPECIFIED., .F., .F. ) 
 B_SPLINE_CURVE_WITH_KNOTS ( ( 3, 2, 2, 3 ),
 ( 0.8096947309984371399, 0.8106060606060605522, 0.8143939393939394478, 0.8181818181818182323 ),
 .UNSPECIFIED. ) 
 CURVE ( )  GEOMETRIC_REPRESENTATION_ITEM ( )  RATIONAL_B_SPLINE_CURVE ( ( 0.9875488213027523443, 0.9918020599134680371, 1.000000000000000000, 0.9659258262890683122, 1.000000000000000000, 0.9659258262890683122, 1.000000000000000000 ) ) 
 REPRESENTATION_ITEM ( '' )  );
#22490=CARTESIAN_POINT ( 'NONE',  ( 0.4461942257217856311, 0.2306618581243847221, -0.2411417322834647770 ) ) ;
#22491=CARTESIAN_POINT ( 'NONE',  ( 1.345144356955381593, -0.2845877964562161244, -0.3641732283464567121 ) ) ;
#22493=CARTESIAN_POINT ( 'NONE',  ( -1.076115485564303809, 0.1283753931104748280, 0.1820866141732283561 ) ) ;
#22494=CARTESIAN_POINT ( 'NONE',  ( 1.266404199475066328, -0.3162353388693409650, -0.4822834645669289433 ) ) ;
#22496=CARTESIAN_POINT ( 'NONE',  ( -0.1377952755905504645, 0.1660481256975885056, 0.3530559997133364547 ) ) ;
#22497=CARTESIAN_POINT ( 'NONE',  ( -1.502624671916009680, -0.2845877964562159024, 0.3641732283464567677 ) ) ;
#22498=CARTESIAN_POINT ( 'NONE',  ( -0.4396325459317579898, 0.1771653543307087630, 0.09757992244046791164 ) ) ;
#22499=CARTESIAN_POINT ( 'NONE',  ( -0.8136482939632537770, -0.6046776061558807314, 0.2411417322834647770 ) ) ;
#22500=CARTESIAN_POINT ( 'NONE',  ( -1.633858267716534529, 0.07958543189024085140, 0.2665933059059887866 ) ) ;
#22502=CARTESIAN_POINT ( 'NONE',  ( 0.3018372703412079971, -0.4281496062992124485, 0.4176697321401328655 ) ) ;
#22507=CARTESIAN_POINT ( 'NONE',  ( -1.364829396325458521, 0.2306618581243847221, -0.2411417322834647770 ) ) ;
#22508=CARTESIAN_POINT ( 'NONE',  ( -0.8136482939632537770, -0.5023911411419708095, 0.1820866141732285504 ) ) ;
#22509=CYLINDRICAL_SURFACE ( 'NONE', #78372, 0.4822834645669291653 ) ;
#22510=CARTESIAN_POINT ( 'NONE',  ( -0.03937007874015669567, 0.2952755905511811885, 0.000000000000000000 ) ) ;
#22511=CARTESIAN_POINT ( 'NONE',  ( 0.3083989501312343062, -0.08942795157528024563, -0.3641732283464568787 ) ) ;
#22512=CARTESIAN_POINT ( 'NONE',  ( -0.7152230971128602510, -0.08942795157528024563, -0.3641732283464568787 ) ) ;
#22513=CARTESIAN_POINT ( 'NONE',  ( -1.601049868766403650, -0.6046776061558807314, 0.2411417322834647770 ) ) ;
#22514=CARTESIAN_POINT ( 'NONE',  ( -1.620734908136482577, -0.6692913385826773087, -0.1292274648535924053 ) ) ;
#22515=CARTESIAN_POINT ( 'NONE',  ( 1.371391076115485941, 0.2952755905511811885, 0.1292274648535926551 ) ) ;
#22517=CARTESIAN_POINT ( 'NONE',  ( 0.9580052493438327987, -0.3690944881889765550, -0.3153832671262227771 ) ) ;
#22518=CARTESIAN_POINT ( 'NONE',  ( 0.8923884514435703741, 0.2306618581243848609, 0.2411417322834645549 ) ) ;
#22519=CARTESIAN_POINT ( 'NONE',  ( 1.568241469816273437, -0.2845877964562159024, 0.3641732283464567677 ) ) ;
#22521=CARTESIAN_POINT ( 'NONE',  ( -1.220472440944881054, -0.6692913385826771977, 8.415575281601705876E-17 ) ) ;
#22522=CARTESIAN_POINT ( 'NONE',  ( -0.9317585301837263412, -0.4281496062992127816, -0.4176697321401328100 ) ) ;
#22523=CARTESIAN_POINT ( 'NONE',  ( 0.2887139107611556010, -0.6046776061558807314, 0.2411417322834647770 ) ) ;
#22524=CARTESIAN_POINT ( 'NONE',  ( -1.318897637795274802, -0.4536011799217368745, -0.2665933059059886201 ) ) ;
#22526=CARTESIAN_POINT ( 'NONE',  ( 1.351706036745407458, -0.3690944881889765550, -0.3153832671262227771 ) ) ;
#22527=CARTESIAN_POINT ( 'NONE',  ( 0.4330708661417329575, 0.2952755905511811885, 0.000000000000000000 ) ) ;
#22528=CARTESIAN_POINT ( 'NONE',  ( 0.7808398950131240079, -0.3162353388693405765, 0.4822834645669290543 ) ) ;
#22529=B_SPLINE_CURVE_WITH_KNOTS ( 'NONE', 3,
 ( #61805, #24320, #30224, #4554 ),
 .UNSPECIFIED., .F., .F.,
 ( 4, 4 ),
 ( 3.593986969179100008E-07, 0.001287825409103298150 ),
 .UNSPECIFIED. ) ;
#22530=CARTESIAN_POINT ( 'NONE',  ( 1.666666666666667185, 0.05413385826771666132, 0.4176697321401328100 ) ) ;
#22534=CARTESIAN_POINT ( 'NONE',  ( -0.7443564562302430465, 1.971400176305090124, -0.5309055118110235227 ) ) ;
#22536=CARTESIAN_POINT ( 'NONE',  ( 0.09842519685039434474, -0.4536011799217368745, -0.2665933059059886201 ) ) ;
#22537=CARTESIAN_POINT ( 'NONE',  ( -0.4593175853018366950, 0.05413385826771666132, 0.4176697321401328100 ) ) ;
#22538=CARTESIAN_POINT ( 'NONE',  ( 0.8267716535433077274, 0.2952755905511811885, 0.000000000000000000 ) ) ;
#22540=CARTESIAN_POINT ( 'NONE',  ( -0.02624671916010428221, 0.1283753931104746893, -0.1820866141732285504 ) ) ;
#22541=CARTESIAN_POINT ( 'NONE',  ( -1.181102362204723644, -0.1870078740157479769, 0.4822834645669291653 ) ) ;
#22542=CARTESIAN_POINT ( 'NONE',  ( 1.371391076115485719, -0.6692913385826773087, -0.1292274648535924053 ) ) ;
#22545=CARTESIAN_POINT ( 'NONE',  ( -1.586052503253846169, 1.850393700787402729, -0.1653254495020583803 ) ) ;
#22548=VERTEX_POINT ( 'NONE', #52776 ) ;
#22549=CARTESIAN_POINT ( 'NONE',  ( 1.141732283464567566, 0.2952755905511811885, 0.000000000000000000 ) ) ;
#22550=CARTESIAN_POINT ( 'NONE',  ( -1.581364829396324945, -0.3162353388693405765, 0.4822834645669290543 ) ) ;
#22551=CARTESIAN_POINT ( 'NONE',  ( -1.200787401574802349, -0.4536011799217367080, 0.2665933059059888421 ) ) ;
#22552=CARTESIAN_POINT ( 'NONE',  ( -1.555118110236219930, -0.5400638737290845981, -0.3530559997133363437 ) ) ;
#22555=CARTESIAN_POINT ( 'NONE',  ( 1.404199475065617708, 0.05413385826771626580, -0.4176697321401330321 ) ) ;
#22556=CARTESIAN_POINT ( 'NONE',  ( -1.686351706036744558, 0.2952755905511810774, -0.1292274648535930714 ) ) ;
#22557=CARTESIAN_POINT ( 'NONE',  ( 0.006561679790026889343, -0.05778040916215522460, 0.4822834645669289988 ) ) ;
#22558=CARTESIAN_POINT ( 'NONE',  ( -0.6955380577427815458, -0.4281496062992127816, -0.4176697321401328100 ) ) ;
#22559=CARTESIAN_POINT ( 'NONE',  ( -1.646981627296586703, -0.05778040916215522460, 0.4822834645669289988 ) ) ;
#22561=CARTESIAN_POINT ( 'NONE',  ( 0.1115485564304467270, -0.6692913385826773087, -0.1292274648535924053 ) ) ;
#22562=AXIS2_PLACEMENT_3D ( 'NONE', #42196, #15725, #61566 ) ;
#22564=CARTESIAN_POINT ( 'NONE',  ( -1.095800524934382292, -0.2845877964562161244, -0.3641732283464567121 ) ) ;
#22568=CARTESIAN_POINT ( 'NONE',  ( -0.6399301791983041943, -2.567464376874931580E-15, -0.4445507791589072832 ) ) ;
#22570=CARTESIAN_POINT ( 'NONE',  ( -1.653543307086613234, -0.1870078740157480879, -0.4822834645669291653 ) ) ;
#22572=DIRECTION ( 'NONE',  ( 1.000000000000000000, 3.096699300667737957E-16, -1.692413147294446216E-16 ) ) ;
#22573=CARTESIAN_POINT ( 'NONE',  ( -1.692913385826770645, 0.2952755905511811885, 0.000000000000000000 ) ) ;
#22576=CARTESIAN_POINT ( 'NONE',  ( -0.4986876640419939388, 0.1283753931104746893, -0.1820866141732285504 ) ) ;
#22577=CARTESIAN_POINT ( 'NONE',  ( -0.7480314960629914633, 0.1771653543307087630, 0.000000000000000000 ) ) ;
#22578=CARTESIAN_POINT ( 'NONE',  ( -1.391076115485563314, -0.6046776061558809534, -0.2411417322834644161 ) ) ;
#22579=CARTESIAN_POINT ( 'NONE',  ( 0.6561679790026253567, 0.2306618581243848609, 0.2411417322834645549 ) ) ;
#22580=CARTESIAN_POINT ( 'NONE',  ( -1.332020997375327642, -0.05778040916215522460, 0.4822834645669289988 ) ) ;
#22582=ORIENTED_EDGE ( 'NONE', *, *, #5358, .F. ) ;
#22583=CARTESIAN_POINT ( 'NONE',  ( -1.377952755905511140, -0.6692913385826771977, 8.415575281601705876E-17 ) ) ;
#22589=CARTESIAN_POINT ( 'NONE',  ( -0.8792650918635160906, -0.4281496062992124485, 0.4176697321401328655 ) ) ;
#22590=CARTESIAN_POINT ( 'NONE',  ( 1.463254593175853824, -0.6692913385826771977, 0.1292274648535927661 ) ) ;
#22591=CARTESIAN_POINT ( 'NONE',  ( -1.660104986876639543, -0.05778040916215560624, -0.4822834645669293319 ) ) ;
#22593=CARTESIAN_POINT ( 'NONE',  ( -1.515748031496062076, 0.1660481256975883668, -0.3530559997133364547 ) ) ;
#22594=CARTESIAN_POINT ( 'NONE',  ( -0.7677165354330699465, 0.1660481256975885056, 0.3530559997133364547 ) ) ;
#22596=CARTESIAN_POINT ( 'NONE',  ( -0.1574803149606292529, -0.1870078740157479769, 0.3641732283464567677 ) ) ;
#22598=CARTESIAN_POINT ( 'NONE',  ( -0.2624671916010490880, -0.5023911411419708095, 0.1820866141732285504 ) ) ;
#22599=CARTESIAN_POINT ( 'NONE',  ( 0.8923884514435701520, -0.5023911411419708095, -0.1820866141732282451 ) ) ;
#22600=CARTESIAN_POINT ( 'NONE',  ( 0.7939632545931766261, -0.05778040916215522460, 0.4822834645669289988 ) ) ;
#22602=CARTESIAN_POINT ( 'NONE',  ( -0.2296587926509179312, -0.08942795157527998196, 0.3641732283464567121 ) ) ;
#22604=CARTESIAN_POINT ( 'NONE',  ( 1.384514435695538337, -0.6692913385826771977, 0.1292274648535927661 ) ) ;
#22605=CARTESIAN_POINT ( 'NONE',  ( -1.345144356955379816, -0.2845877964562159024, 0.3641732283464567677 ) ) ;
#22607=CARTESIAN_POINT ( 'NONE',  ( 0.2493438320209980519, -0.4281496062992127816, -0.4176697321401328100 ) ) ;
#22608=CARTESIAN_POINT ( 'NONE',  ( 0.1115485564304470323, 0.2952755905511811885, 0.1292274648535926551 ) ) ;
#22609=CARTESIAN_POINT ( 'NONE',  ( 1.496062992125985147, -0.1870078740157479769, 0.3641732283464567677 ) ) ;
#22610=CARTESIAN_POINT ( 'NONE',  ( 0.4002624671916016896, -0.2845877964562161244, -0.3641732283464567121 ) ) ;
#22611=CARTESIAN_POINT ( 'NONE',  ( -0.1902887139107604098, -0.5511811023622046335, 0.09757992244046803654 ) ) ;
#22612=CARTESIAN_POINT ( 'NONE',  ( -0.7349081364829387342, -0.6046776061558807314, 0.2411417322834647770 ) ) ;
#22615=CARTESIAN_POINT ( 'NONE',  ( 0.01968503937007957949, -0.5400638737290845981, -0.3530559997133363437 ) ) ;
#22618=CARTESIAN_POINT ( 'NONE',  ( 1.561679790026247350, -0.4281496062992124485, 0.4176697321401328655 ) ) ;
#22619=CARTESIAN_POINT ( 'NONE',  ( -0.04593175853018302557, -0.5511811023622048555, -0.09757992244046775898 ) ) ;
#22620=CARTESIAN_POINT ( 'NONE',  ( -0.1902887139107604098, -0.6692913385826771977, 0.1292274648535927661 ) ) ;
#22621=CARTESIAN_POINT ( 'NONE',  ( -1.522309711286088607, -0.6046776061558807314, 0.2411417322834647770 ) ) ;
#22622=CARTESIAN_POINT ( 'NONE',  ( -1.601049868766403650, 0.1283753931104746893, -0.1820866141732285504 ) ) ;
#22623=CARTESIAN_POINT ( 'NONE',  ( 1.371391076115485941, 0.2952755905511811885, 0.1292274648535926551 ) ) ;
#22624=DIRECTION ( 'NONE',  ( 0.000000000000000000, 0.000000000000000000, -1.000000000000000000 ) ) ;
#22625=CARTESIAN_POINT ( 'NONE',  ( -0.5446194225721777693, -0.2845877964562161244, -0.3641732283464567121 ) ) ;
#22629=CARTESIAN_POINT ( 'NONE',  ( 1.423884514435696413, -0.2845877964562161244, -0.3641732283464567121 ) ) ;
#22630=CARTESIAN_POINT ( 'NONE',  ( 1.220472440944882386, -0.5511811023622047445, 6.969142054262312111E-17 ) ) ;
#22631=CARTESIAN_POINT ( 'NONE',  ( -1.515748031496062076, 0.1660481256975883668, -0.3530559997133364547 ) ) ;
#22632=CARTESIAN_POINT ( 'NONE',  ( 0.8923884514435701520, -0.6046776061558809534, -0.2411417322834644161 ) ) ;
#22634=CARTESIAN_POINT ( 'NONE',  ( 1.043307086614173818, 0.07958543189024085140, 0.2665933059059887866 ) ) ;
#22636=CARTESIAN_POINT ( 'NONE',  ( 0.1706036745406830368, -0.4281496062992127816, -0.4176697321401328100 ) ) ;
#22637=CARTESIAN_POINT ( 'NONE',  ( -1.003937007874014853, 0.1660481256975885056, 0.3530559997133364547 ) ) ;
#22641=CARTESIAN_POINT ( 'NONE',  ( 0.3477690288713918276, 0.1771653543307087630, 0.09757992244046791164 ) ) ;
#22642=VERTEX_POINT ( 'NONE', #34690 ) ;
#22644=VERTEX_POINT ( 'NONE', #28778 ) ;
#22646=CARTESIAN_POINT ( 'NONE',  ( -0.6430446194225716283, -0.4281496062992124485, 0.4176697321401328655 ) ) ;
#22647=CARTESIAN_POINT ( 'NONE',  ( -0.3674540682414689785, 0.2306618581243848609, 0.2411417322834645549 ) ) ;
#22648=CARTESIAN_POINT ( 'NONE',  ( -0.5118110236220466680, 0.1771653543307087630, 0.000000000000000000 ) ) ;
#22649=CARTESIAN_POINT ( 'NONE',  ( 0.8661417322834653598, -0.1870078740157479769, 0.4822834645669291653 ) ) ;
#22650=CARTESIAN_POINT ( 'NONE',  ( -1.056430446194224881, -0.6692913385826771977, 0.1292274648535927661 ) ) ;
#22651=CARTESIAN_POINT ( 'NONE',  ( -0.3740157480314953431, -0.5400638737290845981, -0.3530559997133363437 ) ) ;
#22652=CARTESIAN_POINT ( 'NONE',  ( 1.062992125984252745, -0.6692913385826771977, 8.415575281601705876E-17 ) ) ;
#22653=CARTESIAN_POINT ( 'NONE',  ( 1.023622047244095112, -0.1870078740157480879, -0.4822834645669291653 ) ) ;
#22654=CARTESIAN_POINT ( 'NONE',  ( 0.7020997375328090762, -0.3162353388693405765, 0.4822834645669290543 ) ) ;
#22656=CARTESIAN_POINT ( 'NONE',  ( -0.1771653543307080136, 0.07958543189024071263, -0.2665933059059888421 ) ) ;
#22657=VERTEX_POINT ( 'NONE', #20808 ) ;
#22660=CARTESIAN_POINT ( 'NONE',  ( -0.9251968503937002541, 0.07958543189024085140, 0.2665933059059887866 ) ) ;
#22661=CARTESIAN_POINT ( 'NONE',  ( -0.6496062992125976043, 0.1660481256975883668, -0.3530559997133364547 ) ) ;
#22663=CARTESIAN_POINT ( 'NONE',  ( -0.4461942257217840213, 0.2306618581243848609, 0.2411417322834645549 ) ) ;
#22664=CARTESIAN_POINT ( 'NONE',  ( -0.5380577427821514602, -0.4281496062992127816, -0.4176697321401328100 ) ) ;
#22665=CARTESIAN_POINT ( 'NONE',  ( -1.141732283464566011, 0.2952755905511811885, 0.000000000000000000 ) ) ;
#22666=CARTESIAN_POINT ( 'NONE',  ( -1.587926509186350810, -0.4281496062992124485, 0.4176697321401328655 ) ) ;
#22667=CARTESIAN_POINT ( 'NONE',  ( 0.8267716535433078384, -0.5511811023622047445, 6.969142054262312111E-17 ) ) ;
#22668=LINE ( 'NONE', #48327, #75366 ) ;
#22670=CARTESIAN_POINT ( 'NONE',  ( 0.6036745406824153282, -0.5023911411419708095, 0.1820866141732285504 ) ) ;
#22671=CARTESIAN_POINT ( 'NONE',  ( -0.03280839895013062252, 0.2952755905511810774, -0.1292274648535930714 ) ) ;
#22672=CARTESIAN_POINT ( 'NONE',  ( 0.4724409448818904789, -0.1870078740157480879, -0.4822834645669291653 ) ) ;
#22678=CARTESIAN_POINT ( 'NONE',  ( -0.7998211177050861265, -2.609869883881465018E-15, -0.3464511005275220379 ) ) ;
#22679=CARTESIAN_POINT ( 'NONE',  ( -0.5314960629921254842, -0.4536011799217368745, -0.2665933059059886201 ) ) ;
#22680=CARTESIAN_POINT ( 'NONE',  ( -1.141732283464566011, -0.6692913385826771977, 8.415575281601705876E-17 ) ) ;
#22683=CARTESIAN_POINT ( 'NONE',  ( 1.528871391076116026, 0.2952755905511811885, 0.1292274648535926551 ) ) ;
#22684=CARTESIAN_POINT ( 'NONE',  ( 1.056430446194226436, -0.6692913385826773087, -0.1292274648535924053 ) ) ;
#22685=CARTESIAN_POINT ( 'NONE',  ( 0.6955380577427828781, -0.4281496062992124485, 0.4176697321401328655 ) ) ;
#22686=CARTESIAN_POINT ( 'NONE',  ( -0.6364829396325453192, -0.08942795157528024563, -0.3641732283464568787 ) ) ;
#22687=CARTESIAN_POINT ( 'NONE',  ( -0.006561679790025524116, -0.3162353388693405765, 0.4822834645669290543 ) ) ;
#22689=CARTESIAN_POINT ( 'NONE',  ( -0.3083989501312330295, -0.2845877964562161244, -0.3641732283464567121 ) ) ;
#22690=CARTESIAN_POINT ( 'NONE',  ( -0.3149606299212590610, -0.1870078740157479769, 0.4822834645669291653 ) ) ;
#22692=CARTESIAN_POINT ( 'NONE',  ( -1.574803149606298636, -0.1870078740157479769, 0.4822834645669291653 ) ) ;
#22693=CARTESIAN_POINT ( 'NONE',  ( 0.02624671916010564918, 0.1283753931104748280, 0.1820866141732283561 ) ) ;
#22694=CARTESIAN_POINT ( 'NONE',  ( 1.430446194225722500, -0.3690944881889765550, -0.3153832671262227771 ) ) ;
#22695=CARTESIAN_POINT ( 'NONE',  ( -1.272965879265091305, -0.4281496062992124485, 0.4176697321401328655 ) ) ;
#22696=CARTESIAN_POINT ( 'NONE',  ( -0.7611548556430438595, -0.5023911411419708095, -0.1820866141732282451 ) ) ;
#22697=DIRECTION ( 'NONE',  ( 0.000000000000000000, 0.000000000000000000, -1.000000000000000000 ) ) ;
#22698=CARTESIAN_POINT ( 'NONE',  ( -0.9645669291338575535, -0.5400638737290844871, 0.3530559997133364547 ) ) ;
#22699=CARTESIAN_POINT ( 'NONE',  ( -0.5708661417322825615, -0.5400638737290844871, 0.3530559997133364547 ) ) ;
#22700=CARTESIAN_POINT ( 'NONE',  ( 0.2493438320209980519, 0.05413385826771666132, 0.4176697321401328100 ) ) ;
#22704=CARTESIAN_POINT ( 'NONE',  ( 0.2755905511811031494, 0.1771653543307087630, 0.000000000000000000 ) ) ;
#22705=CARTESIAN_POINT ( 'NONE',  ( 0.9580052493438326877, 0.05413385826771666132, 0.4176697321401328100 ) ) ;
#22706=CARTESIAN_POINT ( 'NONE',  ( -1.148293963254592542, -0.5511811023622048555, -0.09757992244046775898 ) ) ;
#22707=CARTESIAN_POINT ( 'NONE',  ( 1.174540682414699111, -0.3162353388693405765, 0.4822834645669290543 ) ) ;
#22708=CARTESIAN_POINT ( 'NONE',  ( -1.719160104986876103, -0.004921259842519576551, 0.3153832671262227771 ) ) ;
#22710=CARTESIAN_POINT ( 'NONE',  ( -0.4790026246719154557, -0.3162353388693405765, 0.4822834645669290543 ) ) ;
#22711=CARTESIAN_POINT ( 'NONE',  ( 0.1377952755905518800, 0.07958543189024071263, -0.2665933059059888421 ) ) ;
#22713=CARTESIAN_POINT ( 'NONE',  ( 0.7808398950131240079, -0.2845877964562159024, 0.3641732283464567677 ) ) ;
#22714=CARTESIAN_POINT ( 'NONE',  ( -0.03937007874015669567, 0.2952755905511811885, 0.000000000000000000 ) ) ;
#22716=CARTESIAN_POINT ( 'NONE',  ( -0.9251968503937002541, 0.1660481256975885056, 0.3530559997133364547 ) ) ;
#22718=CARTESIAN_POINT ( 'NONE',  ( 0.8989501312335963501, -0.5511811023622048555, -0.09757992244046775898 ) ) ;
#22719=CARTESIAN_POINT ( 'NONE',  ( -0.09842519685039295696, -0.5400638737290844871, 0.3530559997133364547 ) ) ;
#22720=CARTESIAN_POINT ( 'NONE',  ( -0.3215223097112853146, -0.05778040916215560624, -0.4822834645669293319 ) ) ;
#22721=CARTESIAN_POINT ( 'NONE',  ( -0.4330708661417315697, -0.5511811023622047445, 6.969142054262312111E-17 ) ) ;
#22723=CARTESIAN_POINT ( 'NONE',  ( -0.6627296587926501115, 0.1771653543307087075, -0.09757992244046823083 ) ) ;
#22724=CARTESIAN_POINT ( 'NONE',  ( 0.2099737532808405305, -0.6046776061558807314, 0.2411417322834647770 ) ) ;
#22725=CARTESIAN_POINT ( 'NONE',  ( -1.108923884514435132, -0.2845877964562159024, 0.3641732283464567677 ) ) ;
#22727=CARTESIAN_POINT ( 'NONE',  ( -1.003937007874014853, 0.1660481256975885056, 0.3530559997133364547 ) ) ;
#22730=CARTESIAN_POINT ( 'NONE',  ( -1.502624671916009680, -0.08942795157528024563, -0.3641732283464568787 ) ) ;
#22731=CARTESIAN_POINT ( 'NONE',  ( -0.6036745406824141069, 0.2306618581243848609, 0.2411417322834645549 ) ) ;
#22733=CARTESIAN_POINT ( 'NONE',  ( -1.397637795275589623, -0.5400638737290845981, -0.3530559997133363437 ) ) ;
#22736=CARTESIAN_POINT ( 'NONE',  ( 1.522309711286089939, 0.2306618581243848609, 0.2411417322834645549 ) ) ;
#22737=CARTESIAN_POINT ( 'NONE',  ( 0.6036745406824154392, 0.2306618581243847221, -0.2411417322834647770 ) ) ;
#22739=CARTESIAN_POINT ( 'NONE',  ( -1.660104986876639543, -0.05778040916215560624, -0.4822834645669293319 ) ) ;
#22742=CARTESIAN_POINT ( 'NONE',  ( -0.8267716535433065062, 0.1771653543307087630, 0.000000000000000000 ) ) ;
#22745=CARTESIAN_POINT ( 'NONE',  ( 0.6299212598425204535, -0.1870078740157479769, 0.4822834645669291653 ) ) ;
#22746=CARTESIAN_POINT ( 'NONE',  ( -0.4790026246719154557, -0.3162353388693405765, 0.4822834645669290543 ) ) ;
#22747=CARTESIAN_POINT ( 'NONE',  ( -1.227034120734907141, -0.6692913385826773087, -0.1292274648535924053 ) ) ;
#22748=CARTESIAN_POINT ( 'NONE',  ( 1.095800524934383846, -0.05778040916215560624, -0.4822834645669293319 ) ) ;
#22749=CARTESIAN_POINT ( 'NONE',  ( -1.266404199475064773, -0.08942795157528024563, -0.3641732283464568787 ) ) ;
#22751=CARTESIAN_POINT ( 'NONE',  ( 0.4986876640419954376, -0.6046776061558809534, -0.2411417322834644161 ) ) ;
#22752=CARTESIAN_POINT ( 'NONE',  ( -0.6889763779527552368, 0.1660481256975885056, 0.3530559997133364547 ) ) ;
#22754=CARTESIAN_POINT ( 'NONE',  ( -1.174540682414697335, -0.05778040916215522460, 0.4822834645669289988 ) ) ;
#22756=CARTESIAN_POINT ( 'NONE',  ( 0.8070866141732289112, -0.5400638737290845981, -0.3530559997133363437 ) ) ;
#22757=CARTESIAN_POINT ( 'NONE',  ( 1.128608923884515169, -0.5023911411419708095, -0.1820866141732282451 ) ) ;
#22760=CARTESIAN_POINT ( 'NONE',  ( -0.2821522309711278487, -0.6692913385826773087, -0.1292274648535924053 ) ) ;
#22761=ORIENTED_EDGE ( 'NONE', *, *, #31743, .T. ) ;
#22762=CARTESIAN_POINT ( 'NONE',  ( 0.3805774278215230400, -0.004921259842519870586, -0.3153832671262229437 ) ) ;
#22764=CARTESIAN_POINT ( 'NONE',  ( 0.7808398950131240079, -0.3162353388693405765, 0.4822834645669290543 ) ) ;
#22765=CARTESIAN_POINT ( 'NONE',  ( 1.049868766404200127, -0.6046776061558809534, -0.2411417322834644161 ) ) ;
#22766=CARTESIAN_POINT ( 'NONE',  ( -0.3608923884514428360, -0.6692913385826773087, -0.1292274648535924053 ) ) ;
#22768=CARTESIAN_POINT ( 'NONE',  ( -0.8595800524934373854, -0.05778040916215522460, 0.4822834645669289988 ) ) ;
#22770=CARTESIAN_POINT ( 'NONE',  ( -1.614173228346456268, -0.6692913385826771977, 8.415575281601705876E-17 ) ) ;
#22771=CARTESIAN_POINT ( 'NONE',  ( -0.8727034120734901146, -0.3162353388693405765, 0.4822834645669290543 ) ) ;
#22772=CARTESIAN_POINT ( 'NONE',  ( 1.128608923884515169, -0.6046776061558809534, -0.2411417322834644161 ) ) ;
#22775=CARTESIAN_POINT ( 'NONE',  ( -0.8267716535433065062, -0.6692913385826771977, 8.415575281601705876E-17 ) ) ;
#22778=CARTESIAN_POINT ( 'NONE',  ( 0.3608923884514443348, 0.2952755905511810774, -0.1292274648535930714 ) ) ;
#22781=CARTESIAN_POINT ( 'NONE',  ( -0.6167979002624665030, -0.4281496062992127816, -0.4176697321401328100 ) ) ;
#22782=CARTESIAN_POINT ( 'NONE',  ( -1.476377952755905110, 0.07958543189024085140, 0.2665933059059887866 ) ) ;
#22783=CARTESIAN_POINT ( 'NONE',  ( 0.4593175853018380828, -0.004921259842519870586, -0.3153832671262229437 ) ) ;
#22784=CARTESIAN_POINT ( 'NONE',  ( 1.377952755905512472, -0.6692913385826771977, 8.415575281601705876E-17 ) ) ;
#22786=CARTESIAN_POINT ( 'NONE',  ( 0.9908136482939640111, -0.5511811023622046335, 0.09757992244046803654 ) ) ;
#22787=CARTESIAN_POINT ( 'NONE',  ( 0.6102362204724416372, -0.5400638737290844871, 0.3530559997133364547 ) ) ;
#22789=CARTESIAN_POINT ( 'NONE',  ( -0.2952755905511804668, 0.1660481256975885056, 0.3530559997133364547 ) ) ;
#22791=CARTESIAN_POINT ( 'NONE',  ( 1.515748031496063186, -0.4536011799217368745, -0.2665933059059886201 ) ) ;
#22792=CARTESIAN_POINT ( 'NONE',  ( -0.6692913385826764205, -0.6692913385826771977, 8.415575281601705876E-17 ) ) ;
#22794=CARTESIAN_POINT ( 'NONE',  ( 1.259842519685040019, -0.1870078740157480879, -0.4822834645669291653 ) ) ;
#22795=CARTESIAN_POINT ( 'NONE',  ( 0.1706036745406830368, 0.05413385826771666132, 0.4176697321401328100 ) ) ;
#22796=CARTESIAN_POINT ( 'NONE',  ( 0.3937007874015754361, -0.1870078740157479769, 0.3641732283464567677 ) ) ;
#22799=CARTESIAN_POINT ( 'NONE',  ( -0.05905511811023545637, 0.07958543189024085140, 0.2665933059059887866 ) ) ;
#22800=CARTESIAN_POINT ( 'NONE',  ( 0.8202099737532813073, 0.1771653543307087630, 0.09757992244046791164 ) ) ;
#22801=B_SPLINE_CURVE_WITH_KNOTS ( 'NONE', 3,
 ( #72419, #77902, #20233, #40424 ),
 .UNSPECIFIED., .F., .F.,
 ( 4, 4 ),
 ( 3.210432057687317930E-07, 0.001287787053612126330 ),
 .UNSPECIFIED. ) ;
#22802=CARTESIAN_POINT ( 'NONE',  ( -1.607611548556429737, 0.2952755905511810774, -0.1292274648535930714 ) ) ;
#22804=CARTESIAN_POINT ( 'NONE',  ( 0.9317585301837276734, 0.05413385826771626580, -0.4176697321401330321 ) ) ;
#22807=CARTESIAN_POINT ( 'NONE',  ( 1.496062992125985147, -0.1870078740157479769, 0.3641732283464567677 ) ) ;
#22809=CARTESIAN_POINT ( 'NONE',  ( 0.07217847769028949700, -0.08942795157528024563, -0.3641732283464568787 ) ) ;
#22810=CARTESIAN_POINT ( 'NONE',  ( 0.2165354330708668673, -0.5400638737290844871, 0.3530559997133364547 ) ) ;
#22811=CARTESIAN_POINT ( 'NONE',  ( 1.581364829396326277, -0.2845877964562161244, -0.3641732283464567121 ) ) ;
#22812=CARTESIAN_POINT ( 'NONE',  ( -1.463254593175852492, -0.5511811023622048555, -0.09757992244046775898 ) ) ;
#22813=CARTESIAN_POINT ( 'NONE',  ( -1.351706036745406347, 0.05413385826771626580, -0.4176697321401330321 ) ) ;
#22814=CARTESIAN_POINT ( 'NONE',  ( 0.5118110236220480003, -0.6692913385826771977, 8.415575281601705876E-17 ) ) ;
#22815=CARTESIAN_POINT ( 'NONE',  ( 1.056430446194226658, 0.2952755905511811885, 0.1292274648535926551 ) ) ;
#22817=CARTESIAN_POINT ( 'NONE',  ( 0.05249343832021075018, 0.2306618581243847221, -0.2411417322834647770 ) ) ;
#22818=CARTESIAN_POINT ( 'NONE',  ( 1.423884514435696413, -0.3162353388693409650, -0.4822834645669289433 ) ) ;
#22819=CARTESIAN_POINT ( 'NONE',  ( 0.9908136482939640111, -0.6692913385826771977, 0.1292274648535927661 ) ) ;
#22820=CARTESIAN_POINT ( 'NONE',  ( -1.614173228346457378, 1.330640075373402897, 0.1372047244094476981 ) ) ;
#22821=CARTESIAN_POINT ( 'NONE',  ( 0.9251968503937015864, 0.07958543189024071263, -0.2665933059059888421 ) ) ;
#22822=CARTESIAN_POINT ( 'NONE',  ( -1.574803149606298192, -0.1870078740157480601, -0.3641732283464567677 ) ) ;
#22823=CARTESIAN_POINT ( 'NONE',  ( -0.1115485564304456306, 0.1771653543307087075, -0.09757992244046823083 ) ) ;
#22824=CARTESIAN_POINT ( 'NONE',  ( 0.2493438320209980519, 0.05413385826771666132, 0.4176697321401328100 ) ) ;
#22825=CARTESIAN_POINT ( 'NONE',  ( 0.5118110236220478892, 0.2952755905511811885, 0.000000000000000000 ) ) ;
#22826=CARTESIAN_POINT ( 'NONE',  ( -0.2362204724409440182, -0.1870078740157479769, 0.4822834645669291653 ) ) ;
#22827=CARTESIAN_POINT ( 'NONE',  ( -0.3018372703412066094, -0.004921259842519576551, 0.3153832671262227771 ) ) ;
#22828=CARTESIAN_POINT ( 'NONE',  ( 0.7020997375328090762, -0.05778040916215560624, -0.4822834645669293319 ) ) ;
#22829=CARTESIAN_POINT ( 'NONE',  ( 0.9973753280839902091, -0.5023911411419708095, 0.1820866141732285504 ) ) ;
#22834=CARTESIAN_POINT ( 'NONE',  ( -1.351706036745406347, -0.4281496062992124485, 0.4176697321401328655 ) ) ;
#22835=CARTESIAN_POINT ( 'NONE',  ( -0.6889763779527552368, -0.5400638737290845981, -0.3530559997133363437 ) ) ;
#22838=EDGE_LOOP ( 'NONE', ( #60563, #45790, #78348, #79512 ) ) ;
#22839=CARTESIAN_POINT ( 'NONE',  ( 0.6299212598425204535, -0.1870078740157480601, -0.3641732283464567677 ) ) ;
#22841=CARTESIAN_POINT ( 'NONE',  ( 1.089238845144357537, -0.4281496062992124485, 0.4176697321401328655 ) ) ;
#22844=CARTESIAN_POINT ( 'NONE',  ( -1.358267716535432434, 0.07958543189024071263, -0.2665933059059888421 ) ) ;
#22845=CARTESIAN_POINT ( 'NONE',  ( 1.581364829396326277, -0.3162353388693409650, -0.4822834645669289433 ) ) ;
#22846=CARTESIAN_POINT ( 'NONE',  ( 1.358267716535433323, -0.4536011799217368745, -0.2665933059059886201 ) ) ;
#22847=CARTESIAN_POINT ( 'NONE',  ( 0.5183727034120741983, -0.6692913385826771977, 0.1292274648535927661 ) ) ;
#22850=CARTESIAN_POINT ( 'NONE',  ( 0.06561679790026316017, -0.4281496062992124485, 0.4176697321401328655 ) ) ;
#22851=CARTESIAN_POINT ( 'NONE',  ( -0.7217847769028863381, -0.004921259842519870586, -0.3153832671262229437 ) ) ;
#22852=CARTESIAN_POINT ( 'NONE',  ( 0.3674540682414705883, 0.2306618581243847221, -0.2411417322834647770 ) ) ;
#22853=CARTESIAN_POINT ( 'NONE',  ( -0.2362204724409442680, -0.1870078740157480879, -0.4822834645669291653 ) ) ;
#22854=CARTESIAN_POINT ( 'NONE',  ( -1.191441481664478497, -1.283732188437465593E-15, -0.4281993546915544568 ) ) ;
#22855=FACE_OUTER_BOUND ( 'NONE', #39438, .T. ) ;
#22857=CARTESIAN_POINT ( 'NONE',  ( 0.8333333333333340365, -0.6692913385826771977, 0.1292274648535927661 ) ) ;
#22858=CARTESIAN_POINT ( 'NONE',  ( -0.07874015748031421014, -0.1870078740157480879, -0.4822834645669291653 ) ) ;
#22859=CARTESIAN_POINT ( 'NONE',  ( -0.9317585301837263412, -0.4281496062992127816, -0.4176697321401328100 ) ) ;
#22860=CARTESIAN_POINT ( 'NONE',  ( 0.9711286089238851948, 0.2306618581243848609, 0.2411417322834645549 ) ) ;
#22861=CARTESIAN_POINT ( 'NONE',  ( 0.4593175853018380828, 0.05413385826771626580, -0.4176697321401330321 ) ) ;
#22863=CARTESIAN_POINT ( 'NONE',  ( -0.5118110236220466680, -0.6692913385826771977, 8.415575281601705876E-17 ) ) ;
#22864=CARTESIAN_POINT ( 'NONE',  ( 0.3280839895013130669, -0.4281496062992127816, -0.4176697321401328100 ) ) ;
#22865=CARTESIAN_POINT ( 'NONE',  ( -0.5774278215223089816, -0.6046776061558807314, 0.2411417322834647770 ) ) ;
#22866=CARTESIAN_POINT ( 'NONE',  ( 0.6299212598425204535, -0.1870078740157480601, -0.3641732283464567677 ) ) ;
#22867=CARTESIAN_POINT ( 'NONE',  ( -1.732283464566928277, -0.1870078740157479769, 0.4822834645669291653 ) ) ;
#22868=DIRECTION ( 'NONE',  ( -0.2810846377148224495, 0.6785983445458426688, -0.6785983445458504404 ) ) ;
#22869=CARTESIAN_POINT ( 'NONE',  ( 0.5314960629921264834, 0.1660481256975883668, -0.3530559997133364547 ) ) ;
#22872=ORIENTED_EDGE ( 'NONE', *, *, #64509, .F. ) ;
#22874=CARTESIAN_POINT ( 'NONE',  ( 0.5577427821522316087, -0.05778040916215522460, 0.4822834645669289988 ) ) ;
#22875=CARTESIAN_POINT ( 'NONE',  ( 0.3937007874015754361, -0.1870078740157480601, -0.3641732283464567677 ) ) ;
#22883=CARTESIAN_POINT ( 'NONE',  ( 0.8333333333333340365, 0.2952755905511810774, -0.1292274648535930714 ) ) ;
#22884=CARTESIAN_POINT ( 'NONE',  ( -0.7480314960629914633, -0.6692913385826771977, 8.415575281601705876E-17 ) ) ;
#22885=CARTESIAN_POINT ( 'NONE',  ( -0.5577427821522301654, -0.05778040916215560624, -0.4822834645669293319 ) ) ;
#22886=CARTESIAN_POINT ( 'NONE',  ( 0.8727034120734912248, -0.3162353388693409650, -0.4822834645669289433 ) ) ;
#22887=CARTESIAN_POINT ( 'NONE',  ( 1.555118110236221041, -0.5400638737290844871, 0.3530559997133364547 ) ) ;
#22888=CARTESIAN_POINT ( 'NONE',  ( 1.181102362204725198, -0.1870078740157479769, 0.3641732283464567677 ) ) ;
#22889=CARTESIAN_POINT ( 'NONE',  ( -1.141732283464566011, 0.1771653543307087630, 0.000000000000000000 ) ) ;
#22891=CARTESIAN_POINT ( 'NONE',  ( 8.195543980992789655E-16, -0.1870078740157480879, -0.4822834645669291653 ) ) ;
#22892=CARTESIAN_POINT ( 'NONE',  ( -0.5611900217179893735, -2.567464376874931580E-15, -0.4445507791589072832 ) ) ;
#22893=DIRECTION ( 'NONE',  ( 3.096699300667737957E-16, -1.000000000000000000, 0.000000000000000000 ) ) ;
#22894=CARTESIAN_POINT ( 'NONE',  ( -1.089238845144356427, -0.004921259842519576551, 0.3153832671262227771 ) ) ;
#22895=CARTESIAN_POINT ( 'NONE',  ( 0.4527559055118117182, 0.1660481256975883668, -0.3530559997133364547 ) ) ;
#22896=CARTESIAN_POINT ( 'NONE',  ( 1.207349081364829990, -0.5023911411419708095, -0.1820866141732282451 ) ) ;
#22898=AXIS2_PLACEMENT_3D ( 'NONE', #40919, #67428, #16923 ) ;
#22899=CARTESIAN_POINT ( 'NONE',  ( -1.069553805774277722, 0.1771653543307087630, 0.09757992244046791164 ) ) ;
#22900=CARTESIAN_POINT ( 'NONE',  ( 1.417322834645670104, -0.1870078740157480879, -0.4822834645669291653 ) ) ;
#22902=CARTESIAN_POINT ( 'NONE',  ( -0.3674540682414692561, -0.6046776061558809534, -0.2411417322834644161 ) ) ;
#22903=CARTESIAN_POINT ( 'NONE',  ( -1.377952755905511140, -0.5511811023622047445, 6.969142054262312111E-17 ) ) ;
#22904=CARTESIAN_POINT ( 'NONE',  ( -0.7349081364829390672, 0.2306618581243847221, -0.2411417322834647770 ) ) ;
#22905=CARTESIAN_POINT ( 'NONE',  ( -1.358267716535432434, -0.4536011799217367080, 0.2665933059059888421 ) ) ;
#22907=CARTESIAN_POINT ( 'NONE',  ( 0.4658792650918640033, -0.3162353388693405765, 0.4822834645669290543 ) ) ;
#22909=CARTESIAN_POINT ( 'NONE',  ( 1.240157480314961314, -0.5400638737290844871, 0.3530559997133364547 ) ) ;
#22911=CARTESIAN_POINT ( 'NONE',  ( -1.397637795275589623, 0.1660481256975885056, 0.3530559997133364547 ) ) ;
#22912=CARTESIAN_POINT ( 'NONE',  ( -0.7414698162729651543, 0.1771653543307087075, -0.09757992244046823083 ) ) ;
#22914=CARTESIAN_POINT ( 'NONE',  ( -0.4921259842519677408, 0.1012011053420775880, -0.2882089793578256898 ) ) ;
#22915=CARTESIAN_POINT ( 'NONE',  ( -0.1640419947506553400, -0.05778040916215560624, -0.4822834645669293319 ) ) ;
#22916=CARTESIAN_POINT ( 'NONE',  ( 0.5774278215223104249, 0.1283753931104748280, 0.1820866141732283561 ) ) ;
#22917=CARTESIAN_POINT ( 'NONE',  ( -1.115485564304461219, -0.3690944881889763329, 0.3153832671262228327 ) ) ;
#22918=CARTESIAN_POINT ( 'NONE',  ( -1.312335958005248715, -0.6046776061558809534, -0.2411417322834644161 ) ) ;
#22919=CARTESIAN_POINT ( 'NONE',  ( -1.633858267716534529, -0.5400638737290845981, -0.3530559997133363437 ) ) ;
#22921=CARTESIAN_POINT ( 'NONE',  ( 1.299212598425197429, -0.6692913385826771977, 8.415575281601705876E-17 ) ) ;
#22923=CARTESIAN_POINT ( 'NONE',  ( 0.3674540682414705883, -0.5023911411419708095, 0.1820866141732285504 ) ) ;
#22924=CARTESIAN_POINT ( 'NONE',  ( 1.082677165354331228, 0.1660481256975883668, -0.3530559997133364547 ) ) ;
#22927=CARTESIAN_POINT ( 'NONE',  ( 1.305774278215223960, 0.1771653543307087075, -0.09757992244046823083 ) ) ;
#22928=ORIENTED_EDGE ( 'NONE', *, *, #42996, .T. ) ;
#22929=CARTESIAN_POINT ( 'NONE',  ( -1.246719160104985846, -0.4281496062992127816, -0.4176697321401328100 ) ) ;
#22930=CARTESIAN_POINT ( 'NONE',  ( -0.9580052493438311334, 0.05413385826771626580, -0.4176697321401330321 ) ) ;
#22931=CARTESIAN_POINT ( 'NONE',  ( 0.2690288713910767848, -0.6692913385826773087, -0.1292274648535924053 ) ) ;
#22934=CARTESIAN_POINT ( 'NONE',  ( 0.8530183727034126306, 0.05413385826771626580, -0.4176697321401330321 ) ) ;
#22935=CARTESIAN_POINT ( 'NONE',  ( 1.443569553805774897, 0.1283753931104748280, 0.1820866141732283561 ) ) ;
#22936=CARTESIAN_POINT ( 'NONE',  ( 0.1640419947506569498, -0.3162353388693409650, -0.4822834645669289433 ) ) ;
#22937=CARTESIAN_POINT ( 'NONE',  ( 0.6364829396325465405, -0.05778040916215522460, 0.4822834645669289988 ) ) ;
#22943=CARTESIAN_POINT ( 'NONE',  ( 0.03280839895013198948, 0.1771653543307087630, 0.09757992244046791164 ) ) ;
#22944=CARTESIAN_POINT ( 'NONE',  ( -0.3083989501312330295, -0.05778040916215522460, 0.4822834645669289988 ) ) ;
#22945=CARTESIAN_POINT ( 'NONE',  ( 1.049868766404200127, -0.6046776061558809534, -0.2411417322834644161 ) ) ;
#22948=CARTESIAN_POINT ( 'NONE',  ( 0.1706036745406830368, -0.3690944881889765550, -0.3153832671262227771 ) ) ;
#22949=CARTESIAN_POINT ( 'NONE',  ( -1.213910761154854745, -0.6692913385826771977, 0.1292274648535927661 ) ) ;
#22950=CARTESIAN_POINT ( 'NONE',  ( 1.358267716535433323, -0.5400638737290845981, -0.3530559997133363437 ) ) ;
#22953=CARTESIAN_POINT ( 'NONE',  ( 0.4848630542936496757, 1.968099216065433366, 0.4919401540133064299 ) ) ;
#22955=CARTESIAN_POINT ( 'NONE',  ( 1.023622047244095112, -0.1870078740157480879, -0.4822834645669291653 ) ) ;
#22957=CARTESIAN_POINT ( 'NONE',  ( 1.220472440944882386, -0.5511811023622047445, 6.969142054262312111E-17 ) ) ;
#22958=CARTESIAN_POINT ( 'NONE',  ( 1.673228346456693494, 0.1660481256975885056, 0.3530559997133364547 ) ) ;
#22959=CARTESIAN_POINT ( 'NONE',  ( -1.627296587926508442, 0.2306618581243848609, 0.2411417322834645549 ) ) ;
#22962=CARTESIAN_POINT ( 'NONE',  ( 1.181102362204725198, -0.1870078740157479769, 0.4822834645669291653 ) ) ;
#22963=CARTESIAN_POINT ( 'NONE',  ( -1.666666666666665853, 0.05413385826771626580, -0.4176697321401330321 ) ) ;
#22964=CARTESIAN_POINT ( 'NONE',  ( -0.5905511811023615998, 0.2952755905511811885, 0.000000000000000000 ) ) ;
#22965=CARTESIAN_POINT ( 'NONE',  ( -0.5183727034120726440, -0.6692913385826773087, -0.1292274648535924053 ) ) ;
#22966=CARTESIAN_POINT ( 'NONE',  ( 1.423884514435696191, -0.05778040916215522460, 0.4822834645669289988 ) ) ;
#22968=CARTESIAN_POINT ( 'NONE',  ( 0.1181102362204730916, -0.6692913385826771977, 8.415575281601705876E-17 ) ) ;
#22970=CARTESIAN_POINT ( 'NONE',  ( 1.482939632545932307, -0.4281496062992124485, 0.4176697321401328655 ) ) ;
#22973=EDGE_LOOP ( 'NONE', ( #76073, #71015, #22582, #78080 ) ) ;
#22975=CARTESIAN_POINT ( 'NONE',  ( -1.699475065616797398, 0.2952755905511811885, 0.1292274648535926551 ) ) ;
#22977=CARTESIAN_POINT ( 'NONE',  ( -1.646051170424378096, 0.000000000000000000, 0.3464511005275205946 ) ) ;
#22978=CARTESIAN_POINT ( 'NONE',  ( -0.1450607720586916394, 0.000000000000000000, 0.3464511005275205946 ) ) ;
#22979=CARTESIAN_POINT ( 'NONE',  ( 0.4527559055118117182, 0.1660481256975883391, -0.3530559997133364547 ) ) ;
#22980=CARTESIAN_POINT ( 'NONE',  ( 0.9337842054690638216, -6.978086149529499157E-16, -0.3954974714151469617 ) ) ;
#22982=( BOUNDED_CURVE ( )  B_SPLINE_CURVE ( 2, ( #48381, #79997, #60609, #2958, #73673, #28623, #22311 ),
 .UNSPECIFIED., .F., .F. ) 
 B_SPLINE_CURVE_WITH_KNOTS ( ( 3, 2, 2, 3 ),
 ( 0.1363636363636363535, 0.1401515151515151381, 0.1439393939393939503, 0.1448507235470174181 ),
 .UNSPECIFIED. ) 
 CURVE ( )  GEOMETRIC_REPRESENTATION_ITEM ( )  RATIONAL_B_SPLINE_CURVE ( ( 1.000000000000000000, 0.9659258262890683122, 1.000000000000000000, 0.9659258262890683122, 1.000000000000000000, 0.9918020599134675930, 0.9875488213027519002 ) ) 
 REPRESENTATION_ITEM ( '' )  );
#22983=CARTESIAN_POINT ( 'NONE',  ( -0.3543307086614165824, 0.1771653543307087630, 0.000000000000000000 ) ) ;
#22984=CARTESIAN_POINT ( 'NONE',  ( -1.410761154855642463, -0.08942795157527998196, 0.3641732283464567121 ) ) ;
#22985=CARTESIAN_POINT ( 'NONE',  ( -1.220472440944881054, -0.6692913385826771977, 8.415575281601705876E-17 ) ) ;
#22986=CARTESIAN_POINT ( 'NONE',  ( 0.3608923884514443348, 0.2952755905511810774, -0.1292274648535930714 ) ) ;
#22987=CARTESIAN_POINT ( 'NONE',  ( -1.351706036745406347, -0.4281496062992124485, 0.4176697321401328655 ) ) ;
#22988=AXIS2_PLACEMENT_3D ( 'NONE', #9287, #29865, #2971 ) ;
#22991=CARTESIAN_POINT ( 'NONE',  ( -1.240157480314959759, -0.5400638737290845981, -0.3530559997133363437 ) ) ;
#22992=DIRECTION ( 'NONE',  ( -3.096699300667737957E-16, 1.000000000000000000, -0.000000000000000000 ) ) ;
#22996=DIRECTION ( 'NONE',  ( -0.7071067811865487940, 0.000000000000000000, 0.7071067811865463515 ) ) ;
#22997=CARTESIAN_POINT ( 'NONE',  ( -0.6364829396325453192, -0.05778040916215560624, -0.4822834645669293319 ) ) ;
#22998=CARTESIAN_POINT ( 'NONE',  ( 1.384514435695538559, 0.2952755905511810774, -0.1292274648535930714 ) ) ;
#22999=CARTESIAN_POINT ( 'NONE',  ( -1.732283464566928277, -0.1870078740157479769, 0.4822834645669291653 ) ) ;
#23001=CARTESIAN_POINT ( 'NONE',  ( 1.456692913385827515, -0.6692913385826771977, 8.415575281601705876E-17 ) ) ;
#23002=CARTESIAN_POINT ( 'NONE',  ( -0.6692913385826764205, -0.6692913385826771977, 8.415575281601705876E-17 ) ) ;
#23004=CARTESIAN_POINT ( 'NONE',  ( 0.006561679790026889343, -0.08942795157527998196, 0.3641732283464567121 ) ) ;
#23006=CARTESIAN_POINT ( 'NONE',  ( -0.2493438320209966919, -0.3690944881889763329, 0.3153832671262228327 ) ) ;
#23007=CARTESIAN_POINT ( 'NONE',  ( 0.8005249343832027131, -0.004921259842519576551, 0.3153832671262227771 ) ) ;
#23008=CARTESIAN_POINT ( 'NONE',  ( 0.5905511811023629321, -0.6692913385826771977, 8.415575281601705876E-17 ) ) ;
#23009=CARTESIAN_POINT ( 'NONE',  ( -0.1640419947506553400, -0.08942795157528024563, -0.3641732283464568787 ) ) ;
#23011=CARTESIAN_POINT ( 'NONE',  ( -1.646981627296586703, -0.05778040916215522460, 0.4822834645669289988 ) ) ;
#23012=CARTESIAN_POINT ( 'NONE',  ( -1.200787401574802349, -0.4536011799217367080, 0.2665933059059888421 ) ) ;
#23014=CARTESIAN_POINT ( 'NONE',  ( 0.1902887139107617975, 0.2952755905511811885, 0.1292274648535926551 ) ) ;
#23015=EDGE_CURVE ( 'NONE', #35589, #23460, #81482, .T. ) ;
#23016=CARTESIAN_POINT ( 'NONE',  ( -0.4330708661417315697, -0.6692913385826771977, 8.415575281601705876E-17 ) ) ;
#23017=CARTESIAN_POINT ( 'NONE',  ( 1.614173228346457378, -0.5511811023622047445, 6.969142054262312111E-17 ) ) ;
#23018=CARTESIAN_POINT ( 'NONE',  ( 0.01968503937007930540, 0.07958543189024085140, 0.2665933059059887866 ) ) ;
#23019=CARTESIAN_POINT ( 'NONE',  ( -0.1968503937007867743, -0.6692913385826771977, 8.415575281601705876E-17 ) ) ;
#23020=CARTESIAN_POINT ( 'NONE',  ( -0.5511811023622038563, -0.1870078740157479769, 0.4822834645669291653 ) ) ;
#23023=CARTESIAN_POINT ( 'NONE',  ( 0.3543307086614181922, -0.6692913385826771977, 8.415575281601705876E-17 ) ) ;
#23026=CARTESIAN_POINT ( 'NONE',  ( 1.469816272965879911, 0.2306618581243847221, -0.2411417322834647770 ) ) ;
#23027=CARTESIAN_POINT ( 'NONE',  ( -0.5643044619422565855, -0.004921259842519870586, -0.3153832671262229437 ) ) ;
#23028=CARTESIAN_POINT ( 'NONE',  ( -0.4790026246719154557, -0.3162353388693405765, 0.4822834645669290543 ) ) ;
#23029=CARTESIAN_POINT ( 'NONE',  ( -1.646981627296586703, -0.08942795157527998196, 0.3641732283464567121 ) ) ;
#23030=CARTESIAN_POINT ( 'NONE',  ( 1.463254593175853824, -0.6692913385826771977, 0.1292274648535927661 ) ) ;
#23031=CARTESIAN_POINT ( 'NONE',  ( -1.463254593175852492, 0.2952755905511811885, 0.1292274648535926551 ) ) ;
#23032=CARTESIAN_POINT ( 'NONE',  ( -0.8727034120734901146, -0.08942795157528024563, -0.3641732283464568787 ) ) ;
#23036=CARTESIAN_POINT ( 'NONE',  ( 1.391076115485564868, 0.1283753931104746893, -0.1820866141732285504 ) ) ;
#23037=CARTESIAN_POINT ( 'NONE',  ( 1.299212598425197429, 0.1771653543307087630, 0.000000000000000000 ) ) ;
#23038=CARTESIAN_POINT ( 'NONE',  ( 1.023622047244095112, -0.1870078740157480879, -0.4822834645669291653 ) ) ;
#23039=CARTESIAN_POINT ( 'NONE',  ( 0.4593175853018379717, 0.009842519685039147898, -0.3409548833797004797 ) ) ;
#23040=CARTESIAN_POINT ( 'NONE',  ( 0.8727034120734912248, -0.3162353388693409650, -0.4822834645669289433 ) ) ;
#23042=CARTESIAN_POINT ( 'NONE',  ( 1.246719160104987623, -0.004921259842519870586, -0.3153832671262229437 ) ) ;
#23043=CARTESIAN_POINT ( 'NONE',  ( 0.2624671916010504757, 0.2306618581243848609, 0.2411417322834645549 ) ) ;
#23044=CARTESIAN_POINT ( 'NONE',  ( -0.8530183727034112984, 0.05413385826771666132, 0.4176697321401328100 ) ) ;
#23045=CARTESIAN_POINT ( 'NONE',  ( 1.312335958005250269, -0.6046776061558807314, 0.2411417322834647770 ) ) ;
#23048=CARTESIAN_POINT ( 'NONE',  ( 0.2493438320209980519, -0.3690944881889765550, -0.3153832671262227771 ) ) ;
#23052=CARTESIAN_POINT ( 'NONE',  ( -0.8333333333333323711, -0.6692913385826773087, -0.1292274648535924053 ) ) ;
#23053=CARTESIAN_POINT ( 'NONE',  ( -0.3937007874015740483, -0.1870078740157479769, 0.4822834645669291653 ) ) ;
#23054=CARTESIAN_POINT ( 'NONE',  ( -0.3215223097112853146, -0.05778040916215560624, -0.4822834645669293319 ) ) ;
#23055=CARTESIAN_POINT ( 'NONE',  ( 0.7611548556430454138, 0.2306618581243847221, -0.2411417322834647770 ) ) ;
#23056=CARTESIAN_POINT ( 'NONE',  ( -0.8464566929133852113, 0.1660481256975885056, 0.3530559997133364547 ) ) ;
#23057=CARTESIAN_POINT ( 'NONE',  ( -0.5971128608923877978, 0.2952755905511811885, 0.1292274648535926551 ) ) ;
#23058=CARTESIAN_POINT ( 'NONE',  ( 1.194225721784777594, -0.4281496062992127816, -0.4176697321401328100 ) ) ;
#23059=CARTESIAN_POINT ( 'NONE',  ( 0.4921259842519691285, 0.1660481256975885056, 0.3530559997133364547 ) ) ;
#23060=CARTESIAN_POINT ( 'NONE',  ( 0.6364829396325465405, -0.3162353388693409650, -0.4822834645669289433 ) ) ;
#23062=CARTESIAN_POINT ( 'NONE',  ( -0.5643044619422565855, -0.3690944881889763329, 0.3153832671262228327 ) ) ;
#23065=VERTEX_POINT ( 'NONE', #75480 ) ;
#23066=CARTESIAN_POINT ( 'NONE',  ( -0.6955380577427815458, -0.3690944881889765550, -0.3153832671262227771 ) ) ;
#23067=CARTESIAN_POINT ( 'NONE',  ( -0.3280839895013117347, 0.05413385826771626580, -0.4176697321401330321 ) ) ;
#23069=CARTESIAN_POINT ( 'NONE',  ( -0.5446194225721777693, -0.3162353388693409650, -0.4822834645669289433 ) ) ;
#23070=CARTESIAN_POINT ( 'NONE',  ( -1.010498687664041384, -0.4281496062992127816, -0.4176697321401328100 ) ) ;
#23071=CARTESIAN_POINT ( 'NONE',  ( -1.338582677165353729, -0.1870078740157479769, 0.4822834645669291653 ) ) ;
#23072=CARTESIAN_POINT ( 'NONE',  ( -1.259842519685038686, -0.1870078740157479769, 0.4822834645669291653 ) ) ;
#23073=CARTESIAN_POINT ( 'NONE',  ( 0.7611548556430454138, 0.1283753931104746893, -0.1820866141732285504 ) ) ;
#23075=CARTESIAN_POINT ( 'NONE',  ( -1.600415083108464254, 2.375314266909943406, 0.1324231768467336867 ) ) ;
#23076=CARTESIAN_POINT ( 'NONE',  ( 0.4527559055118117182, -0.4536011799217367080, 0.2665933059059888421 ) ) ;
#23077=CARTESIAN_POINT ( 'NONE',  ( 0.2362204724409456558, -0.1870078740157479769, 0.4822834645669291653 ) ) ;
#23078=CARTESIAN_POINT ( 'NONE',  ( -0.1574803149606292529, -0.1870078740157480879, -0.4822834645669291653 ) ) ;
#23080=AXIS2_PLACEMENT_3D ( 'NONE', #39324, #1458, #624 ) ;
#23083=ORIENTED_EDGE ( 'NONE', *, *, #17293, .F. ) ;
#23085=CARTESIAN_POINT ( 'NONE',  ( 1.614173228346457378, 0.2952755905511811885, 0.000000000000000000 ) ) ;
#23086=CARTESIAN_POINT ( 'NONE',  ( -0.9251968503937002541, 0.07958543189024085140, 0.2665933059059887866 ) ) ;
#23087=CARTESIAN_POINT ( 'NONE',  ( -1.023622047244094002, -0.1870078740157480879, -0.4822834645669291653 ) ) ;
#23091=CARTESIAN_POINT ( 'NONE',  ( -1.502624671916009680, -0.2845877964562159024, 0.3641732283464567677 ) ) ;
#23092=CARTESIAN_POINT ( 'NONE',  ( 0.4790026246719167324, -0.05778040916215522460, 0.4822834645669289988 ) ) ;
#23093=CARTESIAN_POINT ( 'NONE',  ( 0.5249343832021005074, -0.6046776061558807314, 0.2411417322834647770 ) ) ;
#23094=CARTESIAN_POINT ( 'NONE',  ( -0.5380577427821514602, -0.004921259842519576551, 0.3153832671262227771 ) ) ;
#23095=CARTESIAN_POINT ( 'NONE',  ( -0.07874015748031421014, -0.1870078740157480879, -0.4822834645669291653 ) ) ;
#23097=CARTESIAN_POINT ( 'NONE',  ( -0.5118110236220466680, -0.6692913385826771977, 8.415575281601705876E-17 ) ) ;
#23099=CARTESIAN_POINT ( 'NONE',  ( 1.259842519685040019, -0.1870078740157479769, 0.3641732283464567677 ) ) ;
#23100=CARTESIAN_POINT ( 'NONE',  ( 0.1443569553805781891, -0.3690944881889763329, 0.3153832671262228327 ) ) ;
#23101=CARTESIAN_POINT ( 'NONE',  ( 1.213910761154856299, 0.1771653543307087630, 0.09757992244046791164 ) ) ;
#23102=CARTESIAN_POINT ( 'NONE',  ( -0.9711286089238838626, -0.6046776061558807314, 0.2411417322834647770 ) ) ;
#23103=CARTESIAN_POINT ( 'NONE',  ( -1.332020997375327642, -0.08942795157527998196, 0.3641732283464567121 ) ) ;
#23104=CARTESIAN_POINT ( 'NONE',  ( -1.614173228346457378, 0.7166040191147894367, 0.1372047244094476981 ) ) ;
#23105=CARTESIAN_POINT ( 'NONE',  ( -1.253280839895012377, -0.05778040916215522460, 0.4822834645669289988 ) ) ;
#23106=CARTESIAN_POINT ( 'NONE',  ( -0.5971128608923877978, -0.6692913385826773087, -0.1292274648535924053 ) ) ;
#23107=EDGE_CURVE ( 'NONE', #25632, #44077, #34222, .T. ) ;
#23108=( BOUNDED_CURVE ( )  B_SPLINE_CURVE ( 1, ( #9425, #60761 ),
 .UNSPECIFIED., .F., .F. ) 
 B_SPLINE_CURVE_WITH_KNOTS ( ( 2, 2 ),
 ( 0.0007457734483630323874, 0.002000000000000001776 ),
 .UNSPECIFIED. ) 
 CURVE ( )  GEOMETRIC_REPRESENTATION_ITEM ( )  RATIONAL_B_SPLINE_CURVE ( ( 0.9875488213027523443, 0.9875488213027523443 ) ) 
 REPRESENTATION_ITEM ( '' )  );
#23109=CARTESIAN_POINT ( 'NONE',  ( 0.3280839895013130669, -0.4281496062992127816, -0.4176697321401328100 ) ) ;
#23112=CARTESIAN_POINT ( 'NONE',  ( 0.1771653543307093182, -0.4536011799217368745, -0.2665933059059886201 ) ) ;
#23113=CARTESIAN_POINT ( 'NONE',  ( 0.8595800524934390507, -0.05778040916215560624, -0.4822834645669293319 ) ) ;
#23115=CARTESIAN_POINT ( 'NONE',  ( 0.5380577427821529035, -0.4281496062992124485, 0.4176697321401328655 ) ) ;
#23116=CARTESIAN_POINT ( 'NONE',  ( -1.528871391076114250, 0.1771653543307087075, -0.09757992244046823083 ) ) ;
#23117=CARTESIAN_POINT ( 'NONE',  ( -1.397637795275589623, 0.1660481256975885056, 0.3530559997133364547 ) ) ;
#23118=CARTESIAN_POINT ( 'NONE',  ( -1.056430446194224881, 0.2952755905511810774, -0.1292274648535930714 ) ) ;
#23119=CARTESIAN_POINT ( 'NONE',  ( -0.4068241469816264999, -0.3690944881889763329, 0.3153832671262228327 ) ) ;
#23121=CARTESIAN_POINT ( 'NONE',  ( 0.7480314960629927956, -0.5511811023622047445, 6.969142054262312111E-17 ) ) ;
#23122=CARTESIAN_POINT ( 'NONE',  ( -0.1509186351706028884, -0.3162353388693409650, -0.4822834645669289433 ) ) ;
#23124=CARTESIAN_POINT ( 'NONE',  ( -1.181102362204723644, -0.1870078740157480879, -0.4822834645669291653 ) ) ;
#23126=CARTESIAN_POINT ( 'NONE',  ( 0.8792650918635177559, -0.3690944881889765550, -0.3153832671262227771 ) ) ;
#23127=CARTESIAN_POINT ( 'NONE',  ( 0.01312335958005323398, -0.4281496062992127816, -0.4176697321401328100 ) ) ;
#23128=CARTESIAN_POINT ( 'NONE',  ( -0.4133858267716528645, -0.5400638737290844871, 0.3530559997133364547 ) ) ;
#23129=CARTESIAN_POINT ( 'NONE',  ( -0.5905511811023613777, -0.5511811023622047445, 6.969142054262312111E-17 ) ) ;
#23131=CARTESIAN_POINT ( 'NONE',  ( -0.5577427821522301654, -0.2845877964562159024, 0.3641732283464567677 ) ) ;
#23132=CARTESIAN_POINT ( 'NONE',  ( 0.4330708661417329575, 0.2952755905511811885, 0.000000000000000000 ) ) ;
#23133=CARTESIAN_POINT ( 'NONE',  ( -0.9776902887139098386, -0.5511811023622046335, 0.09757992244046803654 ) ) ;
#23135=CARTESIAN_POINT ( 'NONE',  ( 1.548556430446194954, -0.6046776061558807314, 0.2411417322834647770 ) ) ;
#23137=CARTESIAN_POINT ( 'NONE',  ( -1.725721784776902190, -0.08942795157527998196, 0.3641732283464567121 ) ) ;
#23138=CARTESIAN_POINT ( 'NONE',  ( -0.4199475065616791736, 0.2306618581243847221, -0.2411417322834647770 ) ) ;
#23139=CARTESIAN_POINT ( 'NONE',  ( -1.076115485564303809, -0.6046776061558809534, -0.2411417322834644161 ) ) ;
#23142=CARTESIAN_POINT ( 'NONE',  ( 1.437007874015748810, -0.5400638737290845981, -0.3530559997133363437 ) ) ;
#23143=CARTESIAN_POINT ( 'NONE',  ( 0.3608923884514443348, -0.6692913385826771977, 0.1292274648535927661 ) ) ;
#23146=CARTESIAN_POINT ( 'NONE',  ( 1.522309711286089939, -0.5023911411419708095, -0.1820866141732282451 ) ) ;
#23149=CARTESIAN_POINT ( 'NONE',  ( -1.069553805774277722, -0.5511811023622048555, -0.09757992244046775898 ) ) ;
#23151=VERTEX_POINT ( 'NONE', #11503 ) ;
#23152=CARTESIAN_POINT ( 'NONE',  ( 0.7874015748031503170, -0.1870078740157479769, 0.4822834645669291653 ) ) ;
#23153=CARTESIAN_POINT ( 'NONE',  ( -0.3543307086614165824, -0.6692913385826771977, 8.415575281601705876E-17 ) ) ;
#23154=CARTESIAN_POINT ( 'NONE',  ( -1.017060367454067249, -0.05778040916215522460, 0.4822834645669289988 ) ) ;
#23155=CARTESIAN_POINT ( 'NONE',  ( 1.076115485564305141, 0.2306618581243847221, -0.2411417322834647770 ) ) ;
#23156=CARTESIAN_POINT ( 'NONE',  ( -1.141732283464566011, 0.1771653543307087630, 0.000000000000000000 ) ) ;
#23158=CARTESIAN_POINT ( 'NONE',  ( 0.1902887139107617975, -0.6692913385826773087, -0.1292274648535924053 ) ) ;
#23159=CARTESIAN_POINT ( 'NONE',  ( -0.8858267716535425107, -0.5400638737290844871, 0.3530559997133364547 ) ) ;
#23163=CARTESIAN_POINT ( 'NONE',  ( 1.062992125984252745, 0.2952755905511811885, 0.000000000000000000 ) ) ;
#23165=CARTESIAN_POINT ( 'NONE',  ( 1.312335958005250269, -0.5023911411419708095, 0.1820866141732285504 ) ) ;
#23168=CARTESIAN_POINT ( 'NONE',  ( -0.5118110236220466680, 0.2952755905511811885, 0.000000000000000000 ) ) ;
#23170=CARTESIAN_POINT ( 'NONE',  ( 0.3215223097112867578, -0.08942795157527998196, 0.3641732283464567121 ) ) ;
#23171=CARTESIAN_POINT ( 'NONE',  ( -1.443569553805773564, -0.6046776061558807314, 0.2411417322834647770 ) ) ;
#23172=CARTESIAN_POINT ( 'NONE',  ( 0.6036745406824153282, -0.6046776061558807314, 0.2411417322834647770 ) ) ;
#23173=CARTESIAN_POINT ( 'NONE',  ( 0.7152230971128614723, -0.3162353388693409650, -0.4822834645669289433 ) ) ;
#23174=CARTESIAN_POINT ( 'NONE',  ( -0.01312335958005186876, -0.4281496062992124485, 0.4176697321401328655 ) ) ;
#23176=CARTESIAN_POINT ( 'NONE',  ( -0.6299212598425188991, -0.1870078740157480879, -0.4822834645669291653 ) ) ;
#23178=CARTESIAN_POINT ( 'NONE',  ( -1.541994750656167090, 0.2952755905511811885, 0.1292274648535926551 ) ) ;
#23179=CARTESIAN_POINT ( 'NONE',  ( -0.8989501312335946848, -0.6692913385826771977, 0.1292274648535927661 ) ) ;
#23180=CARTESIAN_POINT ( 'NONE',  ( 1.404199475065617708, 0.05413385826771626580, -0.4176697321401330321 ) ) ;
#23181=CARTESIAN_POINT ( 'NONE',  ( 1.082677165354331228, 0.1660481256975883668, -0.3530559997133364547 ) ) ;
#23183=CARTESIAN_POINT ( 'NONE',  ( -1.128608923884513837, -0.6046776061558807314, 0.2411417322834647770 ) ) ;
#23185=CARTESIAN_POINT ( 'NONE',  ( 0.1574803149606306130, -0.1870078740157479769, 0.4822834645669291653 ) ) ;
#23187=CARTESIAN_POINT ( 'NONE',  ( -0.4330708661417315697, -0.6692913385826771977, 8.415575281601705876E-17 ) ) ;
#23188=CARTESIAN_POINT ( 'NONE',  ( 1.660104986876641320, -0.05778040916215522460, 0.4822834645669289988 ) ) ;
#23189=CARTESIAN_POINT ( 'NONE',  ( 0.6430446194225729606, -0.3690944881889765550, -0.3153832671262227771 ) ) ;
#23190=CARTESIAN_POINT ( 'NONE',  ( 1.325459317585302665, 0.05413385826771626580, -0.4176697321401330321 ) ) ;
#23192=CARTESIAN_POINT ( 'NONE',  ( 0.5774278215223104249, 0.1283753931104748280, 0.1820866141732283561 ) ) ;
#23193=CARTESIAN_POINT ( 'NONE',  ( 0.9251968503937015864, -0.5400638737290844871, 0.3530559997133364547 ) ) ;
#23194=VECTOR ( 'NONE', #15877, 39.37007874015748143 ) ;
#23196=CARTESIAN_POINT ( 'NONE',  ( -0.8792650918635160906, 0.05413385826771626580, -0.4176697321401330321 ) ) ;
#23197=CARTESIAN_POINT ( 'NONE',  ( -1.614173228346457378, 2.157411728916712068, 0.1372047244094476981 ) ) ;
#23198=CARTESIAN_POINT ( 'NONE',  ( 1.240157480314961314, -0.4536011799217367080, 0.2665933059059888421 ) ) ;
#23199=CARTESIAN_POINT ( 'NONE',  ( -0.7742782152230965886, 0.05413385826771666132, 0.4176697321401328100 ) ) ;
#23200=CARTESIAN_POINT ( 'NONE',  ( 0.1706036745406830368, 0.05413385826771666132, 0.4176697321401328100 ) ) ;
#23201=CARTESIAN_POINT ( 'NONE',  ( 0.1443569553805781891, 0.009842519685039147898, -0.3409548833797004797 ) ) ;
#23202=CARTESIAN_POINT ( 'NONE',  ( 0.07217847769028949700, -0.05778040916215560624, -0.4822834645669293319 ) ) ;
#23203=CARTESIAN_POINT ( 'NONE',  ( 0.3280839895013130669, -0.3690944881889765550, -0.3153832671262227771 ) ) ;
#23204=FACE_OUTER_BOUND ( 'NONE', #37674, .T. ) ;
#23205=CARTESIAN_POINT ( 'NONE',  ( 0.05249343832021075018, -0.5023911411419708095, 0.1820866141732285504 ) ) ;
#23206=CARTESIAN_POINT ( 'NONE',  ( 0.8792650918635177559, -0.3690944881889765550, -0.3153832671262227771 ) ) ;
#23209=CARTESIAN_POINT ( 'NONE',  ( 0.4986876640419954376, -0.6046776061558809534, -0.2411417322834644161 ) ) ;
#23210=ADVANCED_FACE ( 'NONE', ( #62841 ), #70703, .F. ) ;
#23212=CARTESIAN_POINT ( 'NONE',  ( 1.541994750656168645, 0.1771653543307087075, -0.09757992244046823083 ) ) ;
#23214=CARTESIAN_POINT ( 'NONE',  ( 0.08530183727034192087, -0.2845877964562161244, -0.3641732283464567121 ) ) ;
#23215=CARTESIAN_POINT ( 'NONE',  ( 0.08530183727034192087, -0.05778040916215522460, 0.4822834645669289988 ) ) ;
#23216=CARTESIAN_POINT ( 'NONE',  ( 1.259842519685040019, -0.1870078740157480601, -0.3641732283464567677 ) ) ;
#23217=CARTESIAN_POINT ( 'NONE',  ( -1.332020997375327642, -0.2845877964562161244, -0.3641732283464567121 ) ) ;
#23218=CARTESIAN_POINT ( 'NONE',  ( -1.299212598425196097, -0.6692913385826771977, 8.415575281601705876E-17 ) ) ;
#23219=CARTESIAN_POINT ( 'NONE',  ( 0.2296587926509192634, -0.3162353388693405765, 0.4822834645669290543 ) ) ;
#23220=CARTESIAN_POINT ( 'NONE',  ( 1.167979002624672580, -0.4281496062992124485, 0.4176697321401328655 ) ) ;
#23221=CARTESIAN_POINT ( 'NONE',  ( 1.595398199321655275, 1.309738123151863665, -0.1559797534342494130 ) ) ;
#23222=CARTESIAN_POINT ( 'NONE',  ( 0.3608923884514443348, 0.2952755905511810774, -0.1292274648535930714 ) ) ;
#23223=CARTESIAN_POINT ( 'NONE',  ( 1.272965879265092637, -0.4281496062992127816, -0.4176697321401328100 ) ) ;
#23224=CARTESIAN_POINT ( 'NONE',  ( 1.102362204724410155, -0.1870078740157480879, -0.4822834645669291653 ) ) ;
#23225=CARTESIAN_POINT ( 'NONE',  ( -1.673228346456691717, 0.07958543189024071263, -0.2665933059059888421 ) ) ;
#23226=CARTESIAN_POINT ( 'NONE',  ( 0.8727034120734913358, -0.08942795157527998196, 0.3641732283464567121 ) ) ;
#23227=CARTESIAN_POINT ( 'NONE',  ( 1.482939632545932307, -0.4281496062992124485, 0.4176697321401328655 ) ) ;
#23228=CARTESIAN_POINT ( 'NONE',  ( -0.04593175853018302557, -0.5511811023622048555, -0.09757992244046775898 ) ) ;
#23229=CARTESIAN_POINT ( 'NONE',  ( -0.4396325459317577122, -0.6692913385826773087, -0.1292274648535924053 ) ) ;
#23230=CARTESIAN_POINT ( 'NONE',  ( 0.6167979002624678353, -0.4281496062992124485, 0.4176697321401328655 ) ) ;
#23231=CARTESIAN_POINT ( 'NONE',  ( -0.3215223097112853146, -0.05778040916215560624, -0.4822834645669293319 ) ) ;
#23233=EDGE_CURVE ( 'NONE', #13300, #8463, #51821, .T. ) ;
#23235=CARTESIAN_POINT ( 'NONE',  ( -0.1837270341207343505, -0.5023911411419708095, 0.1820866141732285504 ) ) ;
#23236=CARTESIAN_POINT ( 'NONE',  ( 0.6102362204724416372, -0.5400638737290844871, 0.3530559997133364547 ) ) ;
#23237=CARTESIAN_POINT ( 'NONE',  ( 1.030183727034121421, -0.08942795157527998196, 0.3641732283464567121 ) ) ;
#23239=CARTESIAN_POINT ( 'NONE',  ( -1.732283464566928277, -0.1870078740157479769, 0.3641732283464567677 ) ) ;
#23242=CARTESIAN_POINT ( 'NONE',  ( -1.161417322834644716, 0.1660481256975885056, 0.3530559997133364547 ) ) ;
#23243=CARTESIAN_POINT ( 'NONE',  ( -0.5314960629921254842, -0.5400638737290845981, -0.3530559997133363437 ) ) ;
#23247=CARTESIAN_POINT ( 'NONE',  ( 0.5052493438320218022, -0.5511811023622048555, -0.09757992244046775898 ) ) ;
#23250=CARTESIAN_POINT ( 'NONE',  ( 1.305774278215223960, 0.2952755905511810774, -0.1292274648535930714 ) ) ;
#23252=CARTESIAN_POINT ( 'NONE',  ( 1.614173228346457378, 0.7166040191147859950, -0.1372047244094476148 ) ) ;
#23253=CARTESIAN_POINT ( 'NONE',  ( -0.2952755905511805223, 0.1660481256975885056, 0.3530559997133364547 ) ) ;
#23254=CARTESIAN_POINT ( 'NONE',  ( 1.686351706036745890, 0.2952755905511811885, 0.1292274648535926551 ) ) ;
#23255=CARTESIAN_POINT ( 'NONE',  ( 1.253280839895013710, -0.2845877964562159024, 0.3641732283464567677 ) ) ;
#23256=CARTESIAN_POINT ( 'NONE',  ( 0.3346456692913393205, -0.5400638737290845981, -0.3530559997133363437 ) ) ;
#23258=CARTESIAN_POINT ( 'NONE',  ( 0.07217847769028949700, -0.3162353388693405765, 0.4822834645669290543 ) ) ;
#23259=CARTESIAN_POINT ( 'NONE',  ( -0.8070866141732276899, -0.4536011799217367080, 0.2665933059059888421 ) ) ;
#23261=CARTESIAN_POINT ( 'NONE',  ( 0.5380577427821529035, 0.05413385826771626580, -0.4176697321401330321 ) ) ;
#23262=CARTESIAN_POINT ( 'NONE',  ( -0.1706036745406816491, -0.4281496062992124485, 0.4176697321401328655 ) ) ;
#23263=CARTESIAN_POINT ( 'NONE',  ( -1.614173228346456712, 2.094556775020298467, -0.1372047244094478091 ) ) ;
#23266=CARTESIAN_POINT ( 'NONE',  ( 0.7086614173228353852, -0.1870078740157479769, 0.4822834645669291653 ) ) ;
#23267=CARTESIAN_POINT ( 'NONE',  ( -0.3215223097112853146, -0.3162353388693405765, 0.4822834645669290543 ) ) ;
#23268=CARTESIAN_POINT ( 'NONE',  ( -1.345144356955379816, -0.3162353388693405765, 0.4822834645669290543 ) ) ;
#23269=CARTESIAN_POINT ( 'NONE',  ( 1.200787401574803681, -0.5400638737290845981, -0.3530559997133363437 ) ) ;
#23270=CARTESIAN_POINT ( 'NONE',  ( 0.5708661417322842269, 0.1660481256975885056, 0.3530559997133364547 ) ) ;
#23272=CARTESIAN_POINT ( 'NONE',  ( -0.3280839895013117347, -0.4281496062992124485, 0.4176697321401328655 ) ) ;
#23273=CARTESIAN_POINT ( 'NONE',  ( 0.1706036745406830368, -0.4281496062992127816, -0.4176697321401328100 ) ) ;
#23274=CARTESIAN_POINT ( 'NONE',  ( -0.3871391076115476282, -0.05778040916215522460, 0.4822834645669289988 ) ) ;
#23275=CARTESIAN_POINT ( 'NONE',  ( 0.4658792650918641698, -0.08942795157528024563, -0.3641732283464568787 ) ) ;
#23276=CARTESIAN_POINT ( 'NONE',  ( 1.627296587926509996, -0.5023911411419708095, 0.1820866141732285504 ) ) ;
#23278=CARTESIAN_POINT ( 'NONE',  ( 0.4724409448818904789, -0.1870078740157479769, 0.4822834645669291653 ) ) ;
#23279=( NAMED_UNIT ( * ) PLANE_ANGLE_UNIT ( ) SI_UNIT ( $, .RADIAN. ) );
#23280=CARTESIAN_POINT ( 'NONE',  ( 1.345144356955381593, -0.3162353388693409650, -0.4822834645669289433 ) ) ;
#23284=CARTESIAN_POINT ( 'NONE',  ( 0.5839895013123367340, 0.2952755905511811885, 0.1292274648535926551 ) ) ;
#23285=CARTESIAN_POINT ( 'NONE',  ( 0.3805774278215230400, -0.004921259842519870586, -0.3153832671262229437 ) ) ;
#23286=CARTESIAN_POINT ( 'NONE',  ( 1.686351706036745890, 0.1771653543307087630, 0.09757992244046791164 ) ) ;
#23292=CARTESIAN_POINT ( 'NONE',  ( 0.7283464566929140904, -0.5400638737290845981, -0.3530559997133363437 ) ) ;
#23293=CARTESIAN_POINT ( 'NONE',  ( -0.7545931758530176614, -0.6692913385826773087, -0.1292274648535924053 ) ) ;
#23295=CARTESIAN_POINT ( 'NONE',  ( -0.7742782152230965886, 0.05413385826771666132, 0.4176697321401328100 ) ) ;
#23296=CARTESIAN_POINT ( 'NONE',  ( 0.4724409448818904789, -0.1870078740157479769, 0.4822834645669291653 ) ) ;
#23297=CARTESIAN_POINT ( 'NONE',  ( 1.266404199475066328, -0.05778040916215522460, 0.4822834645669289988 ) ) ;
#23300=CARTESIAN_POINT ( 'NONE',  ( 1.364829396325460076, 0.1283753931104748280, 0.1820866141732283561 ) ) ;
#23302=CARTESIAN_POINT ( 'NONE',  ( -1.489501312335957062, -0.08942795157527998196, 0.3641732283464567121 ) ) ;
#23303=CARTESIAN_POINT ( 'NONE',  ( 1.604771003085129433, 0.7690346235818159570, 0.1466069496707750608 ) ) ;
#23304=CARTESIAN_POINT ( 'NONE',  ( 0.3346456692913393205, -0.5400638737290845981, -0.3530559997133363437 ) ) ;
#23305=CARTESIAN_POINT ( 'NONE',  ( 1.102362204724410155, -0.1870078740157480879, -0.4822834645669291653 ) ) ;
#23307=CARTESIAN_POINT ( 'NONE',  ( -1.358267716535432434, 0.07958543189024071263, -0.2665933059059888421 ) ) ;
#23308=CARTESIAN_POINT ( 'NONE',  ( 0.3280839895013130669, -0.4281496062992127816, -0.4176697321401328100 ) ) ;
#23309=CARTESIAN_POINT ( 'NONE',  ( 1.089238845144357537, -0.3690944881889763329, 0.3153832671262228327 ) ) ;
#23312=CARTESIAN_POINT ( 'NONE',  ( -1.358267716535432434, 0.07958543189024071263, -0.2665933059059888421 ) ) ;
#23313=CARTESIAN_POINT ( 'NONE',  ( 1.377952755905512472, 0.2952755905511811885, 0.000000000000000000 ) ) ;
#23315=CARTESIAN_POINT ( 'NONE',  ( 0.07874015748031558404, -0.1870078740157480601, -0.3641732283464567677 ) ) ;
#23316=CARTESIAN_POINT ( 'NONE',  ( -0.07217847769028813698, -0.3162353388693409650, -0.4822834645669289433 ) ) ;
#23317=CARTESIAN_POINT ( 'NONE',  ( -1.167979002624671470, -0.004921259842519576551, 0.3153832671262227771 ) ) ;
#23318=CARTESIAN_POINT ( 'NONE',  ( -0.7545931758530177724, 0.2952755905511811885, 0.1292274648535926551 ) ) ;
#23319=CARTESIAN_POINT ( 'NONE',  ( 1.345144356955381593, -0.05778040916215522460, 0.4822834645669289988 ) ) ;
#23322=CARTESIAN_POINT ( 'NONE',  ( 1.312335958005249825, 0.2306618581243847221, -0.2411417322834647770 ) ) ;
#23324=CARTESIAN_POINT ( 'NONE',  ( -1.069553805774277722, 0.2952755905511811885, 0.1292274648535926551 ) ) ;
#23325=CARTESIAN_POINT ( 'NONE',  ( -1.141732283464566011, 0.1771653543307087630, 0.000000000000000000 ) ) ;
#23326=CARTESIAN_POINT ( 'NONE',  ( -0.5446194225721777693, -0.2845877964562161244, -0.3641732283464567121 ) ) ;
#23328=CARTESIAN_POINT ( 'NONE',  ( 0.02624671916010564918, -0.6046776061558809534, -0.2411417322834644161 ) ) ;
#23329=CARTESIAN_POINT ( 'NONE',  ( -0.01968503937007793844, 0.07958543189024071263, -0.2665933059059888421 ) ) ;
#23330=CARTESIAN_POINT ( 'NONE',  ( -1.161417322834644716, -0.4536011799217368745, -0.2665933059059886201 ) ) ;
#23331=CARTESIAN_POINT ( 'NONE',  ( -1.548556430446193399, 0.2306618581243848609, 0.2411417322834645549 ) ) ;
#23332=CARTESIAN_POINT ( 'NONE',  ( 1.482939632545932307, -0.004921259842519870586, -0.3153832671262229437 ) ) ;
#23333=CARTESIAN_POINT ( 'NONE',  ( 1.266404199475066328, -0.3162353388693409650, -0.4822834645669289433 ) ) ;
#23335=CARTESIAN_POINT ( 'NONE',  ( 0.6102362204724416372, 0.07958543189024071263, -0.2665933059059888421 ) ) ;
#23336=CARTESIAN_POINT ( 'NONE',  ( 0.8136482939632553313, -0.6046776061558809534, -0.2411417322834644161 ) ) ;
#23338=CARTESIAN_POINT ( 'NONE',  ( 0.8661417322834652488, -0.1870078740157480601, -0.3641732283464567677 ) ) ;
#23339=ORIENTED_EDGE ( 'NONE', *, *, #42958, .F. ) ;
#23340=CARTESIAN_POINT ( 'NONE',  ( -1.377952755905511140, -0.6692913385826771977, 8.415575281601705876E-17 ) ) ;
#23341=CARTESIAN_POINT ( 'NONE',  ( -0.7152230971128602510, -0.3162353388693405765, 0.4822834645669290543 ) ) ;
#23342=CARTESIAN_POINT ( 'NONE',  ( -0.1968503937007867743, -0.6692913385826771977, 8.415575281601705876E-17 ) ) ;
#23345=CARTESIAN_POINT ( 'NONE',  ( 0.8398950131233602345, 0.2306618581243847221, -0.2411417322834647770 ) ) ;
#23346=CARTESIAN_POINT ( 'NONE',  ( 1.318897637795276356, 0.07958543189024071263, -0.2665933059059888421 ) ) ;
#23347=CARTESIAN_POINT ( 'NONE',  ( -0.1246719160104980823, -0.6692913385826773087, -0.1292274648535924053 ) ) ;
#23348=CARTESIAN_POINT ( 'NONE',  ( 0.8858267716535438430, -0.5400638737290845981, -0.3530559997133363437 ) ) ;
#23355=CARTESIAN_POINT ( 'NONE',  ( -0.5249343832020990641, -0.5023911411419708095, -0.1820866141732282451 ) ) ;
#23356=CARTESIAN_POINT ( 'NONE',  ( -0.5774278215223089816, 0.2306618581243847221, -0.2411417322834647770 ) ) ;
#23357=CARTESIAN_POINT ( 'NONE',  ( 1.043307086614173818, -0.5400638737290845981, -0.3530559997133363437 ) ) ;
#23359=CARTESIAN_POINT ( 'NONE',  ( -1.574803149606298192, -0.1870078740157480879, -0.4822834645669291653 ) ) ;
#23360=CARTESIAN_POINT ( 'NONE',  ( 1.030183727034121421, -0.3162353388693409650, -0.4822834645669289433 ) ) ;
#23365=CARTESIAN_POINT ( 'NONE',  ( 0.8858267716535438430, -0.5400638737290845981, -0.3530559997133363437 ) ) ;
#23367=CARTESIAN_POINT ( 'NONE',  ( 1.102362204724410155, -0.1870078740157479769, 0.3641732283464567677 ) ) ;
#23369=CARTESIAN_POINT ( 'NONE',  ( 1.607611548556431069, -0.6692913385826773087, -0.1292274648535924053 ) ) ;
#23370=CARTESIAN_POINT ( 'NONE',  ( -1.489501312335957062, -0.05778040916215522460, 0.4822834645669289988 ) ) ;
#23373=CARTESIAN_POINT ( 'NONE',  ( 0.9055118110236227702, 0.2952755905511811885, 0.000000000000000000 ) ) ;
#23374=CARTESIAN_POINT ( 'NONE',  ( 1.371391076115485941, 0.1771653543307087630, 0.09757992244046791164 ) ) ;
#23375=CARTESIAN_POINT ( 'NONE',  ( -0.3674540682414692561, -0.6046776061558809534, -0.2411417322834644161 ) ) ;
#23376=CARTESIAN_POINT ( 'NONE',  ( -0.4790026246719154557, -0.3162353388693405765, 0.4822834645669290543 ) ) ;
#23377=CARTESIAN_POINT ( 'NONE',  ( 1.541994750656168645, -0.6692913385826771977, 0.1292274648535927661 ) ) ;
#23379=CARTESIAN_POINT ( 'NONE',  ( 0.1049868766404206816, -0.6046776061558809534, -0.2411417322834644161 ) ) ;
#23381=CARTESIAN_POINT ( 'NONE',  ( 1.646981627296588035, -0.3162353388693405765, 0.4822834645669290543 ) ) ;
#23382=ORIENTED_EDGE ( 'NONE', *, *, #79680, .T. ) ;
#23386=CARTESIAN_POINT ( 'NONE',  ( -1.679790026246718693, 0.2306618581243847221, -0.2411417322834647770 ) ) ;
#23388=CARTESIAN_POINT ( 'NONE',  ( 1.679790026246720025, 0.1283753931104748280, 0.1820866141732283561 ) ) ;
#23389=CARTESIAN_POINT ( 'NONE',  ( -0.1049868766404193215, 0.1539470093639521697, -0.1968503937007875793 ) ) ;
#23390=CARTESIAN_POINT ( 'NONE',  ( 0.4037097067573611753, 1.223219560026271499E-15, 0.4445507791589056734 ) ) ;
#23391=CARTESIAN_POINT ( 'NONE',  ( 0.9333857237505069904, -6.978086149529499157E-16, -0.3791475997938232867 ) ) ;
#23394=CARTESIAN_POINT ( 'NONE',  ( -0.1443569553805765515, -0.3690944881889765550, -0.3153832671262227771 ) ) ;
#23395=CARTESIAN_POINT ( 'NONE',  ( -1.003937007874015297, -0.4536011799217368745, -0.2665933059059886201 ) ) ;
#23396=CARTESIAN_POINT ( 'NONE',  ( 1.522309711286089939, -0.6046776061558809534, -0.2411417322834644161 ) ) ;
#23398=CARTESIAN_POINT ( 'NONE',  ( 0.4265091863517067039, -0.6692913385826773087, -0.1292274648535924053 ) ) ;
#23399=CARTESIAN_POINT ( 'NONE',  ( -1.535433070866141225, -0.6692913385826771977, 8.415575281601705876E-17 ) ) ;
#23401=ORIENTED_EDGE ( 'NONE', *, *, #36816, .F. ) ;
#23402=CARTESIAN_POINT ( 'NONE',  ( 1.450131233595801428, 0.2952755905511811885, 0.1292274648535926551 ) ) ;
#23403=CARTESIAN_POINT ( 'NONE',  ( -1.586052503253845503, 2.125984251968505045, -0.1653254495020588799 ) ) ;
#23406=PLANE ( 'NONE',  #35853 ) ;
#23407=CARTESIAN_POINT ( 'NONE',  ( -0.7808398950131222316, -0.3162353388693409650, -0.4822834645669289433 ) ) ;
#23408=CARTESIAN_POINT ( 'NONE',  ( 1.515748031496063408, 0.1660481256975885056, 0.3530559997133364547 ) ) ;
#23409=CARTESIAN_POINT ( 'NONE',  ( -0.7186703366786194591, -2.567464376874931580E-15, -0.4445507791589072832 ) ) ;
#23411=CARTESIAN_POINT ( 'NONE',  ( 1.587926509186352586, -0.4281496062992127816, -0.4176697321401328100 ) ) ;
#23412=CARTESIAN_POINT ( 'NONE',  ( -0.7152230971128602510, -0.05778040916215560624, -0.4822834645669293319 ) ) ;
#23414=CARTESIAN_POINT ( 'NONE',  ( -0.01968503937007793844, -0.4536011799217367080, 0.2665933059059888421 ) ) ;
#23417=CARTESIAN_POINT ( 'NONE',  ( -0.1902887139107604098, 0.1771653543307087075, -0.09757992244046823083 ) ) ;
#23418=CARTESIAN_POINT ( 'NONE',  ( 0.5971128608923890191, -0.5511811023622046335, 0.09757992244046803654 ) ) ;
#23419=CARTESIAN_POINT ( 'NONE',  ( 0.3412073490813655186, 0.2306618581243848609, 0.2411417322834645549 ) ) ;
#23420=CARTESIAN_POINT ( 'NONE',  ( -0.1509186351706028884, -0.2845877964562161244, -0.3641732283464567121 ) ) ;
#23422=CARTESIAN_POINT ( 'NONE',  ( 1.496062992125984703, -0.1870078740157480879, -0.4822834645669291653 ) ) ;
#23424=CARTESIAN_POINT ( 'NONE',  ( -1.030183727034119867, -0.3162353388693405765, 0.4822834645669290543 ) ) ;
#23426=CARTESIAN_POINT ( 'NONE',  ( -0.09842519685039295696, 0.1660481256975883668, -0.3530559997133364547 ) ) ;
#23427=CARTESIAN_POINT ( 'NONE',  ( -0.3477690288713902178, 0.2952755905511810774, -0.1292274648535930714 ) ) ;
#23428=CARTESIAN_POINT ( 'NONE',  ( 1.587926509186352586, -0.3690944881889765550, -0.3153832671262227771 ) ) ;
#23430=CARTESIAN_POINT ( 'NONE',  ( -0.08530183727034056085, -0.08942795157528024563, -0.3641732283464568787 ) ) ;
#23431=CARTESIAN_POINT ( 'NONE',  ( -0.3149606299212590610, -0.1870078740157479769, 0.4822834645669291653 ) ) ;
#23432=CARTESIAN_POINT ( 'NONE',  ( -0.7283464566929126471, -0.5400638737290844871, 0.3530559997133364547 ) ) ;
#23433=CARTESIAN_POINT ( 'NONE',  ( 1.522309711286089939, 0.1283753931104748280, 0.1820866141732283561 ) ) ;
#23434=CARTESIAN_POINT ( 'NONE',  ( 0.09842519685039434474, 0.1660481256975885056, 0.3530559997133364547 ) ) ;
#23438=CARTESIAN_POINT ( 'NONE',  ( 0.9842519685039375910, 0.2952755905511811885, 0.000000000000000000 ) ) ;
#23439=CARTESIAN_POINT ( 'NONE',  ( -0.4790026246719154557, -0.2845877964562159024, 0.3641732283464567677 ) ) ;
#23440=CARTESIAN_POINT ( 'NONE',  ( -0.7677165354330699465, 0.1660481256975885056, 0.3530559997133364547 ) ) ;
#23441=CARTESIAN_POINT ( 'NONE',  ( 1.174540682414699111, -0.3162353388693405765, 0.4822834645669290543 ) ) ;
#23442=CARTESIAN_POINT ( 'NONE',  ( 0.7742782152230979209, 0.05413385826771626580, -0.4176697321401330321 ) ) ;
#23443=CARTESIAN_POINT ( 'NONE',  ( -1.614173228346455824, 0.2952755905511811885, 0.000000000000000000 ) ) ;
#23444=CARTESIAN_POINT ( 'NONE',  ( -0.9448818897637790704, -0.1870078740157479769, 0.3641732283464567677 ) ) ;
#23449=CARTESIAN_POINT ( 'NONE',  ( 1.036745406824147508, -0.3690944881889765550, -0.3153832671262227771 ) ) ;
#23450=CARTESIAN_POINT ( 'NONE',  ( 0.5052493438320215802, 0.2952755905511811885, 0.1292274648535926551 ) ) ;
#23451=CARTESIAN_POINT ( 'NONE',  ( -1.555118110236219930, 0.1660481256975885056, 0.3530559997133364547 ) ) ;
#23453=CARTESIAN_POINT ( 'NONE',  ( 0.5971128608923891301, 0.1771653543307087075, -0.09757992244046823083 ) ) ;
#23454=CARTESIAN_POINT ( 'NONE',  ( -0.3871391076115476282, -0.05778040916215522460, 0.4822834645669289988 ) ) ;
#23455=CARTESIAN_POINT ( 'NONE',  ( -0.8398950131233585692, 0.2306618581243848609, 0.2411417322834645549 ) ) ;
#23456=CARTESIAN_POINT ( 'NONE',  ( 1.253280839895013710, -0.05778040916215560624, -0.4822834645669293319 ) ) ;
#23459=CARTESIAN_POINT ( 'NONE',  ( -0.1837270341207343505, -0.5023911411419708095, 0.1820866141732285504 ) ) ;
#23460=VERTEX_POINT ( 'NONE', #32496 ) ;
#23462=ORIENTED_EDGE ( 'NONE', *, *, #34284, .T. ) ;
#23463=CARTESIAN_POINT ( 'NONE',  ( -0.9973753280839886548, -0.6046776061558809534, -0.2411417322834644161 ) ) ;
#23464=CARTESIAN_POINT ( 'NONE',  ( -0.05249343832020911260, 0.2306618581243848609, 0.2411417322834645549 ) ) ;
#23465=CARTESIAN_POINT ( 'NONE',  ( -0.1706036745406816491, 0.05413385826771626580, -0.4176697321401330321 ) ) ;
#23466=VECTOR ( 'NONE', #43991, 39.37007874015748143 ) ;
#23467=CARTESIAN_POINT ( 'NONE',  ( 0.9120734908136490793, 0.2952755905511810774, -0.1292274648535930714 ) ) ;
#23468=CARTESIAN_POINT ( 'NONE',  ( -0.5249343832020990641, 0.2306618581243848609, 0.2411417322834645549 ) ) ;
#23469=CARTESIAN_POINT ( 'NONE',  ( -1.154855643044618851, 0.2306618581243848609, 0.2411417322834645549 ) ) ;
#23470=CARTESIAN_POINT ( 'NONE',  ( -0.4593175853018366950, 0.05413385826771666132, 0.4176697321401328100 ) ) ;
#23471=CARTESIAN_POINT ( 'NONE',  ( 0.5577427821522314977, -0.3162353388693409650, -0.4822834645669289433 ) ) ;
#23472=CARTESIAN_POINT ( 'NONE',  ( 0.6102362204724416372, -0.5400638737290844871, 0.3530559997133364547 ) ) ;
#23474=CARTESIAN_POINT ( 'NONE',  ( -0.2230971128608915943, -0.004921259842519576551, 0.3153832671262227771 ) ) ;
#23475=ORIENTED_EDGE ( 'NONE', *, *, #61940, .T. ) ;
#23478=CARTESIAN_POINT ( 'NONE',  ( -1.404199475065615932, -0.004921259842519576551, 0.3153832671262227771 ) ) ;
#23479=CARTESIAN_POINT ( 'NONE',  ( -0.4855643044619415427, 0.05413385826771626580, -0.4176697321401330321 ) ) ;
#23481=CARTESIAN_POINT ( 'NONE',  ( -0.5708661417322828946, 0.1660481256975883668, -0.3530559997133364547 ) ) ;
#23482=CARTESIAN_POINT ( 'NONE',  ( -0.9120734908136475250, 0.2952755905511811885, 0.1292274648535926551 ) ) ;
#23483=CARTESIAN_POINT ( 'NONE',  ( -1.305774278215222184, 0.2952755905511811885, 0.1292274648535926551 ) ) ;
#23487=CARTESIAN_POINT ( 'NONE',  ( 0.7939632545931766261, -0.2845877964562161244, -0.3641732283464567121 ) ) ;
#23490=CARTESIAN_POINT ( 'NONE',  ( 0.1246719160104994284, -0.5511811023622046335, 0.09757992244046803654 ) ) ;
#23491=CARTESIAN_POINT ( 'NONE',  ( -0.4265091863517051496, -0.6692913385826771977, 0.1292274648535927661 ) ) ;
#23492=CARTESIAN_POINT ( 'NONE',  ( 0.006561679790026889343, -0.3162353388693409650, -0.4822834645669289433 ) ) ;
#23493=VERTEX_POINT ( 'NONE', #13573 ) ;
#23495=CARTESIAN_POINT ( 'NONE',  ( -0.5708661417322828946, 0.1012011053420775880, -0.2882089793578257453 ) ) ;
#23496=ORIENTED_EDGE ( 'NONE', *, *, #61689, .T. ) ;
#23499=CARTESIAN_POINT ( 'NONE',  ( -0.8858267716535425107, 0.07958543189024071263, -0.2665933059059888421 ) ) ;
#23500=CARTESIAN_POINT ( 'NONE',  ( -1.161417322834644716, -0.5400638737290845981, -0.3530559997133363437 ) ) ;
#23504=CARTESIAN_POINT ( 'NONE',  ( 1.299212598425197429, -0.6692913385826771977, 8.415575281601705876E-17 ) ) ;
#23505=CARTESIAN_POINT ( 'NONE',  ( 0.5380577427821529035, 0.05413385826771626580, -0.4176697321401330321 ) ) ;
#23506=CARTESIAN_POINT ( 'NONE',  ( 0.6430446194225729606, -0.4281496062992127816, -0.4176697321401328100 ) ) ;
#23507=CARTESIAN_POINT ( 'NONE',  ( -0.8530183727034112984, -0.004921259842519576551, 0.3153832671262227771 ) ) ;
#23508=CARTESIAN_POINT ( 'NONE',  ( -0.4986876640419942164, -0.6046776061558807314, 0.2411417322834647770 ) ) ;
#23510=CARTESIAN_POINT ( 'NONE',  ( -0.2690288713910754526, 0.2952755905511810774, -0.1292274648535930714 ) ) ;
#23512=CARTESIAN_POINT ( 'NONE',  ( 1.161417322834646271, 0.07958543189024071263, -0.2665933059059888421 ) ) ;
#23513=CARTESIAN_POINT ( 'NONE',  ( -0.2296587926509179312, -0.2845877964562161244, -0.3641732283464567121 ) ) ;
#23514=CARTESIAN_POINT ( 'NONE',  ( 1.194225721784777594, -0.004921259842519576551, 0.3153832671262227771 ) ) ;
#23515=CARTESIAN_POINT ( 'NONE',  ( -1.115485564304461219, -0.4281496062992124485, 0.4176697321401328655 ) ) ;
#23516=CARTESIAN_POINT ( 'NONE',  ( -1.089238845144356427, -0.3690944881889765550, -0.3153832671262227771 ) ) ;
#23518=CARTESIAN_POINT ( 'NONE',  ( -1.292650918635170010, -0.6692913385826771977, 0.1292274648535927661 ) ) ;
#23519=CARTESIAN_POINT ( 'NONE',  ( -0.2362204724409440182, -0.1870078740157479769, 0.4822834645669291653 ) ) ;
#23520=CARTESIAN_POINT ( 'NONE',  ( 0.4265091863517067594, 0.2952755905511811885, 0.1292274648535926551 ) ) ;
#23522=CARTESIAN_POINT ( 'NONE',  ( 0.4002624671916016896, -0.08942795157527998196, 0.3641732283464567121 ) ) ;
#23523=CARTESIAN_POINT ( 'NONE',  ( -1.660104986876639543, -0.08942795157528024563, -0.3641732283464568787 ) ) ;
#23524=CARTESIAN_POINT ( 'NONE',  ( 0.9186351706036752773, 0.2306618581243847221, -0.2411417322834647770 ) ) ;
#23525=CARTESIAN_POINT ( 'NONE',  ( -1.548556430446193399, 0.1283753931104748280, 0.1820866141732283561 ) ) ;
#23526=CARTESIAN_POINT ( 'NONE',  ( 1.515748031496063186, -0.4536011799217368745, -0.2665933059059886201 ) ) ;
#23527=CARTESIAN_POINT ( 'NONE',  ( -1.076115485564303809, 0.2306618581243848609, 0.2411417322834645549 ) ) ;
#23528=CARTESIAN_POINT ( 'NONE',  ( -0.4265091863517051496, -0.5511811023622046335, 0.09757992244046803654 ) ) ;
#23529=DIRECTION ( 'NONE',  ( 0.000000000000000000, 0.000000000000000000, -1.000000000000000000 ) ) ;
#23530=CARTESIAN_POINT ( 'NONE',  ( 0.2296587926509192634, -0.08942795157528024563, -0.3641732283464568787 ) ) ;
#23532=CARTESIAN_POINT ( 'NONE',  ( -0.2624671916010490880, -0.6046776061558807314, 0.2411417322834647770 ) ) ;
#23535=CARTESIAN_POINT ( 'NONE',  ( 0.6167979002624678353, -0.3690944881889763329, 0.3153832671262228327 ) ) ;
#23536=CARTESIAN_POINT ( 'NONE',  ( 0.1115485564304470323, 0.2952755905511811885, 0.1292274648535926551 ) ) ;
#23537=CARTESIAN_POINT ( 'NONE',  ( -0.7086614173228339419, -0.1870078740157479769, 0.4822834645669291653 ) ) ;
#23538=CARTESIAN_POINT ( 'NONE',  ( -0.7874015748031489847, -0.1870078740157480601, -0.3641732283464567677 ) ) ;
#23539=DIRECTION ( 'NONE',  ( 3.096699300667737957E-16, -1.000000000000000000, 0.000000000000000000 ) ) ;
#23540=CARTESIAN_POINT ( 'NONE',  ( -0.5118110236220466680, 0.1771653543307087630, 0.000000000000000000 ) ) ;
#23541=CARTESIAN_POINT ( 'NONE',  ( 0.04593175853018440641, -0.6692913385826771977, 0.1292274648535927661 ) ) ;
#23542=CARTESIAN_POINT ( 'NONE',  ( -1.082677165354329896, 0.07958543189024085140, 0.2665933059059887866 ) ) ;
#23543=VECTOR ( 'NONE', #67593, 39.37007874015748143 ) ;
#23545=CARTESIAN_POINT ( 'NONE',  ( -1.423884514435694859, -0.05778040916215560624, -0.4822834645669293319 ) ) ;
#23546=CARTESIAN_POINT ( 'NONE',  ( 0.4617417521217854204, 1.990046790791744833E-15, -0.4118477457932984698 ) ) ;
#23548=CARTESIAN_POINT ( 'NONE',  ( -1.430446194225721390, -0.3690944881889763329, 0.3153832671262228327 ) ) ;
#23549=CARTESIAN_POINT ( 'NONE',  ( -0.2952755905511804668, 0.1660481256975885056, 0.3530559997133364547 ) ) ;
#23550=CARTESIAN_POINT ( 'NONE',  ( -1.003937007874014853, 0.1660481256975885056, 0.3530559997133364547 ) ) ;
#23553=CARTESIAN_POINT ( 'NONE',  ( 1.227034120734908917, 0.2952755905511810774, -0.1292274648535930714 ) ) ;
#23554=CARTESIAN_POINT ( 'NONE',  ( 0.3280839895013130669, -0.4281496062992127816, -0.4176697321401328100 ) ) ;
#23557=CARTESIAN_POINT ( 'NONE',  ( -1.633858267716534529, -0.5400638737290845981, -0.3530559997133363437 ) ) ;
#23559=ORIENTED_EDGE ( 'NONE', *, *, #9067, .T. ) ;
#23560=CARTESIAN_POINT ( 'NONE',  ( -0.7217847769028863381, -0.3690944881889763329, 0.3153832671262228327 ) ) ;
#23563=CARTESIAN_POINT ( 'NONE',  ( 0.5183727034120741983, 0.2952755905511810774, -0.1292274648535930714 ) ) ;
#23564=CARTESIAN_POINT ( 'NONE',  ( -0.2362204724409442680, -0.1870078740157480879, -0.4822834645669291653 ) ) ;
#23565=CARTESIAN_POINT ( 'NONE',  ( -1.135170603674539924, 0.2952755905511810774, -0.1292274648535930714 ) ) ;
#23566=CARTESIAN_POINT ( 'NONE',  ( 0.9055118110236227702, 0.2952755905511811885, 0.000000000000000000 ) ) ;
#23567=CARTESIAN_POINT ( 'NONE',  ( -1.279527559055116948, 0.07958543189024071263, -0.2665933059059888421 ) ) ;
#23569=CARTESIAN_POINT ( 'NONE',  ( 0.03280839895013198948, -0.6692913385826773087, -0.1292274648535924053 ) ) ;
#23570=CARTESIAN_POINT ( 'NONE',  ( -1.259842519685038686, -0.1870078740157480879, -0.4822834645669291653 ) ) ;
#23572=FACE_OUTER_BOUND ( 'NONE', #45227, .T. ) ;
#23575=CARTESIAN_POINT ( 'NONE',  ( 0.9251968503937015864, 0.07958543189024071263, -0.2665933059059888421 ) ) ;
#23576=ORIENTED_EDGE ( 'NONE', *, *, #28526, .T. ) ;
#23578=CARTESIAN_POINT ( 'NONE',  ( -0.9186351706036736120, -0.6046776061558809534, -0.2411417322834644161 ) ) ;
#23580=CARTESIAN_POINT ( 'NONE',  ( 0.5971128608923890191, -0.5511811023622046335, 0.09757992244046803654 ) ) ;
#23581=CARTESIAN_POINT ( 'NONE',  ( -1.732283464566928277, -0.1870078740157479769, 0.4822834645669291653 ) ) ;
#23582=CARTESIAN_POINT ( 'NONE',  ( 0.4790026246719167324, -0.05778040916215522460, 0.4822834645669289988 ) ) ;
#23583=CARTESIAN_POINT ( 'NONE',  ( 0.3608923884514443348, 0.2952755905511810774, -0.1292274648535930714 ) ) ;
#23584=EDGE_CURVE ( 'NONE', #36616, #65086, #30177, .T. ) ;
#23585=CARTESIAN_POINT ( 'NONE',  ( -0.2427821522309703550, -0.05778040916215560624, -0.4822834645669293319 ) ) ;
#23587=CARTESIAN_POINT ( 'NONE',  ( -0.5839895013123351797, -0.6692913385826771977, 0.1292274648535927661 ) ) ;
#23589=CARTESIAN_POINT ( 'NONE',  ( 1.128608923884514947, 0.1283753931104748280, 0.1820866141732283561 ) ) ;
#23590=CARTESIAN_POINT ( 'NONE',  ( -1.082677165354329896, -0.5400638737290845981, -0.3530559997133363437 ) ) ;
#23591=CARTESIAN_POINT ( 'NONE',  ( 1.430446194225722500, -0.4281496062992127816, -0.4176697321401328100 ) ) ;
#23592=CARTESIAN_POINT ( 'NONE',  ( 1.253280839895013710, -0.05778040916215560624, -0.4822834645669293319 ) ) ;
#23594=CARTESIAN_POINT ( 'NONE',  ( -0.9580052493438311334, -0.4281496062992124485, 0.4176697321401328655 ) ) ;
#23596=CARTESIAN_POINT ( 'NONE',  ( 0.3871391076115492380, -0.05778040916215560624, -0.4822834645669293319 ) ) ;
#23599=CARTESIAN_POINT ( 'NONE',  ( -0.6955380577427815458, 0.05413385826771666132, 0.4176697321401328100 ) ) ;
#23601=CARTESIAN_POINT ( 'NONE',  ( 1.568241469816273659, -0.05778040916215560624, -0.4822834645669293319 ) ) ;
#23602=CARTESIAN_POINT ( 'NONE',  ( 0.4921259842519691285, -0.4536011799217368745, -0.2665933059059886201 ) ) ;
#23603=CARTESIAN_POINT ( 'NONE',  ( 1.141732283464567566, 0.2952755905511811885, 0.000000000000000000 ) ) ;
#23605=CARTESIAN_POINT ( 'NONE',  ( 0.8398950131233602345, -0.5023911411419708095, 0.1820866141732285504 ) ) ;
#23606=CARTESIAN_POINT ( 'NONE',  ( 0.8398950131233602345, 0.2306618581243847221, -0.2411417322834647770 ) ) ;
#23608=CARTESIAN_POINT ( 'NONE',  ( -0.6496062992125976043, -0.5400638737290844871, 0.3530559997133364547 ) ) ;
#23610=CARTESIAN_POINT ( 'NONE',  ( 0.8333333333333340365, 0.1771653543307087075, -0.09757992244046823083 ) ) ;
#23611=CARTESIAN_POINT ( 'NONE',  ( -0.5446194225721777693, -0.3162353388693409650, -0.4822834645669289433 ) ) ;
#23612=CARTESIAN_POINT ( 'NONE',  ( -0.02624671916010428221, -0.6046776061558807314, 0.2411417322834647770 ) ) ;
#23614=CARTESIAN_POINT ( 'NONE',  ( 0.2034120734908142214, 0.2952755905511810774, -0.1292274648535930714 ) ) ;
#23615=CARTESIAN_POINT ( 'NONE',  ( 0.2559055118110243332, 0.07958543189024085140, 0.2665933059059887866 ) ) ;
#23617=CARTESIAN_POINT ( 'NONE',  ( -0.07874015748031421014, -0.1870078740157479769, 0.3641732283464567677 ) ) ;
#23618=CARTESIAN_POINT ( 'NONE',  ( 0.6430446194225728496, -0.004921259842519576551, 0.3153832671262227771 ) ) ;
#23619=CARTESIAN_POINT ( 'NONE',  ( 1.586052503253845281, 1.299212598425198095, 0.1653254495020587411 ) ) ;
#23621=CARTESIAN_POINT ( 'NONE',  ( 0.2755905511811031494, 0.2952755905511811885, 0.000000000000000000 ) ) ;
#23623=CARTESIAN_POINT ( 'NONE',  ( 0.2242874410717144995, -4.069555009745408348E-17, -0.3627989612356146698 ) ) ;
#23625=CARTESIAN_POINT ( 'NONE',  ( -0.3805774278215216522, -0.3690944881889765550, -0.3153832671262227771 ) ) ;
#23626=CARTESIAN_POINT ( 'NONE',  ( -0.4658792650918627265, -0.3162353388693409650, -0.4822834645669289433 ) ) ;
#23627=CARTESIAN_POINT ( 'NONE',  ( 0.9120734908136490793, 0.1771653543307087075, -0.09757992244046823083 ) ) ;
#23628=CARTESIAN_POINT ( 'NONE',  ( -1.699475065616797398, 0.1771653543307087630, 0.09757992244046791164 ) ) ;
#23629=CARTESIAN_POINT ( 'NONE',  ( -1.233595800524933894, 0.2306618581243848609, 0.2411417322834645549 ) ) ;
#23630=CARTESIAN_POINT ( 'NONE',  ( -0.01312335958005186876, 0.05413385826771626580, -0.4176697321401330321 ) ) ;
#23631=CARTESIAN_POINT ( 'NONE',  ( 1.194225721784777594, 0.05413385826771666132, 0.4176697321401328100 ) ) ;
#23632=CARTESIAN_POINT ( 'NONE',  ( 0.3346456692913390985, 0.1660481256975885056, 0.3530559997133364547 ) ) ;
#23633=VECTOR ( 'NONE', #25580, 39.37007874015748143 ) ;
#23634=CARTESIAN_POINT ( 'NONE',  ( 1.325459317585302665, -0.4281496062992124485, 0.4176697321401328655 ) ) ;
#23635=AXIS2_PLACEMENT_3D ( 'NONE', #53736, #77775, #52488 ) ;
#23636=CARTESIAN_POINT ( 'NONE',  ( 0.4527559055118117182, 0.1660481256975883668, -0.3530559997133364547 ) ) ;
#23637=CARTESIAN_POINT ( 'NONE',  ( -1.725721784776902190, -0.08942795157527998196, 0.3641732283464567121 ) ) ;
#23638=CARTESIAN_POINT ( 'NONE',  ( 0.9186351706036752773, 0.1283753931104746893, -0.1820866141732285504 ) ) ;
#23639=CARTESIAN_POINT ( 'NONE',  ( 1.568241469816273659, -0.05778040916215560624, -0.4822834645669293319 ) ) ;
#23640=CARTESIAN_POINT ( 'NONE',  ( 0.2165354330708668673, 0.07958543189024071263, -0.2665933059059888421 ) ) ;
#23641=CARTESIAN_POINT ( 'NONE',  ( -0.2624671916010490880, -0.6046776061558807314, 0.2411417322834647770 ) ) ;
#23642=CARTESIAN_POINT ( 'NONE',  ( 0.6692913385826777528, 0.2952755905511811885, 0.000000000000000000 ) ) ;
#23643=CARTESIAN_POINT ( 'NONE',  ( -0.4593175853018364174, -0.4281496062992127816, -0.4176697321401328100 ) ) ;
#23645=CARTESIAN_POINT ( 'NONE',  ( -0.2887139107611542133, 0.1283753931104748280, 0.1820866141732283561 ) ) ;
#23646=CARTESIAN_POINT ( 'NONE',  ( 0.7349081364829402885, -0.6046776061558809534, -0.2411417322834644161 ) ) ;
#23647=CARTESIAN_POINT ( 'NONE',  ( 1.161417322834646493, -0.4536011799217367080, 0.2665933059059888421 ) ) ;
#23648=CARTESIAN_POINT ( 'NONE',  ( 0.2165354330708668673, -0.5400638737290844871, 0.3530559997133364547 ) ) ;
#23653=B_SPLINE_CURVE_WITH_KNOTS ( 'NONE', 3,
 ( #68455, #37285, #36454, #55387 ),
 .UNSPECIFIED., .F., .F.,
 ( 4, 4 ),
 ( 1.999999999910059834E-07, 0.006970199999999935996 ),
 .UNSPECIFIED. ) ;
#23654=CARTESIAN_POINT ( 'NONE',  ( -1.102362204724408601, -0.1870078740157480879, -0.4822834645669291653 ) ) ;
#23655=CARTESIAN_POINT ( 'NONE',  ( -0.5643044619422565855, 0.05413385826771626580, -0.4176697321401330321 ) ) ;
#23659=CARTESIAN_POINT ( 'NONE',  ( 0.3543307086614181922, -0.5511811023622047445, 6.969142054262312111E-17 ) ) ;
#23661=CARTESIAN_POINT ( 'NONE',  ( 0.5905511811023629321, -0.6692913385826771977, 8.415575281601705876E-17 ) ) ;
#23664=CARTESIAN_POINT ( 'NONE',  ( -0.3018372703412066094, 0.05413385826771666132, 0.4176697321401328100 ) ) ;
#23665=CARTESIAN_POINT ( 'NONE',  ( 1.286089238845145033, 0.1283753931104748280, 0.1820866141732283561 ) ) ;
#23666=CARTESIAN_POINT ( 'NONE',  ( 0.4068241469816281097, 0.05413385826771666132, 0.4176697321401328100 ) ) ;
#23668=CARTESIAN_POINT ( 'NONE',  ( -0.4330708661417315697, -0.6692913385826771977, 8.415575281601705876E-17 ) ) ;
#23669=CARTESIAN_POINT ( 'NONE',  ( -1.010498687664041384, -0.3690944881889765550, -0.3153832671262227771 ) ) ;
#23670=CARTESIAN_POINT ( 'NONE',  ( 0.4002624671916016896, -0.3162353388693409650, -0.4822834645669289433 ) ) ;
#23671=EDGE_CURVE ( 'NONE', #13764, #66254, #64489, .T. ) ;
#23672=CARTESIAN_POINT ( 'NONE',  ( -0.06561679790026180015, -0.4281496062992127816, -0.4176697321401328100 ) ) ;
#23673=CARTESIAN_POINT ( 'NONE',  ( -1.192200019340701855, -5.582469467804009507E-15, -0.3954985857520081360 ) ) ;
#23674=CARTESIAN_POINT ( 'NONE',  ( 0.4606732211678724598, 1.763126522798933227, -0.5309055118110237448 ) ) ;
#23676=CARTESIAN_POINT ( 'NONE',  ( 0.6627296587926517768, -0.6692913385826773087, -0.1292274648535924053 ) ) ;
#23677=CARTESIAN_POINT ( 'NONE',  ( -0.4330708661417315697, 0.2952755905511811885, 0.000000000000000000 ) ) ;
#23678=CARTESIAN_POINT ( 'NONE',  ( -1.325459317585300889, 0.05413385826771666132, 0.4176697321401328100 ) ) ;
#23679=CARTESIAN_POINT ( 'NONE',  ( 0.9055118110236227702, -0.6692913385826771977, 8.415575281601705876E-17 ) ) ;
#23680=CARTESIAN_POINT ( 'NONE',  ( 0.3740157480314966754, -0.5400638737290844871, 0.3530559997133364547 ) ) ;
#23682=CARTESIAN_POINT ( 'NONE',  ( -0.3018372703412066094, 0.05413385826771666132, 0.4176697321401328100 ) ) ;
#23683=CARTESIAN_POINT ( 'NONE',  ( 0.3215223097112867578, -0.3162353388693409650, -0.4822834645669289433 ) ) ;
#23684=CARTESIAN_POINT ( 'NONE',  ( -0.4265091863517051496, -0.6692913385826771977, 0.1292274648535927661 ) ) ;
#23685=CARTESIAN_POINT ( 'NONE',  ( 0.2296587926509192634, -0.2845877964562159024, 0.3641732283464567677 ) ) ;
#23686=CARTESIAN_POINT ( 'NONE',  ( 1.594488188976378673, -0.4536011799217368745, -0.2665933059059886201 ) ) ;
#23688=CARTESIAN_POINT ( 'NONE',  ( 0.2493438320209980519, -0.4281496062992127816, -0.4176697321401328100 ) ) ;
#23690=CARTESIAN_POINT ( 'NONE',  ( 1.430446194225722500, 0.05413385826771666132, 0.4176697321401328100 ) ) ;
#23693=EDGE_LOOP ( 'NONE', ( #33096, #80822, #80661, #61045 ) ) ;
#23695=CARTESIAN_POINT ( 'NONE',  ( 0.5183727034120741983, -0.6692913385826771977, 0.1292274648535927661 ) ) ;
#23696=CARTESIAN_POINT ( 'NONE',  ( 0.2362204724409456558, -0.1870078740157480601, -0.3641732283464567677 ) ) ;
#23698=AXIS2_PLACEMENT_3D ( 'NONE', #29617, #80988, #54034 ) ;
#23700=CARTESIAN_POINT ( 'NONE',  ( -1.595398199321655941, 1.585328674332965315, 0.1559797534342484693 ) ) ;
#23705=CARTESIAN_POINT ( 'NONE',  ( 0.4986876640419954376, 0.2306618581243848609, 0.2411417322834645549 ) ) ;
#23706=CARTESIAN_POINT ( 'NONE',  ( -0.9186351706036736120, -0.6046776061558809534, -0.2411417322834644161 ) ) ;
#23707=CARTESIAN_POINT ( 'NONE',  ( -0.9055118110236215490, 0.2952755905511811885, 0.000000000000000000 ) ) ;
#23708=CARTESIAN_POINT ( 'NONE',  ( 0.8858267716535438430, -0.5400638737290845981, -0.3530559997133363437 ) ) ;
#23709=CARTESIAN_POINT ( 'NONE',  ( 1.371391076115485719, -0.6692913385826773087, -0.1292274648535924053 ) ) ;
#23710=CARTESIAN_POINT ( 'NONE',  ( 1.194225721784777594, -0.004921259842519576551, 0.3153832671262227771 ) ) ;
#23712=CARTESIAN_POINT ( 'NONE',  ( 1.279527559055118724, -0.4536011799217368745, -0.2665933059059886201 ) ) ;
#23713=CARTESIAN_POINT ( 'NONE',  ( -0.7086614173228339419, -0.1870078740157479769, 0.4822834645669291653 ) ) ;
#23715=CARTESIAN_POINT ( 'NONE',  ( 1.515748031496063408, 0.1660481256975885056, 0.3530559997133364547 ) ) ;
#23717=CARTESIAN_POINT ( 'NONE',  ( -0.4068241469816264999, -0.4281496062992124485, 0.4176697321401328655 ) ) ;
#23719=CARTESIAN_POINT ( 'NONE',  ( 1.062992125984252745, 0.2952755905511811885, 0.000000000000000000 ) ) ;
#23720=FACE_OUTER_BOUND ( 'NONE', #58989, .T. ) ;
#23721=CARTESIAN_POINT ( 'NONE',  ( -1.194225721784776262, -0.004921259842519870586, -0.3153832671262229437 ) ) ;
#23722=CARTESIAN_POINT ( 'NONE',  ( 0.4921259842519691285, -0.5400638737290845981, -0.3530559997133363437 ) ) ;
#23723=CARTESIAN_POINT ( 'NONE',  ( 1.043307086614173818, -0.4536011799217368745, -0.2665933059059886201 ) ) ;
#23725=CARTESIAN_POINT ( 'NONE',  ( -1.194225721784776262, -0.004921259842519870586, -0.3153832671262229437 ) ) ;
#23726=CARTESIAN_POINT ( 'NONE',  ( 1.240157480314961314, 0.1660481256975883668, -0.3530559997133364547 ) ) ;
#23728=CARTESIAN_POINT ( 'NONE',  ( -0.2034120734908131112, -0.5511811023622048555, -0.09757992244046775898 ) ) ;
#23729=CARTESIAN_POINT ( 'NONE',  ( -0.1706036745406816491, -0.4281496062992124485, 0.4176697321401328655 ) ) ;
#23730=CARTESIAN_POINT ( 'NONE',  ( -1.299212598425196097, 0.1771653543307087630, 0.000000000000000000 ) ) ;
#23731=CARTESIAN_POINT ( 'NONE',  ( -0.6364829396325453192, -0.3162353388693405765, 0.4822834645669290543 ) ) ;
#23732=CARTESIAN_POINT ( 'NONE',  ( 1.286089238845145033, -0.6046776061558809534, -0.2411417322834644161 ) ) ;
#23734=CARTESIAN_POINT ( 'NONE',  ( -1.062992125984250968, -0.5511811023622047445, 6.969142054262312111E-17 ) ) ;
#23736=CARTESIAN_POINT ( 'NONE',  ( 1.476377952755906220, 0.1660481256975883668, -0.3530559997133364547 ) ) ;
#23738=CARTESIAN_POINT ( 'NONE',  ( -1.141732283464566011, -0.6692913385826771977, 8.415575281601705876E-17 ) ) ;
#23739=CARTESIAN_POINT ( 'NONE',  ( -1.036745406824146176, -0.3690944881889763329, 0.3153832671262228327 ) ) ;
#23740=CARTESIAN_POINT ( 'NONE',  ( -0.6758530183727028406, -0.5511811023622048555, -0.09757992244046775898 ) ) ;
#23741=DIRECTION ( 'NONE',  ( 0.000000000000000000, 0.000000000000000000, 1.000000000000000000 ) ) ;
#23742=CARTESIAN_POINT ( 'NONE',  ( 0.1443569553805781891, 0.05413385826771626580, -0.4176697321401330321 ) ) ;
#23743=CARTESIAN_POINT ( 'NONE',  ( -0.2034120734908128059, 0.1771653543307087630, 0.09757992244046791164 ) ) ;
#23744=CARTESIAN_POINT ( 'NONE',  ( -1.338582677165353729, -0.1870078740157480601, -0.3641732283464567677 ) ) ;
#23745=CARTESIAN_POINT ( 'NONE',  ( -1.404199475065615932, 0.05413385826771666132, 0.4176697321401328100 ) ) ;
#23746=CARTESIAN_POINT ( 'NONE',  ( 1.167979002624672580, -0.004921259842519870586, -0.3153832671262229437 ) ) ;
#23747=CARTESIAN_POINT ( 'NONE',  ( 0.7545931758530189937, 0.2952755905511810774, -0.1292274648535930714 ) ) ;
#23749=CARTESIAN_POINT ( 'NONE',  ( 0.3149606299212606708, -0.1870078740157480601, -0.3641732283464567677 ) ) ;
#23750=CARTESIAN_POINT ( 'NONE',  ( 0.7545931758530189937, 0.2952755905511810774, -0.1292274648535930714 ) ) ;
#23751=CARTESIAN_POINT ( 'NONE',  ( 0.8333333333333340365, 0.1771653543307087075, -0.09757992244046823083 ) ) ;
#23753=CARTESIAN_POINT ( 'NONE',  ( -1.266404199475064773, -0.05778040916215560624, -0.4822834645669293319 ) ) ;
#23754=CARTESIAN_POINT ( 'NONE',  ( -0.8923884514435688198, -0.6046776061558807314, 0.2411417322834647770 ) ) ;
#23755=CARTESIAN_POINT ( 'NONE',  ( -0.2493438320209966919, 0.05413385826771626580, -0.4176697321401330321 ) ) ;
#23756=AXIS2_PLACEMENT_3D ( 'NONE', #40924, #78411, #47223 ) ;
#23759=CARTESIAN_POINT ( 'NONE',  ( 0.3937007874015754361, -0.1870078740157480879, -0.4822834645669291653 ) ) ;
#23760=CARTESIAN_POINT ( 'NONE',  ( 1.364829396325459854, -0.5023911411419708095, -0.1820866141732282451 ) ) ;
#23763=CARTESIAN_POINT ( 'NONE',  ( 0.04593175853018440641, -0.6692913385826771977, 0.1292274648535927661 ) ) ;
#23764=CARTESIAN_POINT ( 'NONE',  ( 0.6692913385826777528, 0.2952755905511811885, 0.000000000000000000 ) ) ;
#23770=CARTESIAN_POINT ( 'NONE',  ( -0.6102362204724400829, 0.07958543189024085140, 0.2665933059059887866 ) ) ;
#23771=CARTESIAN_POINT ( 'NONE',  ( -0.8202099737532801971, -0.6692913385826771977, 0.1292274648535927661 ) ) ;
#23772=CARTESIAN_POINT ( 'NONE',  ( 0.6496062992125991586, 0.1660481256975885056, 0.3530559997133364547 ) ) ;
#23774=CARTESIAN_POINT ( 'NONE',  ( 0.8530183727034128527, -0.4281496062992124485, 0.4176697321401328655 ) ) ;
#23775=CARTESIAN_POINT ( 'NONE',  ( -1.384514435695537005, -0.6692913385826773087, -0.1292274648535924053 ) ) ;
#23776=CARTESIAN_POINT ( 'NONE',  ( 1.391076115485564868, -0.6046776061558807314, 0.2411417322834647770 ) ) ;
#23779=CARTESIAN_POINT ( 'NONE',  ( 0.4847769261806178509, 1.968503937007873850, 0.4915354330708653907 ) ) ;
#23780=CARTESIAN_POINT ( 'NONE',  ( 0.9251968503937015864, -0.5400638737290844871, 0.3530559997133364547 ) ) ;
#23781=CARTESIAN_POINT ( 'NONE',  ( 0.4986876640419954376, 0.2306618581243848609, 0.2411417322834645549 ) ) ;
#23782=CARTESIAN_POINT ( 'NONE',  ( 1.062992125984252745, -0.5511811023622047445, 6.969142054262312111E-17 ) ) ;
#23783=CARTESIAN_POINT ( 'NONE',  ( -1.548556430446193399, -0.5023911411419708095, -0.1820866141732282451 ) ) ;
#23784=CARTESIAN_POINT ( 'NONE',  ( 1.594488188976378673, 0.1660481256975885056, 0.3530559997133364547 ) ) ;
#23786=CARTESIAN_POINT ( 'NONE',  ( 0.9317585301837276734, 0.05413385826771626580, -0.4176697321401330321 ) ) ;
#23787=CARTESIAN_POINT ( 'NONE',  ( 1.627296587926509996, -0.5023911411419708095, 0.1820866141732285504 ) ) ;
#23788=CARTESIAN_POINT ( 'NONE',  ( -0.6758530183727028406, -0.6692913385826773087, -0.1292274648535924053 ) ) ;
#23789=CARTESIAN_POINT ( 'NONE',  ( -0.5446194225721777693, -0.3162353388693409650, -0.4822834645669289433 ) ) ;
#23790=CARTESIAN_POINT ( 'NONE',  ( 1.456692913385827515, 0.2952755905511811885, 0.000000000000000000 ) ) ;
#23792=CARTESIAN_POINT ( 'NONE',  ( 0.3149606299212603933, -0.1870078740157479769, 0.4822834645669291653 ) ) ;
#23794=CARTESIAN_POINT ( 'NONE',  ( -1.509186351706035767, -0.3690944881889763329, 0.3153832671262228327 ) ) ;
#23798=CARTESIAN_POINT ( 'NONE',  ( -0.03280839895013062252, 0.2066929133858267098, -0.1054918080437494132 ) ) ;
#23799=CARTESIAN_POINT ( 'NONE',  ( 1.220472440944882386, -0.5511811023622047445, 6.969142054262312111E-17 ) ) ;
#23801=CARTESIAN_POINT ( 'NONE',  ( 1.535433070866142558, 0.1771653543307087630, 0.000000000000000000 ) ) ;
#23806=CARTESIAN_POINT ( 'NONE',  ( -0.7086614173228339419, -0.1870078740157479769, 0.3641732283464567677 ) ) ;
#23807=CARTESIAN_POINT ( 'NONE',  ( -1.404199475065615932, -0.004921259842519576551, 0.3153832671262227771 ) ) ;
#23808=CARTESIAN_POINT ( 'NONE',  ( 1.437007874015748810, 0.1660481256975885056, 0.3530559997133364547 ) ) ;
#23809=CARTESIAN_POINT ( 'NONE',  ( 0.5052493438320215802, 0.2952755905511811885, 0.1292274648535926551 ) ) ;
#23810=CARTESIAN_POINT ( 'NONE',  ( -1.181102362204723644, -0.1870078740157479769, 0.4822834645669291653 ) ) ;
#23813=ADVANCED_FACE ( 'NONE', ( #5993 ), #72045, .F. ) ;
#23814=CARTESIAN_POINT ( 'NONE',  ( -1.653543307086613234, -0.1870078740157479769, 0.4822834645669291653 ) ) ;
#23823=CARTESIAN_POINT ( 'NONE',  ( -0.7283464566929126471, -0.5400638737290844871, 0.3530559997133364547 ) ) ;
#23824=CARTESIAN_POINT ( 'NONE',  ( 0.8661417322834653598, -0.1870078740157479769, 0.4822834645669291653 ) ) ;
#23828=CARTESIAN_POINT ( 'NONE',  ( 1.496062992125985147, -0.1870078740157479769, 0.4822834645669291653 ) ) ;
#23829=CARTESIAN_POINT ( 'NONE',  ( -0.9317585301837263412, 0.05413385826771666132, 0.4176697321401328100 ) ) ;
#23831=CARTESIAN_POINT ( 'NONE',  ( -0.01312335958005186876, -0.3690944881889763329, 0.3153832671262228327 ) ) ;
#23833=CARTESIAN_POINT ( 'NONE',  ( -0.02624671916010428221, 0.1283753931104746893, -0.1820866141732285504 ) ) ;
#23834=CARTESIAN_POINT ( 'NONE',  ( 0.6561679790026253567, 0.1283753931104748280, 0.1820866141732283561 ) ) ;
#23835=CARTESIAN_POINT ( 'NONE',  ( 0.4265091863517067039, -0.6692913385826773087, -0.1292274648535924053 ) ) ;
#23836=CARTESIAN_POINT ( 'NONE',  ( -0.5118110236220466680, 0.1771653543307087630, 0.000000000000000000 ) ) ;
#23838=CARTESIAN_POINT ( 'NONE',  ( -1.522309711286088607, -0.6046776061558807314, 0.2411417322834647770 ) ) ;
#23840=CARTESIAN_POINT ( 'NONE',  ( -0.9580052493438311334, 0.05413385826771626580, -0.4176697321401330321 ) ) ;
#23842=CARTESIAN_POINT ( 'NONE',  ( -0.02624671916010428221, -0.6046776061558807314, 0.2411417322834647770 ) ) ;
#23843=CARTESIAN_POINT ( 'NONE',  ( -0.5708661417322825615, -0.5400638737290844871, 0.3530559997133364547 ) ) ;
#23844=CARTESIAN_POINT ( 'NONE',  ( 1.200787401574803681, 0.07958543189024085140, 0.2665933059059887866 ) ) ;
#23845=CARTESIAN_POINT ( 'NONE',  ( 0.09186351706036799403, -0.3690944881889765550, -0.3153832671262227771 ) ) ;
#23846=CARTESIAN_POINT ( 'NONE',  ( -0.1837270341207343505, -0.6046776061558807314, 0.2411417322834647770 ) ) ;
#23847=CARTESIAN_POINT ( 'NONE',  ( -1.122047244094487306, 0.1660481256975883668, -0.3530559997133364547 ) ) ;
#23850=CARTESIAN_POINT ( 'NONE',  ( 0.04593175853018440641, -0.6692913385826771977, 0.1292274648535927661 ) ) ;
#23853=CARTESIAN_POINT ( 'NONE',  ( 1.122047244094488860, 0.1660481256975885056, 0.3530559997133364547 ) ) ;
#23854=CARTESIAN_POINT ( 'NONE',  ( -0.7677165354330699465, 0.07958543189024085140, 0.2665933059059887866 ) ) ;
#23855=CARTESIAN_POINT ( 'NONE',  ( -0.4461942257217840213, 0.2306618581243848609, 0.2411417322834645549 ) ) ;
#23856=CARTESIAN_POINT ( 'NONE',  ( 1.148293963254593875, -0.6692913385826771977, 0.1292274648535927661 ) ) ;
#23857=CARTESIAN_POINT ( 'NONE',  ( 1.062992125984252745, 0.2952755905511811885, 0.000000000000000000 ) ) ;
#23858=CARTESIAN_POINT ( 'NONE',  ( -1.627296587926508442, 0.2306618581243848609, 0.2411417322834645549 ) ) ;
#23859=CARTESIAN_POINT ( 'NONE',  ( -0.8989501312335946848, 0.1771653543307087075, -0.09757992244046823083 ) ) ;
#23863=CARTESIAN_POINT ( 'NONE',  ( 1.509186351706037543, -0.004921259842519576551, 0.3153832671262227771 ) ) ;
#23864=CARTESIAN_POINT ( 'NONE',  ( 0.5511811023622054106, -0.1870078740157480601, -0.3641732283464567677 ) ) ;
#23865=CARTESIAN_POINT ( 'NONE',  ( 0.5971128608923890191, -0.6692913385826771977, 0.1292274648535927661 ) ) ;
#23868=CARTESIAN_POINT ( 'NONE',  ( 0.6364829396325465405, -0.2845877964562161244, -0.3641732283464567121 ) ) ;
#23869=CARTESIAN_POINT ( 'NONE',  ( -0.4790026246719152336, -0.05778040916215560624, -0.4822834645669293319 ) ) ;
#23870=CARTESIAN_POINT ( 'NONE',  ( -0.6364829396325453192, -0.05778040916215560624, -0.4822834645669293319 ) ) ;
#23871=CARTESIAN_POINT ( 'NONE',  ( 1.135170603674541256, -0.6692913385826773087, -0.1292274648535924053 ) ) ;
#23875=CARTESIAN_POINT ( 'NONE',  ( -0.1115485564304456306, 0.1771653543307087075, -0.09757992244046823083 ) ) ;
#23876=EDGE_CURVE ( 'NONE', #39166, #34321, #32265, .T. ) ;
#23880=CARTESIAN_POINT ( 'NONE',  ( -0.7742782152230965886, 0.05413385826771666132, 0.4176697321401328100 ) ) ;
#23881=CARTESIAN_POINT ( 'NONE',  ( -0.006561679790025524116, -0.05778040916215560624, -0.4822834645669293319 ) ) ;
#23882=CARTESIAN_POINT ( 'NONE',  ( -0.2559055118110227234, -0.5400638737290844871, 0.3530559997133364547 ) ) ;
#23883=CARTESIAN_POINT ( 'NONE',  ( 0.3740157480314966754, -0.5400638737290844871, 0.3530559997133364547 ) ) ;
#23884=CARTESIAN_POINT ( 'NONE',  ( -0.5905511811023613777, -0.6692913385826771977, 8.415575281601705876E-17 ) ) ;
#23885=CARTESIAN_POINT ( 'NONE',  ( -1.351706036745406347, -0.4281496062992124485, 0.4176697321401328655 ) ) ;
#23886=CARTESIAN_POINT ( 'NONE',  ( -0.9448818897637790704, -0.1870078740157479769, 0.4822834645669291653 ) ) ;
#23887=CARTESIAN_POINT ( 'NONE',  ( 0.7611548556430451917, -0.6046776061558807314, 0.2411417322834647770 ) ) ;
#23888=CARTESIAN_POINT ( 'NONE',  ( 0.4068241469816279987, -0.4281496062992127816, -0.4176697321401328100 ) ) ;
#23891=CARTESIAN_POINT ( 'NONE',  ( -0.3937007874015740483, -0.1870078740157479769, 0.3641732283464567677 ) ) ;
#23892=EDGE_LOOP ( 'NONE', ( #25933, #59152, #61867, #823, #13526 ) ) ;
#23895=CARTESIAN_POINT ( 'NONE',  ( -1.233595800524933894, 0.1283753931104748280, 0.1820866141732283561 ) ) ;
#23896=CARTESIAN_POINT ( 'NONE',  ( -1.062992125984250968, -0.6692913385826771977, 8.415575281601705876E-17 ) ) ;
#23897=CARTESIAN_POINT ( 'NONE',  ( -0.6233595800524928121, -0.3162353388693409650, -0.4822834645669289433 ) ) ;
#23898=CARTESIAN_POINT ( 'NONE',  ( 0.7770624478417551551, 1.702998256715020864E-15, -0.4281989832122454209 ) ) ;
#23899=CARTESIAN_POINT ( 'NONE',  ( -0.5249343832020990641, -0.6046776061558809534, -0.2411417322834644161 ) ) ;
#23900=CARTESIAN_POINT ( 'NONE',  ( -0.9711286089238838626, -0.6046776061558807314, 0.2411417322834647770 ) ) ;
#23903=CARTESIAN_POINT ( 'NONE',  ( 0.8005249343832028242, -0.3690944881889765550, -0.3153832671262227771 ) ) ;
#23906=CARTESIAN_POINT ( 'NONE',  ( 0.05249343832021075018, 0.1283753931104746893, -0.1820866141732285504 ) ) ;
#23907=CARTESIAN_POINT ( 'NONE',  ( -0.5577427821522301654, -0.3162353388693405765, 0.4822834645669290543 ) ) ;
#23908=CARTESIAN_POINT ( 'NONE',  ( -1.614173228346456712, 2.401574803149606474, -0.1372047244094478091 ) ) ;
#23909=CARTESIAN_POINT ( 'NONE',  ( 0.08530183727034192087, -0.05778040916215522460, 0.4822834645669289988 ) ) ;
#23916=CARTESIAN_POINT ( 'NONE',  ( -0.7545931758530177724, 0.1771653543307087630, 0.09757992244046791164 ) ) ;
#23917=CARTESIAN_POINT ( 'NONE',  ( -0.9317585301837263412, 0.05413385826771666132, 0.4176697321401328100 ) ) ;
#23921=CARTESIAN_POINT ( 'NONE',  ( 1.318897637795276356, -0.5400638737290844871, 0.3530559997133364547 ) ) ;
#23922=CARTESIAN_POINT ( 'NONE',  ( 0.2821522309711292364, -0.6692913385826771977, 0.1292274648535927661 ) ) ;
#23923=CARTESIAN_POINT ( 'NONE',  ( 0.4461942257217856311, 0.2306618581243847221, -0.2411417322834647770 ) ) ;
#23924=CARTESIAN_POINT ( 'NONE',  ( -0.6955380577427815458, -0.004921259842519576551, 0.3153832671262227771 ) ) ;
#23925=CARTESIAN_POINT ( 'NONE',  ( -0.5183727034120726440, -0.6692913385826773087, -0.1292274648535924053 ) ) ;
#23927=CARTESIAN_POINT ( 'NONE',  ( -0.7545931758530177724, 0.2952755905511811885, 0.1292274648535926551 ) ) ;
#23929=CARTESIAN_POINT ( 'NONE',  ( 1.220472440944882386, -0.5511811023622047445, 6.969142054262312111E-17 ) ) ;
#23930=CARTESIAN_POINT ( 'NONE',  ( -0.2230971128608915943, -0.3690944881889765550, -0.3153832671262227771 ) ) ;
#23931=CARTESIAN_POINT ( 'NONE',  ( 1.036745406824147731, -0.004921259842519576551, 0.3153832671262227771 ) ) ;
#23932=CARTESIAN_POINT ( 'NONE',  ( 1.587926509186352142, -0.004921259842519576551, 0.3153832671262227771 ) ) ;
#23933=CARTESIAN_POINT ( 'NONE',  ( -1.259842519685038686, -0.1870078740157480601, -0.3641732283464567677 ) ) ;
#23934=CARTESIAN_POINT ( 'NONE',  ( 0.6496062992125991586, -0.4536011799217368745, -0.2665933059059886201 ) ) ;
#23935=CARTESIAN_POINT ( 'NONE',  ( -0.3280839895013117347, 0.05413385826771626580, -0.4176697321401330321 ) ) ;
#23937=CARTESIAN_POINT ( 'NONE',  ( -0.2165354330708654795, 0.07958543189024085140, 0.2665933059059887866 ) ) ;
#23939=CARTESIAN_POINT ( 'NONE',  ( 0.6167979002624679463, 0.05413385826771626580, -0.4176697321401330321 ) ) ;
#23940=CARTESIAN_POINT ( 'NONE',  ( 0.6399301791983058596, -1.374501131054255944E-15, 0.4445507791589066726 ) ) ;
#23941=CARTESIAN_POINT ( 'NONE',  ( 1.469816272965879911, 0.1283753931104746893, -0.1820866141732285504 ) ) ;
#23942=CARTESIAN_POINT ( 'NONE',  ( -0.8792650918635160906, 0.05413385826771626580, -0.4176697321401330321 ) ) ;
#23943=CARTESIAN_POINT ( 'NONE',  ( -0.3280839895013117347, -0.004921259842519870586, -0.3153832671262229437 ) ) ;
#23944=FACE_OUTER_BOUND ( 'NONE', #56873, .T. ) ;
#23945=CARTESIAN_POINT ( 'NONE',  ( 0.3740157480314966754, 0.07958543189024071263, -0.2665933059059888421 ) ) ;
#23946=CARTESIAN_POINT ( 'NONE',  ( -0.4527559055118102749, -0.5400638737290845981, -0.3530559997133363437 ) ) ;
#23949=CARTESIAN_POINT ( 'NONE',  ( 0.6233595800524939223, -0.2845877964562159024, 0.3641732283464567677 ) ) ;
#23950=CARTESIAN_POINT ( 'NONE',  ( -0.3149606299212590610, -0.1870078740157480879, -0.4822834645669291653 ) ) ;
#23951=CARTESIAN_POINT ( 'NONE',  ( -0.8792650918635160906, -0.4281496062992124485, 0.4176697321401328655 ) ) ;
#23952=CARTESIAN_POINT ( 'NONE',  ( -0.6102362204724400829, -0.4536011799217368745, -0.2665933059059886201 ) ) ;
#23954=CARTESIAN_POINT ( 'NONE',  ( -0.01968503937007793844, 0.1660481256975883668, -0.3530559997133364547 ) ) ;
#23956=CARTESIAN_POINT ( 'NONE',  ( -1.279527559055116948, -0.4536011799217367080, 0.2665933059059888421 ) ) ;
#23957=CARTESIAN_POINT ( 'NONE',  ( -1.443569553805773564, 0.2306618581243847221, -0.2411417322834647770 ) ) ;
#23962=CARTESIAN_POINT ( 'NONE',  ( -1.404199475065615932, -0.004921259842519576551, 0.3153832671262227771 ) ) ;
#23963=CARTESIAN_POINT ( 'NONE',  ( -1.371391076115484831, 0.2952755905511810774, -0.1292274648535930714 ) ) ;
#23964=CARTESIAN_POINT ( 'NONE',  ( -1.030183727034119867, -0.05778040916215560624, -0.4822834645669293319 ) ) ;
#23965=CARTESIAN_POINT ( 'NONE',  ( -1.056430446194224881, -0.6692913385826771977, 0.1292274648535927661 ) ) ;
#23968=CARTESIAN_POINT ( 'NONE',  ( 1.030183727034121421, -0.05778040916215522460, 0.4822834645669289988 ) ) ;
#23969=CARTESIAN_POINT ( 'NONE',  ( 0.3215223097112867578, -0.3162353388693409650, -0.4822834645669289433 ) ) ;
#23970=CARTESIAN_POINT ( 'NONE',  ( 1.220472440944879722, 1.496062992125984037, 0.5309055118110233007 ) ) ;
#23972=CARTESIAN_POINT ( 'NONE',  ( 1.148293963254593653, 0.1771653543307087075, -0.09757992244046823083 ) ) ;
#23974=ORIENTED_EDGE ( 'NONE', *, *, #54140, .T. ) ;
#23975=CARTESIAN_POINT ( 'NONE',  ( -0.8464566929133852113, 0.07958543189024085140, 0.2665933059059887866 ) ) ;
#23977=ORIENTED_EDGE ( 'NONE', *, *, #3360, .F. ) ;
#23978=CARTESIAN_POINT ( 'NONE',  ( 0.2099737532808405305, 0.2306618581243847221, -0.2411417322834647770 ) ) ;
#23979=CARTESIAN_POINT ( 'NONE',  ( -0.5118110236220466680, -0.6692913385826771977, 8.415575281601705876E-17 ) ) ;
#23981=CARTESIAN_POINT ( 'NONE',  ( -1.207349081364828436, -0.6046776061558807314, 0.2411417322834647770 ) ) ;
#23982=CARTESIAN_POINT ( 'NONE',  ( 1.233595800524935227, 0.2306618581243847221, -0.2411417322834647770 ) ) ;
#23983=CARTESIAN_POINT ( 'NONE',  ( 1.620734908136483465, -0.6692913385826771977, 0.1292274648535927661 ) ) ;
#23984=CARTESIAN_POINT ( 'NONE',  ( 0.09115970038225353067, 3.421639014772782816E-16, 0.3464511005275203726 ) ) ;
#23985=CARTESIAN_POINT ( 'NONE',  ( -0.06561679790026180015, 0.05413385826771666132, 0.4176697321401328100 ) ) ;
#23986=CARTESIAN_POINT ( 'NONE',  ( -1.062992125984250968, -0.6692913385826771977, 8.415575281601705876E-17 ) ) ;
#23988=CARTESIAN_POINT ( 'NONE',  ( -1.646981627296586703, -0.05778040916215522460, 0.4822834645669289988 ) ) ;
#23989=CARTESIAN_POINT ( 'NONE',  ( 1.489501312335958172, -0.3162353388693405765, 0.4822834645669290543 ) ) ;
#23991=CARTESIAN_POINT ( 'NONE',  ( 0.7414698162729663755, 0.1771653543307087630, 0.09757992244046791164 ) ) ;
#23992=ORIENTED_EDGE ( 'NONE', *, *, #73735, .F. ) ;
#23994=CARTESIAN_POINT ( 'NONE',  ( -1.049868766404198794, -0.6046776061558807314, 0.2411417322834647770 ) ) ;
#23996=CARTESIAN_POINT ( 'NONE',  ( -0.09842519685039295696, 0.07958543189024071263, -0.2665933059059888421 ) ) ;
#23998=CARTESIAN_POINT ( 'NONE',  ( 0.4199475065616803948, -0.6046776061558809534, -0.2411417322834644161 ) ) ;
#23999=CARTESIAN_POINT ( 'NONE',  ( 0.4133858267716541968, -0.5400638737290845981, -0.3530559997133363437 ) ) ;
#24000=CARTESIAN_POINT ( 'NONE',  ( -0.5052493438320203589, -0.6692913385826771977, 0.1292274648535927661 ) ) ;
#24002=CARTESIAN_POINT ( 'NONE',  ( -0.8530183727034112984, 0.05413385826771666132, 0.4176697321401328100 ) ) ;
#24004=CARTESIAN_POINT ( 'NONE',  ( 1.233595800524935227, -0.5023911411419708095, 0.1820866141732285504 ) ) ;
#24005=CARTESIAN_POINT ( 'NONE',  ( -1.181102362204723644, -0.1870078740157479769, 0.4822834645669291653 ) ) ;
#24006=CARTESIAN_POINT ( 'NONE',  ( 0.9711286089238851948, -0.6046776061558809534, -0.2411417322834644161 ) ) ;
#24007=CARTESIAN_POINT ( 'NONE',  ( 1.148293963254593875, -0.6692913385826771977, 0.1292274648535927661 ) ) ;
#24009=CARTESIAN_POINT ( 'NONE',  ( -1.528871391076114250, 0.2952755905511810774, -0.1292274648535930714 ) ) ;
#24011=CARTESIAN_POINT ( 'NONE',  ( 0.4593175853018379162, -0.4281496062992124485, 0.4176697321401328655 ) ) ;
#24013=CARTESIAN_POINT ( 'NONE',  ( -1.581364829396324945, -0.08942795157528024563, -0.3641732283464568787 ) ) ;
#24014=CARTESIAN_POINT ( 'NONE',  ( 0.6036745406824154392, 0.1283753931104746893, -0.1820866141732285504 ) ) ;
#24015=CARTESIAN_POINT ( 'NONE',  ( 0.9973753280839902091, 0.2306618581243847221, -0.2411417322834647770 ) ) ;
#24017=CARTESIAN_POINT ( 'NONE',  ( 0.6824146981627303710, -0.5023911411419708095, 0.1820866141732285504 ) ) ;
#24018=CARTESIAN_POINT ( 'NONE',  ( 0.5118110236220478892, 0.2952755905511811885, 0.000000000000000000 ) ) ;
#24020=CARTESIAN_POINT ( 'NONE',  ( -0.8202099737532801971, -0.6692913385826771977, 0.1292274648535927661 ) ) ;
#24022=CARTESIAN_POINT ( 'NONE',  ( 1.017060367454068581, -0.08942795157528024563, -0.3641732283464568787 ) ) ;
#24023=CARTESIAN_POINT ( 'NONE',  ( -0.07874015748031421014, -0.1870078740157480879, -0.4822834645669291653 ) ) ;
#24024=DIRECTION ( 'NONE',  ( -0.000000000000000000, -1.000000000000000000, -0.000000000000000000 ) ) ;
#24025=CARTESIAN_POINT ( 'NONE',  ( -0.5052493438320203589, -0.6692913385826771977, 0.1292274648535927661 ) ) ;
#24026=CARTESIAN_POINT ( 'NONE',  ( 0.09186351706036827158, -0.004921259842519576551, 0.3153832671262227771 ) ) ;
#24028=CARTESIAN_POINT ( 'NONE',  ( 0.03280839895013198948, -0.5511811023622048555, -0.09757992244046775898 ) ) ;
#24029=CARTESIAN_POINT ( 'NONE',  ( 0.7283464566929140904, -0.4536011799217368745, -0.2665933059059886201 ) ) ;
#24031=CARTESIAN_POINT ( 'NONE',  ( 0.2165354330708668673, -0.5400638737290844871, 0.3530559997133364547 ) ) ;
#24033=CARTESIAN_POINT ( 'NONE',  ( 1.010498687664042716, -0.3690944881889763329, 0.3153832671262228327 ) ) ;
#24034=DIRECTION ( 'NONE',  ( -3.096699300667737957E-16, 1.000000000000000000, -0.000000000000000000 ) ) ;
#24035=CARTESIAN_POINT ( 'NONE',  ( -0.5708661417322828946, 0.07958543189024071263, -0.2665933059059888421 ) ) ;
#24036=CARTESIAN_POINT ( 'NONE',  ( -0.2821522309711278487, 0.1771653543307087630, 0.09757992244046791164 ) ) ;
#24037=CARTESIAN_POINT ( 'NONE',  ( -0.4461942257217840213, -0.6046776061558809534, -0.2411417322834644161 ) ) ;
#24038=CARTESIAN_POINT ( 'NONE',  ( 0.7808398950131241190, -0.08942795157528024563, -0.3641732283464568787 ) ) ;
#24040=CARTESIAN_POINT ( 'NONE',  ( 1.417322834645670104, -0.1870078740157479769, 0.3641732283464567677 ) ) ;
#24041=CARTESIAN_POINT ( 'NONE',  ( 0.02624671916010564918, -0.6046776061558809534, -0.2411417322834644161 ) ) ;
#24042=CARTESIAN_POINT ( 'NONE',  ( 0.9973753280839902091, -0.6046776061558807314, 0.2411417322834647770 ) ) ;
#24044=CARTESIAN_POINT ( 'NONE',  ( 0.2493438320209980519, -0.4281496062992127816, -0.4176697321401328100 ) ) ;
#24046=CARTESIAN_POINT ( 'NONE',  ( 1.036745406824147731, 0.05413385826771666132, 0.4176697321401328100 ) ) ;
#24047=CARTESIAN_POINT ( 'NONE',  ( 0.7086614173228353852, -0.1870078740157479769, 0.4822834645669291653 ) ) ;
#24049=CARTESIAN_POINT ( 'NONE',  ( 0.7152230971128616943, -0.08942795157527998196, 0.3641732283464567121 ) ) ;
#24050=CARTESIAN_POINT ( 'NONE',  ( 1.345144356955381593, -0.05778040916215522460, 0.4822834645669289988 ) ) ;
#24051=EDGE_CURVE ( 'NONE', #52467, #29190, #2611, .T. ) ;
#24052=CARTESIAN_POINT ( 'NONE',  ( 0.2559055118110243332, -0.4536011799217368745, -0.2665933059059886201 ) ) ;
#24053=CARTESIAN_POINT ( 'NONE',  ( -0.1115485564304453947, -0.6692913385826771977, 0.1292274648535927661 ) ) ;
#24054=CARTESIAN_POINT ( 'NONE',  ( 0.4265091863517067039, -0.6692913385826773087, -0.1292274648535924053 ) ) ;
#24055=CARTESIAN_POINT ( 'NONE',  ( -0.6561679790026240244, 0.2306618581243847221, -0.2411417322834647770 ) ) ;
#24056=CARTESIAN_POINT ( 'NONE',  ( -0.4461942257217840213, 0.1283753931104748280, 0.1820866141732283561 ) ) ;
#24057=B_SPLINE_CURVE_WITH_KNOTS ( 'NONE', 3,
 ( #30213, #31868, #30633, #64273 ),
 .UNSPECIFIED., .F., .F.,
 ( 4, 4 ),
 ( 1.999999999910059834E-07, 0.006970199999999935996 ),
 .UNSPECIFIED. ) ;
#24058=CARTESIAN_POINT ( 'NONE',  ( 0.9776902887139113929, 0.2952755905511811885, 0.1292274648535926551 ) ) ;
#24059=CARTESIAN_POINT ( 'NONE',  ( 0.8858267716535438430, 0.07958543189024085140, 0.2665933059059887866 ) ) ;
#24060=CARTESIAN_POINT ( 'NONE',  ( -0.01312335958005186876, 0.05413385826771626580, -0.4176697321401330321 ) ) ;
#24066=CARTESIAN_POINT ( 'NONE',  ( -1.397637795275589623, -0.5400638737290845981, -0.3530559997133363437 ) ) ;
#24067=CARTESIAN_POINT ( 'NONE',  ( -1.003937007874015297, -0.5400638737290845981, -0.3530559997133363437 ) ) ;
#24071=CARTESIAN_POINT ( 'NONE',  ( 0.4593175853018380828, -0.004921259842519870586, -0.3153832671262229437 ) ) ;
#24073=CARTESIAN_POINT ( 'NONE',  ( 0.5118110236220478892, 0.2952755905511811885, 0.000000000000000000 ) ) ;
#24076=CARTESIAN_POINT ( 'NONE',  ( -1.633858267716534529, -0.4536011799217368745, -0.2665933059059886201 ) ) ;
#24077=CARTESIAN_POINT ( 'NONE',  ( 1.082677165354331228, 0.1660481256975883668, -0.3530559997133364547 ) ) ;
#24078=CARTESIAN_POINT ( 'NONE',  ( 1.299212598425197429, 0.1771653543307087630, 0.000000000000000000 ) ) ;
#24079=CARTESIAN_POINT ( 'NONE',  ( 0.09186351706036827158, 0.05413385826771666132, 0.4176697321401328100 ) ) ;
#24081=CARTESIAN_POINT ( 'NONE',  ( -0.5249343832020990641, 0.2306618581243848609, 0.2411417322834645549 ) ) ;
#24082=CARTESIAN_POINT ( 'NONE',  ( -0.9973753280839886548, -0.5023911411419708095, -0.1820866141732282451 ) ) ;
#24083=CARTESIAN_POINT ( 'NONE',  ( 0.5118110236220478892, 0.2952755905511811885, 0.000000000000000000 ) ) ;
#24084=CARTESIAN_POINT ( 'NONE',  ( -0.6889763779527552368, -0.5400638737290845981, -0.3530559997133363437 ) ) ;
#24085=CARTESIAN_POINT ( 'NONE',  ( 1.673228346456693494, 0.1660481256975885056, 0.3530559997133364547 ) ) ;
#24089=CARTESIAN_POINT ( 'NONE',  ( 0.5643044619422579178, 0.05413385826771666132, 0.4176697321401328100 ) ) ;
#24090=CARTESIAN_POINT ( 'NONE',  ( -0.1837270341207343505, -0.6046776061558807314, 0.2411417322834647770 ) ) ;
#24091=CARTESIAN_POINT ( 'NONE',  ( -1.312335958005248715, 0.2306618581243848609, 0.2411417322834645549 ) ) ;
#24093=CARTESIAN_POINT ( 'NONE',  ( 0.7217847769028878924, -0.4281496062992127816, -0.4176697321401328100 ) ) ;
#24094=CARTESIAN_POINT ( 'NONE',  ( 0.2952755905511819101, 0.1660481256975883668, -0.3530559997133364547 ) ) ;
#24096=CARTESIAN_POINT ( 'NONE',  ( -0.6627296587926503335, -0.6692913385826771977, 0.1292274648535927661 ) ) ;
#24097=CARTESIAN_POINT ( 'NONE',  ( 0.3018372703412079971, 0.05413385826771626580, -0.4176697321401330321 ) ) ;
#24098=CARTESIAN_POINT ( 'NONE',  ( -0.3083989501312330295, -0.3162353388693409650, -0.4822834645669289433 ) ) ;
#24099=CARTESIAN_POINT ( 'NONE',  ( 0.09842519685039434474, 0.07958543189024085140, 0.2665933059059887866 ) ) ;
#24100=CARTESIAN_POINT ( 'NONE',  ( -1.646981627296586703, -0.3162353388693409650, -0.4822834645669289433 ) ) ;
#24102=CARTESIAN_POINT ( 'NONE',  ( -0.2690288713910754526, 0.2952755905511810774, -0.1292274648535930714 ) ) ;
#24104=CARTESIAN_POINT ( 'NONE',  ( -1.646981627296586703, -0.05778040916215522460, 0.4822834645669289988 ) ) ;
#24108=CARTESIAN_POINT ( 'NONE',  ( 0.8792650918635177559, 0.05413385826771666132, 0.4176697321401328100 ) ) ;
#24109=CARTESIAN_POINT ( 'NONE',  ( 0.3149606299212603933, -0.1870078740157479769, 0.3641732283464567677 ) ) ;
#24110=CARTESIAN_POINT ( 'NONE',  ( 1.679790026246720025, 0.1283753931104748280, 0.1820866141732283561 ) ) ;
#24114=B_SPLINE_CURVE_WITH_KNOTS ( 'NONE', 3,
 ( #32386, #70695, #52569, #58049, #7985, #71116, #66060 ),
 .UNSPECIFIED., .F., .F.,
 ( 4, 3, 4 ),
 ( 3.469446951953614189E-18, 0.001246230184515548971, 0.002492489877932632051 ),
 .UNSPECIFIED. ) ;
#24116=CARTESIAN_POINT ( 'NONE',  ( 0.3412073490813655186, 0.2306618581243848609, 0.2411417322834645549 ) ) ;
#24117=CARTESIAN_POINT ( 'NONE',  ( -1.030183727034119867, -0.3162353388693405765, 0.4822834645669290543 ) ) ;
#24118=CARTESIAN_POINT ( 'NONE',  ( -1.154855643044618851, -0.6046776061558809534, -0.2411417322834644161 ) ) ;
#24119=CARTESIAN_POINT ( 'NONE',  ( 0.8530183727034126306, 0.05413385826771626580, -0.4176697321401330321 ) ) ;
#24120=CARTESIAN_POINT ( 'NONE',  ( 0.8858267716535438430, -0.5400638737290845981, -0.3530559997133363437 ) ) ;
#24121=CARTESIAN_POINT ( 'NONE',  ( 1.417322834645670104, -0.1870078740157480601, -0.3641732283464567677 ) ) ;
#24122=CARTESIAN_POINT ( 'NONE',  ( 1.056430446194226658, 0.1771653543307087630, 0.09757992244046791164 ) ) ;
#24123=CARTESIAN_POINT ( 'NONE',  ( -0.8727034120734901146, -0.3162353388693405765, 0.4822834645669290543 ) ) ;
#24125=CARTESIAN_POINT ( 'NONE',  ( 1.686351706036745890, 0.2952755905511811885, 0.1292274648535926551 ) ) ;
#24127=CARTESIAN_POINT ( 'NONE',  ( -0.1574803149606292529, -0.1870078740157480879, -0.4822834645669291653 ) ) ;
#24128=CARTESIAN_POINT ( 'NONE',  ( 1.266404199475066328, -0.3162353388693409650, -0.4822834645669289433 ) ) ;
#24131=CARTESIAN_POINT ( 'NONE',  ( 0.4330708661417329575, 0.2952755905511811885, 0.000000000000000000 ) ) ;
#24132=CARTESIAN_POINT ( 'NONE',  ( 1.069553805774278610, -0.5511811023622046335, 0.09757992244046803654 ) ) ;
#24134=CARTESIAN_POINT ( 'NONE',  ( -1.167979002624671470, -0.3690944881889765550, -0.3153832671262227771 ) ) ;
#24135=CARTESIAN_POINT ( 'NONE',  ( 1.069553805774278832, 0.2952755905511810774, -0.1292274648535930714 ) ) ;
#24137=CARTESIAN_POINT ( 'NONE',  ( -0.5905511811023615998, 0.1771653543307087630, 0.000000000000000000 ) ) ;
#24138=CARTESIAN_POINT ( 'NONE',  ( -0.4593175853018366950, 0.05413385826771666132, 0.4176697321401328100 ) ) ;
#24139=CARTESIAN_POINT ( 'NONE',  ( -1.305774278215222184, 0.1771653543307087630, 0.09757992244046791164 ) ) ;
#24140=CARTESIAN_POINT ( 'NONE',  ( -0.7020997375328076329, -0.3162353388693409650, -0.4822834645669289433 ) ) ;
#24141=CARTESIAN_POINT ( 'NONE',  ( 1.535433070866142558, 0.2952755905511811885, 0.000000000000000000 ) ) ;
#24143=CARTESIAN_POINT ( 'NONE',  ( -1.095800524934382292, -0.2845877964562161244, -0.3641732283464567121 ) ) ;
#24146=CARTESIAN_POINT ( 'NONE',  ( 1.496062992125984703, -0.1870078740157480879, -0.4822834645669291653 ) ) ;
#24148=CARTESIAN_POINT ( 'NONE',  ( -1.161417322834644716, -0.5400638737290845981, -0.3530559997133363437 ) ) ;
#24149=CARTESIAN_POINT ( 'NONE',  ( -1.391076115485563314, -0.5023911411419708095, -0.1820866141732282451 ) ) ;
#24150=CARTESIAN_POINT ( 'NONE',  ( -0.4790026246719154557, -0.2845877964562159024, 0.3641732283464567677 ) ) ;
#24152=CARTESIAN_POINT ( 'NONE',  ( -0.4527559055118102749, -0.5400638737290845981, -0.3530559997133363437 ) ) ;
#24153=CARTESIAN_POINT ( 'NONE',  ( 0.01312335958005323398, -0.3690944881889765550, -0.3153832671262227771 ) ) ;
#24154=CARTESIAN_POINT ( 'NONE',  ( -1.332020997375327642, -0.2845877964562161244, -0.3641732283464567121 ) ) ;
#24155=CARTESIAN_POINT ( 'NONE',  ( -1.345144356955379816, -0.05778040916215560624, -0.4822834645669293319 ) ) ;
#24156=CARTESIAN_POINT ( 'NONE',  ( 1.338582677165355062, -0.1870078740157480601, -0.3641732283464567677 ) ) ;
#24157=EDGE_CURVE ( 'NONE', #38268, #66982, #34174, .T. ) ;
#24158=CARTESIAN_POINT ( 'NONE',  ( 0.9908136482939640111, -0.6692913385826771977, 0.1292274648535927661 ) ) ;
#24160=CARTESIAN_POINT ( 'NONE',  ( 0.4396325459317593221, 0.1771653543307087075, -0.09757992244046823083 ) ) ;
#24161=CARTESIAN_POINT ( 'NONE',  ( 0.3083989501312343062, -0.05778040916215560624, -0.4822834645669293319 ) ) ;
#24162=CARTESIAN_POINT ( 'NONE',  ( 0.8267716535433077274, 0.1771653543307087630, 0.000000000000000000 ) ) ;
#24163=ORIENTED_EDGE ( 'NONE', *, *, #55359, .T. ) ;
#24164=CARTESIAN_POINT ( 'NONE',  ( -1.023622047244093558, -0.1870078740157479769, 0.4822834645669291653 ) ) ;
#24165=CARTESIAN_POINT ( 'NONE',  ( -0.8267716535433065062, 0.2952755905511811885, 0.000000000000000000 ) ) ;
#24166=CARTESIAN_POINT ( 'NONE',  ( 0.08530183727034192087, -0.3162353388693409650, -0.4822834645669289433 ) ) ;
#24169=CARTESIAN_POINT ( 'NONE',  ( 0.6102362204724416372, -0.5400638737290844871, 0.3530559997133364547 ) ) ;
#24170=CARTESIAN_POINT ( 'NONE',  ( 1.515748031496063186, -0.4536011799217368745, -0.2665933059059886201 ) ) ;
#24171=CARTESIAN_POINT ( 'NONE',  ( 0.1181102362204730916, 0.2952755905511811885, 0.000000000000000000 ) ) ;
#24172=CARTESIAN_POINT ( 'NONE',  ( 0.8792650918635177559, -0.4281496062992127816, -0.4176697321401328100 ) ) ;
#24178=CARTESIAN_POINT ( 'NONE',  ( -0.4527559055118102749, 0.07958543189024085140, 0.2665933059059887866 ) ) ;
#24179=CARTESIAN_POINT ( 'NONE',  ( -0.9383202099737524282, -0.05778040916215522460, 0.4822834645669289988 ) ) ;
#24180=CARTESIAN_POINT ( 'NONE',  ( 0.4396325459317590445, -0.6692913385826771977, 0.1292274648535927661 ) ) ;
#24182=CARTESIAN_POINT ( 'NONE',  ( 0.8923884514435703741, 0.2306618581243848609, 0.2411417322834645549 ) ) ;
#24183=CARTESIAN_POINT ( 'NONE',  ( -1.561679790026246017, -0.4281496062992127816, -0.4176697321401328100 ) ) ;
#24184=CARTESIAN_POINT ( 'NONE',  ( 0.6036745406824153282, -0.6046776061558807314, 0.2411417322834647770 ) ) ;
#24188=CARTESIAN_POINT ( 'NONE',  ( 0.8464566929133865436, 0.1660481256975883668, -0.3530559997133364547 ) ) ;
#24189=CARTESIAN_POINT ( 'NONE',  ( 0.7939632545931766261, -0.05778040916215522460, 0.4822834645669289988 ) ) ;
#24190=CARTESIAN_POINT ( 'NONE',  ( 1.076115485564305141, -0.5023911411419708095, 0.1820866141732285504 ) ) ;
#24191=CARTESIAN_POINT ( 'NONE',  ( 1.587926509186352586, -0.4281496062992127816, -0.4176697321401328100 ) ) ;
#24192=CARTESIAN_POINT ( 'NONE',  ( 1.601049868766404982, 0.2306618581243848609, 0.2411417322834645549 ) ) ;
#24194=CARTESIAN_POINT ( 'NONE',  ( 0.8727034120734913358, -0.05778040916215522460, 0.4822834645669289988 ) ) ;
#24195=CARTESIAN_POINT ( 'NONE',  ( 1.509186351706037543, -0.004921259842519576551, 0.3153832671262227771 ) ) ;
#24196=CARTESIAN_POINT ( 'NONE',  ( -0.4724409448818890911, -0.1870078740157479769, 0.4822834645669291653 ) ) ;
#24197=CARTESIAN_POINT ( 'NONE',  ( -0.8005249343832013809, -0.4281496062992124485, 0.4176697321401328655 ) ) ;
#24198=CARTESIAN_POINT ( 'NONE',  ( -1.541994750656167090, -0.6692913385826773087, -0.1292274648535924053 ) ) ;
#24202=CARTESIAN_POINT ( 'NONE',  ( -1.640419947506561060, -0.004921259842519576551, 0.3153832671262227771 ) ) ;
#24205=VERTEX_POINT ( 'NONE', #7681 ) ;
#24207=CARTESIAN_POINT ( 'NONE',  ( 1.332020997375328974, -0.08942795157528024563, -0.3641732283464568787 ) ) ;
#24214=CARTESIAN_POINT ( 'NONE',  ( -0.8792650918635160906, -0.3690944881889763329, 0.3153832671262228327 ) ) ;
#24215=CARTESIAN_POINT ( 'NONE',  ( -1.358267716535432434, 0.07958543189024071263, -0.2665933059059888421 ) ) ;
#24216=CARTESIAN_POINT ( 'NONE',  ( -1.332020997375327642, -0.05778040916215522460, 0.4822834645669289988 ) ) ;
#24217=CARTESIAN_POINT ( 'NONE',  ( 0.02624671916010564918, 0.2306618581243848609, 0.2411417322834645549 ) ) ;
#24218=CARTESIAN_POINT ( 'NONE',  ( -1.286089238845143479, 0.2306618581243847221, -0.2411417322834647770 ) ) ;
#24220=ORIENTED_EDGE ( 'NONE', *, *, #60997, .F. ) ;
#24221=CARTESIAN_POINT ( 'NONE',  ( 1.607611548556431069, 0.2952755905511811885, 0.1292274648535926551 ) ) ;
#24222=CARTESIAN_POINT ( 'NONE',  ( -1.135170603674539924, 0.2066929133858267098, -0.1054918080437494132 ) ) ;
#24226=CARTESIAN_POINT ( 'NONE',  ( -0.3543307086614165824, 0.1771653543307087630, 0.000000000000000000 ) ) ;
#24227=CARTESIAN_POINT ( 'NONE',  ( -0.9711286089238838626, 0.2306618581243847221, -0.2411417322834647770 ) ) ;
#24228=CARTESIAN_POINT ( 'NONE',  ( 0.9580052493438327987, -0.4281496062992127816, -0.4176697321401328100 ) ) ;
#24229=ORIENTED_EDGE ( 'NONE', *, *, #52610, .F. ) ;
#24230=CARTESIAN_POINT ( 'NONE',  ( 1.220472440944882386, 0.000000000000000000, -0.4445507791589061175 ) ) ;
#24231=CARTESIAN_POINT ( 'NONE',  ( -1.614173228346457378, 1.606230626554505658, 0.1372047244094476981 ) ) ;
#24232=CARTESIAN_POINT ( 'NONE',  ( 1.640419947506562393, -0.4281496062992124485, 0.4176697321401328655 ) ) ;
#24233=CARTESIAN_POINT ( 'NONE',  ( -1.049868766404198794, 0.2306618581243847221, -0.2411417322834647770 ) ) ;
#24235=CARTESIAN_POINT ( 'NONE',  ( -0.09842519685039295696, 0.07958543189024071263, -0.2665933059059888421 ) ) ;
#24237=CARTESIAN_POINT ( 'NONE',  ( -0.05249343832020911260, 0.1283753931104748280, 0.1820866141732283561 ) ) ;
#24238=CARTESIAN_POINT ( 'NONE',  ( 0.4790026246719167324, -0.08942795157527998196, 0.3641732283464567121 ) ) ;
#24239=CARTESIAN_POINT ( 'NONE',  ( 0.5380577427821529035, 0.05413385826771626580, -0.4176697321401330321 ) ) ;
#24240=CARTESIAN_POINT ( 'NONE',  ( -0.6692913385826764205, 0.1771653543307087630, 0.000000000000000000 ) ) ;
#24242=CARTESIAN_POINT ( 'NONE',  ( 1.207349081364829990, -0.6046776061558809534, -0.2411417322834644161 ) ) ;
#24243=CARTESIAN_POINT ( 'NONE',  ( -1.095800524934382292, -0.3162353388693409650, -0.4822834645669289433 ) ) ;
#24245=CARTESIAN_POINT ( 'NONE',  ( 0.01312335958005323398, 0.05413385826771666132, 0.4176697321401328100 ) ) ;
#24246=CARTESIAN_POINT ( 'NONE',  ( -0.4527559055118102749, -0.5400638737290845981, -0.3530559997133363437 ) ) ;
#24247=CARTESIAN_POINT ( 'NONE',  ( 1.437007874015748810, -0.4536011799217368745, -0.2665933059059886201 ) ) ;
#24248=CARTESIAN_POINT ( 'NONE',  ( 0.05905511811023681640, 0.07958543189024071263, -0.2665933059059888421 ) ) ;
#24249=CARTESIAN_POINT ( 'NONE',  ( -0.3280839895013117347, -0.4281496062992124485, 0.4176697321401328655 ) ) ;
#24250=CARTESIAN_POINT ( 'NONE',  ( -1.069553805774277722, -0.6692913385826773087, -0.1292274648535924053 ) ) ;
#24251=CARTESIAN_POINT ( 'NONE',  ( -0.5944687039322197331, 1.968503937007873850, -0.4915354330708654462 ) ) ;
#24252=CARTESIAN_POINT ( 'NONE',  ( 1.686351706036745890, 0.1771653543307087630, 0.09757992244046791164 ) ) ;
#24253=CARTESIAN_POINT ( 'NONE',  ( -0.4002624671916004129, -0.3162353388693405765, 0.4822834645669290543 ) ) ;
#24257=CARTESIAN_POINT ( 'NONE',  ( 1.102362204724410155, -0.1870078740157479769, 0.4822834645669291653 ) ) ;
#24258=CARTESIAN_POINT ( 'NONE',  ( -0.6102362204724400829, 0.07958543189024085140, 0.2665933059059887866 ) ) ;
#24259=CARTESIAN_POINT ( 'NONE',  ( -0.4133858267716528645, 0.1660481256975883668, -0.3530559997133364547 ) ) ;
#24260=CARTESIAN_POINT ( 'NONE',  ( 1.423884514435696413, -0.3162353388693409650, -0.4822834645669289433 ) ) ;
#24261=CARTESIAN_POINT ( 'NONE',  ( 0.8858267716535438430, 0.1660481256975885056, 0.3530559997133364547 ) ) ;
#24263=CARTESIAN_POINT ( 'NONE',  ( -1.141732283464566011, -0.5511811023622047445, 6.969142054262312111E-17 ) ) ;
#24268=CARTESIAN_POINT ( 'NONE',  ( 1.318897637795276356, -0.4536011799217367080, 0.2665933059059888421 ) ) ;
#24270=CARTESIAN_POINT ( 'NONE',  ( 0.8530183727034126306, -0.004921259842519870586, -0.3153832671262229437 ) ) ;
#24272=CARTESIAN_POINT ( 'NONE',  ( 0.6299212598425204535, -0.1870078740157479769, 0.4822834645669291653 ) ) ;
#24273=DIRECTION ( 'NONE',  ( 0.000000000000000000, -1.000000000000000000, 0.000000000000000000 ) ) ;
#24275=CARTESIAN_POINT ( 'NONE',  ( 0.6561679790026253567, -0.5023911411419708095, -0.1820866141732282451 ) ) ;
#24276=CARTESIAN_POINT ( 'NONE',  ( -0.3215223097112853146, -0.05778040916215560624, -0.4822834645669293319 ) ) ;
#24277=CARTESIAN_POINT ( 'NONE',  ( -0.8070866141732276899, 0.1660481256975883668, -0.3530559997133364547 ) ) ;
#24278=CARTESIAN_POINT ( 'NONE',  ( 1.450131233595801428, -0.6692913385826773087, -0.1292274648535924053 ) ) ;
#24281=CARTESIAN_POINT ( 'NONE',  ( 0.09186351706036799403, -0.3690944881889765550, -0.3153832671262227771 ) ) ;
#24282=EDGE_LOOP ( 'NONE', ( #10961, #49739, #74414, #55790 ) ) ;
#24285=CARTESIAN_POINT ( 'NONE',  ( -0.7414698162729651543, 0.2952755905511810774, -0.1292274648535930714 ) ) ;
#24286=CARTESIAN_POINT ( 'NONE',  ( -0.3018372703412066094, -0.4281496062992127816, -0.4176697321401328100 ) ) ;
#24287=CARTESIAN_POINT ( 'NONE',  ( -0.3346456692913377662, 0.1660481256975883668, -0.3530559997133364547 ) ) ;
#24288=CARTESIAN_POINT ( 'NONE',  ( 0.4068241469816281097, 0.05413385826771666132, 0.4176697321401328100 ) ) ;
#24289=CARTESIAN_POINT ( 'NONE',  ( -0.5314960629921250401, 0.1660481256975885056, 0.3530559997133364547 ) ) ;
#24290=CARTESIAN_POINT ( 'NONE',  ( -1.148293963254592542, 0.2952755905511811885, 0.1292274648535926551 ) ) ;
#24292=CARTESIAN_POINT ( 'NONE',  ( -0.6233595800524928121, -0.05778040916215522460, 0.4822834645669289988 ) ) ;
#24293=CARTESIAN_POINT ( 'NONE',  ( 0.6167979002624678353, -0.4281496062992124485, 0.4176697321401328655 ) ) ;
#24294=EDGE_CURVE ( 'NONE', #4976, #52467, #43284, .T. ) ;
#24296=CARTESIAN_POINT ( 'NONE',  ( -0.2099737532808391705, 0.1283753931104748280, 0.1820866141732283561 ) ) ;
#24297=ORIENTED_EDGE ( 'NONE', *, *, #56065, .F. ) ;
#24299=ORIENTED_EDGE ( 'NONE', *, *, #25913, .T. ) ;
#24300=CARTESIAN_POINT ( 'NONE',  ( -1.122047244094487306, -0.4536011799217367080, 0.2665933059059888421 ) ) ;
#24301=CARTESIAN_POINT ( 'NONE',  ( -1.135170603674539924, 0.2952755905511810774, -0.1292274648535930714 ) ) ;
#24302=CARTESIAN_POINT ( 'NONE',  ( -0.7217847769028863381, -0.4281496062992124485, 0.4176697321401328655 ) ) ;
#24304=CARTESIAN_POINT ( 'NONE',  ( -0.5052493438320203589, -0.6692913385826771977, 0.1292274648535927661 ) ) ;
#24305=CARTESIAN_POINT ( 'NONE',  ( -0.8595800524934373854, -0.3162353388693409650, -0.4822834645669289433 ) ) ;
#24306=CARTESIAN_POINT ( 'NONE',  ( -1.601049868766403650, 0.2306618581243847221, -0.2411417322834647770 ) ) ;
#24308=CARTESIAN_POINT ( 'NONE',  ( 0.7217847769028878924, -0.004921259842519576551, 0.3153832671262227771 ) ) ;
#24309=DIRECTION ( 'NONE',  ( 1.000000000000000000, -0.000000000000000000, -0.000000000000000000 ) ) ;
#24311=CARTESIAN_POINT ( 'NONE',  ( -0.05249343832020938322, -0.5023911411419708095, -0.1820866141732282451 ) ) ;
#24312=CARTESIAN_POINT ( 'NONE',  ( -0.1706036745406816491, 0.05413385826771626580, -0.4176697321401330321 ) ) ;
#24314=CARTESIAN_POINT ( 'NONE',  ( 0.1312335958005257930, 0.2306618581243847221, -0.2411417322834647770 ) ) ;
#24315=ORIENTED_EDGE ( 'NONE', *, *, #22171, .F. ) ;
#24320=CARTESIAN_POINT ( 'NONE',  ( 1.604771003085129433, 0.4514378173630678726, -0.1466069496707749775 ) ) ;
#24321=CARTESIAN_POINT ( 'NONE',  ( -1.069553805774277722, 0.1771653543307087630, 0.09757992244046791164 ) ) ;
#24322=EDGE_CURVE ( 'NONE', #76146, #820, #47328, .T. ) ;
#24323=CARTESIAN_POINT ( 'NONE',  ( -1.417322834645668772, -0.1870078740157479769, 0.4822834645669291653 ) ) ;
#24327=CARTESIAN_POINT ( 'NONE',  ( 1.502624671916010790, -0.05778040916215522460, 0.4822834645669289988 ) ) ;
#24328=CARTESIAN_POINT ( 'NONE',  ( 0.4986876640419954376, 0.2306618581243848609, 0.2411417322834645549 ) ) ;
#24329=CARTESIAN_POINT ( 'NONE',  ( -0.09186351706036663400, -0.4281496062992124485, 0.4176697321401328655 ) ) ;
#24330=CARTESIAN_POINT ( 'NONE',  ( -1.167979002624671470, -0.004921259842519576551, 0.3153832671262227771 ) ) ;
#24331=CARTESIAN_POINT ( 'NONE',  ( -0.5577427821522301654, -0.05778040916215560624, -0.4822834645669293319 ) ) ;
#24333=CARTESIAN_POINT ( 'NONE',  ( -0.8595800524934373854, -0.3162353388693409650, -0.4822834645669289433 ) ) ;
#24335=CARTESIAN_POINT ( 'NONE',  ( 1.312335958005249825, 0.1283753931104746893, -0.1820866141732285504 ) ) ;
#24336=CARTESIAN_POINT ( 'NONE',  ( -0.5118110236220466680, -0.5511811023622047445, 6.969142054262312111E-17 ) ) ;
#24337=CARTESIAN_POINT ( 'NONE',  ( 1.023622047244095334, -0.1870078740157479769, 0.3641732283464567677 ) ) ;
#24338=CARTESIAN_POINT ( 'NONE',  ( -1.496062992125983815, -0.1870078740157480879, -0.4822834645669291653 ) ) ;
#24340=CARTESIAN_POINT ( 'NONE',  ( -1.076115485564303809, -0.5023911411419708095, -0.1820866141732282451 ) ) ;
#24342=CARTESIAN_POINT ( 'NONE',  ( 0.3937007874015754361, -0.1870078740157479769, 0.3641732283464567677 ) ) ;
#24343=CARTESIAN_POINT ( 'NONE',  ( -0.4199475065616791736, -0.6046776061558807314, 0.2411417322834647770 ) ) ;
#24345=CARTESIAN_POINT ( 'NONE',  ( 0.03937007874015833325, -0.5511811023622047445, 6.969142054262312111E-17 ) ) ;
#24346=CARTESIAN_POINT ( 'NONE',  ( -1.528871391076114250, 0.1771653543307087075, -0.09757992244046823083 ) ) ;
#24347=CARTESIAN_POINT ( 'NONE',  ( 0.6364829396325465405, -0.3162353388693409650, -0.4822834645669289433 ) ) ;
#24349=CARTESIAN_POINT ( 'NONE',  ( 1.246719160104987623, -0.3690944881889763329, 0.3153832671262228327 ) ) ;
#24350=CARTESIAN_POINT ( 'NONE',  ( -1.148293963254592542, -0.6692913385826773087, -0.1292274648535924053 ) ) ;
#24351=CARTESIAN_POINT ( 'NONE',  ( -0.2952755905511803003, -0.4536011799217368745, -0.2665933059059886201 ) ) ;
#24353=CARTESIAN_POINT ( 'NONE',  ( 0.3149606299212603933, -0.1870078740157479769, 0.3641732283464567677 ) ) ;
#24354=VECTOR ( 'NONE', #14429, 39.37007874015748143 ) ;
#24355=CARTESIAN_POINT ( 'NONE',  ( -1.128608923884513837, -0.6046776061558807314, 0.2411417322834647770 ) ) ;
#24356=CARTESIAN_POINT ( 'NONE',  ( -0.5249343832020990641, 0.2306618581243848609, 0.2411417322834645549 ) ) ;
#24359=CARTESIAN_POINT ( 'NONE',  ( 0.7349081364829402885, -0.5023911411419708095, -0.1820866141732282451 ) ) ;
#24360=CARTESIAN_POINT ( 'NONE',  ( -0.4002624671916004129, -0.3162353388693405765, 0.4822834645669290543 ) ) ;
#24361=CARTESIAN_POINT ( 'NONE',  ( -0.5118110236220466680, 0.2952755905511811885, 0.000000000000000000 ) ) ;
#24362=CARTESIAN_POINT ( 'NONE',  ( -0.9645669291338575535, 0.07958543189024071263, -0.2665933059059888421 ) ) ;
#24364=CARTESIAN_POINT ( 'NONE',  ( 0.1377952755905518800, 0.1660481256975883668, -0.3530559997133364547 ) ) ;
#24365=CARTESIAN_POINT ( 'NONE',  ( -1.299212598425196097, -0.5511811023622047445, 6.969142054262312111E-17 ) ) ;
#24366=CARTESIAN_POINT ( 'NONE',  ( -1.561679790026246017, -0.4281496062992127816, -0.4176697321401328100 ) ) ;
#24368=VERTEX_POINT ( 'NONE', #39653 ) ;
#24369=EDGE_CURVE ( 'NONE', #26176, #41893, #10232, .T. ) ;
#24370=CARTESIAN_POINT ( 'NONE',  ( -1.660104986876639543, -0.08942795157528024563, -0.3641732283464568787 ) ) ;
#24371=CARTESIAN_POINT ( 'NONE',  ( -1.207349081364828880, 0.2306618581243847221, -0.2411417322834647770 ) ) ;
#24372=CARTESIAN_POINT ( 'NONE',  ( -0.6692913385826764205, -0.6692913385826771977, 8.415575281601705876E-17 ) ) ;
#24373=CARTESIAN_POINT ( 'NONE',  ( 1.594488188976378673, 0.1660481256975885056, 0.3530559997133364547 ) ) ;
#24376=CARTESIAN_POINT ( 'NONE',  ( 0.9448818897637802916, -0.1870078740157480879, -0.4822834645669291653 ) ) ;
#24377=CARTESIAN_POINT ( 'NONE',  ( 0.5577427821522316087, -0.05778040916215522460, 0.4822834645669289988 ) ) ;
#24380=CARTESIAN_POINT ( 'NONE',  ( 1.318897637795276356, 0.07958543189024071263, -0.2665933059059888421 ) ) ;
#24383=CARTESIAN_POINT ( 'NONE',  ( -0.9711286089238838626, 0.1283753931104746893, -0.1820866141732285504 ) ) ;
#24386=CARTESIAN_POINT ( 'NONE',  ( 0.5905511811023629321, -0.6692913385826771977, 8.415575281601705876E-17 ) ) ;
#24387=CARTESIAN_POINT ( 'NONE',  ( -0.6561679790026240244, -0.6046776061558807314, 0.2411417322834647770 ) ) ;
#24388=CARTESIAN_POINT ( 'NONE',  ( -1.364829396325458521, -0.6046776061558807314, 0.2411417322834647770 ) ) ;
#24389=CARTESIAN_POINT ( 'NONE',  ( 1.259842519685040019, -0.1870078740157480879, -0.4822834645669291653 ) ) ;
#24390=CARTESIAN_POINT ( 'NONE',  ( -1.574803149606298192, -0.1870078740157480601, -0.3641732283464567677 ) ) ;
#24392=CARTESIAN_POINT ( 'NONE',  ( -0.2230971128608915943, 0.05413385826771666132, 0.4176697321401328100 ) ) ;
#24394=CARTESIAN_POINT ( 'NONE',  ( -1.240157480314959759, -0.5400638737290845981, -0.3530559997133363437 ) ) ;
#24395=CARTESIAN_POINT ( 'NONE',  ( 1.581364829396326277, -0.05778040916215522460, 0.4822834645669289988 ) ) ;
#24396=CARTESIAN_POINT ( 'NONE',  ( 1.430446194225722500, -0.4281496062992127816, -0.4176697321401328100 ) ) ;
#24398=CARTESIAN_POINT ( 'NONE',  ( 0.6561679790026253567, -0.5023911411419708095, -0.1820866141732282451 ) ) ;
#24401=ORIENTED_EDGE ( 'NONE', *, *, #17293, .T. ) ;
#24402=CARTESIAN_POINT ( 'NONE',  ( 0.04593175853018440641, 0.1771653543307087075, -0.09757992244046823083 ) ) ;
#24403=CARTESIAN_POINT ( 'NONE',  ( -1.666666666666665853, 0.05413385826771626580, -0.4176697321401330321 ) ) ;
#24404=CARTESIAN_POINT ( 'NONE',  ( 0.4265091863517067039, -0.6692913385826773087, -0.1292274648535924053 ) ) ;
#24405=CARTESIAN_POINT ( 'NONE',  ( 0.3740157480314966754, 0.1660481256975883668, -0.3530559997133364547 ) ) ;
#24406=CARTESIAN_POINT ( 'NONE',  ( -0.6561679790026240244, -0.6046776061558807314, 0.2411417322834647770 ) ) ;
#24408=CARTESIAN_POINT ( 'NONE',  ( -1.141732283464566011, 0.2952755905511811885, 0.000000000000000000 ) ) ;
#24410=CARTESIAN_POINT ( 'NONE',  ( 1.266404199475066328, -0.08942795157527998196, 0.3641732283464567121 ) ) ;
#24411=CARTESIAN_POINT ( 'NONE',  ( -0.9645669291338575535, 0.1660481256975883668, -0.3530559997133364547 ) ) ;
#24412=CARTESIAN_POINT ( 'NONE',  ( 0.9645669291338591078, -0.5400638737290845981, -0.3530559997133363437 ) ) ;
#24413=CARTESIAN_POINT ( 'NONE',  ( 1.220472440944882608, 0.2952755905511811885, 0.000000000000000000 ) ) ;
#24415=CARTESIAN_POINT ( 'NONE',  ( -1.286089238845143479, -0.6046776061558807314, 0.2411417322834647770 ) ) ;
#24417=CARTESIAN_POINT ( 'NONE',  ( 0.3543307086614179147, 0.2952755905511811885, 0.000000000000000000 ) ) ;
#24420=CARTESIAN_POINT ( 'NONE',  ( 1.666666666666667185, 0.05413385826771666132, 0.4176697321401328100 ) ) ;
#24421=CARTESIAN_POINT ( 'NONE',  ( 0.1706036745406830368, -0.3690944881889765550, -0.3153832671262227771 ) ) ;
#24422=CARTESIAN_POINT ( 'NONE',  ( 0.9908136482939640111, 0.2952755905511810774, -0.1292274648535930714 ) ) ;
#24424=CARTESIAN_POINT ( 'NONE',  ( 0.6889763779527566800, -0.4536011799217367080, 0.2665933059059888421 ) ) ;
#24425=EDGE_CURVE ( 'NONE', #4446, #74449, #3206, .T. ) ;
#24426=CARTESIAN_POINT ( 'NONE',  ( 0.3937007874015754361, -0.1870078740157480879, -0.4822834645669291653 ) ) ;
#24428=CARTESIAN_POINT ( 'NONE',  ( -0.9383202099737524282, -0.05778040916215522460, 0.4822834645669289988 ) ) ;
#24431=CARTESIAN_POINT ( 'NONE',  ( 0.8070866141732288002, 0.07958543189024085140, 0.2665933059059887866 ) ) ;
#24432=EDGE_CURVE ( 'NONE', #49328, #55671, #29010, .T. ) ;
#24433=CARTESIAN_POINT ( 'NONE',  ( 0.1678194419220257749, 2.459406111854941508E-15, 0.4281989832122456430 ) ) ;
#24434=CARTESIAN_POINT ( 'NONE',  ( -0.3346456692913377662, -0.5400638737290844871, 0.3530559997133364547 ) ) ;
#24435=CARTESIAN_POINT ( 'NONE',  ( 0.1509186351706045259, -0.08942795157528024563, -0.3641732283464568787 ) ) ;
#24437=CARTESIAN_POINT ( 'NONE',  ( -0.2362204724409442680, -0.1870078740157480879, -0.4822834645669291653 ) ) ;
#24438=CARTESIAN_POINT ( 'NONE',  ( 0.5643044619422579178, -0.3690944881889765550, -0.3153832671262227771 ) ) ;
#24439=DIRECTION ( 'NONE',  ( -0.1923134147744552103, 0.6939076129059790210, -0.6939076129060079978 ) ) ;
#24441=CARTESIAN_POINT ( 'NONE',  ( 0.1902887139107617975, -0.6692913385826773087, -0.1292274648535924053 ) ) ;
#24442=CARTESIAN_POINT ( 'NONE',  ( 1.102362204724410155, -0.1870078740157480601, -0.3641732283464567677 ) ) ;
#24443=CARTESIAN_POINT ( 'NONE',  ( 0.3833616679418208051, -1.283732188437465593E-15, -0.4281993546915538462 ) ) ;
#24444=CARTESIAN_POINT ( 'NONE',  ( -0.1968503937007867743, -0.5511811023622047445, 6.969142054262312111E-17 ) ) ;
#24445=CARTESIAN_POINT ( 'NONE',  ( -0.6102362204724400829, 0.07958543189024085140, 0.2665933059059887866 ) ) ;
#24446=CARTESIAN_POINT ( 'NONE',  ( -0.4986876640419939388, 0.2306618581243847221, -0.2411417322834647770 ) ) ;
#24447=CARTESIAN_POINT ( 'NONE',  ( 0.2362204724409456558, -0.1870078740157480879, -0.4822834645669291653 ) ) ;
#24448=CARTESIAN_POINT ( 'NONE',  ( 1.148293963254593875, -0.5511811023622046335, 0.09757992244046803654 ) ) ;
#24450=CARTESIAN_POINT ( 'NONE',  ( -1.673228346456691717, 0.1660481256975883668, -0.3530559997133364547 ) ) ;
#24453=CARTESIAN_POINT ( 'NONE',  ( 0.6824146981627303710, -0.6046776061558807314, 0.2411417322834647770 ) ) ;
#24454=CARTESIAN_POINT ( 'NONE',  ( -1.614173228346457378, 1.818966223839196372, 0.1372047244094476981 ) ) ;
#24455=CARTESIAN_POINT ( 'NONE',  ( 0.09842519685039434474, -0.5400638737290845981, -0.3530559997133363437 ) ) ;
#24457=CARTESIAN_POINT ( 'NONE',  ( 0.9908136482939640111, -0.6692913385826771977, 0.1292274648535927661 ) ) ;
#24458=CARTESIAN_POINT ( 'NONE',  ( 0.5577427821522316087, -0.05778040916215522460, 0.4822834645669289988 ) ) ;
#24460=CARTESIAN_POINT ( 'NONE',  ( 0.4921259842519691285, -0.4536011799217368745, -0.2665933059059886201 ) ) ;
#24461=CARTESIAN_POINT ( 'NONE',  ( 1.023622047244095334, -0.1870078740157479769, 0.4822834645669291653 ) ) ;
#24462=ADVANCED_FACE ( 'NONE', ( #74874 ), #74809, .F. ) ;
#24463=CARTESIAN_POINT ( 'NONE',  ( 0.1181102362204730916, -0.5511811023622047445, 6.969142054262312111E-17 ) ) ;
#24464=CARTESIAN_POINT ( 'NONE',  ( -0.2034120734908128059, 0.2952755905511811885, 0.1292274648535926551 ) ) ;
#24466=CARTESIAN_POINT ( 'NONE',  ( 0.1246719160104994284, -0.6692913385826771977, 0.1292274648535927661 ) ) ;
#24467=CARTESIAN_POINT ( 'NONE',  ( -0.8858267716535425107, -0.5400638737290844871, 0.3530559997133364547 ) ) ;
#24468=CARTESIAN_POINT ( 'NONE',  ( -0.2099737532808391705, -0.5023911411419708095, -0.1820866141732282451 ) ) ;
#24469=CARTESIAN_POINT ( 'NONE',  ( 0.4068241469816279987, -0.4281496062992127816, -0.4176697321401328100 ) ) ;
#24470=CARTESIAN_POINT ( 'NONE',  ( 0.8398950131233602345, -0.5023911411419708095, 0.1820866141732285504 ) ) ;
#24471=CARTESIAN_POINT ( 'NONE',  ( -0.4068241469816264999, -0.4281496062992124485, 0.4176697321401328655 ) ) ;
#24472=ADVANCED_FACE ( 'NONE', ( #55475 ), #64024, .F. ) ;
#24475=CARTESIAN_POINT ( 'NONE',  ( 1.364829396325459854, -0.6046776061558809534, -0.2411417322834644161 ) ) ;
#24476=CARTESIAN_POINT ( 'NONE',  ( 1.496062992125985147, -0.1870078740157479769, 0.4822834645669291653 ) ) ;
#24478=CARTESIAN_POINT ( 'NONE',  ( -1.272965879265091305, 0.05413385826771626580, -0.4176697321401330321 ) ) ;
#24479=CARTESIAN_POINT ( 'NONE',  ( -0.8858267716535425107, 0.1660481256975883668, -0.3530559997133364547 ) ) ;
#24483=CARTESIAN_POINT ( 'NONE',  ( 0.5249343832021005074, -0.5023911411419708095, 0.1820866141732285504 ) ) ;
#24485=CARTESIAN_POINT ( 'NONE',  ( 0.5774278215223103139, -0.6046776061558809534, -0.2411417322834644161 ) ) ;
#24487=CARTESIAN_POINT ( 'NONE',  ( -0.5615202218219585983, -1.283732188437465593E-15, -0.4281993546915544568 ) ) ;
#24488=CARTESIAN_POINT ( 'NONE',  ( -0.6102362204724400829, -0.4536011799217368745, -0.2665933059059886201 ) ) ;
#24489=CARTESIAN_POINT ( 'NONE',  ( -1.620734908136482577, -0.5511811023622048555, -0.09757992244046775898 ) ) ;
#24490=CARTESIAN_POINT ( 'NONE',  ( 1.030183727034121421, -0.05778040916215522460, 0.4822834645669289988 ) ) ;
#24491=CARTESIAN_POINT ( 'NONE',  ( 1.555118110236221041, -0.4536011799217367080, 0.2665933059059888421 ) ) ;
#24492=CARTESIAN_POINT ( 'NONE',  ( 0.1837270341207357105, -0.6046776061558809534, -0.2411417322834644161 ) ) ;
#24494=CARTESIAN_POINT ( 'NONE',  ( -0.2755905511811015396, -0.6692913385826771977, 8.415575281601705876E-17 ) ) ;
#24495=( BOUNDED_SURFACE ( )  B_SPLINE_SURFACE ( 1, 2, ( 
 ( #72437, #72019, #15195, #14787, #46745, #59374, #58966, #73265, #66123, #14375, #33305, #45900, #27389, #40853, #8051, #40443, #53050, #78761, #8459, #47156, #27812, #13949, #53472, #72847, #66538, #57143, #58829, #25997, #46186, #19690, #39468, #82840, #7491, #39041, #761, #57976, #37800, #64726, #77359, #78204, #33160, #70617, #71883, #13389, #20534, #31482, #50830, #63886, #25162, #12972, #64307, #71044, #70197, #63477, #38629, #71462, #5812, #19267, #52495, #65154, #7065, #1186, #32313, #76532, #18860, #45348, #44508, #32734, #44920, #26837, #12552, #38211, #58401, #6224, #31900, #57561, #26422, #20116, #52075, #83252, #77782, #45763, #6641, #25575, #51240, #13809, #341, #76939, #51654, #3396, #2571, #68207, #15623, #21919, #73274, #67793, #73697, #41280, #27819, #55129, #29471, #60632, #10130, #42096, #54730, #9299, #54308, #15203, #16037, #35794, #34137, #79189, #53479, #47163, #53889, #60221, #61461, #80839, #79603, #35381, #34969, #61046, #40863, #16451, #66546, #3809, #23152, #8879, #9710, #59798, #34555, #47581, #22337, #47998, #80019, #41683, #2152, #67376, #28230, #29059, #74521, #21505, #16868, #48821, #66966, #80435, #42505, #72855, #2983, #28648, #22745, #48405, #74105, #18901, #50461, #63522, #24386, #63111, #75338, #62703, #31529, #68605, #69013, #82887, #74937, #56374, #5852, #23563, #4212, #76165, #82477, #82073, #69431, #57185, #61871, #5042, #30711, #49646, #17685, #50057, #75752, #18093, #43727, #44551, #11784, #62280, #37437, #50873, #36202, #76573, #25207, #4618, #5449, #10544, #29876, #43315, #55538, #30289, #31110, #81248, #49234, #18502, #17282, #56777, #24793, #11365, #44145, #42910, #10945, #37022, #36602, #55955, #69837, #81668, #23978, #12187, #37844, #58873, #58446, #45808, #7956, #38255, #64768, #7107, #26040, #77402, #26469, #78669, #52120, #77828, #27296, #59281, #39087, #7536, #25618, #806, #20158, #71505, #20580, #63932, #13853, #26880, #20990, #39939, #33618, #52954, #6268, #32358, #57605, #39511, #14277, #52540, #33208, #76984, #1637, #65200, #19313, #13018, #384, #65625, #51700, #71928, #1231, #38672, #78248, #64350, #70241, #19736, #58019, #45391, #46231, #12596, #71088, #31944, #83296, #51281, #13431, #44966, #70662, #6687, #32777, #66866, #27713, #2880, #80331, #80738, #8365, #66028, #59693, #66440, #72751, #74002, #67687, #8777, #47887, #47475, #73595, #53379, #28955, #79087, #48305, #10022, #21405, #22232, #72345, #47059, #34450, #9196, #60119, #15099, #40756, #67274, #2470, #46651, #9607, #14693, #55031, #34032, #35688, #34869, #40349, #28542, #16349, #2049, #41993, #15937, #35276, #60530, #28129, #41584, #54199, #3707, #61353, #79496, #53784, #60940, #29370, #21811, #73167, #15518, #41176, #79915, #3290, #54620, #22646, #82378, #4113, #4520, #37742, #68099, #48720, #4941, #81970, #63012, #30610, #18405, #74835, #17179, #62183, #24285, #31422, #30189, #55440, #74417, #23880, #56677, #57085, #55852, #63416, #24696, #49956, #44048, #17584, #23052, #5753, #56274, #61772, #75654, #81561, #69740, #10445, #50365, #17994, #16762, #42401, #36101, #11682, #5350, #62599, #29778, #43628, #31009, #49545, #76062, #81148, #69332, #43216, #37339, #23463, #12085, #42812, #49130, #68506, #10846, #36507, #75240, #68914, #11264, #36922, #13748, #77296, #18802, #50775, #699, #25935, #12911, #14172, #76475, #44447, #70139, #70984, #51180, #7426, #13328, #45288, #64250, #38154, #33516, #64664, #76878, #12491, #20474, #6584, #39405, #25515, #52431, #38981, #52016, #32255, #51594, #46128, #57502, #57916, #71822, #63826, #7003, #78142, #6165, #31840, #65088, #71400, #32671, #58337, #39830, #83193, #19627, #26356, #38569, #280, #77722, #7850, #20051, #45704, #65519, #82781, #33097, #58763, #19209, #1126, #26776, #25102, #44857, #70556, #60431, #15843, #9920, #28857, #80234, #16248, #27191, #21304, #46543, #73067, #3193, #41492, #22133, #65927, #22550, #2782, #8264, #1949, #72649, #54519, #14999, #60841, #54101, #27611, #28442, #53274, #59178, #40656, #46957, #66341, #9507, #15416, #8679, #52855, #48212, #73908, #2370, #35180 ),
 ( #41895, #78983, #79817, #60015, #47791, #40244, #67178, #33929, #67589, #1536, #59594, #34772, #78565, #34349, #28026, #47376, #41077, #21712, #66766, #20891, #9099, #53685, #73495, #72242, #14591, #79393, #50271, #4019, #68821, #75968, #43950, #42718, #54938, #29683, #4429, #82284, #69646, #75559, #81878, #55758, #35591, #62500, #75147, #18309, #30916, #68414, #61254, #11166, #3608, #29274, #48623, #61678, #80644, #10754, #62087, #36827, #56175, #11583, #16665, #17081, #22957, #74318, #42304, #17492, #4838, #17899, #43123, #56583, #55346, #81052, #74733, #30513, #68002, #36414, #10347, #36008, #30095, #69235, #23367, #81464, #49036, #37242, #24190, #24602, #23782, #49453, #49859, #43536, #62919, #5252, #76781, #59816, #82688, #40471, #38888, #63321, #11990, #5659, #604, #77626, #51495, #21523, #19529, #21112, #70459, #66149, #47182, #58237, #6490, #26260, #31326, #34155, #6071, #8486, #2171, #46772, #56991, #70044, #77199, #83099, #12816, #51921, #32160, #25007, #50680, #13239, #38473, #25419, #27837, #76378, #18712, #44353, #183, #63732, #72463, #25836, #57816, #19113, #12398, #37644, #45186, #31745, #38055, #53499, #44762, #14812, #57407, #70889, #51084, #64157, #64567, #32575, #6904, #79207, #10148, #23580, #81265, #8897, #10561, #61063, #72874, #54747, #74540, #34574, #42524, #74123, #36219, #47599, #48015, #61888, #53908, #35398, #68227, #2589, #66564, #29488, #61479, #3414, #48424, #4229, #40882, #67393, #9727, #28666, #80036, #29076, #15222, #80453, #22762, #29893, #55556, #41700, #35813, #28248, #16469, #42114, #67811, #23170, #60242, #3828, #55147, #79622, #21939, #73293, #15641, #41298, #34986, #66984, #80858, #16886, #48839, #9316, #60650, #3000, #54327, #22355, #73715, #16054, #76588, #62719, #50888, #44160, #75354, #18517, #17702, #70561, #30727, #37038, #5057, #82902, #5464, #56389, #42927, #70258, #44567, #75767, #25222, #57200, #69852, #24402, #69447, #30306, #31126, #18917, #49251, #10962, #68622, #62298, #69030, #43330, #12613, #38271, #11381, #50476, #50072, #76180, #55972, #31544, #81685, #63948, #6285, #23996, #24809, #74954, #49664, #82088, #37452, #63126, #11799, #56793, #17300, #82493, #18109, #12203, #31961, #36620, #57622, #4635, #43742, #37861, #63537, #5868, #32794, #44984, #19754, #77843, #72361, #34047, #65641, #78684, #39526, #78263, #7123, #20172, #7552, #66044, #51298, #8382, #40364, #77418, #58887, #59710, #25635, #58463, #70680, #45408, #45822, #14709, #77001, #7971, #21006, #65214, #20594, #824, #71521, #46667, #401, #26485, #19332, #6704, #13867, #13036, #38689, #64367, #33634, #14292, #33224, #1246, #32373, #58037, #26895, #52554, #64785, #52136, #46246, #26058, #71942, #39955, #51717, #71104, #59297, #1654, #13447, #27311, #52970, #39103, #35702, #53396, #3305, #42008, #36115, #55045, #23066, #42416, #79103, #47492, #72767, #15953, #29385, #67702, #48319, #8793, #48734, #28970, #34467, #28145, #15534, #80752, #41192, #3721, #80347, #53801, #54635, #79513, #2065, #66882, #73184, #9212, #61369, #41599, #34885, #21422, #74431, #16778, #28561, #68114, #10038, #22660, #60546, #22248, #66457, #67289, #10461, #27730, #47076, #15118, #40772, #21829, #2897, #60135, #2486, #54217, #74016, #79933, #16363, #47904, #73611, #9622, #35293, #60955, #68520, #37353, #4127, #10861, #49561, #49970, #75668, #24300, #18008, #12508, #43642, #30204, #69345, #11697, #63026, #12099, #29792, #5364, #18419, #61787, #31437, #82795, #18817, #55453, #23895, #49145, #31025, #5768, #44061, #24710, #36521, #25117, #56693, #62197, #4534, #75255, #57100, #17599, #63432, #82392, #55866, #50378, #81577, #81162, #43231, #68928, #11277, #37757, #76076, #36936, #23478, #50789, #76490, #4955, #44464, #69753, #70155, #62614, #81986, #42827, #74850, #17194, #30624, #56289, #57518, #51196, #57931, #64265, #65536, #59195, #295, #39422, #38997, #65106, #19224, #20490, #44874, #39846, #1554, #70573, #13765, #63843, #12927, #25951, #26374, #52033, #715, #77738, #72258, #20069, #6599, #45721, #78581, #6181, #20907, #52871, #32271, #71418, #46560, #38169, #45305 ) ),
 .UNSPECIFIED., .F., .F., .F. ) 
 B_SPLINE_SURFACE_WITH_KNOTS ( ( 2, 2 ),
 ( 3, 2, 2, 2, 2, 2, 2, 2, 2, 2, 2, 2, 2, 2, 2, 2, 2, 2, 2, 2, 2, 2, 2, 2, 2, 2, 2, 2, 2, 2, 2, 2, 2, 2, 2, 2, 2, 2, 2, 2, 2, 2, 2, 2, 2, 2, 2, 2, 2, 2, 2, 2, 2, 2, 2, 2, 2, 2, 2, 2, 2, 2, 2, 2, 2, 2, 2, 2, 2, 2, 2, 2, 2, 2, 2, 2, 2, 2, 2, 2, 2, 2, 2, 2, 2, 2, 2, 2, 2, 2, 2, 2, 2, 2, 2, 2, 2, 2, 2, 2, 2, 2, 2, 2, 2, 2, 2, 2, 2, 2, 2, 2, 2, 2, 2, 2, 2, 2, 2, 2, 2, 2, 2, 2, 2, 2, 2, 2, 2, 2, 2, 2, 2, 2, 2, 2, 2, 2, 2, 2, 2, 2, 2, 2, 2, 2, 2, 2, 2, 2, 2, 2, 2, 2, 2, 2, 2, 2, 2, 2, 2, 2, 2, 2, 2, 2, 2, 2, 2, 2, 2, 2, 2, 2, 2, 2, 2, 2, 2, 2, 2, 2, 2, 2, 2, 2, 2, 2, 2, 2, 2, 2, 2, 2, 2, 2, 2, 2, 2, 2, 2, 2, 2, 2, 2, 2, 2, 2, 2, 2, 2, 2, 2, 2, 2, 2, 2, 2, 2, 2, 2, 2, 2, 2, 2, 2, 2, 2, 2, 2, 2, 2, 2, 2, 2, 2, 2, 2, 2, 2, 2, 2, 2, 2, 2, 2, 2, 2, 2, 2, 2, 2, 2, 2, 2, 3 ),
 ( 0.000000000000000000, 1.000000000000000000 ),
 ( 0.000000000000000000, 0.003787878787878787984, 0.007575757575757575968, 0.01136363636363636395, 0.01515151515151515194, 0.01893939393939393992, 0.02272727272727272790, 0.02651515151515151589, 0.03030303030303030387, 0.03409090909090908839, 0.03787878787878787984, 0.04166666666666666435, 0.04545454545454545581, 0.04924242424242424032, 0.05303030303030303177, 0.05681818181818181629, 0.06060606060606060774, 0.06439393939393939226, 0.06818181818181817677, 0.07196969696969697516, 0.07575757575757575968, 0.07954545454545454419, 0.08333333333333332871, 0.08712121212121212710, 0.09090909090909091161, 0.09469696969696969613, 0.09848484848484848064, 0.1022727272727272790, 0.1060606060606060635, 0.1098484848484848481, 0.1136363636363636326, 0.1174242424242424310, 0.1212121212121212155, 0.1250000000000000000, 0.1287878787878787845, 0.1325757575757575690, 0.1363636363636363535, 0.1401515151515151381, 0.1439393939393939503, 0.1477272727272727348, 0.1515151515151515194, 0.1553030303030303039, 0.1590909090909090884, 0.1628787878787878729, 0.1666666666666666574, 0.1704545454545454419, 0.1742424242424242542, 0.1780303030303030387, 0.1818181818181818232, 0.1856060606060606077, 0.1893939393939393923, 0.1931818181818181768, 0.1969696969696969613, 0.2007575757575757458, 0.2045454545454545581, 0.2083333333333333426, 0.2121212121212121271, 0.2159090909090909116, 0.2196969696969696961, 0.2234848484848484806, 0.2272727272727272652, 0.2310606060606060497, 0.2348484848484848619, 0.2386363636363636465, 0.2424242424242424310, 0.2462121212121212155, 0.2500000000000000000, 0.2537878787878787845, 0.2575757575757575690, 0.2613636363636363535, 0.2651515151515151381, 0.2689393939393939226, 0.2727272727272727071, 0.2765151515151514916, 0.2803030303030302761, 0.2840909090909091161, 0.2878787878787879007, 0.2916666666666666852, 0.2954545454545454697, 0.2992424242424242542, 0.3030303030303030387, 0.3068181818181818232, 0.3106060606060606077, 0.3143939393939393923, 0.3181818181818181768, 0.3219696969696969613, 0.3257575757575757458, 0.3295454545454545303, 0.3333333333333333148, 0.3371212121212120993, 0.3409090909090908839, 0.3446969696969697239, 0.3484848484848485084, 0.3522727272727272929, 0.3560606060606060774, 0.3598484848484848619, 0.3636363636363636465, 0.3674242424242424310, 0.3712121212121212155, 0.3750000000000000000, 0.3787878787878787845, 0.3825757575757575690, 0.3863636363636363535, 0.3901515151515151381, 0.3939393939393939226, 0.3977272727272727071, 0.4015151515151514916, 0.4053030303030302761, 0.4090909090909091161, 0.4128787878787879007, 0.4166666666666666852, 0.4204545454545454697, 0.4242424242424242542, 0.4280303030303030387, 0.4318181818181818232, 0.4356060606060606077, 0.4393939393939393923, 0.4431818181818181768, 0.4469696969696969613, 0.4507575757575757458, 0.4545454545454545303, 0.4583333333333333148, 0.4621212121212120993, 0.4659090909090908839, 0.4696969696969697239, 0.4734848484848485084, 0.4772727272727272929, 0.4810606060606060774, 0.4848484848484848619, 0.4886363636363636465, 0.4924242424242424310, 0.4962121212121212155, 0.5000000000000000000, 0.5037878787878787845, 0.5075757575757575690, 0.5113636363636363535, 0.5151515151515151381, 0.5189393939393939226, 0.5227272727272727071, 0.5265151515151514916, 0.5303030303030302761, 0.5340909090909090606, 0.5378787878787878451, 0.5416666666666666297, 0.5454545454545454142, 0.5492424242424241987, 0.5530303030303029832, 0.5568181818181817677, 0.5606060606060605522, 0.5643939393939394478, 0.5681818181818182323, 0.5719696969696970168, 0.5757575757575758013, 0.5795454545454545858, 0.5833333333333333703, 0.5871212121212121549, 0.5909090909090909394, 0.5946969696969697239, 0.5984848484848485084, 0.6022727272727272929, 0.6060606060606060774, 0.6098484848484848619, 0.6136363636363636465, 0.6174242424242424310, 0.6212121212121212155, 0.6250000000000000000, 0.6287878787878787845, 0.6325757575757575690, 0.6363636363636363535, 0.6401515151515151381, 0.6439393939393939226, 0.6477272727272727071, 0.6515151515151514916, 0.6553030303030302761, 0.6590909090909090606, 0.6628787878787878451, 0.6666666666666666297, 0.6704545454545454142, 0.6742424242424241987, 0.6780303030303029832, 0.6818181818181817677, 0.6856060606060605522, 0.6893939393939394478, 0.6931818181818182323, 0.6969696969696970168, 0.7007575757575758013, 0.7045454545454545858, 0.7083333333333333703, 0.7121212121212121549, 0.7159090909090909394, 0.7196969696969697239, 0.7234848484848485084, 0.7272727272727272929, 0.7310606060606060774, 0.7348484848484848619, 0.7386363636363636465, 0.7424242424242424310, 0.7462121212121212155, 0.7500000000000000000, 0.7537878787878787845, 0.7575757575757575690, 0.7613636363636363535, 0.7651515151515151381, 0.7689393939393939226, 0.7727272727272727071, 0.7765151515151514916, 0.7803030303030302761, 0.7840909090909090606, 0.7878787878787878451, 0.7916666666666666297, 0.7954545454545454142, 0.7992424242424241987, 0.8030303030303029832, 0.8068181818181817677, 0.8106060606060605522, 0.8143939393939394478, 0.8181818181818182323, 0.8219696969696970168, 0.8257575757575758013, 0.8295454545454545858, 0.8333333333333333703, 0.8371212121212121549, 0.8409090909090909394, 0.8446969696969697239, 0.8484848484848485084, 0.8522727272727272929, 0.8560606060606060774, 0.8598484848484848619, 0.8636363636363636465, 0.8674242424242424310, 0.8712121212121212155, 0.8750000000000000000, 0.8787878787878787845, 0.8825757575757575690, 0.8863636363636363535, 0.8901515151515151381, 0.8939393939393939226, 0.8977272727272727071, 0.9015151515151514916, 0.9053030303030302761, 0.9090909090909090606, 0.9128787878787878451, 0.9166666666666666297, 0.9204545454545454142, 0.9242424242424241987, 0.9280303030303029832, 0.9318181818181817677, 0.9356060606060605522, 0.9393939393939394478, 0.9431818181818182323, 0.9469696969696970168, 0.9507575757575758013, 0.9545454545454545858, 0.9583333333333333703, 0.9621212121212121549, 0.9659090909090909394 ),
 .UNSPECIFIED. ) 
 GEOMETRIC_REPRESENTATION_ITEM ( )  RATIONAL_B_SPLINE_SURFACE ( (
 ( 1.000000000000000000, 0.9659258262890683122, 1.000000000000000000, 0.9659258262890683122, 1.000000000000000000, 0.9659258262890683122, 1.000000000000000000, 0.9659258262890683122, 1.000000000000000000, 0.9659258262890683122, 1.000000000000000000, 0.9659258262890683122, 1.000000000000000000, 0.9659258262890683122, 1.000000000000000000, 0.9659258262890683122, 1.000000000000000000, 0.9659258262890683122, 1.000000000000000000, 0.9659258262890683122, 1.000000000000000000, 0.9659258262890683122, 1.000000000000000000, 0.9659258262890683122, 1.000000000000000000, 0.9659258262890683122, 1.000000000000000000, 0.9659258262890683122, 1.000000000000000000, 0.9659258262890683122, 1.000000000000000000, 0.9659258262890683122, 1.000000000000000000, 0.9659258262890683122, 1.000000000000000000, 0.9659258262890683122, 1.000000000000000000, 0.9659258262890683122, 1.000000000000000000, 0.9659258262890683122, 1.000000000000000000, 0.9659258262890683122, 1.000000000000000000, 0.9659258262890683122, 1.000000000000000000, 0.9659258262890683122, 1.000000000000000000, 0.9659258262890683122, 1.000000000000000000, 0.9659258262890683122, 1.000000000000000000, 0.9659258262890683122, 1.000000000000000000, 0.9659258262890683122, 1.000000000000000000, 0.9659258262890683122, 1.000000000000000000, 0.9659258262890683122, 1.000000000000000000, 0.9659258262890683122, 1.000000000000000000, 0.9659258262890683122, 1.000000000000000000, 0.9659258262890683122, 1.000000000000000000, 0.9659258262890683122, 1.000000000000000000, 0.9659258262890683122, 1.000000000000000000, 0.9659258262890683122, 1.000000000000000000, 0.9659258262890683122, 1.000000000000000000, 0.9659258262890683122, 1.000000000000000000, 0.9659258262890683122, 1.000000000000000000, 0.9659258262890683122, 1.000000000000000000, 0.9659258262890683122, 1.000000000000000000, 0.9659258262890683122, 1.000000000000000000, 0.9659258262890683122, 1.000000000000000000, 0.9659258262890683122, 1.000000000000000000, 0.9659258262890683122, 1.000000000000000000, 0.9659258262890683122, 1.000000000000000000, 0.9659258262890683122, 1.000000000000000000, 0.9659258262890683122, 1.000000000000000000, 0.9659258262890683122, 1.000000000000000000, 0.9659258262890683122, 1.000000000000000000, 0.9659258262890683122, 1.000000000000000000, 0.9659258262890683122, 1.000000000000000000, 0.9659258262890683122, 1.000000000000000000, 0.9659258262890683122, 1.000000000000000000, 0.9659258262890683122, 1.000000000000000000, 0.9659258262890683122, 1.000000000000000000, 0.9659258262890683122, 1.000000000000000000, 0.9659258262890683122, 1.000000000000000000, 0.9659258262890683122, 1.000000000000000000, 0.9659258262890683122, 1.000000000000000000, 0.9659258262890683122, 1.000000000000000000, 0.9659258262890683122, 1.000000000000000000, 0.9659258262890683122, 1.000000000000000000, 0.9659258262890683122, 1.000000000000000000, 0.9659258262890683122, 1.000000000000000000, 0.9659258262890683122, 1.000000000000000000, 0.9659258262890683122, 1.000000000000000000, 0.9659258262890683122, 1.000000000000000000, 0.9659258262890683122, 1.000000000000000000, 0.9659258262890683122, 1.000000000000000000, 0.9659258262890683122, 1.000000000000000000, 0.9659258262890683122, 1.000000000000000000, 0.9659258262890683122, 1.000000000000000000, 0.9659258262890683122, 1.000000000000000000, 0.9659258262890683122, 1.000000000000000000, 0.9659258262890683122, 1.000000000000000000, 0.9659258262890683122, 1.000000000000000000, 0.9659258262890683122, 1.000000000000000000, 0.9659258262890683122, 1.000000000000000000, 0.9659258262890683122, 1.000000000000000000, 0.9659258262890683122, 1.000000000000000000, 0.9659258262890683122, 1.000000000000000000, 0.9659258262890683122, 1.000000000000000000, 0.9659258262890683122, 1.000000000000000000, 0.9659258262890683122, 1.000000000000000000, 0.9659258262890683122, 1.000000000000000000, 0.9659258262890683122, 1.000000000000000000, 0.9659258262890683122, 1.000000000000000000, 0.9659258262890683122, 1.000000000000000000, 0.9659258262890683122, 1.000000000000000000, 0.9659258262890683122, 1.000000000000000000, 0.9659258262890683122, 1.000000000000000000, 0.9659258262890683122, 1.000000000000000000, 0.9659258262890683122, 1.000000000000000000, 0.9659258262890683122, 1.000000000000000000, 0.9659258262890683122, 1.000000000000000000, 0.9659258262890683122, 1.000000000000000000, 0.9659258262890683122, 1.000000000000000000, 0.9659258262890683122, 1.000000000000000000, 0.9659258262890683122, 1.000000000000000000, 0.9659258262890683122, 1.000000000000000000, 0.9659258262890683122, 1.000000000000000000, 0.9659258262890683122, 1.000000000000000000, 0.9659258262890683122, 1.000000000000000000, 0.9659258262890683122, 1.000000000000000000, 0.9659258262890683122, 1.000000000000000000, 0.9659258262890683122, 1.000000000000000000, 0.9659258262890683122, 1.000000000000000000, 0.9659258262890683122, 1.000000000000000000, 0.9659258262890683122, 1.000000000000000000, 0.9659258262890683122, 1.000000000000000000, 0.9659258262890683122, 1.000000000000000000, 0.9659258262890683122, 1.000000000000000000, 0.9659258262890683122, 1.000000000000000000, 0.9659258262890683122, 1.000000000000000000, 0.9659258262890683122, 1.000000000000000000, 0.9659258262890683122, 1.000000000000000000, 0.9659258262890683122, 1.000000000000000000, 0.9659258262890683122, 1.000000000000000000, 0.9659258262890683122, 1.000000000000000000, 0.9659258262890683122, 1.000000000000000000, 0.9659258262890683122, 1.000000000000000000, 0.9659258262890683122, 1.000000000000000000, 0.9659258262890683122, 1.000000000000000000, 0.9659258262890683122, 1.000000000000000000, 0.9659258262890683122, 1.000000000000000000, 0.9659258262890683122, 1.000000000000000000, 0.9659258262890683122, 1.000000000000000000, 0.9659258262890683122, 1.000000000000000000, 0.9659258262890683122, 1.000000000000000000, 0.9659258262890683122, 1.000000000000000000, 0.9659258262890683122, 1.000000000000000000, 0.9659258262890683122, 1.000000000000000000, 0.9659258262890683122, 1.000000000000000000, 0.9659258262890683122, 1.000000000000000000, 0.9659258262890683122, 1.000000000000000000, 0.9659258262890683122, 1.000000000000000000, 0.9659258262890683122, 1.000000000000000000, 0.9659258262890683122, 1.000000000000000000, 0.9659258262890683122, 1.000000000000000000, 0.9659258262890683122, 1.000000000000000000, 0.9659258262890683122, 1.000000000000000000, 0.9659258262890683122, 1.000000000000000000, 0.9659258262890683122, 1.000000000000000000, 0.9659258262890683122, 1.000000000000000000, 0.9659258262890683122, 1.000000000000000000, 0.9659258262890683122, 1.000000000000000000, 0.9659258262890683122, 1.000000000000000000, 0.9659258262890683122, 1.000000000000000000, 0.9659258262890683122, 1.000000000000000000, 0.9659258262890683122, 1.000000000000000000, 0.9659258262890683122, 1.000000000000000000, 0.9659258262890683122, 1.000000000000000000, 0.9659258262890683122, 1.000000000000000000, 0.9659258262890683122, 1.000000000000000000, 0.9659258262890683122, 1.000000000000000000, 0.9659258262890683122, 1.000000000000000000, 0.9659258262890683122, 1.000000000000000000, 0.9659258262890683122, 1.000000000000000000, 0.9659258262890683122, 1.000000000000000000, 0.9659258262890683122, 1.000000000000000000, 0.9659258262890683122, 1.000000000000000000, 0.9659258262890683122, 1.000000000000000000, 0.9659258262890683122, 1.000000000000000000, 0.9659258262890683122, 1.000000000000000000, 0.9659258262890683122, 1.000000000000000000, 0.9659258262890683122, 1.000000000000000000, 0.9659258262890683122, 1.000000000000000000, 0.9659258262890683122, 1.000000000000000000, 0.9659258262890683122, 1.000000000000000000, 0.9659258262890683122, 1.000000000000000000, 0.9659258262890683122, 1.000000000000000000, 0.9659258262890683122, 1.000000000000000000, 0.9659258262890683122, 1.000000000000000000, 0.9659258262890683122, 1.000000000000000000, 0.9659258262890683122, 1.000000000000000000, 0.9659258262890683122, 1.000000000000000000, 0.9659258262890683122, 1.000000000000000000, 0.9659258262890683122, 1.000000000000000000, 0.9659258262890683122, 1.000000000000000000, 0.9659258262890683122, 1.000000000000000000, 0.9659258262890683122, 1.000000000000000000, 0.9659258262890683122, 1.000000000000000000, 0.9659258262890683122, 1.000000000000000000, 0.9659258262890683122, 1.000000000000000000, 0.9659258262890683122, 1.000000000000000000, 0.9659258262890683122, 1.000000000000000000, 0.9659258262890683122, 1.000000000000000000, 0.9659258262890683122, 1.000000000000000000, 0.9659258262890683122, 1.000000000000000000, 0.9659258262890683122, 1.000000000000000000, 0.9659258262890683122, 1.000000000000000000, 0.9659258262890683122, 1.000000000000000000, 0.9659258262890683122, 1.000000000000000000, 0.9659258262890683122, 1.000000000000000000, 0.9659258262890683122, 1.000000000000000000, 0.9659258262890683122, 1.000000000000000000, 0.9659258262890683122, 1.000000000000000000, 0.9659258262890683122, 1.000000000000000000, 0.9659258262890683122, 1.000000000000000000, 0.9659258262890683122, 1.000000000000000000, 0.9659258262890683122, 1.000000000000000000, 0.9659258262890683122, 1.000000000000000000, 0.9659258262890683122, 1.000000000000000000, 0.9659258262890683122, 1.000000000000000000, 0.9659258262890683122, 1.000000000000000000, 0.9659258262890683122, 1.000000000000000000, 0.9659258262890683122, 1.000000000000000000, 0.9659258262890683122, 1.000000000000000000, 0.9659258262890683122, 1.000000000000000000, 0.9659258262890683122, 1.000000000000000000, 0.9659258262890683122, 1.000000000000000000, 0.9659258262890683122, 1.000000000000000000, 0.9659258262890683122, 1.000000000000000000, 0.9659258262890683122, 1.000000000000000000, 0.9659258262890683122, 1.000000000000000000, 0.9659258262890683122, 1.000000000000000000, 0.9659258262890683122, 1.000000000000000000, 0.9659258262890683122, 1.000000000000000000, 0.9659258262890683122, 1.000000000000000000, 0.9659258262890683122, 1.000000000000000000, 0.9659258262890683122, 1.000000000000000000, 0.9659258262890683122, 1.000000000000000000, 0.9659258262890683122, 1.000000000000000000, 0.9659258262890683122, 1.000000000000000000, 0.9659258262890683122, 1.000000000000000000, 0.9659258262890683122, 1.000000000000000000, 0.9659258262890683122, 1.000000000000000000, 0.9659258262890683122, 1.000000000000000000, 0.9659258262890683122, 1.000000000000000000, 0.9659258262890683122, 1.000000000000000000, 0.9659258262890683122, 1.000000000000000000, 0.9659258262890683122, 1.000000000000000000, 0.9659258262890683122, 1.000000000000000000, 0.9659258262890683122, 1.000000000000000000, 0.9659258262890683122, 1.000000000000000000, 0.9659258262890683122, 1.000000000000000000, 0.9659258262890683122, 1.000000000000000000, 0.9659258262890683122, 1.000000000000000000, 0.9659258262890683122, 1.000000000000000000, 0.9659258262890683122, 1.000000000000000000, 0.9659258262890683122, 1.000000000000000000, 0.9659258262890683122, 1.000000000000000000, 0.9659258262890683122, 1.000000000000000000, 0.9659258262890683122, 1.000000000000000000, 0.9659258262890683122, 1.000000000000000000, 0.9659258262890683122, 1.000000000000000000, 0.9659258262890683122, 1.000000000000000000, 0.9659258262890683122, 1.000000000000000000, 0.9659258262890683122, 1.000000000000000000, 0.9659258262890683122, 1.000000000000000000, 0.9659258262890683122, 1.000000000000000000, 0.9659258262890683122, 1.000000000000000000, 0.9659258262890683122, 1.000000000000000000, 0.9659258262890683122, 1.000000000000000000, 0.9659258262890683122, 1.000000000000000000),
 ( 1.000000000000000000, 0.9659258262890683122, 1.000000000000000000, 0.9659258262890683122, 1.000000000000000000, 0.9659258262890683122, 1.000000000000000000, 0.9659258262890683122, 1.000000000000000000, 0.9659258262890683122, 1.000000000000000000, 0.9659258262890683122, 1.000000000000000000, 0.9659258262890683122, 1.000000000000000000, 0.9659258262890683122, 1.000000000000000000, 0.9659258262890683122, 1.000000000000000000, 0.9659258262890683122, 1.000000000000000000, 0.9659258262890683122, 1.000000000000000000, 0.9659258262890683122, 1.000000000000000000, 0.9659258262890683122, 1.000000000000000000, 0.9659258262890683122, 1.000000000000000000, 0.9659258262890683122, 1.000000000000000000, 0.9659258262890683122, 1.000000000000000000, 0.9659258262890683122, 1.000000000000000000, 0.9659258262890683122, 1.000000000000000000, 0.9659258262890683122, 1.000000000000000000, 0.9659258262890683122, 1.000000000000000000, 0.9659258262890683122, 1.000000000000000000, 0.9659258262890683122, 1.000000000000000000, 0.9659258262890683122, 1.000000000000000000, 0.9659258262890683122, 1.000000000000000000, 0.9659258262890683122, 1.000000000000000000, 0.9659258262890683122, 1.000000000000000000, 0.9659258262890683122, 1.000000000000000000, 0.9659258262890683122, 1.000000000000000000, 0.9659258262890683122, 1.000000000000000000, 0.9659258262890683122, 1.000000000000000000, 0.9659258262890683122, 1.000000000000000000, 0.9659258262890683122, 1.000000000000000000, 0.9659258262890683122, 1.000000000000000000, 0.9659258262890683122, 1.000000000000000000, 0.9659258262890683122, 1.000000000000000000, 0.9659258262890683122, 1.000000000000000000, 0.9659258262890683122, 1.000000000000000000, 0.9659258262890683122, 1.000000000000000000, 0.9659258262890683122, 1.000000000000000000, 0.9659258262890683122, 1.000000000000000000, 0.9659258262890683122, 1.000000000000000000, 0.9659258262890683122, 1.000000000000000000, 0.9659258262890683122, 1.000000000000000000, 0.9659258262890683122, 1.000000000000000000, 0.9659258262890683122, 1.000000000000000000, 0.9659258262890683122, 1.000000000000000000, 0.9659258262890683122, 1.000000000000000000, 0.9659258262890683122, 1.000000000000000000, 0.9659258262890683122, 1.000000000000000000, 0.9659258262890683122, 1.000000000000000000, 0.9659258262890683122, 1.000000000000000000, 0.9659258262890683122, 1.000000000000000000, 0.9659258262890683122, 1.000000000000000000, 0.9659258262890683122, 1.000000000000000000, 0.9659258262890683122, 1.000000000000000000, 0.9659258262890683122, 1.000000000000000000, 0.9659258262890683122, 1.000000000000000000, 0.9659258262890683122, 1.000000000000000000, 0.9659258262890683122, 1.000000000000000000, 0.9659258262890683122, 1.000000000000000000, 0.9659258262890683122, 1.000000000000000000, 0.9659258262890683122, 1.000000000000000000, 0.9659258262890683122, 1.000000000000000000, 0.9659258262890683122, 1.000000000000000000, 0.9659258262890683122, 1.000000000000000000, 0.9659258262890683122, 1.000000000000000000, 0.9659258262890683122, 1.000000000000000000, 0.9659258262890683122, 1.000000000000000000, 0.9659258262890683122, 1.000000000000000000, 0.9659258262890683122, 1.000000000000000000, 0.9659258262890683122, 1.000000000000000000, 0.9659258262890683122, 1.000000000000000000, 0.9659258262890683122, 1.000000000000000000, 0.9659258262890683122, 1.000000000000000000, 0.9659258262890683122, 1.000000000000000000, 0.9659258262890683122, 1.000000000000000000, 0.9659258262890683122, 1.000000000000000000, 0.9659258262890683122, 1.000000000000000000, 0.9659258262890683122, 1.000000000000000000, 0.9659258262890683122, 1.000000000000000000, 0.9659258262890683122, 1.000000000000000000, 0.9659258262890683122, 1.000000000000000000, 0.9659258262890683122, 1.000000000000000000, 0.9659258262890683122, 1.000000000000000000, 0.9659258262890683122, 1.000000000000000000, 0.9659258262890683122, 1.000000000000000000, 0.9659258262890683122, 1.000000000000000000, 0.9659258262890683122, 1.000000000000000000, 0.9659258262890683122, 1.000000000000000000, 0.9659258262890683122, 1.000000000000000000, 0.9659258262890683122, 1.000000000000000000, 0.9659258262890683122, 1.000000000000000000, 0.9659258262890683122, 1.000000000000000000, 0.9659258262890683122, 1.000000000000000000, 0.9659258262890683122, 1.000000000000000000, 0.9659258262890683122, 1.000000000000000000, 0.9659258262890683122, 1.000000000000000000, 0.9659258262890683122, 1.000000000000000000, 0.9659258262890683122, 1.000000000000000000, 0.9659258262890683122, 1.000000000000000000, 0.9659258262890683122, 1.000000000000000000, 0.9659258262890683122, 1.000000000000000000, 0.9659258262890683122, 1.000000000000000000, 0.9659258262890683122, 1.000000000000000000, 0.9659258262890683122, 1.000000000000000000, 0.9659258262890683122, 1.000000000000000000, 0.9659258262890683122, 1.000000000000000000, 0.9659258262890683122, 1.000000000000000000, 0.9659258262890683122, 1.000000000000000000, 0.9659258262890683122, 1.000000000000000000, 0.9659258262890683122, 1.000000000000000000, 0.9659258262890683122, 1.000000000000000000, 0.9659258262890683122, 1.000000000000000000, 0.9659258262890683122, 1.000000000000000000, 0.9659258262890683122, 1.000000000000000000, 0.9659258262890683122, 1.000000000000000000, 0.9659258262890683122, 1.000000000000000000, 0.9659258262890683122, 1.000000000000000000, 0.9659258262890683122, 1.000000000000000000, 0.9659258262890683122, 1.000000000000000000, 0.9659258262890683122, 1.000000000000000000, 0.9659258262890683122, 1.000000000000000000, 0.9659258262890683122, 1.000000000000000000, 0.9659258262890683122, 1.000000000000000000, 0.9659258262890683122, 1.000000000000000000, 0.9659258262890683122, 1.000000000000000000, 0.9659258262890683122, 1.000000000000000000, 0.9659258262890683122, 1.000000000000000000, 0.9659258262890683122, 1.000000000000000000, 0.9659258262890683122, 1.000000000000000000, 0.9659258262890683122, 1.000000000000000000, 0.9659258262890683122, 1.000000000000000000, 0.9659258262890683122, 1.000000000000000000, 0.9659258262890683122, 1.000000000000000000, 0.9659258262890683122, 1.000000000000000000, 0.9659258262890683122, 1.000000000000000000, 0.9659258262890683122, 1.000000000000000000, 0.9659258262890683122, 1.000000000000000000, 0.9659258262890683122, 1.000000000000000000, 0.9659258262890683122, 1.000000000000000000, 0.9659258262890683122, 1.000000000000000000, 0.9659258262890683122, 1.000000000000000000, 0.9659258262890683122, 1.000000000000000000, 0.9659258262890683122, 1.000000000000000000, 0.9659258262890683122, 1.000000000000000000, 0.9659258262890683122, 1.000000000000000000, 0.9659258262890683122, 1.000000000000000000, 0.9659258262890683122, 1.000000000000000000, 0.9659258262890683122, 1.000000000000000000, 0.9659258262890683122, 1.000000000000000000, 0.9659258262890683122, 1.000000000000000000, 0.9659258262890683122, 1.000000000000000000, 0.9659258262890683122, 1.000000000000000000, 0.9659258262890683122, 1.000000000000000000, 0.9659258262890683122, 1.000000000000000000, 0.9659258262890683122, 1.000000000000000000, 0.9659258262890683122, 1.000000000000000000, 0.9659258262890683122, 1.000000000000000000, 0.9659258262890683122, 1.000000000000000000, 0.9659258262890683122, 1.000000000000000000, 0.9659258262890683122, 1.000000000000000000, 0.9659258262890683122, 1.000000000000000000, 0.9659258262890683122, 1.000000000000000000, 0.9659258262890683122, 1.000000000000000000, 0.9659258262890683122, 1.000000000000000000, 0.9659258262890683122, 1.000000000000000000, 0.9659258262890683122, 1.000000000000000000, 0.9659258262890683122, 1.000000000000000000, 0.9659258262890683122, 1.000000000000000000, 0.9659258262890683122, 1.000000000000000000, 0.9659258262890683122, 1.000000000000000000, 0.9659258262890683122, 1.000000000000000000, 0.9659258262890683122, 1.000000000000000000, 0.9659258262890683122, 1.000000000000000000, 0.9659258262890683122, 1.000000000000000000, 0.9659258262890683122, 1.000000000000000000, 0.9659258262890683122, 1.000000000000000000, 0.9659258262890683122, 1.000000000000000000, 0.9659258262890683122, 1.000000000000000000, 0.9659258262890683122, 1.000000000000000000, 0.9659258262890683122, 1.000000000000000000, 0.9659258262890683122, 1.000000000000000000, 0.9659258262890683122, 1.000000000000000000, 0.9659258262890683122, 1.000000000000000000, 0.9659258262890683122, 1.000000000000000000, 0.9659258262890683122, 1.000000000000000000, 0.9659258262890683122, 1.000000000000000000, 0.9659258262890683122, 1.000000000000000000, 0.9659258262890683122, 1.000000000000000000, 0.9659258262890683122, 1.000000000000000000, 0.9659258262890683122, 1.000000000000000000, 0.9659258262890683122, 1.000000000000000000, 0.9659258262890683122, 1.000000000000000000, 0.9659258262890683122, 1.000000000000000000, 0.9659258262890683122, 1.000000000000000000, 0.9659258262890683122, 1.000000000000000000, 0.9659258262890683122, 1.000000000000000000, 0.9659258262890683122, 1.000000000000000000, 0.9659258262890683122, 1.000000000000000000, 0.9659258262890683122, 1.000000000000000000, 0.9659258262890683122, 1.000000000000000000, 0.9659258262890683122, 1.000000000000000000, 0.9659258262890683122, 1.000000000000000000, 0.9659258262890683122, 1.000000000000000000, 0.9659258262890683122, 1.000000000000000000, 0.9659258262890683122, 1.000000000000000000, 0.9659258262890683122, 1.000000000000000000, 0.9659258262890683122, 1.000000000000000000, 0.9659258262890683122, 1.000000000000000000, 0.9659258262890683122, 1.000000000000000000, 0.9659258262890683122, 1.000000000000000000, 0.9659258262890683122, 1.000000000000000000, 0.9659258262890683122, 1.000000000000000000, 0.9659258262890683122, 1.000000000000000000, 0.9659258262890683122, 1.000000000000000000, 0.9659258262890683122, 1.000000000000000000, 0.9659258262890683122, 1.000000000000000000, 0.9659258262890683122, 1.000000000000000000, 0.9659258262890683122, 1.000000000000000000, 0.9659258262890683122, 1.000000000000000000, 0.9659258262890683122, 1.000000000000000000, 0.9659258262890683122, 1.000000000000000000, 0.9659258262890683122, 1.000000000000000000, 0.9659258262890683122, 1.000000000000000000, 0.9659258262890683122, 1.000000000000000000, 0.9659258262890683122, 1.000000000000000000, 0.9659258262890683122, 1.000000000000000000, 0.9659258262890683122, 1.000000000000000000, 0.9659258262890683122, 1.000000000000000000, 0.9659258262890683122, 1.000000000000000000, 0.9659258262890683122, 1.000000000000000000, 0.9659258262890683122, 1.000000000000000000, 0.9659258262890683122, 1.000000000000000000, 0.9659258262890683122, 1.000000000000000000, 0.9659258262890683122, 1.000000000000000000, 0.9659258262890683122, 1.000000000000000000, 0.9659258262890683122, 1.000000000000000000, 0.9659258262890683122, 1.000000000000000000, 0.9659258262890683122, 1.000000000000000000, 0.9659258262890683122, 1.000000000000000000, 0.9659258262890683122, 1.000000000000000000, 0.9659258262890683122, 1.000000000000000000, 0.9659258262890683122, 1.000000000000000000, 0.9659258262890683122, 1.000000000000000000, 0.9659258262890683122, 1.000000000000000000, 0.9659258262890683122, 1.000000000000000000, 0.9659258262890683122, 1.000000000000000000, 0.9659258262890683122, 1.000000000000000000, 0.9659258262890683122, 1.000000000000000000, 0.9659258262890683122, 1.000000000000000000, 0.9659258262890683122, 1.000000000000000000, 0.9659258262890683122, 1.000000000000000000, 0.9659258262890683122, 1.000000000000000000, 0.9659258262890683122, 1.000000000000000000, 0.9659258262890683122, 1.000000000000000000) ) ) 
 REPRESENTATION_ITEM ( '' )  SURFACE ( )  );
#24496=CARTESIAN_POINT ( 'NONE',  ( -1.423884514435694859, -0.2845877964562159024, 0.3641732283464567677 ) ) ;
#24497=CARTESIAN_POINT ( 'NONE',  ( -0.6299212598425188991, -0.1870078740157479769, 0.4822834645669291653 ) ) ;
#24502=CARTESIAN_POINT ( 'NONE',  ( 0.3346456692913393205, -0.5400638737290845981, -0.3530559997133363437 ) ) ;
#24504=CARTESIAN_POINT ( 'NONE',  ( -0.5118110236220466680, -0.6692913385826771977, 8.415575281601705876E-17 ) ) ;
#24505=CARTESIAN_POINT ( 'NONE',  ( -1.391076115485563314, -0.6046776061558809534, -0.2411417322834644161 ) ) ;
#24506=CARTESIAN_POINT ( 'NONE',  ( 0.5708661417322841158, -0.5400638737290845981, -0.3530559997133363437 ) ) ;
#24507=CARTESIAN_POINT ( 'NONE',  ( -0.09186351706036663400, -0.4281496062992124485, 0.4176697321401328655 ) ) ;
#24509=CARTESIAN_POINT ( 'NONE',  ( -0.6561679790026240244, -0.6046776061558807314, 0.2411417322834647770 ) ) ;
#24510=CARTESIAN_POINT ( 'NONE',  ( 0.3674540682414705883, -0.6046776061558807314, 0.2411417322834647770 ) ) ;
#24511=CARTESIAN_POINT ( 'NONE',  ( -0.3805774278215216522, 0.05413385826771666132, 0.4176697321401328100 ) ) ;
#24512=CARTESIAN_POINT ( 'NONE',  ( 0.2362204724409456558, -0.1870078740157479769, 0.3641732283464567677 ) ) ;
#24514=CARTESIAN_POINT ( 'NONE',  ( 0.09186351706036799403, -0.4281496062992127816, -0.4176697321401328100 ) ) ;
#24516=CARTESIAN_POINT ( 'NONE',  ( -0.7080320533160963103, 1.900312960331933976, -0.5309055118110235227 ) ) ;
#24517=CARTESIAN_POINT ( 'NONE',  ( 1.548556430446194954, -0.6046776061558807314, 0.2411417322834647770 ) ) ;
#24519=ORIENTED_EDGE ( 'NONE', *, *, #82130, .F. ) ;
#24520=ORIENTED_EDGE ( 'NONE', *, *, #28027, .F. ) ;
#24521=CARTESIAN_POINT ( 'NONE',  ( 0.8070866141732289112, -0.5400638737290845981, -0.3530559997133363437 ) ) ;
#24522=CARTESIAN_POINT ( 'NONE',  ( 0.1574803149606306130, -0.1870078740157479769, 0.3641732283464567677 ) ) ;
#24524=CARTESIAN_POINT ( 'NONE',  ( -2.795275590551183242, 1.614173228346456712, -1.327125379919507468E-16 ) ) ;
#24530=CARTESIAN_POINT ( 'NONE',  ( 0.3740157480314966754, 0.1660481256975883668, -0.3530559997133364547 ) ) ;
#24531=CARTESIAN_POINT ( 'NONE',  ( -1.095800524934382292, -0.3162353388693409650, -0.4822834645669289433 ) ) ;
#24532=CARTESIAN_POINT ( 'NONE',  ( -1.246719160104986512, 0.05413385826771666132, 0.4176697321401328100 ) ) ;
#24533=CARTESIAN_POINT ( 'NONE',  ( 0.2362204724409456558, -0.1870078740157480879, -0.4822834645669291653 ) ) ;
#24534=CARTESIAN_POINT ( 'NONE',  ( 0.9317585301837276734, -0.4281496062992124485, 0.4176697321401328655 ) ) ;
#24535=CARTESIAN_POINT ( 'NONE',  ( 1.502624671916010790, -0.08942795157527998196, 0.3641732283464567121 ) ) ;
#24537=CARTESIAN_POINT ( 'NONE',  ( 1.194225721784777594, -0.004921259842519576551, 0.3153832671262227771 ) ) ;
#24538=CARTESIAN_POINT ( 'NONE',  ( -0.7611548556430438595, -0.6046776061558809534, -0.2411417322834644161 ) ) ;
#24540=CARTESIAN_POINT ( 'NONE',  ( -1.555118110236219930, -0.4536011799217368745, -0.2665933059059886201 ) ) ;
#24543=CARTESIAN_POINT ( 'NONE',  ( -0.2034120734908128059, 0.2952755905511811885, 0.1292274648535926551 ) ) ;
#24544=CARTESIAN_POINT ( 'NONE',  ( 0.9580052493438327987, -0.4281496062992127816, -0.4176697321401328100 ) ) ;
#24546=CARTESIAN_POINT ( 'NONE',  ( -1.423884514435694859, -0.2845877964562159024, 0.3641732283464567677 ) ) ;
#24547=CARTESIAN_POINT ( 'NONE',  ( -0.08530183727034056085, -0.3162353388693405765, 0.4822834645669290543 ) ) ;
#24548=CARTESIAN_POINT ( 'NONE',  ( 0.7480314960629927956, -0.5511811023622047445, 6.969142054262312111E-17 ) ) ;
#24549=CARTESIAN_POINT ( 'NONE',  ( -1.535433070866141225, 0.1771653543307087630, 0.000000000000000000 ) ) ;
#24550=CARTESIAN_POINT ( 'NONE',  ( 1.148293963254593875, -0.6692913385826771977, 0.1292274648535927661 ) ) ;
#24552=CARTESIAN_POINT ( 'NONE',  ( -0.4396325459317579898, 0.1771653543307087630, 0.09757992244046791164 ) ) ;
#24553=CARTESIAN_POINT ( 'NONE',  ( -0.4658792650918627265, -0.05778040916215522460, 0.4822834645669289988 ) ) ;
#24554=CARTESIAN_POINT ( 'NONE',  ( -1.640419947506561060, -0.004921259842519576551, 0.3153832671262227771 ) ) ;
#24555=CARTESIAN_POINT ( 'NONE',  ( -1.279527559055116948, -0.5400638737290844871, 0.3530559997133364547 ) ) ;
#24556=CARTESIAN_POINT ( 'NONE',  ( 1.272965879265092637, -0.4281496062992127816, -0.4176697321401328100 ) ) ;
#24558=CARTESIAN_POINT ( 'NONE',  ( -1.377952755905511140, -0.5511811023622047445, 6.969142054262312111E-17 ) ) ;
#24560=CARTESIAN_POINT ( 'NONE',  ( 1.469816272965879911, 0.2306618581243847221, -0.2411417322834647770 ) ) ;
#24562=CARTESIAN_POINT ( 'NONE',  ( -1.437007874015747477, -0.5400638737290844871, 0.3530559997133364547 ) ) ;
#24563=CARTESIAN_POINT ( 'NONE',  ( 1.633858267716535639, -0.5400638737290844871, 0.3530559997133364547 ) ) ;
#24564=CARTESIAN_POINT ( 'NONE',  ( -1.017060367454067249, -0.2845877964562161244, -0.3641732283464567121 ) ) ;
#24565=CARTESIAN_POINT ( 'NONE',  ( -0.5380577427821514602, 0.05413385826771666132, 0.4176697321401328100 ) ) ;
#24566=CARTESIAN_POINT ( 'NONE',  ( -0.07874015748031421014, -0.1870078740157479769, 0.3641732283464567677 ) ) ;
#24567=CARTESIAN_POINT ( 'NONE',  ( -1.200787401574802349, 0.07958543189024071263, -0.2665933059059888421 ) ) ;
#24568=CARTESIAN_POINT ( 'NONE',  ( 1.351706036745407458, -0.3690944881889765550, -0.3153832671262227771 ) ) ;
#24570=CARTESIAN_POINT ( 'NONE',  ( 0.8727034120734913358, -0.05778040916215522460, 0.4822834645669289988 ) ) ;
#24571=CARTESIAN_POINT ( 'NONE',  ( 1.601049868766404982, 0.2306618581243848609, 0.2411417322834645549 ) ) ;
#24572=CARTESIAN_POINT ( 'NONE',  ( 0.5249343832021005074, -0.5023911411419708095, 0.1820866141732285504 ) ) ;
#24573=CARTESIAN_POINT ( 'NONE',  ( 0.4199475065616805614, 0.2306618581243848609, 0.2411417322834645549 ) ) ;
#24574=CARTESIAN_POINT ( 'NONE',  ( 0.7808398950131240079, -0.2845877964562159024, 0.3641732283464567677 ) ) ;
#24575=VERTEX_POINT ( 'NONE', #18842 ) ;
#24576=CARTESIAN_POINT ( 'NONE',  ( 1.548556430446194954, -0.6046776061558807314, 0.2411417322834647770 ) ) ;
#24577=CARTESIAN_POINT ( 'NONE',  ( -1.187664041994749731, -0.3162353388693405765, 0.4822834645669290543 ) ) ;
#24578=CARTESIAN_POINT ( 'NONE',  ( 0.07217847769028949700, -0.05778040916215560624, -0.4822834645669293319 ) ) ;
#24579=CARTESIAN_POINT ( 'NONE',  ( 0.5387615594602676028, 2.409604939980833412E-17, -0.3464511005275205946 ) ) ;
#24581=CARTESIAN_POINT ( 'NONE',  ( 0.6233595800524939223, -0.3162353388693405765, 0.4822834645669290543 ) ) ;
#24582=CARTESIAN_POINT ( 'NONE',  ( 1.299212598425197429, 0.1771653543307087630, 0.000000000000000000 ) ) ;
#24583=CARTESIAN_POINT ( 'NONE',  ( -0.1640419947506553400, -0.05778040916215560624, -0.4822834645669293319 ) ) ;
#24584=CARTESIAN_POINT ( 'NONE',  ( 0.2427821522309716595, -0.3162353388693409650, -0.4822834645669289433 ) ) ;
#24590=CARTESIAN_POINT ( 'NONE',  ( -0.6167979002624665030, -0.004921259842519576551, 0.3153832671262227771 ) ) ;
#24591=CARTESIAN_POINT ( 'NONE',  ( -0.8858267716535425107, 0.1660481256975883668, -0.3530559997133364547 ) ) ;
#24592=CARTESIAN_POINT ( 'NONE',  ( 0.5708661417322841158, -0.5400638737290845981, -0.3530559997133363437 ) ) ;
#24594=CARTESIAN_POINT ( 'NONE',  ( 0.7545931758530189937, 0.2952755905511810774, -0.1292274648535930714 ) ) ;
#24595=CARTESIAN_POINT ( 'NONE',  ( -1.587926509186350810, 0.05413385826771626580, -0.4176697321401330321 ) ) ;
#24596=CARTESIAN_POINT ( 'NONE',  ( 0.8727034120734912248, -0.3162353388693409650, -0.4822834645669289433 ) ) ;
#24599=CARTESIAN_POINT ( 'NONE',  ( -0.7426113562971994320, 2.199547029021313715, 0.5309055118110236338 ) ) ;
#24600=CARTESIAN_POINT ( 'NONE',  ( 0.8530183727034126306, 0.05413385826771626580, -0.4176697321401330321 ) ) ;
#24601=CARTESIAN_POINT ( 'NONE',  ( 0.5249343832021003964, 0.2306618581243847221, -0.2411417322834647770 ) ) ;
#24602=CARTESIAN_POINT ( 'NONE',  ( 1.069553805774278610, -0.5511811023622046335, 0.09757992244046803654 ) ) ;
#24603=CARTESIAN_POINT ( 'NONE',  ( 1.594488188976378673, -0.5400638737290845981, -0.3530559997133363437 ) ) ;
#24606=CARTESIAN_POINT ( 'NONE',  ( 0.6233595800524942554, -0.05778040916215560624, -0.4822834645669293319 ) ) ;
#24609=CARTESIAN_POINT ( 'NONE',  ( -0.5446194225721777693, -0.3162353388693409650, -0.4822834645669289433 ) ) ;
#24610=CARTESIAN_POINT ( 'NONE',  ( -1.062992125984250968, 0.2952755905511811885, 0.000000000000000000 ) ) ;
#24611=CARTESIAN_POINT ( 'NONE',  ( 1.325459317585302665, 0.05413385826771626580, -0.4176697321401330321 ) ) ;
#24615=CARTESIAN_POINT ( 'NONE',  ( 1.555118110236221041, 0.1660481256975883668, -0.3530559997133364547 ) ) ;
#24616=VERTEX_POINT ( 'NONE', #36544 ) ;
#24620=CARTESIAN_POINT ( 'NONE',  ( 1.469816272965879911, 0.1283753931104746893, -0.1820866141732285504 ) ) ;
#24622=CARTESIAN_POINT ( 'NONE',  ( 1.476377952755906442, -0.4536011799217367080, 0.2665933059059888421 ) ) ;
#24624=CARTESIAN_POINT ( 'NONE',  ( 0.3836918680457899744, 8.471767977567108961E-16, -0.4445507791589058955 ) ) ;
#24628=CARTESIAN_POINT ( 'NONE',  ( -0.7874015748031489847, -0.1870078740157480601, -0.3641732283464567677 ) ) ;
#24629=CARTESIAN_POINT ( 'NONE',  ( -1.227034120734907585, 0.1771653543307087630, 0.09757992244046791164 ) ) ;
#24630=CARTESIAN_POINT ( 'NONE',  ( -1.397637795275589623, -0.5400638737290845981, -0.3530559997133363437 ) ) ;
#24631=CARTESIAN_POINT ( 'NONE',  ( 0.1837270341207354329, 0.2306618581243848609, 0.2411417322834645549 ) ) ;
#24632=CARTESIAN_POINT ( 'NONE',  ( 1.528871391076116026, -0.6692913385826773087, -0.1292274648535924053 ) ) ;
#24634=CARTESIAN_POINT ( 'NONE',  ( 1.456692913385827515, 0.2952755905511811885, 0.000000000000000000 ) ) ;
#24635=CARTESIAN_POINT ( 'NONE',  ( -1.614173228346457378, 0.2753471884572480932, 0.1372047244094471985 ) ) ;
#24637=FACE_OUTER_BOUND ( 'NONE', #30203, .T. ) ;
#24638=CARTESIAN_POINT ( 'NONE',  ( -0.3149606299212590610, -0.1870078740157480601, -0.3641732283464567677 ) ) ;
#24639=CARTESIAN_POINT ( 'NONE',  ( -1.338582677165353729, -0.1870078740157479769, 0.4822834645669291653 ) ) ;
#24640=CARTESIAN_POINT ( 'NONE',  ( 1.082677165354331228, 0.1660481256975883668, -0.3530559997133364547 ) ) ;
#24642=CARTESIAN_POINT ( 'NONE',  ( -1.220472440944882386, -0.1870078740157480046, 1.254653134982923898E-17 ) ) ;
#24643=CYLINDRICAL_SURFACE ( 'NONE', #27728, 0.3937007874015748254 ) ;
#24644=CARTESIAN_POINT ( 'NONE',  ( 1.561679790026247350, 0.05413385826771626580, -0.4176697321401330321 ) ) ;
#24645=CARTESIAN_POINT ( 'NONE',  ( -1.089238845144356427, 0.05413385826771666132, 0.4176697321401328100 ) ) ;
#24647=CARTESIAN_POINT ( 'NONE',  ( -0.3674540682414692561, -0.5023911411419708095, -0.1820866141732282451 ) ) ;
#24649=CARTESIAN_POINT ( 'NONE',  ( -0.5839895013123351797, -0.5511811023622046335, 0.09757992244046803654 ) ) ;
#24650=CARTESIAN_POINT ( 'NONE',  ( 0.3871391076115492380, -0.08942795157528024563, -0.3641732283464568787 ) ) ;
#24651=CARTESIAN_POINT ( 'NONE',  ( 0.6889763779527563470, 0.1660481256975883668, -0.3530559997133364547 ) ) ;
#24652=CARTESIAN_POINT ( 'NONE',  ( -0.6233595800524928121, -0.2845877964562161244, -0.3641732283464567121 ) ) ;
#24654=CARTESIAN_POINT ( 'NONE',  ( 1.364829396325459854, -0.6046776061558809534, -0.2411417322834644161 ) ) ;
#24655=CARTESIAN_POINT ( 'NONE',  ( -1.200787401574802349, -0.5400638737290844871, 0.3530559997133364547 ) ) ;
#24657=CARTESIAN_POINT ( 'NONE',  ( -0.3477690288713905509, -0.6692913385826771977, 0.1292274648535927661 ) ) ;
#24658=CARTESIAN_POINT ( 'NONE',  ( -0.5314960629921250401, 0.1660481256975885056, 0.3530559997133364547 ) ) ;
#24659=CARTESIAN_POINT ( 'NONE',  ( 1.122047244094488860, -0.4536011799217368745, -0.2665933059059886201 ) ) ;
#24660=CARTESIAN_POINT ( 'NONE',  ( 0.2230971128608929543, -0.004921259842519870586, -0.3153832671262229437 ) ) ;
#24661=CARTESIAN_POINT ( 'NONE',  ( -0.2034120734908131112, -0.6692913385826773087, -0.1292274648535924053 ) ) ;
#24662=CARTESIAN_POINT ( 'NONE',  ( -1.187664041994749731, -0.3162353388693405765, 0.4822834645669290543 ) ) ;
#24664=CARTESIAN_POINT ( 'NONE',  ( -1.013282927784338705, 2.320010949979154579E-15, 0.4281993546915509041 ) ) ;
#24666=CARTESIAN_POINT ( 'NONE',  ( -0.3149606299212590610, -0.1870078740157480879, -0.4822834645669291653 ) ) ;
#24667=CARTESIAN_POINT ( 'NONE',  ( -0.8989501312335946848, 0.2952755905511810774, -0.1292274648535930714 ) ) ;
#24670=CARTESIAN_POINT ( 'NONE',  ( 1.115485564304462551, 0.05413385826771666132, 0.4176697321401328100 ) ) ;
#24671=CARTESIAN_POINT ( 'NONE',  ( -0.5774278215223089816, 0.1283753931104746893, -0.1820866141732285504 ) ) ;
#24672=CARTESIAN_POINT ( 'NONE',  ( -0.6364829396325453192, -0.3162353388693405765, 0.4822834645669290543 ) ) ;
#24673=CARTESIAN_POINT ( 'NONE',  ( 1.299212598425197429, -0.6692913385826771977, 8.415575281601705876E-17 ) ) ;
#24674=CARTESIAN_POINT ( 'NONE',  ( 1.017060367454068803, -0.3162353388693405765, 0.4822834645669290543 ) ) ;
#24675=CARTESIAN_POINT ( 'NONE',  ( 1.509186351706037543, -0.4281496062992127816, -0.4176697321401328100 ) ) ;
#24676=CARTESIAN_POINT ( 'NONE',  ( -1.049868766404198794, 0.1283753931104746893, -0.1820866141732285504 ) ) ;
#24682=CARTESIAN_POINT ( 'NONE',  ( 1.272965879265092637, -0.3690944881889765550, -0.3153832671262227771 ) ) ;
#24683=CARTESIAN_POINT ( 'NONE',  ( 0.7152230971128614723, -0.2845877964562161244, -0.3641732283464567121 ) ) ;
#24684=CARTESIAN_POINT ( 'NONE',  ( 0.6233595800524939223, -0.3162353388693405765, 0.4822834645669290543 ) ) ;
#24685=CARTESIAN_POINT ( 'NONE',  ( 1.528871391076116026, -0.6692913385826773087, -0.1292274648535924053 ) ) ;
#24687=CARTESIAN_POINT ( 'NONE',  ( 0.9448818897637802916, -0.1870078740157480601, -0.3641732283464567677 ) ) ;
#24688=CARTESIAN_POINT ( 'NONE',  ( -0.3608923884514428360, 0.2952755905511811885, 0.1292274648535926551 ) ) ;
#24689=CARTESIAN_POINT ( 'NONE',  ( -1.108923884514435132, -0.05778040916215560624, -0.4822834645669293319 ) ) ;
#24690=CARTESIAN_POINT ( 'NONE',  ( 1.167979002624672580, -0.4281496062992124485, 0.4176697321401328655 ) ) ;
#24693=CARTESIAN_POINT ( 'NONE',  ( -0.04593175853018302557, -0.5511811023622048555, -0.09757992244046775898 ) ) ;
#24696=CARTESIAN_POINT ( 'NONE',  ( -0.8070866141732276899, -0.5400638737290844871, 0.3530559997133364547 ) ) ;
#24697=CARTESIAN_POINT ( 'NONE',  ( -0.7939632545931750718, -0.05778040916215560624, -0.4822834645669293319 ) ) ;
#24698=CARTESIAN_POINT ( 'NONE',  ( -0.1837270341207340729, 0.2306618581243847221, -0.2411417322834647770 ) ) ;
#24699=CARTESIAN_POINT ( 'NONE',  ( 0.4855643044619430415, -0.4281496062992127816, -0.4176697321401328100 ) ) ;
#24700=CARTESIAN_POINT ( 'NONE',  ( -0.3215223097112853146, -0.05778040916215560624, -0.4822834645669293319 ) ) ;
#24701=CARTESIAN_POINT ( 'NONE',  ( -1.358267716535432434, -0.5400638737290844871, 0.3530559997133364547 ) ) ;
#24702=CARTESIAN_POINT ( 'NONE',  ( -0.7939632545931754048, -0.3162353388693405765, 0.4822834645669290543 ) ) ;
#24703=CARTESIAN_POINT ( 'NONE',  ( 0.7874015748031503170, -0.1870078740157479769, 0.4822834645669291653 ) ) ;
#24704=EDGE_CURVE ( 'NONE', #20803, #19838, #57125, .T. ) ;
#24706=CARTESIAN_POINT ( 'NONE',  ( -0.4790026246719152336, -0.08942795157528024563, -0.3641732283464568787 ) ) ;
#24707=VERTEX_POINT ( 'NONE', #49995 ) ;
#24709=ORIENTED_EDGE ( 'NONE', *, *, #44487, .T. ) ;
#24710=CARTESIAN_POINT ( 'NONE',  ( -1.266404199475064773, -0.2845877964562159024, 0.3641732283464567677 ) ) ;
#24711=CARTESIAN_POINT ( 'NONE',  ( -0.8989501312335946848, -0.6692913385826771977, 0.1292274648535927661 ) ) ;
#24712=CARTESIAN_POINT ( 'NONE',  ( -0.6955380577427815458, 0.05413385826771666132, 0.4176697321401328100 ) ) ;
#24714=CARTESIAN_POINT ( 'NONE',  ( -0.9317585301837263412, 0.05413385826771666132, 0.4176697321401328100 ) ) ;
#24715=CARTESIAN_POINT ( 'NONE',  ( -0.6299212598425188991, -0.1870078740157479769, 0.4822834645669291653 ) ) ;
#24716=CARTESIAN_POINT ( 'NONE',  ( -1.627296587926508442, 0.2306618581243848609, 0.2411417322834645549 ) ) ;
#24717=CARTESIAN_POINT ( 'NONE',  ( -1.686351706036744558, 0.2952755905511810774, -0.1292274648535930714 ) ) ;
#24718=CARTESIAN_POINT ( 'NONE',  ( 0.4068241469816281097, -0.004921259842519576551, 0.3153832671262227771 ) ) ;
#24721=CARTESIAN_POINT ( 'NONE',  ( 0.09186351706036799403, -0.3690944881889765550, -0.3153832671262227771 ) ) ;
#24723=CARTESIAN_POINT ( 'NONE',  ( -0.5118110236220466680, 0.2952755905511811885, 0.000000000000000000 ) ) ;
#24724=CARTESIAN_POINT ( 'NONE',  ( 1.338582677165355062, -0.1870078740157480879, -0.4822834645669291653 ) ) ;
#24725=CARTESIAN_POINT ( 'NONE',  ( -0.1377952755905504645, -0.5400638737290845981, -0.3530559997133363437 ) ) ;
#24728=CARTESIAN_POINT ( 'NONE',  ( -0.8533690079452078692, 0.004960608223778821026, 0.3437734562760189072 ) ) ;
#24731=CARTESIAN_POINT ( 'NONE',  ( 1.122047244094488860, 0.1660481256975885056, 0.3530559997133364547 ) ) ;
#24732=CARTESIAN_POINT ( 'NONE',  ( -1.102362204724408601, -0.1870078740157479769, 0.3641732283464567677 ) ) ;
#24733=CARTESIAN_POINT ( 'NONE',  ( -1.587926509186350810, -0.4281496062992124485, 0.4176697321401328655 ) ) ;
#24735=DIRECTION ( 'NONE',  ( 0.000000000000000000, 0.000000000000000000, -1.000000000000000000 ) ) ;
#24737=CARTESIAN_POINT ( 'NONE',  ( 1.397637795275591177, 0.1660481256975883668, -0.3530559997133364547 ) ) ;
#24739=CARTESIAN_POINT ( 'NONE',  ( 0.2690288713910767848, 0.2952755905511811885, 0.1292274648535926551 ) ) ;
#24740=CARTESIAN_POINT ( 'NONE',  ( -1.279527559055116948, 0.07958543189024071263, -0.2665933059059888421 ) ) ;
#24741=CARTESIAN_POINT ( 'NONE',  ( -0.3543307086614165824, -0.6692913385826771977, 8.415575281601705876E-17 ) ) ;
#24743=CARTESIAN_POINT ( 'NONE',  ( -1.069553805774277722, 0.2952755905511811885, 0.1292274648535926551 ) ) ;
#24746=CARTESIAN_POINT ( 'NONE',  ( 1.174540682414699111, -0.08942795157528024563, -0.3641732283464568787 ) ) ;
#24747=CARTESIAN_POINT ( 'NONE',  ( -0.4133858267716528645, 0.07958543189024071263, -0.2665933059059888421 ) ) ;
#24748=CARTESIAN_POINT ( 'NONE',  ( 0.7808398950131241190, -0.08942795157528024563, -0.3641732283464568787 ) ) ;
#24749=CARTESIAN_POINT ( 'NONE',  ( -1.423884514435694859, -0.3162353388693405765, 0.4822834645669290543 ) ) ;
#24750=CARTESIAN_POINT ( 'NONE',  ( 0.6299212598425204535, -0.1870078740157480601, -0.3641732283464567677 ) ) ;
#24751=CARTESIAN_POINT ( 'NONE',  ( -0.7874015748031489847, -0.1870078740157480879, -0.4822834645669291653 ) ) ;
#24753=CARTESIAN_POINT ( 'NONE',  ( 0.09186351706036827158, -0.004921259842519576551, 0.3153832671262227771 ) ) ;
#24755=CARTESIAN_POINT ( 'NONE',  ( 0.6955380577427828781, -0.4281496062992124485, 0.4176697321401328655 ) ) ;
#24757=CARTESIAN_POINT ( 'NONE',  ( 1.581364829396326277, -0.08942795157527998196, 0.3641732283464567121 ) ) ;
#24758=CARTESIAN_POINT ( 'NONE',  ( -1.161417322834644716, -0.5400638737290845981, -0.3530559997133363437 ) ) ;
#24759=CARTESIAN_POINT ( 'NONE',  ( -0.4133858267716528645, -0.4536011799217367080, 0.2665933059059888421 ) ) ;
#24761=CARTESIAN_POINT ( 'NONE',  ( 0.06561679790026316017, -0.004921259842519870586, -0.3153832671262229437 ) ) ;
#24762=CARTESIAN_POINT ( 'NONE',  ( -1.299212598425196097, -0.6692913385826771977, 8.415575281601705876E-17 ) ) ;
#24763=CARTESIAN_POINT ( 'NONE',  ( -0.6561679790026240244, 0.2306618581243847221, -0.2411417322834647770 ) ) ;
#24766=CARTESIAN_POINT ( 'NONE',  ( 0.6299212598425204535, -0.1870078740157479769, 0.3641732283464567677 ) ) ;
#24767=CARTESIAN_POINT ( 'NONE',  ( -0.2952755905511803003, -0.5400638737290845981, -0.3530559997133363437 ) ) ;
#24768=CARTESIAN_POINT ( 'NONE',  ( -0.8661417322834640276, -0.1870078740157479769, 0.4822834645669291653 ) ) ;
#24769=CARTESIAN_POINT ( 'NONE',  ( -0.7808398950131222316, -0.2845877964562161244, -0.3641732283464567121 ) ) ;
#24771=CARTESIAN_POINT ( 'NONE',  ( -0.09842519685039295696, -0.5400638737290844871, 0.3530559997133364547 ) ) ;
#24772=CARTESIAN_POINT ( 'NONE',  ( 1.114781747626347963, 3.405574981839577511E-16, 0.3464511005275203726 ) ) ;
#24773=CARTESIAN_POINT ( 'NONE',  ( -1.646981627296586703, -0.05778040916215522460, 0.4822834645669289988 ) ) ;
#24776=CIRCLE ( 'NONE', #47626, 1.220472440944881942 ) ;
#24777=CARTESIAN_POINT ( 'NONE',  ( -1.646051170424378096, 0.000000000000000000, 0.3464511005275205946 ) ) ;
#24778=CARTESIAN_POINT ( 'NONE',  ( -1.489501312335957062, -0.3162353388693409650, -0.4822834645669289433 ) ) ;
#24779=CARTESIAN_POINT ( 'NONE',  ( -1.010498687664041384, -0.4281496062992127816, -0.4176697321401328100 ) ) ;
#24780=CARTESIAN_POINT ( 'NONE',  ( -1.463254593175852492, 0.2952755905511811885, 0.1292274648535926551 ) ) ;
#24783=CARTESIAN_POINT ( 'NONE',  ( 0.7677165354330716118, 0.1660481256975883668, -0.3530559997133364547 ) ) ;
#24784=CARTESIAN_POINT ( 'NONE',  ( 0.2230971128608932319, -0.4281496062992124485, 0.4176697321401328655 ) ) ;
#24786=CARTESIAN_POINT ( 'NONE',  ( -0.6889763779527551257, 0.1660481256975885056, 0.3530559997133364547 ) ) ;
#24787=CARTESIAN_POINT ( 'NONE',  ( 1.246719160104987623, -0.3690944881889763329, 0.3153832671262228327 ) ) ;
#24792=VERTEX_POINT ( 'NONE', #37379 ) ;
#24793=CARTESIAN_POINT ( 'NONE',  ( 0.2755905511811031494, -0.6692913385826771977, 8.415575281601705876E-17 ) ) ;
#24794=CARTESIAN_POINT ( 'NONE',  ( -0.7874015748031489847, -0.1870078740157479769, 0.4822834645669291653 ) ) ;
#24795=CARTESIAN_POINT ( 'NONE',  ( -1.515748031496062076, -0.5400638737290844871, 0.3530559997133364547 ) ) ;
#24796=CARTESIAN_POINT ( 'NONE',  ( 0.7349081364829403995, 0.2306618581243848609, 0.2411417322834645549 ) ) ;
#24797=CARTESIAN_POINT ( 'NONE',  ( 1.496062992125985147, -0.1870078740157479769, 0.4822834645669291653 ) ) ;
#24798=CARTESIAN_POINT ( 'NONE',  ( 1.561679790026247350, -0.4281496062992124485, 0.4176697321401328655 ) ) ;
#24799=CARTESIAN_POINT ( 'NONE',  ( -0.2755905511811015396, -0.6692913385826771977, 8.415575281601705876E-17 ) ) ;
#24800=CARTESIAN_POINT ( 'NONE',  ( -1.076115485564303809, -0.6046776061558809534, -0.2411417322834644161 ) ) ;
#24802=CARTESIAN_POINT ( 'NONE',  ( 1.456692913385827515, -0.6692913385826771977, 8.415575281601705876E-17 ) ) ;
#24803=( BOUNDED_SURFACE ( )  B_SPLINE_SURFACE ( 1, 2, ( 
 ( #2520, #79136, #28178, #8825, #9247, #54670, #21862, #59744, #40395, #22282, #8003, #35328, #29004, #67324, #78715, #2098, #54253, #79969, #60991, #33667, #27763, #47110, #47527, #73218, #1685, #15568, #53428, #41228, #66077, #80381, #47942, #3340, #65676, #66915, #59329, #28596, #8413, #73645, #39986, #72800, #22694, #27344, #14328, #53002, #21040, #15149, #72392, #40806, #56325, #37391, #68965, #74050, #36973, #18046, #55489, #82024, #4571, #49183, #48769, #61405, #50007, #68151, #62233, #35737, #81199, #48353, #74886, #75292, #29826, #43267, #3754, #74468, #30242, #23101, #10896, #55905, #23514, #17232, #75705, #69382, #11736, #82429, #68555, #42044, #42862, #36149, #62653, #36556, #29418, #11314, #43679, #4994, #63063, #5400, #31063, #61821, #55077, #81617, #80785, #30662, #23931, #16815, #24337, #56731, #16398, #67740, #42451, #49598, #17635, #4161, #10073, #10495, #58395, #58823, #69792, #44099, #44914, #70192, #13382, #45342, #82835, #12547, #44502, #57968, #57555, #25569, #20109, #76115, #51648, #38205, #12138, #63879, #335, #70611, #83246, #63472, #25157, #39035, #19261, #24748, #6635, #18855, #37794, #5807, #13803, #64718, #71038, #51234, #31477, #77776, #50415, #18456, #12966, #57138, #19684, #50825, #32307, #76527, #39461, #7059, #755, #32728, #25990, #45757, #6218, #76933, #65148, #31894, #38623, #26416, #52069, #77352, #71454, #7484, #64301, #33154, #20942, #34400, #15470, #65573, #66818, #47010, #47427, #28079, #7907, #27246, #46600, #73119, #40707, #72704, #52905, #60481, #65979, #53329, #46180, #72296, #59645, #66392, #8730, #14226, #15051, #8316, #2423, #78619, #41540, #2832, #54153, #78197, #60068, #20528, #53737, #14642, #9151, #52489, #33983, #79445, #71877, #79868, #33568, #67229, #40298, #21357, #59230, #34824, #73548, #21764, #26831, #41127, #22185, #2001, #28493, #47842, #27663, #1591, #39886, #15891, #79038, #9559, #35229, #1180, #60893, #4064, #29731, #36055, #17538, #49083, #43583, #28908, #54571, #11631, #10398, #80285, #74783, #3661, #56228, #41944, #17134, #81511, #43170, #42766, #68051, #10800, #23833, #36875, #67640, #81100, #24237, #61303, #61727, #29324, #36460, #68866, #48673, #55393, #35643, #3244, #42353, #11215, #80693, #9973, #55805, #81926, #62553, #62134, #68462, #49910, #49501, #23417, #30562, #4888, #75607, #54985, #17946, #4474, #30144, #75194, #23006, #69284, #22598, #48259, #16302, #73955, #74369, #16713, #44398, #25466, #31790, #57865, #20003, #51132, #82733, #63368, #70937, #56630, #650, #77673, #32622, #44000, #25052, #19577, #45237, #26307, #77248, #64614, #38520, #76014, #71349, #13282, #76826, #70090, #19159, #57453, #232, #45654, #44809, #50727, #5702, #38934, #82331, #51965, #37291, #58284, #69693, #76426, #6952, #62966, #5304, #24649, #18754, #12444, #70505, #12863, #50317, #64203, #38103, #6537, #31374, #30963, #18356, #12036, #37693, #32207, #57039, #25883, #63779, #6118, #83146, #51544, #53219, #58710, #66711, #78091, #54048, #39773, #33878, #46075, #21662, #2727, #34299, #39352, #2316, #9044, #20838, #47322, #78929, #14543, #14121, #26728, #15364, #33467, #27560, #1075, #46490, #13696, #40195, #65878, #72185, #53634, #1899, #79762, #65036, #7372, #47738, #8213, #33041, #21251, #65468, #34719, #20422, #46906, #59960, #79342, #72601, #59544, #14947, #27976, #73013, #71768, #40606, #60379, #7802, #66289, #59129, #8628, #41025, #1486, #28388, #27140, #52382, #78514, #22079, #52804, #80182, #68369, #68770, #30043, #23317, #55294, #62447, #62038, #35959, #43073, #17443, #81413, #73855, #55705, #48986, #29633, #81003, #48160, #28805, #74685, #48570, #29223, #17031, #4783, #23730, #24139, #35123, #9452, #10292, #35539, #4375, #10707, #16196, #61201, #9870, #42670, #22903, #74268, #11114, #41438, #36363, #3558, #60789, #54890, #49401, #61628, #16611, #54469, #41842, #75095, #67949, #73436, #36771, #67532, #3142, #22497, #30459, #56123, #81829, #42254, #80595, #15786, #67122, #3970, #12350, #37187, #44713, #30867, #31693, #18255, #64518, #12766, #25787, #64105, #57352, #70841, #24554, #24952, #38839 ),
 ( #56532, #70410, #45137, #6440, #83048, #25371, #6855, #38423, #38006, #19484, #77152, #57770, #50220, #32112, #51034, #6022, #76733, #75916, #132, #13190, #19065, #5203, #557, #51449, #63684, #56942, #32525, #44304, #58188, #49809, #75510, #11940, #43897, #17849, #69179, #43483, #11530, #62866, #82235, #37595, #69594, #63268, #5609, #31277, #82639, #50625, #76330, #18660, #69995, #15582, #8839, #28608, #21466, #34515, #79562, #28191, #54266, #60180, #22294, #64938, #53441, #41240, #2112, #73231, #66928, #2533, #53849, #29018, #48365, #74064, #61417, #47541, #19910, #21876, #15163, #16000, #9260, #7278, #47955, #22707, #41647, #16410, #42056, #67752, #40820, #13602, #34932, #34094, #9671, #60595, #27777, #73658, #10086, #61004, #26210, #59757, #79981, #2944, #66505, #67338, #35751, #3353, #51872, #71256, #45560, #35341, #72814, #54684, #80395, #79149, #77578, #47124, #39256, #36565, #4580, #82437, #55089, #30673, #23524, #74480, #49194, #36984, #49606, #62242, #42463, #4173, #75714, #81628, #3767, #68974, #81209, #48782, #16827, #76123, #18055, #50016, #30251, #68163, #56740, #29431, #80798, #75301, #10506, #82033, #36159, #11324, #55500, #18465, #43688, #63073, #69393, #62663, #24755, #61833, #55915, #44108, #29837, #10907, #11745, #37401, #56334, #24347, #5410, #74895, #23939, #17243, #5003, #31072, #42872, #50423, #17645, #69800, #12147, #68565, #43277, #37804, #23115, #19695, #26001, #6229, #39472, #57147, #14237, #12977, #82846, #51659, #31904, #58833, #44513, #77363, #765, #45767, #45352, #70621, #13393, #26427, #65159, #70201, #345, #26840, #63890, #38633, #57565, #39046, #71466, #51243, #64311, #38215, #63482, #44924, #13814, #83257, #12556, #58406, #1191, #20120, #64731, #71049, #52499, #52079, #7069, #33165, #7496, #78208, #25579, #20540, #32738, #77787, #46191, #76945, #71887, #5815, #31486, #18864, #25167, #50836, #76536, #6645, #19271, #57980, #32318, #22608, #28091, #2012, #65990, #73557, #59241, #3254, #80294, #35239, #46611, #27676, #22195, #47853, #28916, #1600, #53341, #15062, #21775, #15901, #20954, #27256, #41550, #39896, #78630, #41138, #40718, #79050, #79458, #54584, #67238, #73966, #52915, #72307, #60080, #21368, #28506, #60492, #14654, #47023, #59656, #73130, #72715, #66403, #60903, #7917, #66828, #8741, #40311, #34412, #15481, #2434, #53748, #8328, #33994, #54163, #47437, #65584, #9161, #34833, #2842, #79877, #48268, #9568, #33578, #74796, #54994, #69294, #50326, #49919, #30153, #23427, #4485, #10809, #36885, #82340, #55815, #61736, #42364, #75617, #35652, #62975, #56639, #11643, #23016, #4073, #81935, #24246, #5314, #61315, #29740, #17143, #37301, #48683, #67649, #36064, #81110, #17547, #10407, #24658, #17955, #30972, #9985, #81523, #3670, #23843, #68063, #43592, #29333, #49092, #49510, #80702, #16311, #74379, #41955, #55404, #36469, #16722, #42775, #68471, #62562, #62144, #4901, #75203, #43179, #68876, #11225, #30572, #56238, #5713, #77683, #12453, #6546, #63377, #25475, #76024, #19170, #44818, #51142, #32633, #64212, #58723, #44009, #69703, #26738, #76836, #12046, #32217, #18764, #71360, #57048, #57875, #13291, #58296, #242, #83156, #25894, #38943, #51978, #82742, #12872, #39362, #76435, #70515, #44407, #51554, #661, #63788, #38531, #50737, #18369, #57462, #26317, #38114, #25063, #70946, #13708, #20013, #77257, #19587, #65047, #64626, #45249, #45664, #7384, #33052, #70101, #1086, #6962, #37704, #31383, #6127, #31802, #79773, #53646, #7812, #9462, #65889, #39785, #59971, #33478, #34730, #2330, #60390, #59140, #65480, #2740, #52392, #1498, #79354, #27571, #8224, #8638, #41449, #28400, #3152, #14132, #71778, #72611, #14554, #41035, #73024, #27150, #40206, #72201, #27986, #1909, #53229, #47749, #20432, #21673, #33888, #52814, #59554, #47334, #14959, #78945, #78525, #20848, #66721, #46918, #78101, #34309, #46501, #21263, #40616, #67133, #9058, #15374, #66299, #54058, #22089, #46086, #73448, #15798, #35136, #60798, #9880, #10718, #80604, #43495, #75108, #4794, #43084, #36375, #49821, #3567, #3980, #17860, #35549, #35969 ) ),
 .UNSPECIFIED., .F., .F., .F. ) 
 B_SPLINE_SURFACE_WITH_KNOTS ( ( 2, 2 ),
 ( 3, 2, 2, 2, 2, 2, 2, 2, 2, 2, 2, 2, 2, 2, 2, 2, 2, 2, 2, 2, 2, 2, 2, 2, 2, 2, 2, 2, 2, 2, 2, 2, 2, 2, 2, 2, 2, 2, 2, 2, 2, 2, 2, 2, 2, 2, 2, 2, 2, 2, 2, 2, 2, 2, 2, 2, 2, 2, 2, 2, 2, 2, 2, 2, 2, 2, 2, 2, 2, 2, 2, 2, 2, 2, 2, 2, 2, 2, 2, 2, 2, 2, 2, 2, 2, 2, 2, 2, 2, 2, 2, 2, 2, 2, 2, 2, 2, 2, 2, 2, 2, 2, 2, 2, 2, 2, 2, 2, 2, 2, 2, 2, 2, 2, 2, 2, 2, 2, 2, 2, 2, 2, 2, 2, 2, 2, 2, 2, 2, 2, 2, 2, 2, 2, 2, 2, 2, 2, 2, 2, 2, 2, 2, 2, 2, 2, 2, 2, 2, 2, 2, 2, 2, 2, 2, 2, 2, 2, 2, 2, 2, 2, 2, 2, 2, 2, 2, 2, 2, 2, 2, 2, 2, 2, 2, 2, 2, 2, 2, 2, 2, 2, 2, 2, 2, 2, 2, 2, 2, 2, 2, 2, 2, 2, 2, 2, 2, 2, 2, 2, 2, 2, 2, 2, 2, 2, 2, 2, 2, 2, 2, 2, 2, 2, 2, 2, 2, 2, 2, 2, 2, 2, 2, 2, 2, 2, 2, 2, 2, 2, 2, 2, 2, 2, 2, 2, 2, 2, 2, 2, 2, 2, 2, 2, 2, 2, 2, 2, 2, 2, 2, 2, 2, 2, 2, 3 ),
 ( 0.000000000000000000, 1.000000000000000000 ),
 ( 0.000000000000000000, 0.003787878787878787984, 0.007575757575757575968, 0.01136363636363636395, 0.01515151515151515194, 0.01893939393939393992, 0.02272727272727272790, 0.02651515151515151589, 0.03030303030303030387, 0.03409090909090908839, 0.03787878787878787984, 0.04166666666666666435, 0.04545454545454545581, 0.04924242424242424032, 0.05303030303030303177, 0.05681818181818181629, 0.06060606060606060774, 0.06439393939393939226, 0.06818181818181817677, 0.07196969696969697516, 0.07575757575757575968, 0.07954545454545454419, 0.08333333333333332871, 0.08712121212121212710, 0.09090909090909091161, 0.09469696969696969613, 0.09848484848484848064, 0.1022727272727272790, 0.1060606060606060635, 0.1098484848484848481, 0.1136363636363636326, 0.1174242424242424310, 0.1212121212121212155, 0.1250000000000000000, 0.1287878787878787845, 0.1325757575757575690, 0.1363636363636363535, 0.1401515151515151381, 0.1439393939393939503, 0.1477272727272727348, 0.1515151515151515194, 0.1553030303030303039, 0.1590909090909090884, 0.1628787878787878729, 0.1666666666666666574, 0.1704545454545454419, 0.1742424242424242542, 0.1780303030303030387, 0.1818181818181818232, 0.1856060606060606077, 0.1893939393939393923, 0.1931818181818181768, 0.1969696969696969613, 0.2007575757575757458, 0.2045454545454545581, 0.2083333333333333426, 0.2121212121212121271, 0.2159090909090909116, 0.2196969696969696961, 0.2234848484848484806, 0.2272727272727272652, 0.2310606060606060497, 0.2348484848484848619, 0.2386363636363636465, 0.2424242424242424310, 0.2462121212121212155, 0.2500000000000000000, 0.2537878787878787845, 0.2575757575757575690, 0.2613636363636363535, 0.2651515151515151381, 0.2689393939393939226, 0.2727272727272727071, 0.2765151515151514916, 0.2803030303030302761, 0.2840909090909091161, 0.2878787878787879007, 0.2916666666666666852, 0.2954545454545454697, 0.2992424242424242542, 0.3030303030303030387, 0.3068181818181818232, 0.3106060606060606077, 0.3143939393939393923, 0.3181818181818181768, 0.3219696969696969613, 0.3257575757575757458, 0.3295454545454545303, 0.3333333333333333148, 0.3371212121212120993, 0.3409090909090908839, 0.3446969696969697239, 0.3484848484848485084, 0.3522727272727272929, 0.3560606060606060774, 0.3598484848484848619, 0.3636363636363636465, 0.3674242424242424310, 0.3712121212121212155, 0.3750000000000000000, 0.3787878787878787845, 0.3825757575757575690, 0.3863636363636363535, 0.3901515151515151381, 0.3939393939393939226, 0.3977272727272727071, 0.4015151515151514916, 0.4053030303030302761, 0.4090909090909091161, 0.4128787878787879007, 0.4166666666666666852, 0.4204545454545454697, 0.4242424242424242542, 0.4280303030303030387, 0.4318181818181818232, 0.4356060606060606077, 0.4393939393939393923, 0.4431818181818181768, 0.4469696969696969613, 0.4507575757575757458, 0.4545454545454545303, 0.4583333333333333148, 0.4621212121212120993, 0.4659090909090908839, 0.4696969696969697239, 0.4734848484848485084, 0.4772727272727272929, 0.4810606060606060774, 0.4848484848484848619, 0.4886363636363636465, 0.4924242424242424310, 0.4962121212121212155, 0.5000000000000000000, 0.5037878787878787845, 0.5075757575757575690, 0.5113636363636363535, 0.5151515151515151381, 0.5189393939393939226, 0.5227272727272727071, 0.5265151515151514916, 0.5303030303030302761, 0.5340909090909090606, 0.5378787878787878451, 0.5416666666666666297, 0.5454545454545454142, 0.5492424242424241987, 0.5530303030303029832, 0.5568181818181817677, 0.5606060606060605522, 0.5643939393939394478, 0.5681818181818182323, 0.5719696969696970168, 0.5757575757575758013, 0.5795454545454545858, 0.5833333333333333703, 0.5871212121212121549, 0.5909090909090909394, 0.5946969696969697239, 0.5984848484848485084, 0.6022727272727272929, 0.6060606060606060774, 0.6098484848484848619, 0.6136363636363636465, 0.6174242424242424310, 0.6212121212121212155, 0.6250000000000000000, 0.6287878787878787845, 0.6325757575757575690, 0.6363636363636363535, 0.6401515151515151381, 0.6439393939393939226, 0.6477272727272727071, 0.6515151515151514916, 0.6553030303030302761, 0.6590909090909090606, 0.6628787878787878451, 0.6666666666666666297, 0.6704545454545454142, 0.6742424242424241987, 0.6780303030303029832, 0.6818181818181817677, 0.6856060606060605522, 0.6893939393939394478, 0.6931818181818182323, 0.6969696969696970168, 0.7007575757575758013, 0.7045454545454545858, 0.7083333333333333703, 0.7121212121212121549, 0.7159090909090909394, 0.7196969696969697239, 0.7234848484848485084, 0.7272727272727272929, 0.7310606060606060774, 0.7348484848484848619, 0.7386363636363636465, 0.7424242424242424310, 0.7462121212121212155, 0.7500000000000000000, 0.7537878787878787845, 0.7575757575757575690, 0.7613636363636363535, 0.7651515151515151381, 0.7689393939393939226, 0.7727272727272727071, 0.7765151515151514916, 0.7803030303030302761, 0.7840909090909090606, 0.7878787878787878451, 0.7916666666666666297, 0.7954545454545454142, 0.7992424242424241987, 0.8030303030303029832, 0.8068181818181817677, 0.8106060606060605522, 0.8143939393939394478, 0.8181818181818182323, 0.8219696969696970168, 0.8257575757575758013, 0.8295454545454545858, 0.8333333333333333703, 0.8371212121212121549, 0.8409090909090909394, 0.8446969696969697239, 0.8484848484848485084, 0.8522727272727272929, 0.8560606060606060774, 0.8598484848484848619, 0.8636363636363636465, 0.8674242424242424310, 0.8712121212121212155, 0.8750000000000000000, 0.8787878787878787845, 0.8825757575757575690, 0.8863636363636363535, 0.8901515151515151381, 0.8939393939393939226, 0.8977272727272727071, 0.9015151515151514916, 0.9053030303030302761, 0.9090909090909090606, 0.9128787878787878451, 0.9166666666666666297, 0.9204545454545454142, 0.9242424242424241987, 0.9280303030303029832, 0.9318181818181817677, 0.9356060606060605522, 0.9393939393939394478, 0.9431818181818182323, 0.9469696969696970168, 0.9507575757575758013, 0.9545454545454545858, 0.9583333333333333703, 0.9621212121212121549, 0.9659090909090909394 ),
 .UNSPECIFIED. ) 
 GEOMETRIC_REPRESENTATION_ITEM ( )  RATIONAL_B_SPLINE_SURFACE ( (
 ( 1.000000000000000000, 0.9659258262890683122, 1.000000000000000000, 0.9659258262890683122, 1.000000000000000000, 0.9659258262890683122, 1.000000000000000000, 0.9659258262890683122, 1.000000000000000000, 0.9659258262890683122, 1.000000000000000000, 0.9659258262890683122, 1.000000000000000000, 0.9659258262890683122, 1.000000000000000000, 0.9659258262890683122, 1.000000000000000000, 0.9659258262890683122, 1.000000000000000000, 0.9659258262890683122, 1.000000000000000000, 0.9659258262890683122, 1.000000000000000000, 0.9659258262890683122, 1.000000000000000000, 0.9659258262890683122, 1.000000000000000000, 0.9659258262890683122, 1.000000000000000000, 0.9659258262890683122, 1.000000000000000000, 0.9659258262890683122, 1.000000000000000000, 0.9659258262890683122, 1.000000000000000000, 0.9659258262890683122, 1.000000000000000000, 0.9659258262890683122, 1.000000000000000000, 0.9659258262890683122, 1.000000000000000000, 0.9659258262890683122, 1.000000000000000000, 0.9659258262890683122, 1.000000000000000000, 0.9659258262890683122, 1.000000000000000000, 0.9659258262890683122, 1.000000000000000000, 0.9659258262890683122, 1.000000000000000000, 0.9659258262890683122, 1.000000000000000000, 0.9659258262890683122, 1.000000000000000000, 0.9659258262890683122, 1.000000000000000000, 0.9659258262890683122, 1.000000000000000000, 0.9659258262890683122, 1.000000000000000000, 0.9659258262890683122, 1.000000000000000000, 0.9659258262890683122, 1.000000000000000000, 0.9659258262890683122, 1.000000000000000000, 0.9659258262890683122, 1.000000000000000000, 0.9659258262890683122, 1.000000000000000000, 0.9659258262890683122, 1.000000000000000000, 0.9659258262890683122, 1.000000000000000000, 0.9659258262890683122, 1.000000000000000000, 0.9659258262890683122, 1.000000000000000000, 0.9659258262890683122, 1.000000000000000000, 0.9659258262890683122, 1.000000000000000000, 0.9659258262890683122, 1.000000000000000000, 0.9659258262890683122, 1.000000000000000000, 0.9659258262890683122, 1.000000000000000000, 0.9659258262890683122, 1.000000000000000000, 0.9659258262890683122, 1.000000000000000000, 0.9659258262890683122, 1.000000000000000000, 0.9659258262890683122, 1.000000000000000000, 0.9659258262890683122, 1.000000000000000000, 0.9659258262890683122, 1.000000000000000000, 0.9659258262890683122, 1.000000000000000000, 0.9659258262890683122, 1.000000000000000000, 0.9659258262890683122, 1.000000000000000000, 0.9659258262890683122, 1.000000000000000000, 0.9659258262890683122, 1.000000000000000000, 0.9659258262890683122, 1.000000000000000000, 0.9659258262890683122, 1.000000000000000000, 0.9659258262890683122, 1.000000000000000000, 0.9659258262890683122, 1.000000000000000000, 0.9659258262890683122, 1.000000000000000000, 0.9659258262890683122, 1.000000000000000000, 0.9659258262890683122, 1.000000000000000000, 0.9659258262890683122, 1.000000000000000000, 0.9659258262890683122, 1.000000000000000000, 0.9659258262890683122, 1.000000000000000000, 0.9659258262890683122, 1.000000000000000000, 0.9659258262890683122, 1.000000000000000000, 0.9659258262890683122, 1.000000000000000000, 0.9659258262890683122, 1.000000000000000000, 0.9659258262890683122, 1.000000000000000000, 0.9659258262890683122, 1.000000000000000000, 0.9659258262890683122, 1.000000000000000000, 0.9659258262890683122, 1.000000000000000000, 0.9659258262890683122, 1.000000000000000000, 0.9659258262890683122, 1.000000000000000000, 0.9659258262890683122, 1.000000000000000000, 0.9659258262890683122, 1.000000000000000000, 0.9659258262890683122, 1.000000000000000000, 0.9659258262890683122, 1.000000000000000000, 0.9659258262890683122, 1.000000000000000000, 0.9659258262890683122, 1.000000000000000000, 0.9659258262890683122, 1.000000000000000000, 0.9659258262890683122, 1.000000000000000000, 0.9659258262890683122, 1.000000000000000000, 0.9659258262890683122, 1.000000000000000000, 0.9659258262890683122, 1.000000000000000000, 0.9659258262890683122, 1.000000000000000000, 0.9659258262890683122, 1.000000000000000000, 0.9659258262890683122, 1.000000000000000000, 0.9659258262890683122, 1.000000000000000000, 0.9659258262890683122, 1.000000000000000000, 0.9659258262890683122, 1.000000000000000000, 0.9659258262890683122, 1.000000000000000000, 0.9659258262890683122, 1.000000000000000000, 0.9659258262890683122, 1.000000000000000000, 0.9659258262890683122, 1.000000000000000000, 0.9659258262890683122, 1.000000000000000000, 0.9659258262890683122, 1.000000000000000000, 0.9659258262890683122, 1.000000000000000000, 0.9659258262890683122, 1.000000000000000000, 0.9659258262890683122, 1.000000000000000000, 0.9659258262890683122, 1.000000000000000000, 0.9659258262890683122, 1.000000000000000000, 0.9659258262890683122, 1.000000000000000000, 0.9659258262890683122, 1.000000000000000000, 0.9659258262890683122, 1.000000000000000000, 0.9659258262890683122, 1.000000000000000000, 0.9659258262890683122, 1.000000000000000000, 0.9659258262890683122, 1.000000000000000000, 0.9659258262890683122, 1.000000000000000000, 0.9659258262890683122, 1.000000000000000000, 0.9659258262890683122, 1.000000000000000000, 0.9659258262890683122, 1.000000000000000000, 0.9659258262890683122, 1.000000000000000000, 0.9659258262890683122, 1.000000000000000000, 0.9659258262890683122, 1.000000000000000000, 0.9659258262890683122, 1.000000000000000000, 0.9659258262890683122, 1.000000000000000000, 0.9659258262890683122, 1.000000000000000000, 0.9659258262890683122, 1.000000000000000000, 0.9659258262890683122, 1.000000000000000000, 0.9659258262890683122, 1.000000000000000000, 0.9659258262890683122, 1.000000000000000000, 0.9659258262890683122, 1.000000000000000000, 0.9659258262890683122, 1.000000000000000000, 0.9659258262890683122, 1.000000000000000000, 0.9659258262890683122, 1.000000000000000000, 0.9659258262890683122, 1.000000000000000000, 0.9659258262890683122, 1.000000000000000000, 0.9659258262890683122, 1.000000000000000000, 0.9659258262890683122, 1.000000000000000000, 0.9659258262890683122, 1.000000000000000000, 0.9659258262890683122, 1.000000000000000000, 0.9659258262890683122, 1.000000000000000000, 0.9659258262890683122, 1.000000000000000000, 0.9659258262890683122, 1.000000000000000000, 0.9659258262890683122, 1.000000000000000000, 0.9659258262890683122, 1.000000000000000000, 0.9659258262890683122, 1.000000000000000000, 0.9659258262890683122, 1.000000000000000000, 0.9659258262890683122, 1.000000000000000000, 0.9659258262890683122, 1.000000000000000000, 0.9659258262890683122, 1.000000000000000000, 0.9659258262890683122, 1.000000000000000000, 0.9659258262890683122, 1.000000000000000000, 0.9659258262890683122, 1.000000000000000000, 0.9659258262890683122, 1.000000000000000000, 0.9659258262890683122, 1.000000000000000000, 0.9659258262890683122, 1.000000000000000000, 0.9659258262890683122, 1.000000000000000000, 0.9659258262890683122, 1.000000000000000000, 0.9659258262890683122, 1.000000000000000000, 0.9659258262890683122, 1.000000000000000000, 0.9659258262890683122, 1.000000000000000000, 0.9659258262890683122, 1.000000000000000000, 0.9659258262890683122, 1.000000000000000000, 0.9659258262890683122, 1.000000000000000000, 0.9659258262890683122, 1.000000000000000000, 0.9659258262890683122, 1.000000000000000000, 0.9659258262890683122, 1.000000000000000000, 0.9659258262890683122, 1.000000000000000000, 0.9659258262890683122, 1.000000000000000000, 0.9659258262890683122, 1.000000000000000000, 0.9659258262890683122, 1.000000000000000000, 0.9659258262890683122, 1.000000000000000000, 0.9659258262890683122, 1.000000000000000000, 0.9659258262890683122, 1.000000000000000000, 0.9659258262890683122, 1.000000000000000000, 0.9659258262890683122, 1.000000000000000000, 0.9659258262890683122, 1.000000000000000000, 0.9659258262890683122, 1.000000000000000000, 0.9659258262890683122, 1.000000000000000000, 0.9659258262890683122, 1.000000000000000000, 0.9659258262890683122, 1.000000000000000000, 0.9659258262890683122, 1.000000000000000000, 0.9659258262890683122, 1.000000000000000000, 0.9659258262890683122, 1.000000000000000000, 0.9659258262890683122, 1.000000000000000000, 0.9659258262890683122, 1.000000000000000000, 0.9659258262890683122, 1.000000000000000000, 0.9659258262890683122, 1.000000000000000000, 0.9659258262890683122, 1.000000000000000000, 0.9659258262890683122, 1.000000000000000000, 0.9659258262890683122, 1.000000000000000000, 0.9659258262890683122, 1.000000000000000000, 0.9659258262890683122, 1.000000000000000000, 0.9659258262890683122, 1.000000000000000000, 0.9659258262890683122, 1.000000000000000000, 0.9659258262890683122, 1.000000000000000000, 0.9659258262890683122, 1.000000000000000000, 0.9659258262890683122, 1.000000000000000000, 0.9659258262890683122, 1.000000000000000000, 0.9659258262890683122, 1.000000000000000000, 0.9659258262890683122, 1.000000000000000000, 0.9659258262890683122, 1.000000000000000000, 0.9659258262890683122, 1.000000000000000000, 0.9659258262890683122, 1.000000000000000000, 0.9659258262890683122, 1.000000000000000000, 0.9659258262890683122, 1.000000000000000000, 0.9659258262890683122, 1.000000000000000000, 0.9659258262890683122, 1.000000000000000000, 0.9659258262890683122, 1.000000000000000000, 0.9659258262890683122, 1.000000000000000000, 0.9659258262890683122, 1.000000000000000000, 0.9659258262890683122, 1.000000000000000000, 0.9659258262890683122, 1.000000000000000000, 0.9659258262890683122, 1.000000000000000000, 0.9659258262890683122, 1.000000000000000000, 0.9659258262890683122, 1.000000000000000000, 0.9659258262890683122, 1.000000000000000000, 0.9659258262890683122, 1.000000000000000000, 0.9659258262890683122, 1.000000000000000000, 0.9659258262890683122, 1.000000000000000000, 0.9659258262890683122, 1.000000000000000000, 0.9659258262890683122, 1.000000000000000000, 0.9659258262890683122, 1.000000000000000000, 0.9659258262890683122, 1.000000000000000000, 0.9659258262890683122, 1.000000000000000000, 0.9659258262890683122, 1.000000000000000000, 0.9659258262890683122, 1.000000000000000000, 0.9659258262890683122, 1.000000000000000000, 0.9659258262890683122, 1.000000000000000000, 0.9659258262890683122, 1.000000000000000000, 0.9659258262890683122, 1.000000000000000000, 0.9659258262890683122, 1.000000000000000000, 0.9659258262890683122, 1.000000000000000000, 0.9659258262890683122, 1.000000000000000000, 0.9659258262890683122, 1.000000000000000000, 0.9659258262890683122, 1.000000000000000000, 0.9659258262890683122, 1.000000000000000000, 0.9659258262890683122, 1.000000000000000000, 0.9659258262890683122, 1.000000000000000000, 0.9659258262890683122, 1.000000000000000000, 0.9659258262890683122, 1.000000000000000000, 0.9659258262890683122, 1.000000000000000000, 0.9659258262890683122, 1.000000000000000000, 0.9659258262890683122, 1.000000000000000000, 0.9659258262890683122, 1.000000000000000000, 0.9659258262890683122, 1.000000000000000000, 0.9659258262890683122, 1.000000000000000000, 0.9659258262890683122, 1.000000000000000000, 0.9659258262890683122, 1.000000000000000000, 0.9659258262890683122, 1.000000000000000000, 0.9659258262890683122, 1.000000000000000000, 0.9659258262890683122, 1.000000000000000000, 0.9659258262890683122, 1.000000000000000000, 0.9659258262890683122, 1.000000000000000000, 0.9659258262890683122, 1.000000000000000000, 0.9659258262890683122, 1.000000000000000000, 0.9659258262890683122, 1.000000000000000000, 0.9659258262890683122, 1.000000000000000000, 0.9659258262890683122, 1.000000000000000000, 0.9659258262890683122, 1.000000000000000000, 0.9659258262890683122, 1.000000000000000000, 0.9659258262890683122, 1.000000000000000000),
 ( 1.000000000000000000, 0.9659258262890683122, 1.000000000000000000, 0.9659258262890683122, 1.000000000000000000, 0.9659258262890683122, 1.000000000000000000, 0.9659258262890683122, 1.000000000000000000, 0.9659258262890683122, 1.000000000000000000, 0.9659258262890683122, 1.000000000000000000, 0.9659258262890683122, 1.000000000000000000, 0.9659258262890683122, 1.000000000000000000, 0.9659258262890683122, 1.000000000000000000, 0.9659258262890683122, 1.000000000000000000, 0.9659258262890683122, 1.000000000000000000, 0.9659258262890683122, 1.000000000000000000, 0.9659258262890683122, 1.000000000000000000, 0.9659258262890683122, 1.000000000000000000, 0.9659258262890683122, 1.000000000000000000, 0.9659258262890683122, 1.000000000000000000, 0.9659258262890683122, 1.000000000000000000, 0.9659258262890683122, 1.000000000000000000, 0.9659258262890683122, 1.000000000000000000, 0.9659258262890683122, 1.000000000000000000, 0.9659258262890683122, 1.000000000000000000, 0.9659258262890683122, 1.000000000000000000, 0.9659258262890683122, 1.000000000000000000, 0.9659258262890683122, 1.000000000000000000, 0.9659258262890683122, 1.000000000000000000, 0.9659258262890683122, 1.000000000000000000, 0.9659258262890683122, 1.000000000000000000, 0.9659258262890683122, 1.000000000000000000, 0.9659258262890683122, 1.000000000000000000, 0.9659258262890683122, 1.000000000000000000, 0.9659258262890683122, 1.000000000000000000, 0.9659258262890683122, 1.000000000000000000, 0.9659258262890683122, 1.000000000000000000, 0.9659258262890683122, 1.000000000000000000, 0.9659258262890683122, 1.000000000000000000, 0.9659258262890683122, 1.000000000000000000, 0.9659258262890683122, 1.000000000000000000, 0.9659258262890683122, 1.000000000000000000, 0.9659258262890683122, 1.000000000000000000, 0.9659258262890683122, 1.000000000000000000, 0.9659258262890683122, 1.000000000000000000, 0.9659258262890683122, 1.000000000000000000, 0.9659258262890683122, 1.000000000000000000, 0.9659258262890683122, 1.000000000000000000, 0.9659258262890683122, 1.000000000000000000, 0.9659258262890683122, 1.000000000000000000, 0.9659258262890683122, 1.000000000000000000, 0.9659258262890683122, 1.000000000000000000, 0.9659258262890683122, 1.000000000000000000, 0.9659258262890683122, 1.000000000000000000, 0.9659258262890683122, 1.000000000000000000, 0.9659258262890683122, 1.000000000000000000, 0.9659258262890683122, 1.000000000000000000, 0.9659258262890683122, 1.000000000000000000, 0.9659258262890683122, 1.000000000000000000, 0.9659258262890683122, 1.000000000000000000, 0.9659258262890683122, 1.000000000000000000, 0.9659258262890683122, 1.000000000000000000, 0.9659258262890683122, 1.000000000000000000, 0.9659258262890683122, 1.000000000000000000, 0.9659258262890683122, 1.000000000000000000, 0.9659258262890683122, 1.000000000000000000, 0.9659258262890683122, 1.000000000000000000, 0.9659258262890683122, 1.000000000000000000, 0.9659258262890683122, 1.000000000000000000, 0.9659258262890683122, 1.000000000000000000, 0.9659258262890683122, 1.000000000000000000, 0.9659258262890683122, 1.000000000000000000, 0.9659258262890683122, 1.000000000000000000, 0.9659258262890683122, 1.000000000000000000, 0.9659258262890683122, 1.000000000000000000, 0.9659258262890683122, 1.000000000000000000, 0.9659258262890683122, 1.000000000000000000, 0.9659258262890683122, 1.000000000000000000, 0.9659258262890683122, 1.000000000000000000, 0.9659258262890683122, 1.000000000000000000, 0.9659258262890683122, 1.000000000000000000, 0.9659258262890683122, 1.000000000000000000, 0.9659258262890683122, 1.000000000000000000, 0.9659258262890683122, 1.000000000000000000, 0.9659258262890683122, 1.000000000000000000, 0.9659258262890683122, 1.000000000000000000, 0.9659258262890683122, 1.000000000000000000, 0.9659258262890683122, 1.000000000000000000, 0.9659258262890683122, 1.000000000000000000, 0.9659258262890683122, 1.000000000000000000, 0.9659258262890683122, 1.000000000000000000, 0.9659258262890683122, 1.000000000000000000, 0.9659258262890683122, 1.000000000000000000, 0.9659258262890683122, 1.000000000000000000, 0.9659258262890683122, 1.000000000000000000, 0.9659258262890683122, 1.000000000000000000, 0.9659258262890683122, 1.000000000000000000, 0.9659258262890683122, 1.000000000000000000, 0.9659258262890683122, 1.000000000000000000, 0.9659258262890683122, 1.000000000000000000, 0.9659258262890683122, 1.000000000000000000, 0.9659258262890683122, 1.000000000000000000, 0.9659258262890683122, 1.000000000000000000, 0.9659258262890683122, 1.000000000000000000, 0.9659258262890683122, 1.000000000000000000, 0.9659258262890683122, 1.000000000000000000, 0.9659258262890683122, 1.000000000000000000, 0.9659258262890683122, 1.000000000000000000, 0.9659258262890683122, 1.000000000000000000, 0.9659258262890683122, 1.000000000000000000, 0.9659258262890683122, 1.000000000000000000, 0.9659258262890683122, 1.000000000000000000, 0.9659258262890683122, 1.000000000000000000, 0.9659258262890683122, 1.000000000000000000, 0.9659258262890683122, 1.000000000000000000, 0.9659258262890683122, 1.000000000000000000, 0.9659258262890683122, 1.000000000000000000, 0.9659258262890683122, 1.000000000000000000, 0.9659258262890683122, 1.000000000000000000, 0.9659258262890683122, 1.000000000000000000, 0.9659258262890683122, 1.000000000000000000, 0.9659258262890683122, 1.000000000000000000, 0.9659258262890683122, 1.000000000000000000, 0.9659258262890683122, 1.000000000000000000, 0.9659258262890683122, 1.000000000000000000, 0.9659258262890683122, 1.000000000000000000, 0.9659258262890683122, 1.000000000000000000, 0.9659258262890683122, 1.000000000000000000, 0.9659258262890683122, 1.000000000000000000, 0.9659258262890683122, 1.000000000000000000, 0.9659258262890683122, 1.000000000000000000, 0.9659258262890683122, 1.000000000000000000, 0.9659258262890683122, 1.000000000000000000, 0.9659258262890683122, 1.000000000000000000, 0.9659258262890683122, 1.000000000000000000, 0.9659258262890683122, 1.000000000000000000, 0.9659258262890683122, 1.000000000000000000, 0.9659258262890683122, 1.000000000000000000, 0.9659258262890683122, 1.000000000000000000, 0.9659258262890683122, 1.000000000000000000, 0.9659258262890683122, 1.000000000000000000, 0.9659258262890683122, 1.000000000000000000, 0.9659258262890683122, 1.000000000000000000, 0.9659258262890683122, 1.000000000000000000, 0.9659258262890683122, 1.000000000000000000, 0.9659258262890683122, 1.000000000000000000, 0.9659258262890683122, 1.000000000000000000, 0.9659258262890683122, 1.000000000000000000, 0.9659258262890683122, 1.000000000000000000, 0.9659258262890683122, 1.000000000000000000, 0.9659258262890683122, 1.000000000000000000, 0.9659258262890683122, 1.000000000000000000, 0.9659258262890683122, 1.000000000000000000, 0.9659258262890683122, 1.000000000000000000, 0.9659258262890683122, 1.000000000000000000, 0.9659258262890683122, 1.000000000000000000, 0.9659258262890683122, 1.000000000000000000, 0.9659258262890683122, 1.000000000000000000, 0.9659258262890683122, 1.000000000000000000, 0.9659258262890683122, 1.000000000000000000, 0.9659258262890683122, 1.000000000000000000, 0.9659258262890683122, 1.000000000000000000, 0.9659258262890683122, 1.000000000000000000, 0.9659258262890683122, 1.000000000000000000, 0.9659258262890683122, 1.000000000000000000, 0.9659258262890683122, 1.000000000000000000, 0.9659258262890683122, 1.000000000000000000, 0.9659258262890683122, 1.000000000000000000, 0.9659258262890683122, 1.000000000000000000, 0.9659258262890683122, 1.000000000000000000, 0.9659258262890683122, 1.000000000000000000, 0.9659258262890683122, 1.000000000000000000, 0.9659258262890683122, 1.000000000000000000, 0.9659258262890683122, 1.000000000000000000, 0.9659258262890683122, 1.000000000000000000, 0.9659258262890683122, 1.000000000000000000, 0.9659258262890683122, 1.000000000000000000, 0.9659258262890683122, 1.000000000000000000, 0.9659258262890683122, 1.000000000000000000, 0.9659258262890683122, 1.000000000000000000, 0.9659258262890683122, 1.000000000000000000, 0.9659258262890683122, 1.000000000000000000, 0.9659258262890683122, 1.000000000000000000, 0.9659258262890683122, 1.000000000000000000, 0.9659258262890683122, 1.000000000000000000, 0.9659258262890683122, 1.000000000000000000, 0.9659258262890683122, 1.000000000000000000, 0.9659258262890683122, 1.000000000000000000, 0.9659258262890683122, 1.000000000000000000, 0.9659258262890683122, 1.000000000000000000, 0.9659258262890683122, 1.000000000000000000, 0.9659258262890683122, 1.000000000000000000, 0.9659258262890683122, 1.000000000000000000, 0.9659258262890683122, 1.000000000000000000, 0.9659258262890683122, 1.000000000000000000, 0.9659258262890683122, 1.000000000000000000, 0.9659258262890683122, 1.000000000000000000, 0.9659258262890683122, 1.000000000000000000, 0.9659258262890683122, 1.000000000000000000, 0.9659258262890683122, 1.000000000000000000, 0.9659258262890683122, 1.000000000000000000, 0.9659258262890683122, 1.000000000000000000, 0.9659258262890683122, 1.000000000000000000, 0.9659258262890683122, 1.000000000000000000, 0.9659258262890683122, 1.000000000000000000, 0.9659258262890683122, 1.000000000000000000, 0.9659258262890683122, 1.000000000000000000, 0.9659258262890683122, 1.000000000000000000, 0.9659258262890683122, 1.000000000000000000, 0.9659258262890683122, 1.000000000000000000, 0.9659258262890683122, 1.000000000000000000, 0.9659258262890683122, 1.000000000000000000, 0.9659258262890683122, 1.000000000000000000, 0.9659258262890683122, 1.000000000000000000, 0.9659258262890683122, 1.000000000000000000, 0.9659258262890683122, 1.000000000000000000, 0.9659258262890683122, 1.000000000000000000, 0.9659258262890683122, 1.000000000000000000, 0.9659258262890683122, 1.000000000000000000, 0.9659258262890683122, 1.000000000000000000, 0.9659258262890683122, 1.000000000000000000, 0.9659258262890683122, 1.000000000000000000, 0.9659258262890683122, 1.000000000000000000, 0.9659258262890683122, 1.000000000000000000, 0.9659258262890683122, 1.000000000000000000, 0.9659258262890683122, 1.000000000000000000, 0.9659258262890683122, 1.000000000000000000, 0.9659258262890683122, 1.000000000000000000, 0.9659258262890683122, 1.000000000000000000, 0.9659258262890683122, 1.000000000000000000, 0.9659258262890683122, 1.000000000000000000, 0.9659258262890683122, 1.000000000000000000, 0.9659258262890683122, 1.000000000000000000, 0.9659258262890683122, 1.000000000000000000, 0.9659258262890683122, 1.000000000000000000, 0.9659258262890683122, 1.000000000000000000, 0.9659258262890683122, 1.000000000000000000, 0.9659258262890683122, 1.000000000000000000, 0.9659258262890683122, 1.000000000000000000, 0.9659258262890683122, 1.000000000000000000, 0.9659258262890683122, 1.000000000000000000, 0.9659258262890683122, 1.000000000000000000, 0.9659258262890683122, 1.000000000000000000, 0.9659258262890683122, 1.000000000000000000, 0.9659258262890683122, 1.000000000000000000, 0.9659258262890683122, 1.000000000000000000, 0.9659258262890683122, 1.000000000000000000, 0.9659258262890683122, 1.000000000000000000, 0.9659258262890683122, 1.000000000000000000, 0.9659258262890683122, 1.000000000000000000, 0.9659258262890683122, 1.000000000000000000, 0.9659258262890683122, 1.000000000000000000, 0.9659258262890683122, 1.000000000000000000, 0.9659258262890683122, 1.000000000000000000, 0.9659258262890683122, 1.000000000000000000, 0.9659258262890683122, 1.000000000000000000, 0.9659258262890683122, 1.000000000000000000, 0.9659258262890683122, 1.000000000000000000, 0.9659258262890683122, 1.000000000000000000) ) ) 
 REPRESENTATION_ITEM ( '' )  SURFACE ( )  );
#24805=CARTESIAN_POINT ( 'NONE',  ( 0.7152230971128616943, -0.08942795157527998196, 0.3641732283464567121 ) ) ;
#24808=VERTEX_POINT ( 'NONE', #82819 ) ;
#24809=CARTESIAN_POINT ( 'NONE',  ( -0.1049868766404193215, 0.1283753931104746893, -0.1820866141732285504 ) ) ;
#24811=CARTESIAN_POINT ( 'NONE',  ( 0.7545931758530188826, -0.6692913385826771977, 0.1292274648535927661 ) ) ;
#24812=CARTESIAN_POINT ( 'NONE',  ( 0.2427821522309716595, -0.3162353388693409650, -0.4822834645669289433 ) ) ;
#24813=CARTESIAN_POINT ( 'NONE',  ( -0.5774278215223089816, 0.2306618581243847221, -0.2411417322834647770 ) ) ;
#24815=CARTESIAN_POINT ( 'NONE',  ( -1.220472440944881054, -0.6692913385826771977, 8.415575281601705876E-17 ) ) ;
#24817=CARTESIAN_POINT ( 'NONE',  ( 1.338582677165355062, -0.1870078740157480601, -0.3641732283464567677 ) ) ;
#24818=CARTESIAN_POINT ( 'NONE',  ( -1.509186351706035767, -0.4281496062992124485, 0.4176697321401328655 ) ) ;
#24819=CARTESIAN_POINT ( 'NONE',  ( 0.8989501312335964611, 0.2952755905511811885, 0.1292274648535926551 ) ) ;
#24820=CARTESIAN_POINT ( 'NONE',  ( 1.154855643044620184, -0.6046776061558807314, 0.2411417322834647770 ) ) ;
#24822=CARTESIAN_POINT ( 'NONE',  ( -1.345144356955379816, -0.05778040916215560624, -0.4822834645669293319 ) ) ;
#24824=CARTESIAN_POINT ( 'NONE',  ( -0.2624671916010490880, 0.2306618581243847221, -0.2411417322834647770 ) ) ;
#24827=CARTESIAN_POINT ( 'NONE',  ( 1.377952755905512472, 0.2952755905511811885, 0.000000000000000000 ) ) ;
#24828=CARTESIAN_POINT ( 'NONE',  ( 0.05905511811023709395, -0.4536011799217367080, 0.2665933059059888421 ) ) ;
#24829=CARTESIAN_POINT ( 'NONE',  ( 0.7939632545931766261, -0.05778040916215522460, 0.4822834645669289988 ) ) ;
#24831=CARTESIAN_POINT ( 'NONE',  ( 0.6496062992125991586, -0.4536011799217368745, -0.2665933059059886201 ) ) ;
#24832=CARTESIAN_POINT ( 'NONE',  ( 0.2230971128608929543, 0.05413385826771626580, -0.4176697321401330321 ) ) ;
#24834=CARTESIAN_POINT ( 'NONE',  ( -0.9645669291338575535, -0.5400638737290844871, 0.3530559997133364547 ) ) ;
#24835=CARTESIAN_POINT ( 'NONE',  ( -0.1902887139107604098, 0.2952755905511810219, -0.1292274648535930437 ) ) ;
#24837=CARTESIAN_POINT ( 'NONE',  ( 0.7808398950131240079, -0.2845877964562159024, 0.3641732283464567677 ) ) ;
#24839=CARTESIAN_POINT ( 'NONE',  ( -0.3871391076115479057, -0.3162353388693409650, -0.4822834645669289433 ) ) ;
#24841=CARTESIAN_POINT ( 'NONE',  ( 0.1837270341207357105, -0.5023911411419708095, -0.1820866141732282451 ) ) ;
#24843=CARTESIAN_POINT ( 'NONE',  ( -0.1574803149606292529, -0.1870078740157479769, 0.4822834645669291653 ) ) ;
#24844=CARTESIAN_POINT ( 'NONE',  ( 0.4068241469816279987, -0.3690944881889765550, -0.3153832671262227771 ) ) ;
#24846=CARTESIAN_POINT ( 'NONE',  ( 0.4330708661417329575, 0.2952755905511811885, 0.000000000000000000 ) ) ;
#24847=EDGE_CURVE ( 'NONE', #7338, #24368, #72398, .T. ) ;
#24848=CARTESIAN_POINT ( 'NONE',  ( 1.122047244094488860, -0.4536011799217368745, -0.2665933059059886201 ) ) ;
#24849=CARTESIAN_POINT ( 'NONE',  ( 0.1690661813110321821, 0.02791078216816225699, 0.4328096321851905293 ) ) ;
#24850=CARTESIAN_POINT ( 'NONE',  ( -0.5971128608923877978, 0.1771653543307087630, 0.09757992244046791164 ) ) ;
#24851=CARTESIAN_POINT ( 'NONE',  ( -0.8464566929133852113, -0.4536011799217368745, -0.2665933059059886201 ) ) ;
#24852=CARTESIAN_POINT ( 'NONE',  ( -0.2755905511811015396, -0.6692913385826771977, 8.415575281601705876E-17 ) ) ;
#24853=CARTESIAN_POINT ( 'NONE',  ( 0.1115485564304467270, -0.6692913385826773087, -0.1292274648535924053 ) ) ;
#24854=CARTESIAN_POINT ( 'NONE',  ( 0.9580052493438327987, -0.3690944881889765550, -0.3153832671262227771 ) ) ;
#24856=CARTESIAN_POINT ( 'NONE',  ( 1.568241469816273437, -0.2845877964562159024, 0.3641732283464567677 ) ) ;
#24857=CARTESIAN_POINT ( 'NONE',  ( 0.6889763779527566800, -0.5400638737290844871, 0.3530559997133364547 ) ) ;
#24859=CARTESIAN_POINT ( 'NONE',  ( -1.614173228346456712, 1.818966223839196816, -0.1372047244094478091 ) ) ;
#24860=CARTESIAN_POINT ( 'NONE',  ( -0.2493438320209966919, 0.05413385826771626580, -0.4176697321401330321 ) ) ;
#24862=CARTESIAN_POINT ( 'NONE',  ( 0.8398950131233602345, -0.6046776061558807314, 0.2411417322834647770 ) ) ;
#24863=CARTESIAN_POINT ( 'NONE',  ( 0.4133858267716541968, 0.1660481256975885056, 0.3530559997133364547 ) ) ;
#24866=CARTESIAN_POINT ( 'NONE',  ( 0.4855643044619430415, -0.3690944881889765550, -0.3153832671262227771 ) ) ;
#24867=CARTESIAN_POINT ( 'NONE',  ( 1.076115485564305141, 0.2306618581243847221, -0.2411417322834647770 ) ) ;
#24868=CARTESIAN_POINT ( 'NONE',  ( -0.3543307086614165824, -0.5511811023622047445, 6.969142054262312111E-17 ) ) ;
#24869=CARTESIAN_POINT ( 'NONE',  ( -0.3674540682414689785, 0.2306618581243848609, 0.2411417322834645549 ) ) ;
#24871=CARTESIAN_POINT ( 'NONE',  ( 0.2230971128608929543, 0.05413385826771626580, -0.4176697321401330321 ) ) ;
#24872=CARTESIAN_POINT ( 'NONE',  ( -0.8727034120734901146, -0.3162353388693405765, 0.4822834645669290543 ) ) ;
#24873=CARTESIAN_POINT ( 'NONE',  ( -0.6758530183727028406, -0.5511811023622048555, -0.09757992244046775898 ) ) ;
#24874=CARTESIAN_POINT ( 'NONE',  ( 0.4265091863517067039, -0.6692913385826773087, -0.1292274648535924053 ) ) ;
#24875=CARTESIAN_POINT ( 'NONE',  ( -1.148293963254592542, -0.6692913385826773087, -0.1292274648535924053 ) ) ;
#24876=CARTESIAN_POINT ( 'NONE',  ( -0.3149606299212590610, -0.1870078740157480879, -0.4822834645669291653 ) ) ;
#24878=CARTESIAN_POINT ( 'NONE',  ( -0.9341826970036740674, -2.609244250047836720E-15, 0.4118477457933002461 ) ) ;
#24879=CARTESIAN_POINT ( 'NONE',  ( 1.522309711286089939, -0.6046776061558809534, -0.2411417322834644161 ) ) ;
#24880=CARTESIAN_POINT ( 'NONE',  ( 1.633858267716535639, -0.5400638737290844871, 0.3530559997133364547 ) ) ;
#24883=CARTESIAN_POINT ( 'NONE',  ( -1.089238845144356427, 0.05413385826771666132, 0.4176697321401328100 ) ) ;
#24886=ORIENTED_EDGE ( 'NONE', *, *, #56212, .F. ) ;
#24887=CARTESIAN_POINT ( 'NONE',  ( 0.1837270341207357105, -0.5023911411419708095, -0.1820866141732282451 ) ) ;
#24889=CARTESIAN_POINT ( 'NONE',  ( 0.5708661417322841158, -0.5400638737290845981, -0.3530559997133363437 ) ) ;
#24892=CARTESIAN_POINT ( 'NONE',  ( -0.4593175853018364174, -0.3690944881889765550, -0.3153832671262227771 ) ) ;
#24893=CARTESIAN_POINT ( 'NONE',  ( -0.2624671916010490880, 0.2306618581243847221, -0.2411417322834647770 ) ) ;
#24894=CARTESIAN_POINT ( 'NONE',  ( 1.292650918635171564, -0.6692913385826773087, -0.1292274648535924053 ) ) ;
#24895=CARTESIAN_POINT ( 'NONE',  ( 0.9580052493438326877, -0.004921259842519576551, 0.3153832671262227771 ) ) ;
#24896=CARTESIAN_POINT ( 'NONE',  ( 0.1771653543307093182, -0.5400638737290845981, -0.3530559997133363437 ) ) ;
#24898=CARTESIAN_POINT ( 'NONE',  ( -0.4986876640419939388, 0.2306618581243847221, -0.2411417322834647770 ) ) ;
#24899=CARTESIAN_POINT ( 'NONE',  ( -1.312335958005248715, -0.5023911411419708095, -0.1820866141732282451 ) ) ;
#24900=CARTESIAN_POINT ( 'NONE',  ( -0.4396325459317579898, 0.2952755905511811885, 0.1292274648535926551 ) ) ;
#24901=CARTESIAN_POINT ( 'NONE',  ( 1.692913385826772421, 0.2952755905511811885, 0.000000000000000000 ) ) ;
#24902=CARTESIAN_POINT ( 'NONE',  ( 0.6410189441372368124, -2.592014407703319119E-15, 0.3954974714151467952 ) ) ;
#24903=EDGE_LOOP ( 'NONE', ( #78683, #22872, #46098, #58115 ) ) ;
#24905=CARTESIAN_POINT ( 'NONE',  ( 0.2296587926509192634, -0.3162353388693405765, 0.4822834645669290543 ) ) ;
#24908=CARTESIAN_POINT ( 'NONE',  ( -0.5511811023622041894, -0.1870078740157480879, -0.4822834645669291653 ) ) ;
#24909=CARTESIAN_POINT ( 'NONE',  ( -1.358267716535432434, -0.5400638737290844871, 0.3530559997133364547 ) ) ;
#24910=CARTESIAN_POINT ( 'NONE',  ( 0.7808398950131240079, -0.3162353388693405765, 0.4822834645669290543 ) ) ;
#24911=CARTESIAN_POINT ( 'NONE',  ( 0.2034120734908144990, -0.6692913385826771977, 0.1292274648535927661 ) ) ;
#24913=CARTESIAN_POINT ( 'NONE',  ( -0.6364829396325453192, -0.3162353388693405765, 0.4822834645669290543 ) ) ;
#24914=CARTESIAN_POINT ( 'NONE',  ( -0.2821522309711278487, -0.6692913385826773087, -0.1292274648535924053 ) ) ;
#24915=CARTESIAN_POINT ( 'NONE',  ( -0.7283464566929126471, -0.5400638737290844871, 0.3530559997133364547 ) ) ;
#24916=CARTESIAN_POINT ( 'NONE',  ( 0.4855643044619430415, -0.3690944881889765550, -0.3153832671262227771 ) ) ;
#24918=CARTESIAN_POINT ( 'NONE',  ( -0.2755905511811018171, 0.2952755905511811885, 0.000000000000000000 ) ) ;
#24919=DIRECTION ( 'NONE',  ( 0.000000000000000000, 0.000000000000000000, 1.000000000000000000 ) ) ;
#24921=CARTESIAN_POINT ( 'NONE',  ( 1.115485564304462551, 0.05413385826771666132, 0.4176697321401328100 ) ) ;
#24925=CARTESIAN_POINT ( 'NONE',  ( 0.2690288713910767848, 0.2952755905511811885, 0.1292274648535926551 ) ) ;
#24926=CARTESIAN_POINT ( 'NONE',  ( -0.02624671916010428221, -0.5023911411419708095, 0.1820866141732285504 ) ) ;
#24927=CARTESIAN_POINT ( 'NONE',  ( 1.653543307086614789, -0.1870078740157479769, 0.3641732283464567677 ) ) ;
#24931=CARTESIAN_POINT ( 'NONE',  ( 0.2559055118110243332, -0.5400638737290845981, -0.3530559997133363437 ) ) ;
#24932=CARTESIAN_POINT ( 'NONE',  ( -1.200787401574802349, -0.5400638737290844871, 0.3530559997133364547 ) ) ;
#24933=CARTESIAN_POINT ( 'NONE',  ( -1.141732283464566011, -0.6692913385826771977, 8.415575281601705876E-17 ) ) ;
#24934=CARTESIAN_POINT ( 'NONE',  ( 0.1574803149606306130, -0.1870078740157479769, 0.4822834645669291653 ) ) ;
#24935=CARTESIAN_POINT ( 'NONE',  ( 0.9908136482939640111, 0.2952755905511810774, -0.1292274648535930714 ) ) ;
#24936=CARTESIAN_POINT ( 'NONE',  ( 1.555118110236221041, 0.07958543189024071263, -0.2665933059059888421 ) ) ;
#24937=CARTESIAN_POINT ( 'NONE',  ( 0.7283464566929143125, 0.07958543189024085140, 0.2665933059059887866 ) ) ;
#24938=CARTESIAN_POINT ( 'NONE',  ( -0.7283464566929126471, -0.5400638737290844871, 0.3530559997133364547 ) ) ;
#24940=CARTESIAN_POINT ( 'NONE',  ( 1.469816272965879911, -0.6046776061558807314, 0.2411417322834647770 ) ) ;
#24942=CARTESIAN_POINT ( 'NONE',  ( 1.312335958005250269, -0.6046776061558807314, 0.2411417322834647770 ) ) ;
#24944=CARTESIAN_POINT ( 'NONE',  ( -1.719160104986876103, -0.004921259842519576551, 0.3153832671262227771 ) ) ;
#24945=CARTESIAN_POINT ( 'NONE',  ( -0.01968503937007793844, 0.1660481256975883668, -0.3530559997133364547 ) ) ;
#24946=CARTESIAN_POINT ( 'NONE',  ( 0.7808398950131240079, -0.2845877964562159024, 0.3641732283464567677 ) ) ;
#24947=CARTESIAN_POINT ( 'NONE',  ( -1.699475065616797398, 0.1771653543307087630, 0.09757992244046791164 ) ) ;
#24948=CARTESIAN_POINT ( 'NONE',  ( 1.056430446194226658, 0.2952755905511811885, 0.1292274648535926551 ) ) ;
#24950=CARTESIAN_POINT ( 'NONE',  ( -0.5774278215223089816, 0.1283753931104746893, -0.1820866141732285504 ) ) ;
#24951=CARTESIAN_POINT ( 'NONE',  ( -0.6102362204724400829, 0.1660481256975885056, 0.3530559997133364547 ) ) ;
#24952=CARTESIAN_POINT ( 'NONE',  ( -1.646981627296586703, -0.08942795157527998196, 0.3641732283464567121 ) ) ;
#24953=CARTESIAN_POINT ( 'NONE',  ( -1.286089238845143479, -0.6046776061558807314, 0.2411417322834647770 ) ) ;
#24954=CARTESIAN_POINT ( 'NONE',  ( 1.187664041994751285, -0.05778040916215522460, 0.4822834645669289988 ) ) ;
#24956=CARTESIAN_POINT ( 'NONE',  ( -1.364829396325458521, -0.5023911411419708095, 0.1820866141732285504 ) ) ;
#24959=CARTESIAN_POINT ( 'NONE',  ( 1.030183727034121421, -0.3162353388693409650, -0.4822834645669289433 ) ) ;
#24962=CARTESIAN_POINT ( 'NONE',  ( -1.601049868766403650, -0.6046776061558807314, 0.2411417322834647770 ) ) ;
#24963=CARTESIAN_POINT ( 'NONE',  ( -1.450131233595799651, 0.1771653543307087075, -0.09757992244046823083 ) ) ;
#24964=CARTESIAN_POINT ( 'NONE',  ( -1.049868766404198794, 0.1283753931104746893, -0.1820866141732285504 ) ) ;
#24965=CARTESIAN_POINT ( 'NONE',  ( 1.627296587926509996, -0.5023911411419708095, 0.1820866141732285504 ) ) ;
#24966=CARTESIAN_POINT ( 'NONE',  ( -0.3477690288713902178, 0.2952755905511810774, -0.1292274648535930714 ) ) ;
#24967=CARTESIAN_POINT ( 'NONE',  ( 0.1968503937007881344, -0.5511811023622047445, 6.969142054262312111E-17 ) ) ;
#24968=CARTESIAN_POINT ( 'NONE',  ( -1.482939632545930975, -0.3690944881889765550, -0.3153832671262227771 ) ) ;
#24969=CARTESIAN_POINT ( 'NONE',  ( 1.266404199475066328, -0.08942795157527998196, 0.3641732283464567121 ) ) ;
#24970=CARTESIAN_POINT ( 'NONE',  ( 1.030183727034121421, -0.05778040916215522460, 0.4822834645669289988 ) ) ;
#24971=CARTESIAN_POINT ( 'NONE',  ( 1.423884514435696191, -0.05778040916215522460, 0.4822834645669289988 ) ) ;
#24972=CARTESIAN_POINT ( 'NONE',  ( -0.01968503937007793844, 0.07958543189024071263, -0.2665933059059888421 ) ) ;
#24973=CARTESIAN_POINT ( 'NONE',  ( 0.2821522309711292364, 0.2952755905511810774, -0.1292274648535930714 ) ) ;
#24974=CARTESIAN_POINT ( 'NONE',  ( 0.9251968503937015864, -0.4536011799217367080, 0.2665933059059888421 ) ) ;
#24976=CARTESIAN_POINT ( 'NONE',  ( -1.502624671916009680, -0.3162353388693405765, 0.4822834645669290543 ) ) ;
#24978=CARTESIAN_POINT ( 'NONE',  ( -1.318897637795274802, 0.1660481256975885056, 0.3530559997133364547 ) ) ;
#24979=CARTESIAN_POINT ( 'NONE',  ( 0.05249343832021075018, 0.2306618581243847221, -0.2411417322834647770 ) ) ;
#24982=CARTESIAN_POINT ( 'NONE',  ( 0.5446194225721792126, -0.05778040916215560624, -0.4822834645669293319 ) ) ;
#24983=CARTESIAN_POINT ( 'NONE',  ( 0.9973753280839902091, 0.1283753931104746893, -0.1820866141732285504 ) ) ;
#24984=CARTESIAN_POINT ( 'NONE',  ( -0.4133858267716528645, -0.5400638737290844871, 0.3530559997133364547 ) ) ;
#24985=CARTESIAN_POINT ( 'NONE',  ( 0.5052493438320215802, 0.2952755905511811885, 0.1292274648535926551 ) ) ;
#24986=EDGE_CURVE ( 'NONE', #30946, #8463, #70179, .T. ) ;
#24990=CARTESIAN_POINT ( 'NONE',  ( 0.3249695492770460770, 1.223219560026271499E-15, 0.4445507791589056734 ) ) ;
#24993=CARTESIAN_POINT ( 'NONE',  ( -0.6692913385826764205, -0.5511811023622047445, 6.969142054262312111E-17 ) ) ;
#24994=CARTESIAN_POINT ( 'NONE',  ( -0.6824146981627291497, -0.6046776061558809534, -0.2411417322834644161 ) ) ;
#24996=CARTESIAN_POINT ( 'NONE',  ( 0.6889763779527566800, -0.5400638737290844871, 0.3530559997133364547 ) ) ;
#24997=CARTESIAN_POINT ( 'NONE',  ( -1.607611548556429737, 0.2952755905511810774, -0.1292274648535930714 ) ) ;
#24998=CARTESIAN_POINT ( 'NONE',  ( 0.6233595800524939223, -0.3162353388693405765, 0.4822834645669290543 ) ) ;
#25005=CARTESIAN_POINT ( 'NONE',  ( 1.115485564304462551, 0.05413385826771666132, 0.4176697321401328100 ) ) ;
#25006=CARTESIAN_POINT ( 'NONE',  ( 0.5774278215223103139, -0.6046776061558809534, -0.2411417322834644161 ) ) ;
#25007=CARTESIAN_POINT ( 'NONE',  ( 0.8070866141732288002, 0.07958543189024085140, 0.2665933059059887866 ) ) ;
#25008=CARTESIAN_POINT ( 'NONE',  ( 1.213910761154856299, 0.2952755905511811885, 0.1292274648535926551 ) ) ;
#25010=CARTESIAN_POINT ( 'NONE',  ( -1.604771003085129433, 2.104981124449682106, 0.1466069496707750608 ) ) ;
#25011=CARTESIAN_POINT ( 'NONE',  ( 0.7152230971128616943, -0.05778040916215522460, 0.4822834645669289988 ) ) ;
#25012=CARTESIAN_POINT ( 'NONE',  ( 1.496062992125985147, -0.1870078740157479769, 0.3641732283464567677 ) ) ;
#25013=CARTESIAN_POINT ( 'NONE',  ( -0.8858267716535425107, 0.1660481256975883668, -0.3530559997133364547 ) ) ;
#25014=CARTESIAN_POINT ( 'NONE',  ( -0.9580052493438311334, -0.4281496062992124485, 0.4176697321401328655 ) ) ;
#25015=CARTESIAN_POINT ( 'NONE',  ( 1.253280839895013710, -0.3162353388693405765, 0.4822834645669290543 ) ) ;
#25022=CARTESIAN_POINT ( 'NONE',  ( -0.03937007874015669567, 0.2066929133858268208, 0.000000000000000000 ) ) ;
#25023=AXIS2_PLACEMENT_3D ( 'NONE', #30228, #43667, #24735 ) ;
#25024=CARTESIAN_POINT ( 'NONE',  ( 1.305774278215223960, 0.1771653543307087075, -0.09757992244046823083 ) ) ;
#25026=CARTESIAN_POINT ( 'NONE',  ( 1.318897637795276356, -0.4536011799217367080, 0.2665933059059888421 ) ) ;
#25031=CARTESIAN_POINT ( 'NONE',  ( -0.6036745406824141069, -0.5023911411419708095, -0.1820866141732282451 ) ) ;
#25032=CARTESIAN_POINT ( 'NONE',  ( -1.607611548556429737, -0.5511811023622046335, 0.09757992244046803654 ) ) ;
#25033=CARTESIAN_POINT ( 'NONE',  ( -1.450131233595799651, 0.2952755905511810774, -0.1292274648535930714 ) ) ;
#25034=CARTESIAN_POINT ( 'NONE',  ( -0.02624671916010428221, -0.6046776061558807314, 0.2411417322834647770 ) ) ;
#25035=CARTESIAN_POINT ( 'NONE',  ( -1.548556430446193399, -0.6046776061558809534, -0.2411417322834644161 ) ) ;
#25036=ORIENTED_EDGE ( 'NONE', *, *, #51779, .T. ) ;
#25038=( NAMED_UNIT ( * ) PLANE_ANGLE_UNIT ( ) SI_UNIT ( $, .RADIAN. ) );
#25040=CARTESIAN_POINT ( 'NONE',  ( -1.604771003085130099, 1.553800022087478583, 0.1466069496707745334 ) ) ;
#25041=CARTESIAN_POINT ( 'NONE',  ( -0.3346456692913377662, 0.07958543189024071263, -0.2665933059059888421 ) ) ;
#25042=CARTESIAN_POINT ( 'NONE',  ( -1.279527559055116948, 0.1660481256975883668, -0.3530559997133364547 ) ) ;
#25043=CARTESIAN_POINT ( 'NONE',  ( 1.043307086614173818, 0.1660481256975885056, 0.3530559997133364547 ) ) ;
#25046=FACE_OUTER_BOUND ( 'NONE', #80231, .T. ) ;
#25047=CARTESIAN_POINT ( 'NONE',  ( 1.089238845144357759, 0.05413385826771626580, -0.4176697321401330321 ) ) ;
#25048=CARTESIAN_POINT ( 'NONE',  ( -1.115485564304461219, -0.4281496062992124485, 0.4176697321401328655 ) ) ;
#25050=CARTESIAN_POINT ( 'NONE',  ( -0.3149606299212590610, -0.1870078740157479769, 0.3641732283464567677 ) ) ;
#25052=CARTESIAN_POINT ( 'NONE',  ( -0.3937007874015740483, -0.1870078740157479769, 0.3641732283464567677 ) ) ;
#25053=CARTESIAN_POINT ( 'NONE',  ( 0.3280839895013130669, -0.004921259842519576551, 0.3153832671262227771 ) ) ;
#25054=CARTESIAN_POINT ( 'NONE',  ( 0.2099737532808405305, 0.2306618581243847221, -0.2411417322834647770 ) ) ;
#25055=CARTESIAN_POINT ( 'NONE',  ( -0.7086614173228339419, -0.1870078740157479769, 0.3641732283464567677 ) ) ;
#25057=CARTESIAN_POINT ( 'NONE',  ( 1.345144356955381593, -0.3162353388693409650, -0.4822834645669289433 ) ) ;
#25058=AXIS2_PLACEMENT_3D ( 'NONE', #41429, #35114, #29214 ) ;
#25059=CARTESIAN_POINT ( 'NONE',  ( -1.437007874015747477, 0.1660481256975883668, -0.3530559997133364547 ) ) ;
#25061=CIRCLE ( 'NONE', #23698, 1.181102362204724310 ) ;
#25062=CARTESIAN_POINT ( 'NONE',  ( -0.3215223097112853146, -0.3162353388693405765, 0.4822834645669290543 ) ) ;
#25063=CARTESIAN_POINT ( 'NONE',  ( -1.023622047244093558, -0.1870078740157479769, 0.4822834645669291653 ) ) ;
#25064=CARTESIAN_POINT ( 'NONE',  ( 1.332020997375329197, -0.2845877964562159024, 0.3641732283464567677 ) ) ;
#25065=CARTESIAN_POINT ( 'NONE',  ( -0.4330708661417315697, 0.1771653543307087630, 0.000000000000000000 ) ) ;
#25066=CARTESIAN_POINT ( 'NONE',  ( -0.7414698162729651543, 0.2952755905511810774, -0.1292274648535930714 ) ) ;
#25067=CARTESIAN_POINT ( 'NONE',  ( -1.095800524934382292, -0.3162353388693409650, -0.4822834645669289433 ) ) ;
#25068=CARTESIAN_POINT ( 'NONE',  ( -0.4047984445375523710, 5.961526036605507449E-15, -0.3954985857520045833 ) ) ;
#25069=CARTESIAN_POINT ( 'NONE',  ( 1.141732283464567788, -0.5511811023622047445, 6.969142054262312111E-17 ) ) ;
#25070=CARTESIAN_POINT ( 'NONE',  ( -0.3346456692913377662, 0.1660481256975883668, -0.3530559997133364547 ) ) ;
#25071=CARTESIAN_POINT ( 'NONE',  ( -0.9186351706036736120, 0.2306618581243848609, 0.2411417322834645549 ) ) ;
#25074=CARTESIAN_POINT ( 'NONE',  ( -0.9973753280839886548, 0.1283753931104748280, 0.1820866141732283561 ) ) ;
#25075=CARTESIAN_POINT ( 'NONE',  ( 1.338582677165355062, -0.1870078740157480879, -0.4822834645669291653 ) ) ;
#25076=CARTESIAN_POINT ( 'NONE',  ( -1.181102362204723644, -0.1870078740157480601, -0.3641732283464567677 ) ) ;
#25078=CARTESIAN_POINT ( 'NONE',  ( -1.043307086614172707, 0.1660481256975883668, -0.3530559997133364547 ) ) ;
#25079=CARTESIAN_POINT ( 'NONE',  ( 1.391076115485564868, 0.2306618581243847221, -0.2411417322834647770 ) ) ;
#25080=CARTESIAN_POINT ( 'NONE',  ( 0.8005249343832028242, -0.4281496062992127816, -0.4176697321401328100 ) ) ;
#25082=CARTESIAN_POINT ( 'NONE',  ( -1.174540682414697335, -0.2845877964562161244, -0.3641732283464567121 ) ) ;
#25088=CARTESIAN_POINT ( 'NONE',  ( 1.332020997375329197, -0.2845877964562159024, 0.3641732283464567677 ) ) ;
#25089=CARTESIAN_POINT ( 'NONE',  ( 0.6627296587926515548, 0.1771653543307087630, 0.09757992244046791164 ) ) ;
#25090=CARTESIAN_POINT ( 'NONE',  ( 0.5118110236220478892, 0.2952755905511811885, 0.000000000000000000 ) ) ;
#25092=B_SPLINE_CURVE_WITH_KNOTS ( 'NONE', 3,
 ( #83219, #69763, #82804, #50388, #70583, #55875, #44883 ),
 .UNSPECIFIED., .F., .F.,
 ( 4, 3, 4 ),
 ( 1.908195823574488112E-17, 0.001246230184515590604, 0.002492489877932652868 ),
 .UNSPECIFIED. ) ;
#25094=CARTESIAN_POINT ( 'NONE',  ( 0.8005249343832028242, -0.3690944881889765550, -0.3153832671262227771 ) ) ;
#25095=CARTESIAN_POINT ( 'NONE',  ( -0.4593175853018364174, -0.4281496062992127816, -0.4176697321401328100 ) ) ;
#25096=CARTESIAN_POINT ( 'NONE',  ( -1.194225721784776262, -0.4281496062992124485, 0.4176697321401328655 ) ) ;
#25097=CARTESIAN_POINT ( 'NONE',  ( 0.8792650918635177559, 0.05413385826771666132, 0.4176697321401328100 ) ) ;
#25101=ORIENTED_EDGE ( 'NONE', *, *, #37233, .F. ) ;
#25102=CARTESIAN_POINT ( 'NONE',  ( -1.469816272965878357, -0.6046776061558809534, -0.2411417322834644161 ) ) ;
#25103=CARTESIAN_POINT ( 'NONE',  ( -0.6364829396325453192, -0.05778040916215560624, -0.4822834645669293319 ) ) ;
#25104=CARTESIAN_POINT ( 'NONE',  ( -0.7808398950131222316, -0.2845877964562161244, -0.3641732283464567121 ) ) ;
#25105=CARTESIAN_POINT ( 'NONE',  ( -0.8727034120734901146, -0.3162353388693405765, 0.4822834645669290543 ) ) ;
#25106=CARTESIAN_POINT ( 'NONE',  ( 0.3543307086614181922, -0.6692913385826771977, 8.415575281601705876E-17 ) ) ;
#25107=CARTESIAN_POINT ( 'NONE',  ( -0.5183727034120726440, 0.2952755905511811885, 0.1292274648535926551 ) ) ;
#25108=CARTESIAN_POINT ( 'NONE',  ( -1.181102362204723644, -0.1870078740157479769, 0.4822834645669291653 ) ) ;
#25109=CARTESIAN_POINT ( 'NONE',  ( -0.8464566929133852113, -0.5400638737290845981, -0.3530559997133363437 ) ) ;
#25110=CARTESIAN_POINT ( 'NONE',  ( 0.6561679790026253567, 0.2306618581243848609, 0.2411417322834645549 ) ) ;
#25113=CARTESIAN_POINT ( 'NONE',  ( -0.9514435695538050464, -0.08942795157528024563, -0.3641732283464568787 ) ) ;
#25117=CARTESIAN_POINT ( 'NONE',  ( -1.279527559055116948, -0.4536011799217367080, 0.2665933059059888421 ) ) ;
#25120=CARTESIAN_POINT ( 'NONE',  ( -1.148293963254592542, 0.2952755905511811885, 0.1292274648535926551 ) ) ;
#25121=CARTESIAN_POINT ( 'NONE',  ( -0.8595800524934373854, -0.05778040916215522460, 0.4822834645669289988 ) ) ;
#25123=CARTESIAN_POINT ( 'NONE',  ( -0.9120734908136475250, 0.2952755905511811885, 0.1292274648535926551 ) ) ;
#25124=CARTESIAN_POINT ( 'NONE',  ( -1.443569553805773564, -0.6046776061558807314, 0.2411417322834647770 ) ) ;
#25125=CARTESIAN_POINT ( 'NONE',  ( -1.607611548556429737, 0.2952755905511810774, -0.1292274648535930714 ) ) ;
#25126=CARTESIAN_POINT ( 'NONE',  ( -1.633858267716534529, -0.5400638737290845981, -0.3530559997133363437 ) ) ;
#25127=CARTESIAN_POINT ( 'NONE',  ( 0.4724409448818904789, -0.1870078740157480601, -0.3641732283464567677 ) ) ;
#25128=DIRECTION ( 'NONE',  ( 1.000000000000000000, -0.000000000000000000, -0.000000000000000000 ) ) ;
#25130=CARTESIAN_POINT ( 'NONE',  ( -0.05905511811023545637, -0.4536011799217368745, -0.2665933059059886201 ) ) ;
#25131=CARTESIAN_POINT ( 'NONE',  ( -0.2887139107611542133, -0.6046776061558809534, -0.2411417322834644161 ) ) ;
#25132=CARTESIAN_POINT ( 'NONE',  ( 1.391076115485564868, -0.6046776061558807314, 0.2411417322834647770 ) ) ;
#25133=CARTESIAN_POINT ( 'NONE',  ( -0.3083989501312330295, -0.3162353388693409650, -0.4822834645669289433 ) ) ;
#25134=ORIENTED_EDGE ( 'NONE', *, *, #60455, .F. ) ;
#25135=CARTESIAN_POINT ( 'NONE',  ( -0.5639538267004599037, 0.004960608223778500969, -0.3437734562760191848 ) ) ;
#25138=CARTESIAN_POINT ( 'NONE',  ( -0.4921259842519677963, 0.1660481256975883668, -0.3530559997133364547 ) ) ;
#25139=CARTESIAN_POINT ( 'NONE',  ( 1.410761154855643795, -0.3162353388693405765, 0.4822834645669290543 ) ) ;
#25140=CARTESIAN_POINT ( 'NONE',  ( -1.010498687664041384, -0.3690944881889765550, -0.3153832671262227771 ) ) ;
#25141=CARTESIAN_POINT ( 'NONE',  ( -1.200787401574802349, 0.1660481256975883668, -0.3530559997133364547 ) ) ;
#25143=B_SPLINE_CURVE_WITH_KNOTS ( 'NONE', 3,
 ( #73971, #80707, #3675, #30577 ),
 .UNSPECIFIED., .F., .F.,
 ( 4, 4 ),
 ( 3.210432057704302528E-07, 0.001287787053612143027 ),
 .UNSPECIFIED. ) ;
#25146=CARTESIAN_POINT ( 'NONE',  ( 1.312335958005250269, -0.6046776061558807314, 0.2411417322834647770 ) ) ;
#25148=CARTESIAN_POINT ( 'NONE',  ( 0.01968503937007957949, -0.5400638737290845981, -0.3530559997133363437 ) ) ;
#25149=CARTESIAN_POINT ( 'NONE',  ( -1.187664041994749731, -0.2845877964562159024, 0.3641732283464567677 ) ) ;
#25150=CARTESIAN_POINT ( 'NONE',  ( -0.2952755905511804668, 0.1660481256975885056, 0.3530559997133364547 ) ) ;
#25152=CARTESIAN_POINT ( 'NONE',  ( -0.9186351706036736120, 0.2306618581243848609, 0.2411417322834645549 ) ) ;
#25153=CARTESIAN_POINT ( 'NONE',  ( -1.181102362204723644, -0.1870078740157480879, -0.4822834645669291653 ) ) ;
#25155=CARTESIAN_POINT ( 'NONE',  ( 0.9645669291338588858, 0.07958543189024085140, 0.2665933059059887866 ) ) ;
#25156=CARTESIAN_POINT ( 'NONE',  ( -0.1181102362204717315, 0.1771653543307087630, 0.000000000000000000 ) ) ;
#25157=CARTESIAN_POINT ( 'NONE',  ( 0.8005249343832028242, -0.3690944881889765550, -0.3153832671262227771 ) ) ;
#25158=CARTESIAN_POINT ( 'NONE',  ( -1.587926509186350810, -0.4281496062992124485, 0.4176697321401328655 ) ) ;
#25159=CARTESIAN_POINT ( 'NONE',  ( 1.423884514435696191, -0.05778040916215522460, 0.4822834645669289988 ) ) ;
#25160=CARTESIAN_POINT ( 'NONE',  ( 0.4593175853018380828, -0.004921259842519870586, -0.3153832671262229437 ) ) ;
#25161=CARTESIAN_POINT ( 'NONE',  ( -0.6692913385826764205, 0.2952755905511811885, 0.000000000000000000 ) ) ;
#25162=CARTESIAN_POINT ( 'NONE',  ( 1.299212598425197429, 0.2952755905511811885, 0.000000000000000000 ) ) ;
#25164=CARTESIAN_POINT ( 'NONE',  ( -0.1902887139107604098, 0.1771653543307087075, -0.09757992244046823083 ) ) ;
#25165=CARTESIAN_POINT ( 'NONE',  ( 1.614173228346457378, 0.7794589730111999293, 0.1372047244094478369 ) ) ;
#25167=CARTESIAN_POINT ( 'NONE',  ( 0.1574803149606306130, -0.1870078740157480879, -0.4822834645669291653 ) ) ;
#25169=CARTESIAN_POINT ( 'NONE',  ( 1.555118110236221041, -0.4536011799217367080, 0.2665933059059888421 ) ) ;
#25170=CARTESIAN_POINT ( 'NONE',  ( 0.07874015748031558404, -0.1870078740157480601, -0.3641732283464567677 ) ) ;
#25171=CARTESIAN_POINT ( 'NONE',  ( -1.522309711286088607, 0.2306618581243847221, -0.2411417322834647770 ) ) ;
#25172=CARTESIAN_POINT ( 'NONE',  ( -0.7808398950131222316, -0.2845877964562161244, -0.3641732283464567121 ) ) ;
#25173=DIRECTION ( 'NONE',  ( 1.000000000000000000, 3.083952846180990281E-16, 0.000000000000000000 ) ) ;
#25174=CARTESIAN_POINT ( 'NONE',  ( -1.174540682414697335, -0.3162353388693409650, -0.4822834645669289433 ) ) ;
#25175=CARTESIAN_POINT ( 'NONE',  ( -0.5905511811023613777, -0.6692913385826771977, 8.415575281601705876E-17 ) ) ;
#25179=CARTESIAN_POINT ( 'NONE',  ( 0.7677165354330716118, -0.4536011799217367080, 0.2665933059059888421 ) ) ;
#25180=CARTESIAN_POINT ( 'NONE',  ( -0.2099737532808391705, 0.2306618581243848609, 0.2411417322834645549 ) ) ;
#25181=CIRCLE ( 'NONE', #29230, 2.401574803149606474 ) ;
#25182=CARTESIAN_POINT ( 'NONE',  ( -0.6167979002624665030, -0.4281496062992127816, -0.4176697321401328100 ) ) ;
#25183=CARTESIAN_POINT ( 'NONE',  ( -0.8792650918635160906, -0.3690944881889763329, 0.3153832671262228327 ) ) ;
#25185=CARTESIAN_POINT ( 'NONE',  ( 0.07874015748031558404, -0.1870078740157479769, 0.4822834645669291653 ) ) ;
#25186=CARTESIAN_POINT ( 'NONE',  ( -1.456692913385826182, -0.5511811023622047445, 6.969142054262312111E-17 ) ) ;
#25187=CARTESIAN_POINT ( 'NONE',  ( 1.312335958005249825, 0.2306618581243847221, -0.2411417322834647770 ) ) ;
#25192=CARTESIAN_POINT ( 'NONE',  ( -0.2251228153049663061, -4.992347309556208597E-15, 0.3954985857520076920 ) ) ;
#25193=CARTESIAN_POINT ( 'NONE',  ( -1.364829396325458521, 0.2306618581243847221, -0.2411417322834647770 ) ) ;
#25194=CARTESIAN_POINT ( 'NONE',  ( -0.7742782152230965886, 0.05413385826771666132, 0.4176697321401328100 ) ) ;
#25195=CARTESIAN_POINT ( 'NONE',  ( 1.548556430446194954, -0.6046776061558807314, 0.2411417322834647770 ) ) ;
#25198=CARTESIAN_POINT ( 'NONE',  ( 1.069553805774278832, 0.2952755905511810774, -0.1292274648535930714 ) ) ;
#25199=CARTESIAN_POINT ( 'NONE',  ( 0.1640419947506569498, -0.3162353388693409650, -0.4822834645669289433 ) ) ;
#25202=CARTESIAN_POINT ( 'NONE',  ( 1.023622047244095112, -0.1870078740157480601, -0.3641732283464567677 ) ) ;
#25206=EDGE_LOOP ( 'NONE', ( #25036, #49928, #24401, #58970 ) ) ;
#25207=CARTESIAN_POINT ( 'NONE',  ( 0.3674540682414705883, 0.2306618581243847221, -0.2411417322834647770 ) ) ;
#25208=CARTESIAN_POINT ( 'NONE',  ( -0.8858267716535425107, 0.1660481256975883668, -0.3530559997133364547 ) ) ;
#25209=CARTESIAN_POINT ( 'NONE',  ( -1.627296587926508442, 0.2306618581243848609, 0.2411417322834645549 ) ) ;
#25210=CARTESIAN_POINT ( 'NONE',  ( 0.4855643044619430415, -0.4281496062992127816, -0.4176697321401328100 ) ) ;
#25211=CARTESIAN_POINT ( 'NONE',  ( -1.555118110236219930, -0.4536011799217368745, -0.2665933059059886201 ) ) ;
#25212=CARTESIAN_POINT ( 'NONE',  ( 1.489501312335958172, -0.05778040916215560624, -0.4822834645669293319 ) ) ;
#25213=CARTESIAN_POINT ( 'NONE',  ( 0.06561679790026316017, -0.4281496062992124485, 0.4176697321401328655 ) ) ;
#25214=CARTESIAN_POINT ( 'NONE',  ( -1.397637795275589623, -0.5400638737290845981, -0.3530559997133363437 ) ) ;
#25215=CARTESIAN_POINT ( 'NONE',  ( 1.279527559055118724, 0.1660481256975885056, 0.3530559997133364547 ) ) ;
#25218=CARTESIAN_POINT ( 'NONE',  ( 0.9120734908136490793, 0.1771653543307087075, -0.09757992244046823083 ) ) ;
#25222=CARTESIAN_POINT ( 'NONE',  ( 0.06561679790026316017, -0.004921259842519870586, -0.3153832671262229437 ) ) ;
#25225=CARTESIAN_POINT ( 'NONE',  ( 0.1049868766404206816, -0.6046776061558809534, -0.2411417322834644161 ) ) ;
#25226=CARTESIAN_POINT ( 'NONE',  ( 0.3805774278215230400, 0.05413385826771626580, -0.4176697321401330321 ) ) ;
#25227=CARTESIAN_POINT ( 'NONE',  ( -0.5905511811023615998, 0.2952755905511811885, 0.000000000000000000 ) ) ;
#25229=CARTESIAN_POINT ( 'NONE',  ( -1.312335958005248715, 0.2306618581243848609, 0.2411417322834645549 ) ) ;
#25231=CARTESIAN_POINT ( 'NONE',  ( 1.312335958005249825, 0.1283753931104746893, -0.1820866141732285504 ) ) ;
#25232=CARTESIAN_POINT ( 'NONE',  ( 0.7545931758530189937, 0.2952755905511810774, -0.1292274648535930714 ) ) ;
#25233=CARTESIAN_POINT ( 'NONE',  ( 0.5774278215223104249, 0.2306618581243848609, 0.2411417322834645549 ) ) ;
#25235=CARTESIAN_POINT ( 'NONE',  ( -1.450131233595799651, -0.6692913385826771977, 0.1292274648535927661 ) ) ;
#25238=CARTESIAN_POINT ( 'NONE',  ( -0.2165354330708654795, -0.5400638737290845981, -0.3530559997133363437 ) ) ;
#25241=CARTESIAN_POINT ( 'NONE',  ( 1.200787401574803681, -0.5400638737290845981, -0.3530559997133363437 ) ) ;
#25242=AXIS2_PLACEMENT_3D ( 'NONE', #68581, #23539, #29447 ) ;
#25243=CARTESIAN_POINT ( 'NONE',  ( 1.548556430446194954, 0.2306618581243847221, -0.2411417322834647770 ) ) ;
#25244=CARTESIAN_POINT ( 'NONE',  ( -0.01968503937007793844, 0.07958543189024071263, -0.2665933059059888421 ) ) ;
#25245=CARTESIAN_POINT ( 'NONE',  ( 1.010498687664042716, 0.05413385826771626580, -0.4176697321401330321 ) ) ;
#25247=CARTESIAN_POINT ( 'NONE',  ( 0.5511811023622055217, -0.1870078740157479769, 0.3641732283464567677 ) ) ;
#25248=CARTESIAN_POINT ( 'NONE',  ( 0.2034120734908142214, 0.2952755905511810774, -0.1292274648535930714 ) ) ;
#25251=CARTESIAN_POINT ( 'NONE',  ( -1.358267716535432434, 0.1660481256975883668, -0.3530559997133364547 ) ) ;
#25252=CARTESIAN_POINT ( 'NONE',  ( 0.8661417322834652488, -0.1870078740157480601, -0.3641732283464567677 ) ) ;
#25254=CARTESIAN_POINT ( 'NONE',  ( -0.3805774278215216522, -0.4281496062992127816, -0.4176697321401328100 ) ) ;
#25255=CARTESIAN_POINT ( 'NONE',  ( 0.01968503937007957949, -0.4536011799217368745, -0.2665933059059886201 ) ) ;
#25257=CARTESIAN_POINT ( 'NONE',  ( -0.3346456692913377662, -0.5400638737290844871, 0.3530559997133364547 ) ) ;
#25258=CARTESIAN_POINT ( 'NONE',  ( 0.1771653543307093182, 0.07958543189024085140, 0.2665933059059887866 ) ) ;
#25260=CARTESIAN_POINT ( 'NONE',  ( -0.2099737532808391705, 0.2306618581243848609, 0.2411417322834645549 ) ) ;
#25261=CARTESIAN_POINT ( 'NONE',  ( 1.233595800524935227, 0.1283753931104746893, -0.1820866141732285504 ) ) ;
#25262=CARTESIAN_POINT ( 'NONE',  ( 0.2246346060905436703, 0.02791078216816508459, -0.4328096321851889194 ) ) ;
#25263=CARTESIAN_POINT ( 'NONE',  ( -0.1902887139107604098, -0.5511811023622046335, 0.09757992244046803654 ) ) ;
#25264=CARTESIAN_POINT ( 'NONE',  ( -0.7020997375328076329, -0.2845877964562161244, -0.3641732283464567121 ) ) ;
#25265=CARTESIAN_POINT ( 'NONE',  ( -0.1443569553805765515, -0.4281496062992127816, -0.4176697321401328100 ) ) ;
#25266=CARTESIAN_POINT ( 'NONE',  ( 0.07874015748031558404, -0.1870078740157480879, -0.4822834645669291653 ) ) ;
#25267=CARTESIAN_POINT ( 'NONE',  ( 1.122047244094488860, -0.4536011799217368745, -0.2665933059059886201 ) ) ;
#25269=CARTESIAN_POINT ( 'NONE',  ( 1.535433070866142335, -0.5511811023622047445, 6.969142054262312111E-17 ) ) ;
#25270=CARTESIAN_POINT ( 'NONE',  ( 0.5511811023622055217, -0.1870078740157479769, 0.4822834645669291653 ) ) ;
#25272=CARTESIAN_POINT ( 'NONE',  ( -0.2755905511811018171, 0.2952755905511811885, 0.000000000000000000 ) ) ;
#25274=CARTESIAN_POINT ( 'NONE',  ( 0.9055118110236227702, 0.2952755905511811885, 0.000000000000000000 ) ) ;
#25275=CARTESIAN_POINT ( 'NONE',  ( 0.5839895013123367340, 0.2952755905511811885, 0.1292274648535926551 ) ) ;
#25277=CARTESIAN_POINT ( 'NONE',  ( 0.2887139107611556010, 0.1283753931104746893, -0.1820866141732285504 ) ) ;
#25278=CARTESIAN_POINT ( 'NONE',  ( 1.233595800524935227, 0.2306618581243847221, -0.2411417322834647770 ) ) ;
#25279=CARTESIAN_POINT ( 'NONE',  ( -0.4527559055118102749, 0.07958543189024085140, 0.2665933059059887866 ) ) ;
#25280=CARTESIAN_POINT ( 'NONE',  ( -0.6233595800524928121, -0.3162353388693409650, -0.4822834645669289433 ) ) ;
#25282=CARTESIAN_POINT ( 'NONE',  ( 0.1902887139107617975, 0.2952755905511811885, 0.1292274648535926551 ) ) ;
#25283=CARTESIAN_POINT ( 'NONE',  ( -0.9120734908136475250, -0.6692913385826773087, -0.1292274648535924053 ) ) ;
#25284=CARTESIAN_POINT ( 'NONE',  ( -0.4921259842519677963, -0.4536011799217367080, 0.2665933059059888421 ) ) ;
#25285=CARTESIAN_POINT ( 'NONE',  ( 0.3937007874015754361, -0.1870078740157480879, -0.4822834645669291653 ) ) ;
#25286=CARTESIAN_POINT ( 'NONE',  ( -1.095800524934382292, -0.05778040916215522460, 0.4822834645669289988 ) ) ;
#25287=CARTESIAN_POINT ( 'NONE',  ( -0.5052493438320203589, 0.2952755905511810774, -0.1292274648535930714 ) ) ;
#25288=( BOUNDED_CURVE ( )  B_SPLINE_CURVE ( 2, ( #72496, #28701, #21557, #35850, #46805, #73330, #80075, #14845, #61519, #59854, #2206, #79242, #47218 ),
 .UNSPECIFIED., .F., .F. ) 
 B_SPLINE_CURVE_WITH_KNOTS ( ( 3, 2, 2, 2, 2, 2, 3 ),
 ( 0.1853969023887781231, 0.1856060606060606633, 0.1893939393939394478, 0.1931818181818182323, 0.1969696969696970168, 0.2007575757575758013, 0.2009667339748583414 ),
 .UNSPECIFIED. ) 
 CURVE ( )  GEOMETRIC_REPRESENTATION_ITEM ( )  RATIONAL_B_SPLINE_CURVE ( ( 0.9964447847208416364, 0.9981185001348089614, 1.000000000000000000, 0.9659258262890683122, 1.000000000000000000, 0.9659258262890683122, 1.000000000000000000, 0.9659258262890683122, 1.000000000000000000, 0.9659258262890683122, 1.000000000000000000, 0.9981185001348089614, 0.9964447847208417475 ) ) 
 REPRESENTATION_ITEM ( '' )  );
#25291=CARTESIAN_POINT ( 'NONE',  ( 1.515748031496063186, -0.5400638737290845981, -0.3530559997133363437 ) ) ;
#25292=CARTESIAN_POINT ( 'NONE',  ( 1.220472440944882608, 0.2952755905511811885, 0.000000000000000000 ) ) ;
#25295=CARTESIAN_POINT ( 'NONE',  ( -1.102362204724408601, -0.1870078740157479769, 0.4822834645669291653 ) ) ;
#25299=CARTESIAN_POINT ( 'NONE',  ( -0.09842519685039295696, -0.4536011799217367080, 0.2665933059059888421 ) ) ;
#25301=B_SPLINE_CURVE_WITH_KNOTS ( 'NONE', 3,
 ( #40241, #78138, #47372, #33093 ),
 .UNSPECIFIED., .F., .F.,
 ( 4, 4 ),
 ( 1.999999999910059834E-07, 0.006970199999999934261 ),
 .UNSPECIFIED. ) ;
#25302=CARTESIAN_POINT ( 'NONE',  ( 0.5511811023622054106, -0.1870078740157480879, -0.4822834645669291653 ) ) ;
#25305=CARTESIAN_POINT ( 'NONE',  ( -0.5446194225721777693, -0.08942795157527998196, 0.3641732283464567121 ) ) ;
#25307=CARTESIAN_POINT ( 'NONE',  ( 1.318897637795276356, -0.5400638737290844871, 0.3530559997133364547 ) ) ;
#25309=CARTESIAN_POINT ( 'NONE',  ( 1.049868766404200127, -0.5023911411419708095, -0.1820866141732282451 ) ) ;
#25310=CARTESIAN_POINT ( 'NONE',  ( -0.1312335958005241554, -0.6046776061558809534, -0.2411417322834644161 ) ) ;
#25312=CARTESIAN_POINT ( 'NONE',  ( -0.5446194225721777693, -0.05778040916215522460, 0.4822834645669289988 ) ) ;
#25313=CARTESIAN_POINT ( 'NONE',  ( -1.174540682414697335, -0.2845877964562161244, -0.3641732283464567121 ) ) ;
#25314=CARTESIAN_POINT ( 'NONE',  ( -0.5446194225721777693, -0.3162353388693409650, -0.4822834645669289433 ) ) ;
#25319=CARTESIAN_POINT ( 'NONE',  ( 0.4921259842519691285, -0.5400638737290845981, -0.3530559997133363437 ) ) ;
#25321=CARTESIAN_POINT ( 'NONE',  ( -0.9448818897637790704, -0.1870078740157479769, 0.4822834645669291653 ) ) ;
#25322=CARTESIAN_POINT ( 'NONE',  ( 1.213910761154856299, -0.6692913385826773087, -0.1292274648535924053 ) ) ;
#25323=CARTESIAN_POINT ( 'NONE',  ( 0.8661417322834652488, -0.1870078740157480879, -0.4822834645669291653 ) ) ;
#25324=CARTESIAN_POINT ( 'NONE',  ( 0.03937007874015833325, -0.6692913385826771977, 8.415575281601705876E-17 ) ) ;
#25326=CARTESIAN_POINT ( 'NONE',  ( -0.5905511811023615998, 0.2952755905511811885, 0.000000000000000000 ) ) ;
#25327=CARTESIAN_POINT ( 'NONE',  ( -0.1902887139107604098, 0.2952755905511810774, -0.1292274648535930714 ) ) ;
#25328=CARTESIAN_POINT ( 'NONE',  ( -1.049868766404198794, -0.6046776061558807314, 0.2411417322834647770 ) ) ;
#25329=CARTESIAN_POINT ( 'NONE',  ( -0.09186351706036663400, -0.3690944881889763329, 0.3153832671262228327 ) ) ;
#25331=CARTESIAN_POINT ( 'NONE',  ( -0.1837270341207343505, -0.6046776061558807314, 0.2411417322834647770 ) ) ;
#25333=ADVANCED_FACE ( 'NONE', ( #53312 ), #16288, .F. ) ;
#25334=CARTESIAN_POINT ( 'NONE',  ( 1.286089238845145033, 0.2306618581243848609, 0.2411417322834645549 ) ) ;
#25336=ORIENTED_EDGE ( 'NONE', *, *, #24369, .T. ) ;
#25339=CARTESIAN_POINT ( 'NONE',  ( 0.1049868766404206816, 0.2306618581243848609, 0.2411417322834645549 ) ) ;
#25340=CARTESIAN_POINT ( 'NONE',  ( -0.3740157480314953431, -0.4536011799217368745, -0.2665933059059886201 ) ) ;
#25341=CARTESIAN_POINT ( 'NONE',  ( 1.325459317585302665, -0.3690944881889763329, 0.3153832671262228327 ) ) ;
#25345=CARTESIAN_POINT ( 'NONE',  ( 1.555118110236221041, 0.07958543189024071263, -0.2665933059059888421 ) ) ;
#25346=CARTESIAN_POINT ( 'NONE',  ( 1.587926509186352142, 0.05413385826771666132, 0.4176697321401328100 ) ) ;
#25348=CARTESIAN_POINT ( 'NONE',  ( 0.6430446194225728496, 0.05413385826771666132, 0.4176697321401328100 ) ) ;
#25349=CARTESIAN_POINT ( 'NONE',  ( -1.233595800524933894, -0.6046776061558809534, -0.2411417322834644161 ) ) ;
#25350=CARTESIAN_POINT ( 'NONE',  ( -1.305774278215222184, -0.6692913385826773087, -0.1292274648535924053 ) ) ;
#25351=CARTESIAN_POINT ( 'NONE',  ( 0.3018372703412079971, -0.4281496062992124485, 0.4176697321401328655 ) ) ;
#25353=CARTESIAN_POINT ( 'NONE',  ( -1.607611548556429737, 0.1771653543307087075, -0.09757992244046823083 ) ) ;
#25354=CARTESIAN_POINT ( 'NONE',  ( 0.9973753280839902091, 0.2306618581243847221, -0.2411417322834647770 ) ) ;
#25355=CARTESIAN_POINT ( 'NONE',  ( 1.397637795275591177, 0.07958543189024071263, -0.2665933059059888421 ) ) ;
#25357=CARTESIAN_POINT ( 'NONE',  ( 0.8530183727034128527, -0.3690944881889763329, 0.3153832671262228327 ) ) ;
#25358=CARTESIAN_POINT ( 'NONE',  ( -0.9448818897637790704, -0.1870078740157480879, -0.4822834645669291653 ) ) ;
#25360=CARTESIAN_POINT ( 'NONE',  ( 1.522309711286089939, 0.2306618581243848609, 0.2411417322834645549 ) ) ;
#25362=CARTESIAN_POINT ( 'NONE',  ( 0.6299212598425204535, -0.1870078740157480879, -0.4822834645669291653 ) ) ;
#25364=CARTESIAN_POINT ( 'NONE',  ( -1.482939632545930975, -0.3690944881889765550, -0.3153832671262227771 ) ) ;
#25365=CARTESIAN_POINT ( 'NONE',  ( -0.01312335958005186876, 0.05413385826771626580, -0.4176697321401330321 ) ) ;
#25366=CARTESIAN_POINT ( 'NONE',  ( 1.049868766404200127, -0.5023911411419708095, -0.1820866141732282451 ) ) ;
#25367=CARTESIAN_POINT ( 'NONE',  ( 0.9317585301837276734, 0.05413385826771626580, -0.4176697321401330321 ) ) ;
#25369=CARTESIAN_POINT ( 'NONE',  ( -0.3346456692913377662, -0.4536011799217367080, 0.2665933059059888421 ) ) ;
#25370=CARTESIAN_POINT ( 'NONE',  ( -0.5577427821522301654, -0.05778040916215560624, -0.4822834645669293319 ) ) ;
#25371=CARTESIAN_POINT ( 'NONE',  ( 1.660104986876641320, -0.05778040916215522460, 0.4822834645669289988 ) ) ;
#25372=CARTESIAN_POINT ( 'NONE',  ( -1.010498687664041384, -0.4281496062992127816, -0.4176697321401328100 ) ) ;
#25373=CARTESIAN_POINT ( 'NONE',  ( 1.030183727034121421, -0.05778040916215522460, 0.4822834645669289988 ) ) ;
#25375=CARTESIAN_POINT ( 'NONE',  ( -1.469816272965878357, 0.1283753931104748280, 0.1820866141732283561 ) ) ;
#25376=CARTESIAN_POINT ( 'NONE',  ( -0.7426113562971995430, 1.972848275015057995, -0.5309055118110235227 ) ) ;
#25377=CARTESIAN_POINT ( 'NONE',  ( 1.128608923884514947, 0.2306618581243848609, 0.2411417322834645549 ) ) ;
#25379=CARTESIAN_POINT ( 'NONE',  ( -1.489501312335957062, -0.3162353388693409650, -0.4822834645669289433 ) ) ;
#25380=CARTESIAN_POINT ( 'NONE',  ( 1.614173228346457378, -0.6692913385826771977, 8.415575281601705876E-17 ) ) ;
#25381=CARTESIAN_POINT ( 'NONE',  ( -1.154855643044618851, -0.5023911411419708095, -0.1820866141732282451 ) ) ;
#25382=CARTESIAN_POINT ( 'NONE',  ( 1.581364829396326277, -0.2845877964562161244, -0.3641732283464567121 ) ) ;
#25383=CARTESIAN_POINT ( 'NONE',  ( -0.4265091863517051496, -0.6692913385826771977, 0.1292274648535927661 ) ) ;
#25384=CARTESIAN_POINT ( 'NONE',  ( -0.2952755905511803003, -0.4536011799217368745, -0.2665933059059886201 ) ) ;
#25385=CARTESIAN_POINT ( 'NONE',  ( -1.692913385826770645, 0.1771653543307087630, 0.000000000000000000 ) ) ;
#25386=CARTESIAN_POINT ( 'NONE',  ( 1.023622047244095112, -0.1870078740157480601, -0.3641732283464567677 ) ) ;
#25387=CARTESIAN_POINT ( 'NONE',  ( 0.9383202099737538715, -0.05778040916215560624, -0.4822834645669293319 ) ) ;
#25388=CARTESIAN_POINT ( 'NONE',  ( 1.404199475065617264, -0.4281496062992124485, 0.4176697321401328655 ) ) ;
#25389=CARTESIAN_POINT ( 'NONE',  ( 0.1443569553805781891, -0.004921259842519870586, -0.3153832671262229437 ) ) ;
#25390=CARTESIAN_POINT ( 'NONE',  ( 0.6299212598425204535, -0.1870078740157480879, -0.4822834645669291653 ) ) ;
#25391=CARTESIAN_POINT ( 'NONE',  ( 0.5183727034120741983, 0.1771653543307087075, -0.09757992244046823083 ) ) ;
#25392=CARTESIAN_POINT ( 'NONE',  ( 1.489501312335958172, -0.05778040916215560624, -0.4822834645669293319 ) ) ;
#25393=ADVANCED_FACE ( 'NONE', ( #60052 ), #18326, .T. ) ;
#25394=CARTESIAN_POINT ( 'NONE',  ( -1.253280839895012377, -0.3162353388693409650, -0.4822834645669289433 ) ) ;
#25395=CARTESIAN_POINT ( 'NONE',  ( -0.4855643044619415427, -0.4281496062992124485, 0.4176697321401328655 ) ) ;
#25398=CARTESIAN_POINT ( 'NONE',  ( 0.5774278215223103139, -0.6046776061558809534, -0.2411417322834644161 ) ) ;
#25399=CARTESIAN_POINT ( 'NONE',  ( 0.9580052493438326877, -0.004921259842519576551, 0.3153832671262227771 ) ) ;
#25400=CARTESIAN_POINT ( 'NONE',  ( -0.4527559055118102749, -0.5400638737290845981, -0.3530559997133363437 ) ) ;
#25401=CARTESIAN_POINT ( 'NONE',  ( 0.3215223097112867578, -0.05778040916215522460, 0.4822834645669289988 ) ) ;
#25402=VECTOR ( 'NONE', #39854, 39.37007874015748143 ) ;
#25408=CARTESIAN_POINT ( 'NONE',  ( -1.043307086614172707, 0.07958543189024071263, -0.2665933059059888421 ) ) ;
#25409=CARTESIAN_POINT ( 'NONE',  ( -1.358267716535432434, 0.1660481256975883668, -0.3530559997133364547 ) ) ;
#25411=CARTESIAN_POINT ( 'NONE',  ( 0.7939632545931766261, -0.3162353388693409650, -0.4822834645669289433 ) ) ;
#25412=CARTESIAN_POINT ( 'NONE',  ( 1.338582677165355062, -0.1870078740157480879, -0.4822834645669291653 ) ) ;
#25413=CARTESIAN_POINT ( 'NONE',  ( 0.9317585301837276734, -0.4281496062992124485, 0.4176697321401328655 ) ) ;
#25416=CARTESIAN_POINT ( 'NONE',  ( 1.666666666666667185, 0.05413385826771666132, 0.4176697321401328100 ) ) ;
#25417=CARTESIAN_POINT ( 'NONE',  ( 0.4265091863517067039, -0.6692913385826773087, -0.1292274648535924053 ) ) ;
#25418=CARTESIAN_POINT ( 'NONE',  ( 0.5708661417322841158, -0.5400638737290845981, -0.3530559997133363437 ) ) ;
#25419=CARTESIAN_POINT ( 'NONE',  ( 0.7808398950131240079, -0.2845877964562159024, 0.3641732283464567677 ) ) ;
#25420=CARTESIAN_POINT ( 'NONE',  ( 1.509186351706037543, 0.05413385826771666132, 0.4176697321401328100 ) ) ;
#25422=CARTESIAN_POINT ( 'NONE',  ( 0.6036745406824153282, -0.6046776061558807314, 0.2411417322834647770 ) ) ;
#25423=CARTESIAN_POINT ( 'NONE',  ( 1.148293963254593875, -0.6692913385826771977, 0.1292274648535927661 ) ) ;
#25424=CARTESIAN_POINT ( 'NONE',  ( 0.2427821522309719648, -0.05778040916215522460, 0.4822834645669289988 ) ) ;
#25425=CARTESIAN_POINT ( 'NONE',  ( 1.345144356955381593, -0.08942795157527998196, 0.3641732283464567121 ) ) ;
#25426=CARTESIAN_POINT ( 'NONE',  ( -0.7545931758530177724, 0.2952755905511811885, 0.1292274648535926551 ) ) ;
#25427=CARTESIAN_POINT ( 'NONE',  ( -0.9908136482939626788, -0.6692913385826773087, -0.1292274648535924053 ) ) ;
#25428=CARTESIAN_POINT ( 'NONE',  ( 1.187664041994751285, -0.3162353388693409650, -0.4822834645669289433 ) ) ;
#25432=VERTEX_POINT ( 'NONE', #54556 ) ;
#25435=CARTESIAN_POINT ( 'NONE',  ( 1.489501312335958172, -0.3162353388693405765, 0.4822834645669290543 ) ) ;
#25436=CARTESIAN_POINT ( 'NONE',  ( 1.259842519685040019, -0.1870078740157479769, 0.3641732283464567677 ) ) ;
#25438=CARTESIAN_POINT ( 'NONE',  ( 1.496062992125985147, -0.1870078740157479769, 0.3641732283464567677 ) ) ;
#25440=CARTESIAN_POINT ( 'NONE',  ( -0.09032602383071618168, 0.02791078216816508459, -0.4328096321851889194 ) ) ;
#25443=CARTESIAN_POINT ( 'NONE',  ( -0.5839895013123351797, -0.5511811023622046335, 0.09757992244046803654 ) ) ;
#25444=CARTESIAN_POINT ( 'NONE',  ( -1.535433070866141225, 0.1771653543307087630, 0.000000000000000000 ) ) ;
#25446=CARTESIAN_POINT ( 'NONE',  ( -1.187664041994749731, -0.3162353388693405765, 0.4822834645669290543 ) ) ;
#25447=CARTESIAN_POINT ( 'NONE',  ( 0.1246719160104994284, -0.6692913385826771977, 0.1292274648535927661 ) ) ;
#25448=CARTESIAN_POINT ( 'NONE',  ( 1.515748031496063186, -0.5400638737290845981, -0.3530559997133363437 ) ) ;
#25449=ORIENTED_EDGE ( 'NONE', *, *, #43371, .F. ) ;
#25450=CARTESIAN_POINT ( 'NONE',  ( -1.167979002624671248, 0.009842519685039467087, 0.3409548833797002021 ) ) ;
#25452=CARTESIAN_POINT ( 'NONE',  ( -1.614173228346457378, 1.543375672658094944, 0.1372047244094476981 ) ) ;
#25453=CARTESIAN_POINT ( 'NONE',  ( -0.6824146981627288167, 0.1283753931104748280, 0.1820866141732283561 ) ) ;
#25454=CARTESIAN_POINT ( 'NONE',  ( -1.305774278215222184, 0.2952755905511811885, 0.1292274648535926551 ) ) ;
#25455=CARTESIAN_POINT ( 'NONE',  ( 1.213910761154856299, 0.2952755905511811885, 0.1292274648535926551 ) ) ;
#25456=ORIENTED_EDGE ( 'NONE', *, *, #38303, .T. ) ;
#25457=CARTESIAN_POINT ( 'NONE',  ( -0.08874907683609993547, 8.471767977567108961E-16, -0.4445507791589058955 ) ) ;
#25460=CARTESIAN_POINT ( 'NONE',  ( 1.069553805774278832, 0.2952755905511810774, -0.1292274648535930714 ) ) ;
#25461=CARTESIAN_POINT ( 'NONE',  ( -1.417322834645668772, -0.1870078740157479769, 0.4822834645669291653 ) ) ;
#25463=CARTESIAN_POINT ( 'NONE',  ( -0.4658792650918627265, -0.08942795157527998196, 0.3641732283464567121 ) ) ;
#25465=ADVANCED_FACE ( 'NONE', ( #54139 ), #15879, .T. ) ;
#25466=CARTESIAN_POINT ( 'NONE',  ( -0.3083989501312330295, -0.2845877964562161244, -0.3641732283464567121 ) ) ;
#25467=CARTESIAN_POINT ( 'NONE',  ( 0.02624671916010564918, 0.1283753931104748280, 0.1820866141732283561 ) ) ;
#25468=CARTESIAN_POINT ( 'NONE',  ( -0.05249343832020938322, -0.6046776061558809534, -0.2411417322834644161 ) ) ;
#25469=CARTESIAN_POINT ( 'NONE',  ( -0.8070866141732276899, 0.07958543189024071263, -0.2665933059059888421 ) ) ;
#25471=CARTESIAN_POINT ( 'NONE',  ( 1.161417322834646271, 0.1660481256975883668, -0.3530559997133364547 ) ) ;
#25472=CARTESIAN_POINT ( 'NONE',  ( -1.292650918635170010, 0.2952755905511810774, -0.1292274648535930714 ) ) ;
#25474=CARTESIAN_POINT ( 'NONE',  ( -0.4002624671916004129, -0.05778040916215560624, -0.4822834645669293319 ) ) ;
#25475=CARTESIAN_POINT ( 'NONE',  ( -0.7611548556430438595, -0.6046776061558809534, -0.2411417322834644161 ) ) ;
#25476=CARTESIAN_POINT ( 'NONE',  ( 1.069553805774278832, 0.1771653543307087075, -0.09757992244046823083 ) ) ;
#25477=CARTESIAN_POINT ( 'NONE',  ( -0.4396325459317579898, 0.1771653543307087630, 0.09757992244046791164 ) ) ;
#25478=CARTESIAN_POINT ( 'NONE',  ( -0.5905511811023615998, 0.2952755905511811885, 0.000000000000000000 ) ) ;
#25479=CARTESIAN_POINT ( 'NONE',  ( -1.305774278215222184, 0.2952755905511811885, 0.1292274648535926551 ) ) ;
#25481=CARTESIAN_POINT ( 'NONE',  ( 1.128608923884515169, -0.5023911411419708095, -0.1820866141732282451 ) ) ;
#25482=CARTESIAN_POINT ( 'NONE',  ( -0.3280839895013117347, 0.05413385826771626580, -0.4176697321401330321 ) ) ;
#25483=CARTESIAN_POINT ( 'NONE',  ( -1.358267716535432434, 0.1660481256975883668, -0.3530559997133364547 ) ) ;
#25485=EDGE_CURVE ( 'NONE', #77295, #21005, #69245, .T. ) ;
#25487=CARTESIAN_POINT ( 'NONE',  ( -0.9383202099737524282, -0.2845877964562161244, -0.3641732283464567121 ) ) ;
#25488=CARTESIAN_POINT ( 'NONE',  ( 0.8792650918635177559, -0.4281496062992127816, -0.4176697321401328100 ) ) ;
#25489=CARTESIAN_POINT ( 'NONE',  ( -0.8989501312335946848, 0.1771653543307087075, -0.09757992244046823083 ) ) ;
#25491=CARTESIAN_POINT ( 'NONE',  ( -1.108923884514435132, -0.3162353388693405765, 0.4822834645669290543 ) ) ;
#25492=CARTESIAN_POINT ( 'NONE',  ( 0.8005249343832028242, -0.4281496062992127816, -0.4176697321401328100 ) ) ;
#25493=CARTESIAN_POINT ( 'NONE',  ( 0.2952755905511819101, 0.1660481256975883668, -0.3530559997133364547 ) ) ;
#25494=CARTESIAN_POINT ( 'NONE',  ( 1.502624671916010790, -0.3162353388693409650, -0.4822834645669289433 ) ) ;
#25495=CARTESIAN_POINT ( 'NONE',  ( -1.548556430446193399, 0.1283753931104748280, 0.1820866141732283561 ) ) ;
#25501=CARTESIAN_POINT ( 'NONE',  ( 1.161417322834646493, -0.4536011799217367080, 0.2665933059059888421 ) ) ;
#25502=CARTESIAN_POINT ( 'NONE',  ( 0.5905511811023629321, -0.5511811023622047445, 6.969142054262312111E-17 ) ) ;
#25503=CARTESIAN_POINT ( 'NONE',  ( 0.1509186351706042484, -0.3162353388693405765, 0.4822834645669290543 ) ) ;
#25506=CARTESIAN_POINT ( 'NONE',  ( 0.3280839895013130669, -0.3690944881889765550, -0.3153832671262227771 ) ) ;
#25508=CARTESIAN_POINT ( 'NONE',  ( -0.7152230971128602510, -0.3162353388693405765, 0.4822834645669290543 ) ) ;
#25509=CARTESIAN_POINT ( 'NONE',  ( -1.167979002624671470, 0.05413385826771666132, 0.4176697321401328100 ) ) ;
#25510=CARTESIAN_POINT ( 'NONE',  ( 0.7217847769028878924, 0.05413385826771666132, 0.4176697321401328100 ) ) ;
#25514=ORIENTED_EDGE ( 'NONE', *, *, #49009, .F. ) ;
#25515=CARTESIAN_POINT ( 'NONE',  ( -1.233595800524933894, 0.2306618581243848609, 0.2411417322834645549 ) ) ;
#25516=CARTESIAN_POINT ( 'NONE',  ( -0.4330708661417315697, -0.6692913385826771977, 8.415575281601705876E-17 ) ) ;
#25517=CARTESIAN_POINT ( 'NONE',  ( -0.7545931758530176614, -0.5511811023622048555, -0.09757992244046775898 ) ) ;
#25518=CARTESIAN_POINT ( 'NONE',  ( -0.8398950131233585692, 0.2306618581243848609, 0.2411417322834645549 ) ) ;
#25521=CARTESIAN_POINT ( 'NONE',  ( 1.456692913385827515, -0.6692913385826771977, 8.415575281601705876E-17 ) ) ;
#25522=CARTESIAN_POINT ( 'NONE',  ( 1.338582677165355062, -0.1870078740157480879, -0.4822834645669291653 ) ) ;
#25523=CARTESIAN_POINT ( 'NONE',  ( -0.7611548556430438595, 0.2306618581243848609, 0.2411417322834645549 ) ) ;
#25524=CARTESIAN_POINT ( 'NONE',  ( 0.4133858267716541968, -0.5400638737290845981, -0.3530559997133363437 ) ) ;
#25525=CARTESIAN_POINT ( 'NONE',  ( -0.9251968503937002541, -0.5400638737290845981, -0.3530559997133363437 ) ) ;
#25527=CARTESIAN_POINT ( 'NONE',  ( -0.8398950131233585692, 0.1283753931104748280, 0.1820866141732283561 ) ) ;
#25530=ORIENTED_EDGE ( 'NONE', *, *, #37828, .F. ) ;
#25531=LINE ( 'NONE', #58354, #51561 ) ;
#25532=CARTESIAN_POINT ( 'NONE',  ( -0.9711286089238838626, 0.2306618581243847221, -0.2411417322834647770 ) ) ;
#25533=CARTESIAN_POINT ( 'NONE',  ( -1.076115485564303809, -0.6046776061558809534, -0.2411417322834644161 ) ) ;
#25535=CARTESIAN_POINT ( 'NONE',  ( -1.187664041994750175, -0.05778040916215560624, -0.4822834645669293319 ) ) ;
#25536=CARTESIAN_POINT ( 'NONE',  ( -1.187664041994750175, -0.05778040916215560624, -0.4822834645669293319 ) ) ;
#25537=CARTESIAN_POINT ( 'NONE',  ( -1.653543307086613234, -0.1870078740157479769, 0.4822834645669291653 ) ) ;
#25539=CARTESIAN_POINT ( 'NONE',  ( 0.7283464566929143125, 0.07958543189024085140, 0.2665933059059887866 ) ) ;
#25540=CARTESIAN_POINT ( 'NONE',  ( 0.4687364453272602205, 1.550612376216559563, 0.5180075785468909455 ) ) ;
#25542=CARTESIAN_POINT ( 'NONE',  ( -0.4002624671916004129, -0.08942795157528024563, -0.3641732283464568787 ) ) ;
#25543=CARTESIAN_POINT ( 'NONE',  ( -0.6102362204724400829, -0.5400638737290845981, -0.3530559997133363437 ) ) ;
#25544=CARTESIAN_POINT ( 'NONE',  ( 1.417322834645670104, -0.1870078740157479769, 0.4822834645669291653 ) ) ;
#25545=CARTESIAN_POINT ( 'NONE',  ( -0.2952755905511803003, -0.5400638737290845981, -0.3530559997133363437 ) ) ;
#25549=CARTESIAN_POINT ( 'NONE',  ( -0.7480314960629914633, -0.6692913385826771977, 8.415575281601705876E-17 ) ) ;
#25550=CARTESIAN_POINT ( 'NONE',  ( 1.305774278215223960, 0.2952755905511810774, -0.1292274648535930714 ) ) ;
#25551=CARTESIAN_POINT ( 'NONE',  ( -1.305774278215222184, -0.5511811023622048555, -0.09757992244046775898 ) ) ;
#25552=CARTESIAN_POINT ( 'NONE',  ( -1.194225721784776262, 0.05413385826771626580, -0.4176697321401330321 ) ) ;
#25557=CARTESIAN_POINT ( 'NONE',  ( 0.2559055118110243332, 0.1660481256975885056, 0.3530559997133364547 ) ) ;
#25558=CARTESIAN_POINT ( 'NONE',  ( -1.049868766404198794, -0.5023911411419708095, 0.1820866141732285504 ) ) ;
#25559=CARTESIAN_POINT ( 'NONE',  ( -0.9186351706036736120, 0.2306618581243848609, 0.2411417322834645549 ) ) ;
#25561=CARTESIAN_POINT ( 'NONE',  ( -0.9514435695538050464, -0.3162353388693405765, 0.4822834645669290543 ) ) ;
#25562=EDGE_CURVE ( 'NONE', #43155, #74503, #43133, .T. ) ;
#25563=CARTESIAN_POINT ( 'NONE',  ( -1.030183727034119867, -0.05778040916215560624, -0.4822834645669293319 ) ) ;
#25564=CARTESIAN_POINT ( 'NONE',  ( 0.1049868766404206816, -0.6046776061558809534, -0.2411417322834644161 ) ) ;
#25566=CARTESIAN_POINT ( 'NONE',  ( 0.7545931758530188826, -0.5511811023622046335, 0.09757992244046803654 ) ) ;
#25568=CARTESIAN_POINT ( 'NONE',  ( -0.8267716535433065062, -0.5511811023622047445, 6.969142054262312111E-17 ) ) ;
#25569=CARTESIAN_POINT ( 'NONE',  ( 0.8727034120734913358, -0.08942795157527998196, 0.3641732283464567121 ) ) ;
#25570=CARTESIAN_POINT ( 'NONE',  ( 1.371391076115485719, -0.5511811023622048555, -0.09757992244046775898 ) ) ;
#25571=CARTESIAN_POINT ( 'NONE',  ( 1.476377952755906220, 0.1660481256975883668, -0.3530559997133364547 ) ) ;
#25572=CARTESIAN_POINT ( 'NONE',  ( 0.3674540682414705883, -0.5023911411419708095, 0.1820866141732285504 ) ) ;
#25574=CARTESIAN_POINT ( 'NONE',  ( -0.6824146981627288167, 0.2306618581243848609, 0.2411417322834645549 ) ) ;
#25575=CARTESIAN_POINT ( 'NONE',  ( 1.069553805774278610, -0.6692913385826771977, 0.1292274648535927661 ) ) ;
#25577=CARTESIAN_POINT ( 'NONE',  ( -0.1837270341207340729, 0.1283753931104746893, -0.1820866141732285504 ) ) ;
#25579=CARTESIAN_POINT ( 'NONE',  ( 0.2230971128608932319, -0.4281496062992124485, 0.4176697321401328655 ) ) ;
#25580=DIRECTION ( 'NONE',  ( 3.096699300667737957E-16, -1.000000000000000000, 0.000000000000000000 ) ) ;
#25581=CARTESIAN_POINT ( 'NONE',  ( 0.9580052493438326877, -0.004921259842519576551, 0.3153832671262227771 ) ) ;
#25582=CARTESIAN_POINT ( 'NONE',  ( 0.2362204724409456558, -0.1870078740157480601, -0.3641732283464567677 ) ) ;
#25583=CARTESIAN_POINT ( 'NONE',  ( 0.1443569553805781891, 0.05413385826771626580, -0.4176697321401330321 ) ) ;
#25584=CARTESIAN_POINT ( 'NONE',  ( -1.299212598425196097, -0.6692913385826771977, 8.415575281601705876E-17 ) ) ;
#25585=CARTESIAN_POINT ( 'NONE',  ( -0.8858267716535425107, -0.4536011799217367080, 0.2665933059059888421 ) ) ;
#25587=B_SPLINE_CURVE_WITH_KNOTS ( 'NONE', 3,
 ( #71191, #489, #5956, #31626 ),
 .UNSPECIFIED., .F., .F.,
 ( 4, 4 ),
 ( 3.210432057671751052E-07, 0.001287787053611966735 ),
 .UNSPECIFIED. ) ;
#25588=CARTESIAN_POINT ( 'NONE',  ( -0.4986876640419939388, 0.2306618581243847221, -0.2411417322834647770 ) ) ;
#25591=CARTESIAN_POINT ( 'NONE',  ( 0.06561679790026316017, -0.004921259842519870586, -0.3153832671262229437 ) ) ;
#25592=CARTESIAN_POINT ( 'NONE',  ( -0.4461942257217840213, -0.6046776061558809534, -0.2411417322834644161 ) ) ;
#25593=CARTESIAN_POINT ( 'NONE',  ( -1.286089238845143479, 0.2306618581243847221, -0.2411417322834647770 ) ) ;
#25594=CARTESIAN_POINT ( 'NONE',  ( -1.220472440944881054, -0.5511811023622047445, 6.969142054262312111E-17 ) ) ;
#25596=CARTESIAN_POINT ( 'NONE',  ( -0.6036745406824141069, -0.6046776061558809534, -0.2411417322834644161 ) ) ;
#25597=CARTESIAN_POINT ( 'NONE',  ( -1.043307086614172041, -0.4536011799217367080, 0.2665933059059888421 ) ) ;
#25598=CARTESIAN_POINT ( 'NONE',  ( -1.640419947506561060, -0.3690944881889765550, -0.3153832671262227771 ) ) ;
#25599=CARTESIAN_POINT ( 'NONE',  ( 1.167979002624672580, 0.05413385826771626580, -0.4176697321401330321 ) ) ;
#25600=CARTESIAN_POINT ( 'NONE',  ( 2.795275590551181466, 2.204724409448820310, 0.000000000000000000 ) ) ;
#25603=CARTESIAN_POINT ( 'NONE',  ( 1.614173228346457378, 1.055049524192302357, 0.1372047244094478369 ) ) ;
#25604=CARTESIAN_POINT ( 'NONE',  ( -1.535433070866141225, 0.2952755905511811885, 0.000000000000000000 ) ) ;
#25605=CARTESIAN_POINT ( 'NONE',  ( -0.9973753280839886548, -0.6046776061558809534, -0.2411417322834644161 ) ) ;
#25606=CARTESIAN_POINT ( 'NONE',  ( 1.522309711286089939, -0.6046776061558809534, -0.2411417322834644161 ) ) ;
#25609=CARTESIAN_POINT ( 'NONE',  ( 1.135170603674541256, -0.6692913385826773087, -0.1292274648535924053 ) ) ;
#25610=CARTESIAN_POINT ( 'NONE',  ( -0.09842519685039295696, -0.5400638737290844871, 0.3530559997133364547 ) ) ;
#25613=CARTESIAN_POINT ( 'NONE',  ( 1.049868766404200127, -0.5023911411419708095, -0.1820866141732282451 ) ) ;
#25617=ORIENTED_EDGE ( 'NONE', *, *, #30136, .T. ) ;
#25618=CARTESIAN_POINT ( 'NONE',  ( 0.07874015748031558404, -0.1870078740157480879, -0.4822834645669291653 ) ) ;
#25619=CARTESIAN_POINT ( 'NONE',  ( -0.7086614173228339419, -0.1870078740157480879, -0.4822834645669291653 ) ) ;
#25620=CARTESIAN_POINT ( 'NONE',  ( -1.371391076115484609, -0.6692913385826771977, 0.1292274648535927661 ) ) ;
#25621=CARTESIAN_POINT ( 'NONE',  ( 0.5577427821522316087, -0.05778040916215522460, 0.4822834645669289988 ) ) ;
#25622=CARTESIAN_POINT ( 'NONE',  ( 1.430446194225722500, -0.4281496062992127816, -0.4176697321401328100 ) ) ;
#25623=CARTESIAN_POINT ( 'NONE',  ( 1.318897637795276356, 0.1660481256975883668, -0.3530559997133364547 ) ) ;
#25624=CARTESIAN_POINT ( 'NONE',  ( -0.5643044619422565855, -0.4281496062992124485, 0.4176697321401328655 ) ) ;
#25625=CARTESIAN_POINT ( 'NONE',  ( 0.6036745406824153282, -0.6046776061558807314, 0.2411417322834647770 ) ) ;
#25626=CARTESIAN_POINT ( 'NONE',  ( 1.555118110236221041, -0.5400638737290844871, 0.3530559997133364547 ) ) ;
#25627=CARTESIAN_POINT ( 'NONE',  ( 1.423884514435696191, -0.05778040916215522460, 0.4822834645669289988 ) ) ;
#25628=CARTESIAN_POINT ( 'NONE',  ( 1.443569553805774897, -0.6046776061558809534, -0.2411417322834644161 ) ) ;
#25629=CARTESIAN_POINT ( 'NONE',  ( -0.1837270341207343505, -0.6046776061558807314, 0.2411417322834647770 ) ) ;
#25631=CARTESIAN_POINT ( 'NONE',  ( 0.3149606299212606708, -0.1870078740157480601, -0.3641732283464567677 ) ) ;
#25632=VERTEX_POINT ( 'NONE', #68855 ) ;
#25634=ORIENTED_EDGE ( 'NONE', *, *, #40829, .F. ) ;
#25635=CARTESIAN_POINT ( 'NONE',  ( -0.3674540682414692561, -0.5023911411419708095, -0.1820866141732282451 ) ) ;
#25637=CARTESIAN_POINT ( 'NONE',  ( 0.3346456692913390985, 0.1660481256975885056, 0.3530559997133364547 ) ) ;
#25638=CARTESIAN_POINT ( 'NONE',  ( 0.1181102362204730916, -0.6692913385826771977, 8.415575281601705876E-17 ) ) ;
#25639=B_SPLINE_CURVE_WITH_KNOTS ( 'NONE', 3,
 ( #4727, #31221, #56889, #63217 ),
 .UNSPECIFIED., .F., .F.,
 ( 4, 4 ),
 ( 3.210432057682506253E-07, 0.001287787053612032872 ),
 .UNSPECIFIED. ) ;
#25640=CARTESIAN_POINT ( 'NONE',  ( -0.3805774278215216522, -0.4281496062992127816, -0.4176697321401328100 ) ) ;
#25642=CARTESIAN_POINT ( 'NONE',  ( -1.259842519685038686, -0.1870078740157480879, -0.4822834645669291653 ) ) ;
#25644=CARTESIAN_POINT ( 'NONE',  ( 0.6889763779527563470, 0.07958543189024071263, -0.2665933059059888421 ) ) ;
#25645=CARTESIAN_POINT ( 'NONE',  ( 0.6167979002624679463, 0.05413385826771626580, -0.4176697321401330321 ) ) ;
#25646=CARTESIAN_POINT ( 'NONE',  ( 0.9448818897637802916, -0.1870078740157480879, -0.4822834645669291653 ) ) ;
#25649=CARTESIAN_POINT ( 'NONE',  ( -1.463254593175852492, -0.6692913385826773087, -0.1292274648535924053 ) ) ;
#25652=CARTESIAN_POINT ( 'NONE',  ( 0.07874015748031558404, -0.1870078740157480879, -0.4822834645669291653 ) ) ;
#25655=CARTESIAN_POINT ( 'NONE',  ( -1.069553805774277722, -0.5511811023622048555, -0.09757992244046775898 ) ) ;
#25656=CARTESIAN_POINT ( 'NONE',  ( 1.227034120734908917, -0.6692913385826771977, 0.1292274648535927661 ) ) ;
#25657=CARTESIAN_POINT ( 'NONE',  ( 1.463254593175853824, -0.6692913385826771977, 0.1292274648535927661 ) ) ;
#25658=CARTESIAN_POINT ( 'NONE',  ( 0.3083989501312343062, -0.08942795157528024563, -0.3641732283464568787 ) ) ;
#25659=CARTESIAN_POINT ( 'NONE',  ( 0.9842519685039375910, 0.2952755905511811885, 0.000000000000000000 ) ) ;
#25661=CARTESIAN_POINT ( 'NONE',  ( 0.5183727034120741983, -0.5511811023622046335, 0.09757992244046803654 ) ) ;
#25662=( BOUNDED_CURVE ( )  B_SPLINE_CURVE ( 1, ( #49973, #49564 ),
 .UNSPECIFIED., .F., .F. ) 
 B_SPLINE_CURVE_WITH_KNOTS ( ( 2, 2 ),
 ( 5.204170427930421283E-18, 0.002000000000000005246 ),
 .UNSPECIFIED. ) 
 CURVE ( )  GEOMETRIC_REPRESENTATION_ITEM ( )  RATIONAL_B_SPLINE_CURVE ( ( 0.9875488213027523443, 0.9875488213027523443 ) ) 
 REPRESENTATION_ITEM ( '' )  );
#25663=CARTESIAN_POINT ( 'NONE',  ( 0.5905511811023629321, -0.6692913385826771977, 8.415575281601705876E-17 ) ) ;
#25665=CARTESIAN_POINT ( 'NONE',  ( -1.108923884514435132, -0.3162353388693405765, 0.4822834645669290543 ) ) ;
#25666=CARTESIAN_POINT ( 'NONE',  ( 0.3215223097112867578, -0.08942795157527998196, 0.3641732283464567121 ) ) ;
#25669=CARTESIAN_POINT ( 'NONE',  ( -0.1706036745406816491, -0.4281496062992124485, 0.4176697321401328655 ) ) ;
#25670=CARTESIAN_POINT ( 'NONE',  ( -0.2099737532808391705, 0.1283753931104748280, 0.1820866141732283561 ) ) ;
#25672=CARTESIAN_POINT ( 'NONE',  ( -0.4068241469816267775, 0.05413385826771626580, -0.4176697321401330321 ) ) ;
#25673=CARTESIAN_POINT ( 'NONE',  ( 0.2165354330708668673, 0.07958543189024071263, -0.2665933059059888421 ) ) ;
#25675=CARTESIAN_POINT ( 'NONE',  ( -0.1837270341207340729, 0.2306618581243847221, -0.2411417322834647770 ) ) ;
#25677=CARTESIAN_POINT ( 'NONE',  ( 1.082677165354331228, 0.07958543189024071263, -0.2665933059059888421 ) ) ;
#25678=CARTESIAN_POINT ( 'NONE',  ( 0.3836918680457899744, 8.471767977567108961E-16, -0.4445507791589058955 ) ) ;
#25679=CARTESIAN_POINT ( 'NONE',  ( -0.7217847769028863381, -0.004921259842519870586, -0.3153832671262229437 ) ) ;
#25680=CARTESIAN_POINT ( 'NONE',  ( -0.8858267716535425107, 0.07958543189024071263, -0.2665933059059888421 ) ) ;
#25681=CARTESIAN_POINT ( 'NONE',  ( -0.8333333333333323711, 0.2952755905511811885, 0.1292274648535926551 ) ) ;
#25682=CARTESIAN_POINT ( 'NONE',  ( -0.3083989501312330295, -0.05778040916215522460, 0.4822834645669289988 ) ) ;
#25683=CARTESIAN_POINT ( 'NONE',  ( 0.6692913385826778638, -0.5511811023622047445, 6.969142054262312111E-17 ) ) ;
#25685=CARTESIAN_POINT ( 'NONE',  ( 1.345144356955381593, -0.2845877964562161244, -0.3641732283464567121 ) ) ;
#25686=CARTESIAN_POINT ( 'NONE',  ( 0.9514435695538062676, -0.3162353388693409650, -0.4822834645669289433 ) ) ;
#25688=CARTESIAN_POINT ( 'NONE',  ( -0.4068241469816267775, 0.05413385826771626580, -0.4176697321401330321 ) ) ;
#25690=CARTESIAN_POINT ( 'NONE',  ( 1.443569553805774897, 0.1283753931104748280, 0.1820866141732283561 ) ) ;
#25691=CARTESIAN_POINT ( 'NONE',  ( 1.069553805774278832, 0.2952755905511810774, -0.1292274648535930714 ) ) ;
#25692=CARTESIAN_POINT ( 'NONE',  ( 0.1377952755905518800, 0.1660481256975883668, -0.3530559997133364547 ) ) ;
#25694=CARTESIAN_POINT ( 'NONE',  ( 0.5052493438320218022, -0.5511811023622048555, -0.09757992244046775898 ) ) ;
#25695=CARTESIAN_POINT ( 'NONE',  ( 1.128608923884515169, -0.6046776061558809534, -0.2411417322834644161 ) ) ;
#25696=CARTESIAN_POINT ( 'NONE',  ( -0.3412073490813641308, -0.5023911411419708095, 0.1820866141732285504 ) ) ;
#25697=CARTESIAN_POINT ( 'NONE',  ( -0.9055118110236215490, -0.6692913385826771977, 8.415575281601705876E-17 ) ) ;
#25699=CARTESIAN_POINT ( 'NONE',  ( 0.2755905511811031494, -0.6692913385826771977, 8.415575281601705876E-17 ) ) ;
#25700=CARTESIAN_POINT ( 'NONE',  ( -0.9973753280839886548, 0.2306618581243848609, 0.2411417322834645549 ) ) ;
#25701=CARTESIAN_POINT ( 'NONE',  ( -0.7283464566929126471, 0.07958543189024071263, -0.2665933059059888421 ) ) ;
#25703=CARTESIAN_POINT ( 'NONE',  ( 0.5052493438320215802, 0.2952755905511811885, 0.1292274648535926551 ) ) ;
#25704=CARTESIAN_POINT ( 'NONE',  ( -1.049868766404198794, 0.2306618581243847221, -0.2411417322834647770 ) ) ;
#25705=CARTESIAN_POINT ( 'NONE',  ( -0.3674540682414689785, 0.2306618581243848609, 0.2411417322834645549 ) ) ;
#25707=CARTESIAN_POINT ( 'NONE',  ( -0.9337842054690626004, -2.609244250047836720E-15, 0.3954974714151479609 ) ) ;
#25708=CARTESIAN_POINT ( 'NONE',  ( 1.318897637795276356, 0.1660481256975883668, -0.3530559997133364547 ) ) ;
#25709=CARTESIAN_POINT ( 'NONE',  ( 1.332020997375329197, -0.3162353388693405765, 0.4822834645669290543 ) ) ;
#25711=CARTESIAN_POINT ( 'NONE',  ( -1.502624671916009680, -0.3162353388693405765, 0.4822834645669290543 ) ) ;
#25712=CARTESIAN_POINT ( 'NONE',  ( -0.8464566929133852113, -0.5400638737290845981, -0.3530559997133363437 ) ) ;
#25715=ORIENTED_EDGE ( 'NONE', *, *, #24847, .F. ) ;
#25716=CARTESIAN_POINT ( 'NONE',  ( -0.2034120734908128059, 0.1771653543307087630, 0.09757992244046791164 ) ) ;
#25719=CARTESIAN_POINT ( 'NONE',  ( 0.4396325459317590445, -0.6692913385826771977, 0.1292274648535927661 ) ) ;
#25721=CARTESIAN_POINT ( 'NONE',  ( -1.604771003085129655, 1.871396828306225224, -0.1466069496707748387 ) ) ;
#25722=CARTESIAN_POINT ( 'NONE',  ( -0.5577427821522301654, -0.2845877964562159024, 0.3641732283464567677 ) ) ;
#25723=CARTESIAN_POINT ( 'NONE',  ( 0.3280839895013130669, 0.05413385826771666132, 0.4176697321401328100 ) ) ;
#25724=CARTESIAN_POINT ( 'NONE',  ( 1.207349081364829990, 0.2306618581243848609, 0.2411417322834645549 ) ) ;
#25725=CARTESIAN_POINT ( 'NONE',  ( 1.082677165354331228, -0.4536011799217367080, 0.2665933059059888421 ) ) ;
#25726=CARTESIAN_POINT ( 'NONE',  ( 0.1049868766404206816, 0.2306618581243848609, 0.2411417322834645549 ) ) ;
#25728=CARTESIAN_POINT ( 'NONE',  ( -0.8989501312335946848, -0.6692913385826771977, 0.1292274648535927661 ) ) ;
#25729=CARTESIAN_POINT ( 'NONE',  ( -1.450131233595799651, -0.5511811023622046335, 0.09757992244046803654 ) ) ;
#25730=CARTESIAN_POINT ( 'NONE',  ( -0.6102362204724400829, 0.1660481256975885056, 0.3530559997133364547 ) ) ;
#25732=CARTESIAN_POINT ( 'NONE',  ( 1.666666666666667185, -0.004921259842519576551, 0.3153832671262227771 ) ) ;
#25733=ORIENTED_EDGE ( 'NONE', *, *, #64478, .T. ) ;
#25735=CARTESIAN_POINT ( 'NONE',  ( 0.2165354330708668673, -0.5400638737290844871, 0.3530559997133364547 ) ) ;
#25737=CARTESIAN_POINT ( 'NONE',  ( -0.6627296587926503335, -0.6692913385826771977, 0.1292274648535927661 ) ) ;
#25738=CARTESIAN_POINT ( 'NONE',  ( 1.338582677165355062, -0.1870078740157480879, -0.4822834645669291653 ) ) ;
#25739=CARTESIAN_POINT ( 'NONE',  ( 1.115485564304462551, 0.05413385826771666132, 0.4176697321401328100 ) ) ;
#25740=CARTESIAN_POINT ( 'NONE',  ( 0.8595800524934390507, -0.05778040916215560624, -0.4822834645669293319 ) ) ;
#25741=CARTESIAN_POINT ( 'NONE',  ( 0.1115485564304470323, 0.2952755905511811885, 0.1292274648535926551 ) ) ;
#25743=CARTESIAN_POINT ( 'NONE',  ( -1.095800524934382292, -0.05778040916215522460, 0.4822834645669289988 ) ) ;
#25744=CARTESIAN_POINT ( 'NONE',  ( -0.3477690288713902178, 0.2952755905511810774, -0.1292274648535930714 ) ) ;
#25745=CARTESIAN_POINT ( 'NONE',  ( -0.08530183727034056085, -0.2845877964562159024, 0.3641732283464567677 ) ) ;
#25747=CARTESIAN_POINT ( 'NONE',  ( 0.01312335958005323398, 0.05413385826771666132, 0.4176697321401328100 ) ) ;
#25749=CARTESIAN_POINT ( 'NONE',  ( 1.076115485564305141, -0.6046776061558807314, 0.2411417322834647770 ) ) ;
#25752=ADVANCED_FACE ( 'NONE', ( #24637 ), #55794, .F. ) ;
#25754=CARTESIAN_POINT ( 'NONE',  ( 0.2296587926509192634, -0.3162353388693405765, 0.4822834645669290543 ) ) ;
#25755=CARTESIAN_POINT ( 'NONE',  ( -0.1509186351706028884, -0.08942795157527998196, 0.3641732283464567121 ) ) ;
#25756=CARTESIAN_POINT ( 'NONE',  ( 1.332020997375329197, -0.2845877964562159024, 0.3641732283464567677 ) ) ;
#25757=CARTESIAN_POINT ( 'NONE',  ( -0.06724401132814883386, -3.915482057279200494E-15, 0.3791483426435196535 ) ) ;
#25760=CARTESIAN_POINT ( 'NONE',  ( 1.541994750656168645, 0.1771653543307087075, -0.09757992244046823083 ) ) ;
#25761=CARTESIAN_POINT ( 'NONE',  ( -1.502624671916009680, -0.3162353388693405765, 0.4822834645669290543 ) ) ;
#25764=CARTESIAN_POINT ( 'NONE',  ( 0.01968503937007930540, 0.1660481256975885056, 0.3530559997133364547 ) ) ;
#25765=CARTESIAN_POINT ( 'NONE',  ( -1.404199475065615932, -0.4281496062992127816, -0.4176697321401328100 ) ) ;
#25766=CARTESIAN_POINT ( 'NONE',  ( -0.9973753280839886548, -0.6046776061558809534, -0.2411417322834644161 ) ) ;
#25767=CARTESIAN_POINT ( 'NONE',  ( 0.1509186351706042484, -0.3162353388693405765, 0.4822834645669290543 ) ) ;
#25769=CARTESIAN_POINT ( 'NONE',  ( -1.568241469816272105, -0.2845877964562161244, -0.3641732283464567121 ) ) ;
#25770=CARTESIAN_POINT ( 'NONE',  ( 0.9580052493438326877, 0.05413385826771666132, 0.4176697321401328100 ) ) ;
#25771=CARTESIAN_POINT ( 'NONE',  ( 0.9251968503937015864, 0.07958543189024071263, -0.2665933059059888421 ) ) ;
#25772=CARTESIAN_POINT ( 'NONE',  ( -0.06873123812452887338, -2.191421614605370878E-15, 0.4445507791589071167 ) ) ;
#25773=CARTESIAN_POINT ( 'NONE',  ( 0.9776902887139113929, -0.5511811023622048555, -0.09757992244046775898 ) ) ;
#25774=CARTESIAN_POINT ( 'NONE',  ( -1.299212598425196097, 0.2952755905511811885, 0.000000000000000000 ) ) ;
#25776=CARTESIAN_POINT ( 'NONE',  ( 1.049868766404200349, 0.2306618581243848609, 0.2411417322834645549 ) ) ;
#25778=CARTESIAN_POINT ( 'NONE',  ( 0.6824146981627303710, -0.6046776061558807314, 0.2411417322834647770 ) ) ;
#25781=CARTESIAN_POINT ( 'NONE',  ( 0.1443569553805781891, 0.05413385826771626580, -0.4176697321401330321 ) ) ;
#25782=CARTESIAN_POINT ( 'NONE',  ( 0.2493438320209980519, -0.3690944881889765550, -0.3153832671262227771 ) ) ;
#25783=CARTESIAN_POINT ( 'NONE',  ( 0.7808398950131241190, -0.05778040916215560624, -0.4822834645669293319 ) ) ;
#25784=CARTESIAN_POINT ( 'NONE',  ( 0.7742782152230979209, 0.009842519685039147898, -0.3409548833797004797 ) ) ;
#25785=CARTESIAN_POINT ( 'NONE',  ( -0.5708661417322828946, 0.07958543189024071263, -0.2665933059059888421 ) ) ;
#25786=CARTESIAN_POINT ( 'NONE',  ( -0.7939632545931754048, -0.3162353388693405765, 0.4822834645669290543 ) ) ;
#25787=CARTESIAN_POINT ( 'NONE',  ( -1.614173228346455824, 0.1771653543307087630, 0.000000000000000000 ) ) ;
#25789=CARTESIAN_POINT ( 'NONE',  ( -1.338582677165353729, -0.1870078740157480879, -0.4822834645669291653 ) ) ;
#25790=CARTESIAN_POINT ( 'NONE',  ( 1.141732283464567788, -0.6692913385826771977, 8.415575281601705876E-17 ) ) ;
#25791=CARTESIAN_POINT ( 'NONE',  ( -1.528871391076114250, -0.5511811023622046335, 0.09757992244046803654 ) ) ;
#25792=( BOUNDED_CURVE ( )  B_SPLINE_CURVE ( 1, ( #77974, #14836 ),
 .UNSPECIFIED., .F., .F. ) 
 B_SPLINE_CURVE_WITH_KNOTS ( ( 2, 2 ),
 ( 1.734723475976807094E-18, 0.002000000000000003511 ),
 .UNSPECIFIED. ) 
 CURVE ( )  GEOMETRIC_REPRESENTATION_ITEM ( )  RATIONAL_B_SPLINE_CURVE ( ( 0.9875488213027523443, 0.9875488213027523443 ) ) 
 REPRESENTATION_ITEM ( '' )  );
#25794=CARTESIAN_POINT ( 'NONE',  ( 1.187664041994751285, -0.3162353388693409650, -0.4822834645669289433 ) ) ;
#25796=CARTESIAN_POINT ( 'NONE',  ( -1.522309711286088607, 0.2306618581243847221, -0.2411417322834647770 ) ) ;
#25797=CARTESIAN_POINT ( 'NONE',  ( -1.581364829396324945, -0.08942795157528024563, -0.3641732283464568787 ) ) ;
#25798=CARTESIAN_POINT ( 'NONE',  ( -0.8595800524934373854, -0.2845877964562161244, -0.3641732283464567121 ) ) ;
#25799=CARTESIAN_POINT ( 'NONE',  ( 1.489501312335958172, -0.2845877964562159024, 0.3641732283464567677 ) ) ;
#25800=CARTESIAN_POINT ( 'NONE',  ( -0.2559055118110227234, -0.5400638737290844871, 0.3530559997133364547 ) ) ;
#25801=CARTESIAN_POINT ( 'NONE',  ( -0.3477690288713902178, 0.1771653543307087075, -0.09757992244046823083 ) ) ;
#25802=CARTESIAN_POINT ( 'NONE',  ( -1.614173228346456268, -0.5511811023622047445, 6.969142054262312111E-17 ) ) ;
#25803=CARTESIAN_POINT ( 'NONE',  ( 0.8989501312335963501, -0.5511811023622048555, -0.09757992244046775898 ) ) ;
#25804=CARTESIAN_POINT ( 'NONE',  ( 0.4461942257217856311, 0.2306618581243847221, -0.2411417322834647770 ) ) ;
#25806=CARTESIAN_POINT ( 'NONE',  ( 0.6692913385826778638, -0.6692913385826771977, 8.415575281601705876E-17 ) ) ;
#25807=CARTESIAN_POINT ( 'NONE',  ( 0.6036745406824153282, -0.5023911411419708095, 0.1820866141732285504 ) ) ;
#25808=CARTESIAN_POINT ( 'NONE',  ( -1.548556430446193399, -0.6046776061558809534, -0.2411417322834644161 ) ) ;
#25810=CARTESIAN_POINT ( 'NONE',  ( -1.430446194225720724, 0.05413385826771626580, -0.4176697321401330321 ) ) ;
#25811=CARTESIAN_POINT ( 'NONE',  ( -0.4002624671916004129, -0.05778040916215560624, -0.4822834645669293319 ) ) ;
#25814=CARTESIAN_POINT ( 'NONE',  ( 0.09842519685039434474, -0.5400638737290845981, -0.3530559997133363437 ) ) ;
#25815=CARTESIAN_POINT ( 'NONE',  ( 1.010498687664042716, -0.004921259842519870586, -0.3153832671262229437 ) ) ;
#25816=CARTESIAN_POINT ( 'NONE',  ( -0.5249343832020990641, 0.2306618581243848609, 0.2411417322834645549 ) ) ;
#25817=CARTESIAN_POINT ( 'NONE',  ( 0.4461942257217855201, -0.6046776061558807314, 0.2411417322834647770 ) ) ;
#25823=CARTESIAN_POINT ( 'NONE',  ( -0.8530183727034112984, -0.3690944881889765550, -0.3153832671262227771 ) ) ;
#25824=CARTESIAN_POINT ( 'NONE',  ( -1.279527559055116948, -0.5400638737290844871, 0.3530559997133364547 ) ) ;
#25825=AXIS2_PLACEMENT_3D ( 'NONE', #4274, #11005, #16928 ) ;
#25827=CARTESIAN_POINT ( 'NONE',  ( 0.3215223097112867578, -0.3162353388693409650, -0.4822834645669289433 ) ) ;
#25828=CARTESIAN_POINT ( 'NONE',  ( 1.187664041994751285, -0.3162353388693409650, -0.4822834645669289433 ) ) ;
#25829=CARTESIAN_POINT ( 'NONE',  ( 0.7677165354330716118, -0.5400638737290844871, 0.3530559997133364547 ) ) ;
#25833=CARTESIAN_POINT ( 'NONE',  ( 1.535433070866142558, 0.2952755905511811885, 0.000000000000000000 ) ) ;
#25834=CARTESIAN_POINT ( 'NONE',  ( 0.3477690288713918276, 0.2952755905511811885, 0.1292274648535926551 ) ) ;
#25835=CARTESIAN_POINT ( 'NONE',  ( 0.07874015748031558404, -0.1870078740157480879, -0.4822834645669291653 ) ) ;
#25836=CARTESIAN_POINT ( 'NONE',  ( 0.7283464566929140904, -0.4536011799217368745, -0.2665933059059886201 ) ) ;
#25837=CARTESIAN_POINT ( 'NONE',  ( 1.318897637795276356, -0.5400638737290844871, 0.3530559997133364547 ) ) ;
#25839=CARTESIAN_POINT ( 'NONE',  ( 0.5577427821522314977, -0.3162353388693409650, -0.4822834645669289433 ) ) ;
#25840=CARTESIAN_POINT ( 'NONE',  ( 0.9448818897637802916, -0.1870078740157480879, -0.4822834645669291653 ) ) ;
#25841=CARTESIAN_POINT ( 'NONE',  ( 0.1837270341207357105, -0.6046776061558809534, -0.2411417322834644161 ) ) ;
#25842=CARTESIAN_POINT ( 'NONE',  ( 1.056430446194226658, 0.1771653543307087630, 0.09757992244046791164 ) ) ;
#25843=CARTESIAN_POINT ( 'NONE',  ( -1.036745406824146176, 0.05413385826771626580, -0.4176697321401330321 ) ) ;
#25844=CARTESIAN_POINT ( 'NONE',  ( -1.108923884514435132, -0.3162353388693405765, 0.4822834645669290543 ) ) ;
#25845=CARTESIAN_POINT ( 'NONE',  ( 1.227034120734908917, -0.6692913385826771977, 0.1292274648535927661 ) ) ;
#25851=VERTEX_POINT ( 'NONE', #62537 ) ;
#25852=CARTESIAN_POINT ( 'NONE',  ( 1.410761154855643795, -0.05778040916215560624, -0.4822834645669293319 ) ) ;
#25853=CARTESIAN_POINT ( 'NONE',  ( 0.9580052493438326877, -0.004921259842519576551, 0.3153832671262227771 ) ) ;
#25855=CARTESIAN_POINT ( 'NONE',  ( 1.207349081364829990, 0.1283753931104748280, 0.1820866141732283561 ) ) ;
#25856=CARTESIAN_POINT ( 'NONE',  ( 0.8761506516392508770, -4.927456884911482678E-16, 0.4445507791589062840 ) ) ;
#25861=CARTESIAN_POINT ( 'NONE',  ( -0.9908136482939626788, 0.1771653543307087630, 0.09757992244046791164 ) ) ;
#25862=CARTESIAN_POINT ( 'NONE',  ( -1.482939632545930975, -0.3690944881889765550, -0.3153832671262227771 ) ) ;
#25863=CARTESIAN_POINT ( 'NONE',  ( -1.482939632545930975, 0.05413385826771666132, 0.4176697321401328100 ) ) ;
#25864=CARTESIAN_POINT ( 'NONE',  ( -0.08530183727034056085, -0.05778040916215560624, -0.4822834645669293319 ) ) ;
#25865=CARTESIAN_POINT ( 'NONE',  ( 1.587926509186352142, 0.05413385826771666132, 0.4176697321401328100 ) ) ;
#25866=ORIENTED_EDGE ( 'NONE', *, *, #80420, .T. ) ;
#25869=CARTESIAN_POINT ( 'NONE',  ( -0.3025410870193214197, 0.000000000000000000, 0.3464511005275205946 ) ) ;
#25870=CARTESIAN_POINT ( 'NONE',  ( -1.082677165354329896, -0.4536011799217368745, -0.2665933059059886201 ) ) ;
#25871=CARTESIAN_POINT ( 'NONE',  ( -1.318897637795274802, 0.1660481256975885056, 0.3530559997133364547 ) ) ;
#25872=CARTESIAN_POINT ( 'NONE',  ( 0.5971128608923891301, 0.2952755905511810774, -0.1292274648535930714 ) ) ;
#25876=CARTESIAN_POINT ( 'NONE',  ( 1.397637795275591177, 0.1660481256975883668, -0.3530559997133364547 ) ) ;
#25877=CARTESIAN_POINT ( 'NONE',  ( -1.666666666666665853, 0.05413385826771626580, -0.4176697321401330321 ) ) ;
#25880=CARTESIAN_POINT ( 'NONE',  ( -0.5839895013123351797, 0.1771653543307087075, -0.09757992244046823083 ) ) ;
#25881=CARTESIAN_POINT ( 'NONE',  ( -1.213910761154854745, -0.5511811023622046335, 0.09757992244046803654 ) ) ;
#25883=CARTESIAN_POINT ( 'NONE',  ( -0.6889763779527552368, 0.07958543189024085140, 0.2665933059059887866 ) ) ;
#25884=CARTESIAN_POINT ( 'NONE',  ( -0.09186351706036689768, -0.004921259842519870586, -0.3153832671262229437 ) ) ;
#25886=CARTESIAN_POINT ( 'NONE',  ( 0.1968503937007881344, 0.2952755905511811885, 0.000000000000000000 ) ) ;
#25887=CARTESIAN_POINT ( 'NONE',  ( -1.089238845144356427, -0.3690944881889765550, -0.3153832671262227771 ) ) ;
#25889=CARTESIAN_POINT ( 'NONE',  ( 1.089238845144357537, -0.4281496062992124485, 0.4176697321401328655 ) ) ;
#25890=ADVANCED_FACE ( 'NONE', ( #4875 ), #17934, .F. ) ;
#25891=CARTESIAN_POINT ( 'NONE',  ( -1.502624671916009680, -0.3162353388693405765, 0.4822834645669290543 ) ) ;
#25893=CARTESIAN_POINT ( 'NONE',  ( -0.3083989501312330295, -0.05778040916215522460, 0.4822834645669289988 ) ) ;
#25894=CARTESIAN_POINT ( 'NONE',  ( -0.9055118110236215490, -0.6692913385826771977, 8.415575281601705876E-17 ) ) ;
#25895=CARTESIAN_POINT ( 'NONE',  ( 0.9317585301837276734, -0.004921259842519870586, -0.3153832671262229437 ) ) ;
#25896=CARTESIAN_POINT ( 'NONE',  ( -0.5052493438320203589, -0.5511811023622046335, 0.09757992244046803654 ) ) ;
#25897=CARTESIAN_POINT ( 'NONE',  ( -0.4921259842519677963, -0.5400638737290844871, 0.3530559997133364547 ) ) ;
#25898=CARTESIAN_POINT ( 'NONE',  ( -1.358267716535432434, -0.5400638737290844871, 0.3530559997133364547 ) ) ;
#25900=CARTESIAN_POINT ( 'NONE',  ( 1.181102362204725198, -0.1870078740157479769, 0.3641732283464567677 ) ) ;
#25901=CARTESIAN_POINT ( 'NONE',  ( -0.4527559055118102749, -0.5400638737290845981, -0.3530559997133363437 ) ) ;
#25902=CARTESIAN_POINT ( 'NONE',  ( -1.410761154855642463, -0.05778040916215522460, 0.4822834645669289988 ) ) ;
#25903=ORIENTED_EDGE ( 'NONE', *, *, #6471, .T. ) ;
#25906=CARTESIAN_POINT ( 'NONE',  ( -0.9186351706036736120, -0.5023911411419708095, -0.1820866141732282451 ) ) ;
#25907=CARTESIAN_POINT ( 'NONE',  ( 0.7086614173228352742, -0.1870078740157480879, -0.4822834645669291653 ) ) ;
#25908=CARTESIAN_POINT ( 'NONE',  ( -0.8595800524934373854, -0.2845877964562161244, -0.3641732283464567121 ) ) ;
#25910=CARTESIAN_POINT ( 'NONE',  ( -1.030183727034119867, -0.05778040916215560624, -0.4822834645669293319 ) ) ;
#25911=CARTESIAN_POINT ( 'NONE',  ( 0.9055118110236227702, 0.2952755905511811885, 0.000000000000000000 ) ) ;
#25912=CARTESIAN_POINT ( 'NONE',  ( 0.5643044619422579178, 0.05413385826771666132, 0.4176697321401328100 ) ) ;
#25913=EDGE_CURVE ( 'NONE', #47146, #31420, #81913, .T. ) ;
#25914=CARTESIAN_POINT ( 'NONE',  ( 1.423884514435696191, -0.05778040916215522460, 0.4822834645669289988 ) ) ;
#25915=CARTESIAN_POINT ( 'NONE',  ( -1.404199475065615932, -0.004921259842519576551, 0.3153832671262227771 ) ) ;
#25922=CARTESIAN_POINT ( 'NONE',  ( 1.010498687664042716, -0.3690944881889763329, 0.3153832671262228327 ) ) ;
#25923=CARTESIAN_POINT ( 'NONE',  ( 0.2887139107611556010, -0.5023911411419708095, 0.1820866141732285504 ) ) ;
#25924=CARTESIAN_POINT ( 'NONE',  ( 0.1902887139107617975, 0.2952755905511811885, 0.1292274648535926551 ) ) ;
#25925=CARTESIAN_POINT ( 'NONE',  ( 1.496062992125984703, -0.1870078740157480879, -0.4822834645669291653 ) ) ;
#25927=CARTESIAN_POINT ( 'NONE',  ( 0.4986876640419954376, -0.5023911411419708095, -0.1820866141732282451 ) ) ;
#25928=CARTESIAN_POINT ( 'NONE',  ( -0.7939632545931750718, -0.05778040916215560624, -0.4822834645669293319 ) ) ;
#25929=CARTESIAN_POINT ( 'NONE',  ( -1.443569553805773564, 0.2306618581243847221, -0.2411417322834647770 ) ) ;
#25930=CARTESIAN_POINT ( 'NONE',  ( 0.6496062992125991586, -0.5400638737290845981, -0.3530559997133363437 ) ) ;
#25933=ORIENTED_EDGE ( 'NONE', *, *, #3931, .F. ) ;
#25935=CARTESIAN_POINT ( 'NONE',  ( -1.102362204724408601, -0.1870078740157479769, 0.4822834645669291653 ) ) ;
#25936=CARTESIAN_POINT ( 'NONE',  ( -0.5905511811023613777, -0.6692913385826771977, 8.415575281601705876E-17 ) ) ;
#25937=CARTESIAN_POINT ( 'NONE',  ( -0.9645669291338575535, 0.07958543189024071263, -0.2665933059059888421 ) ) ;
#25938=CARTESIAN_POINT ( 'NONE',  ( -0.8005249343832011588, 0.05413385826771626580, -0.4176697321401330321 ) ) ;
#25942=CARTESIAN_POINT ( 'NONE',  ( -1.620734908136482577, 0.1771653543307087630, 0.09757992244046791164 ) ) ;
#25943=CARTESIAN_POINT ( 'NONE',  ( -1.049868766404198794, 0.2306618581243847221, -0.2411417322834647770 ) ) ;
#25944=CARTESIAN_POINT ( 'NONE',  ( 0.2427821522309716595, -0.3162353388693409650, -0.4822834645669289433 ) ) ;
#25945=CARTESIAN_POINT ( 'NONE',  ( -0.8136482939632537770, 0.2306618581243847221, -0.2411417322834647770 ) ) ;
#25947=CARTESIAN_POINT ( 'NONE',  ( -0.9580052493438311334, -0.004921259842519870586, -0.3153832671262229437 ) ) ;
#25948=ORIENTED_EDGE ( 'NONE', *, *, #4963, .F. ) ;
#25950=EDGE_LOOP ( 'NONE', ( #48533, #38568, #69253, #17816 ) ) ;
#25951=CARTESIAN_POINT ( 'NONE',  ( -1.620734908136482577, -0.5511811023622048555, -0.09757992244046775898 ) ) ;
#25952=CARTESIAN_POINT ( 'NONE',  ( -1.246719160104986512, 0.05413385826771666132, 0.4176697321401328100 ) ) ;
#25953=CARTESIAN_POINT ( 'NONE',  ( -0.8727034120734901146, -0.3162353388693405765, 0.4822834645669290543 ) ) ;
#25955=CARTESIAN_POINT ( 'NONE',  ( -0.9776902887139098386, -0.6692913385826771977, 0.1292274648535927661 ) ) ;
#25956=CARTESIAN_POINT ( 'NONE',  ( -1.430446194225721390, -0.4281496062992124485, 0.4176697321401328655 ) ) ;
#25959=CARTESIAN_POINT ( 'NONE',  ( 0.6036745406824154392, 0.1283753931104746893, -0.1820866141732285504 ) ) ;
#25962=CARTESIAN_POINT ( 'NONE',  ( -0.4199475065616791736, 0.1283753931104746893, -0.1820866141732285504 ) ) ;
#25963=CARTESIAN_POINT ( 'NONE',  ( -0.7414698162729651543, -0.6692913385826771977, 0.1292274648535927661 ) ) ;
#25964=CARTESIAN_POINT ( 'NONE',  ( 1.515748031496063186, -0.5400638737290845981, -0.3530559997133363437 ) ) ;
#25965=CARTESIAN_POINT ( 'NONE',  ( -0.6364829396325453192, -0.05778040916215560624, -0.4822834645669293319 ) ) ;
#25966=VERTEX_POINT ( 'NONE', #37278 ) ;
#25969=CARTESIAN_POINT ( 'NONE',  ( -1.108923884514435132, -0.05778040916215560624, -0.4822834645669293319 ) ) ;
#25970=CARTESIAN_POINT ( 'NONE',  ( 1.423884514435696191, -0.05778040916215522460, 0.4822834645669289988 ) ) ;
#25971=CARTESIAN_POINT ( 'NONE',  ( -1.161417322834644716, -0.4536011799217368745, -0.2665933059059886201 ) ) ;
#25972=CARTESIAN_POINT ( 'NONE',  ( -1.384514435695537005, 0.2952755905511811885, 0.1292274648535926551 ) ) ;
#25978=CARTESIAN_POINT ( 'NONE',  ( -0.02624671916010428221, 0.2306618581243847221, -0.2411417322834647770 ) ) ;
#25979=CARTESIAN_POINT ( 'NONE',  ( -1.154855643044618851, 0.1283753931104748280, 0.1820866141732283561 ) ) ;
#25980=CARTESIAN_POINT ( 'NONE',  ( -0.6955380577427815458, -0.4281496062992127816, -0.4176697321401328100 ) ) ;
#25982=CARTESIAN_POINT ( 'NONE',  ( -1.423884514435694859, -0.3162353388693405765, 0.4822834645669290543 ) ) ;
#25983=CARTESIAN_POINT ( 'NONE',  ( -1.167979002624671470, -0.4281496062992127816, -0.4176697321401328100 ) ) ;
#25984=CARTESIAN_POINT ( 'NONE',  ( 0.1377952755905518800, -0.5400638737290844871, 0.3530559997133364547 ) ) ;
#25986=CARTESIAN_POINT ( 'NONE',  ( 1.030183727034121421, -0.2845877964562161244, -0.3641732283464567121 ) ) ;
#25987=CARTESIAN_POINT ( 'NONE',  ( -0.6364829396325453192, -0.2845877964562159024, 0.3641732283464567677 ) ) ;
#25990=CARTESIAN_POINT ( 'NONE',  ( 0.6299212598425204535, -0.1870078740157480601, -0.3641732283464567677 ) ) ;
#25991=CARTESIAN_POINT ( 'NONE',  ( 1.515748031496063186, -0.4536011799217368745, -0.2665933059059886201 ) ) ;
#25992=CARTESIAN_POINT ( 'NONE',  ( 1.194225721784777594, -0.4281496062992127816, -0.4176697321401328100 ) ) ;
#25994=CARTESIAN_POINT ( 'NONE',  ( -0.06561679790026180015, -0.004921259842519576551, 0.3153832671262227771 ) ) ;
#25996=CARTESIAN_POINT ( 'NONE',  ( -1.030183727034119867, -0.3162353388693405765, 0.4822834645669290543 ) ) ;
#25997=CARTESIAN_POINT ( 'NONE',  ( 1.437007874015748810, 0.1660481256975885056, 0.3530559997133364547 ) ) ;
#26000=CARTESIAN_POINT ( 'NONE',  ( -0.5249343832020990641, 0.1283753931104748280, 0.1820866141732283561 ) ) ;
#26001=CARTESIAN_POINT ( 'NONE',  ( 0.5249343832021005074, -0.6046776061558807314, 0.2411417322834647770 ) ) ;
#26004=CARTESIAN_POINT ( 'NONE',  ( 1.003937007874016185, 0.07958543189024071263, -0.2665933059059888421 ) ) ;
#26005=CARTESIAN_POINT ( 'NONE',  ( 0.01312335958005323398, -0.004921259842519576551, 0.3153832671262227771 ) ) ;
#26006=CARTESIAN_POINT ( 'NONE',  ( 0.2952755905511819101, 0.1660481256975883668, -0.3530559997133364547 ) ) ;
#26007=CARTESIAN_POINT ( 'NONE',  ( -1.318897637795274802, -0.5400638737290845981, -0.3530559997133363437 ) ) ;
#26008=CARTESIAN_POINT ( 'NONE',  ( -0.8267716535433065062, 0.1771653543307087630, 0.000000000000000000 ) ) ;
#26010=CARTESIAN_POINT ( 'NONE',  ( -0.9776902887139098386, 0.2952755905511810774, -0.1292274648535930714 ) ) ;
#26013=CARTESIAN_POINT ( 'NONE',  ( 0.2099737532808405305, 0.1283753931104746893, -0.1820866141732285504 ) ) ;
#26014=CARTESIAN_POINT ( 'NONE',  ( -0.6299212598425188991, -0.1870078740157480879, -0.4822834645669291653 ) ) ;
#26015=CARTESIAN_POINT ( 'NONE',  ( -1.089238845144356427, -0.4281496062992127816, -0.4176697321401328100 ) ) ;
#26016=CARTESIAN_POINT ( 'NONE',  ( -1.062992125984250968, -0.5511811023622047445, 6.969142054262312111E-17 ) ) ;
#26017=CARTESIAN_POINT ( 'NONE',  ( 1.541994750656168645, 0.2952755905511810774, -0.1292274648535930714 ) ) ;
#26018=CARTESIAN_POINT ( 'NONE',  ( -0.8792650918635160906, -0.3690944881889763329, 0.3153832671262228327 ) ) ;
#26019=CARTESIAN_POINT ( 'NONE',  ( -1.692913385826770645, 0.1771653543307087630, 0.000000000000000000 ) ) ;
#26020=CARTESIAN_POINT ( 'NONE',  ( 1.489501312335958172, -0.05778040916215560624, -0.4822834645669293319 ) ) ;
#26025=CARTESIAN_POINT ( 'NONE',  ( 1.404199475065617264, -0.3690944881889763329, 0.3153832671262228327 ) ) ;
#26026=CARTESIAN_POINT ( 'NONE',  ( -1.122047244094487306, -0.5400638737290844871, 0.3530559997133364547 ) ) ;
#26027=CARTESIAN_POINT ( 'NONE',  ( 1.161417322834646271, 0.1660481256975883668, -0.3530559997133364547 ) ) ;
#26030=CARTESIAN_POINT ( 'NONE',  ( 0.5708661417322842269, 0.1660481256975885056, 0.3530559997133364547 ) ) ;
#26031=CARTESIAN_POINT ( 'NONE',  ( -0.05249343832020911260, 0.2306618581243848609, 0.2411417322834645549 ) ) ;
#26032=CARTESIAN_POINT ( 'NONE',  ( -0.6967283859536032020, -3.965272662620685221E-15, 0.3627989612356152249 ) ) ;
#26033=LINE ( 'NONE', #58013, #14355 ) ;
#26034=CARTESIAN_POINT ( 'NONE',  ( 0.6692913385826777528, 0.1771653543307087630, 0.000000000000000000 ) ) ;
#26035=EDGE_CURVE ( 'NONE', #36796, #25632, #22143, .T. ) ;
#26037=ORIENTED_EDGE ( 'NONE', *, *, #60455, .T. ) ;
#26040=CARTESIAN_POINT ( 'NONE',  ( 0.1443569553805781891, -0.4281496062992124485, 0.4176697321401328655 ) ) ;
#26041=CARTESIAN_POINT ( 'NONE',  ( -1.404199475065615932, -0.4281496062992127816, -0.4176697321401328100 ) ) ;
#26042=CARTESIAN_POINT ( 'NONE',  ( 0.5052493438320218022, -0.6692913385826773087, -0.1292274648535924053 ) ) ;
#26043=VECTOR ( 'NONE', #36845, 39.37007874015748143 ) ;
#26044=CARTESIAN_POINT ( 'NONE',  ( 1.207349081364829990, 0.2306618581243848609, 0.2411417322834645549 ) ) ;
#26045=CARTESIAN_POINT ( 'NONE',  ( 1.397637795275591177, -0.5400638737290844871, 0.3530559997133364547 ) ) ;
#26047=CARTESIAN_POINT ( 'NONE',  ( -0.3871391076115476282, -0.05778040916215522460, 0.4822834645669289988 ) ) ;
#26048=CARTESIAN_POINT ( 'NONE',  ( -0.1837270341207343505, -0.6046776061558807314, 0.2411417322834647770 ) ) ;
#26049=CARTESIAN_POINT ( 'NONE',  ( 1.443569553805774897, 0.2306618581243848609, 0.2411417322834645549 ) ) ;
#26050=CARTESIAN_POINT ( 'NONE',  ( 1.502624671916010790, -0.3162353388693409650, -0.4822834645669289433 ) ) ;
#26051=CARTESIAN_POINT ( 'NONE',  ( 1.259842519685040019, -0.1870078740157480879, -0.4822834645669291653 ) ) ;
#26052=CARTESIAN_POINT ( 'NONE',  ( -0.3149606299212590610, -0.1870078740157479769, 0.4822834645669291653 ) ) ;
#26054=CARTESIAN_POINT ( 'NONE',  ( 0.2624671916010504757, 0.1283753931104748280, 0.1820866141732283561 ) ) ;
#26057=ORIENTED_EDGE ( 'NONE', *, *, #36412, .T. ) ;
#26058=CARTESIAN_POINT ( 'NONE',  ( -0.5839895013123351797, 0.1771653543307087075, -0.09757992244046823083 ) ) ;
#26060=CARTESIAN_POINT ( 'NONE',  ( 0.3149606299212603933, -0.1870078740157479769, 0.4822834645669291653 ) ) ;
#26061=CARTESIAN_POINT ( 'NONE',  ( 0.1902887139107617975, 0.2952755905511811885, 0.1292274648535926551 ) ) ;
#26062=CARTESIAN_POINT ( 'NONE',  ( -0.8398950131233589023, -0.6046776061558809534, -0.2411417322834644161 ) ) ;
#26063=VECTOR ( 'NONE', #8835, 39.37007874015748854 ) ;
#26065=CARTESIAN_POINT ( 'NONE',  ( -1.345144356955379816, -0.3162353388693405765, 0.4822834645669290543 ) ) ;
#26067=CARTESIAN_POINT ( 'NONE',  ( 1.043307086614173818, -0.4536011799217368745, -0.2665933059059886201 ) ) ;
#26068=CARTESIAN_POINT ( 'NONE',  ( 0.3280839895013130669, -0.4281496062992127816, -0.4176697321401328100 ) ) ;
#26069=CARTESIAN_POINT ( 'NONE',  ( 0.5905511811023629321, 0.2952755905511811885, 0.000000000000000000 ) ) ;
#26074=CARTESIAN_POINT ( 'NONE',  ( -0.3215223097112853146, -0.3162353388693405765, 0.4822834645669290543 ) ) ;
#26077=CARTESIAN_POINT ( 'NONE',  ( -1.338582677165353729, -0.1870078740157479769, 0.3641732283464567677 ) ) ;
#26078=CARTESIAN_POINT ( 'NONE',  ( 1.476377952755906220, 0.1660481256975883668, -0.3530559997133364547 ) ) ;
#26079=CARTESIAN_POINT ( 'NONE',  ( 1.167979002624672580, -0.4281496062992124485, 0.4176697321401328655 ) ) ;
#26080=CARTESIAN_POINT ( 'NONE',  ( 0.2755905511811031494, 0.1771653543307087630, 0.000000000000000000 ) ) ;
#26081=CARTESIAN_POINT ( 'NONE',  ( 0.4790026246719167324, -0.05778040916215522460, 0.4822834645669289988 ) ) ;
#26083=CARTESIAN_POINT ( 'NONE',  ( 0.4921259842519691285, -0.4536011799217368745, -0.2665933059059886201 ) ) ;
#26084=CARTESIAN_POINT ( 'NONE',  ( 0.1377952755905518800, -0.5400638737290844871, 0.3530559997133364547 ) ) ;
#26086=CARTESIAN_POINT ( 'NONE',  ( -1.213910761154854745, 0.2952755905511810774, -0.1292274648535930714 ) ) ;
#26087=CARTESIAN_POINT ( 'NONE',  ( 0.5118110236220478892, 0.1771653543307087630, 0.000000000000000000 ) ) ;
#26088=CARTESIAN_POINT ( 'NONE',  ( -1.220472440944882386, -0.1870078740157480046, 1.254653134982923898E-17 ) ) ;
#26089=CARTESIAN_POINT ( 'NONE',  ( -0.5314960629921254842, -0.5400638737290845981, -0.3530559997133363437 ) ) ;
#26090=CARTESIAN_POINT ( 'NONE',  ( -0.2559055118110227234, -0.4536011799217367080, 0.2665933059059888421 ) ) ;
#26092=CARTESIAN_POINT ( 'NONE',  ( -0.3215223097112853146, -0.3162353388693405765, 0.4822834645669290543 ) ) ;
#26093=CARTESIAN_POINT ( 'NONE',  ( -0.4265091863517051496, -0.6692913385826771977, 0.1292274648535927661 ) ) ;
#26094=CARTESIAN_POINT ( 'NONE',  ( 0.3608923884514443348, 0.1771653543307087075, -0.09757992244046823083 ) ) ;
#26096=CARTESIAN_POINT ( 'NONE',  ( -0.1902887139107604098, 0.2952755905511810774, -0.1292274648535930714 ) ) ;
#26098=CARTESIAN_POINT ( 'NONE',  ( 0.8333333333333340365, -0.5511811023622046335, 0.09757992244046803654 ) ) ;
#26099=CARTESIAN_POINT ( 'NONE',  ( 1.253280839895013710, -0.3162353388693405765, 0.4822834645669290543 ) ) ;
#26100=CARTESIAN_POINT ( 'NONE',  ( -0.7283464566929126471, 0.07958543189024071263, -0.2665933059059888421 ) ) ;
#26101=CARTESIAN_POINT ( 'NONE',  ( -0.6561679790026240244, -0.5023911411419708095, 0.1820866141732285504 ) ) ;
#26102=CARTESIAN_POINT ( 'NONE',  ( -0.6364829396325453192, -0.05778040916215560624, -0.4822834645669293319 ) ) ;
#26103=CARTESIAN_POINT ( 'NONE',  ( -0.2230971128608915943, -0.4281496062992127816, -0.4176697321401328100 ) ) ;
#26104=CARTESIAN_POINT ( 'NONE',  ( 0.7480314960629927956, 0.1771653543307087630, 0.000000000000000000 ) ) ;
#26106=CARTESIAN_POINT ( 'NONE',  ( 1.154855643044620184, 0.1283753931104746893, -0.1820866141732285504 ) ) ;
#26107=VECTOR ( 'NONE', #54146, 39.37007874015748143 ) ;
#26108=CARTESIAN_POINT ( 'NONE',  ( 0.9317585301837276734, 0.05413385826771626580, -0.4176697321401330321 ) ) ;
#26110=CARTESIAN_POINT ( 'NONE',  ( -0.2952755905511804668, 0.1660481256975885056, 0.3530559997133364547 ) ) ;
#26112=CARTESIAN_POINT ( 'NONE',  ( 1.502624671916010790, -0.2845877964562161244, -0.3641732283464567121 ) ) ;
#26113=CARTESIAN_POINT ( 'NONE',  ( 0.4921259842519691285, -0.5400638737290845981, -0.3530559997133363437 ) ) ;
#26114=CARTESIAN_POINT ( 'NONE',  ( 0.2230971128608932319, -0.4281496062992124485, 0.4176697321401328655 ) ) ;
#26116=CARTESIAN_POINT ( 'NONE',  ( 0.4790026246719168435, -0.2845877964562161244, -0.3641732283464567121 ) ) ;
#26117=CARTESIAN_POINT ( 'NONE',  ( 0.8398950131233602345, -0.6046776061558807314, 0.2411417322834647770 ) ) ;
#26118=CARTESIAN_POINT ( 'NONE',  ( -0.2624671916010490880, 0.1283753931104746893, -0.1820866141732285504 ) ) ;
#26120=CARTESIAN_POINT ( 'NONE',  ( -0.7939632545931750718, -0.05778040916215560624, -0.4822834645669293319 ) ) ;
#26122=CARTESIAN_POINT ( 'NONE',  ( -0.2165354330708654795, -0.5400638737290845981, -0.3530559997133363437 ) ) ;
#26123=CARTESIAN_POINT ( 'NONE',  ( -1.102362204724408601, -0.1870078740157480879, -0.4822834645669291653 ) ) ;
#26124=CARTESIAN_POINT ( 'NONE',  ( -0.7808398950131225646, -0.08942795157527998196, 0.3641732283464567121 ) ) ;
#26125=CARTESIAN_POINT ( 'NONE',  ( 0.5314960629921264834, 0.1660481256975883668, -0.3530559997133364547 ) ) ;
#26126=CARTESIAN_POINT ( 'NONE',  ( -1.391076115485563758, 0.2306618581243848609, 0.2411417322834645549 ) ) ;
#26127=CARTESIAN_POINT ( 'NONE',  ( -0.4921259842519677963, 0.1660481256975883668, -0.3530559997133364547 ) ) ;
#26129=CARTESIAN_POINT ( 'NONE',  ( 1.351706036745407458, -0.4281496062992127816, -0.4176697321401328100 ) ) ;
#26130=CARTESIAN_POINT ( 'NONE',  ( 1.240157480314961314, 0.1660481256975883668, -0.3530559997133364547 ) ) ;
#26132=CARTESIAN_POINT ( 'NONE',  ( 0.4606732211678724598, 1.763126522798933227, -0.5309055118110237448 ) ) ;
#26133=CARTESIAN_POINT ( 'NONE',  ( -1.115485564304461219, -0.4281496062992124485, 0.4176697321401328655 ) ) ;
#26138=CARTESIAN_POINT ( 'NONE',  ( 0.03280839895013198948, -0.5511811023622048555, -0.09757992244046775898 ) ) ;
#26141=CARTESIAN_POINT ( 'NONE',  ( 0.3280839895013130669, 0.05413385826771666132, 0.4176697321401328100 ) ) ;
#26142=CARTESIAN_POINT ( 'NONE',  ( 0.5314960629921264834, 0.1660481256975883668, -0.3530559997133364547 ) ) ;
#26144=CARTESIAN_POINT ( 'NONE',  ( 2.795275590551181910, 1.805669738366189048, 0.000000000000000000 ) ) ;
#26145=CARTESIAN_POINT ( 'NONE',  ( -0.2821522309711278487, -0.5511811023622048555, -0.09757992244046775898 ) ) ;
#26147=CARTESIAN_POINT ( 'NONE',  ( 0.9580052493438327987, -0.4281496062992127816, -0.4176697321401328100 ) ) ;
#26148=CARTESIAN_POINT ( 'NONE',  ( 1.076115485564305141, -0.5023911411419708095, 0.1820866141732285504 ) ) ;
#26149=CARTESIAN_POINT ( 'NONE',  ( -0.5183727034120726440, 0.2952755905511811885, 0.1292274648535926551 ) ) ;
#26151=CARTESIAN_POINT ( 'NONE',  ( -0.9973753280839886548, 0.2306618581243848609, 0.2411417322834645549 ) ) ;
#26152=CARTESIAN_POINT ( 'NONE',  ( -1.437007874015747477, -0.4536011799217367080, 0.2665933059059888421 ) ) ;
#26153=CARTESIAN_POINT ( 'NONE',  ( -1.030183727034119867, -0.05778040916215560624, -0.4822834645669293319 ) ) ;
#26154=CARTESIAN_POINT ( 'NONE',  ( 1.187664041994751285, -0.05778040916215522460, 0.4822834645669289988 ) ) ;
#26156=ORIENTED_EDGE ( 'NONE', *, *, #54694, .T. ) ;
#26158=CARTESIAN_POINT ( 'NONE',  ( -0.03937007874015669567, 0.2952755905511811885, 0.000000000000000000 ) ) ;
#26159=ORIENTED_EDGE ( 'NONE', *, *, #54850, .F. ) ;
#26160=CARTESIAN_POINT ( 'NONE',  ( -0.8070866141732276899, -0.5400638737290844871, 0.3530559997133364547 ) ) ;
#26161=CARTESIAN_POINT ( 'NONE',  ( 1.541994750656168645, -0.6692913385826771977, 0.1292274648535927661 ) ) ;
#26162=CARTESIAN_POINT ( 'NONE',  ( 1.076115485564305141, -0.6046776061558807314, 0.2411417322834647770 ) ) ;
#26163=( BOUNDED_SURFACE ( )  B_SPLINE_SURFACE ( 1, 2, ( 
 ( #79887, #73566, #9580, #16321, #29751, #35661, #48692, #80303, #22618, #79062, #61746, #47033, #53758, #22205, #68072, #15491, #9996, #48277, #41966, #80711, #28104, #41148, #23026, #67248, #74390, #16734, #66837, #9171, #34842, #10417, #36075, #8751, #60505, #34425, #2853, #47861, #15910, #28517, #36896, #50338, #10820, #81533, #25075, #56651, #57060, #49102, #4913, #30582, #82753, #76449, #4496, #55826, #63389, #56248, #37313, #76035, #50749, #18776, #36480, #18380, #44419, #44021, #70114, #69714, #12465, #63801, #49520, #17966, #81944, #81121, #11654, #74806, #17153, #42786, #5724, #23853, #24670, #82352, #24257, #75628, #62155, #62986, #31395, #6139, #68481, #30163, #43603, #68886, #12058, #55414, #5325, #62572, #37715, #49930, #75213, #38127, #23438, #17557, #69305, #43190, #11236, #30983, #64224, #33068, #32230, #71794, #57888, #6558, #1100, #65903, #38544, #39800, #25488, #71373, #20866, #26751, #65062, #78541, #7400, #72218, #40221, #38955, #6976, #26329, #45677, #52406, #31814, #14147, #1513, #13723, #58738, #57474, #14569, #83168, #255, #32645, #46516, #12884, #25907, #51567, #77270, #19599, #45262, #27167, #39377, #78115, #51154, #76849, #19182, #70958, #58310, #44831, #13303, #64639, #675, #51991, #77696, #20026, #20448, #46101, #65494, #7826, #33493, #59155, #52829, #70529, #54076, #54495, #35155, #14974, #34325, #53662, #80206, #47767, #79791, #59987, #67563, #73040, #60406, #9075, #60815, #15389, #3167, #46934, #2346, #61229, #9480, #9895, #1925, #41051, #66736, #35566, #29249, #40633, #8654, #16222, #34746, #73465, #28831, #3582, #54913, #72626, #22523, #80619, #48185, #22931, #73882, #48597, #16639, #28002, #22107, #2757, #33905, #15817, #27588, #53245, #78960, #41869, #79369, #74293, #42279, #28416, #41466, #66315, #67151, #8239, #59569, #21279, #21688, #47351, #81441, #37214, #76355, #24166, #49429, #24578, #75123, #42696, #24979, #67977, #11557, #30486, #29659, #61654, #62063, #17056, #69208, #68393, #50245, #10732, #36389, #62893, #18687, #74710, #75941, #3995, #49835, #56966, #5228, #17874, #31302, #43508, #50652, #10319, #17468, #43099, #62475, #81855, #30892, #35984, #18282, #56559, #36799, #82664, #55321, #81030, #23342, #63297, #49013, #82260, #4402, #68795, #30070, #55733, #23755, #43924, #56151, #11140, #4810, #69621, #75534, #11966, #37621, #5635, #57791, #59060, #38032, #12374, #63707, #32548, #12790, #52312, #27071, #51059, #51471, #52730, #64129, #25811, #71276, #77174, #33398, #64964, #76759, #83074, #6464, #6047, #45583, #31719, #158, #57379, #25395, #19089, #78019, #20347, #45999, #1415, #32134, #13625, #71695, #70433, #45159, #14049, #39703, #39277, #64541, #44330, #7300, #578, #44738, #38446, #19505, #78441, #19934, #70021, #70863, #13214, #38860, #6878, #77600, #65395, #32969, #58637, #7730, #58212, #26232, #1004, #51895, #26659, #78857, #59473, #40123, #55937, #53144, #80104, #33808, #66218, #3065, #40539, #27486, #15709, #16118, #60716, #53977, #2657, #9791, #9380, #66632, #73782, #48080, #28732, #21182, #54393, #79689, #60308, #28316, #46837, #2240, #1826, #72531, #14879, #20767, #22423, #34643, #27905, #8557, #41764, #22006, #53565, #72940, #34225, #73361, #47666, #79274, #40952, #59886, #41366, #67457, #46420, #65810, #8143, #8969, #21589, #67047, #30274, #35050, #47251, #35463, #15292, #61127, #3478, #72112, #14470, #44131, #43300, #75323, #75737, #30695, #82869, #82057, #38240, #24371, #56359, #50859, #32344, #5027, #6252, #17669, #37830, #70647, #76559, #31512, #44950, #57171, #38658, #6672, #5435, #56762, #76148, #12172, #18887, #81652, #63916, #51267, #63506, #25193, #23963, #64335, #49629, #50041, #82462, #13002, #62685, #18078, #43713, #69415, #11769, #37423, #63096, #12581, #5838, #44536, #70227, #31095, #24778, #31929, #69823, #57591, #83281, #50446, #18488, #25604, #76969, #19299, #68997, #11349, #37007, #39497, #26865, #58858, #1623, #65185, #52940, #13416, #792, #27700, #59266, #59679, #51685, #7521, #33190, #2035, #79074, #7093, #58430, #66015, #1216, #39921, #78654, #53364, #21390, #39073 ),
 ( #77387, #8351, #52105, #32763, #27280, #26451, #14678, #77813, #20144, #20975, #8762, #64754, #34019, #19719, #14263, #47046, #46634, #7941, #72738, #33603, #15085, #66427, #52526, #78232, #20566, #71913, #72330, #58005, #40334, #40743, #65611, #370, #26025, #45377, #71074, #45793, #46217, #71491, #13839, #9182, #60516, #2865, #66849, #41160, #34854, #48703, #16334, #35672, #23037, #28528, #54185, #16746, #80315, #80723, #61337, #79899, #22217, #47873, #74402, #73988, #22630, #73577, #10429, #15923, #3276, #35261, #3690, #41570, #29355, #73153, #67260, #4094, #55014, #36086, #28115, #9593, #60926, #61757, #55425, #28939, #54606, #42385, #48291, #41977, #68084, #29763, #81133, #15502, #23449, #49114, #74819, #17164, #42798, #68492, #34437, #67671, #10007, #60103, #2457, #53769, #79482, #21796, #47460, #44433, #36908, #63402, #37728, #69317, #30995, #75225, #50350, #70127, #44845, #55837, #30174, #82364, #24270, #5738, #19196, #76048, #75640, #50762, #17979, #68897, #51167, #10831, #31409, #56664, #81546, #4506, #57073, #6153, #76463, #44034, #18392, #83181, #82767, #24683, #63814, #38142, #18789, #11250, #12478, #69726, #12071, #25089, #62584, #43616, #17569, #4926, #30594, #36491, #31827, #57488, #11668, #56260, #25502, #76864, #37326, #62998, #62167, #5337, #23864, #49531, #43202, #81956, #49942, #33916, #33504, #45276, #77709, #6572, #32243, #32658, #46115, #58751, #13736, #52004, #27178, #38557, #59581, #1524, #7414, #687, #1938, #64237, #57902, #268, #1113, #38969, #78553, #53260, #77283, #20039, #78971, #6990, #45690, #14160, #71387, #27600, #7837, #19614, #25923, #58325, #51581, #71809, #70971, #26343, #13316, #64652, #39392, #20878, #46530, #72230, #21292, #65076, #39816, #14579, #33084, #26764, #40232, #65915, #65505, #52419, #70543, #59166, #78128, #20462, #52842, #8251, #12898, #22536, #29671, #40644, #60002, #9087, #34759, #80220, #54925, #48199, #67575, #22943, #28013, #79804, #73894, #67164, #46945, #21700, #2357, #66328, #81042, #79381, #48610, #53673, #60419, #29261, #66753, #47363, #73054, #80632, #9494, #9907, #16234, #15404, #41064, #2770, #35579, #3180, #35167, #28429, #74305, #54089, #15831, #47779, #41881, #22120, #61242, #73481, #41479, #16652, #3596, #42292, #8666, #60828, #28844, #67989, #10334, #54506, #35996, #61666, #4007, #55333, #72637, #14985, #34337, #4414, #18294, #18700, #11978, #38044, #69633, #63720, #31731, #17480, #69221, #81866, #49026, #62905, #42708, #68404, #10744, #56979, #49441, #75956, #50258, #24178, #43523, #30083, #5240, #82676, #57396, #36401, #62076, #11569, #36812, #43939, #23355, #30904, #4822, #63309, #30500, #81453, #6060, #74722, #37633, #37228, #55745, #17071, #43111, #23770, #24590, #75135, #5647, #68807, #11154, #31314, #62488, #56163, #24993, #49847, #56571, #12386, #50667, #82272, #70033, #76367, #75546, #17886, #44342, #58223, #77612, #13636, #20360, #8153, #39714, #52743, #39289, #1016, #83086, #65820, #51071, #57804, #590, #72123, #64144, #170, #25823, #51483, #32147, #6478, #77186, #14060, #64975, #26669, #71706, #19518, #45171, #70877, #7743, #26246, #7312, #46010, #1425, #20777, #13226, #78030, #78451, #65405, #14481, #33408, #40135, #33818, #38875, #45595, #51905, #25408, #32981, #19101, #44750, #70446, #59070, #64553, #52324, #27081, #19945, #71289, #6891, #58649, #46431, #76770, #12803, #38458, #32560, #72952, #28745, #67891, #15724, #40966, #16131, #66648, #34237, #16551, #59484, #3081, #22019, #21192, #53154, #53575, #8567, #60729, #59898, #41777, #2250, #27916, #54407, #10228, #66229, #67471, #78866, #41379, #48503, #80118, #9393, #22844, #35064, #42195, #1838, #8984, #34657, #53991, #73374, #22436, #27498, #9805, #29158, #67060, #48096, #46846, #72541, #14888, #79284, #60321, #74204, #40548, #21601, #47262, #15303, #2670, #28329, #79703, #73795, #35477, #61141, #3493, #47679, #54828, #80533, #81766, #82172, #62806, #42606, #61974, #81351, #24489, #75445, #24076, #4312, #11881, #17381, #4717, #36705, #5140, #43011, #30805, #74623, #29976, #5548, #37122, #37533, #29569, #68705 ) ),
 .UNSPECIFIED., .F., .F., .F. ) 
 B_SPLINE_SURFACE_WITH_KNOTS ( ( 2, 2 ),
 ( 3, 2, 2, 2, 2, 2, 2, 2, 2, 2, 2, 2, 2, 2, 2, 2, 2, 2, 2, 2, 2, 2, 2, 2, 2, 2, 2, 2, 2, 2, 2, 2, 2, 2, 2, 2, 2, 2, 2, 2, 2, 2, 2, 2, 2, 2, 2, 2, 2, 2, 2, 2, 2, 2, 2, 2, 2, 2, 2, 2, 2, 2, 2, 2, 2, 2, 2, 2, 2, 2, 2, 2, 2, 2, 2, 2, 2, 2, 2, 2, 2, 2, 2, 2, 2, 2, 2, 2, 2, 2, 2, 2, 2, 2, 2, 2, 2, 2, 2, 2, 2, 2, 2, 2, 2, 2, 2, 2, 2, 2, 2, 2, 2, 2, 2, 2, 2, 2, 2, 2, 2, 2, 2, 2, 2, 2, 2, 2, 2, 2, 2, 2, 2, 2, 2, 2, 2, 2, 2, 2, 2, 2, 2, 2, 2, 2, 2, 2, 2, 2, 2, 2, 2, 2, 2, 2, 2, 2, 2, 2, 2, 2, 2, 2, 2, 2, 2, 2, 2, 2, 2, 2, 2, 2, 2, 2, 2, 2, 2, 2, 2, 2, 2, 2, 2, 2, 2, 2, 2, 2, 2, 2, 2, 2, 2, 2, 2, 2, 2, 2, 2, 2, 2, 2, 2, 2, 2, 2, 2, 2, 2, 2, 2, 2, 2, 2, 2, 2, 2, 2, 2, 2, 2, 2, 2, 2, 2, 2, 2, 2, 2, 2, 2, 2, 2, 2, 2, 2, 2, 2, 2, 2, 2, 2, 2, 2, 2, 2, 2, 2, 2, 2, 2, 2, 2, 3 ),
 ( 0.000000000000000000, 1.000000000000000000 ),
 ( 0.000000000000000000, 0.003787878787878787984, 0.007575757575757575968, 0.01136363636363636395, 0.01515151515151515194, 0.01893939393939393992, 0.02272727272727272790, 0.02651515151515151589, 0.03030303030303030387, 0.03409090909090908839, 0.03787878787878787984, 0.04166666666666666435, 0.04545454545454545581, 0.04924242424242424032, 0.05303030303030303177, 0.05681818181818181629, 0.06060606060606060774, 0.06439393939393939226, 0.06818181818181817677, 0.07196969696969697516, 0.07575757575757575968, 0.07954545454545454419, 0.08333333333333332871, 0.08712121212121212710, 0.09090909090909091161, 0.09469696969696969613, 0.09848484848484848064, 0.1022727272727272790, 0.1060606060606060635, 0.1098484848484848481, 0.1136363636363636326, 0.1174242424242424310, 0.1212121212121212155, 0.1250000000000000000, 0.1287878787878787845, 0.1325757575757575690, 0.1363636363636363535, 0.1401515151515151381, 0.1439393939393939503, 0.1477272727272727348, 0.1515151515151515194, 0.1553030303030303039, 0.1590909090909090884, 0.1628787878787878729, 0.1666666666666666574, 0.1704545454545454419, 0.1742424242424242542, 0.1780303030303030387, 0.1818181818181818232, 0.1856060606060606077, 0.1893939393939393923, 0.1931818181818181768, 0.1969696969696969613, 0.2007575757575757458, 0.2045454545454545581, 0.2083333333333333426, 0.2121212121212121271, 0.2159090909090909116, 0.2196969696969696961, 0.2234848484848484806, 0.2272727272727272652, 0.2310606060606060497, 0.2348484848484848619, 0.2386363636363636465, 0.2424242424242424310, 0.2462121212121212155, 0.2500000000000000000, 0.2537878787878787845, 0.2575757575757575690, 0.2613636363636363535, 0.2651515151515151381, 0.2689393939393939226, 0.2727272727272727071, 0.2765151515151514916, 0.2803030303030302761, 0.2840909090909091161, 0.2878787878787879007, 0.2916666666666666852, 0.2954545454545454697, 0.2992424242424242542, 0.3030303030303030387, 0.3068181818181818232, 0.3106060606060606077, 0.3143939393939393923, 0.3181818181818181768, 0.3219696969696969613, 0.3257575757575757458, 0.3295454545454545303, 0.3333333333333333148, 0.3371212121212120993, 0.3409090909090908839, 0.3446969696969697239, 0.3484848484848485084, 0.3522727272727272929, 0.3560606060606060774, 0.3598484848484848619, 0.3636363636363636465, 0.3674242424242424310, 0.3712121212121212155, 0.3750000000000000000, 0.3787878787878787845, 0.3825757575757575690, 0.3863636363636363535, 0.3901515151515151381, 0.3939393939393939226, 0.3977272727272727071, 0.4015151515151514916, 0.4053030303030302761, 0.4090909090909091161, 0.4128787878787879007, 0.4166666666666666852, 0.4204545454545454697, 0.4242424242424242542, 0.4280303030303030387, 0.4318181818181818232, 0.4356060606060606077, 0.4393939393939393923, 0.4431818181818181768, 0.4469696969696969613, 0.4507575757575757458, 0.4545454545454545303, 0.4583333333333333148, 0.4621212121212120993, 0.4659090909090908839, 0.4696969696969697239, 0.4734848484848485084, 0.4772727272727272929, 0.4810606060606060774, 0.4848484848484848619, 0.4886363636363636465, 0.4924242424242424310, 0.4962121212121212155, 0.5000000000000000000, 0.5037878787878787845, 0.5075757575757575690, 0.5113636363636363535, 0.5151515151515151381, 0.5189393939393939226, 0.5227272727272727071, 0.5265151515151514916, 0.5303030303030302761, 0.5340909090909090606, 0.5378787878787878451, 0.5416666666666666297, 0.5454545454545454142, 0.5492424242424241987, 0.5530303030303029832, 0.5568181818181817677, 0.5606060606060605522, 0.5643939393939394478, 0.5681818181818182323, 0.5719696969696970168, 0.5757575757575758013, 0.5795454545454545858, 0.5833333333333333703, 0.5871212121212121549, 0.5909090909090909394, 0.5946969696969697239, 0.5984848484848485084, 0.6022727272727272929, 0.6060606060606060774, 0.6098484848484848619, 0.6136363636363636465, 0.6174242424242424310, 0.6212121212121212155, 0.6250000000000000000, 0.6287878787878787845, 0.6325757575757575690, 0.6363636363636363535, 0.6401515151515151381, 0.6439393939393939226, 0.6477272727272727071, 0.6515151515151514916, 0.6553030303030302761, 0.6590909090909090606, 0.6628787878787878451, 0.6666666666666666297, 0.6704545454545454142, 0.6742424242424241987, 0.6780303030303029832, 0.6818181818181817677, 0.6856060606060605522, 0.6893939393939394478, 0.6931818181818182323, 0.6969696969696970168, 0.7007575757575758013, 0.7045454545454545858, 0.7083333333333333703, 0.7121212121212121549, 0.7159090909090909394, 0.7196969696969697239, 0.7234848484848485084, 0.7272727272727272929, 0.7310606060606060774, 0.7348484848484848619, 0.7386363636363636465, 0.7424242424242424310, 0.7462121212121212155, 0.7500000000000000000, 0.7537878787878787845, 0.7575757575757575690, 0.7613636363636363535, 0.7651515151515151381, 0.7689393939393939226, 0.7727272727272727071, 0.7765151515151514916, 0.7803030303030302761, 0.7840909090909090606, 0.7878787878787878451, 0.7916666666666666297, 0.7954545454545454142, 0.7992424242424241987, 0.8030303030303029832, 0.8068181818181817677, 0.8106060606060605522, 0.8143939393939394478, 0.8181818181818182323, 0.8219696969696970168, 0.8257575757575758013, 0.8295454545454545858, 0.8333333333333333703, 0.8371212121212121549, 0.8409090909090909394, 0.8446969696969697239, 0.8484848484848485084, 0.8522727272727272929, 0.8560606060606060774, 0.8598484848484848619, 0.8636363636363636465, 0.8674242424242424310, 0.8712121212121212155, 0.8750000000000000000, 0.8787878787878787845, 0.8825757575757575690, 0.8863636363636363535, 0.8901515151515151381, 0.8939393939393939226, 0.8977272727272727071, 0.9015151515151514916, 0.9053030303030302761, 0.9090909090909090606, 0.9128787878787878451, 0.9166666666666666297, 0.9204545454545454142, 0.9242424242424241987, 0.9280303030303029832, 0.9318181818181817677, 0.9356060606060605522, 0.9393939393939394478, 0.9431818181818182323, 0.9469696969696970168, 0.9507575757575758013, 0.9545454545454545858, 0.9583333333333333703, 0.9621212121212121549, 0.9659090909090909394 ),
 .UNSPECIFIED. ) 
 GEOMETRIC_REPRESENTATION_ITEM ( )  RATIONAL_B_SPLINE_SURFACE ( (
 ( 1.000000000000000000, 0.9659258262890683122, 1.000000000000000000, 0.9659258262890683122, 1.000000000000000000, 0.9659258262890683122, 1.000000000000000000, 0.9659258262890683122, 1.000000000000000000, 0.9659258262890683122, 1.000000000000000000, 0.9659258262890683122, 1.000000000000000000, 0.9659258262890683122, 1.000000000000000000, 0.9659258262890683122, 1.000000000000000000, 0.9659258262890683122, 1.000000000000000000, 0.9659258262890683122, 1.000000000000000000, 0.9659258262890683122, 1.000000000000000000, 0.9659258262890683122, 1.000000000000000000, 0.9659258262890683122, 1.000000000000000000, 0.9659258262890683122, 1.000000000000000000, 0.9659258262890683122, 1.000000000000000000, 0.9659258262890683122, 1.000000000000000000, 0.9659258262890683122, 1.000000000000000000, 0.9659258262890683122, 1.000000000000000000, 0.9659258262890683122, 1.000000000000000000, 0.9659258262890683122, 1.000000000000000000, 0.9659258262890683122, 1.000000000000000000, 0.9659258262890683122, 1.000000000000000000, 0.9659258262890683122, 1.000000000000000000, 0.9659258262890683122, 1.000000000000000000, 0.9659258262890683122, 1.000000000000000000, 0.9659258262890683122, 1.000000000000000000, 0.9659258262890683122, 1.000000000000000000, 0.9659258262890683122, 1.000000000000000000, 0.9659258262890683122, 1.000000000000000000, 0.9659258262890683122, 1.000000000000000000, 0.9659258262890683122, 1.000000000000000000, 0.9659258262890683122, 1.000000000000000000, 0.9659258262890683122, 1.000000000000000000, 0.9659258262890683122, 1.000000000000000000, 0.9659258262890683122, 1.000000000000000000, 0.9659258262890683122, 1.000000000000000000, 0.9659258262890683122, 1.000000000000000000, 0.9659258262890683122, 1.000000000000000000, 0.9659258262890683122, 1.000000000000000000, 0.9659258262890683122, 1.000000000000000000, 0.9659258262890683122, 1.000000000000000000, 0.9659258262890683122, 1.000000000000000000, 0.9659258262890683122, 1.000000000000000000, 0.9659258262890683122, 1.000000000000000000, 0.9659258262890683122, 1.000000000000000000, 0.9659258262890683122, 1.000000000000000000, 0.9659258262890683122, 1.000000000000000000, 0.9659258262890683122, 1.000000000000000000, 0.9659258262890683122, 1.000000000000000000, 0.9659258262890683122, 1.000000000000000000, 0.9659258262890683122, 1.000000000000000000, 0.9659258262890683122, 1.000000000000000000, 0.9659258262890683122, 1.000000000000000000, 0.9659258262890683122, 1.000000000000000000, 0.9659258262890683122, 1.000000000000000000, 0.9659258262890683122, 1.000000000000000000, 0.9659258262890683122, 1.000000000000000000, 0.9659258262890683122, 1.000000000000000000, 0.9659258262890683122, 1.000000000000000000, 0.9659258262890683122, 1.000000000000000000, 0.9659258262890683122, 1.000000000000000000, 0.9659258262890683122, 1.000000000000000000, 0.9659258262890683122, 1.000000000000000000, 0.9659258262890683122, 1.000000000000000000, 0.9659258262890683122, 1.000000000000000000, 0.9659258262890683122, 1.000000000000000000, 0.9659258262890683122, 1.000000000000000000, 0.9659258262890683122, 1.000000000000000000, 0.9659258262890683122, 1.000000000000000000, 0.9659258262890683122, 1.000000000000000000, 0.9659258262890683122, 1.000000000000000000, 0.9659258262890683122, 1.000000000000000000, 0.9659258262890683122, 1.000000000000000000, 0.9659258262890683122, 1.000000000000000000, 0.9659258262890683122, 1.000000000000000000, 0.9659258262890683122, 1.000000000000000000, 0.9659258262890683122, 1.000000000000000000, 0.9659258262890683122, 1.000000000000000000, 0.9659258262890683122, 1.000000000000000000, 0.9659258262890683122, 1.000000000000000000, 0.9659258262890683122, 1.000000000000000000, 0.9659258262890683122, 1.000000000000000000, 0.9659258262890683122, 1.000000000000000000, 0.9659258262890683122, 1.000000000000000000, 0.9659258262890683122, 1.000000000000000000, 0.9659258262890683122, 1.000000000000000000, 0.9659258262890683122, 1.000000000000000000, 0.9659258262890683122, 1.000000000000000000, 0.9659258262890683122, 1.000000000000000000, 0.9659258262890683122, 1.000000000000000000, 0.9659258262890683122, 1.000000000000000000, 0.9659258262890683122, 1.000000000000000000, 0.9659258262890683122, 1.000000000000000000, 0.9659258262890683122, 1.000000000000000000, 0.9659258262890683122, 1.000000000000000000, 0.9659258262890683122, 1.000000000000000000, 0.9659258262890683122, 1.000000000000000000, 0.9659258262890683122, 1.000000000000000000, 0.9659258262890683122, 1.000000000000000000, 0.9659258262890683122, 1.000000000000000000, 0.9659258262890683122, 1.000000000000000000, 0.9659258262890683122, 1.000000000000000000, 0.9659258262890683122, 1.000000000000000000, 0.9659258262890683122, 1.000000000000000000, 0.9659258262890683122, 1.000000000000000000, 0.9659258262890683122, 1.000000000000000000, 0.9659258262890683122, 1.000000000000000000, 0.9659258262890683122, 1.000000000000000000, 0.9659258262890683122, 1.000000000000000000, 0.9659258262890683122, 1.000000000000000000, 0.9659258262890683122, 1.000000000000000000, 0.9659258262890683122, 1.000000000000000000, 0.9659258262890683122, 1.000000000000000000, 0.9659258262890683122, 1.000000000000000000, 0.9659258262890683122, 1.000000000000000000, 0.9659258262890683122, 1.000000000000000000, 0.9659258262890683122, 1.000000000000000000, 0.9659258262890683122, 1.000000000000000000, 0.9659258262890683122, 1.000000000000000000, 0.9659258262890683122, 1.000000000000000000, 0.9659258262890683122, 1.000000000000000000, 0.9659258262890683122, 1.000000000000000000, 0.9659258262890683122, 1.000000000000000000, 0.9659258262890683122, 1.000000000000000000, 0.9659258262890683122, 1.000000000000000000, 0.9659258262890683122, 1.000000000000000000, 0.9659258262890683122, 1.000000000000000000, 0.9659258262890683122, 1.000000000000000000, 0.9659258262890683122, 1.000000000000000000, 0.9659258262890683122, 1.000000000000000000, 0.9659258262890683122, 1.000000000000000000, 0.9659258262890683122, 1.000000000000000000, 0.9659258262890683122, 1.000000000000000000, 0.9659258262890683122, 1.000000000000000000, 0.9659258262890683122, 1.000000000000000000, 0.9659258262890683122, 1.000000000000000000, 0.9659258262890683122, 1.000000000000000000, 0.9659258262890683122, 1.000000000000000000, 0.9659258262890683122, 1.000000000000000000, 0.9659258262890683122, 1.000000000000000000, 0.9659258262890683122, 1.000000000000000000, 0.9659258262890683122, 1.000000000000000000, 0.9659258262890683122, 1.000000000000000000, 0.9659258262890683122, 1.000000000000000000, 0.9659258262890683122, 1.000000000000000000, 0.9659258262890683122, 1.000000000000000000, 0.9659258262890683122, 1.000000000000000000, 0.9659258262890683122, 1.000000000000000000, 0.9659258262890683122, 1.000000000000000000, 0.9659258262890683122, 1.000000000000000000, 0.9659258262890683122, 1.000000000000000000, 0.9659258262890683122, 1.000000000000000000, 0.9659258262890683122, 1.000000000000000000, 0.9659258262890683122, 1.000000000000000000, 0.9659258262890683122, 1.000000000000000000, 0.9659258262890683122, 1.000000000000000000, 0.9659258262890683122, 1.000000000000000000, 0.9659258262890683122, 1.000000000000000000, 0.9659258262890683122, 1.000000000000000000, 0.9659258262890683122, 1.000000000000000000, 0.9659258262890683122, 1.000000000000000000, 0.9659258262890683122, 1.000000000000000000, 0.9659258262890683122, 1.000000000000000000, 0.9659258262890683122, 1.000000000000000000, 0.9659258262890683122, 1.000000000000000000, 0.9659258262890683122, 1.000000000000000000, 0.9659258262890683122, 1.000000000000000000, 0.9659258262890683122, 1.000000000000000000, 0.9659258262890683122, 1.000000000000000000, 0.9659258262890683122, 1.000000000000000000, 0.9659258262890683122, 1.000000000000000000, 0.9659258262890683122, 1.000000000000000000, 0.9659258262890683122, 1.000000000000000000, 0.9659258262890683122, 1.000000000000000000, 0.9659258262890683122, 1.000000000000000000, 0.9659258262890683122, 1.000000000000000000, 0.9659258262890683122, 1.000000000000000000, 0.9659258262890683122, 1.000000000000000000, 0.9659258262890683122, 1.000000000000000000, 0.9659258262890683122, 1.000000000000000000, 0.9659258262890683122, 1.000000000000000000, 0.9659258262890683122, 1.000000000000000000, 0.9659258262890683122, 1.000000000000000000, 0.9659258262890683122, 1.000000000000000000, 0.9659258262890683122, 1.000000000000000000, 0.9659258262890683122, 1.000000000000000000, 0.9659258262890683122, 1.000000000000000000, 0.9659258262890683122, 1.000000000000000000, 0.9659258262890683122, 1.000000000000000000, 0.9659258262890683122, 1.000000000000000000, 0.9659258262890683122, 1.000000000000000000, 0.9659258262890683122, 1.000000000000000000, 0.9659258262890683122, 1.000000000000000000, 0.9659258262890683122, 1.000000000000000000, 0.9659258262890683122, 1.000000000000000000, 0.9659258262890683122, 1.000000000000000000, 0.9659258262890683122, 1.000000000000000000, 0.9659258262890683122, 1.000000000000000000, 0.9659258262890683122, 1.000000000000000000, 0.9659258262890683122, 1.000000000000000000, 0.9659258262890683122, 1.000000000000000000, 0.9659258262890683122, 1.000000000000000000, 0.9659258262890683122, 1.000000000000000000, 0.9659258262890683122, 1.000000000000000000, 0.9659258262890683122, 1.000000000000000000, 0.9659258262890683122, 1.000000000000000000, 0.9659258262890683122, 1.000000000000000000, 0.9659258262890683122, 1.000000000000000000, 0.9659258262890683122, 1.000000000000000000, 0.9659258262890683122, 1.000000000000000000, 0.9659258262890683122, 1.000000000000000000, 0.9659258262890683122, 1.000000000000000000, 0.9659258262890683122, 1.000000000000000000, 0.9659258262890683122, 1.000000000000000000, 0.9659258262890683122, 1.000000000000000000, 0.9659258262890683122, 1.000000000000000000, 0.9659258262890683122, 1.000000000000000000, 0.9659258262890683122, 1.000000000000000000, 0.9659258262890683122, 1.000000000000000000, 0.9659258262890683122, 1.000000000000000000, 0.9659258262890683122, 1.000000000000000000, 0.9659258262890683122, 1.000000000000000000, 0.9659258262890683122, 1.000000000000000000, 0.9659258262890683122, 1.000000000000000000, 0.9659258262890683122, 1.000000000000000000, 0.9659258262890683122, 1.000000000000000000, 0.9659258262890683122, 1.000000000000000000, 0.9659258262890683122, 1.000000000000000000, 0.9659258262890683122, 1.000000000000000000, 0.9659258262890683122, 1.000000000000000000, 0.9659258262890683122, 1.000000000000000000, 0.9659258262890683122, 1.000000000000000000, 0.9659258262890683122, 1.000000000000000000, 0.9659258262890683122, 1.000000000000000000, 0.9659258262890683122, 1.000000000000000000, 0.9659258262890683122, 1.000000000000000000, 0.9659258262890683122, 1.000000000000000000, 0.9659258262890683122, 1.000000000000000000, 0.9659258262890683122, 1.000000000000000000, 0.9659258262890683122, 1.000000000000000000, 0.9659258262890683122, 1.000000000000000000, 0.9659258262890683122, 1.000000000000000000, 0.9659258262890683122, 1.000000000000000000, 0.9659258262890683122, 1.000000000000000000, 0.9659258262890683122, 1.000000000000000000, 0.9659258262890683122, 1.000000000000000000, 0.9659258262890683122, 1.000000000000000000, 0.9659258262890683122, 1.000000000000000000, 0.9659258262890683122, 1.000000000000000000, 0.9659258262890683122, 1.000000000000000000, 0.9659258262890683122, 1.000000000000000000, 0.9659258262890683122, 1.000000000000000000, 0.9659258262890683122, 1.000000000000000000, 0.9659258262890683122, 1.000000000000000000, 0.9659258262890683122, 1.000000000000000000),
 ( 1.000000000000000000, 0.9659258262890683122, 1.000000000000000000, 0.9659258262890683122, 1.000000000000000000, 0.9659258262890683122, 1.000000000000000000, 0.9659258262890683122, 1.000000000000000000, 0.9659258262890683122, 1.000000000000000000, 0.9659258262890683122, 1.000000000000000000, 0.9659258262890683122, 1.000000000000000000, 0.9659258262890683122, 1.000000000000000000, 0.9659258262890683122, 1.000000000000000000, 0.9659258262890683122, 1.000000000000000000, 0.9659258262890683122, 1.000000000000000000, 0.9659258262890683122, 1.000000000000000000, 0.9659258262890683122, 1.000000000000000000, 0.9659258262890683122, 1.000000000000000000, 0.9659258262890683122, 1.000000000000000000, 0.9659258262890683122, 1.000000000000000000, 0.9659258262890683122, 1.000000000000000000, 0.9659258262890683122, 1.000000000000000000, 0.9659258262890683122, 1.000000000000000000, 0.9659258262890683122, 1.000000000000000000, 0.9659258262890683122, 1.000000000000000000, 0.9659258262890683122, 1.000000000000000000, 0.9659258262890683122, 1.000000000000000000, 0.9659258262890683122, 1.000000000000000000, 0.9659258262890683122, 1.000000000000000000, 0.9659258262890683122, 1.000000000000000000, 0.9659258262890683122, 1.000000000000000000, 0.9659258262890683122, 1.000000000000000000, 0.9659258262890683122, 1.000000000000000000, 0.9659258262890683122, 1.000000000000000000, 0.9659258262890683122, 1.000000000000000000, 0.9659258262890683122, 1.000000000000000000, 0.9659258262890683122, 1.000000000000000000, 0.9659258262890683122, 1.000000000000000000, 0.9659258262890683122, 1.000000000000000000, 0.9659258262890683122, 1.000000000000000000, 0.9659258262890683122, 1.000000000000000000, 0.9659258262890683122, 1.000000000000000000, 0.9659258262890683122, 1.000000000000000000, 0.9659258262890683122, 1.000000000000000000, 0.9659258262890683122, 1.000000000000000000, 0.9659258262890683122, 1.000000000000000000, 0.9659258262890683122, 1.000000000000000000, 0.9659258262890683122, 1.000000000000000000, 0.9659258262890683122, 1.000000000000000000, 0.9659258262890683122, 1.000000000000000000, 0.9659258262890683122, 1.000000000000000000, 0.9659258262890683122, 1.000000000000000000, 0.9659258262890683122, 1.000000000000000000, 0.9659258262890683122, 1.000000000000000000, 0.9659258262890683122, 1.000000000000000000, 0.9659258262890683122, 1.000000000000000000, 0.9659258262890683122, 1.000000000000000000, 0.9659258262890683122, 1.000000000000000000, 0.9659258262890683122, 1.000000000000000000, 0.9659258262890683122, 1.000000000000000000, 0.9659258262890683122, 1.000000000000000000, 0.9659258262890683122, 1.000000000000000000, 0.9659258262890683122, 1.000000000000000000, 0.9659258262890683122, 1.000000000000000000, 0.9659258262890683122, 1.000000000000000000, 0.9659258262890683122, 1.000000000000000000, 0.9659258262890683122, 1.000000000000000000, 0.9659258262890683122, 1.000000000000000000, 0.9659258262890683122, 1.000000000000000000, 0.9659258262890683122, 1.000000000000000000, 0.9659258262890683122, 1.000000000000000000, 0.9659258262890683122, 1.000000000000000000, 0.9659258262890683122, 1.000000000000000000, 0.9659258262890683122, 1.000000000000000000, 0.9659258262890683122, 1.000000000000000000, 0.9659258262890683122, 1.000000000000000000, 0.9659258262890683122, 1.000000000000000000, 0.9659258262890683122, 1.000000000000000000, 0.9659258262890683122, 1.000000000000000000, 0.9659258262890683122, 1.000000000000000000, 0.9659258262890683122, 1.000000000000000000, 0.9659258262890683122, 1.000000000000000000, 0.9659258262890683122, 1.000000000000000000, 0.9659258262890683122, 1.000000000000000000, 0.9659258262890683122, 1.000000000000000000, 0.9659258262890683122, 1.000000000000000000, 0.9659258262890683122, 1.000000000000000000, 0.9659258262890683122, 1.000000000000000000, 0.9659258262890683122, 1.000000000000000000, 0.9659258262890683122, 1.000000000000000000, 0.9659258262890683122, 1.000000000000000000, 0.9659258262890683122, 1.000000000000000000, 0.9659258262890683122, 1.000000000000000000, 0.9659258262890683122, 1.000000000000000000, 0.9659258262890683122, 1.000000000000000000, 0.9659258262890683122, 1.000000000000000000, 0.9659258262890683122, 1.000000000000000000, 0.9659258262890683122, 1.000000000000000000, 0.9659258262890683122, 1.000000000000000000, 0.9659258262890683122, 1.000000000000000000, 0.9659258262890683122, 1.000000000000000000, 0.9659258262890683122, 1.000000000000000000, 0.9659258262890683122, 1.000000000000000000, 0.9659258262890683122, 1.000000000000000000, 0.9659258262890683122, 1.000000000000000000, 0.9659258262890683122, 1.000000000000000000, 0.9659258262890683122, 1.000000000000000000, 0.9659258262890683122, 1.000000000000000000, 0.9659258262890683122, 1.000000000000000000, 0.9659258262890683122, 1.000000000000000000, 0.9659258262890683122, 1.000000000000000000, 0.9659258262890683122, 1.000000000000000000, 0.9659258262890683122, 1.000000000000000000, 0.9659258262890683122, 1.000000000000000000, 0.9659258262890683122, 1.000000000000000000, 0.9659258262890683122, 1.000000000000000000, 0.9659258262890683122, 1.000000000000000000, 0.9659258262890683122, 1.000000000000000000, 0.9659258262890683122, 1.000000000000000000, 0.9659258262890683122, 1.000000000000000000, 0.9659258262890683122, 1.000000000000000000, 0.9659258262890683122, 1.000000000000000000, 0.9659258262890683122, 1.000000000000000000, 0.9659258262890683122, 1.000000000000000000, 0.9659258262890683122, 1.000000000000000000, 0.9659258262890683122, 1.000000000000000000, 0.9659258262890683122, 1.000000000000000000, 0.9659258262890683122, 1.000000000000000000, 0.9659258262890683122, 1.000000000000000000, 0.9659258262890683122, 1.000000000000000000, 0.9659258262890683122, 1.000000000000000000, 0.9659258262890683122, 1.000000000000000000, 0.9659258262890683122, 1.000000000000000000, 0.9659258262890683122, 1.000000000000000000, 0.9659258262890683122, 1.000000000000000000, 0.9659258262890683122, 1.000000000000000000, 0.9659258262890683122, 1.000000000000000000, 0.9659258262890683122, 1.000000000000000000, 0.9659258262890683122, 1.000000000000000000, 0.9659258262890683122, 1.000000000000000000, 0.9659258262890683122, 1.000000000000000000, 0.9659258262890683122, 1.000000000000000000, 0.9659258262890683122, 1.000000000000000000, 0.9659258262890683122, 1.000000000000000000, 0.9659258262890683122, 1.000000000000000000, 0.9659258262890683122, 1.000000000000000000, 0.9659258262890683122, 1.000000000000000000, 0.9659258262890683122, 1.000000000000000000, 0.9659258262890683122, 1.000000000000000000, 0.9659258262890683122, 1.000000000000000000, 0.9659258262890683122, 1.000000000000000000, 0.9659258262890683122, 1.000000000000000000, 0.9659258262890683122, 1.000000000000000000, 0.9659258262890683122, 1.000000000000000000, 0.9659258262890683122, 1.000000000000000000, 0.9659258262890683122, 1.000000000000000000, 0.9659258262890683122, 1.000000000000000000, 0.9659258262890683122, 1.000000000000000000, 0.9659258262890683122, 1.000000000000000000, 0.9659258262890683122, 1.000000000000000000, 0.9659258262890683122, 1.000000000000000000, 0.9659258262890683122, 1.000000000000000000, 0.9659258262890683122, 1.000000000000000000, 0.9659258262890683122, 1.000000000000000000, 0.9659258262890683122, 1.000000000000000000, 0.9659258262890683122, 1.000000000000000000, 0.9659258262890683122, 1.000000000000000000, 0.9659258262890683122, 1.000000000000000000, 0.9659258262890683122, 1.000000000000000000, 0.9659258262890683122, 1.000000000000000000, 0.9659258262890683122, 1.000000000000000000, 0.9659258262890683122, 1.000000000000000000, 0.9659258262890683122, 1.000000000000000000, 0.9659258262890683122, 1.000000000000000000, 0.9659258262890683122, 1.000000000000000000, 0.9659258262890683122, 1.000000000000000000, 0.9659258262890683122, 1.000000000000000000, 0.9659258262890683122, 1.000000000000000000, 0.9659258262890683122, 1.000000000000000000, 0.9659258262890683122, 1.000000000000000000, 0.9659258262890683122, 1.000000000000000000, 0.9659258262890683122, 1.000000000000000000, 0.9659258262890683122, 1.000000000000000000, 0.9659258262890683122, 1.000000000000000000, 0.9659258262890683122, 1.000000000000000000, 0.9659258262890683122, 1.000000000000000000, 0.9659258262890683122, 1.000000000000000000, 0.9659258262890683122, 1.000000000000000000, 0.9659258262890683122, 1.000000000000000000, 0.9659258262890683122, 1.000000000000000000, 0.9659258262890683122, 1.000000000000000000, 0.9659258262890683122, 1.000000000000000000, 0.9659258262890683122, 1.000000000000000000, 0.9659258262890683122, 1.000000000000000000, 0.9659258262890683122, 1.000000000000000000, 0.9659258262890683122, 1.000000000000000000, 0.9659258262890683122, 1.000000000000000000, 0.9659258262890683122, 1.000000000000000000, 0.9659258262890683122, 1.000000000000000000, 0.9659258262890683122, 1.000000000000000000, 0.9659258262890683122, 1.000000000000000000, 0.9659258262890683122, 1.000000000000000000, 0.9659258262890683122, 1.000000000000000000, 0.9659258262890683122, 1.000000000000000000, 0.9659258262890683122, 1.000000000000000000, 0.9659258262890683122, 1.000000000000000000, 0.9659258262890683122, 1.000000000000000000, 0.9659258262890683122, 1.000000000000000000, 0.9659258262890683122, 1.000000000000000000, 0.9659258262890683122, 1.000000000000000000, 0.9659258262890683122, 1.000000000000000000, 0.9659258262890683122, 1.000000000000000000, 0.9659258262890683122, 1.000000000000000000, 0.9659258262890683122, 1.000000000000000000, 0.9659258262890683122, 1.000000000000000000, 0.9659258262890683122, 1.000000000000000000, 0.9659258262890683122, 1.000000000000000000, 0.9659258262890683122, 1.000000000000000000, 0.9659258262890683122, 1.000000000000000000, 0.9659258262890683122, 1.000000000000000000, 0.9659258262890683122, 1.000000000000000000, 0.9659258262890683122, 1.000000000000000000, 0.9659258262890683122, 1.000000000000000000, 0.9659258262890683122, 1.000000000000000000, 0.9659258262890683122, 1.000000000000000000, 0.9659258262890683122, 1.000000000000000000, 0.9659258262890683122, 1.000000000000000000, 0.9659258262890683122, 1.000000000000000000, 0.9659258262890683122, 1.000000000000000000, 0.9659258262890683122, 1.000000000000000000, 0.9659258262890683122, 1.000000000000000000, 0.9659258262890683122, 1.000000000000000000, 0.9659258262890683122, 1.000000000000000000, 0.9659258262890683122, 1.000000000000000000, 0.9659258262890683122, 1.000000000000000000, 0.9659258262890683122, 1.000000000000000000, 0.9659258262890683122, 1.000000000000000000, 0.9659258262890683122, 1.000000000000000000, 0.9659258262890683122, 1.000000000000000000, 0.9659258262890683122, 1.000000000000000000, 0.9659258262890683122, 1.000000000000000000, 0.9659258262890683122, 1.000000000000000000, 0.9659258262890683122, 1.000000000000000000, 0.9659258262890683122, 1.000000000000000000, 0.9659258262890683122, 1.000000000000000000, 0.9659258262890683122, 1.000000000000000000, 0.9659258262890683122, 1.000000000000000000, 0.9659258262890683122, 1.000000000000000000, 0.9659258262890683122, 1.000000000000000000, 0.9659258262890683122, 1.000000000000000000, 0.9659258262890683122, 1.000000000000000000, 0.9659258262890683122, 1.000000000000000000, 0.9659258262890683122, 1.000000000000000000, 0.9659258262890683122, 1.000000000000000000, 0.9659258262890683122, 1.000000000000000000, 0.9659258262890683122, 1.000000000000000000, 0.9659258262890683122, 1.000000000000000000, 0.9659258262890683122, 1.000000000000000000, 0.9659258262890683122, 1.000000000000000000) ) ) 
 REPRESENTATION_ITEM ( '' )  SURFACE ( )  );
#26164=CARTESIAN_POINT ( 'NONE',  ( 0.05249343832021075018, 0.2306618581243847221, -0.2411417322834647770 ) ) ;
#26165=CARTESIAN_POINT ( 'NONE',  ( 0.04593175853018440641, -0.6692913385826771977, 0.1292274648535927661 ) ) ;
#26167=CARTESIAN_POINT ( 'NONE',  ( -1.076115485564303809, 0.2306618581243848609, 0.2411417322834645549 ) ) ;
#26168=CARTESIAN_POINT ( 'NONE',  ( -0.3674540682414689785, 0.2306618581243848609, 0.2411417322834645549 ) ) ;
#26169=CARTESIAN_POINT ( 'NONE',  ( 0.02624671916010564918, -0.5023911411419708095, -0.1820866141732282451 ) ) ;
#26170=CARTESIAN_POINT ( 'NONE',  ( 1.587926509186352586, -0.4281496062992127816, -0.4176697321401328100 ) ) ;
#26171=CARTESIAN_POINT ( 'NONE',  ( 1.437007874015748810, -0.5400638737290845981, -0.3530559997133363437 ) ) ;
#26172=CARTESIAN_POINT ( 'NONE',  ( -0.6430446194225716283, -0.4281496062992124485, 0.4176697321401328655 ) ) ;
#26174=CARTESIAN_POINT ( 'NONE',  ( 1.246719160104987623, -0.4281496062992124485, 0.4176697321401328655 ) ) ;
#26175=CARTESIAN_POINT ( 'NONE',  ( 0.5249343832021003964, 0.1539470093639521697, -0.1968503937007875793 ) ) ;
#26176=VERTEX_POINT ( 'NONE', #77656 ) ;
#26177=ORIENTED_EDGE ( 'NONE', *, *, #46912, .T. ) ;
#26178=CARTESIAN_POINT ( 'NONE',  ( 0.3280839895013130669, -0.4281496062992127816, -0.4176697321401328100 ) ) ;
#26179=CARTESIAN_POINT ( 'NONE',  ( -0.4790026246719154557, -0.2845877964562159024, 0.3641732283464567677 ) ) ;
#26180=CARTESIAN_POINT ( 'NONE',  ( 1.528871391076116026, 0.1771653543307087630, 0.09757992244046791164 ) ) ;
#26184=CARTESIAN_POINT ( 'NONE',  ( 1.509186351706037543, -0.4281496062992127816, -0.4176697321401328100 ) ) ;
#26187=CARTESIAN_POINT ( 'NONE',  ( -0.1640419947506555343, -0.3162353388693405765, 0.4822834645669290543 ) ) ;
#26189=CARTESIAN_POINT ( 'NONE',  ( -1.555118110236219930, 0.1660481256975885056, 0.3530559997133364547 ) ) ;
#26190=CARTESIAN_POINT ( 'NONE',  ( 0.1246719160104994284, -0.6692913385826771977, 0.1292274648535927661 ) ) ;
#26192=CARTESIAN_POINT ( 'NONE',  ( 1.614173228346457378, -0.6692913385826771977, 8.415575281601705876E-17 ) ) ;
#26193=CARTESIAN_POINT ( 'NONE',  ( 0.4790026246719167324, -0.05778040916215522460, 0.4822834645669289988 ) ) ;
#26194=CARTESIAN_POINT ( 'NONE',  ( 1.089238845144357759, -0.004921259842519870586, -0.3153832671262229437 ) ) ;
#26195=LINE ( 'NONE', #53110, #80207 ) ;
#26196=CARTESIAN_POINT ( 'NONE',  ( 0.6692913385826778638, -0.5511811023622047445, 6.969142054262312111E-17 ) ) ;
#26197=CARTESIAN_POINT ( 'NONE',  ( -1.108923884514435132, -0.05778040916215560624, -0.4822834645669293319 ) ) ;
#26199=CARTESIAN_POINT ( 'NONE',  ( 1.128608923884515169, -0.6046776061558809534, -0.2411417322834644161 ) ) ;
#26201=CARTESIAN_POINT ( 'NONE',  ( 0.7086614173228353852, -0.1870078740157479769, 0.4822834645669291653 ) ) ;
#26203=DIRECTION ( 'NONE',  ( -0.7071067811865472397, 0.000000000000000000, -0.7071067811865476838 ) ) ;
#26204=CARTESIAN_POINT ( 'NONE',  ( 0.3477690288713918276, 0.1771653543307087630, 0.09757992244046791164 ) ) ;
#26205=B_SPLINE_CURVE_WITH_KNOTS ( 'NONE', 3,
 ( #82811, #74867, #69362, #62213, #75685, #56306, #69772 ),
 .UNSPECIFIED., .F., .F.,
 ( 4, 3, 4 ),
 ( 3.643951726750583631E-17, 0.001246232571205249445, 0.002492492258783241162 ),
 .UNSPECIFIED. ) ;
#26206=CARTESIAN_POINT ( 'NONE',  ( 0.4855643044619430415, -0.4281496062992127816, -0.4176697321401328100 ) ) ;
#26207=CARTESIAN_POINT ( 'NONE',  ( 1.673228346456693494, 0.07958543189024085140, 0.2665933059059887866 ) ) ;
#26208=CARTESIAN_POINT ( 'NONE',  ( -1.076115485564303809, 0.1283753931104748280, 0.1820866141732283561 ) ) ;
#26209=CARTESIAN_POINT ( 'NONE',  ( -1.076115485564303809, 0.2306618581243848609, 0.2411417322834645549 ) ) ;
#26210=CARTESIAN_POINT ( 'NONE',  ( 1.076115485564305141, 0.2306618581243847221, -0.2411417322834647770 ) ) ;
#26211=CARTESIAN_POINT ( 'NONE',  ( -1.095800524934382292, -0.05778040916215522460, 0.4822834645669289988 ) ) ;
#26212=CARTESIAN_POINT ( 'NONE',  ( 1.095800524934383846, -0.05778040916215560624, -0.4822834645669293319 ) ) ;
#26213=CARTESIAN_POINT ( 'NONE',  ( -1.463254593175852492, 0.1771653543307087630, 0.09757992244046791164 ) ) ;
#26215=CARTESIAN_POINT ( 'NONE',  ( 0.9055118110236227702, -0.6692913385826771977, 8.415575281601705876E-17 ) ) ;
#26217=CARTESIAN_POINT ( 'NONE',  ( -0.08943933388982759636, 1.809133623825372073E-16, -0.4118484887281974038 ) ) ;
#26218=CARTESIAN_POINT ( 'NONE',  ( 1.482939632545932307, -0.4281496062992124485, 0.4176697321401328655 ) ) ;
#26219=CARTESIAN_POINT ( 'NONE',  ( -1.095800524934382292, -0.08942795157527998196, 0.3641732283464567121 ) ) ;
#26221=CARTESIAN_POINT ( 'NONE',  ( -1.397637795275589623, -0.4536011799217368745, -0.2665933059059886201 ) ) ;
#26222=CARTESIAN_POINT ( 'NONE',  ( -0.5183727034120726440, 0.1771653543307087630, 0.09757992244046791164 ) ) ;
#26223=CARTESIAN_POINT ( 'NONE',  ( -1.568241469816272105, -0.08942795157527998196, 0.3641732283464567121 ) ) ;
#26224=CARTESIAN_POINT ( 'NONE',  ( 0.9317585301837276734, -0.3690944881889763329, 0.3153832671262228327 ) ) ;
#26225=CARTESIAN_POINT ( 'NONE',  ( 0.6758530183727039509, -0.6692913385826771977, 0.1292274648535927661 ) ) ;
#26226=CARTESIAN_POINT ( 'NONE',  ( 1.266404199475066328, -0.05778040916215522460, 0.4822834645669289988 ) ) ;
#26227=CARTESIAN_POINT ( 'NONE',  ( 0.02624671916010564918, -0.6046776061558809534, -0.2411417322834644161 ) ) ;
#26228=CARTESIAN_POINT ( 'NONE',  ( 0.7414698162729663755, -0.5511811023622048555, -0.09757992244046775898 ) ) ;
#26229=CARTESIAN_POINT ( 'NONE',  ( 1.581364829396326277, -0.05778040916215522460, 0.4822834645669289988 ) ) ;
#26231=CARTESIAN_POINT ( 'NONE',  ( -1.476377952755905110, 0.1660481256975885056, 0.3530559997133364547 ) ) ;
#26232=CARTESIAN_POINT ( 'NONE',  ( -0.7086614173228339419, -0.1870078740157480879, -0.4822834645669291653 ) ) ;
#26234=FACE_OUTER_BOUND ( 'NONE', #73824, .T. ) ;
#26235=CARTESIAN_POINT ( 'NONE',  ( -0.09186351706036689768, 0.05413385826771626580, -0.4176697321401330321 ) ) ;
#26236=CARTESIAN_POINT ( 'NONE',  ( -0.4265091863517051496, -0.6692913385826771977, 0.1292274648535927661 ) ) ;
#26238=CARTESIAN_POINT ( 'NONE',  ( 0.5314960629921264834, 0.1660481256975883668, -0.3530559997133364547 ) ) ;
#26240=AXIS2_PLACEMENT_3D ( 'NONE', #7854, #46132, #71826 ) ;
#26244=EDGE_CURVE ( 'NONE', #53395, #80562, #71751, .T. ) ;
#26246=CARTESIAN_POINT ( 'NONE',  ( -0.9383202099737524282, -0.08942795157527998196, 0.3641732283464567121 ) ) ;
#26248=CARTESIAN_POINT ( 'NONE',  ( -1.325459317585300889, -0.4281496062992127816, -0.4176697321401328100 ) ) ;
#26250=CARTESIAN_POINT ( 'NONE',  ( 0.4265091863517067594, 0.2952755905511811885, 0.1292274648535926551 ) ) ;
#26251=CARTESIAN_POINT ( 'NONE',  ( 5.463695987328526437E-16, -0.1870078740157479769, 0.3641732283464567677 ) ) ;
#26252=CARTESIAN_POINT ( 'NONE',  ( 1.115485564304462551, 0.05413385826771666132, 0.4176697321401328100 ) ) ;
#26253=CARTESIAN_POINT ( 'NONE',  ( 0.5118110236220478892, 0.2952755905511811885, 0.000000000000000000 ) ) ;
#26257=CARTESIAN_POINT ( 'NONE',  ( 1.272965879265092637, -0.4281496062992127816, -0.4176697321401328100 ) ) ;
#26258=CARTESIAN_POINT ( 'NONE',  ( 0.6036745406824153282, -0.6046776061558807314, 0.2411417322834647770 ) ) ;
#26259=CARTESIAN_POINT ( 'NONE',  ( 0.2821522309711292364, -0.6692913385826771977, 0.1292274648535927661 ) ) ;
#26260=CARTESIAN_POINT ( 'NONE',  ( 0.8989501312335963501, -0.5511811023622048555, -0.09757992244046775898 ) ) ;
#26261=CARTESIAN_POINT ( 'NONE',  ( 1.272965879265092637, -0.4281496062992127816, -0.4176697321401328100 ) ) ;
#26263=CARTESIAN_POINT ( 'NONE',  ( 0.1640419947506569498, -0.05778040916215522460, 0.4822834645669289988 ) ) ;
#26264=CARTESIAN_POINT ( 'NONE',  ( 1.010498687664042716, -0.4281496062992124485, 0.4176697321401328655 ) ) ;
#26265=CARTESIAN_POINT ( 'NONE',  ( 0.5511811023622055217, -0.1870078740157479769, 0.4822834645669291653 ) ) ;
#26266=CARTESIAN_POINT ( 'NONE',  ( 1.286089238845145033, -0.5023911411419708095, -0.1820866141732282451 ) ) ;
#26267=CARTESIAN_POINT ( 'NONE',  ( -1.062992125984250968, 0.2952755905511811885, 0.000000000000000000 ) ) ;
#26268=CARTESIAN_POINT ( 'NONE',  ( -1.509186351706035767, 0.05413385826771626580, -0.4176697321401330321 ) ) ;
#26269=CARTESIAN_POINT ( 'NONE',  ( 1.062992125984252745, -0.6692913385826771977, 8.415575281601705876E-17 ) ) ;
#26276=CARTESIAN_POINT ( 'NONE',  ( 1.496062992125985147, -0.1870078740157479769, 0.4822834645669291653 ) ) ;
#26277=CARTESIAN_POINT ( 'NONE',  ( 0.8202099737532813073, 0.1771653543307087630, 0.09757992244046791164 ) ) ;
#26282=CARTESIAN_POINT ( 'NONE',  ( -1.259842519685038686, -0.1870078740157480601, -0.3641732283464567677 ) ) ;
#26283=CARTESIAN_POINT ( 'NONE',  ( -1.633858267716534529, -0.4536011799217368745, -0.2665933059059886201 ) ) ;
#26285=CARTESIAN_POINT ( 'NONE',  ( -0.1706036745406816491, -0.4281496062992124485, 0.4176697321401328655 ) ) ;
#26286=CARTESIAN_POINT ( 'NONE',  ( 1.522309711286089939, -0.6046776061558809534, -0.2411417322834644161 ) ) ;
#26292=CARTESIAN_POINT ( 'NONE',  ( -1.102362204724408601, -0.1870078740157480601, -0.3641732283464567677 ) ) ;
#26293=( BOUNDED_CURVE ( )  B_SPLINE_CURVE ( 1, ( #53936, #80884 ),
 .UNSPECIFIED., .F., .F. ) 
 B_SPLINE_CURVE_WITH_KNOTS ( ( 2, 2 ),
 ( 5.421010862427522170E-20, 0.002000000000000006113 ),
 .UNSPECIFIED. ) 
 CURVE ( )  GEOMETRIC_REPRESENTATION_ITEM ( )  RATIONAL_B_SPLINE_CURVE ( ( 0.9875488213027530104, 0.9875488213027530104 ) ) 
 REPRESENTATION_ITEM ( '' )  );
#26294=CARTESIAN_POINT ( 'NONE',  ( -1.633858267716534529, 0.1660481256975885056, 0.3530559997133364547 ) ) ;
#26295=CARTESIAN_POINT ( 'NONE',  ( 0.4593175853018380828, 0.05413385826771626580, -0.4176697321401330321 ) ) ;
#26297=ORIENTED_EDGE ( 'NONE', *, *, #27035, .F. ) ;
#26300=CARTESIAN_POINT ( 'NONE',  ( 1.227034120734908917, 0.2952755905511810774, -0.1292274648535930714 ) ) ;
#26301=CARTESIAN_POINT ( 'NONE',  ( 1.601049868766404982, 0.1283753931104748280, 0.1820866141732283561 ) ) ;
#26303=CARTESIAN_POINT ( 'NONE',  ( -0.5643044619422565855, -0.004921259842519870586, -0.3153832671262229437 ) ) ;
#26305=CARTESIAN_POINT ( 'NONE',  ( -1.371391076115484609, -0.5511811023622046335, 0.09757992244046803654 ) ) ;
#26306=DIRECTION ( 'NONE',  ( 1.000000000000000000, -0.000000000000000000, -0.000000000000000000 ) ) ;
#26307=CARTESIAN_POINT ( 'NONE',  ( -0.4133858267716528645, -0.4536011799217367080, 0.2665933059059888421 ) ) ;
#26308=CARTESIAN_POINT ( 'NONE',  ( 0.09842519685039434474, -0.4536011799217368745, -0.2665933059059886201 ) ) ;
#26309=CARTESIAN_POINT ( 'NONE',  ( -0.06561679790026180015, -0.4281496062992127816, -0.4176697321401328100 ) ) ;
#26310=CARTESIAN_POINT ( 'NONE',  ( -1.227034120734907141, -0.5511811023622048555, -0.09757992244046775898 ) ) ;
#26312=CARTESIAN_POINT ( 'NONE',  ( 0.9383202099737536495, -0.3162353388693405765, 0.4822834645669290543 ) ) ;
#26313=CARTESIAN_POINT ( 'NONE',  ( -1.371391076115484609, -0.6692913385826771977, 0.1292274648535927661 ) ) ;
#26315=CARTESIAN_POINT ( 'NONE',  ( -0.4199475065616791736, 0.2306618581243847221, -0.2411417322834647770 ) ) ;
#26316=CARTESIAN_POINT ( 'NONE',  ( 0.09186351706036799403, -0.3690944881889765550, -0.3153832671262227771 ) ) ;
#26317=CARTESIAN_POINT ( 'NONE',  ( -1.010498687664041384, 0.05413385826771666132, 0.4176697321401328100 ) ) ;
#26318=CARTESIAN_POINT ( 'NONE',  ( 0.7939632545931766261, -0.2845877964562161244, -0.3641732283464567121 ) ) ;
#26319=CARTESIAN_POINT ( 'NONE',  ( -0.2034120734908131112, -0.5511811023622048555, -0.09757992244046775898 ) ) ;
#26320=CARTESIAN_POINT ( 'NONE',  ( -0.4461942257217840213, 0.2306618581243848609, 0.2411417322834645549 ) ) ;
#26321=FACE_OUTER_BOUND ( 'NONE', #34770, .T. ) ;
#26323=CARTESIAN_POINT ( 'NONE',  ( 1.496062992125985147, -0.1870078740157479769, 0.3641732283464567677 ) ) ;
#26324=CARTESIAN_POINT ( 'NONE',  ( -1.397637795275589623, -0.5400638737290845981, -0.3530559997133363437 ) ) ;
#26325=CARTESIAN_POINT ( 'NONE',  ( -1.443569553805773564, -0.6046776061558807314, 0.2411417322834647770 ) ) ;
#26328=CARTESIAN_POINT ( 'NONE',  ( -1.023622047244093558, -0.1870078740157479769, 0.3641732283464567677 ) ) ;
#26329=CARTESIAN_POINT ( 'NONE',  ( 0.8070866141732288002, 0.1660481256975885056, 0.3530559997133364547 ) ) ;
#26330=CARTESIAN_POINT ( 'NONE',  ( -1.128608923884513837, -0.5023911411419708095, 0.1820866141732285504 ) ) ;
#26332=CARTESIAN_POINT ( 'NONE',  ( -1.181102362204723644, -0.1870078740157480879, -0.4822834645669291653 ) ) ;
#26334=CARTESIAN_POINT ( 'NONE',  ( 0.8398950131233602345, -0.6046776061558807314, 0.2411417322834647770 ) ) ;
#26335=CARTESIAN_POINT ( 'NONE',  ( 0.3674540682414705883, -0.6046776061558807314, 0.2411417322834647770 ) ) ;
#26336=CARTESIAN_POINT ( 'NONE',  ( 1.561679790026247350, -0.4281496062992124485, 0.4176697321401328655 ) ) ;
#26337=CARTESIAN_POINT ( 'NONE',  ( -1.627296587926508442, -0.5023911411419708095, -0.1820866141732282451 ) ) ;
#26342=CARTESIAN_POINT ( 'NONE',  ( 0.8267716535433078384, -0.5511811023622047445, 6.969142054262312111E-17 ) ) ;
#26343=CARTESIAN_POINT ( 'NONE',  ( 0.2559055118110243332, -0.4536011799217368745, -0.2665933059059886201 ) ) ;
#26344=CARTESIAN_POINT ( 'NONE',  ( -0.05905511811023545637, -0.5400638737290845981, -0.3530559997133363437 ) ) ;
#26345=CARTESIAN_POINT ( 'NONE',  ( 1.364829396325459854, -0.6046776061558809534, -0.2411417322834644161 ) ) ;
#26347=CARTESIAN_POINT ( 'NONE',  ( 0.5577427821522316087, -0.08942795157527998196, 0.3641732283464567121 ) ) ;
#26348=CARTESIAN_POINT ( 'NONE',  ( -0.8989501312335946848, -0.6692913385826771977, 0.1292274648535927661 ) ) ;
#26349=CARTESIAN_POINT ( 'NONE',  ( -1.141732283464566011, 0.2952755905511811885, 0.000000000000000000 ) ) ;
#26350=CARTESIAN_POINT ( 'NONE',  ( 0.6692913385826778638, -0.6692913385826771977, 8.415575281601705876E-17 ) ) ;
#26354=ORIENTED_EDGE ( 'NONE', *, *, #63984, .F. ) ;
#26356=CARTESIAN_POINT ( 'NONE',  ( -1.377952755905511140, 0.2952755905511811885, 0.000000000000000000 ) ) ;
#26357=CARTESIAN_POINT ( 'NONE',  ( -0.5249343832020990641, 0.2306618581243848609, 0.2411417322834645549 ) ) ;
#26358=CARTESIAN_POINT ( 'NONE',  ( -0.9383202099737524282, -0.2845877964562161244, -0.3641732283464567121 ) ) ;
#26359=CARTESIAN_POINT ( 'NONE',  ( -0.6955380577427815458, 0.05413385826771666132, 0.4176697321401328100 ) ) ;
#26362=CARTESIAN_POINT ( 'NONE',  ( 1.646981627296588035, -0.3162353388693405765, 0.4822834645669290543 ) ) ;
#26363=CARTESIAN_POINT ( 'NONE',  ( -1.253280839895012377, -0.05778040916215522460, 0.4822834645669289988 ) ) ;
#26364=CARTESIAN_POINT ( 'NONE',  ( 0.1640419947506569498, -0.05778040916215522460, 0.4822834645669289988 ) ) ;
#26366=CARTESIAN_POINT ( 'NONE',  ( -0.8267716535433065062, 0.2952755905511811885, 0.000000000000000000 ) ) ;
#26368=CARTESIAN_POINT ( 'NONE',  ( 0.7283464566929140904, -0.5400638737290845981, -0.3530559997133363437 ) ) ;
#26370=CARTESIAN_POINT ( 'NONE',  ( -0.7808398950131222316, -0.2845877964562161244, -0.3641732283464567121 ) ) ;
#26374=CARTESIAN_POINT ( 'NONE',  ( -1.627296587926508442, -0.5023911411419708095, -0.1820866141732282451 ) ) ;
#26375=CARTESIAN_POINT ( 'NONE',  ( -1.213910761154854745, 0.2952755905511810774, -0.1292274648535930714 ) ) ;
#26376=CARTESIAN_POINT ( 'NONE',  ( -1.181102362204723644, -0.1870078740157479769, 0.4822834645669291653 ) ) ;
#26378=CARTESIAN_POINT ( 'NONE',  ( -0.9448818897637790704, -0.1870078740157479769, 0.4822834645669291653 ) ) ;
#26379=CARTESIAN_POINT ( 'NONE',  ( -1.312335958005248715, -0.6046776061558809534, -0.2411417322834644161 ) ) ;
#26380=CARTESIAN_POINT ( 'NONE',  ( -1.601049868766403650, 0.2306618581243847221, -0.2411417322834647770 ) ) ;
#26384=CARTESIAN_POINT ( 'NONE',  ( 0.2624671916010504757, 0.1283753931104748280, 0.1820866141732283561 ) ) ;
#26387=CARTESIAN_POINT ( 'NONE',  ( -0.2427821522309703550, -0.08942795157528024563, -0.3641732283464568787 ) ) ;
#26388=CARTESIAN_POINT ( 'NONE',  ( -0.9514435695538050464, -0.05778040916215560624, -0.4822834645669293319 ) ) ;
#26389=CARTESIAN_POINT ( 'NONE',  ( 1.253280839895013710, -0.3162353388693405765, 0.4822834645669290543 ) ) ;
#26390=CARTESIAN_POINT ( 'NONE',  ( -0.3280839895013117347, 0.05413385826771626580, -0.4176697321401330321 ) ) ;
#26392=ORIENTED_EDGE ( 'NONE', *, *, #12851, .F. ) ;
#26394=CARTESIAN_POINT ( 'NONE',  ( -0.9842519685039360366, 0.2952755905511811885, 0.000000000000000000 ) ) ;
#26395=CARTESIAN_POINT ( 'NONE',  ( 1.286089238845145033, 0.2306618581243848609, 0.2411417322834645549 ) ) ;
#26396=CARTESIAN_POINT ( 'NONE',  ( -1.502624671916009680, -0.08942795157528024563, -0.3641732283464568787 ) ) ;
#26403=CARTESIAN_POINT ( 'NONE',  ( -0.2165354330708654795, 0.1660481256975885056, 0.3530559997133364547 ) ) ;
#26404=CARTESIAN_POINT ( 'NONE',  ( -1.410761154855641575, -0.2845877964562161244, -0.3641732283464567121 ) ) ;
#26406=VECTOR ( 'NONE', #6937, 39.37007874015748143 ) ;
#26407=CARTESIAN_POINT ( 'NONE',  ( -0.8989501312335946848, 0.2952755905511810774, -0.1292274648535930714 ) ) ;
#26409=CARTESIAN_POINT ( 'NONE',  ( -1.338582677165353729, -0.1870078740157480879, -0.4822834645669291653 ) ) ;
#26410=LINE ( 'NONE', #50098, #79480 ) ;
#26411=CARTESIAN_POINT ( 'NONE',  ( -1.062992125984250968, 0.2952755905511811885, 0.000000000000000000 ) ) ;
#26412=CARTESIAN_POINT ( 'NONE',  ( -0.4790026246719154557, -0.3162353388693405765, 0.4822834645669290543 ) ) ;
#26414=CARTESIAN_POINT ( 'NONE',  ( 0.8661417322834652488, -0.1870078740157480601, -0.3641732283464567677 ) ) ;
#26416=CARTESIAN_POINT ( 'NONE',  ( 0.5839895013123367340, 0.1771653543307087630, 0.09757992244046791164 ) ) ;
#26417=CARTESIAN_POINT ( 'NONE',  ( 1.312335958005249825, 0.1283753931104746893, -0.1820866141732285504 ) ) ;
#26418=CARTESIAN_POINT ( 'NONE',  ( 1.410761154855643795, -0.3162353388693405765, 0.4822834645669290543 ) ) ;
#26419=CARTESIAN_POINT ( 'NONE',  ( 0.08530183727034192087, -0.08942795157527998196, 0.3641732283464567121 ) ) ;
#26421=CARTESIAN_POINT ( 'NONE',  ( -0.9711286089238838626, 0.2306618581243847221, -0.2411417322834647770 ) ) ;
#26422=CARTESIAN_POINT ( 'NONE',  ( 1.115485564304462551, 0.05413385826771666132, 0.4176697321401328100 ) ) ;
#26425=CARTESIAN_POINT ( 'NONE',  ( -0.3149606299212590610, -0.1870078740157480601, -0.3641732283464567677 ) ) ;
#26427=CARTESIAN_POINT ( 'NONE',  ( 0.4133858267716541968, 0.1660481256975885056, 0.3530559997133364547 ) ) ;
#26429=CARTESIAN_POINT ( 'NONE',  ( 1.135170603674541256, 0.1771653543307087630, 0.09757992244046791164 ) ) ;
#26430=CARTESIAN_POINT ( 'NONE',  ( 0.3280839895013130669, -0.004921259842519576551, 0.3153832671262227771 ) ) ;
#26431=CARTESIAN_POINT ( 'NONE',  ( -0.4790026246719152336, -0.05778040916215560624, -0.4822834645669293319 ) ) ;
#26432=CARTESIAN_POINT ( 'NONE',  ( -1.430446194225721390, -0.4281496062992124485, 0.4176697321401328655 ) ) ;
#26433=CARTESIAN_POINT ( 'NONE',  ( -0.5249343832020990641, 0.1283753931104748280, 0.1820866141732283561 ) ) ;
#26435=CARTESIAN_POINT ( 'NONE',  ( 0.6627296587926517768, -0.6692913385826773087, -0.1292274648535924053 ) ) ;
#26436=CARTESIAN_POINT ( 'NONE',  ( -0.8398950131233585692, 0.2306618581243848609, 0.2411417322834645549 ) ) ;
#26439=CARTESIAN_POINT ( 'NONE',  ( 0.2362204724409456558, -0.1870078740157480601, -0.3641732283464567677 ) ) ;
#26440=CARTESIAN_POINT ( 'NONE',  ( -0.8464566929133852113, 0.1660481256975885056, 0.3530559997133364547 ) ) ;
#26441=CARTESIAN_POINT ( 'NONE',  ( -1.305774278215222184, 0.2952755905511811885, 0.1292274648535926551 ) ) ;
#26442=CARTESIAN_POINT ( 'NONE',  ( -1.161417322834644716, 0.07958543189024085140, 0.2665933059059887866 ) ) ;
#26443=CARTESIAN_POINT ( 'NONE',  ( 1.640419947506562393, -0.4281496062992124485, 0.4176697321401328655 ) ) ;
#26444=CARTESIAN_POINT ( 'NONE',  ( -1.062992125984250968, -0.5511811023622047445, 6.969142054262312111E-17 ) ) ;
#26445=CARTESIAN_POINT ( 'NONE',  ( -1.653543307086613234, -0.1870078740157480601, -0.3641732283464567677 ) ) ;
#26446=CARTESIAN_POINT ( 'NONE',  ( 1.181102362204724976, -0.1870078740157480879, -0.4822834645669291653 ) ) ;
#26450=CARTESIAN_POINT ( 'NONE',  ( -0.7426113562971994320, 1.972848275015058439, 0.5309055118110236338 ) ) ;
#26451=CARTESIAN_POINT ( 'NONE',  ( 1.581364829396326277, -0.08942795157527998196, 0.3641732283464567121 ) ) ;
#26452=CARTESIAN_POINT ( 'NONE',  ( -1.233595800524933894, 0.2306618581243848609, 0.2411417322834645549 ) ) ;
#26454=EDGE_CURVE ( 'NONE', #81796, #11874, #64189, .T. ) ;
#26455=CARTESIAN_POINT ( 'NONE',  ( 1.371391076115485719, -0.6692913385826773087, -0.1292274648535924053 ) ) ;
#26457=CARTESIAN_POINT ( 'NONE',  ( -0.7480314960629916854, 2.165354330708661124, 0.000000000000000000 ) ) ;
#26458=CARTESIAN_POINT ( 'NONE',  ( 0.6496062992125991586, -0.5400638737290845981, -0.3530559997133363437 ) ) ;
#26459=CARTESIAN_POINT ( 'NONE',  ( -0.03937007874015669567, 0.2952755905511811885, 0.000000000000000000 ) ) ;
#26464=CARTESIAN_POINT ( 'NONE',  ( 0.7349081364829402885, -0.5023911411419708095, -0.1820866141732282451 ) ) ;
#26469=CARTESIAN_POINT ( 'NONE',  ( 0.1312335958005255154, -0.6046776061558807314, 0.2411417322834647770 ) ) ;
#26470=CARTESIAN_POINT ( 'NONE',  ( 1.417322834645670104, -0.1870078740157479769, 0.4822834645669291653 ) ) ;
#26471=CARTESIAN_POINT ( 'NONE',  ( 0.6955380577427828781, -0.4281496062992124485, 0.4176697321401328655 ) ) ;
#26472=CARTESIAN_POINT ( 'NONE',  ( 1.056430446194226658, 0.2952755905511811885, 0.1292274648535926551 ) ) ;
#26473=CARTESIAN_POINT ( 'NONE',  ( 1.522309711286089939, -0.6046776061558809534, -0.2411417322834644161 ) ) ;
#26474=CARTESIAN_POINT ( 'NONE',  ( -0.6824146981627288167, 0.2306618581243848609, 0.2411417322834645549 ) ) ;
#26475=CARTESIAN_POINT ( 'NONE',  ( 0.04593175853018440641, 0.2952755905511810774, -0.1292274648535930714 ) ) ;
#26476=CARTESIAN_POINT ( 'NONE',  ( 1.397637795275591177, -0.5400638737290844871, 0.3530559997133364547 ) ) ;
#26477=CARTESIAN_POINT ( 'NONE',  ( 1.220472440944882386, -0.6692913385826771977, 8.415575281601705876E-17 ) ) ;
#26478=CARTESIAN_POINT ( 'NONE',  ( 1.108923884514436686, -0.3162353388693409650, -0.4822834645669289433 ) ) ;
#26479=CARTESIAN_POINT ( 'NONE',  ( -0.05905511811023545637, -0.5400638737290845981, -0.3530559997133363437 ) ) ;
#26481=CARTESIAN_POINT ( 'NONE',  ( 0.6299212598425204535, -0.1870078740157480601, -0.3641732283464567677 ) ) ;
#26484=VERTEX_POINT ( 'NONE', #39334 ) ;
#26485=CARTESIAN_POINT ( 'NONE',  ( -0.4658792650918627265, -0.08942795157527998196, 0.3641732283464567121 ) ) ;
#26486=CARTESIAN_POINT ( 'NONE',  ( 0.006561679790026889343, -0.3162353388693409650, -0.4822834645669289433 ) ) ;
#26488=CARTESIAN_POINT ( 'NONE',  ( 0.1968503937007881344, 0.2952755905511811885, 0.000000000000000000 ) ) ;
#26489=CARTESIAN_POINT ( 'NONE',  ( -0.1837270341207343505, -0.6046776061558807314, 0.2411417322834647770 ) ) ;
#26490=CARTESIAN_POINT ( 'NONE',  ( -0.9448818897637790704, -0.1870078740157479769, 0.4822834645669291653 ) ) ;
#26491=CARTESIAN_POINT ( 'NONE',  ( 1.476377952755906442, -0.4536011799217367080, 0.2665933059059888421 ) ) ;
#26494=CARTESIAN_POINT ( 'NONE',  ( 0.8333333333333340365, 0.1771653543307087075, -0.09757992244046823083 ) ) ;
#26495=CARTESIAN_POINT ( 'NONE',  ( 0.3871391076115493490, -0.3162353388693405765, 0.4822834645669290543 ) ) ;
#26496=CARTESIAN_POINT ( 'NONE',  ( 0.7480314960629927956, 0.2952755905511811885, 0.000000000000000000 ) ) ;
#26501=CARTESIAN_POINT ( 'NONE',  ( -0.05249343832020938322, -0.6046776061558809534, -0.2411417322834644161 ) ) ;
#26504=CARTESIAN_POINT ( 'NONE',  ( -1.023622047244093558, -0.1870078740157479769, 0.3641732283464567677 ) ) ;
#26505=CARTESIAN_POINT ( 'NONE',  ( 1.299212598425197429, 0.2952755905511811885, 0.000000000000000000 ) ) ;
#26506=CARTESIAN_POINT ( 'NONE',  ( 1.391076115485564868, 0.2306618581243847221, -0.2411417322834647770 ) ) ;
#26507=CARTESIAN_POINT ( 'NONE',  ( -0.2952755905511803003, -0.4536011799217368745, -0.2665933059059886201 ) ) ;
#26508=CARTESIAN_POINT ( 'NONE',  ( 0.6430446194225728496, 0.05413385826771666132, 0.4176697321401328100 ) ) ;
#26510=CARTESIAN_POINT ( 'NONE',  ( 0.2821522309711292364, 0.1771653543307087075, -0.09757992244046823083 ) ) ;
#26511=CARTESIAN_POINT ( 'NONE',  ( -0.01968503937007793844, -0.5400638737290844871, 0.3530559997133364547 ) ) ;
#26513=CARTESIAN_POINT ( 'NONE',  ( -1.049868766404198794, 0.2306618581243847221, -0.2411417322834647770 ) ) ;
#26514=CARTESIAN_POINT ( 'NONE',  ( 0.3346456692913390985, 0.07958543189024085140, 0.2665933059059887866 ) ) ;
#26516=CARTESIAN_POINT ( 'NONE',  ( -0.8202099737532801971, -0.6692913385826771977, 0.1292274648535927661 ) ) ;
#26517=CARTESIAN_POINT ( 'NONE',  ( -0.4396325459317577122, -0.5511811023622048555, -0.09757992244046775898 ) ) ;
#26519=CARTESIAN_POINT ( 'NONE',  ( -0.6102362204724400829, 0.1660481256975885056, 0.3530559997133364547 ) ) ;
#26520=CARTESIAN_POINT ( 'NONE',  ( -0.1509186351706028884, -0.3162353388693409650, -0.4822834645669289433 ) ) ;
#26521=CARTESIAN_POINT ( 'NONE',  ( 0.2887139107611556010, -0.5023911411419708095, 0.1820866141732285504 ) ) ;
#26523=CARTESIAN_POINT ( 'NONE',  ( 0.01968503937007957949, -0.5400638737290845981, -0.3530559997133363437 ) ) ;
#26526=CARTESIAN_POINT ( 'NONE',  ( -1.640419947506561060, -0.3690944881889765550, -0.3153832671262227771 ) ) ;
#26527=CARTESIAN_POINT ( 'NONE',  ( 0.7480314960629927956, 0.1771653543307087630, 0.000000000000000000 ) ) ;
#26528=CARTESIAN_POINT ( 'NONE',  ( 1.561679790026247350, -0.4281496062992124485, 0.4176697321401328655 ) ) ;
#26529=CARTESIAN_POINT ( 'NONE',  ( -0.8858267716535425107, 0.07958543189024071263, -0.2665933059059888421 ) ) ;
#26531=CARTESIAN_POINT ( 'NONE',  ( -1.358267716535432434, 0.07958543189024071263, -0.2665933059059888421 ) ) ;
#26532=CARTESIAN_POINT ( 'NONE',  ( -0.5708661417322825615, -0.5400638737290844871, 0.3530559997133364547 ) ) ;
#26533=CARTESIAN_POINT ( 'NONE',  ( -0.2821522309711278487, 0.2952755905511811885, 0.1292274648535926551 ) ) ;
#26534=CARTESIAN_POINT ( 'NONE',  ( 0.6955380577427828781, -0.3690944881889763329, 0.3153832671262228327 ) ) ;
#26536=CARTESIAN_POINT ( 'NONE',  ( 1.069553805774278610, -0.5511811023622046335, 0.09757992244046803654 ) ) ;
#26538=CARTESIAN_POINT ( 'NONE',  ( 0.4986876640419954376, -0.6046776061558809534, -0.2411417322834644161 ) ) ;
#26539=DIRECTION ( 'NONE',  ( 1.000000000000000000, -0.000000000000000000, -0.000000000000000000 ) ) ;
#26540=CARTESIAN_POINT ( 'NONE',  ( -0.7414698162729651543, 0.2952755905511810774, -0.1292274648535930714 ) ) ;
#26542=CARTESIAN_POINT ( 'NONE',  ( 1.305774278215223960, 0.1771653543307087075, -0.09757992244046823083 ) ) ;
#26543=CARTESIAN_POINT ( 'NONE',  ( 0.4527559055118117182, 0.1660481256975883668, -0.3530559997133364547 ) ) ;
#26544=CARTESIAN_POINT ( 'NONE',  ( 0.09186351706036827158, 0.05413385826771666132, 0.4176697321401328100 ) ) ;
#26546=CARTESIAN_POINT ( 'NONE',  ( 0.07874015748031558404, -0.1870078740157479769, 0.3641732283464567677 ) ) ;
#26547=CARTESIAN_POINT ( 'NONE',  ( 0.9317585301837276734, 0.05413385826771626580, -0.4176697321401330321 ) ) ;
#26548=CARTESIAN_POINT ( 'NONE',  ( -0.5314960629921254842, -0.4536011799217368745, -0.2665933059059886201 ) ) ;
#26549=CARTESIAN_POINT ( 'NONE',  ( -0.7874015748031489847, -0.1870078740157480879, -0.4822834645669291653 ) ) ;
#26551=CARTESIAN_POINT ( 'NONE',  ( -0.3346456692913377662, -0.5400638737290844871, 0.3530559997133364547 ) ) ;
#26553=CARTESIAN_POINT ( 'NONE',  ( -1.030183727034119867, -0.3162353388693405765, 0.4822834645669290543 ) ) ;
#26554=CARTESIAN_POINT ( 'NONE',  ( -0.7939632545931754048, -0.2845877964562159024, 0.3641732283464567677 ) ) ;
#26555=CARTESIAN_POINT ( 'NONE',  ( 5.463695987328526437E-16, -0.1870078740157479769, 0.4822834645669291653 ) ) ;
#26556=CARTESIAN_POINT ( 'NONE',  ( -1.167979002624671470, -0.4281496062992127816, -0.4176697321401328100 ) ) ;
#26557=CARTESIAN_POINT ( 'NONE',  ( -0.8333333333333323711, 0.2952755905511811885, 0.1292274648535926551 ) ) ;
#26559=CARTESIAN_POINT ( 'NONE',  ( 1.056430446194226658, 0.2952755905511811885, 0.1292274648535926551 ) ) ;
#26560=CARTESIAN_POINT ( 'NONE',  ( 0.8267716535433077274, 0.2952755905511811885, 0.000000000000000000 ) ) ;
#26561=CARTESIAN_POINT ( 'NONE',  ( 1.108923884514436686, -0.3162353388693409650, -0.4822834645669289433 ) ) ;
#26563=CARTESIAN_POINT ( 'NONE',  ( -1.535433070866141225, -0.6692913385826771977, 8.415575281601705876E-17 ) ) ;
#26564=CARTESIAN_POINT ( 'NONE',  ( -1.246719160104986512, 0.05413385826771666132, 0.4176697321401328100 ) ) ;
#26568=EDGE_CURVE ( 'NONE', #41893, #15840, #17092, .T. ) ;
#26569=CARTESIAN_POINT ( 'NONE',  ( -0.05905511811023545637, 0.07958543189024085140, 0.2665933059059887866 ) ) ;
#26572=CARTESIAN_POINT ( 'NONE',  ( 0.1312335958005255154, -0.6046776061558807314, 0.2411417322834647770 ) ) ;
#26573=CARTESIAN_POINT ( 'NONE',  ( -0.01968503937007793844, -0.5400638737290844871, 0.3530559997133364547 ) ) ;
#26576=CARTESIAN_POINT ( 'NONE',  ( -0.7677165354330699465, -0.4536011799217368745, -0.2665933059059886201 ) ) ;
#26578=CARTESIAN_POINT ( 'NONE',  ( 0.6102362204724416372, 0.1660481256975883668, -0.3530559997133364547 ) ) ;
#26579=CARTESIAN_POINT ( 'NONE',  ( 0.8398950131233602345, 0.1283753931104746893, -0.1820866141732285504 ) ) ;
#26580=CARTESIAN_POINT ( 'NONE',  ( -0.3608923884514428360, 0.2952755905511811885, 0.1292274648535926551 ) ) ;
#26582=CARTESIAN_POINT ( 'NONE',  ( -0.8333333333333323711, 0.2952755905511811885, 0.1292274648535926551 ) ) ;
#26583=CARTESIAN_POINT ( 'NONE',  ( 1.595398199321655275, 0.7375059713363276703, 0.1559797534342493575 ) ) ;
#26584=CARTESIAN_POINT ( 'NONE',  ( 1.312335958005250269, -0.6046776061558807314, 0.2411417322834647770 ) ) ;
#26585=CARTESIAN_POINT ( 'NONE',  ( 1.587926509186352586, -0.3690944881889765550, -0.3153832671262227771 ) ) ;
#26588=CARTESIAN_POINT ( 'NONE',  ( -0.2034120734908128059, 0.2952755905511811885, 0.1292274648535926551 ) ) ;
#26589=ORIENTED_EDGE ( 'NONE', *, *, #5285, .T. ) ;
#26591=CARTESIAN_POINT ( 'NONE',  ( -0.5708661417322828946, 0.1660481256975883668, -0.3530559997133364547 ) ) ;
#26592=CARTESIAN_POINT ( 'NONE',  ( 1.397637795275591177, -0.5400638737290844871, 0.3530559997133364547 ) ) ;
#26593=CARTESIAN_POINT ( 'NONE',  ( 1.279527559055118724, 0.1660481256975885056, 0.3530559997133364547 ) ) ;
#26594=CARTESIAN_POINT ( 'NONE',  ( 0.3215223097112867578, -0.05778040916215522460, 0.4822834645669289988 ) ) ;
#26595=CARTESIAN_POINT ( 'NONE',  ( -0.2887139107611542133, -0.6046776061558809534, -0.2411417322834644161 ) ) ;
#26597=CARTESIAN_POINT ( 'NONE',  ( -1.003937007874015297, -0.5400638737290845981, -0.3530559997133363437 ) ) ;
#26598=CARTESIAN_POINT ( 'NONE',  ( 0.006561679790026889343, -0.3162353388693409650, -0.4822834645669289433 ) ) ;
#26599=CARTESIAN_POINT ( 'NONE',  ( -0.07874015748031421014, -0.1870078740157479769, 0.3641732283464567677 ) ) ;
#26600=CARTESIAN_POINT ( 'NONE',  ( 1.594488188976378673, -0.5400638737290845981, -0.3530559997133363437 ) ) ;
#26601=CARTESIAN_POINT ( 'NONE',  ( 1.338582677165355062, -0.1870078740157479769, 0.4822834645669291653 ) ) ;
#26602=CARTESIAN_POINT ( 'NONE',  ( -0.5314960629921254842, -0.5400638737290845981, -0.3530559997133363437 ) ) ;
#26604=CARTESIAN_POINT ( 'NONE',  ( 1.279527559055118724, 0.1660481256975885056, 0.3530559997133364547 ) ) ;
#26605=CARTESIAN_POINT ( 'NONE',  ( 2.795275590551181466, 2.793565526369266916, 0.000000000000000000 ) ) ;
#26606=ORIENTED_EDGE ( 'NONE', *, *, #34823, .F. ) ;
#26607=CARTESIAN_POINT ( 'NONE',  ( 0.4330708661417329575, 0.2952755905511811885, 0.000000000000000000 ) ) ;
#26608=CARTESIAN_POINT ( 'NONE',  ( -0.1312335958005241554, 0.1283753931104748280, 0.1820866141732283561 ) ) ;
#26609=CARTESIAN_POINT ( 'NONE',  ( 1.292650918635171564, -0.5511811023622048555, -0.09757992244046775898 ) ) ;
#26610=CARTESIAN_POINT ( 'NONE',  ( -0.9321091654255228010, 0.004960608223778174841, 0.3437734562760193513 ) ) ;
#26612=CARTESIAN_POINT ( 'NONE',  ( -1.614173228346457378, 1.330640075373402897, -0.1372047244094477536 ) ) ;
#26613=CARTESIAN_POINT ( 'NONE',  ( 1.279527559055118724, 0.1660481256975885056, 0.3530559997133364547 ) ) ;
#26615=CARTESIAN_POINT ( 'NONE',  ( 0.2099737532808405305, 0.2306618581243847221, -0.2411417322834647770 ) ) ;
#26616=CARTESIAN_POINT ( 'NONE',  ( -1.548556430446193399, -0.6046776061558809534, -0.2411417322834644161 ) ) ;
#26617=CARTESIAN_POINT ( 'NONE',  ( -1.574803149606298636, -0.1870078740157479769, 0.4822834645669291653 ) ) ;
#26618=CARTESIAN_POINT ( 'NONE',  ( -0.1115485564304456306, 0.2952755905511810774, -0.1292274648535930714 ) ) ;
#26620=CARTESIAN_POINT ( 'NONE',  ( 1.548556430446194954, 0.2306618581243847221, -0.2411417322834647770 ) ) ;
#26621=CARTESIAN_POINT ( 'NONE',  ( 0.6889763779527563470, 0.1660481256975883668, -0.3530559997133364547 ) ) ;
#26622=CARTESIAN_POINT ( 'NONE',  ( 1.122047244094488860, -0.4536011799217368745, -0.2665933059059886201 ) ) ;
#26624=CARTESIAN_POINT ( 'NONE',  ( 0.8661417322834653598, -0.1870078740157479769, 0.3641732283464567677 ) ) ;
#26625=CARTESIAN_POINT ( 'NONE',  ( -1.181102362204723644, -0.1870078740157479769, 0.4822834645669291653 ) ) ;
#26627=CARTESIAN_POINT ( 'NONE',  ( 1.332020997375329197, -0.3162353388693405765, 0.4822834645669290543 ) ) ;
#26629=CARTESIAN_POINT ( 'NONE',  ( 0.5839895013123367340, 0.2952755905511811885, 0.1292274648535926551 ) ) ;
#26631=FACE_OUTER_BOUND ( 'NONE', #7245, .T. ) ;
#26632=CARTESIAN_POINT ( 'NONE',  ( 0.5052493438320215802, 0.1771653543307087630, 0.09757992244046791164 ) ) ;
#26634=CARTESIAN_POINT ( 'NONE',  ( 0.4068241469816281097, 0.05413385826771666132, 0.4176697321401328100 ) ) ;
#26635=CARTESIAN_POINT ( 'NONE',  ( 1.679790026246720025, 0.1283753931104748280, 0.1820866141732283561 ) ) ;
#26636=CARTESIAN_POINT ( 'NONE',  ( -0.8464566929133852113, -0.4536011799217368745, -0.2665933059059886201 ) ) ;
#26637=CARTESIAN_POINT ( 'NONE',  ( -1.102362204724408601, -0.1870078740157479769, 0.4822834645669291653 ) ) ;
#26638=CARTESIAN_POINT ( 'NONE',  ( -1.719160104986876103, 0.05413385826771666132, 0.4176697321401328100 ) ) ;
#26639=CARTESIAN_POINT ( 'NONE',  ( 0.9842519685039378130, -0.6692913385826771977, 8.415575281601705876E-17 ) ) ;
#26640=CARTESIAN_POINT ( 'NONE',  ( 1.607611548556431069, -0.6692913385826773087, -0.1292274648535924053 ) ) ;
#26642=CARTESIAN_POINT ( 'NONE',  ( 0.8595800524934390507, -0.05778040916215560624, -0.4822834645669293319 ) ) ;
#26645=CARTESIAN_POINT ( 'NONE',  ( 1.279527559055118724, -0.5400638737290845981, -0.3530559997133363437 ) ) ;
#26646=CARTESIAN_POINT ( 'NONE',  ( -1.279527559055116948, -0.4536011799217367080, 0.2665933059059888421 ) ) ;
#26647=CARTESIAN_POINT ( 'NONE',  ( 1.089238845144357759, -0.004921259842519870586, -0.3153832671262229437 ) ) ;
#26648=CARTESIAN_POINT ( 'NONE',  ( -1.502624671916009680, -0.2845877964562159024, 0.3641732283464567677 ) ) ;
#26649=CARTESIAN_POINT ( 'NONE',  ( -0.5971128608923877978, -0.5511811023622048555, -0.09757992244046775898 ) ) ;
#26651=CARTESIAN_POINT ( 'NONE',  ( 0.7480314960629927956, -0.5511811023622047445, 6.969142054262312111E-17 ) ) ;
#26652=CARTESIAN_POINT ( 'NONE',  ( 0.5380577427821529035, -0.4281496062992124485, 0.4176697321401328655 ) ) ;
#26653=CARTESIAN_POINT ( 'NONE',  ( 0.9842519685039375910, 0.2952755905511811885, 0.000000000000000000 ) ) ;
#26654=CARTESIAN_POINT ( 'NONE',  ( -0.07874015748031421014, -0.1870078740157479769, 0.4822834645669291653 ) ) ;
#26655=CARTESIAN_POINT ( 'NONE',  ( 0.7283464566929140904, -0.4536011799217368745, -0.2665933059059886201 ) ) ;
#26656=B_SPLINE_CURVE_WITH_KNOTS ( 'NONE', 3,
 ( #2029, #9178, #66421, #40329, #73149, #21792, #2453 ),
 .UNSPECIFIED., .F., .F.,
 ( 4, 3, 4 ),
 ( 1.561251128379126385E-17, 0.001246230184515585400, 0.002492489877932648965 ),
 .UNSPECIFIED. ) ;
#26657=CARTESIAN_POINT ( 'NONE',  ( 1.286089238845145033, 0.2306618581243848609, 0.2411417322834645549 ) ) ;
#26659=CARTESIAN_POINT ( 'NONE',  ( -0.7283464566929126471, 0.1660481256975883668, -0.3530559997133364547 ) ) ;
#26661=CARTESIAN_POINT ( 'NONE',  ( 0.2296587926509192634, -0.05778040916215560624, -0.4822834645669293319 ) ) ;
#26662=CARTESIAN_POINT ( 'NONE',  ( -0.2427821522309703550, -0.3162353388693405765, 0.4822834645669290543 ) ) ;
#26663=CARTESIAN_POINT ( 'NONE',  ( -0.1246719160104980823, 0.2952755905511811885, 0.1292274648535926551 ) ) ;
#26669=CARTESIAN_POINT ( 'NONE',  ( -0.8989501312335946848, 0.1771653543307087075, -0.09757992244046823083 ) ) ;
#26671=CARTESIAN_POINT ( 'NONE',  ( -0.9776902887139098386, -0.6692913385826771977, 0.1292274648535927661 ) ) ;
#26673=CARTESIAN_POINT ( 'NONE',  ( 0.2362204724409456558, -0.1870078740157479769, 0.4822834645669291653 ) ) ;
#26674=CARTESIAN_POINT ( 'NONE',  ( -0.4986876640419942164, -0.5023911411419708095, 0.1820866141732285504 ) ) ;
#26675=CARTESIAN_POINT ( 'NONE',  ( 1.148293963254593653, 0.2952755905511810774, -0.1292274648535930714 ) ) ;
#26676=CARTESIAN_POINT ( 'NONE',  ( 0.2099737532808405305, 0.2306618581243847221, -0.2411417322834647770 ) ) ;
#26680=CARTESIAN_POINT ( 'NONE',  ( 1.351706036745407680, 0.05413385826771666132, 0.4176697321401328100 ) ) ;
#26681=CARTESIAN_POINT ( 'NONE',  ( 0.4790026246719167324, -0.05778040916215522460, 0.4822834645669289988 ) ) ;
#26682=CARTESIAN_POINT ( 'NONE',  ( 0.2624671916010504757, -0.6046776061558809534, -0.2411417322834644161 ) ) ;
#26683=CARTESIAN_POINT ( 'NONE',  ( 1.338582677165355062, -0.1870078740157479769, 0.4822834645669291653 ) ) ;
#26686=CARTESIAN_POINT ( 'NONE',  ( -0.05905511811023545637, -0.5400638737290845981, -0.3530559997133363437 ) ) ;
#26687=CARTESIAN_POINT ( 'NONE',  ( 0.9251968503937015864, 0.1660481256975883668, -0.3530559997133364547 ) ) ;
#26688=CARTESIAN_POINT ( 'NONE',  ( 0.3608923884514443348, -0.6692913385826771977, 0.1292274648535927661 ) ) ;
#26689=CARTESIAN_POINT ( 'NONE',  ( 0.9645669291338591078, -0.4536011799217368745, -0.2665933059059886201 ) ) ;
#26690=CARTESIAN_POINT ( 'NONE',  ( -1.108923884514435132, -0.3162353388693405765, 0.4822834645669290543 ) ) ;
#26691=CARTESIAN_POINT ( 'NONE',  ( -1.417322834645668772, -0.1870078740157479769, 0.4822834645669291653 ) ) ;
#26692=CARTESIAN_POINT ( 'NONE',  ( 0.6824146981627303710, 0.2306618581243847221, -0.2411417322834647770 ) ) ;
#26698=CARTESIAN_POINT ( 'NONE',  ( 1.430446194225722500, -0.4281496062992127816, -0.4176697321401328100 ) ) ;
#26699=CARTESIAN_POINT ( 'NONE',  ( 1.115485564304462551, -0.004921259842519576551, 0.3153832671262227771 ) ) ;
#26701=CARTESIAN_POINT ( 'NONE',  ( -0.7080320533160963103, 2.401574803149606474, 0.4915354330708645025 ) ) ;
#26704=CARTESIAN_POINT ( 'NONE',  ( -1.318897637795274802, 0.07958543189024085140, 0.2665933059059887866 ) ) ;
#26705=CARTESIAN_POINT ( 'NONE',  ( 1.548556430446194954, -0.6046776061558807314, 0.2411417322834647770 ) ) ;
#26707=CARTESIAN_POINT ( 'NONE',  ( -0.4658792650918627265, -0.05778040916215522460, 0.4822834645669289988 ) ) ;
#26708=CARTESIAN_POINT ( 'NONE',  ( 1.023622047244095112, -0.1870078740157480879, -0.4822834645669291653 ) ) ;
#26709=ORIENTED_EDGE ( 'NONE', *, *, #79843, .T. ) ;
#26710=CARTESIAN_POINT ( 'NONE',  ( -1.528871391076114250, 0.2952755905511810774, -0.1292274648535930714 ) ) ;
#26711=CARTESIAN_POINT ( 'NONE',  ( -0.7197590744588117095, -5.642773921931522838E-15, -0.3954985857520079695 ) ) ;
#26714=CARTESIAN_POINT ( 'NONE',  ( -0.8464566929133852113, 0.07958543189024085140, 0.2665933059059887866 ) ) ;
#26717=CARTESIAN_POINT ( 'NONE',  ( 0.4002624671916016896, -0.05778040916215522460, 0.4822834645669289988 ) ) ;
#26721=CARTESIAN_POINT ( 'NONE',  ( 1.377952755905512472, 0.2952755905511811885, 0.000000000000000000 ) ) ;
#26722=CARTESIAN_POINT ( 'NONE',  ( 1.607611548556431069, 0.1771653543307087630, 0.09757992244046791164 ) ) ;
#26724=CARTESIAN_POINT ( 'NONE',  ( -0.9973753280839886548, -0.5023911411419708095, -0.1820866141732282451 ) ) ;
#26725=CARTESIAN_POINT ( 'NONE',  ( -1.469816272965878357, 0.1283753931104748280, 0.1820866141732283561 ) ) ;
#26727=CARTESIAN_POINT ( 'NONE',  ( 0.4068241469816279987, -0.4281496062992127816, -0.4176697321401328100 ) ) ;
#26728=CARTESIAN_POINT ( 'NONE',  ( -0.8464566929133852113, 0.07958543189024085140, 0.2665933059059887866 ) ) ;
#26729=CARTESIAN_POINT ( 'NONE',  ( 5.463695987328526437E-16, -0.1870078740157479769, 0.3641732283464567677 ) ) ;
#26730=CARTESIAN_POINT ( 'NONE',  ( 0.2887139107611556010, -0.6046776061558807314, 0.2411417322834647770 ) ) ;
#26731=CARTESIAN_POINT ( 'NONE',  ( -1.181102362204723644, -0.1870078740157479769, 0.3641732283464567677 ) ) ;
#26733=CARTESIAN_POINT ( 'NONE',  ( 0.8267716535433077274, 0.2952755905511811885, 0.000000000000000000 ) ) ;
#26734=CARTESIAN_POINT ( 'NONE',  ( -1.587926509186350810, 0.05413385826771626580, -0.4176697321401330321 ) ) ;
#26736=CARTESIAN_POINT ( 'NONE',  ( -0.6102362204724400829, 0.1660481256975885056, 0.3530559997133364547 ) ) ;
#26737=CARTESIAN_POINT ( 'NONE',  ( 0.006561679790026889343, -0.08942795157527998196, 0.3641732283464567121 ) ) ;
#26738=CARTESIAN_POINT ( 'NONE',  ( -0.8267716535433065062, 0.2952755905511811885, 0.000000000000000000 ) ) ;
#26739=CARTESIAN_POINT ( 'NONE',  ( 0.7086614173228353852, -0.1870078740157479769, 0.3641732283464567677 ) ) ;
#26740=CARTESIAN_POINT ( 'NONE',  ( -0.2165354330708654795, -0.4536011799217368745, -0.2665933059059886201 ) ) ;
#26741=CARTESIAN_POINT ( 'NONE',  ( -0.6561679790026240244, -0.6046776061558807314, 0.2411417322834647770 ) ) ;
#26742=CARTESIAN_POINT ( 'NONE',  ( -1.069553805774277722, 0.2952755905511811885, 0.1292274648535926551 ) ) ;
#26743=CARTESIAN_POINT ( 'NONE',  ( 2.787279214012418738, 0.000000000000000000, 0.000000000000000000 ) ) ;
#26744=CARTESIAN_POINT ( 'NONE',  ( 1.423884514435696413, -0.2845877964562161244, -0.3641732283464567121 ) ) ;
#26745=CARTESIAN_POINT ( 'NONE',  ( 0.4593175853018380828, 0.05413385826771626580, -0.4176697321401330321 ) ) ;
#26747=CARTESIAN_POINT ( 'NONE',  ( -1.679790026246718693, 0.2306618581243847221, -0.2411417322834647770 ) ) ;
#26748=ORIENTED_EDGE ( 'NONE', *, *, #48534, .F. ) ;
#26750=CARTESIAN_POINT ( 'NONE',  ( -0.8398950131233585692, 0.1283753931104748280, 0.1820866141732283561 ) ) ;
#26751=CARTESIAN_POINT ( 'NONE',  ( 0.8595800524934390507, -0.05778040916215560624, -0.4822834645669293319 ) ) ;
#26752=CARTESIAN_POINT ( 'NONE',  ( -1.207349081364828880, 0.1283753931104746893, -0.1820866141732285504 ) ) ;
#26754=CARTESIAN_POINT ( 'NONE',  ( -0.8858267716535425107, 0.1660481256975883668, -0.3530559997133364547 ) ) ;
#26755=CARTESIAN_POINT ( 'NONE',  ( 0.9711286089238851948, -0.6046776061558809534, -0.2411417322834644161 ) ) ;
#26756=CARTESIAN_POINT ( 'NONE',  ( 0.5118110236220480003, -0.6692913385826771977, 8.415575281601705876E-17 ) ) ;
#26757=CARTESIAN_POINT ( 'NONE',  ( 1.194225721784777594, -0.4281496062992127816, -0.4176697321401328100 ) ) ;
#26758=CARTESIAN_POINT ( 'NONE',  ( -1.535433070866141225, 0.1771653543307087630, 0.000000000000000000 ) ) ;
#26762=CARTESIAN_POINT ( 'NONE',  ( 1.191111281560510715, -4.927456884911482678E-16, 0.4445507791589062840 ) ) ;
#26763=CARTESIAN_POINT ( 'NONE',  ( 0.7808398950131241190, -0.08942795157528024563, -0.3641732283464568787 ) ) ;
#26764=CARTESIAN_POINT ( 'NONE',  ( 0.1771653543307093182, 0.07958543189024085140, 0.2665933059059887866 ) ) ;
#26765=CARTESIAN_POINT ( 'NONE',  ( -0.08530183727034056085, -0.05778040916215560624, -0.4822834645669293319 ) ) ;
#26766=CARTESIAN_POINT ( 'NONE',  ( 1.102362204724410155, -0.1870078740157479769, 0.4822834645669291653 ) ) ;
#26768=CARTESIAN_POINT ( 'NONE',  ( 0.3215223097112867578, -0.2845877964562161244, -0.3641732283464567121 ) ) ;
#26769=CARTESIAN_POINT ( 'NONE',  ( -0.7808398950131222316, -0.3162353388693409650, -0.4822834645669289433 ) ) ;
#26770=CARTESIAN_POINT ( 'NONE',  ( 1.410761154855643795, -0.3162353388693405765, 0.4822834645669290543 ) ) ;
#26771=CARTESIAN_POINT ( 'NONE',  ( 0.9186351706036752773, 0.2306618581243847221, -0.2411417322834647770 ) ) ;
#26775=EDGE_LOOP ( 'NONE', ( #26037, #10638, #15451, #32705 ) ) ;
#26776=CARTESIAN_POINT ( 'NONE',  ( -1.463254593175852492, -0.6692913385826773087, -0.1292274648535924053 ) ) ;
#26777=CARTESIAN_POINT ( 'NONE',  ( -0.7742782152230962556, -0.3690944881889765550, -0.3153832671262227771 ) ) ;
#26778=CARTESIAN_POINT ( 'NONE',  ( -0.6299212598425188991, -0.1870078740157480879, -0.4822834645669291653 ) ) ;
#26780=FACE_OUTER_BOUND ( 'NONE', #82780, .T. ) ;
#26781=CARTESIAN_POINT ( 'NONE',  ( 1.489501312335958172, -0.3162353388693405765, 0.4822834645669290543 ) ) ;
#26782=CARTESIAN_POINT ( 'NONE',  ( -1.187664041994750175, -0.05778040916215560624, -0.4822834645669293319 ) ) ;
#26783=CARTESIAN_POINT ( 'NONE',  ( 0.3543307086614179147, 0.2952755905511811885, 0.000000000000000000 ) ) ;
#26784=CARTESIAN_POINT ( 'NONE',  ( -1.128608923884513837, 0.2306618581243847221, -0.2411417322834647770 ) ) ;
#26786=CARTESIAN_POINT ( 'NONE',  ( 0.5118110236220478892, 0.2952755905511811885, 0.000000000000000000 ) ) ;
#26788=CARTESIAN_POINT ( 'NONE',  ( -0.8858267716535425107, -0.4536011799217367080, 0.2665933059059888421 ) ) ;
#26791=EDGE_LOOP ( 'NONE', ( #58372, #8776, #52661, #63335 ) ) ;
#26792=CARTESIAN_POINT ( 'NONE',  ( -0.6423408027444563739, -2.609869883881465018E-15, -0.3464511005275220379 ) ) ;
#26793=CARTESIAN_POINT ( 'NONE',  ( -1.259842519685038686, -0.1870078740157479769, 0.4822834645669291653 ) ) ;
#26794=CARTESIAN_POINT ( 'NONE',  ( -1.115485564304461219, 0.05413385826771626580, -0.4176697321401330321 ) ) ;
#26796=CARTESIAN_POINT ( 'NONE',  ( -1.423884514435694859, -0.3162353388693405765, 0.4822834645669290543 ) ) ;
#26797=CARTESIAN_POINT ( 'NONE',  ( -1.213910761154854745, 0.2952755905511810774, -0.1292274648535930714 ) ) ;
#26798=VECTOR ( 'NONE', #32943, 39.37007874015748143 ) ;
#26799=CARTESIAN_POINT ( 'NONE',  ( -1.325459317585300889, 0.05413385826771666132, 0.4176697321401328100 ) ) ;
#26800=CARTESIAN_POINT ( 'NONE',  ( -0.3812812444996365180, -2.294479370626195693E-15, 0.3464511005275217603 ) ) ;
#26801=CARTESIAN_POINT ( 'NONE',  ( -0.6962418744208963561, -2.294479370626195693E-15, 0.3464511005275217603 ) ) ;
#26802=CARTESIAN_POINT ( 'NONE',  ( 0.06561679790026316017, -0.3690944881889763329, 0.3153832671262228327 ) ) ;
#26803=FACE_OUTER_BOUND ( 'NONE', #28891, .T. ) ;
#26805=CARTESIAN_POINT ( 'NONE',  ( -0.1706036745406816491, -0.3690944881889763329, 0.3153832671262228327 ) ) ;
#26806=CARTESIAN_POINT ( 'NONE',  ( -0.9251968503937002541, -0.5400638737290845981, -0.3530559997133363437 ) ) ;
#26807=CARTESIAN_POINT ( 'NONE',  ( 0.8595800524934390507, -0.05778040916215560624, -0.4822834645669293319 ) ) ;
#26808=CARTESIAN_POINT ( 'NONE',  ( -0.5643044619422565855, -0.4281496062992124485, 0.4176697321401328655 ) ) ;
#26812=CARTESIAN_POINT ( 'NONE',  ( -0.7677165354330699465, -0.5400638737290845981, -0.3530559997133363437 ) ) ;
#26813=CARTESIAN_POINT ( 'NONE',  ( 1.062992125984252745, -0.6692913385826771977, 8.415575281601705876E-17 ) ) ;
#26820=CARTESIAN_POINT ( 'NONE',  ( -0.4593175853018364174, -0.4281496062992127816, -0.4176697321401328100 ) ) ;
#26821=CARTESIAN_POINT ( 'NONE',  ( -1.561679790026246017, -0.3690944881889765550, -0.3153832671262227771 ) ) ;
#26822=CARTESIAN_POINT ( 'NONE',  ( -0.8267716535433065062, -0.6692913385826771977, 8.415575281601705876E-17 ) ) ;
#26824=CARTESIAN_POINT ( 'NONE',  ( -1.318897637795274802, -0.5400638737290845981, -0.3530559997133363437 ) ) ;
#26825=DIRECTION ( 'NONE',  ( -3.096699300667737957E-16, 1.000000000000000000, -0.000000000000000000 ) ) ;
#26826=CARTESIAN_POINT ( 'NONE',  ( -0.7939632545931754048, -0.3162353388693405765, 0.4822834645669290543 ) ) ;
#26827=CARTESIAN_POINT ( 'NONE',  ( -0.2099737532808391705, -0.6046776061558809534, -0.2411417322834644161 ) ) ;
#26829=CARTESIAN_POINT ( 'NONE',  ( 0.8070866141732288002, 0.07958543189024085140, 0.2665933059059887866 ) ) ;
#26831=CARTESIAN_POINT ( 'NONE',  ( 0.2099737532808405305, -0.5023911411419708095, 0.1820866141732285504 ) ) ;
#26832=CARTESIAN_POINT ( 'NONE',  ( 1.522309711286089939, -0.5023911411419708095, -0.1820866141732282451 ) ) ;
#26833=CARTESIAN_POINT ( 'NONE',  ( 1.561679790026247350, -0.4281496062992124485, 0.4176697321401328655 ) ) ;
#26834=CARTESIAN_POINT ( 'NONE',  ( -0.01312335958005186876, -0.004921259842519870586, -0.3153832671262229437 ) ) ;
#26836=CARTESIAN_POINT ( 'NONE',  ( -1.194225721784776262, -0.4281496062992124485, 0.4176697321401328655 ) ) ;
#26837=CARTESIAN_POINT ( 'NONE',  ( 1.161417322834646271, 0.1660481256975883668, -0.3530559997133364547 ) ) ;
#26839=CARTESIAN_POINT ( 'NONE',  ( -0.3674540682414689785, 0.1283753931104748280, 0.1820866141732283561 ) ) ;
#26840=CARTESIAN_POINT ( 'NONE',  ( 0.3871391076115493490, -0.3162353388693405765, 0.4822834645669290543 ) ) ;
#26842=CARTESIAN_POINT ( 'NONE',  ( 1.062992125984252745, -0.5511811023622047445, 6.969142054262312111E-17 ) ) ;
#26843=CARTESIAN_POINT ( 'NONE',  ( 0.2493438320209980519, -0.3690944881889765550, -0.3153832671262227771 ) ) ;
#26844=CARTESIAN_POINT ( 'NONE',  ( -0.3412073490813641308, 0.2306618581243847221, -0.2411417322834647770 ) ) ;
#26846=CARTESIAN_POINT ( 'NONE',  ( -0.8989501312335946848, -0.5511811023622046335, 0.09757992244046803654 ) ) ;
#26847=FACE_OUTER_BOUND ( 'NONE', #9577, .T. ) ;
#26848=ADVANCED_FACE ( 'NONE', ( #27543 ), #9029, .F. ) ;
#26849=CARTESIAN_POINT ( 'NONE',  ( 0.5905511811023629321, 0.2952755905511811885, 0.000000000000000000 ) ) ;
#26850=CARTESIAN_POINT ( 'NONE',  ( -1.069553805774277722, -0.6692913385826773087, -0.1292274648535924053 ) ) ;
#26853=CARTESIAN_POINT ( 'NONE',  ( 0.1509186351706042484, -0.2845877964562159024, 0.3641732283464567677 ) ) ;
#26854=CARTESIAN_POINT ( 'NONE',  ( -0.8333333333333323711, 0.2952755905511811885, 0.1292274648535926551 ) ) ;
#26855=CARTESIAN_POINT ( 'NONE',  ( -1.023622047244093558, -0.1870078740157479769, 0.4822834645669291653 ) ) ;
#26856=CARTESIAN_POINT ( 'NONE',  ( -1.332020997375327642, -0.08942795157527998196, 0.3641732283464567121 ) ) ;
#26857=CARTESIAN_POINT ( 'NONE',  ( 1.679790026246720025, 0.2306618581243848609, 0.2411417322834645549 ) ) ;
#26858=CARTESIAN_POINT ( 'NONE',  ( -0.7939632545931750718, -0.08942795157528024563, -0.3641732283464568787 ) ) ;
#26859=CARTESIAN_POINT ( 'NONE',  ( -1.586052503253846169, 1.850393700787402729, 0.1653254495020583248 ) ) ;
#26860=CARTESIAN_POINT ( 'NONE',  ( 1.122047244094488860, 0.1660481256975885056, 0.3530559997133364547 ) ) ;
#26865=CARTESIAN_POINT ( 'NONE',  ( -1.581364829396324945, -0.3162353388693405765, 0.4822834645669290543 ) ) ;
#26866=CARTESIAN_POINT ( 'NONE',  ( -1.397637795275589623, 0.1660481256975885056, 0.3530559997133364547 ) ) ;
#26867=CARTESIAN_POINT ( 'NONE',  ( 1.358267716535433323, -0.5400638737290845981, -0.3530559997133363437 ) ) ;
#26871=CARTESIAN_POINT ( 'NONE',  ( 0.5577427821522316087, -0.05778040916215522460, 0.4822834645669289988 ) ) ;
#26872=CARTESIAN_POINT ( 'NONE',  ( -0.4265091863517051496, -0.6692913385826771977, 0.1292274648535927661 ) ) ;
#26874=CARTESIAN_POINT ( 'NONE',  ( 0.7974104941589355011, -4.927456884911482678E-16, 0.4445507791589062840 ) ) ;
#26875=CARTESIAN_POINT ( 'NONE',  ( 0.9645669291338588858, 0.07958543189024085140, 0.2665933059059887866 ) ) ;
#26877=ORIENTED_EDGE ( 'NONE', *, *, #22300, .T. ) ;
#26879=ORIENTED_EDGE ( 'NONE', *, *, #57231, .T. ) ;
#26880=CARTESIAN_POINT ( 'NONE',  ( 0.03280839895013198948, 0.2952755905511811885, 0.1292274648535926551 ) ) ;
#26881=CARTESIAN_POINT ( 'NONE',  ( 1.450131233595801428, 0.2952755905511811885, 0.1292274648535926551 ) ) ;
#26882=CARTESIAN_POINT ( 'NONE',  ( 0.3871391076115493490, -0.3162353388693405765, 0.4822834645669290543 ) ) ;
#26883=CARTESIAN_POINT ( 'NONE',  ( 1.240157480314961314, 0.1660481256975883668, -0.3530559997133364547 ) ) ;
#26884=CARTESIAN_POINT ( 'NONE',  ( -0.4724409448818890911, -0.1870078740157480879, -0.4822834645669291653 ) ) ;
#26885=CARTESIAN_POINT ( 'NONE',  ( -0.1115485564304456306, 0.2952755905511810774, -0.1292274648535930714 ) ) ;
#26886=CARTESIAN_POINT ( 'NONE',  ( -1.568241469816272105, -0.3162353388693409650, -0.4822834645669289433 ) ) ;
#26887=CARTESIAN_POINT ( 'NONE',  ( 1.187664041994751285, -0.3162353388693409650, -0.4822834645669289433 ) ) ;
#26888=ADVANCED_FACE ( 'NONE', ( #65862 ), #14529, .F. ) ;
#26889=CARTESIAN_POINT ( 'NONE',  ( 1.358267716535433323, 0.1660481256975885056, 0.3530559997133364547 ) ) ;
#26891=CARTESIAN_POINT ( 'NONE',  ( 0.5249343832021005074, -0.5023911411419708095, 0.1820866141732285504 ) ) ;
#26895=CARTESIAN_POINT ( 'NONE',  ( -0.5511811023622041894, -0.1870078740157480601, -0.3641732283464567677 ) ) ;
#26896=CARTESIAN_POINT ( 'NONE',  ( 0.05249343832021075018, -0.6046776061558807314, 0.2411417322834647770 ) ) ;
#26898=CARTESIAN_POINT ( 'NONE',  ( 0.1115485564304467270, -0.6692913385826773087, -0.1292274648535924053 ) ) ;
#26899=CARTESIAN_POINT ( 'NONE',  ( 0.1837270341207354329, 0.2306618581243848609, 0.2411417322834645549 ) ) ;
#26900=CARTESIAN_POINT ( 'NONE',  ( -0.8202099737532799750, 0.2952755905511810774, -0.1292274648535930714 ) ) ;
#26901=CARTESIAN_POINT ( 'NONE',  ( -0.8923884514435688198, 0.2306618581243847221, -0.2411417322834647770 ) ) ;
#26902=CARTESIAN_POINT ( 'NONE',  ( 1.430446194225722500, -0.3690944881889765550, -0.3153832671262227771 ) ) ;
#26903=CARTESIAN_POINT ( 'NONE',  ( -1.489501312335957062, -0.05778040916215522460, 0.4822834645669289988 ) ) ;
#26905=CARTESIAN_POINT ( 'NONE',  ( 0.9383202099737536495, -0.2845877964562159024, 0.3641732283464567677 ) ) ;
#26906=CARTESIAN_POINT ( 'NONE',  ( 0.3543307086614181922, -0.6692913385826771977, 8.415575281601705876E-17 ) ) ;
#26907=CARTESIAN_POINT ( 'NONE',  ( 0.6299212598425204535, -0.1870078740157480879, -0.4822834645669291653 ) ) ;
#26912=CARTESIAN_POINT ( 'NONE',  ( -0.5511811023622041894, -0.1870078740157480879, -0.4822834645669291653 ) ) ;
#26915=CARTESIAN_POINT ( 'NONE',  ( -1.253280839895012377, -0.2845877964562161244, -0.3641732283464567121 ) ) ;
#26916=CARTESIAN_POINT ( 'NONE',  ( 1.207349081364829990, -0.6046776061558809534, -0.2411417322834644161 ) ) ;
#26917=CARTESIAN_POINT ( 'NONE',  ( 1.089238845144357759, 0.05413385826771626580, -0.4176697321401330321 ) ) ;
#26918=CARTESIAN_POINT ( 'NONE',  ( -0.05905511811023545637, 0.07958543189024085140, 0.2665933059059887866 ) ) ;
#26919=CARTESIAN_POINT ( 'NONE',  ( 0.6889763779527563470, 0.1660481256975883668, -0.3530559997133364547 ) ) ;
#26921=CARTESIAN_POINT ( 'NONE',  ( -0.1509186351706028884, -0.2845877964562161244, -0.3641732283464567121 ) ) ;
#26922=CARTESIAN_POINT ( 'NONE',  ( -0.2165354330708654795, -0.5400638737290845981, -0.3530559997133363437 ) ) ;
#26924=CIRCLE ( 'NONE', #22898, 1.220472440944881942 ) ;
#26925=CARTESIAN_POINT ( 'NONE',  ( -1.220472440944881054, 0.2952755905511811885, 0.000000000000000000 ) ) ;
#26926=CARTESIAN_POINT ( 'NONE',  ( 0.6824146981627303710, 0.1283753931104746893, -0.1820866141732285504 ) ) ;
#26927=CARTESIAN_POINT ( 'NONE',  ( 0.5027385518334777093, 1.496062992125983815, -0.5309055118110237448 ) ) ;
#26928=CARTESIAN_POINT ( 'NONE',  ( -0.8398950131233589023, -0.6046776061558809534, -0.2411417322834644161 ) ) ;
#26929=CARTESIAN_POINT ( 'NONE',  ( -0.2165354330708654795, 0.07958543189024085140, 0.2665933059059887866 ) ) ;
#26930=PLANE ( 'NONE',  #56068 ) ;
#26931=CARTESIAN_POINT ( 'NONE',  ( -0.7086614173228339419, -0.1870078740157480879, -0.4822834645669291653 ) ) ;
#26932=CARTESIAN_POINT ( 'NONE',  ( -0.5052493438320203589, 0.2952755905511810774, -0.1292274648535930714 ) ) ;
#26933=CARTESIAN_POINT ( 'NONE',  ( 0.1902887139107617975, -0.6692913385826773087, -0.1292274648535924053 ) ) ;
#26936=CARTESIAN_POINT ( 'NONE',  ( -1.548556430446193399, 0.1283753931104748280, 0.1820866141732283561 ) ) ;
#26937=CARTESIAN_POINT ( 'NONE',  ( 0.6561679790026253567, -0.5023911411419708095, -0.1820866141732282451 ) ) ;
#26938=CARTESIAN_POINT ( 'NONE',  ( 1.391076115485564868, -0.6046776061558807314, 0.2411417322834647770 ) ) ;
#26939=CARTESIAN_POINT ( 'NONE',  ( -0.7086614173228339419, -0.1870078740157480601, -0.3641732283464567677 ) ) ;
#26940=CARTESIAN_POINT ( 'NONE',  ( -1.030183727034119867, -0.08942795157528024563, -0.3641732283464568787 ) ) ;
#26942=CARTESIAN_POINT ( 'NONE',  ( -0.7611548556430438595, -0.6046776061558809534, -0.2411417322834644161 ) ) ;
#26943=CARTESIAN_POINT ( 'NONE',  ( -0.1181102362204717315, 0.2952755905511811885, 0.000000000000000000 ) ) ;
#26944=CARTESIAN_POINT ( 'NONE',  ( 0.7414698162729663755, 0.1771653543307087630, 0.09757992244046791164 ) ) ;
#26946=CARTESIAN_POINT ( 'NONE',  ( 1.089238845144357537, -0.3690944881889763329, 0.3153832671262228327 ) ) ;
#26947=CARTESIAN_POINT ( 'NONE',  ( 0.2952755905511819101, 0.1660481256975883668, -0.3530559997133364547 ) ) ;
#26949=CARTESIAN_POINT ( 'NONE',  ( -0.8464566929133852113, -0.5400638737290845981, -0.3530559997133363437 ) ) ;
#26951=CARTESIAN_POINT ( 'NONE',  ( 1.332020997375328974, -0.08942795157528024563, -0.3641732283464568787 ) ) ;
#26952=CARTESIAN_POINT ( 'NONE',  ( 0.5511811023622055217, -0.1870078740157479769, 0.4822834645669291653 ) ) ;
#26953=CARTESIAN_POINT ( 'NONE',  ( 0.3149606299212606708, -0.1870078740157480879, -0.4822834645669291653 ) ) ;
#26954=CARTESIAN_POINT ( 'NONE',  ( 0.04593175853018440641, -0.5511811023622046335, 0.09757992244046803654 ) ) ;
#26956=CARTESIAN_POINT ( 'NONE',  ( -0.1246719160104980823, -0.5511811023622048555, -0.09757992244046775898 ) ) ;
#26957=CARTESIAN_POINT ( 'NONE',  ( 0.8005249343832028242, -0.4281496062992127816, -0.4176697321401328100 ) ) ;
#26958=CARTESIAN_POINT ( 'NONE',  ( -0.7808398950131225646, -0.08942795157527998196, 0.3641732283464567121 ) ) ;
#26959=CARTESIAN_POINT ( 'NONE',  ( -0.6430446194225712953, 0.05413385826771626580, -0.4176697321401330321 ) ) ;
#26961=EDGE_LOOP ( 'NONE', ( #16360, #81777, #39740, #46559 ) ) ;
#26962=CARTESIAN_POINT ( 'NONE',  ( -1.043307086614172041, -0.5400638737290844871, 0.3530559997133364547 ) ) ;
#26963=CARTESIAN_POINT ( 'NONE',  ( -1.305774278215222184, -0.5511811023622048555, -0.09757992244046775898 ) ) ;
#26964=CARTESIAN_POINT ( 'NONE',  ( -0.1049868766404193215, 0.2306618581243847221, -0.2411417322834647770 ) ) ;
#26965=CARTESIAN_POINT ( 'NONE',  ( -1.535433070866141225, 0.2952755905511811885, 0.000000000000000000 ) ) ;
#26966=CARTESIAN_POINT ( 'NONE',  ( -0.8070866141732276899, 0.1660481256975883668, -0.3530559997133364547 ) ) ;
#26968=CARTESIAN_POINT ( 'NONE',  ( 1.036745406824147731, 0.05413385826771666132, 0.4176697321401328100 ) ) ;
#26969=CARTESIAN_POINT ( 'NONE',  ( 1.115485564304462551, 0.05413385826771666132, 0.4176697321401328100 ) ) ;
#26970=CARTESIAN_POINT ( 'NONE',  ( 1.286089238845145033, -0.6046776061558809534, -0.2411417322834644161 ) ) ;
#26973=CARTESIAN_POINT ( 'NONE',  ( -1.292650918635170010, -0.6692913385826771977, 0.1292274648535927661 ) ) ;
#26976=ORIENTED_EDGE ( 'NONE', *, *, #22300, .F. ) ;
#26977=CARTESIAN_POINT ( 'NONE',  ( -0.2755905511811015396, -0.5511811023622047445, 6.969142054262312111E-17 ) ) ;
#26980=CARTESIAN_POINT ( 'NONE',  ( 0.3215223097112867578, -0.05778040916215522460, 0.4822834645669289988 ) ) ;
#26981=CARTESIAN_POINT ( 'NONE',  ( 0.1509186351706042484, -0.3162353388693405765, 0.4822834645669290543 ) ) ;
#26982=CARTESIAN_POINT ( 'NONE',  ( -0.6692913385826764205, 0.2952755905511811885, 0.000000000000000000 ) ) ;
#26984=CARTESIAN_POINT ( 'NONE',  ( -0.9711286089238838626, 0.1283753931104746893, -0.1820866141732285504 ) ) ;
#26985=CARTESIAN_POINT ( 'NONE',  ( 0.3477690288713918276, 0.2952755905511811885, 0.1292274648535926551 ) ) ;
#26986=CARTESIAN_POINT ( 'NONE',  ( 0.7086614173228353852, -0.1870078740157479769, 0.4822834645669291653 ) ) ;
#26987=CARTESIAN_POINT ( 'NONE',  ( 0.4461942257217855201, -0.5023911411419708095, 0.1820866141732285504 ) ) ;
#26988=CIRCLE ( 'NONE', #67326, 2.362204724409449064 ) ;
#26989=CARTESIAN_POINT ( 'NONE',  ( -0.2493438320209966919, -0.4281496062992124485, 0.4176697321401328655 ) ) ;
#26991=CARTESIAN_POINT ( 'NONE',  ( -0.7677165354330699465, -0.5400638737290845981, -0.3530559997133363437 ) ) ;
#26993=CARTESIAN_POINT ( 'NONE',  ( 1.240157480314961314, 0.1660481256975883668, -0.3530559997133364547 ) ) ;
#26994=CARTESIAN_POINT ( 'NONE',  ( 1.686351706036745890, 0.1771653543307087630, 0.09757992244046791164 ) ) ;
#26995=ORIENTED_EDGE ( 'NONE', *, *, #65114, .T. ) ;
#26997=CARTESIAN_POINT ( 'NONE',  ( -0.02624671916010428221, 0.2306618581243847221, -0.2411417322834647770 ) ) ;
#26999=CARTESIAN_POINT ( 'NONE',  ( -1.325459317585300889, -0.4281496062992127816, -0.4176697321401328100 ) ) ;
#27000=CARTESIAN_POINT ( 'NONE',  ( 1.292650918635171564, 0.2952755905511811885, 0.1292274648535926551 ) ) ;
#27001=CARTESIAN_POINT ( 'NONE',  ( 1.318897637795276356, 0.1660481256975883668, -0.3530559997133364547 ) ) ;
#27003=CARTESIAN_POINT ( 'NONE',  ( 0.3871391076115492380, -0.05778040916215560624, -0.4822834645669293319 ) ) ;
#27004=CARTESIAN_POINT ( 'NONE',  ( -0.2362204724409440182, -0.1870078740157479769, 0.4822834645669291653 ) ) ;
#27006=CARTESIAN_POINT ( 'NONE',  ( -1.246719160104986512, 0.05413385826771666132, 0.4176697321401328100 ) ) ;
#27007=CARTESIAN_POINT ( 'NONE',  ( -0.7217847769028863381, -0.4281496062992124485, 0.4176697321401328655 ) ) ;
#27009=CARTESIAN_POINT ( 'NONE',  ( 0.05905511811023709395, -0.4536011799217367080, 0.2665933059059888421 ) ) ;
#27011=CARTESIAN_POINT ( 'NONE',  ( -0.6299212598425188991, -0.1870078740157479769, 0.4822834645669291653 ) ) ;
#27012=CARTESIAN_POINT ( 'NONE',  ( -1.220472440944881054, 0.2952755905511811885, 0.000000000000000000 ) ) ;
#27013=CARTESIAN_POINT ( 'NONE',  ( 0.7086614173228352742, -0.1870078740157480879, -0.4822834645669291653 ) ) ;
#27016=CARTESIAN_POINT ( 'NONE',  ( -0.1312335958005241554, -0.6046776061558809534, -0.2411417322834644161 ) ) ;
#27017=CARTESIAN_POINT ( 'NONE',  ( -0.3149606299212590610, -0.1870078740157479769, 0.3641732283464567677 ) ) ;
#27018=CARTESIAN_POINT ( 'NONE',  ( 1.187664041994751285, -0.08942795157527998196, 0.3641732283464567121 ) ) ;
#27019=DIRECTION ( 'NONE',  ( -1.000000000000000000, 0.000000000000000000, 0.000000000000000000 ) ) ;
#27021=CARTESIAN_POINT ( 'NONE',  ( 1.581364829396326277, -0.2845877964562161244, -0.3641732283464567121 ) ) ;
#27022=CARTESIAN_POINT ( 'NONE',  ( 1.272965879265092637, 0.05413385826771666132, 0.4176697321401328100 ) ) ;
#27024=CARTESIAN_POINT ( 'NONE',  ( 0.1574803149606306130, -0.1870078740157479769, 0.4822834645669291653 ) ) ;
#27025=CARTESIAN_POINT ( 'NONE',  ( -1.496062992125983815, -0.1870078740157479769, 0.4822834645669291653 ) ) ;
#27026=CARTESIAN_POINT ( 'NONE',  ( -1.476377952755905110, -0.5400638737290845981, -0.3530559997133363437 ) ) ;
#27027=CARTESIAN_POINT ( 'NONE',  ( -0.02624671916010428221, -0.6046776061558807314, 0.2411417322834647770 ) ) ;
#27029=CARTESIAN_POINT ( 'NONE',  ( 1.594488188976378673, -0.5400638737290845981, -0.3530559997133363437 ) ) ;
#27030=CARTESIAN_POINT ( 'NONE',  ( 0.5118110236220478892, 0.2952755905511811885, 0.000000000000000000 ) ) ;
#27031=CARTESIAN_POINT ( 'NONE',  ( 1.115485564304462551, -0.3690944881889765550, -0.3153832671262227771 ) ) ;
#27033=CARTESIAN_POINT ( 'NONE',  ( 0.2034120734908144990, -0.5511811023622046335, 0.09757992244046803654 ) ) ;
#27034=CARTESIAN_POINT ( 'NONE',  ( -1.154855643044618851, 0.2306618581243848609, 0.2411417322834645549 ) ) ;
#27035=EDGE_CURVE ( 'NONE', #11962, #11380, #50135, .T. ) ;
#27037=CARTESIAN_POINT ( 'NONE',  ( 1.318897637795276356, -0.5400638737290844871, 0.3530559997133364547 ) ) ;
#27039=CARTESIAN_POINT ( 'NONE',  ( 0.9383202099737538715, -0.05778040916215560624, -0.4822834645669293319 ) ) ;
#27040=CARTESIAN_POINT ( 'NONE',  ( 0.8777275986338668456, 0.02791078216816225699, 0.4328096321851905293 ) ) ;
#27042=CARTESIAN_POINT ( 'NONE',  ( 0.4724409448818904789, -0.1870078740157479769, 0.3641732283464567677 ) ) ;
#27043=EDGE_CURVE ( 'NONE', #43326, #29291, #78692, .T. ) ;
#27044=CARTESIAN_POINT ( 'NONE',  ( 0.5183727034120741983, -0.6692913385826771977, 0.1292274648535927661 ) ) ;
#27045=CARTESIAN_POINT ( 'NONE',  ( 0.7545931758530189937, 0.2066929133858267098, -0.1054918080437494132 ) ) ;
#27046=CARTESIAN_POINT ( 'NONE',  ( -0.8070866141732276899, -0.4536011799217367080, 0.2665933059059888421 ) ) ;
#27047=CARTESIAN_POINT ( 'NONE',  ( -1.128608923884513837, -0.6046776061558807314, 0.2411417322834647770 ) ) ;
#27048=CARTESIAN_POINT ( 'NONE',  ( -1.555118110236219930, 0.1660481256975885056, 0.3530559997133364547 ) ) ;
#27050=CARTESIAN_POINT ( 'NONE',  ( 0.8136482939632553313, -0.6046776061558809534, -0.2411417322834644161 ) ) ;
#27051=CARTESIAN_POINT ( 'NONE',  ( -1.587926509186350810, -0.004921259842519870586, -0.3153832671262229437 ) ) ;
#27054=CARTESIAN_POINT ( 'NONE',  ( 0.5839895013123367340, -0.6692913385826773087, -0.1292274648535924053 ) ) ;
#27057=CARTESIAN_POINT ( 'NONE',  ( 1.587926509186352586, -0.4281496062992127816, -0.4176697321401328100 ) ) ;
#27058=CARTESIAN_POINT ( 'NONE',  ( -1.496062992125983815, -0.1870078740157480601, -0.3641732283464567677 ) ) ;
#27059=CARTESIAN_POINT ( 'NONE',  ( 1.141732283464567788, -0.5511811023622047445, 6.969142054262312111E-17 ) ) ;
#27060=CARTESIAN_POINT ( 'NONE',  ( -1.253280839895012377, -0.2845877964562161244, -0.3641732283464567121 ) ) ;
#27061=CARTESIAN_POINT ( 'NONE',  ( -0.6299212598425188991, -0.1870078740157480601, -0.3641732283464567677 ) ) ;
#27063=CARTESIAN_POINT ( 'NONE',  ( 0.9776902887139113929, 0.1771653543307087630, 0.09757992244046791164 ) ) ;
#27064=CARTESIAN_POINT ( 'NONE',  ( 0.7480314960629927956, 0.2952755905511811885, 0.000000000000000000 ) ) ;
#27065=CARTESIAN_POINT ( 'NONE',  ( 1.108923884514436242, -0.05778040916215522460, 0.4822834645669289988 ) ) ;
#27066=CARTESIAN_POINT ( 'NONE',  ( 0.09186351706036827158, 0.05413385826771666132, 0.4176697321401328100 ) ) ;
#27068=CARTESIAN_POINT ( 'NONE',  ( 0.6233595800524939223, -0.2845877964562159024, 0.3641732283464567677 ) ) ;
#27069=CARTESIAN_POINT ( 'NONE',  ( 1.174540682414699111, -0.05778040916215560624, -0.4822834645669293319 ) ) ;
#27071=CARTESIAN_POINT ( 'NONE',  ( -0.3674540682414692561, -0.6046776061558809534, -0.2411417322834644161 ) ) ;
#27074=CARTESIAN_POINT ( 'NONE',  ( 0.09186351706036799403, -0.4281496062992127816, -0.4176697321401328100 ) ) ;
#27075=CARTESIAN_POINT ( 'NONE',  ( -0.6430446194225712953, 0.05413385826771626580, -0.4176697321401330321 ) ) ;
#27076=CARTESIAN_POINT ( 'NONE',  ( -0.2362204724409442680, -0.1870078740157480879, -0.4822834645669291653 ) ) ;
#27081=CARTESIAN_POINT ( 'NONE',  ( -1.095800524934382292, -0.08942795157527998196, 0.3641732283464567121 ) ) ;
#27083=CARTESIAN_POINT ( 'NONE',  ( -1.640419947506561060, -0.4281496062992127816, -0.4176697321401328100 ) ) ;
#27085=CARTESIAN_POINT ( 'NONE',  ( 0.3740157480314966754, -0.5400638737290844871, 0.3530559997133364547 ) ) ;
#27086=CARTESIAN_POINT ( 'NONE',  ( -0.6496062992125976043, -0.4536011799217367080, 0.2665933059059888421 ) ) ;
#27087=CARTESIAN_POINT ( 'NONE',  ( 1.279527559055118724, 0.1660481256975885056, 0.3530559997133364547 ) ) ;
#27088=CARTESIAN_POINT ( 'NONE',  ( 0.3346456692913390985, 0.1660481256975885056, 0.3530559997133364547 ) ) ;
#27092=CARTESIAN_POINT ( 'NONE',  ( 1.181102362204725198, -0.1870078740157479769, 0.4822834645669291653 ) ) ;
#27093=CARTESIAN_POINT ( 'NONE',  ( 0.4986876640419954376, 0.2306618581243848609, 0.2411417322834645549 ) ) ;
#27095=CARTESIAN_POINT ( 'NONE',  ( 0.2690288713910767848, -0.6692913385826773087, -0.1292274648535924053 ) ) ;
#27096=CARTESIAN_POINT ( 'NONE',  ( 1.404199475065617264, -0.4281496062992124485, 0.4176697321401328655 ) ) ;
#27097=CARTESIAN_POINT ( 'NONE',  ( 0.8792650918635177559, 0.05413385826771666132, 0.4176697321401328100 ) ) ;
#27099=CARTESIAN_POINT ( 'NONE',  ( -0.01312335958005186876, -0.4281496062992124485, 0.4176697321401328655 ) ) ;
#27100=CARTESIAN_POINT ( 'NONE',  ( 1.069553805774278832, 0.2952755905511810774, -0.1292274648535930714 ) ) ;
#27101=CARTESIAN_POINT ( 'NONE',  ( 0.3149606299212606708, -0.1870078740157480879, -0.4822834645669291653 ) ) ;
#27102=CARTESIAN_POINT ( 'NONE',  ( 0.9908136482939640111, -0.5511811023622046335, 0.09757992244046803654 ) ) ;
#27103=CARTESIAN_POINT ( 'NONE',  ( -1.345144356955379816, -0.05778040916215560624, -0.4822834645669293319 ) ) ;
#27104=CARTESIAN_POINT ( 'NONE',  ( -1.286089238845143479, -0.6046776061558807314, 0.2411417322834647770 ) ) ;
#27105=CARTESIAN_POINT ( 'NONE',  ( 0.5708661417322841158, -0.5400638737290845981, -0.3530559997133363437 ) ) ;
#27110=ORIENTED_EDGE ( 'NONE', *, *, #60977, .F. ) ;
#27111=CARTESIAN_POINT ( 'NONE',  ( 1.135170603674541256, -0.6692913385826773087, -0.1292274648535924053 ) ) ;
#27112=CARTESIAN_POINT ( 'NONE',  ( 0.7742782152230978099, -0.3690944881889763329, 0.3153832671262228327 ) ) ;
#27117=CARTESIAN_POINT ( 'NONE',  ( 1.443569553805774897, 0.2306618581243848609, 0.2411417322834645549 ) ) ;
#27119=CARTESIAN_POINT ( 'NONE',  ( -0.1115485564304456306, 0.2952755905511810774, -0.1292274648535930714 ) ) ;
#27120=CARTESIAN_POINT ( 'NONE',  ( 0.9711286089238851948, 0.2306618581243848609, 0.2411417322834645549 ) ) ;
#27122=CARTESIAN_POINT ( 'NONE',  ( -1.660104986876639543, -0.05778040916215560624, -0.4822834645669293319 ) ) ;
#27123=CARTESIAN_POINT ( 'NONE',  ( -0.7193605937323468424, -5.642773921931522838E-15, -0.4118484887281985696 ) ) ;
#27125=CARTESIAN_POINT ( 'NONE',  ( 1.528871391076116026, 0.1771653543307087630, 0.09757992244046791164 ) ) ;
#27126=CARTESIAN_POINT ( 'NONE',  ( -0.3042614371611541690, -2.551093532135090261E-15, 0.4118477457933002461 ) ) ;
#27127=CARTESIAN_POINT ( 'NONE',  ( -0.9448818897637790704, -0.1870078740157480601, -0.3641732283464567677 ) ) ;
#27128=CARTESIAN_POINT ( 'NONE',  ( 0.8792650918635177559, 0.009842519685039467087, 0.3409548833797002021 ) ) ;
#27129=CARTESIAN_POINT ( 'NONE',  ( 0.7939632545931766261, -0.3162353388693409650, -0.4822834645669289433 ) ) ;
#27133=CARTESIAN_POINT ( 'NONE',  ( 0.9908136482939640111, -0.6692913385826771977, 0.1292274648535927661 ) ) ;
#27134=CARTESIAN_POINT ( 'NONE',  ( -1.476377952755905110, -0.5400638737290845981, -0.3530559997133363437 ) ) ;
#27136=CARTESIAN_POINT ( 'NONE',  ( -0.6299212598425188991, -0.1870078740157479769, 0.3641732283464567677 ) ) ;
#27137=CARTESIAN_POINT ( 'NONE',  ( -1.607611548556429737, 0.1771653543307087075, -0.09757992244046823083 ) ) ;
#27139=CARTESIAN_POINT ( 'NONE',  ( 0.4855643044619428750, 0.05413385826771666132, 0.4176697321401328100 ) ) ;
#27140=CARTESIAN_POINT ( 'NONE',  ( -1.108923884514435132, -0.08942795157528024563, -0.3641732283464568787 ) ) ;
#27141=CARTESIAN_POINT ( 'NONE',  ( 0.07217847769028949700, -0.08942795157528024563, -0.3641732283464568787 ) ) ;
#27142=CARTESIAN_POINT ( 'NONE',  ( -0.1246719160104980823, 0.2952755905511811885, 0.1292274648535926551 ) ) ;
#27143=CARTESIAN_POINT ( 'NONE',  ( -0.9580052493438311334, -0.004921259842519870586, -0.3153832671262229437 ) ) ;
#27145=CARTESIAN_POINT ( 'NONE',  ( 0.8727034120734912248, -0.3162353388693409650, -0.4822834645669289433 ) ) ;
#27148=CARTESIAN_POINT ( 'NONE',  ( -0.9186351706036736120, 0.2306618581243848609, 0.2411417322834645549 ) ) ;
#27149=CARTESIAN_POINT ( 'NONE',  ( -0.2821522309711278487, 0.1771653543307087630, 0.09757992244046791164 ) ) ;
#27150=CARTESIAN_POINT ( 'NONE',  ( -1.338582677165353729, -0.1870078740157479769, 0.4822834645669291653 ) ) ;
#27151=CARTESIAN_POINT ( 'NONE',  ( 0.8333333333333340365, -0.5511811023622046335, 0.09757992244046803654 ) ) ;
#27152=CARTESIAN_POINT ( 'NONE',  ( -0.9186351706036736120, 0.1283753931104748280, 0.1820866141732283561 ) ) ;
#27153=CARTESIAN_POINT ( 'NONE',  ( -1.194225721784776262, 0.05413385826771626580, -0.4176697321401330321 ) ) ;
#27154=CARTESIAN_POINT ( 'NONE',  ( -1.030183727034119867, -0.05778040916215560624, -0.4822834645669293319 ) ) ;
#27155=CARTESIAN_POINT ( 'NONE',  ( 1.660104986876641320, -0.05778040916215522460, 0.4822834645669289988 ) ) ;
#27157=CARTESIAN_POINT ( 'NONE',  ( 0.8267716535433078384, -0.5511811023622047445, 6.969142054262312111E-17 ) ) ;
#27159=CARTESIAN_POINT ( 'NONE',  ( 0.4527559055118117182, 0.1660481256975883668, -0.3530559997133364547 ) ) ;
#27160=CARTESIAN_POINT ( 'NONE',  ( -1.522309711286088607, -0.6046776061558807314, 0.2411417322834647770 ) ) ;
#27161=CARTESIAN_POINT ( 'NONE',  ( -1.620734908136482577, -0.6692913385826773087, -0.1292274648535924053 ) ) ;
#27162=VECTOR ( 'NONE', #82159, 39.37007874015748143 ) ;
#27165=CARTESIAN_POINT ( 'NONE',  ( -1.430446194225720724, -0.004921259842519870586, -0.3153832671262229437 ) ) ;
#27166=CARTESIAN_POINT ( 'NONE',  ( -0.4593175853018364174, -0.4281496062992127816, -0.4176697321401328100 ) ) ;
#27167=CARTESIAN_POINT ( 'NONE',  ( 0.6758530183727039509, 0.2952755905511810774, -0.1292274648535930714 ) ) ;
#27168=CARTESIAN_POINT ( 'NONE',  ( -1.476377952755905110, -0.4536011799217368745, -0.2665933059059886201 ) ) ;
#27170=CARTESIAN_POINT ( 'NONE',  ( -1.384514435695537005, 0.2952755905511811885, 0.1292274648535926551 ) ) ;
#27171=CARTESIAN_POINT ( 'NONE',  ( 0.9317585301837276734, 0.05413385826771626580, -0.4176697321401330321 ) ) ;
#27172=CARTESIAN_POINT ( 'NONE',  ( 0.4396325459317593221, 0.2952755905511810774, -0.1292274648535930714 ) ) ;
#27173=CARTESIAN_POINT ( 'NONE',  ( 1.377952755905512472, -0.6692913385826771977, 8.415575281601705876E-17 ) ) ;
#27174=FACE_OUTER_BOUND ( 'NONE', #48335, .T. ) ;
#27177=CYLINDRICAL_SURFACE ( 'NONE', #58716, 3.543307086614173151 ) ;
#27178=CARTESIAN_POINT ( 'NONE',  ( 0.4461942257217855201, -0.5023911411419708095, 0.1820866141732285504 ) ) ;
#27179=CARTESIAN_POINT ( 'NONE',  ( 0.07217847769028949700, -0.05778040916215560624, -0.4822834645669293319 ) ) ;
#27180=CARTESIAN_POINT ( 'NONE',  ( 1.200787401574803681, -0.5400638737290845981, -0.3530559997133363437 ) ) ;
#27182=CARTESIAN_POINT ( 'NONE',  ( 0.5052493438320218022, -0.5511811023622048555, -0.09757992244046775898 ) ) ;
#27183=CARTESIAN_POINT ( 'NONE',  ( -0.6758530183727028406, 0.2952755905511811885, 0.1292274648535926551 ) ) ;
#27184=CARTESIAN_POINT ( 'NONE',  ( 1.535433070866142335, -0.6692913385826771977, 8.415575281601705876E-17 ) ) ;
#27185=CARTESIAN_POINT ( 'NONE',  ( 0.5446194225721792126, -0.3162353388693405765, 0.4822834645669290543 ) ) ;
#27188=ORIENTED_EDGE ( 'NONE', *, *, #2315, .T. ) ;
#27191=CARTESIAN_POINT ( 'NONE',  ( -1.528871391076114250, 0.2952755905511810774, -0.1292274648535930714 ) ) ;
#27192=CARTESIAN_POINT ( 'NONE',  ( -1.345144356955379816, -0.2845877964562159024, 0.3641732283464567677 ) ) ;
#27193=CARTESIAN_POINT ( 'NONE',  ( -1.036745406824146176, -0.4281496062992124485, 0.4176697321401328655 ) ) ;
#27196=CARTESIAN_POINT ( 'NONE',  ( -1.633858267716534529, 0.07958543189024085140, 0.2665933059059887866 ) ) ;
#27197=CARTESIAN_POINT ( 'NONE',  ( -1.259842519685038686, -0.1870078740157479769, 0.4822834645669291653 ) ) ;
#27198=CARTESIAN_POINT ( 'NONE',  ( 0.2493438320209980519, -0.4281496062992127816, -0.4176697321401328100 ) ) ;
#27199=CARTESIAN_POINT ( 'NONE',  ( -1.174540682414697335, -0.05778040916215522460, 0.4822834645669289988 ) ) ;
#27202=CARTESIAN_POINT ( 'NONE',  ( 0.7874015748031503170, -0.1870078740157479769, 0.4822834645669291653 ) ) ;
#27204=CARTESIAN_POINT ( 'NONE',  ( -1.141732283464566011, 0.1771653543307087630, 0.000000000000000000 ) ) ;
#27205=ORIENTED_EDGE ( 'NONE', *, *, #31652, .F. ) ;
#27208=DIRECTION ( 'NONE',  ( -3.096699300667737957E-16, 1.000000000000000000, -0.000000000000000000 ) ) ;
#27209=CARTESIAN_POINT ( 'NONE',  ( -1.135170603674539924, -0.6692913385826771977, 0.1292274648535927661 ) ) ;
#27210=CARTESIAN_POINT ( 'NONE',  ( -1.135170603674539924, 0.2952755905511810774, -0.1292274648535930714 ) ) ;
#27212=CARTESIAN_POINT ( 'NONE',  ( -1.351706036745406347, 0.05413385826771626580, -0.4176697321401330321 ) ) ;
#27213=CARTESIAN_POINT ( 'NONE',  ( -1.469816272965878357, -0.6046776061558809534, -0.2411417322834644161 ) ) ;
#27214=CARTESIAN_POINT ( 'NONE',  ( -1.279527559055116948, 0.1660481256975883668, -0.3530559997133364547 ) ) ;
#27216=CARTESIAN_POINT ( 'NONE',  ( -0.8202099737532798640, 0.2952755905511810219, -0.1292274648535930437 ) ) ;
#27218=CARTESIAN_POINT ( 'NONE',  ( -0.05249343832020911260, 0.1283753931104748280, 0.1820866141732283561 ) ) ;
#27221=CARTESIAN_POINT ( 'NONE',  ( -0.6102362204724400829, 0.07958543189024085140, 0.2665933059059887866 ) ) ;
#27222=CARTESIAN_POINT ( 'NONE',  ( -0.7808398950131222316, -0.3162353388693409650, -0.4822834645669289433 ) ) ;
#27223=CARTESIAN_POINT ( 'NONE',  ( 0.8070866141732288002, 0.1660481256975885056, 0.3530559997133364547 ) ) ;
#27224=CARTESIAN_POINT ( 'NONE',  ( -1.036745406824146176, -0.4281496062992124485, 0.4176697321401328655 ) ) ;
#27226=VERTEX_POINT ( 'NONE', #10469 ) ;
#27227=CARTESIAN_POINT ( 'NONE',  ( -1.076115485564303809, -0.6046776061558809534, -0.2411417322834644161 ) ) ;
#27229=CARTESIAN_POINT ( 'NONE',  ( 0.8858267716535438430, -0.5400638737290845981, -0.3530559997133363437 ) ) ;
#27230=CARTESIAN_POINT ( 'NONE',  ( -1.548556430446193399, 0.1283753931104748280, 0.1820866141732283561 ) ) ;
#27236=CARTESIAN_POINT ( 'NONE',  ( -0.3937007874015740483, -0.1870078740157479769, 0.4822834645669291653 ) ) ;
#27237=CARTESIAN_POINT ( 'NONE',  ( -1.371391076115484609, -0.5511811023622046335, 0.09757992244046803654 ) ) ;
#27239=CARTESIAN_POINT ( 'NONE',  ( -1.496062992125983815, -0.1870078740157480879, -0.4822834645669291653 ) ) ;
#27241=CARTESIAN_POINT ( 'NONE',  ( -1.574803149606298636, -0.1870078740157479769, 0.4822834645669291653 ) ) ;
#27242=CARTESIAN_POINT ( 'NONE',  ( -0.2559055118110230564, 0.1660481256975883668, -0.3530559997133364547 ) ) ;
#27244=CARTESIAN_POINT ( 'NONE',  ( 0.3346456692913390985, 0.07958543189024085140, 0.2665933059059887866 ) ) ;
#27246=CARTESIAN_POINT ( 'NONE',  ( 0.4790026246719168435, -0.2845877964562161244, -0.3641732283464567121 ) ) ;
#27247=CARTESIAN_POINT ( 'NONE',  ( 1.555118110236221041, -0.4536011799217367080, 0.2665933059059888421 ) ) ;
#27248=CARTESIAN_POINT ( 'NONE',  ( 1.017060367454068581, -0.05778040916215560624, -0.4822834645669293319 ) ) ;
#27249=CARTESIAN_POINT ( 'NONE',  ( 0.09186351706036827158, -0.004921259842519576551, 0.3153832671262227771 ) ) ;
#27251=CARTESIAN_POINT ( 'NONE',  ( -1.154855643044618851, 0.2306618581243848609, 0.2411417322834645549 ) ) ;
#27252=CARTESIAN_POINT ( 'NONE',  ( 0.01312335958005323398, -0.004921259842519576551, 0.3153832671262227771 ) ) ;
#27254=CARTESIAN_POINT ( 'NONE',  ( -0.3018372703412066094, -0.3690944881889765550, -0.3153832671262227771 ) ) ;
#27255=CARTESIAN_POINT ( 'NONE',  ( 2.795275590551181910, 1.488513638086842006, 0.000000000000000000 ) ) ;
#27256=CARTESIAN_POINT ( 'NONE',  ( -0.01968503937007793844, 0.1660481256975883668, -0.3530559997133364547 ) ) ;
#27258=CARTESIAN_POINT ( 'NONE',  ( 1.076115485564305141, -0.5023911411419708095, 0.1820866141732285504 ) ) ;
#27259=CARTESIAN_POINT ( 'NONE',  ( -0.3149606299212590610, -0.1870078740157479769, 0.3641732283464567677 ) ) ;
#27260=CARTESIAN_POINT ( 'NONE',  ( -0.1049868766404193215, -0.6046776061558807314, 0.2411417322834647770 ) ) ;
#27262=CARTESIAN_POINT ( 'NONE',  ( -0.9383202099737524282, -0.2845877964562161244, -0.3641732283464567121 ) ) ;
#27264=CARTESIAN_POINT ( 'NONE',  ( 0.6233595800524942554, -0.05778040916215560624, -0.4822834645669293319 ) ) ;
#27265=CARTESIAN_POINT ( 'NONE',  ( -0.8267716535433065062, 0.2952755905511811885, 0.000000000000000000 ) ) ;
#27268=CARTESIAN_POINT ( 'NONE',  ( 0.1902887139107617975, 0.1771653543307087630, 0.09757992244046791164 ) ) ;
#27269=CARTESIAN_POINT ( 'NONE',  ( -0.7152230971128602510, -0.3162353388693405765, 0.4822834645669290543 ) ) ;
#27270=CARTESIAN_POINT ( 'NONE',  ( -1.082677165354329896, -0.5400638737290845981, -0.3530559997133363437 ) ) ;
#27271=CARTESIAN_POINT ( 'NONE',  ( -1.207349081364828436, -0.5023911411419708095, 0.1820866141732285504 ) ) ;
#27273=CARTESIAN_POINT ( 'NONE',  ( -1.003937007874014853, 0.07958543189024085140, 0.2665933059059887866 ) ) ;
#27274=CARTESIAN_POINT ( 'NONE',  ( -0.7214341416610897673, 0.004960608223778500969, -0.3437734562760191848 ) ) ;
#27275=CARTESIAN_POINT ( 'NONE',  ( 0.9711286089238851948, 0.2306618581243848609, 0.2411417322834645549 ) ) ;
#27279=CARTESIAN_POINT ( 'NONE',  ( -0.8561328129276786214, -2.191421614605370878E-15, 0.4445507791589071167 ) ) ;
#27280=CARTESIAN_POINT ( 'NONE',  ( 1.587926509186352142, -0.004921259842519576551, 0.3153832671262227771 ) ) ;
#27281=CARTESIAN_POINT ( 'NONE',  ( -1.443569553805773564, -0.6046776061558807314, 0.2411417322834647770 ) ) ;
#27282=CARTESIAN_POINT ( 'NONE',  ( 1.423884514435696191, -0.05778040916215522460, 0.4822834645669289988 ) ) ;
#27284=CARTESIAN_POINT ( 'NONE',  ( 1.686351706036745890, 0.1771653543307087630, 0.09757992244046791164 ) ) ;
#27286=( BOUNDED_SURFACE ( )  B_SPLINE_SURFACE ( 1, 2, ( 
 ( #50927, #6330, #58507, #71564, #7597, #2110, #20638, #870, #26528, #64828, #59755, #79147, #51760, #53439, #52182, #32416, #38732, #39144, #27775, #32838, #8424, #34092, #77885, #20217, #58930, #1289, #6744, #21464, #21052, #47122, #7167, #13914, #33678, #46712, #26938, #65687, #8014, #14753, #45866, #40407, #13079, #65261, #1697, #64409, #52600, #39999, #77462, #58078, #46290, #27355, #45449, #19800, #39571, #444, #13488, #26099, #33271, #78306, #71986, #78728, #14339, #71146, #59340, #53014, #72404, #66089, #80393, #79560, #41645, #34930, #16408, #79979, #73229, #9669, #53847, #60178, #74062, #22292, #74478, #40818, #47953, #2531, #66502, #73656, #42054, #15580, #28189, #54681, #3765, #67750, #35338, #67336, #8837, #61002, #54263, #9258, #15998, #10084, #3350, #29016, #22705, #15161, #29429, #21873, #34513, #48363, #60592, #55087, #47539, #2942, #35748, #80796, #41238, #28606, #61415, #23113, #48779, #16825, #66926, #72811, #33526, #73078, #58348, #1548, #77732, #709, #27202, #46968, #1136, #71412, #59604, #60026, #21315, #14601, #46554, #26368, #20901, #65529, #20484, #59189, #72662, #52865, #72252, #78575, #7013, #2381, #20063, #32681, #40255, #46138, #28038, #52026, #71833, #7862, #53696, #45715, #14182, #78995, #65938, #47387, #66352, #65100, #79405, #13759, #21724, #15428, #8274, #39416, #26786, #15010, #40667, #64674, #7437, #52443, #39840, #33940, #33108, #1959, #78153, #27621, #58776, #53284, #8690, #34360, #81475, #28868, #60442, #66777, #67188, #30106, #60852, #36425, #62098, #54530, #3205, #3619, #29286, #34783, #23792, #49047, #4440, #9519, #16260, #61690, #74744, #54949, #10358, #36018, #42729, #35191, #68425, #55768, #9931, #29695, #9110, #80655, #68014, #79828, #49464, #48634, #55357, #73506, #22145, #67600, #2794, #41503, #54113, #80246, #22968, #22561, #23379, #48223, #28453, #74329, #42315, #73919, #4030, #81063, #15854, #16676, #41906, #17094, #35603, #61265, #10765, #47803, #75158, #41088, #30975, #17550, #62978, #5317, #81113, #4076, #30156, #55818, #61318, #50330, #75620, #56642, #10410, #42778, #4904, #17958, #81526, #36889, #62565, #69297, #61739, #11646, #82343, #36472, #56241, #9989, #23846, #11228, #23019, #24661, #75206, #81938, #16726, #48686, #10812, #35655, #68066, #80705, #29743, #49513, #36067, #49922, #55407, #3673, #43182, #68879, #23431, #30575, #24249, #42367, #43595, #49095, #37304, #62147, #74799, #76027, #74383, #17146, #18372, #4488, #67652, #29336, #54997, #68474, #37707, #64215, #26320, #63792, #50740, #38946, #39365, #665, #77261, #25897, #63380, #245, #44821, #83159, #12875, #51981, #6549, #51557, #38534, #69706, #65050, #82745, #12049, #19590, #25478, #7388, #5716, #51145, #70519, #33055, #31386, #76839, #58299, #32220, #26741, #45667, #44410, #58726, #57052, #1089, #52395, #45252, #76438, #6130, #77686, #20016, #78104, #25066, #31805, #19173, #57878, #44012, #70949, #57465, #13294, #12456, #18767, #70104, #38117, #64629, #6965, #32636, #71363, #13711, #15802, #14557, #46089, #15377, #34733, #33891, #7815, #20852, #52817, #41453, #79777, #2333, #67137, #66724, #9466, #33481, #27575, #47337, #59557, #47754, #20435, #41039, #22093, #40619, #54484, #46504, #65892, #21676, #59143, #8227, #27989, #1501, #71781, #35140, #73027, #9061, #60393, #46921, #72204, #3156, #1912, #14136, #28819, #8641, #2744, #53232, #60802, #40209, #78948, #34313, #39788, #65483, #27153, #28404, #66302, #54062, #73452, #78528, #21266, #72614, #14962, #59974, #53649, #79357, #36379, #80608, #62053, #80195, #35973, #56139, #22918, #38328, #18969, #41857, #55720, #24155, #29238, #36787, #4391, #81844, #70313, #30059, #81430, #43088, #23745, #48585, #81018, #50941, #10722, #67965, #67549, #74282, #9884, #44618, #12668, #64001, #10307, #35553, #49418, #61216, #62463, #16626, #42268, #76638, #75112, #3984, #23331, #29648, #61643, #55310, #6343, #32015, #49001, #3571, #22513, #54902, #17458, #48174, #4798, #73870, #16210, #74700, #30475, #17045, #68785, #11129, #42685, #68383, #57675, #13500, #33691, #58091, #14764, #78740, #19387 ),
 ( #51351, #72415, #21063, #13927, #64421, #19813, #40011, #65698, #46723, #45039, #45462, #32850, #52195, #40420, #65273, #71160, #39156, #26112, #66101, #8437, #13092, #37, #64841, #77054, #8028, #7179, #25690, #7610, #53027, #70739, #58519, #77477, #20230, #45878, #38745, #6756, #59352, #32428, #456, #883, #78320, #1711, #71576, #26951, #52614, #27366, #51773, #26542, #77899, #39584, #46304, #33283, #58944, #1302, #20651, #71998, #14352, #48377, #66517, #15175, #60605, #2123, #34527, #47134, #53860, #73669, #60192, #16422, #28201, #27789, #67348, #35352, #2543, #80406, #54698, #8849, #47968, #73244, #74076, #2954, #79572, #41657, #40832, #72825, #42068, #28619, #42473, #53451, #54277, #21888, #79159, #79993, #67763, #47552, #15593, #29029, #29443, #10099, #9681, #16011, #21476, #61014, #34942, #41252, #22307, #35763, #3365, #66939, #9271, #22718, #61431, #80811, #23126, #74492, #3780, #55102, #48794, #16839, #68176, #34107, #59768, #37816, #11757, #17658, #11335, #43289, #36575, #4590, #31499, #25179, #68986, #17254, #76547, #74906, #24359, #50847, #50434, #61844, #57158, #81640, #44119, #42882, #18066, #43700, #69811, #81219, #5826, #30261, #36171, #5422, #24766, #23949, #23535, #10918, #68577, #82858, #12160, #75726, #18875, #56751, #44524, #49204, #36994, #37412, #49617, #63492, #10517, #31084, #4185, #30684, #29848, #62254, #55925, #63084, #75311, #62674, #69404, #5015, #55511, #56345, #82451, #76136, #18477, #82046, #50029, #52929, #32330, #63903, #78642, #58418, #71479, #356, #59255, #12989, #38644, #777, #20965, #1612, #83268, #52512, #32751, #33177, #13826, #76956, #64322, #57992, #58845, #6658, #39485, #20132, #26439, #70632, #52091, #70212, #26013, #46205, #51671, #27268, #7929, #31915, #45780, #14250, #19284, #26853, #77800, #71899, #12568, #65172, #7508, #1203, #78220, #77374, #71060, #39909, #38226, #6239, #25591, #20553, #65596, #33590, #57577, #44935, #19706, #45364, #51254, #13404, #39059, #64742, #7080, #47034, #28518, #46624, #2446, #22619, #72728, #3680, #67660, #8341, #22206, #73976, #79063, #3265, #54174, #48278, #35662, #2854, #79888, #9581, #47862, #15074, #47448, #16322, #60506, #34426, #34007, #40732, #59669, #9997, #61325, #29344, #60092, #2024, #73567, #27689, #28926, #66416, #8752, #41967, #15911, #53759, #73143, #79470, #28105, #21786, #55004, #80712, #15492, #53353, #72320, #21380, #41560, #14666, #54594, #40324, #66002, #41149, #80304, #66838, #67249, #35250, #9172, #34843, #60914, #17154, #48693, #17967, #37314, #36481, #10418, #23439, #55415, #44022, #82353, #4914, #69715, #69306, #12059, #36076, #30164, #49931, #62156, #50339, #23027, #43604, #24671, #43191, #57061, #49103, #68482, #24258, #61747, #10821, #30583, #4084, #74391, #37716, #75629, #11655, #62987, #49521, #74808, #5725, #4497, #16735, #31396, #11237, #5326, #55827, #63390, #42787, #81534, #36897, #76036, #23854, #18381, #42375, #75214, #30984, #68073, #62573, #56652, #29752, #81122, #56249, #17559, #68887, #81945, #25908, #50750, #83169, #12466, #19183, #38956, #25489, #65063, #76850, #76450, #32646, #676, #51155, #45678, #20027, #57475, #13304, #38545, #39378, #51568, #44832, #6977, #6140, #38128, #7401, #77271, #7827, #18777, #19600, #63802, #44420, #45263, #33070, #70530, #31815, #77697, #78116, #58739, #58311, #64640, #70115, #26330, #256, #64225, #70959, #1101, #51992, #71374, #13724, #25076, #20449, #12885, #6559, #26752, #32231, #46102, #57889, #52407, #71795, #14148, #39802, #65495, #33494, #82754, #41870, #60816, #59570, #73883, #52830, #16223, #22524, #15390, #65904, #21280, #41467, #67152, #48186, #20867, #46935, #34326, #53663, #67564, #66738, #72627, #14975, #27589, #9896, #59156, #14570, #1514, #40634, #78542, #9481, #66316, #27168, #9076, #54496, #80208, #8655, #78961, #21689, #47352, #46518, #72219, #35156, #40222, #1926, #59989, #79792, #3168, #73041, #28417, #54077, #79370, #28832, #2347, #8240, #22108, #33906, #15818, #34747, #41052, #53247, #60407, #28003, #2758, #47768, #73467, #55734, #17469, #30071, #61230, #30893, #74294 ) ),
 .UNSPECIFIED., .F., .F., .F. ) 
 B_SPLINE_SURFACE_WITH_KNOTS ( ( 2, 2 ),
 ( 3, 2, 2, 2, 2, 2, 2, 2, 2, 2, 2, 2, 2, 2, 2, 2, 2, 2, 2, 2, 2, 2, 2, 2, 2, 2, 2, 2, 2, 2, 2, 2, 2, 2, 2, 2, 2, 2, 2, 2, 2, 2, 2, 2, 2, 2, 2, 2, 2, 2, 2, 2, 2, 2, 2, 2, 2, 2, 2, 2, 2, 2, 2, 2, 2, 2, 2, 2, 2, 2, 2, 2, 2, 2, 2, 2, 2, 2, 2, 2, 2, 2, 2, 2, 2, 2, 2, 2, 2, 2, 2, 2, 2, 2, 2, 2, 2, 2, 2, 2, 2, 2, 2, 2, 2, 2, 2, 2, 2, 2, 2, 2, 2, 2, 2, 2, 2, 2, 2, 2, 2, 2, 2, 2, 2, 2, 2, 2, 2, 2, 2, 2, 2, 2, 2, 2, 2, 2, 2, 2, 2, 2, 2, 2, 2, 2, 2, 2, 2, 2, 2, 2, 2, 2, 2, 2, 2, 2, 2, 2, 2, 2, 2, 2, 2, 2, 2, 2, 2, 2, 2, 2, 2, 2, 2, 2, 2, 2, 2, 2, 2, 2, 2, 2, 2, 2, 2, 2, 2, 2, 2, 2, 2, 2, 2, 2, 2, 2, 2, 2, 2, 2, 2, 2, 2, 2, 2, 2, 2, 2, 2, 2, 2, 2, 2, 2, 2, 2, 2, 2, 2, 2, 2, 2, 2, 2, 2, 2, 2, 2, 2, 2, 2, 2, 2, 2, 2, 2, 2, 2, 2, 2, 2, 2, 2, 2, 2, 2, 2, 2, 2, 2, 2, 2, 2, 3 ),
 ( 0.000000000000000000, 1.000000000000000000 ),
 ( 0.000000000000000000, 0.003787878787878787984, 0.007575757575757575968, 0.01136363636363636395, 0.01515151515151515194, 0.01893939393939393992, 0.02272727272727272790, 0.02651515151515151589, 0.03030303030303030387, 0.03409090909090908839, 0.03787878787878787984, 0.04166666666666666435, 0.04545454545454545581, 0.04924242424242424032, 0.05303030303030303177, 0.05681818181818181629, 0.06060606060606060774, 0.06439393939393939226, 0.06818181818181817677, 0.07196969696969697516, 0.07575757575757575968, 0.07954545454545454419, 0.08333333333333332871, 0.08712121212121212710, 0.09090909090909091161, 0.09469696969696969613, 0.09848484848484848064, 0.1022727272727272790, 0.1060606060606060635, 0.1098484848484848481, 0.1136363636363636326, 0.1174242424242424310, 0.1212121212121212155, 0.1250000000000000000, 0.1287878787878787845, 0.1325757575757575690, 0.1363636363636363535, 0.1401515151515151381, 0.1439393939393939503, 0.1477272727272727348, 0.1515151515151515194, 0.1553030303030303039, 0.1590909090909090884, 0.1628787878787878729, 0.1666666666666666574, 0.1704545454545454419, 0.1742424242424242542, 0.1780303030303030387, 0.1818181818181818232, 0.1856060606060606077, 0.1893939393939393923, 0.1931818181818181768, 0.1969696969696969613, 0.2007575757575757458, 0.2045454545454545581, 0.2083333333333333426, 0.2121212121212121271, 0.2159090909090909116, 0.2196969696969696961, 0.2234848484848484806, 0.2272727272727272652, 0.2310606060606060497, 0.2348484848484848619, 0.2386363636363636465, 0.2424242424242424310, 0.2462121212121212155, 0.2500000000000000000, 0.2537878787878787845, 0.2575757575757575690, 0.2613636363636363535, 0.2651515151515151381, 0.2689393939393939226, 0.2727272727272727071, 0.2765151515151514916, 0.2803030303030302761, 0.2840909090909091161, 0.2878787878787879007, 0.2916666666666666852, 0.2954545454545454697, 0.2992424242424242542, 0.3030303030303030387, 0.3068181818181818232, 0.3106060606060606077, 0.3143939393939393923, 0.3181818181818181768, 0.3219696969696969613, 0.3257575757575757458, 0.3295454545454545303, 0.3333333333333333148, 0.3371212121212120993, 0.3409090909090908839, 0.3446969696969697239, 0.3484848484848485084, 0.3522727272727272929, 0.3560606060606060774, 0.3598484848484848619, 0.3636363636363636465, 0.3674242424242424310, 0.3712121212121212155, 0.3750000000000000000, 0.3787878787878787845, 0.3825757575757575690, 0.3863636363636363535, 0.3901515151515151381, 0.3939393939393939226, 0.3977272727272727071, 0.4015151515151514916, 0.4053030303030302761, 0.4090909090909091161, 0.4128787878787879007, 0.4166666666666666852, 0.4204545454545454697, 0.4242424242424242542, 0.4280303030303030387, 0.4318181818181818232, 0.4356060606060606077, 0.4393939393939393923, 0.4431818181818181768, 0.4469696969696969613, 0.4507575757575757458, 0.4545454545454545303, 0.4583333333333333148, 0.4621212121212120993, 0.4659090909090908839, 0.4696969696969697239, 0.4734848484848485084, 0.4772727272727272929, 0.4810606060606060774, 0.4848484848484848619, 0.4886363636363636465, 0.4924242424242424310, 0.4962121212121212155, 0.5000000000000000000, 0.5037878787878787845, 0.5075757575757575690, 0.5113636363636363535, 0.5151515151515151381, 0.5189393939393939226, 0.5227272727272727071, 0.5265151515151514916, 0.5303030303030302761, 0.5340909090909090606, 0.5378787878787878451, 0.5416666666666666297, 0.5454545454545454142, 0.5492424242424241987, 0.5530303030303029832, 0.5568181818181817677, 0.5606060606060605522, 0.5643939393939394478, 0.5681818181818182323, 0.5719696969696970168, 0.5757575757575758013, 0.5795454545454545858, 0.5833333333333333703, 0.5871212121212121549, 0.5909090909090909394, 0.5946969696969697239, 0.5984848484848485084, 0.6022727272727272929, 0.6060606060606060774, 0.6098484848484848619, 0.6136363636363636465, 0.6174242424242424310, 0.6212121212121212155, 0.6250000000000000000, 0.6287878787878787845, 0.6325757575757575690, 0.6363636363636363535, 0.6401515151515151381, 0.6439393939393939226, 0.6477272727272727071, 0.6515151515151514916, 0.6553030303030302761, 0.6590909090909090606, 0.6628787878787878451, 0.6666666666666666297, 0.6704545454545454142, 0.6742424242424241987, 0.6780303030303029832, 0.6818181818181817677, 0.6856060606060605522, 0.6893939393939394478, 0.6931818181818182323, 0.6969696969696970168, 0.7007575757575758013, 0.7045454545454545858, 0.7083333333333333703, 0.7121212121212121549, 0.7159090909090909394, 0.7196969696969697239, 0.7234848484848485084, 0.7272727272727272929, 0.7310606060606060774, 0.7348484848484848619, 0.7386363636363636465, 0.7424242424242424310, 0.7462121212121212155, 0.7500000000000000000, 0.7537878787878787845, 0.7575757575757575690, 0.7613636363636363535, 0.7651515151515151381, 0.7689393939393939226, 0.7727272727272727071, 0.7765151515151514916, 0.7803030303030302761, 0.7840909090909090606, 0.7878787878787878451, 0.7916666666666666297, 0.7954545454545454142, 0.7992424242424241987, 0.8030303030303029832, 0.8068181818181817677, 0.8106060606060605522, 0.8143939393939394478, 0.8181818181818182323, 0.8219696969696970168, 0.8257575757575758013, 0.8295454545454545858, 0.8333333333333333703, 0.8371212121212121549, 0.8409090909090909394, 0.8446969696969697239, 0.8484848484848485084, 0.8522727272727272929, 0.8560606060606060774, 0.8598484848484848619, 0.8636363636363636465, 0.8674242424242424310, 0.8712121212121212155, 0.8750000000000000000, 0.8787878787878787845, 0.8825757575757575690, 0.8863636363636363535, 0.8901515151515151381, 0.8939393939393939226, 0.8977272727272727071, 0.9015151515151514916, 0.9053030303030302761, 0.9090909090909090606, 0.9128787878787878451, 0.9166666666666666297, 0.9204545454545454142, 0.9242424242424241987, 0.9280303030303029832, 0.9318181818181817677, 0.9356060606060605522, 0.9393939393939394478, 0.9431818181818182323, 0.9469696969696970168, 0.9507575757575758013, 0.9545454545454545858, 0.9583333333333333703, 0.9621212121212121549, 0.9659090909090909394 ),
 .UNSPECIFIED. ) 
 GEOMETRIC_REPRESENTATION_ITEM ( )  RATIONAL_B_SPLINE_SURFACE ( (
 ( 1.000000000000000000, 0.9659258262890683122, 1.000000000000000000, 0.9659258262890683122, 1.000000000000000000, 0.9659258262890683122, 1.000000000000000000, 0.9659258262890683122, 1.000000000000000000, 0.9659258262890683122, 1.000000000000000000, 0.9659258262890683122, 1.000000000000000000, 0.9659258262890683122, 1.000000000000000000, 0.9659258262890683122, 1.000000000000000000, 0.9659258262890683122, 1.000000000000000000, 0.9659258262890683122, 1.000000000000000000, 0.9659258262890683122, 1.000000000000000000, 0.9659258262890683122, 1.000000000000000000, 0.9659258262890683122, 1.000000000000000000, 0.9659258262890683122, 1.000000000000000000, 0.9659258262890683122, 1.000000000000000000, 0.9659258262890683122, 1.000000000000000000, 0.9659258262890683122, 1.000000000000000000, 0.9659258262890683122, 1.000000000000000000, 0.9659258262890683122, 1.000000000000000000, 0.9659258262890683122, 1.000000000000000000, 0.9659258262890683122, 1.000000000000000000, 0.9659258262890683122, 1.000000000000000000, 0.9659258262890683122, 1.000000000000000000, 0.9659258262890683122, 1.000000000000000000, 0.9659258262890683122, 1.000000000000000000, 0.9659258262890683122, 1.000000000000000000, 0.9659258262890683122, 1.000000000000000000, 0.9659258262890683122, 1.000000000000000000, 0.9659258262890683122, 1.000000000000000000, 0.9659258262890683122, 1.000000000000000000, 0.9659258262890683122, 1.000000000000000000, 0.9659258262890683122, 1.000000000000000000, 0.9659258262890683122, 1.000000000000000000, 0.9659258262890683122, 1.000000000000000000, 0.9659258262890683122, 1.000000000000000000, 0.9659258262890683122, 1.000000000000000000, 0.9659258262890683122, 1.000000000000000000, 0.9659258262890683122, 1.000000000000000000, 0.9659258262890683122, 1.000000000000000000, 0.9659258262890683122, 1.000000000000000000, 0.9659258262890683122, 1.000000000000000000, 0.9659258262890683122, 1.000000000000000000, 0.9659258262890683122, 1.000000000000000000, 0.9659258262890683122, 1.000000000000000000, 0.9659258262890683122, 1.000000000000000000, 0.9659258262890683122, 1.000000000000000000, 0.9659258262890683122, 1.000000000000000000, 0.9659258262890683122, 1.000000000000000000, 0.9659258262890683122, 1.000000000000000000, 0.9659258262890683122, 1.000000000000000000, 0.9659258262890683122, 1.000000000000000000, 0.9659258262890683122, 1.000000000000000000, 0.9659258262890683122, 1.000000000000000000, 0.9659258262890683122, 1.000000000000000000, 0.9659258262890683122, 1.000000000000000000, 0.9659258262890683122, 1.000000000000000000, 0.9659258262890683122, 1.000000000000000000, 0.9659258262890683122, 1.000000000000000000, 0.9659258262890683122, 1.000000000000000000, 0.9659258262890683122, 1.000000000000000000, 0.9659258262890683122, 1.000000000000000000, 0.9659258262890683122, 1.000000000000000000, 0.9659258262890683122, 1.000000000000000000, 0.9659258262890683122, 1.000000000000000000, 0.9659258262890683122, 1.000000000000000000, 0.9659258262890683122, 1.000000000000000000, 0.9659258262890683122, 1.000000000000000000, 0.9659258262890683122, 1.000000000000000000, 0.9659258262890683122, 1.000000000000000000, 0.9659258262890683122, 1.000000000000000000, 0.9659258262890683122, 1.000000000000000000, 0.9659258262890683122, 1.000000000000000000, 0.9659258262890683122, 1.000000000000000000, 0.9659258262890683122, 1.000000000000000000, 0.9659258262890683122, 1.000000000000000000, 0.9659258262890683122, 1.000000000000000000, 0.9659258262890683122, 1.000000000000000000, 0.9659258262890683122, 1.000000000000000000, 0.9659258262890683122, 1.000000000000000000, 0.9659258262890683122, 1.000000000000000000, 0.9659258262890683122, 1.000000000000000000, 0.9659258262890683122, 1.000000000000000000, 0.9659258262890683122, 1.000000000000000000, 0.9659258262890683122, 1.000000000000000000, 0.9659258262890683122, 1.000000000000000000, 0.9659258262890683122, 1.000000000000000000, 0.9659258262890683122, 1.000000000000000000, 0.9659258262890683122, 1.000000000000000000, 0.9659258262890683122, 1.000000000000000000, 0.9659258262890683122, 1.000000000000000000, 0.9659258262890683122, 1.000000000000000000, 0.9659258262890683122, 1.000000000000000000, 0.9659258262890683122, 1.000000000000000000, 0.9659258262890683122, 1.000000000000000000, 0.9659258262890683122, 1.000000000000000000, 0.9659258262890683122, 1.000000000000000000, 0.9659258262890683122, 1.000000000000000000, 0.9659258262890683122, 1.000000000000000000, 0.9659258262890683122, 1.000000000000000000, 0.9659258262890683122, 1.000000000000000000, 0.9659258262890683122, 1.000000000000000000, 0.9659258262890683122, 1.000000000000000000, 0.9659258262890683122, 1.000000000000000000, 0.9659258262890683122, 1.000000000000000000, 0.9659258262890683122, 1.000000000000000000, 0.9659258262890683122, 1.000000000000000000, 0.9659258262890683122, 1.000000000000000000, 0.9659258262890683122, 1.000000000000000000, 0.9659258262890683122, 1.000000000000000000, 0.9659258262890683122, 1.000000000000000000, 0.9659258262890683122, 1.000000000000000000, 0.9659258262890683122, 1.000000000000000000, 0.9659258262890683122, 1.000000000000000000, 0.9659258262890683122, 1.000000000000000000, 0.9659258262890683122, 1.000000000000000000, 0.9659258262890683122, 1.000000000000000000, 0.9659258262890683122, 1.000000000000000000, 0.9659258262890683122, 1.000000000000000000, 0.9659258262890683122, 1.000000000000000000, 0.9659258262890683122, 1.000000000000000000, 0.9659258262890683122, 1.000000000000000000, 0.9659258262890683122, 1.000000000000000000, 0.9659258262890683122, 1.000000000000000000, 0.9659258262890683122, 1.000000000000000000, 0.9659258262890683122, 1.000000000000000000, 0.9659258262890683122, 1.000000000000000000, 0.9659258262890683122, 1.000000000000000000, 0.9659258262890683122, 1.000000000000000000, 0.9659258262890683122, 1.000000000000000000, 0.9659258262890683122, 1.000000000000000000, 0.9659258262890683122, 1.000000000000000000, 0.9659258262890683122, 1.000000000000000000, 0.9659258262890683122, 1.000000000000000000, 0.9659258262890683122, 1.000000000000000000, 0.9659258262890683122, 1.000000000000000000, 0.9659258262890683122, 1.000000000000000000, 0.9659258262890683122, 1.000000000000000000, 0.9659258262890683122, 1.000000000000000000, 0.9659258262890683122, 1.000000000000000000, 0.9659258262890683122, 1.000000000000000000, 0.9659258262890683122, 1.000000000000000000, 0.9659258262890683122, 1.000000000000000000, 0.9659258262890683122, 1.000000000000000000, 0.9659258262890683122, 1.000000000000000000, 0.9659258262890683122, 1.000000000000000000, 0.9659258262890683122, 1.000000000000000000, 0.9659258262890683122, 1.000000000000000000, 0.9659258262890683122, 1.000000000000000000, 0.9659258262890683122, 1.000000000000000000, 0.9659258262890683122, 1.000000000000000000, 0.9659258262890683122, 1.000000000000000000, 0.9659258262890683122, 1.000000000000000000, 0.9659258262890683122, 1.000000000000000000, 0.9659258262890683122, 1.000000000000000000, 0.9659258262890683122, 1.000000000000000000, 0.9659258262890683122, 1.000000000000000000, 0.9659258262890683122, 1.000000000000000000, 0.9659258262890683122, 1.000000000000000000, 0.9659258262890683122, 1.000000000000000000, 0.9659258262890683122, 1.000000000000000000, 0.9659258262890683122, 1.000000000000000000, 0.9659258262890683122, 1.000000000000000000, 0.9659258262890683122, 1.000000000000000000, 0.9659258262890683122, 1.000000000000000000, 0.9659258262890683122, 1.000000000000000000, 0.9659258262890683122, 1.000000000000000000, 0.9659258262890683122, 1.000000000000000000, 0.9659258262890683122, 1.000000000000000000, 0.9659258262890683122, 1.000000000000000000, 0.9659258262890683122, 1.000000000000000000, 0.9659258262890683122, 1.000000000000000000, 0.9659258262890683122, 1.000000000000000000, 0.9659258262890683122, 1.000000000000000000, 0.9659258262890683122, 1.000000000000000000, 0.9659258262890683122, 1.000000000000000000, 0.9659258262890683122, 1.000000000000000000, 0.9659258262890683122, 1.000000000000000000, 0.9659258262890683122, 1.000000000000000000, 0.9659258262890683122, 1.000000000000000000, 0.9659258262890683122, 1.000000000000000000, 0.9659258262890683122, 1.000000000000000000, 0.9659258262890683122, 1.000000000000000000, 0.9659258262890683122, 1.000000000000000000, 0.9659258262890683122, 1.000000000000000000, 0.9659258262890683122, 1.000000000000000000, 0.9659258262890683122, 1.000000000000000000, 0.9659258262890683122, 1.000000000000000000, 0.9659258262890683122, 1.000000000000000000, 0.9659258262890683122, 1.000000000000000000, 0.9659258262890683122, 1.000000000000000000, 0.9659258262890683122, 1.000000000000000000, 0.9659258262890683122, 1.000000000000000000, 0.9659258262890683122, 1.000000000000000000, 0.9659258262890683122, 1.000000000000000000, 0.9659258262890683122, 1.000000000000000000, 0.9659258262890683122, 1.000000000000000000, 0.9659258262890683122, 1.000000000000000000, 0.9659258262890683122, 1.000000000000000000, 0.9659258262890683122, 1.000000000000000000, 0.9659258262890683122, 1.000000000000000000, 0.9659258262890683122, 1.000000000000000000, 0.9659258262890683122, 1.000000000000000000, 0.9659258262890683122, 1.000000000000000000, 0.9659258262890683122, 1.000000000000000000, 0.9659258262890683122, 1.000000000000000000, 0.9659258262890683122, 1.000000000000000000, 0.9659258262890683122, 1.000000000000000000, 0.9659258262890683122, 1.000000000000000000, 0.9659258262890683122, 1.000000000000000000, 0.9659258262890683122, 1.000000000000000000, 0.9659258262890683122, 1.000000000000000000, 0.9659258262890683122, 1.000000000000000000, 0.9659258262890683122, 1.000000000000000000, 0.9659258262890683122, 1.000000000000000000, 0.9659258262890683122, 1.000000000000000000, 0.9659258262890683122, 1.000000000000000000, 0.9659258262890683122, 1.000000000000000000, 0.9659258262890683122, 1.000000000000000000, 0.9659258262890683122, 1.000000000000000000, 0.9659258262890683122, 1.000000000000000000, 0.9659258262890683122, 1.000000000000000000, 0.9659258262890683122, 1.000000000000000000, 0.9659258262890683122, 1.000000000000000000, 0.9659258262890683122, 1.000000000000000000, 0.9659258262890683122, 1.000000000000000000, 0.9659258262890683122, 1.000000000000000000, 0.9659258262890683122, 1.000000000000000000, 0.9659258262890683122, 1.000000000000000000, 0.9659258262890683122, 1.000000000000000000, 0.9659258262890683122, 1.000000000000000000, 0.9659258262890683122, 1.000000000000000000, 0.9659258262890683122, 1.000000000000000000, 0.9659258262890683122, 1.000000000000000000, 0.9659258262890683122, 1.000000000000000000, 0.9659258262890683122, 1.000000000000000000, 0.9659258262890683122, 1.000000000000000000, 0.9659258262890683122, 1.000000000000000000, 0.9659258262890683122, 1.000000000000000000, 0.9659258262890683122, 1.000000000000000000, 0.9659258262890683122, 1.000000000000000000, 0.9659258262890683122, 1.000000000000000000, 0.9659258262890683122, 1.000000000000000000, 0.9659258262890683122, 1.000000000000000000, 0.9659258262890683122, 1.000000000000000000, 0.9659258262890683122, 1.000000000000000000, 0.9659258262890683122, 1.000000000000000000, 0.9659258262890683122, 1.000000000000000000, 0.9659258262890683122, 1.000000000000000000, 0.9659258262890683122, 1.000000000000000000, 0.9659258262890683122, 1.000000000000000000, 0.9659258262890683122, 1.000000000000000000, 0.9659258262890683122, 1.000000000000000000, 0.9659258262890683122, 1.000000000000000000, 0.9659258262890683122, 1.000000000000000000, 0.9659258262890683122, 1.000000000000000000),
 ( 1.000000000000000000, 0.9659258262890683122, 1.000000000000000000, 0.9659258262890683122, 1.000000000000000000, 0.9659258262890683122, 1.000000000000000000, 0.9659258262890683122, 1.000000000000000000, 0.9659258262890683122, 1.000000000000000000, 0.9659258262890683122, 1.000000000000000000, 0.9659258262890683122, 1.000000000000000000, 0.9659258262890683122, 1.000000000000000000, 0.9659258262890683122, 1.000000000000000000, 0.9659258262890683122, 1.000000000000000000, 0.9659258262890683122, 1.000000000000000000, 0.9659258262890683122, 1.000000000000000000, 0.9659258262890683122, 1.000000000000000000, 0.9659258262890683122, 1.000000000000000000, 0.9659258262890683122, 1.000000000000000000, 0.9659258262890683122, 1.000000000000000000, 0.9659258262890683122, 1.000000000000000000, 0.9659258262890683122, 1.000000000000000000, 0.9659258262890683122, 1.000000000000000000, 0.9659258262890683122, 1.000000000000000000, 0.9659258262890683122, 1.000000000000000000, 0.9659258262890683122, 1.000000000000000000, 0.9659258262890683122, 1.000000000000000000, 0.9659258262890683122, 1.000000000000000000, 0.9659258262890683122, 1.000000000000000000, 0.9659258262890683122, 1.000000000000000000, 0.9659258262890683122, 1.000000000000000000, 0.9659258262890683122, 1.000000000000000000, 0.9659258262890683122, 1.000000000000000000, 0.9659258262890683122, 1.000000000000000000, 0.9659258262890683122, 1.000000000000000000, 0.9659258262890683122, 1.000000000000000000, 0.9659258262890683122, 1.000000000000000000, 0.9659258262890683122, 1.000000000000000000, 0.9659258262890683122, 1.000000000000000000, 0.9659258262890683122, 1.000000000000000000, 0.9659258262890683122, 1.000000000000000000, 0.9659258262890683122, 1.000000000000000000, 0.9659258262890683122, 1.000000000000000000, 0.9659258262890683122, 1.000000000000000000, 0.9659258262890683122, 1.000000000000000000, 0.9659258262890683122, 1.000000000000000000, 0.9659258262890683122, 1.000000000000000000, 0.9659258262890683122, 1.000000000000000000, 0.9659258262890683122, 1.000000000000000000, 0.9659258262890683122, 1.000000000000000000, 0.9659258262890683122, 1.000000000000000000, 0.9659258262890683122, 1.000000000000000000, 0.9659258262890683122, 1.000000000000000000, 0.9659258262890683122, 1.000000000000000000, 0.9659258262890683122, 1.000000000000000000, 0.9659258262890683122, 1.000000000000000000, 0.9659258262890683122, 1.000000000000000000, 0.9659258262890683122, 1.000000000000000000, 0.9659258262890683122, 1.000000000000000000, 0.9659258262890683122, 1.000000000000000000, 0.9659258262890683122, 1.000000000000000000, 0.9659258262890683122, 1.000000000000000000, 0.9659258262890683122, 1.000000000000000000, 0.9659258262890683122, 1.000000000000000000, 0.9659258262890683122, 1.000000000000000000, 0.9659258262890683122, 1.000000000000000000, 0.9659258262890683122, 1.000000000000000000, 0.9659258262890683122, 1.000000000000000000, 0.9659258262890683122, 1.000000000000000000, 0.9659258262890683122, 1.000000000000000000, 0.9659258262890683122, 1.000000000000000000, 0.9659258262890683122, 1.000000000000000000, 0.9659258262890683122, 1.000000000000000000, 0.9659258262890683122, 1.000000000000000000, 0.9659258262890683122, 1.000000000000000000, 0.9659258262890683122, 1.000000000000000000, 0.9659258262890683122, 1.000000000000000000, 0.9659258262890683122, 1.000000000000000000, 0.9659258262890683122, 1.000000000000000000, 0.9659258262890683122, 1.000000000000000000, 0.9659258262890683122, 1.000000000000000000, 0.9659258262890683122, 1.000000000000000000, 0.9659258262890683122, 1.000000000000000000, 0.9659258262890683122, 1.000000000000000000, 0.9659258262890683122, 1.000000000000000000, 0.9659258262890683122, 1.000000000000000000, 0.9659258262890683122, 1.000000000000000000, 0.9659258262890683122, 1.000000000000000000, 0.9659258262890683122, 1.000000000000000000, 0.9659258262890683122, 1.000000000000000000, 0.9659258262890683122, 1.000000000000000000, 0.9659258262890683122, 1.000000000000000000, 0.9659258262890683122, 1.000000000000000000, 0.9659258262890683122, 1.000000000000000000, 0.9659258262890683122, 1.000000000000000000, 0.9659258262890683122, 1.000000000000000000, 0.9659258262890683122, 1.000000000000000000, 0.9659258262890683122, 1.000000000000000000, 0.9659258262890683122, 1.000000000000000000, 0.9659258262890683122, 1.000000000000000000, 0.9659258262890683122, 1.000000000000000000, 0.9659258262890683122, 1.000000000000000000, 0.9659258262890683122, 1.000000000000000000, 0.9659258262890683122, 1.000000000000000000, 0.9659258262890683122, 1.000000000000000000, 0.9659258262890683122, 1.000000000000000000, 0.9659258262890683122, 1.000000000000000000, 0.9659258262890683122, 1.000000000000000000, 0.9659258262890683122, 1.000000000000000000, 0.9659258262890683122, 1.000000000000000000, 0.9659258262890683122, 1.000000000000000000, 0.9659258262890683122, 1.000000000000000000, 0.9659258262890683122, 1.000000000000000000, 0.9659258262890683122, 1.000000000000000000, 0.9659258262890683122, 1.000000000000000000, 0.9659258262890683122, 1.000000000000000000, 0.9659258262890683122, 1.000000000000000000, 0.9659258262890683122, 1.000000000000000000, 0.9659258262890683122, 1.000000000000000000, 0.9659258262890683122, 1.000000000000000000, 0.9659258262890683122, 1.000000000000000000, 0.9659258262890683122, 1.000000000000000000, 0.9659258262890683122, 1.000000000000000000, 0.9659258262890683122, 1.000000000000000000, 0.9659258262890683122, 1.000000000000000000, 0.9659258262890683122, 1.000000000000000000, 0.9659258262890683122, 1.000000000000000000, 0.9659258262890683122, 1.000000000000000000, 0.9659258262890683122, 1.000000000000000000, 0.9659258262890683122, 1.000000000000000000, 0.9659258262890683122, 1.000000000000000000, 0.9659258262890683122, 1.000000000000000000, 0.9659258262890683122, 1.000000000000000000, 0.9659258262890683122, 1.000000000000000000, 0.9659258262890683122, 1.000000000000000000, 0.9659258262890683122, 1.000000000000000000, 0.9659258262890683122, 1.000000000000000000, 0.9659258262890683122, 1.000000000000000000, 0.9659258262890683122, 1.000000000000000000, 0.9659258262890683122, 1.000000000000000000, 0.9659258262890683122, 1.000000000000000000, 0.9659258262890683122, 1.000000000000000000, 0.9659258262890683122, 1.000000000000000000, 0.9659258262890683122, 1.000000000000000000, 0.9659258262890683122, 1.000000000000000000, 0.9659258262890683122, 1.000000000000000000, 0.9659258262890683122, 1.000000000000000000, 0.9659258262890683122, 1.000000000000000000, 0.9659258262890683122, 1.000000000000000000, 0.9659258262890683122, 1.000000000000000000, 0.9659258262890683122, 1.000000000000000000, 0.9659258262890683122, 1.000000000000000000, 0.9659258262890683122, 1.000000000000000000, 0.9659258262890683122, 1.000000000000000000, 0.9659258262890683122, 1.000000000000000000, 0.9659258262890683122, 1.000000000000000000, 0.9659258262890683122, 1.000000000000000000, 0.9659258262890683122, 1.000000000000000000, 0.9659258262890683122, 1.000000000000000000, 0.9659258262890683122, 1.000000000000000000, 0.9659258262890683122, 1.000000000000000000, 0.9659258262890683122, 1.000000000000000000, 0.9659258262890683122, 1.000000000000000000, 0.9659258262890683122, 1.000000000000000000, 0.9659258262890683122, 1.000000000000000000, 0.9659258262890683122, 1.000000000000000000, 0.9659258262890683122, 1.000000000000000000, 0.9659258262890683122, 1.000000000000000000, 0.9659258262890683122, 1.000000000000000000, 0.9659258262890683122, 1.000000000000000000, 0.9659258262890683122, 1.000000000000000000, 0.9659258262890683122, 1.000000000000000000, 0.9659258262890683122, 1.000000000000000000, 0.9659258262890683122, 1.000000000000000000, 0.9659258262890683122, 1.000000000000000000, 0.9659258262890683122, 1.000000000000000000, 0.9659258262890683122, 1.000000000000000000, 0.9659258262890683122, 1.000000000000000000, 0.9659258262890683122, 1.000000000000000000, 0.9659258262890683122, 1.000000000000000000, 0.9659258262890683122, 1.000000000000000000, 0.9659258262890683122, 1.000000000000000000, 0.9659258262890683122, 1.000000000000000000, 0.9659258262890683122, 1.000000000000000000, 0.9659258262890683122, 1.000000000000000000, 0.9659258262890683122, 1.000000000000000000, 0.9659258262890683122, 1.000000000000000000, 0.9659258262890683122, 1.000000000000000000, 0.9659258262890683122, 1.000000000000000000, 0.9659258262890683122, 1.000000000000000000, 0.9659258262890683122, 1.000000000000000000, 0.9659258262890683122, 1.000000000000000000, 0.9659258262890683122, 1.000000000000000000, 0.9659258262890683122, 1.000000000000000000, 0.9659258262890683122, 1.000000000000000000, 0.9659258262890683122, 1.000000000000000000, 0.9659258262890683122, 1.000000000000000000, 0.9659258262890683122, 1.000000000000000000, 0.9659258262890683122, 1.000000000000000000, 0.9659258262890683122, 1.000000000000000000, 0.9659258262890683122, 1.000000000000000000, 0.9659258262890683122, 1.000000000000000000, 0.9659258262890683122, 1.000000000000000000, 0.9659258262890683122, 1.000000000000000000, 0.9659258262890683122, 1.000000000000000000, 0.9659258262890683122, 1.000000000000000000, 0.9659258262890683122, 1.000000000000000000, 0.9659258262890683122, 1.000000000000000000, 0.9659258262890683122, 1.000000000000000000, 0.9659258262890683122, 1.000000000000000000, 0.9659258262890683122, 1.000000000000000000, 0.9659258262890683122, 1.000000000000000000, 0.9659258262890683122, 1.000000000000000000, 0.9659258262890683122, 1.000000000000000000, 0.9659258262890683122, 1.000000000000000000, 0.9659258262890683122, 1.000000000000000000, 0.9659258262890683122, 1.000000000000000000, 0.9659258262890683122, 1.000000000000000000, 0.9659258262890683122, 1.000000000000000000, 0.9659258262890683122, 1.000000000000000000, 0.9659258262890683122, 1.000000000000000000, 0.9659258262890683122, 1.000000000000000000, 0.9659258262890683122, 1.000000000000000000, 0.9659258262890683122, 1.000000000000000000, 0.9659258262890683122, 1.000000000000000000, 0.9659258262890683122, 1.000000000000000000, 0.9659258262890683122, 1.000000000000000000, 0.9659258262890683122, 1.000000000000000000, 0.9659258262890683122, 1.000000000000000000, 0.9659258262890683122, 1.000000000000000000, 0.9659258262890683122, 1.000000000000000000, 0.9659258262890683122, 1.000000000000000000, 0.9659258262890683122, 1.000000000000000000, 0.9659258262890683122, 1.000000000000000000, 0.9659258262890683122, 1.000000000000000000, 0.9659258262890683122, 1.000000000000000000, 0.9659258262890683122, 1.000000000000000000, 0.9659258262890683122, 1.000000000000000000, 0.9659258262890683122, 1.000000000000000000, 0.9659258262890683122, 1.000000000000000000, 0.9659258262890683122, 1.000000000000000000, 0.9659258262890683122, 1.000000000000000000, 0.9659258262890683122, 1.000000000000000000, 0.9659258262890683122, 1.000000000000000000, 0.9659258262890683122, 1.000000000000000000, 0.9659258262890683122, 1.000000000000000000, 0.9659258262890683122, 1.000000000000000000, 0.9659258262890683122, 1.000000000000000000, 0.9659258262890683122, 1.000000000000000000, 0.9659258262890683122, 1.000000000000000000, 0.9659258262890683122, 1.000000000000000000, 0.9659258262890683122, 1.000000000000000000, 0.9659258262890683122, 1.000000000000000000, 0.9659258262890683122, 1.000000000000000000, 0.9659258262890683122, 1.000000000000000000, 0.9659258262890683122, 1.000000000000000000, 0.9659258262890683122, 1.000000000000000000, 0.9659258262890683122, 1.000000000000000000, 0.9659258262890683122, 1.000000000000000000) ) ) 
 REPRESENTATION_ITEM ( '' )  SURFACE ( )  );
#27287=CARTESIAN_POINT ( 'NONE',  ( 0.3937007874015754361, -0.1870078740157479769, 0.4822834645669291653 ) ) ;
#27288=CARTESIAN_POINT ( 'NONE',  ( -0.4002624671916004129, -0.3162353388693405765, 0.4822834645669290543 ) ) ;
#27291=CARTESIAN_POINT ( 'NONE',  ( 0.5971128608923890191, -0.5511811023622046335, 0.09757992244046803654 ) ) ;
#27293=VERTEX_POINT ( 'NONE', #42835 ) ;
#27295=ORIENTED_EDGE ( 'NONE', *, *, #5901, .T. ) ;
#27296=CARTESIAN_POINT ( 'NONE',  ( 0.1049868766404206816, -0.6046776061558809534, -0.2411417322834644161 ) ) ;
#27297=CARTESIAN_POINT ( 'NONE',  ( 1.240157480314961314, -0.5400638737290844871, 0.3530559997133364547 ) ) ;
#27298=CARTESIAN_POINT ( 'NONE',  ( 0.1115485564304470323, 0.2952755905511811885, 0.1292274648535926551 ) ) ;
#27299=CARTESIAN_POINT ( 'NONE',  ( -0.2493438320209966919, -0.3690944881889763329, 0.3153832671262228327 ) ) ;
#27300=CARTESIAN_POINT ( 'NONE',  ( 1.115485564304462551, -0.4281496062992127816, -0.4176697321401328100 ) ) ;
#27301=CARTESIAN_POINT ( 'NONE',  ( -0.5314960629921250401, 0.1660481256975885056, 0.3530559997133364547 ) ) ;
#27302=CARTESIAN_POINT ( 'NONE',  ( -0.1706036745406816491, -0.4281496062992124485, 0.4176697321401328655 ) ) ;
#27303=CARTESIAN_POINT ( 'NONE',  ( -1.489501312335957062, -0.05778040916215522460, 0.4822834645669289988 ) ) ;
#27304=CARTESIAN_POINT ( 'NONE',  ( 0.9580052493438326877, 0.05413385826771666132, 0.4176697321401328100 ) ) ;
#27305=CARTESIAN_POINT ( 'NONE',  ( 1.213910761154856299, 0.2952755905511811885, 0.1292274648535926551 ) ) ;
#27307=CARTESIAN_POINT ( 'NONE',  ( 0.4002624671916016896, -0.08942795157527998196, 0.3641732283464567121 ) ) ;
#27311=CARTESIAN_POINT ( 'NONE',  ( -0.6364829396325453192, -0.2845877964562159024, 0.3641732283464567677 ) ) ;
#27312=CARTESIAN_POINT ( 'NONE',  ( 0.1443569553805781891, 0.05413385826771626580, -0.4176697321401330321 ) ) ;
#27314=CARTESIAN_POINT ( 'NONE',  ( -0.1968503937007867743, -0.6692913385826771977, 8.415575281601705876E-17 ) ) ;
#27315=CARTESIAN_POINT ( 'NONE',  ( -0.08530183727034056085, -0.05778040916215560624, -0.4822834645669293319 ) ) ;
#27316=CARTESIAN_POINT ( 'NONE',  ( -0.7086614173228339419, -0.1870078740157479769, 0.4822834645669291653 ) ) ;
#27317=CARTESIAN_POINT ( 'NONE',  ( -1.122047244094487306, -0.5400638737290844871, 0.3530559997133364547 ) ) ;
#27318=CARTESIAN_POINT ( 'NONE',  ( 1.502624671916010790, -0.08942795157527998196, 0.3641732283464567121 ) ) ;
#27320=CARTESIAN_POINT ( 'NONE',  ( 0.9842519685039375910, 0.1771653543307087630, 0.000000000000000000 ) ) ;
#27321=AXIS2_PLACEMENT_3D ( 'NONE', #80399, #29022, #28613 ) ;
#27322=CARTESIAN_POINT ( 'NONE',  ( 0.6430446194225729606, -0.4281496062992127816, -0.4176697321401328100 ) ) ;
#27323=CARTESIAN_POINT ( 'NONE',  ( 0.4265091863517067594, 0.2952755905511811885, 0.1292274648535926551 ) ) ;
#27328=CARTESIAN_POINT ( 'NONE',  ( -0.3543307086614165824, -0.6692913385826771977, 8.415575281601705876E-17 ) ) ;
#27331=CARTESIAN_POINT ( 'NONE',  ( -1.332020997375327642, -0.08942795157527998196, 0.3641732283464567121 ) ) ;
#27332=CARTESIAN_POINT ( 'NONE',  ( 1.030183727034121421, -0.3162353388693409650, -0.4822834645669289433 ) ) ;
#27333=CARTESIAN_POINT ( 'NONE',  ( 0.9186351706036752773, 0.2306618581243847221, -0.2411417322834647770 ) ) ;
#27334=CARTESIAN_POINT ( 'NONE',  ( -0.2296587926509179312, -0.08942795157527998196, 0.3641732283464567121 ) ) ;
#27335=CARTESIAN_POINT ( 'NONE',  ( 0.3149606299212603933, -0.1870078740157479769, 0.4822834645669291653 ) ) ;
#27337=CARTESIAN_POINT ( 'NONE',  ( -0.2165354330708654795, 0.07958543189024085140, 0.2665933059059887866 ) ) ;
#27338=B_SPLINE_CURVE_WITH_KNOTS ( 'NONE', 3,
 ( #52702, #33370, #40095, #27459, #40511, #66192, #8528 ),
 .UNSPECIFIED., .F., .F.,
 ( 4, 3, 4 ),
 ( 1.734723475976807094E-17, 0.001246230184515588870, 0.002492489877932651133 ),
 .UNSPECIFIED. ) ;
#27339=CARTESIAN_POINT ( 'NONE',  ( -0.09186351706036689768, 0.05413385826771626580, -0.4176697321401330321 ) ) ;
#27342=CARTESIAN_POINT ( 'NONE',  ( -1.463254593175852492, -0.6692913385826773087, -0.1292274648535924053 ) ) ;
#27343=CARTESIAN_POINT ( 'NONE',  ( 0.3937007874015754361, -0.1870078740157480601, -0.3641732283464567677 ) ) ;
#27344=CARTESIAN_POINT ( 'NONE',  ( 1.423884514435696413, -0.2845877964562161244, -0.3641732283464567121 ) ) ;
#27345=CARTESIAN_POINT ( 'NONE',  ( -0.9120734908136475250, 0.2952755905511811885, 0.1292274648535926551 ) ) ;
#27346=CARTESIAN_POINT ( 'NONE',  ( -0.3674540682414689785, 0.1283753931104748280, 0.1820866141732283561 ) ) ;
#27348=CARTESIAN_POINT ( 'NONE',  ( -0.5708661417322828946, 0.1660481256975883668, -0.3530559997133364547 ) ) ;
#27349=CARTESIAN_POINT ( 'NONE',  ( -0.5643044619422565855, -0.4281496062992124485, 0.4176697321401328655 ) ) ;
#27350=CARTESIAN_POINT ( 'NONE',  ( -0.09842519685039295696, -0.5400638737290844871, 0.3530559997133364547 ) ) ;
#27353=CARTESIAN_POINT ( 'NONE',  ( -1.686351706036744558, 0.1771653543307087075, -0.09757992244046823083 ) ) ;
#27354=CARTESIAN_POINT ( 'NONE',  ( 0.6889763779527566800, -0.4536011799217367080, 0.2665933059059888421 ) ) ;
#27355=CARTESIAN_POINT ( 'NONE',  ( 1.292650918635171564, 0.2952755905511811885, 0.1292274648535926551 ) ) ;
#27356=CARTESIAN_POINT ( 'NONE',  ( -1.082677165354329896, 0.07958543189024085140, 0.2665933059059887866 ) ) ;
#27357=CARTESIAN_POINT ( 'NONE',  ( -0.9580052493438311334, -0.3690944881889763329, 0.3153832671262228327 ) ) ;
#27358=CARTESIAN_POINT ( 'NONE',  ( -0.4265091863517051496, 0.2952755905511810774, -0.1292274648535930714 ) ) ;
#27359=CARTESIAN_POINT ( 'NONE',  ( 0.5380577427821529035, -0.3690944881889763329, 0.3153832671262228327 ) ) ;
#27361=CARTESIAN_POINT ( 'NONE',  ( 0.9711286089238851948, 0.1283753931104748280, 0.1820866141732283561 ) ) ;
#27362=CARTESIAN_POINT ( 'NONE',  ( 0.5052493438320218022, -0.6692913385826773087, -0.1292274648535924053 ) ) ;
#27364=CARTESIAN_POINT ( 'NONE',  ( -0.5905511811023615998, 0.2952755905511811885, 0.000000000000000000 ) ) ;
#27366=CARTESIAN_POINT ( 'NONE',  ( 1.318897637795276356, 0.07958543189024071263, -0.2665933059059888421 ) ) ;
#27367=CARTESIAN_POINT ( 'NONE',  ( 0.6036745406824154392, 0.2306618581243847221, -0.2411417322834647770 ) ) ;
#27368=CARTESIAN_POINT ( 'NONE',  ( 0.1312335958005257930, 0.2306618581243847221, -0.2411417322834647770 ) ) ;
#27369=CARTESIAN_POINT ( 'NONE',  ( 0.2099737532808405305, -0.5023911411419708095, 0.1820866141732285504 ) ) ;
#27370=CARTESIAN_POINT ( 'NONE',  ( -1.646051170424378096, 0.000000000000000000, -0.3464511005275205946 ) ) ;
#27371=CARTESIAN_POINT ( 'NONE',  ( -0.2034120734908128059, 0.1771653543307087630, 0.09757992244046791164 ) ) ;
#27372=CARTESIAN_POINT ( 'NONE',  ( 0.6233595800524942554, -0.05778040916215560624, -0.4822834645669293319 ) ) ;
#27373=CARTESIAN_POINT ( 'NONE',  ( -0.8005249343832013809, -0.3690944881889763329, 0.3153832671262228327 ) ) ;
#27375=CARTESIAN_POINT ( 'NONE',  ( -0.9776902887139098386, 0.2952755905511810774, -0.1292274648535930714 ) ) ;
#27376=CARTESIAN_POINT ( 'NONE',  ( 0.1771653543307093459, 0.1012011053420777407, 0.2882089793578257453 ) ) ;
#27378=CARTESIAN_POINT ( 'NONE',  ( -1.351706036745406347, -0.4281496062992124485, 0.4176697321401328655 ) ) ;
#27379=AXIS2_PLACEMENT_3D ( 'NONE', #34839, #54169, #9575 ) ;
#27380=CARTESIAN_POINT ( 'NONE',  ( -0.9448818897637790704, -0.1870078740157479769, 0.3641732283464567677 ) ) ;
#27381=CARTESIAN_POINT ( 'NONE',  ( 0.1443569553805781891, -0.4281496062992124485, 0.4176697321401328655 ) ) ;
#27382=CARTESIAN_POINT ( 'NONE',  ( -1.653543307086613234, -0.1870078740157480879, -0.4822834645669291653 ) ) ;
#27383=CARTESIAN_POINT ( 'NONE',  ( -0.6102362204724400829, -0.5400638737290845981, -0.3530559997133363437 ) ) ;
#27385=CARTESIAN_POINT ( 'NONE',  ( 1.607611548556431069, -0.6692913385826773087, -0.1292274648535924053 ) ) ;
#27386=CARTESIAN_POINT ( 'NONE',  ( 0.8005249343832027131, 0.05413385826771666132, 0.4176697321401328100 ) ) ;
#27387=CARTESIAN_POINT ( 'NONE',  ( 0.9908136482939640111, -0.6692913385826771977, 0.1292274648535927661 ) ) ;
#27389=CARTESIAN_POINT ( 'NONE',  ( 1.535433070866142335, -0.6692913385826771977, 8.415575281601705876E-17 ) ) ;
#27390=CARTESIAN_POINT ( 'NONE',  ( -1.377952755905511140, 0.2952755905511811885, 0.000000000000000000 ) ) ;
#27393=CARTESIAN_POINT ( 'NONE',  ( -0.6364829396325453192, -0.08942795157528024563, -0.3641732283464568787 ) ) ;
#27394=AXIS2_PLACEMENT_3D ( 'NONE', #68971, #59238, #57977 ) ;
#27397=CARTESIAN_POINT ( 'NONE',  ( 0.4593175853018379162, -0.4281496062992124485, 0.4176697321401328655 ) ) ;
#27398=CARTESIAN_POINT ( 'NONE',  ( -0.08530183727034056085, -0.05778040916215560624, -0.4822834645669293319 ) ) ;
#27399=CARTESIAN_POINT ( 'NONE',  ( -0.7808398950131222316, -0.3162353388693409650, -0.4822834645669289433 ) ) ;
#27400=CARTESIAN_POINT ( 'NONE',  ( 1.391076115485564868, 0.2306618581243847221, -0.2411417322834647770 ) ) ;
#27401=CARTESIAN_POINT ( 'NONE',  ( -0.9842519685039360366, 0.1771653543307087630, 0.000000000000000000 ) ) ;
#27403=CARTESIAN_POINT ( 'NONE',  ( 0.6692913385826778638, -0.6692913385826771977, 8.415575281601705876E-17 ) ) ;
#27404=CARTESIAN_POINT ( 'NONE',  ( 0.5183727034120741983, 0.1771653543307087075, -0.09757992244046823083 ) ) ;
#27405=CARTESIAN_POINT ( 'NONE',  ( -0.2821522309711278487, -0.6692913385826773087, -0.1292274648535924053 ) ) ;
#27407=CARTESIAN_POINT ( 'NONE',  ( -0.9580052493438311334, 0.05413385826771626580, -0.4176697321401330321 ) ) ;
#27408=CARTESIAN_POINT ( 'NONE',  ( -1.666666666666665853, -0.004921259842519870586, -0.3153832671262229437 ) ) ;
#27409=CARTESIAN_POINT ( 'NONE',  ( 1.437007874015748810, -0.5400638737290845981, -0.3530559997133363437 ) ) ;
#27410=CARTESIAN_POINT ( 'NONE',  ( 1.548556430446194954, 0.1283753931104746893, -0.1820866141732285504 ) ) ;
#27413=CARTESIAN_POINT ( 'NONE',  ( 8.195543980992789655E-16, -0.1870078740157480879, -0.4822834645669291653 ) ) ;
#27415=CARTESIAN_POINT ( 'NONE',  ( -1.076115485564303809, 0.2306618581243848609, 0.2411417322834645549 ) ) ;
#27416=CARTESIAN_POINT ( 'NONE',  ( 1.187664041994751285, -0.3162353388693409650, -0.4822834645669289433 ) ) ;
#27417=CARTESIAN_POINT ( 'NONE',  ( 1.286089238845145033, 0.2306618581243848609, 0.2411417322834645549 ) ) ;
#27418=CARTESIAN_POINT ( 'NONE',  ( 0.2034120734908142214, 0.2952755905511810774, -0.1292274648535930714 ) ) ;
#27419=CARTESIAN_POINT ( 'NONE',  ( -0.4199475065616791736, -0.6046776061558807314, 0.2411417322834647770 ) ) ;
#27421=CARTESIAN_POINT ( 'NONE',  ( -1.318897637795274802, -0.5400638737290845981, -0.3530559997133363437 ) ) ;
#27422=CARTESIAN_POINT ( 'NONE',  ( -0.5971128608923877978, -0.6692913385826773087, -0.1292274648535924053 ) ) ;
#27423=CARTESIAN_POINT ( 'NONE',  ( -0.4265091863517051496, -0.5511811023622046335, 0.09757992244046803654 ) ) ;
#27426=CARTESIAN_POINT ( 'NONE',  ( -0.4593175853018366950, 0.05413385826771666132, 0.4176697321401328100 ) ) ;
#27427=CARTESIAN_POINT ( 'NONE',  ( -1.200787401574802349, 0.1660481256975883391, -0.3530559997133364547 ) ) ;
#27428=CARTESIAN_POINT ( 'NONE',  ( 0.9186351706036751663, -0.6046776061558807314, 0.2411417322834647770 ) ) ;
#27432=CARTESIAN_POINT ( 'NONE',  ( -0.2821522309711278487, -0.6692913385826773087, -0.1292274648535924053 ) ) ;
#27433=CARTESIAN_POINT ( 'NONE',  ( 1.154855643044620184, -0.5023911411419708095, 0.1820866141732285504 ) ) ;
#27434=CARTESIAN_POINT ( 'NONE',  ( 0.6986524979670498681, 8.471767977567108961E-16, -0.4445507791589058955 ) ) ;
#27436=CARTESIAN_POINT ( 'NONE',  ( 1.167979002624672580, -0.3690944881889763329, 0.3153832671262228327 ) ) ;
#27437=B_SPLINE_CURVE_WITH_KNOTS ( 'NONE', 3,
 ( #50980, #17391, #70355, #24902, #43022, #31637, #57297 ),
 .UNSPECIFIED., .F., .F.,
 ( 4, 3, 4 ),
 ( 5.204170427930421283E-18, 0.001246230184515576727, 0.002492489877932660240 ),
 .UNSPECIFIED. ) ;
#27438=CARTESIAN_POINT ( 'NONE',  ( 1.207349081364829990, -0.6046776061558809534, -0.2411417322834644161 ) ) ;
#27440=CARTESIAN_POINT ( 'NONE',  ( -0.01312335958005186876, -0.4281496062992124485, 0.4176697321401328655 ) ) ;
#27441=CARTESIAN_POINT ( 'NONE',  ( -0.7080320533160963103, 2.362204724409448620, -0.5309055118110235227 ) ) ;
#27442=AXIS2_PLACEMENT_3D ( 'NONE', #13111, #12690, #82975 ) ;
#27443=CARTESIAN_POINT ( 'NONE',  ( -1.430446194225721390, -0.4281496062992124485, 0.4176697321401328655 ) ) ;
#27444=CARTESIAN_POINT ( 'NONE',  ( -0.08530183727034056085, -0.05778040916215560624, -0.4822834645669293319 ) ) ;
#27446=CARTESIAN_POINT ( 'NONE',  ( 1.181102362204725198, -0.1870078740157479769, 0.4822834645669291653 ) ) ;
#27447=CARTESIAN_POINT ( 'NONE',  ( 0.5971128608923890191, -0.6692913385826771977, 0.1292274648535927661 ) ) ;
#27448=CARTESIAN_POINT ( 'NONE',  ( 0.8661417322834653598, -0.1870078740157479769, 0.3641732283464567677 ) ) ;
#27450=CARTESIAN_POINT ( 'NONE',  ( 0.5971128608923891301, 0.1771653543307087075, -0.09757992244046823083 ) ) ;
#27451=CARTESIAN_POINT ( 'NONE',  ( -1.076115485564303809, -0.6046776061558809534, -0.2411417322834644161 ) ) ;
#27453=CARTESIAN_POINT ( 'NONE',  ( 1.213910761154856299, 0.2952755905511811885, 0.1292274648535926551 ) ) ;
#27457=CARTESIAN_POINT ( 'NONE',  ( 0.3543307086614181922, -0.6692913385826771977, 8.415575281601705876E-17 ) ) ;
#27458=CARTESIAN_POINT ( 'NONE',  ( 0.9120734908136490793, 0.2952755905511810219, -0.1292274648535930437 ) ) ;
#27459=CARTESIAN_POINT ( 'NONE',  ( -0.7984992590978650107, -3.187520833735697382E-15, -0.3954974714151482384 ) ) ;
#27460=CARTESIAN_POINT ( 'NONE',  ( 0.2690288713910767848, -0.5511811023622048555, -0.09757992244046775898 ) ) ;
#27462=CARTESIAN_POINT ( 'NONE',  ( 0.3805774278215230400, -0.4281496062992124485, 0.4176697321401328655 ) ) ;
#27464=CARTESIAN_POINT ( 'NONE',  ( -0.8727034120734901146, -0.08942795157528024563, -0.3641732283464568787 ) ) ;
#27465=CARTESIAN_POINT ( 'NONE',  ( -0.9711286089238838626, -0.6046776061558807314, 0.2411417322834647770 ) ) ;
#27466=CARTESIAN_POINT ( 'NONE',  ( -1.640419947506561060, -0.4281496062992127816, -0.4176697321401328100 ) ) ;
#27467=CARTESIAN_POINT ( 'NONE',  ( 0.4396325459317593221, 0.2952755905511810774, -0.1292274648535930714 ) ) ;
#27468=CARTESIAN_POINT ( 'NONE',  ( -1.640419947506561060, -0.004921259842519576551, 0.3153832671262227771 ) ) ;
#27470=CARTESIAN_POINT ( 'NONE',  ( 0.5708661417322841158, -0.5400638737290845981, -0.3530559997133363437 ) ) ;
#27472=CARTESIAN_POINT ( 'NONE',  ( 1.561679790026247350, 0.05413385826771626580, -0.4176697321401330321 ) ) ;
#27473=CARTESIAN_POINT ( 'NONE',  ( 1.272965879265092637, -0.4281496062992127816, -0.4176697321401328100 ) ) ;
#27474=CARTESIAN_POINT ( 'NONE',  ( -1.410761154855642463, -0.08942795157527998196, 0.3641732283464567121 ) ) ;
#27475=CARTESIAN_POINT ( 'NONE',  ( 1.292650918635171564, -0.5511811023622048555, -0.09757992244046775898 ) ) ;
#27476=CARTESIAN_POINT ( 'NONE',  ( -1.463254593175852492, 0.1771653543307087630, 0.09757992244046791164 ) ) ;
#27477=CARTESIAN_POINT ( 'NONE',  ( -0.7742782152230962556, -0.3690944881889765550, -0.3153832671262227771 ) ) ;
#27478=CARTESIAN_POINT ( 'NONE',  ( 1.568241469816273437, -0.3162353388693405765, 0.4822834645669290543 ) ) ;
#27479=CARTESIAN_POINT ( 'NONE',  ( 0.4724409448818904789, -0.1870078740157479769, 0.3641732283464567677 ) ) ;
#27480=CARTESIAN_POINT ( 'NONE',  ( 0.6167979002624679463, 0.05413385826771626580, -0.4176697321401330321 ) ) ;
#27481=CARTESIAN_POINT ( 'NONE',  ( 1.286089238845145033, 0.2306618581243848609, 0.2411417322834645549 ) ) ;
#27482=CARTESIAN_POINT ( 'NONE',  ( 0.1049868766404206816, 0.2306618581243848609, 0.2411417322834645549 ) ) ;
#27483=CARTESIAN_POINT ( 'NONE',  ( 0.3543307086614179147, 0.1771653543307087630, 0.000000000000000000 ) ) ;
#27484=CARTESIAN_POINT ( 'NONE',  ( 1.371391076115485719, -0.6692913385826773087, -0.1292274648535924053 ) ) ;
#27485=CARTESIAN_POINT ( 'NONE',  ( -1.568241469816272105, -0.3162353388693409650, -0.4822834645669289433 ) ) ;
#27486=CARTESIAN_POINT ( 'NONE',  ( -0.8005249343832013809, -0.4281496062992124485, 0.4176697321401328655 ) ) ;
#27488=DIRECTION ( 'NONE',  ( -1.000000000000000000, -3.050063254464715288E-16, 0.000000000000000000 ) ) ;
#27489=CARTESIAN_POINT ( 'NONE',  ( -0.03280839895013062252, -0.6692913385826771977, 0.1292274648535927661 ) ) ;
#27490=CARTESIAN_POINT ( 'NONE',  ( -0.7611548556430438595, -0.6046776061558809534, -0.2411417322834644161 ) ) ;
#27492=CARTESIAN_POINT ( 'NONE',  ( -0.1574803149606292529, -0.1870078740157479769, 0.4822834645669291653 ) ) ;
#27498=CARTESIAN_POINT ( 'NONE',  ( -1.417322834645668772, -0.1870078740157479769, 0.3641732283464567677 ) ) ;
#27500=CARTESIAN_POINT ( 'NONE',  ( -1.450131233595799651, -0.6692913385826771977, 0.1292274648535927661 ) ) ;
#27503=CARTESIAN_POINT ( 'NONE',  ( 0.4461942257217856311, 0.2306618581243847221, -0.2411417322834647770 ) ) ;
#27504=CARTESIAN_POINT ( 'NONE',  ( -0.6036745406824141069, 0.1283753931104748280, 0.1820866141732283561 ) ) ;
#27505=CARTESIAN_POINT ( 'NONE',  ( 0.7217847769028878924, -0.4281496062992127816, -0.4176697321401328100 ) ) ;
#27506=CARTESIAN_POINT ( 'NONE',  ( 0.1640419947506569498, -0.05778040916215522460, 0.4822834645669289988 ) ) ;
#27510=CARTESIAN_POINT ( 'NONE',  ( 1.095800524934383846, -0.05778040916215560624, -0.4822834645669293319 ) ) ;
#27511=CARTESIAN_POINT ( 'NONE',  ( 0.1640419947506569498, -0.05778040916215522460, 0.4822834645669289988 ) ) ;
#27513=CARTESIAN_POINT ( 'NONE',  ( 1.515748031496063186, -0.5400638737290845981, -0.3530559997133363437 ) ) ;
#27514=CARTESIAN_POINT ( 'NONE',  ( 0.8530183727034128527, -0.4281496062992124485, 0.4176697321401328655 ) ) ;
#27516=CARTESIAN_POINT ( 'NONE',  ( 0.2165354330708668673, 0.1660481256975883668, -0.3530559997133364547 ) ) ;
#27517=CARTESIAN_POINT ( 'NONE',  ( 0.6496062992125991586, -0.5400638737290845981, -0.3530559997133363437 ) ) ;
#27518=CARTESIAN_POINT ( 'NONE',  ( 0.1377952755905518800, 0.1660481256975883668, -0.3530559997133364547 ) ) ;
#27519=CARTESIAN_POINT ( 'NONE',  ( 0.6364829396325465405, -0.2845877964562161244, -0.3641732283464567121 ) ) ;
#27520=CARTESIAN_POINT ( 'NONE',  ( -1.233595800524933894, 0.2306618581243848609, 0.2411417322834645549 ) ) ;
#27521=CARTESIAN_POINT ( 'NONE',  ( -1.541994750656167090, 0.2952755905511811885, 0.1292274648535926551 ) ) ;
#27522=CARTESIAN_POINT ( 'NONE',  ( 0.6496062992125991586, 0.1660481256975885056, 0.3530559997133364547 ) ) ;
#27525=( BOUNDED_SURFACE ( )  B_SPLINE_SURFACE ( 1, 2, ( 
 ( #56580, #57404, #76375, #63728, #25416, #64153, #69231, #18708, #70886, #50267, #63318, #6487, #56987, #82684, #12395, #5656, #62916, #56172, #11987, #57813, #75965, #11579, #83095, #180, #25833, #76778, #19110, #44350, #43947, #13235, #81875, #75556, #17895, #43532, #37238, #39725, #51916, #79295, #78041, #21203, #8577, #65831, #19956, #15314, #14899, #78463, #71717, #52755, #59081, #1849, #47273, #20788, #26680, #7323, #40559, #46444, #59495, #64988, #6901, #71300, #52335, #46858, #72552, #27928, #26257, #20371, #65418, #72135, #14493, #66240, #2263, #53586, #64564, #1436, #58234, #7754, #46023, #53167, #27092, #33829, #40146, #21613, #32572, #72963, #601, #77623, #14072, #45606, #8164, #13648, #34248, #27510, #39301, #78880, #32992, #59910, #58661, #1027, #33419, #16145, #80130, #80545, #29990, #74636, #75047, #2681, #60333, #61153, #3093, #29581, #61577, #15736, #28757, #60741, #74218, #73808, #41792, #36311, #8997, #35489, #16563, #34670, #10240, #42208, #3505, #67483, #79714, #41391, #55244, #29172, #40977, #22857, #35075, #28341, #54002, #55653, #80951, #3920, #9818, #22030, #10656, #66659, #47691, #54840, #73385, #35910, #67073, #48518, #9405, #81363, #23266, #67903, #16979, #48935, #42620, #54419, #68319, #23676, #22449, #48110, #61987, #4324, #49348, #44662, #63221, #44255, #50168, #75459, #17393, #82185, #82998, #37135, #24089, #12300, #12713, #57300, #50574, #82586, #37546, #69129, #5561, #62820, #70358, #25319, #17797, #50983, #75864, #4731, #32059, #30817, #76681, #38372, #18612, #56072, #51396, #19014, #6388, #64048, #43024, #62394, #36718, #31225, #5153, #5971, #37956, #43432, #56482, #24502, #76280, #18206, #43842, #57719, #68718, #11893, #69945, #11060, #63633, #31640, #56893, #69544, #81779, #11479, #82, #24905, #30405, #25735, #49759, #38789, #64466, #66147, #8075, #40055, #52241, #32474, #46769, #77100, #70787, #39631, #6803, #72043, #58136, #58991, #45508, #8484, #65742, #7659, #53074, #77945, #71622, #51819, #20274, #34153, #505, #931, #1756, #59398, #20697, #7226, #27413, #45924, #33738, #13548, #26997, #78785, #26158, #21110, #65321, #72461, #46348, #77524, #19859, #39204, #14810, #59814, #14399, #40469, #32898, #58565, #13974, #33329, #2169, #27835, #19432, #45083, #13138, #1347, #71205, #52660, #78366, #26588, #64887, #55145, #74538, #16884, #4227, #73712, #47180, #80034, #41296, #42112, #16052, #22760, #41698, #10559, #53496, #42522, #68225, #36217, #66981, #40880, #61061, #34572, #35811, #3412, #28246, #16467, #61886, #3825, #79205, #8895, #54745, #28664, #9314, #9725, #67809, #48013, #21521, #35396, #47597, #15220, #66562, #72872, #10146, #61477, #54325, #60239, #23168, #2587, #53906, #67391, #79620, #48422, #21937, #29074, #73291, #15639, #29486, #80450, #80856, #22353, #74121, #34984, #48837, #60648, #2998, #37036, #38990, #13337, #57925, #43328, #64673, #57512, #45297, #49662, #64259, #70993, #10960, #7012, #76888, #77307, #289, #36618, #55970, #75352, #19636, #13757, #51603, #32680, #69028, #11379, #83203, #31849, #25945, #58347, #26366, #55554, #708, #44867, #4633, #19218, #70566, #63837, #6174, #52025, #77731, #20060, #65098, #51190, #23578, #25525, #17700, #45713, #12921, #71410, #38578, #39414, #29891, #81263, #49249, #74952, #6593, #17298, #32264, #62296, #42925, #68620, #30304, #81683, #23994, #41086, #7435, #46136, #8688, #65936, #46552, #46966, #79826, #66775, #41501, #52440, #26784, #27619, #52863, #79403, #28036, #65527, #78573, #27199, #40665, #40253, #8272, #2792, #58772, #1957, #66349, #1134, #60024, #34358, #53282, #33937, #71830, #7859, #2379, #21722, #14180, #73076, #78993, #53694, #47385, #39838, #33524, #20899, #15425, #73504, #9108, #34781, #72250, #14599, #59602, #21313, #60440, #28451, #54111, #33105, #22142, #72660, #59187, #15008, #47800, #15852, #78151, #20482, #1545, #30522, #17909, #4028, #60850, #10356, #54947, #55766, #29693, #36423, #55355, #24198, #67186, #56184, #81887, #49869, #80653, #54528, #74742, #48221, #49462, #17091, #41904, #30104, #4847, #17501, #9517, #22559, #68423 ),
 ( #9929, #81061, #16258, #75156, #75568, #35189, #42313, #11176, #3203, #74327, #43132, #23377, #68012, #67598, #80243, #68829, #3617, #49045, #73917, #16674, #28866, #36016, #61687, #42727, #23790, #10763, #35601, #61263, #29283, #22966, #62096, #48632, #4438, #81473, #62509, #36836, #57416, #77209, #11998, #12825, #63741, #76791, #64166, #19538, #24611, #6080, #6914, #43958, #76386, #37652, #70898, #31754, #70468, #18719, #18316, #25015, #12407, #44361, #38482, #25845, #38897, #69244, #51505, #83109, #69654, #25428, #51093, #70053, #38065, #45195, #64576, #32585, #77635, #19122, #37252, #44771, #31334, #32169, #6499, #57825, #193, #613, #43545, #58248, #26269, #51930, #56999, #30925, #13248, #50278, #11592, #62927, #63330, #5261, #56592, #82292, #75976, #5667, #82696, #50688, #59093, #59507, #9010, #53598, #54014, #65000, #39312, #40158, #65433, #8590, #40570, #78054, #7766, #39737, #53178, #52767, #20800, #15327, #71312, #14505, #78893, #13660, #72563, #21214, #65842, #78476, #58673, #20384, #34261, #8175, #19967, #1860, #14085, #7335, #33003, #34682, #59922, #66251, #46456, #1038, #72975, #45618, #26692, #33841, #52347, #14910, #46035, #27522, #71730, #60345, #2277, #46869, #79307, #72149, #27940, #33432, #21625, #2693, #1448, #27105, #47285, #40992, #66671, #28353, #61999, #22869, #10669, #16157, #29593, #36325, #60753, #4336, #42220, #42634, #23278, #3105, #22464, #41804, #68331, #62406, #16991, #81375, #35502, #10252, #67085, #29186, #79726, #48530, #74230, #54854, #30002, #67916, #4745, #47703, #73399, #30418, #80557, #15749, #35923, #48122, #75059, #28770, #61589, #55666, #73820, #48948, #16575, #55256, #23688, #49362, #54432, #3935, #43036, #80142, #80963, #67495, #17406, #74649, #68732, #11072, #9831, #22043, #61166, #36731, #3517, #41403, #9417, #35087, #12725, #5984, #37969, #76293, #24514, #18624, #75877, #94, #64061, #56495, #38384, #31238, #43444, #70799, #69557, #6400, #25747, #57312, #11493, #6817, #32071, #69958, #63233, #44267, #50586, #76693, #38802, #12312, #18219, #82197, #57731, #63645, #50995, #50182, #81791, #62832, #43854, #51410, #77112, #19445, #17811, #11905, #56905, #31655, #83010, #69143, #25331, #37559, #19027, #5573, #13152, #45095, #64479, #49771, #44675, #75471, #70370, #82601, #56086, #24102, #24918, #37147, #5166, #30830, #13563, #72886, #58579, #52672, #64902, #40483, #21535, #15235, #7671, #59830, #79219, #39644, #66161, #72056, #33342, #32913, #45522, #34167, #52254, #32487, #13988, #14823, #77960, #39217, #27426, #27850, #72474, #65754, #14413, #78380, #944, #20710, #20289, #2183, #8501, #26602, #53511, #59004, #19873, #47195, #45938, #40895, #66576, #33751, #71218, #58150, #519, #46363, #65335, #40067, #27011, #53087, #26172, #8087, #71636, #1359, #51833, #59412, #78799, #1768, #77538, #7239, #21123, #46783, #16899, #55570, #53922, #54340, #67406, #74137, #48437, #21952, #80465, #73729, #10161, #3012, #49265, #68240, #61902, #2602, #22775, #28260, #16481, #60664, #42538, #60254, #16067, #42128, #79634, #4243, #73306, #74967, #34998, #29089, #41311, #10575, #81278, #17313, #9740, #36232, #23594, #41713, #29906, #67823, #35411, #9328, #47610, #42941, #28679, #35827, #15654, #61075, #8911, #3426, #54759, #61493, #48853, #3841, #34586, #66996, #80050, #22369, #29501, #48028, #55161, #80871, #23183, #74554, #82506, #18931, #37051, #37875, #5479, #18530, #5883, #44579, #49677, #31140, #31974, #69045, #18123, #62733, #12626, #56807, #12218, #43755, #43343, #51311, #31556, #70272, #24415, #50085, #37466, #69461, #63549, #50900, #63961, #10975, #76600, #24822, #11394, #50490, #76193, #11811, #63139, #38285, #6298, #57634, #19346, #44173, #62311, #69866, #56403, #57213, #82915, #25235, #22215, #25649, #68636, #77014, #36635, #4648, #82102, #55987, #30319, #75368, #81698, #24009, #5071, #17715, #30740, #75781, #44996, #415, #46261, #20185, #840, #1261, #34063, #78698, #79119, #6716, #64380, #65229, #7136, #33649, #65656, #19767, #32809, #64797, #78277, #77856, #45836, #40377, #13048, #39541, #20609, #38701, #14309 ) ),
 .UNSPECIFIED., .F., .F., .F. ) 
 B_SPLINE_SURFACE_WITH_KNOTS ( ( 2, 2 ),
 ( 3, 2, 2, 2, 2, 2, 2, 2, 2, 2, 2, 2, 2, 2, 2, 2, 2, 2, 2, 2, 2, 2, 2, 2, 2, 2, 2, 2, 2, 2, 2, 2, 2, 2, 2, 2, 2, 2, 2, 2, 2, 2, 2, 2, 2, 2, 2, 2, 2, 2, 2, 2, 2, 2, 2, 2, 2, 2, 2, 2, 2, 2, 2, 2, 2, 2, 2, 2, 2, 2, 2, 2, 2, 2, 2, 2, 2, 2, 2, 2, 2, 2, 2, 2, 2, 2, 2, 2, 2, 2, 2, 2, 2, 2, 2, 2, 2, 2, 2, 2, 2, 2, 2, 2, 2, 2, 2, 2, 2, 2, 2, 2, 2, 2, 2, 2, 2, 2, 2, 2, 2, 2, 2, 2, 2, 2, 2, 2, 2, 2, 2, 2, 2, 2, 2, 2, 2, 2, 2, 2, 2, 2, 2, 2, 2, 2, 2, 2, 2, 2, 2, 2, 2, 2, 2, 2, 2, 2, 2, 2, 2, 2, 2, 2, 2, 2, 2, 2, 2, 2, 2, 2, 2, 2, 2, 2, 2, 2, 2, 2, 2, 2, 2, 2, 2, 2, 2, 2, 2, 2, 2, 2, 2, 2, 2, 2, 2, 2, 2, 2, 2, 2, 2, 2, 2, 2, 2, 2, 2, 2, 2, 2, 2, 2, 2, 2, 2, 2, 2, 2, 2, 2, 2, 2, 2, 2, 2, 2, 2, 2, 2, 2, 2, 2, 2, 2, 2, 2, 2, 2, 2, 2, 2, 2, 2, 2, 2, 2, 2, 2, 2, 2, 2, 2, 2, 3 ),
 ( 0.000000000000000000, 1.000000000000000000 ),
 ( 0.000000000000000000, 0.003787878787878787984, 0.007575757575757575968, 0.01136363636363636395, 0.01515151515151515194, 0.01893939393939393992, 0.02272727272727272790, 0.02651515151515151589, 0.03030303030303030387, 0.03409090909090908839, 0.03787878787878787984, 0.04166666666666666435, 0.04545454545454545581, 0.04924242424242424032, 0.05303030303030303177, 0.05681818181818181629, 0.06060606060606060774, 0.06439393939393939226, 0.06818181818181817677, 0.07196969696969697516, 0.07575757575757575968, 0.07954545454545454419, 0.08333333333333332871, 0.08712121212121212710, 0.09090909090909091161, 0.09469696969696969613, 0.09848484848484848064, 0.1022727272727272790, 0.1060606060606060635, 0.1098484848484848481, 0.1136363636363636326, 0.1174242424242424310, 0.1212121212121212155, 0.1250000000000000000, 0.1287878787878787845, 0.1325757575757575690, 0.1363636363636363535, 0.1401515151515151381, 0.1439393939393939503, 0.1477272727272727348, 0.1515151515151515194, 0.1553030303030303039, 0.1590909090909090884, 0.1628787878787878729, 0.1666666666666666574, 0.1704545454545454419, 0.1742424242424242542, 0.1780303030303030387, 0.1818181818181818232, 0.1856060606060606077, 0.1893939393939393923, 0.1931818181818181768, 0.1969696969696969613, 0.2007575757575757458, 0.2045454545454545581, 0.2083333333333333426, 0.2121212121212121271, 0.2159090909090909116, 0.2196969696969696961, 0.2234848484848484806, 0.2272727272727272652, 0.2310606060606060497, 0.2348484848484848619, 0.2386363636363636465, 0.2424242424242424310, 0.2462121212121212155, 0.2500000000000000000, 0.2537878787878787845, 0.2575757575757575690, 0.2613636363636363535, 0.2651515151515151381, 0.2689393939393939226, 0.2727272727272727071, 0.2765151515151514916, 0.2803030303030302761, 0.2840909090909091161, 0.2878787878787879007, 0.2916666666666666852, 0.2954545454545454697, 0.2992424242424242542, 0.3030303030303030387, 0.3068181818181818232, 0.3106060606060606077, 0.3143939393939393923, 0.3181818181818181768, 0.3219696969696969613, 0.3257575757575757458, 0.3295454545454545303, 0.3333333333333333148, 0.3371212121212120993, 0.3409090909090908839, 0.3446969696969697239, 0.3484848484848485084, 0.3522727272727272929, 0.3560606060606060774, 0.3598484848484848619, 0.3636363636363636465, 0.3674242424242424310, 0.3712121212121212155, 0.3750000000000000000, 0.3787878787878787845, 0.3825757575757575690, 0.3863636363636363535, 0.3901515151515151381, 0.3939393939393939226, 0.3977272727272727071, 0.4015151515151514916, 0.4053030303030302761, 0.4090909090909091161, 0.4128787878787879007, 0.4166666666666666852, 0.4204545454545454697, 0.4242424242424242542, 0.4280303030303030387, 0.4318181818181818232, 0.4356060606060606077, 0.4393939393939393923, 0.4431818181818181768, 0.4469696969696969613, 0.4507575757575757458, 0.4545454545454545303, 0.4583333333333333148, 0.4621212121212120993, 0.4659090909090908839, 0.4696969696969697239, 0.4734848484848485084, 0.4772727272727272929, 0.4810606060606060774, 0.4848484848484848619, 0.4886363636363636465, 0.4924242424242424310, 0.4962121212121212155, 0.5000000000000000000, 0.5037878787878787845, 0.5075757575757575690, 0.5113636363636363535, 0.5151515151515151381, 0.5189393939393939226, 0.5227272727272727071, 0.5265151515151514916, 0.5303030303030302761, 0.5340909090909090606, 0.5378787878787878451, 0.5416666666666666297, 0.5454545454545454142, 0.5492424242424241987, 0.5530303030303029832, 0.5568181818181817677, 0.5606060606060605522, 0.5643939393939394478, 0.5681818181818182323, 0.5719696969696970168, 0.5757575757575758013, 0.5795454545454545858, 0.5833333333333333703, 0.5871212121212121549, 0.5909090909090909394, 0.5946969696969697239, 0.5984848484848485084, 0.6022727272727272929, 0.6060606060606060774, 0.6098484848484848619, 0.6136363636363636465, 0.6174242424242424310, 0.6212121212121212155, 0.6250000000000000000, 0.6287878787878787845, 0.6325757575757575690, 0.6363636363636363535, 0.6401515151515151381, 0.6439393939393939226, 0.6477272727272727071, 0.6515151515151514916, 0.6553030303030302761, 0.6590909090909090606, 0.6628787878787878451, 0.6666666666666666297, 0.6704545454545454142, 0.6742424242424241987, 0.6780303030303029832, 0.6818181818181817677, 0.6856060606060605522, 0.6893939393939394478, 0.6931818181818182323, 0.6969696969696970168, 0.7007575757575758013, 0.7045454545454545858, 0.7083333333333333703, 0.7121212121212121549, 0.7159090909090909394, 0.7196969696969697239, 0.7234848484848485084, 0.7272727272727272929, 0.7310606060606060774, 0.7348484848484848619, 0.7386363636363636465, 0.7424242424242424310, 0.7462121212121212155, 0.7500000000000000000, 0.7537878787878787845, 0.7575757575757575690, 0.7613636363636363535, 0.7651515151515151381, 0.7689393939393939226, 0.7727272727272727071, 0.7765151515151514916, 0.7803030303030302761, 0.7840909090909090606, 0.7878787878787878451, 0.7916666666666666297, 0.7954545454545454142, 0.7992424242424241987, 0.8030303030303029832, 0.8068181818181817677, 0.8106060606060605522, 0.8143939393939394478, 0.8181818181818182323, 0.8219696969696970168, 0.8257575757575758013, 0.8295454545454545858, 0.8333333333333333703, 0.8371212121212121549, 0.8409090909090909394, 0.8446969696969697239, 0.8484848484848485084, 0.8522727272727272929, 0.8560606060606060774, 0.8598484848484848619, 0.8636363636363636465, 0.8674242424242424310, 0.8712121212121212155, 0.8750000000000000000, 0.8787878787878787845, 0.8825757575757575690, 0.8863636363636363535, 0.8901515151515151381, 0.8939393939393939226, 0.8977272727272727071, 0.9015151515151514916, 0.9053030303030302761, 0.9090909090909090606, 0.9128787878787878451, 0.9166666666666666297, 0.9204545454545454142, 0.9242424242424241987, 0.9280303030303029832, 0.9318181818181817677, 0.9356060606060605522, 0.9393939393939394478, 0.9431818181818182323, 0.9469696969696970168, 0.9507575757575758013, 0.9545454545454545858, 0.9583333333333333703, 0.9621212121212121549, 0.9659090909090909394 ),
 .UNSPECIFIED. ) 
 GEOMETRIC_REPRESENTATION_ITEM ( )  RATIONAL_B_SPLINE_SURFACE ( (
 ( 1.000000000000000000, 0.9659258262890683122, 1.000000000000000000, 0.9659258262890683122, 1.000000000000000000, 0.9659258262890683122, 1.000000000000000000, 0.9659258262890683122, 1.000000000000000000, 0.9659258262890683122, 1.000000000000000000, 0.9659258262890683122, 1.000000000000000000, 0.9659258262890683122, 1.000000000000000000, 0.9659258262890683122, 1.000000000000000000, 0.9659258262890683122, 1.000000000000000000, 0.9659258262890683122, 1.000000000000000000, 0.9659258262890683122, 1.000000000000000000, 0.9659258262890683122, 1.000000000000000000, 0.9659258262890683122, 1.000000000000000000, 0.9659258262890683122, 1.000000000000000000, 0.9659258262890683122, 1.000000000000000000, 0.9659258262890683122, 1.000000000000000000, 0.9659258262890683122, 1.000000000000000000, 0.9659258262890683122, 1.000000000000000000, 0.9659258262890683122, 1.000000000000000000, 0.9659258262890683122, 1.000000000000000000, 0.9659258262890683122, 1.000000000000000000, 0.9659258262890683122, 1.000000000000000000, 0.9659258262890683122, 1.000000000000000000, 0.9659258262890683122, 1.000000000000000000, 0.9659258262890683122, 1.000000000000000000, 0.9659258262890683122, 1.000000000000000000, 0.9659258262890683122, 1.000000000000000000, 0.9659258262890683122, 1.000000000000000000, 0.9659258262890683122, 1.000000000000000000, 0.9659258262890683122, 1.000000000000000000, 0.9659258262890683122, 1.000000000000000000, 0.9659258262890683122, 1.000000000000000000, 0.9659258262890683122, 1.000000000000000000, 0.9659258262890683122, 1.000000000000000000, 0.9659258262890683122, 1.000000000000000000, 0.9659258262890683122, 1.000000000000000000, 0.9659258262890683122, 1.000000000000000000, 0.9659258262890683122, 1.000000000000000000, 0.9659258262890683122, 1.000000000000000000, 0.9659258262890683122, 1.000000000000000000, 0.9659258262890683122, 1.000000000000000000, 0.9659258262890683122, 1.000000000000000000, 0.9659258262890683122, 1.000000000000000000, 0.9659258262890683122, 1.000000000000000000, 0.9659258262890683122, 1.000000000000000000, 0.9659258262890683122, 1.000000000000000000, 0.9659258262890683122, 1.000000000000000000, 0.9659258262890683122, 1.000000000000000000, 0.9659258262890683122, 1.000000000000000000, 0.9659258262890683122, 1.000000000000000000, 0.9659258262890683122, 1.000000000000000000, 0.9659258262890683122, 1.000000000000000000, 0.9659258262890683122, 1.000000000000000000, 0.9659258262890683122, 1.000000000000000000, 0.9659258262890683122, 1.000000000000000000, 0.9659258262890683122, 1.000000000000000000, 0.9659258262890683122, 1.000000000000000000, 0.9659258262890683122, 1.000000000000000000, 0.9659258262890683122, 1.000000000000000000, 0.9659258262890683122, 1.000000000000000000, 0.9659258262890683122, 1.000000000000000000, 0.9659258262890683122, 1.000000000000000000, 0.9659258262890683122, 1.000000000000000000, 0.9659258262890683122, 1.000000000000000000, 0.9659258262890683122, 1.000000000000000000, 0.9659258262890683122, 1.000000000000000000, 0.9659258262890683122, 1.000000000000000000, 0.9659258262890683122, 1.000000000000000000, 0.9659258262890683122, 1.000000000000000000, 0.9659258262890683122, 1.000000000000000000, 0.9659258262890683122, 1.000000000000000000, 0.9659258262890683122, 1.000000000000000000, 0.9659258262890683122, 1.000000000000000000, 0.9659258262890683122, 1.000000000000000000, 0.9659258262890683122, 1.000000000000000000, 0.9659258262890683122, 1.000000000000000000, 0.9659258262890683122, 1.000000000000000000, 0.9659258262890683122, 1.000000000000000000, 0.9659258262890683122, 1.000000000000000000, 0.9659258262890683122, 1.000000000000000000, 0.9659258262890683122, 1.000000000000000000, 0.9659258262890683122, 1.000000000000000000, 0.9659258262890683122, 1.000000000000000000, 0.9659258262890683122, 1.000000000000000000, 0.9659258262890683122, 1.000000000000000000, 0.9659258262890683122, 1.000000000000000000, 0.9659258262890683122, 1.000000000000000000, 0.9659258262890683122, 1.000000000000000000, 0.9659258262890683122, 1.000000000000000000, 0.9659258262890683122, 1.000000000000000000, 0.9659258262890683122, 1.000000000000000000, 0.9659258262890683122, 1.000000000000000000, 0.9659258262890683122, 1.000000000000000000, 0.9659258262890683122, 1.000000000000000000, 0.9659258262890683122, 1.000000000000000000, 0.9659258262890683122, 1.000000000000000000, 0.9659258262890683122, 1.000000000000000000, 0.9659258262890683122, 1.000000000000000000, 0.9659258262890683122, 1.000000000000000000, 0.9659258262890683122, 1.000000000000000000, 0.9659258262890683122, 1.000000000000000000, 0.9659258262890683122, 1.000000000000000000, 0.9659258262890683122, 1.000000000000000000, 0.9659258262890683122, 1.000000000000000000, 0.9659258262890683122, 1.000000000000000000, 0.9659258262890683122, 1.000000000000000000, 0.9659258262890683122, 1.000000000000000000, 0.9659258262890683122, 1.000000000000000000, 0.9659258262890683122, 1.000000000000000000, 0.9659258262890683122, 1.000000000000000000, 0.9659258262890683122, 1.000000000000000000, 0.9659258262890683122, 1.000000000000000000, 0.9659258262890683122, 1.000000000000000000, 0.9659258262890683122, 1.000000000000000000, 0.9659258262890683122, 1.000000000000000000, 0.9659258262890683122, 1.000000000000000000, 0.9659258262890683122, 1.000000000000000000, 0.9659258262890683122, 1.000000000000000000, 0.9659258262890683122, 1.000000000000000000, 0.9659258262890683122, 1.000000000000000000, 0.9659258262890683122, 1.000000000000000000, 0.9659258262890683122, 1.000000000000000000, 0.9659258262890683122, 1.000000000000000000, 0.9659258262890683122, 1.000000000000000000, 0.9659258262890683122, 1.000000000000000000, 0.9659258262890683122, 1.000000000000000000, 0.9659258262890683122, 1.000000000000000000, 0.9659258262890683122, 1.000000000000000000, 0.9659258262890683122, 1.000000000000000000, 0.9659258262890683122, 1.000000000000000000, 0.9659258262890683122, 1.000000000000000000, 0.9659258262890683122, 1.000000000000000000, 0.9659258262890683122, 1.000000000000000000, 0.9659258262890683122, 1.000000000000000000, 0.9659258262890683122, 1.000000000000000000, 0.9659258262890683122, 1.000000000000000000, 0.9659258262890683122, 1.000000000000000000, 0.9659258262890683122, 1.000000000000000000, 0.9659258262890683122, 1.000000000000000000, 0.9659258262890683122, 1.000000000000000000, 0.9659258262890683122, 1.000000000000000000, 0.9659258262890683122, 1.000000000000000000, 0.9659258262890683122, 1.000000000000000000, 0.9659258262890683122, 1.000000000000000000, 0.9659258262890683122, 1.000000000000000000, 0.9659258262890683122, 1.000000000000000000, 0.9659258262890683122, 1.000000000000000000, 0.9659258262890683122, 1.000000000000000000, 0.9659258262890683122, 1.000000000000000000, 0.9659258262890683122, 1.000000000000000000, 0.9659258262890683122, 1.000000000000000000, 0.9659258262890683122, 1.000000000000000000, 0.9659258262890683122, 1.000000000000000000, 0.9659258262890683122, 1.000000000000000000, 0.9659258262890683122, 1.000000000000000000, 0.9659258262890683122, 1.000000000000000000, 0.9659258262890683122, 1.000000000000000000, 0.9659258262890683122, 1.000000000000000000, 0.9659258262890683122, 1.000000000000000000, 0.9659258262890683122, 1.000000000000000000, 0.9659258262890683122, 1.000000000000000000, 0.9659258262890683122, 1.000000000000000000, 0.9659258262890683122, 1.000000000000000000, 0.9659258262890683122, 1.000000000000000000, 0.9659258262890683122, 1.000000000000000000, 0.9659258262890683122, 1.000000000000000000, 0.9659258262890683122, 1.000000000000000000, 0.9659258262890683122, 1.000000000000000000, 0.9659258262890683122, 1.000000000000000000, 0.9659258262890683122, 1.000000000000000000, 0.9659258262890683122, 1.000000000000000000, 0.9659258262890683122, 1.000000000000000000, 0.9659258262890683122, 1.000000000000000000, 0.9659258262890683122, 1.000000000000000000, 0.9659258262890683122, 1.000000000000000000, 0.9659258262890683122, 1.000000000000000000, 0.9659258262890683122, 1.000000000000000000, 0.9659258262890683122, 1.000000000000000000, 0.9659258262890683122, 1.000000000000000000, 0.9659258262890683122, 1.000000000000000000, 0.9659258262890683122, 1.000000000000000000, 0.9659258262890683122, 1.000000000000000000, 0.9659258262890683122, 1.000000000000000000, 0.9659258262890683122, 1.000000000000000000, 0.9659258262890683122, 1.000000000000000000, 0.9659258262890683122, 1.000000000000000000, 0.9659258262890683122, 1.000000000000000000, 0.9659258262890683122, 1.000000000000000000, 0.9659258262890683122, 1.000000000000000000, 0.9659258262890683122, 1.000000000000000000, 0.9659258262890683122, 1.000000000000000000, 0.9659258262890683122, 1.000000000000000000, 0.9659258262890683122, 1.000000000000000000, 0.9659258262890683122, 1.000000000000000000, 0.9659258262890683122, 1.000000000000000000, 0.9659258262890683122, 1.000000000000000000, 0.9659258262890683122, 1.000000000000000000, 0.9659258262890683122, 1.000000000000000000, 0.9659258262890683122, 1.000000000000000000, 0.9659258262890683122, 1.000000000000000000, 0.9659258262890683122, 1.000000000000000000, 0.9659258262890683122, 1.000000000000000000, 0.9659258262890683122, 1.000000000000000000, 0.9659258262890683122, 1.000000000000000000, 0.9659258262890683122, 1.000000000000000000, 0.9659258262890683122, 1.000000000000000000, 0.9659258262890683122, 1.000000000000000000, 0.9659258262890683122, 1.000000000000000000, 0.9659258262890683122, 1.000000000000000000, 0.9659258262890683122, 1.000000000000000000, 0.9659258262890683122, 1.000000000000000000, 0.9659258262890683122, 1.000000000000000000, 0.9659258262890683122, 1.000000000000000000, 0.9659258262890683122, 1.000000000000000000, 0.9659258262890683122, 1.000000000000000000, 0.9659258262890683122, 1.000000000000000000, 0.9659258262890683122, 1.000000000000000000, 0.9659258262890683122, 1.000000000000000000, 0.9659258262890683122, 1.000000000000000000, 0.9659258262890683122, 1.000000000000000000, 0.9659258262890683122, 1.000000000000000000, 0.9659258262890683122, 1.000000000000000000, 0.9659258262890683122, 1.000000000000000000, 0.9659258262890683122, 1.000000000000000000, 0.9659258262890683122, 1.000000000000000000, 0.9659258262890683122, 1.000000000000000000, 0.9659258262890683122, 1.000000000000000000, 0.9659258262890683122, 1.000000000000000000, 0.9659258262890683122, 1.000000000000000000, 0.9659258262890683122, 1.000000000000000000, 0.9659258262890683122, 1.000000000000000000, 0.9659258262890683122, 1.000000000000000000, 0.9659258262890683122, 1.000000000000000000, 0.9659258262890683122, 1.000000000000000000, 0.9659258262890683122, 1.000000000000000000, 0.9659258262890683122, 1.000000000000000000, 0.9659258262890683122, 1.000000000000000000, 0.9659258262890683122, 1.000000000000000000, 0.9659258262890683122, 1.000000000000000000, 0.9659258262890683122, 1.000000000000000000, 0.9659258262890683122, 1.000000000000000000, 0.9659258262890683122, 1.000000000000000000, 0.9659258262890683122, 1.000000000000000000, 0.9659258262890683122, 1.000000000000000000, 0.9659258262890683122, 1.000000000000000000, 0.9659258262890683122, 1.000000000000000000, 0.9659258262890683122, 1.000000000000000000, 0.9659258262890683122, 1.000000000000000000, 0.9659258262890683122, 1.000000000000000000, 0.9659258262890683122, 1.000000000000000000, 0.9659258262890683122, 1.000000000000000000, 0.9659258262890683122, 1.000000000000000000, 0.9659258262890683122, 1.000000000000000000, 0.9659258262890683122, 1.000000000000000000, 0.9659258262890683122, 1.000000000000000000),
 ( 1.000000000000000000, 0.9659258262890683122, 1.000000000000000000, 0.9659258262890683122, 1.000000000000000000, 0.9659258262890683122, 1.000000000000000000, 0.9659258262890683122, 1.000000000000000000, 0.9659258262890683122, 1.000000000000000000, 0.9659258262890683122, 1.000000000000000000, 0.9659258262890683122, 1.000000000000000000, 0.9659258262890683122, 1.000000000000000000, 0.9659258262890683122, 1.000000000000000000, 0.9659258262890683122, 1.000000000000000000, 0.9659258262890683122, 1.000000000000000000, 0.9659258262890683122, 1.000000000000000000, 0.9659258262890683122, 1.000000000000000000, 0.9659258262890683122, 1.000000000000000000, 0.9659258262890683122, 1.000000000000000000, 0.9659258262890683122, 1.000000000000000000, 0.9659258262890683122, 1.000000000000000000, 0.9659258262890683122, 1.000000000000000000, 0.9659258262890683122, 1.000000000000000000, 0.9659258262890683122, 1.000000000000000000, 0.9659258262890683122, 1.000000000000000000, 0.9659258262890683122, 1.000000000000000000, 0.9659258262890683122, 1.000000000000000000, 0.9659258262890683122, 1.000000000000000000, 0.9659258262890683122, 1.000000000000000000, 0.9659258262890683122, 1.000000000000000000, 0.9659258262890683122, 1.000000000000000000, 0.9659258262890683122, 1.000000000000000000, 0.9659258262890683122, 1.000000000000000000, 0.9659258262890683122, 1.000000000000000000, 0.9659258262890683122, 1.000000000000000000, 0.9659258262890683122, 1.000000000000000000, 0.9659258262890683122, 1.000000000000000000, 0.9659258262890683122, 1.000000000000000000, 0.9659258262890683122, 1.000000000000000000, 0.9659258262890683122, 1.000000000000000000, 0.9659258262890683122, 1.000000000000000000, 0.9659258262890683122, 1.000000000000000000, 0.9659258262890683122, 1.000000000000000000, 0.9659258262890683122, 1.000000000000000000, 0.9659258262890683122, 1.000000000000000000, 0.9659258262890683122, 1.000000000000000000, 0.9659258262890683122, 1.000000000000000000, 0.9659258262890683122, 1.000000000000000000, 0.9659258262890683122, 1.000000000000000000, 0.9659258262890683122, 1.000000000000000000, 0.9659258262890683122, 1.000000000000000000, 0.9659258262890683122, 1.000000000000000000, 0.9659258262890683122, 1.000000000000000000, 0.9659258262890683122, 1.000000000000000000, 0.9659258262890683122, 1.000000000000000000, 0.9659258262890683122, 1.000000000000000000, 0.9659258262890683122, 1.000000000000000000, 0.9659258262890683122, 1.000000000000000000, 0.9659258262890683122, 1.000000000000000000, 0.9659258262890683122, 1.000000000000000000, 0.9659258262890683122, 1.000000000000000000, 0.9659258262890683122, 1.000000000000000000, 0.9659258262890683122, 1.000000000000000000, 0.9659258262890683122, 1.000000000000000000, 0.9659258262890683122, 1.000000000000000000, 0.9659258262890683122, 1.000000000000000000, 0.9659258262890683122, 1.000000000000000000, 0.9659258262890683122, 1.000000000000000000, 0.9659258262890683122, 1.000000000000000000, 0.9659258262890683122, 1.000000000000000000, 0.9659258262890683122, 1.000000000000000000, 0.9659258262890683122, 1.000000000000000000, 0.9659258262890683122, 1.000000000000000000, 0.9659258262890683122, 1.000000000000000000, 0.9659258262890683122, 1.000000000000000000, 0.9659258262890683122, 1.000000000000000000, 0.9659258262890683122, 1.000000000000000000, 0.9659258262890683122, 1.000000000000000000, 0.9659258262890683122, 1.000000000000000000, 0.9659258262890683122, 1.000000000000000000, 0.9659258262890683122, 1.000000000000000000, 0.9659258262890683122, 1.000000000000000000, 0.9659258262890683122, 1.000000000000000000, 0.9659258262890683122, 1.000000000000000000, 0.9659258262890683122, 1.000000000000000000, 0.9659258262890683122, 1.000000000000000000, 0.9659258262890683122, 1.000000000000000000, 0.9659258262890683122, 1.000000000000000000, 0.9659258262890683122, 1.000000000000000000, 0.9659258262890683122, 1.000000000000000000, 0.9659258262890683122, 1.000000000000000000, 0.9659258262890683122, 1.000000000000000000, 0.9659258262890683122, 1.000000000000000000, 0.9659258262890683122, 1.000000000000000000, 0.9659258262890683122, 1.000000000000000000, 0.9659258262890683122, 1.000000000000000000, 0.9659258262890683122, 1.000000000000000000, 0.9659258262890683122, 1.000000000000000000, 0.9659258262890683122, 1.000000000000000000, 0.9659258262890683122, 1.000000000000000000, 0.9659258262890683122, 1.000000000000000000, 0.9659258262890683122, 1.000000000000000000, 0.9659258262890683122, 1.000000000000000000, 0.9659258262890683122, 1.000000000000000000, 0.9659258262890683122, 1.000000000000000000, 0.9659258262890683122, 1.000000000000000000, 0.9659258262890683122, 1.000000000000000000, 0.9659258262890683122, 1.000000000000000000, 0.9659258262890683122, 1.000000000000000000, 0.9659258262890683122, 1.000000000000000000, 0.9659258262890683122, 1.000000000000000000, 0.9659258262890683122, 1.000000000000000000, 0.9659258262890683122, 1.000000000000000000, 0.9659258262890683122, 1.000000000000000000, 0.9659258262890683122, 1.000000000000000000, 0.9659258262890683122, 1.000000000000000000, 0.9659258262890683122, 1.000000000000000000, 0.9659258262890683122, 1.000000000000000000, 0.9659258262890683122, 1.000000000000000000, 0.9659258262890683122, 1.000000000000000000, 0.9659258262890683122, 1.000000000000000000, 0.9659258262890683122, 1.000000000000000000, 0.9659258262890683122, 1.000000000000000000, 0.9659258262890683122, 1.000000000000000000, 0.9659258262890683122, 1.000000000000000000, 0.9659258262890683122, 1.000000000000000000, 0.9659258262890683122, 1.000000000000000000, 0.9659258262890683122, 1.000000000000000000, 0.9659258262890683122, 1.000000000000000000, 0.9659258262890683122, 1.000000000000000000, 0.9659258262890683122, 1.000000000000000000, 0.9659258262890683122, 1.000000000000000000, 0.9659258262890683122, 1.000000000000000000, 0.9659258262890683122, 1.000000000000000000, 0.9659258262890683122, 1.000000000000000000, 0.9659258262890683122, 1.000000000000000000, 0.9659258262890683122, 1.000000000000000000, 0.9659258262890683122, 1.000000000000000000, 0.9659258262890683122, 1.000000000000000000, 0.9659258262890683122, 1.000000000000000000, 0.9659258262890683122, 1.000000000000000000, 0.9659258262890683122, 1.000000000000000000, 0.9659258262890683122, 1.000000000000000000, 0.9659258262890683122, 1.000000000000000000, 0.9659258262890683122, 1.000000000000000000, 0.9659258262890683122, 1.000000000000000000, 0.9659258262890683122, 1.000000000000000000, 0.9659258262890683122, 1.000000000000000000, 0.9659258262890683122, 1.000000000000000000, 0.9659258262890683122, 1.000000000000000000, 0.9659258262890683122, 1.000000000000000000, 0.9659258262890683122, 1.000000000000000000, 0.9659258262890683122, 1.000000000000000000, 0.9659258262890683122, 1.000000000000000000, 0.9659258262890683122, 1.000000000000000000, 0.9659258262890683122, 1.000000000000000000, 0.9659258262890683122, 1.000000000000000000, 0.9659258262890683122, 1.000000000000000000, 0.9659258262890683122, 1.000000000000000000, 0.9659258262890683122, 1.000000000000000000, 0.9659258262890683122, 1.000000000000000000, 0.9659258262890683122, 1.000000000000000000, 0.9659258262890683122, 1.000000000000000000, 0.9659258262890683122, 1.000000000000000000, 0.9659258262890683122, 1.000000000000000000, 0.9659258262890683122, 1.000000000000000000, 0.9659258262890683122, 1.000000000000000000, 0.9659258262890683122, 1.000000000000000000, 0.9659258262890683122, 1.000000000000000000, 0.9659258262890683122, 1.000000000000000000, 0.9659258262890683122, 1.000000000000000000, 0.9659258262890683122, 1.000000000000000000, 0.9659258262890683122, 1.000000000000000000, 0.9659258262890683122, 1.000000000000000000, 0.9659258262890683122, 1.000000000000000000, 0.9659258262890683122, 1.000000000000000000, 0.9659258262890683122, 1.000000000000000000, 0.9659258262890683122, 1.000000000000000000, 0.9659258262890683122, 1.000000000000000000, 0.9659258262890683122, 1.000000000000000000, 0.9659258262890683122, 1.000000000000000000, 0.9659258262890683122, 1.000000000000000000, 0.9659258262890683122, 1.000000000000000000, 0.9659258262890683122, 1.000000000000000000, 0.9659258262890683122, 1.000000000000000000, 0.9659258262890683122, 1.000000000000000000, 0.9659258262890683122, 1.000000000000000000, 0.9659258262890683122, 1.000000000000000000, 0.9659258262890683122, 1.000000000000000000, 0.9659258262890683122, 1.000000000000000000, 0.9659258262890683122, 1.000000000000000000, 0.9659258262890683122, 1.000000000000000000, 0.9659258262890683122, 1.000000000000000000, 0.9659258262890683122, 1.000000000000000000, 0.9659258262890683122, 1.000000000000000000, 0.9659258262890683122, 1.000000000000000000, 0.9659258262890683122, 1.000000000000000000, 0.9659258262890683122, 1.000000000000000000, 0.9659258262890683122, 1.000000000000000000, 0.9659258262890683122, 1.000000000000000000, 0.9659258262890683122, 1.000000000000000000, 0.9659258262890683122, 1.000000000000000000, 0.9659258262890683122, 1.000000000000000000, 0.9659258262890683122, 1.000000000000000000, 0.9659258262890683122, 1.000000000000000000, 0.9659258262890683122, 1.000000000000000000, 0.9659258262890683122, 1.000000000000000000, 0.9659258262890683122, 1.000000000000000000, 0.9659258262890683122, 1.000000000000000000, 0.9659258262890683122, 1.000000000000000000, 0.9659258262890683122, 1.000000000000000000, 0.9659258262890683122, 1.000000000000000000, 0.9659258262890683122, 1.000000000000000000, 0.9659258262890683122, 1.000000000000000000, 0.9659258262890683122, 1.000000000000000000, 0.9659258262890683122, 1.000000000000000000, 0.9659258262890683122, 1.000000000000000000, 0.9659258262890683122, 1.000000000000000000, 0.9659258262890683122, 1.000000000000000000, 0.9659258262890683122, 1.000000000000000000, 0.9659258262890683122, 1.000000000000000000, 0.9659258262890683122, 1.000000000000000000, 0.9659258262890683122, 1.000000000000000000, 0.9659258262890683122, 1.000000000000000000, 0.9659258262890683122, 1.000000000000000000, 0.9659258262890683122, 1.000000000000000000, 0.9659258262890683122, 1.000000000000000000, 0.9659258262890683122, 1.000000000000000000, 0.9659258262890683122, 1.000000000000000000, 0.9659258262890683122, 1.000000000000000000, 0.9659258262890683122, 1.000000000000000000, 0.9659258262890683122, 1.000000000000000000, 0.9659258262890683122, 1.000000000000000000, 0.9659258262890683122, 1.000000000000000000, 0.9659258262890683122, 1.000000000000000000, 0.9659258262890683122, 1.000000000000000000, 0.9659258262890683122, 1.000000000000000000, 0.9659258262890683122, 1.000000000000000000, 0.9659258262890683122, 1.000000000000000000, 0.9659258262890683122, 1.000000000000000000, 0.9659258262890683122, 1.000000000000000000, 0.9659258262890683122, 1.000000000000000000, 0.9659258262890683122, 1.000000000000000000, 0.9659258262890683122, 1.000000000000000000, 0.9659258262890683122, 1.000000000000000000, 0.9659258262890683122, 1.000000000000000000, 0.9659258262890683122, 1.000000000000000000, 0.9659258262890683122, 1.000000000000000000, 0.9659258262890683122, 1.000000000000000000, 0.9659258262890683122, 1.000000000000000000, 0.9659258262890683122, 1.000000000000000000, 0.9659258262890683122, 1.000000000000000000, 0.9659258262890683122, 1.000000000000000000, 0.9659258262890683122, 1.000000000000000000, 0.9659258262890683122, 1.000000000000000000, 0.9659258262890683122, 1.000000000000000000, 0.9659258262890683122, 1.000000000000000000, 0.9659258262890683122, 1.000000000000000000, 0.9659258262890683122, 1.000000000000000000) ) ) 
 REPRESENTATION_ITEM ( '' )  SURFACE ( )  );
#27529=CARTESIAN_POINT ( 'NONE',  ( 1.043307086614173818, 0.1660481256975885056, 0.3530559997133364547 ) ) ;
#27530=CARTESIAN_POINT ( 'NONE',  ( 0.7677165354330716118, -0.4536011799217367080, 0.2665933059059888421 ) ) ;
#27535=CARTESIAN_POINT ( 'NONE',  ( 1.450131233595801428, 0.2952755905511811885, 0.1292274648535926551 ) ) ;
#27537=CARTESIAN_POINT ( 'NONE',  ( -0.3543307086614165824, -0.6692913385826771977, 8.415575281601705876E-17 ) ) ;
#27538=CARTESIAN_POINT ( 'NONE',  ( 1.167979002624672580, 0.05413385826771626580, -0.4176697321401330321 ) ) ;
#27540=CARTESIAN_POINT ( 'NONE',  ( -1.555118110236219930, 0.1660481256975885056, 0.3530559997133364547 ) ) ;
#27543=FACE_OUTER_BOUND ( 'NONE', #39763, .T. ) ;
#27545=CARTESIAN_POINT ( 'NONE',  ( -0.7217847769028863381, -0.3690944881889763329, 0.3153832671262228327 ) ) ;
#27546=CARTESIAN_POINT ( 'NONE',  ( -1.601049868766403650, 0.2306618581243847221, -0.2411417322834647770 ) ) ;
#27547=CARTESIAN_POINT ( 'NONE',  ( 0.6627296587926517768, -0.6692913385826773087, -0.1292274648535924053 ) ) ;
#27548=ORIENTED_EDGE ( 'NONE', *, *, #68575, .F. ) ;
#27549=CARTESIAN_POINT ( 'NONE',  ( 1.463254593175853824, -0.6692913385826771977, 0.1292274648535927661 ) ) ;
#27551=CARTESIAN_POINT ( 'NONE',  ( -0.6102362204724400829, 0.07958543189024085140, 0.2665933059059887866 ) ) ;
#27552=CARTESIAN_POINT ( 'NONE',  ( 0.8202099737532814183, -0.6692913385826773087, -0.1292274648535924053 ) ) ;
#27553=CARTESIAN_POINT ( 'NONE',  ( -1.706036745406823485, 0.2306618581243848609, 0.2411417322834645549 ) ) ;
#27555=CARTESIAN_POINT ( 'NONE',  ( -0.6496062992125976043, -0.4536011799217367080, 0.2665933059059888421 ) ) ;
#27556=CARTESIAN_POINT ( 'NONE',  ( -1.633858267716534529, 0.07958543189024085140, 0.2665933059059887866 ) ) ;
#27559=CARTESIAN_POINT ( 'NONE',  ( 0.3805774278215230400, 0.05413385826771626580, -0.4176697321401330321 ) ) ;
#27560=CARTESIAN_POINT ( 'NONE',  ( -0.8661417322834640276, -0.1870078740157479769, 0.3641732283464567677 ) ) ;
#27561=CARTESIAN_POINT ( 'NONE',  ( -0.4986876640419942164, -0.5023911411419708095, 0.1820866141732285504 ) ) ;
#27562=CARTESIAN_POINT ( 'NONE',  ( -0.1706036745406816491, -0.4281496062992124485, 0.4176697321401328655 ) ) ;
#27563=CARTESIAN_POINT ( 'NONE',  ( -0.9645669291338575535, 0.07958543189024071263, -0.2665933059059888421 ) ) ;
#27565=CARTESIAN_POINT ( 'NONE',  ( 0.5905511811023629321, -0.6692913385826771977, 8.415575281601705876E-17 ) ) ;
#27568=CARTESIAN_POINT ( 'NONE',  ( -0.9645669291338575535, -0.5400638737290844871, 0.3530559997133364547 ) ) ;
#27569=CARTESIAN_POINT ( 'NONE',  ( -0.09842519685039295696, 0.07958543189024071263, -0.2665933059059888421 ) ) ;
#27570=EDGE_CURVE ( 'NONE', #30126, #69738, #68124, .T. ) ;
#27571=CARTESIAN_POINT ( 'NONE',  ( -1.259842519685038686, -0.1870078740157480879, -0.4822834645669291653 ) ) ;
#27572=CARTESIAN_POINT ( 'NONE',  ( 0.6561679790026253567, -0.5023911411419708095, -0.1820866141732282451 ) ) ;
#27574=CARTESIAN_POINT ( 'NONE',  ( -0.6824146981627291497, -0.5023911411419708095, -0.1820866141732282451 ) ) ;
#27575=CARTESIAN_POINT ( 'NONE',  ( -0.9580052493438311334, -0.4281496062992124485, 0.4176697321401328655 ) ) ;
#27576=CARTESIAN_POINT ( 'NONE',  ( -1.509186351706035767, 0.05413385826771626580, -0.4176697321401330321 ) ) ;
#27577=CARTESIAN_POINT ( 'NONE',  ( 1.614173228346457378, -0.6692913385826771977, 8.415575281601705876E-17 ) ) ;
#27579=CARTESIAN_POINT ( 'NONE',  ( 0.7545931758530189937, 0.1771653543307087075, -0.09757992244046823083 ) ) ;
#27580=CARTESIAN_POINT ( 'NONE',  ( 0.3871391076115493490, -0.3162353388693405765, 0.4822834645669290543 ) ) ;
#27581=EDGE_CURVE ( 'NONE', #11346, #71641, #22668, .T. ) ;
#27583=CARTESIAN_POINT ( 'NONE',  ( 1.240157480314961314, -0.4536011799217367080, 0.2665933059059888421 ) ) ;
#27586=CARTESIAN_POINT ( 'NONE',  ( -1.410761154855641575, -0.2845877964562161244, -0.3641732283464567121 ) ) ;
#27587=CARTESIAN_POINT ( 'NONE',  ( -0.6102362204724400829, -0.5400638737290845981, -0.3530559997133363437 ) ) ;
#27588=CARTESIAN_POINT ( 'NONE',  ( 0.2099737532808405305, 0.2306618581243847221, -0.2411417322834647770 ) ) ;
#27589=CARTESIAN_POINT ( 'NONE',  ( -1.417322834645668772, -0.1870078740157479769, 0.3641732283464567677 ) ) ;
#27591=CARTESIAN_POINT ( 'NONE',  ( -1.391076115485563758, 0.2306618581243848609, 0.2411417322834645549 ) ) ;
#27592=CARTESIAN_POINT ( 'NONE',  ( 0.4265091863517067594, 0.2952755905511811885, 0.1292274648535926551 ) ) ;
#27593=CARTESIAN_POINT ( 'NONE',  ( -0.07874015748031421014, -0.1870078740157479769, 0.4822834645669291653 ) ) ;
#27594=CARTESIAN_POINT ( 'NONE',  ( 1.017060367454068581, -0.05778040916215560624, -0.4822834645669293319 ) ) ;
#27595=B_SPLINE_CURVE_WITH_KNOTS ( 'NONE', 3,
 ( #55934, #787, #45373, #45788, #56759, #31092, #83277 ),
 .UNSPECIFIED., .F., .F.,
 ( 4, 3, 4 ),
 ( 3.471140604459641645E-18, 0.001246230184515550706, 0.002492489877932668914 ),
 .UNSPECIFIED. ) ;
#27600=CARTESIAN_POINT ( 'NONE',  ( 0.3083989501312343062, -0.2845877964562159024, 0.3641732283464567677 ) ) ;
#27601=CARTESIAN_POINT ( 'NONE',  ( -0.4724409448818890911, -0.1870078740157479769, 0.4822834645669291653 ) ) ;
#27602=CARTESIAN_POINT ( 'NONE',  ( 1.213910761154856299, -0.6692913385826773087, -0.1292274648535924053 ) ) ;
#27604=CARTESIAN_POINT ( 'NONE',  ( -0.1246719160104980823, -0.5511811023622048555, -0.09757992244046775898 ) ) ;
#27605=CARTESIAN_POINT ( 'NONE',  ( -1.036745406824146176, -0.4281496062992124485, 0.4176697321401328655 ) ) ;
#27606=CARTESIAN_POINT ( 'NONE',  ( 1.594488188976378673, 0.1660481256975885056, 0.3530559997133364547 ) ) ;
#27609=ORIENTED_EDGE ( 'NONE', *, *, #73756, .F. ) ;
#27610=ORIENTED_EDGE ( 'NONE', *, *, #40280, .T. ) ;
#27611=CARTESIAN_POINT ( 'NONE',  ( -1.640419947506561060, -0.4281496062992127816, -0.4176697321401328100 ) ) ;
#27612=CARTESIAN_POINT ( 'NONE',  ( -1.161417322834644716, 0.07958543189024085140, 0.2665933059059887866 ) ) ;
#27613=CARTESIAN_POINT ( 'NONE',  ( -1.043307086614172041, -0.5400638737290844871, 0.3530559997133364547 ) ) ;
#27615=CARTESIAN_POINT ( 'NONE',  ( -0.9576546141020345626, 0.004960608223778509643, -0.3437734562760191848 ) ) ;
#27616=CARTESIAN_POINT ( 'NONE',  ( 1.069553805774278832, 0.2952755905511810774, -0.1292274648535930714 ) ) ;
#27617=CARTESIAN_POINT ( 'NONE',  ( -1.200787401574802349, 0.1660481256975883668, -0.3530559997133364547 ) ) ;
#27618=CARTESIAN_POINT ( 'NONE',  ( -0.1312335958005241554, 0.2306618581243848609, 0.2411417322834645549 ) ) ;
#27619=CARTESIAN_POINT ( 'NONE',  ( -1.135170603674539924, 0.2952755905511810774, -0.1292274648535930714 ) ) ;
#27621=CARTESIAN_POINT ( 'NONE',  ( 0.4396325459317590445, -0.6692913385826771977, 0.1292274648535927661 ) ) ;
#27623=CARTESIAN_POINT ( 'NONE',  ( -1.076115485564303809, -0.5023911411419708095, -0.1820866141732282451 ) ) ;
#27626=ORIENTED_EDGE ( 'NONE', *, *, #72060, .F. ) ;
#27629=CARTESIAN_POINT ( 'NONE',  ( -1.023622047244094002, -0.1870078740157480879, -0.4822834645669291653 ) ) ;
#27630=CARTESIAN_POINT ( 'NONE',  ( -1.325459317585300889, 0.05413385826771666132, 0.4176697321401328100 ) ) ;
#27632=CARTESIAN_POINT ( 'NONE',  ( -1.489501312335957062, -0.3162353388693409650, -0.4822834645669289433 ) ) ;
#27633=CARTESIAN_POINT ( 'NONE',  ( -1.535433070866141225, 0.2952755905511811885, 0.000000000000000000 ) ) ;
#27634=CARTESIAN_POINT ( 'NONE',  ( -1.456692913385826182, 0.2952755905511811885, 0.000000000000000000 ) ) ;
#27635=CARTESIAN_POINT ( 'NONE',  ( -1.646051170424378096, 0.000000000000000000, -0.3464511005275205946 ) ) ;
#27637=CARTESIAN_POINT ( 'NONE',  ( 0.006561679790026889343, -0.2845877964562161244, -0.3641732283464567121 ) ) ;
#27639=CARTESIAN_POINT ( 'NONE',  ( -0.8530183727034112984, -0.3690944881889765550, -0.3153832671262227771 ) ) ;
#27640=CARTESIAN_POINT ( 'NONE',  ( -1.076115485564303809, -0.6046776061558809534, -0.2411417322834644161 ) ) ;
#27641=CARTESIAN_POINT ( 'NONE',  ( 1.069553805774278610, -0.6692913385826771977, 0.1292274648535927661 ) ) ;
#27642=CARTESIAN_POINT ( 'NONE',  ( -0.8267716535433065062, 0.2952755905511811885, 0.000000000000000000 ) ) ;
#27644=ORIENTED_EDGE ( 'NONE', *, *, #67069, .T. ) ;
#27645=CARTESIAN_POINT ( 'NONE',  ( -0.8202099737532799750, 0.2952755905511810774, -0.1292274648535930714 ) ) ;
#27646=CARTESIAN_POINT ( 'NONE',  ( 0.9580052493438326877, 0.05413385826771666132, 0.4176697321401328100 ) ) ;
#27647=CARTESIAN_POINT ( 'NONE',  ( -1.430446194225721390, -0.3690944881889763329, 0.3153832671262228327 ) ) ;
#27648=CARTESIAN_POINT ( 'NONE',  ( -1.614173228346456268, -0.6692913385826771977, 8.415575281601705876E-17 ) ) ;
#27653=CARTESIAN_POINT ( 'NONE',  ( -0.2690288713910754526, -0.6692913385826771977, 0.1292274648535927661 ) ) ;
#27654=CARTESIAN_POINT ( 'NONE',  ( -1.496062992125983815, -0.1870078740157479769, 0.3641732283464567677 ) ) ;
#27656=CARTESIAN_POINT ( 'NONE',  ( -1.115485564304461219, -0.4281496062992124485, 0.4176697321401328655 ) ) ;
#27658=CARTESIAN_POINT ( 'NONE',  ( -1.601049868766403650, -0.6046776061558807314, 0.2411417322834647770 ) ) ;
#27659=CARTESIAN_POINT ( 'NONE',  ( -0.2821522309711278487, 0.2952755905511811885, 0.1292274648535926551 ) ) ;
#27661=CARTESIAN_POINT ( 'NONE',  ( 0.5183727034120741983, 0.1771653543307087075, -0.09757992244046823083 ) ) ;
#27663=CARTESIAN_POINT ( 'NONE',  ( 0.1706036745406830368, -0.3690944881889765550, -0.3153832671262227771 ) ) ;
#27664=CARTESIAN_POINT ( 'NONE',  ( 0.7349081364829402885, -0.5023911411419708095, -0.1820866141732282451 ) ) ;
#27665=CARTESIAN_POINT ( 'NONE',  ( 0.8727034120734912248, -0.3162353388693409650, -0.4822834645669289433 ) ) ;
#27666=CARTESIAN_POINT ( 'NONE',  ( 0.3149606299212606708, -0.1870078740157480601, -0.3641732283464567677 ) ) ;
#27668=CARTESIAN_POINT ( 'NONE',  ( -1.305774278215222184, 0.2952755905511811885, 0.1292274648535926551 ) ) ;
#27669=CARTESIAN_POINT ( 'NONE',  ( -0.1902887139107604098, -0.5511811023622046335, 0.09757992244046803654 ) ) ;
#27670=CARTESIAN_POINT ( 'NONE',  ( -1.115485564304461219, -0.004921259842519870586, -0.3153832671262229437 ) ) ;
#27673=CARTESIAN_POINT ( 'NONE',  ( -0.5839895013123351797, -0.5511811023622046335, 0.09757992244046803654 ) ) ;
#27676=CARTESIAN_POINT ( 'NONE',  ( 0.04593175853018440641, -0.6692913385826771977, 0.1292274648535927661 ) ) ;
#27678=CARTESIAN_POINT ( 'NONE',  ( 0.6824146981627303710, 0.1283753931104746893, -0.1820866141732285504 ) ) ;
#27679=CARTESIAN_POINT ( 'NONE',  ( -0.2427821522309703550, -0.08942795157528024563, -0.3641732283464568787 ) ) ;
#27680=CARTESIAN_POINT ( 'NONE',  ( -0.1377952755905504645, -0.5400638737290845981, -0.3530559997133363437 ) ) ;
#27681=CARTESIAN_POINT ( 'NONE',  ( -1.686351706036744558, 0.2952755905511810774, -0.1292274648535930714 ) ) ;
#27682=CARTESIAN_POINT ( 'NONE',  ( -1.161417322834644716, 0.07958543189024085140, 0.2665933059059887866 ) ) ;
#27684=CARTESIAN_POINT ( 'NONE',  ( 0.4527559055118117182, 0.1660481256975883668, -0.3530559997133364547 ) ) ;
#27688=B_SPLINE_CURVE_WITH_KNOTS ( 'NONE', 3,
 ( #24231, #69278, #36048, #35636 ),
 .UNSPECIFIED., .F., .F.,
 ( 4, 4 ),
 ( 1.999999999927407068E-07, 0.006970199999999936863 ),
 .UNSPECIFIED. ) ;
#27689=CARTESIAN_POINT ( 'NONE',  ( -0.2427821522309703550, -0.08942795157528024563, -0.3641732283464568787 ) ) ;
#27691=CARTESIAN_POINT ( 'NONE',  ( -1.423884514435694859, -0.05778040916215560624, -0.4822834645669293319 ) ) ;
#27692=CARTESIAN_POINT ( 'NONE',  ( -1.614173228346455824, 0.1771653543307087630, 0.000000000000000000 ) ) ;
#27694=CARTESIAN_POINT ( 'NONE',  ( -0.7611548556430438595, 0.1283753931104748280, 0.1820866141732283561 ) ) ;
#27695=CARTESIAN_POINT ( 'NONE',  ( -0.7742782152230965886, 0.009842519685039463617, 0.3409548833797002576 ) ) ;
#27696=CARTESIAN_POINT ( 'NONE',  ( 0.6692913385826777528, 0.2952755905511811885, 0.000000000000000000 ) ) ;
#27700=CARTESIAN_POINT ( 'NONE',  ( -1.627296587926508442, -0.6046776061558809534, -0.2411417322834644161 ) ) ;
#27701=CARTESIAN_POINT ( 'NONE',  ( -1.167979002624671470, -0.4281496062992127816, -0.4176697321401328100 ) ) ;
#27702=CARTESIAN_POINT ( 'NONE',  ( 1.417322834645670104, -0.1870078740157479769, 0.4822834645669291653 ) ) ;
#27704=CARTESIAN_POINT ( 'NONE',  ( 1.456692913385827515, -0.5511811023622047445, 6.969142054262312111E-17 ) ) ;
#27705=CARTESIAN_POINT ( 'NONE',  ( 0.4986876640419954376, -0.6046776061558809534, -0.2411417322834644161 ) ) ;
#27706=CARTESIAN_POINT ( 'NONE',  ( -0.4921259842519677963, 0.1660481256975883668, -0.3530559997133364547 ) ) ;
#27708=CARTESIAN_POINT ( 'NONE',  ( 0.06764250034433770542, 1.722984403643211298E-16, -0.3954985857520063597 ) ) ;
#27709=CARTESIAN_POINT ( 'NONE',  ( 0.9448818897637802916, -0.1870078740157479769, 0.3641732283464567677 ) ) ;
#27712=ORIENTED_EDGE ( 'NONE', *, *, #9952, .T. ) ;
#27713=CARTESIAN_POINT ( 'NONE',  ( -0.2362204724409442680, -0.1870078740157480879, -0.4822834645669291653 ) ) ;
#27714=CARTESIAN_POINT ( 'NONE',  ( 1.358267716535433323, -0.5400638737290845981, -0.3530559997133363437 ) ) ;
#27715=CARTESIAN_POINT ( 'NONE',  ( 0.07217847769028949700, -0.3162353388693405765, 0.4822834645669290543 ) ) ;
#27716=CARTESIAN_POINT ( 'NONE',  ( -0.2690288713910754526, -0.5511811023622046335, 0.09757992244046803654 ) ) ;
#27717=CARTESIAN_POINT ( 'NONE',  ( 1.043307086614173818, 0.1660481256975885056, 0.3530559997133364547 ) ) ;
#27718=CARTESIAN_POINT ( 'NONE',  ( -0.7217847769028863381, -0.4281496062992124485, 0.4176697321401328655 ) ) ;
#27719=CARTESIAN_POINT ( 'NONE',  ( -0.09186351706036689768, 0.05413385826771626580, -0.4176697321401330321 ) ) ;
#27720=CARTESIAN_POINT ( 'NONE',  ( -0.7349081364829390672, 0.2306618581243847221, -0.2411417322834647770 ) ) ;
#27721=CARTESIAN_POINT ( 'NONE',  ( 1.154855643044620184, 0.2306618581243847221, -0.2411417322834647770 ) ) ;
#27722=CARTESIAN_POINT ( 'NONE',  ( 0.9776902887139113929, 0.2952755905511811885, 0.1292274648535926551 ) ) ;
#27723=CARTESIAN_POINT ( 'NONE',  ( 1.141732283464567788, -0.6692913385826771977, 8.415575281601705876E-17 ) ) ;
#27725=CARTESIAN_POINT ( 'NONE',  ( -0.07874015748031421014, -0.1870078740157479769, 0.3641732283464567677 ) ) ;
#27726=ORIENTED_EDGE ( 'NONE', *, *, #40829, .T. ) ;
#27728=AXIS2_PLACEMENT_3D ( 'NONE', #38514, #6943, #12030 ) ;
#27729=ORIENTED_EDGE ( 'NONE', *, *, #37854, .F. ) ;
#27730=CARTESIAN_POINT ( 'NONE',  ( -0.9645669291338575535, -0.4536011799217367080, 0.2665933059059888421 ) ) ;
#27732=CARTESIAN_POINT ( 'NONE',  ( -0.1115485564304453947, -0.6692913385826771977, 0.1292274648535927661 ) ) ;
#27733=CARTESIAN_POINT ( 'NONE',  ( 1.595398199321655275, 0.4829664696085563258, -0.1559797534342493575 ) ) ;
#27734=CARTESIAN_POINT ( 'NONE',  ( -0.2821522309711278487, 0.2952755905511811885, 0.1292274648535926551 ) ) ;
#27735=CARTESIAN_POINT ( 'NONE',  ( -0.4527559055118102749, 0.1660481256975885056, 0.3530559997133364547 ) ) ;
#27736=CARTESIAN_POINT ( 'NONE',  ( -0.6758530183727028406, 0.2952755905511811885, 0.1292274648535926551 ) ) ;
#27737=CARTESIAN_POINT ( 'NONE',  ( -1.030183727034119867, -0.05778040916215560624, -0.4822834645669293319 ) ) ;
#27738=CARTESIAN_POINT ( 'NONE',  ( 1.535433070866142558, 0.1771653543307087630, 0.000000000000000000 ) ) ;
#27739=CARTESIAN_POINT ( 'NONE',  ( -1.476377952755905110, 0.1660481256975885056, 0.3530559997133364547 ) ) ;
#27741=CARTESIAN_POINT ( 'NONE',  ( 0.3805774278215230400, -0.004921259842519870586, -0.3153832671262229437 ) ) ;
#27742=CARTESIAN_POINT ( 'NONE',  ( 0.07217847769028949700, -0.3162353388693405765, 0.4822834645669290543 ) ) ;
#27743=CARTESIAN_POINT ( 'NONE',  ( 0.4790026246719168435, -0.3162353388693409650, -0.4822834645669289433 ) ) ;
#27744=ORIENTED_EDGE ( 'NONE', *, *, #4245, .T. ) ;
#27749=CARTESIAN_POINT ( 'NONE',  ( -0.3674540682414692561, -0.6046776061558809534, -0.2411417322834644161 ) ) ;
#27752=CARTESIAN_POINT ( 'NONE',  ( -1.476377952755905110, 0.07958543189024085140, 0.2665933059059887866 ) ) ;
#27753=CARTESIAN_POINT ( 'NONE',  ( 0.7742782152230978099, -0.4281496062992124485, 0.4176697321401328655 ) ) ;
#27754=CARTESIAN_POINT ( 'NONE',  ( 0.8792650918635177559, 0.05413385826771666132, 0.4176697321401328100 ) ) ;
#27755=CARTESIAN_POINT ( 'NONE',  ( -0.1706036745406816491, -0.004921259842519870586, -0.3153832671262229437 ) ) ;
#27756=CARTESIAN_POINT ( 'NONE',  ( 0.3608923884514443348, 0.2952755905511810774, -0.1292274648535930714 ) ) ;
#27758=CARTESIAN_POINT ( 'NONE',  ( 0.01312335958005323398, -0.3690944881889765550, -0.3153832671262227771 ) ) ;
#27759=CARTESIAN_POINT ( 'NONE',  ( -0.1706036745406816491, -0.4281496062992124485, 0.4176697321401328655 ) ) ;
#27761=CARTESIAN_POINT ( 'NONE',  ( -1.640419947506561060, -0.4281496062992127816, -0.4176697321401328100 ) ) ;
#27762=CARTESIAN_POINT ( 'NONE',  ( -0.06561679790026180015, -0.3690944881889765550, -0.3153832671262227771 ) ) ;
#27763=CARTESIAN_POINT ( 'NONE',  ( 1.561679790026247350, -0.004921259842519870586, -0.3153832671262229437 ) ) ;
#27764=CARTESIAN_POINT ( 'NONE',  ( -0.9251968503937002541, 0.1660481256975885056, 0.3530559997133364547 ) ) ;
#27765=CARTESIAN_POINT ( 'NONE',  ( -0.5708661417322825615, -0.4536011799217367080, 0.2665933059059888421 ) ) ;
#27767=CARTESIAN_POINT ( 'NONE',  ( -0.8923884514435688198, 0.2306618581243847221, -0.2411417322834647770 ) ) ;
#27768=CARTESIAN_POINT ( 'NONE',  ( -0.4724409448818890911, -0.1870078740157480879, -0.4822834645669291653 ) ) ;
#27769=CARTESIAN_POINT ( 'NONE',  ( 0.1181102362204730916, 0.2952755905511811885, 0.000000000000000000 ) ) ;
#27771=EDGE_CURVE ( 'NONE', #44890, #9475, #63273, .T. ) ;
#27774=CARTESIAN_POINT ( 'NONE',  ( 0.7283464566929143125, 0.07958543189024085140, 0.2665933059059887866 ) ) ;
#27775=CARTESIAN_POINT ( 'NONE',  ( 1.496062992125984703, -0.1870078740157480879, -0.4822834645669291653 ) ) ;
#27776=CARTESIAN_POINT ( 'NONE',  ( -1.036745406824146176, -0.004921259842519870586, -0.3153832671262229437 ) ) ;
#27777=CARTESIAN_POINT ( 'NONE',  ( 1.102362204724410155, -0.1870078740157480879, -0.4822834645669291653 ) ) ;
#27778=CARTESIAN_POINT ( 'NONE',  ( -1.312335958005248715, -0.5023911411419708095, -0.1820866141732282451 ) ) ;
#27780=CARTESIAN_POINT ( 'NONE',  ( -0.3608923884514428360, -0.6692913385826773087, -0.1292274648535924053 ) ) ;
#27781=CARTESIAN_POINT ( 'NONE',  ( 0.2165354330708668673, -0.4536011799217367080, 0.2665933059059888421 ) ) ;
#27783=CARTESIAN_POINT ( 'NONE',  ( 1.253280839895013710, -0.2845877964562159024, 0.3641732283464567677 ) ) ;
#27784=CARTESIAN_POINT ( 'NONE',  ( 0.1968503937007881344, -0.6692913385826771977, 8.415575281601705876E-17 ) ) ;
#27786=CARTESIAN_POINT ( 'NONE',  ( -0.5971128608923877978, 0.2952755905511811885, 0.1292274648535926551 ) ) ;
#27787=VECTOR ( 'NONE', #22893, 39.37007874015748143 ) ;
#27789=CARTESIAN_POINT ( 'NONE',  ( 1.161417322834646271, 0.07958543189024071263, -0.2665933059059888421 ) ) ;
#27790=AXIS2_PLACEMENT_3D ( 'NONE', #73286, #29480, #41693 ) ;
#27791=CARTESIAN_POINT ( 'NONE',  ( 0.3018372703412079971, 0.05413385826771626580, -0.4176697321401330321 ) ) ;
#27793=CARTESIAN_POINT ( 'NONE',  ( -0.2362204724409440182, -0.1870078740157479769, 0.4822834645669291653 ) ) ;
#27794=CARTESIAN_POINT ( 'NONE',  ( 0.06561679790026316017, -0.3690944881889763329, 0.3153832671262228327 ) ) ;
#27796=CARTESIAN_POINT ( 'NONE',  ( -0.01312335958005186876, -0.004921259842519870586, -0.3153832671262229437 ) ) ;
#27797=CARTESIAN_POINT ( 'NONE',  ( 0.1968503937007881344, -0.6692913385826771977, 8.415575281601705876E-17 ) ) ;
#27798=CARTESIAN_POINT ( 'NONE',  ( -0.8792650918635160906, -0.004921259842519870586, -0.3153832671262229437 ) ) ;
#27800=CARTESIAN_POINT ( 'NONE',  ( -1.187664041994749731, -0.3162353388693405765, 0.4822834645669290543 ) ) ;
#27802=ORIENTED_EDGE ( 'NONE', *, *, #10106, .F. ) ;
#27803=CARTESIAN_POINT ( 'NONE',  ( -0.9186351706036736120, 0.1283753931104748280, 0.1820866141732283561 ) ) ;
#27804=CARTESIAN_POINT ( 'NONE',  ( -0.07217847769028813698, -0.3162353388693409650, -0.4822834645669289433 ) ) ;
#27805=CARTESIAN_POINT ( 'NONE',  ( -1.574803149606298636, -0.1870078740157479769, 0.4822834645669291653 ) ) ;
#27806=CARTESIAN_POINT ( 'NONE',  ( -0.7283464566929126471, -0.5400638737290844871, 0.3530559997133364547 ) ) ;
#27808=CARTESIAN_POINT ( 'NONE',  ( -0.8777275986338654024, 0.02791078216816347476, -0.4328096321851898631 ) ) ;
#27809=CARTESIAN_POINT ( 'NONE',  ( 1.128608923884514947, 0.2306618581243848609, 0.2411417322834645549 ) ) ;
#27810=CARTESIAN_POINT ( 'NONE',  ( 0.7677165354330716118, 0.1660481256975883668, -0.3530559997133364547 ) ) ;
#27812=CARTESIAN_POINT ( 'NONE',  ( 1.482939632545932307, 0.05413385826771626580, -0.4176697321401330321 ) ) ;
#27813=CARTESIAN_POINT ( 'NONE',  ( -1.233595800524933894, 0.2306618581243848609, 0.2411417322834645549 ) ) ;
#27816=CARTESIAN_POINT ( 'NONE',  ( -0.3083989501312330295, -0.2845877964562161244, -0.3641732283464567121 ) ) ;
#27819=CARTESIAN_POINT ( 'NONE',  ( 0.9711286089238851948, 0.2306618581243848609, 0.2411417322834645549 ) ) ;
#27820=CARTESIAN_POINT ( 'NONE',  ( 0.04593175853018440641, 0.2952755905511810774, -0.1292274648535930714 ) ) ;
#27821=CARTESIAN_POINT ( 'NONE',  ( -0.6758530183727028406, 0.2952755905511811885, 0.1292274648535926551 ) ) ;
#27822=CARTESIAN_POINT ( 'NONE',  ( 1.443569553805774897, -0.6046776061558809534, -0.2411417322834644161 ) ) ;
#27823=CARTESIAN_POINT ( 'NONE',  ( -0.6692913385826764205, 0.1771653543307087630, 0.000000000000000000 ) ) ;
#27825=CARTESIAN_POINT ( 'NONE',  ( 0.1377952755905518800, 0.1660481256975883668, -0.3530559997133364547 ) ) ;
#27826=CARTESIAN_POINT ( 'NONE',  ( 0.6955380577427828781, -0.004921259842519870586, -0.3153832671262229437 ) ) ;
#27827=CARTESIAN_POINT ( 'NONE',  ( -0.5643044619422565855, -0.4281496062992124485, 0.4176697321401328655 ) ) ;
#27829=CARTESIAN_POINT ( 'NONE',  ( -1.108923884514435132, -0.05778040916215560624, -0.4822834645669293319 ) ) ;
#27831=CARTESIAN_POINT ( 'NONE',  ( 1.246719160104987623, 0.05413385826771626580, -0.4176697321401330321 ) ) ;
#27832=CARTESIAN_POINT ( 'NONE',  ( 1.384514435695538559, 0.1771653543307087075, -0.09757992244046823083 ) ) ;
#27835=CARTESIAN_POINT ( 'NONE',  ( -0.1509186351706028884, -0.3162353388693409650, -0.4822834645669289433 ) ) ;
#27836=ORIENTED_EDGE ( 'NONE', *, *, #58308, .T. ) ;
#27837=CARTESIAN_POINT ( 'NONE',  ( 0.7742782152230978099, -0.3690944881889763329, 0.3153832671262228327 ) ) ;
#27838=CARTESIAN_POINT ( 'NONE',  ( -1.030183727034119867, -0.05778040916215560624, -0.4822834645669293319 ) ) ;
#27839=CARTESIAN_POINT ( 'NONE',  ( 0.9973753280839902091, 0.2306618581243847221, -0.2411417322834647770 ) ) ;
#27840=CARTESIAN_POINT ( 'NONE',  ( 0.7874015748031503170, -0.1870078740157479769, 0.4822834645669291653 ) ) ;
#27841=CARTESIAN_POINT ( 'NONE',  ( 0.3608923884514443348, 0.2952755905511810774, -0.1292274648535930714 ) ) ;
#27843=CARTESIAN_POINT ( 'NONE',  ( -0.4855643044619415427, 0.05413385826771626580, -0.4176697321401330321 ) ) ;
#27845=CARTESIAN_POINT ( 'NONE',  ( 1.574803149606299746, -0.1870078740157479769, 0.3641732283464567677 ) ) ;
#27846=CARTESIAN_POINT ( 'NONE',  ( -0.4461942257217840213, -0.6046776061558809534, -0.2411417322834644161 ) ) ;
#27847=CARTESIAN_POINT ( 'NONE',  ( -0.5708661417322825615, -0.4536011799217367080, 0.2665933059059888421 ) ) ;
#27848=CARTESIAN_POINT ( 'NONE',  ( 1.686351706036745890, 0.2952755905511811885, 0.1292274648535926551 ) ) ;
#27849=CARTESIAN_POINT ( 'NONE',  ( 2.795275590551181466, 0.7480314960629931287, -2.695814348275282069E-16 ) ) ;
#27850=CARTESIAN_POINT ( 'NONE',  ( -0.4658792650918627265, -0.05778040916215522460, 0.4822834645669289988 ) ) ;
#27853=CARTESIAN_POINT ( 'NONE',  ( 0.5183727034120741983, 0.2952755905511810774, -0.1292274648535930714 ) ) ;
#27857=CARTESIAN_POINT ( 'NONE',  ( -0.01312335958005186876, 0.05413385826771626580, -0.4176697321401330321 ) ) ;
#27858=VECTOR ( 'NONE', #39218, 39.37007874015748143 ) ;
#27859=CARTESIAN_POINT ( 'NONE',  ( 0.9842519685039378130, -0.5511811023622047445, 6.969142054262312111E-17 ) ) ;
#27861=CARTESIAN_POINT ( 'NONE',  ( 1.023622047244095334, -0.1870078740157479769, 0.3641732283464567677 ) ) ;
#27862=CARTESIAN_POINT ( 'NONE',  ( 1.062992125984252745, -0.6692913385826771977, 8.415575281601705876E-17 ) ) ;
#27864=CARTESIAN_POINT ( 'NONE',  ( -0.4068241469816267775, 0.05413385826771626580, -0.4176697321401330321 ) ) ;
#27865=CARTESIAN_POINT ( 'NONE',  ( -1.581364829396324945, -0.05778040916215560624, -0.4822834645669293319 ) ) ;
#27866=CARTESIAN_POINT ( 'NONE',  ( -1.640419947506561060, -0.4281496062992127816, -0.4176697321401328100 ) ) ;
#27867=CARTESIAN_POINT ( 'NONE',  ( -0.1312335958005241554, 0.2306618581243848609, 0.2411417322834645549 ) ) ;
#27869=CARTESIAN_POINT ( 'NONE',  ( 1.102362204724410155, -0.1870078740157480879, -0.4822834645669291653 ) ) ;
#27870=CARTESIAN_POINT ( 'NONE',  ( 0.4461942257217855201, -0.6046776061558807314, 0.2411417322834647770 ) ) ;
#27871=CARTESIAN_POINT ( 'NONE',  ( 0.6167979002624679463, -0.004921259842519870586, -0.3153832671262229437 ) ) ;
#27873=CARTESIAN_POINT ( 'NONE',  ( 0.2427821522309719648, -0.08942795157527998196, 0.3641732283464567121 ) ) ;
#27876=CARTESIAN_POINT ( 'NONE',  ( 0.8989501312335964611, 0.2952755905511811885, 0.1292274648535926551 ) ) ;
#27880=CARTESIAN_POINT ( 'NONE',  ( 0.05249343832021075018, 0.1283753931104746893, -0.1820866141732285504 ) ) ;
#27881=CARTESIAN_POINT ( 'NONE',  ( 0.3215223097112867578, -0.3162353388693409650, -0.4822834645669289433 ) ) ;
#27882=CARTESIAN_POINT ( 'NONE',  ( 1.213910761154856299, 0.1771653543307087630, 0.09757992244046791164 ) ) ;
#27883=CARTESIAN_POINT ( 'NONE',  ( -1.246719160104986512, -0.004921259842519576551, 0.3153832671262227771 ) ) ;
#27884=CARTESIAN_POINT ( 'NONE',  ( -0.9317585301837263412, 0.05413385826771666132, 0.4176697321401328100 ) ) ;
#27885=CARTESIAN_POINT ( 'NONE',  ( -1.548556430446193399, 0.2306618581243848609, 0.2411417322834645549 ) ) ;
#27886=CARTESIAN_POINT ( 'NONE',  ( 0.4790026246719168435, -0.3162353388693409650, -0.4822834645669289433 ) ) ;
#27887=CARTESIAN_POINT ( 'NONE',  ( 1.548556430446194954, 0.2306618581243847221, -0.2411417322834647770 ) ) ;
#27889=CARTESIAN_POINT ( 'NONE',  ( 0.7808398950131240079, -0.3162353388693405765, 0.4822834645669290543 ) ) ;
#27892=CARTESIAN_POINT ( 'NONE',  ( 1.253280839895013710, -0.05778040916215560624, -0.4822834645669293319 ) ) ;
#27893=CARTESIAN_POINT ( 'NONE',  ( -1.364829396325458521, 0.1283753931104746893, -0.1820866141732285504 ) ) ;
#27894=CARTESIAN_POINT ( 'NONE',  ( 1.082677165354331228, 0.07958543189024071263, -0.2665933059059888421 ) ) ;
#27895=CARTESIAN_POINT ( 'NONE',  ( -1.286089238845143479, 0.1283753931104746893, -0.1820866141732285504 ) ) ;
#27896=CARTESIAN_POINT ( 'NONE',  ( -0.8464566929133852113, 0.07958543189024085140, 0.2665933059059887866 ) ) ;
#27897=CARTESIAN_POINT ( 'NONE',  ( 0.5643044619422579178, -0.3690944881889765550, -0.3153832671262227771 ) ) ;
#27898=CARTESIAN_POINT ( 'NONE',  ( 0.2362204724409456558, -0.1870078740157479769, 0.4822834645669291653 ) ) ;
#27899=CARTESIAN_POINT ( 'NONE',  ( 1.305774278215223960, 0.2952755905511810774, -0.1292274648535930714 ) ) ;
#27900=CARTESIAN_POINT ( 'NONE',  ( 0.1246719160104994284, 0.2952755905511810774, -0.1292274648535930714 ) ) ;
#27901=EDGE_CURVE ( 'NONE', #83014, #43155, #78358, .T. ) ;
#27902=CARTESIAN_POINT ( 'NONE',  ( 0.2493438320209980519, -0.3690944881889765550, -0.3153832671262227771 ) ) ;
#27903=CARTESIAN_POINT ( 'NONE',  ( 1.122047244094488860, 0.1660481256975885056, 0.3530559997133364547 ) ) ;
#27904=CARTESIAN_POINT ( 'NONE',  ( -1.627296587926508442, 0.2306618581243848609, 0.2411417322834645549 ) ) ;
#27905=CARTESIAN_POINT ( 'NONE',  ( -0.9645669291338575535, -0.5400638737290844871, 0.3530559997133364547 ) ) ;
#27909=CARTESIAN_POINT ( 'NONE',  ( -0.7152230971128602510, -0.3162353388693405765, 0.4822834645669290543 ) ) ;
#27910=CARTESIAN_POINT ( 'NONE',  ( -0.2034120734908131112, -0.6692913385826773087, -0.1292274648535924053 ) ) ;
#27915=DIRECTION ( 'NONE',  ( -2.956072690630991240E-16, 1.000000000000000000, 5.002896285981958034E-32 ) ) ;
#27916=CARTESIAN_POINT ( 'NONE',  ( -1.292650918635170010, -0.5511811023622046335, 0.09757992244046803654 ) ) ;
#27918=CARTESIAN_POINT ( 'NONE',  ( -1.456692913385826182, -0.6692913385826771977, 8.415575281601705876E-17 ) ) ;
#27920=CARTESIAN_POINT ( 'NONE',  ( -0.1312335958005241554, -0.6046776061558809534, -0.2411417322834644161 ) ) ;
#27921=CARTESIAN_POINT ( 'NONE',  ( -0.3937007874015740483, -0.1870078740157480601, -0.3641732283464567677 ) ) ;
#27922=EDGE_CURVE ( 'NONE', #49068, #11380, #24057, .T. ) ;
#27923=CARTESIAN_POINT ( 'NONE',  ( 0.8070866141732288002, 0.1660481256975885056, 0.3530559997133364547 ) ) ;
#27924=CARTESIAN_POINT ( 'NONE',  ( 0.4724409448818904789, -0.1870078740157479769, 0.4822834645669291653 ) ) ;
#27928=CARTESIAN_POINT ( 'NONE',  ( 1.279527559055118724, -0.5400638737290845981, -0.3530559997133363437 ) ) ;
#27929=CARTESIAN_POINT ( 'NONE',  ( -0.06561679790026180015, -0.4281496062992127816, -0.4176697321401328100 ) ) ;
#27930=CARTESIAN_POINT ( 'NONE',  ( -1.095800524934382292, -0.3162353388693409650, -0.4822834645669289433 ) ) ;
#27931=CARTESIAN_POINT ( 'NONE',  ( -1.561679790026246017, -0.4281496062992127816, -0.4176697321401328100 ) ) ;
#27932=CARTESIAN_POINT ( 'NONE',  ( 0.8661417322834653598, -0.1870078740157479769, 0.4822834645669291653 ) ) ;
#27934=CARTESIAN_POINT ( 'NONE',  ( 0.1312335958005255154, -0.6046776061558807314, 0.2411417322834647770 ) ) ;
#27935=CARTESIAN_POINT ( 'NONE',  ( 0.4921259842519691285, -0.5400638737290845981, -0.3530559997133363437 ) ) ;
#27936=CARTESIAN_POINT ( 'NONE',  ( -0.02624671916010428221, 0.2306618581243847221, -0.2411417322834647770 ) ) ;
#27937=CARTESIAN_POINT ( 'NONE',  ( 0.7217847769028878924, -0.004921259842519576551, 0.3153832671262227771 ) ) ;
#27938=CARTESIAN_POINT ( 'NONE',  ( -1.391076115485563758, 0.2306618581243848609, 0.2411417322834645549 ) ) ;
#27939=CARTESIAN_POINT ( 'NONE',  ( -1.620734908136482577, -0.6692913385826773087, -0.1292274648535924053 ) ) ;
#27940=CARTESIAN_POINT ( 'NONE',  ( 0.6036745406824153282, -0.6046776061558807314, 0.2411417322834647770 ) ) ;
#27946=CARTESIAN_POINT ( 'NONE',  ( 1.312335958005250269, -0.6046776061558807314, 0.2411417322834647770 ) ) ;
#27947=CARTESIAN_POINT ( 'NONE',  ( 0.5643044619422579178, -0.3690944881889765550, -0.3153832671262227771 ) ) ;
#27953=CARTESIAN_POINT ( 'NONE',  ( -0.1246719160104980823, 0.2952755905511811885, 0.1292274648535926551 ) ) ;
#27954=CARTESIAN_POINT ( 'NONE',  ( 0.9251968503937015864, -0.5400638737290844871, 0.3530559997133364547 ) ) ;
#27956=CARTESIAN_POINT ( 'NONE',  ( -1.469816272965878357, -0.6046776061558809534, -0.2411417322834644161 ) ) ;
#27957=CARTESIAN_POINT ( 'NONE',  ( 1.666666666666667185, -0.004921259842519576551, 0.3153832671262227771 ) ) ;
#27959=CARTESIAN_POINT ( 'NONE',  ( 1.594488188976378673, -0.4536011799217368745, -0.2665933059059886201 ) ) ;
#27961=CARTESIAN_POINT ( 'NONE',  ( -1.154855643044618851, 0.1283753931104748280, 0.1820866141732283561 ) ) ;
#27962=CARTESIAN_POINT ( 'NONE',  ( -1.417322834645668772, -0.1870078740157480879, -0.4822834645669291653 ) ) ;
#27963=CARTESIAN_POINT ( 'NONE',  ( 0.1509186351706045259, -0.05778040916215560624, -0.4822834645669293319 ) ) ;
#27964=AXIS2_PLACEMENT_3D ( 'NONE', #10922, #55929, #81645 ) ;
#27966=CARTESIAN_POINT ( 'NONE',  ( 1.666666666666667185, 0.05413385826771666132, 0.4176697321401328100 ) ) ;
#27968=CARTESIAN_POINT ( 'NONE',  ( -0.8661417322834640276, -0.1870078740157480601, -0.3641732283464567677 ) ) ;
#27969=CARTESIAN_POINT ( 'NONE',  ( 0.9448818897637802916, -0.1870078740157480879, -0.4822834645669291653 ) ) ;
#27970=CARTESIAN_POINT ( 'NONE',  ( 1.194225721784777594, -0.3690944881889765550, -0.3153832671262227771 ) ) ;
#27972=CARTESIAN_POINT ( 'NONE',  ( -0.6955380577427815458, -0.3690944881889765550, -0.3153832671262227771 ) ) ;
#27973=CARTESIAN_POINT ( 'NONE',  ( -1.450131233595799651, 0.1771653543307087075, -0.09757992244046823083 ) ) ;
#27975=CARTESIAN_POINT ( 'NONE',  ( 0.6758530183727039509, 0.2952755905511810774, -0.1292274648535930714 ) ) ;
#27976=CARTESIAN_POINT ( 'NONE',  ( -1.030183727034119867, -0.2845877964562159024, 0.3641732283464567677 ) ) ;
#27977=CARTESIAN_POINT ( 'NONE',  ( -0.3608923884514428360, -0.5511811023622048555, -0.09757992244046775898 ) ) ;
#27978=CARTESIAN_POINT ( 'NONE',  ( -0.1443569553805768291, 0.05413385826771666132, 0.4176697321401328100 ) ) ;
#27979=CARTESIAN_POINT ( 'NONE',  ( -1.496062992125983815, -0.1870078740157479769, 0.3641732283464567677 ) ) ;
#27981=CARTESIAN_POINT ( 'NONE',  ( 0.5577427821522314977, -0.3162353388693409650, -0.4822834645669289433 ) ) ;
#27984=CARTESIAN_POINT ( 'NONE',  ( -0.8070866141732276899, -0.5400638737290844871, 0.3530559997133364547 ) ) ;
#27985=CARTESIAN_POINT ( 'NONE',  ( -0.3740157480314953431, -0.4536011799217368745, -0.2665933059059886201 ) ) ;
#27986=CARTESIAN_POINT ( 'NONE',  ( -1.358267716535432434, -0.5400638737290844871, 0.3530559997133364547 ) ) ;
#27987=CARTESIAN_POINT ( 'NONE',  ( 0.3740157480314966754, -0.4536011799217367080, 0.2665933059059888421 ) ) ;
#27988=CARTESIAN_POINT ( 'NONE',  ( -0.5708661417322828946, 0.07958543189024071263, -0.2665933059059888421 ) ) ;
#27989=CARTESIAN_POINT ( 'NONE',  ( -1.049868766404198794, 0.2306618581243847221, -0.2411417322834647770 ) ) ;
#27990=CARTESIAN_POINT ( 'NONE',  ( -1.712598425196849572, 0.1660481256975885056, 0.3530559997133364547 ) ) ;
#27991=CARTESIAN_POINT ( 'NONE',  ( 1.253280839895013710, -0.05778040916215560624, -0.4822834645669293319 ) ) ;
#27992=FACE_OUTER_BOUND ( 'NONE', #40995, .T. ) ;
#27993=CARTESIAN_POINT ( 'NONE',  ( 0.9973753280839902091, -0.5023911411419708095, 0.1820866141732285504 ) ) ;
#27994=CARTESIAN_POINT ( 'NONE',  ( 0.2755905511811031494, 0.2952755905511811885, 0.000000000000000000 ) ) ;
#27995=EDGE_CURVE ( 'NONE', #41294, #41264, #25092, .T. ) ;
#27996=CARTESIAN_POINT ( 'NONE',  ( -1.364829396325458521, -0.6046776061558807314, 0.2411417322834647770 ) ) ;
#27997=CARTESIAN_POINT ( 'NONE',  ( 1.450131233595801428, 0.1771653543307087630, 0.09757992244046791164 ) ) ;
#27998=ORIENTED_EDGE ( 'NONE', *, *, #23876, .F. ) ;
#28000=CARTESIAN_POINT ( 'NONE',  ( -1.338582677165353729, -0.1870078740157479769, 0.3641732283464567677 ) ) ;
#28001=CARTESIAN_POINT ( 'NONE',  ( -0.3608923884514428360, 0.2952755905511811885, 0.1292274648535926551 ) ) ;
#28002=CARTESIAN_POINT ( 'NONE',  ( 0.2427821522309716595, -0.3162353388693409650, -0.4822834645669289433 ) ) ;
#28003=CARTESIAN_POINT ( 'NONE',  ( -1.673228346456691717, 0.07958543189024071263, -0.2665933059059888421 ) ) ;
#28005=CARTESIAN_POINT ( 'NONE',  ( -1.233595800524933894, 0.2306618581243848609, 0.2411417322834645549 ) ) ;
#28006=CARTESIAN_POINT ( 'NONE',  ( 0.5511811023622055217, -0.1870078740157479769, 0.4822834645669291653 ) ) ;
#28007=CARTESIAN_POINT ( 'NONE',  ( -0.02624671916010428221, 0.2306618581243847221, -0.2411417322834647770 ) ) ;
#28008=CARTESIAN_POINT ( 'NONE',  ( 1.259842519685040019, -0.1870078740157479769, 0.4822834645669291653 ) ) ;
#28013=CARTESIAN_POINT ( 'NONE',  ( 0.02624671916010564918, 0.1283753931104748280, 0.1820866141732283561 ) ) ;
#28014=CARTESIAN_POINT ( 'NONE',  ( -0.1509186351706028884, -0.05778040916215522460, 0.4822834645669289988 ) ) ;
#28015=CARTESIAN_POINT ( 'NONE',  ( 0.7611548556430451917, -0.6046776061558807314, 0.2411417322834647770 ) ) ;
#28017=CARTESIAN_POINT ( 'NONE',  ( -0.2165354330708654795, 0.07958543189024085140, 0.2665933059059887866 ) ) ;
#28018=( BOUNDED_SURFACE ( )  B_SPLINE_SURFACE ( 1, 2, ( 
 ( #37853, #18510, #48830, #44153, #63530, #24395, #5861, #31537, #57193, #74531, #61880, #42514, #68217, #13439, #70249, #32366, #82895, #26050, #51708, #58029, #39519, #71096, #65633, #50881, #76581, #33626, #392, #18909, #39095, #25627, #78256, #63940, #64777, #20165, #65207, #7115, #6696, #32786, #45815, #58880, #6277, #19745, #46239, #83305, #77410, #51290, #58455, #7544, #70671, #45399, #57614, #25215, #64359, #33216, #19323, #31953, #77835, #20587, #1238, #814, #26477, #71935, #71514, #52127, #52547, #26887, #14284, #76993, #39948, #13860, #7964, #44560, #44975, #12605, #38262, #13027, #38681, #10030, #9615, #73177, #66450, #21415, #15527, #47068, #35286, #47484, #72760, #2058, #60947, #78677, #22653, #16356, #54627, #66036, #15110, #41592, #67282, #27722, #46660, #42001, #27304, #80339, #8375, #48312, #34040, #34459, #74009, #40357, #8786, #3298, #28962, #2890, #28553, #22241, #72354, #79505, #79096, #9205, #73604, #59703, #67695, #21822, #47896, #54209, #53389, #40765, #60128, #15946, #41185, #66875, #2479, #59289, #28138, #53794, #34878, #79925, #60539, #1647, #14701, #52963, #20998, #10453, #81570, #75248, #68514, #10854, #38476, #57819, #74424, #74843, #17593, #80745, #62191, #23472, #25422, #55860, #16771, #31748, #32163, #51087, #186, #25839, #77203, #49139, #44765, #42820, #6493, #12401, #68922, #19116, #42408, #23059, #70462, #35695, #68106, #38058, #36515, #17188, #43224, #51498, #12819, #70892, #48727, #55038, #23888, #4528, #6074, #45189, #36108, #81156, #55447, #63735, #30198, #49554, #19532, #3714, #57410, #83103, #61779, #76784, #64160, #61361, #29377, #4120, #29785, #1854, #7760, #13242, #78469, #7329, #58241, #607, #2271, #27516, #59501, #71723, #51924, #66245, #38891, #6907, #59087, #26263, #8169, #77629, #20794, #64993, #27934, #53172, #72557, #78887, #46450, #21208, #1442, #8583, #40564, #46863, #13653, #14904, #72143, #52761, #14499, #71306, #34255, #59916, #40152, #19961, #47279, #53592, #27099, #20377, #58667, #65836, #1032, #79301, #33834, #26686, #39306, #21619, #32579, #64570, #45612, #32997, #52341, #78048, #46029, #14079, #39731, #65427, #33426, #40985, #68325, #22037, #66665, #9411, #54426, #74224, #67079, #29996, #48941, #42628, #9004, #61160, #34676, #3511, #41397, #80957, #55659, #79720, #80136, #81369, #10663, #54008, #23682, #15743, #9825, #47697, #23272, #61993, #10246, #15320, #61583, #36318, #22457, #74643, #29180, #73814, #73392, #2687, #16985, #35081, #54847, #60339, #48116, #72969, #16151, #41798, #67489, #29587, #80551, #28347, #60747, #3099, #28763, #35495, #22863, #48524, #16569, #4330, #42214, #67910, #35917, #55250, #3928, #56490, #82594, #69953, #25326, #30412, #69552, #12720, #49765, #82192, #75465, #24913, #57307, #37141, #24509, #24096, #49356, #30825, #31649, #69135, #56080, #44262, #44670, #5978, #50581, #31233, #38380, #62826, #37964, #11900, #81785, #12307, #70365, #63640, #64056, #6396, #32066, #5161, #83005, #50176, #19022, #76288, #18619, #50990, #17804, #36724, #76688, #75053, #4739, #57727, #75871, #18214, #5568, #90, #17400, #43030, #11066, #68725, #37554, #43849, #62400, #43438, #11487, #63228, #56900, #58999, #58574, #26597, #21119, #77108, #52668, #45517, #13147, #71213, #1355, #71631, #939, #64474, #26167, #14409, #20283, #25743, #7667, #19868, #70795, #38798, #14819, #40063, #72052, #52249, #6811, #78795, #51406, #19440, #13983, #32482, #20706, #58145, #33338, #77533, #40478, #65750, #1764, #8083, #27006, #46779, #514, #77954, #66156, #51828, #32907, #33746, #59407, #78375, #46358, #27421, #13556, #45932, #39212, #53082, #72470, #64897, #8495, #39639, #34162, #59823, #7234, #65330, #45091, #48433, #41709, #48023, #28255, #61488, #66991, #54335, #3007, #29085, #9323, #80461, #40889, #53916, #16062, #60249, #73723, #67401, #34993, #60658, #3836, #23178, #66571, #41305, #9736, #47189, #28674, #80045, #73300, #74132, #22364, #8905, #22770, #80866, #16477, #48848, #74549, #42533, #15649, #10156, #35407, #55155, #61071, #3422, #67819, #34581, #72881, #35822, #2178, #2597, #54755 ),
 ( #79629, #42124, #21947, #29496, #16894, #68235, #27845, #10570, #36227, #53506, #79214, #21530, #15230, #47606, #74962, #63545, #81693, #75776, #49260, #11389, #61896, #5066, #30735, #37046, #18525, #50080, #44575, #29901, #55565, #12622, #62728, #81273, #18117, #4643, #57209, #42936, #43750, #82501, #44168, #69456, #69039, #11806, #24817, #37870, #68630, #82096, #25231, #62306, #56398, #30314, #37461, #69861, #49672, #24410, #36629, #4237, #43338, #12212, #24004, #10970, #56802, #82910, #5879, #63134, #5473, #50896, #50484, #31135, #31552, #76596, #18926, #55982, #70267, #76188, #23589, #17308, #75362, #17710, #65652, #39537, #77009, #72371, #71952, #52146, #45416, #410, #77852, #26067, #14305, #1257, #39965, #52564, #45831, #59307, #13044, #13455, #27320, #19342, #71112, #46257, #20604, #65225, #7563, #26905, #51307, #58472, #58045, #71530, #78273, #44992, #7981, #836, #33645, #33235, #70691, #64375, #51726, #1664, #20181, #26494, #6712, #52981, #19763, #7131, #39111, #58897, #64793, #78694, #38697, #32381, #13877, #77428, #21017, #46678, #32805, #38281, #63957, #6294, #31969, #57630, #36925, #25644, #41204, #2496, #3316, #34895, #79114, #9633, #10049, #28980, #61382, #3731, #55054, #28156, #22670, #21839, #67712, #73621, #47916, #80357, #21432, #2076, #48329, #14720, #53406, #15963, #73195, #53811, #54227, #29395, #74026, #48744, #59721, #34057, #2907, #79524, #67299, #23076, #72777, #60145, #34479, #41610, #47502, #15545, #35712, #66055, #35303, #66892, #27741, #9222, #60965, #60557, #28571, #47087, #15127, #54647, #79944, #40373, #22258, #8803, #40782, #66468, #80762, #16372, #42019, #8392, #29802, #44073, #74442, #68126, #36948, #61797, #69356, #55463, #56300, #42837, #5779, #62625, #10471, #4968, #68530, #82403, #57112, #81172, #81589, #82806, #69765, #23490, #31448, #17204, #11288, #49156, #24721, #63443, #11710, #16789, #63037, #12110, #23906, #50390, #30635, #75267, #74862, #4137, #76087, #10871, #81997, #36531, #49571, #42426, #17610, #43241, #68939, #31036, #24311, #25130, #36124, #62207, #4544, #49981, #30215, #75679, #55877, #37768, #18019, #43654, #37365, #56704, #5375, #18431, #729, #71429, #26805, #31870, #71011, #14201, #51208, #307, #13355, #44885, #76501, #33544, #70585, #26387, #65119, #57530, #33126, #39008, #13776, #77750, #83221, #76905, #12939, #39433, #7031, #64692, #19235, #52463, #32281, #19654, #51620, #20083, #57941, #45733, #6192, #38597, #32700, #25542, #58366, #52045, #25962, #77325, #78171, #71851, #64275, #6610, #7456, #12519, #45316, #58796, #1154, #20502, #46156, #39858, #65549, #7880, #59206, #1567, #50800, #18829, #44475, #70166, #38180, #63855, #60458, #9535, #8291, #14618, #60868, #27221, #65955, #28468, #2398, #66369, #66793, #9128, #60042, #28055, #28885, #48238, #33959, #8706, #34799, #72270, #53713, #15027, #15870, #47405, #59621, #22160, #22577, #41518, #73934, #16277, #67616, #40683, #35206, #34377, #80261, #2809, #54129, #3221, #1975, #40272, #54546, #52882, #27639, #79844, #79420, #21740, #47820, #41922, #9946, #61282, #53301, #46572, #15445, #73094, #73521, #35618, #79013, #72679, #46985, #67203, #41105, #78593, #20918, #21333, #30539, #23395, #74346, #49062, #36854, #49480, #62113, #42330, #4045, #75587, #81491, #3634, #68847, #81079, #48650, #16691, #75993, #17926, #49886, #4456, #68029, #56609, #29302, #80671, #75173, #10374, #81904, #36031, #11195, #55373, #18335, #43562, #62945, #69263, #62527, #24629, #61705, #30121, #43975, #29710, #10780, #11610, #37269, #56203, #17518, #74761, #54964, #69672, #17110, #4865, #5280, #42745, #30942, #43150, #82309, #24215, #68440, #36440, #55783, #50295, #12015, #37670, #23807, #22984, #44788, #32186, #64182, #6929, #70484, #58263, #18735, #6097, #77225, #38082, #25862, #12841, #6516, #58686, #31351, #32600, #83125, #50705, #25444, #13263, #51522, #38500, #44377, #63756, #51944, #57841, #63347, #45213, #57432, #25032, #76403, #52361, #77649, #26283, #209, #70069, #33016, #5682, #57017, #19554, #12424, #627, #31771, #70914, #51110, #78067, #19982, #39327, #45632 ) ),
 .UNSPECIFIED., .F., .F., .F. ) 
 B_SPLINE_SURFACE_WITH_KNOTS ( ( 2, 2 ),
 ( 3, 2, 2, 2, 2, 2, 2, 2, 2, 2, 2, 2, 2, 2, 2, 2, 2, 2, 2, 2, 2, 2, 2, 2, 2, 2, 2, 2, 2, 2, 2, 2, 2, 2, 2, 2, 2, 2, 2, 2, 2, 2, 2, 2, 2, 2, 2, 2, 2, 2, 2, 2, 2, 2, 2, 2, 2, 2, 2, 2, 2, 2, 2, 2, 2, 2, 2, 2, 2, 2, 2, 2, 2, 2, 2, 2, 2, 2, 2, 2, 2, 2, 2, 2, 2, 2, 2, 2, 2, 2, 2, 2, 2, 2, 2, 2, 2, 2, 2, 2, 2, 2, 2, 2, 2, 2, 2, 2, 2, 2, 2, 2, 2, 2, 2, 2, 2, 2, 2, 2, 2, 2, 2, 2, 2, 2, 2, 2, 2, 2, 2, 2, 2, 2, 2, 2, 2, 2, 2, 2, 2, 2, 2, 2, 2, 2, 2, 2, 2, 2, 2, 2, 2, 2, 2, 2, 2, 2, 2, 2, 2, 2, 2, 2, 2, 2, 2, 2, 2, 2, 2, 2, 2, 2, 2, 2, 2, 2, 2, 2, 2, 2, 2, 2, 2, 2, 2, 2, 2, 2, 2, 2, 2, 2, 2, 2, 2, 2, 2, 2, 2, 2, 2, 2, 2, 2, 2, 2, 2, 2, 2, 2, 2, 2, 2, 2, 2, 2, 2, 2, 2, 2, 2, 2, 2, 2, 2, 2, 2, 2, 2, 2, 2, 2, 2, 2, 2, 2, 2, 2, 2, 2, 2, 2, 2, 2, 2, 2, 2, 2, 2, 2, 2, 2, 2, 3 ),
 ( 0.000000000000000000, 1.000000000000000000 ),
 ( 0.000000000000000000, 0.003787878787878787984, 0.007575757575757575968, 0.01136363636363636395, 0.01515151515151515194, 0.01893939393939393992, 0.02272727272727272790, 0.02651515151515151589, 0.03030303030303030387, 0.03409090909090908839, 0.03787878787878787984, 0.04166666666666666435, 0.04545454545454545581, 0.04924242424242424032, 0.05303030303030303177, 0.05681818181818181629, 0.06060606060606060774, 0.06439393939393939226, 0.06818181818181817677, 0.07196969696969697516, 0.07575757575757575968, 0.07954545454545454419, 0.08333333333333332871, 0.08712121212121212710, 0.09090909090909091161, 0.09469696969696969613, 0.09848484848484848064, 0.1022727272727272790, 0.1060606060606060635, 0.1098484848484848481, 0.1136363636363636326, 0.1174242424242424310, 0.1212121212121212155, 0.1250000000000000000, 0.1287878787878787845, 0.1325757575757575690, 0.1363636363636363535, 0.1401515151515151381, 0.1439393939393939503, 0.1477272727272727348, 0.1515151515151515194, 0.1553030303030303039, 0.1590909090909090884, 0.1628787878787878729, 0.1666666666666666574, 0.1704545454545454419, 0.1742424242424242542, 0.1780303030303030387, 0.1818181818181818232, 0.1856060606060606077, 0.1893939393939393923, 0.1931818181818181768, 0.1969696969696969613, 0.2007575757575757458, 0.2045454545454545581, 0.2083333333333333426, 0.2121212121212121271, 0.2159090909090909116, 0.2196969696969696961, 0.2234848484848484806, 0.2272727272727272652, 0.2310606060606060497, 0.2348484848484848619, 0.2386363636363636465, 0.2424242424242424310, 0.2462121212121212155, 0.2500000000000000000, 0.2537878787878787845, 0.2575757575757575690, 0.2613636363636363535, 0.2651515151515151381, 0.2689393939393939226, 0.2727272727272727071, 0.2765151515151514916, 0.2803030303030302761, 0.2840909090909091161, 0.2878787878787879007, 0.2916666666666666852, 0.2954545454545454697, 0.2992424242424242542, 0.3030303030303030387, 0.3068181818181818232, 0.3106060606060606077, 0.3143939393939393923, 0.3181818181818181768, 0.3219696969696969613, 0.3257575757575757458, 0.3295454545454545303, 0.3333333333333333148, 0.3371212121212120993, 0.3409090909090908839, 0.3446969696969697239, 0.3484848484848485084, 0.3522727272727272929, 0.3560606060606060774, 0.3598484848484848619, 0.3636363636363636465, 0.3674242424242424310, 0.3712121212121212155, 0.3750000000000000000, 0.3787878787878787845, 0.3825757575757575690, 0.3863636363636363535, 0.3901515151515151381, 0.3939393939393939226, 0.3977272727272727071, 0.4015151515151514916, 0.4053030303030302761, 0.4090909090909091161, 0.4128787878787879007, 0.4166666666666666852, 0.4204545454545454697, 0.4242424242424242542, 0.4280303030303030387, 0.4318181818181818232, 0.4356060606060606077, 0.4393939393939393923, 0.4431818181818181768, 0.4469696969696969613, 0.4507575757575757458, 0.4545454545454545303, 0.4583333333333333148, 0.4621212121212120993, 0.4659090909090908839, 0.4696969696969697239, 0.4734848484848485084, 0.4772727272727272929, 0.4810606060606060774, 0.4848484848484848619, 0.4886363636363636465, 0.4924242424242424310, 0.4962121212121212155, 0.5000000000000000000, 0.5037878787878787845, 0.5075757575757575690, 0.5113636363636363535, 0.5151515151515151381, 0.5189393939393939226, 0.5227272727272727071, 0.5265151515151514916, 0.5303030303030302761, 0.5340909090909090606, 0.5378787878787878451, 0.5416666666666666297, 0.5454545454545454142, 0.5492424242424241987, 0.5530303030303029832, 0.5568181818181817677, 0.5606060606060605522, 0.5643939393939394478, 0.5681818181818182323, 0.5719696969696970168, 0.5757575757575758013, 0.5795454545454545858, 0.5833333333333333703, 0.5871212121212121549, 0.5909090909090909394, 0.5946969696969697239, 0.5984848484848485084, 0.6022727272727272929, 0.6060606060606060774, 0.6098484848484848619, 0.6136363636363636465, 0.6174242424242424310, 0.6212121212121212155, 0.6250000000000000000, 0.6287878787878787845, 0.6325757575757575690, 0.6363636363636363535, 0.6401515151515151381, 0.6439393939393939226, 0.6477272727272727071, 0.6515151515151514916, 0.6553030303030302761, 0.6590909090909090606, 0.6628787878787878451, 0.6666666666666666297, 0.6704545454545454142, 0.6742424242424241987, 0.6780303030303029832, 0.6818181818181817677, 0.6856060606060605522, 0.6893939393939394478, 0.6931818181818182323, 0.6969696969696970168, 0.7007575757575758013, 0.7045454545454545858, 0.7083333333333333703, 0.7121212121212121549, 0.7159090909090909394, 0.7196969696969697239, 0.7234848484848485084, 0.7272727272727272929, 0.7310606060606060774, 0.7348484848484848619, 0.7386363636363636465, 0.7424242424242424310, 0.7462121212121212155, 0.7500000000000000000, 0.7537878787878787845, 0.7575757575757575690, 0.7613636363636363535, 0.7651515151515151381, 0.7689393939393939226, 0.7727272727272727071, 0.7765151515151514916, 0.7803030303030302761, 0.7840909090909090606, 0.7878787878787878451, 0.7916666666666666297, 0.7954545454545454142, 0.7992424242424241987, 0.8030303030303029832, 0.8068181818181817677, 0.8106060606060605522, 0.8143939393939394478, 0.8181818181818182323, 0.8219696969696970168, 0.8257575757575758013, 0.8295454545454545858, 0.8333333333333333703, 0.8371212121212121549, 0.8409090909090909394, 0.8446969696969697239, 0.8484848484848485084, 0.8522727272727272929, 0.8560606060606060774, 0.8598484848484848619, 0.8636363636363636465, 0.8674242424242424310, 0.8712121212121212155, 0.8750000000000000000, 0.8787878787878787845, 0.8825757575757575690, 0.8863636363636363535, 0.8901515151515151381, 0.8939393939393939226, 0.8977272727272727071, 0.9015151515151514916, 0.9053030303030302761, 0.9090909090909090606, 0.9128787878787878451, 0.9166666666666666297, 0.9204545454545454142, 0.9242424242424241987, 0.9280303030303029832, 0.9318181818181817677, 0.9356060606060605522, 0.9393939393939394478, 0.9431818181818182323, 0.9469696969696970168, 0.9507575757575758013, 0.9545454545454545858, 0.9583333333333333703, 0.9621212121212121549, 0.9659090909090909394 ),
 .UNSPECIFIED. ) 
 GEOMETRIC_REPRESENTATION_ITEM ( )  RATIONAL_B_SPLINE_SURFACE ( (
 ( 1.000000000000000000, 0.9659258262890683122, 1.000000000000000000, 0.9659258262890683122, 1.000000000000000000, 0.9659258262890683122, 1.000000000000000000, 0.9659258262890683122, 1.000000000000000000, 0.9659258262890683122, 1.000000000000000000, 0.9659258262890683122, 1.000000000000000000, 0.9659258262890683122, 1.000000000000000000, 0.9659258262890683122, 1.000000000000000000, 0.9659258262890683122, 1.000000000000000000, 0.9659258262890683122, 1.000000000000000000, 0.9659258262890683122, 1.000000000000000000, 0.9659258262890683122, 1.000000000000000000, 0.9659258262890683122, 1.000000000000000000, 0.9659258262890683122, 1.000000000000000000, 0.9659258262890683122, 1.000000000000000000, 0.9659258262890683122, 1.000000000000000000, 0.9659258262890683122, 1.000000000000000000, 0.9659258262890683122, 1.000000000000000000, 0.9659258262890683122, 1.000000000000000000, 0.9659258262890683122, 1.000000000000000000, 0.9659258262890683122, 1.000000000000000000, 0.9659258262890683122, 1.000000000000000000, 0.9659258262890683122, 1.000000000000000000, 0.9659258262890683122, 1.000000000000000000, 0.9659258262890683122, 1.000000000000000000, 0.9659258262890683122, 1.000000000000000000, 0.9659258262890683122, 1.000000000000000000, 0.9659258262890683122, 1.000000000000000000, 0.9659258262890683122, 1.000000000000000000, 0.9659258262890683122, 1.000000000000000000, 0.9659258262890683122, 1.000000000000000000, 0.9659258262890683122, 1.000000000000000000, 0.9659258262890683122, 1.000000000000000000, 0.9659258262890683122, 1.000000000000000000, 0.9659258262890683122, 1.000000000000000000, 0.9659258262890683122, 1.000000000000000000, 0.9659258262890683122, 1.000000000000000000, 0.9659258262890683122, 1.000000000000000000, 0.9659258262890683122, 1.000000000000000000, 0.9659258262890683122, 1.000000000000000000, 0.9659258262890683122, 1.000000000000000000, 0.9659258262890683122, 1.000000000000000000, 0.9659258262890683122, 1.000000000000000000, 0.9659258262890683122, 1.000000000000000000, 0.9659258262890683122, 1.000000000000000000, 0.9659258262890683122, 1.000000000000000000, 0.9659258262890683122, 1.000000000000000000, 0.9659258262890683122, 1.000000000000000000, 0.9659258262890683122, 1.000000000000000000, 0.9659258262890683122, 1.000000000000000000, 0.9659258262890683122, 1.000000000000000000, 0.9659258262890683122, 1.000000000000000000, 0.9659258262890683122, 1.000000000000000000, 0.9659258262890683122, 1.000000000000000000, 0.9659258262890683122, 1.000000000000000000, 0.9659258262890683122, 1.000000000000000000, 0.9659258262890683122, 1.000000000000000000, 0.9659258262890683122, 1.000000000000000000, 0.9659258262890683122, 1.000000000000000000, 0.9659258262890683122, 1.000000000000000000, 0.9659258262890683122, 1.000000000000000000, 0.9659258262890683122, 1.000000000000000000, 0.9659258262890683122, 1.000000000000000000, 0.9659258262890683122, 1.000000000000000000, 0.9659258262890683122, 1.000000000000000000, 0.9659258262890683122, 1.000000000000000000, 0.9659258262890683122, 1.000000000000000000, 0.9659258262890683122, 1.000000000000000000, 0.9659258262890683122, 1.000000000000000000, 0.9659258262890683122, 1.000000000000000000, 0.9659258262890683122, 1.000000000000000000, 0.9659258262890683122, 1.000000000000000000, 0.9659258262890683122, 1.000000000000000000, 0.9659258262890683122, 1.000000000000000000, 0.9659258262890683122, 1.000000000000000000, 0.9659258262890683122, 1.000000000000000000, 0.9659258262890683122, 1.000000000000000000, 0.9659258262890683122, 1.000000000000000000, 0.9659258262890683122, 1.000000000000000000, 0.9659258262890683122, 1.000000000000000000, 0.9659258262890683122, 1.000000000000000000, 0.9659258262890683122, 1.000000000000000000, 0.9659258262890683122, 1.000000000000000000, 0.9659258262890683122, 1.000000000000000000, 0.9659258262890683122, 1.000000000000000000, 0.9659258262890683122, 1.000000000000000000, 0.9659258262890683122, 1.000000000000000000, 0.9659258262890683122, 1.000000000000000000, 0.9659258262890683122, 1.000000000000000000, 0.9659258262890683122, 1.000000000000000000, 0.9659258262890683122, 1.000000000000000000, 0.9659258262890683122, 1.000000000000000000, 0.9659258262890683122, 1.000000000000000000, 0.9659258262890683122, 1.000000000000000000, 0.9659258262890683122, 1.000000000000000000, 0.9659258262890683122, 1.000000000000000000, 0.9659258262890683122, 1.000000000000000000, 0.9659258262890683122, 1.000000000000000000, 0.9659258262890683122, 1.000000000000000000, 0.9659258262890683122, 1.000000000000000000, 0.9659258262890683122, 1.000000000000000000, 0.9659258262890683122, 1.000000000000000000, 0.9659258262890683122, 1.000000000000000000, 0.9659258262890683122, 1.000000000000000000, 0.9659258262890683122, 1.000000000000000000, 0.9659258262890683122, 1.000000000000000000, 0.9659258262890683122, 1.000000000000000000, 0.9659258262890683122, 1.000000000000000000, 0.9659258262890683122, 1.000000000000000000, 0.9659258262890683122, 1.000000000000000000, 0.9659258262890683122, 1.000000000000000000, 0.9659258262890683122, 1.000000000000000000, 0.9659258262890683122, 1.000000000000000000, 0.9659258262890683122, 1.000000000000000000, 0.9659258262890683122, 1.000000000000000000, 0.9659258262890683122, 1.000000000000000000, 0.9659258262890683122, 1.000000000000000000, 0.9659258262890683122, 1.000000000000000000, 0.9659258262890683122, 1.000000000000000000, 0.9659258262890683122, 1.000000000000000000, 0.9659258262890683122, 1.000000000000000000, 0.9659258262890683122, 1.000000000000000000, 0.9659258262890683122, 1.000000000000000000, 0.9659258262890683122, 1.000000000000000000, 0.9659258262890683122, 1.000000000000000000, 0.9659258262890683122, 1.000000000000000000, 0.9659258262890683122, 1.000000000000000000, 0.9659258262890683122, 1.000000000000000000, 0.9659258262890683122, 1.000000000000000000, 0.9659258262890683122, 1.000000000000000000, 0.9659258262890683122, 1.000000000000000000, 0.9659258262890683122, 1.000000000000000000, 0.9659258262890683122, 1.000000000000000000, 0.9659258262890683122, 1.000000000000000000, 0.9659258262890683122, 1.000000000000000000, 0.9659258262890683122, 1.000000000000000000, 0.9659258262890683122, 1.000000000000000000, 0.9659258262890683122, 1.000000000000000000, 0.9659258262890683122, 1.000000000000000000, 0.9659258262890683122, 1.000000000000000000, 0.9659258262890683122, 1.000000000000000000, 0.9659258262890683122, 1.000000000000000000, 0.9659258262890683122, 1.000000000000000000, 0.9659258262890683122, 1.000000000000000000, 0.9659258262890683122, 1.000000000000000000, 0.9659258262890683122, 1.000000000000000000, 0.9659258262890683122, 1.000000000000000000, 0.9659258262890683122, 1.000000000000000000, 0.9659258262890683122, 1.000000000000000000, 0.9659258262890683122, 1.000000000000000000, 0.9659258262890683122, 1.000000000000000000, 0.9659258262890683122, 1.000000000000000000, 0.9659258262890683122, 1.000000000000000000, 0.9659258262890683122, 1.000000000000000000, 0.9659258262890683122, 1.000000000000000000, 0.9659258262890683122, 1.000000000000000000, 0.9659258262890683122, 1.000000000000000000, 0.9659258262890683122, 1.000000000000000000, 0.9659258262890683122, 1.000000000000000000, 0.9659258262890683122, 1.000000000000000000, 0.9659258262890683122, 1.000000000000000000, 0.9659258262890683122, 1.000000000000000000, 0.9659258262890683122, 1.000000000000000000, 0.9659258262890683122, 1.000000000000000000, 0.9659258262890683122, 1.000000000000000000, 0.9659258262890683122, 1.000000000000000000, 0.9659258262890683122, 1.000000000000000000, 0.9659258262890683122, 1.000000000000000000, 0.9659258262890683122, 1.000000000000000000, 0.9659258262890683122, 1.000000000000000000, 0.9659258262890683122, 1.000000000000000000, 0.9659258262890683122, 1.000000000000000000, 0.9659258262890683122, 1.000000000000000000, 0.9659258262890683122, 1.000000000000000000, 0.9659258262890683122, 1.000000000000000000, 0.9659258262890683122, 1.000000000000000000, 0.9659258262890683122, 1.000000000000000000, 0.9659258262890683122, 1.000000000000000000, 0.9659258262890683122, 1.000000000000000000, 0.9659258262890683122, 1.000000000000000000, 0.9659258262890683122, 1.000000000000000000, 0.9659258262890683122, 1.000000000000000000, 0.9659258262890683122, 1.000000000000000000, 0.9659258262890683122, 1.000000000000000000, 0.9659258262890683122, 1.000000000000000000, 0.9659258262890683122, 1.000000000000000000, 0.9659258262890683122, 1.000000000000000000, 0.9659258262890683122, 1.000000000000000000, 0.9659258262890683122, 1.000000000000000000, 0.9659258262890683122, 1.000000000000000000, 0.9659258262890683122, 1.000000000000000000, 0.9659258262890683122, 1.000000000000000000, 0.9659258262890683122, 1.000000000000000000, 0.9659258262890683122, 1.000000000000000000, 0.9659258262890683122, 1.000000000000000000, 0.9659258262890683122, 1.000000000000000000, 0.9659258262890683122, 1.000000000000000000, 0.9659258262890683122, 1.000000000000000000, 0.9659258262890683122, 1.000000000000000000, 0.9659258262890683122, 1.000000000000000000, 0.9659258262890683122, 1.000000000000000000, 0.9659258262890683122, 1.000000000000000000, 0.9659258262890683122, 1.000000000000000000, 0.9659258262890683122, 1.000000000000000000, 0.9659258262890683122, 1.000000000000000000, 0.9659258262890683122, 1.000000000000000000, 0.9659258262890683122, 1.000000000000000000, 0.9659258262890683122, 1.000000000000000000, 0.9659258262890683122, 1.000000000000000000, 0.9659258262890683122, 1.000000000000000000, 0.9659258262890683122, 1.000000000000000000, 0.9659258262890683122, 1.000000000000000000, 0.9659258262890683122, 1.000000000000000000, 0.9659258262890683122, 1.000000000000000000, 0.9659258262890683122, 1.000000000000000000, 0.9659258262890683122, 1.000000000000000000, 0.9659258262890683122, 1.000000000000000000, 0.9659258262890683122, 1.000000000000000000, 0.9659258262890683122, 1.000000000000000000, 0.9659258262890683122, 1.000000000000000000, 0.9659258262890683122, 1.000000000000000000, 0.9659258262890683122, 1.000000000000000000, 0.9659258262890683122, 1.000000000000000000, 0.9659258262890683122, 1.000000000000000000, 0.9659258262890683122, 1.000000000000000000, 0.9659258262890683122, 1.000000000000000000, 0.9659258262890683122, 1.000000000000000000, 0.9659258262890683122, 1.000000000000000000, 0.9659258262890683122, 1.000000000000000000, 0.9659258262890683122, 1.000000000000000000, 0.9659258262890683122, 1.000000000000000000, 0.9659258262890683122, 1.000000000000000000, 0.9659258262890683122, 1.000000000000000000, 0.9659258262890683122, 1.000000000000000000, 0.9659258262890683122, 1.000000000000000000, 0.9659258262890683122, 1.000000000000000000, 0.9659258262890683122, 1.000000000000000000, 0.9659258262890683122, 1.000000000000000000, 0.9659258262890683122, 1.000000000000000000, 0.9659258262890683122, 1.000000000000000000, 0.9659258262890683122, 1.000000000000000000, 0.9659258262890683122, 1.000000000000000000, 0.9659258262890683122, 1.000000000000000000, 0.9659258262890683122, 1.000000000000000000, 0.9659258262890683122, 1.000000000000000000, 0.9659258262890683122, 1.000000000000000000, 0.9659258262890683122, 1.000000000000000000, 0.9659258262890683122, 1.000000000000000000, 0.9659258262890683122, 1.000000000000000000, 0.9659258262890683122, 1.000000000000000000, 0.9659258262890683122, 1.000000000000000000, 0.9659258262890683122, 1.000000000000000000, 0.9659258262890683122, 1.000000000000000000, 0.9659258262890683122, 1.000000000000000000, 0.9659258262890683122, 1.000000000000000000),
 ( 1.000000000000000000, 0.9659258262890683122, 1.000000000000000000, 0.9659258262890683122, 1.000000000000000000, 0.9659258262890683122, 1.000000000000000000, 0.9659258262890683122, 1.000000000000000000, 0.9659258262890683122, 1.000000000000000000, 0.9659258262890683122, 1.000000000000000000, 0.9659258262890683122, 1.000000000000000000, 0.9659258262890683122, 1.000000000000000000, 0.9659258262890683122, 1.000000000000000000, 0.9659258262890683122, 1.000000000000000000, 0.9659258262890683122, 1.000000000000000000, 0.9659258262890683122, 1.000000000000000000, 0.9659258262890683122, 1.000000000000000000, 0.9659258262890683122, 1.000000000000000000, 0.9659258262890683122, 1.000000000000000000, 0.9659258262890683122, 1.000000000000000000, 0.9659258262890683122, 1.000000000000000000, 0.9659258262890683122, 1.000000000000000000, 0.9659258262890683122, 1.000000000000000000, 0.9659258262890683122, 1.000000000000000000, 0.9659258262890683122, 1.000000000000000000, 0.9659258262890683122, 1.000000000000000000, 0.9659258262890683122, 1.000000000000000000, 0.9659258262890683122, 1.000000000000000000, 0.9659258262890683122, 1.000000000000000000, 0.9659258262890683122, 1.000000000000000000, 0.9659258262890683122, 1.000000000000000000, 0.9659258262890683122, 1.000000000000000000, 0.9659258262890683122, 1.000000000000000000, 0.9659258262890683122, 1.000000000000000000, 0.9659258262890683122, 1.000000000000000000, 0.9659258262890683122, 1.000000000000000000, 0.9659258262890683122, 1.000000000000000000, 0.9659258262890683122, 1.000000000000000000, 0.9659258262890683122, 1.000000000000000000, 0.9659258262890683122, 1.000000000000000000, 0.9659258262890683122, 1.000000000000000000, 0.9659258262890683122, 1.000000000000000000, 0.9659258262890683122, 1.000000000000000000, 0.9659258262890683122, 1.000000000000000000, 0.9659258262890683122, 1.000000000000000000, 0.9659258262890683122, 1.000000000000000000, 0.9659258262890683122, 1.000000000000000000, 0.9659258262890683122, 1.000000000000000000, 0.9659258262890683122, 1.000000000000000000, 0.9659258262890683122, 1.000000000000000000, 0.9659258262890683122, 1.000000000000000000, 0.9659258262890683122, 1.000000000000000000, 0.9659258262890683122, 1.000000000000000000, 0.9659258262890683122, 1.000000000000000000, 0.9659258262890683122, 1.000000000000000000, 0.9659258262890683122, 1.000000000000000000, 0.9659258262890683122, 1.000000000000000000, 0.9659258262890683122, 1.000000000000000000, 0.9659258262890683122, 1.000000000000000000, 0.9659258262890683122, 1.000000000000000000, 0.9659258262890683122, 1.000000000000000000, 0.9659258262890683122, 1.000000000000000000, 0.9659258262890683122, 1.000000000000000000, 0.9659258262890683122, 1.000000000000000000, 0.9659258262890683122, 1.000000000000000000, 0.9659258262890683122, 1.000000000000000000, 0.9659258262890683122, 1.000000000000000000, 0.9659258262890683122, 1.000000000000000000, 0.9659258262890683122, 1.000000000000000000, 0.9659258262890683122, 1.000000000000000000, 0.9659258262890683122, 1.000000000000000000, 0.9659258262890683122, 1.000000000000000000, 0.9659258262890683122, 1.000000000000000000, 0.9659258262890683122, 1.000000000000000000, 0.9659258262890683122, 1.000000000000000000, 0.9659258262890683122, 1.000000000000000000, 0.9659258262890683122, 1.000000000000000000, 0.9659258262890683122, 1.000000000000000000, 0.9659258262890683122, 1.000000000000000000, 0.9659258262890683122, 1.000000000000000000, 0.9659258262890683122, 1.000000000000000000, 0.9659258262890683122, 1.000000000000000000, 0.9659258262890683122, 1.000000000000000000, 0.9659258262890683122, 1.000000000000000000, 0.9659258262890683122, 1.000000000000000000, 0.9659258262890683122, 1.000000000000000000, 0.9659258262890683122, 1.000000000000000000, 0.9659258262890683122, 1.000000000000000000, 0.9659258262890683122, 1.000000000000000000, 0.9659258262890683122, 1.000000000000000000, 0.9659258262890683122, 1.000000000000000000, 0.9659258262890683122, 1.000000000000000000, 0.9659258262890683122, 1.000000000000000000, 0.9659258262890683122, 1.000000000000000000, 0.9659258262890683122, 1.000000000000000000, 0.9659258262890683122, 1.000000000000000000, 0.9659258262890683122, 1.000000000000000000, 0.9659258262890683122, 1.000000000000000000, 0.9659258262890683122, 1.000000000000000000, 0.9659258262890683122, 1.000000000000000000, 0.9659258262890683122, 1.000000000000000000, 0.9659258262890683122, 1.000000000000000000, 0.9659258262890683122, 1.000000000000000000, 0.9659258262890683122, 1.000000000000000000, 0.9659258262890683122, 1.000000000000000000, 0.9659258262890683122, 1.000000000000000000, 0.9659258262890683122, 1.000000000000000000, 0.9659258262890683122, 1.000000000000000000, 0.9659258262890683122, 1.000000000000000000, 0.9659258262890683122, 1.000000000000000000, 0.9659258262890683122, 1.000000000000000000, 0.9659258262890683122, 1.000000000000000000, 0.9659258262890683122, 1.000000000000000000, 0.9659258262890683122, 1.000000000000000000, 0.9659258262890683122, 1.000000000000000000, 0.9659258262890683122, 1.000000000000000000, 0.9659258262890683122, 1.000000000000000000, 0.9659258262890683122, 1.000000000000000000, 0.9659258262890683122, 1.000000000000000000, 0.9659258262890683122, 1.000000000000000000, 0.9659258262890683122, 1.000000000000000000, 0.9659258262890683122, 1.000000000000000000, 0.9659258262890683122, 1.000000000000000000, 0.9659258262890683122, 1.000000000000000000, 0.9659258262890683122, 1.000000000000000000, 0.9659258262890683122, 1.000000000000000000, 0.9659258262890683122, 1.000000000000000000, 0.9659258262890683122, 1.000000000000000000, 0.9659258262890683122, 1.000000000000000000, 0.9659258262890683122, 1.000000000000000000, 0.9659258262890683122, 1.000000000000000000, 0.9659258262890683122, 1.000000000000000000, 0.9659258262890683122, 1.000000000000000000, 0.9659258262890683122, 1.000000000000000000, 0.9659258262890683122, 1.000000000000000000, 0.9659258262890683122, 1.000000000000000000, 0.9659258262890683122, 1.000000000000000000, 0.9659258262890683122, 1.000000000000000000, 0.9659258262890683122, 1.000000000000000000, 0.9659258262890683122, 1.000000000000000000, 0.9659258262890683122, 1.000000000000000000, 0.9659258262890683122, 1.000000000000000000, 0.9659258262890683122, 1.000000000000000000, 0.9659258262890683122, 1.000000000000000000, 0.9659258262890683122, 1.000000000000000000, 0.9659258262890683122, 1.000000000000000000, 0.9659258262890683122, 1.000000000000000000, 0.9659258262890683122, 1.000000000000000000, 0.9659258262890683122, 1.000000000000000000, 0.9659258262890683122, 1.000000000000000000, 0.9659258262890683122, 1.000000000000000000, 0.9659258262890683122, 1.000000000000000000, 0.9659258262890683122, 1.000000000000000000, 0.9659258262890683122, 1.000000000000000000, 0.9659258262890683122, 1.000000000000000000, 0.9659258262890683122, 1.000000000000000000, 0.9659258262890683122, 1.000000000000000000, 0.9659258262890683122, 1.000000000000000000, 0.9659258262890683122, 1.000000000000000000, 0.9659258262890683122, 1.000000000000000000, 0.9659258262890683122, 1.000000000000000000, 0.9659258262890683122, 1.000000000000000000, 0.9659258262890683122, 1.000000000000000000, 0.9659258262890683122, 1.000000000000000000, 0.9659258262890683122, 1.000000000000000000, 0.9659258262890683122, 1.000000000000000000, 0.9659258262890683122, 1.000000000000000000, 0.9659258262890683122, 1.000000000000000000, 0.9659258262890683122, 1.000000000000000000, 0.9659258262890683122, 1.000000000000000000, 0.9659258262890683122, 1.000000000000000000, 0.9659258262890683122, 1.000000000000000000, 0.9659258262890683122, 1.000000000000000000, 0.9659258262890683122, 1.000000000000000000, 0.9659258262890683122, 1.000000000000000000, 0.9659258262890683122, 1.000000000000000000, 0.9659258262890683122, 1.000000000000000000, 0.9659258262890683122, 1.000000000000000000, 0.9659258262890683122, 1.000000000000000000, 0.9659258262890683122, 1.000000000000000000, 0.9659258262890683122, 1.000000000000000000, 0.9659258262890683122, 1.000000000000000000, 0.9659258262890683122, 1.000000000000000000, 0.9659258262890683122, 1.000000000000000000, 0.9659258262890683122, 1.000000000000000000, 0.9659258262890683122, 1.000000000000000000, 0.9659258262890683122, 1.000000000000000000, 0.9659258262890683122, 1.000000000000000000, 0.9659258262890683122, 1.000000000000000000, 0.9659258262890683122, 1.000000000000000000, 0.9659258262890683122, 1.000000000000000000, 0.9659258262890683122, 1.000000000000000000, 0.9659258262890683122, 1.000000000000000000, 0.9659258262890683122, 1.000000000000000000, 0.9659258262890683122, 1.000000000000000000, 0.9659258262890683122, 1.000000000000000000, 0.9659258262890683122, 1.000000000000000000, 0.9659258262890683122, 1.000000000000000000, 0.9659258262890683122, 1.000000000000000000, 0.9659258262890683122, 1.000000000000000000, 0.9659258262890683122, 1.000000000000000000, 0.9659258262890683122, 1.000000000000000000, 0.9659258262890683122, 1.000000000000000000, 0.9659258262890683122, 1.000000000000000000, 0.9659258262890683122, 1.000000000000000000, 0.9659258262890683122, 1.000000000000000000, 0.9659258262890683122, 1.000000000000000000, 0.9659258262890683122, 1.000000000000000000, 0.9659258262890683122, 1.000000000000000000, 0.9659258262890683122, 1.000000000000000000, 0.9659258262890683122, 1.000000000000000000, 0.9659258262890683122, 1.000000000000000000, 0.9659258262890683122, 1.000000000000000000, 0.9659258262890683122, 1.000000000000000000, 0.9659258262890683122, 1.000000000000000000, 0.9659258262890683122, 1.000000000000000000, 0.9659258262890683122, 1.000000000000000000, 0.9659258262890683122, 1.000000000000000000, 0.9659258262890683122, 1.000000000000000000, 0.9659258262890683122, 1.000000000000000000, 0.9659258262890683122, 1.000000000000000000, 0.9659258262890683122, 1.000000000000000000, 0.9659258262890683122, 1.000000000000000000, 0.9659258262890683122, 1.000000000000000000, 0.9659258262890683122, 1.000000000000000000, 0.9659258262890683122, 1.000000000000000000, 0.9659258262890683122, 1.000000000000000000, 0.9659258262890683122, 1.000000000000000000, 0.9659258262890683122, 1.000000000000000000, 0.9659258262890683122, 1.000000000000000000, 0.9659258262890683122, 1.000000000000000000, 0.9659258262890683122, 1.000000000000000000, 0.9659258262890683122, 1.000000000000000000, 0.9659258262890683122, 1.000000000000000000, 0.9659258262890683122, 1.000000000000000000, 0.9659258262890683122, 1.000000000000000000, 0.9659258262890683122, 1.000000000000000000, 0.9659258262890683122, 1.000000000000000000, 0.9659258262890683122, 1.000000000000000000, 0.9659258262890683122, 1.000000000000000000, 0.9659258262890683122, 1.000000000000000000, 0.9659258262890683122, 1.000000000000000000, 0.9659258262890683122, 1.000000000000000000, 0.9659258262890683122, 1.000000000000000000, 0.9659258262890683122, 1.000000000000000000, 0.9659258262890683122, 1.000000000000000000, 0.9659258262890683122, 1.000000000000000000, 0.9659258262890683122, 1.000000000000000000, 0.9659258262890683122, 1.000000000000000000, 0.9659258262890683122, 1.000000000000000000, 0.9659258262890683122, 1.000000000000000000, 0.9659258262890683122, 1.000000000000000000, 0.9659258262890683122, 1.000000000000000000, 0.9659258262890683122, 1.000000000000000000, 0.9659258262890683122, 1.000000000000000000, 0.9659258262890683122, 1.000000000000000000, 0.9659258262890683122, 1.000000000000000000, 0.9659258262890683122, 1.000000000000000000, 0.9659258262890683122, 1.000000000000000000) ) ) 
 REPRESENTATION_ITEM ( '' )  SURFACE ( )  );
#28019=CARTESIAN_POINT ( 'NONE',  ( -0.9908136482939626788, 0.2952755905511811885, 0.1292274648535926551 ) ) ;
#28020=CARTESIAN_POINT ( 'NONE',  ( -1.653543307086613234, -0.1870078740157479769, 0.4822834645669291653 ) ) ;
#28022=CARTESIAN_POINT ( 'NONE',  ( 1.614173228346456712, 1.496062992125984037, -0.1372047244094475871 ) ) ;
#28023=ORIENTED_EDGE ( 'NONE', *, *, #13917, .F. ) ;
#28025=CARTESIAN_POINT ( 'NONE',  ( 0.8136482939632553313, 0.2306618581243848609, 0.2411417322834645549 ) ) ;
#28026=CARTESIAN_POINT ( 'NONE',  ( 1.522309711286089939, -0.5023911411419708095, -0.1820866141732282451 ) ) ;
#28027=EDGE_CURVE ( 'NONE', #74430, #43140, #26988, .T. ) ;
#28028=CARTESIAN_POINT ( 'NONE',  ( -1.246719160104985846, -0.3690944881889765550, -0.3153832671262227771 ) ) ;
#28029=CARTESIAN_POINT ( 'NONE',  ( -1.122047244094487306, 0.1660481256975883668, -0.3530559997133364547 ) ) ;
#28031=CARTESIAN_POINT ( 'NONE',  ( -0.9645669291338576645, 0.1012011053420775880, -0.2882089793578256898 ) ) ;
#28032=CARTESIAN_POINT ( 'NONE',  ( 1.030183727034121421, -0.05778040916215522460, 0.4822834645669289988 ) ) ;
#28033=CARTESIAN_POINT ( 'NONE',  ( -1.515748031496062076, 0.1660481256975883668, -0.3530559997133364547 ) ) ;
#28034=CARTESIAN_POINT ( 'NONE',  ( -0.2690288713910754526, 0.2952755905511810774, -0.1292274648535930714 ) ) ;
#28035=CARTESIAN_POINT ( 'NONE',  ( -0.3412073490813641308, -0.6046776061558807314, 0.2411417322834647770 ) ) ;
#28036=CARTESIAN_POINT ( 'NONE',  ( -1.154855643044618851, 0.2306618581243848609, 0.2411417322834645549 ) ) ;
#28038=CARTESIAN_POINT ( 'NONE',  ( 0.6299212598425204535, -0.1870078740157479769, 0.4822834645669291653 ) ) ;
#28040=CARTESIAN_POINT ( 'NONE',  ( -1.154855643044618851, 0.1283753931104748280, 0.1820866141732283561 ) ) ;
#28045=CARTESIAN_POINT ( 'NONE',  ( -1.627296587926508442, -0.6046776061558809534, -0.2411417322834644161 ) ) ;
#28046=CARTESIAN_POINT ( 'NONE',  ( -1.338582677165353729, -0.1870078740157479769, 0.4822834645669291653 ) ) ;
#28048=CARTESIAN_POINT ( 'NONE',  ( -1.384514435695537005, 0.2952755905511811885, 0.1292274648535926551 ) ) ;
#28050=CARTESIAN_POINT ( 'NONE',  ( -1.012036180893692183, 0.02791078216816064370, 0.4328096321851915285 ) ) ;
#28051=CARTESIAN_POINT ( 'NONE',  ( -0.3346456692913378217, 0.1660481256975883391, -0.3530559997133364547 ) ) ;
#28052=ADVANCED_FACE ( 'NONE', ( #44071 ), #12108, .F. ) ;
#28054=CARTESIAN_POINT ( 'NONE',  ( -0.09186351706036663400, -0.3690944881889763329, 0.3153832671262228327 ) ) ;
#28055=CARTESIAN_POINT ( 'NONE',  ( -0.6627296587926503335, -0.5511811023622046335, 0.09757992244046803654 ) ) ;
#28056=CARTESIAN_POINT ( 'NONE',  ( -1.384514435695537005, -0.6692913385826773087, -0.1292274648535924053 ) ) ;
#28058=CARTESIAN_POINT ( 'NONE',  ( 0.9908136482939640111, 0.2952755905511810774, -0.1292274648535930714 ) ) ;
#28059=CARTESIAN_POINT ( 'NONE',  ( -0.7808398950131222316, -0.3162353388693409650, -0.4822834645669289433 ) ) ;
#28062=CARTESIAN_POINT ( 'NONE',  ( -1.555118110236219930, -0.5400638737290845981, -0.3530559997133363437 ) ) ;
#28063=CARTESIAN_POINT ( 'NONE',  ( -1.410761154855642463, -0.08942795157527998196, 0.3641732283464567121 ) ) ;
#28064=DIRECTION ( 'NONE',  ( 1.000000000000000000, 0.000000000000000000, 0.000000000000000000 ) ) ;
#28069=CARTESIAN_POINT ( 'NONE',  ( -0.5314960629921250401, 0.1660481256975885056, 0.3530559997133364547 ) ) ;
#28070=CARTESIAN_POINT ( 'NONE',  ( -1.463254593175852492, 0.1771653543307087630, 0.09757992244046791164 ) ) ;
#28072=CARTESIAN_POINT ( 'NONE',  ( -0.7443564586553569340, 2.201272808259610692, -0.5309055118110235227 ) ) ;
#28073=CARTESIAN_POINT ( 'NONE',  ( -0.6426939841807746134, 0.004960608223778509643, -0.3437734562760191848 ) ) ;
#28074=CARTESIAN_POINT ( 'NONE',  ( -1.259842519685038686, -0.1870078740157479769, 0.4822834645669291653 ) ) ;
#28075=CARTESIAN_POINT ( 'NONE',  ( -0.2034120734908131112, -0.6692913385826773087, -0.1292274648535924053 ) ) ;
#28077=CARTESIAN_POINT ( 'NONE',  ( 0.4002624671916016896, -0.2845877964562161244, -0.3641732283464567121 ) ) ;
#28079=CARTESIAN_POINT ( 'NONE',  ( 0.4921259842519691285, -0.4536011799217368745, -0.2665933059059886201 ) ) ;
#28080=CARTESIAN_POINT ( 'NONE',  ( 0.7611548556430451917, -0.5023911411419708095, 0.1820866141732285504 ) ) ;
#28081=CARTESIAN_POINT ( 'NONE',  ( 0.9645669291338588858, 0.1660481256975885056, 0.3530559997133364547 ) ) ;
#28082=CARTESIAN_POINT ( 'NONE',  ( -0.4396325459317577122, -0.5511811023622048555, -0.09757992244046775898 ) ) ;
#28084=CARTESIAN_POINT ( 'NONE',  ( -1.227034120734907141, -0.6692913385826773087, -0.1292274648535924053 ) ) ;
#28085=CARTESIAN_POINT ( 'NONE',  ( -0.1181102362204717315, 0.1771653543307087630, 0.000000000000000000 ) ) ;
#28086=EDGE_CURVE ( 'NONE', #16126, #30161, #49569, .T. ) ;
#28087=CARTESIAN_POINT ( 'NONE',  ( -1.443569553805773564, 0.1283753931104746893, -0.1820866141732285504 ) ) ;
#28089=CARTESIAN_POINT ( 'NONE',  ( -0.8398950131233585692, 0.1283753931104748280, 0.1820866141732283561 ) ) ;
#28091=CARTESIAN_POINT ( 'NONE',  ( 0.1049868766404206816, 0.2306618581243848609, 0.2411417322834645549 ) ) ;
#28092=CARTESIAN_POINT ( 'NONE',  ( 1.469816272965879911, -0.5023911411419708095, 0.1820866141732285504 ) ) ;
#28094=CARTESIAN_POINT ( 'NONE',  ( 0.6102362204724416372, -0.4536011799217367080, 0.2665933059059888421 ) ) ;
#28095=CARTESIAN_POINT ( 'NONE',  ( -0.07217847769028813698, -0.2845877964562161244, -0.3641732283464567121 ) ) ;
#28096=CARTESIAN_POINT ( 'NONE',  ( -0.3346456692913377662, 0.1660481256975883668, -0.3530559997133364547 ) ) ;
#28097=CARTESIAN_POINT ( 'NONE',  ( -1.220472440944882386, 0.000000000000000000, 0.4445507791589061175 ) ) ;
#28098=CARTESIAN_POINT ( 'NONE',  ( -1.017060367454067249, -0.08942795157527998196, 0.3641732283464567121 ) ) ;
#28100=CARTESIAN_POINT ( 'NONE',  ( 0.5380577427821529035, -0.4281496062992124485, 0.4176697321401328655 ) ) ;
#28103=EDGE_CURVE ( 'NONE', #23065, #58545, #49979, .T. ) ;
#28104=CARTESIAN_POINT ( 'NONE',  ( 1.482939632545932307, 0.05413385826771626580, -0.4176697321401330321 ) ) ;
#28105=CARTESIAN_POINT ( 'NONE',  ( -0.3018372703412066094, -0.004921259842519576551, 0.3153832671262227771 ) ) ;
#28106=CARTESIAN_POINT ( 'NONE',  ( -0.01968503937007793844, -0.5400638737290844871, 0.3530559997133364547 ) ) ;
#28107=CARTESIAN_POINT ( 'NONE',  ( -1.397637795275589623, -0.5400638737290845981, -0.3530559997133363437 ) ) ;
#28108=CARTESIAN_POINT ( 'NONE',  ( 1.561679790026247350, 0.05413385826771626580, -0.4176697321401330321 ) ) ;
#28109=CARTESIAN_POINT ( 'NONE',  ( 1.299212598425197429, -0.6692913385826771977, 8.415575281601705876E-17 ) ) ;
#28110=CARTESIAN_POINT ( 'NONE',  ( -0.7152230971128602510, -0.08942795157528024563, -0.3641732283464568787 ) ) ;
#28115=CARTESIAN_POINT ( 'NONE',  ( 1.128608923884514947, 0.1283753931104748280, 0.1820866141732283561 ) ) ;
#28116=CARTESIAN_POINT ( 'NONE',  ( 0.4064735117398315944, 0.004960608223780119466, 0.3437734562760182411 ) ) ;
#28117=CARTESIAN_POINT ( 'NONE',  ( 0.9186351706036751663, -0.6046776061558807314, 0.2411417322834647770 ) ) ;
#28119=CARTESIAN_POINT ( 'NONE',  ( 1.128608923884515169, -0.5023911411419708095, -0.1820866141732282451 ) ) ;
#28120=CARTESIAN_POINT ( 'NONE',  ( 0.2559055118110243332, 0.1660481256975885056, 0.3530559997133364547 ) ) ;
#28121=CARTESIAN_POINT ( 'NONE',  ( -0.2887139107611542133, -0.6046776061558809534, -0.2411417322834644161 ) ) ;
#28122=CARTESIAN_POINT ( 'NONE',  ( 1.646981627296588035, -0.3162353388693405765, 0.4822834645669290543 ) ) ;
#28124=CARTESIAN_POINT ( 'NONE',  ( 0.2427821522309716595, -0.2845877964562161244, -0.3641732283464567121 ) ) ;
#28126=EDGE_LOOP ( 'NONE', ( #82376, #26606, #9619, #77399 ) ) ;
#28129=CARTESIAN_POINT ( 'NONE',  ( -0.5380577427821514602, -0.4281496062992127816, -0.4176697321401328100 ) ) ;
#28130=CARTESIAN_POINT ( 'NONE',  ( 1.227034120734908917, -0.6692913385826771977, 0.1292274648535927661 ) ) ;
#28131=CARTESIAN_POINT ( 'NONE',  ( 0.1246719160104994284, 0.2952755905511810774, -0.1292274648535930714 ) ) ;
#28132=CARTESIAN_POINT ( 'NONE',  ( -0.3215223097112853146, -0.08942795157528024563, -0.3641732283464568787 ) ) ;
#28133=CARTESIAN_POINT ( 'NONE',  ( 0.8595800524934390507, -0.3162353388693405765, 0.4822834645669290543 ) ) ;
#28134=CARTESIAN_POINT ( 'NONE',  ( -0.9514435695538050464, -0.05778040916215560624, -0.4822834645669293319 ) ) ;
#28135=CARTESIAN_POINT ( 'NONE',  ( -0.2690288713910754526, 0.2952755905511810774, -0.1292274648535930714 ) ) ;
#28136=CARTESIAN_POINT ( 'NONE',  ( -0.8858267716535425107, 0.1660481256975883668, -0.3530559997133364547 ) ) ;
#28137=CARTESIAN_POINT ( 'NONE',  ( 1.102362204724410155, -0.1870078740157479769, 0.4822834645669291653 ) ) ;
#28138=CARTESIAN_POINT ( 'NONE',  ( 0.7480314960629927956, -0.6692913385826771977, 8.415575281601705876E-17 ) ) ;
#28139=CARTESIAN_POINT ( 'NONE',  ( 0.9383202099737538715, -0.05778040916215560624, -0.4822834645669293319 ) ) ;
#28141=CARTESIAN_POINT ( 'NONE',  ( 0.1837270341207357105, -0.5023911411419708095, -0.1820866141732282451 ) ) ;
#28145=CARTESIAN_POINT ( 'NONE',  ( -0.7808398950131225646, -0.08942795157527998196, 0.3641732283464567121 ) ) ;
#28146=CARTESIAN_POINT ( 'NONE',  ( 0.1377952755905518800, 0.1660481256975883668, -0.3530559997133364547 ) ) ;
#28148=CARTESIAN_POINT ( 'NONE',  ( -0.1771653543307080136, -0.5400638737290844871, 0.3530559997133364547 ) ) ;
#28149=CARTESIAN_POINT ( 'NONE',  ( -0.4133858267716528645, 0.1660481256975883668, -0.3530559997133364547 ) ) ;
#28150=CARTESIAN_POINT ( 'NONE',  ( -1.496062992125983815, -0.1870078740157479769, 0.4822834645669291653 ) ) ;
#28152=CARTESIAN_POINT ( 'NONE',  ( -1.266404199475064773, -0.3162353388693405765, 0.4822834645669290543 ) ) ;
#28153=CARTESIAN_POINT ( 'NONE',  ( 1.272965879265092637, -0.3690944881889765550, -0.3153832671262227771 ) ) ;
#28154=CARTESIAN_POINT ( 'NONE',  ( -1.607611548556429737, 0.2952755905511810774, -0.1292274648535930714 ) ) ;
#28156=CARTESIAN_POINT ( 'NONE',  ( 0.6102362204724416372, -0.4536011799217367080, 0.2665933059059888421 ) ) ;
#28157=CARTESIAN_POINT ( 'NONE',  ( 0.2165354330708668673, -0.5400638737290844871, 0.3530559997133364547 ) ) ;
#28158=CARTESIAN_POINT ( 'NONE',  ( 0.2099737532808405305, -0.6046776061558807314, 0.2411417322834647770 ) ) ;
#28159=ORIENTED_EDGE ( 'NONE', *, *, #3251, .F. ) ;
#28161=CARTESIAN_POINT ( 'NONE',  ( -0.5905511811023615998, 0.2066929133858268208, 0.000000000000000000 ) ) ;
#28164=CARTESIAN_POINT ( 'NONE',  ( -0.5839895013123351797, 0.2952755905511810774, -0.1292274648535930714 ) ) ;
#28167=CARTESIAN_POINT ( 'NONE',  ( -1.646981627296586703, -0.08942795157527998196, 0.3641732283464567121 ) ) ;
#28168=CARTESIAN_POINT ( 'NONE',  ( 0.7545931758530188826, -0.6692913385826771977, 0.1292274648535927661 ) ) ;
#28169=CARTESIAN_POINT ( 'NONE',  ( 0.7545931758530189937, 0.2952755905511810774, -0.1292274648535930714 ) ) ;
#28170=CARTESIAN_POINT ( 'NONE',  ( -0.3871391076115476282, -0.08942795157527998196, 0.3641732283464567121 ) ) ;
#28171=CARTESIAN_POINT ( 'NONE',  ( -0.01968503937007793844, -0.5400638737290844871, 0.3530559997133364547 ) ) ;
#28173=CARTESIAN_POINT ( 'NONE',  ( -0.2493438320209966919, -0.3690944881889763329, 0.3153832671262228327 ) ) ;
#28174=CARTESIAN_POINT ( 'NONE',  ( -0.5052493438320203589, -0.6692913385826771977, 0.1292274648535927661 ) ) ;
#28176=CARTESIAN_POINT ( 'NONE',  ( -1.699475065616797398, 0.2952755905511811885, 0.1292274648535926551 ) ) ;
#28177=CARTESIAN_POINT ( 'NONE',  ( 0.1640419947506569498, -0.08942795157527998196, 0.3641732283464567121 ) ) ;
#28178=CARTESIAN_POINT ( 'NONE',  ( 1.679790026246720025, 0.1283753931104748280, 0.1820866141732283561 ) ) ;
#28179=CARTESIAN_POINT ( 'NONE',  ( -1.108923884514435132, -0.3162353388693405765, 0.4822834645669290543 ) ) ;
#28180=CARTESIAN_POINT ( 'NONE',  ( -0.6627296587926501115, 0.1771653543307087075, -0.09757992244046823083 ) ) ;
#28182=CARTESIAN_POINT ( 'NONE',  ( -1.338582677165353729, -0.1870078740157480879, -0.4822834645669291653 ) ) ;
#28183=CARTESIAN_POINT ( 'NONE',  ( -0.6430446194225712953, 0.05413385826771626580, -0.4176697321401330321 ) ) ;
#28184=CARTESIAN_POINT ( 'NONE',  ( -0.1377952755905504645, -0.5400638737290845981, -0.3530559997133363437 ) ) ;
#28188=CARTESIAN_POINT ( 'NONE',  ( 0.5314960629921267055, -0.4536011799217367080, 0.2665933059059888421 ) ) ;
#28189=CARTESIAN_POINT ( 'NONE',  ( 1.049868766404200127, -0.6046776061558809534, -0.2411417322834644161 ) ) ;
#28190=CARTESIAN_POINT ( 'NONE',  ( -1.043307086614172707, 0.07958543189024071263, -0.2665933059059888421 ) ) ;
#28191=CARTESIAN_POINT ( 'NONE',  ( 1.332020997375329197, -0.3162353388693405765, 0.4822834645669290543 ) ) ;
#28192=CARTESIAN_POINT ( 'NONE',  ( -1.450131233595799651, -0.5511811023622046335, 0.09757992244046803654 ) ) ;
#28193=CARTESIAN_POINT ( 'NONE',  ( -0.3740157480314953431, -0.5400638737290845981, -0.3530559997133363437 ) ) ;
#28194=CARTESIAN_POINT ( 'NONE',  ( 0.2887139107611556010, 0.1283753931104746893, -0.1820866141732285504 ) ) ;
#28196=CARTESIAN_POINT ( 'NONE',  ( 0.5708661417322841158, -0.4536011799217368745, -0.2665933059059886201 ) ) ;
#28197=CARTESIAN_POINT ( 'NONE',  ( 0.2034120734908144990, -0.6692913385826771977, 0.1292274648535927661 ) ) ;
#28199=CARTESIAN_POINT ( 'NONE',  ( -0.5446194225721777693, -0.3162353388693409650, -0.4822834645669289433 ) ) ;
#28201=CARTESIAN_POINT ( 'NONE',  ( 1.167979002624672580, -0.004921259842519870586, -0.3153832671262229437 ) ) ;
#28202=CARTESIAN_POINT ( 'NONE',  ( 0.05249343832021075018, -0.6046776061558807314, 0.2411417322834647770 ) ) ;
#28203=CARTESIAN_POINT ( 'NONE',  ( -0.4921259842519677963, 0.1660481256975883668, -0.3530559997133364547 ) ) ;
#28204=CARTESIAN_POINT ( 'NONE',  ( -0.4855643044619415427, -0.004921259842519870586, -0.3153832671262229437 ) ) ;
#28205=CARTESIAN_POINT ( 'NONE',  ( -1.586052503253848167, 1.023622047244095556, 0.1653254495020564929 ) ) ;
#28206=CARTESIAN_POINT ( 'NONE',  ( -0.03937007874015669567, 0.1771653543307087630, 0.000000000000000000 ) ) ;
#28207=CARTESIAN_POINT ( 'NONE',  ( 0.4002624671916016896, -0.05778040916215522460, 0.4822834645669289988 ) ) ;
#28208=CARTESIAN_POINT ( 'NONE',  ( -0.7414698162729651543, 0.1771653543307087075, -0.09757992244046823083 ) ) ;
#28210=CARTESIAN_POINT ( 'NONE',  ( -1.266404199475064773, -0.05778040916215560624, -0.4822834645669293319 ) ) ;
#28213=CARTESIAN_POINT ( 'NONE',  ( -1.115485564304461219, -0.3690944881889763329, 0.3153832671262228327 ) ) ;
#28214=CARTESIAN_POINT ( 'NONE',  ( -0.1115485564304456306, 0.2952755905511810774, -0.1292274648535930714 ) ) ;
#28216=CARTESIAN_POINT ( 'NONE',  ( -0.7020997375328074108, -0.05778040916215522460, 0.4822834645669289988 ) ) ;
#28218=CARTESIAN_POINT ( 'NONE',  ( 1.292650918635171564, -0.6692913385826773087, -0.1292274648535924053 ) ) ;
#28219=CARTESIAN_POINT ( 'NONE',  ( 0.6758530183727039509, -0.6692913385826771977, 0.1292274648535927661 ) ) ;
#28220=CARTESIAN_POINT ( 'NONE',  ( -0.2489931967792003153, 0.004960608223781096116, -0.3437734562760177970 ) ) ;
#28223=B_SPLINE_CURVE_WITH_KNOTS ( 'NONE', 3,
 ( #20247, #45896, #47152, #15192 ),
 .UNSPECIFIED., .F., .F.,
 ( 4, 4 ),
 ( 0.02768037499106720811, 0.02925281078410804994 ),
 .UNSPECIFIED. ) ;
#28224=CARTESIAN_POINT ( 'NONE',  ( -1.601049868766403650, -0.6046776061558807314, 0.2411417322834647770 ) ) ;
#28227=CARTESIAN_POINT ( 'NONE',  ( -0.4724409448818890911, -0.1870078740157480601, -0.3641732283464567677 ) ) ;
#28230=CARTESIAN_POINT ( 'NONE',  ( 0.7086614173228352742, -0.1870078740157480879, -0.4822834645669291653 ) ) ;
#28231=CARTESIAN_POINT ( 'NONE',  ( -0.05905511811023545637, -0.5400638737290845981, -0.3530559997133363437 ) ) ;
#28232=CARTESIAN_POINT ( 'NONE',  ( -0.8923884514435688198, -0.6046776061558807314, 0.2411417322834647770 ) ) ;
#28233=CARTESIAN_POINT ( 'NONE',  ( 1.450131233595801428, -0.6692913385826773087, -0.1292274648535924053 ) ) ;
#28234=CARTESIAN_POINT ( 'NONE',  ( -0.7611548556430438595, -0.5023911411419708095, -0.1820866141732282451 ) ) ;
#28236=CARTESIAN_POINT ( 'NONE',  ( 0.4133858267716541968, 0.1660481256975885056, 0.3530559997133364547 ) ) ;
#28237=CARTESIAN_POINT ( 'NONE',  ( 0.3740157480314966754, 0.07958543189024071263, -0.2665933059059888421 ) ) ;
#28238=CARTESIAN_POINT ( 'NONE',  ( -0.6627296587926501115, 0.2952755905511810774, -0.1292274648535930714 ) ) ;
#28240=CARTESIAN_POINT ( 'NONE',  ( -1.207349081364828436, -0.6046776061558807314, 0.2411417322834647770 ) ) ;
#28242=CARTESIAN_POINT ( 'NONE',  ( 0.9251968503937015864, 0.1660481256975883668, -0.3530559997133364547 ) ) ;
#28243=CARTESIAN_POINT ( 'NONE',  ( 1.141732283464567788, -0.5511811023622047445, 6.969142054262312111E-17 ) ) ;
#28244=ORIENTED_EDGE ( 'NONE', *, *, #73800, .F. ) ;
#28246=CARTESIAN_POINT ( 'NONE',  ( -0.3674540682414689785, 0.2306618581243848609, 0.2411417322834645549 ) ) ;
#28247=ORIENTED_EDGE ( 'NONE', *, *, #43470, .T. ) ;
#28248=CARTESIAN_POINT ( 'NONE',  ( 0.3477690288713918276, 0.1771653543307087630, 0.09757992244046791164 ) ) ;
#28249=CARTESIAN_POINT ( 'NONE',  ( -1.397637795275589623, 0.1660481256975885056, 0.3530559997133364547 ) ) ;
#28250=CARTESIAN_POINT ( 'NONE',  ( 0.8202099737532813073, 0.2952755905511811885, 0.1292274648535926551 ) ) ;
#28251=CARTESIAN_POINT ( 'NONE',  ( 0.9842519685039375910, 0.2952755905511811885, 0.000000000000000000 ) ) ;
#28252=CARTESIAN_POINT ( 'NONE',  ( -0.3280839895013117347, -0.4281496062992124485, 0.4176697321401328655 ) ) ;
#28253=CARTESIAN_POINT ( 'NONE',  ( -0.2624671916010490880, -0.6046776061558807314, 0.2411417322834647770 ) ) ;
#28255=CARTESIAN_POINT ( 'NONE',  ( -1.430446194225721390, -0.4281496062992124485, 0.4176697321401328655 ) ) ;
#28256=CARTESIAN_POINT ( 'NONE',  ( -0.6496062992125976043, 0.1660481256975883668, -0.3530559997133364547 ) ) ;
#28257=CARTESIAN_POINT ( 'NONE',  ( -0.4199475065616791736, -0.5023911411419708095, 0.1820866141732285504 ) ) ;
#28258=CARTESIAN_POINT ( 'NONE',  ( 1.108923884514436686, -0.3162353388693409650, -0.4822834645669289433 ) ) ;
#28260=CARTESIAN_POINT ( 'NONE',  ( -0.8333333333333323711, -0.6692913385826773087, -0.1292274648535924053 ) ) ;
#28262=CARTESIAN_POINT ( 'NONE',  ( 0.8136482939632553313, 0.2306618581243848609, 0.2411417322834645549 ) ) ;
#28265=CARTESIAN_POINT ( 'NONE',  ( -0.05905511811023545637, 0.1660481256975885056, 0.3530559997133364547 ) ) ;
#28266=CARTESIAN_POINT ( 'NONE',  ( -1.345144356955379816, -0.2845877964562159024, 0.3641732283464567677 ) ) ;
#28267=CARTESIAN_POINT ( 'NONE',  ( 1.108923884514436686, -0.2845877964562161244, -0.3641732283464567121 ) ) ;
#28268=CARTESIAN_POINT ( 'NONE',  ( -1.603475055217291612, 0.7793870273546338323, 0.04573490813648253134 ) ) ;
#28270=CARTESIAN_POINT ( 'NONE',  ( 1.135170603674541256, -0.5511811023622048555, -0.09757992244046775898 ) ) ;
#28271=CARTESIAN_POINT ( 'NONE',  ( 0.7742782152230978099, -0.4281496062992124485, 0.4176697321401328655 ) ) ;
#28273=CARTESIAN_POINT ( 'NONE',  ( -0.4527559055118102749, 0.1660481256975885056, 0.3530559997133364547 ) ) ;
#28275=CARTESIAN_POINT ( 'NONE',  ( 1.318897637795276356, 0.07958543189024071263, -0.2665933059059888421 ) ) ;
#28276=CARTESIAN_POINT ( 'NONE',  ( -0.2624671916010490880, 0.2306618581243847221, -0.2411417322834647770 ) ) ;
#28278=CARTESIAN_POINT ( 'NONE',  ( 1.069553805774278832, 0.2952755905511810774, -0.1292274648535930714 ) ) ;
#28279=CARTESIAN_POINT ( 'NONE',  ( -0.06561679790026180015, -0.4281496062992127816, -0.4176697321401328100 ) ) ;
#28280=CARTESIAN_POINT ( 'NONE',  ( 0.6233595800524942554, -0.08942795157528024563, -0.3641732283464568787 ) ) ;
#28282=CARTESIAN_POINT ( 'NONE',  ( 0.6102362204724416372, 0.07958543189024071263, -0.2665933059059888421 ) ) ;
#28283=CARTESIAN_POINT ( 'NONE',  ( -1.574803149606298192, -0.1870078740157480879, -0.4822834645669291653 ) ) ;
#28285=CARTESIAN_POINT ( 'NONE',  ( 0.9186351706036752773, 0.2306618581243847221, -0.2411417322834647770 ) ) ;
#28287=CARTESIAN_POINT ( 'NONE',  ( 1.686351706036745890, 0.1771653543307087630, 0.09757992244046791164 ) ) ;
#28288=CARTESIAN_POINT ( 'NONE',  ( 0.08874907683610111508, -2.191421614605370878E-15, 0.4445507791589071167 ) ) ;
#28289=CARTESIAN_POINT ( 'NONE',  ( 0.1574803149606306130, -0.1870078740157479769, 0.3641732283464567677 ) ) ;
#28290=CARTESIAN_POINT ( 'NONE',  ( 0.1312335958005257930, 0.2306618581243847221, -0.2411417322834647770 ) ) ;
#28292=CARTESIAN_POINT ( 'NONE',  ( 1.601049868766404982, -0.5023911411419708095, -0.1820866141732282451 ) ) ;
#28293=CARTESIAN_POINT ( 'NONE',  ( -1.515748031496062076, 0.07958543189024071263, -0.2665933059059888421 ) ) ;
#28294=CARTESIAN_POINT ( 'NONE',  ( -1.259842519685038686, -0.1870078740157479769, 0.4822834645669291653 ) ) ;
#28295=CARTESIAN_POINT ( 'NONE',  ( 0.5577427821522316087, -0.05778040916215522460, 0.4822834645669289988 ) ) ;
#28296=CARTESIAN_POINT ( 'NONE',  ( 1.397637795275591177, 0.1660481256975883668, -0.3530559997133364547 ) ) ;
#28298=CARTESIAN_POINT ( 'NONE',  ( 0.3805774278215230400, 0.05413385826771626580, -0.4176697321401330321 ) ) ;
#28300=CARTESIAN_POINT ( 'NONE',  ( 1.168682819302787168, 2.409604939980833412E-17, -0.3464511005275205946 ) ) ;
#28301=CARTESIAN_POINT ( 'NONE',  ( 0.9514435695538062676, -0.3162353388693409650, -0.4822834645669289433 ) ) ;
#28302=CARTESIAN_POINT ( 'NONE',  ( -1.607611548556429737, -0.5511811023622046335, 0.09757992244046803654 ) ) ;
#28303=CARTESIAN_POINT ( 'NONE',  ( 1.194225721784777594, -0.004921259842519576551, 0.3153832671262227771 ) ) ;
#28304=CARTESIAN_POINT ( 'NONE',  ( -1.640419947506561060, -0.004921259842519576551, 0.3153832671262227771 ) ) ;
#28305=CARTESIAN_POINT ( 'NONE',  ( -0.7086614173228339419, -0.1870078740157479769, 0.3641732283464567677 ) ) ;
#28307=CARTESIAN_POINT ( 'NONE',  ( 0.6758530183727039509, 0.1771653543307087075, -0.09757992244046823083 ) ) ;
#28308=CARTESIAN_POINT ( 'NONE',  ( 0.09842519685039434474, 0.1660481256975885056, 0.3530559997133364547 ) ) ;
#28309=CARTESIAN_POINT ( 'NONE',  ( 0.6036745406824153282, -0.6046776061558807314, 0.2411417322834647770 ) ) ;
#28310=B_SPLINE_CURVE_WITH_KNOTS ( 'NONE', 3,
 ( #46058, #20407, #77234, #52368 ),
 .UNSPECIFIED., .F., .F.,
 ( 4, 4 ),
 ( 1.999999999910059834E-07, 0.006970199999999936863 ),
 .UNSPECIFIED. ) ;
#28311=CARTESIAN_POINT ( 'NONE',  ( -0.3740157480314953431, 0.1660481256975885056, 0.3530559997133364547 ) ) ;
#28312=CARTESIAN_POINT ( 'NONE',  ( 0.3346456692913390985, 0.07958543189024085140, 0.2665933059059887866 ) ) ;
#28314=CARTESIAN_POINT ( 'NONE',  ( 1.017060367454068581, -0.05778040916215560624, -0.4822834645669293319 ) ) ;
#28316=CARTESIAN_POINT ( 'NONE',  ( -0.9055118110236215490, 0.2952755905511811885, 0.000000000000000000 ) ) ;
#28317=CARTESIAN_POINT ( 'NONE',  ( -1.574803149606298636, -0.1870078740157479769, 0.3641732283464567677 ) ) ;
#28320=CARTESIAN_POINT ( 'NONE',  ( -0.9645669291338575535, 0.1660481256975883668, -0.3530559997133364547 ) ) ;
#28321=CARTESIAN_POINT ( 'NONE',  ( 0.07217847769028949700, -0.05778040916215560624, -0.4822834645669293319 ) ) ;
#28324=ORIENTED_EDGE ( 'NONE', *, *, #24847, .T. ) ;
#28325=CARTESIAN_POINT ( 'NONE',  ( 0.7677165354330716118, 0.07958543189024071263, -0.2665933059059888421 ) ) ;
#28327=CARTESIAN_POINT ( 'NONE',  ( 1.069553805774278610, -0.6692913385826771977, 0.1292274648535927661 ) ) ;
#28329=CARTESIAN_POINT ( 'NONE',  ( -1.522309711286088607, 0.1283753931104746893, -0.1820866141732285504 ) ) ;
#28330=CARTESIAN_POINT ( 'NONE',  ( 1.515748031496063408, 0.1660481256975885056, 0.3530559997133364547 ) ) ;
#28331=CARTESIAN_POINT ( 'NONE',  ( -1.535433070866141225, 0.2952755905511811885, 0.000000000000000000 ) ) ;
#28333=CARTESIAN_POINT ( 'NONE',  ( 8.195543980992789655E-16, -0.1870078740157480879, -0.4822834645669291653 ) ) ;
#28334=CARTESIAN_POINT ( 'NONE',  ( -0.4658792650918627265, -0.08942795157527998196, 0.3641732283464567121 ) ) ;
#28335=CARTESIAN_POINT ( 'NONE',  ( 0.9842519685039375910, 0.2952755905511811885, 0.000000000000000000 ) ) ;
#28337=CARTESIAN_POINT ( 'NONE',  ( -0.1443569553805768291, 0.05413385826771666132, 0.4176697321401328100 ) ) ;
#28341=CARTESIAN_POINT ( 'NONE',  ( 0.8202099737532814183, -0.6692913385826773087, -0.1292274648535924053 ) ) ;
#28342=CARTESIAN_POINT ( 'NONE',  ( -0.01968503937007793844, -0.5400638737290844871, 0.3530559997133364547 ) ) ;
#28343=CARTESIAN_POINT ( 'NONE',  ( -0.9383202099737524282, -0.3162353388693409650, -0.4822834645669289433 ) ) ;
#28344=CARTESIAN_POINT ( 'NONE',  ( 1.555118110236221041, -0.5400638737290844871, 0.3530559997133364547 ) ) ;
#28345=CARTESIAN_POINT ( 'NONE',  ( 0.8333333333333340365, -0.6692913385826771977, 0.1292274648535927661 ) ) ;
#28347=CARTESIAN_POINT ( 'NONE',  ( -0.4790026246719154557, -0.3162353388693405765, 0.4822834645669290543 ) ) ;
#28348=CARTESIAN_POINT ( 'NONE',  ( 0.7545931758530189937, 0.2952755905511810774, -0.1292274648535930714 ) ) ;
#28349=CARTESIAN_POINT ( 'NONE',  ( -0.1115485564304453947, -0.6692913385826771977, 0.1292274648535927661 ) ) ;
#28350=CARTESIAN_POINT ( 'NONE',  ( 0.5314960629921267055, -0.4536011799217367080, 0.2665933059059888421 ) ) ;
#28351=CARTESIAN_POINT ( 'NONE',  ( -1.174540682414697335, -0.3162353388693409650, -0.4822834645669289433 ) ) ;
#28353=CARTESIAN_POINT ( 'NONE',  ( 0.5446194225721792126, -0.05778040916215560624, -0.4822834645669293319 ) ) ;
#28354=( CONVERSION_BASED_UNIT ( 'INCH', #54433 ) LENGTH_UNIT ( ) NAMED_UNIT ( #81973 ) );
#28357=ORIENTED_EDGE ( 'NONE', *, *, #66673, .T. ) ;
#28358=CARTESIAN_POINT ( 'NONE',  ( 1.318897637795276356, -0.5400638737290844871, 0.3530559997133364547 ) ) ;
#28359=CARTESIAN_POINT ( 'NONE',  ( 0.4921259842519691285, 0.07958543189024085140, 0.2665933059059887866 ) ) ;
#28360=CARTESIAN_POINT ( 'NONE',  ( 0.5708661417322842269, 0.1660481256975885056, 0.3530559997133364547 ) ) ;
#28365=CARTESIAN_POINT ( 'NONE',  ( -0.9711286089238838626, 0.2306618581243847221, -0.2411417322834647770 ) ) ;
#28366=CARTESIAN_POINT ( 'NONE',  ( -0.8136482939632537770, -0.6046776061558807314, 0.2411417322834647770 ) ) ;
#28367=CARTESIAN_POINT ( 'NONE',  ( 1.233595800524935227, -0.6046776061558807314, 0.2411417322834647770 ) ) ;
#28370=CARTESIAN_POINT ( 'NONE',  ( -1.607611548556429737, -0.6692913385826771977, 0.1292274648535927661 ) ) ;
#28374=CARTESIAN_POINT ( 'NONE',  ( -1.312335958005248715, 0.1283753931104748280, 0.1820866141732283561 ) ) ;
#28376=CARTESIAN_POINT ( 'NONE',  ( 0.2690288713910767848, 0.2952755905511811885, 0.1292274648535926551 ) ) ;
#28377=CARTESIAN_POINT ( 'NONE',  ( 1.391076115485564868, 0.2306618581243847221, -0.2411417322834647770 ) ) ;
#28379=CARTESIAN_POINT ( 'NONE',  ( -0.6561679790026240244, -0.5023911411419708095, 0.1820866141732285504 ) ) ;
#28380=( BOUNDED_CURVE ( )  B_SPLINE_CURVE ( 2, ( #49604, #75711, #30248, #43685, #4170, #10904, #18052, #36562, #82434, #11742, #81624, #75298, #50420 ),
 .UNSPECIFIED., .F., .F. ) 
 B_SPLINE_CURVE_WITH_KNOTS ( ( 3, 2, 2, 2, 2, 2, 3 ),
 ( 0.4006038219075281348, 0.4015151515151514916, 0.4053030303030302761, 0.4090909090909091161, 0.4128787878787879007, 0.4166666666666666852, 0.4175779962742901530 ),
 .UNSPECIFIED. ) 
 CURVE ( )  GEOMETRIC_REPRESENTATION_ITEM ( )  RATIONAL_B_SPLINE_CURVE ( ( 0.9875488213027530104, 0.9918020599134685922, 1.000000000000000000, 0.9659258262890683122, 1.000000000000000000, 0.9659258262890683122, 1.000000000000000000, 0.9659258262890683122, 1.000000000000000000, 0.9659258262890683122, 1.000000000000000000, 0.9918020599134675930, 0.9875488213027519002 ) ) 
 REPRESENTATION_ITEM ( '' )  );
#28381=CARTESIAN_POINT ( 'NONE',  ( 0.9842519685039378130, -0.6692913385826771977, 8.415575281601705876E-17 ) ) ;
#28382=CARTESIAN_POINT ( 'NONE',  ( 1.450131233595801428, 0.1771653543307087630, 0.09757992244046791164 ) ) ;
#28384=CARTESIAN_POINT ( 'NONE',  ( -0.8661417322834640276, -0.1870078740157480601, -0.3641732283464567677 ) ) ;
#28385=CARTESIAN_POINT ( 'NONE',  ( 1.181102362204725198, -0.1870078740157479769, 0.4822834645669291653 ) ) ;
#28387=CARTESIAN_POINT ( 'NONE',  ( 0.3346456692913390985, 0.1660481256975885056, 0.3530559997133364547 ) ) ;
#28388=CARTESIAN_POINT ( 'NONE',  ( -1.102362204724408601, -0.1870078740157480601, -0.3641732283464567677 ) ) ;
#28389=CARTESIAN_POINT ( 'NONE',  ( -0.3083989501312330295, -0.08942795157527998196, 0.3641732283464567121 ) ) ;
#28391=CARTESIAN_POINT ( 'NONE',  ( -0.3871391076115479057, -0.3162353388693409650, -0.4822834645669289433 ) ) ;
#28392=CARTESIAN_POINT ( 'NONE',  ( -1.417322834645668772, -0.1870078740157480601, -0.3641732283464567677 ) ) ;
#28394=CARTESIAN_POINT ( 'NONE',  ( 0.4855643044619428750, 0.05413385826771666132, 0.4176697321401328100 ) ) ;
#28395=EDGE_CURVE ( 'NONE', #30126, #36535, #13538, .T. ) ;
#28398=CARTESIAN_POINT ( 'NONE',  ( -0.9973753280839886548, -0.6046776061558809534, -0.2411417322834644161 ) ) ;
#28399=CARTESIAN_POINT ( 'NONE',  ( -0.06561679790026180015, -0.3690944881889765550, -0.3153832671262227771 ) ) ;
#28400=CARTESIAN_POINT ( 'NONE',  ( -1.286089238845143479, 0.2306618581243847221, -0.2411417322834647770 ) ) ;
#28401=CARTESIAN_POINT ( 'NONE',  ( -0.07874015748031421014, -0.1870078740157479769, 0.4822834645669291653 ) ) ;
#28402=CARTESIAN_POINT ( 'NONE',  ( 0.5052493438320218022, -0.5511811023622048555, -0.09757992244046775898 ) ) ;
#28403=CARTESIAN_POINT ( 'NONE',  ( -0.6627296587926503335, -0.5511811023622046335, 0.09757992244046803654 ) ) ;
#28404=CARTESIAN_POINT ( 'NONE',  ( -1.200787401574802349, 0.1660481256975883668, -0.3530559997133364547 ) ) ;
#28405=CARTESIAN_POINT ( 'NONE',  ( 1.607611548556431069, 0.1771653543307087630, 0.09757992244046791164 ) ) ;
#28406=CARTESIAN_POINT ( 'NONE',  ( 1.194225721784777594, 0.05413385826771666132, 0.4176697321401328100 ) ) ;
#28407=CYLINDRICAL_SURFACE ( 'NONE', #74386, 1.181102362204724310 ) ;
#28408=CARTESIAN_POINT ( 'NONE',  ( 0.8398950131233602345, -0.5023911411419708095, 0.1820866141732285504 ) ) ;
#28409=CARTESIAN_POINT ( 'NONE',  ( 0.7349081364829403995, 0.2306618581243848609, 0.2411417322834645549 ) ) ;
#28411=CARTESIAN_POINT ( 'NONE',  ( 1.417322834645670104, -0.1870078740157479769, 0.3641732283464567677 ) ) ;
#28414=CARTESIAN_POINT ( 'NONE',  ( -1.194225721784776262, -0.3690944881889763329, 0.3153832671262228327 ) ) ;
#28415=CARTESIAN_POINT ( 'NONE',  ( -0.4986876640419939388, 0.2306618581243847221, -0.2411417322834647770 ) ) ;
#28416=CARTESIAN_POINT ( 'NONE',  ( 0.1640419947506569498, -0.05778040916215522460, 0.4822834645669289988 ) ) ;
#28417=CARTESIAN_POINT ( 'NONE',  ( -1.587926509186350810, -0.3690944881889763329, 0.3153832671262228327 ) ) ;
#28419=CARTESIAN_POINT ( 'NONE',  ( -1.417322834645668772, -0.1870078740157479769, 0.4822834645669291653 ) ) ;
#28420=CARTESIAN_POINT ( 'NONE',  ( 0.4527559055118117182, 0.1660481256975883668, -0.3530559997133364547 ) ) ;
#28421=CARTESIAN_POINT ( 'NONE',  ( -0.1181102362204717315, -0.6692913385826771977, 8.415575281601705876E-17 ) ) ;
#28422=CARTESIAN_POINT ( 'NONE',  ( 1.003937007874016185, 0.1660481256975883668, -0.3530559997133364547 ) ) ;
#28423=CARTESIAN_POINT ( 'NONE',  ( 1.509186351706037543, 0.05413385826771666132, 0.4176697321401328100 ) ) ;
#28429=CARTESIAN_POINT ( 'NONE',  ( -0.1509186351706028884, -0.08942795157527998196, 0.3641732283464567121 ) ) ;
#28431=CARTESIAN_POINT ( 'NONE',  ( -0.2624671916010490880, 0.2306618581243847221, -0.2411417322834647770 ) ) ;
#28432=CARTESIAN_POINT ( 'NONE',  ( 0.7217847769028878924, -0.4281496062992127816, -0.4176697321401328100 ) ) ;
#28434=CARTESIAN_POINT ( 'NONE',  ( -0.2427821522309703550, -0.2845877964562159024, 0.3641732283464567677 ) ) ;
#28435=CARTESIAN_POINT ( 'NONE',  ( -0.9580052493438311334, 0.05413385826771626580, -0.4176697321401330321 ) ) ;
#28436=CARTESIAN_POINT ( 'NONE',  ( 1.463254593175853824, 0.2952755905511810774, -0.1292274648535930714 ) ) ;
#28438=CARTESIAN_POINT ( 'NONE',  ( 1.115485564304462551, 0.05413385826771666132, 0.4176697321401328100 ) ) ;
#28439=VERTEX_POINT ( 'NONE', #52461 ) ;
#28441=CARTESIAN_POINT ( 'NONE',  ( 0.9580052493438326877, 0.05413385826771666132, 0.4176697321401328100 ) ) ;
#28442=CARTESIAN_POINT ( 'NONE',  ( -1.646981627296586703, -0.3162353388693409650, -0.4822834645669289433 ) ) ;
#28443=CARTESIAN_POINT ( 'NONE',  ( -1.397637795275589623, -0.4536011799217368745, -0.2665933059059886201 ) ) ;
#28444=CARTESIAN_POINT ( 'NONE',  ( -1.030183727034119867, -0.3162353388693405765, 0.4822834645669290543 ) ) ;
#28446=CARTESIAN_POINT ( 'NONE',  ( 1.191111281560510715, -4.927456884911482678E-16, 0.4445507791589062840 ) ) ;
#28447=CARTESIAN_POINT ( 'NONE',  ( 1.082677165354331228, 0.1660481256975883668, -0.3530559997133364547 ) ) ;
#28449=CARTESIAN_POINT ( 'NONE',  ( -0.1574803149606292529, -0.1870078740157479769, 0.4822834645669291653 ) ) ;
#28450=CARTESIAN_POINT ( 'NONE',  ( -0.06561679790026180015, -0.4281496062992127816, -0.4176697321401328100 ) ) ;
#28451=CARTESIAN_POINT ( 'NONE',  ( -1.397637795275589623, -0.5400638737290845981, -0.3530559997133363437 ) ) ;
#28453=CARTESIAN_POINT ( 'NONE',  ( 0.09186351706036799403, -0.4281496062992127816, -0.4176697321401328100 ) ) ;
#28455=CARTESIAN_POINT ( 'NONE',  ( -1.102362204724408601, -0.1870078740157480601, -0.3641732283464567677 ) ) ;
#28460=CARTESIAN_POINT ( 'NONE',  ( -1.397637795275589623, 0.1660481256975885056, 0.3530559997133364547 ) ) ;
#28462=CARTESIAN_POINT ( 'NONE',  ( -1.509186351706035767, 0.05413385826771626580, -0.4176697321401330321 ) ) ;
#28463=CARTESIAN_POINT ( 'NONE',  ( -1.679790026246718693, 0.2306618581243847221, -0.2411417322834647770 ) ) ;
#28464=CARTESIAN_POINT ( 'NONE',  ( 0.4199475065616805614, 0.2306618581243848609, 0.2411417322834645549 ) ) ;
#28465=CARTESIAN_POINT ( 'NONE',  ( -0.3821149210511725069, 0.02791078216816064370, 0.4328096321851915285 ) ) ;
#28467=CARTESIAN_POINT ( 'NONE',  ( -0.3871391076115476282, -0.08942795157527998196, 0.3641732283464567121 ) ) ;
#28468=CARTESIAN_POINT ( 'NONE',  ( -0.6233595800524928121, -0.08942795157527998196, 0.3641732283464567121 ) ) ;
#28469=CARTESIAN_POINT ( 'NONE',  ( -1.417322834645668772, -0.1870078740157480879, -0.4822834645669291653 ) ) ;
#28470=CARTESIAN_POINT ( 'NONE',  ( 0.9448818897637802916, -0.1870078740157479769, 0.4822834645669291653 ) ) ;
#28471=CARTESIAN_POINT ( 'NONE',  ( -1.049868766404198794, -0.6046776061558807314, 0.2411417322834647770 ) ) ;
#28475=CARTESIAN_POINT ( 'NONE',  ( -1.482939632545930975, 0.05413385826771666132, 0.4176697321401328100 ) ) ;
#28476=CARTESIAN_POINT ( 'NONE',  ( 2.795275590551181466, 2.793565526369266916, 0.000000000000000000 ) ) ;
#28479=DIRECTION ( 'NONE',  ( 3.096699300667737957E-16, -1.000000000000000000, 0.000000000000000000 ) ) ;
#28480=EDGE_CURVE ( 'NONE', #36616, #11962, #31154, .T. ) ;
#28483=CARTESIAN_POINT ( 'NONE',  ( -0.5643044619422565855, -0.4281496062992124485, 0.4176697321401328655 ) ) ;
#28484=CARTESIAN_POINT ( 'NONE',  ( 1.410761154855643795, -0.05778040916215560624, -0.4822834645669293319 ) ) ;
#28486=CARTESIAN_POINT ( 'NONE',  ( -1.725721784776902190, -0.05778040916215522460, 0.4822834645669289988 ) ) ;
#28488=CARTESIAN_POINT ( 'NONE',  ( -1.213910761154854745, 0.2952755905511810774, -0.1292274648535930714 ) ) ;
#28489=CARTESIAN_POINT ( 'NONE',  ( -0.7545931758530177724, 0.2952755905511811885, 0.1292274648535926551 ) ) ;
#28491=CARTESIAN_POINT ( 'NONE',  ( 0.4527559055118117182, -0.4536011799217367080, 0.2665933059059888421 ) ) ;
#28493=CARTESIAN_POINT ( 'NONE',  ( 0.1837270341207357105, -0.5023911411419708095, -0.1820866141732282451 ) ) ;
#28494=CARTESIAN_POINT ( 'NONE',  ( 1.122047244094488860, 0.07958543189024085140, 0.2665933059059887866 ) ) ;
#28495=CARTESIAN_POINT ( 'NONE',  ( 0.8858267716535438430, -0.5400638737290845981, -0.3530559997133363437 ) ) ;
#28497=AXIS2_PLACEMENT_3D ( 'NONE', #56833, #24034, #5099 ) ;
#28498=CARTESIAN_POINT ( 'NONE',  ( -0.4986876640419939388, 0.1283753931104746893, -0.1820866141732285504 ) ) ;
#28500=CARTESIAN_POINT ( 'NONE',  ( -1.318897637795274802, 0.1660481256975885056, 0.3530559997133364547 ) ) ;
#28502=CARTESIAN_POINT ( 'NONE',  ( -1.312335958005248715, 0.1283753931104748280, 0.1820866141732283561 ) ) ;
#28504=CARTESIAN_POINT ( 'NONE',  ( -0.7611548556430438595, -0.5023911411419708095, -0.1820866141732282451 ) ) ;
#28506=CARTESIAN_POINT ( 'NONE',  ( -0.1181102362204717315, -0.6692913385826771977, 8.415575281601705876E-17 ) ) ;
#28507=CARTESIAN_POINT ( 'NONE',  ( 1.607611548556431069, -0.5511811023622048555, -0.09757992244046775898 ) ) ;
#28508=CARTESIAN_POINT ( 'NONE',  ( 0.7086614173228352742, -0.1870078740157480601, -0.3641732283464567677 ) ) ;
#28509=CARTESIAN_POINT ( 'NONE',  ( -0.05905511811023545637, -0.4536011799217368745, -0.2665933059059886201 ) ) ;
#28510=CARTESIAN_POINT ( 'NONE',  ( -0.7152230971128602510, -0.3162353388693405765, 0.4822834645669290543 ) ) ;
#28511=CARTESIAN_POINT ( 'NONE',  ( -1.587926509186350810, -0.4281496062992124485, 0.4176697321401328655 ) ) ;
#28512=LINE ( 'NONE', #73563, #40783 ) ;
#28513=CARTESIAN_POINT ( 'NONE',  ( 0.07217847769028949700, -0.3162353388693405765, 0.4822834645669290543 ) ) ;
#28514=ORIENTED_EDGE ( 'NONE', *, *, #10113, .F. ) ;
#28516=( BOUNDED_SURFACE ( )  B_SPLINE_SURFACE ( 1, 2, ( 
 ( #75602, #62546, #43577, #9966, #4883, #30557, #81094, #43165, #24232, #16707, #17941, #55799, #56223, #81921, #42348, #4059, #23411, #49904, #49077, #69279, #24644, #76009, #18351, #74778, #17129, #35637, #61298, #3656, #29319, #54980, #23828, #42761, #49496, #75189, #10795, #36455, #23001, #62129, #30137, #17533, #13276, #31368, #7364, #57033, #39343, #25876, #38928, #6532, #26721, #69688, #33034, #58702, #52375, #83140, #82728, #77241, #50722, #51959, #1068, #643, #76420, #77665, #32202, #32616, #64608, #18749, #12438, #31785, #58278, #44393, #19571, #26300, #65029, #19996, #70085, #57448, #6945, #45647, #78083, #12031, #71342, #226, #38098, #57859, #51538, #19153, #44804, #13689, #20415, #37688, #63363, #5697, #25047, #63772, #6113, #25460, #45230, #51127, #70931, #76821, #70499, #12857, #38515, #64198, #59535, #33460, #53627, #27133, #28381, #9445, #15779, #80175, #40187, #59953, #27969, #54461, #46483, #21244, #1892, #2308, #35116, #79754, #46067, #7794, #65461, #1479, #53211, #47731, #20830, #40599, #3134, #8206, #66281, #27552, #46899, #47315, #8621, #34292, #21655, #39766, #15357, #2720, #67114, #78922, #41431, #72593, #78507, #71760, #72178, #79335, #65871, #59122, #52797, #14940, #73005, #14113, #60782, #14536, #41018, #66704, #33871, #9037, #28798, #34711, #60372, #54041, #22071, #73429, #11106, #30034, #43476, #35532, #81821, #80588, #80995, #11523, #3550, #29625, #30451, #4775, #49393, #56115, #56525, #23722, #75087, #42247, #55697, #75502, #55285, #22895, #22490, #3962, #24131, #67942, #29216, #17434, #17841, #62438, #81405, #4366, #35950, #48563, #17023, #61620, #43065, #68762, #36354, #10284, #23308, #9862, #37180, #48978, #49800, #69172, #36762, #61194, #48153, #62859, #62030, #74677, #5195, #30860, #73848, #16188, #41835, #42662, #74261, #67525, #54883, #16603, #68360, #10699, #11933, #56935, #12759, #38417, #25781, #75909, #82631, #18653, #69587, #64098, #19059, #37588, #19478, #6434, #63261, #44297, #32105, #57764, #50211, #63675, #18248, #6016, #31269, #126, #50618, #5602, #43890, #31687, #25365, #24945, #76323, #69988, #51442, #77145, #12343, #37999, #45130, #57346, #82227, #24547, #83042, #51028, #76727, #44707, #70403, #49132, #10024, #82381, #81563, #10447, #61355, #3709, #23465, #29780, #24698, #63014, #50367, #49547, #68508, #80740, #10848, #31011, #4115, #68916, #61774, #23882, #5352, #4943, #75242, #37341, #29372, #75656, #74419, #74837, #56679, #23054, #17181, #24287, #81972, #43218, #49959, #16351, #17586, #69334, #17996, #48722, #55442, #11266, #43630, #11684, #41995, #67689, #30191, #16764, #62185, #55854, #42814, #36509, #35690, #55033, #42403, #36924, #62601, #68101, #36103, #81150, #4522, #30612, #56276, #12915, #33099, #76064, #39408, #65091, #58765, #6168, #63419, #283, #57088, #58340, #7429, #45707, #26778, #70142, #6587, #57919, #1128, #76478, #51183, #31843, #32258, #18407, #26359, #44050, #37744, #12087, #31426, #83196, #77725, #50778, #70559, #69742, #38157, #38572, #57505, #76881, #77299, #64253, #25938, #51597, #5756, #45291, #32674, #13751, #25518, #71403, #19212, #44860, #82784, #25105, #19630, #12494, #18805, #44450, #70987, #13331, #63830, #38984, #64667, #7006, #702, #52019, #20054, #67180, #40246, #21714, #14593, #60017, #15845, #41079, #2372, #73497, #65521, #28444, #27193, #27613, #41494, #33518, #59596, #60433, #34774, #79395, #2784, #3195, #53687, #47378, #72244, #28029, #66768, #59181, #54103, #15001, #15418, #73069, #1538, #78567, #65929, #9101, #52857, #79819, #22135, #47793, #9509, #35182, #60843, #52434, #14174, #78144, #39832, #20476, #8681, #46130, #72651, #71824, #7852, #20893, #46546, #8266, #33931, #1951, #53276, #78986, #21306, #46959, #40658, #66343, #34351, #42720, #10756, #37245, #29276, #4021, #68004, #68416, #17901, #62502, #62921, #73910, #48214, #67591, #36010, #30515, #3610, #23370, #69237, #74320, #49038, #10349, #29685, #30097, #74735, #17083, #4431, #22552, #81466, #68823, #49861, #61680, #81880, #55348, #81054, #16250, #11585, #36416, #22959, #41897, #9922, #62089, #42306 ),
 ( #56177, #55760, #24192, #23784, #49455, #4840, #35593, #75149, #75561, #54940, #17494, #43125, #61256, #11168, #43538, #36829, #80646, #28859, #54521, #80236, #48625, #16667, #1351, #1760, #46352, #39635, #71626, #19864, #64470, #935, #45512, #65326, #13978, #20278, #51824, #64891, #77104, #21115, #71209, #72048, #33742, #7663, #45087, #40474, #40059, #27001, #57723, #53078, #30918, #5254, #27417, #26593, #52664, #70791, #59402, #52245, #78790, #45928, #33334, #46775, #32478, #86, #72466, #13552, #8079, #58995, #78370, #65746, #13142, #77949, #14815, #6807, #39208, #20702, #38794, #14404, #25739, #7230, #58140, #51400, #32902, #19436, #26162, #509, #77528, #58570, #22765, #16057, #48018, #79625, #40885, #60653, #21942, #41703, #73718, #80039, #28251, #41301, #53502, #80861, #47602, #48427, #10151, #67396, #21526, #16889, #16472, #22359, #73296, #9730, #35817, #35401, #61066, #61482, #3003, #66567, #42117, #3417, #29080, #8901, #8489, #72877, #53911, #74126, #67814, #29491, #27840, #15645, #66987, #47185, #3831, #54750, #15225, #48842, #55150, #34577, #9319, #23173, #74543, #59819, #54330, #2174, #80456, #60245, #66152, #34989, #2592, #28669, #34158, #79210, #42930, #62301, #17303, #31547, #12206, #29896, #4638, #82905, #17705, #69855, #5871, #68625, #43745, #10965, #4232, #5060, #61891, #50891, #36624, #56392, #55559, #75357, #42528, #81688, #43333, #69451, #62723, #37041, #18112, #36222, #11801, #82496, #63540, #23999, #37864, #69033, #11384, #81268, #25226, #24405, #30309, #23583, #49255, #49667, #55976, #76591, #57204, #68230, #75770, #30730, #74957, #82091, #10564, #50075, #37455, #63129, #5467, #31129, #56796, #24812, #50479, #76183, #18520, #44163, #77423, #7975, #62468, #26061, #26899, #1250, #45826, #52558, #52974, #20176, #71525, #38692, #52140, #33228, #25638, #78267, #64788, #65218, #13871, #51301, #44987, #64370, #7557, #77004, #77847, #58891, #71946, #20598, #19335, #6707, #39530, #46250, #14298, #44570, #39959, #32798, #70685, #7126, #58467, #51720, #19757, #65645, #33638, #59301, #1658, #27315, #63952, #18920, #6289, #70261, #830, #12616, #39106, #38274, #31964, #57625, #13039, #32376, #58040, #404, #26489, #45411, #71107, #13450, #48323, #29389, #72771, #9216, #60550, #3725, #79107, #53805, #34473, #34889, #67706, #28974, #78688, #40368, #14713, #34051, #2490, #80351, #53400, #73188, #35706, #40776, #15538, #21426, #66048, #41198, #8386, #21011, #47080, #2901, #59714, #28149, #46671, #15957, #72365, #42012, #2069, #27735, #74020, #66886, #41603, #15122, #16366, #28565, #10042, #54221, #79937, #61375, #66461, #8797, #22664, #79518, #60139, #22252, #67293, #54641, #21833, #47910, #47496, #73615, #9626, #35297, #60959, #3309, #24715, #4538, #29796, #55049, #36525, #37358, #74856, #61791, #49975, #50383, #11704, #4961, #36941, #68524, #55457, #49566, #10865, #30629, #62619, #68933, #17198, #30208, #42420, #69758, #62201, #63031, #82397, #56294, #10465, #5773, #5369, #11282, #55870, #81991, #76081, #24305, #75673, #18425, #75260, #81166, #31030, #18013, #43647, #23482, #80756, #4131, #42831, #56698, #44066, #12104, #16782, #81583, #23900, #36118, #37762, #69350, #49149, #63437, #23070, #17604, #43236, #48738, #74435, #68120, #19649, #50794, #45310, #83214, #39427, #12932, #6186, #70160, #71005, #7024, #31864, #51201, #57523, #20495, #1147, #18822, #76899, #71844, #6604, #58789, #78164, #25536, #32692, #44879, #71423, #26797, #58359, #12513, #65542, #65111, #13348, #38592, #39002, #52454, #64685, #721, #46149, #51614, #19229, #7449, #26379, #52039, #70578, #57105, #38174, #64270, #13770, #33119, #14194, #76495, #32276, #57936, #63848, #39851, #77743, #300, #31442, #82800, #25956, #77319, #25124, #44469, #20074, #45726, #27213, #79416, #59615, #15865, #72673, #65949, #46565, #21735, #66788, #8285, #27633, #33951, #80256, #60862, #78586, #53295, #48233, #66363, #35201, #54541, #1970, #9123, #79007, #52876, #53707, #20912, #16271, #21326, #47398, #72264, #40678, #7873, #28463, #59200, #22573, #33537, #41916, #3216, #2393, #54124, #14612 ) ),
 .UNSPECIFIED., .F., .F., .F. ) 
 B_SPLINE_SURFACE_WITH_KNOTS ( ( 2, 2 ),
 ( 3, 2, 2, 2, 2, 2, 2, 2, 2, 2, 2, 2, 2, 2, 2, 2, 2, 2, 2, 2, 2, 2, 2, 2, 2, 2, 2, 2, 2, 2, 2, 2, 2, 2, 2, 2, 2, 2, 2, 2, 2, 2, 2, 2, 2, 2, 2, 2, 2, 2, 2, 2, 2, 2, 2, 2, 2, 2, 2, 2, 2, 2, 2, 2, 2, 2, 2, 2, 2, 2, 2, 2, 2, 2, 2, 2, 2, 2, 2, 2, 2, 2, 2, 2, 2, 2, 2, 2, 2, 2, 2, 2, 2, 2, 2, 2, 2, 2, 2, 2, 2, 2, 2, 2, 2, 2, 2, 2, 2, 2, 2, 2, 2, 2, 2, 2, 2, 2, 2, 2, 2, 2, 2, 2, 2, 2, 2, 2, 2, 2, 2, 2, 2, 2, 2, 2, 2, 2, 2, 2, 2, 2, 2, 2, 2, 2, 2, 2, 2, 2, 2, 2, 2, 2, 2, 2, 2, 2, 2, 2, 2, 2, 2, 2, 2, 2, 2, 2, 2, 2, 2, 2, 2, 2, 2, 2, 2, 2, 2, 2, 2, 2, 2, 2, 2, 2, 2, 2, 2, 2, 2, 2, 2, 2, 2, 2, 2, 2, 2, 2, 2, 2, 2, 2, 2, 2, 2, 2, 2, 2, 2, 2, 2, 2, 2, 2, 2, 2, 2, 2, 2, 2, 2, 2, 2, 2, 2, 2, 2, 2, 2, 2, 2, 2, 2, 2, 2, 2, 2, 2, 2, 2, 2, 2, 2, 2, 2, 2, 2, 2, 2, 2, 2, 2, 2, 3 ),
 ( 0.000000000000000000, 1.000000000000000000 ),
 ( 0.000000000000000000, 0.003787878787878787984, 0.007575757575757575968, 0.01136363636363636395, 0.01515151515151515194, 0.01893939393939393992, 0.02272727272727272790, 0.02651515151515151589, 0.03030303030303030387, 0.03409090909090908839, 0.03787878787878787984, 0.04166666666666666435, 0.04545454545454545581, 0.04924242424242424032, 0.05303030303030303177, 0.05681818181818181629, 0.06060606060606060774, 0.06439393939393939226, 0.06818181818181817677, 0.07196969696969697516, 0.07575757575757575968, 0.07954545454545454419, 0.08333333333333332871, 0.08712121212121212710, 0.09090909090909091161, 0.09469696969696969613, 0.09848484848484848064, 0.1022727272727272790, 0.1060606060606060635, 0.1098484848484848481, 0.1136363636363636326, 0.1174242424242424310, 0.1212121212121212155, 0.1250000000000000000, 0.1287878787878787845, 0.1325757575757575690, 0.1363636363636363535, 0.1401515151515151381, 0.1439393939393939503, 0.1477272727272727348, 0.1515151515151515194, 0.1553030303030303039, 0.1590909090909090884, 0.1628787878787878729, 0.1666666666666666574, 0.1704545454545454419, 0.1742424242424242542, 0.1780303030303030387, 0.1818181818181818232, 0.1856060606060606077, 0.1893939393939393923, 0.1931818181818181768, 0.1969696969696969613, 0.2007575757575757458, 0.2045454545454545581, 0.2083333333333333426, 0.2121212121212121271, 0.2159090909090909116, 0.2196969696969696961, 0.2234848484848484806, 0.2272727272727272652, 0.2310606060606060497, 0.2348484848484848619, 0.2386363636363636465, 0.2424242424242424310, 0.2462121212121212155, 0.2500000000000000000, 0.2537878787878787845, 0.2575757575757575690, 0.2613636363636363535, 0.2651515151515151381, 0.2689393939393939226, 0.2727272727272727071, 0.2765151515151514916, 0.2803030303030302761, 0.2840909090909091161, 0.2878787878787879007, 0.2916666666666666852, 0.2954545454545454697, 0.2992424242424242542, 0.3030303030303030387, 0.3068181818181818232, 0.3106060606060606077, 0.3143939393939393923, 0.3181818181818181768, 0.3219696969696969613, 0.3257575757575757458, 0.3295454545454545303, 0.3333333333333333148, 0.3371212121212120993, 0.3409090909090908839, 0.3446969696969697239, 0.3484848484848485084, 0.3522727272727272929, 0.3560606060606060774, 0.3598484848484848619, 0.3636363636363636465, 0.3674242424242424310, 0.3712121212121212155, 0.3750000000000000000, 0.3787878787878787845, 0.3825757575757575690, 0.3863636363636363535, 0.3901515151515151381, 0.3939393939393939226, 0.3977272727272727071, 0.4015151515151514916, 0.4053030303030302761, 0.4090909090909091161, 0.4128787878787879007, 0.4166666666666666852, 0.4204545454545454697, 0.4242424242424242542, 0.4280303030303030387, 0.4318181818181818232, 0.4356060606060606077, 0.4393939393939393923, 0.4431818181818181768, 0.4469696969696969613, 0.4507575757575757458, 0.4545454545454545303, 0.4583333333333333148, 0.4621212121212120993, 0.4659090909090908839, 0.4696969696969697239, 0.4734848484848485084, 0.4772727272727272929, 0.4810606060606060774, 0.4848484848484848619, 0.4886363636363636465, 0.4924242424242424310, 0.4962121212121212155, 0.5000000000000000000, 0.5037878787878787845, 0.5075757575757575690, 0.5113636363636363535, 0.5151515151515151381, 0.5189393939393939226, 0.5227272727272727071, 0.5265151515151514916, 0.5303030303030302761, 0.5340909090909090606, 0.5378787878787878451, 0.5416666666666666297, 0.5454545454545454142, 0.5492424242424241987, 0.5530303030303029832, 0.5568181818181817677, 0.5606060606060605522, 0.5643939393939394478, 0.5681818181818182323, 0.5719696969696970168, 0.5757575757575758013, 0.5795454545454545858, 0.5833333333333333703, 0.5871212121212121549, 0.5909090909090909394, 0.5946969696969697239, 0.5984848484848485084, 0.6022727272727272929, 0.6060606060606060774, 0.6098484848484848619, 0.6136363636363636465, 0.6174242424242424310, 0.6212121212121212155, 0.6250000000000000000, 0.6287878787878787845, 0.6325757575757575690, 0.6363636363636363535, 0.6401515151515151381, 0.6439393939393939226, 0.6477272727272727071, 0.6515151515151514916, 0.6553030303030302761, 0.6590909090909090606, 0.6628787878787878451, 0.6666666666666666297, 0.6704545454545454142, 0.6742424242424241987, 0.6780303030303029832, 0.6818181818181817677, 0.6856060606060605522, 0.6893939393939394478, 0.6931818181818182323, 0.6969696969696970168, 0.7007575757575758013, 0.7045454545454545858, 0.7083333333333333703, 0.7121212121212121549, 0.7159090909090909394, 0.7196969696969697239, 0.7234848484848485084, 0.7272727272727272929, 0.7310606060606060774, 0.7348484848484848619, 0.7386363636363636465, 0.7424242424242424310, 0.7462121212121212155, 0.7500000000000000000, 0.7537878787878787845, 0.7575757575757575690, 0.7613636363636363535, 0.7651515151515151381, 0.7689393939393939226, 0.7727272727272727071, 0.7765151515151514916, 0.7803030303030302761, 0.7840909090909090606, 0.7878787878787878451, 0.7916666666666666297, 0.7954545454545454142, 0.7992424242424241987, 0.8030303030303029832, 0.8068181818181817677, 0.8106060606060605522, 0.8143939393939394478, 0.8181818181818182323, 0.8219696969696970168, 0.8257575757575758013, 0.8295454545454545858, 0.8333333333333333703, 0.8371212121212121549, 0.8409090909090909394, 0.8446969696969697239, 0.8484848484848485084, 0.8522727272727272929, 0.8560606060606060774, 0.8598484848484848619, 0.8636363636363636465, 0.8674242424242424310, 0.8712121212121212155, 0.8750000000000000000, 0.8787878787878787845, 0.8825757575757575690, 0.8863636363636363535, 0.8901515151515151381, 0.8939393939393939226, 0.8977272727272727071, 0.9015151515151514916, 0.9053030303030302761, 0.9090909090909090606, 0.9128787878787878451, 0.9166666666666666297, 0.9204545454545454142, 0.9242424242424241987, 0.9280303030303029832, 0.9318181818181817677, 0.9356060606060605522, 0.9393939393939394478, 0.9431818181818182323, 0.9469696969696970168, 0.9507575757575758013, 0.9545454545454545858, 0.9583333333333333703, 0.9621212121212121549, 0.9659090909090909394 ),
 .UNSPECIFIED. ) 
 GEOMETRIC_REPRESENTATION_ITEM ( )  RATIONAL_B_SPLINE_SURFACE ( (
 ( 1.000000000000000000, 0.9659258262890683122, 1.000000000000000000, 0.9659258262890683122, 1.000000000000000000, 0.9659258262890683122, 1.000000000000000000, 0.9659258262890683122, 1.000000000000000000, 0.9659258262890683122, 1.000000000000000000, 0.9659258262890683122, 1.000000000000000000, 0.9659258262890683122, 1.000000000000000000, 0.9659258262890683122, 1.000000000000000000, 0.9659258262890683122, 1.000000000000000000, 0.9659258262890683122, 1.000000000000000000, 0.9659258262890683122, 1.000000000000000000, 0.9659258262890683122, 1.000000000000000000, 0.9659258262890683122, 1.000000000000000000, 0.9659258262890683122, 1.000000000000000000, 0.9659258262890683122, 1.000000000000000000, 0.9659258262890683122, 1.000000000000000000, 0.9659258262890683122, 1.000000000000000000, 0.9659258262890683122, 1.000000000000000000, 0.9659258262890683122, 1.000000000000000000, 0.9659258262890683122, 1.000000000000000000, 0.9659258262890683122, 1.000000000000000000, 0.9659258262890683122, 1.000000000000000000, 0.9659258262890683122, 1.000000000000000000, 0.9659258262890683122, 1.000000000000000000, 0.9659258262890683122, 1.000000000000000000, 0.9659258262890683122, 1.000000000000000000, 0.9659258262890683122, 1.000000000000000000, 0.9659258262890683122, 1.000000000000000000, 0.9659258262890683122, 1.000000000000000000, 0.9659258262890683122, 1.000000000000000000, 0.9659258262890683122, 1.000000000000000000, 0.9659258262890683122, 1.000000000000000000, 0.9659258262890683122, 1.000000000000000000, 0.9659258262890683122, 1.000000000000000000, 0.9659258262890683122, 1.000000000000000000, 0.9659258262890683122, 1.000000000000000000, 0.9659258262890683122, 1.000000000000000000, 0.9659258262890683122, 1.000000000000000000, 0.9659258262890683122, 1.000000000000000000, 0.9659258262890683122, 1.000000000000000000, 0.9659258262890683122, 1.000000000000000000, 0.9659258262890683122, 1.000000000000000000, 0.9659258262890683122, 1.000000000000000000, 0.9659258262890683122, 1.000000000000000000, 0.9659258262890683122, 1.000000000000000000, 0.9659258262890683122, 1.000000000000000000, 0.9659258262890683122, 1.000000000000000000, 0.9659258262890683122, 1.000000000000000000, 0.9659258262890683122, 1.000000000000000000, 0.9659258262890683122, 1.000000000000000000, 0.9659258262890683122, 1.000000000000000000, 0.9659258262890683122, 1.000000000000000000, 0.9659258262890683122, 1.000000000000000000, 0.9659258262890683122, 1.000000000000000000, 0.9659258262890683122, 1.000000000000000000, 0.9659258262890683122, 1.000000000000000000, 0.9659258262890683122, 1.000000000000000000, 0.9659258262890683122, 1.000000000000000000, 0.9659258262890683122, 1.000000000000000000, 0.9659258262890683122, 1.000000000000000000, 0.9659258262890683122, 1.000000000000000000, 0.9659258262890683122, 1.000000000000000000, 0.9659258262890683122, 1.000000000000000000, 0.9659258262890683122, 1.000000000000000000, 0.9659258262890683122, 1.000000000000000000, 0.9659258262890683122, 1.000000000000000000, 0.9659258262890683122, 1.000000000000000000, 0.9659258262890683122, 1.000000000000000000, 0.9659258262890683122, 1.000000000000000000, 0.9659258262890683122, 1.000000000000000000, 0.9659258262890683122, 1.000000000000000000, 0.9659258262890683122, 1.000000000000000000, 0.9659258262890683122, 1.000000000000000000, 0.9659258262890683122, 1.000000000000000000, 0.9659258262890683122, 1.000000000000000000, 0.9659258262890683122, 1.000000000000000000, 0.9659258262890683122, 1.000000000000000000, 0.9659258262890683122, 1.000000000000000000, 0.9659258262890683122, 1.000000000000000000, 0.9659258262890683122, 1.000000000000000000, 0.9659258262890683122, 1.000000000000000000, 0.9659258262890683122, 1.000000000000000000, 0.9659258262890683122, 1.000000000000000000, 0.9659258262890683122, 1.000000000000000000, 0.9659258262890683122, 1.000000000000000000, 0.9659258262890683122, 1.000000000000000000, 0.9659258262890683122, 1.000000000000000000, 0.9659258262890683122, 1.000000000000000000, 0.9659258262890683122, 1.000000000000000000, 0.9659258262890683122, 1.000000000000000000, 0.9659258262890683122, 1.000000000000000000, 0.9659258262890683122, 1.000000000000000000, 0.9659258262890683122, 1.000000000000000000, 0.9659258262890683122, 1.000000000000000000, 0.9659258262890683122, 1.000000000000000000, 0.9659258262890683122, 1.000000000000000000, 0.9659258262890683122, 1.000000000000000000, 0.9659258262890683122, 1.000000000000000000, 0.9659258262890683122, 1.000000000000000000, 0.9659258262890683122, 1.000000000000000000, 0.9659258262890683122, 1.000000000000000000, 0.9659258262890683122, 1.000000000000000000, 0.9659258262890683122, 1.000000000000000000, 0.9659258262890683122, 1.000000000000000000, 0.9659258262890683122, 1.000000000000000000, 0.9659258262890683122, 1.000000000000000000, 0.9659258262890683122, 1.000000000000000000, 0.9659258262890683122, 1.000000000000000000, 0.9659258262890683122, 1.000000000000000000, 0.9659258262890683122, 1.000000000000000000, 0.9659258262890683122, 1.000000000000000000, 0.9659258262890683122, 1.000000000000000000, 0.9659258262890683122, 1.000000000000000000, 0.9659258262890683122, 1.000000000000000000, 0.9659258262890683122, 1.000000000000000000, 0.9659258262890683122, 1.000000000000000000, 0.9659258262890683122, 1.000000000000000000, 0.9659258262890683122, 1.000000000000000000, 0.9659258262890683122, 1.000000000000000000, 0.9659258262890683122, 1.000000000000000000, 0.9659258262890683122, 1.000000000000000000, 0.9659258262890683122, 1.000000000000000000, 0.9659258262890683122, 1.000000000000000000, 0.9659258262890683122, 1.000000000000000000, 0.9659258262890683122, 1.000000000000000000, 0.9659258262890683122, 1.000000000000000000, 0.9659258262890683122, 1.000000000000000000, 0.9659258262890683122, 1.000000000000000000, 0.9659258262890683122, 1.000000000000000000, 0.9659258262890683122, 1.000000000000000000, 0.9659258262890683122, 1.000000000000000000, 0.9659258262890683122, 1.000000000000000000, 0.9659258262890683122, 1.000000000000000000, 0.9659258262890683122, 1.000000000000000000, 0.9659258262890683122, 1.000000000000000000, 0.9659258262890683122, 1.000000000000000000, 0.9659258262890683122, 1.000000000000000000, 0.9659258262890683122, 1.000000000000000000, 0.9659258262890683122, 1.000000000000000000, 0.9659258262890683122, 1.000000000000000000, 0.9659258262890683122, 1.000000000000000000, 0.9659258262890683122, 1.000000000000000000, 0.9659258262890683122, 1.000000000000000000, 0.9659258262890683122, 1.000000000000000000, 0.9659258262890683122, 1.000000000000000000, 0.9659258262890683122, 1.000000000000000000, 0.9659258262890683122, 1.000000000000000000, 0.9659258262890683122, 1.000000000000000000, 0.9659258262890683122, 1.000000000000000000, 0.9659258262890683122, 1.000000000000000000, 0.9659258262890683122, 1.000000000000000000, 0.9659258262890683122, 1.000000000000000000, 0.9659258262890683122, 1.000000000000000000, 0.9659258262890683122, 1.000000000000000000, 0.9659258262890683122, 1.000000000000000000, 0.9659258262890683122, 1.000000000000000000, 0.9659258262890683122, 1.000000000000000000, 0.9659258262890683122, 1.000000000000000000, 0.9659258262890683122, 1.000000000000000000, 0.9659258262890683122, 1.000000000000000000, 0.9659258262890683122, 1.000000000000000000, 0.9659258262890683122, 1.000000000000000000, 0.9659258262890683122, 1.000000000000000000, 0.9659258262890683122, 1.000000000000000000, 0.9659258262890683122, 1.000000000000000000, 0.9659258262890683122, 1.000000000000000000, 0.9659258262890683122, 1.000000000000000000, 0.9659258262890683122, 1.000000000000000000, 0.9659258262890683122, 1.000000000000000000, 0.9659258262890683122, 1.000000000000000000, 0.9659258262890683122, 1.000000000000000000, 0.9659258262890683122, 1.000000000000000000, 0.9659258262890683122, 1.000000000000000000, 0.9659258262890683122, 1.000000000000000000, 0.9659258262890683122, 1.000000000000000000, 0.9659258262890683122, 1.000000000000000000, 0.9659258262890683122, 1.000000000000000000, 0.9659258262890683122, 1.000000000000000000, 0.9659258262890683122, 1.000000000000000000, 0.9659258262890683122, 1.000000000000000000, 0.9659258262890683122, 1.000000000000000000, 0.9659258262890683122, 1.000000000000000000, 0.9659258262890683122, 1.000000000000000000, 0.9659258262890683122, 1.000000000000000000, 0.9659258262890683122, 1.000000000000000000, 0.9659258262890683122, 1.000000000000000000, 0.9659258262890683122, 1.000000000000000000, 0.9659258262890683122, 1.000000000000000000, 0.9659258262890683122, 1.000000000000000000, 0.9659258262890683122, 1.000000000000000000, 0.9659258262890683122, 1.000000000000000000, 0.9659258262890683122, 1.000000000000000000, 0.9659258262890683122, 1.000000000000000000, 0.9659258262890683122, 1.000000000000000000, 0.9659258262890683122, 1.000000000000000000, 0.9659258262890683122, 1.000000000000000000, 0.9659258262890683122, 1.000000000000000000, 0.9659258262890683122, 1.000000000000000000, 0.9659258262890683122, 1.000000000000000000, 0.9659258262890683122, 1.000000000000000000, 0.9659258262890683122, 1.000000000000000000, 0.9659258262890683122, 1.000000000000000000, 0.9659258262890683122, 1.000000000000000000, 0.9659258262890683122, 1.000000000000000000, 0.9659258262890683122, 1.000000000000000000, 0.9659258262890683122, 1.000000000000000000, 0.9659258262890683122, 1.000000000000000000, 0.9659258262890683122, 1.000000000000000000, 0.9659258262890683122, 1.000000000000000000, 0.9659258262890683122, 1.000000000000000000, 0.9659258262890683122, 1.000000000000000000, 0.9659258262890683122, 1.000000000000000000, 0.9659258262890683122, 1.000000000000000000, 0.9659258262890683122, 1.000000000000000000, 0.9659258262890683122, 1.000000000000000000, 0.9659258262890683122, 1.000000000000000000, 0.9659258262890683122, 1.000000000000000000, 0.9659258262890683122, 1.000000000000000000, 0.9659258262890683122, 1.000000000000000000, 0.9659258262890683122, 1.000000000000000000, 0.9659258262890683122, 1.000000000000000000, 0.9659258262890683122, 1.000000000000000000, 0.9659258262890683122, 1.000000000000000000, 0.9659258262890683122, 1.000000000000000000, 0.9659258262890683122, 1.000000000000000000, 0.9659258262890683122, 1.000000000000000000, 0.9659258262890683122, 1.000000000000000000, 0.9659258262890683122, 1.000000000000000000, 0.9659258262890683122, 1.000000000000000000, 0.9659258262890683122, 1.000000000000000000, 0.9659258262890683122, 1.000000000000000000, 0.9659258262890683122, 1.000000000000000000, 0.9659258262890683122, 1.000000000000000000, 0.9659258262890683122, 1.000000000000000000, 0.9659258262890683122, 1.000000000000000000, 0.9659258262890683122, 1.000000000000000000, 0.9659258262890683122, 1.000000000000000000, 0.9659258262890683122, 1.000000000000000000, 0.9659258262890683122, 1.000000000000000000, 0.9659258262890683122, 1.000000000000000000, 0.9659258262890683122, 1.000000000000000000, 0.9659258262890683122, 1.000000000000000000, 0.9659258262890683122, 1.000000000000000000, 0.9659258262890683122, 1.000000000000000000, 0.9659258262890683122, 1.000000000000000000, 0.9659258262890683122, 1.000000000000000000, 0.9659258262890683122, 1.000000000000000000, 0.9659258262890683122, 1.000000000000000000, 0.9659258262890683122, 1.000000000000000000, 0.9659258262890683122, 1.000000000000000000, 0.9659258262890683122, 1.000000000000000000, 0.9659258262890683122, 1.000000000000000000, 0.9659258262890683122, 1.000000000000000000, 0.9659258262890683122, 1.000000000000000000, 0.9659258262890683122, 1.000000000000000000),
 ( 1.000000000000000000, 0.9659258262890683122, 1.000000000000000000, 0.9659258262890683122, 1.000000000000000000, 0.9659258262890683122, 1.000000000000000000, 0.9659258262890683122, 1.000000000000000000, 0.9659258262890683122, 1.000000000000000000, 0.9659258262890683122, 1.000000000000000000, 0.9659258262890683122, 1.000000000000000000, 0.9659258262890683122, 1.000000000000000000, 0.9659258262890683122, 1.000000000000000000, 0.9659258262890683122, 1.000000000000000000, 0.9659258262890683122, 1.000000000000000000, 0.9659258262890683122, 1.000000000000000000, 0.9659258262890683122, 1.000000000000000000, 0.9659258262890683122, 1.000000000000000000, 0.9659258262890683122, 1.000000000000000000, 0.9659258262890683122, 1.000000000000000000, 0.9659258262890683122, 1.000000000000000000, 0.9659258262890683122, 1.000000000000000000, 0.9659258262890683122, 1.000000000000000000, 0.9659258262890683122, 1.000000000000000000, 0.9659258262890683122, 1.000000000000000000, 0.9659258262890683122, 1.000000000000000000, 0.9659258262890683122, 1.000000000000000000, 0.9659258262890683122, 1.000000000000000000, 0.9659258262890683122, 1.000000000000000000, 0.9659258262890683122, 1.000000000000000000, 0.9659258262890683122, 1.000000000000000000, 0.9659258262890683122, 1.000000000000000000, 0.9659258262890683122, 1.000000000000000000, 0.9659258262890683122, 1.000000000000000000, 0.9659258262890683122, 1.000000000000000000, 0.9659258262890683122, 1.000000000000000000, 0.9659258262890683122, 1.000000000000000000, 0.9659258262890683122, 1.000000000000000000, 0.9659258262890683122, 1.000000000000000000, 0.9659258262890683122, 1.000000000000000000, 0.9659258262890683122, 1.000000000000000000, 0.9659258262890683122, 1.000000000000000000, 0.9659258262890683122, 1.000000000000000000, 0.9659258262890683122, 1.000000000000000000, 0.9659258262890683122, 1.000000000000000000, 0.9659258262890683122, 1.000000000000000000, 0.9659258262890683122, 1.000000000000000000, 0.9659258262890683122, 1.000000000000000000, 0.9659258262890683122, 1.000000000000000000, 0.9659258262890683122, 1.000000000000000000, 0.9659258262890683122, 1.000000000000000000, 0.9659258262890683122, 1.000000000000000000, 0.9659258262890683122, 1.000000000000000000, 0.9659258262890683122, 1.000000000000000000, 0.9659258262890683122, 1.000000000000000000, 0.9659258262890683122, 1.000000000000000000, 0.9659258262890683122, 1.000000000000000000, 0.9659258262890683122, 1.000000000000000000, 0.9659258262890683122, 1.000000000000000000, 0.9659258262890683122, 1.000000000000000000, 0.9659258262890683122, 1.000000000000000000, 0.9659258262890683122, 1.000000000000000000, 0.9659258262890683122, 1.000000000000000000, 0.9659258262890683122, 1.000000000000000000, 0.9659258262890683122, 1.000000000000000000, 0.9659258262890683122, 1.000000000000000000, 0.9659258262890683122, 1.000000000000000000, 0.9659258262890683122, 1.000000000000000000, 0.9659258262890683122, 1.000000000000000000, 0.9659258262890683122, 1.000000000000000000, 0.9659258262890683122, 1.000000000000000000, 0.9659258262890683122, 1.000000000000000000, 0.9659258262890683122, 1.000000000000000000, 0.9659258262890683122, 1.000000000000000000, 0.9659258262890683122, 1.000000000000000000, 0.9659258262890683122, 1.000000000000000000, 0.9659258262890683122, 1.000000000000000000, 0.9659258262890683122, 1.000000000000000000, 0.9659258262890683122, 1.000000000000000000, 0.9659258262890683122, 1.000000000000000000, 0.9659258262890683122, 1.000000000000000000, 0.9659258262890683122, 1.000000000000000000, 0.9659258262890683122, 1.000000000000000000, 0.9659258262890683122, 1.000000000000000000, 0.9659258262890683122, 1.000000000000000000, 0.9659258262890683122, 1.000000000000000000, 0.9659258262890683122, 1.000000000000000000, 0.9659258262890683122, 1.000000000000000000, 0.9659258262890683122, 1.000000000000000000, 0.9659258262890683122, 1.000000000000000000, 0.9659258262890683122, 1.000000000000000000, 0.9659258262890683122, 1.000000000000000000, 0.9659258262890683122, 1.000000000000000000, 0.9659258262890683122, 1.000000000000000000, 0.9659258262890683122, 1.000000000000000000, 0.9659258262890683122, 1.000000000000000000, 0.9659258262890683122, 1.000000000000000000, 0.9659258262890683122, 1.000000000000000000, 0.9659258262890683122, 1.000000000000000000, 0.9659258262890683122, 1.000000000000000000, 0.9659258262890683122, 1.000000000000000000, 0.9659258262890683122, 1.000000000000000000, 0.9659258262890683122, 1.000000000000000000, 0.9659258262890683122, 1.000000000000000000, 0.9659258262890683122, 1.000000000000000000, 0.9659258262890683122, 1.000000000000000000, 0.9659258262890683122, 1.000000000000000000, 0.9659258262890683122, 1.000000000000000000, 0.9659258262890683122, 1.000000000000000000, 0.9659258262890683122, 1.000000000000000000, 0.9659258262890683122, 1.000000000000000000, 0.9659258262890683122, 1.000000000000000000, 0.9659258262890683122, 1.000000000000000000, 0.9659258262890683122, 1.000000000000000000, 0.9659258262890683122, 1.000000000000000000, 0.9659258262890683122, 1.000000000000000000, 0.9659258262890683122, 1.000000000000000000, 0.9659258262890683122, 1.000000000000000000, 0.9659258262890683122, 1.000000000000000000, 0.9659258262890683122, 1.000000000000000000, 0.9659258262890683122, 1.000000000000000000, 0.9659258262890683122, 1.000000000000000000, 0.9659258262890683122, 1.000000000000000000, 0.9659258262890683122, 1.000000000000000000, 0.9659258262890683122, 1.000000000000000000, 0.9659258262890683122, 1.000000000000000000, 0.9659258262890683122, 1.000000000000000000, 0.9659258262890683122, 1.000000000000000000, 0.9659258262890683122, 1.000000000000000000, 0.9659258262890683122, 1.000000000000000000, 0.9659258262890683122, 1.000000000000000000, 0.9659258262890683122, 1.000000000000000000, 0.9659258262890683122, 1.000000000000000000, 0.9659258262890683122, 1.000000000000000000, 0.9659258262890683122, 1.000000000000000000, 0.9659258262890683122, 1.000000000000000000, 0.9659258262890683122, 1.000000000000000000, 0.9659258262890683122, 1.000000000000000000, 0.9659258262890683122, 1.000000000000000000, 0.9659258262890683122, 1.000000000000000000, 0.9659258262890683122, 1.000000000000000000, 0.9659258262890683122, 1.000000000000000000, 0.9659258262890683122, 1.000000000000000000, 0.9659258262890683122, 1.000000000000000000, 0.9659258262890683122, 1.000000000000000000, 0.9659258262890683122, 1.000000000000000000, 0.9659258262890683122, 1.000000000000000000, 0.9659258262890683122, 1.000000000000000000, 0.9659258262890683122, 1.000000000000000000, 0.9659258262890683122, 1.000000000000000000, 0.9659258262890683122, 1.000000000000000000, 0.9659258262890683122, 1.000000000000000000, 0.9659258262890683122, 1.000000000000000000, 0.9659258262890683122, 1.000000000000000000, 0.9659258262890683122, 1.000000000000000000, 0.9659258262890683122, 1.000000000000000000, 0.9659258262890683122, 1.000000000000000000, 0.9659258262890683122, 1.000000000000000000, 0.9659258262890683122, 1.000000000000000000, 0.9659258262890683122, 1.000000000000000000, 0.9659258262890683122, 1.000000000000000000, 0.9659258262890683122, 1.000000000000000000, 0.9659258262890683122, 1.000000000000000000, 0.9659258262890683122, 1.000000000000000000, 0.9659258262890683122, 1.000000000000000000, 0.9659258262890683122, 1.000000000000000000, 0.9659258262890683122, 1.000000000000000000, 0.9659258262890683122, 1.000000000000000000, 0.9659258262890683122, 1.000000000000000000, 0.9659258262890683122, 1.000000000000000000, 0.9659258262890683122, 1.000000000000000000, 0.9659258262890683122, 1.000000000000000000, 0.9659258262890683122, 1.000000000000000000, 0.9659258262890683122, 1.000000000000000000, 0.9659258262890683122, 1.000000000000000000, 0.9659258262890683122, 1.000000000000000000, 0.9659258262890683122, 1.000000000000000000, 0.9659258262890683122, 1.000000000000000000, 0.9659258262890683122, 1.000000000000000000, 0.9659258262890683122, 1.000000000000000000, 0.9659258262890683122, 1.000000000000000000, 0.9659258262890683122, 1.000000000000000000, 0.9659258262890683122, 1.000000000000000000, 0.9659258262890683122, 1.000000000000000000, 0.9659258262890683122, 1.000000000000000000, 0.9659258262890683122, 1.000000000000000000, 0.9659258262890683122, 1.000000000000000000, 0.9659258262890683122, 1.000000000000000000, 0.9659258262890683122, 1.000000000000000000, 0.9659258262890683122, 1.000000000000000000, 0.9659258262890683122, 1.000000000000000000, 0.9659258262890683122, 1.000000000000000000, 0.9659258262890683122, 1.000000000000000000, 0.9659258262890683122, 1.000000000000000000, 0.9659258262890683122, 1.000000000000000000, 0.9659258262890683122, 1.000000000000000000, 0.9659258262890683122, 1.000000000000000000, 0.9659258262890683122, 1.000000000000000000, 0.9659258262890683122, 1.000000000000000000, 0.9659258262890683122, 1.000000000000000000, 0.9659258262890683122, 1.000000000000000000, 0.9659258262890683122, 1.000000000000000000, 0.9659258262890683122, 1.000000000000000000, 0.9659258262890683122, 1.000000000000000000, 0.9659258262890683122, 1.000000000000000000, 0.9659258262890683122, 1.000000000000000000, 0.9659258262890683122, 1.000000000000000000, 0.9659258262890683122, 1.000000000000000000, 0.9659258262890683122, 1.000000000000000000, 0.9659258262890683122, 1.000000000000000000, 0.9659258262890683122, 1.000000000000000000, 0.9659258262890683122, 1.000000000000000000, 0.9659258262890683122, 1.000000000000000000, 0.9659258262890683122, 1.000000000000000000, 0.9659258262890683122, 1.000000000000000000, 0.9659258262890683122, 1.000000000000000000, 0.9659258262890683122, 1.000000000000000000, 0.9659258262890683122, 1.000000000000000000, 0.9659258262890683122, 1.000000000000000000, 0.9659258262890683122, 1.000000000000000000, 0.9659258262890683122, 1.000000000000000000, 0.9659258262890683122, 1.000000000000000000, 0.9659258262890683122, 1.000000000000000000, 0.9659258262890683122, 1.000000000000000000, 0.9659258262890683122, 1.000000000000000000, 0.9659258262890683122, 1.000000000000000000, 0.9659258262890683122, 1.000000000000000000, 0.9659258262890683122, 1.000000000000000000, 0.9659258262890683122, 1.000000000000000000, 0.9659258262890683122, 1.000000000000000000, 0.9659258262890683122, 1.000000000000000000, 0.9659258262890683122, 1.000000000000000000, 0.9659258262890683122, 1.000000000000000000, 0.9659258262890683122, 1.000000000000000000, 0.9659258262890683122, 1.000000000000000000, 0.9659258262890683122, 1.000000000000000000, 0.9659258262890683122, 1.000000000000000000, 0.9659258262890683122, 1.000000000000000000, 0.9659258262890683122, 1.000000000000000000, 0.9659258262890683122, 1.000000000000000000, 0.9659258262890683122, 1.000000000000000000, 0.9659258262890683122, 1.000000000000000000, 0.9659258262890683122, 1.000000000000000000, 0.9659258262890683122, 1.000000000000000000, 0.9659258262890683122, 1.000000000000000000, 0.9659258262890683122, 1.000000000000000000, 0.9659258262890683122, 1.000000000000000000, 0.9659258262890683122, 1.000000000000000000, 0.9659258262890683122, 1.000000000000000000, 0.9659258262890683122, 1.000000000000000000, 0.9659258262890683122, 1.000000000000000000, 0.9659258262890683122, 1.000000000000000000, 0.9659258262890683122, 1.000000000000000000, 0.9659258262890683122, 1.000000000000000000, 0.9659258262890683122, 1.000000000000000000, 0.9659258262890683122, 1.000000000000000000, 0.9659258262890683122, 1.000000000000000000, 0.9659258262890683122, 1.000000000000000000, 0.9659258262890683122, 1.000000000000000000) ) ) 
 REPRESENTATION_ITEM ( '' )  SURFACE ( )  );
#28517=CARTESIAN_POINT ( 'NONE',  ( 1.371391076115485719, -0.6692913385826773087, -0.1292274648535924053 ) ) ;
#28518=CARTESIAN_POINT ( 'NONE',  ( -0.02624671916010428221, -0.5023911411419708095, 0.1820866141732285504 ) ) ;
#28519=CARTESIAN_POINT ( 'NONE',  ( 0.01968503937007930540, 0.1660481256975885056, 0.3530559997133364547 ) ) ;
#28520=CARTESIAN_POINT ( 'NONE',  ( -1.633858267716534529, 0.1660481256975885056, 0.3530559997133364547 ) ) ;
#28521=CARTESIAN_POINT ( 'NONE',  ( 1.620734908136483465, -0.6692913385826771977, 0.1292274648535927661 ) ) ;
#28522=CARTESIAN_POINT ( 'NONE',  ( 1.135170603674541256, -0.6692913385826773087, -0.1292274648535924053 ) ) ;
#28523=CARTESIAN_POINT ( 'NONE',  ( -0.7742782152230965886, -0.004921259842519576551, 0.3153832671262227771 ) ) ;
#28526=EDGE_CURVE ( 'NONE', #26176, #62181, #80152, .T. ) ;
#28528=CARTESIAN_POINT ( 'NONE',  ( 1.292650918635171564, 0.1771653543307087630, 0.09757992244046791164 ) ) ;
#28530=CARTESIAN_POINT ( 'NONE',  ( 0.8070866141732288002, 0.1660481256975885056, 0.3530559997133364547 ) ) ;
#28532=CARTESIAN_POINT ( 'NONE',  ( 1.404199475065617708, -0.004921259842519870586, -0.3153832671262229437 ) ) ;
#28533=CARTESIAN_POINT ( 'NONE',  ( 0.05249343832021075018, -0.6046776061558807314, 0.2411417322834647770 ) ) ;
#28534=CARTESIAN_POINT ( 'NONE',  ( -0.3083989501312330295, -0.3162353388693409650, -0.4822834645669289433 ) ) ;
#28538=CARTESIAN_POINT ( 'NONE',  ( 0.4265091863517067039, -0.5511811023622048555, -0.09757992244046775898 ) ) ;
#28542=CARTESIAN_POINT ( 'NONE',  ( -0.4921259842519677963, -0.5400638737290844871, 0.3530559997133364547 ) ) ;
#28543=PRODUCT_DEFINITION_SHAPE ( 'NONE', 'NONE',  #5877 ) ;
#28544=CARTESIAN_POINT ( 'NONE',  ( 0.8858267716535438430, -0.5400638737290845981, -0.3530559997133363437 ) ) ;
#28545=CARTESIAN_POINT ( 'NONE',  ( 0.03280839895013198948, -0.6692913385826773087, -0.1292274648535924053 ) ) ;
#28546=CARTESIAN_POINT ( 'NONE',  ( -0.3543307086614165824, 0.1771653543307087630, 0.000000000000000000 ) ) ;
#28547=CARTESIAN_POINT ( 'NONE',  ( 0.7808398950131241190, -0.05778040916215560624, -0.4822834645669293319 ) ) ;
#28548=CARTESIAN_POINT ( 'NONE',  ( -0.7677165354330699465, -0.5400638737290845981, -0.3530559997133363437 ) ) ;
#28549=CARTESIAN_POINT ( 'NONE',  ( -0.2034120734908131112, -0.6692913385826773087, -0.1292274648535924053 ) ) ;
#28550=CARTESIAN_POINT ( 'NONE',  ( -0.9776902887139098386, -0.6692913385826771977, 0.1292274648535927661 ) ) ;
#28551=CARTESIAN_POINT ( 'NONE',  ( 1.345144356955381593, -0.3162353388693409650, -0.4822834645669289433 ) ) ;
#28552=AXIS2_PLACEMENT_3D ( 'NONE', #64963, #8556, #34224 ) ;
#28553=CARTESIAN_POINT ( 'NONE',  ( 0.8792650918635177559, -0.4281496062992127816, -0.4176697321401328100 ) ) ;
#28555=CARTESIAN_POINT ( 'NONE',  ( 0.7808398950131241190, -0.05778040916215560624, -0.4822834645669293319 ) ) ;
#28557=CARTESIAN_POINT ( 'NONE',  ( -0.05249343832020911260, 0.1283753931104748280, 0.1820866141732283561 ) ) ;
#28561=CARTESIAN_POINT ( 'NONE',  ( -0.9055118110236215490, 0.1771653543307087630, 0.000000000000000000 ) ) ;
#28562=CARTESIAN_POINT ( 'NONE',  ( -0.4986876640419939388, 0.2306618581243847221, -0.2411417322834647770 ) ) ;
#28564=CARTESIAN_POINT ( 'NONE',  ( -0.09186351706036689768, 0.05413385826771626580, -0.4176697321401330321 ) ) ;
#28565=CARTESIAN_POINT ( 'NONE',  ( -0.4921259842519677963, -0.5400638737290844871, 0.3530559997133364547 ) ) ;
#28566=CARTESIAN_POINT ( 'NONE',  ( -1.410761154855641575, -0.3162353388693409650, -0.4822834645669289433 ) ) ;
#28567=CARTESIAN_POINT ( 'NONE',  ( -1.528871391076114250, 0.2952755905511810774, -0.1292274648535930714 ) ) ;
#28568=CARTESIAN_POINT ( 'NONE',  ( 1.043307086614173818, 0.07958543189024085140, 0.2665933059059887866 ) ) ;
#28571=CARTESIAN_POINT ( 'NONE',  ( 0.3543307086614179147, 0.1771653543307087630, 0.000000000000000000 ) ) ;
#28572=CARTESIAN_POINT ( 'NONE',  ( -0.01968503937007793844, 0.1660481256975883668, -0.3530559997133364547 ) ) ;
#28573=CARTESIAN_POINT ( 'NONE',  ( 0.4133858267716541968, 0.1660481256975885056, 0.3530559997133364547 ) ) ;
#28574=ORIENTED_EDGE ( 'NONE', *, *, #40435, .T. ) ;
#28576=CARTESIAN_POINT ( 'NONE',  ( -2.795275590551184131, 1.062992125984252079, -2.654250759839014936E-16 ) ) ;
#28580=CARTESIAN_POINT ( 'NONE',  ( -0.6692913385826764205, -0.5511811023622047445, 6.969142054262312111E-17 ) ) ;
#28581=CARTESIAN_POINT ( 'NONE',  ( -0.6233595800524928121, -0.05778040916215522460, 0.4822834645669289988 ) ) ;
#28585=CARTESIAN_POINT ( 'NONE',  ( 1.581364829396326277, -0.3162353388693409650, -0.4822834645669289433 ) ) ;
#28586=CARTESIAN_POINT ( 'NONE',  ( 0.8136482939632553313, 0.2306618581243848609, 0.2411417322834645549 ) ) ;
#28587=CARTESIAN_POINT ( 'NONE',  ( 1.010498687664042716, -0.4281496062992124485, 0.4176697321401328655 ) ) ;
#28588=CARTESIAN_POINT ( 'NONE',  ( -0.5708661417322825615, -0.4536011799217367080, 0.2665933059059888421 ) ) ;
#28589=CARTESIAN_POINT ( 'NONE',  ( 0.1837270341207354329, 0.2306618581243848609, 0.2411417322834645549 ) ) ;
#28591=CARTESIAN_POINT ( 'NONE',  ( -0.06561679790026180015, -0.004921259842519576551, 0.3153832671262227771 ) ) ;
#28592=CARTESIAN_POINT ( 'NONE',  ( -0.6496062992125976043, -0.5400638737290844871, 0.3530559997133364547 ) ) ;
#28594=CARTESIAN_POINT ( 'NONE',  ( 1.515748031496063186, -0.4536011799217368745, -0.2665933059059886201 ) ) ;
#28595=CARTESIAN_POINT ( 'NONE',  ( -0.05249343832020938322, -0.5023911411419708095, -0.1820866141732282451 ) ) ;
#28596=CARTESIAN_POINT ( 'NONE',  ( 1.463254593175853824, -0.5511811023622046335, 0.09757992244046803654 ) ) ;
#28597=CARTESIAN_POINT ( 'NONE',  ( -1.194225721784776262, 0.05413385826771626580, -0.4176697321401330321 ) ) ;
#28598=CARTESIAN_POINT ( 'NONE',  ( -0.6496062992125976043, 0.07958543189024071263, -0.2665933059059888421 ) ) ;
#28599=CARTESIAN_POINT ( 'NONE',  ( -1.168682819302786058, -2.294479370626195693E-15, 0.3464511005275217603 ) ) ;
#28600=CARTESIAN_POINT ( 'NONE',  ( -1.062992125984250968, 0.2952755905511811885, 0.000000000000000000 ) ) ;
#28601=CARTESIAN_POINT ( 'NONE',  ( -0.2034120734908128059, 0.2952755905511811885, 0.1292274648535926551 ) ) ;
#28605=CARTESIAN_POINT ( 'NONE',  ( 0.4330708661417329575, 0.1771653543307087630, 0.000000000000000000 ) ) ;
#28606=CARTESIAN_POINT ( 'NONE',  ( 0.8727034120734912248, -0.3162353388693409650, -0.4822834645669289433 ) ) ;
#28607=CARTESIAN_POINT ( 'NONE',  ( -1.279527559055116948, -0.4536011799217367080, 0.2665933059059888421 ) ) ;
#28608=CARTESIAN_POINT ( 'NONE',  ( 1.358267716535433323, 0.1660481256975885056, 0.3530559997133364547 ) ) ;
#28609=CARTESIAN_POINT ( 'NONE',  ( -1.456692913385826182, -0.5511811023622047445, 6.969142054262312111E-17 ) ) ;
#28610=AXIS2_PLACEMENT_3D ( 'NONE', #26088, #45014, #71133 ) ;
#28611=CARTESIAN_POINT ( 'NONE',  ( -0.4724409448818890911, -0.1870078740157479769, 0.4822834645669291653 ) ) ;
#28612=CARTESIAN_POINT ( 'NONE',  ( 0.07874015748031558404, -0.1870078740157479769, 0.3641732283464567677 ) ) ;
#28613=DIRECTION ( 'NONE',  ( 0.7071067811865495711, 0.000000000000000000, -0.7071067811865454633 ) ) ;
#28614=CARTESIAN_POINT ( 'NONE',  ( 0.6036745406824153282, -0.5023911411419708095, 0.1820866141732285504 ) ) ;
#28615=CARTESIAN_POINT ( 'NONE',  ( 0.05905511811023709395, -0.5400638737290844871, 0.3530559997133364547 ) ) ;
#28617=CARTESIAN_POINT ( 'NONE',  ( -1.069553805774277722, 0.2952755905511811885, 0.1292274648535926551 ) ) ;
#28619=CARTESIAN_POINT ( 'NONE',  ( 1.056430446194226436, -0.5511811023622048555, -0.09757992244046775898 ) ) ;
#28620=CARTESIAN_POINT ( 'NONE',  ( -0.05249343832020911260, 0.2306618581243848609, 0.2411417322834645549 ) ) ;
#28621=CARTESIAN_POINT ( 'NONE',  ( -0.4330708661417315697, -0.6692913385826771977, 8.415575281601705876E-17 ) ) ;
#28622=CARTESIAN_POINT ( 'NONE',  ( -0.4593175853018364174, -0.3690944881889765550, -0.3153832671262227771 ) ) ;
#28623=CARTESIAN_POINT ( 'NONE',  ( 1.192688228555126795, 0.02791078216816225699, 0.4328096321851905293 ) ) ;
#28624=CARTESIAN_POINT ( 'NONE',  ( -0.4199475065616791736, -0.5023911411419708095, 0.1820866141732285504 ) ) ;
#28625=CARTESIAN_POINT ( 'NONE',  ( 0.2821522309711292364, 0.2952755905511810774, -0.1292274648535930714 ) ) ;
#28626=EDGE_CURVE ( 'NONE', #58699, #36200, #23108, .T. ) ;
#28627=CARTESIAN_POINT ( 'NONE',  ( -0.5380577427821514602, -0.3690944881889765550, -0.3153832671262227771 ) ) ;
#28629=CARTESIAN_POINT ( 'NONE',  ( -1.292650918635170010, 0.2952755905511810774, -0.1292274648535930714 ) ) ;
#28633=CARTESIAN_POINT ( 'NONE',  ( -0.9580052493438311334, -0.3690944881889763329, 0.3153832671262228327 ) ) ;
#28634=CARTESIAN_POINT ( 'NONE',  ( -0.4921259842519677963, -0.5400638737290844871, 0.3530559997133364547 ) ) ;
#28635=CARTESIAN_POINT ( 'NONE',  ( -1.614173228346456268, -0.6692913385826771977, 8.415575281601705876E-17 ) ) ;
#28636=CARTESIAN_POINT ( 'NONE',  ( -1.371391076115484609, -0.6692913385826771977, 0.1292274648535927661 ) ) ;
#28638=CARTESIAN_POINT ( 'NONE',  ( 1.423884514435696413, -0.3162353388693409650, -0.4822834645669289433 ) ) ;
#28639=CARTESIAN_POINT ( 'NONE',  ( 1.062992125984252745, 0.2952755905511811885, 0.000000000000000000 ) ) ;
#28642=CARTESIAN_POINT ( 'NONE',  ( 1.430446194225722500, -0.004921259842519576551, 0.3153832671262227771 ) ) ;
#28645=CARTESIAN_POINT ( 'NONE',  ( -0.6955380577427815458, -0.004921259842519576551, 0.3153832671262227771 ) ) ;
#28648=CARTESIAN_POINT ( 'NONE',  ( 0.6364829396325465405, -0.05778040916215522460, 0.4822834645669289988 ) ) ;
#28649=CARTESIAN_POINT ( 'NONE',  ( -0.4330708661417315697, 0.2952755905511811885, 0.000000000000000000 ) ) ;
#28650=CARTESIAN_POINT ( 'NONE',  ( -0.5249343832020990641, 0.2306618581243848609, 0.2411417322834645549 ) ) ;
#28651=CARTESIAN_POINT ( 'NONE',  ( 1.594488188976378673, -0.5400638737290845981, -0.3530559997133363437 ) ) ;
#28653=CARTESIAN_POINT ( 'NONE',  ( -1.253280839895012377, -0.2845877964562161244, -0.3641732283464567121 ) ) ;
#28655=CARTESIAN_POINT ( 'NONE',  ( 0.2362204724409456558, -0.1870078740157479769, 0.4822834645669291653 ) ) ;
#28656=CARTESIAN_POINT ( 'NONE',  ( -0.8202099737532799750, 0.2952755905511810774, -0.1292274648535930714 ) ) ;
#28658=CARTESIAN_POINT ( 'NONE',  ( -1.397637795275589623, -0.5400638737290845981, -0.3530559997133363437 ) ) ;
#28660=CARTESIAN_POINT ( 'NONE',  ( 1.128608923884515169, -0.6046776061558809534, -0.2411417322834644161 ) ) ;
#28661=CARTESIAN_POINT ( 'NONE',  ( 1.332020997375329197, -0.2845877964562159024, 0.3641732283464567677 ) ) ;
#28662=EDGE_LOOP ( 'NONE', ( #44564, #36197, #82410, #80642 ) ) ;
#28664=CARTESIAN_POINT ( 'NONE',  ( -0.4133858267716528645, -0.5400638737290844871, 0.3530559997133364547 ) ) ;
#28665=ORIENTED_EDGE ( 'NONE', *, *, #45132, .T. ) ;
#28666=CARTESIAN_POINT ( 'NONE',  ( 0.4133858267716541968, -0.4536011799217368745, -0.2665933059059886201 ) ) ;
#28667=CARTESIAN_POINT ( 'NONE',  ( -1.108923884514435132, -0.3162353388693405765, 0.4822834645669290543 ) ) ;
#28668=CARTESIAN_POINT ( 'NONE',  ( 0.8070866141732288002, 0.1660481256975885056, 0.3530559997133364547 ) ) ;
#28669=CARTESIAN_POINT ( 'NONE',  ( 0.6496062992125991586, 0.1660481256975885056, 0.3530559997133364547 ) ) ;
#28670=CARTESIAN_POINT ( 'NONE',  ( -0.1771653543307080136, -0.5400638737290844871, 0.3530559997133364547 ) ) ;
#28671=AXIS2_PLACEMENT_3D ( 'NONE', #25600, #37825, #51263 ) ;
#28672=CARTESIAN_POINT ( 'NONE',  ( -0.6955380577427815458, 0.05413385826771666132, 0.4176697321401328100 ) ) ;
#28674=CARTESIAN_POINT ( 'NONE',  ( -1.574803149606298636, -0.1870078740157479769, 0.4822834645669291653 ) ) ;
#28675=CARTESIAN_POINT ( 'NONE',  ( -0.6627296587926501115, 0.2952755905511810774, -0.1292274648535930714 ) ) ;
#28676=CARTESIAN_POINT ( 'NONE',  ( -0.3477690288713902178, 0.1771653543307087075, -0.09757992244046823083 ) ) ;
#28677=CARTESIAN_POINT ( 'NONE',  ( 1.469816272965879911, -0.6046776061558807314, 0.2411417322834647770 ) ) ;
#28678=CARTESIAN_POINT ( 'NONE',  ( 1.437007874015748810, -0.5400638737290845981, -0.3530559997133363437 ) ) ;
#28679=CARTESIAN_POINT ( 'NONE',  ( -1.010498687664041384, -0.4281496062992127816, -0.4176697321401328100 ) ) ;
#28681=CARTESIAN_POINT ( 'NONE',  ( 0.7611548556430451917, -0.6046776061558807314, 0.2411417322834647770 ) ) ;
#28684=CARTESIAN_POINT ( 'NONE',  ( -0.2690288713910754526, -0.6692913385826771977, 0.1292274648535927661 ) ) ;
#28685=CARTESIAN_POINT ( 'NONE',  ( -0.9645669291338575535, 0.07958543189024071263, -0.2665933059059888421 ) ) ;
#28686=CARTESIAN_POINT ( 'NONE',  ( 1.141732283464567788, -0.5511811023622047445, 6.969142054262312111E-17 ) ) ;
#28688=CARTESIAN_POINT ( 'NONE',  ( 1.148293963254593875, -0.5511811023622046335, 0.09757992244046803654 ) ) ;
#28689=CARTESIAN_POINT ( 'NONE',  ( 0.6299212598425204535, -0.1870078740157479769, 0.4822834645669291653 ) ) ;
#28691=CARTESIAN_POINT ( 'NONE',  ( -0.5249343832020990641, -0.6046776061558809534, -0.2411417322834644161 ) ) ;
#28692=CARTESIAN_POINT ( 'NONE',  ( -0.3812812444996365180, -2.294479370626195693E-15, 0.3464511005275217603 ) ) ;
#28693=CARTESIAN_POINT ( 'NONE',  ( 1.305774278215223960, 0.1771653543307087075, -0.09757992244046823083 ) ) ;
#28694=CARTESIAN_POINT ( 'NONE',  ( -0.4658792650918627265, -0.05778040916215522460, 0.4822834645669289988 ) ) ;
#28696=CARTESIAN_POINT ( 'NONE',  ( 1.122047244094488860, -0.5400638737290845981, -0.3530559997133363437 ) ) ;
#28697=CARTESIAN_POINT ( 'NONE',  ( 0.1771653543307093182, 0.1660481256975885056, 0.3530559997133364547 ) ) ;
#28698=CARTESIAN_POINT ( 'NONE',  ( 0.7086614173228353852, -0.1870078740157479769, 0.3641732283464567677 ) ) ;
#28700=CARTESIAN_POINT ( 'NONE',  ( 0.2952755905511819101, 0.07958543189024071263, -0.2665933059059888421 ) ) ;
#28701=CARTESIAN_POINT ( 'NONE',  ( -1.089589480386152998, 0.004960608223778174841, 0.3437734562760193513 ) ) ;
#28703=CARTESIAN_POINT ( 'NONE',  ( 0.8398950131233602345, -0.6046776061558807314, 0.2411417322834647770 ) ) ;
#28705=CARTESIAN_POINT ( 'NONE',  ( 1.502624671916010790, -0.08942795157527998196, 0.3641732283464567121 ) ) ;
#28707=CARTESIAN_POINT ( 'NONE',  ( 0.2099737532808405305, 0.1283753931104746893, -0.1820866141732285504 ) ) ;
#28708=CARTESIAN_POINT ( 'NONE',  ( 0.05249343832021075018, -0.6046776061558807314, 0.2411417322834647770 ) ) ;
#28709=CARTESIAN_POINT ( 'NONE',  ( 1.371391076115485941, 0.1771653543307087630, 0.09757992244046791164 ) ) ;
#28710=CARTESIAN_POINT ( 'NONE',  ( -1.292650918635170010, -0.5511811023622046335, 0.09757992244046803654 ) ) ;
#28711=CARTESIAN_POINT ( 'NONE',  ( -1.522309711286088607, 0.2306618581243847221, -0.2411417322834647770 ) ) ;
#28712=AXIS2_PLACEMENT_3D ( 'NONE', #57572, #58840, #83264 ) ;
#28713=CARTESIAN_POINT ( 'NONE',  ( 0.3805774278215230400, -0.4281496062992124485, 0.4176697321401328655 ) ) ;
#28714=CARTESIAN_POINT ( 'NONE',  ( 1.246719160104987623, 0.05413385826771626580, -0.4176697321401330321 ) ) ;
#28716=CARTESIAN_POINT ( 'NONE',  ( 0.5052493438320215802, 0.2952755905511811885, 0.1292274648535926551 ) ) ;
#28717=CARTESIAN_POINT ( 'NONE',  ( 1.345144356955381593, -0.05778040916215522460, 0.4822834645669289988 ) ) ;
#28718=CARTESIAN_POINT ( 'NONE',  ( 0.8070866141732289112, -0.5400638737290845981, -0.3530559997133363437 ) ) ;
#28720=CARTESIAN_POINT ( 'NONE',  ( 0.6299212598425204535, -0.1870078740157480601, -0.3641732283464567677 ) ) ;
#28721=CARTESIAN_POINT ( 'NONE',  ( -1.633858267716534529, 0.07958543189024085140, 0.2665933059059887866 ) ) ;
#28722=CARTESIAN_POINT ( 'NONE',  ( -0.9580052493438311334, -0.004921259842519870586, -0.3153832671262229437 ) ) ;
#28724=CARTESIAN_POINT ( 'NONE',  ( 0.6364829396325465405, -0.08942795157527998196, 0.3641732283464567121 ) ) ;
#28726=CARTESIAN_POINT ( 'NONE',  ( -0.01968503937007793844, 0.1660481256975883668, -0.3530559997133364547 ) ) ;
#28727=CARTESIAN_POINT ( 'NONE',  ( 0.6496062992125991586, 0.1660481256975885056, 0.3530559997133364547 ) ) ;
#28728=CARTESIAN_POINT ( 'NONE',  ( -0.4658792650918627265, -0.3162353388693409650, -0.4822834645669289433 ) ) ;
#28729=CARTESIAN_POINT ( 'NONE',  ( 0.2952755905511816326, -0.4536011799217367080, 0.2665933059059888421 ) ) ;
#28730=CARTESIAN_POINT ( 'NONE',  ( 0.8595800524934390507, -0.05778040916215560624, -0.4822834645669293319 ) ) ;
#28732=CARTESIAN_POINT ( 'NONE',  ( -0.8727034120734901146, -0.05778040916215560624, -0.4822834645669293319 ) ) ;
#28733=CARTESIAN_POINT ( 'NONE',  ( -1.089238845144356427, 0.05413385826771666132, 0.4176697321401328100 ) ) ;
#28736=CARTESIAN_POINT ( 'NONE',  ( -0.7939632545931750718, -0.05778040916215560624, -0.4822834645669293319 ) ) ;
#28737=CARTESIAN_POINT ( 'NONE',  ( -0.6364829396325453192, -0.3162353388693405765, 0.4822834645669290543 ) ) ;
#28741=CARTESIAN_POINT ( 'NONE',  ( 0.8464566929133866546, -0.4536011799217367080, 0.2665933059059888421 ) ) ;
#28743=CARTESIAN_POINT ( 'NONE',  ( 1.233595800524935227, -0.6046776061558807314, 0.2411417322834647770 ) ) ;
#28745=CARTESIAN_POINT ( 'NONE',  ( -1.167979002624671470, -0.3690944881889765550, -0.3153832671262227771 ) ) ;
#28746=CARTESIAN_POINT ( 'NONE',  ( 1.522309711286089939, 0.2306618581243848609, 0.2411417322834645549 ) ) ;
#28747=CARTESIAN_POINT ( 'NONE',  ( -1.692913385826770645, 0.2952755905511811885, 0.000000000000000000 ) ) ;
#28748=CARTESIAN_POINT ( 'NONE',  ( 0.5052493438320218022, -0.6692913385826773087, -0.1292274648535924053 ) ) ;
#28750=CARTESIAN_POINT ( 'NONE',  ( -0.06561679790026180015, 0.05413385826771666132, 0.4176697321401328100 ) ) ;
#28751=CARTESIAN_POINT ( 'NONE',  ( -0.8595800524934373854, -0.2845877964562161244, -0.3641732283464567121 ) ) ;
#28752=CARTESIAN_POINT ( 'NONE',  ( 0.7480314960629927956, -0.6692913385826771977, 8.415575281601705876E-17 ) ) ;
#28753=CARTESIAN_POINT ( 'NONE',  ( -0.01312335958005186876, -0.4281496062992124485, 0.4176697321401328655 ) ) ;
#28757=CARTESIAN_POINT ( 'NONE',  ( 0.9580052493438327987, -0.4281496062992127816, -0.4176697321401328100 ) ) ;
#28758=CARTESIAN_POINT ( 'NONE',  ( -0.04593175853018302557, -0.6692913385826773087, -0.1292274648535924053 ) ) ;
#28759=CARTESIAN_POINT ( 'NONE',  ( -1.069553805774277722, -0.6692913385826773087, -0.1292274648535924053 ) ) ;
#28760=CARTESIAN_POINT ( 'NONE',  ( 0.9973753280839902091, 0.2306618581243847221, -0.2411417322834647770 ) ) ;
#28761=CARTESIAN_POINT ( 'NONE',  ( 0.3871391076115493490, -0.3162353388693405765, 0.4822834645669290543 ) ) ;
#28763=CARTESIAN_POINT ( 'NONE',  ( -0.4986876640419942164, -0.6046776061558807314, 0.2411417322834647770 ) ) ;
#28764=CARTESIAN_POINT ( 'NONE',  ( 0.8005249343832028242, -0.4281496062992127816, -0.4176697321401328100 ) ) ;
#28765=CARTESIAN_POINT ( 'NONE',  ( 0.1181102362204730916, 0.2952755905511811885, 0.000000000000000000 ) ) ;
#28767=CARTESIAN_POINT ( 'NONE',  ( 0.8136482939632553313, -0.5023911411419708095, -0.1820866141732282451 ) ) ;
#28768=CARTESIAN_POINT ( 'NONE',  ( -1.404199475065615932, 0.05413385826771666132, 0.4176697321401328100 ) ) ;
#28770=CARTESIAN_POINT ( 'NONE',  ( 0.2952755905511816326, -0.5400638737290844871, 0.3530559997133364547 ) ) ;
#28774=ORIENTED_EDGE ( 'NONE', *, *, #75224, .T. ) ;
#28775=CARTESIAN_POINT ( 'NONE',  ( 1.279527559055118724, -0.5400638737290845981, -0.3530559997133363437 ) ) ;
#28776=CARTESIAN_POINT ( 'NONE',  ( 0.5314960629921264834, 0.07958543189024071263, -0.2665933059059888421 ) ) ;
#28778=CARTESIAN_POINT ( 'NONE',  ( 0.2238009295390077091, 2.409604939980833412E-17, -0.3464511005275205946 ) ) ;
#28784=CARTESIAN_POINT ( 'NONE',  ( -0.7742782152230962556, -0.4281496062992127816, -0.4176697321401328100 ) ) ;
#28785=CARTESIAN_POINT ( 'NONE',  ( -0.5774278215223089816, 0.2306618581243847221, -0.2411417322834647770 ) ) ;
#28786=CARTESIAN_POINT ( 'NONE',  ( 0.8202099737532813073, 0.2952755905511811885, 0.1292274648535926551 ) ) ;
#28788=CARTESIAN_POINT ( 'NONE',  ( 1.417322834645670104, -0.1870078740157479769, 0.4822834645669291653 ) ) ;
#28789=FACE_OUTER_BOUND ( 'NONE', #29455, .T. ) ;
#28792=CARTESIAN_POINT ( 'NONE',  ( -1.253280839895012377, -0.2845877964562161244, -0.3641732283464567121 ) ) ;
#28794=CARTESIAN_POINT ( 'NONE',  ( 0.1640419947506569498, -0.3162353388693409650, -0.4822834645669289433 ) ) ;
#28795=CARTESIAN_POINT ( 'NONE',  ( 1.496062992125985147, -0.1870078740157479769, 0.4822834645669291653 ) ) ;
#28797=CARTESIAN_POINT ( 'NONE',  ( -1.292650918635170010, -0.5511811023622046335, 0.09757992244046803654 ) ) ;
#28798=CARTESIAN_POINT ( 'NONE',  ( 0.6299212598425204535, -0.1870078740157480879, -0.4822834645669291653 ) ) ;
#28799=CARTESIAN_POINT ( 'NONE',  ( 1.200787401574803681, -0.4536011799217368745, -0.2665933059059886201 ) ) ;
#28801=CARTESIAN_POINT ( 'NONE',  ( -1.430446194225721390, -0.3690944881889763329, 0.3153832671262228327 ) ) ;
#28802=CARTESIAN_POINT ( 'NONE',  ( 1.430446194225722500, -0.4281496062992127816, -0.4176697321401328100 ) ) ;
#28804=CARTESIAN_POINT ( 'NONE',  ( -0.01312335958005186876, -0.4281496062992124485, 0.4176697321401328655 ) ) ;
#28805=CARTESIAN_POINT ( 'NONE',  ( -1.259842519685038686, -0.1870078740157480601, -0.3641732283464567677 ) ) ;
#28806=CARTESIAN_POINT ( 'NONE',  ( -0.4724409448818890911, -0.1870078740157479769, 0.3641732283464567677 ) ) ;
#28807=CARTESIAN_POINT ( 'NONE',  ( -0.6627296587926503335, -0.6692913385826771977, 0.1292274648535927661 ) ) ;
#28808=CARTESIAN_POINT ( 'NONE',  ( -1.391076115485563314, -0.5023911411419708095, -0.1820866141732282451 ) ) ;
#28810=CARTESIAN_POINT ( 'NONE',  ( 0.3215223097112867578, -0.05778040916215522460, 0.4822834645669289988 ) ) ;
#28814=CARTESIAN_POINT ( 'NONE',  ( -1.089238845144356427, 0.05413385826771666132, 0.4176697321401328100 ) ) ;
#28815=CARTESIAN_POINT ( 'NONE',  ( -0.4068241469816267775, -0.004921259842519870586, -0.3153832671262229437 ) ) ;
#28816=CARTESIAN_POINT ( 'NONE',  ( 0.1115485564304470323, 0.2952755905511811885, 0.1292274648535926551 ) ) ;
#28817=CARTESIAN_POINT ( 'NONE',  ( 0.3937007874015754361, -0.1870078740157479769, 0.3641732283464567677 ) ) ;
#28818=CARTESIAN_POINT ( 'NONE',  ( -0.5446194225721777693, -0.2845877964562161244, -0.3641732283464567121 ) ) ;
#28819=CARTESIAN_POINT ( 'NONE',  ( -1.128608923884513837, -0.6046776061558807314, 0.2411417322834647770 ) ) ;
#28820=CARTESIAN_POINT ( 'NONE',  ( -1.430446194225721390, -0.4281496062992124485, 0.4176697321401328655 ) ) ;
#28822=CARTESIAN_POINT ( 'NONE',  ( 1.423884514435696413, -0.3162353388693409650, -0.4822834645669289433 ) ) ;
#28824=CARTESIAN_POINT ( 'NONE',  ( 1.049868766404200349, 0.1283753931104748280, 0.1820866141732283561 ) ) ;
#28825=CARTESIAN_POINT ( 'NONE',  ( 0.9251968503937015864, 0.1660481256975883668, -0.3530559997133364547 ) ) ;
#28826=LINE ( 'NONE', #5524, #52800 ) ;
#28827=CARTESIAN_POINT ( 'NONE',  ( 1.456692913385827515, 0.1771653543307087630, 0.000000000000000000 ) ) ;
#28829=CARTESIAN_POINT ( 'NONE',  ( -0.9120734908136475250, -0.6692913385826773087, -0.1292274648535924053 ) ) ;
#28830=CARTESIAN_POINT ( 'NONE',  ( -1.003937007874014853, 0.1660481256975885056, 0.3530559997133364547 ) ) ;
#28831=CARTESIAN_POINT ( 'NONE',  ( 0.3149606299212603933, -0.1870078740157479769, 0.4822834645669291653 ) ) ;
#28832=CARTESIAN_POINT ( 'NONE',  ( -1.607611548556429737, -0.5511811023622046335, 0.09757992244046803654 ) ) ;
#28834=CARTESIAN_POINT ( 'NONE',  ( 1.384514435695538337, -0.5511811023622046335, 0.09757992244046803654 ) ) ;
#28835=CARTESIAN_POINT ( 'NONE',  ( 0.6167979002624679463, 0.05413385826771626580, -0.4176697321401330321 ) ) ;
#28836=CARTESIAN_POINT ( 'NONE',  ( 0.9317585301837276734, -0.4281496062992124485, 0.4176697321401328655 ) ) ;
#28837=CARTESIAN_POINT ( 'NONE',  ( -1.604771003085130099, 1.278209470906376932, -0.1466069496707745889 ) ) ;
#28844=CARTESIAN_POINT ( 'NONE',  ( -0.2493438320209966919, -0.004921259842519870586, -0.3153832671262229437 ) ) ;
#28845=CARTESIAN_POINT ( 'NONE',  ( -0.5052493438320203589, -0.6692913385826771977, 0.1292274648535927661 ) ) ;
#28846=CARTESIAN_POINT ( 'NONE',  ( 1.056430446194226436, -0.6692913385826773087, -0.1292274648535924053 ) ) ;
#28848=CARTESIAN_POINT ( 'NONE',  ( 0.1049868766404206816, 0.1283753931104748280, 0.1820866141732283561 ) ) ;
#28849=CARTESIAN_POINT ( 'NONE',  ( -1.312335958005248715, 0.2306618581243848609, 0.2411417322834645549 ) ) ;
#28850=CARTESIAN_POINT ( 'NONE',  ( 1.259842519685040019, -0.1870078740157479769, 0.4822834645669291653 ) ) ;
#28854=ORIENTED_EDGE ( 'NONE', *, *, #26244, .F. ) ;
#28856=CARTESIAN_POINT ( 'NONE',  ( 1.194225721784777594, -0.4281496062992127816, -0.4176697321401328100 ) ) ;
#28857=CARTESIAN_POINT ( 'NONE',  ( -1.509186351706035767, 0.05413385826771626580, -0.4176697321401330321 ) ) ;
#28858=CARTESIAN_POINT ( 'NONE',  ( -1.227034120734907141, -0.5511811023622048555, -0.09757992244046775898 ) ) ;
#28859=CARTESIAN_POINT ( 'NONE',  ( 1.502624671916010790, -0.3162353388693409650, -0.4822834645669289433 ) ) ;
#28861=CARTESIAN_POINT ( 'NONE',  ( -1.011202504342156416, -2.294479370626195693E-15, 0.3464511005275217603 ) ) ;
#28862=CARTESIAN_POINT ( 'NONE',  ( 1.259842519685040019, -0.1870078740157480879, -0.4822834645669291653 ) ) ;
#28864=CARTESIAN_POINT ( 'NONE',  ( -0.1509186351706028884, -0.05778040916215522460, 0.4822834645669289988 ) ) ;
#28865=CARTESIAN_POINT ( 'NONE',  ( -0.5511811023622041894, -0.1870078740157480879, -0.4822834645669291653 ) ) ;
#28866=CARTESIAN_POINT ( 'NONE',  ( 1.482939632545932307, 0.05413385826771626580, -0.4176697321401330321 ) ) ;
#28868=CARTESIAN_POINT ( 'NONE',  ( 0.4002624671916016896, -0.3162353388693409650, -0.4822834645669289433 ) ) ;
#28870=CARTESIAN_POINT ( 'NONE',  ( -1.187664041994749731, -0.2845877964562159024, 0.3641732283464567677 ) ) ;
#28875=CARTESIAN_POINT ( 'NONE',  ( -1.601049868766403650, -0.6046776061558807314, 0.2411417322834647770 ) ) ;
#28877=CARTESIAN_POINT ( 'NONE',  ( -0.7874015748031497619, 1.968503937007873850, 0.000000000000000000 ) ) ;
#28879=CARTESIAN_POINT ( 'NONE',  ( 0.4133858267716541968, 0.1660481256975885056, 0.3530559997133364547 ) ) ;
#28880=FACE_OUTER_BOUND ( 'NONE', #81084, .T. ) ;
#28882=( BOUNDED_SURFACE ( )  B_SPLINE_SURFACE ( 1, 2, ( 
 ( #78645, #7933, #26857, #78224, #45369, #20136, #51675, #782, #26443, #64326, #20968, #33594, #45784, #71483, #66005, #1616, #7513, #33181, #14669, #6662, #32334, #57996, #360, #26017, #42378, #10421, #10000, #21790, #54178, #61329, #15077, #80715, #73571, #35254, #15916, #23030, #67253, #47867, #16738, #74394, #48282, #9585, #47037, #73980, #3269, #40735, #66419, #53763, #61750, #22623, #29755, #8755, #60096, #9176, #34847, #80308, #55007, #16326, #67663, #48696, #28109, #79892, #41970, #60918, #72731, #47452, #2451, #34431, #81125, #79474, #68077, #73147, #60510, #29348, #66842, #15496, #35665, #4087, #41154, #36079, #54599, #55418, #3683, #28930, #2858, #28522, #22210, #41564, #5729, #82356, #62990, #5329, #81538, #4918, #4500, #49524, #23857, #57479, #57065, #37317, #30586, #43194, #18781, #24674, #56252, #75632, #56655, #17970, #12470, #42790, #70119, #63806, #44424, #38132, #69718, #75217, #81948, #37720, #74812, #82759, #49934, #11659, #43607, #24261, #63394, #17157, #6145, #31400, #69309, #36900, #31819, #68485, #10824, #36484, #30987, #17562, #25080, #62159, #30167, #50754, #23442, #68890, #50342, #76039, #18384, #49106, #44025, #55830, #11240, #12062, #62576, #76454, #260, #38960, #19187, #38549, #76854, #7831, #59160, #33498, #72223, #46524, #1518, #13728, #1105, #83173, #65908, #51159, #57893, #58315, #14574, #64229, #25912, #51572, #77275, #32235, #6563, #19605, #14152, #65067, #26756, #71799, #45267, #70963, #65499, #45682, #46106, #52411, #13308, #58743, #39808, #27172, #39382, #71378, #64644, #52834, #6981, #51996, #680, #78120, #32650, #20453, #26335, #77701, #78546, #20871, #40226, #44836, #20031, #7405, #8245, #33910, #33076, #25493, #70534, #12890, #41471, #81334, #62363, #81749, #40638, #55625, #56041, #49319, #75427, #23648, #17769, #69100, #4701, #30374, #66320, #54081, #15822, #78965, #21284, #46939, #11031, #2351, #29960, #4297, #34751, #79796, #8659, #67156, #36688, #11448, #72631, #14979, #53253, #34330, #60820, #75020, #9485, #41056, #17366, #66744, #59995, #43401, #59574, #42994, #24060, #49729, #28007, #35160, #53667, #68689, #79374, #1930, #21693, #47356, #27593, #73045, #9080, #15394, #60411, #2762, #28421, #22112, #47772, #73473, #70328, #77492, #45477, #44225, #12269, #31610, #50955, #57689, #71174, #77069, #6771, #64436, #38342, #57271, #37104, #64017, #76652, #30790, #5123, #43810, #51788, #12684, #19827, #56454, #50138, #82558, #24876, #6358, #45053, #32030, #51, #13105, #18177, #69915, #25705, #82969, #62789, #11863, #75836, #82156, #24471, #69514, #38759, #37516, #50544, #19402, #56861, #63191, #51365, #5531, #31195, #32443, #44632, #26127, #70754, #25287, #58105, #471, #76248, #18582, #37927, #63604, #18984, #5940, #71591, #78336, #77914, #39600, #13943, #47567, #47150, #27383, #20667, #33299, #8864, #72431, #46320, #65714, #46739, #8045, #2558, #32866, #60208, #53875, #34542, #28216, #59784, #65289, #72013, #27806, #64856, #72841, #40026, #1726, #33707, #14369, #53466, #7194, #79590, #79175, #59368, #26966, #21905, #58534, #900, #26557, #53044, #7627, #21491, #52210, #20245, #15190, #13515, #58960, #78756, #40437, #21081, #39172, #34123, #45894, #1317, #14781, #52631, #66117, #8452, #2138, #40847, #66533, #66954, #81234, #49218, #23550, #62267, #36589, #74924, #17269, #10116, #74092, #42897, #23965, #4604, #68193, #23139, #30276, #48808, #55939, #81654, #80422, #48392, #67778, #3794, #10531, #73260, #29863, #68591, #29458, #74507, #15609, #41268, #9286, #47986, #16438, #34957, #54294, #73685, #16025, #41672, #22322, #80009, #67364, #4199, #55116, #16854, #61858, #9697, #35367, #55525, #35778, #36186, #42489, #61032, #10932, #60620, #2970, #80825, #61447, #3382, #28636, #54715, #42083, #29044, #22733, #31098, #44538, #5029, #75739, #19301, #50861, #51269, #43302, #82464, #24780, #76971, #70649, #82060, #50044, #57593, #50448, #31515, #70229, #44953, #13004, #30697, #12584, #38660, #38242, #64337, #63919, #6674, #58007, #32346, #372, #56361, #44133, #5840, #69000, #11351, #37009, #83283, #18080, #18889 ),
 ( #56765, #6254, #76150, #24373, #49632, #75325, #76561, #17671, #62687, #43715, #25195, #69417, #31931, #11772, #25606, #37425, #63098, #5437, #18490, #69825, #12174, #37832, #63510, #57173, #82871, #20977, #64756, #52107, #79076, #27282, #27702, #19721, #58861, #1218, #53366, #47048, #58432, #26455, #34021, #26867, #7944, #46637, #21392, #72740, #7095, #72332, #15087, #14680, #40745, #40337, #66429, #34439, #8764, #60106, #32765, #20568, #65613, #45379, #71076, #13418, #59681, #77815, #78656, #52942, #52528, #46219, #794, #33605, #2037, #26027, #39075, #20146, #45795, #71493, #66017, #8353, #59268, #7523, #51687, #33193, #13841, #77390, #39499, #65187, #78235, #71915, #14265, #1625, #39924, #16337, #9184, #29358, #60518, #66852, #67674, #29766, #73579, #2867, #61760, #2459, #36089, #35675, #73990, #10432, #41980, #4098, #28117, #41572, #9595, #3278, #22632, #61340, #53772, #23040, #68087, #48293, #10010, #79484, #21798, #15504, #54187, #28942, #47462, #28530, #79902, #47875, #15925, #22219, #67262, #35263, #74405, #3693, #55017, #48707, #60928, #54608, #42388, #80726, #16749, #73154, #80317, #41162, #34856, #27975, #33877, #40194, #20421, #53633, #59128, #46489, #8627, #59543, #78928, #66288, #1074, #78090, #59959, #65877, #40605, #21250, #46074, #53217, #34298, #79341, #1898, #8212, #71766, #21661, #1485, #72184, #78513, #46905, #27139, #72600, #33040, #14120, #47321, #14946, #73012, #71348, #52803, #20836, #15363, #41024, #26727, #39772, #2314, #14542, #27559, #66710, #9043, #34717, #58709, #60378, #2726, #28387, #77672, #20002, #45653, #13695, #39350, #65035, #52381, #7371, #65467, #7801, #33466, #73964, #22607, #55814, #81109, #68062, #69292, #48267, #16310, #41954, #42774, #23014, #62561, #67648, #61314, #4900, #37300, #74378, #36063, #81522, #4072, #43591, #75202, #3669, #9983, #17142, #16721, #80701, #54993, #10406, #35651, #29332, #48682, #30571, #56237, #81934, #11642, #17954, #24245, #49918, #74794, #55402, #75616, #62974, #23842, #68470, #54583, #49509, #10808, #42362, #61735, #29739, #5313, #30152, #80293, #23426, #49091, #36468, #62143, #4482, #17546, #43178, #68875, #11224, #36883, #63787, #6545, #51141, #30971, #5712, #69702, #76835, #77256, #57874, #82741, #32215, #19586, #64623, #70514, #19169, #57047, #6960, #12452, #83154, #31801, #241, #38113, #25893, #12045, #25062, #659, #51553, #32631, #24657, #6126, #57461, #58294, #51976, #63376, #31382, #38942, #25474, #12871, #45248, #26315, #77681, #37703, #70945, #20011, #13290, #45662, #71358, #13705, #39360, #65045, #56638, #50735, #44817, #38530, #50325, #76023, #18367, #64211, #82339, #44008, #76434, #18763, #44406, #70100, #46915, #41033, #41446, #52390, #26736, #1084, #78099, #8636, #79352, #72609, #72199, #47332, #14552, #65478, #47747, #7382, #34307, #9055, #54056, #14130, #66297, #39783, #59968, #7810, #73022, #33476, #59138, #2328, #33050, #40203, #1496, #73446, #58721, #79771, #27984, #40614, #22087, #53644, #15796, #20430, #65887, #8222, #1907, #21261, #21671, #46083, #15372, #60387, #14957, #66719, #71776, #27148, #52812, #78522, #33886, #20846, #46499, #59552, #27568, #53227, #78943, #34728, #2738, #28398, #48994, #68376, #55713, #73863, #67543, #49411, #4383, #42262, #3977, #48168, #23324, #17451, #17857, #28814, #3150, #60796, #54478, #10715, #81423, #74693, #48579, #23738, #74276, #41851, #24148, #67130, #36372, #68778, #30468, #16204, #42678, #9878, #62046, #35547, #75104, #61210, #3565, #30051, #9460, #16620, #29232, #49818, #35134, #56132, #43081, #17038, #81837, #11122, #75518, #80190, #67958, #10300, #61636, #81010, #36779, #22507, #62455, #4791, #54896, #80602, #22911, #35966, #29641, #55302, #18668, #32532, #24562, #18264, #69603, #11949, #75924, #50228, #43905, #57777, #25379, #44721, #32119, #37604, #63278, #25796, #6031, #6449, #70419, #5619, #19073, #140, #77159, #83057, #31703, #31285, #19491, #24962, #12358, #44313, #12774, #50633, #38431, #82243, #56950, #13199, #64114, #45145, #37195, #76338, #70003, #70848, #64526, #82647, #38016, #51456, #63692, #51042 ) ),
 .UNSPECIFIED., .F., .F., .F. ) 
 B_SPLINE_SURFACE_WITH_KNOTS ( ( 2, 2 ),
 ( 3, 2, 2, 2, 2, 2, 2, 2, 2, 2, 2, 2, 2, 2, 2, 2, 2, 2, 2, 2, 2, 2, 2, 2, 2, 2, 2, 2, 2, 2, 2, 2, 2, 2, 2, 2, 2, 2, 2, 2, 2, 2, 2, 2, 2, 2, 2, 2, 2, 2, 2, 2, 2, 2, 2, 2, 2, 2, 2, 2, 2, 2, 2, 2, 2, 2, 2, 2, 2, 2, 2, 2, 2, 2, 2, 2, 2, 2, 2, 2, 2, 2, 2, 2, 2, 2, 2, 2, 2, 2, 2, 2, 2, 2, 2, 2, 2, 2, 2, 2, 2, 2, 2, 2, 2, 2, 2, 2, 2, 2, 2, 2, 2, 2, 2, 2, 2, 2, 2, 2, 2, 2, 2, 2, 2, 2, 2, 2, 2, 2, 2, 2, 2, 2, 2, 2, 2, 2, 2, 2, 2, 2, 2, 2, 2, 2, 2, 2, 2, 2, 2, 2, 2, 2, 2, 2, 2, 2, 2, 2, 2, 2, 2, 2, 2, 2, 2, 2, 2, 2, 2, 2, 2, 2, 2, 2, 2, 2, 2, 2, 2, 2, 2, 2, 2, 2, 2, 2, 2, 2, 2, 2, 2, 2, 2, 2, 2, 2, 2, 2, 2, 2, 2, 2, 2, 2, 2, 2, 2, 2, 2, 2, 2, 2, 2, 2, 2, 2, 2, 2, 2, 2, 2, 2, 2, 2, 2, 2, 2, 2, 2, 2, 2, 2, 2, 2, 2, 2, 2, 2, 2, 2, 2, 2, 2, 2, 2, 2, 2, 2, 2, 2, 2, 2, 2, 3 ),
 ( 0.000000000000000000, 1.000000000000000000 ),
 ( 0.000000000000000000, 0.003787878787878787984, 0.007575757575757575968, 0.01136363636363636395, 0.01515151515151515194, 0.01893939393939393992, 0.02272727272727272790, 0.02651515151515151589, 0.03030303030303030387, 0.03409090909090908839, 0.03787878787878787984, 0.04166666666666666435, 0.04545454545454545581, 0.04924242424242424032, 0.05303030303030303177, 0.05681818181818181629, 0.06060606060606060774, 0.06439393939393939226, 0.06818181818181817677, 0.07196969696969697516, 0.07575757575757575968, 0.07954545454545454419, 0.08333333333333332871, 0.08712121212121212710, 0.09090909090909091161, 0.09469696969696969613, 0.09848484848484848064, 0.1022727272727272790, 0.1060606060606060635, 0.1098484848484848481, 0.1136363636363636326, 0.1174242424242424310, 0.1212121212121212155, 0.1250000000000000000, 0.1287878787878787845, 0.1325757575757575690, 0.1363636363636363535, 0.1401515151515151381, 0.1439393939393939503, 0.1477272727272727348, 0.1515151515151515194, 0.1553030303030303039, 0.1590909090909090884, 0.1628787878787878729, 0.1666666666666666574, 0.1704545454545454419, 0.1742424242424242542, 0.1780303030303030387, 0.1818181818181818232, 0.1856060606060606077, 0.1893939393939393923, 0.1931818181818181768, 0.1969696969696969613, 0.2007575757575757458, 0.2045454545454545581, 0.2083333333333333426, 0.2121212121212121271, 0.2159090909090909116, 0.2196969696969696961, 0.2234848484848484806, 0.2272727272727272652, 0.2310606060606060497, 0.2348484848484848619, 0.2386363636363636465, 0.2424242424242424310, 0.2462121212121212155, 0.2500000000000000000, 0.2537878787878787845, 0.2575757575757575690, 0.2613636363636363535, 0.2651515151515151381, 0.2689393939393939226, 0.2727272727272727071, 0.2765151515151514916, 0.2803030303030302761, 0.2840909090909091161, 0.2878787878787879007, 0.2916666666666666852, 0.2954545454545454697, 0.2992424242424242542, 0.3030303030303030387, 0.3068181818181818232, 0.3106060606060606077, 0.3143939393939393923, 0.3181818181818181768, 0.3219696969696969613, 0.3257575757575757458, 0.3295454545454545303, 0.3333333333333333148, 0.3371212121212120993, 0.3409090909090908839, 0.3446969696969697239, 0.3484848484848485084, 0.3522727272727272929, 0.3560606060606060774, 0.3598484848484848619, 0.3636363636363636465, 0.3674242424242424310, 0.3712121212121212155, 0.3750000000000000000, 0.3787878787878787845, 0.3825757575757575690, 0.3863636363636363535, 0.3901515151515151381, 0.3939393939393939226, 0.3977272727272727071, 0.4015151515151514916, 0.4053030303030302761, 0.4090909090909091161, 0.4128787878787879007, 0.4166666666666666852, 0.4204545454545454697, 0.4242424242424242542, 0.4280303030303030387, 0.4318181818181818232, 0.4356060606060606077, 0.4393939393939393923, 0.4431818181818181768, 0.4469696969696969613, 0.4507575757575757458, 0.4545454545454545303, 0.4583333333333333148, 0.4621212121212120993, 0.4659090909090908839, 0.4696969696969697239, 0.4734848484848485084, 0.4772727272727272929, 0.4810606060606060774, 0.4848484848484848619, 0.4886363636363636465, 0.4924242424242424310, 0.4962121212121212155, 0.5000000000000000000, 0.5037878787878787845, 0.5075757575757575690, 0.5113636363636363535, 0.5151515151515151381, 0.5189393939393939226, 0.5227272727272727071, 0.5265151515151514916, 0.5303030303030302761, 0.5340909090909090606, 0.5378787878787878451, 0.5416666666666666297, 0.5454545454545454142, 0.5492424242424241987, 0.5530303030303029832, 0.5568181818181817677, 0.5606060606060605522, 0.5643939393939394478, 0.5681818181818182323, 0.5719696969696970168, 0.5757575757575758013, 0.5795454545454545858, 0.5833333333333333703, 0.5871212121212121549, 0.5909090909090909394, 0.5946969696969697239, 0.5984848484848485084, 0.6022727272727272929, 0.6060606060606060774, 0.6098484848484848619, 0.6136363636363636465, 0.6174242424242424310, 0.6212121212121212155, 0.6250000000000000000, 0.6287878787878787845, 0.6325757575757575690, 0.6363636363636363535, 0.6401515151515151381, 0.6439393939393939226, 0.6477272727272727071, 0.6515151515151514916, 0.6553030303030302761, 0.6590909090909090606, 0.6628787878787878451, 0.6666666666666666297, 0.6704545454545454142, 0.6742424242424241987, 0.6780303030303029832, 0.6818181818181817677, 0.6856060606060605522, 0.6893939393939394478, 0.6931818181818182323, 0.6969696969696970168, 0.7007575757575758013, 0.7045454545454545858, 0.7083333333333333703, 0.7121212121212121549, 0.7159090909090909394, 0.7196969696969697239, 0.7234848484848485084, 0.7272727272727272929, 0.7310606060606060774, 0.7348484848484848619, 0.7386363636363636465, 0.7424242424242424310, 0.7462121212121212155, 0.7500000000000000000, 0.7537878787878787845, 0.7575757575757575690, 0.7613636363636363535, 0.7651515151515151381, 0.7689393939393939226, 0.7727272727272727071, 0.7765151515151514916, 0.7803030303030302761, 0.7840909090909090606, 0.7878787878787878451, 0.7916666666666666297, 0.7954545454545454142, 0.7992424242424241987, 0.8030303030303029832, 0.8068181818181817677, 0.8106060606060605522, 0.8143939393939394478, 0.8181818181818182323, 0.8219696969696970168, 0.8257575757575758013, 0.8295454545454545858, 0.8333333333333333703, 0.8371212121212121549, 0.8409090909090909394, 0.8446969696969697239, 0.8484848484848485084, 0.8522727272727272929, 0.8560606060606060774, 0.8598484848484848619, 0.8636363636363636465, 0.8674242424242424310, 0.8712121212121212155, 0.8750000000000000000, 0.8787878787878787845, 0.8825757575757575690, 0.8863636363636363535, 0.8901515151515151381, 0.8939393939393939226, 0.8977272727272727071, 0.9015151515151514916, 0.9053030303030302761, 0.9090909090909090606, 0.9128787878787878451, 0.9166666666666666297, 0.9204545454545454142, 0.9242424242424241987, 0.9280303030303029832, 0.9318181818181817677, 0.9356060606060605522, 0.9393939393939394478, 0.9431818181818182323, 0.9469696969696970168, 0.9507575757575758013, 0.9545454545454545858, 0.9583333333333333703, 0.9621212121212121549, 0.9659090909090909394 ),
 .UNSPECIFIED. ) 
 GEOMETRIC_REPRESENTATION_ITEM ( )  RATIONAL_B_SPLINE_SURFACE ( (
 ( 1.000000000000000000, 0.9659258262890683122, 1.000000000000000000, 0.9659258262890683122, 1.000000000000000000, 0.9659258262890683122, 1.000000000000000000, 0.9659258262890683122, 1.000000000000000000, 0.9659258262890683122, 1.000000000000000000, 0.9659258262890683122, 1.000000000000000000, 0.9659258262890683122, 1.000000000000000000, 0.9659258262890683122, 1.000000000000000000, 0.9659258262890683122, 1.000000000000000000, 0.9659258262890683122, 1.000000000000000000, 0.9659258262890683122, 1.000000000000000000, 0.9659258262890683122, 1.000000000000000000, 0.9659258262890683122, 1.000000000000000000, 0.9659258262890683122, 1.000000000000000000, 0.9659258262890683122, 1.000000000000000000, 0.9659258262890683122, 1.000000000000000000, 0.9659258262890683122, 1.000000000000000000, 0.9659258262890683122, 1.000000000000000000, 0.9659258262890683122, 1.000000000000000000, 0.9659258262890683122, 1.000000000000000000, 0.9659258262890683122, 1.000000000000000000, 0.9659258262890683122, 1.000000000000000000, 0.9659258262890683122, 1.000000000000000000, 0.9659258262890683122, 1.000000000000000000, 0.9659258262890683122, 1.000000000000000000, 0.9659258262890683122, 1.000000000000000000, 0.9659258262890683122, 1.000000000000000000, 0.9659258262890683122, 1.000000000000000000, 0.9659258262890683122, 1.000000000000000000, 0.9659258262890683122, 1.000000000000000000, 0.9659258262890683122, 1.000000000000000000, 0.9659258262890683122, 1.000000000000000000, 0.9659258262890683122, 1.000000000000000000, 0.9659258262890683122, 1.000000000000000000, 0.9659258262890683122, 1.000000000000000000, 0.9659258262890683122, 1.000000000000000000, 0.9659258262890683122, 1.000000000000000000, 0.9659258262890683122, 1.000000000000000000, 0.9659258262890683122, 1.000000000000000000, 0.9659258262890683122, 1.000000000000000000, 0.9659258262890683122, 1.000000000000000000, 0.9659258262890683122, 1.000000000000000000, 0.9659258262890683122, 1.000000000000000000, 0.9659258262890683122, 1.000000000000000000, 0.9659258262890683122, 1.000000000000000000, 0.9659258262890683122, 1.000000000000000000, 0.9659258262890683122, 1.000000000000000000, 0.9659258262890683122, 1.000000000000000000, 0.9659258262890683122, 1.000000000000000000, 0.9659258262890683122, 1.000000000000000000, 0.9659258262890683122, 1.000000000000000000, 0.9659258262890683122, 1.000000000000000000, 0.9659258262890683122, 1.000000000000000000, 0.9659258262890683122, 1.000000000000000000, 0.9659258262890683122, 1.000000000000000000, 0.9659258262890683122, 1.000000000000000000, 0.9659258262890683122, 1.000000000000000000, 0.9659258262890683122, 1.000000000000000000, 0.9659258262890683122, 1.000000000000000000, 0.9659258262890683122, 1.000000000000000000, 0.9659258262890683122, 1.000000000000000000, 0.9659258262890683122, 1.000000000000000000, 0.9659258262890683122, 1.000000000000000000, 0.9659258262890683122, 1.000000000000000000, 0.9659258262890683122, 1.000000000000000000, 0.9659258262890683122, 1.000000000000000000, 0.9659258262890683122, 1.000000000000000000, 0.9659258262890683122, 1.000000000000000000, 0.9659258262890683122, 1.000000000000000000, 0.9659258262890683122, 1.000000000000000000, 0.9659258262890683122, 1.000000000000000000, 0.9659258262890683122, 1.000000000000000000, 0.9659258262890683122, 1.000000000000000000, 0.9659258262890683122, 1.000000000000000000, 0.9659258262890683122, 1.000000000000000000, 0.9659258262890683122, 1.000000000000000000, 0.9659258262890683122, 1.000000000000000000, 0.9659258262890683122, 1.000000000000000000, 0.9659258262890683122, 1.000000000000000000, 0.9659258262890683122, 1.000000000000000000, 0.9659258262890683122, 1.000000000000000000, 0.9659258262890683122, 1.000000000000000000, 0.9659258262890683122, 1.000000000000000000, 0.9659258262890683122, 1.000000000000000000, 0.9659258262890683122, 1.000000000000000000, 0.9659258262890683122, 1.000000000000000000, 0.9659258262890683122, 1.000000000000000000, 0.9659258262890683122, 1.000000000000000000, 0.9659258262890683122, 1.000000000000000000, 0.9659258262890683122, 1.000000000000000000, 0.9659258262890683122, 1.000000000000000000, 0.9659258262890683122, 1.000000000000000000, 0.9659258262890683122, 1.000000000000000000, 0.9659258262890683122, 1.000000000000000000, 0.9659258262890683122, 1.000000000000000000, 0.9659258262890683122, 1.000000000000000000, 0.9659258262890683122, 1.000000000000000000, 0.9659258262890683122, 1.000000000000000000, 0.9659258262890683122, 1.000000000000000000, 0.9659258262890683122, 1.000000000000000000, 0.9659258262890683122, 1.000000000000000000, 0.9659258262890683122, 1.000000000000000000, 0.9659258262890683122, 1.000000000000000000, 0.9659258262890683122, 1.000000000000000000, 0.9659258262890683122, 1.000000000000000000, 0.9659258262890683122, 1.000000000000000000, 0.9659258262890683122, 1.000000000000000000, 0.9659258262890683122, 1.000000000000000000, 0.9659258262890683122, 1.000000000000000000, 0.9659258262890683122, 1.000000000000000000, 0.9659258262890683122, 1.000000000000000000, 0.9659258262890683122, 1.000000000000000000, 0.9659258262890683122, 1.000000000000000000, 0.9659258262890683122, 1.000000000000000000, 0.9659258262890683122, 1.000000000000000000, 0.9659258262890683122, 1.000000000000000000, 0.9659258262890683122, 1.000000000000000000, 0.9659258262890683122, 1.000000000000000000, 0.9659258262890683122, 1.000000000000000000, 0.9659258262890683122, 1.000000000000000000, 0.9659258262890683122, 1.000000000000000000, 0.9659258262890683122, 1.000000000000000000, 0.9659258262890683122, 1.000000000000000000, 0.9659258262890683122, 1.000000000000000000, 0.9659258262890683122, 1.000000000000000000, 0.9659258262890683122, 1.000000000000000000, 0.9659258262890683122, 1.000000000000000000, 0.9659258262890683122, 1.000000000000000000, 0.9659258262890683122, 1.000000000000000000, 0.9659258262890683122, 1.000000000000000000, 0.9659258262890683122, 1.000000000000000000, 0.9659258262890683122, 1.000000000000000000, 0.9659258262890683122, 1.000000000000000000, 0.9659258262890683122, 1.000000000000000000, 0.9659258262890683122, 1.000000000000000000, 0.9659258262890683122, 1.000000000000000000, 0.9659258262890683122, 1.000000000000000000, 0.9659258262890683122, 1.000000000000000000, 0.9659258262890683122, 1.000000000000000000, 0.9659258262890683122, 1.000000000000000000, 0.9659258262890683122, 1.000000000000000000, 0.9659258262890683122, 1.000000000000000000, 0.9659258262890683122, 1.000000000000000000, 0.9659258262890683122, 1.000000000000000000, 0.9659258262890683122, 1.000000000000000000, 0.9659258262890683122, 1.000000000000000000, 0.9659258262890683122, 1.000000000000000000, 0.9659258262890683122, 1.000000000000000000, 0.9659258262890683122, 1.000000000000000000, 0.9659258262890683122, 1.000000000000000000, 0.9659258262890683122, 1.000000000000000000, 0.9659258262890683122, 1.000000000000000000, 0.9659258262890683122, 1.000000000000000000, 0.9659258262890683122, 1.000000000000000000, 0.9659258262890683122, 1.000000000000000000, 0.9659258262890683122, 1.000000000000000000, 0.9659258262890683122, 1.000000000000000000, 0.9659258262890683122, 1.000000000000000000, 0.9659258262890683122, 1.000000000000000000, 0.9659258262890683122, 1.000000000000000000, 0.9659258262890683122, 1.000000000000000000, 0.9659258262890683122, 1.000000000000000000, 0.9659258262890683122, 1.000000000000000000, 0.9659258262890683122, 1.000000000000000000, 0.9659258262890683122, 1.000000000000000000, 0.9659258262890683122, 1.000000000000000000, 0.9659258262890683122, 1.000000000000000000, 0.9659258262890683122, 1.000000000000000000, 0.9659258262890683122, 1.000000000000000000, 0.9659258262890683122, 1.000000000000000000, 0.9659258262890683122, 1.000000000000000000, 0.9659258262890683122, 1.000000000000000000, 0.9659258262890683122, 1.000000000000000000, 0.9659258262890683122, 1.000000000000000000, 0.9659258262890683122, 1.000000000000000000, 0.9659258262890683122, 1.000000000000000000, 0.9659258262890683122, 1.000000000000000000, 0.9659258262890683122, 1.000000000000000000, 0.9659258262890683122, 1.000000000000000000, 0.9659258262890683122, 1.000000000000000000, 0.9659258262890683122, 1.000000000000000000, 0.9659258262890683122, 1.000000000000000000, 0.9659258262890683122, 1.000000000000000000, 0.9659258262890683122, 1.000000000000000000, 0.9659258262890683122, 1.000000000000000000, 0.9659258262890683122, 1.000000000000000000, 0.9659258262890683122, 1.000000000000000000, 0.9659258262890683122, 1.000000000000000000, 0.9659258262890683122, 1.000000000000000000, 0.9659258262890683122, 1.000000000000000000, 0.9659258262890683122, 1.000000000000000000, 0.9659258262890683122, 1.000000000000000000, 0.9659258262890683122, 1.000000000000000000, 0.9659258262890683122, 1.000000000000000000, 0.9659258262890683122, 1.000000000000000000, 0.9659258262890683122, 1.000000000000000000, 0.9659258262890683122, 1.000000000000000000, 0.9659258262890683122, 1.000000000000000000, 0.9659258262890683122, 1.000000000000000000, 0.9659258262890683122, 1.000000000000000000, 0.9659258262890683122, 1.000000000000000000, 0.9659258262890683122, 1.000000000000000000, 0.9659258262890683122, 1.000000000000000000, 0.9659258262890683122, 1.000000000000000000, 0.9659258262890683122, 1.000000000000000000, 0.9659258262890683122, 1.000000000000000000, 0.9659258262890683122, 1.000000000000000000, 0.9659258262890683122, 1.000000000000000000, 0.9659258262890683122, 1.000000000000000000, 0.9659258262890683122, 1.000000000000000000, 0.9659258262890683122, 1.000000000000000000, 0.9659258262890683122, 1.000000000000000000, 0.9659258262890683122, 1.000000000000000000, 0.9659258262890683122, 1.000000000000000000, 0.9659258262890683122, 1.000000000000000000, 0.9659258262890683122, 1.000000000000000000, 0.9659258262890683122, 1.000000000000000000, 0.9659258262890683122, 1.000000000000000000, 0.9659258262890683122, 1.000000000000000000, 0.9659258262890683122, 1.000000000000000000, 0.9659258262890683122, 1.000000000000000000, 0.9659258262890683122, 1.000000000000000000, 0.9659258262890683122, 1.000000000000000000, 0.9659258262890683122, 1.000000000000000000, 0.9659258262890683122, 1.000000000000000000, 0.9659258262890683122, 1.000000000000000000, 0.9659258262890683122, 1.000000000000000000, 0.9659258262890683122, 1.000000000000000000, 0.9659258262890683122, 1.000000000000000000, 0.9659258262890683122, 1.000000000000000000, 0.9659258262890683122, 1.000000000000000000, 0.9659258262890683122, 1.000000000000000000, 0.9659258262890683122, 1.000000000000000000, 0.9659258262890683122, 1.000000000000000000, 0.9659258262890683122, 1.000000000000000000, 0.9659258262890683122, 1.000000000000000000, 0.9659258262890683122, 1.000000000000000000, 0.9659258262890683122, 1.000000000000000000, 0.9659258262890683122, 1.000000000000000000, 0.9659258262890683122, 1.000000000000000000, 0.9659258262890683122, 1.000000000000000000, 0.9659258262890683122, 1.000000000000000000, 0.9659258262890683122, 1.000000000000000000, 0.9659258262890683122, 1.000000000000000000, 0.9659258262890683122, 1.000000000000000000, 0.9659258262890683122, 1.000000000000000000, 0.9659258262890683122, 1.000000000000000000, 0.9659258262890683122, 1.000000000000000000, 0.9659258262890683122, 1.000000000000000000, 0.9659258262890683122, 1.000000000000000000, 0.9659258262890683122, 1.000000000000000000, 0.9659258262890683122, 1.000000000000000000, 0.9659258262890683122, 1.000000000000000000, 0.9659258262890683122, 1.000000000000000000, 0.9659258262890683122, 1.000000000000000000),
 ( 1.000000000000000000, 0.9659258262890683122, 1.000000000000000000, 0.9659258262890683122, 1.000000000000000000, 0.9659258262890683122, 1.000000000000000000, 0.9659258262890683122, 1.000000000000000000, 0.9659258262890683122, 1.000000000000000000, 0.9659258262890683122, 1.000000000000000000, 0.9659258262890683122, 1.000000000000000000, 0.9659258262890683122, 1.000000000000000000, 0.9659258262890683122, 1.000000000000000000, 0.9659258262890683122, 1.000000000000000000, 0.9659258262890683122, 1.000000000000000000, 0.9659258262890683122, 1.000000000000000000, 0.9659258262890683122, 1.000000000000000000, 0.9659258262890683122, 1.000000000000000000, 0.9659258262890683122, 1.000000000000000000, 0.9659258262890683122, 1.000000000000000000, 0.9659258262890683122, 1.000000000000000000, 0.9659258262890683122, 1.000000000000000000, 0.9659258262890683122, 1.000000000000000000, 0.9659258262890683122, 1.000000000000000000, 0.9659258262890683122, 1.000000000000000000, 0.9659258262890683122, 1.000000000000000000, 0.9659258262890683122, 1.000000000000000000, 0.9659258262890683122, 1.000000000000000000, 0.9659258262890683122, 1.000000000000000000, 0.9659258262890683122, 1.000000000000000000, 0.9659258262890683122, 1.000000000000000000, 0.9659258262890683122, 1.000000000000000000, 0.9659258262890683122, 1.000000000000000000, 0.9659258262890683122, 1.000000000000000000, 0.9659258262890683122, 1.000000000000000000, 0.9659258262890683122, 1.000000000000000000, 0.9659258262890683122, 1.000000000000000000, 0.9659258262890683122, 1.000000000000000000, 0.9659258262890683122, 1.000000000000000000, 0.9659258262890683122, 1.000000000000000000, 0.9659258262890683122, 1.000000000000000000, 0.9659258262890683122, 1.000000000000000000, 0.9659258262890683122, 1.000000000000000000, 0.9659258262890683122, 1.000000000000000000, 0.9659258262890683122, 1.000000000000000000, 0.9659258262890683122, 1.000000000000000000, 0.9659258262890683122, 1.000000000000000000, 0.9659258262890683122, 1.000000000000000000, 0.9659258262890683122, 1.000000000000000000, 0.9659258262890683122, 1.000000000000000000, 0.9659258262890683122, 1.000000000000000000, 0.9659258262890683122, 1.000000000000000000, 0.9659258262890683122, 1.000000000000000000, 0.9659258262890683122, 1.000000000000000000, 0.9659258262890683122, 1.000000000000000000, 0.9659258262890683122, 1.000000000000000000, 0.9659258262890683122, 1.000000000000000000, 0.9659258262890683122, 1.000000000000000000, 0.9659258262890683122, 1.000000000000000000, 0.9659258262890683122, 1.000000000000000000, 0.9659258262890683122, 1.000000000000000000, 0.9659258262890683122, 1.000000000000000000, 0.9659258262890683122, 1.000000000000000000, 0.9659258262890683122, 1.000000000000000000, 0.9659258262890683122, 1.000000000000000000, 0.9659258262890683122, 1.000000000000000000, 0.9659258262890683122, 1.000000000000000000, 0.9659258262890683122, 1.000000000000000000, 0.9659258262890683122, 1.000000000000000000, 0.9659258262890683122, 1.000000000000000000, 0.9659258262890683122, 1.000000000000000000, 0.9659258262890683122, 1.000000000000000000, 0.9659258262890683122, 1.000000000000000000, 0.9659258262890683122, 1.000000000000000000, 0.9659258262890683122, 1.000000000000000000, 0.9659258262890683122, 1.000000000000000000, 0.9659258262890683122, 1.000000000000000000, 0.9659258262890683122, 1.000000000000000000, 0.9659258262890683122, 1.000000000000000000, 0.9659258262890683122, 1.000000000000000000, 0.9659258262890683122, 1.000000000000000000, 0.9659258262890683122, 1.000000000000000000, 0.9659258262890683122, 1.000000000000000000, 0.9659258262890683122, 1.000000000000000000, 0.9659258262890683122, 1.000000000000000000, 0.9659258262890683122, 1.000000000000000000, 0.9659258262890683122, 1.000000000000000000, 0.9659258262890683122, 1.000000000000000000, 0.9659258262890683122, 1.000000000000000000, 0.9659258262890683122, 1.000000000000000000, 0.9659258262890683122, 1.000000000000000000, 0.9659258262890683122, 1.000000000000000000, 0.9659258262890683122, 1.000000000000000000, 0.9659258262890683122, 1.000000000000000000, 0.9659258262890683122, 1.000000000000000000, 0.9659258262890683122, 1.000000000000000000, 0.9659258262890683122, 1.000000000000000000, 0.9659258262890683122, 1.000000000000000000, 0.9659258262890683122, 1.000000000000000000, 0.9659258262890683122, 1.000000000000000000, 0.9659258262890683122, 1.000000000000000000, 0.9659258262890683122, 1.000000000000000000, 0.9659258262890683122, 1.000000000000000000, 0.9659258262890683122, 1.000000000000000000, 0.9659258262890683122, 1.000000000000000000, 0.9659258262890683122, 1.000000000000000000, 0.9659258262890683122, 1.000000000000000000, 0.9659258262890683122, 1.000000000000000000, 0.9659258262890683122, 1.000000000000000000, 0.9659258262890683122, 1.000000000000000000, 0.9659258262890683122, 1.000000000000000000, 0.9659258262890683122, 1.000000000000000000, 0.9659258262890683122, 1.000000000000000000, 0.9659258262890683122, 1.000000000000000000, 0.9659258262890683122, 1.000000000000000000, 0.9659258262890683122, 1.000000000000000000, 0.9659258262890683122, 1.000000000000000000, 0.9659258262890683122, 1.000000000000000000, 0.9659258262890683122, 1.000000000000000000, 0.9659258262890683122, 1.000000000000000000, 0.9659258262890683122, 1.000000000000000000, 0.9659258262890683122, 1.000000000000000000, 0.9659258262890683122, 1.000000000000000000, 0.9659258262890683122, 1.000000000000000000, 0.9659258262890683122, 1.000000000000000000, 0.9659258262890683122, 1.000000000000000000, 0.9659258262890683122, 1.000000000000000000, 0.9659258262890683122, 1.000000000000000000, 0.9659258262890683122, 1.000000000000000000, 0.9659258262890683122, 1.000000000000000000, 0.9659258262890683122, 1.000000000000000000, 0.9659258262890683122, 1.000000000000000000, 0.9659258262890683122, 1.000000000000000000, 0.9659258262890683122, 1.000000000000000000, 0.9659258262890683122, 1.000000000000000000, 0.9659258262890683122, 1.000000000000000000, 0.9659258262890683122, 1.000000000000000000, 0.9659258262890683122, 1.000000000000000000, 0.9659258262890683122, 1.000000000000000000, 0.9659258262890683122, 1.000000000000000000, 0.9659258262890683122, 1.000000000000000000, 0.9659258262890683122, 1.000000000000000000, 0.9659258262890683122, 1.000000000000000000, 0.9659258262890683122, 1.000000000000000000, 0.9659258262890683122, 1.000000000000000000, 0.9659258262890683122, 1.000000000000000000, 0.9659258262890683122, 1.000000000000000000, 0.9659258262890683122, 1.000000000000000000, 0.9659258262890683122, 1.000000000000000000, 0.9659258262890683122, 1.000000000000000000, 0.9659258262890683122, 1.000000000000000000, 0.9659258262890683122, 1.000000000000000000, 0.9659258262890683122, 1.000000000000000000, 0.9659258262890683122, 1.000000000000000000, 0.9659258262890683122, 1.000000000000000000, 0.9659258262890683122, 1.000000000000000000, 0.9659258262890683122, 1.000000000000000000, 0.9659258262890683122, 1.000000000000000000, 0.9659258262890683122, 1.000000000000000000, 0.9659258262890683122, 1.000000000000000000, 0.9659258262890683122, 1.000000000000000000, 0.9659258262890683122, 1.000000000000000000, 0.9659258262890683122, 1.000000000000000000, 0.9659258262890683122, 1.000000000000000000, 0.9659258262890683122, 1.000000000000000000, 0.9659258262890683122, 1.000000000000000000, 0.9659258262890683122, 1.000000000000000000, 0.9659258262890683122, 1.000000000000000000, 0.9659258262890683122, 1.000000000000000000, 0.9659258262890683122, 1.000000000000000000, 0.9659258262890683122, 1.000000000000000000, 0.9659258262890683122, 1.000000000000000000, 0.9659258262890683122, 1.000000000000000000, 0.9659258262890683122, 1.000000000000000000, 0.9659258262890683122, 1.000000000000000000, 0.9659258262890683122, 1.000000000000000000, 0.9659258262890683122, 1.000000000000000000, 0.9659258262890683122, 1.000000000000000000, 0.9659258262890683122, 1.000000000000000000, 0.9659258262890683122, 1.000000000000000000, 0.9659258262890683122, 1.000000000000000000, 0.9659258262890683122, 1.000000000000000000, 0.9659258262890683122, 1.000000000000000000, 0.9659258262890683122, 1.000000000000000000, 0.9659258262890683122, 1.000000000000000000, 0.9659258262890683122, 1.000000000000000000, 0.9659258262890683122, 1.000000000000000000, 0.9659258262890683122, 1.000000000000000000, 0.9659258262890683122, 1.000000000000000000, 0.9659258262890683122, 1.000000000000000000, 0.9659258262890683122, 1.000000000000000000, 0.9659258262890683122, 1.000000000000000000, 0.9659258262890683122, 1.000000000000000000, 0.9659258262890683122, 1.000000000000000000, 0.9659258262890683122, 1.000000000000000000, 0.9659258262890683122, 1.000000000000000000, 0.9659258262890683122, 1.000000000000000000, 0.9659258262890683122, 1.000000000000000000, 0.9659258262890683122, 1.000000000000000000, 0.9659258262890683122, 1.000000000000000000, 0.9659258262890683122, 1.000000000000000000, 0.9659258262890683122, 1.000000000000000000, 0.9659258262890683122, 1.000000000000000000, 0.9659258262890683122, 1.000000000000000000, 0.9659258262890683122, 1.000000000000000000, 0.9659258262890683122, 1.000000000000000000, 0.9659258262890683122, 1.000000000000000000, 0.9659258262890683122, 1.000000000000000000, 0.9659258262890683122, 1.000000000000000000, 0.9659258262890683122, 1.000000000000000000, 0.9659258262890683122, 1.000000000000000000, 0.9659258262890683122, 1.000000000000000000, 0.9659258262890683122, 1.000000000000000000, 0.9659258262890683122, 1.000000000000000000, 0.9659258262890683122, 1.000000000000000000, 0.9659258262890683122, 1.000000000000000000, 0.9659258262890683122, 1.000000000000000000, 0.9659258262890683122, 1.000000000000000000, 0.9659258262890683122, 1.000000000000000000, 0.9659258262890683122, 1.000000000000000000, 0.9659258262890683122, 1.000000000000000000, 0.9659258262890683122, 1.000000000000000000, 0.9659258262890683122, 1.000000000000000000, 0.9659258262890683122, 1.000000000000000000, 0.9659258262890683122, 1.000000000000000000, 0.9659258262890683122, 1.000000000000000000, 0.9659258262890683122, 1.000000000000000000, 0.9659258262890683122, 1.000000000000000000, 0.9659258262890683122, 1.000000000000000000, 0.9659258262890683122, 1.000000000000000000, 0.9659258262890683122, 1.000000000000000000, 0.9659258262890683122, 1.000000000000000000, 0.9659258262890683122, 1.000000000000000000, 0.9659258262890683122, 1.000000000000000000, 0.9659258262890683122, 1.000000000000000000, 0.9659258262890683122, 1.000000000000000000, 0.9659258262890683122, 1.000000000000000000, 0.9659258262890683122, 1.000000000000000000, 0.9659258262890683122, 1.000000000000000000, 0.9659258262890683122, 1.000000000000000000, 0.9659258262890683122, 1.000000000000000000, 0.9659258262890683122, 1.000000000000000000, 0.9659258262890683122, 1.000000000000000000, 0.9659258262890683122, 1.000000000000000000, 0.9659258262890683122, 1.000000000000000000, 0.9659258262890683122, 1.000000000000000000, 0.9659258262890683122, 1.000000000000000000, 0.9659258262890683122, 1.000000000000000000, 0.9659258262890683122, 1.000000000000000000, 0.9659258262890683122, 1.000000000000000000, 0.9659258262890683122, 1.000000000000000000, 0.9659258262890683122, 1.000000000000000000, 0.9659258262890683122, 1.000000000000000000, 0.9659258262890683122, 1.000000000000000000, 0.9659258262890683122, 1.000000000000000000, 0.9659258262890683122, 1.000000000000000000, 0.9659258262890683122, 1.000000000000000000, 0.9659258262890683122, 1.000000000000000000, 0.9659258262890683122, 1.000000000000000000) ) ) 
 REPRESENTATION_ITEM ( '' )  SURFACE ( )  );
#28883=CARTESIAN_POINT ( 'NONE',  ( -0.2690288713910754526, -0.5511811023622046335, 0.09757992244046803654 ) ) ;
#28884=ADVANCED_FACE ( 'NONE', ( #26803 ), #53837, .F. ) ;
#28885=CARTESIAN_POINT ( 'NONE',  ( -0.6692913385826764205, -0.5511811023622047445, 6.969142054262312111E-17 ) ) ;
#28887=CARTESIAN_POINT ( 'NONE',  ( -1.332020997375327642, -0.05778040916215522460, 0.4822834645669289988 ) ) ;
#28888=CARTESIAN_POINT ( 'NONE',  ( 0.4527559055118117182, -0.5400638737290844871, 0.3530559997133364547 ) ) ;
#28889=CARTESIAN_POINT ( 'NONE',  ( -1.043307086614172041, -0.5400638737290844871, 0.3530559997133364547 ) ) ;
#28891=EDGE_LOOP ( 'NONE', ( #3823, #2283, #73063, #25336 ) ) ;
#28892=CARTESIAN_POINT ( 'NONE',  ( -1.601049868766403650, 0.2306618581243847221, -0.2411417322834647770 ) ) ;
#28895=CARTESIAN_POINT ( 'NONE',  ( -1.646051170424378096, -0.1870078740157480046, 1.254653134982923898E-17 ) ) ;
#28898=CARTESIAN_POINT ( 'NONE',  ( -0.8530183727034112984, 0.05413385826771666132, 0.4176697321401328100 ) ) ;
#28899=CARTESIAN_POINT ( 'NONE',  ( 1.332020997375329197, -0.3162353388693405765, 0.4822834645669290543 ) ) ;
#28900=CARTESIAN_POINT ( 'NONE',  ( -1.627296587926508442, -0.6046776061558809534, -0.2411417322834644161 ) ) ;
#28902=CARTESIAN_POINT ( 'NONE',  ( -1.220472440944881054, 0.2952755905511811885, 0.000000000000000000 ) ) ;
#28903=CARTESIAN_POINT ( 'NONE',  ( -0.9842519685039365918, -0.6692913385826771977, 8.415575281601705876E-17 ) ) ;
#28906=CARTESIAN_POINT ( 'NONE',  ( 0.4855643044619428750, -0.004921259842519576551, 0.3153832671262227771 ) ) ;
#28908=CARTESIAN_POINT ( 'NONE',  ( 0.07217847769028949700, -0.2845877964562159024, 0.3641732283464567677 ) ) ;
#28909=CARTESIAN_POINT ( 'NONE',  ( 0.9383202099737536495, -0.2845877964562159024, 0.3641732283464567677 ) ) ;
#28910=CARTESIAN_POINT ( 'NONE',  ( 0.8333333333333340365, 0.2952755905511810774, -0.1292274648535930714 ) ) ;
#28911=CARTESIAN_POINT ( 'NONE',  ( -0.2821522309711278487, -0.5511811023622048555, -0.09757992244046775898 ) ) ;
#28913=CARTESIAN_POINT ( 'NONE',  ( 1.574803149606299746, -0.1870078740157479769, 0.4822834645669291653 ) ) ;
#28914=CARTESIAN_POINT ( 'NONE',  ( -1.417322834645668772, -0.1870078740157480601, -0.3641732283464567677 ) ) ;
#28916=CARTESIAN_POINT ( 'NONE',  ( 0.02624671916010564918, -0.6046776061558809534, -0.2411417322834644161 ) ) ;
#28917=CARTESIAN_POINT ( 'NONE',  ( 1.489501312335958172, -0.2845877964562159024, 0.3641732283464567677 ) ) ;
#28918=CARTESIAN_POINT ( 'NONE',  ( 0.6430446194225728496, -0.004921259842519576551, 0.3153832671262227771 ) ) ;
#28919=CARTESIAN_POINT ( 'NONE',  ( -0.2493438320209966919, -0.004921259842519870586, -0.3153832671262229437 ) ) ;
#28920=CARTESIAN_POINT ( 'NONE',  ( -0.6889763779527552368, 0.1660481256975885056, 0.3530559997133364547 ) ) ;
#28921=LINE ( 'NONE', #16728, #6261 ) ;
#28923=CARTESIAN_POINT ( 'NONE',  ( 0.2099737532808405305, -0.6046776061558807314, 0.2411417322834647770 ) ) ;
#28926=CARTESIAN_POINT ( 'NONE',  ( -0.2493438320209966919, -0.004921259842519870586, -0.3153832671262229437 ) ) ;
#28927=CARTESIAN_POINT ( 'NONE',  ( 0.03280839895013198948, 0.2952755905511811885, 0.1292274648535926551 ) ) ;
#28928=CARTESIAN_POINT ( 'NONE',  ( -1.614173228346455824, 0.2952755905511811885, 0.000000000000000000 ) ) ;
#28929=CARTESIAN_POINT ( 'NONE',  ( -1.548556430446193399, -0.5023911411419708095, -0.1820866141732282451 ) ) ;
#28930=CARTESIAN_POINT ( 'NONE',  ( 1.148293963254593875, -0.6692913385826771977, 0.1292274648535927661 ) ) ;
#28931=CARTESIAN_POINT ( 'NONE',  ( -1.259842519685038686, -0.1870078740157480879, -0.4822834645669291653 ) ) ;
#28932=CARTESIAN_POINT ( 'NONE',  ( -0.8005249343832013809, -0.3690944881889763329, 0.3153832671262228327 ) ) ;
#28936=CARTESIAN_POINT ( 'NONE',  ( 0.6167979002624679463, 0.05413385826771626580, -0.4176697321401330321 ) ) ;
#28939=CARTESIAN_POINT ( 'NONE',  ( 1.095800524934383846, -0.2845877964562159024, 0.3641732283464567677 ) ) ;
#28942=CARTESIAN_POINT ( 'NONE',  ( 0.8202099737532813073, 0.2952755905511811885, 0.1292274648535926551 ) ) ;
#28944=CARTESIAN_POINT ( 'NONE',  ( 1.062992125984252745, 0.1771653543307087630, 0.000000000000000000 ) ) ;
#28946=CARTESIAN_POINT ( 'NONE',  ( 0.2034120734908144990, -0.6692913385826771977, 0.1292274648535927661 ) ) ;
#28947=CARTESIAN_POINT ( 'NONE',  ( -0.9055118110236215490, -0.6692913385826771977, 8.415575281601705876E-17 ) ) ;
#28951=CARTESIAN_POINT ( 'NONE',  ( 0.4002624671916016896, -0.2845877964562161244, -0.3641732283464567121 ) ) ;
#28952=ORIENTED_EDGE ( 'NONE', *, *, #58971, .F. ) ;
#28955=CARTESIAN_POINT ( 'NONE',  ( -0.3412073490813641308, -0.6046776061558807314, 0.2411417322834647770 ) ) ;
#28956=CARTESIAN_POINT ( 'NONE',  ( -0.3412073490813641308, 0.2306618581243847221, -0.2411417322834647770 ) ) ;
#28957=CARTESIAN_POINT ( 'NONE',  ( -0.4002624671916004129, -0.2845877964562159024, 0.3641732283464567677 ) ) ;
#28958=CARTESIAN_POINT ( 'NONE',  ( 0.6758530183727039509, -0.6692913385826771977, 0.1292274648535927661 ) ) ;
#28959=CARTESIAN_POINT ( 'NONE',  ( -0.7939632545931750718, -0.05778040916215560624, -0.4822834645669293319 ) ) ;
#28960=CARTESIAN_POINT ( 'NONE',  ( -0.3608923884514428360, -0.6692913385826773087, -0.1292274648535924053 ) ) ;
#28961=CARTESIAN_POINT ( 'NONE',  ( 1.023622047244095112, -0.1870078740157480879, -0.4822834645669291653 ) ) ;
#28962=CARTESIAN_POINT ( 'NONE',  ( 0.8923884514435701520, -0.6046776061558809534, -0.2411417322834644161 ) ) ;
#28963=CARTESIAN_POINT ( 'NONE',  ( 0.8661417322834653598, -0.1870078740157479769, 0.4822834645669291653 ) ) ;
#28966=CARTESIAN_POINT ( 'NONE',  ( -0.1574803149606292529, -0.1870078740157480601, -0.3641732283464567677 ) ) ;
#28970=CARTESIAN_POINT ( 'NONE',  ( -0.7677165354330699465, 0.07958543189024085140, 0.2665933059059887866 ) ) ;
#28971=CARTESIAN_POINT ( 'NONE',  ( -0.6102362204724400829, -0.5400638737290845981, -0.3530559997133363437 ) ) ;
#28973=CARTESIAN_POINT ( 'NONE',  ( -0.2296587926509179312, -0.3162353388693409650, -0.4822834645669289433 ) ) ;
#28974=CARTESIAN_POINT ( 'NONE',  ( -0.2821522309711278487, 0.2952755905511811885, 0.1292274648535926551 ) ) ;
#28975=CARTESIAN_POINT ( 'NONE',  ( -1.233595800524933894, -0.6046776061558809534, -0.2411417322834644161 ) ) ;
#28976=CARTESIAN_POINT ( 'NONE',  ( -1.410761154855642463, -0.05778040916215522460, 0.4822834645669289988 ) ) ;
#28977=CARTESIAN_POINT ( 'NONE',  ( 0.9908136482939640111, -0.5511811023622046335, 0.09757992244046803654 ) ) ;
#28980=CARTESIAN_POINT ( 'NONE',  ( 0.6364829396325465405, -0.08942795157527998196, 0.3641732283464567121 ) ) ;
#28981=CARTESIAN_POINT ( 'NONE',  ( 0.06561679790026316017, -0.4281496062992124485, 0.4176697321401328655 ) ) ;
#28982=CARTESIAN_POINT ( 'NONE',  ( 0.4527559055118117182, 0.1660481256975883668, -0.3530559997133364547 ) ) ;
#28986=ORIENTED_EDGE ( 'NONE', *, *, #64378, .T. ) ;
#28989=CARTESIAN_POINT ( 'NONE',  ( -0.7808398950131225646, -0.08942795157527998196, 0.3641732283464567121 ) ) ;
#28990=CARTESIAN_POINT ( 'NONE',  ( -1.115485564304461219, -0.4281496062992124485, 0.4176697321401328655 ) ) ;
#28993=CARTESIAN_POINT ( 'NONE',  ( 1.653543307086614789, -0.1870078740157479769, 0.4822834645669291653 ) ) ;
#28994=CARTESIAN_POINT ( 'NONE',  ( 0.7283464566929140904, -0.5400638737290845981, -0.3530559997133363437 ) ) ;
#28995=CARTESIAN_POINT ( 'NONE',  ( 0.6692913385826778638, -0.6692913385826771977, 8.415575281601705876E-17 ) ) ;
#28996=CARTESIAN_POINT ( 'NONE',  ( -0.5183727034120726440, 0.1771653543307087630, 0.09757992244046791164 ) ) ;
#28997=CARTESIAN_POINT ( 'NONE',  ( 0.06561679790026316017, 0.05413385826771626580, -0.4176697321401330321 ) ) ;
#28999=CARTESIAN_POINT ( 'NONE',  ( -0.7020997375328074108, -0.08942795157527998196, 0.3641732283464567121 ) ) ;
#29000=CARTESIAN_POINT ( 'NONE',  ( -0.3018372703412066094, 0.05413385826771666132, 0.4176697321401328100 ) ) ;
#29002=CARTESIAN_POINT ( 'NONE',  ( -1.528871391076114250, 0.2952755905511810774, -0.1292274648535930714 ) ) ;
#29003=CARTESIAN_POINT ( 'NONE',  ( -0.1049868766404193215, 0.1283753931104746893, -0.1820866141732285504 ) ) ;
#29004=CARTESIAN_POINT ( 'NONE',  ( 1.614173228346457378, -0.5511811023622047445, 6.969142054262312111E-17 ) ) ;
#29005=CARTESIAN_POINT ( 'NONE',  ( -1.089238845144356427, 0.05413385826771666132, 0.4176697321401328100 ) ) ;
#29006=CARTESIAN_POINT ( 'NONE',  ( -0.8333333333333323711, 0.1771653543307087630, 0.09757992244046791164 ) ) ;
#29008=CARTESIAN_POINT ( 'NONE',  ( -1.043307086614172707, 0.1660481256975883668, -0.3530559997133364547 ) ) ;
#29009=CARTESIAN_POINT ( 'NONE',  ( -0.5183727034120726440, 0.2952755905511811885, 0.1292274648535926551 ) ) ;
#29010=( BOUNDED_CURVE ( )  B_SPLINE_CURVE ( 3, ( #47203, #72893, #15243, #37782 ),
 .UNSPECIFIED., .F., .F. ) 
 B_SPLINE_CURVE_WITH_KNOTS ( ( 4, 4 ),
 ( 4.502511237001506572, 4.502773989760327389 ),
 .UNSPECIFIED. ) 
 CURVE ( )  GEOMETRIC_REPRESENTATION_ITEM ( )  RATIONAL_B_SPLINE_CURVE ( ( 1.000000000000000000, 0.9999999942467490133, 0.9999999942467490133, 1.000000000000000000 ) ) 
 REPRESENTATION_ITEM ( '' )  );
#29011=CARTESIAN_POINT ( 'NONE',  ( 0.1771653543307093182, -0.5400638737290845981, -0.3530559997133363437 ) ) ;
#29015=CARTESIAN_POINT ( 'NONE',  ( 0.2624671916010504757, 0.1283753931104748280, 0.1820866141732283561 ) ) ;
#29016=CARTESIAN_POINT ( 'NONE',  ( 0.9645669291338588858, 0.1660481256975885056, 0.3530559997133364547 ) ) ;
#29017=CARTESIAN_POINT ( 'NONE',  ( -1.161417322834644716, -0.4536011799217368745, -0.2665933059059886201 ) ) ;
#29018=CARTESIAN_POINT ( 'NONE',  ( 1.253280839895013710, -0.05778040916215560624, -0.4822834645669293319 ) ) ;
#29019=CARTESIAN_POINT ( 'NONE',  ( -1.581364829396324945, -0.2845877964562159024, 0.3641732283464567677 ) ) ;
#29020=CARTESIAN_POINT ( 'NONE',  ( -0.4002624671916004129, -0.05778040916215560624, -0.4822834645669293319 ) ) ;
#29021=CARTESIAN_POINT ( 'NONE',  ( 0.2821522309711292364, 0.1771653543307087075, -0.09757992244046823083 ) ) ;
#29022=DIRECTION ( 'NONE',  ( -0.4999999999999886202, 0.7071067811865615615, -0.4999999999999915068 ) ) ;
#29023=CARTESIAN_POINT ( 'NONE',  ( 0.6430446194225728496, -0.004921259842519576551, 0.3153832671262227771 ) ) ;
#29025=CARTESIAN_POINT ( 'NONE',  ( -0.2296587926509179312, -0.05778040916215522460, 0.4822834645669289988 ) ) ;
#29027=CARTESIAN_POINT ( 'NONE',  ( -0.9842519685039365918, -0.6692913385826771977, 8.415575281601705876E-17 ) ) ;
#29029=CARTESIAN_POINT ( 'NONE',  ( 0.9908136482939640111, 0.1771653543307087075, -0.09757992244046823083 ) ) ;
#29030=CARTESIAN_POINT ( 'NONE',  ( 8.195543980992789655E-16, -0.1870078740157480879, -0.4822834645669291653 ) ) ;
#29031=CARTESIAN_POINT ( 'NONE',  ( -0.4396325459317577122, -0.6692913385826773087, -0.1292274648535924053 ) ) ;
#29032=CARTESIAN_POINT ( 'NONE',  ( -0.3805774278215216522, -0.004921259842519576551, 0.3153832671262227771 ) ) ;
#29034=CARTESIAN_POINT ( 'NONE',  ( -0.3805774278215216522, -0.004921259842519576551, 0.3153832671262227771 ) ) ;
#29035=CARTESIAN_POINT ( 'NONE',  ( 0.3674540682414705883, -0.6046776061558807314, 0.2411417322834647770 ) ) ;
#29036=CARTESIAN_POINT ( 'NONE',  ( -1.338582677165353729, -0.1870078740157480601, -0.3641732283464567677 ) ) ;
#29038=CARTESIAN_POINT ( 'NONE',  ( -1.259842519685038686, -0.1870078740157480879, -0.4822834645669291653 ) ) ;
#29041=CARTESIAN_POINT ( 'NONE',  ( -1.450131233595799651, -0.5511811023622046335, 0.09757992244046803654 ) ) ;
#29042=CARTESIAN_POINT ( 'NONE',  ( -0.5839895013123351797, 0.2952755905511810774, -0.1292274648535930714 ) ) ;
#29044=CARTESIAN_POINT ( 'NONE',  ( -1.391076115485563314, -0.6046776061558809534, -0.2411417322834644161 ) ) ;
#29047=CARTESIAN_POINT ( 'NONE',  ( 1.351706036745407680, 0.05413385826771666132, 0.4176697321401328100 ) ) ;
#29048=CARTESIAN_POINT ( 'NONE',  ( 0.7874015748031503170, -0.1870078740157480879, -0.4822834645669291653 ) ) ;
#29049=CARTESIAN_POINT ( 'NONE',  ( 1.092353285368624860, -4.408777212815537393E-16, -0.4445507791589063395 ) ) ;
#29053=CARTESIAN_POINT ( 'NONE',  ( 1.561679790026247350, -0.3690944881889763329, 0.3153832671262228327 ) ) ;
#29056=CARTESIAN_POINT ( 'NONE',  ( -0.6824146981627288167, 0.1283753931104748280, 0.1820866141732283561 ) ) ;
#29059=CARTESIAN_POINT ( 'NONE',  ( 0.7020997375328090762, -0.05778040916215560624, -0.4822834645669293319 ) ) ;
#29060=CARTESIAN_POINT ( 'NONE',  ( -0.2690288713910754526, 0.2952755905511810774, -0.1292274648535930714 ) ) ;
#29061=CARTESIAN_POINT ( 'NONE',  ( -0.9711286089238838626, 0.2306618581243847221, -0.2411417322834647770 ) ) ;
#29062=CARTESIAN_POINT ( 'NONE',  ( 1.410761154855643795, -0.05778040916215560624, -0.4822834645669293319 ) ) ;
#29063=CARTESIAN_POINT ( 'NONE',  ( -1.391076115485563314, -0.5023911411419708095, -0.1820866141732282451 ) ) ;
#29065=CARTESIAN_POINT ( 'NONE',  ( 0.3543307086614181922, -0.6692913385826771977, 8.415575281601705876E-17 ) ) ;
#29066=CARTESIAN_POINT ( 'NONE',  ( -0.9186351706036736120, -0.6046776061558809534, -0.2411417322834644161 ) ) ;
#29068=CARTESIAN_POINT ( 'NONE',  ( -1.102362204724408601, -0.1870078740157480879, -0.4822834645669291653 ) ) ;
#29070=CARTESIAN_POINT ( 'NONE',  ( 0.8530183727034128527, -0.4281496062992124485, 0.4176697321401328655 ) ) ;
#29071=CARTESIAN_POINT ( 'NONE',  ( 1.305774278215223960, -0.5511811023622046335, 0.09757992244046803654 ) ) ;
#29072=VERTEX_POINT ( 'NONE', #80565 ) ;
#29074=CARTESIAN_POINT ( 'NONE',  ( -0.5577427821522301654, -0.3162353388693405765, 0.4822834645669290543 ) ) ;
#29076=CARTESIAN_POINT ( 'NONE',  ( 0.4002624671916016896, -0.2845877964562161244, -0.3641732283464567121 ) ) ;
#29079=CARTESIAN_POINT ( 'NONE',  ( 0.9383202099737536495, -0.3162353388693405765, 0.4822834645669290543 ) ) ;
#29080=CARTESIAN_POINT ( 'NONE',  ( 0.8398950131233602345, 0.2306618581243847221, -0.2411417322834647770 ) ) ;
#29081=CARTESIAN_POINT ( 'NONE',  ( -0.3477690288713905509, -0.6692913385826771977, 0.1292274648535927661 ) ) ;
#29083=CARTESIAN_POINT ( 'NONE',  ( -0.7480314960629914633, -0.6692913385826771977, 8.415575281601705876E-17 ) ) ;
#29085=CARTESIAN_POINT ( 'NONE',  ( -1.463254593175852492, -0.6692913385826773087, -0.1292274648535924053 ) ) ;
#29086=CARTESIAN_POINT ( 'NONE',  ( -1.010498687664041384, 0.05413385826771666132, 0.4176697321401328100 ) ) ;
#29087=CARTESIAN_POINT ( 'NONE',  ( 1.397637795275591177, 0.1660481256975883668, -0.3530559997133364547 ) ) ;
#29089=CARTESIAN_POINT ( 'NONE',  ( -0.9120734908136475250, 0.2952755905511811885, 0.1292274648535926551 ) ) ;
#29091=CARTESIAN_POINT ( 'NONE',  ( 0.1706036745406830368, 0.05413385826771666132, 0.4176697321401328100 ) ) ;
#29093=CARTESIAN_POINT ( 'NONE',  ( -0.5577427821522301654, -0.3162353388693405765, 0.4822834645669290543 ) ) ;
#29094=CARTESIAN_POINT ( 'NONE',  ( -1.450131233595799651, 0.1771653543307087075, -0.09757992244046823083 ) ) ;
#29095=CARTESIAN_POINT ( 'NONE',  ( 0.5380577427821529035, -0.3690944881889763329, 0.3153832671262228327 ) ) ;
#29096=CARTESIAN_POINT ( 'NONE',  ( 1.213910761154856299, -0.6692913385826773087, -0.1292274648535924053 ) ) ;
#29098=CARTESIAN_POINT ( 'NONE',  ( 1.154855643044620184, -0.5023911411419708095, 0.1820866141732285504 ) ) ;
#29100=CARTESIAN_POINT ( 'NONE',  ( 0.7283464566929140904, -0.5400638737290845981, -0.3530559997133363437 ) ) ;
#29102=CARTESIAN_POINT ( 'NONE',  ( -0.5446194225721777693, -0.3162353388693409650, -0.4822834645669289433 ) ) ;
#29104=CARTESIAN_POINT ( 'NONE',  ( 1.496062992125984703, -0.1870078740157480601, -0.3641732283464567677 ) ) ;
#29105=CARTESIAN_POINT ( 'NONE',  ( -0.4921259842519677963, -0.5400638737290844871, 0.3530559997133364547 ) ) ;
#29108=CARTESIAN_POINT ( 'NONE',  ( 1.430446194225722500, -0.4281496062992127816, -0.4176697321401328100 ) ) ;
#29109=CARTESIAN_POINT ( 'NONE',  ( 0.06561679790026316017, 0.05413385826771626580, -0.4176697321401330321 ) ) ;
#29110=CARTESIAN_POINT ( 'NONE',  ( 0.5708661417322842269, 0.07958543189024085140, 0.2665933059059887866 ) ) ;
#29112=CARTESIAN_POINT ( 'NONE',  ( -0.1181102362204717315, -0.5511811023622047445, 6.969142054262312111E-17 ) ) ;
#29113=CARTESIAN_POINT ( 'NONE',  ( -1.528871391076114250, -0.6692913385826771977, 0.1292274648535927661 ) ) ;
#29115=CARTESIAN_POINT ( 'NONE',  ( 0.8202099737532814183, -0.6692913385826773087, -0.1292274648535924053 ) ) ;
#29120=CARTESIAN_POINT ( 'NONE',  ( 1.614173228346457378, -0.5511811023622047445, 6.969142054262312111E-17 ) ) ;
#29122=CARTESIAN_POINT ( 'NONE',  ( -0.1706036745406816491, -0.3690944881889763329, 0.3153832671262228327 ) ) ;
#29123=CARTESIAN_POINT ( 'NONE',  ( 0.02624671916010564918, -0.6046776061558809534, -0.2411417322834644161 ) ) ;
#29124=CARTESIAN_POINT ( 'NONE',  ( 1.266404199475066328, -0.2845877964562161244, -0.3641732283464567121 ) ) ;
#29125=CARTESIAN_POINT ( 'NONE',  ( -1.325459317585300889, -0.3690944881889765550, -0.3153832671262227771 ) ) ;
#29126=CARTESIAN_POINT ( 'NONE',  ( -1.253280839895012377, -0.05778040916215522460, 0.4822834645669289988 ) ) ;
#29127=CARTESIAN_POINT ( 'NONE',  ( 0.5183727034120741983, -0.6692913385826771977, 0.1292274648535927661 ) ) ;
#29129=CARTESIAN_POINT ( 'NONE',  ( 1.299212598425197429, -0.6692913385826771977, 8.415575281601705876E-17 ) ) ;
#29131=CARTESIAN_POINT ( 'NONE',  ( -0.04593175853018302557, -0.6692913385826773087, -0.1292274648535924053 ) ) ;
#29132=CARTESIAN_POINT ( 'NONE',  ( 1.187664041994751285, -0.05778040916215522460, 0.4822834645669289988 ) ) ;
#29133=CARTESIAN_POINT ( 'NONE',  ( 0.9186351706036752773, 0.2306618581243847221, -0.2411417322834647770 ) ) ;
#29134=CARTESIAN_POINT ( 'NONE',  ( 1.614173228346456712, 2.401574803149606474, 0.1372047244094478646 ) ) ;
#29135=CARTESIAN_POINT ( 'NONE',  ( 0.9514435695538062676, -0.2845877964562161244, -0.3641732283464567121 ) ) ;
#29136=CARTESIAN_POINT ( 'NONE',  ( -1.522309711286088607, -0.5023911411419708095, 0.1820866141732285504 ) ) ;
#29138=CARTESIAN_POINT ( 'NONE',  ( -0.03280839895013062252, -0.5511811023622046335, 0.09757992244046803654 ) ) ;
#29139=CARTESIAN_POINT ( 'NONE',  ( 0.05905511811023709395, -0.5400638737290844871, 0.3530559997133364547 ) ) ;
#29140=CARTESIAN_POINT ( 'NONE',  ( 0.8202099737532813073, 0.2952755905511811885, 0.1292274648535926551 ) ) ;
#29141=CARTESIAN_POINT ( 'NONE',  ( -0.2230971128608915943, 0.05413385826771666132, 0.4176697321401328100 ) ) ;
#29142=CARTESIAN_POINT ( 'NONE',  ( -0.2427821522309703550, -0.08942795157528024563, -0.3641732283464568787 ) ) ;
#29143=CARTESIAN_POINT ( 'NONE',  ( 0.8070866141732288002, 0.1660481256975885056, 0.3530559997133364547 ) ) ;
#29144=CARTESIAN_POINT ( 'NONE',  ( 0.7808398950131241190, -0.08942795157528024563, -0.3641732283464568787 ) ) ;
#29149=CARTESIAN_POINT ( 'NONE',  ( -1.259842519685038686, -0.1870078740157480879, -0.4822834645669291653 ) ) ;
#29150=CARTESIAN_POINT ( 'NONE',  ( -0.6758530183727028406, -0.6692913385826773087, -0.1292274648535924053 ) ) ;
#29154=CARTESIAN_POINT ( 'NONE',  ( 0.8595800524934390507, -0.2845877964562159024, 0.3641732283464567677 ) ) ;
#29156=CARTESIAN_POINT ( 'NONE',  ( 0.9842519685039375910, 0.2952755905511811885, 0.000000000000000000 ) ) ;
#29158=CARTESIAN_POINT ( 'NONE',  ( -1.430446194225721390, -0.3690944881889763329, 0.3153832671262228327 ) ) ;
#29159=CARTESIAN_POINT ( 'NONE',  ( 1.541994750656168645, 0.2952755905511810774, -0.1292274648535930714 ) ) ;
#29160=CARTESIAN_POINT ( 'NONE',  ( 1.423884514435696191, -0.08942795157527998196, 0.3641732283464567121 ) ) ;
#29161=CARTESIAN_POINT ( 'NONE',  ( 0.3280839895013130669, -0.4281496062992127816, -0.4176697321401328100 ) ) ;
#29162=AXIS2_PLACEMENT_3D ( 'NONE', #60822, #67158, #9487 ) ;
#29164=CARTESIAN_POINT ( 'NONE',  ( 0.1049868766404206816, 0.2306618581243848609, 0.2411417322834645549 ) ) ;
#29165=CARTESIAN_POINT ( 'NONE',  ( -0.7020997375328076329, -0.2845877964562161244, -0.3641732283464567121 ) ) ;
#29166=CARTESIAN_POINT ( 'NONE',  ( 0.8333333333333340365, 0.2952755905511810774, -0.1292274648535930714 ) ) ;
#29167=CARTESIAN_POINT ( 'NONE',  ( -0.1246719160104980823, 0.2952755905511811885, 0.1292274648535926551 ) ) ;
#29169=AXIS2_PLACEMENT_3D ( 'NONE', #61825, #81620, #17235 ) ;
#29172=CARTESIAN_POINT ( 'NONE',  ( 0.8464566929133866546, -0.5400638737290844871, 0.3530559997133364547 ) ) ;
#29175=CARTESIAN_POINT ( 'NONE',  ( -0.03937007874015669567, -0.6692913385826771977, 8.415575281601705876E-17 ) ) ;
#29176=CARTESIAN_POINT ( 'NONE',  ( -0.8595800524934373854, -0.05778040916215522460, 0.4822834645669289988 ) ) ;
#29177=CARTESIAN_POINT ( 'NONE',  ( 1.233595800524935227, -0.6046776061558807314, 0.2411417322834647770 ) ) ;
#29178=CARTESIAN_POINT ( 'NONE',  ( 0.6561679790026253567, -0.6046776061558809534, -0.2411417322834644161 ) ) ;
#29180=CARTESIAN_POINT ( 'NONE',  ( -0.3805774278215216522, -0.4281496062992127816, -0.4176697321401328100 ) ) ;
#29181=CARTESIAN_POINT ( 'NONE',  ( 0.5577427821522316087, -0.05778040916215522460, 0.4822834645669289988 ) ) ;
#29182=CARTESIAN_POINT ( 'NONE',  ( -0.1443569553805765515, -0.4281496062992127816, -0.4176697321401328100 ) ) ;
#29183=CARTESIAN_POINT ( 'NONE',  ( 0.5905511811023629321, 0.1771653543307087630, 0.000000000000000000 ) ) ;
#29184=CARTESIAN_POINT ( 'NONE',  ( -1.568241469816272105, -0.05778040916215522460, 0.4822834645669289988 ) ) ;
#29186=CARTESIAN_POINT ( 'NONE',  ( 0.4002624671916016896, -0.3162353388693409650, -0.4822834645669289433 ) ) ;
#29187=PRESENTATION_STYLE_ASSIGNMENT (( #55667 ) ) ;
#29190=VERTEX_POINT ( 'NONE', #81799 ) ;
#29191=CARTESIAN_POINT ( 'NONE',  ( 0.6233595800524942554, -0.05778040916215560624, -0.4822834645669293319 ) ) ;
#29192=CARTESIAN_POINT ( 'NONE',  ( 0.6430446194225728496, -0.004921259842519576551, 0.3153832671262227771 ) ) ;
#29199=EDGE_CURVE ( 'NONE', #64485, #18885, #67225, .T. ) ;
#29201=CARTESIAN_POINT ( 'NONE',  ( 1.023622047244095112, -0.1870078740157480879, -0.4822834645669291653 ) ) ;
#29202=CARTESIAN_POINT ( 'NONE',  ( -1.010498687664041384, 0.05413385826771666132, 0.4176697321401328100 ) ) ;
#29203=CARTESIAN_POINT ( 'NONE',  ( -0.8202099737532801971, -0.6692913385826771977, 0.1292274648535927661 ) ) ;
#29204=CARTESIAN_POINT ( 'NONE',  ( 0.7283464566929140904, -0.5400638737290845981, -0.3530559997133363437 ) ) ;
#29205=CARTESIAN_POINT ( 'NONE',  ( 1.213910761154856299, -0.6692913385826773087, -0.1292274648535924053 ) ) ;
#29208=CARTESIAN_POINT ( 'NONE',  ( 1.286089238845145033, -0.5023911411419708095, -0.1820866141732282451 ) ) ;
#29210=CARTESIAN_POINT ( 'NONE',  ( -1.437007874015747477, 0.07958543189024071263, -0.2665933059059888421 ) ) ;
#29212=CARTESIAN_POINT ( 'NONE',  ( 0.006561679790026889343, -0.3162353388693409650, -0.4822834645669289433 ) ) ;
#29213=CARTESIAN_POINT ( 'NONE',  ( 1.528871391076116026, 0.2952755905511811885, 0.1292274648535926551 ) ) ;
#29214=DIRECTION ( 'NONE',  ( -1.000000000000000000, 0.000000000000000000, 0.000000000000000000 ) ) ;
#29215=CARTESIAN_POINT ( 'NONE',  ( -1.161417322834644716, -0.4536011799217368745, -0.2665933059059886201 ) ) ;
#29216=CARTESIAN_POINT ( 'NONE',  ( 0.4199475065616805614, 0.2306618581243848609, 0.2411417322834645549 ) ) ;
#29217=CARTESIAN_POINT ( 'NONE',  ( 1.259842519685040019, -0.1870078740157479769, 0.3641732283464567677 ) ) ;
#29219=CARTESIAN_POINT ( 'NONE',  ( -1.148293963254592542, -0.5511811023622048555, -0.09757992244046775898 ) ) ;
#29220=CARTESIAN_POINT ( 'NONE',  ( 1.522309711286089939, 0.2306618581243848609, 0.2411417322834645549 ) ) ;
#29222=CARTESIAN_POINT ( 'NONE',  ( -0.1115485564304456306, 0.2952755905511810774, -0.1292274648535930714 ) ) ;
#29223=CARTESIAN_POINT ( 'NONE',  ( -1.279527559055116948, 0.07958543189024071263, -0.2665933059059888421 ) ) ;
#29224=CARTESIAN_POINT ( 'NONE',  ( -0.5183727034120726440, -0.6692913385826773087, -0.1292274648535924053 ) ) ;
#29225=CARTESIAN_POINT ( 'NONE',  ( -1.646981627296586703, -0.08942795157527998196, 0.3641732283464567121 ) ) ;
#29227=CARTESIAN_POINT ( 'NONE',  ( 0.1246719160104994284, -0.6692913385826771977, 0.1292274648535927661 ) ) ;
#29229=CARTESIAN_POINT ( 'NONE',  ( 1.410761154855643795, -0.3162353388693405765, 0.4822834645669290543 ) ) ;
#29230=AXIS2_PLACEMENT_3D ( 'NONE', #15073, #40731, #66415 ) ;
#29232=CARTESIAN_POINT ( 'NONE',  ( -1.266404199475064773, -0.3162353388693405765, 0.4822834645669290543 ) ) ;
#29233=CARTESIAN_POINT ( 'NONE',  ( -0.6692913385826764205, -0.5511811023622047445, 6.969142054262312111E-17 ) ) ;
#29235=CARTESIAN_POINT ( 'NONE',  ( -0.02624671916010428221, 0.2306618581243847221, -0.2411417322834647770 ) ) ;
#29236=CARTESIAN_POINT ( 'NONE',  ( 0.5249343832021005074, -0.5023911411419708095, 0.1820866141732285504 ) ) ;
#29237=CARTESIAN_POINT ( 'NONE',  ( -1.056430446194224881, 0.1771653543307087075, -0.09757992244046823083 ) ) ;
#29238=CARTESIAN_POINT ( 'NONE',  ( -1.351706036745406347, 0.05413385826771626580, -0.4176697321401330321 ) ) ;
#29239=CARTESIAN_POINT ( 'NONE',  ( -1.614173228346456268, -0.6692913385826771977, 8.415575281601705876E-17 ) ) ;
#29240=CARTESIAN_POINT ( 'NONE',  ( 1.358267716535433323, 0.1660481256975885056, 0.3530559997133364547 ) ) ;
#29242=CARTESIAN_POINT ( 'NONE',  ( 0.4855643044619430415, -0.3690944881889765550, -0.3153832671262227771 ) ) ;
#29243=CARTESIAN_POINT ( 'NONE',  ( 0.9448818897637802916, -0.1870078740157480879, -0.4822834645669291653 ) ) ;
#29245=CARTESIAN_POINT ( 'NONE',  ( 1.594488188976378673, 0.07958543189024085140, 0.2665933059059887866 ) ) ;
#29247=CARTESIAN_POINT ( 'NONE',  ( -1.115485564304461219, 0.05413385826771626580, -0.4176697321401330321 ) ) ;
#29248=CARTESIAN_POINT ( 'NONE',  ( -0.9186351706036736120, -0.6046776061558809534, -0.2411417322834644161 ) ) ;
#29249=CARTESIAN_POINT ( 'NONE',  ( 0.3543307086614179147, 0.2952755905511811885, 0.000000000000000000 ) ) ;
#29250=CARTESIAN_POINT ( 'NONE',  ( 0.5400834452262274210, 1.809133623825372073E-16, -0.3954985857520062487 ) ) ;
#29252=CARTESIAN_POINT ( 'NONE',  ( 1.010498687664042716, 0.05413385826771626580, -0.4176697321401330321 ) ) ;
#29253=CARTESIAN_POINT ( 'NONE',  ( 1.463254593175853824, 0.1771653543307087075, -0.09757992244046823083 ) ) ;
#29254=CARTESIAN_POINT ( 'NONE',  ( 0.4724409448818904789, -0.1870078740157480879, -0.4822834645669291653 ) ) ;
#29255=CARTESIAN_POINT ( 'NONE',  ( 0.6233595800524939223, -0.3162353388693405765, 0.4822834645669290543 ) ) ;
#29259=CARTESIAN_POINT ( 'NONE',  ( -0.7426113562971995430, 1.972848275015057995, -0.5309055118110235227 ) ) ;
#29261=CARTESIAN_POINT ( 'NONE',  ( -0.05905511811023545637, -0.4536011799217368745, -0.2665933059059886201 ) ) ;
#29262=CARTESIAN_POINT ( 'NONE',  ( -0.2099737532808391705, -0.6046776061558809534, -0.2411417322834644161 ) ) ;
#29263=CARTESIAN_POINT ( 'NONE',  ( 0.8989501312335963501, -0.6692913385826773087, -0.1292274648535924053 ) ) ;
#29265=CARTESIAN_POINT ( 'NONE',  ( 0.04593175853018440641, -0.5511811023622046335, 0.09757992244046803654 ) ) ;
#29266=CARTESIAN_POINT ( 'NONE',  ( -1.102362204724408601, -0.1870078740157480879, -0.4822834645669291653 ) ) ;
#29267=CARTESIAN_POINT ( 'NONE',  ( 1.102362204724410155, -0.1870078740157479769, 0.4822834645669291653 ) ) ;
#29270=DIRECTION ( 'NONE',  ( 0.000000000000000000, 0.000000000000000000, 1.000000000000000000 ) ) ;
#29272=ORIENTED_EDGE ( 'NONE', *, *, #31494, .T. ) ;
#29273=CARTESIAN_POINT ( 'NONE',  ( 1.043307086614173818, -0.5400638737290845981, -0.3530559997133363437 ) ) ;
#29274=CARTESIAN_POINT ( 'NONE',  ( 1.292650918635171564, 0.1771653543307087630, 0.09757992244046791164 ) ) ;
#29275=CARTESIAN_POINT ( 'NONE',  ( -1.417322834645668772, -0.1870078740157480601, -0.3641732283464567677 ) ) ;
#29276=CARTESIAN_POINT ( 'NONE',  ( -1.404199475065615932, -0.4281496062992127816, -0.4176697321401328100 ) ) ;
#29279=CARTESIAN_POINT ( 'NONE',  ( 1.338582677165355062, -0.1870078740157479769, 0.4822834645669291653 ) ) ;
#29280=CARTESIAN_POINT ( 'NONE',  ( -1.522309711286088607, 0.2306618581243847221, -0.2411417322834647770 ) ) ;
#29281=CARTESIAN_POINT ( 'NONE',  ( 0.1246719160104994284, -0.6692913385826771977, 0.1292274648535927661 ) ) ;
#29282=CARTESIAN_POINT ( 'NONE',  ( -0.5577427821522301654, -0.05778040916215560624, -0.4822834645669293319 ) ) ;
#29283=CARTESIAN_POINT ( 'NONE',  ( 1.430446194225722500, 0.05413385826771666132, 0.4176697321401328100 ) ) ;
#29285=ADVANCED_FACE ( 'NONE', ( #55263 ), #11320, .F. ) ;
#29286=CARTESIAN_POINT ( 'NONE',  ( 0.3280839895013130669, 0.05413385826771666132, 0.4176697321401328100 ) ) ;
#29288=CARTESIAN_POINT ( 'NONE',  ( 1.541994750656168645, 0.2952755905511810774, -0.1292274648535930714 ) ) ;
#29291=VERTEX_POINT ( 'NONE', #40612 ) ;
#29292=CARTESIAN_POINT ( 'NONE',  ( 0.4849061582275024929, 1.726086921369708538, -0.4921425059946356040 ) ) ;
#29294=CARTESIAN_POINT ( 'NONE',  ( -1.725721784776902190, -0.05778040916215522460, 0.4822834645669289988 ) ) ;
#29296=CARTESIAN_POINT ( 'NONE',  ( -0.1450607720586916394, 0.000000000000000000, 0.3464511005275205946 ) ) ;
#29301=CARTESIAN_POINT ( 'NONE',  ( -0.4658792650918627265, -0.2845877964562161244, -0.3641732283464567121 ) ) ;
#29302=CARTESIAN_POINT ( 'NONE',  ( -1.141732283464566011, -0.5511811023622047445, 6.969142054262312111E-17 ) ) ;
#29303=CARTESIAN_POINT ( 'NONE',  ( -1.141732283464566011, 0.2952755905511811885, 0.000000000000000000 ) ) ;
#29304=CARTESIAN_POINT ( 'NONE',  ( 0.3871391076115492380, -0.05778040916215560624, -0.4822834645669293319 ) ) ;
#29305=CARTESIAN_POINT ( 'NONE',  ( -1.299212598425196097, 0.2952755905511811885, 0.000000000000000000 ) ) ;
#29308=CARTESIAN_POINT ( 'NONE',  ( -1.417322834645668772, -0.1870078740157480879, -0.4822834645669291653 ) ) ;
#29312=DIRECTION ( 'NONE',  ( -0.7119855458575274909, 0.7021941202331152265, 0.000000000000000000 ) ) ;
#29314=CARTESIAN_POINT ( 'NONE',  ( 0.4849061582275024929, 1.568468489416427580, -0.4921425059946356040 ) ) ;
#29315=CARTESIAN_POINT ( 'NONE',  ( -0.9251968503937002541, -0.5400638737290845981, -0.3530559997133363437 ) ) ;
#29316=CARTESIAN_POINT ( 'NONE',  ( 1.325459317585302665, -0.4281496062992124485, 0.4176697321401328655 ) ) ;
#29319=CARTESIAN_POINT ( 'NONE',  ( 1.509186351706037543, 0.05413385826771666132, 0.4176697321401328100 ) ) ;
#29320=CARTESIAN_POINT ( 'NONE',  ( -0.7939632545931754048, -0.3162353388693405765, 0.4822834645669290543 ) ) ;
#29322=CARTESIAN_POINT ( 'NONE',  ( 0.1246719160104994284, -0.5511811023622046335, 0.09757992244046803654 ) ) ;
#29324=CARTESIAN_POINT ( 'NONE',  ( -0.07217847769028787330, -0.08942795157527998196, 0.3641732283464567121 ) ) ;
#29325=CARTESIAN_POINT ( 'NONE',  ( 0.8333333333333340365, 0.1771653543307087075, -0.09757992244046823083 ) ) ;
#29326=CARTESIAN_POINT ( 'NONE',  ( 0.6233595800524939223, -0.3162353388693405765, 0.4822834645669290543 ) ) ;
#29327=CARTESIAN_POINT ( 'NONE',  ( -0.3871391076115476282, -0.08942795157527998196, 0.3641732283464567121 ) ) ;
#29329=CARTESIAN_POINT ( 'NONE',  ( -1.574803149606298192, -0.1870078740157480879, -0.4822834645669291653 ) ) ;
#29330=CARTESIAN_POINT ( 'NONE',  ( -1.456692913385826182, 0.1771653543307087630, 0.000000000000000000 ) ) ;
#29332=CARTESIAN_POINT ( 'NONE',  ( 0.05905511811023681640, 0.1660481256975883668, -0.3530559997133364547 ) ) ;
#29333=CARTESIAN_POINT ( 'NONE',  ( -0.5905511811023613777, -0.6692913385826771977, 8.415575281601705876E-17 ) ) ;
#29334=CARTESIAN_POINT ( 'NONE',  ( 1.594488188976378673, -0.4536011799217368745, -0.2665933059059886201 ) ) ;
#29335=CARTESIAN_POINT ( 'NONE',  ( 0.4461942257217855201, -0.5023911411419708095, 0.1820866141732285504 ) ) ;
#29336=CARTESIAN_POINT ( 'NONE',  ( -0.4133858267716528645, 0.1660481256975883668, -0.3530559997133364547 ) ) ;
#29337=CARTESIAN_POINT ( 'NONE',  ( -0.7808398950131222316, -0.3162353388693409650, -0.4822834645669289433 ) ) ;
#29338=DIRECTION ( 'NONE',  ( 0.7071067811865489050, 2.189697074797801291E-16, -0.7071067811865460184 ) ) ;
#29339=CARTESIAN_POINT ( 'NONE',  ( 1.535433070866142558, 0.1771653543307087630, 0.000000000000000000 ) ) ;
#29340=CARTESIAN_POINT ( 'NONE',  ( -0.05249343832020911260, 0.2306618581243848609, 0.2411417322834645549 ) ) ;
#29341=ORIENTED_EDGE ( 'NONE', *, *, #42486, .T. ) ;
#29344=CARTESIAN_POINT ( 'NONE',  ( -0.2165354330708654795, -0.4536011799217368745, -0.2665933059059886201 ) ) ;
#29346=CARTESIAN_POINT ( 'NONE',  ( -0.4658792650918627265, -0.05778040916215522460, 0.4822834645669289988 ) ) ;
#29347=CARTESIAN_POINT ( 'NONE',  ( -1.476377952755905110, 0.07958543189024085140, 0.2665933059059887866 ) ) ;
#29348=CARTESIAN_POINT ( 'NONE',  ( 1.213910761154856299, 0.2952755905511811885, 0.1292274648535926551 ) ) ;
#29349=CARTESIAN_POINT ( 'NONE',  ( -1.423884514435694859, -0.05778040916215560624, -0.4822834645669293319 ) ) ;
#29350=CARTESIAN_POINT ( 'NONE',  ( -0.4921259842519677963, -0.4536011799217367080, 0.2665933059059888421 ) ) ;
#29354=CARTESIAN_POINT ( 'NONE',  ( 1.666666666666667185, -0.004921259842519576551, 0.3153832671262227771 ) ) ;
#29355=CARTESIAN_POINT ( 'NONE',  ( 1.167979002624672580, -0.004921259842519870586, -0.3153832671262229437 ) ) ;
#29356=CARTESIAN_POINT ( 'NONE',  ( 1.003937007874016185, 0.1660481256975883668, -0.3530559997133364547 ) ) ;
#29358=CARTESIAN_POINT ( 'NONE',  ( 1.017060367454068581, -0.05778040916215560624, -0.4822834645669293319 ) ) ;
#29360=CARTESIAN_POINT ( 'NONE',  ( 1.430446194225722500, -0.3690944881889765550, -0.3153832671262227771 ) ) ;
#29361=CARTESIAN_POINT ( 'NONE',  ( 0.1574803149606306130, -0.1870078740157480879, -0.4822834645669291653 ) ) ;
#29362=CARTESIAN_POINT ( 'NONE',  ( -0.6758530183727028406, 0.2952755905511811885, 0.1292274648535926551 ) ) ;
#29366=CARTESIAN_POINT ( 'NONE',  ( 0.2690288713910767848, -0.5511811023622048555, -0.09757992244046775898 ) ) ;
#29370=CARTESIAN_POINT ( 'NONE',  ( -0.5905511811023615998, 0.2952755905511811885, 0.000000000000000000 ) ) ;
#29371=CARTESIAN_POINT ( 'NONE',  ( -0.3740157480314953431, 0.1660481256975885056, 0.3530559997133364547 ) ) ;
#29372=CARTESIAN_POINT ( 'NONE',  ( -0.2887139107611542133, -0.6046776061558809534, -0.2411417322834644161 ) ) ;
#29373=CARTESIAN_POINT ( 'NONE',  ( 0.7939632545931766261, -0.3162353388693409650, -0.4822834645669289433 ) ) ;
#29374=CARTESIAN_POINT ( 'NONE',  ( -0.8923884514435688198, -0.6046776061558807314, 0.2411417322834647770 ) ) ;
#29375=CARTESIAN_POINT ( 'NONE',  ( -0.3018372703412066094, 0.05413385826771666132, 0.4176697321401328100 ) ) ;
#29376=CARTESIAN_POINT ( 'NONE',  ( 1.305774278215223960, 0.2952755905511810774, -0.1292274648535930714 ) ) ;
#29377=CARTESIAN_POINT ( 'NONE',  ( 0.2887139107611556010, -0.6046776061558807314, 0.2411417322834647770 ) ) ;
#29378=CARTESIAN_POINT ( 'NONE',  ( 0.8727034120734913358, -0.05778040916215522460, 0.4822834645669289988 ) ) ;
#29379=EDGE_CURVE ( 'NONE', #57515, #1754, #8038, .T. ) ;
#29381=CARTESIAN_POINT ( 'NONE',  ( 0.2099737532808405305, -0.5023911411419708095, 0.1820866141732285504 ) ) ;
#29385=CARTESIAN_POINT ( 'NONE',  ( -0.7349081364829390672, 0.1283753931104746893, -0.1820866141732285504 ) ) ;
#29386=CARTESIAN_POINT ( 'NONE',  ( -0.4921259842519677963, 0.1660481256975883668, -0.3530559997133364547 ) ) ;
#29388=CARTESIAN_POINT ( 'NONE',  ( -0.5118110236220466680, -0.6692913385826771977, 8.415575281601705876E-17 ) ) ;
#29389=CARTESIAN_POINT ( 'NONE',  ( -0.2165354330708654795, -0.5400638737290845981, -0.3530559997133363437 ) ) ;
#29390=CARTESIAN_POINT ( 'NONE',  ( -1.128608923884513837, 0.2306618581243847221, -0.2411417322834647770 ) ) ;
#29391=CARTESIAN_POINT ( 'NONE',  ( -1.568241469816272105, -0.05778040916215522460, 0.4822834645669289988 ) ) ;
#29392=CARTESIAN_POINT ( 'NONE',  ( 0.9645669291338591078, -0.4536011799217368745, -0.2665933059059886201 ) ) ;
#29393=CARTESIAN_POINT ( 'NONE',  ( -0.7874015748031497619, 1.968503937007873850, 0.000000000000000000 ) ) ;
#29395=CARTESIAN_POINT ( 'NONE',  ( 0.5052493438320215802, 0.1771653543307087630, 0.09757992244046791164 ) ) ;
#29396=CARTESIAN_POINT ( 'NONE',  ( -0.1115485564304453947, -0.6692913385826771977, 0.1292274648535927661 ) ) ;
#29397=CARTESIAN_POINT ( 'NONE',  ( 0.01968503937007957949, -0.5400638737290845981, -0.3530559997133363437 ) ) ;
#29404=CARTESIAN_POINT ( 'NONE',  ( -0.7677165354330699465, 0.07958543189024085140, 0.2665933059059887866 ) ) ;
#29405=CARTESIAN_POINT ( 'NONE',  ( -0.9580052493438311334, -0.4281496062992124485, 0.4176697321401328655 ) ) ;
#29408=CARTESIAN_POINT ( 'NONE',  ( 1.633858267716535639, -0.5400638737290844871, 0.3530559997133364547 ) ) ;
#29409=CARTESIAN_POINT ( 'NONE',  ( 0.5314960629921264834, 0.1660481256975883668, -0.3530559997133364547 ) ) ;
#29410=CARTESIAN_POINT ( 'NONE',  ( 0.5380577427821529035, -0.4281496062992124485, 0.4176697321401328655 ) ) ;
#29411=CARTESIAN_POINT ( 'NONE',  ( -0.7611548556430438595, -0.5023911411419708095, -0.1820866141732282451 ) ) ;
#29412=CARTESIAN_POINT ( 'NONE',  ( 0.05249343832021075018, 0.2306618581243847221, -0.2411417322834647770 ) ) ;
#29414=CARTESIAN_POINT ( 'NONE',  ( -0.5183727034120726440, -0.6692913385826773087, -0.1292274648535924053 ) ) ;
#29416=CARTESIAN_POINT ( 'NONE',  ( 1.089238845144357537, -0.3690944881889763329, 0.3153832671262228327 ) ) ;
#29417=CARTESIAN_POINT ( 'NONE',  ( 0.01968503937007930540, 0.07958543189024085140, 0.2665933059059887866 ) ) ;
#29418=CARTESIAN_POINT ( 'NONE',  ( 1.115485564304462551, -0.3690944881889765550, -0.3153832671262227771 ) ) ;
#29419=CARTESIAN_POINT ( 'NONE',  ( -1.003937007874015297, -0.5400638737290845981, -0.3530559997133363437 ) ) ;
#29421=CARTESIAN_POINT ( 'NONE',  ( -1.312335958005248715, 0.1283753931104748280, 0.1820866141732283561 ) ) ;
#29422=CARTESIAN_POINT ( 'NONE',  ( -1.614173228346457378, 1.055049524192299693, 0.1372047244094476981 ) ) ;
#29423=CARTESIAN_POINT ( 'NONE',  ( -1.246719160104986512, 0.05413385826771666132, 0.4176697321401328100 ) ) ;
#29424=CARTESIAN_POINT ( 'NONE',  ( -0.6233595800524928121, -0.3162353388693409650, -0.4822834645669289433 ) ) ;
#29425=CARTESIAN_POINT ( 'NONE',  ( 0.1706036745406830368, -0.4281496062992127816, -0.4176697321401328100 ) ) ;
#29428=CARTESIAN_POINT ( 'NONE',  ( 0.4593175853018380828, -0.004921259842519870586, -0.3153832671262229437 ) ) ;
#29429=CARTESIAN_POINT ( 'NONE',  ( 0.9448818897637802916, -0.1870078740157479769, 0.4822834645669291653 ) ) ;
#29430=CARTESIAN_POINT ( 'NONE',  ( -1.456692913385826182, -0.5511811023622047445, 6.969142054262312111E-17 ) ) ;
#29431=CARTESIAN_POINT ( 'NONE',  ( 0.7808398950131241190, -0.05778040916215560624, -0.4822834645669293319 ) ) ;
#29432=CARTESIAN_POINT ( 'NONE',  ( -1.574803149606298636, -0.1870078740157479769, 0.3641732283464567677 ) ) ;
#29433=CARTESIAN_POINT ( 'NONE',  ( -1.410761154855642463, -0.05778040916215522460, 0.4822834645669289988 ) ) ;
#29434=CARTESIAN_POINT ( 'NONE',  ( -0.7414698162729651543, 0.2952755905511810774, -0.1292274648535930714 ) ) ;
#29435=CARTESIAN_POINT ( 'NONE',  ( -0.01968503937007793844, 0.07958543189024071263, -0.2665933059059888421 ) ) ;
#29436=CARTESIAN_POINT ( 'NONE',  ( 1.606354222338493454, 0.2948481568435550315, 0.02349281142910526754 ) ) ;
#29437=CARTESIAN_POINT ( 'NONE',  ( 0.8005249343832027131, -0.004921259842519576551, 0.3153832671262227771 ) ) ;
#29438=CARTESIAN_POINT ( 'NONE',  ( -0.1115485564304453947, -0.6692913385826771977, 0.1292274648535927661 ) ) ;
#29439=EDGE_CURVE ( 'NONE', #81026, #50981, #47744, .T. ) ;
#29441=CARTESIAN_POINT ( 'NONE',  ( -1.161417322834644716, -0.5400638737290845981, -0.3530559997133363437 ) ) ;
#29443=CARTESIAN_POINT ( 'NONE',  ( 0.9842519685039375910, 0.1771653543307087630, 0.000000000000000000 ) ) ;
#29444=CARTESIAN_POINT ( 'NONE',  ( 0.1574803149606306130, -0.1870078740157480879, -0.4822834645669291653 ) ) ;
#29445=CARTESIAN_POINT ( 'NONE',  ( -0.3543307086614165824, 0.2952755905511811885, 0.000000000000000000 ) ) ;
#29446=CARTESIAN_POINT ( 'NONE',  ( -0.5839895013123351797, -0.5511811023622046335, 0.09757992244046803654 ) ) ;
#29447=DIRECTION ( 'NONE',  ( 1.000000000000000000, 2.238352872228138170E-16, 0.000000000000000000 ) ) ;
#29448=CARTESIAN_POINT ( 'NONE',  ( -0.3937007874015740483, -0.1870078740157479769, 0.3641732283464567677 ) ) ;
#29449=CARTESIAN_POINT ( 'NONE',  ( 0.3215223097112867578, -0.3162353388693409650, -0.4822834645669289433 ) ) ;
#29451=CARTESIAN_POINT ( 'NONE',  ( -1.292650918635170010, -0.5511811023622046335, 0.09757992244046803654 ) ) ;
#29453=CARTESIAN_POINT ( 'NONE',  ( -1.614173228346455824, 0.2952755905511811885, 0.000000000000000000 ) ) ;
#29455=EDGE_LOOP ( 'NONE', ( #24297, #15531, #51625, #46973 ) ) ;
#29456=CARTESIAN_POINT ( 'NONE',  ( -1.469816272965878357, -0.5023911411419708095, -0.1820866141732282451 ) ) ;
#29457=CARTESIAN_POINT ( 'NONE',  ( -0.6496062992125976043, -0.5400638737290844871, 0.3530559997133364547 ) ) ;
#29458=CARTESIAN_POINT ( 'NONE',  ( -1.161417322834644716, 0.1660481256975885056, 0.3530559997133364547 ) ) ;
#29461=CARTESIAN_POINT ( 'NONE',  ( 1.469816272965879911, -0.6046776061558807314, 0.2411417322834647770 ) ) ;
#29462=CARTESIAN_POINT ( 'NONE',  ( 0.2624671916010504757, 0.2306618581243848609, 0.2411417322834645549 ) ) ;
#29463=CARTESIAN_POINT ( 'NONE',  ( -0.2755905511811018171, 0.2066929133858268208, 0.000000000000000000 ) ) ;
#29465=CARTESIAN_POINT ( 'NONE',  ( -1.535433070866141225, 0.2952755905511811885, 0.000000000000000000 ) ) ;
#29468=CARTESIAN_POINT ( 'NONE',  ( -0.8202099737532799750, 0.1771653543307087075, -0.09757992244046823083 ) ) ;
#29471=CARTESIAN_POINT ( 'NONE',  ( 0.9580052493438326877, 0.05413385826771666132, 0.4176697321401328100 ) ) ;
#29472=CARTESIAN_POINT ( 'NONE',  ( -0.5314960629921254842, -0.5400638737290845981, -0.3530559997133363437 ) ) ;
#29473=CARTESIAN_POINT ( 'NONE',  ( -1.312335958005248715, 0.2306618581243848609, 0.2411417322834645549 ) ) ;
#29474=CARTESIAN_POINT ( 'NONE',  ( 1.148293963254593875, -0.6692913385826771977, 0.1292274648535927661 ) ) ;
#29475=CARTESIAN_POINT ( 'NONE',  ( -1.246719160104985846, -0.3690944881889765550, -0.3153832671262227771 ) ) ;
#29476=CARTESIAN_POINT ( 'NONE',  ( 0.1837270341207357105, -0.6046776061558809534, -0.2411417322834644161 ) ) ;
#29477=CARTESIAN_POINT ( 'NONE',  ( -0.8595800524934373854, -0.05778040916215522460, 0.4822834645669289988 ) ) ;
#29479=CARTESIAN_POINT ( 'NONE',  ( -1.410761154855641575, -0.3162353388693409650, -0.4822834645669289433 ) ) ;
#29480=DIRECTION ( 'NONE',  ( 1.196716813021145407E-16, 0.7071067811865622277, 0.7071067811865328068 ) ) ;
#29481=CARTESIAN_POINT ( 'NONE',  ( 0.8923884514435703741, 0.2306618581243848609, 0.2411417322834645549 ) ) ;
#29483=CARTESIAN_POINT ( 'NONE',  ( 1.240157480314961314, 0.07958543189024071263, -0.2665933059059888421 ) ) ;
#29484=EDGE_LOOP ( 'NONE', ( #70803, #24315, #58137, #21710 ) ) ;
#29486=CARTESIAN_POINT ( 'NONE',  ( -0.5774278215223089816, -0.6046776061558807314, 0.2411417322834647770 ) ) ;
#29488=CARTESIAN_POINT ( 'NONE',  ( 0.4658792650918640033, -0.2845877964562159024, 0.3641732283464567677 ) ) ;
#29489=CARTESIAN_POINT ( 'NONE',  ( -1.509186351706035767, 0.05413385826771626580, -0.4176697321401330321 ) ) ;
#29490=CARTESIAN_POINT ( 'NONE',  ( 0.6692913385826777528, 0.2952755905511811885, 0.000000000000000000 ) ) ;
#29491=CARTESIAN_POINT ( 'NONE',  ( 0.7939632545931766261, -0.05778040916215522460, 0.4822834645669289988 ) ) ;
#29492=CARTESIAN_POINT ( 'NONE',  ( -0.09186351706036689768, 0.05413385826771626580, -0.4176697321401330321 ) ) ;
#29494=CARTESIAN_POINT ( 'NONE',  ( -0.6824146981627288167, 0.2306618581243848609, 0.2411417322834645549 ) ) ;
#29496=CARTESIAN_POINT ( 'NONE',  ( 1.594488188976378673, 0.07958543189024085140, 0.2665933059059887866 ) ) ;
#29497=CARTESIAN_POINT ( 'NONE',  ( -0.9448818897637790704, -0.1870078740157480879, -0.4822834645669291653 ) ) ;
#29498=CARTESIAN_POINT ( 'NONE',  ( 1.102362204724410155, -0.1870078740157480879, -0.4822834645669291653 ) ) ;
#29499=CARTESIAN_POINT ( 'NONE',  ( 1.194225721784777594, 0.05413385826771666132, 0.4176697321401328100 ) ) ;
#29501=CARTESIAN_POINT ( 'NONE',  ( -1.102362204724408601, -0.1870078740157479769, 0.4822834645669291653 ) ) ;
#29503=CARTESIAN_POINT ( 'NONE',  ( 0.4330708661417329575, -0.6692913385826771977, 8.415575281601705876E-17 ) ) ;
#29505=CARTESIAN_POINT ( 'NONE',  ( -0.3608923884514428360, 0.2952755905511811885, 0.1292274648535926551 ) ) ;
#29506=CARTESIAN_POINT ( 'NONE',  ( -1.496062992125983815, -0.1870078740157479769, 0.3641732283464567677 ) ) ;
#29507=CARTESIAN_POINT ( 'NONE',  ( 0.6496062992125991586, -0.4536011799217368745, -0.2665933059059886201 ) ) ;
#29508=CARTESIAN_POINT ( 'NONE',  ( 1.397637795275591177, -0.5400638737290844871, 0.3530559997133364547 ) ) ;
#29510=CARTESIAN_POINT ( 'NONE',  ( 0.5839895013123367340, 0.1771653543307087630, 0.09757992244046791164 ) ) ;
#29511=CARTESIAN_POINT ( 'NONE',  ( 0.9711286089238851948, 0.2306618581243848609, 0.2411417322834645549 ) ) ;
#29513=CARTESIAN_POINT ( 'NONE',  ( -0.1837270341207343505, -0.6046776061558807314, 0.2411417322834647770 ) ) ;
#29515=CARTESIAN_POINT ( 'NONE',  ( 1.286089238845145033, 0.1283753931104748280, 0.1820866141732283561 ) ) ;
#29516=CARTESIAN_POINT ( 'NONE',  ( -0.7677165354330699465, 0.1660481256975885056, 0.3530559997133364547 ) ) ;
#29517=CARTESIAN_POINT ( 'NONE',  ( 0.07217847769028949700, -0.05778040916215560624, -0.4822834645669293319 ) ) ;
#29519=CARTESIAN_POINT ( 'NONE',  ( -0.05905511811023545637, -0.5400638737290845981, -0.3530559997133363437 ) ) ;
#29520=CARTESIAN_POINT ( 'NONE',  ( 0.7414698162729663755, 0.1771653543307087630, 0.09757992244046791164 ) ) ;
#29522=CARTESIAN_POINT ( 'NONE',  ( -0.1443569553805765515, -0.3690944881889765550, -0.3153832671262227771 ) ) ;
#29523=CARTESIAN_POINT ( 'NONE',  ( 0.6692913385826777528, 0.1771653543307087630, 0.000000000000000000 ) ) ;
#29526=CARTESIAN_POINT ( 'NONE',  ( 0.1443569553805781891, 0.05413385826771626580, -0.4176697321401330321 ) ) ;
#29528=CARTESIAN_POINT ( 'NONE',  ( 1.515748031496063408, 0.07958543189024085140, 0.2665933059059887866 ) ) ;
#29530=CARTESIAN_POINT ( 'NONE',  ( 0.1246719160104994284, -0.5511811023622046335, 0.09757992244046803654 ) ) ;
#29531=CARTESIAN_POINT ( 'NONE',  ( 0.1574803149606306130, -0.1870078740157480879, -0.4822834645669291653 ) ) ;
#29532=CARTESIAN_POINT ( 'NONE',  ( 1.391076115485564868, 0.1283753931104746893, -0.1820866141732285504 ) ) ;
#29533=CARTESIAN_POINT ( 'NONE',  ( -1.266404199475064773, -0.2845877964562159024, 0.3641732283464567677 ) ) ;
#29534=CARTESIAN_POINT ( 'NONE',  ( -1.463254593175852492, -0.6692913385826773087, -0.1292274648535924053 ) ) ;
#29535=CARTESIAN_POINT ( 'NONE',  ( 0.1837270341207357105, -0.6046776061558809534, -0.2411417322834644161 ) ) ;
#29536=CARTESIAN_POINT ( 'NONE',  ( 1.122047244094488860, -0.5400638737290845981, -0.3530559997133363437 ) ) ;
#29538=CARTESIAN_POINT ( 'NONE',  ( 0.1902887139107617975, 0.2952755905511811885, 0.1292274648535926551 ) ) ;
#29539=CARTESIAN_POINT ( 'NONE',  ( 1.148293963254593875, -0.6692913385826771977, 0.1292274648535927661 ) ) ;
#29540=CARTESIAN_POINT ( 'NONE',  ( 0.8792650918635177559, 0.05413385826771666132, 0.4176697321401328100 ) ) ;
#29541=EDGE_CURVE ( 'NONE', #24707, #30109, #33057, .T. ) ;
#29543=CARTESIAN_POINT ( 'NONE',  ( 0.7349081364829403995, 0.1283753931104748280, 0.1820866141732283561 ) ) ;
#29544=CARTESIAN_POINT ( 'NONE',  ( -1.627296587926508442, 0.1283753931104748280, 0.1820866141732283561 ) ) ;
#29545=CARTESIAN_POINT ( 'NONE',  ( 0.1771653543307093182, 0.07958543189024085140, 0.2665933059059887866 ) ) ;
#29546=CARTESIAN_POINT ( 'NONE',  ( 0.1049868766404206816, 0.2306618581243848609, 0.2411417322834645549 ) ) ;
#29547=CARTESIAN_POINT ( 'NONE',  ( 0.5643044619422579178, -0.4281496062992127816, -0.4176697321401328100 ) ) ;
#29548=CARTESIAN_POINT ( 'NONE',  ( -0.5314960629921250401, 0.1660481256975885056, 0.3530559997133364547 ) ) ;
#29550=CARTESIAN_POINT ( 'NONE',  ( -0.09842519685039295696, 0.07958543189024071263, -0.2665933059059888421 ) ) ;
#29551=CARTESIAN_POINT ( 'NONE',  ( 0.9186351706036751663, -0.6046776061558807314, 0.2411417322834647770 ) ) ;
#29552=CARTESIAN_POINT ( 'NONE',  ( 1.062992125984252745, 0.1771653543307087630, 0.000000000000000000 ) ) ;
#29553=LINE ( 'NONE', #22005, #46013 ) ;
#29555=CARTESIAN_POINT ( 'NONE',  ( -0.7874015748031492068, 2.204724409448818978, 0.000000000000000000 ) ) ;
#29557=CARTESIAN_POINT ( 'NONE',  ( -1.364829396325458521, -0.6046776061558807314, 0.2411417322834647770 ) ) ;
#29558=CARTESIAN_POINT ( 'NONE',  ( -0.5052493438320203589, -0.6692913385826771977, 0.1292274648535927661 ) ) ;
#29559=EDGE_CURVE ( 'NONE', #8463, #24368, #76671, .T. ) ;
#29563=CARTESIAN_POINT ( 'NONE',  ( 0.3608923884514443348, -0.5511811023622046335, 0.09757992244046803654 ) ) ;
#29565=CARTESIAN_POINT ( 'NONE',  ( 1.194225721784777594, -0.4281496062992127816, -0.4176697321401328100 ) ) ;
#29569=CARTESIAN_POINT ( 'NONE',  ( -1.725721784776902190, -0.08942795157527998196, 0.3641732283464567121 ) ) ;
#29570=FACE_OUTER_BOUND ( 'NONE', #7551, .T. ) ;
#29571=CARTESIAN_POINT ( 'NONE',  ( 1.371391076115485719, -0.5511811023622048555, -0.09757992244046775898 ) ) ;
#29572=CARTESIAN_POINT ( 'NONE',  ( 0.2296587926509192634, -0.3162353388693405765, 0.4822834645669290543 ) ) ;
#29574=CARTESIAN_POINT ( 'NONE',  ( 0.09842519685039434474, 0.1660481256975885056, 0.3530559997133364547 ) ) ;
#29575=CARTESIAN_POINT ( 'NONE',  ( -0.9711286089238838626, -0.5023911411419708095, 0.1820866141732285504 ) ) ;
#29576=CARTESIAN_POINT ( 'NONE',  ( 0.5971128608923890191, -0.6692913385826771977, 0.1292274648535927661 ) ) ;
#29577=CARTESIAN_POINT ( 'NONE',  ( -0.07217847769028813698, -0.3162353388693409650, -0.4822834645669289433 ) ) ;
#29581=CARTESIAN_POINT ( 'NONE',  ( 0.9776902887139113929, -0.6692913385826773087, -0.1292274648535924053 ) ) ;
#29582=CARTESIAN_POINT ( 'NONE',  ( -0.2034120734908131112, -0.6692913385826773087, -0.1292274648535924053 ) ) ;
#29583=CARTESIAN_POINT ( 'NONE',  ( -0.9908136482939626788, 0.2952755905511811885, 0.1292274648535926551 ) ) ;
#29584=CARTESIAN_POINT ( 'NONE',  ( 1.030183727034121421, -0.3162353388693409650, -0.4822834645669289433 ) ) ;
#29585=CARTESIAN_POINT ( 'NONE',  ( 0.5380577427821529035, -0.4281496062992124485, 0.4176697321401328655 ) ) ;
#29587=CARTESIAN_POINT ( 'NONE',  ( -0.4658792650918627265, -0.05778040916215522460, 0.4822834645669289988 ) ) ;
#29588=CARTESIAN_POINT ( 'NONE',  ( 0.2559055118110243332, 0.1660481256975885056, 0.3530559997133364547 ) ) ;
#29589=CARTESIAN_POINT ( 'NONE',  ( -0.4921259842519677963, 0.1660481256975883668, -0.3530559997133364547 ) ) ;
#29590=CARTESIAN_POINT ( 'NONE',  ( 0.1706036745406830368, -0.3690944881889765550, -0.3153832671262227771 ) ) ;
#29591=CARTESIAN_POINT ( 'NONE',  ( 1.673228346456693494, 0.07958543189024085140, 0.2665933059059887866 ) ) ;
#29593=CARTESIAN_POINT ( 'NONE',  ( 0.5118110236220478892, 0.2952755905511811885, 0.000000000000000000 ) ) ;
#29596=CARTESIAN_POINT ( 'NONE',  ( 1.364829396325459854, -0.6046776061558809534, -0.2411417322834644161 ) ) ;
#29600=CARTESIAN_POINT ( 'NONE',  ( 0.7217847769028878924, 0.05413385826771666132, 0.4176697321401328100 ) ) ;
#29601=CARTESIAN_POINT ( 'NONE',  ( 0.4199475065616803948, -0.5023911411419708095, -0.1820866141732282451 ) ) ;
#29605=DIRECTION ( 'NONE',  ( 1.000000000000000000, 3.096699300667737957E-16, 0.000000000000000000 ) ) ;
#29609=CARTESIAN_POINT ( 'NONE',  ( 0.7939632545931766261, -0.05778040916215522460, 0.4822834645669289988 ) ) ;
#29610=CARTESIAN_POINT ( 'NONE',  ( -0.7611548556430438595, -0.6046776061558809534, -0.2411417322834644161 ) ) ;
#29611=CARTESIAN_POINT ( 'NONE',  ( -0.7283464566929126471, 0.1660481256975883668, -0.3530559997133364547 ) ) ;
#29612=CARTESIAN_POINT ( 'NONE',  ( 0.5643044619422579178, -0.4281496062992127816, -0.4176697321401328100 ) ) ;
#29613=CARTESIAN_POINT ( 'NONE',  ( 1.509186351706037543, -0.4281496062992127816, -0.4176697321401328100 ) ) ;
#29614=DIRECTION ( 'NONE',  ( 0.000000000000000000, 0.000000000000000000, -1.000000000000000000 ) ) ;
#29616=CARTESIAN_POINT ( 'NONE',  ( 1.233595800524935227, 0.1283753931104746893, -0.1820866141732285504 ) ) ;
#29617=CARTESIAN_POINT ( 'NONE',  ( 2.787279214012418738, 1.496062992125984481, 0.000000000000000000 ) ) ;
#29618=CARTESIAN_POINT ( 'NONE',  ( -1.417322834645668772, -0.1870078740157480601, -0.3641732283464567677 ) ) ;
#29621=CARTESIAN_POINT ( 'NONE',  ( 0.2427821522309719648, -0.05778040916215522460, 0.4822834645669289988 ) ) ;
#29622=CARTESIAN_POINT ( 'NONE',  ( 1.122047244094488860, -0.5400638737290845981, -0.3530559997133363437 ) ) ;
#29623=CARTESIAN_POINT ( 'NONE',  ( 0.4849061582275024929, 1.805669738366188382, -0.4921425059946357150 ) ) ;
#29624=CARTESIAN_POINT ( 'NONE',  ( -1.233595800524933894, 0.1283753931104748280, 0.1820866141732283561 ) ) ;
#29625=CARTESIAN_POINT ( 'NONE',  ( 0.5314960629921267055, -0.5400638737290844871, 0.3530559997133364547 ) ) ;
#29626=CARTESIAN_POINT ( 'NONE',  ( 1.404199475065617264, -0.3690944881889763329, 0.3153832671262228327 ) ) ;
#29628=CARTESIAN_POINT ( 'NONE',  ( -1.364829396325458521, 0.1283753931104746893, -0.1820866141732285504 ) ) ;
#29629=CARTESIAN_POINT ( 'NONE',  ( 1.456692913385827515, -0.6692913385826771977, 8.415575281601705876E-17 ) ) ;
#29631=CARTESIAN_POINT ( 'NONE',  ( -0.2887139107611542133, 0.1283753931104748280, 0.1820866141732283561 ) ) ;
#29632=CARTESIAN_POINT ( 'NONE',  ( -0.3871391076115479057, -0.3162353388693409650, -0.4822834645669289433 ) ) ;
#29633=CARTESIAN_POINT ( 'NONE',  ( -1.240157480314959759, -0.4536011799217368745, -0.2665933059059886201 ) ) ;
#29634=CARTESIAN_POINT ( 'NONE',  ( -0.7874015748031489847, -0.1870078740157479769, 0.4822834645669291653 ) ) ;
#29635=VECTOR ( 'NONE', #8634, 39.37007874015748143 ) ;
#29636=CARTESIAN_POINT ( 'NONE',  ( 1.174540682414699111, -0.3162353388693405765, 0.4822834645669290543 ) ) ;
#29639=CARTESIAN_POINT ( 'NONE',  ( 1.522309711286089939, -0.6046776061558809534, -0.2411417322834644161 ) ) ;
#29641=CARTESIAN_POINT ( 'NONE',  ( -1.410761154855642463, -0.05778040916215522460, 0.4822834645669289988 ) ) ;
#29642=CARTESIAN_POINT ( 'NONE',  ( -0.9580052493438311334, -0.004921259842519870586, -0.3153832671262229437 ) ) ;
#29643=CARTESIAN_POINT ( 'NONE',  ( -0.7939632545931754048, -0.2845877964562159024, 0.3641732283464567677 ) ) ;
#29644=CARTESIAN_POINT ( 'NONE',  ( 1.586052503253845281, 1.023622047244095556, -0.1653254495020587966 ) ) ;
#29645=CARTESIAN_POINT ( 'NONE',  ( 0.1181102362204730916, 0.2952755905511811885, 0.000000000000000000 ) ) ;
#29646=CARTESIAN_POINT ( 'NONE',  ( -0.1837270341207340729, 0.1283753931104746893, -0.1820866141732285504 ) ) ;
#29647=CARTESIAN_POINT ( 'NONE',  ( -1.030183727034119867, -0.08942795157528024563, -0.3641732283464568787 ) ) ;
#29648=CARTESIAN_POINT ( 'NONE',  ( -1.555118110236219930, 0.1660481256975885056, 0.3530559997133364547 ) ) ;
#29649=CARTESIAN_POINT ( 'NONE',  ( 1.187664041994751285, -0.2845877964562161244, -0.3641732283464567121 ) ) ;
#29650=CARTESIAN_POINT ( 'NONE',  ( 1.397637795275591177, 0.1660481256975883668, -0.3530559997133364547 ) ) ;
#29652=CARTESIAN_POINT ( 'NONE',  ( 0.3477690288713918276, -0.5511811023622048555, -0.09757992244046775898 ) ) ;
#29653=CARTESIAN_POINT ( 'NONE',  ( 0.8792650918635177559, 0.05413385826771666132, 0.4176697321401328100 ) ) ;
#29655=CARTESIAN_POINT ( 'NONE',  ( 1.062992125984252745, -0.5511811023622047445, 6.969142054262312111E-17 ) ) ;
#29657=CARTESIAN_POINT ( 'NONE',  ( -1.200787401574802349, -0.5400638737290844871, 0.3530559997133364547 ) ) ;
#29658=CARTESIAN_POINT ( 'NONE',  ( -0.9973753280839886548, 0.2306618581243848609, 0.2411417322834645549 ) ) ;
#29659=CARTESIAN_POINT ( 'NONE',  ( 0.02624671916010564918, 0.2306618581243848609, 0.2411417322834645549 ) ) ;
#29662=CARTESIAN_POINT ( 'NONE',  ( 0.8858267716535438430, -0.5400638737290845981, -0.3530559997133363437 ) ) ;
#29663=CARTESIAN_POINT ( 'NONE',  ( 1.489501312335958172, -0.08942795157528024563, -0.3641732283464568787 ) ) ;
#29664=CARTESIAN_POINT ( 'NONE',  ( 0.1706036745406830368, -0.4281496062992127816, -0.4176697321401328100 ) ) ;
#29665=CARTESIAN_POINT ( 'NONE',  ( 0.6955380577427828781, 0.05413385826771626580, -0.4176697321401330321 ) ) ;
#29671=CARTESIAN_POINT ( 'NONE',  ( 0.09186351706036799403, -0.3690944881889765550, -0.3153832671262227771 ) ) ;
#29672=CARTESIAN_POINT ( 'NONE',  ( -0.7086614173228339419, -0.1870078740157480879, -0.4822834645669291653 ) ) ;
#29673=CARTESIAN_POINT ( 'NONE',  ( 0.9645669291338588858, 0.1660481256975885056, 0.3530559997133364547 ) ) ;
#29675=CARTESIAN_POINT ( 'NONE',  ( -0.4921259842519677963, 0.07958543189024071263, -0.2665933059059888421 ) ) ;
#29676=CARTESIAN_POINT ( 'NONE',  ( -1.535433070866141225, -0.6692913385826771977, 8.415575281601705876E-17 ) ) ;
#29677=CARTESIAN_POINT ( 'NONE',  ( 1.174540682414699111, -0.05778040916215560624, -0.4822834645669293319 ) ) ;
#29680=CARTESIAN_POINT ( 'NONE',  ( 1.112371124080195450, -4.927456884911482678E-16, 0.4445507791589062840 ) ) ;
#29682=CARTESIAN_POINT ( 'NONE',  ( 0.9383202099737536495, -0.3162353388693405765, 0.4822834645669290543 ) ) ;
#29683=CARTESIAN_POINT ( 'NONE',  ( 1.397637795275591177, -0.4536011799217367080, 0.2665933059059888421 ) ) ;
#29684=CARTESIAN_POINT ( 'NONE',  ( 1.633858267716535639, -0.5400638737290844871, 0.3530559997133364547 ) ) ;
#29685=CARTESIAN_POINT ( 'NONE',  ( -1.522309711286088607, -0.6046776061558807314, 0.2411417322834647770 ) ) ;
#29688=CARTESIAN_POINT ( 'NONE',  ( 0.8398950131233602345, -0.6046776061558807314, 0.2411417322834647770 ) ) ;
#29689=CARTESIAN_POINT ( 'NONE',  ( -1.594488188976377563, -0.5400638737290844871, 0.3530559997133364547 ) ) ;
#29690=CARTESIAN_POINT ( 'NONE',  ( -0.6496062992125976043, -0.5400638737290844871, 0.3530559997133364547 ) ) ;
#29691=CARTESIAN_POINT ( 'NONE',  ( -0.3871391076115479057, -0.3162353388693409650, -0.4822834645669289433 ) ) ;
#29693=CARTESIAN_POINT ( 'NONE',  ( -1.522309711286088607, -0.6046776061558807314, 0.2411417322834647770 ) ) ;
#29695=CARTESIAN_POINT ( 'NONE',  ( 0.2165354330708668673, 0.1660481256975883668, -0.3530559997133364547 ) ) ;
#29697=CARTESIAN_POINT ( 'NONE',  ( -1.627296587926508442, 0.1283753931104748280, 0.1820866141732283561 ) ) ;
#29700=EDGE_LOOP ( 'NONE', ( #62264, #12881, #10255, #80015 ) ) ;
#29701=CARTESIAN_POINT ( 'NONE',  ( -0.7426113562972006532, 2.209901789876323797, -0.5309055118110235227 ) ) ;
#29702=CARTESIAN_POINT ( 'NONE',  ( -1.364829396325458521, 0.2306618581243847221, -0.2411417322834647770 ) ) ;
#29704=CARTESIAN_POINT ( 'NONE',  ( 1.594488188976378673, -0.4536011799217368745, -0.2665933059059886201 ) ) ;
#29705=CARTESIAN_POINT ( 'NONE',  ( -0.1181102362204717315, 0.2066929133858268208, 0.000000000000000000 ) ) ;
#29707=CARTESIAN_POINT ( 'NONE',  ( -0.3674540682414689785, 0.2306618581243848609, 0.2411417322834645549 ) ) ;
#29709=CARTESIAN_POINT ( 'NONE',  ( -0.2296587926509179312, -0.08942795157527998196, 0.3641732283464567121 ) ) ;
#29710=CARTESIAN_POINT ( 'NONE',  ( -1.253280839895012377, -0.08942795157527998196, 0.3641732283464567121 ) ) ;
#29711=CARTESIAN_POINT ( 'NONE',  ( -1.607611548556429737, 0.2952755905511810774, -0.1292274648535930714 ) ) ;
#29712=CARTESIAN_POINT ( 'NONE',  ( 0.5183727034120741983, 0.2952755905511810774, -0.1292274648535930714 ) ) ;
#29713=CARTESIAN_POINT ( 'NONE',  ( -1.377952755905511140, -0.6692913385826771977, 8.415575281601705876E-17 ) ) ;
#29716=ORIENTED_EDGE ( 'NONE', *, *, #69619, .T. ) ;
#29717=CARTESIAN_POINT ( 'NONE',  ( 1.430446194225722500, 0.05413385826771666132, 0.4176697321401328100 ) ) ;
#29718=DIRECTION ( 'NONE',  ( -1.000000000000000000, -3.083952846180990774E-16, 0.000000000000000000 ) ) ;
#29722=CARTESIAN_POINT ( 'NONE',  ( -0.8989501312335946848, -0.6692913385826771977, 0.1292274648535927661 ) ) ;
#29723=CARTESIAN_POINT ( 'NONE',  ( 1.299212598425197429, -0.6692913385826771977, 8.415575281601705876E-17 ) ) ;
#29726=CARTESIAN_POINT ( 'NONE',  ( -1.653543307086613234, -0.1870078740157480879, -0.4822834645669291653 ) ) ;
#29727=CARTESIAN_POINT ( 'NONE',  ( -0.8070866141732276899, -0.5400638737290844871, 0.3530559997133364547 ) ) ;
#29729=CARTESIAN_POINT ( 'NONE',  ( 0.2230971128608929543, -0.004921259842519870586, -0.3153832671262229437 ) ) ;
#29731=CARTESIAN_POINT ( 'NONE',  ( 0.1049868766404206816, 0.1283753931104748280, 0.1820866141732283561 ) ) ;
#29732=CARTESIAN_POINT ( 'NONE',  ( 0.5905511811023629321, -0.5511811023622047445, 6.969142054262312111E-17 ) ) ;
#29733=CARTESIAN_POINT ( 'NONE',  ( 0.3543307086614179147, 0.2952755905511811885, 0.000000000000000000 ) ) ;
#29734=CARTESIAN_POINT ( 'NONE',  ( -0.4199475065616791736, -0.5023911411419708095, 0.1820866141732285504 ) ) ;
#29736=CARTESIAN_POINT ( 'NONE',  ( 1.528871391076116026, -0.6692913385826773087, -0.1292274648535924053 ) ) ;
#29737=CARTESIAN_POINT ( 'NONE',  ( -0.8923884514435688198, -0.6046776061558807314, 0.2411417322834647770 ) ) ;
#29739=CARTESIAN_POINT ( 'NONE',  ( -0.07217847769028813698, -0.3162353388693409650, -0.4822834645669289433 ) ) ;
#29740=CARTESIAN_POINT ( 'NONE',  ( -0.4724409448818890911, -0.1870078740157480879, -0.4822834645669291653 ) ) ;
#29741=CARTESIAN_POINT ( 'NONE',  ( 1.528871391076116026, 0.1771653543307087630, 0.09757992244046791164 ) ) ;
#29742=CARTESIAN_POINT ( 'NONE',  ( 0.03937007874015806264, 0.1771653543307087630, 0.000000000000000000 ) ) ;
#29743=CARTESIAN_POINT ( 'NONE',  ( -0.2624671916010490880, 0.2306618581243847221, -0.2411417322834647770 ) ) ;
#29744=CARTESIAN_POINT ( 'NONE',  ( -0.5774278215223089816, -0.6046776061558807314, 0.2411417322834647770 ) ) ;
#29747=CARTESIAN_POINT ( 'NONE',  ( 0.3477690288713918276, -0.6692913385826773087, -0.1292274648535924053 ) ) ;
#29751=CARTESIAN_POINT ( 'NONE',  ( 1.587926509186352142, 0.05413385826771666132, 0.4176697321401328100 ) ) ;
#29752=CARTESIAN_POINT ( 'NONE',  ( -0.8202099737532801971, -0.5511811023622046335, 0.09757992244046803654 ) ) ;
#29753=CARTESIAN_POINT ( 'NONE',  ( -0.7414698162729651543, 0.2952755905511810774, -0.1292274648535930714 ) ) ;
#29754=CARTESIAN_POINT ( 'NONE',  ( 1.240157480314961314, 0.1660481256975883668, -0.3530559997133364547 ) ) ;
#29755=CARTESIAN_POINT ( 'NONE',  ( 1.364829396325460076, 0.2306618581243848609, 0.2411417322834645549 ) ) ;
#29756=CARTESIAN_POINT ( 'NONE',  ( -1.430446194225720724, 0.05413385826771626580, -0.4176697321401330321 ) ) ;
#29757=CARTESIAN_POINT ( 'NONE',  ( -1.023622047244094002, -0.1870078740157480601, -0.3641732283464567677 ) ) ;
#29759=ADVANCED_FACE ( 'NONE', ( #35545 ), #55298, .F. ) ;
#29762=CARTESIAN_POINT ( 'NONE',  ( 1.535433070866142558, 0.1771653543307087630, 0.000000000000000000 ) ) ;
#29763=CARTESIAN_POINT ( 'NONE',  ( 1.056430446194226436, -0.5511811023622048555, -0.09757992244046775898 ) ) ;
#29764=CARTESIAN_POINT ( 'NONE',  ( 0.7152230971128614723, -0.3162353388693409650, -0.4822834645669289433 ) ) ;
#29765=CARTESIAN_POINT ( 'NONE',  ( -1.699475065616797398, 0.2952755905511811885, 0.1292274648535926551 ) ) ;
#29766=CARTESIAN_POINT ( 'NONE',  ( 0.9908136482939640111, 0.2952755905511810774, -0.1292274648535930714 ) ) ;
#29768=CARTESIAN_POINT ( 'NONE',  ( 1.305774278215223960, -0.5511811023622046335, 0.09757992244046803654 ) ) ;
#29769=CARTESIAN_POINT ( 'NONE',  ( 0.07874015748031558404, -0.1870078740157479769, 0.4822834645669291653 ) ) ;
#29770=CARTESIAN_POINT ( 'NONE',  ( -0.9908136482939626788, 0.2952755905511811885, 0.1292274648535926551 ) ) ;
#29771=CARTESIAN_POINT ( 'NONE',  ( 1.174540682414699111, -0.3162353388693405765, 0.4822834645669290543 ) ) ;
#29774=CARTESIAN_POINT ( 'NONE',  ( 0.4133858267716541968, -0.4536011799217368745, -0.2665933059059886201 ) ) ;
#29775=VERTEX_POINT ( 'NONE', #80418 ) ;
#29777=EDGE_LOOP ( 'NONE', ( #3410, #2554, #49127 ) ) ;
#29778=CARTESIAN_POINT ( 'NONE',  ( -0.9383202099737524282, -0.05778040916215522460, 0.4822834645669289988 ) ) ;
#29779=CARTESIAN_POINT ( 'NONE',  ( -0.1968503937007867743, 0.2952755905511811885, 0.000000000000000000 ) ) ;
#29780=CARTESIAN_POINT ( 'NONE',  ( -0.1771653543307080136, 0.1660481256975883668, -0.3530559997133364547 ) ) ;
#29781=CARTESIAN_POINT ( 'NONE',  ( 0.8989501312335964611, 0.2952755905511811885, 0.1292274648535926551 ) ) ;
#29782=CARTESIAN_POINT ( 'NONE',  ( -1.207349081364828436, -0.6046776061558807314, 0.2411417322834647770 ) ) ;
#29783=CARTESIAN_POINT ( 'NONE',  ( -0.3083989501312330295, -0.05778040916215522460, 0.4822834645669289988 ) ) ;
#29784=CARTESIAN_POINT ( 'NONE',  ( 0.6299212598425204535, -0.1870078740157479769, 0.4822834645669291653 ) ) ;
#29785=CARTESIAN_POINT ( 'NONE',  ( 0.2755905511811031494, -0.6692913385826771977, 8.415575281601705876E-17 ) ) ;
#29788=CARTESIAN_POINT ( 'NONE',  ( -0.3740157480314953431, 0.07958543189024085140, 0.2665933059059887866 ) ) ;
#29791=VERTEX_POINT ( 'NONE', #58429 ) ;
#29792=CARTESIAN_POINT ( 'NONE',  ( -1.181102362204723644, -0.1870078740157480601, -0.3641732283464567677 ) ) ;
#29793=CARTESIAN_POINT ( 'NONE',  ( -0.5839895013123351797, -0.6692913385826771977, 0.1292274648535927661 ) ) ;
#29795=CARTESIAN_POINT ( 'NONE',  ( -0.8792650918635160906, 0.05413385826771626580, -0.4176697321401330321 ) ) ;
#29796=CARTESIAN_POINT ( 'NONE',  ( -0.6430446194225716283, -0.4281496062992124485, 0.4176697321401328655 ) ) ;
#29797=CARTESIAN_POINT ( 'NONE',  ( -1.430446194225720724, 0.05413385826771626580, -0.4176697321401330321 ) ) ;
#29798=CARTESIAN_POINT ( 'NONE',  ( -1.535433070866141225, 0.2952755905511811885, 0.000000000000000000 ) ) ;
#29799=CARTESIAN_POINT ( 'NONE',  ( 0.8333333333333340365, -0.5511811023622046335, 0.09757992244046803654 ) ) ;
#29802=CARTESIAN_POINT ( 'NONE',  ( 0.2624671916010504757, -0.5023911411419708095, -0.1820866141732282451 ) ) ;
#29803=CARTESIAN_POINT ( 'NONE',  ( -0.2952755905511803003, -0.5400638737290845981, -0.3530559997133363437 ) ) ;
#29804=CARTESIAN_POINT ( 'NONE',  ( -0.2624671916010490880, -0.6046776061558807314, 0.2411417322834647770 ) ) ;
#29811=CARTESIAN_POINT ( 'NONE',  ( -0.5249343832020990641, -0.5023911411419708095, -0.1820866141732282451 ) ) ;
#29812=CARTESIAN_POINT ( 'NONE',  ( -1.043307086614172707, 0.1660481256975883668, -0.3530559997133364547 ) ) ;
#29816=CARTESIAN_POINT ( 'NONE',  ( 1.345144356955381593, -0.05778040916215522460, 0.4822834645669289988 ) ) ;
#29817=CARTESIAN_POINT ( 'NONE',  ( 0.4265091863517067039, -0.6692913385826773087, -0.1292274648535924053 ) ) ;
#29818=CARTESIAN_POINT ( 'NONE',  ( 0.4330708661417329575, 0.2952755905511811885, 0.000000000000000000 ) ) ;
#29819=CARTESIAN_POINT ( 'NONE',  ( -0.5052493438320203589, 0.1771653543307087075, -0.09757992244046823083 ) ) ;
#29820=CARTESIAN_POINT ( 'NONE',  ( -0.4330708661417315697, 0.2952755905511811885, 0.000000000000000000 ) ) ;
#29822=CARTESIAN_POINT ( 'NONE',  ( -0.4724409448818890911, -0.1870078740157479769, 0.4822834645669291653 ) ) ;
#29824=CARTESIAN_POINT ( 'NONE',  ( 1.338582677165355062, -0.1870078740157480601, -0.3641732283464567677 ) ) ;
#29825=CARTESIAN_POINT ( 'NONE',  ( -0.3149606299212590610, -0.1870078740157479769, 0.3641732283464567677 ) ) ;
#29826=CARTESIAN_POINT ( 'NONE',  ( 1.246719160104987623, -0.004921259842519870586, -0.3153832671262229437 ) ) ;
#29827=CARTESIAN_POINT ( 'NONE',  ( -1.141732283464566011, -0.6692913385826771977, 8.415575281601705876E-17 ) ) ;
#29828=CARTESIAN_POINT ( 'NONE',  ( -0.9580052493438311334, -0.004921259842519870586, -0.3153832671262229437 ) ) ;
#29830=CARTESIAN_POINT ( 'NONE',  ( -1.207349081364828880, 0.2306618581243847221, -0.2411417322834647770 ) ) ;
#29831=CARTESIAN_POINT ( 'NONE',  ( -0.3674540682414689785, 0.2306618581243848609, 0.2411417322834645549 ) ) ;
#29832=CARTESIAN_POINT ( 'NONE',  ( 0.2624671916010504757, 0.2306618581243848609, 0.2411417322834645549 ) ) ;
#29835=CARTESIAN_POINT ( 'NONE',  ( 0.5446194225721792126, -0.2845877964562159024, 0.3641732283464567677 ) ) ;
#29836=CARTESIAN_POINT ( 'NONE',  ( -1.627296587926508442, -0.5023911411419708095, -0.1820866141732282451 ) ) ;
#29837=CARTESIAN_POINT ( 'NONE',  ( 0.6692913385826778638, -0.6692913385826771977, 8.415575281601705876E-17 ) ) ;
#29838=CARTESIAN_POINT ( 'NONE',  ( -1.496062992125983815, -0.1870078740157480601, -0.3641732283464567677 ) ) ;
#29839=CARTESIAN_POINT ( 'NONE',  ( 1.561679790026247350, -0.3690944881889763329, 0.3153832671262228327 ) ) ;
#29840=CARTESIAN_POINT ( 'NONE',  ( -1.030183727034119867, -0.05778040916215560624, -0.4822834645669293319 ) ) ;
#29841=CARTESIAN_POINT ( 'NONE',  ( -0.4658792650918627265, -0.2845877964562161244, -0.3641732283464567121 ) ) ;
#29842=CARTESIAN_POINT ( 'NONE',  ( 2.795275590551181466, 2.001539355558160871, 0.000000000000000000 ) ) ;
#29843=CARTESIAN_POINT ( 'NONE',  ( 0.5577427821522314977, -0.2845877964562161244, -0.3641732283464567121 ) ) ;
#29844=CARTESIAN_POINT ( 'NONE',  ( -0.2362204724409440182, -0.1870078740157479769, 0.4822834645669291653 ) ) ;
#29846=EDGE_CURVE ( 'NONE', #75163, #51509, #36052, .T. ) ;
#29848=CARTESIAN_POINT ( 'NONE',  ( 0.4986876640419954376, 0.1283753931104748280, 0.1820866141732283561 ) ) ;
#29849=CARTESIAN_POINT ( 'NONE',  ( 0.1968503937007881344, -0.6692913385826771977, 8.415575281601705876E-17 ) ) ;
#29850=CARTESIAN_POINT ( 'NONE',  ( -0.5052493438320203589, 0.2952755905511810774, -0.1292274648535930714 ) ) ;
#29851=CARTESIAN_POINT ( 'NONE',  ( -0.2362204724409440182, -0.1870078740157479769, 0.3641732283464567677 ) ) ;
#29853=CARTESIAN_POINT ( 'NONE',  ( -0.3477690288713902178, 0.1771653543307087075, -0.09757992244046823083 ) ) ;
#29854=CARTESIAN_POINT ( 'NONE',  ( 0.1181102362204730916, 0.2952755905511811885, 0.000000000000000000 ) ) ;
#29855=CARTESIAN_POINT ( 'NONE',  ( -1.010498687664041384, -0.3690944881889765550, -0.3153832671262227771 ) ) ;
#29857=CARTESIAN_POINT ( 'NONE',  ( -1.456692913385826182, 0.2952755905511811885, 0.000000000000000000 ) ) ;
#29858=CARTESIAN_POINT ( 'NONE',  ( 0.4600214019799526155, 2.784432375088962958E-17, -0.3464511005275205946 ) ) ;
#29860=CARTESIAN_POINT ( 'NONE',  ( -1.509186351706035767, -0.004921259842519870586, -0.3153832671262229437 ) ) ;
#29861=CIRCLE ( 'NONE', #28497, 2.362204724409449064 ) ;
#29862=CARTESIAN_POINT ( 'NONE',  ( -0.5774278215223089816, 0.2306618581243847221, -0.2411417322834647770 ) ) ;
#29863=CARTESIAN_POINT ( 'NONE',  ( -1.148293963254592542, 0.2952755905511811885, 0.1292274648535926551 ) ) ;
#29865=DIRECTION ( 'NONE',  ( -3.096699300667737957E-16, 1.000000000000000000, -0.000000000000000000 ) ) ;
#29866=CARTESIAN_POINT ( 'NONE',  ( 1.240157480314961314, 0.1660481256975883668, -0.3530559997133364547 ) ) ;
#29867=CARTESIAN_POINT ( 'NONE',  ( 0.4330708661417329575, 0.2952755905511811885, 0.000000000000000000 ) ) ;
#29870=CARTESIAN_POINT ( 'NONE',  ( 1.581364829396326277, -0.08942795157527998196, 0.3641732283464567121 ) ) ;
#29872=ORIENTED_EDGE ( 'NONE', *, *, #69643, .T. ) ;
#29873=CARTESIAN_POINT ( 'NONE',  ( -1.030183727034119867, -0.2845877964562159024, 0.3641732283464567677 ) ) ;
#29876=CARTESIAN_POINT ( 'NONE',  ( 0.3412073490813655186, 0.2306618581243848609, 0.2411417322834645549 ) ) ;
#29877=CARTESIAN_POINT ( 'NONE',  ( -0.2099737532808391705, -0.6046776061558809534, -0.2411417322834644161 ) ) ;
#29878=CARTESIAN_POINT ( 'NONE',  ( -0.9973753280839886548, 0.2306618581243848609, 0.2411417322834645549 ) ) ;
#29879=CARTESIAN_POINT ( 'NONE',  ( 1.115485564304462551, -0.4281496062992127816, -0.4176697321401328100 ) ) ;
#29880=CARTESIAN_POINT ( 'NONE',  ( -1.351706036745406347, -0.3690944881889763329, 0.3153832671262228327 ) ) ;
#29881=CARTESIAN_POINT ( 'NONE',  ( -0.7974104941589342799, -2.567464376874931580E-15, -0.4445507791589072832 ) ) ;
#29882=CARTESIAN_POINT ( 'NONE',  ( 0.1049868766404206816, 0.2306618581243848609, 0.2411417322834645549 ) ) ;
#29883=CARTESIAN_POINT ( 'NONE',  ( -0.9842519685039360366, 0.2952755905511811885, 0.000000000000000000 ) ) ;
#29885=CARTESIAN_POINT ( 'NONE',  ( -1.548556430446193399, -0.6046776061558809534, -0.2411417322834644161 ) ) ;
#29886=LINE ( 'NONE', #4222, #15682 ) ;
#29888=CARTESIAN_POINT ( 'NONE',  ( 1.062992125984252745, 0.1771653543307087630, 0.000000000000000000 ) ) ;
#29891=CARTESIAN_POINT ( 'NONE',  ( -0.9711286089238838626, 0.2306618581243847221, -0.2411417322834647770 ) ) ;
#29893=CARTESIAN_POINT ( 'NONE',  ( 0.3740157480314966754, 0.07958543189024071263, -0.2665933059059888421 ) ) ;
#29894=CARTESIAN_POINT ( 'NONE',  ( -1.561679790026246017, 0.05413385826771666132, 0.4176697321401328100 ) ) ;
#29895=CARTESIAN_POINT ( 'NONE',  ( 0.4921259842519691285, 0.1660481256975885056, 0.3530559997133364547 ) ) ;
#29896=CARTESIAN_POINT ( 'NONE',  ( 0.5971128608923890191, -0.6692913385826771977, 0.1292274648535927661 ) ) ;
#29897=CARTESIAN_POINT ( 'NONE',  ( -0.09842519685039295696, 0.1660481256975883668, -0.3530559997133364547 ) ) ;
#29899=CARTESIAN_POINT ( 'NONE',  ( -0.9711286089238838626, 0.2306618581243847221, -0.2411417322834647770 ) ) ;
#29901=CARTESIAN_POINT ( 'NONE',  ( 1.437007874015748810, 0.07958543189024085140, 0.2665933059059887866 ) ) ;
#29902=CARTESIAN_POINT ( 'NONE',  ( -1.023622047244093558, -0.1870078740157479769, 0.4822834645669291653 ) ) ;
#29903=CARTESIAN_POINT ( 'NONE',  ( 1.207349081364829990, 0.2306618581243848609, 0.2411417322834645549 ) ) ;
#29904=CARTESIAN_POINT ( 'NONE',  ( 1.338582677165355062, -0.1870078740157479769, 0.4822834645669291653 ) ) ;
#29906=CARTESIAN_POINT ( 'NONE',  ( -0.9711286089238838626, -0.6046776061558807314, 0.2411417322834647770 ) ) ;
#29908=CARTESIAN_POINT ( 'NONE',  ( 0.2493438320209980519, -0.4281496062992127816, -0.4176697321401328100 ) ) ;
#29910=CARTESIAN_POINT ( 'NONE',  ( -0.6889763779527552368, 0.1660481256975885056, 0.3530559997133364547 ) ) ;
#29911=CARTESIAN_POINT ( 'NONE',  ( -1.423884514435694859, -0.08942795157528024563, -0.3641732283464568787 ) ) ;
#29912=CARTESIAN_POINT ( 'NONE',  ( 0.5774278215223104249, 0.1283753931104748280, 0.1820866141732283561 ) ) ;
#29913=CARTESIAN_POINT ( 'NONE',  ( 1.351706036745407458, -0.4281496062992127816, -0.4176697321401328100 ) ) ;
#29915=CARTESIAN_POINT ( 'NONE',  ( 0.7152230971128616943, -0.08942795157527998196, 0.3641732283464567121 ) ) ;
#29916=CARTESIAN_POINT ( 'NONE',  ( 0.9317585301837276734, -0.4281496062992124485, 0.4176697321401328655 ) ) ;
#29919=CARTESIAN_POINT ( 'NONE',  ( -0.7545931758530177724, 0.2952755905511811885, 0.1292274648535926551 ) ) ;
#29920=CARTESIAN_POINT ( 'NONE',  ( 1.614173228346456712, 0.8346805926620878280, 0.1372047244094478646 ) ) ;
#29921=CARTESIAN_POINT ( 'NONE',  ( 1.417322834645670104, -0.1870078740157479769, 0.3641732283464567677 ) ) ;
#29922=CARTESIAN_POINT ( 'NONE',  ( -0.4527559055118102749, 0.1660481256975885056, 0.3530559997133364547 ) ) ;
#29923=CARTESIAN_POINT ( 'NONE',  ( 5.463695987328526437E-16, -0.1870078740157479769, 0.4822834645669291653 ) ) ;
#29924=CARTESIAN_POINT ( 'NONE',  ( -1.586052503253849499, 0.4724409448818907564, 0.1653254495020552439 ) ) ;
#29925=CARTESIAN_POINT ( 'NONE',  ( 0.1902887139107617975, 0.2952755905511811885, 0.1292274648535926551 ) ) ;
#29926=CARTESIAN_POINT ( 'NONE',  ( 0.2821522309711292364, 0.1771653543307087075, -0.09757992244046823083 ) ) ;
#29928=CARTESIAN_POINT ( 'NONE',  ( 0.1968503937007881344, -0.5511811023622047445, 6.969142054262312111E-17 ) ) ;
#29929=CARTESIAN_POINT ( 'NONE',  ( 0.7020997375328090762, -0.08942795157528024563, -0.3641732283464568787 ) ) ;
#29932=CARTESIAN_POINT ( 'NONE',  ( 0.2624671916010504757, 0.2306618581243848609, 0.2411417322834645549 ) ) ;
#29934=CARTESIAN_POINT ( 'NONE',  ( 1.601049868766404982, -0.5023911411419708095, -0.1820866141732282451 ) ) ;
#29935=CARTESIAN_POINT ( 'NONE',  ( 0.1312335958005257930, 0.2306618581243847221, -0.2411417322834647770 ) ) ;
#29936=CARTESIAN_POINT ( 'NONE',  ( -0.4068241469816267775, -0.004921259842519870586, -0.3153832671262229437 ) ) ;
#29937=CARTESIAN_POINT ( 'NONE',  ( -0.05905511811023545637, 0.1660481256975885056, 0.3530559997133364547 ) ) ;
#29938=CARTESIAN_POINT ( 'NONE',  ( 1.141732283464567788, -0.5511811023622047445, 6.969142054262312111E-17 ) ) ;
#29940=CARTESIAN_POINT ( 'NONE',  ( -1.377952755905511140, 0.2952755905511811885, 0.000000000000000000 ) ) ;
#29941=CARTESIAN_POINT ( 'NONE',  ( 0.01968503937007957949, -0.5400638737290845981, -0.3530559997133363437 ) ) ;
#29943=CARTESIAN_POINT ( 'NONE',  ( 1.141732283464567788, -0.6692913385826771977, 8.415575281601705876E-17 ) ) ;
#29944=CARTESIAN_POINT ( 'NONE',  ( -1.614173228346457378, 1.881821177735609085, -0.1372047244094477536 ) ) ;
#29945=CARTESIAN_POINT ( 'NONE',  ( 0.006561679790026889343, -0.05778040916215522460, 0.4822834645669289988 ) ) ;
#29946=CARTESIAN_POINT ( 'NONE',  ( 1.371391076115485941, 0.2952755905511811885, 0.1292274648535926551 ) ) ;
#29947=CARTESIAN_POINT ( 'NONE',  ( 0.7808398950131241190, -0.05778040916215560624, -0.4822834645669293319 ) ) ;
#29948=CARTESIAN_POINT ( 'NONE',  ( -1.712598425196849572, 0.07958543189024085140, 0.2665933059059887866 ) ) ;
#29949=CARTESIAN_POINT ( 'NONE',  ( 0.8595800524934390507, -0.2845877964562159024, 0.3641732283464567677 ) ) ;
#29950=CARTESIAN_POINT ( 'NONE',  ( -1.528871391076114250, -0.5511811023622046335, 0.09757992244046803654 ) ) ;
#29951=CARTESIAN_POINT ( 'NONE',  ( 0.2755905511811031494, -0.5511811023622047445, 6.969142054262312111E-17 ) ) ;
#29952=CARTESIAN_POINT ( 'NONE',  ( -0.2952755905511803003, -0.5400638737290845981, -0.3530559997133363437 ) ) ;
#29953=CARTESIAN_POINT ( 'NONE',  ( 0.5052493438320215802, 0.2952755905511811885, 0.1292274648535926551 ) ) ;
#29954=CARTESIAN_POINT ( 'NONE',  ( -0.2624671916010490880, -0.6046776061558807314, 0.2411417322834647770 ) ) ;
#29957=CARTESIAN_POINT ( 'NONE',  ( -0.3083989501312330295, -0.08942795157527998196, 0.3641732283464567121 ) ) ;
#29958=CARTESIAN_POINT ( 'NONE',  ( 0.9711286089238851948, 0.2306618581243848609, 0.2411417322834645549 ) ) ;
#29959=CARTESIAN_POINT ( 'NONE',  ( 1.082677165354331228, 0.07958543189024071263, -0.2665933059059888421 ) ) ;
#29960=CARTESIAN_POINT ( 'NONE',  ( 0.1312335958005257930, 0.2306618581243847221, -0.2411417322834647770 ) ) ;
#29963=CARTESIAN_POINT ( 'NONE',  ( 1.581364829396326277, -0.05778040916215522460, 0.4822834645669289988 ) ) ;
#29965=CARTESIAN_POINT ( 'NONE',  ( -1.312335958005248715, 0.2306618581243848609, 0.2411417322834645549 ) ) ;
#29966=CARTESIAN_POINT ( 'NONE',  ( -0.3805774278215216522, -0.4281496062992127816, -0.4176697321401328100 ) ) ;
#29970=CARTESIAN_POINT ( 'NONE',  ( 0.4396325459317593221, 0.1771653543307087075, -0.09757992244046823083 ) ) ;
#29971=AXIS2_PLACEMENT_3D ( 'NONE', #11344, #74502, #16850 ) ;
#29973=CARTESIAN_POINT ( 'NONE',  ( 0.9317585301837276734, -0.4281496062992124485, 0.4176697321401328655 ) ) ;
#29975=CARTESIAN_POINT ( 'NONE',  ( 1.010498687664042716, 0.05413385826771626580, -0.4176697321401330321 ) ) ;
#29976=CARTESIAN_POINT ( 'NONE',  ( -1.699475065616797398, 0.1771653543307087630, 0.09757992244046791164 ) ) ;
#29977=CARTESIAN_POINT ( 'NONE',  ( 1.437007874015748810, -0.5400638737290845981, -0.3530559997133363437 ) ) ;
#29978=EDGE_CURVE ( 'NONE', #39084, #74503, #49152, .T. ) ;
#29979=CARTESIAN_POINT ( 'NONE',  ( 1.194225721784777594, -0.3690944881889765550, -0.3153832671262227771 ) ) ;
#29980=CARTESIAN_POINT ( 'NONE',  ( 0.4724409448818904789, -0.1870078740157480879, -0.4822834645669291653 ) ) ;
#29982=CARTESIAN_POINT ( 'NONE',  ( -0.2690288713910754526, -0.6692913385826771977, 0.1292274648535927661 ) ) ;
#29983=CARTESIAN_POINT ( 'NONE',  ( -1.023622047244094002, -0.1870078740157480601, -0.3641732283464567677 ) ) ;
#29984=CARTESIAN_POINT ( 'NONE',  ( 0.3937007874015754361, -0.1870078740157480879, -0.4822834645669291653 ) ) ;
#29985=CARTESIAN_POINT ( 'NONE',  ( -0.1574803149606292529, -0.1870078740157479769, 0.4822834645669291653 ) ) ;
#29987=CARTESIAN_POINT ( 'NONE',  ( 0.5118110236220478892, 0.2952755905511811885, 0.000000000000000000 ) ) ;
#29988=CARTESIAN_POINT ( 'NONE',  ( 2.795275590551181910, 1.535433070866142335, 0.000000000000000000 ) ) ;
#29990=CARTESIAN_POINT ( 'NONE',  ( 1.023622047244095334, -0.1870078740157479769, 0.4822834645669291653 ) ) ;
#29991=CARTESIAN_POINT ( 'NONE',  ( -0.4133858267716528645, 0.1660481256975883668, -0.3530559997133364547 ) ) ;
#29992=CARTESIAN_POINT ( 'NONE',  ( -1.371391076115484609, -0.6692913385826771977, 0.1292274648535927661 ) ) ;
#29993=CARTESIAN_POINT ( 'NONE',  ( 0.9317585301837276734, -0.4281496062992124485, 0.4176697321401328655 ) ) ;
#29994=CARTESIAN_POINT ( 'NONE',  ( 0.5314960629921267055, -0.5400638737290844871, 0.3530559997133364547 ) ) ;
#29996=CARTESIAN_POINT ( 'NONE',  ( -0.2034120734908131112, -0.6692913385826773087, -0.1292274648535924053 ) ) ;
#29997=CARTESIAN_POINT ( 'NONE',  ( 0.07874015748031558404, -0.1870078740157479769, 0.4822834645669291653 ) ) ;
#29998=CARTESIAN_POINT ( 'NONE',  ( -0.3740157480314953431, 0.1660481256975885056, 0.3530559997133364547 ) ) ;
#29999=CARTESIAN_POINT ( 'NONE',  ( 0.4199475065616805614, 0.1283753931104748280, 0.1820866141732283561 ) ) ;
#30000=CARTESIAN_POINT ( 'NONE',  ( 1.620734908136483465, -0.5511811023622046335, 0.09757992244046803654 ) ) ;
#30002=CARTESIAN_POINT ( 'NONE',  ( 0.3674540682414705883, 0.2306618581243847221, -0.2411417322834647770 ) ) ;
#30004=CARTESIAN_POINT ( 'NONE',  ( -1.620734908136482577, 0.2952755905511811885, 0.1292274648535926551 ) ) ;
#30005=CARTESIAN_POINT ( 'NONE',  ( 0.4921259842519691841, 0.1012011053420777407, 0.2882089793578257453 ) ) ;
#30008=ORIENTED_EDGE ( 'NONE', *, *, #55359, .F. ) ;
#30009=CARTESIAN_POINT ( 'NONE',  ( 0.5511811023622055217, -0.1870078740157479769, 0.4822834645669291653 ) ) ;
#30010=CARTESIAN_POINT ( 'NONE',  ( 0.1377952755905518800, -0.4536011799217367080, 0.2665933059059888421 ) ) ;
#30014=CARTESIAN_POINT ( 'NONE',  ( -0.9568149321855660139, 1.315108829465093930E-15, -0.3627985898453513491 ) ) ;
#30017=CARTESIAN_POINT ( 'NONE',  ( 0.5511811023622054106, -0.1870078740157480879, -0.4822834645669291653 ) ) ;
#30018=CARTESIAN_POINT ( 'NONE',  ( -0.8136482939632537770, 0.2306618581243847221, -0.2411417322834647770 ) ) ;
#30020=CARTESIAN_POINT ( 'NONE',  ( -0.8858267716535425107, 0.1660481256975883668, -0.3530559997133364547 ) ) ;
#30021=CARTESIAN_POINT ( 'NONE',  ( 0.5905511811023629321, -0.6692913385826771977, 8.415575281601705876E-17 ) ) ;
#30022=CARTESIAN_POINT ( 'NONE',  ( 1.574803149606299746, -0.1870078740157479769, 0.4822834645669291653 ) ) ;
#30023=CARTESIAN_POINT ( 'NONE',  ( 1.240157480314961314, 0.07958543189024071263, -0.2665933059059888421 ) ) ;
#30025=CARTESIAN_POINT ( 'NONE',  ( 1.115485564304462551, -0.3690944881889765550, -0.3153832671262227771 ) ) ;
#30026=CARTESIAN_POINT ( 'NONE',  ( -0.7742782152230962556, -0.4281496062992127816, -0.4176697321401328100 ) ) ;
#30028=CARTESIAN_POINT ( 'NONE',  ( 1.541994750656168645, 0.2952755905511810774, -0.1292274648535930714 ) ) ;
#30030=CARTESIAN_POINT ( 'NONE',  ( -0.3805774278215216522, 0.05413385826771666132, 0.4176697321401328100 ) ) ;
#30031=CARTESIAN_POINT ( 'NONE',  ( 1.036745406824147731, 0.05413385826771666132, 0.4176697321401328100 ) ) ;
#30032=CARTESIAN_POINT ( 'NONE',  ( 0.000000000000000000, 2.401574803149606474, 0.000000000000000000 ) ) ;
#30033=CARTESIAN_POINT ( 'NONE',  ( -1.056430446194224881, 0.1771653543307087075, -0.09757992244046823083 ) ) ;
#30034=CARTESIAN_POINT ( 'NONE',  ( 0.5839895013123367340, 0.2952755905511811885, 0.1292274648535926551 ) ) ;
#30035=CARTESIAN_POINT ( 'NONE',  ( 0.9580052493438326877, -0.004921259842519576551, 0.3153832671262227771 ) ) ;
#30038=CARTESIAN_POINT ( 'NONE',  ( -1.181102362204723644, -0.1870078740157480601, -0.3641732283464567677 ) ) ;
#30039=CARTESIAN_POINT ( 'NONE',  ( 1.253280839895013710, -0.05778040916215560624, -0.4822834645669293319 ) ) ;
#30041=CARTESIAN_POINT ( 'NONE',  ( -0.1837270341207343505, -0.5023911411419708095, 0.1820866141732285504 ) ) ;
#30042=CARTESIAN_POINT ( 'NONE',  ( -0.3018372703412066094, 0.05413385826771666132, 0.4176697321401328100 ) ) ;
#30043=CARTESIAN_POINT ( 'NONE',  ( -1.161417322834644716, 0.07958543189024085140, 0.2665933059059887866 ) ) ;
#30044=CARTESIAN_POINT ( 'NONE',  ( -0.5971128608923877978, 0.2952755905511811885, 0.1292274648535926551 ) ) ;
#30045=CARTESIAN_POINT ( 'NONE',  ( 1.338582677165355062, -0.1870078740157479769, 0.4822834645669291653 ) ) ;
#30047=CARTESIAN_POINT ( 'NONE',  ( -0.9055118110236215490, -0.5511811023622047445, 6.969142054262312111E-17 ) ) ;
#30049=CARTESIAN_POINT ( 'NONE',  ( 1.325459317585302665, 0.05413385826771626580, -0.4176697321401330321 ) ) ;
#30051=CARTESIAN_POINT ( 'NONE',  ( -1.246719160104986512, 0.05413385826771666132, 0.4176697321401328100 ) ) ;
#30052=CARTESIAN_POINT ( 'NONE',  ( -1.227034120734907141, -0.5511811023622048555, -0.09757992244046775898 ) ) ;
#30053=EDGE_CURVE ( 'NONE', #30109, #58566, #18077, .T. ) ;
#30054=CARTESIAN_POINT ( 'NONE',  ( -0.5511811023622041894, -0.1870078740157480601, -0.3641732283464567677 ) ) ;
#30055=CARTESIAN_POINT ( 'NONE',  ( -0.5314960629921250401, 0.1012011053420777407, 0.2882089793578256898 ) ) ;
#30056=CARTESIAN_POINT ( 'NONE',  ( 0.1771653543307093182, -0.5400638737290845981, -0.3530559997133363437 ) ) ;
#30057=CARTESIAN_POINT ( 'NONE',  ( 0.1443569553805781891, -0.004921259842519870586, -0.3153832671262229437 ) ) ;
#30058=CARTESIAN_POINT ( 'NONE',  ( -1.312335958005248715, -0.5023911411419708095, -0.1820866141732282451 ) ) ;
#30059=CARTESIAN_POINT ( 'NONE',  ( -1.384514435695537005, 0.2952755905511811885, 0.1292274648535926551 ) ) ;
#30060=CARTESIAN_POINT ( 'NONE',  ( 1.364829396325459854, -0.5023911411419708095, -0.1820866141732282451 ) ) ;
#30061=CARTESIAN_POINT ( 'NONE',  ( 1.167979002624672580, -0.4281496062992124485, 0.4176697321401328655 ) ) ;
#30063=CARTESIAN_POINT ( 'NONE',  ( 0.2493438320209980519, -0.004921259842519576551, 0.3153832671262227771 ) ) ;
#30064=CARTESIAN_POINT ( 'NONE',  ( 0.7808398950131241190, -0.05778040916215560624, -0.4822834645669293319 ) ) ;
#30065=CARTESIAN_POINT ( 'NONE',  ( 0.9186351706036751663, -0.5023911411419708095, 0.1820866141732285504 ) ) ;
#30067=CARTESIAN_POINT ( 'NONE',  ( -1.181102362204723644, -0.1870078740157479769, 0.4822834645669291653 ) ) ;
#30069=CARTESIAN_POINT ( 'NONE',  ( -1.095800524934382292, -0.3162353388693409650, -0.4822834645669289433 ) ) ;
#30070=CARTESIAN_POINT ( 'NONE',  ( -0.2362204724409442680, -0.1870078740157480879, -0.4822834645669291653 ) ) ;
#30071=CARTESIAN_POINT ( 'NONE',  ( -1.712598425196849572, 0.07958543189024085140, 0.2665933059059887866 ) ) ;
#30073=CARTESIAN_POINT ( 'NONE',  ( 0.7020997375328090762, -0.05778040916215560624, -0.4822834645669293319 ) ) ;
#30074=CARTESIAN_POINT ( 'NONE',  ( -1.692913385826770645, 0.2952755905511811885, 0.000000000000000000 ) ) ;
#30075=CARTESIAN_POINT ( 'NONE',  ( 8.195543980992789655E-16, -0.1870078740157480879, -0.4822834645669291653 ) ) ;
#30076=CARTESIAN_POINT ( 'NONE',  ( 0.9120734908136489683, -0.6692913385826771977, 0.1292274648535927661 ) ) ;
#30080=CARTESIAN_POINT ( 'NONE',  ( 0.000000000000000000, 0.000000000000000000, 0.000000000000000000 ) ) ;
#30081=VECTOR ( 'NONE', #54120, 39.37007874015748143 ) ;
#30083=CARTESIAN_POINT ( 'NONE',  ( -0.4658792650918627265, -0.08942795157527998196, 0.3641732283464567121 ) ) ;
#30084=CARTESIAN_POINT ( 'NONE',  ( -0.6430446194225716283, -0.4281496062992124485, 0.4176697321401328655 ) ) ;
#30085=CARTESIAN_POINT ( 'NONE',  ( 0.3280839895013130669, 0.05413385826771666132, 0.4176697321401328100 ) ) ;
#30087=CARTESIAN_POINT ( 'NONE',  ( -1.640419947506561060, 0.05413385826771666132, 0.4176697321401328100 ) ) ;
#30088=CARTESIAN_POINT ( 'NONE',  ( 1.364829396325459854, -0.6046776061558809534, -0.2411417322834644161 ) ) ;
#30092=CARTESIAN_POINT ( 'NONE',  ( 0.8070866141732288002, 0.1660481256975885056, 0.3530559997133364547 ) ) ;
#30093=CARTESIAN_POINT ( 'NONE',  ( 0.6364829396325465405, -0.05778040916215522460, 0.4822834645669289988 ) ) ;
#30095=CARTESIAN_POINT ( 'NONE',  ( 1.115485564304462551, -0.004921259842519576551, 0.3153832671262227771 ) ) ;
#30096=CARTESIAN_POINT ( 'NONE',  ( -1.437007874015747477, 0.07958543189024071263, -0.2665933059059888421 ) ) ;
#30097=CARTESIAN_POINT ( 'NONE',  ( -1.528871391076114250, -0.6692913385826771977, 0.1292274648535927661 ) ) ;
#30100=CARTESIAN_POINT ( 'NONE',  ( 0.8923884514435703741, 0.2306618581243848609, 0.2411417322834645549 ) ) ;
#30101=CARTESIAN_POINT ( 'NONE',  ( -2.795275590551181466, 2.165354330708661568, 0.000000000000000000 ) ) ;
#30102=CARTESIAN_POINT ( 'NONE',  ( -0.4527559055118102749, 0.1660481256975885056, 0.3530559997133364547 ) ) ;
#30103=CARTESIAN_POINT ( 'NONE',  ( -0.7086614173228339419, -0.1870078740157480879, -0.4822834645669291653 ) ) ;
#30104=CARTESIAN_POINT ( 'NONE',  ( -1.620734908136482577, 0.2952755905511811885, 0.1292274648535926551 ) ) ;
#30106=CARTESIAN_POINT ( 'NONE',  ( 0.3740157480314966754, 0.1660481256975883668, -0.3530559997133364547 ) ) ;
#30108=CARTESIAN_POINT ( 'NONE',  ( 1.496062992125985147, -0.1870078740157479769, 0.4822834645669291653 ) ) ;
#30109=VERTEX_POINT ( 'NONE', #38657 ) ;
#30113=CARTESIAN_POINT ( 'NONE',  ( 1.187664041994751285, -0.2845877964562161244, -0.3641732283464567121 ) ) ;
#30115=CARTESIAN_POINT ( 'NONE',  ( 1.548556430446194954, 0.1283753931104746893, -0.1820866141732285504 ) ) ;
#30120=CARTESIAN_POINT ( 'NONE',  ( -0.2230971128608915943, -0.004921259842519576551, 0.3153832671262227771 ) ) ;
#30121=CARTESIAN_POINT ( 'NONE',  ( -1.240157480314959759, 0.07958543189024085140, 0.2665933059059887866 ) ) ;
#30122=CARTESIAN_POINT ( 'NONE',  ( 1.450131233595801428, 0.2952755905511811885, 0.1292274648535926551 ) ) ;
#30123=CARTESIAN_POINT ( 'NONE',  ( 0.5314960629921264834, 0.1660481256975883668, -0.3530559997133364547 ) ) ;
#30124=CARTESIAN_POINT ( 'NONE',  ( -1.272965879265091305, 0.05413385826771626580, -0.4176697321401330321 ) ) ;
#30126=VERTEX_POINT ( 'NONE', #76968 ) ;
#30127=CARTESIAN_POINT ( 'NONE',  ( 1.417322834645670104, -0.1870078740157479769, 0.4822834645669291653 ) ) ;
#30128=CARTESIAN_POINT ( 'NONE',  ( -1.614173228346457378, 0.2753471884572478157, -0.1372047244094478091 ) ) ;
#30130=CARTESIAN_POINT ( 'NONE',  ( 1.604771003085129433, 1.044625174762918496, -0.1466069496707749775 ) ) ;
#30132=CARTESIAN_POINT ( 'NONE',  ( -0.6102362204724400829, -0.5400638737290845981, -0.3530559997133363437 ) ) ;
#30133=CARTESIAN_POINT ( 'NONE',  ( 1.279527559055118724, -0.5400638737290845981, -0.3530559997133363437 ) ) ;
#30136=EDGE_CURVE ( 'NONE', #11377, #36098, #75263, .T. ) ;
#30137=CARTESIAN_POINT ( 'NONE',  ( 1.443569553805774897, -0.6046776061558809534, -0.2411417322834644161 ) ) ;
#30138=CARTESIAN_POINT ( 'NONE',  ( -0.8595800524934373854, -0.3162353388693409650, -0.4822834645669289433 ) ) ;
#30140=CARTESIAN_POINT ( 'NONE',  ( -0.1312335958005241554, 0.1283753931104748280, 0.1820866141732283561 ) ) ;
#30143=EDGE_CURVE ( 'NONE', #53475, #77295, #50445, .T. ) ;
#30144=CARTESIAN_POINT ( 'NONE',  ( -0.2362204724409440182, -0.1870078740157479769, 0.3641732283464567677 ) ) ;
#30145=CARTESIAN_POINT ( 'NONE',  ( 0.4658792650918640033, -0.2845877964562159024, 0.3641732283464567677 ) ) ;
#30146=CARTESIAN_POINT ( 'NONE',  ( 0.6627296587926515548, 0.2952755905511811885, 0.1292274648535926551 ) ) ;
#30147=CARTESIAN_POINT ( 'NONE',  ( -0.8923884514435688198, -0.5023911411419708095, 0.1820866141732285504 ) ) ;
#30149=CARTESIAN_POINT ( 'NONE',  ( -1.633858267716534529, 0.1660481256975885056, 0.3530559997133364547 ) ) ;
#30150=CARTESIAN_POINT ( 'NONE',  ( -1.062992125984250968, -0.6692913385826771977, 8.415575281601705876E-17 ) ) ;
#30152=CARTESIAN_POINT ( 'NONE',  ( -0.08530183727034056085, -0.05778040916215560624, -0.4822834645669293319 ) ) ;
#30153=CARTESIAN_POINT ( 'NONE',  ( -0.3412073490813641308, 0.2306618581243847221, -0.2411417322834647770 ) ) ;
#30154=CARTESIAN_POINT ( 'NONE',  ( 1.292650918635171564, -0.5511811023622048555, -0.09757992244046775898 ) ) ;
#30155=CARTESIAN_POINT ( 'NONE',  ( 0.2887139107611556010, -0.5023911411419708095, 0.1820866141732285504 ) ) ;
#30156=CARTESIAN_POINT ( 'NONE',  ( -0.05249343832020938322, -0.6046776061558809534, -0.2411417322834644161 ) ) ;
#30157=CARTESIAN_POINT ( 'NONE',  ( -0.8005249343832011588, 0.05413385826771626580, -0.4176697321401330321 ) ) ;
#30158=CARTESIAN_POINT ( 'NONE',  ( -0.6365311798326280801, 1.942272084518505082, -0.5177672855602343249 ) ) ;
#30159=CARTESIAN_POINT ( 'NONE',  ( 1.502624671916010790, -0.08942795157527998196, 0.3641732283464567121 ) ) ;
#30160=CARTESIAN_POINT ( 'NONE',  ( 0.1181102362204730916, 0.2952755905511811885, 0.000000000000000000 ) ) ;
#30161=VERTEX_POINT ( 'NONE', #44535 ) ;
#30163=CARTESIAN_POINT ( 'NONE',  ( 1.056430446194226436, -0.6692913385826773087, -0.1292274648535924053 ) ) ;
#30164=CARTESIAN_POINT ( 'NONE',  ( -0.5380577427821514602, -0.3690944881889765550, -0.3153832671262227771 ) ) ;
#30165=CARTESIAN_POINT ( 'NONE',  ( -0.7808398950131225646, -0.05778040916215522460, 0.4822834645669289988 ) ) ;
#30166=CARTESIAN_POINT ( 'NONE',  ( 1.108923884514436686, -0.3162353388693409650, -0.4822834645669289433 ) ) ;
#30167=CARTESIAN_POINT ( 'NONE',  ( 0.7874015748031503170, -0.1870078740157480879, -0.4822834645669291653 ) ) ;
#30168=CARTESIAN_POINT ( 'NONE',  ( -1.561679790026246017, -0.4281496062992127816, -0.4176697321401328100 ) ) ;
#30169=CARTESIAN_POINT ( 'NONE',  ( -1.200787401574802349, 0.07958543189024071263, -0.2665933059059888421 ) ) ;
#30173=CARTESIAN_POINT ( 'NONE',  ( 1.646981627296588035, -0.2845877964562159024, 0.3641732283464567677 ) ) ;
#30174=CARTESIAN_POINT ( 'NONE',  ( 0.8661417322834652488, -0.1870078740157480601, -0.3641732283464567677 ) ) ;
#30175=CARTESIAN_POINT ( 'NONE',  ( 0.6036745406824153282, -0.6046776061558807314, 0.2411417322834647770 ) ) ;
#30176=CARTESIAN_POINT ( 'NONE',  ( 1.541994750656168645, -0.6692913385826771977, 0.1292274648535927661 ) ) ;
#30177=B_SPLINE_CURVE_WITH_KNOTS ( 'NONE', 3,
 ( #13161, #39227, #63654, #7249 ),
 .UNSPECIFIED., .F., .F.,
 ( 4, 4 ),
 ( 1.999999999910059834E-07, 0.006970199999999934261 ),
 .UNSPECIFIED. ) ;
#30179=CARTESIAN_POINT ( 'NONE',  ( 0.7349081364829403995, 0.1283753931104748280, 0.1820866141732283561 ) ) ;
#30180=CARTESIAN_POINT ( 'NONE',  ( -0.1443569553805765515, -0.4281496062992127816, -0.4176697321401328100 ) ) ;
#30181=CARTESIAN_POINT ( 'NONE',  ( -0.9842519685039360366, 0.2952755905511811885, 0.000000000000000000 ) ) ;
#30182=CARTESIAN_POINT ( 'NONE',  ( 1.437007874015748810, -0.5400638737290845981, -0.3530559997133363437 ) ) ;
#30185=CARTESIAN_POINT ( 'NONE',  ( -0.1181102362204717315, 0.1771653543307087630, 0.000000000000000000 ) ) ;
#30186=ORIENTED_EDGE ( 'NONE', *, *, #19084, .F. ) ;
#30189=CARTESIAN_POINT ( 'NONE',  ( -0.7545931758530177724, 0.2952755905511811885, 0.1292274648535926551 ) ) ;
#30190=CARTESIAN_POINT ( 'NONE',  ( -0.01968503937007793844, 0.1660481256975883668, -0.3530559997133364547 ) ) ;
#30191=CARTESIAN_POINT ( 'NONE',  ( -0.4330708661417315697, -0.6692913385826771977, 8.415575281601705876E-17 ) ) ;
#30193=CARTESIAN_POINT ( 'NONE',  ( 0.5577427821522316087, -0.05778040916215522460, 0.4822834645669289988 ) ) ;
#30194=CARTESIAN_POINT ( 'NONE',  ( -0.6299212598425188991, -0.1870078740157480879, -0.4822834645669291653 ) ) ;
#30195=CARTESIAN_POINT ( 'NONE',  ( -1.443569553805773564, 0.2306618581243847221, -0.2411417322834647770 ) ) ;
#30196=CARTESIAN_POINT ( 'NONE',  ( -0.6692913385826764205, -0.6692913385826771977, 8.415575281601705876E-17 ) ) ;
#30197=CARTESIAN_POINT ( 'NONE',  ( 0.7349081364829402885, -0.6046776061558809534, -0.2411417322834644161 ) ) ;
#30198=CARTESIAN_POINT ( 'NONE',  ( 0.3543307086614179147, 0.2952755905511811885, 0.000000000000000000 ) ) ;
#30200=CARTESIAN_POINT ( 'NONE',  ( -0.3477690288713902178, 0.1771653543307087075, -0.09757992244046823083 ) ) ;
#30203=EDGE_LOOP ( 'NONE', ( #3108, #76570, #40755, #13359 ) ) ;
#30204=CARTESIAN_POINT ( 'NONE',  ( -1.148293963254592542, -0.5511811023622048555, -0.09757992244046775898 ) ) ;
#30205=CARTESIAN_POINT ( 'NONE',  ( -0.4199475065616791736, -0.6046776061558807314, 0.2411417322834647770 ) ) ;
#30207=CARTESIAN_POINT ( 'NONE',  ( -0.7152230971128602510, -0.05778040916215560624, -0.4822834645669293319 ) ) ;
#30208=CARTESIAN_POINT ( 'NONE',  ( -0.7677165354330699465, 0.1660481256975885056, 0.3530559997133364547 ) ) ;
#30209=CARTESIAN_POINT ( 'NONE',  ( -0.7137454485294948414, 2.793565526369265584, -0.4917280318828583519 ) ) ;
#30212=CARTESIAN_POINT ( 'NONE',  ( 1.089238845144357759, -0.004921259842519870586, -0.3153832671262229437 ) ) ;
#30213=CARTESIAN_POINT ( 'NONE',  ( 1.614173228346457378, 0.4410134679336836783, -0.1372047244094476148 ) ) ;
#30215=CARTESIAN_POINT ( 'NONE',  ( -0.09186351706036689768, -0.004921259842519870586, -0.3153832671262229437 ) ) ;
#30216=CARTESIAN_POINT ( 'NONE',  ( -0.1968503937007867743, 0.2952755905511811885, 0.000000000000000000 ) ) ;
#30218=CARTESIAN_POINT ( 'NONE',  ( -0.2821522309711278487, -0.6692913385826773087, -0.1292274648535924053 ) ) ;
#30224=CARTESIAN_POINT ( 'NONE',  ( 1.595398199321655275, 0.4619154201552251315, -0.1559797534342493852 ) ) ;
#30225=CARTESIAN_POINT ( 'NONE',  ( -0.8661417322834640276, -0.1870078740157480601, -0.3641732283464567677 ) ) ;
#30226=CARTESIAN_POINT ( 'NONE',  ( -0.8464566929133852113, -0.5400638737290845981, -0.3530559997133363437 ) ) ;
#30228=CARTESIAN_POINT ( 'NONE',  ( -2.795275590551181910, 1.889763779527559251, -6.635626899597537341E-17 ) ) ;
#30231=CARTESIAN_POINT ( 'NONE',  ( 1.489501312335958172, -0.3162353388693405765, 0.4822834645669290543 ) ) ;
#30232=CARTESIAN_POINT ( 'NONE',  ( 0.6102362204724416372, -0.5400638737290844871, 0.3530559997133364547 ) ) ;
#30233=CARTESIAN_POINT ( 'NONE',  ( 0.4724409448818904789, -0.1870078740157480879, -0.4822834645669291653 ) ) ;
#30234=CARTESIAN_POINT ( 'NONE',  ( -0.7414698162729651543, -0.5511811023622046335, 0.09757992244046803654 ) ) ;
#30235=CARTESIAN_POINT ( 'NONE',  ( -0.4658792650918627265, -0.05778040916215522460, 0.4822834645669289988 ) ) ;
#30237=CARTESIAN_POINT ( 'NONE',  ( -1.017060367454067249, -0.3162353388693409650, -0.4822834645669289433 ) ) ;
#30240=CARTESIAN_POINT ( 'NONE',  ( 1.148293963254593653, 0.1771653543307087075, -0.09757992244046823083 ) ) ;
#30241=CARTESIAN_POINT ( 'NONE',  ( -0.4790026246719154557, -0.2845877964562159024, 0.3641732283464567677 ) ) ;
#30242=CARTESIAN_POINT ( 'NONE',  ( 1.220472440944882608, 0.1771653543307087630, 0.000000000000000000 ) ) ;
#30243=CARTESIAN_POINT ( 'NONE',  ( -1.692913385826770645, 0.2952755905511811885, 0.000000000000000000 ) ) ;
#30244=CARTESIAN_POINT ( 'NONE',  ( -1.056430446194224881, -0.5511811023622046335, 0.09757992244046803654 ) ) ;
#30246=CARTESIAN_POINT ( 'NONE',  ( 0.3346456692913393205, -0.4536011799217368745, -0.2665933059059886201 ) ) ;
#30247=CARTESIAN_POINT ( 'NONE',  ( -0.3149606299212590610, -0.1870078740157480879, -0.4822834645669291653 ) ) ;
#30248=CARTESIAN_POINT ( 'NONE',  ( 0.3018372703412079971, 0.05413385826771626580, -0.4176697321401330321 ) ) ;
#30249=CARTESIAN_POINT ( 'NONE',  ( -0.06561679790026180015, -0.004921259842519576551, 0.3153832671262227771 ) ) ;
#30250=CARTESIAN_POINT ( 'NONE',  ( -1.725721784776902190, -0.08942795157527998196, 0.3641732283464567121 ) ) ;
#30251=CARTESIAN_POINT ( 'NONE',  ( 0.8005249343832028242, -0.4281496062992127816, -0.4176697321401328100 ) ) ;
#30252=CYLINDRICAL_SURFACE ( 'NONE', #31741, 0.3937007874015748254 ) ;
#30253=CARTESIAN_POINT ( 'NONE',  ( 1.338582677165355062, -0.1870078740157480601, -0.3641732283464567677 ) ) ;
#30254=CARTESIAN_POINT ( 'NONE',  ( -0.9186351706036736120, 0.2306618581243848609, 0.2411417322834645549 ) ) ;
#30255=CARTESIAN_POINT ( 'NONE',  ( -0.2624671916010490880, -0.5023911411419708095, 0.1820866141732285504 ) ) ;
#30257=CARTESIAN_POINT ( 'NONE',  ( 0.4002624671916016896, -0.2845877964562161244, -0.3641732283464567121 ) ) ;
#30258=CARTESIAN_POINT ( 'NONE',  ( 0.04593175853018440641, -0.6692913385826771977, 0.1292274648535927661 ) ) ;
#30261=CARTESIAN_POINT ( 'NONE',  ( 0.6496062992125991586, 0.07958543189024085140, 0.2665933059059887866 ) ) ;
#30262=CARTESIAN_POINT ( 'NONE',  ( -0.2559055118110227234, -0.5400638737290844871, 0.3530559997133364547 ) ) ;
#30263=CARTESIAN_POINT ( 'NONE',  ( -0.8070866141732276899, 0.1660481256975883668, -0.3530559997133364547 ) ) ;
#30264=CARTESIAN_POINT ( 'NONE',  ( -0.8595800524934373854, -0.08942795157527998196, 0.3641732283464567121 ) ) ;
#30266=CARTESIAN_POINT ( 'NONE',  ( -0.7020997375328074108, -0.08942795157527998196, 0.3641732283464567121 ) ) ;
#30267=CARTESIAN_POINT ( 'NONE',  ( -0.006561679790025524116, -0.05778040916215560624, -0.4822834645669293319 ) ) ;
#30268=CARTESIAN_POINT ( 'NONE',  ( -1.128608923884513837, -0.5023911411419708095, 0.1820866141732285504 ) ) ;
#30270=CARTESIAN_POINT ( 'NONE',  ( -1.410761154855641575, -0.3162353388693409650, -0.4822834645669289433 ) ) ;
#30273=CARTESIAN_POINT ( 'NONE',  ( -1.325459317585300889, -0.3690944881889765550, -0.3153832671262227771 ) ) ;
#30274=CARTESIAN_POINT ( 'NONE',  ( -1.095800524934382292, -0.05778040916215522460, 0.4822834645669289988 ) ) ;
#30275=CARTESIAN_POINT ( 'NONE',  ( -0.4265091863517051496, 0.2952755905511810774, -0.1292274648535930714 ) ) ;
#30276=CARTESIAN_POINT ( 'NONE',  ( -1.082677165354329896, -0.5400638737290845981, -0.3530559997133363437 ) ) ;
#30279=CARTESIAN_POINT ( 'NONE',  ( 0.8136482939632553313, -0.6046776061558809534, -0.2411417322834644161 ) ) ;
#30280=CARTESIAN_POINT ( 'NONE',  ( 0.4199475065616805614, 0.2306618581243848609, 0.2411417322834645549 ) ) ;
#30283=CARTESIAN_POINT ( 'NONE',  ( 1.227034120734908917, -0.5511811023622046335, 0.09757992244046803654 ) ) ;
#30286=CARTESIAN_POINT ( 'NONE',  ( -0.8989501312335946848, -0.5511811023622046335, 0.09757992244046803654 ) ) ;
#30288=ORIENTED_EDGE ( 'NONE', *, *, #68572, .T. ) ;
#30289=CARTESIAN_POINT ( 'NONE',  ( 0.3215223097112867578, -0.05778040916215522460, 0.4822834645669289988 ) ) ;
#30290=CARTESIAN_POINT ( 'NONE',  ( -0.3477690288713905509, -0.6692913385826771977, 0.1292274648535927661 ) ) ;
#30291=CARTESIAN_POINT ( 'NONE',  ( -0.9908136482939626788, 0.2952755905511811885, 0.1292274648535926551 ) ) ;
#30292=CARTESIAN_POINT ( 'NONE',  ( 1.141732283464567788, -0.6692913385826771977, 8.415575281601705876E-17 ) ) ;
#30293=CARTESIAN_POINT ( 'NONE',  ( -1.128608923884513837, 0.1283753931104746893, -0.1820866141732285504 ) ) ;
#30295=CARTESIAN_POINT ( 'NONE',  ( 0.1181102362204730916, 0.2952755905511811885, 0.000000000000000000 ) ) ;
#30296=CARTESIAN_POINT ( 'NONE',  ( -1.272965879265091305, 0.05413385826771626580, -0.4176697321401330321 ) ) ;
#30298=CARTESIAN_POINT ( 'NONE',  ( -1.476377952755905110, 0.1660481256975885056, 0.3530559997133364547 ) ) ;
#30301=CARTESIAN_POINT ( 'NONE',  ( 0.7742782152230979209, -0.004921259842519870586, -0.3153832671262229437 ) ) ;
#30304=CARTESIAN_POINT ( 'NONE',  ( -1.036745406824146176, -0.4281496062992124485, 0.4176697321401328655 ) ) ;
#30306=CARTESIAN_POINT ( 'NONE',  ( 0.03280839895013198948, 0.1771653543307087630, 0.09757992244046791164 ) ) ;
#30307=CARTESIAN_POINT ( 'NONE',  ( -1.437007874015747477, -0.5400638737290844871, 0.3530559997133364547 ) ) ;
#30308=CARTESIAN_POINT ( 'NONE',  ( 0.3608923884514443348, 0.2952755905511810774, -0.1292274648535930714 ) ) ;
#30309=CARTESIAN_POINT ( 'NONE',  ( 0.3674540682414705883, 0.2306618581243847221, -0.2411417322834647770 ) ) ;
#30310=CARTESIAN_POINT ( 'NONE',  ( -0.7217847769028863381, 0.05413385826771626580, -0.4176697321401330321 ) ) ;
#30312=CARTESIAN_POINT ( 'NONE',  ( -0.7611548556430438595, -0.6046776061558809534, -0.2411417322834644161 ) ) ;
#30314=CARTESIAN_POINT ( 'NONE',  ( 1.292650918635171564, 0.1771653543307087630, 0.09757992244046791164 ) ) ;
#30315=CARTESIAN_POINT ( 'NONE',  ( -0.9251968503937002541, -0.5400638737290845981, -0.3530559997133363437 ) ) ;
#30316=CARTESIAN_POINT ( 'NONE',  ( 0.9514435695538062676, -0.3162353388693409650, -0.4822834645669289433 ) ) ;
#30317=CARTESIAN_POINT ( 'NONE',  ( 1.286089238845145033, -0.6046776061558809534, -0.2411417322834644161 ) ) ;
#30319=CARTESIAN_POINT ( 'NONE',  ( -1.509186351706035767, 0.05413385826771626580, -0.4176697321401330321 ) ) ;
#30321=CARTESIAN_POINT ( 'NONE',  ( 0.2690288713910767848, -0.6692913385826773087, -0.1292274648535924053 ) ) ;
#30325=CARTESIAN_POINT ( 'NONE',  ( -1.391076115485563314, -0.5023911411419708095, -0.1820866141732282451 ) ) ;
#30326=CARTESIAN_POINT ( 'NONE',  ( 0.4396325459317593221, 0.1771653543307087075, -0.09757992244046823083 ) ) ;
#30327=CARTESIAN_POINT ( 'NONE',  ( 0.8661417322834652488, -0.1870078740157480879, -0.4822834645669291653 ) ) ;
#30329=CARTESIAN_POINT ( 'NONE',  ( 0.8464566929133866546, -0.4536011799217367080, 0.2665933059059888421 ) ) ;
#30330=CARTESIAN_POINT ( 'NONE',  ( 0.2690288713910767848, -0.6692913385826773087, -0.1292274648535924053 ) ) ;
#30333=CARTESIAN_POINT ( 'NONE',  ( -0.9055118110236215490, 0.2952755905511811885, 0.000000000000000000 ) ) ;
#30335=CARTESIAN_POINT ( 'NONE',  ( 0.8595800524934390507, -0.08942795157528024563, -0.3641732283464568787 ) ) ;
#30336=CARTESIAN_POINT ( 'NONE',  ( 0.1115485564304467270, -0.6692913385826773087, -0.1292274648535924053 ) ) ;
#30338=CARTESIAN_POINT ( 'NONE',  ( -0.3937007874015740483, -0.1870078740157480879, -0.4822834645669291653 ) ) ;
#30339=CARTESIAN_POINT ( 'NONE',  ( 0.07217847769028949700, -0.2845877964562159024, 0.3641732283464567677 ) ) ;
#30341=CARTESIAN_POINT ( 'NONE',  ( 0.08530183727034192087, -0.08942795157527998196, 0.3641732283464567121 ) ) ;
#30342=CARTESIAN_POINT ( 'NONE',  ( 0.7217847769028878924, -0.3690944881889765550, -0.3153832671262227771 ) ) ;
#30345=CARTESIAN_POINT ( 'NONE',  ( 0.3215223097112867578, -0.3162353388693409650, -0.4822834645669289433 ) ) ;
#30347=CARTESIAN_POINT ( 'NONE',  ( 1.305774278215223960, -0.5511811023622046335, 0.09757992244046803654 ) ) ;
#30348=CARTESIAN_POINT ( 'NONE',  ( 0.1674892343164159914, -2.191421614605370878E-15, 0.4445507791589071167 ) ) ;
#30349=CARTESIAN_POINT ( 'NONE',  ( -0.4593175853018366950, -0.004921259842519576551, 0.3153832671262227771 ) ) ;
#30350=CARTESIAN_POINT ( 'NONE',  ( -0.2624671916010490880, 0.1283753931104746893, -0.1820866141732285504 ) ) ;
#30351=CARTESIAN_POINT ( 'NONE',  ( -0.2887139107611542133, -0.6046776061558809534, -0.2411417322834644161 ) ) ;
#30352=CARTESIAN_POINT ( 'NONE',  ( 0.8136482939632553313, -0.5023911411419708095, -0.1820866141732282451 ) ) ;
#30354=CARTESIAN_POINT ( 'NONE',  ( 1.292650918635171564, 0.1771653543307087630, 0.09757992244046791164 ) ) ;
#30355=CARTESIAN_POINT ( 'NONE',  ( 0.006561679790026889343, -0.3162353388693409650, -0.4822834645669289433 ) ) ;
#30356=CARTESIAN_POINT ( 'NONE',  ( 1.115485564304462551, -0.4281496062992127816, -0.4176697321401328100 ) ) ;
#30358=CARTESIAN_POINT ( 'NONE',  ( 0.2690288713910767848, -0.6692913385826773087, -0.1292274648535924053 ) ) ;
#30361=CARTESIAN_POINT ( 'NONE',  ( 1.364829396325460076, 0.2306618581243848609, 0.2411417322834645549 ) ) ;
#30363=CARTESIAN_POINT ( 'NONE',  ( 0.6627296587926517768, -0.6692913385826773087, -0.1292274648535924053 ) ) ;
#30365=CARTESIAN_POINT ( 'NONE',  ( 0.8661417322834653598, -0.1870078740157479769, 0.3641732283464567677 ) ) ;
#30366=CARTESIAN_POINT ( 'NONE',  ( 1.148293963254593875, -0.6692913385826771977, 0.1292274648535927661 ) ) ;
#30367=CARTESIAN_POINT ( 'NONE',  ( -0.01968503937007793844, -0.4536011799217367080, 0.2665933059059888421 ) ) ;
#30368=CARTESIAN_POINT ( 'NONE',  ( -0.3477690288713902178, 0.2952755905511810774, -0.1292274648535930714 ) ) ;
#30369=CARTESIAN_POINT ( 'NONE',  ( 0.2099737532808405305, 0.2306618581243847221, -0.2411417322834647770 ) ) ;
#30370=CARTESIAN_POINT ( 'NONE',  ( -0.6889763779527552368, 0.1660481256975885056, 0.3530559997133364547 ) ) ;
#30371=CARTESIAN_POINT ( 'NONE',  ( -0.1771653543307080136, -0.4536011799217367080, 0.2665933059059888421 ) ) ;
#30372=CARTESIAN_POINT ( 'NONE',  ( 0.7545931758530188826, -0.6692913385826771977, 0.1292274648535927661 ) ) ;
#30373=CARTESIAN_POINT ( 'NONE',  ( 0.9317585301837276734, -0.004921259842519870586, -0.3153832671262229437 ) ) ;
#30374=CARTESIAN_POINT ( 'NONE',  ( 0.1902887139107617975, -0.6692913385826773087, -0.1292274648535924053 ) ) ;
#30376=DIRECTION ( 'NONE',  ( 0.000000000000000000, 1.000000000000000000, 0.000000000000000000 ) ) ;
#30378=CARTESIAN_POINT ( 'NONE',  ( 1.220472440944879722, 0.4405861044731111953, 0.5309055118110233007 ) ) ;
#30380=CARTESIAN_POINT ( 'NONE',  ( -1.207349081364828436, -0.6046776061558807314, 0.2411417322834647770 ) ) ;
#30382=CARTESIAN_POINT ( 'NONE',  ( -0.4724409448818890911, -0.1870078740157479769, 0.4822834645669291653 ) ) ;
#30386=CARTESIAN_POINT ( 'NONE',  ( 0.1509186351706045259, -0.08942795157528024563, -0.3641732283464568787 ) ) ;
#30388=CARTESIAN_POINT ( 'NONE',  ( 0.6036745406824153282, -0.6046776061558807314, 0.2411417322834647770 ) ) ;
#30392=CARTESIAN_POINT ( 'NONE',  ( 1.122047244094488860, -0.5400638737290845981, -0.3530559997133363437 ) ) ;
#30393=CARTESIAN_POINT ( 'NONE',  ( 1.325459317585302665, -0.004921259842519870586, -0.3153832671262229437 ) ) ;
#30394=CARTESIAN_POINT ( 'NONE',  ( 0.1509186351706045259, -0.05778040916215560624, -0.4822834645669293319 ) ) ;
#30396=CARTESIAN_POINT ( 'NONE',  ( -0.2099737532808391705, 0.2306618581243848609, 0.2411417322834645549 ) ) ;
#30397=( BOUNDED_CURVE ( )  B_SPLINE_CURVE ( 3, ( #41651, #66932, #53853, #55095 ),
 .UNSPECIFIED., .F., .F. ) 
 B_SPLINE_CURVE_WITH_KNOTS ( ( 4, 4 ),
 ( 3.539787554096436306, 4.423914789137159964 ),
 .UNSPECIFIED. ) 
 CURVE ( )  GEOMETRIC_REPRESENTATION_ITEM ( )  RATIONAL_B_SPLINE_CURVE ( ( 1.000000000000000000, 0.9359138408343250504, 0.9359138408343250504, 1.000000000000000000 ) ) 
 REPRESENTATION_ITEM ( '' )  );
#30398=CARTESIAN_POINT ( 'NONE',  ( -1.115485564304461219, -0.3690944881889763329, 0.3153832671262228327 ) ) ;
#30399=CARTESIAN_POINT ( 'NONE',  ( 0.5446194225721792126, -0.05778040916215560624, -0.4822834645669293319 ) ) ;
#30400=CARTESIAN_POINT ( 'NONE',  ( -0.6758530183727028406, -0.6692913385826773087, -0.1292274648535924053 ) ) ;
#30401=CARTESIAN_POINT ( 'NONE',  ( 1.633858267716535639, -0.5400638737290844871, 0.3530559997133364547 ) ) ;
#30405=CARTESIAN_POINT ( 'NONE',  ( 0.2230971128608932319, -0.4281496062992124485, 0.4176697321401328655 ) ) ;
#30406=CARTESIAN_POINT ( 'NONE',  ( -0.4921259842519677963, -0.5400638737290844871, 0.3530559997133364547 ) ) ;
#30407=CARTESIAN_POINT ( 'NONE',  ( -1.509186351706035767, -0.4281496062992124485, 0.4176697321401328655 ) ) ;
#30409=CARTESIAN_POINT ( 'NONE',  ( 0.5118110236220478892, 0.2952755905511811885, 0.000000000000000000 ) ) ;
#30410=CARTESIAN_POINT ( 'NONE',  ( 0.5839895013123367340, 0.2952755905511811885, 0.1292274648535926551 ) ) ;
#30412=CARTESIAN_POINT ( 'NONE',  ( -0.5971128608923877978, 0.2952755905511811885, 0.1292274648535926551 ) ) ;
#30413=CARTESIAN_POINT ( 'NONE',  ( 0.02624671916010564918, -0.6046776061558809534, -0.2411417322834644161 ) ) ;
#30414=CARTESIAN_POINT ( 'NONE',  ( -0.2427821522309703550, -0.3162353388693405765, 0.4822834645669290543 ) ) ;
#30415=CARTESIAN_POINT ( 'NONE',  ( 0.1181102362204730916, 0.1771653543307087630, 0.000000000000000000 ) ) ;
#30416=CARTESIAN_POINT ( 'NONE',  ( -1.673228346456691717, 0.1660481256975883668, -0.3530559997133364547 ) ) ;
#30418=CARTESIAN_POINT ( 'NONE',  ( 0.3346456692913390985, 0.1660481256975885056, 0.3530559997133364547 ) ) ;
#30420=CARTESIAN_POINT ( 'NONE',  ( -1.614173228346455824, 0.2952755905511811885, 0.000000000000000000 ) ) ;
#30425=CARTESIAN_POINT ( 'NONE',  ( 0.7349081364829403995, 0.2306618581243848609, 0.2411417322834645549 ) ) ;
#30426=CARTESIAN_POINT ( 'NONE',  ( 0.1640419947506569498, -0.08942795157527998196, 0.3641732283464567121 ) ) ;
#30428=VECTOR ( 'NONE', #72239, 39.37007874015748854 ) ;
#30433=CARTESIAN_POINT ( 'NONE',  ( 0.7193605937323486188, 1.521610601467410833E-15, 0.4118484887281966822 ) ) ;
#30435=CARTESIAN_POINT ( 'NONE',  ( 0.6233595800524939223, -0.3162353388693405765, 0.4822834645669290543 ) ) ;
#30436=CARTESIAN_POINT ( 'NONE',  ( -1.187664041994749731, -0.3162353388693405765, 0.4822834645669290543 ) ) ;
#30437=CARTESIAN_POINT ( 'NONE',  ( -1.200787401574802349, 0.1660481256975883668, -0.3530559997133364547 ) ) ;
#30438=CARTESIAN_POINT ( 'NONE',  ( 0.8595800524934390507, -0.05778040916215560624, -0.4822834645669293319 ) ) ;
#30439=CARTESIAN_POINT ( 'NONE',  ( 1.272965879265092637, 0.05413385826771666132, 0.4176697321401328100 ) ) ;
#30440=CARTESIAN_POINT ( 'NONE',  ( 1.581364829396326277, -0.2845877964562161244, -0.3641732283464567121 ) ) ;
#30441=CARTESIAN_POINT ( 'NONE',  ( 1.423884514435696413, -0.2845877964562161244, -0.3641732283464567121 ) ) ;
#30442=CARTESIAN_POINT ( 'NONE',  ( -0.7480314960629914633, -0.6692913385826771977, 8.415575281601705876E-17 ) ) ;
#30444=CARTESIAN_POINT ( 'NONE',  ( 1.397637795275591177, 0.1660481256975883668, -0.3530559997133364547 ) ) ;
#30446=CARTESIAN_POINT ( 'NONE',  ( -0.03937007874015669567, 0.2952755905511811885, 0.000000000000000000 ) ) ;
#30448=CARTESIAN_POINT ( 'NONE',  ( 1.279527559055118724, -0.5400638737290845981, -0.3530559997133363437 ) ) ;
#30449=CARTESIAN_POINT ( 'NONE',  ( -1.603475055217291612, 1.543447618314657932, -0.04573490813648263542 ) ) ;
#30450=CARTESIAN_POINT ( 'NONE',  ( -0.9908136482939626788, -0.5511811023622048555, -0.09757992244046775898 ) ) ;
#30451=CARTESIAN_POINT ( 'NONE',  ( 0.5249343832021005074, -0.6046776061558807314, 0.2411417322834647770 ) ) ;
#30452=CARTESIAN_POINT ( 'NONE',  ( 0.8727034120734912248, -0.2845877964562161244, -0.3641732283464567121 ) ) ;
#30454=CARTESIAN_POINT ( 'NONE',  ( -1.049868766404198794, 0.1283753931104746893, -0.1820866141732285504 ) ) ;
#30455=CARTESIAN_POINT ( 'NONE',  ( 0.9186351706036752773, 0.2306618581243847221, -0.2411417322834647770 ) ) ;
#30456=CARTESIAN_POINT ( 'NONE',  ( -0.4986876640419939388, 0.2306618581243847221, -0.2411417322834647770 ) ) ;
#30457=CARTESIAN_POINT ( 'NONE',  ( -0.5183727034120726440, -0.5511811023622048555, -0.09757992244046775898 ) ) ;
#30458=CARTESIAN_POINT ( 'NONE',  ( -0.4330708661417315697, 0.2952755905511811885, 0.000000000000000000 ) ) ;
#30459=CARTESIAN_POINT ( 'NONE',  ( -1.509186351706035767, -0.3690944881889763329, 0.3153832671262228327 ) ) ;
#30461=CARTESIAN_POINT ( 'NONE',  ( -0.8727034120734901146, -0.05778040916215560624, -0.4822834645669293319 ) ) ;
#30462=CARTESIAN_POINT ( 'NONE',  ( 1.279527559055118724, -0.5400638737290845981, -0.3530559997133363437 ) ) ;
#30464=CARTESIAN_POINT ( 'NONE',  ( -1.089238845144356427, -0.3690944881889765550, -0.3153832671262227771 ) ) ;
#30466=CARTESIAN_POINT ( 'NONE',  ( 1.515748031496063186, -0.5400638737290845981, -0.3530559997133363437 ) ) ;
#30468=CARTESIAN_POINT ( 'NONE',  ( -1.187664041994750175, -0.05778040916215560624, -0.4822834645669293319 ) ) ;
#30469=CARTESIAN_POINT ( 'NONE',  ( -1.456692913385826182, 0.1771653543307087630, 0.000000000000000000 ) ) ;
#30470=CARTESIAN_POINT ( 'NONE',  ( -0.8070866141732276899, -0.4536011799217367080, 0.2665933059059888421 ) ) ;
#30471=CARTESIAN_POINT ( 'NONE',  ( -0.5249343832020990641, 0.1539470093639523085, 0.1968503937007873850 ) ) ;
#30472=CARTESIAN_POINT ( 'NONE',  ( -0.5183727034120726440, 0.2952755905511811885, 0.1292274648535926551 ) ) ;
#30473=CARTESIAN_POINT ( 'NONE',  ( -0.03280839895013062252, 0.1771653543307087075, -0.09757992244046823083 ) ) ;
#30474=CARTESIAN_POINT ( 'NONE',  ( -1.259842519685038686, -0.1870078740157479769, 0.3641732283464567677 ) ) ;
#30475=CARTESIAN_POINT ( 'NONE',  ( -1.653543307086613234, -0.1870078740157480879, -0.4822834645669291653 ) ) ;
#30476=CARTESIAN_POINT ( 'NONE',  ( 1.148293963254593653, 0.1771653543307087075, -0.09757992244046823083 ) ) ;
#30477=CARTESIAN_POINT ( 'NONE',  ( 1.089238845144357759, 0.05413385826771626580, -0.4176697321401330321 ) ) ;
#30479=CARTESIAN_POINT ( 'NONE',  ( 0.4461942257217856311, 0.1283753931104746893, -0.1820866141732285504 ) ) ;
#30480=CARTESIAN_POINT ( 'NONE',  ( 0.3149606299212606708, -0.1870078740157480879, -0.4822834645669291653 ) ) ;
#30481=CARTESIAN_POINT ( 'NONE',  ( 1.043307086614173818, -0.4536011799217368745, -0.2665933059059886201 ) ) ;
#30483=CARTESIAN_POINT ( 'NONE',  ( -1.089238845144356427, -0.4281496062992127816, -0.4176697321401328100 ) ) ;
#30485=CARTESIAN_POINT ( 'NONE',  ( -0.8595800524934373854, -0.05778040916215522460, 0.4822834645669289988 ) ) ;
#30486=CARTESIAN_POINT ( 'NONE',  ( 0.03280839895013198948, 0.2952755905511811885, 0.1292274648535926551 ) ) ;
#30489=CARTESIAN_POINT ( 'NONE',  ( 0.5643044619422579178, -0.4281496062992127816, -0.4176697321401328100 ) ) ;
#30490=CARTESIAN_POINT ( 'NONE',  ( -1.732283464566928277, -0.1870078740157479769, 0.4822834645669291653 ) ) ;
#30493=CARTESIAN_POINT ( 'NONE',  ( 0.09842519685039434474, 0.1660481256975885056, 0.3530559997133364547 ) ) ;
#30494=CARTESIAN_POINT ( 'NONE',  ( 0.6561679790026253567, 0.2306618581243848609, 0.2411417322834645549 ) ) ;
#30500=CARTESIAN_POINT ( 'NONE',  ( -0.5511811023622041894, -0.1870078740157480601, -0.3641732283464567677 ) ) ;
#30501=CARTESIAN_POINT ( 'NONE',  ( -0.9120734908136475250, 0.2952755905511811885, 0.1292274648535926551 ) ) ;
#30502=CARTESIAN_POINT ( 'NONE',  ( 0.5249343832021003964, 0.2306618581243847221, -0.2411417322834647770 ) ) ;
#30505=CARTESIAN_POINT ( 'NONE',  ( 1.036745406824147731, 0.05413385826771666132, 0.4176697321401328100 ) ) ;
#30506=CARTESIAN_POINT ( 'NONE',  ( -1.430446194225720724, 0.05413385826771626580, -0.4176697321401330321 ) ) ;
#30507=CARTESIAN_POINT ( 'NONE',  ( 1.279527559055118724, 0.1660481256975885056, 0.3530559997133364547 ) ) ;
#30511=CARTESIAN_POINT ( 'NONE',  ( 0.8398950131233602345, 0.2306618581243847221, -0.2411417322834647770 ) ) ;
#30512=CARTESIAN_POINT ( 'NONE',  ( 0.4461942257217855201, -0.6046776061558807314, 0.2411417322834647770 ) ) ;
#30513=CARTESIAN_POINT ( 'NONE',  ( 1.148293963254593653, 0.1771653543307087075, -0.09757992244046823083 ) ) ;
#30514=CARTESIAN_POINT ( 'NONE',  ( 1.679790026246720025, 0.2306618581243848609, 0.2411417322834645549 ) ) ;
#30515=CARTESIAN_POINT ( 'NONE',  ( -1.476377952755905110, 0.1660481256975885056, 0.3530559997133364547 ) ) ;
#30518=CARTESIAN_POINT ( 'NONE',  ( 0.6758530183727039509, -0.6692913385826771977, 0.1292274648535927661 ) ) ;
#30519=CARTESIAN_POINT ( 'NONE',  ( 1.443569553805774897, -0.5023911411419708095, -0.1820866141732282451 ) ) ;
#30520=CARTESIAN_POINT ( 'NONE',  ( -0.3937007874015740483, -0.1870078740157480879, -0.4822834645669291653 ) ) ;
#30521=CARTESIAN_POINT ( 'NONE',  ( -0.4855643044619415427, -0.4281496062992124485, 0.4176697321401328655 ) ) ;
#30522=CARTESIAN_POINT ( 'NONE',  ( -1.476377952755905110, 0.1660481256975885056, 0.3530559997133364547 ) ) ;
#30526=CARTESIAN_POINT ( 'NONE',  ( -1.515748031496062076, -0.4536011799217367080, 0.2665933059059888421 ) ) ;
#30530=CARTESIAN_POINT ( 'NONE',  ( -0.01312335958005186529, 0.009842519685039147898, -0.3409548833797004797 ) ) ;
#30531=CARTESIAN_POINT ( 'NONE',  ( 1.489501312335958172, -0.08942795157528024563, -0.3641732283464568787 ) ) ;
#30533=CARTESIAN_POINT ( 'NONE',  ( 1.627296587926509996, -0.5023911411419708095, 0.1820866141732285504 ) ) ;
#30538=CARTESIAN_POINT ( 'NONE',  ( -0.7742782152230962556, -0.3690944881889765550, -0.3153832671262227771 ) ) ;
#30539=CARTESIAN_POINT ( 'NONE',  ( -0.9973753280839886548, -0.5023911411419708095, -0.1820866141732282451 ) ) ;
#30540=CARTESIAN_POINT ( 'NONE',  ( 0.5643044619422579178, -0.4281496062992127816, -0.4176697321401328100 ) ) ;
#30541=CARTESIAN_POINT ( 'NONE',  ( -1.292650918635170010, 0.2952755905511810774, -0.1292274648535930714 ) ) ;
#30543=ORIENTED_EDGE ( 'NONE', *, *, #73157, .F. ) ;
#30544=CARTESIAN_POINT ( 'NONE',  ( 1.345144356955381593, -0.3162353388693409650, -0.4822834645669289433 ) ) ;
#30549=CARTESIAN_POINT ( 'NONE',  ( -0.5971128608923877978, -0.5511811023622048555, -0.09757992244046775898 ) ) ;
#30552=CARTESIAN_POINT ( 'NONE',  ( -1.069553805774277722, -0.6692913385826773087, -0.1292274648535924053 ) ) ;
#30553=CARTESIAN_POINT ( 'NONE',  ( 1.069553805774278832, 0.2952755905511810774, -0.1292274648535930714 ) ) ;
#30556=CARTESIAN_POINT ( 'NONE',  ( 0.6824146981627303710, 0.1539470093639521697, -0.1968503937007875793 ) ) ;
#30557=CARTESIAN_POINT ( 'NONE',  ( 1.660104986876641320, -0.05778040916215522460, 0.4822834645669289988 ) ) ;
#30558=CARTESIAN_POINT ( 'NONE',  ( -1.351706036745406347, 0.05413385826771626580, -0.4176697321401330321 ) ) ;
#30560=CARTESIAN_POINT ( 'NONE',  ( 0.1640419947506569498, -0.08942795157527998196, 0.3641732283464567121 ) ) ;
#30562=CARTESIAN_POINT ( 'NONE',  ( -0.1968503937007867743, 0.1771653543307087630, 0.000000000000000000 ) ) ;
#30563=CARTESIAN_POINT ( 'NONE',  ( 0.4133858267716541968, -0.4536011799217368745, -0.2665933059059886201 ) ) ;
#30564=EDGE_CURVE ( 'NONE', #39863, #57436, #81138, .T. ) ;
#30565=CARTESIAN_POINT ( 'NONE',  ( 0.5708661417322841158, -0.5400638737290845981, -0.3530559997133363437 ) ) ;
#30566=CARTESIAN_POINT ( 'NONE',  ( -0.9186351706036736120, -0.5023911411419708095, -0.1820866141732282451 ) ) ;
#30568=CARTESIAN_POINT ( 'NONE',  ( 1.489501312335958172, -0.05778040916215560624, -0.4822834645669293319 ) ) ;
#30569=CARTESIAN_POINT ( 'NONE',  ( -1.089238845144356427, -0.4281496062992127816, -0.4176697321401328100 ) ) ;
#30571=CARTESIAN_POINT ( 'NONE',  ( 0.04593175853018440641, 0.2952755905511810774, -0.1292274648535930714 ) ) ;
#30572=CARTESIAN_POINT ( 'NONE',  ( -0.7152230971128602510, -0.3162353388693405765, 0.4822834645669290543 ) ) ;
#30573=CARTESIAN_POINT ( 'NONE',  ( 1.240157480314961314, 0.07958543189024071263, -0.2665933059059888421 ) ) ;
#30574=CARTESIAN_POINT ( 'NONE',  ( -0.05905511811023545637, -0.4536011799217368745, -0.2665933059059886201 ) ) ;
#30575=CARTESIAN_POINT ( 'NONE',  ( -0.3215223097112853146, -0.3162353388693405765, 0.4822834645669290543 ) ) ;
#30576=CARTESIAN_POINT ( 'NONE',  ( -1.089238845144356427, -0.4281496062992127816, -0.4176697321401328100 ) ) ;
#30577=CARTESIAN_POINT ( 'NONE',  ( -1.614173228346457378, 2.157411728916712068, 0.1372047244094476981 ) ) ;
#30578=CARTESIAN_POINT ( 'NONE',  ( -1.012125901091927904, 5.991678263669262536E-15, 0.3791483426435162674 ) ) ;
#30579=CARTESIAN_POINT ( 'NONE',  ( -0.1640419947506553400, -0.05778040916215560624, -0.4822834645669293319 ) ) ;
#30580=VERTEX_POINT ( 'NONE', #47045 ) ;
#30582=CARTESIAN_POINT ( 'NONE',  ( 1.305774278215223960, 0.2952755905511810774, -0.1292274648535930714 ) ) ;
#30583=CARTESIAN_POINT ( 'NONE',  ( -0.6299212598425188991, -0.1870078740157479769, 0.3641732283464567677 ) ) ;
#30584=CARTESIAN_POINT ( 'NONE',  ( -0.6889763779527552368, -0.5400638737290845981, -0.3530559997133363437 ) ) ;
#30585=CARTESIAN_POINT ( 'NONE',  ( 1.430446194225722500, -0.4281496062992127816, -0.4176697321401328100 ) ) ;
#30586=CARTESIAN_POINT ( 'NONE',  ( 1.036745406824147731, 0.05413385826771666132, 0.4176697321401328100 ) ) ;
#30588=CARTESIAN_POINT ( 'NONE',  ( -0.9514435695538050464, -0.2845877964562159024, 0.3641732283464567677 ) ) ;
#30593=CARTESIAN_POINT ( 'NONE',  ( 0.9842519685039378130, -0.5511811023622047445, 6.969142054262312111E-17 ) ) ;
#30594=CARTESIAN_POINT ( 'NONE',  ( 0.6299212598425204535, -0.1870078740157479769, 0.3641732283464567677 ) ) ;
#30595=CARTESIAN_POINT ( 'NONE',  ( 0.3280839895013130669, 0.05413385826771666132, 0.4176697321401328100 ) ) ;
#30598=CARTESIAN_POINT ( 'NONE',  ( 0.9711286089238851948, -0.5023911411419708095, -0.1820866141732282451 ) ) ;
#30599=CARTESIAN_POINT ( 'NONE',  ( -0.2230971128608915943, 0.05413385826771666132, 0.4176697321401328100 ) ) ;
#30600=CARTESIAN_POINT ( 'NONE',  ( -0.8595800524934373854, -0.05778040916215522460, 0.4822834645669289988 ) ) ;
#30601=CARTESIAN_POINT ( 'NONE',  ( 1.095800524934383846, -0.05778040916215560624, -0.4822834645669293319 ) ) ;
#30605=CARTESIAN_POINT ( 'NONE',  ( -0.07217847769028813698, -0.2845877964562161244, -0.3641732283464567121 ) ) ;
#30607=ORIENTED_EDGE ( 'NONE', *, *, #69950, .F. ) ;
#30610=CARTESIAN_POINT ( 'NONE',  ( -0.7086614173228339419, -0.1870078740157480879, -0.4822834645669291653 ) ) ;
#30611=CARTESIAN_POINT ( 'NONE',  ( -0.2230971128608915943, 0.05413385826771666132, 0.4176697321401328100 ) ) ;
#30612=CARTESIAN_POINT ( 'NONE',  ( -0.5314960629921250401, 0.1660481256975885056, 0.3530559997133364547 ) ) ;
#30613=CARTESIAN_POINT ( 'NONE',  ( 0.5511811023622055217, -0.1870078740157479769, 0.4822834645669291653 ) ) ;
#30615=CARTESIAN_POINT ( 'NONE',  ( -0.5118110236220466680, 0.2952755905511811885, 0.000000000000000000 ) ) ;
#30616=CARTESIAN_POINT ( 'NONE',  ( -1.476377952755905110, 0.1660481256975885056, 0.3530559997133364547 ) ) ;
#30617=CARTESIAN_POINT ( 'NONE',  ( -0.7217847769028863381, 0.05413385826771626580, -0.4176697321401330321 ) ) ;
#30618=CARTESIAN_POINT ( 'NONE',  ( 0.6758530183727039509, 0.2952755905511810774, -0.1292274648535930714 ) ) ;
#30620=CARTESIAN_POINT ( 'NONE',  ( -0.5052493438320203589, 0.1771653543307087075, -0.09757992244046823083 ) ) ;
#30621=ORIENTED_EDGE ( 'NONE', *, *, #78936, .T. ) ;
#30624=CARTESIAN_POINT ( 'NONE',  ( -1.482939632545930975, -0.3690944881889765550, -0.3153832671262227771 ) ) ;
#30625=CARTESIAN_POINT ( 'NONE',  ( -1.082677165354329896, -0.5400638737290845981, -0.3530559997133363437 ) ) ;
#30626=CARTESIAN_POINT ( 'NONE',  ( -0.9645669291338575535, 0.1660481256975883668, -0.3530559997133364547 ) ) ;
#30628=CARTESIAN_POINT ( 'NONE',  ( -0.5971128608923877978, 0.2952755905511811885, 0.1292274648535926551 ) ) ;
#30629=CARTESIAN_POINT ( 'NONE',  ( -0.7414698162729651543, 0.2952755905511810774, -0.1292274648535930714 ) ) ;
#30632=CARTESIAN_POINT ( 'NONE',  ( 0.7152230971128616943, -0.08942795157527998196, 0.3641732283464567121 ) ) ;
#30633=CARTESIAN_POINT ( 'NONE',  ( 1.603475055217291612, 0.4410854135902469442, 0.04573490813648272563 ) ) ;
#30635=CARTESIAN_POINT ( 'NONE',  ( 0.03937007874015806264, 0.1771653543307087630, 0.000000000000000000 ) ) ;
#30636=CARTESIAN_POINT ( 'NONE',  ( -0.2821522309711278487, -0.6692913385826773087, -0.1292274648535924053 ) ) ;
#30638=CARTESIAN_POINT ( 'NONE',  ( -0.1049868766404193215, -0.6046776061558807314, 0.2411417322834647770 ) ) ;
#30645=CARTESIAN_POINT ( 'NONE',  ( -1.227034120734907585, 0.1771653543307087630, 0.09757992244046791164 ) ) ;
#30646=CARTESIAN_POINT ( 'NONE',  ( -1.036745406824146176, 0.05413385826771626580, -0.4176697321401330321 ) ) ;
#30651=CARTESIAN_POINT ( 'NONE',  ( 1.430446194225722500, -0.4281496062992127816, -0.4176697321401328100 ) ) ;
#30652=CARTESIAN_POINT ( 'NONE',  ( 0.5708661417322841158, -0.5400638737290845981, -0.3530559997133363437 ) ) ;
#30653=CARTESIAN_POINT ( 'NONE',  ( 0.3674540682414705883, -0.6046776061558807314, 0.2411417322834647770 ) ) ;
#30654=CARTESIAN_POINT ( 'NONE',  ( -1.253280839895012377, -0.2845877964562161244, -0.3641732283464567121 ) ) ;
#30655=CARTESIAN_POINT ( 'NONE',  ( -0.4855643044619415427, -0.4281496062992124485, 0.4176697321401328655 ) ) ;
#30657=CARTESIAN_POINT ( 'NONE',  ( -0.7874015748031489847, -0.1870078740157479769, 0.4822834645669291653 ) ) ;
#30660=CARTESIAN_POINT ( 'NONE',  ( 1.391076115485564868, -0.5023911411419708095, 0.1820866141732285504 ) ) ;
#30661=CARTESIAN_POINT ( 'NONE',  ( -0.3412073490813641308, -0.5023911411419708095, 0.1820866141732285504 ) ) ;
#30662=CARTESIAN_POINT ( 'NONE',  ( 1.043307086614173818, 0.07958543189024085140, 0.2665933059059887866 ) ) ;
#30663=CARTESIAN_POINT ( 'NONE',  ( -1.463254593175852492, -0.6692913385826773087, -0.1292274648535924053 ) ) ;
#30664=CARTESIAN_POINT ( 'NONE',  ( -0.9383202099737524282, -0.2845877964562161244, -0.3641732283464567121 ) ) ;
#30665=CARTESIAN_POINT ( 'NONE',  ( 0.1463826306659141430, 2.110655687203366066E-15, -0.3954974714151459625 ) ) ;
#30666=CARTESIAN_POINT ( 'NONE',  ( 0.4068241469816281097, -0.004921259842519576551, 0.3153832671262227771 ) ) ;
#30667=CARTESIAN_POINT ( 'NONE',  ( -0.2624671916010490880, -0.6046776061558807314, 0.2411417322834647770 ) ) ;
#30670=CARTESIAN_POINT ( 'NONE',  ( -0.2238009295390064879, -2.294479370626195693E-15, 0.3464511005275217603 ) ) ;
#30671=CARTESIAN_POINT ( 'NONE',  ( 0.1246719160104994284, 0.1771653543307087075, -0.09757992244046823083 ) ) ;
#30673=CARTESIAN_POINT ( 'NONE',  ( 0.9251968503937015864, 0.1660481256975883668, -0.3530559997133364547 ) ) ;
#30674=LINE ( 'NONE', #43278, #23633 ) ;
#30675=CARTESIAN_POINT ( 'NONE',  ( 1.496062992125984703, -0.1870078740157480601, -0.3641732283464567677 ) ) ;
#30676=CARTESIAN_POINT ( 'NONE',  ( -1.128608923884513837, -0.6046776061558807314, 0.2411417322834647770 ) ) ;
#30677=CARTESIAN_POINT ( 'NONE',  ( -0.1049868766404193215, -0.5023911411419708095, 0.1820866141732285504 ) ) ;
#30678=CARTESIAN_POINT ( 'NONE',  ( -0.7233796917120556280, 1.992010844874188447, 0.5048038503170210189 ) ) ;
#30679=CARTESIAN_POINT ( 'NONE',  ( 0.2427821522309716595, -0.2845877964562161244, -0.3641732283464567121 ) ) ;
#30680=CARTESIAN_POINT ( 'NONE',  ( -1.338582677165353729, -0.1870078740157480879, -0.4822834645669291653 ) ) ;
#30681=CARTESIAN_POINT ( 'NONE',  ( -0.4396325459317577122, -0.6692913385826773087, -0.1292274648535924053 ) ) ;
#30684=CARTESIAN_POINT ( 'NONE',  ( 0.5052493438320215802, 0.1771653543307087630, 0.09757992244046791164 ) ) ;
#30685=CARTESIAN_POINT ( 'NONE',  ( -0.3805774278215216522, 0.05413385826771666132, 0.4176697321401328100 ) ) ;
#30686=CARTESIAN_POINT ( 'NONE',  ( -0.7283464566929126471, -0.5400638737290844871, 0.3530559997133364547 ) ) ;
#30687=CARTESIAN_POINT ( 'NONE',  ( -0.9514435695538050464, -0.08942795157528024563, -0.3641732283464568787 ) ) ;
#30689=CARTESIAN_POINT ( 'NONE',  ( 0.05905511811023709395, -0.5400638737290844871, 0.3530559997133364547 ) ) ;
#30690=CARTESIAN_POINT ( 'NONE',  ( -1.259842519685038686, -0.1870078740157479769, 0.3641732283464567677 ) ) ;
#30691=CARTESIAN_POINT ( 'NONE',  ( -1.594488188976377119, 0.1660481256975883668, -0.3530559997133364547 ) ) ;
#30694=CARTESIAN_POINT ( 'NONE',  ( -1.601049868766403650, -0.5023911411419708095, 0.1820866141732285504 ) ) ;
#30695=CARTESIAN_POINT ( 'NONE',  ( -1.181102362204723644, -0.1870078740157480879, -0.4822834645669291653 ) ) ;
#30696=CARTESIAN_POINT ( 'NONE',  ( -0.9186351706036736120, 0.2306618581243848609, 0.2411417322834645549 ) ) ;
#30697=CARTESIAN_POINT ( 'NONE',  ( -1.535433070866141225, -0.6692913385826771977, 8.415575281601705876E-17 ) ) ;
#30700=CARTESIAN_POINT ( 'NONE',  ( 1.043307086614173818, 0.1660481256975885056, 0.3530559997133364547 ) ) ;
#30701=CARTESIAN_POINT ( 'NONE',  ( 0.5380577427821529035, -0.4281496062992124485, 0.4176697321401328655 ) ) ;
#30704=CARTESIAN_POINT ( 'NONE',  ( 1.122047244094488860, 0.07958543189024085140, 0.2665933059059887866 ) ) ;
#30707=VERTEX_POINT ( 'NONE', #73152 ) ;
#30708=CARTESIAN_POINT ( 'NONE',  ( -0.9580052493438311334, -0.004921259842519870586, -0.3153832671262229437 ) ) ;
#30710=ORIENTED_EDGE ( 'NONE', *, *, #63585, .T. ) ;
#30711=CARTESIAN_POINT ( 'NONE',  ( 0.4593175853018379162, -0.4281496062992124485, 0.4176697321401328655 ) ) ;
#30712=CARTESIAN_POINT ( 'NONE',  ( -0.7677165354330699465, 0.1660481256975885056, 0.3530559997133364547 ) ) ;
#30713=CARTESIAN_POINT ( 'NONE',  ( -0.9120734908136475250, -0.6692913385826773087, -0.1292274648535924053 ) ) ;
#30714=CARTESIAN_POINT ( 'NONE',  ( 0.9383202099737538715, -0.05778040916215560624, -0.4822834645669293319 ) ) ;
#30715=CARTESIAN_POINT ( 'NONE',  ( 1.581364829396326277, -0.3162353388693409650, -0.4822834645669289433 ) ) ;
#30717=CARTESIAN_POINT ( 'NONE',  ( 0.01312335958005323398, -0.4281496062992127816, -0.4176697321401328100 ) ) ;
#30718=CARTESIAN_POINT ( 'NONE',  ( -1.187664041994749731, -0.3162353388693405765, 0.4822834645669290543 ) ) ;
#30719=CARTESIAN_POINT ( 'NONE',  ( -1.614173228346457378, 1.606230626554505658, -0.1372047244094477536 ) ) ;
#30720=CARTESIAN_POINT ( 'NONE',  ( 1.535433070866142558, 0.2952755905511811885, 0.000000000000000000 ) ) ;
#30723=CARTESIAN_POINT ( 'NONE',  ( 0.6824146981627303710, -0.5023911411419708095, 0.1820866141732285504 ) ) ;
#30727=CARTESIAN_POINT ( 'NONE',  ( 0.1312335958005255154, -0.5023911411419708095, 0.1820866141732285504 ) ) ;
#30729=CARTESIAN_POINT ( 'NONE',  ( 0.4658792650918640033, -0.3162353388693405765, 0.4822834645669290543 ) ) ;
#30730=CARTESIAN_POINT ( 'NONE',  ( 0.3083989501312343062, -0.3162353388693405765, 0.4822834645669290543 ) ) ;
#30731=CARTESIAN_POINT ( 'NONE',  ( -0.5839895013123351797, 0.2952755905511810774, -0.1292274648535930714 ) ) ;
#30733=CARTESIAN_POINT ( 'NONE',  ( -1.410761154855641575, -0.3162353388693409650, -0.4822834645669289433 ) ) ;
#30735=CARTESIAN_POINT ( 'NONE',  ( 1.469816272965879911, 0.1283753931104746893, -0.1820866141732285504 ) ) ;
#30736=CARTESIAN_POINT ( 'NONE',  ( -1.056430446194224881, -0.6692913385826771977, 0.1292274648535927661 ) ) ;
#30737=CARTESIAN_POINT ( 'NONE',  ( 0.9908136482939640111, -0.6692913385826771977, 0.1292274648535927661 ) ) ;
#30738=CARTESIAN_POINT ( 'NONE',  ( 1.377952755905512472, 0.2952755905511811885, 0.000000000000000000 ) ) ;
#30740=CARTESIAN_POINT ( 'NONE',  ( -1.548556430446193399, 0.2306618581243848609, 0.2411417322834645549 ) ) ;
#30742=CARTESIAN_POINT ( 'NONE',  ( 0.4265091863517067039, -0.6692913385826773087, -0.1292274648535924053 ) ) ;
#30745=CARTESIAN_POINT ( 'NONE',  ( 1.692913385826772421, 0.2952755905511811885, 0.000000000000000000 ) ) ;
#30746=CARTESIAN_POINT ( 'NONE',  ( 0.8136482939632553313, -0.5023911411419708095, -0.1820866141732282451 ) ) ;
#30747=CARTESIAN_POINT ( 'NONE',  ( 0.7677165354330716118, -0.5400638737290844871, 0.3530559997133364547 ) ) ;
#30749=CARTESIAN_POINT ( 'NONE',  ( 0.6561679790026253567, -0.5023911411419708095, -0.1820866141732282451 ) ) ;
#30750=CARTESIAN_POINT ( 'NONE',  ( 0.3608923884514443348, 0.2952755905511810774, -0.1292274648535930714 ) ) ;
#30752=CARTESIAN_POINT ( 'NONE',  ( -0.6036745406824141069, 0.2306618581243848609, 0.2411417322834645549 ) ) ;
#30753=CARTESIAN_POINT ( 'NONE',  ( 0.2462293917967310342, -2.191421614605370878E-15, 0.4445507791589071167 ) ) ;
#30754=CARTESIAN_POINT ( 'NONE',  ( 0.8398950131233602345, 0.1283753931104746893, -0.1820866141732285504 ) ) ;
#30755=CARTESIAN_POINT ( 'NONE',  ( 0.1837270341207354329, 0.2306618581243848609, 0.2411417322834645549 ) ) ;
#30756=CARTESIAN_POINT ( 'NONE',  ( 0.1685779992553469442, -2.839693391405754848E-15, 0.3954974714151476278 ) ) ;
#30757=CARTESIAN_POINT ( 'NONE',  ( -0.1443569553805768291, 0.05413385826771666132, 0.4176697321401328100 ) ) ;
#30758=CARTESIAN_POINT ( 'NONE',  ( 0.09842519685039434474, 0.07958543189024085140, 0.2665933059059887866 ) ) ;
#30760=CARTESIAN_POINT ( 'NONE',  ( -0.1706036745406816491, -0.4281496062992124485, 0.4176697321401328655 ) ) ;
#30761=CARTESIAN_POINT ( 'NONE',  ( 0.5708661417322841158, -0.4536011799217368745, -0.2665933059059886201 ) ) ;
#30764=CARTESIAN_POINT ( 'NONE',  ( 0.2821522309711292364, 0.2952755905511810774, -0.1292274648535930714 ) ) ;
#30765=CARTESIAN_POINT ( 'NONE',  ( 1.312335958005250269, -0.5023911411419708095, 0.1820866141732285504 ) ) ;
#30766=CARTESIAN_POINT ( 'NONE',  ( 1.220472440944882386, 1.277248692536265747E-15, -0.4445507791589058955 ) ) ;
#30767=CARTESIAN_POINT ( 'NONE',  ( -0.4002624671916004129, -0.08942795157528024563, -0.3641732283464568787 ) ) ;
#30768=CARTESIAN_POINT ( 'NONE',  ( -0.9448818897637790704, -0.1870078740157479769, 0.3641732283464567677 ) ) ;
#30769=CARTESIAN_POINT ( 'NONE',  ( -0.2099737532808391705, 0.2306618581243848609, 0.2411417322834645549 ) ) ;
#30770=CARTESIAN_POINT ( 'NONE',  ( 0.1902887139107617975, 0.2952755905511811885, 0.1292274648535926551 ) ) ;
#30771=CARTESIAN_POINT ( 'NONE',  ( 0.9711286089238851948, -0.5023911411419708095, -0.1820866141732282451 ) ) ;
#30772=CARTESIAN_POINT ( 'NONE',  ( -1.719160104986876103, -0.004921259842519576551, 0.3153832671262227771 ) ) ;
#30773=CARTESIAN_POINT ( 'NONE',  ( 1.541994750656168645, -0.5511811023622046335, 0.09757992244046803654 ) ) ;
#30774=CARTESIAN_POINT ( 'NONE',  ( 0.7874015748031503170, -0.1870078740157480879, -0.4822834645669291653 ) ) ;
#30776=CARTESIAN_POINT ( 'NONE',  ( 0.03280839895013198948, 0.2952755905511811885, 0.1292274648535926551 ) ) ;
#30778=CARTESIAN_POINT ( 'NONE',  ( 1.030183727034121421, -0.05778040916215522460, 0.4822834645669289988 ) ) ;
#30779=CARTESIAN_POINT ( 'NONE',  ( 0.7349081364829403995, 0.2306618581243848609, 0.2411417322834645549 ) ) ;
#30781=CARTESIAN_POINT ( 'NONE',  ( 0.3608923884514443348, -0.5511811023622046335, 0.09757992244046803654 ) ) ;
#30782=CARTESIAN_POINT ( 'NONE',  ( 1.397637795275591177, 0.1660481256975883668, -0.3530559997133364547 ) ) ;
#30783=CARTESIAN_POINT ( 'NONE',  ( 0.1968503937007881344, 0.1771653543307087630, 0.000000000000000000 ) ) ;
#30784=CARTESIAN_POINT ( 'NONE',  ( -0.4593175853018364174, -0.4281496062992127816, -0.4176697321401328100 ) ) ;
#30785=CARTESIAN_POINT ( 'NONE',  ( 0.1968503937007881344, 0.2952755905511811885, 0.000000000000000000 ) ) ;
#30786=CARTESIAN_POINT ( 'NONE',  ( -0.8333333333333323711, 0.2952755905511811885, 0.1292274648535926551 ) ) ;
#30787=CARTESIAN_POINT ( 'NONE',  ( -0.3937007874015740483, -0.1870078740157480601, -0.3641732283464567677 ) ) ;
#30788=CARTESIAN_POINT ( 'NONE',  ( 0.5577427821522314977, -0.3162353388693409650, -0.4822834645669289433 ) ) ;
#30789=CARTESIAN_POINT ( 'NONE',  ( 0.9120734908136490793, 0.1771653543307087075, -0.09757992244046823083 ) ) ;
#30790=CARTESIAN_POINT ( 'NONE',  ( -0.2559055118110227234, -0.5400638737290844871, 0.3530559997133364547 ) ) ;
#30792=CARTESIAN_POINT ( 'NONE',  ( 1.515748031496063408, 0.1660481256975885056, 0.3530559997133364547 ) ) ;
#30794=CARTESIAN_POINT ( 'NONE',  ( -1.069553805774277722, -0.6692913385826773087, -0.1292274648535924053 ) ) ;
#30795=CARTESIAN_POINT ( 'NONE',  ( -0.9514435695538050464, -0.3162353388693405765, 0.4822834645669290543 ) ) ;
#30800=CARTESIAN_POINT ( 'NONE',  ( 0.2165354330708668673, -0.4536011799217367080, 0.2665933059059888421 ) ) ;
#30802=CARTESIAN_POINT ( 'NONE',  ( 0.6692913385826777528, 0.2952755905511811885, 0.000000000000000000 ) ) ;
#30805=CARTESIAN_POINT ( 'NONE',  ( -1.686351706036744558, 0.1771653543307087075, -0.09757992244046823083 ) ) ;
#30806=CARTESIAN_POINT ( 'NONE',  ( 1.358267716535433323, 0.1660481256975885056, 0.3530559997133364547 ) ) ;
#30807=CARTESIAN_POINT ( 'NONE',  ( 1.312335958005249825, 0.1283753931104746893, -0.1820866141732285504 ) ) ;
#30808=CARTESIAN_POINT ( 'NONE',  ( 0.03937007874015833325, -0.6692913385826771977, 8.415575281601705876E-17 ) ) ;
#30810=CARTESIAN_POINT ( 'NONE',  ( -0.3477690288713902178, 0.2952755905511810774, -0.1292274648535930714 ) ) ;
#30811=CARTESIAN_POINT ( 'NONE',  ( -1.410761154855642463, -0.08942795157527998196, 0.3641732283464567121 ) ) ;
#30812=CARTESIAN_POINT ( 'NONE',  ( -0.2952755905511804668, 0.1660481256975885056, 0.3530559997133364547 ) ) ;
#30813=CARTESIAN_POINT ( 'NONE',  ( 1.614173228346457378, 0.4410134679336836783, -0.1372047244094476148 ) ) ;
#30817=CARTESIAN_POINT ( 'NONE',  ( 0.4527559055118117182, 0.1660481256975883668, -0.3530559997133364547 ) ) ;
#30819=CARTESIAN_POINT ( 'NONE',  ( -0.3740157480314953431, -0.5400638737290845981, -0.3530559997133363437 ) ) ;
#30820=CARTESIAN_POINT ( 'NONE',  ( -1.574803149606298192, -0.1870078740157480879, -0.4822834645669291653 ) ) ;
#30821=VECTOR ( 'NONE', #15239, 39.37007874015748143 ) ;
#30822=CARTESIAN_POINT ( 'NONE',  ( 0.6627296587926515548, 0.2952755905511811885, 0.1292274648535926551 ) ) ;
#30823=CARTESIAN_POINT ( 'NONE',  ( 8.195543980992789655E-16, -0.1870078740157480879, -0.4822834645669291653 ) ) ;
#30825=CARTESIAN_POINT ( 'NONE',  ( -0.6758530183727028406, -0.6692913385826773087, -0.1292274648535924053 ) ) ;
#30826=CARTESIAN_POINT ( 'NONE',  ( 0.3740157480314966754, -0.5400638737290844871, 0.3530559997133364547 ) ) ;
#30827=CARTESIAN_POINT ( 'NONE',  ( -0.4986876640419939388, 0.2306618581243847221, -0.2411417322834647770 ) ) ;
#30828=CARTESIAN_POINT ( 'NONE',  ( 0.5118110236220480003, -0.5511811023622047445, 6.969142054262312111E-17 ) ) ;
#30830=CARTESIAN_POINT ( 'NONE',  ( -0.2952755905511804668, 0.1660481256975885056, 0.3530559997133364547 ) ) ;
#30832=CARTESIAN_POINT ( 'NONE',  ( 1.607611548556431069, 0.2952755905511811885, 0.1292274648535926551 ) ) ;
#30835=ORIENTED_EDGE ( 'NONE', *, *, #68572, .F. ) ;
#30836=CARTESIAN_POINT ( 'NONE',  ( 0.7677165354330716118, 0.1660481256975883668, -0.3530559997133364547 ) ) ;
#30837=CARTESIAN_POINT ( 'NONE',  ( 0.1049868766404206816, -0.5023911411419708095, -0.1820866141732282451 ) ) ;
#30844=CARTESIAN_POINT ( 'NONE',  ( 0.4199475065616803948, -0.6046776061558809534, -0.2411417322834644161 ) ) ;
#30845=CARTESIAN_POINT ( 'NONE',  ( -1.076115485564303809, -0.6046776061558809534, -0.2411417322834644161 ) ) ;
#30846=CARTESIAN_POINT ( 'NONE',  ( -1.128608923884513837, -0.6046776061558807314, 0.2411417322834647770 ) ) ;
#30847=CARTESIAN_POINT ( 'NONE',  ( 0.4068241469816279987, -0.4281496062992127816, -0.4176697321401328100 ) ) ;
#30848=CARTESIAN_POINT ( 'NONE',  ( 1.076115485564305141, -0.6046776061558807314, 0.2411417322834647770 ) ) ;
#30849=CARTESIAN_POINT ( 'NONE',  ( 1.213910761154856299, 0.1771653543307087630, 0.09757992244046791164 ) ) ;
#30851=CARTESIAN_POINT ( 'NONE',  ( 1.456692913385827515, -0.5511811023622047445, 6.969142054262312111E-17 ) ) ;
#30852=CARTESIAN_POINT ( 'NONE',  ( -0.7808398950131222316, -0.3162353388693409650, -0.4822834645669289433 ) ) ;
#30854=CARTESIAN_POINT ( 'NONE',  ( 1.633858267716535639, -0.5400638737290844871, 0.3530559997133364547 ) ) ;
#30856=CARTESIAN_POINT ( 'NONE',  ( -0.3937007874015740483, -0.1870078740157479769, 0.4822834645669291653 ) ) ;
#30857=CARTESIAN_POINT ( 'NONE',  ( 0.9645669291338591078, -0.5400638737290845981, -0.3530559997133363437 ) ) ;
#30859=CARTESIAN_POINT ( 'NONE',  ( -1.555118110236219930, 0.07958543189024085140, 0.2665933059059887866 ) ) ;
#30860=CARTESIAN_POINT ( 'NONE',  ( 0.2427821522309719648, -0.05778040916215522460, 0.4822834645669289988 ) ) ;
#30861=CARTESIAN_POINT ( 'NONE',  ( 0.7874015748031503170, -0.1870078740157479769, 0.3641732283464567677 ) ) ;
#30863=CARTESIAN_POINT ( 'NONE',  ( 1.036745406824147731, 0.05413385826771666132, 0.4176697321401328100 ) ) ;
#30865=CARTESIAN_POINT ( 'NONE',  ( -0.4068241469816267775, -0.004921259842519870586, -0.3153832671262229437 ) ) ;
#30866=CARTESIAN_POINT ( 'NONE',  ( -0.4855643044619415427, -0.4281496062992124485, 0.4176697321401328655 ) ) ;
#30867=CARTESIAN_POINT ( 'NONE',  ( -1.581364829396324945, -0.08942795157528024563, -0.3641732283464568787 ) ) ;
#30868=CARTESIAN_POINT ( 'NONE',  ( -1.259842519685038686, -0.1870078740157479769, 0.4822834645669291653 ) ) ;
#30869=CARTESIAN_POINT ( 'NONE',  ( 1.371391076115485941, 0.2952755905511811885, 0.1292274648535926551 ) ) ;
#30871=CARTESIAN_POINT ( 'NONE',  ( -1.502624671916009680, -0.2845877964562159024, 0.3641732283464567677 ) ) ;
#30873=CARTESIAN_POINT ( 'NONE',  ( 1.541994750656168645, -0.6692913385826771977, 0.1292274648535927661 ) ) ;
#30876=CARTESIAN_POINT ( 'NONE',  ( 1.692913385826772421, 0.2952755905511811885, 0.000000000000000000 ) ) ;
#30877=CARTESIAN_POINT ( 'NONE',  ( -0.9186351706036736120, 0.1283753931104748280, 0.1820866141732283561 ) ) ;
#30878=FACE_OUTER_BOUND ( 'NONE', #81230, .T. ) ;
#30879=CARTESIAN_POINT ( 'NONE',  ( -0.2493438320209966919, -0.4281496062992124485, 0.4176697321401328655 ) ) ;
#30880=CARTESIAN_POINT ( 'NONE',  ( 0.1312335958005257930, 0.1283753931104746893, -0.1820866141732285504 ) ) ;
#30881=CARTESIAN_POINT ( 'NONE',  ( -1.049868766404198794, 0.1283753931104746893, -0.1820866141732285504 ) ) ;
#30882=CARTESIAN_POINT ( 'NONE',  ( 1.469816272965879911, 0.1283753931104746893, -0.1820866141732285504 ) ) ;
#30883=CARTESIAN_POINT ( 'NONE',  ( 0.9120734908136490793, 0.2952755905511810774, -0.1292274648535930714 ) ) ;
#30885=CARTESIAN_POINT ( 'NONE',  ( 0.3346456692913393205, -0.4536011799217368745, -0.2665933059059886201 ) ) ;
#30886=CARTESIAN_POINT ( 'NONE',  ( 0.5905511811023629321, 0.2952755905511811885, 0.000000000000000000 ) ) ;
#30887=CARTESIAN_POINT ( 'NONE',  ( 0.7939632545931766261, -0.08942795157527998196, 0.3641732283464567121 ) ) ;
#30888=ORIENTED_EDGE ( 'NONE', *, *, #69043, .T. ) ;
#30889=CARTESIAN_POINT ( 'NONE',  ( -1.017060367454067249, -0.05778040916215522460, 0.4822834645669289988 ) ) ;
#30890=ADVANCED_FACE ( 'NONE', ( #43201 ), #42384, .F. ) ;
#30891=CARTESIAN_POINT ( 'NONE',  ( -1.522309711286088607, -0.6046776061558807314, 0.2411417322834647770 ) ) ;
#30892=CARTESIAN_POINT ( 'NONE',  ( -0.1443569553805768291, 0.05413385826771666132, 0.4176697321401328100 ) ) ;
#30893=CARTESIAN_POINT ( 'NONE',  ( -1.725721784776902190, -0.08942795157527998196, 0.3641732283464567121 ) ) ;
#30895=CARTESIAN_POINT ( 'NONE',  ( 0.4265091863517067039, -0.6692913385826773087, -0.1292274648535924053 ) ) ;
#30896=CARTESIAN_POINT ( 'NONE',  ( 1.213910761154856299, -0.5511811023622048555, -0.09757992244046775898 ) ) ;
#30897=CARTESIAN_POINT ( 'NONE',  ( 0.1509186351706045259, -0.05778040916215560624, -0.4822834645669293319 ) ) ;
#30898=CARTESIAN_POINT ( 'NONE',  ( 0.4921259842519691285, 0.1660481256975885056, 0.3530559997133364547 ) ) ;
#30904=CARTESIAN_POINT ( 'NONE',  ( -0.5314960629921254842, -0.4536011799217368745, -0.2665933059059886201 ) ) ;
#30905=CARTESIAN_POINT ( 'NONE',  ( -0.7611548556430438595, 0.2306618581243848609, 0.2411417322834645549 ) ) ;
#30906=CARTESIAN_POINT ( 'NONE',  ( 0.6364829396325465405, -0.05778040916215522460, 0.4822834645669289988 ) ) ;
#30908=CARTESIAN_POINT ( 'NONE',  ( 0.8333333333333340365, -0.6692913385826771977, 0.1292274648535927661 ) ) ;
#30909=CARTESIAN_POINT ( 'NONE',  ( -1.633858267716534529, 0.1660481256975885056, 0.3530559997133364547 ) ) ;
#30910=CARTESIAN_POINT ( 'NONE',  ( 0.8464566929133865436, 0.1660481256975883668, -0.3530559997133364547 ) ) ;
#30911=DIRECTION ( 'NONE',  ( -0.000000000000000000, 1.000000000000000000, -0.000000000000000000 ) ) ;
#30914=CARTESIAN_POINT ( 'NONE',  ( 1.023622047244095112, -0.1870078740157480879, -0.4822834645669291653 ) ) ;
#30915=CARTESIAN_POINT ( 'NONE',  ( 0.4068241469816279987, -0.4281496062992127816, -0.4176697321401328100 ) ) ;
#30916=CARTESIAN_POINT ( 'NONE',  ( 1.325459317585302665, -0.004921259842519870586, -0.3153832671262229437 ) ) ;
#30917=CARTESIAN_POINT ( 'NONE',  ( 1.568241469816273659, -0.05778040916215560624, -0.4822834645669293319 ) ) ;
#30918=CARTESIAN_POINT ( 'NONE',  ( 1.299212598425197429, 0.2952755905511811885, 0.000000000000000000 ) ) ;
#30921=CARTESIAN_POINT ( 'NONE',  ( 0.6561679790026253567, -0.6046776061558809534, -0.2411417322834644161 ) ) ;
#30922=CARTESIAN_POINT ( 'NONE',  ( 1.528871391076116026, 0.1771653543307087630, 0.09757992244046791164 ) ) ;
#30923=CARTESIAN_POINT ( 'NONE',  ( -0.3608923884514428360, -0.6692913385826773087, -0.1292274648535924053 ) ) ;
#30924=CARTESIAN_POINT ( 'NONE',  ( -1.030183727034119867, -0.05778040916215560624, -0.4822834645669293319 ) ) ;
#30925=CARTESIAN_POINT ( 'NONE',  ( 1.043307086614173818, -0.5400638737290845981, -0.3530559997133363437 ) ) ;
#30929=CARTESIAN_POINT ( 'NONE',  ( 1.581364829396326277, -0.3162353388693409650, -0.4822834645669289433 ) ) ;
#30933=CARTESIAN_POINT ( 'NONE',  ( -1.595398199321656385, 1.585328674332965315, -0.1559797534342482472 ) ) ;
#30934=CARTESIAN_POINT ( 'NONE',  ( 1.292650918635171564, 0.1771653543307087630, 0.09757992244046791164 ) ) ;
#30936=CARTESIAN_POINT ( 'NONE',  ( 1.515748031496063408, 0.07958543189024085140, 0.2665933059059887866 ) ) ;
#30941=CARTESIAN_POINT ( 'NONE',  ( -0.8530183727034112984, -0.004921259842519576551, 0.3153832671262227771 ) ) ;
#30942=CARTESIAN_POINT ( 'NONE',  ( -1.338582677165353729, -0.1870078740157480601, -0.3641732283464567677 ) ) ;
#30943=CARTESIAN_POINT ( 'NONE',  ( -1.095800524934382292, -0.3162353388693409650, -0.4822834645669289433 ) ) ;
#30944=CARTESIAN_POINT ( 'NONE',  ( -0.03280839895013062252, -0.6692913385826771977, 0.1292274648535927661 ) ) ;
#30945=CARTESIAN_POINT ( 'NONE',  ( 1.561679790026247350, -0.4281496062992124485, 0.4176697321401328655 ) ) ;
#30946=VERTEX_POINT ( 'NONE', #68083 ) ;
#30947=CARTESIAN_POINT ( 'NONE',  ( 1.437007874015748810, 0.1660481256975885056, 0.3530559997133364547 ) ) ;
#30951=CARTESIAN_POINT ( 'NONE',  ( 1.614173228346457378, 1.055049524192302579, -0.1372047244094476148 ) ) ;
#30952=CARTESIAN_POINT ( 'NONE',  ( -0.4461942257217840213, -0.5023911411419708095, -0.1820866141732282451 ) ) ;
#30953=CARTESIAN_POINT ( 'NONE',  ( -1.115485564304461219, 0.05413385826771626580, -0.4176697321401330321 ) ) ;
#30954=CARTESIAN_POINT ( 'NONE',  ( 0.9251968503937015864, 0.1660481256975883668, -0.3530559997133364547 ) ) ;
#30955=ORIENTED_EDGE ( 'NONE', *, *, #69950, .T. ) ;
#30958=FACE_OUTER_BOUND ( 'NONE', #17099, .T. ) ;
#30959=CARTESIAN_POINT ( 'NONE',  ( -1.148293963254592542, -0.6692913385826773087, -0.1292274648535924053 ) ) ;
#30961=CARTESIAN_POINT ( 'NONE',  ( 0.01312335958005323398, -0.004921259842519576551, 0.3153832671262227771 ) ) ;
#30963=CARTESIAN_POINT ( 'NONE',  ( -0.6496062992125976043, 0.07958543189024071263, -0.2665933059059888421 ) ) ;
#30964=CARTESIAN_POINT ( 'NONE',  ( 0.4855643044619428750, -0.004921259842519576551, 0.3153832671262227771 ) ) ;
#30965=CARTESIAN_POINT ( 'NONE',  ( 0.6299212598425204535, -0.1870078740157479769, 0.4822834645669291653 ) ) ;
#30966=CARTESIAN_POINT ( 'NONE',  ( -0.5708661417322825615, -0.4536011799217367080, 0.2665933059059888421 ) ) ;
#30968=CARTESIAN_POINT ( 'NONE',  ( 1.213910761154856299, -0.6692913385826773087, -0.1292274648535924053 ) ) ;
#30969=CARTESIAN_POINT ( 'NONE',  ( -0.8989501312335946848, -0.6692913385826771977, 0.1292274648535927661 ) ) ;
#30971=CARTESIAN_POINT ( 'NONE',  ( -0.1837270341207343505, -0.6046776061558807314, 0.2411417322834647770 ) ) ;
#30972=CARTESIAN_POINT ( 'NONE',  ( -0.5446194225721777693, -0.05778040916215522460, 0.4822834645669289988 ) ) ;
#30973=CARTESIAN_POINT ( 'NONE',  ( 1.443569553805774897, -0.5023911411419708095, -0.1820866141732282451 ) ) ;
#30974=CARTESIAN_POINT ( 'NONE',  ( 0.01312335958005323398, -0.004921259842519576551, 0.3153832671262227771 ) ) ;
#30975=CARTESIAN_POINT ( 'NONE',  ( -0.01312335958005186876, -0.4281496062992124485, 0.4176697321401328655 ) ) ;
#30976=CARTESIAN_POINT ( 'NONE',  ( -1.246719160104985846, -0.4281496062992127816, -0.4176697321401328100 ) ) ;
#30977=CARTESIAN_POINT ( 'NONE',  ( 1.614173228346457378, 1.055049524192302579, -0.1372047244094476148 ) ) ;
#30979=CARTESIAN_POINT ( 'NONE',  ( -0.2362204724409440182, -0.1870078740157479769, 0.4822834645669291653 ) ) ;
#30980=CARTESIAN_POINT ( 'NONE',  ( -0.9711286089238838626, -0.6046776061558807314, 0.2411417322834647770 ) ) ;
#30981=ORIENTED_EDGE ( 'NONE', *, *, #40285, .F. ) ;
#30983=CARTESIAN_POINT ( 'NONE',  ( 0.9514435695538062676, -0.05778040916215522460, 0.4822834645669289988 ) ) ;
#30984=CARTESIAN_POINT ( 'NONE',  ( -0.7939632545931754048, -0.2845877964562159024, 0.3641732283464567677 ) ) ;
#30985=CARTESIAN_POINT ( 'NONE',  ( -0.7020997375328076329, -0.3162353388693409650, -0.4822834645669289433 ) ) ;
#30986=CARTESIAN_POINT ( 'NONE',  ( 1.154855643044620184, -0.6046776061558807314, 0.2411417322834647770 ) ) ;
#30987=CARTESIAN_POINT ( 'NONE',  ( 0.8136482939632553313, -0.6046776061558809534, -0.2411417322834644161 ) ) ;
#30988=CARTESIAN_POINT ( 'NONE',  ( 1.594488188976378673, 0.1660481256975885056, 0.3530559997133364547 ) ) ;
#30989=CARTESIAN_POINT ( 'NONE',  ( -0.9055118110236215490, 0.1771653543307087630, 0.000000000000000000 ) ) ;
#30994=CARTESIAN_POINT ( 'NONE',  ( 0.9973753280839902091, -0.5023911411419708095, 0.1820866141732285504 ) ) ;
#30995=CARTESIAN_POINT ( 'NONE',  ( 0.9055118110236227702, -0.5511811023622047445, 6.969142054262312111E-17 ) ) ;
#30997=CARTESIAN_POINT ( 'NONE',  ( 0.5774278215223103139, -0.6046776061558809534, -0.2411417322834644161 ) ) ;
#31000=CARTESIAN_POINT ( 'NONE',  ( 0.7677165354330716118, 0.07958543189024071263, -0.2665933059059888421 ) ) ;
#31001=CARTESIAN_POINT ( 'NONE',  ( -0.2952755905511803003, -0.5400638737290845981, -0.3530559997133363437 ) ) ;
#31002=CARTESIAN_POINT ( 'NONE',  ( -1.200787401574802349, -0.5400638737290844871, 0.3530559997133364547 ) ) ;
#31003=CARTESIAN_POINT ( 'NONE',  ( 1.410761154855643795, -0.05778040916215560624, -0.4822834645669293319 ) ) ;
#31006=CARTESIAN_POINT ( 'NONE',  ( 0.006561679790026889343, -0.08942795157527998196, 0.3641732283464567121 ) ) ;
#31009=CARTESIAN_POINT ( 'NONE',  ( -0.9514435695538050464, -0.3162353388693405765, 0.4822834645669290543 ) ) ;
#31010=CARTESIAN_POINT ( 'NONE',  ( -0.4527559055118102749, -0.5400638737290845981, -0.3530559997133363437 ) ) ;
#31011=CARTESIAN_POINT ( 'NONE',  ( -0.2296587926509179312, -0.05778040916215522460, 0.4822834645669289988 ) ) ;
#31012=CARTESIAN_POINT ( 'NONE',  ( 0.5249343832021005074, -0.6046776061558807314, 0.2411417322834647770 ) ) ;
#31013=CARTESIAN_POINT ( 'NONE',  ( -0.2952755905511803003, -0.5400638737290845981, -0.3530559997133363437 ) ) ;
#31014=CARTESIAN_POINT ( 'NONE',  ( -1.332020997375327642, -0.05778040916215522460, 0.4822834645669289988 ) ) ;
#31016=CARTESIAN_POINT ( 'NONE',  ( -0.9973753280839886548, -0.6046776061558809534, -0.2411417322834644161 ) ) ;
#31017=CARTESIAN_POINT ( 'NONE',  ( 0.8923884514435701520, -0.6046776061558809534, -0.2411417322834644161 ) ) ;
#31018=ADVANCED_FACE ( 'NONE', ( #73987 ), #45198, .F. ) ;
#31019=EDGE_CURVE ( 'NONE', #73693, #81247, #16319, .T. ) ;
#31021=CARTESIAN_POINT ( 'NONE',  ( -0.4593175853018364174, -0.3690944881889765550, -0.3153832671262227771 ) ) ;
#31024=EDGE_LOOP ( 'NONE', ( #61366, #74352, #80749, #14533 ) ) ;
#31025=CARTESIAN_POINT ( 'NONE',  ( -1.246719160104986512, -0.004921259842519576551, 0.3153832671262227771 ) ) ;
#31026=CARTESIAN_POINT ( 'NONE',  ( -1.167979002624671470, 0.05413385826771666132, 0.4176697321401328100 ) ) ;
#31027=CARTESIAN_POINT ( 'NONE',  ( -0.7152230971128602510, -0.3162353388693405765, 0.4822834645669290543 ) ) ;
#31029=CARTESIAN_POINT ( 'NONE',  ( -0.8398950131233589023, -0.6046776061558809534, -0.2411417322834644161 ) ) ;
#31030=CARTESIAN_POINT ( 'NONE',  ( -0.8923884514435688198, 0.2306618581243847221, -0.2411417322834647770 ) ) ;
#31032=CARTESIAN_POINT ( 'NONE',  ( -1.673228346456691717, 0.1660481256975883668, -0.3530559997133364547 ) ) ;
#31033=CARTESIAN_POINT ( 'NONE',  ( 0.5118110236220480003, -0.5511811023622047445, 6.969142054262312111E-17 ) ) ;
#31034=CARTESIAN_POINT ( 'NONE',  ( 1.614173228346457378, 0.9921945702958886448, -0.1372047244094476148 ) ) ;
#31036=CARTESIAN_POINT ( 'NONE',  ( -0.04593175853018302557, -0.5511811023622048555, -0.09757992244046775898 ) ) ;
#31037=CARTESIAN_POINT ( 'NONE',  ( -0.3215223097112853146, -0.05778040916215560624, -0.4822834645669293319 ) ) ;
#31038=CARTESIAN_POINT ( 'NONE',  ( 1.299212598425197429, 0.2952755905511811885, 0.000000000000000000 ) ) ;
#31039=CARTESIAN_POINT ( 'NONE',  ( -0.1312335958005241554, -0.6046776061558809534, -0.2411417322834644161 ) ) ;
#31042=CARTESIAN_POINT ( 'NONE',  ( -0.8005249343832011588, 0.009842519685039147898, -0.3409548833797004797 ) ) ;
#31043=ORIENTED_EDGE ( 'NONE', *, *, #34523, .F. ) ;
#31045=CARTESIAN_POINT ( 'NONE',  ( 1.135170603674541256, 0.2952755905511811885, 0.1292274648535926551 ) ) ;
#31046=CARTESIAN_POINT ( 'NONE',  ( -0.9908136482939626788, -0.5511811023622048555, -0.09757992244046775898 ) ) ;
#31047=CARTESIAN_POINT ( 'NONE',  ( -1.227034120734907585, 0.2952755905511811885, 0.1292274648535926551 ) ) ;
#31050=EDGE_CURVE ( 'NONE', #24575, #12831, #81992, .T. ) ;
#31052=CARTESIAN_POINT ( 'NONE',  ( 1.148293963254593875, -0.6692913385826771977, 0.1292274648535927661 ) ) ;
#31053=CARTESIAN_POINT ( 'NONE',  ( 0.6364829396325465405, -0.05778040916215522460, 0.4822834645669289988 ) ) ;
#31054=CARTESIAN_POINT ( 'NONE',  ( 0.1443569553805781891, 0.05413385826771626580, -0.4176697321401330321 ) ) ;
#31055=CARTESIAN_POINT ( 'NONE',  ( -1.102362204724408601, -0.1870078740157480601, -0.3641732283464567677 ) ) ;
#31056=CARTESIAN_POINT ( 'NONE',  ( -0.1837270341207343505, -0.6046776061558807314, 0.2411417322834647770 ) ) ;
#31059=CARTESIAN_POINT ( 'NONE',  ( -0.7283464566929126471, 0.1660481256975883668, -0.3530559997133364547 ) ) ;
#31061=CARTESIAN_POINT ( 'NONE',  ( 1.207349081364829990, -0.5023911411419708095, -0.1820866141732282451 ) ) ;
#31062=CARTESIAN_POINT ( 'NONE',  ( -0.3280839895013117347, -0.3690944881889763329, 0.3153832671262228327 ) ) ;
#31063=CARTESIAN_POINT ( 'NONE',  ( 1.076115485564305141, 0.1283753931104746893, -0.1820866141732285504 ) ) ;
#31064=CARTESIAN_POINT ( 'NONE',  ( -1.601049868766403650, -0.6046776061558807314, 0.2411417322834647770 ) ) ;
#31065=CARTESIAN_POINT ( 'NONE',  ( -1.135170603674539924, 0.1771653543307087075, -0.09757992244046823083 ) ) ;
#31066=CARTESIAN_POINT ( 'NONE',  ( 0.6824146981627303710, -0.5023911411419708095, 0.1820866141732285504 ) ) ;
#31067=CARTESIAN_POINT ( 'NONE',  ( -0.7020997375328074108, -0.05778040916215522460, 0.4822834645669289988 ) ) ;
#31069=CARTESIAN_POINT ( 'NONE',  ( 0.08530183727034192087, -0.08942795157527998196, 0.3641732283464567121 ) ) ;
#31070=CARTESIAN_POINT ( 'NONE',  ( -1.594488188976377563, -0.4536011799217367080, 0.2665933059059888421 ) ) ;
#31072=CARTESIAN_POINT ( 'NONE',  ( 0.5971128608923891301, 0.2952755905511810774, -0.1292274648535930714 ) ) ;
#31073=CARTESIAN_POINT ( 'NONE',  ( 0.6627296587926515548, 0.2952755905511811885, 0.1292274648535926551 ) ) ;
#31074=CARTESIAN_POINT ( 'NONE',  ( 1.463254593175853824, 0.1771653543307087075, -0.09757992244046823083 ) ) ;
#31075=CARTESIAN_POINT ( 'NONE',  ( -0.9711286089238838626, -0.6046776061558807314, 0.2411417322834647770 ) ) ;
#31076=CARTESIAN_POINT ( 'NONE',  ( -0.1312335958005241554, -0.5023911411419708095, -0.1820866141732282451 ) ) ;
#31078=CARTESIAN_POINT ( 'NONE',  ( 0.4199475065616803948, -0.5023911411419708095, -0.1820866141732282451 ) ) ;
#31080=CARTESIAN_POINT ( 'NONE',  ( -1.233595800524933894, 0.2306618581243848609, 0.2411417322834645549 ) ) ;
#31081=CARTESIAN_POINT ( 'NONE',  ( -0.3805774278215216522, 0.05413385826771666132, 0.4176697321401328100 ) ) ;
#31084=CARTESIAN_POINT ( 'NONE',  ( 0.5183727034120741983, 0.1771653543307087075, -0.09757992244046823083 ) ) ;
#31085=CARTESIAN_POINT ( 'NONE',  ( -0.3018372703412066094, -0.4281496062992127816, -0.4176697321401328100 ) ) ;
#31086=CARTESIAN_POINT ( 'NONE',  ( -0.8464566929133852113, 0.1660481256975885056, 0.3530559997133364547 ) ) ;
#31087=CARTESIAN_POINT ( 'NONE',  ( -0.7480314960629914633, -0.5511811023622047445, 6.969142054262312111E-17 ) ) ;
#31089=CARTESIAN_POINT ( 'NONE',  ( -0.2230971128608915943, 0.05413385826771666132, 0.4176697321401328100 ) ) ;
#31090=CARTESIAN_POINT ( 'NONE',  ( -1.666666666666665853, -0.004921259842519870586, -0.3153832671262229437 ) ) ;
#31091=CARTESIAN_POINT ( 'NONE',  ( 1.581364829396326277, -0.05778040916215522460, 0.4822834645669289988 ) ) ;
#31092=CARTESIAN_POINT ( 'NONE',  ( 0.01033912696139590269, 2.459406111854941508E-15, 0.4281989832122450323 ) ) ;
#31095=CARTESIAN_POINT ( 'NONE',  ( -1.482939632545930975, -0.4281496062992127816, -0.4176697321401328100 ) ) ;
#31096=CARTESIAN_POINT ( 'NONE',  ( -0.7545931758530177724, 0.2952755905511811885, 0.1292274648535926551 ) ) ;
#31097=EDGE_CURVE ( 'NONE', #949, #13300, #31865, .T. ) ;
#31098=CARTESIAN_POINT ( 'NONE',  ( -1.404199475065615932, -0.4281496062992127816, -0.4176697321401328100 ) ) ;
#31101=CARTESIAN_POINT ( 'NONE',  ( 0.8923884514435703741, 0.2306618581243848609, 0.2411417322834645549 ) ) ;
#31102=CARTESIAN_POINT ( 'NONE',  ( 0.4855643044619430415, -0.4281496062992127816, -0.4176697321401328100 ) ) ;
#31104=LINE ( 'NONE', #76567, #3588 ) ;
#31105=CARTESIAN_POINT ( 'NONE',  ( 1.076115485564305141, -0.5023911411419708095, 0.1820866141732285504 ) ) ;
#31109=ORIENTED_EDGE ( 'NONE', *, *, #68162, .F. ) ;
#31110=CARTESIAN_POINT ( 'NONE',  ( 0.3149606299212603933, -0.1870078740157479769, 0.4822834645669291653 ) ) ;
#31111=CARTESIAN_POINT ( 'NONE',  ( -0.8333333333333323711, -0.6692913385826773087, -0.1292274648535924053 ) ) ;
#31112=CARTESIAN_POINT ( 'NONE',  ( -1.437007874015747477, 0.1660481256975883668, -0.3530559997133364547 ) ) ;
#31113=CARTESIAN_POINT ( 'NONE',  ( 1.069553805774278832, 0.2952755905511810774, -0.1292274648535930714 ) ) ;
#31114=CARTESIAN_POINT ( 'NONE',  ( 1.515748031496063408, 0.1660481256975885056, 0.3530559997133364547 ) ) ;
#31116=CARTESIAN_POINT ( 'NONE',  ( -0.2624671916010490880, -0.6046776061558807314, 0.2411417322834647770 ) ) ;
#31118=CARTESIAN_POINT ( 'NONE',  ( -1.332020997375327642, -0.05778040916215522460, 0.4822834645669289988 ) ) ;
#31119=CARTESIAN_POINT ( 'NONE',  ( -1.482939632545930975, 0.05413385826771666132, 0.4176697321401328100 ) ) ;
#31120=CARTESIAN_POINT ( 'NONE',  ( 1.515748031496063408, 0.1660481256975885056, 0.3530559997133364547 ) ) ;
#31122=CARTESIAN_POINT ( 'NONE',  ( 0.8202099737532814183, -0.5511811023622048555, -0.09757992244046775898 ) ) ;
#31126=CARTESIAN_POINT ( 'NONE',  ( 0.02624671916010564918, 0.1283753931104748280, 0.1820866141732283561 ) ) ;
#31128=CARTESIAN_POINT ( 'NONE',  ( 0.4986876640419954376, 0.2306618581243848609, 0.2411417322834645549 ) ) ;
#31129=CARTESIAN_POINT ( 'NONE',  ( 0.2559055118110243332, -0.5400638737290845981, -0.3530559997133363437 ) ) ;
#31130=B_SPLINE_CURVE_WITH_KNOTS ( 'NONE', 3,
 ( #79325, #48968, #2710, #21644, #73420, #9436, #67932 ),
 .UNSPECIFIED., .F., .F.,
 ( 4, 3, 4 ),
 ( 1.734723475976806902E-18, 0.001246232571205225376, 0.002492492258783241162 ),
 .UNSPECIFIED. ) ;
#31131=CARTESIAN_POINT ( 'NONE',  ( -0.7480314960629914633, 0.2952755905511811885, 0.000000000000000000 ) ) ;
#31133=CARTESIAN_POINT ( 'NONE',  ( -1.253280839895012377, -0.3162353388693409650, -0.4822834645669289433 ) ) ;
#31135=CARTESIAN_POINT ( 'NONE',  ( 1.174540682414699111, -0.08942795157528024563, -0.3641732283464568787 ) ) ;
#31136=CARTESIAN_POINT ( 'NONE',  ( -1.318897637795274802, 0.1660481256975885056, 0.3530559997133364547 ) ) ;
#31137=CARTESIAN_POINT ( 'NONE',  ( 0.8136482939632553313, -0.6046776061558809534, -0.2411417322834644161 ) ) ;
#31138=CARTESIAN_POINT ( 'NONE',  ( 1.062992125984252745, 0.2952755905511811885, 0.000000000000000000 ) ) ;
#31140=CARTESIAN_POINT ( 'NONE',  ( -1.200787401574802349, 0.1660481256975883668, -0.3530559997133364547 ) ) ;
#31142=CARTESIAN_POINT ( 'NONE',  ( -0.2296587926509179312, -0.3162353388693409650, -0.4822834645669289433 ) ) ;
#31144=ADVANCED_FACE ( 'NONE', ( #50795 ), #4539, .F. ) ;
#31146=CARTESIAN_POINT ( 'NONE',  ( 1.437007874015748810, -0.5400638737290845981, -0.3530559997133363437 ) ) ;
#31147=CARTESIAN_POINT ( 'NONE',  ( 0.3608923884514443348, -0.5511811023622046335, 0.09757992244046803654 ) ) ;
#31148=CARTESIAN_POINT ( 'NONE',  ( 1.023622047244095112, -0.1870078740157480879, -0.4822834645669291653 ) ) ;
#31150=CARTESIAN_POINT ( 'NONE',  ( 0.7480314960629927956, 0.1771653543307087630, 0.000000000000000000 ) ) ;
#31151=CARTESIAN_POINT ( 'NONE',  ( 0.4921259842519691285, 0.1660481256975885056, 0.3530559997133364547 ) ) ;
#31153=CARTESIAN_POINT ( 'NONE',  ( -0.9317585301837263412, 0.05413385826771666132, 0.4176697321401328100 ) ) ;
#31154=B_SPLINE_CURVE_WITH_KNOTS ( 'NONE', 3,
 ( #46154, #77323, #39431, #6608 ),
 .UNSPECIFIED., .F., .F.,
 ( 4, 4 ),
 ( 3.593986969215047557E-07, 0.001287825409103288176 ),
 .UNSPECIFIED. ) ;
#31156=CARTESIAN_POINT ( 'NONE',  ( 0.8792650918635177559, -0.3690944881889765550, -0.3153832671262227771 ) ) ;
#31157=CARTESIAN_POINT ( 'NONE',  ( 0.1681795077207355327, -2.839693391405754848E-15, 0.4118477457932995245 ) ) ;
#31158=CARTESIAN_POINT ( 'NONE',  ( -0.2296587926509179312, -0.3162353388693409650, -0.4822834645669289433 ) ) ;
#31159=CARTESIAN_POINT ( 'NONE',  ( -0.09186351706036663400, -0.3690944881889763329, 0.3153832671262228327 ) ) ;
#31161=CARTESIAN_POINT ( 'NONE',  ( -0.1246719160104980823, 0.2952755905511811885, 0.1292274648535926551 ) ) ;
#31162=CARTESIAN_POINT ( 'NONE',  ( 0.9251968503937015864, -0.4536011799217367080, 0.2665933059059888421 ) ) ;
#31164=CARTESIAN_POINT ( 'NONE',  ( 0.2887139107611556010, 0.2306618581243847221, -0.2411417322834647770 ) ) ;
#31165=CARTESIAN_POINT ( 'NONE',  ( 1.358267716535433323, 0.07958543189024085140, 0.2665933059059887866 ) ) ;
#31166=CARTESIAN_POINT ( 'NONE',  ( 1.614173228346456712, 1.267785121476991517, 0.1372047244094478646 ) ) ;
#31167=CARTESIAN_POINT ( 'NONE',  ( -0.5118110236220466680, -0.5511811023622047445, 6.969142054262312111E-17 ) ) ;
#31169=CARTESIAN_POINT ( 'NONE',  ( -0.8070866141732276899, -0.4536011799217367080, 0.2665933059059888421 ) ) ;
#31170=CARTESIAN_POINT ( 'NONE',  ( -0.1509186351706028884, -0.3162353388693409650, -0.4822834645669289433 ) ) ;
#31171=CARTESIAN_POINT ( 'NONE',  ( 0.1706036745406830368, 0.05413385826771666132, 0.4176697321401328100 ) ) ;
#31172=CARTESIAN_POINT ( 'NONE',  ( 0.8398950131233602345, -0.5023911411419708095, 0.1820866141732285504 ) ) ;
#31174=CARTESIAN_POINT ( 'NONE',  ( 1.528871391076116026, -0.5511811023622048555, -0.09757992244046775898 ) ) ;
#31177=CARTESIAN_POINT ( 'NONE',  ( 0.7808398950131241190, -0.05778040916215560624, -0.4822834645669293319 ) ) ;
#31179=CARTESIAN_POINT ( 'NONE',  ( -0.1049868766404193215, 0.2306618581243847221, -0.2411417322834647770 ) ) ;
#31181=CARTESIAN_POINT ( 'NONE',  ( 1.023622047244095334, -0.1870078740157479769, 0.4822834645669291653 ) ) ;
#31182=CARTESIAN_POINT ( 'NONE',  ( 0.4396325459317593221, 0.2952755905511810774, -0.1292274648535930714 ) ) ;
#31185=CARTESIAN_POINT ( 'NONE',  ( 0.1968503937007881344, -0.5511811023622047445, 6.969142054262312111E-17 ) ) ;
#31186=CARTESIAN_POINT ( 'NONE',  ( 1.161417322834646493, -0.5400638737290844871, 0.3530559997133364547 ) ) ;
#31187=CARTESIAN_POINT ( 'NONE',  ( -0.2296587926509179312, -0.2845877964562161244, -0.3641732283464567121 ) ) ;
#31188=CARTESIAN_POINT ( 'NONE',  ( -0.3018372703412066094, -0.4281496062992127816, -0.4176697321401328100 ) ) ;
#31189=CARTESIAN_POINT ( 'NONE',  ( -1.220472440944881054, 2.401574803149606474, 0.5309055118110237448 ) ) ;
#31190=CARTESIAN_POINT ( 'NONE',  ( 0.3740157480314966754, 0.1660481256975883668, -0.3530559997133364547 ) ) ;
#31191=CARTESIAN_POINT ( 'NONE',  ( -0.9645669291338575535, 0.1660481256975883668, -0.3530559997133364547 ) ) ;
#31192=CARTESIAN_POINT ( 'NONE',  ( -0.6627296587926503335, -0.5511811023622046335, 0.09757992244046803654 ) ) ;
#31193=CARTESIAN_POINT ( 'NONE',  ( 0.2559055118110243332, -0.5400638737290845981, -0.3530559997133363437 ) ) ;
#31194=CARTESIAN_POINT ( 'NONE',  ( -1.384514435695537005, 0.2952755905511811885, 0.1292274648535926551 ) ) ;
#31195=CARTESIAN_POINT ( 'NONE',  ( -0.4724409448818890911, -0.1870078740157480879, -0.4822834645669291653 ) ) ;
#31196=( BOUNDED_CURVE ( )  B_SPLINE_CURVE ( 2, ( #19364, #51748, #82931, #65248, #76617, #52587, #38304, #32404, #44595, #20203, #1278, #32826, #37891 ),
 .UNSPECIFIED., .F., .F. ) 
 B_SPLINE_CURVE_WITH_KNOTS ( ( 3, 2, 2, 2, 2, 2, 3 ),
 ( 0.5944878114796872115, 0.5946969696969697239, 0.5984848484848485084, 0.6022727272727272929, 0.6060606060606060774, 0.6098484848484848619, 0.6100576430657673743 ),
 .UNSPECIFIED. ) 
 CURVE ( )  GEOMETRIC_REPRESENTATION_ITEM ( )  RATIONAL_B_SPLINE_CURVE ( ( 0.9964447847208419695, 0.9981185001348091834, 1.000000000000000000, 0.9659258262890683122, 1.000000000000000000, 0.9659258262890683122, 1.000000000000000000, 0.9659258262890683122, 1.000000000000000000, 0.9659258262890683122, 1.000000000000000000, 0.9981185001348091834, 0.9964447847208420805 ) ) 
 REPRESENTATION_ITEM ( '' )  );
#31199=CARTESIAN_POINT ( 'NONE',  ( 1.292650918635171564, 0.2952755905511811885, 0.1292274648535926551 ) ) ;
#31200=CARTESIAN_POINT ( 'NONE',  ( 1.587926509186352586, -0.4281496062992127816, -0.4176697321401328100 ) ) ;
#31203=CARTESIAN_POINT ( 'NONE',  ( -0.7349081364829390672, 0.2306618581243847221, -0.2411417322834647770 ) ) ;
#31206=ORIENTED_EDGE ( 'NONE', *, *, #28480, .F. ) ;
#31207=CARTESIAN_POINT ( 'NONE',  ( 0.3674540682414705883, -0.5023911411419708095, 0.1820866141732285504 ) ) ;
#31209=CARTESIAN_POINT ( 'NONE',  ( 0.5971128608923890191, -0.6692913385826771977, 0.1292274648535927661 ) ) ;
#31211=CARTESIAN_POINT ( 'NONE',  ( -0.5626772485143695102, -5.582469467804009507E-15, -0.3791483426435192650 ) ) ;
#31212=CARTESIAN_POINT ( 'NONE',  ( -0.4002624671916004129, -0.2845877964562159024, 0.3641732283464567677 ) ) ;
#31213=CARTESIAN_POINT ( 'NONE',  ( -0.2559055118110230564, 0.1660481256975883391, -0.3530559997133364547 ) ) ;
#31214=CARTESIAN_POINT ( 'NONE',  ( 1.135170603674541256, -0.6692913385826773087, -0.1292274648535924053 ) ) ;
#31215=CARTESIAN_POINT ( 'NONE',  ( 0.8136482939632553313, 0.1283753931104748280, 0.1820866141732283561 ) ) ;
#31216=CARTESIAN_POINT ( 'NONE',  ( -0.09842519685039295696, -0.5400638737290844871, 0.3530559997133364547 ) ) ;
#31218=CARTESIAN_POINT ( 'NONE',  ( -0.3740157480314953431, 0.1660481256975885056, 0.3530559997133364547 ) ) ;
#31219=CARTESIAN_POINT ( 'NONE',  ( -1.509186351706035767, -0.004921259842519870586, -0.3153832671262229437 ) ) ;
#31220=CARTESIAN_POINT ( 'NONE',  ( -0.4658792650918627265, -0.05778040916215522460, 0.4822834645669289988 ) ) ;
#31221=CARTESIAN_POINT ( 'NONE',  ( -1.595398199321656829, 1.034147571970760238, 0.1559797534342477754 ) ) ;
#31225=CARTESIAN_POINT ( 'NONE',  ( 0.3740157480314966754, -0.5400638737290844871, 0.3530559997133364547 ) ) ;
#31226=ORIENTED_EDGE ( 'NONE', *, *, #37675, .T. ) ;
#31227=CARTESIAN_POINT ( 'NONE',  ( -0.4068241469816267775, 0.05413385826771626580, -0.4176697321401330321 ) ) ;
#31228=CARTESIAN_POINT ( 'NONE',  ( -1.548556430446193399, -0.6046776061558809534, -0.2411417322834644161 ) ) ;
#31229=CARTESIAN_POINT ( 'NONE',  ( 0.8202099737532813073, 0.2952755905511811885, 0.1292274648535926551 ) ) ;
#31231=CARTESIAN_POINT ( 'NONE',  ( 0.1443569553805781891, 0.05413385826771626580, -0.4176697321401330321 ) ) ;
#31233=CARTESIAN_POINT ( 'NONE',  ( -0.7283464566929126471, 0.1660481256975883668, -0.3530559997133364547 ) ) ;
#31234=CARTESIAN_POINT ( 'NONE',  ( 0.2362204724409456558, -0.1870078740157479769, 0.4822834645669291653 ) ) ;
#31235=CARTESIAN_POINT ( 'NONE',  ( -0.6430446194225712953, 0.05413385826771626580, -0.4176697321401330321 ) ) ;
#31236=CARTESIAN_POINT ( 'NONE',  ( 0.2165354330708668673, -0.4536011799217367080, 0.2665933059059888421 ) ) ;
#31238=CARTESIAN_POINT ( 'NONE',  ( 0.04593175853018440641, 0.2952755905511810774, -0.1292274648535930714 ) ) ;
#31239=CONICAL_SURFACE ( 'NONE', #37970, 2.401574803149606918, 0.6981317007977250189 ) ;
#31240=DIRECTION ( 'NONE',  ( 0.000000000000000000, 0.000000000000000000, 1.000000000000000000 ) ) ;
#31241=CARTESIAN_POINT ( 'NONE',  ( -1.653543307086613234, -0.1870078740157479769, 0.4822834645669291653 ) ) ;
#31244=ORIENTED_EDGE ( 'NONE', *, *, #13149, .T. ) ;
#31245=CARTESIAN_POINT ( 'NONE',  ( 0.4068241469816281097, 0.05413385826771666132, 0.4176697321401328100 ) ) ;
#31246=CARTESIAN_POINT ( 'NONE',  ( -0.03280839895013062252, -0.5511811023622046335, 0.09757992244046803654 ) ) ;
#31247=CARTESIAN_POINT ( 'NONE',  ( 1.640419947506562393, -0.3690944881889763329, 0.3153832671262228327 ) ) ;
#31253=CARTESIAN_POINT ( 'NONE',  ( 0.3543307086614179147, 0.2952755905511811885, 0.000000000000000000 ) ) ;
#31254=CARTESIAN_POINT ( 'NONE',  ( -1.437007874015747477, 0.1660481256975883668, -0.3530559997133364547 ) ) ;
#31255=CARTESIAN_POINT ( 'NONE',  ( -1.036745406824146176, 0.05413385826771626580, -0.4176697321401330321 ) ) ;
#31256=CARTESIAN_POINT ( 'NONE',  ( 0.09186351706036799403, -0.4281496062992127816, -0.4176697321401328100 ) ) ;
#31257=CARTESIAN_POINT ( 'NONE',  ( 0.8727034120734912248, -0.3162353388693409650, -0.4822834645669289433 ) ) ;
#31258=CARTESIAN_POINT ( 'NONE',  ( 1.384514435695538559, 0.1771653543307087075, -0.09757992244046823083 ) ) ;
#31260=CARTESIAN_POINT ( 'NONE',  ( 0.7217847769028878924, -0.004921259842519576551, 0.3153832671262227771 ) ) ;
#31261=CARTESIAN_POINT ( 'NONE',  ( -1.056430446194224881, -0.6692913385826771977, 0.1292274648535927661 ) ) ;
#31263=CARTESIAN_POINT ( 'NONE',  ( 1.476377952755906442, -0.5400638737290844871, 0.3530559997133364547 ) ) ;
#31266=CARTESIAN_POINT ( 'NONE',  ( 1.181102362204725198, -0.1870078740157479769, 0.4822834645669291653 ) ) ;
#31268=CARTESIAN_POINT ( 'NONE',  ( -1.679790026246718693, 0.1283753931104746893, -0.1820866141732285504 ) ) ;
#31269=CARTESIAN_POINT ( 'NONE',  ( 0.02624671916010564918, -0.6046776061558809534, -0.2411417322834644161 ) ) ;
#31270=CARTESIAN_POINT ( 'NONE',  ( 0.6627296587926515548, 0.1771653543307087630, 0.09757992244046791164 ) ) ;
#31272=CARTESIAN_POINT ( 'NONE',  ( -1.443569553805773564, -0.5023911411419708095, 0.1820866141732285504 ) ) ;
#31273=CARTESIAN_POINT ( 'NONE',  ( 0.8923884514435703741, 0.2306618581243848609, 0.2411417322834645549 ) ) ;
#31275=CARTESIAN_POINT ( 'NONE',  ( -0.4330708661417315697, 0.1771653543307087630, 0.000000000000000000 ) ) ;
#31276=CARTESIAN_POINT ( 'NONE',  ( -0.6889763779527552368, -0.5400638737290845981, -0.3530559997133363437 ) ) ;
#31277=CARTESIAN_POINT ( 'NONE',  ( 1.410761154855643795, -0.05778040916215560624, -0.4822834645669293319 ) ) ;
#31278=CARTESIAN_POINT ( 'NONE',  ( -1.181102362204723644, -0.1870078740157480879, -0.4822834645669291653 ) ) ;
#31279=CARTESIAN_POINT ( 'NONE',  ( 1.555118110236221041, 0.1660481256975883668, -0.3530559997133364547 ) ) ;
#31281=CARTESIAN_POINT ( 'NONE',  ( -1.279527559055116948, 0.07958543189024071263, -0.2665933059059888421 ) ) ;
#31283=CARTESIAN_POINT ( 'NONE',  ( 0.7939632545931766261, -0.05778040916215522460, 0.4822834645669289988 ) ) ;
#31285=CARTESIAN_POINT ( 'NONE',  ( -1.587926509186350810, -0.4281496062992124485, 0.4176697321401328655 ) ) ;
#31286=CARTESIAN_POINT ( 'NONE',  ( -1.535433070866141225, -0.5511811023622047445, 6.969142054262312111E-17 ) ) ;
#31287=CARTESIAN_POINT ( 'NONE',  ( -1.023622047244094002, -0.1870078740157480601, -0.3641732283464567677 ) ) ;
#31288=CARTESIAN_POINT ( 'NONE',  ( 1.528871391076116026, 0.1771653543307087630, 0.09757992244046791164 ) ) ;
#31289=CARTESIAN_POINT ( 'NONE',  ( -0.5643044619422565855, -0.4281496062992124485, 0.4176697321401328655 ) ) ;
#31290=CARTESIAN_POINT ( 'NONE',  ( -0.06561679790026180015, -0.004921259842519576551, 0.3153832671262227771 ) ) ;
#31291=CARTESIAN_POINT ( 'NONE',  ( -1.555118110236219930, 0.07958543189024085140, 0.2665933059059887866 ) ) ;
#31292=CARTESIAN_POINT ( 'NONE',  ( 1.286089238845145033, 0.1283753931104748280, 0.1820866141732283561 ) ) ;
#31294=CARTESIAN_POINT ( 'NONE',  ( 0.8464566929133866546, -0.5400638737290844871, 0.3530559997133364547 ) ) ;
#31295=CARTESIAN_POINT ( 'NONE',  ( 1.574803149606299746, -0.1870078740157479769, 0.4822834645669291653 ) ) ;
#31296=CARTESIAN_POINT ( 'NONE',  ( 0.01968503937007957949, -0.4536011799217368745, -0.2665933059059886201 ) ) ;
#31297=CARTESIAN_POINT ( 'NONE',  ( 0.4527559055118117182, 0.1660481256975883668, -0.3530559997133364547 ) ) ;
#31298=CARTESIAN_POINT ( 'NONE',  ( 1.102362204724410155, -0.1870078740157479769, 0.3641732283464567677 ) ) ;
#31299=ORIENTED_EDGE ( 'NONE', *, *, #50451, .T. ) ;
#31300=CARTESIAN_POINT ( 'NONE',  ( -1.515748031496062076, -0.5400638737290844871, 0.3530559997133364547 ) ) ;
#31301=CARTESIAN_POINT ( 'NONE',  ( -1.207349081364828436, -0.6046776061558807314, 0.2411417322834647770 ) ) ;
#31302=CARTESIAN_POINT ( 'NONE',  ( -0.09186351706036689768, 0.05413385826771626580, -0.4176697321401330321 ) ) ;
#31305=CARTESIAN_POINT ( 'NONE',  ( 0.3083989501312343062, -0.3162353388693405765, 0.4822834645669290543 ) ) ;
#31306=CARTESIAN_POINT ( 'NONE',  ( 1.023622047244095112, -0.1870078740157480601, -0.3641732283464567677 ) ) ;
#31307=CARTESIAN_POINT ( 'NONE',  ( 0.1443569553805781891, 0.05413385826771626580, -0.4176697321401330321 ) ) ;
#31308=CARTESIAN_POINT ( 'NONE',  ( 0.4593175853018379162, -0.4281496062992124485, 0.4176697321401328655 ) ) ;
#31314=CARTESIAN_POINT ( 'NONE',  ( -0.6496062992125976043, -0.4536011799217367080, 0.2665933059059888421 ) ) ;
#31315=CARTESIAN_POINT ( 'NONE',  ( -0.5839895013123351797, 0.2952755905511810774, -0.1292274648535930714 ) ) ;
#31317=CARTESIAN_POINT ( 'NONE',  ( 0.7020997375328090762, -0.3162353388693405765, 0.4822834645669290543 ) ) ;
#31318=CARTESIAN_POINT ( 'NONE',  ( -1.391076115485563314, -0.6046776061558809534, -0.2411417322834644161 ) ) ;
#31319=CARTESIAN_POINT ( 'NONE',  ( 0.6692913385826777528, 0.2952755905511811885, 0.000000000000000000 ) ) ;
#31322=DIRECTION ( 'NONE',  ( 0.000000000000000000, 0.000000000000000000, -1.000000000000000000 ) ) ;
#31323=B_SPLINE_CURVE_WITH_KNOTS ( 'NONE', 3,
 ( #4447, #75577, #30933, #11184 ),
 .UNSPECIFIED., .F., .F.,
 ( 4, 4 ),
 ( 3.593986969189856268E-07, 0.001287825409103220521 ),
 .UNSPECIFIED. ) ;
#31324=CARTESIAN_POINT ( 'NONE',  ( 1.076115485564305141, -0.6046776061558807314, 0.2411417322834647770 ) ) ;
#31325=CARTESIAN_POINT ( 'NONE',  ( 0.6561679790026253567, 0.2306618581243848609, 0.2411417322834645549 ) ) ;
#31326=CARTESIAN_POINT ( 'NONE',  ( 0.8923884514435701520, -0.5023911411419708095, -0.1820866141732282451 ) ) ;
#31327=CARTESIAN_POINT ( 'NONE',  ( 1.259842519685040019, -0.1870078740157480879, -0.4822834645669291653 ) ) ;
#31330=CARTESIAN_POINT ( 'NONE',  ( 0.7020997375328090762, -0.3162353388693405765, 0.4822834645669290543 ) ) ;
#31331=CARTESIAN_POINT ( 'NONE',  ( 1.692913385826772421, 0.1771653543307087630, 0.000000000000000000 ) ) ;
#31332=CARTESIAN_POINT ( 'NONE',  ( -0.5314960629921254842, -0.5400638737290845981, -0.3530559997133363437 ) ) ;
#31333=CARTESIAN_POINT ( 'NONE',  ( -1.174540682414697335, -0.3162353388693409650, -0.4822834645669289433 ) ) ;
#31334=CARTESIAN_POINT ( 'NONE',  ( 1.115485564304462551, 0.05413385826771666132, 0.4176697321401328100 ) ) ;
#31338=ORIENTED_EDGE ( 'NONE', *, *, #64032, .F. ) ;
#31341=CARTESIAN_POINT ( 'NONE',  ( -0.01968503937007793844, 0.1012011053420775880, -0.2882089793578256898 ) ) ;
#31342=CARTESIAN_POINT ( 'NONE',  ( 1.502624671916010790, -0.2845877964562161244, -0.3641732283464567121 ) ) ;
#31344=CARTESIAN_POINT ( 'NONE',  ( 1.351706036745407680, -0.004921259842519576551, 0.3153832671262227771 ) ) ;
#31345=CARTESIAN_POINT ( 'NONE',  ( -0.7137454485294953965, 2.244094488188976388, 0.4917280318828573527 ) ) ;
#31350=CARTESIAN_POINT ( 'NONE',  ( -0.7545931758530176614, -0.5511811023622048555, -0.09757992244046775898 ) ) ;
#31351=CARTESIAN_POINT ( 'NONE',  ( -1.509186351706035767, -0.004921259842519870586, -0.3153832671262229437 ) ) ;
#31352=CARTESIAN_POINT ( 'NONE',  ( -1.279527559055116948, 0.1660481256975883668, -0.3530559997133364547 ) ) ;
#31353=CARTESIAN_POINT ( 'NONE',  ( -0.01968503937007793844, -0.5400638737290844871, 0.3530559997133364547 ) ) ;
#31354=CARTESIAN_POINT ( 'NONE',  ( -1.574803149606298192, -0.1870078740157480879, -0.4822834645669291653 ) ) ;
#31356=CARTESIAN_POINT ( 'NONE',  ( 1.489501312335958172, -0.05778040916215560624, -0.4822834645669293319 ) ) ;
#31361=CARTESIAN_POINT ( 'NONE',  ( -0.4199475065616791736, -0.5023911411419708095, 0.1820866141732285504 ) ) ;
#31363=CARTESIAN_POINT ( 'NONE',  ( -1.043307086614172041, -0.5400638737290844871, 0.3530559997133364547 ) ) ;
#31364=CARTESIAN_POINT ( 'NONE',  ( 1.187664041994751285, -0.05778040916215522460, 0.4822834645669289988 ) ) ;
#31368=CARTESIAN_POINT ( 'NONE',  ( 1.423884514435696413, -0.3162353388693409650, -0.4822834645669289433 ) ) ;
#31369=CARTESIAN_POINT ( 'NONE',  ( -1.187664041994750175, -0.05778040916215560624, -0.4822834645669293319 ) ) ;
#31372=CARTESIAN_POINT ( 'NONE',  ( -0.3280839895013117347, -0.3690944881889763329, 0.3153832671262228327 ) ) ;
#31374=CARTESIAN_POINT ( 'NONE',  ( -0.6430446194225712953, -0.004921259842519870586, -0.3153832671262229437 ) ) ;
#31375=CARTESIAN_POINT ( 'NONE',  ( 0.6430446194225728496, -0.004921259842519576551, 0.3153832671262227771 ) ) ;
#31376=CARTESIAN_POINT ( 'NONE',  ( 0.1181102362204730916, -0.6692913385826771977, 8.415575281601705876E-17 ) ) ;
#31377=CARTESIAN_POINT ( 'NONE',  ( -0.5249343832020990641, 0.1283753931104748280, 0.1820866141732283561 ) ) ;
#31379=CARTESIAN_POINT ( 'NONE',  ( 1.108923884514436242, -0.05778040916215522460, 0.4822834645669289988 ) ) ;
#31380=CARTESIAN_POINT ( 'NONE',  ( -0.8661417322834640276, -0.1870078740157479769, 0.4822834645669291653 ) ) ;
#31382=CARTESIAN_POINT ( 'NONE',  ( -0.3871391076115479057, -0.3162353388693409650, -0.4822834645669289433 ) ) ;
#31383=CARTESIAN_POINT ( 'NONE',  ( -1.128608923884513837, 0.2306618581243847221, -0.2411417322834647770 ) ) ;
#31384=CARTESIAN_POINT ( 'NONE',  ( 1.102362204724410155, -0.1870078740157480601, -0.3641732283464567677 ) ) ;
#31385=CARTESIAN_POINT ( 'NONE',  ( -0.2362204724409442680, -0.1870078740157480601, -0.3641732283464567677 ) ) ;
#31386=CARTESIAN_POINT ( 'NONE',  ( -0.6299212598425188991, -0.1870078740157479769, 0.4822834645669291653 ) ) ;
#31387=CARTESIAN_POINT ( 'NONE',  ( -1.049868766404198794, -0.6046776061558807314, 0.2411417322834647770 ) ) ;
#31388=CARTESIAN_POINT ( 'NONE',  ( -0.4037097067573596210, -2.567464376874931580E-15, -0.4445507791589072832 ) ) ;
#31389=CARTESIAN_POINT ( 'NONE',  ( 1.108923884514436686, -0.2845877964562161244, -0.3641732283464567121 ) ) ;
#31390=CONICAL_SURFACE ( 'NONE', #78472, 3.543307086614173596, 1.047197551196599408 ) ;
#31391=CARTESIAN_POINT ( 'NONE',  ( -0.2296587926509179312, -0.05778040916215522460, 0.4822834645669289988 ) ) ;
#31392=CARTESIAN_POINT ( 'NONE',  ( -1.017060367454067249, -0.3162353388693409650, -0.4822834645669289433 ) ) ;
#31395=CARTESIAN_POINT ( 'NONE',  ( 1.076115485564305141, -0.6046776061558807314, 0.2411417322834647770 ) ) ;
#31396=CARTESIAN_POINT ( 'NONE',  ( -0.7086614173228339419, -0.1870078740157480601, -0.3641732283464567677 ) ) ;
#31398=CARTESIAN_POINT ( 'NONE',  ( -0.8792650918635160906, 0.05413385826771626580, -0.4176697321401330321 ) ) ;
#31399=CARTESIAN_POINT ( 'NONE',  ( 1.482939632545932307, -0.4281496062992124485, 0.4176697321401328655 ) ) ;
#31400=CARTESIAN_POINT ( 'NONE',  ( 0.8595800524934390507, -0.3162353388693405765, 0.4822834645669290543 ) ) ;
#31402=CARTESIAN_POINT ( 'NONE',  ( -0.9973753280839886548, -0.5023911411419708095, -0.1820866141732282451 ) ) ;
#31408=CARTESIAN_POINT ( 'NONE',  ( 1.292650918635171564, -0.5511811023622048555, -0.09757992244046775898 ) ) ;
#31409=CARTESIAN_POINT ( 'NONE',  ( 0.7874015748031503170, -0.1870078740157479769, 0.3641732283464567677 ) ) ;
#31410=CARTESIAN_POINT ( 'NONE',  ( 0.4396325459317590445, -0.6692913385826771977, 0.1292274648535927661 ) ) ;
#31411=CARTESIAN_POINT ( 'NONE',  ( 1.548556430446194954, -0.6046776061558807314, 0.2411417322834647770 ) ) ;
#31413=CARTESIAN_POINT ( 'NONE',  ( 0.7414698162729663755, 0.1771653543307087630, 0.09757992244046791164 ) ) ;
#31414=CARTESIAN_POINT ( 'NONE',  ( -0.4461942257217840213, -0.6046776061558809534, -0.2411417322834644161 ) ) ;
#31415=CARTESIAN_POINT ( 'NONE',  ( -1.174540682414697335, -0.05778040916215522460, 0.4822834645669289988 ) ) ;
#31416=CARTESIAN_POINT ( 'NONE',  ( 0.9317585301837276734, 0.05413385826771626580, -0.4176697321401330321 ) ) ;
#31418=CARTESIAN_POINT ( 'NONE',  ( -0.7480314960629914633, 0.2952755905511811885, 0.000000000000000000 ) ) ;
#31419=CARTESIAN_POINT ( 'NONE',  ( 0.1312335958005255154, -0.5023911411419708095, 0.1820866141732285504 ) ) ;
#31420=VERTEX_POINT ( 'NONE', #18014 ) ;
#31421=ORIENTED_EDGE ( 'NONE', *, *, #12583, .F. ) ;
#31422=CARTESIAN_POINT ( 'NONE',  ( -0.7480314960629914633, 0.2952755905511811885, 0.000000000000000000 ) ) ;
#31424=CARTESIAN_POINT ( 'NONE',  ( -0.6036745406824141069, -0.6046776061558809534, -0.2411417322834644161 ) ) ;
#31425=CARTESIAN_POINT ( 'NONE',  ( -0.9251968503937002541, -0.4536011799217368745, -0.2665933059059886201 ) ) ;
#31426=CARTESIAN_POINT ( 'NONE',  ( -0.7217847769028863381, -0.4281496062992124485, 0.4176697321401328655 ) ) ;
#31427=CARTESIAN_POINT ( 'NONE',  ( 0.2559055118110243332, 0.1660481256975885056, 0.3530559997133364547 ) ) ;
#31428=CARTESIAN_POINT ( 'NONE',  ( -0.3740157480314953431, 0.1660481256975885056, 0.3530559997133364547 ) ) ;
#31429=CARTESIAN_POINT ( 'NONE',  ( -1.391076115485563314, -0.6046776061558809534, -0.2411417322834644161 ) ) ;
#31430=CARTESIAN_POINT ( 'NONE',  ( -0.6102362204724400829, 0.1660481256975885056, 0.3530559997133364547 ) ) ;
#31431=CARTESIAN_POINT ( 'NONE',  ( 0.8661417322834652488, -0.1870078740157480879, -0.4822834645669291653 ) ) ;
#31433=CARTESIAN_POINT ( 'NONE',  ( -0.4986876640419939388, 0.1283753931104746893, -0.1820866141732285504 ) ) ;
#31436=ORIENTED_EDGE ( 'NONE', *, *, #22324, .F. ) ;
#31437=CARTESIAN_POINT ( 'NONE',  ( -1.207349081364828880, 0.1283753931104746893, -0.1820866141732285504 ) ) ;
#31438=CARTESIAN_POINT ( 'NONE',  ( -1.102362204724408601, -0.1870078740157480879, -0.4822834645669291653 ) ) ;
#31439=CARTESIAN_POINT ( 'NONE',  ( -1.017060367454067249, -0.05778040916215522460, 0.4822834645669289988 ) ) ;
#31441=CARTESIAN_POINT ( 'NONE',  ( -0.9580052493438311334, -0.4281496062992124485, 0.4176697321401328655 ) ) ;
#31442=CARTESIAN_POINT ( 'NONE',  ( -1.417322834645668772, -0.1870078740157479769, 0.4822834645669291653 ) ) ;
#31443=CARTESIAN_POINT ( 'NONE',  ( -1.620734908136482577, 0.2952755905511811885, 0.1292274648535926551 ) ) ;
#31445=CARTESIAN_POINT ( 'NONE',  ( 0.6299212598425204535, -0.1870078740157480601, -0.3641732283464567677 ) ) ;
#31448=CARTESIAN_POINT ( 'NONE',  ( 0.1181102362204730916, -0.5511811023622047445, 6.969142054262312111E-17 ) ) ;
#31450=CARTESIAN_POINT ( 'NONE',  ( -0.3083989501312330295, -0.3162353388693409650, -0.4822834645669289433 ) ) ;
#31451=CARTESIAN_POINT ( 'NONE',  ( 1.194225721784777594, -0.4281496062992127816, -0.4176697321401328100 ) ) ;
#31452=CARTESIAN_POINT ( 'NONE',  ( -0.5905511811023613777, -0.6692913385826771977, 8.415575281601705876E-17 ) ) ;
#31455=CARTESIAN_POINT ( 'NONE',  ( -1.614173228346456712, 2.401574803149606474, 0.1372047244094477536 ) ) ;
#31458=CARTESIAN_POINT ( 'NONE',  ( -0.7283464566929126471, -0.5400638737290844871, 0.3530559997133364547 ) ) ;
#31459=CARTESIAN_POINT ( 'NONE',  ( 1.397637795275591177, -0.5400638737290844871, 0.3530559997133364547 ) ) ;
#31460=CARTESIAN_POINT ( 'NONE',  ( -0.9514435695538050464, -0.2845877964562159024, 0.3641732283464567677 ) ) ;
#31461=CARTESIAN_POINT ( 'NONE',  ( -1.430446194225721390, -0.4281496062992124485, 0.4176697321401328655 ) ) ;
#31463=DIRECTION ( 'NONE',  ( 3.096699300667737957E-16, -1.000000000000000000, 0.000000000000000000 ) ) ;
#31465=CARTESIAN_POINT ( 'NONE',  ( 1.122047244094488860, -0.5400638737290845981, -0.3530559997133363437 ) ) ;
#31467=CARTESIAN_POINT ( 'NONE',  ( 0.04593175853018440641, -0.6692913385826771977, 0.1292274648535927661 ) ) ;
#31468=CARTESIAN_POINT ( 'NONE',  ( -0.9383202099737524282, -0.2845877964562161244, -0.3641732283464567121 ) ) ;
#31469=CARTESIAN_POINT ( 'NONE',  ( -0.2690288713910754526, 0.2952755905511810774, -0.1292274648535930714 ) ) ;
#31471=CARTESIAN_POINT ( 'NONE',  ( -0.9973753280839886548, -0.6046776061558809534, -0.2411417322834644161 ) ) ;
#31472=CARTESIAN_POINT ( 'NONE',  ( -0.7611548556430438595, 0.2306618581243848609, 0.2411417322834645549 ) ) ;
#31475=CARTESIAN_POINT ( 'NONE',  ( 0.6758530183727039509, 0.1771653543307087075, -0.09757992244046823083 ) ) ;
#31476=CARTESIAN_POINT ( 'NONE',  ( -0.1377952755905504645, 0.07958543189024085140, 0.2665933059059887866 ) ) ;
#31477=CARTESIAN_POINT ( 'NONE',  ( 0.7217847769028878924, -0.004921259842519576551, 0.3153832671262227771 ) ) ;
#31478=CARTESIAN_POINT ( 'NONE',  ( -1.391076115485563758, 0.2306618581243848609, 0.2411417322834645549 ) ) ;
#31479=CARTESIAN_POINT ( 'NONE',  ( 1.587926509186352142, 0.05413385826771666132, 0.4176697321401328100 ) ) ;
#31480=CARTESIAN_POINT ( 'NONE',  ( 0.5380577427821529035, -0.3690944881889763329, 0.3153832671262228327 ) ) ;
#31481=CARTESIAN_POINT ( 'NONE',  ( -0.8267716535433065062, 0.2952755905511811885, 0.000000000000000000 ) ) ;
#31482=CARTESIAN_POINT ( 'NONE',  ( 1.318897637795276356, 0.1660481256975883668, -0.3530559997133364547 ) ) ;
#31484=CARTESIAN_POINT ( 'NONE',  ( -0.1443569553805765515, -0.3690944881889765550, -0.3153832671262227771 ) ) ;
#31485=CARTESIAN_POINT ( 'NONE',  ( 0.06715429112991387617, 0.02791078216816508459, -0.4328096321851889194 ) ) ;
#31486=CARTESIAN_POINT ( 'NONE',  ( 0.1706036745406830368, -0.4281496062992127816, -0.4176697321401328100 ) ) ;
#31488=CARTESIAN_POINT ( 'NONE',  ( 1.522309711286089939, -0.5023911411419708095, -0.1820866141732282451 ) ) ;
#31489=CARTESIAN_POINT ( 'NONE',  ( 0.1509186351706042484, -0.2845877964562159024, 0.3641732283464567677 ) ) ;
#31490=CARTESIAN_POINT ( 'NONE',  ( -1.476377952755905110, -0.5400638737290845981, -0.3530559997133363437 ) ) ;
#31491=CARTESIAN_POINT ( 'NONE',  ( -0.1902887139107604098, 0.1771653543307087075, -0.09757992244046823083 ) ) ;
#31492=CARTESIAN_POINT ( 'NONE',  ( 1.034719704380073102, 4.339766966676338660E-16, 0.3954985857520057491 ) ) ;
#31493=CARTESIAN_POINT ( 'NONE',  ( -1.167979002624671470, -0.4281496062992127816, -0.4176697321401328100 ) ) ;
#31494=EDGE_CURVE ( 'NONE', #11380, #71856, #46981, .T. ) ;
#31495=CARTESIAN_POINT ( 'NONE',  ( -0.5183727034120726440, 0.2952755905511811885, 0.1292274648535926551 ) ) ;
#31497=EDGE_CURVE ( 'NONE', #5170, #9025, #37081, .T. ) ;
#31499=CARTESIAN_POINT ( 'NONE',  ( 0.7742782152230978099, -0.3690944881889763329, 0.3153832671262228327 ) ) ;
#31500=CARTESIAN_POINT ( 'NONE',  ( -0.5446194225721777693, -0.05778040916215522460, 0.4822834645669289988 ) ) ;
#31501=CARTESIAN_POINT ( 'NONE',  ( -0.5708661417322825615, -0.5400638737290844871, 0.3530559997133364547 ) ) ;
#31502=CARTESIAN_POINT ( 'NONE',  ( -0.8333333333333323711, 0.1771653543307087630, 0.09757992244046791164 ) ) ;
#31504=CARTESIAN_POINT ( 'NONE',  ( -0.2427821522309703550, -0.3162353388693405765, 0.4822834645669290543 ) ) ;
#31505=CARTESIAN_POINT ( 'NONE',  ( -1.646981627296586703, -0.2845877964562161244, -0.3641732283464567121 ) ) ;
#31506=CARTESIAN_POINT ( 'NONE',  ( 1.397637795275591177, -0.5400638737290844871, 0.3530559997133364547 ) ) ;
#31512=CARTESIAN_POINT ( 'NONE',  ( -1.272965879265091305, -0.4281496062992124485, 0.4176697321401328655 ) ) ;
#31513=CARTESIAN_POINT ( 'NONE',  ( -0.8989501312335946848, 0.2952755905511810774, -0.1292274648535930714 ) ) ;
#31515=CARTESIAN_POINT ( 'NONE',  ( -1.509186351706035767, -0.4281496062992124485, 0.4176697321401328655 ) ) ;
#31519=CARTESIAN_POINT ( 'NONE',  ( 0.7874015748031503170, -0.1870078740157480879, -0.4822834645669291653 ) ) ;
#31520=CARTESIAN_POINT ( 'NONE',  ( 0.02624671916010564918, -0.6046776061558809534, -0.2411417322834644161 ) ) ;
#31523=CARTESIAN_POINT ( 'NONE',  ( 1.371391076115485719, -0.5511811023622048555, -0.09757992244046775898 ) ) ;
#31529=CARTESIAN_POINT ( 'NONE',  ( 0.5643044619422579178, -0.4281496062992127816, -0.4176697321401328100 ) ) ;
#31530=CARTESIAN_POINT ( 'NONE',  ( -0.7939632545931754048, -0.3162353388693405765, 0.4822834645669290543 ) ) ;
#31531=CARTESIAN_POINT ( 'NONE',  ( -1.601049868766403650, 0.2306618581243847221, -0.2411417322834647770 ) ) ;
#31532=CARTESIAN_POINT ( 'NONE',  ( 0.8202099737532814183, -0.6692913385826773087, -0.1292274648535924053 ) ) ;
#31533=CARTESIAN_POINT ( 'NONE',  ( -1.614173228346455824, 0.1771653543307087630, 0.000000000000000000 ) ) ;
#31534=CARTESIAN_POINT ( 'NONE',  ( 1.548556430446194954, -0.6046776061558807314, 0.2411417322834647770 ) ) ;
#31535=CARTESIAN_POINT ( 'NONE',  ( -0.2559055118110227234, -0.5400638737290844871, 0.3530559997133364547 ) ) ;
#31536=CARTESIAN_POINT ( 'NONE',  ( -1.056430446194224881, -0.6692913385826771977, 0.1292274648535927661 ) ) ;
#31537=CARTESIAN_POINT ( 'NONE',  ( 1.568241469816273437, -0.3162353388693405765, 0.4822834645669290543 ) ) ;
#31538=CARTESIAN_POINT ( 'NONE',  ( 1.522309711286089939, 0.2306618581243848609, 0.2411417322834645549 ) ) ;
#31540=CARTESIAN_POINT ( 'NONE',  ( 0.6889763779527566800, -0.4536011799217367080, 0.2665933059059888421 ) ) ;
#31544=CARTESIAN_POINT ( 'NONE',  ( -0.07217847769028813698, -0.2845877964562161244, -0.3641732283464567121 ) ) ;
#31546=CARTESIAN_POINT ( 'NONE',  ( 0.2493438320209980519, -0.4281496062992127816, -0.4176697321401328100 ) ) ;
#31547=CARTESIAN_POINT ( 'NONE',  ( 0.6102362204724416372, -0.5400638737290844871, 0.3530559997133364547 ) ) ;
#31548=CARTESIAN_POINT ( 'NONE',  ( -0.6496062992125976043, -0.5400638737290844871, 0.3530559997133364547 ) ) ;
#31550=CARTESIAN_POINT ( 'NONE',  ( -1.299212598425196097, 0.2952755905511811885, 0.000000000000000000 ) ) ;
#31552=CARTESIAN_POINT ( 'NONE',  ( 1.167979002624672580, -0.004921259842519870586, -0.3153832671262229437 ) ) ;
#31553=CARTESIAN_POINT ( 'NONE',  ( 0.9186351706036752773, 0.2306618581243847221, -0.2411417322834647770 ) ) ;
#31554=CARTESIAN_POINT ( 'NONE',  ( 0.6955380577427828781, -0.4281496062992124485, 0.4176697321401328655 ) ) ;
#31556=CARTESIAN_POINT ( 'NONE',  ( -1.272965879265091305, -0.4281496062992124485, 0.4176697321401328655 ) ) ;
#31559=CARTESIAN_POINT ( 'NONE',  ( -0.3280839895013117347, -0.4281496062992124485, 0.4176697321401328655 ) ) ;
#31562=CARTESIAN_POINT ( 'NONE',  ( 1.082677165354331228, -0.5400638737290844871, 0.3530559997133364547 ) ) ;
#31563=CARTESIAN_POINT ( 'NONE',  ( 1.325459317585302665, -0.4281496062992124485, 0.4176697321401328655 ) ) ;
#31564=CARTESIAN_POINT ( 'NONE',  ( 0.3346456692913393205, -0.4536011799217368745, -0.2665933059059886201 ) ) ;
#31565=CARTESIAN_POINT ( 'NONE',  ( 0.6955380577427828781, 0.05413385826771626580, -0.4176697321401330321 ) ) ;
#31567=CARTESIAN_POINT ( 'NONE',  ( 0.3477690288713918276, -0.5511811023622048555, -0.09757992244046775898 ) ) ;
#31568=( BOUNDED_SURFACE ( )  B_SPLINE_SURFACE ( 1, 2, ( 
 ( #70129, #12480, #56666, #5339, #57490, #63816, #37731, #82366, #4508, #5740, #31411, #30176, #75227, #24685, #50352, #76465, #18791, #6574, #25925, #58327, #689, #46117, #20880, #71811, #33506, #72232, #77285, #45692, #14162, #33086, #12900, #70973, #51583, #32245, #46947, #45278, #14581, #19616, #26345, #78555, #32660, #13318, #7839, #53262, #38559, #8254, #20464, #1940, #1526, #58753, #65917, #40234, #46532, #38971, #64654, #6992, #33918, #13738, #78131, #59168, #59583, #27602, #52006, #27180, #78973, #52844, #21294, #64239, #57905, #270, #77711, #20041, #71389, #7416, #52421, #39394, #65078, #1115, #26766, #39818, #65507, #9909, #47781, #9496, #53675, #28846, #22945, #23357, #34339, #8668, #2359, #9089, #15406, #16654, #54927, #73483, #55335, #73056, #47365, #29673, #72639, #16236, #74307, #35998, #79383, #48201, #21702, #73896, #41066, #29263, #66755, #34761, #41884, #14988, #79806, #60421, #81044, #40646, #61668, #67577, #22538, #4009, #35581, #66330, #60004, #22122, #15833, #67166, #3182, #61244, #28015, #80634, #42294, #54508, #3598, #2772, #28432, #54091, #41481, #35169, #60830, #80222, #48613, #67991, #10336, #81455, #55747, #23772, #64450, #30906, #50260, #38773, #49443, #75137, #32458, #11571, #13122, #75958, #17482, #24592, #6786, #487, #5242, #37230, #43113, #26142, #30502, #17888, #49849, #19417, #56165, #45068, #4416, #68809, #19843, #70771, #51803, #42710, #81868, #24180, #77508, #71189, #17073, #11156, #64871, #58120, #32881, #68406, #62078, #36814, #62490, #82274, #45492, #13531, #39187, #7211, #30085, #75548, #58550, #69223, #49028, #4824, #43525, #10746, #916, #62907, #74724, #56573, #36403, #8880, #46334, #33314, #21506, #66967, #52226, #21920, #34138, #15624, #15204, #72446, #79604, #53890, #34556, #26981, #60222, #2153, #66131, #8468, #1332, #8060, #7644, #52646, #78350, #60633, #2572, #40452, #33721, #72027, #47582, #27820, #59383, #78770, #59799, #21094, #41281, #45909, #73276, #9300, #34970, #26573, #72856, #20682, #1741, #40865, #77929, #28231, #53058, #14795, #46753, #27398, #66547, #71606, #20260, #53480, #79190, #40041, #13959, #39616, #65305, #58976, #47164, #14383, #65727, #16869, #48822, #67794, #41684, #61462, #29877, #75339, #49647, #17686, #23564, #9711, #67377, #74522, #48406, #29060, #3397, #42097, #22339, #35382, #80020, #10946, #62281, #36603, #43316, #69014, #4619, #30290, #23153, #3810, #55956, #81669, #4213, #42506, #2984, #55539, #68208, #47999, #11366, #37023, #28649, #49235, #61047, #54731, #10545, #74106, #80436, #22746, #10131, #73698, #16452, #16038, #23979, #54309, #35795, #29472, #55130, #80840, #36203, #61872, #81249, #74938, #17283, #42911, #68606, #62704, #18902, #82888, #56375, #82074, #69432, #13019, #76574, #64351, #24387, #75753, #56778, #82478, #50874, #57606, #44552, #12597, #25619, #43728, #18503, #70242, #63523, #5043, #37438, #18094, #50058, #30712, #76166, #11785, #24794, #31530, #6688, #5853, #44146, #44967, #63112, #31111, #5450, #38673, #50462, #69838, #12188, #37845, #57186, #25208, #70663, #38256, #63933, #6269, #31945, #83297, #51282, #76985, #19314, #57154, #12155, #37812, #65484, #1502, #11752, #63080, #71782, #63488, #44520, #1090, #7816, #27154, #43695, #58727, #59144, #52396, #78529, #26742, #20853, #72205, #33482, #52818, #69400, #82853, #18871, #82041, #24355, #50023, #5822, #39789, #14137, #78105, #31493, #25174, #37408, #70208, #46505, #14558, #75722, #18062, #5418, #82445, #31080, #62670, #46090, #44115, #50843, #76543, #7389, #69807, #20436, #56747, #24762, #13712, #39366, #65051, #33056, #5010, #30680, #56341, #50430, #76130, #18472, #48175, #41040, #22094, #60803, #41858, #61217, #21267, #35141, #35554, #28820, #54903, #3157, #80609, #48586, #67550, #9885, #46922, #34734, #79778, #59558, #1913, #27576, #66725, #16211, #73871, #54485, #15378, #60394, #72615, #47755, #3572, #74283, #53233, #78949, #14963, #59975, #66303, #29239, #22514, #9062, #22919, #40620, #8642, #40210, #65893, #67138, #8228, #33892, #34314, #15803, #2334, #41454, #27990, #80196, #53650, #79358 ),
 ( #2745, #28405, #54063, #21677, #47338, #73028, #73453, #9467, #17864, #16627, #82654, #67966, #74701, #75113, #5626, #81019, #17046, #42686, #68384, #49002, #23332, #10723, #30882, #81845, #43499, #5218, #36380, #62054, #82250, #62464, #62883, #69197, #4392, #75525, #56549, #50235, #56140, #4799, #30060, #75931, #24568, #17459, #24156, #37202, #18272, #37611, #55721, #11546, #11956, #43912, #31292, #69610, #56957, #24969, #63286, #50641, #81431, #11130, #49825, #35974, #61644, #3985, #43089, #42269, #10308, #29649, #68786, #36788, #23746, #55311, #49419, #30476, #38023, #12365, #6038, #12781, #19080, #20339, #58629, #77166, #59053, #76750, #51049, #33391, #76345, #19926, #78011, #39696, #83065, #51888, #25386, #77592, #44728, #32962, #70425, #38438, #45576, #27063, #148, #64121, #1407, #18675, #65387, #71269, #26224, #7722, #13616, #44320, #70010, #25803, #51464, #70855, #6870, #39270, #63699, #997, #45991, #32539, #64952, #31710, #57370, #6456, #32126, #19498, #57784, #45152, #13206, #38853, #64533, #58203, #571, #7292, #26651, #52305, #71687, #14039, #59466, #53137, #35043, #15284, #15702, #79682, #21175, #28307, #41359, #3057, #8962, #40945, #78848, #28724, #34216, #21581, #53558, #21998, #59879, #47659, #8136, #46830, #79266, #66624, #27897, #47244, #2233, #72933, #54386, #73775, #1817, #72522, #22416, #34636, #53969, #52722, #35454, #20761, #27479, #60300, #41755, #33801, #14871, #40532, #66211, #8549, #2650, #73354, #67040, #9372, #60708, #80097, #48073, #16111, #67450, #9784, #61120, #3471, #78433, #46411, #72105, #14463, #40115, #65803, #55207, #5116, #10621, #81326, #29951, #56034, #36277, #24052, #67868, #80915, #55615, #17358, #4289, #23640, #61949, #49310, #30783, #50128, #61541, #29545, #37097, #75012, #11023, #49722, #56445, #75828, #10206, #75419, #24463, #17762, #43802, #43393, #69506, #37508, #82147, #18169, #35874, #42987, #68681, #48481, #74182, #16529, #36680, #11855, #62782, #69093, #62355, #4693, #3885, #30367, #63183, #29138, #42173, #23228, #48898, #74600, #16943, #54804, #11441, #81742, #80508, #42585, #68285, #22823, #5522, #32434, #7185, #52201, #12261, #64428, #37919, #6762, #5931, #45468, #31602, #63595, #58097, #39590, #12674, #57262, #71582, #31187, #77905, #462, #38751, #20236, #26118, #45884, #13933, #38334, #64009, #43, #19394, #51780, #56852, #71166, #58525, #69907, #25696, #45045, #24868, #50536, #76240, #32021, #64847, #13506, #77484, #6350, #51357, #82961, #70746, #39162, #82549, #18574, #44217, #25279, #50947, #76644, #32856, #891, #57681, #18975, #44624, #70320, #77060, #13098, #19819, #26548, #28627, #72005, #40839, #14361, #66524, #65706, #21895, #8035, #40018, #34534, #16018, #72422, #33699, #47977, #65279, #54284, #60199, #15182, #80000, #8856, #22314, #73677, #14772, #40427, #59775, #79166, #2550, #7618, #47558, #34949, #21483, #28208, #33291, #58951, #1309, #59359, #66108, #26958, #46311, #1718, #27373, #53034, #78747, #21072, #46730, #79580, #47142, #53867, #73251, #8444, #34114, #15600, #27798, #41260, #66946, #2130, #9278, #60612, #2961, #72832, #53458, #52622, #78327, #20658, #10524, #42481, #68584, #23133, #36582, #80413, #67770, #68185, #29855, #16846, #36179, #74499, #61851, #43295, #62680, #74083, #42075, #49624, #4192, #23542, #62261, #68992, #5022, #22725, #4597, #37001, #30268, #56353, #55932, #82052, #50035, #11342, #75317, #74916, #81647, #17664, #48384, #55518, #17261, #81226, #41664, #16429, #10107, #61022, #75732, #35770, #30690, #54707, #3787, #23956, #61440, #29451, #24365, #67355, #9688, #35359, #49211, #3372, #29036, #42890, #55109, #80818, #48801, #10925, #363, #76963, #57584, #83275, #76142, #12166, #7086, #63910, #52098, #18072, #51678, #31923, #25186, #37823, #13410, #19292, #50853, #70219, #51261, #12575, #32757, #37418, #64748, #58424, #39065, #785, #64329, #18483, #76553, #32337, #69410, #77381, #44530, #6246, #38232, #82864, #57999, #63091, #11764, #44943, #25598, #31505, #26445, #5429, #31090, #56757, #70640, #69817, #26019, #12996, #38652, #18881, #82457, #6665, #19712 ) ),
 .UNSPECIFIED., .F., .F., .F. ) 
 B_SPLINE_SURFACE_WITH_KNOTS ( ( 2, 2 ),
 ( 3, 2, 2, 2, 2, 2, 2, 2, 2, 2, 2, 2, 2, 2, 2, 2, 2, 2, 2, 2, 2, 2, 2, 2, 2, 2, 2, 2, 2, 2, 2, 2, 2, 2, 2, 2, 2, 2, 2, 2, 2, 2, 2, 2, 2, 2, 2, 2, 2, 2, 2, 2, 2, 2, 2, 2, 2, 2, 2, 2, 2, 2, 2, 2, 2, 2, 2, 2, 2, 2, 2, 2, 2, 2, 2, 2, 2, 2, 2, 2, 2, 2, 2, 2, 2, 2, 2, 2, 2, 2, 2, 2, 2, 2, 2, 2, 2, 2, 2, 2, 2, 2, 2, 2, 2, 2, 2, 2, 2, 2, 2, 2, 2, 2, 2, 2, 2, 2, 2, 2, 2, 2, 2, 2, 2, 2, 2, 2, 2, 2, 2, 2, 2, 2, 2, 2, 2, 2, 2, 2, 2, 2, 2, 2, 2, 2, 2, 2, 2, 2, 2, 2, 2, 2, 2, 2, 2, 2, 2, 2, 2, 2, 2, 2, 2, 2, 2, 2, 2, 2, 2, 2, 2, 2, 2, 2, 2, 2, 2, 2, 2, 2, 2, 2, 2, 2, 2, 2, 2, 2, 2, 2, 2, 2, 2, 2, 2, 2, 2, 2, 2, 2, 2, 2, 2, 2, 2, 2, 2, 2, 2, 2, 2, 2, 2, 2, 2, 2, 2, 2, 2, 2, 2, 2, 2, 2, 2, 2, 2, 2, 2, 2, 2, 2, 2, 2, 2, 2, 2, 2, 2, 2, 2, 2, 2, 2, 2, 2, 2, 2, 2, 2, 2, 2, 2, 3 ),
 ( 0.000000000000000000, 1.000000000000000000 ),
 ( 0.000000000000000000, 0.003787878787878787984, 0.007575757575757575968, 0.01136363636363636395, 0.01515151515151515194, 0.01893939393939393992, 0.02272727272727272790, 0.02651515151515151589, 0.03030303030303030387, 0.03409090909090908839, 0.03787878787878787984, 0.04166666666666666435, 0.04545454545454545581, 0.04924242424242424032, 0.05303030303030303177, 0.05681818181818181629, 0.06060606060606060774, 0.06439393939393939226, 0.06818181818181817677, 0.07196969696969697516, 0.07575757575757575968, 0.07954545454545454419, 0.08333333333333332871, 0.08712121212121212710, 0.09090909090909091161, 0.09469696969696969613, 0.09848484848484848064, 0.1022727272727272790, 0.1060606060606060635, 0.1098484848484848481, 0.1136363636363636326, 0.1174242424242424310, 0.1212121212121212155, 0.1250000000000000000, 0.1287878787878787845, 0.1325757575757575690, 0.1363636363636363535, 0.1401515151515151381, 0.1439393939393939503, 0.1477272727272727348, 0.1515151515151515194, 0.1553030303030303039, 0.1590909090909090884, 0.1628787878787878729, 0.1666666666666666574, 0.1704545454545454419, 0.1742424242424242542, 0.1780303030303030387, 0.1818181818181818232, 0.1856060606060606077, 0.1893939393939393923, 0.1931818181818181768, 0.1969696969696969613, 0.2007575757575757458, 0.2045454545454545581, 0.2083333333333333426, 0.2121212121212121271, 0.2159090909090909116, 0.2196969696969696961, 0.2234848484848484806, 0.2272727272727272652, 0.2310606060606060497, 0.2348484848484848619, 0.2386363636363636465, 0.2424242424242424310, 0.2462121212121212155, 0.2500000000000000000, 0.2537878787878787845, 0.2575757575757575690, 0.2613636363636363535, 0.2651515151515151381, 0.2689393939393939226, 0.2727272727272727071, 0.2765151515151514916, 0.2803030303030302761, 0.2840909090909091161, 0.2878787878787879007, 0.2916666666666666852, 0.2954545454545454697, 0.2992424242424242542, 0.3030303030303030387, 0.3068181818181818232, 0.3106060606060606077, 0.3143939393939393923, 0.3181818181818181768, 0.3219696969696969613, 0.3257575757575757458, 0.3295454545454545303, 0.3333333333333333148, 0.3371212121212120993, 0.3409090909090908839, 0.3446969696969697239, 0.3484848484848485084, 0.3522727272727272929, 0.3560606060606060774, 0.3598484848484848619, 0.3636363636363636465, 0.3674242424242424310, 0.3712121212121212155, 0.3750000000000000000, 0.3787878787878787845, 0.3825757575757575690, 0.3863636363636363535, 0.3901515151515151381, 0.3939393939393939226, 0.3977272727272727071, 0.4015151515151514916, 0.4053030303030302761, 0.4090909090909091161, 0.4128787878787879007, 0.4166666666666666852, 0.4204545454545454697, 0.4242424242424242542, 0.4280303030303030387, 0.4318181818181818232, 0.4356060606060606077, 0.4393939393939393923, 0.4431818181818181768, 0.4469696969696969613, 0.4507575757575757458, 0.4545454545454545303, 0.4583333333333333148, 0.4621212121212120993, 0.4659090909090908839, 0.4696969696969697239, 0.4734848484848485084, 0.4772727272727272929, 0.4810606060606060774, 0.4848484848484848619, 0.4886363636363636465, 0.4924242424242424310, 0.4962121212121212155, 0.5000000000000000000, 0.5037878787878787845, 0.5075757575757575690, 0.5113636363636363535, 0.5151515151515151381, 0.5189393939393939226, 0.5227272727272727071, 0.5265151515151514916, 0.5303030303030302761, 0.5340909090909090606, 0.5378787878787878451, 0.5416666666666666297, 0.5454545454545454142, 0.5492424242424241987, 0.5530303030303029832, 0.5568181818181817677, 0.5606060606060605522, 0.5643939393939394478, 0.5681818181818182323, 0.5719696969696970168, 0.5757575757575758013, 0.5795454545454545858, 0.5833333333333333703, 0.5871212121212121549, 0.5909090909090909394, 0.5946969696969697239, 0.5984848484848485084, 0.6022727272727272929, 0.6060606060606060774, 0.6098484848484848619, 0.6136363636363636465, 0.6174242424242424310, 0.6212121212121212155, 0.6250000000000000000, 0.6287878787878787845, 0.6325757575757575690, 0.6363636363636363535, 0.6401515151515151381, 0.6439393939393939226, 0.6477272727272727071, 0.6515151515151514916, 0.6553030303030302761, 0.6590909090909090606, 0.6628787878787878451, 0.6666666666666666297, 0.6704545454545454142, 0.6742424242424241987, 0.6780303030303029832, 0.6818181818181817677, 0.6856060606060605522, 0.6893939393939394478, 0.6931818181818182323, 0.6969696969696970168, 0.7007575757575758013, 0.7045454545454545858, 0.7083333333333333703, 0.7121212121212121549, 0.7159090909090909394, 0.7196969696969697239, 0.7234848484848485084, 0.7272727272727272929, 0.7310606060606060774, 0.7348484848484848619, 0.7386363636363636465, 0.7424242424242424310, 0.7462121212121212155, 0.7500000000000000000, 0.7537878787878787845, 0.7575757575757575690, 0.7613636363636363535, 0.7651515151515151381, 0.7689393939393939226, 0.7727272727272727071, 0.7765151515151514916, 0.7803030303030302761, 0.7840909090909090606, 0.7878787878787878451, 0.7916666666666666297, 0.7954545454545454142, 0.7992424242424241987, 0.8030303030303029832, 0.8068181818181817677, 0.8106060606060605522, 0.8143939393939394478, 0.8181818181818182323, 0.8219696969696970168, 0.8257575757575758013, 0.8295454545454545858, 0.8333333333333333703, 0.8371212121212121549, 0.8409090909090909394, 0.8446969696969697239, 0.8484848484848485084, 0.8522727272727272929, 0.8560606060606060774, 0.8598484848484848619, 0.8636363636363636465, 0.8674242424242424310, 0.8712121212121212155, 0.8750000000000000000, 0.8787878787878787845, 0.8825757575757575690, 0.8863636363636363535, 0.8901515151515151381, 0.8939393939393939226, 0.8977272727272727071, 0.9015151515151514916, 0.9053030303030302761, 0.9090909090909090606, 0.9128787878787878451, 0.9166666666666666297, 0.9204545454545454142, 0.9242424242424241987, 0.9280303030303029832, 0.9318181818181817677, 0.9356060606060605522, 0.9393939393939394478, 0.9431818181818182323, 0.9469696969696970168, 0.9507575757575758013, 0.9545454545454545858, 0.9583333333333333703, 0.9621212121212121549, 0.9659090909090909394 ),
 .UNSPECIFIED. ) 
 GEOMETRIC_REPRESENTATION_ITEM ( )  RATIONAL_B_SPLINE_SURFACE ( (
 ( 1.000000000000000000, 0.9659258262890683122, 1.000000000000000000, 0.9659258262890683122, 1.000000000000000000, 0.9659258262890683122, 1.000000000000000000, 0.9659258262890683122, 1.000000000000000000, 0.9659258262890683122, 1.000000000000000000, 0.9659258262890683122, 1.000000000000000000, 0.9659258262890683122, 1.000000000000000000, 0.9659258262890683122, 1.000000000000000000, 0.9659258262890683122, 1.000000000000000000, 0.9659258262890683122, 1.000000000000000000, 0.9659258262890683122, 1.000000000000000000, 0.9659258262890683122, 1.000000000000000000, 0.9659258262890683122, 1.000000000000000000, 0.9659258262890683122, 1.000000000000000000, 0.9659258262890683122, 1.000000000000000000, 0.9659258262890683122, 1.000000000000000000, 0.9659258262890683122, 1.000000000000000000, 0.9659258262890683122, 1.000000000000000000, 0.9659258262890683122, 1.000000000000000000, 0.9659258262890683122, 1.000000000000000000, 0.9659258262890683122, 1.000000000000000000, 0.9659258262890683122, 1.000000000000000000, 0.9659258262890683122, 1.000000000000000000, 0.9659258262890683122, 1.000000000000000000, 0.9659258262890683122, 1.000000000000000000, 0.9659258262890683122, 1.000000000000000000, 0.9659258262890683122, 1.000000000000000000, 0.9659258262890683122, 1.000000000000000000, 0.9659258262890683122, 1.000000000000000000, 0.9659258262890683122, 1.000000000000000000, 0.9659258262890683122, 1.000000000000000000, 0.9659258262890683122, 1.000000000000000000, 0.9659258262890683122, 1.000000000000000000, 0.9659258262890683122, 1.000000000000000000, 0.9659258262890683122, 1.000000000000000000, 0.9659258262890683122, 1.000000000000000000, 0.9659258262890683122, 1.000000000000000000, 0.9659258262890683122, 1.000000000000000000, 0.9659258262890683122, 1.000000000000000000, 0.9659258262890683122, 1.000000000000000000, 0.9659258262890683122, 1.000000000000000000, 0.9659258262890683122, 1.000000000000000000, 0.9659258262890683122, 1.000000000000000000, 0.9659258262890683122, 1.000000000000000000, 0.9659258262890683122, 1.000000000000000000, 0.9659258262890683122, 1.000000000000000000, 0.9659258262890683122, 1.000000000000000000, 0.9659258262890683122, 1.000000000000000000, 0.9659258262890683122, 1.000000000000000000, 0.9659258262890683122, 1.000000000000000000, 0.9659258262890683122, 1.000000000000000000, 0.9659258262890683122, 1.000000000000000000, 0.9659258262890683122, 1.000000000000000000, 0.9659258262890683122, 1.000000000000000000, 0.9659258262890683122, 1.000000000000000000, 0.9659258262890683122, 1.000000000000000000, 0.9659258262890683122, 1.000000000000000000, 0.9659258262890683122, 1.000000000000000000, 0.9659258262890683122, 1.000000000000000000, 0.9659258262890683122, 1.000000000000000000, 0.9659258262890683122, 1.000000000000000000, 0.9659258262890683122, 1.000000000000000000, 0.9659258262890683122, 1.000000000000000000, 0.9659258262890683122, 1.000000000000000000, 0.9659258262890683122, 1.000000000000000000, 0.9659258262890683122, 1.000000000000000000, 0.9659258262890683122, 1.000000000000000000, 0.9659258262890683122, 1.000000000000000000, 0.9659258262890683122, 1.000000000000000000, 0.9659258262890683122, 1.000000000000000000, 0.9659258262890683122, 1.000000000000000000, 0.9659258262890683122, 1.000000000000000000, 0.9659258262890683122, 1.000000000000000000, 0.9659258262890683122, 1.000000000000000000, 0.9659258262890683122, 1.000000000000000000, 0.9659258262890683122, 1.000000000000000000, 0.9659258262890683122, 1.000000000000000000, 0.9659258262890683122, 1.000000000000000000, 0.9659258262890683122, 1.000000000000000000, 0.9659258262890683122, 1.000000000000000000, 0.9659258262890683122, 1.000000000000000000, 0.9659258262890683122, 1.000000000000000000, 0.9659258262890683122, 1.000000000000000000, 0.9659258262890683122, 1.000000000000000000, 0.9659258262890683122, 1.000000000000000000, 0.9659258262890683122, 1.000000000000000000, 0.9659258262890683122, 1.000000000000000000, 0.9659258262890683122, 1.000000000000000000, 0.9659258262890683122, 1.000000000000000000, 0.9659258262890683122, 1.000000000000000000, 0.9659258262890683122, 1.000000000000000000, 0.9659258262890683122, 1.000000000000000000, 0.9659258262890683122, 1.000000000000000000, 0.9659258262890683122, 1.000000000000000000, 0.9659258262890683122, 1.000000000000000000, 0.9659258262890683122, 1.000000000000000000, 0.9659258262890683122, 1.000000000000000000, 0.9659258262890683122, 1.000000000000000000, 0.9659258262890683122, 1.000000000000000000, 0.9659258262890683122, 1.000000000000000000, 0.9659258262890683122, 1.000000000000000000, 0.9659258262890683122, 1.000000000000000000, 0.9659258262890683122, 1.000000000000000000, 0.9659258262890683122, 1.000000000000000000, 0.9659258262890683122, 1.000000000000000000, 0.9659258262890683122, 1.000000000000000000, 0.9659258262890683122, 1.000000000000000000, 0.9659258262890683122, 1.000000000000000000, 0.9659258262890683122, 1.000000000000000000, 0.9659258262890683122, 1.000000000000000000, 0.9659258262890683122, 1.000000000000000000, 0.9659258262890683122, 1.000000000000000000, 0.9659258262890683122, 1.000000000000000000, 0.9659258262890683122, 1.000000000000000000, 0.9659258262890683122, 1.000000000000000000, 0.9659258262890683122, 1.000000000000000000, 0.9659258262890683122, 1.000000000000000000, 0.9659258262890683122, 1.000000000000000000, 0.9659258262890683122, 1.000000000000000000, 0.9659258262890683122, 1.000000000000000000, 0.9659258262890683122, 1.000000000000000000, 0.9659258262890683122, 1.000000000000000000, 0.9659258262890683122, 1.000000000000000000, 0.9659258262890683122, 1.000000000000000000, 0.9659258262890683122, 1.000000000000000000, 0.9659258262890683122, 1.000000000000000000, 0.9659258262890683122, 1.000000000000000000, 0.9659258262890683122, 1.000000000000000000, 0.9659258262890683122, 1.000000000000000000, 0.9659258262890683122, 1.000000000000000000, 0.9659258262890683122, 1.000000000000000000, 0.9659258262890683122, 1.000000000000000000, 0.9659258262890683122, 1.000000000000000000, 0.9659258262890683122, 1.000000000000000000, 0.9659258262890683122, 1.000000000000000000, 0.9659258262890683122, 1.000000000000000000, 0.9659258262890683122, 1.000000000000000000, 0.9659258262890683122, 1.000000000000000000, 0.9659258262890683122, 1.000000000000000000, 0.9659258262890683122, 1.000000000000000000, 0.9659258262890683122, 1.000000000000000000, 0.9659258262890683122, 1.000000000000000000, 0.9659258262890683122, 1.000000000000000000, 0.9659258262890683122, 1.000000000000000000, 0.9659258262890683122, 1.000000000000000000, 0.9659258262890683122, 1.000000000000000000, 0.9659258262890683122, 1.000000000000000000, 0.9659258262890683122, 1.000000000000000000, 0.9659258262890683122, 1.000000000000000000, 0.9659258262890683122, 1.000000000000000000, 0.9659258262890683122, 1.000000000000000000, 0.9659258262890683122, 1.000000000000000000, 0.9659258262890683122, 1.000000000000000000, 0.9659258262890683122, 1.000000000000000000, 0.9659258262890683122, 1.000000000000000000, 0.9659258262890683122, 1.000000000000000000, 0.9659258262890683122, 1.000000000000000000, 0.9659258262890683122, 1.000000000000000000, 0.9659258262890683122, 1.000000000000000000, 0.9659258262890683122, 1.000000000000000000, 0.9659258262890683122, 1.000000000000000000, 0.9659258262890683122, 1.000000000000000000, 0.9659258262890683122, 1.000000000000000000, 0.9659258262890683122, 1.000000000000000000, 0.9659258262890683122, 1.000000000000000000, 0.9659258262890683122, 1.000000000000000000, 0.9659258262890683122, 1.000000000000000000, 0.9659258262890683122, 1.000000000000000000, 0.9659258262890683122, 1.000000000000000000, 0.9659258262890683122, 1.000000000000000000, 0.9659258262890683122, 1.000000000000000000, 0.9659258262890683122, 1.000000000000000000, 0.9659258262890683122, 1.000000000000000000, 0.9659258262890683122, 1.000000000000000000, 0.9659258262890683122, 1.000000000000000000, 0.9659258262890683122, 1.000000000000000000, 0.9659258262890683122, 1.000000000000000000, 0.9659258262890683122, 1.000000000000000000, 0.9659258262890683122, 1.000000000000000000, 0.9659258262890683122, 1.000000000000000000, 0.9659258262890683122, 1.000000000000000000, 0.9659258262890683122, 1.000000000000000000, 0.9659258262890683122, 1.000000000000000000, 0.9659258262890683122, 1.000000000000000000, 0.9659258262890683122, 1.000000000000000000, 0.9659258262890683122, 1.000000000000000000, 0.9659258262890683122, 1.000000000000000000, 0.9659258262890683122, 1.000000000000000000, 0.9659258262890683122, 1.000000000000000000, 0.9659258262890683122, 1.000000000000000000, 0.9659258262890683122, 1.000000000000000000, 0.9659258262890683122, 1.000000000000000000, 0.9659258262890683122, 1.000000000000000000, 0.9659258262890683122, 1.000000000000000000, 0.9659258262890683122, 1.000000000000000000, 0.9659258262890683122, 1.000000000000000000, 0.9659258262890683122, 1.000000000000000000, 0.9659258262890683122, 1.000000000000000000, 0.9659258262890683122, 1.000000000000000000, 0.9659258262890683122, 1.000000000000000000, 0.9659258262890683122, 1.000000000000000000, 0.9659258262890683122, 1.000000000000000000, 0.9659258262890683122, 1.000000000000000000, 0.9659258262890683122, 1.000000000000000000, 0.9659258262890683122, 1.000000000000000000, 0.9659258262890683122, 1.000000000000000000, 0.9659258262890683122, 1.000000000000000000, 0.9659258262890683122, 1.000000000000000000, 0.9659258262890683122, 1.000000000000000000, 0.9659258262890683122, 1.000000000000000000, 0.9659258262890683122, 1.000000000000000000, 0.9659258262890683122, 1.000000000000000000, 0.9659258262890683122, 1.000000000000000000, 0.9659258262890683122, 1.000000000000000000, 0.9659258262890683122, 1.000000000000000000, 0.9659258262890683122, 1.000000000000000000, 0.9659258262890683122, 1.000000000000000000, 0.9659258262890683122, 1.000000000000000000, 0.9659258262890683122, 1.000000000000000000, 0.9659258262890683122, 1.000000000000000000, 0.9659258262890683122, 1.000000000000000000, 0.9659258262890683122, 1.000000000000000000, 0.9659258262890683122, 1.000000000000000000, 0.9659258262890683122, 1.000000000000000000, 0.9659258262890683122, 1.000000000000000000, 0.9659258262890683122, 1.000000000000000000, 0.9659258262890683122, 1.000000000000000000, 0.9659258262890683122, 1.000000000000000000, 0.9659258262890683122, 1.000000000000000000, 0.9659258262890683122, 1.000000000000000000, 0.9659258262890683122, 1.000000000000000000, 0.9659258262890683122, 1.000000000000000000, 0.9659258262890683122, 1.000000000000000000, 0.9659258262890683122, 1.000000000000000000, 0.9659258262890683122, 1.000000000000000000, 0.9659258262890683122, 1.000000000000000000, 0.9659258262890683122, 1.000000000000000000, 0.9659258262890683122, 1.000000000000000000, 0.9659258262890683122, 1.000000000000000000, 0.9659258262890683122, 1.000000000000000000, 0.9659258262890683122, 1.000000000000000000, 0.9659258262890683122, 1.000000000000000000, 0.9659258262890683122, 1.000000000000000000, 0.9659258262890683122, 1.000000000000000000, 0.9659258262890683122, 1.000000000000000000, 0.9659258262890683122, 1.000000000000000000, 0.9659258262890683122, 1.000000000000000000, 0.9659258262890683122, 1.000000000000000000, 0.9659258262890683122, 1.000000000000000000, 0.9659258262890683122, 1.000000000000000000, 0.9659258262890683122, 1.000000000000000000, 0.9659258262890683122, 1.000000000000000000, 0.9659258262890683122, 1.000000000000000000, 0.9659258262890683122, 1.000000000000000000, 0.9659258262890683122, 1.000000000000000000),
 ( 1.000000000000000000, 0.9659258262890683122, 1.000000000000000000, 0.9659258262890683122, 1.000000000000000000, 0.9659258262890683122, 1.000000000000000000, 0.9659258262890683122, 1.000000000000000000, 0.9659258262890683122, 1.000000000000000000, 0.9659258262890683122, 1.000000000000000000, 0.9659258262890683122, 1.000000000000000000, 0.9659258262890683122, 1.000000000000000000, 0.9659258262890683122, 1.000000000000000000, 0.9659258262890683122, 1.000000000000000000, 0.9659258262890683122, 1.000000000000000000, 0.9659258262890683122, 1.000000000000000000, 0.9659258262890683122, 1.000000000000000000, 0.9659258262890683122, 1.000000000000000000, 0.9659258262890683122, 1.000000000000000000, 0.9659258262890683122, 1.000000000000000000, 0.9659258262890683122, 1.000000000000000000, 0.9659258262890683122, 1.000000000000000000, 0.9659258262890683122, 1.000000000000000000, 0.9659258262890683122, 1.000000000000000000, 0.9659258262890683122, 1.000000000000000000, 0.9659258262890683122, 1.000000000000000000, 0.9659258262890683122, 1.000000000000000000, 0.9659258262890683122, 1.000000000000000000, 0.9659258262890683122, 1.000000000000000000, 0.9659258262890683122, 1.000000000000000000, 0.9659258262890683122, 1.000000000000000000, 0.9659258262890683122, 1.000000000000000000, 0.9659258262890683122, 1.000000000000000000, 0.9659258262890683122, 1.000000000000000000, 0.9659258262890683122, 1.000000000000000000, 0.9659258262890683122, 1.000000000000000000, 0.9659258262890683122, 1.000000000000000000, 0.9659258262890683122, 1.000000000000000000, 0.9659258262890683122, 1.000000000000000000, 0.9659258262890683122, 1.000000000000000000, 0.9659258262890683122, 1.000000000000000000, 0.9659258262890683122, 1.000000000000000000, 0.9659258262890683122, 1.000000000000000000, 0.9659258262890683122, 1.000000000000000000, 0.9659258262890683122, 1.000000000000000000, 0.9659258262890683122, 1.000000000000000000, 0.9659258262890683122, 1.000000000000000000, 0.9659258262890683122, 1.000000000000000000, 0.9659258262890683122, 1.000000000000000000, 0.9659258262890683122, 1.000000000000000000, 0.9659258262890683122, 1.000000000000000000, 0.9659258262890683122, 1.000000000000000000, 0.9659258262890683122, 1.000000000000000000, 0.9659258262890683122, 1.000000000000000000, 0.9659258262890683122, 1.000000000000000000, 0.9659258262890683122, 1.000000000000000000, 0.9659258262890683122, 1.000000000000000000, 0.9659258262890683122, 1.000000000000000000, 0.9659258262890683122, 1.000000000000000000, 0.9659258262890683122, 1.000000000000000000, 0.9659258262890683122, 1.000000000000000000, 0.9659258262890683122, 1.000000000000000000, 0.9659258262890683122, 1.000000000000000000, 0.9659258262890683122, 1.000000000000000000, 0.9659258262890683122, 1.000000000000000000, 0.9659258262890683122, 1.000000000000000000, 0.9659258262890683122, 1.000000000000000000, 0.9659258262890683122, 1.000000000000000000, 0.9659258262890683122, 1.000000000000000000, 0.9659258262890683122, 1.000000000000000000, 0.9659258262890683122, 1.000000000000000000, 0.9659258262890683122, 1.000000000000000000, 0.9659258262890683122, 1.000000000000000000, 0.9659258262890683122, 1.000000000000000000, 0.9659258262890683122, 1.000000000000000000, 0.9659258262890683122, 1.000000000000000000, 0.9659258262890683122, 1.000000000000000000, 0.9659258262890683122, 1.000000000000000000, 0.9659258262890683122, 1.000000000000000000, 0.9659258262890683122, 1.000000000000000000, 0.9659258262890683122, 1.000000000000000000, 0.9659258262890683122, 1.000000000000000000, 0.9659258262890683122, 1.000000000000000000, 0.9659258262890683122, 1.000000000000000000, 0.9659258262890683122, 1.000000000000000000, 0.9659258262890683122, 1.000000000000000000, 0.9659258262890683122, 1.000000000000000000, 0.9659258262890683122, 1.000000000000000000, 0.9659258262890683122, 1.000000000000000000, 0.9659258262890683122, 1.000000000000000000, 0.9659258262890683122, 1.000000000000000000, 0.9659258262890683122, 1.000000000000000000, 0.9659258262890683122, 1.000000000000000000, 0.9659258262890683122, 1.000000000000000000, 0.9659258262890683122, 1.000000000000000000, 0.9659258262890683122, 1.000000000000000000, 0.9659258262890683122, 1.000000000000000000, 0.9659258262890683122, 1.000000000000000000, 0.9659258262890683122, 1.000000000000000000, 0.9659258262890683122, 1.000000000000000000, 0.9659258262890683122, 1.000000000000000000, 0.9659258262890683122, 1.000000000000000000, 0.9659258262890683122, 1.000000000000000000, 0.9659258262890683122, 1.000000000000000000, 0.9659258262890683122, 1.000000000000000000, 0.9659258262890683122, 1.000000000000000000, 0.9659258262890683122, 1.000000000000000000, 0.9659258262890683122, 1.000000000000000000, 0.9659258262890683122, 1.000000000000000000, 0.9659258262890683122, 1.000000000000000000, 0.9659258262890683122, 1.000000000000000000, 0.9659258262890683122, 1.000000000000000000, 0.9659258262890683122, 1.000000000000000000, 0.9659258262890683122, 1.000000000000000000, 0.9659258262890683122, 1.000000000000000000, 0.9659258262890683122, 1.000000000000000000, 0.9659258262890683122, 1.000000000000000000, 0.9659258262890683122, 1.000000000000000000, 0.9659258262890683122, 1.000000000000000000, 0.9659258262890683122, 1.000000000000000000, 0.9659258262890683122, 1.000000000000000000, 0.9659258262890683122, 1.000000000000000000, 0.9659258262890683122, 1.000000000000000000, 0.9659258262890683122, 1.000000000000000000, 0.9659258262890683122, 1.000000000000000000, 0.9659258262890683122, 1.000000000000000000, 0.9659258262890683122, 1.000000000000000000, 0.9659258262890683122, 1.000000000000000000, 0.9659258262890683122, 1.000000000000000000, 0.9659258262890683122, 1.000000000000000000, 0.9659258262890683122, 1.000000000000000000, 0.9659258262890683122, 1.000000000000000000, 0.9659258262890683122, 1.000000000000000000, 0.9659258262890683122, 1.000000000000000000, 0.9659258262890683122, 1.000000000000000000, 0.9659258262890683122, 1.000000000000000000, 0.9659258262890683122, 1.000000000000000000, 0.9659258262890683122, 1.000000000000000000, 0.9659258262890683122, 1.000000000000000000, 0.9659258262890683122, 1.000000000000000000, 0.9659258262890683122, 1.000000000000000000, 0.9659258262890683122, 1.000000000000000000, 0.9659258262890683122, 1.000000000000000000, 0.9659258262890683122, 1.000000000000000000, 0.9659258262890683122, 1.000000000000000000, 0.9659258262890683122, 1.000000000000000000, 0.9659258262890683122, 1.000000000000000000, 0.9659258262890683122, 1.000000000000000000, 0.9659258262890683122, 1.000000000000000000, 0.9659258262890683122, 1.000000000000000000, 0.9659258262890683122, 1.000000000000000000, 0.9659258262890683122, 1.000000000000000000, 0.9659258262890683122, 1.000000000000000000, 0.9659258262890683122, 1.000000000000000000, 0.9659258262890683122, 1.000000000000000000, 0.9659258262890683122, 1.000000000000000000, 0.9659258262890683122, 1.000000000000000000, 0.9659258262890683122, 1.000000000000000000, 0.9659258262890683122, 1.000000000000000000, 0.9659258262890683122, 1.000000000000000000, 0.9659258262890683122, 1.000000000000000000, 0.9659258262890683122, 1.000000000000000000, 0.9659258262890683122, 1.000000000000000000, 0.9659258262890683122, 1.000000000000000000, 0.9659258262890683122, 1.000000000000000000, 0.9659258262890683122, 1.000000000000000000, 0.9659258262890683122, 1.000000000000000000, 0.9659258262890683122, 1.000000000000000000, 0.9659258262890683122, 1.000000000000000000, 0.9659258262890683122, 1.000000000000000000, 0.9659258262890683122, 1.000000000000000000, 0.9659258262890683122, 1.000000000000000000, 0.9659258262890683122, 1.000000000000000000, 0.9659258262890683122, 1.000000000000000000, 0.9659258262890683122, 1.000000000000000000, 0.9659258262890683122, 1.000000000000000000, 0.9659258262890683122, 1.000000000000000000, 0.9659258262890683122, 1.000000000000000000, 0.9659258262890683122, 1.000000000000000000, 0.9659258262890683122, 1.000000000000000000, 0.9659258262890683122, 1.000000000000000000, 0.9659258262890683122, 1.000000000000000000, 0.9659258262890683122, 1.000000000000000000, 0.9659258262890683122, 1.000000000000000000, 0.9659258262890683122, 1.000000000000000000, 0.9659258262890683122, 1.000000000000000000, 0.9659258262890683122, 1.000000000000000000, 0.9659258262890683122, 1.000000000000000000, 0.9659258262890683122, 1.000000000000000000, 0.9659258262890683122, 1.000000000000000000, 0.9659258262890683122, 1.000000000000000000, 0.9659258262890683122, 1.000000000000000000, 0.9659258262890683122, 1.000000000000000000, 0.9659258262890683122, 1.000000000000000000, 0.9659258262890683122, 1.000000000000000000, 0.9659258262890683122, 1.000000000000000000, 0.9659258262890683122, 1.000000000000000000, 0.9659258262890683122, 1.000000000000000000, 0.9659258262890683122, 1.000000000000000000, 0.9659258262890683122, 1.000000000000000000, 0.9659258262890683122, 1.000000000000000000, 0.9659258262890683122, 1.000000000000000000, 0.9659258262890683122, 1.000000000000000000, 0.9659258262890683122, 1.000000000000000000, 0.9659258262890683122, 1.000000000000000000, 0.9659258262890683122, 1.000000000000000000, 0.9659258262890683122, 1.000000000000000000, 0.9659258262890683122, 1.000000000000000000, 0.9659258262890683122, 1.000000000000000000, 0.9659258262890683122, 1.000000000000000000, 0.9659258262890683122, 1.000000000000000000, 0.9659258262890683122, 1.000000000000000000, 0.9659258262890683122, 1.000000000000000000, 0.9659258262890683122, 1.000000000000000000, 0.9659258262890683122, 1.000000000000000000, 0.9659258262890683122, 1.000000000000000000, 0.9659258262890683122, 1.000000000000000000, 0.9659258262890683122, 1.000000000000000000, 0.9659258262890683122, 1.000000000000000000, 0.9659258262890683122, 1.000000000000000000, 0.9659258262890683122, 1.000000000000000000, 0.9659258262890683122, 1.000000000000000000, 0.9659258262890683122, 1.000000000000000000, 0.9659258262890683122, 1.000000000000000000, 0.9659258262890683122, 1.000000000000000000, 0.9659258262890683122, 1.000000000000000000, 0.9659258262890683122, 1.000000000000000000, 0.9659258262890683122, 1.000000000000000000, 0.9659258262890683122, 1.000000000000000000, 0.9659258262890683122, 1.000000000000000000, 0.9659258262890683122, 1.000000000000000000, 0.9659258262890683122, 1.000000000000000000, 0.9659258262890683122, 1.000000000000000000, 0.9659258262890683122, 1.000000000000000000, 0.9659258262890683122, 1.000000000000000000, 0.9659258262890683122, 1.000000000000000000, 0.9659258262890683122, 1.000000000000000000, 0.9659258262890683122, 1.000000000000000000, 0.9659258262890683122, 1.000000000000000000, 0.9659258262890683122, 1.000000000000000000, 0.9659258262890683122, 1.000000000000000000, 0.9659258262890683122, 1.000000000000000000, 0.9659258262890683122, 1.000000000000000000, 0.9659258262890683122, 1.000000000000000000, 0.9659258262890683122, 1.000000000000000000, 0.9659258262890683122, 1.000000000000000000, 0.9659258262890683122, 1.000000000000000000, 0.9659258262890683122, 1.000000000000000000, 0.9659258262890683122, 1.000000000000000000, 0.9659258262890683122, 1.000000000000000000, 0.9659258262890683122, 1.000000000000000000, 0.9659258262890683122, 1.000000000000000000, 0.9659258262890683122, 1.000000000000000000, 0.9659258262890683122, 1.000000000000000000, 0.9659258262890683122, 1.000000000000000000, 0.9659258262890683122, 1.000000000000000000, 0.9659258262890683122, 1.000000000000000000, 0.9659258262890683122, 1.000000000000000000, 0.9659258262890683122, 1.000000000000000000) ) ) 
 REPRESENTATION_ITEM ( '' )  SURFACE ( )  );
#31569=CARTESIAN_POINT ( 'NONE',  ( 0.2362204724409456558, -0.1870078740157480879, -0.4822834645669291653 ) ) ;
#31571=CARTESIAN_POINT ( 'NONE',  ( -0.9908136482939626788, -0.6692913385826773087, -0.1292274648535924053 ) ) ;
#31572=CARTESIAN_POINT ( 'NONE',  ( 1.023622047244095334, -0.1870078740157479769, 0.4822834645669291653 ) ) ;
#31573=CARTESIAN_POINT ( 'NONE',  ( 0.8923884514435701520, -0.5023911411419708095, -0.1820866141732282451 ) ) ;
#31574=DIRECTION ( 'NONE',  ( 0.000000000000000000, 0.000000000000000000, -1.000000000000000000 ) ) ;
#31575=CARTESIAN_POINT ( 'NONE',  ( -0.1771653543307080136, -0.5400638737290844871, 0.3530559997133364547 ) ) ;
#31576=CARTESIAN_POINT ( 'NONE',  ( 0.06561679790026316017, -0.3690944881889763329, 0.3153832671262228327 ) ) ;
#31578=CARTESIAN_POINT ( 'NONE',  ( -0.2887139107611542133, 0.2306618581243848609, 0.2411417322834645549 ) ) ;
#31579=CARTESIAN_POINT ( 'NONE',  ( 0.4133858267716541968, -0.4536011799217368745, -0.2665933059059886201 ) ) ;
#31580=EDGE_CURVE ( 'NONE', #68837, #77522, #9969, .T. ) ;
#31582=CARTESIAN_POINT ( 'NONE',  ( -0.09842519685039295696, -0.5400638737290844871, 0.3530559997133364547 ) ) ;
#31583=CARTESIAN_POINT ( 'NONE',  ( 0.9842519685039378130, -0.5511811023622047445, 6.969142054262312111E-17 ) ) ;
#31585=CARTESIAN_POINT ( 'NONE',  ( -0.4396325459317579898, 0.1771653543307087630, 0.09757992244046791164 ) ) ;
#31586=AXIS2_PLACEMENT_3D ( 'NONE', #79734, #68341, #4347 ) ;
#31587=CARTESIAN_POINT ( 'NONE',  ( -0.7874015748031489847, -0.1870078740157479769, 0.3641732283464567677 ) ) ;
#31588=CARTESIAN_POINT ( 'NONE',  ( -0.2362204724409440182, -0.1870078740157479769, 0.4822834645669291653 ) ) ;
#31589=CARTESIAN_POINT ( 'NONE',  ( -0.1509186351706028884, -0.05778040916215522460, 0.4822834645669289988 ) ) ;
#31590=CARTESIAN_POINT ( 'NONE',  ( 1.062992125984252745, 0.1771653543307087630, 0.000000000000000000 ) ) ;
#31591=CARTESIAN_POINT ( 'NONE',  ( -1.581364829396324945, -0.2845877964562159024, 0.3641732283464567677 ) ) ;
#31592=CARTESIAN_POINT ( 'NONE',  ( 1.555118110236221041, -0.4536011799217367080, 0.2665933059059888421 ) ) ;
#31593=CARTESIAN_POINT ( 'NONE',  ( 0.6036745406824154392, 0.2306618581243847221, -0.2411417322834647770 ) ) ;
#31595=CARTESIAN_POINT ( 'NONE',  ( -0.4461942257217840213, 0.2306618581243848609, 0.2411417322834645549 ) ) ;
#31597=CARTESIAN_POINT ( 'NONE',  ( 0.8923884514435703741, 0.2306618581243848609, 0.2411417322834645549 ) ) ;
#31598=CARTESIAN_POINT ( 'NONE',  ( 0.7283464566929143125, 0.1660481256975885056, 0.3530559997133364547 ) ) ;
#31599=DIRECTION ( 'NONE',  ( -0.000000000000000000, 1.000000000000000000, -0.000000000000000000 ) ) ;
#31600=CARTESIAN_POINT ( 'NONE',  ( 0.5183727034120741983, -0.5511811023622046335, 0.09757992244046803654 ) ) ;
#31601=CARTESIAN_POINT ( 'NONE',  ( 1.338582677165355062, -0.1870078740157479769, 0.4822834645669291653 ) ) ;
#31602=CARTESIAN_POINT ( 'NONE',  ( -0.1837270341207343505, -0.5023911411419708095, 0.1820866141732285504 ) ) ;
#31603=CARTESIAN_POINT ( 'NONE',  ( -0.4265091863517051496, -0.6692913385826771977, 0.1292274648535927661 ) ) ;
#31605=CARTESIAN_POINT ( 'NONE',  ( 0.3083989501312343062, -0.3162353388693405765, 0.4822834645669290543 ) ) ;
#31606=CARTESIAN_POINT ( 'NONE',  ( -0.9711286089238838626, 0.2306618581243847221, -0.2411417322834647770 ) ) ;
#31607=CARTESIAN_POINT ( 'NONE',  ( -0.8661417322834640276, -0.1870078740157480601, -0.3641732283464567677 ) ) ;
#31608=CARTESIAN_POINT ( 'NONE',  ( 0.4724409448818904789, -0.1870078740157479769, 0.4822834645669291653 ) ) ;
#31609=CARTESIAN_POINT ( 'NONE',  ( -1.410761154855642463, -0.05778040916215522460, 0.4822834645669289988 ) ) ;
#31610=CARTESIAN_POINT ( 'NONE',  ( -0.1771653543307080136, 0.1660481256975883668, -0.3530559997133364547 ) ) ;
#31613=CARTESIAN_POINT ( 'NONE',  ( 1.391076115485564868, -0.6046776061558807314, 0.2411417322834647770 ) ) ;
#31614=CARTESIAN_POINT ( 'NONE',  ( 1.279527559055118724, -0.5400638737290845981, -0.3530559997133363437 ) ) ;
#31616=CARTESIAN_POINT ( 'NONE',  ( -1.607611548556429737, 0.2952755905511810774, -0.1292274648535930714 ) ) ;
#31617=CARTESIAN_POINT ( 'NONE',  ( -1.069553805774277722, 0.2952755905511811885, 0.1292274648535926551 ) ) ;
#31621=CARTESIAN_POINT ( 'NONE',  ( -0.2690288713910754526, -0.5511811023622046335, 0.09757992244046803654 ) ) ;
#31623=CARTESIAN_POINT ( 'NONE',  ( 0.6364829396325465405, -0.05778040916215522460, 0.4822834645669289988 ) ) ;
#31626=CARTESIAN_POINT ( 'NONE',  ( -1.614173228346457378, 0.5038684218300931716, 0.1372047244094476981 ) ) ;
#31627=CARTESIAN_POINT ( 'NONE',  ( -0.3674540682414689785, 0.1283753931104748280, 0.1820866141732283561 ) ) ;
#31629=CARTESIAN_POINT ( 'NONE',  ( 1.345144356955381593, -0.05778040916215522460, 0.4822834645669289988 ) ) ;
#31630=CARTESIAN_POINT ( 'NONE',  ( 1.122047244094488860, 0.07958543189024085140, 0.2665933059059887866 ) ) ;
#31631=CARTESIAN_POINT ( 'NONE',  ( -0.006561679790025524116, -0.05778040916215560624, -0.4822834645669293319 ) ) ;
#31633=CARTESIAN_POINT ( 'NONE',  ( -0.3937007874015740483, -0.1870078740157479769, 0.4822834645669291653 ) ) ;
#31634=CARTESIAN_POINT ( 'NONE',  ( -1.463254593175852492, -0.5511811023622048555, -0.09757992244046775898 ) ) ;
#31635=CARTESIAN_POINT ( 'NONE',  ( -0.5183727034120726440, -0.6692913385826773087, -0.1292274648535924053 ) ) ;
#31636=CARTESIAN_POINT ( 'NONE',  ( 1.574803149606299746, -0.1870078740157480879, -0.4822834645669291653 ) ) ;
#31637=CARTESIAN_POINT ( 'NONE',  ( 0.6402603868039153934, -2.736035270306112984E-15, 0.4281989832122460871 ) ) ;
#31640=CARTESIAN_POINT ( 'NONE',  ( 0.2690288713910767848, 0.2952755905511811885, 0.1292274648535926551 ) ) ;
#31643=CARTESIAN_POINT ( 'NONE',  ( -0.7349081364829390672, 0.2306618581243847221, -0.2411417322834647770 ) ) ;
#31644=CARTESIAN_POINT ( 'NONE',  ( -1.496062992125983815, -0.1870078740157479769, 0.4822834645669291653 ) ) ;
#31646=CARTESIAN_POINT ( 'NONE',  ( 0.4986876640419954376, 0.2306618581243848609, 0.2411417322834645549 ) ) ;
#31647=CARTESIAN_POINT ( 'NONE',  ( -0.1377952755905504645, -0.5400638737290845981, -0.3530559997133363437 ) ) ;
#31649=CARTESIAN_POINT ( 'NONE',  ( -0.6824146981627291497, -0.6046776061558809534, -0.2411417322834644161 ) ) ;
#31650=CARTESIAN_POINT ( 'NONE',  ( -0.2099737532808391705, 0.2306618581243848609, 0.2411417322834645549 ) ) ;
#31651=CARTESIAN_POINT ( 'NONE',  ( -1.056430446194224881, -0.6692913385826771977, 0.1292274648535927661 ) ) ;
#31652=EDGE_CURVE ( 'NONE', #44157, #40053, #33435, .T. ) ;
#31653=CARTESIAN_POINT ( 'NONE',  ( -0.1312335958005241554, -0.5023911411419708095, -0.1820866141732282451 ) ) ;
#31655=CARTESIAN_POINT ( 'NONE',  ( -0.1640419947506555343, -0.3162353388693405765, 0.4822834645669290543 ) ) ;
#31656=FACE_OUTER_BOUND ( 'NONE', #73292, .T. ) ;
#31657=CARTESIAN_POINT ( 'NONE',  ( 1.227034120734908917, -0.6692913385826771977, 0.1292274648535927661 ) ) ;
#31660=EDGE_LOOP ( 'NONE', ( #62060, #3902, #32613, #65002 ) ) ;
#31661=CARTESIAN_POINT ( 'NONE',  ( 0.1574803149606306130, -0.1870078740157480879, -0.4822834645669291653 ) ) ;
#31662=CARTESIAN_POINT ( 'NONE',  ( -0.06561679790026180015, -0.3690944881889765550, -0.3153832671262227771 ) ) ;
#31663=CARTESIAN_POINT ( 'NONE',  ( 1.423884514435696413, -0.2845877964562161244, -0.3641732283464567121 ) ) ;
#31667=CARTESIAN_POINT ( 'NONE',  ( 1.482939632545932307, -0.3690944881889763329, 0.3153832671262228327 ) ) ;
#31668=CARTESIAN_POINT ( 'NONE',  ( -1.522309711286088607, -0.6046776061558807314, 0.2411417322834647770 ) ) ;
#31670=CARTESIAN_POINT ( 'NONE',  ( 0.6496062992125991586, 0.1660481256975885056, 0.3530559997133364547 ) ) ;
#31671=CARTESIAN_POINT ( 'NONE',  ( -1.148293963254592542, 0.2952755905511811885, 0.1292274648535926551 ) ) ;
#31672=CARTESIAN_POINT ( 'NONE',  ( -0.9580052493438311334, -0.4281496062992124485, 0.4176697321401328655 ) ) ;
#31673=CARTESIAN_POINT ( 'NONE',  ( 0.08530183727034192087, -0.3162353388693409650, -0.4822834645669289433 ) ) ;
#31674=CARTESIAN_POINT ( 'NONE',  ( 0.7939632545931766261, -0.05778040916215522460, 0.4822834645669289988 ) ) ;
#31675=CARTESIAN_POINT ( 'NONE',  ( 1.345144356955381593, -0.08942795157527998196, 0.3641732283464567121 ) ) ;
#31677=CARTESIAN_POINT ( 'NONE',  ( 0.8005249343832028242, -0.3690944881889765550, -0.3153832671262227771 ) ) ;
#31678=CARTESIAN_POINT ( 'NONE',  ( -0.9645669291338575535, 0.1660481256975883668, -0.3530559997133364547 ) ) ;
#31679=EDGE_CURVE ( 'NONE', #44891, #68517, #33953, .T. ) ;
#31681=CARTESIAN_POINT ( 'NONE',  ( 1.646981627296588035, -0.3162353388693405765, 0.4822834645669290543 ) ) ;
#31683=VECTOR ( 'NONE', #64613, 39.37007874015748143 ) ;
#31684=CARTESIAN_POINT ( 'NONE',  ( 0.7939632545931766261, -0.3162353388693409650, -0.4822834645669289433 ) ) ;
#31686=CARTESIAN_POINT ( 'NONE',  ( -1.397637795275589623, 0.07958543189024085140, 0.2665933059059887866 ) ) ;
#31687=CARTESIAN_POINT ( 'NONE',  ( -0.006561679790025524116, -0.05778040916215560624, -0.4822834645669293319 ) ) ;
#31688=CARTESIAN_POINT ( 'NONE',  ( 0.8595800524934390507, -0.08942795157528024563, -0.3641732283464568787 ) ) ;
#31689=EDGE_CURVE ( 'NONE', #31856, #66355, #4419, .T. ) ;
#31690=CARTESIAN_POINT ( 'NONE',  ( 1.030183727034121421, -0.05778040916215522460, 0.4822834645669289988 ) ) ;
#31691=CARTESIAN_POINT ( 'NONE',  ( -0.3543307086614165824, -0.5511811023622047445, 6.969142054262312111E-17 ) ) ;
#31692=CARTESIAN_POINT ( 'NONE',  ( -0.4790026246719154557, -0.3162353388693405765, 0.4822834645669290543 ) ) ;
#31693=CARTESIAN_POINT ( 'NONE',  ( -1.587926509186350810, -0.004921259842519870586, -0.3153832671262229437 ) ) ;
#31694=CARTESIAN_POINT ( 'NONE',  ( -1.299212598425196097, -0.6692913385826771977, 8.415575281601705876E-17 ) ) ;
#31695=CARTESIAN_POINT ( 'NONE',  ( 0.9448818897637802916, -0.1870078740157480879, -0.4822834645669291653 ) ) ;
#31697=CARTESIAN_POINT ( 'NONE',  ( -1.437007874015747477, 0.07958543189024071263, -0.2665933059059888421 ) ) ;
#31698=( BOUNDED_CURVE ( )  B_SPLINE_CURVE ( 2, ( #59472, #1825, #66217, #53143, #45998, #78440, #47250, #78856, #21181, #72530, #53564, #71694, #8968 ),
 .UNSPECIFIED., .F., .F. ) 
 B_SPLINE_CURVE_WITH_KNOTS ( ( 3, 2, 2, 2, 2, 2, 3 ),
 ( 0.5376696296615053328, 0.5378787878787878451, 0.5416666666666666297, 0.5454545454545454142, 0.5492424242424241987, 0.5530303030303029832, 0.5532394612475854956 ),
 .UNSPECIFIED. ) 
 CURVE ( )  GEOMETRIC_REPRESENTATION_ITEM ( )  RATIONAL_B_SPLINE_CURVE ( ( 0.9964447847208419695, 0.9981185001348091834, 1.000000000000000000, 0.9659258262890683122, 1.000000000000000000, 0.9659258262890683122, 1.000000000000000000, 0.9659258262890683122, 1.000000000000000000, 0.9659258262890683122, 1.000000000000000000, 0.9981185001348091834, 0.9964447847208420805 ) ) 
 REPRESENTATION_ITEM ( '' )  );
#31700=CARTESIAN_POINT ( 'NONE',  ( 0.8923884514435701520, -0.6046776061558809534, -0.2411417322834644161 ) ) ;
#31703=CARTESIAN_POINT ( 'NONE',  ( -1.581364829396324945, -0.3162353388693405765, 0.4822834645669290543 ) ) ;
#31704=CARTESIAN_POINT ( 'NONE',  ( 1.640419947506562393, -0.4281496062992124485, 0.4176697321401328655 ) ) ;
#31705=CARTESIAN_POINT ( 'NONE',  ( -1.122047244094487306, -0.4536011799217367080, 0.2665933059059888421 ) ) ;
#31706=CARTESIAN_POINT ( 'NONE',  ( 1.607611548556431069, -0.5511811023622048555, -0.09757992244046775898 ) ) ;
#31707=CARTESIAN_POINT ( 'NONE',  ( -0.4199475065616791736, -0.6046776061558807314, 0.2411417322834647770 ) ) ;
#31708=CARTESIAN_POINT ( 'NONE',  ( -0.6102362204724400829, -0.4536011799217368745, -0.2665933059059886201 ) ) ;
#31709=CARTESIAN_POINT ( 'NONE',  ( -1.725721784776902190, -0.08942795157527998196, 0.3641732283464567121 ) ) ;
#31710=CARTESIAN_POINT ( 'NONE',  ( 0.8333333333333340365, 0.1771653543307087075, -0.09757992244046823083 ) ) ;
#31711=CARTESIAN_POINT ( 'NONE',  ( 1.069553805774278832, 0.2952755905511810774, -0.1292274648535930714 ) ) ;
#31712=CYLINDRICAL_SURFACE ( 'NONE', #52840, 0.3937007874015748254 ) ;
#31713=CARTESIAN_POINT ( 'NONE',  ( -0.08530183727034056085, -0.2845877964562159024, 0.3641732283464567677 ) ) ;
#31715=CARTESIAN_POINT ( 'NONE',  ( 0.3608923884514443348, -0.6692913385826771977, 0.1292274648535927661 ) ) ;
#31716=CARTESIAN_POINT ( 'NONE',  ( 0.6299212598425204535, -0.1870078740157479769, 0.3641732283464567677 ) ) ;
#31717=CARTESIAN_POINT ( 'NONE',  ( 1.574803149606299746, -0.1870078740157479769, 0.4822834645669291653 ) ) ;
#31718=CARTESIAN_POINT ( 'NONE',  ( -1.128608923884513837, 0.2306618581243847221, -0.2411417322834647770 ) ) ;
#31719=CARTESIAN_POINT ( 'NONE',  ( -0.4658792650918627265, -0.05778040916215522460, 0.4822834645669289988 ) ) ;
#31722=CARTESIAN_POINT ( 'NONE',  ( 0.3871391076115492380, -0.05778040916215560624, -0.4822834645669293319 ) ) ;
#31723=CARTESIAN_POINT ( 'NONE',  ( 0.9776902887139113929, 0.1771653543307087630, 0.09757992244046791164 ) ) ;
#31724=CARTESIAN_POINT ( 'NONE',  ( -0.4986876640419939388, 0.2306618581243847221, -0.2411417322834647770 ) ) ;
#31725=CARTESIAN_POINT ( 'NONE',  ( 0.3149606299212603933, -0.1870078740157479769, 0.4822834645669291653 ) ) ;
#31731=CARTESIAN_POINT ( 'NONE',  ( -0.3674540682414692561, -0.5023911411419708095, -0.1820866141732282451 ) ) ;
#31732=CARTESIAN_POINT ( 'NONE',  ( -1.233595800524933894, 0.2306618581243848609, 0.2411417322834645549 ) ) ;
#31734=CARTESIAN_POINT ( 'NONE',  ( 0.8727034120734913358, -0.05778040916215522460, 0.4822834645669289988 ) ) ;
#31735=CARTESIAN_POINT ( 'NONE',  ( 1.456692913385827515, 0.2952755905511811885, 0.000000000000000000 ) ) ;
#31736=CARTESIAN_POINT ( 'NONE',  ( 0.6627296587926515548, 0.2952755905511811885, 0.1292274648535926551 ) ) ;
#31738=AXIS2_PLACEMENT_3D ( 'NONE', #50721, #32201, #70498 ) ;
#31741=AXIS2_PLACEMENT_3D ( 'NONE', #7070, #13394, #33579 ) ;
#31742=CARTESIAN_POINT ( 'NONE',  ( 0.6496062992125991586, 0.1660481256975885056, 0.3530559997133364547 ) ) ;
#31743=EDGE_CURVE ( 'NONE', #2914, #79410, #78086, .T. ) ;
#31744=CARTESIAN_POINT ( 'NONE',  ( 0.7086614173228352742, -0.1870078740157480879, -0.4822834645669291653 ) ) ;
#31745=CARTESIAN_POINT ( 'NONE',  ( 0.6889763779527563470, 0.07958543189024071263, -0.2665933059059888421 ) ) ;
#31746=CARTESIAN_POINT ( 'NONE',  ( 1.292650918635171564, -0.6692913385826773087, -0.1292274648535924053 ) ) ;
#31748=CARTESIAN_POINT ( 'NONE',  ( 0.5839895013123367340, -0.6692913385826773087, -0.1292274648535924053 ) ) ;
#31749=CARTESIAN_POINT ( 'NONE',  ( 1.115485564304462551, -0.4281496062992127816, -0.4176697321401328100 ) ) ;
#31750=CARTESIAN_POINT ( 'NONE',  ( 0.2362204724409456558, -0.1870078740157479769, 0.4822834645669291653 ) ) ;
#31751=CARTESIAN_POINT ( 'NONE',  ( 1.377952755905512472, 0.1771653543307087630, 0.000000000000000000 ) ) ;
#31752=CARTESIAN_POINT ( 'NONE',  ( -0.7611548556430438595, 0.2306618581243848609, 0.2411417322834645549 ) ) ;
#31753=CARTESIAN_POINT ( 'NONE',  ( -0.8398950131233589023, -0.6046776061558809534, -0.2411417322834644161 ) ) ;
#31754=CARTESIAN_POINT ( 'NONE',  ( 1.279527559055118724, 0.1660481256975885056, 0.3530559997133364547 ) ) ;
#31760=ORIENTED_EDGE ( 'NONE', *, *, #5222, .T. ) ;
#31761=CARTESIAN_POINT ( 'NONE',  ( 1.646981627296588035, -0.3162353388693405765, 0.4822834645669290543 ) ) ;
#31763=CARTESIAN_POINT ( 'NONE',  ( 1.312335958005249825, 0.1283753931104746893, -0.1820866141732285504 ) ) ;
#31765=CARTESIAN_POINT ( 'NONE',  ( 1.312335958005250269, -0.5023911411419708095, 0.1820866141732285504 ) ) ;
#31766=CARTESIAN_POINT ( 'NONE',  ( -0.1674892343164145203, -2.567464376874931580E-15, -0.4445507791589072832 ) ) ;
#31768=CARTESIAN_POINT ( 'NONE',  ( 0.4581547954228972763, 1.765968763542725251, 0.5309055118110234117 ) ) ;
#31770=CARTESIAN_POINT ( 'NONE',  ( -0.6233595800524928121, -0.2845877964562161244, -0.3641732283464567121 ) ) ;
#31771=CARTESIAN_POINT ( 'NONE',  ( -1.692913385826770645, 0.1771653543307087630, 0.000000000000000000 ) ) ;
#31772=CARTESIAN_POINT ( 'NONE',  ( -1.384514435695537005, -0.6692913385826773087, -0.1292274648535924053 ) ) ;
#31773=CARTESIAN_POINT ( 'NONE',  ( 0.006561679790026889343, -0.05778040916215522460, 0.4822834645669289988 ) ) ;
#31774=CARTESIAN_POINT ( 'NONE',  ( 1.568241469816273437, -0.3162353388693405765, 0.4822834645669290543 ) ) ;
#31775=ORIENTED_EDGE ( 'NONE', *, *, #42014, .F. ) ;
#31779=CARTESIAN_POINT ( 'NONE',  ( -0.6364829396325453192, -0.08942795157528024563, -0.3641732283464568787 ) ) ;
#31780=CARTESIAN_POINT ( 'NONE',  ( -1.010498687664041384, 0.05413385826771666132, 0.4176697321401328100 ) ) ;
#31781=CARTESIAN_POINT ( 'NONE',  ( 0.9842519685039378130, -0.6692913385826771977, 8.415575281601705876E-17 ) ) ;
#31785=CARTESIAN_POINT ( 'NONE',  ( 1.253280839895013710, -0.05778040916215560624, -0.4822834645669293319 ) ) ;
#31786=CARTESIAN_POINT ( 'NONE',  ( -1.397637795275589623, 0.1660481256975885056, 0.3530559997133364547 ) ) ;
#31788=CARTESIAN_POINT ( 'NONE',  ( -0.5183727034120726440, -0.5511811023622048555, -0.09757992244046775898 ) ) ;
#31790=CARTESIAN_POINT ( 'NONE',  ( -0.3149606299212590610, -0.1870078740157480601, -0.3641732283464567677 ) ) ;
#31791=CARTESIAN_POINT ( 'NONE',  ( -0.1049868766404193215, 0.1283753931104746893, -0.1820866141732285504 ) ) ;
#31792=CARTESIAN_POINT ( 'NONE',  ( 0.1443569553805781891, -0.4281496062992124485, 0.4176697321401328655 ) ) ;
#31793=CARTESIAN_POINT ( 'NONE',  ( -0.8398950131233585692, 0.1283753931104748280, 0.1820866141732283561 ) ) ;
#31795=CARTESIAN_POINT ( 'NONE',  ( 1.338582677165355062, -0.1870078740157480879, -0.4822834645669291653 ) ) ;
#31796=CIRCLE ( 'NONE', #49291, 0.4822834645669291653 ) ;
#31797=CARTESIAN_POINT ( 'NONE',  ( -1.509186351706035767, -0.4281496062992124485, 0.4176697321401328655 ) ) ;
#31801=CARTESIAN_POINT ( 'NONE',  ( -0.2887139107611542133, 0.2306618581243848609, 0.2411417322834645549 ) ) ;
#31802=CARTESIAN_POINT ( 'NONE',  ( -1.141732283464566011, 0.2952755905511811885, 0.000000000000000000 ) ) ;
#31803=CARTESIAN_POINT ( 'NONE',  ( 1.095800524934383846, -0.08942795157528024563, -0.3641732283464568787 ) ) ;
#31804=CARTESIAN_POINT ( 'NONE',  ( -0.3149606299212590610, -0.1870078740157479769, 0.3641732283464567677 ) ) ;
#31805=CARTESIAN_POINT ( 'NONE',  ( -0.7480314960629914633, 0.2952755905511811885, 0.000000000000000000 ) ) ;
#31806=CARTESIAN_POINT ( 'NONE',  ( -1.279527559055116948, 0.1660481256975883668, -0.3530559997133364547 ) ) ;
#31807=CARTESIAN_POINT ( 'NONE',  ( -0.4056338187708053988, 4.650002066398565039E-15, -0.3627989612356129490 ) ) ;
#31808=CARTESIAN_POINT ( 'NONE',  ( 1.338582677165355062, -0.1870078740157479769, 0.3641732283464567677 ) ) ;
#31809=CARTESIAN_POINT ( 'NONE',  ( -0.2952755905511803003, -0.5400638737290845981, -0.3530559997133363437 ) ) ;
#31810=CARTESIAN_POINT ( 'NONE',  ( -1.706036745406823485, 0.2306618581243848609, 0.2411417322834645549 ) ) ;
#31813=CARTESIAN_POINT ( 'NONE',  ( -0.9055118110236215490, -0.5511811023622047445, 6.969142054262312111E-17 ) ) ;
#31814=CARTESIAN_POINT ( 'NONE',  ( 0.7874015748031503170, -0.1870078740157479769, 0.4822834645669291653 ) ) ;
#31815=CARTESIAN_POINT ( 'NONE',  ( -1.082677165354329896, 0.07958543189024085140, 0.2665933059059887866 ) ) ;
#31817=CARTESIAN_POINT ( 'NONE',  ( -1.135170603674539924, -0.6692913385826771977, 0.1292274648535927661 ) ) ;
#31818=CARTESIAN_POINT ( 'NONE',  ( 0.9908136482939640111, -0.6692913385826771977, 0.1292274648535927661 ) ) ;
#31819=CARTESIAN_POINT ( 'NONE',  ( 0.8398950131233602345, -0.6046776061558807314, 0.2411417322834647770 ) ) ;
#31820=CARTESIAN_POINT ( 'NONE',  ( 1.601049868766404982, 0.2306618581243848609, 0.2411417322834645549 ) ) ;
#31821=CARTESIAN_POINT ( 'NONE',  ( -1.338582677165353729, -0.1870078740157480601, -0.3641732283464567677 ) ) ;
#31826=CARTESIAN_POINT ( 'NONE',  ( 1.345144356955381593, -0.08942795157527998196, 0.3641732283464567121 ) ) ;
#31827=CARTESIAN_POINT ( 'NONE',  ( 0.6167979002624678353, -0.3690944881889763329, 0.3153832671262228327 ) ) ;
#31828=CARTESIAN_POINT ( 'NONE',  ( -0.01312335958005186876, -0.4281496062992124485, 0.4176697321401328655 ) ) ;
#31831=CARTESIAN_POINT ( 'NONE',  ( 0.2362204724409456558, -0.1870078740157479769, 0.3641732283464567677 ) ) ;
#31832=ADVANCED_FACE ( 'NONE', ( #28880 ), #134, .F. ) ;
#31833=CARTESIAN_POINT ( 'NONE',  ( -0.8005249343832011588, 0.05413385826771626580, -0.4176697321401330321 ) ) ;
#31834=CARTESIAN_POINT ( 'NONE',  ( -1.095800524934382292, -0.3162353388693409650, -0.4822834645669289433 ) ) ;
#31835=CARTESIAN_POINT ( 'NONE',  ( 0.7414698162729663755, 0.2952755905511811885, 0.1292274648535926551 ) ) ;
#31838=ORIENTED_EDGE ( 'NONE', *, *, #40285, .T. ) ;
#31839=VERTEX_POINT ( 'NONE', #22157 ) ;
#31840=CARTESIAN_POINT ( 'NONE',  ( -1.325459317585300889, -0.4281496062992127816, -0.4176697321401328100 ) ) ;
#31841=CARTESIAN_POINT ( 'NONE',  ( -0.8005249343832011588, 0.05413385826771626580, -0.4176697321401330321 ) ) ;
#31842=CARTESIAN_POINT ( 'NONE',  ( -0.8727034120734901146, -0.2845877964562159024, 0.3641732283464567677 ) ) ;
#31843=CARTESIAN_POINT ( 'NONE',  ( -0.6758530183727028406, 0.2952755905511811885, 0.1292274648535926551 ) ) ;
#31845=CARTESIAN_POINT ( 'NONE',  ( -0.3805774278215216522, 0.05413385826771666132, 0.4176697321401328100 ) ) ;
#31846=CARTESIAN_POINT ( 'NONE',  ( 1.528871391076116026, -0.6692913385826773087, -0.1292274648535924053 ) ) ;
#31847=CARTESIAN_POINT ( 'NONE',  ( -0.7086614173228339419, -0.1870078740157480879, -0.4822834645669291653 ) ) ;
#31848=CARTESIAN_POINT ( 'NONE',  ( 0.4527559055118117182, -0.5400638737290844871, 0.3530559997133364547 ) ) ;
#31849=CARTESIAN_POINT ( 'NONE',  ( -0.8070866141732276899, 0.1660481256975883668, -0.3530559997133364547 ) ) ;
#31852=CARTESIAN_POINT ( 'NONE',  ( -0.7020997375328074108, -0.08942795157527998196, 0.3641732283464567121 ) ) ;
#31856=VERTEX_POINT ( 'NONE', #42327 ) ;
#31860=CARTESIAN_POINT ( 'NONE',  ( -1.240157480314959759, -0.5400638737290845981, -0.3530559997133363437 ) ) ;
#31861=CARTESIAN_POINT ( 'NONE',  ( -0.9186351706036736120, -0.6046776061558809534, -0.2411417322834644161 ) ) ;
#31863=CARTESIAN_POINT ( 'NONE',  ( -1.095800524934382292, -0.05778040916215522460, 0.4822834645669289988 ) ) ;
#31864=CARTESIAN_POINT ( 'NONE',  ( -1.115485564304461219, -0.4281496062992124485, 0.4176697321401328655 ) ) ;
#31865=LINE ( 'NONE', #30209, #5528 ) ;
#31867=CARTESIAN_POINT ( 'NONE',  ( 0.4396325459317593221, 0.1771653543307087075, -0.09757992244046823083 ) ) ;
#31868=CARTESIAN_POINT ( 'NONE',  ( 1.603475055217291612, 0.4410854135902468887, -0.04573490813648244807 ) ) ;
#31870=CARTESIAN_POINT ( 'NONE',  ( -0.1771653543307080136, -0.4536011799217367080, 0.2665933059059888421 ) ) ;
#31871=CARTESIAN_POINT ( 'NONE',  ( -0.7742782152230962556, -0.4281496062992127816, -0.4176697321401328100 ) ) ;
#31872=CARTESIAN_POINT ( 'NONE',  ( 1.371391076115485719, -0.6692913385826773087, -0.1292274648535924053 ) ) ;
#31873=CARTESIAN_POINT ( 'NONE',  ( -0.5118110236220466680, 0.2952755905511811885, 0.000000000000000000 ) ) ;
#31874=EDGE_LOOP ( 'NONE', ( #61744, #56388, #55522, #23401 ) ) ;
#31877=CARTESIAN_POINT ( 'NONE',  ( -0.6364829396325453192, -0.05778040916215560624, -0.4822834645669293319 ) ) ;
#31878=CARTESIAN_POINT ( 'NONE',  ( 1.443569553805774897, 0.2306618581243848609, 0.2411417322834645549 ) ) ;
#31879=CARTESIAN_POINT ( 'NONE',  ( -1.266404199475064773, -0.2845877964562159024, 0.3641732283464567677 ) ) ;
#31880=CARTESIAN_POINT ( 'NONE',  ( -1.325459317585300889, -0.4281496062992127816, -0.4176697321401328100 ) ) ;
#31885=CARTESIAN_POINT ( 'NONE',  ( 0.3018372703412079971, 0.05413385826771626580, -0.4176697321401330321 ) ) ;
#31886=CARTESIAN_POINT ( 'NONE',  ( -1.095800524934382292, -0.2845877964562161244, -0.3641732283464567121 ) ) ;
#31887=CARTESIAN_POINT ( 'NONE',  ( -0.6036745406824141069, 0.2306618581243848609, 0.2411417322834645549 ) ) ;
#31889=CARTESIAN_POINT ( 'NONE',  ( -0.8989501312335946848, 0.2952755905511810774, -0.1292274648535930714 ) ) ;
#31890=CARTESIAN_POINT ( 'NONE',  ( -0.9514435695538050464, -0.3162353388693405765, 0.4822834645669290543 ) ) ;
#31892=CARTESIAN_POINT ( 'NONE',  ( 1.043307086614173818, -0.4536011799217368745, -0.2665933059059886201 ) ) ;
#31893=CARTESIAN_POINT ( 'NONE',  ( -0.6692913385826764205, -0.5511811023622047445, 6.969142054262312111E-17 ) ) ;
#31894=CARTESIAN_POINT ( 'NONE',  ( 0.5971128608923891301, 0.1771653543307087075, -0.09757992244046823083 ) ) ;
#31895=CARTESIAN_POINT ( 'NONE',  ( -1.522309711286088607, 0.2306618581243847221, -0.2411417322834647770 ) ) ;
#31896=CARTESIAN_POINT ( 'NONE',  ( 1.430446194225722500, 0.05413385826771666132, 0.4176697321401328100 ) ) ;
#31897=CARTESIAN_POINT ( 'NONE',  ( 0.4658792650918641698, -0.08942795157528024563, -0.3641732283464568787 ) ) ;
#31899=CARTESIAN_POINT ( 'NONE',  ( -0.8661417322834640276, -0.1870078740157479769, 0.4822834645669291653 ) ) ;
#31900=CARTESIAN_POINT ( 'NONE',  ( 1.128608923884514947, 0.2306618581243848609, 0.2411417322834645549 ) ) ;
#31902=CARTESIAN_POINT ( 'NONE',  ( 0.05905511811023709395, -0.4536011799217367080, 0.2665933059059888421 ) ) ;
#31904=CARTESIAN_POINT ( 'NONE',  ( 0.4724409448818904789, -0.1870078740157480879, -0.4822834645669291653 ) ) ;
#31906=CARTESIAN_POINT ( 'NONE',  ( 1.010498687664042716, -0.004921259842519870586, -0.3153832671262229437 ) ) ;
#31907=CARTESIAN_POINT ( 'NONE',  ( 0.3608923884514443348, 0.1771653543307087075, -0.09757992244046823083 ) ) ;
#31908=CARTESIAN_POINT ( 'NONE',  ( 0.08530183727034192087, -0.05778040916215522460, 0.4822834645669289988 ) ) ;
#31909=CARTESIAN_POINT ( 'NONE',  ( -1.417322834645668772, -0.1870078740157479769, 0.4822834645669291653 ) ) ;
#31910=CARTESIAN_POINT ( 'NONE',  ( -0.6102362204724400829, -0.4536011799217368745, -0.2665933059059886201 ) ) ;
#31911=FACE_OUTER_BOUND ( 'NONE', #80145, .T. ) ;
#31912=CARTESIAN_POINT ( 'NONE',  ( -0.4199475065616791736, -0.6046776061558807314, 0.2411417322834647770 ) ) ;
#31915=CARTESIAN_POINT ( 'NONE',  ( 0.1771653543307093182, 0.07958543189024085140, 0.2665933059059887866 ) ) ;
#31916=CARTESIAN_POINT ( 'NONE',  ( -0.4527559055118102749, -0.5400638737290845981, -0.3530559997133363437 ) ) ;
#31918=CARTESIAN_POINT ( 'NONE',  ( -1.187664041994749731, -0.3162353388693405765, 0.4822834645669290543 ) ) ;
#31919=CARTESIAN_POINT ( 'NONE',  ( -1.122047244094487306, 0.07958543189024071263, -0.2665933059059888421 ) ) ;
#31920=FACE_OUTER_BOUND ( 'NONE', #14510, .T. ) ;
#31921=CARTESIAN_POINT ( 'NONE',  ( -0.6496062992125976043, 0.1660481256975883668, -0.3530559997133364547 ) ) ;
#31922=CARTESIAN_POINT ( 'NONE',  ( -1.036745406824146176, -0.3690944881889763329, 0.3153832671262228327 ) ) ;
#31923=CARTESIAN_POINT ( 'NONE',  ( -1.450131233595799651, -0.5511811023622046335, 0.09757992244046803654 ) ) ;
#31924=CARTESIAN_POINT ( 'NONE',  ( 1.240157480314961314, -0.5400638737290844871, 0.3530559997133364547 ) ) ;
#31928=CARTESIAN_POINT ( 'NONE',  ( -0.2255212960314310344, -4.992347309556208597E-15, 0.4118484887281982920 ) ) ;
#31929=CARTESIAN_POINT ( 'NONE',  ( -1.496062992125983815, -0.1870078740157480879, -0.4822834645669291653 ) ) ;
#31930=CARTESIAN_POINT ( 'NONE',  ( -0.9776902887139098386, -0.6692913385826771977, 0.1292274648535927661 ) ) ;
#31931=CARTESIAN_POINT ( 'NONE',  ( 1.535433070866142335, -0.6692913385826771977, 8.415575281601705876E-17 ) ) ;
#31934=EDGE_CURVE ( 'NONE', #34136, #36844, #47816, .T. ) ;
#31935=CARTESIAN_POINT ( 'NONE',  ( 1.056430446194226658, 0.2952755905511811885, 0.1292274648535926551 ) ) ;
#31936=CARTESIAN_POINT ( 'NONE',  ( 0.1246719160104994284, 0.2952755905511810774, -0.1292274648535930714 ) ) ;
#31938=LINE ( 'NONE', #38666, #68061 ) ;
#31939=CARTESIAN_POINT ( 'NONE',  ( 1.115485564304462551, -0.004921259842519576551, 0.3153832671262227771 ) ) ;
#31941=ORIENTED_EDGE ( 'NONE', *, *, #69249, .F. ) ;
#31944=CARTESIAN_POINT ( 'NONE',  ( -0.1771653543307080136, -0.5400638737290844871, 0.3530559997133364547 ) ) ;
#31945=CARTESIAN_POINT ( 'NONE',  ( -0.9186351706036736120, 0.2306618581243848609, 0.2411417322834645549 ) ) ;
#31946=CARTESIAN_POINT ( 'NONE',  ( -1.541994750656167090, -0.6692913385826773087, -0.1292274648535924053 ) ) ;
#31947=CARTESIAN_POINT ( 'NONE',  ( 0.7939632545931766261, -0.3162353388693409650, -0.4822834645669289433 ) ) ;
#31948=CARTESIAN_POINT ( 'NONE',  ( -1.568241469816272105, -0.2845877964562161244, -0.3641732283464567121 ) ) ;
#31949=CARTESIAN_POINT ( 'NONE',  ( 1.351706036745407458, -0.4281496062992127816, -0.4176697321401328100 ) ) ;
#31950=CARTESIAN_POINT ( 'NONE',  ( -0.5118110236220466680, 0.2952755905511811885, 0.000000000000000000 ) ) ;
#31951=CARTESIAN_POINT ( 'NONE',  ( 0.4986876640419954376, 0.2306618581243848609, 0.2411417322834645549 ) ) ;
#31952=CARTESIAN_POINT ( 'NONE',  ( -1.115485564304461219, 0.05413385826771626580, -0.4176697321401330321 ) ) ;
#31953=CARTESIAN_POINT ( 'NONE',  ( 1.253280839895013710, -0.3162353388693405765, 0.4822834645669290543 ) ) ;
#31954=CARTESIAN_POINT ( 'NONE',  ( 1.476377952755906442, -0.5400638737290844871, 0.3530559997133364547 ) ) ;
#31955=CARTESIAN_POINT ( 'NONE',  ( -0.01312335958005186876, -0.4281496062992124485, 0.4176697321401328655 ) ) ;
#31957=CARTESIAN_POINT ( 'NONE',  ( 0.3674540682414705883, -0.5023911411419708095, 0.1820866141732285504 ) ) ;
#31961=CARTESIAN_POINT ( 'NONE',  ( -0.1837270341207343505, -0.5023911411419708095, 0.1820866141732285504 ) ) ;
#31963=CARTESIAN_POINT ( 'NONE',  ( 0.3018372703412079971, -0.4281496062992124485, 0.4176697321401328655 ) ) ;
#31964=CARTESIAN_POINT ( 'NONE',  ( -0.1443569553805768291, 0.05413385826771666132, 0.4176697321401328100 ) ) ;
#31965=CARTESIAN_POINT ( 'NONE',  ( -0.4265091863517051496, 0.2952755905511810774, -0.1292274648535930714 ) ) ;
#31967=CARTESIAN_POINT ( 'NONE',  ( -1.089238845144356427, -0.4281496062992127816, -0.4176697321401328100 ) ) ;
#31969=CARTESIAN_POINT ( 'NONE',  ( 0.7086614173228352742, -0.1870078740157480601, -0.3641732283464567677 ) ) ;
#31970=CARTESIAN_POINT ( 'NONE',  ( 1.069553805774278832, 0.2952755905511810774, -0.1292274648535930714 ) ) ;
#31971=CARTESIAN_POINT ( 'NONE',  ( 0.7020997375328090762, -0.3162353388693405765, 0.4822834645669290543 ) ) ;
#31972=EDGE_CURVE ( 'NONE', #6163, #5170, #82841, .T. ) ;
#31974=CARTESIAN_POINT ( 'NONE',  ( -1.207349081364828880, 0.2306618581243847221, -0.2411417322834647770 ) ) ;
#31977=CARTESIAN_POINT ( 'NONE',  ( -0.04593175853018302557, -0.6692913385826773087, -0.1292274648535924053 ) ) ;
#31980=CARTESIAN_POINT ( 'NONE',  ( 1.437007874015748810, 0.1660481256975885056, 0.3530559997133364547 ) ) ;
#31982=CARTESIAN_POINT ( 'NONE',  ( 1.200787401574803681, 0.1660481256975885056, 0.3530559997133364547 ) ) ;
#31983=CARTESIAN_POINT ( 'NONE',  ( 0.1181102362204730916, 0.1771653543307087630, 0.000000000000000000 ) ) ;
#31984=CARTESIAN_POINT ( 'NONE',  ( 0.7349081364829402885, -0.6046776061558809534, -0.2411417322834644161 ) ) ;
#31986=CARTESIAN_POINT ( 'NONE',  ( 0.1443569553805781891, -0.004921259842519870586, -0.3153832671262229437 ) ) ;
#31987=CARTESIAN_POINT ( 'NONE',  ( 0.5774278215223103139, -0.6046776061558809534, -0.2411417322834644161 ) ) ;
#31989=CARTESIAN_POINT ( 'NONE',  ( -1.128608923884513837, -0.6046776061558807314, 0.2411417322834647770 ) ) ;
#31990=CARTESIAN_POINT ( 'NONE',  ( 0.9251968503937015864, -0.4536011799217367080, 0.2665933059059888421 ) ) ;
#31991=CARTESIAN_POINT ( 'NONE',  ( -1.154855643044618851, 0.2306618581243848609, 0.2411417322834645549 ) ) ;
#31992=CARTESIAN_POINT ( 'NONE',  ( -0.2624671916010490880, 0.2306618581243847221, -0.2411417322834647770 ) ) ;
#31993=B_SPLINE_CURVE_WITH_KNOTS ( 'NONE', 3,
 ( #62872, #63689, #81834, #76335 ),
 .UNSPECIFIED., .F., .F.,
 ( 4, 4 ),
 ( 0.000000000000000000, 0.001510660848369282418 ),
 .UNSPECIFIED. ) ;
#31994=CARTESIAN_POINT ( 'NONE',  ( -0.4002624671916004129, -0.2845877964562159024, 0.3641732283464567677 ) ) ;
#31996=CARTESIAN_POINT ( 'NONE',  ( -0.4396325459317579898, 0.2952755905511811885, 0.1292274648535926551 ) ) ;
#31997=CARTESIAN_POINT ( 'NONE',  ( 0.3083989501312343062, -0.2845877964562159024, 0.3641732283464567677 ) ) ;
#31999=CARTESIAN_POINT ( 'NONE',  ( 0.04593175853018440641, -0.6692913385826771977, 0.1292274648535927661 ) ) ;
#32002=CARTESIAN_POINT ( 'NONE',  ( 1.187664041994751285, -0.08942795157527998196, 0.3641732283464567121 ) ) ;
#32004=CARTESIAN_POINT ( 'NONE',  ( -0.6364829396325453192, -0.2845877964562159024, 0.3641732283464567677 ) ) ;
#32005=CARTESIAN_POINT ( 'NONE',  ( -0.6299212598425188991, -0.1870078740157479769, 0.3641732283464567677 ) ) ;
#32006=CARTESIAN_POINT ( 'NONE',  ( -0.8398950131233585692, 0.2306618581243848609, 0.2411417322834645549 ) ) ;
#32007=CARTESIAN_POINT ( 'NONE',  ( -0.1837270341207343505, -0.6046776061558807314, 0.2411417322834647770 ) ) ;
#32008=CARTESIAN_POINT ( 'NONE',  ( 0.6299212598425204535, -0.1870078740157480601, -0.3641732283464567677 ) ) ;
#32010=CARTESIAN_POINT ( 'NONE',  ( 1.364829396325459854, -0.5023911411419708095, -0.1820866141732282451 ) ) ;
#32011=CARTESIAN_POINT ( 'NONE',  ( 0.7152230971128616943, -0.05778040916215522460, 0.4822834645669289988 ) ) ;
#32013=CARTESIAN_POINT ( 'NONE',  ( -0.2624671916010490880, 0.2306618581243847221, -0.2411417322834647770 ) ) ;
#32015=CARTESIAN_POINT ( 'NONE',  ( -1.581364829396324945, -0.3162353388693405765, 0.4822834645669290543 ) ) ;
#32016=CARTESIAN_POINT ( 'NONE',  ( 0.8530183727034128527, -0.4281496062992124485, 0.4176697321401328655 ) ) ;
#32017=CARTESIAN_POINT ( 'NONE',  ( 0.3674540682414705883, -0.6046776061558807314, 0.2411417322834647770 ) ) ;
#32019=CARTESIAN_POINT ( 'NONE',  ( 0.1771653543307093182, -0.4536011799217368745, -0.2665933059059886201 ) ) ;
#32020=CARTESIAN_POINT ( 'NONE',  ( 1.377952755905512472, 0.2952755905511811885, 0.000000000000000000 ) ) ;
#32021=CARTESIAN_POINT ( 'NONE',  ( -0.3740157480314953431, -0.4536011799217368745, -0.2665933059059886201 ) ) ;
#32022=CARTESIAN_POINT ( 'NONE',  ( -0.5380577427821514602, 0.05413385826771666132, 0.4176697321401328100 ) ) ;
#32023=CARTESIAN_POINT ( 'NONE',  ( 0.8545558659330633189, 0.02791078216816508459, -0.4328096321851889194 ) ) ;
#32024=CARTESIAN_POINT ( 'NONE',  ( 0.08530183727034192087, -0.3162353388693409650, -0.4822834645669289433 ) ) ;
#32025=CARTESIAN_POINT ( 'NONE',  ( -0.6627296587926501115, 0.2952755905511810774, -0.1292274648535930714 ) ) ;
#32026=CARTESIAN_POINT ( 'NONE',  ( -0.8267716535433065062, -0.5511811023622047445, 6.969142054262312111E-17 ) ) ;
#32027=CARTESIAN_POINT ( 'NONE',  ( 0.3149606299212603933, -0.1870078740157479769, 0.4822834645669291653 ) ) ;
#32028=B_SPLINE_CURVE_WITH_KNOTS ( 'NONE', 3,
 ( #45293, #20478, #13753, #20056, #70989, #33520, #45709 ),
 .UNSPECIFIED., .F., .F.,
 ( 4, 3, 4 ),
 ( 1.387778780781445676E-17, 0.001246230184515618360, 0.002492489877932651567 ),
 .UNSPECIFIED. ) ;
#32029=CARTESIAN_POINT ( 'NONE',  ( -1.220472440944881054, 0.2952755905511811885, 0.000000000000000000 ) ) ;
#32030=CARTESIAN_POINT ( 'NONE',  ( -0.3346456692913377662, 0.1660481256975883668, -0.3530559997133364547 ) ) ;
#32033=CARTESIAN_POINT ( 'NONE',  ( 1.528871391076116026, -0.6692913385826773087, -0.1292274648535924053 ) ) ;
#32034=CARTESIAN_POINT ( 'NONE',  ( 1.122047244094488860, -0.5400638737290845981, -0.3530559997133363437 ) ) ;
#32036=CARTESIAN_POINT ( 'NONE',  ( -1.496062992125983815, -0.1870078740157479769, 0.4822834645669291653 ) ) ;
#32037=CARTESIAN_POINT ( 'NONE',  ( -0.8005249343832013809, -0.4281496062992124485, 0.4176697321401328655 ) ) ;
#32041=CARTESIAN_POINT ( 'NONE',  ( -0.05249343832020911260, 0.1283753931104748280, 0.1820866141732283561 ) ) ;
#32043=CARTESIAN_POINT ( 'NONE',  ( 0.6889763779527563470, 0.1660481256975883668, -0.3530559997133364547 ) ) ;
#32045=CARTESIAN_POINT ( 'NONE',  ( -1.586052503253846169, 1.850393700787402729, -0.1653254495020583803 ) ) ;
#32046=CARTESIAN_POINT ( 'NONE',  ( -0.3740157480314953431, 0.07958543189024085140, 0.2665933059059887866 ) ) ;
#32048=CARTESIAN_POINT ( 'NONE',  ( 1.279527559055118724, -0.5400638737290845981, -0.3530559997133363437 ) ) ;
#32049=CARTESIAN_POINT ( 'NONE',  ( 0.7414698162729663755, -0.5511811023622048555, -0.09757992244046775898 ) ) ;
#32050=CARTESIAN_POINT ( 'NONE',  ( -0.06561679790026180015, 0.05413385826771666132, 0.4176697321401328100 ) ) ;
#32052=CARTESIAN_POINT ( 'NONE',  ( -1.023622047244093558, -0.1870078740157479769, 0.4822834645669291653 ) ) ;
#32053=CARTESIAN_POINT ( 'NONE',  ( -1.148293963254592542, -0.5511811023622048555, -0.09757992244046775898 ) ) ;
#32054=CARTESIAN_POINT ( 'NONE',  ( -0.4790026246719154557, -0.3162353388693405765, 0.4822834645669290543 ) ) ;
#32055=LINE ( 'NONE', #62815, #11246 ) ;
#32059=CARTESIAN_POINT ( 'NONE',  ( 0.4593175853018380828, 0.05413385826771626580, -0.4176697321401330321 ) ) ;
#32061=CARTESIAN_POINT ( 'NONE',  ( -0.5774278215223089816, 0.2306618581243847221, -0.2411417322834647770 ) ) ;
#32062=CARTESIAN_POINT ( 'NONE',  ( 1.574803149606299746, -0.1870078740157479769, 0.4822834645669291653 ) ) ;
#32063=CARTESIAN_POINT ( 'NONE',  ( 0.6692913385826777528, 0.2952755905511811885, 0.000000000000000000 ) ) ;
#32064=CARTESIAN_POINT ( 'NONE',  ( 0.2362204724409456558, -0.1870078740157479769, 0.4822834645669291653 ) ) ;
#32066=CARTESIAN_POINT ( 'NONE',  ( -0.8005249343832013809, -0.4281496062992124485, 0.4176697321401328655 ) ) ;
#32067=CARTESIAN_POINT ( 'NONE',  ( -0.05249343832020911260, 0.2306618581243848609, 0.2411417322834645549 ) ) ;
#32068=CARTESIAN_POINT ( 'NONE',  ( -0.05905511811023545637, 0.07958543189024085140, 0.2665933059059887866 ) ) ;
#32070=EDGE_CURVE ( 'NONE', #38656, #7120, #82153, .T. ) ;
#32071=CARTESIAN_POINT ( 'NONE',  ( -0.01312335958005186876, -0.4281496062992124485, 0.4176697321401328655 ) ) ;
#32073=CARTESIAN_POINT ( 'NONE',  ( 1.135170603674541256, 0.2952755905511811885, 0.1292274648535926551 ) ) ;
#32075=ORIENTED_EDGE ( 'NONE', *, *, #60399, .F. ) ;
#32077=CARTESIAN_POINT ( 'NONE',  ( 0.08530183727034192087, -0.05778040916215522460, 0.4822834645669289988 ) ) ;
#32078=CARTESIAN_POINT ( 'NONE',  ( -0.1443569553805768291, -0.004921259842519576551, 0.3153832671262227771 ) ) ;
#32079=CARTESIAN_POINT ( 'NONE',  ( 1.456692913385827515, -0.5511811023622047445, 6.969142054262312111E-17 ) ) ;
#32080=DIRECTION ( 'NONE',  ( 1.000000000000000000, -0.000000000000000000, -0.000000000000000000 ) ) ;
#32083=CARTESIAN_POINT ( 'NONE',  ( 1.423884514435696413, -0.2845877964562161244, -0.3641732283464567121 ) ) ;
#32084=CARTESIAN_POINT ( 'NONE',  ( 1.456692913385827515, 0.2952755905511811885, 0.000000000000000000 ) ) ;
#32086=CARTESIAN_POINT ( 'NONE',  ( -0.07874015748031421014, -0.1870078740157480879, -0.4822834645669291653 ) ) ;
#32087=CARTESIAN_POINT ( 'NONE',  ( -1.338582677165353729, -0.1870078740157479769, 0.4822834645669291653 ) ) ;
#32088=CARTESIAN_POINT ( 'NONE',  ( -1.069553805774277722, 0.2952755905511811885, 0.1292274648535926551 ) ) ;
#32089=CARTESIAN_POINT ( 'NONE',  ( 0.3412073490813655186, 0.2306618581243848609, 0.2411417322834645549 ) ) ;
#32091=CARTESIAN_POINT ( 'NONE',  ( -1.581364829396324945, -0.08942795157528024563, -0.3641732283464568787 ) ) ;
#32092=CARTESIAN_POINT ( 'NONE',  ( 1.102362204724410155, -0.1870078740157479769, 0.4822834645669291653 ) ) ;
#32093=CARTESIAN_POINT ( 'NONE',  ( 0.7677165354330716118, 0.07958543189024071263, -0.2665933059059888421 ) ) ;
#32094=CARTESIAN_POINT ( 'NONE',  ( 0.8136482939632553313, 0.1539470093639523085, 0.1968503937007873850 ) ) ;
#32095=CARTESIAN_POINT ( 'NONE',  ( 0.9383202099737538715, -0.08942795157528024563, -0.3641732283464568787 ) ) ;
#32096=CARTESIAN_POINT ( 'NONE',  ( -1.482939632545930975, 0.05413385826771666132, 0.4176697321401328100 ) ) ;
#32098=CARTESIAN_POINT ( 'NONE',  ( 1.220472440944882608, 0.2952755905511811885, 0.000000000000000000 ) ) ;
#32102=CARTESIAN_POINT ( 'NONE',  ( 0.5380577427821529035, -0.4281496062992124485, 0.4176697321401328655 ) ) ;
#32103=CARTESIAN_POINT ( 'NONE',  ( 1.586052503253845281, 0.7480314960629931287, -0.1653254495020588799 ) ) ;
#32104=CARTESIAN_POINT ( 'NONE',  ( -1.568241469816272105, -0.08942795157527998196, 0.3641732283464567121 ) ) ;
#32105=CARTESIAN_POINT ( 'NONE',  ( 0.06561679790026316017, -0.4281496062992124485, 0.4176697321401328655 ) ) ;
#32106=CARTESIAN_POINT ( 'NONE',  ( 0.5183727034120741983, 0.1771653543307087075, -0.09757992244046823083 ) ) ;
#32107=CARTESIAN_POINT ( 'NONE',  ( 0.9842519685039378130, -0.6692913385826771977, 8.415575281601705876E-17 ) ) ;
#32109=CARTESIAN_POINT ( 'NONE',  ( 0.7746288504648943807, 0.004960608223779807216, -0.3437734562760184631 ) ) ;
#32110=CARTESIAN_POINT ( 'NONE',  ( -0.6955380577427815458, -0.3690944881889765550, -0.3153832671262227771 ) ) ;
#32111=CARTESIAN_POINT ( 'NONE',  ( -0.7677165354330699465, 0.1660481256975885056, 0.3530559997133364547 ) ) ;
#32112=CARTESIAN_POINT ( 'NONE',  ( 1.607611548556431069, -0.6692913385826773087, -0.1292274648535924053 ) ) ;
#32113=CARTESIAN_POINT ( 'NONE',  ( -1.167979002624671470, -0.4281496062992127816, -0.4176697321401328100 ) ) ;
#32114=CARTESIAN_POINT ( 'NONE',  ( 0.9251968503937015864, 0.1660481256975883668, -0.3530559997133364547 ) ) ;
#32115=CARTESIAN_POINT ( 'NONE',  ( -1.358267716535432434, -0.4536011799217367080, 0.2665933059059888421 ) ) ;
#32117=CARTESIAN_POINT ( 'NONE',  ( 0.8398950131233602345, 0.2306618581243847221, -0.2411417322834647770 ) ) ;
#32119=CARTESIAN_POINT ( 'NONE',  ( -1.502624671916009680, -0.05778040916215560624, -0.4822834645669293319 ) ) ;
#32120=CARTESIAN_POINT ( 'NONE',  ( -1.594488188976377119, 0.07958543189024071263, -0.2665933059059888421 ) ) ;
#32121=CARTESIAN_POINT ( 'NONE',  ( -1.167979002624671470, -0.3690944881889765550, -0.3153832671262227771 ) ) ;
#32122=CARTESIAN_POINT ( 'NONE',  ( 1.535433070866142558, 0.1771653543307087630, 0.000000000000000000 ) ) ;
#32123=CARTESIAN_POINT ( 'NONE',  ( -0.5511811023622038563, -0.1870078740157479769, 0.4822834645669291653 ) ) ;
#32124=CARTESIAN_POINT ( 'NONE',  ( -0.2755905511811015396, -0.5511811023622047445, 6.969142054262312111E-17 ) ) ;
#32125=CARTESIAN_POINT ( 'NONE',  ( -1.561679790026246017, -0.004921259842519576551, 0.3153832671262227771 ) ) ;
#32126=CARTESIAN_POINT ( 'NONE',  ( 0.8136482939632553313, 0.1283753931104748280, 0.1820866141732283561 ) ) ;
#32127=CARTESIAN_POINT ( 'NONE',  ( 0.4133858267716541968, 0.1660481256975885056, 0.3530559997133364547 ) ) ;
#32128=CARTESIAN_POINT ( 'NONE',  ( 1.417322834645670104, -0.1870078740157479769, 0.4822834645669291653 ) ) ;
#32129=CARTESIAN_POINT ( 'NONE',  ( 0.6233595800524942554, -0.05778040916215560624, -0.4822834645669293319 ) ) ;
#32131=CARTESIAN_POINT ( 'NONE',  ( 0.5118110236220478892, 0.1771653543307087630, 0.000000000000000000 ) ) ;
#32132=CARTESIAN_POINT ( 'NONE',  ( 1.515748031496063186, -0.5400638737290845981, -0.3530559997133363437 ) ) ;
#32133=CARTESIAN_POINT ( 'NONE',  ( -1.181102362204723644, -0.1870078740157479769, 0.4822834645669291653 ) ) ;
#32134=CARTESIAN_POINT ( 'NONE',  ( -0.5249343832020990641, -0.6046776061558809534, -0.2411417322834644161 ) ) ;
#32137=CARTESIAN_POINT ( 'NONE',  ( 0.4330708661417329575, -0.6692913385826771977, 8.415575281601705876E-17 ) ) ;
#32138=CARTESIAN_POINT ( 'NONE',  ( 1.266404199475066328, -0.08942795157527998196, 0.3641732283464567121 ) ) ;
#32139=CARTESIAN_POINT ( 'NONE',  ( -0.3543307086614165824, 0.2952755905511811885, 0.000000000000000000 ) ) ;
#32140=CARTESIAN_POINT ( 'NONE',  ( 0.3805774278215230400, 0.05413385826771626580, -0.4176697321401330321 ) ) ;
#32147=CARTESIAN_POINT ( 'NONE',  ( -0.8661417322834640276, -0.1870078740157480601, -0.3641732283464567677 ) ) ;
#32148=CARTESIAN_POINT ( 'NONE',  ( -1.010498687664041384, -0.4281496062992127816, -0.4176697321401328100 ) ) ;
#32150=ADVANCED_FACE ( 'NONE', ( #73091 ), #20200, .F. ) ;
#32151=CARTESIAN_POINT ( 'NONE',  ( 0.9186351706036752773, 0.2306618581243847221, -0.2411417322834647770 ) ) ;
#32152=CARTESIAN_POINT ( 'NONE',  ( 1.305774278215223960, 0.2952755905511810774, -0.1292274648535930714 ) ) ;
#32153=CARTESIAN_POINT ( 'NONE',  ( 0.8333333333333340365, 0.2952755905511810774, -0.1292274648535930714 ) ) ;
#32154=CARTESIAN_POINT ( 'NONE',  ( -0.6195821328811238482, -4.378520898609941727E-15, 0.4281989832122462536 ) ) ;
#32157=CARTESIAN_POINT ( 'NONE',  ( -0.7443564587111901609, 2.201272808314826079, 0.5309055118110236338 ) ) ;
#32158=CARTESIAN_POINT ( 'NONE',  ( 0.5839895013123367340, -0.6692913385826773087, -0.1292274648535924053 ) ) ;
#32159=CARTESIAN_POINT ( 'NONE',  ( 0.2230971128608929543, 0.05413385826771626580, -0.4176697321401330321 ) ) ;
#32160=CARTESIAN_POINT ( 'NONE',  ( 0.8136482939632553313, 0.1283753931104748280, 0.1820866141732283561 ) ) ;
#32161=CARTESIAN_POINT ( 'NONE',  ( 1.515748031496063408, 0.1660481256975885056, 0.3530559997133364547 ) ) ;
#32163=CARTESIAN_POINT ( 'NONE',  ( 0.5774278215223103139, -0.6046776061558809534, -0.2411417322834644161 ) ) ;
#32164=CARTESIAN_POINT ( 'NONE',  ( 1.253280839895013710, -0.05778040916215560624, -0.4822834645669293319 ) ) ;
#32165=CARTESIAN_POINT ( 'NONE',  ( 0.1968503937007881344, -0.6692913385826771977, 8.415575281601705876E-17 ) ) ;
#32166=CARTESIAN_POINT ( 'NONE',  ( 1.135170603674541256, -0.5511811023622048555, -0.09757992244046775898 ) ) ;
#32167=CARTESIAN_POINT ( 'NONE',  ( -1.030183727034119867, -0.05778040916215560624, -0.4822834645669293319 ) ) ;
#32168=CARTESIAN_POINT ( 'NONE',  ( -0.8464566929133852113, -0.5400638737290845981, -0.3530559997133363437 ) ) ;
#32169=CARTESIAN_POINT ( 'NONE',  ( 1.108923884514436242, -0.05778040916215522460, 0.4822834645669289988 ) ) ;
#32174=EDGE_LOOP ( 'NONE', ( #67055, #63431, #56708, #2134, #26995, #74416, #78364, #48209, #47489, #52224, #75653, #12028, #28247, #10379, #41523, #39437, #33130, #3521, #22761, #9388, #56891, #18279, #33006, #82389, #44873, #5849, #26877, #36698, #11891, #58275, #61800, #36330, #81576, #66879, #56676, #20412, #20661, #8896, #48953, #79493, #64679, #8711, #13686, #71623, #38901, #34265, #77213, #76699, #45805, #27712, #49967, #47886, #34685, #52050, #74013, #2247, #30888, #32774, #41928, #82407, #28665, #58762, #61169, #12019, #41989, #52969, #33716, #72725, #10415 ) ) ;
#32176=VERTEX_POINT ( 'NONE', #50702 ) ;
#32177=CARTESIAN_POINT ( 'NONE',  ( 1.377952755905512472, 0.2952755905511811885, 0.000000000000000000 ) ) ;
#32178=CARTESIAN_POINT ( 'NONE',  ( 1.122047244094488860, 0.07958543189024085140, 0.2665933059059887866 ) ) ;
#32180=CARTESIAN_POINT ( 'NONE',  ( 1.233595800524935227, 0.1283753931104746893, -0.1820866141732285504 ) ) ;
#32181=CARTESIAN_POINT ( 'NONE',  ( 0.4556365139439955136, 1.537493841899424618, -0.5309055118110237448 ) ) ;
#32182=CARTESIAN_POINT ( 'NONE',  ( -0.1377952755905504645, 0.1660481256975885056, 0.3530559997133364547 ) ) ;
#32185=CARTESIAN_POINT ( 'NONE',  ( -1.213910761154854745, -0.5511811023622046335, 0.09757992244046803654 ) ) ;
#32186=CARTESIAN_POINT ( 'NONE',  ( -1.423884514435694859, -0.2845877964562159024, 0.3641732283464567677 ) ) ;
#32187=CARTESIAN_POINT ( 'NONE',  ( -1.122047244094487306, 0.1660481256975883668, -0.3530559997133364547 ) ) ;
#32188=CARTESIAN_POINT ( 'NONE',  ( 0.03937007874015806264, 0.2952755905511811885, 0.000000000000000000 ) ) ;
#32189=CARTESIAN_POINT ( 'NONE',  ( 1.423884514435696191, -0.05778040916215522460, 0.4822834645669289988 ) ) ;
#32191=CARTESIAN_POINT ( 'NONE',  ( -1.141732283464566011, 0.2066929133858268208, 0.000000000000000000 ) ) ;
#32195=CARTESIAN_POINT ( 'NONE',  ( -0.9973753280839886548, 0.1283753931104748280, 0.1820866141732283561 ) ) ;
#32196=( BOUNDED_CURVE ( )  B_SPLINE_CURVE ( 3, ( #46281, #7588, #861, #58497 ),
 .UNSPECIFIED., .F., .F. ) 
 B_SPLINE_CURVE_WITH_KNOTS ( ( 4, 4 ),
 ( 1.859270518042426046, 2.743397753083149482 ),
 .UNSPECIFIED. ) 
 CURVE ( )  GEOMETRIC_REPRESENTATION_ITEM ( )  RATIONAL_B_SPLINE_CURVE ( ( 1.000000000000000000, 0.9359138408343250504, 0.9359138408343250504, 1.000000000000000000 ) ) 
 REPRESENTATION_ITEM ( '' )  );
#32197=CARTESIAN_POINT ( 'NONE',  ( -1.272965879265091305, 0.05413385826771626580, -0.4176697321401330321 ) ) ;
#32198=CARTESIAN_POINT ( 'NONE',  ( 1.194225721784777594, 0.05413385826771666132, 0.4176697321401328100 ) ) ;
#32201=DIRECTION ( 'NONE',  ( -0.000000000000000000, 1.000000000000000000, -0.000000000000000000 ) ) ;
#32202=CARTESIAN_POINT ( 'NONE',  ( 1.286089238845145033, -0.6046776061558809534, -0.2411417322834644161 ) ) ;
#32203=CARTESIAN_POINT ( 'NONE',  ( -1.167979002624671470, -0.4281496062992127816, -0.4176697321401328100 ) ) ;
#32205=CARTESIAN_POINT ( 'NONE',  ( -0.4461942257217840213, 0.1283753931104748280, 0.1820866141732283561 ) ) ;
#32207=CARTESIAN_POINT ( 'NONE',  ( -0.6758530183727028406, 0.1771653543307087630, 0.09757992244046791164 ) ) ;
#32208=CARTESIAN_POINT ( 'NONE',  ( -0.05905511811023545637, -0.4536011799217368745, -0.2665933059059886201 ) ) ;
#32209=CARTESIAN_POINT ( 'NONE',  ( 0.2034120734908142214, 0.2952755905511810774, -0.1292274648535930714 ) ) ;
#32210=CARTESIAN_POINT ( 'NONE',  ( -1.345144356955379816, -0.2845877964562159024, 0.3641732283464567677 ) ) ;
#32212=CARTESIAN_POINT ( 'NONE',  ( 1.194225721784777594, -0.4281496062992127816, -0.4176697321401328100 ) ) ;
#32213=CARTESIAN_POINT ( 'NONE',  ( -1.541994750656167090, -0.6692913385826773087, -0.1292274648535924053 ) ) ;
#32215=CARTESIAN_POINT ( 'NONE',  ( -0.2296587926509179312, -0.3162353388693409650, -0.4822834645669289433 ) ) ;
#32217=CARTESIAN_POINT ( 'NONE',  ( -0.8464566929133852113, 0.1660481256975885056, 0.3530559997133364547 ) ) ;
#32218=CARTESIAN_POINT ( 'NONE',  ( 0.7545931758530189937, 0.1771653543307087075, -0.09757992244046823083 ) ) ;
#32219=CARTESIAN_POINT ( 'NONE',  ( -0.3215223097112853146, -0.2845877964562159024, 0.3641732283464567677 ) ) ;
#32220=CARTESIAN_POINT ( 'NONE',  ( -0.6496062992125976043, -0.5400638737290844871, 0.3530559997133364547 ) ) ;
#32221=CARTESIAN_POINT ( 'NONE',  ( -1.614173228346455824, 0.2952755905511811885, 0.000000000000000000 ) ) ;
#32223=CARTESIAN_POINT ( 'NONE',  ( 1.213910761154856299, 0.1771653543307087630, 0.09757992244046791164 ) ) ;
#32225=CARTESIAN_POINT ( 'NONE',  ( -0.1312335958005241554, -0.6046776061558809534, -0.2411417322834644161 ) ) ;
#32226=CARTESIAN_POINT ( 'NONE',  ( -1.509186351706035767, 0.05413385826771626580, -0.4176697321401330321 ) ) ;
#32229=CARTESIAN_POINT ( 'NONE',  ( -0.8333333333333323711, 0.1771653543307087630, 0.09757992244046791164 ) ) ;
#32230=CARTESIAN_POINT ( 'NONE',  ( 0.9317585301837276734, -0.4281496062992124485, 0.4176697321401328655 ) ) ;
#32231=CARTESIAN_POINT ( 'NONE',  ( -1.213910761154854745, 0.1771653543307087075, -0.09757992244046823083 ) ) ;
#32233=CARTESIAN_POINT ( 'NONE',  ( -0.9383202099737524282, -0.05778040916215522460, 0.4822834645669289988 ) ) ;
#32234=CARTESIAN_POINT ( 'NONE',  ( 0.7545931758530189937, 0.2952755905511810774, -0.1292274648535930714 ) ) ;
#32235=CARTESIAN_POINT ( 'NONE',  ( 0.5446194225721792126, -0.3162353388693405765, 0.4822834645669290543 ) ) ;
#32236=CARTESIAN_POINT ( 'NONE',  ( 1.581364829396326277, -0.05778040916215522460, 0.4822834645669289988 ) ) ;
#32237=CARTESIAN_POINT ( 'NONE',  ( -1.358267716535432434, 0.07958543189024071263, -0.2665933059059888421 ) ) ;
#32242=CARTESIAN_POINT ( 'NONE',  ( 1.049868766404200349, 0.1283753931104748280, 0.1820866141732283561 ) ) ;
#32243=CARTESIAN_POINT ( 'NONE',  ( 0.4855643044619428750, -0.004921259842519576551, 0.3153832671262227771 ) ) ;
#32244=CARTESIAN_POINT ( 'NONE',  ( 0.3018372703412079971, -0.4281496062992124485, 0.4176697321401328655 ) ) ;
#32245=CARTESIAN_POINT ( 'NONE',  ( 1.397637795275591177, -0.5400638737290844871, 0.3530559997133364547 ) ) ;
#32247=CARTESIAN_POINT ( 'NONE',  ( 0.2952755905511819101, 0.07958543189024071263, -0.2665933059059888421 ) ) ;
#32248=CARTESIAN_POINT ( 'NONE',  ( -0.8858267716535425107, -0.5400638737290844871, 0.3530559997133364547 ) ) ;
#32249=CARTESIAN_POINT ( 'NONE',  ( -1.430446194225720724, 0.05413385826771626580, -0.4176697321401330321 ) ) ;
#32250=CARTESIAN_POINT ( 'NONE',  ( 0.9251968503937015864, 0.1660481256975883668, -0.3530559997133364547 ) ) ;
#32252=CARTESIAN_POINT ( 'NONE',  ( -1.220472440944881276, 0.4405861044731111953, 0.5309055118110234117 ) ) ;
#32255=CARTESIAN_POINT ( 'NONE',  ( -1.259842519685038686, -0.1870078740157479769, 0.4822834645669291653 ) ) ;
#32256=CARTESIAN_POINT ( 'NONE',  ( -0.6758530183727028406, 0.2952755905511811885, 0.1292274648535926551 ) ) ;
#32257=CARTESIAN_POINT ( 'NONE',  ( -0.9317585301837263412, -0.3690944881889765550, -0.3153832671262227771 ) ) ;
#32258=CARTESIAN_POINT ( 'NONE',  ( -0.6824146981627288167, 0.2306618581243848609, 0.2411417322834645549 ) ) ;
#32261=CARTESIAN_POINT ( 'NONE',  ( -1.581364829396324945, -0.08942795157528024563, -0.3641732283464568787 ) ) ;
#32262=CARTESIAN_POINT ( 'NONE',  ( -1.345144356955379816, -0.05778040916215560624, -0.4822834645669293319 ) ) ;
#32263=CARTESIAN_POINT ( 'NONE',  ( 0.5249343832021003964, 0.2306618581243847221, -0.2411417322834647770 ) ) ;
#32264=CARTESIAN_POINT ( 'NONE',  ( -1.010498687664041384, 0.05413385826771666132, 0.4176697321401328100 ) ) ;
#32265=B_SPLINE_CURVE_WITH_KNOTS ( 'NONE', 3,
 ( #37568, #76703, #5582, #103, #25757, #19454, #70811 ),
 .UNSPECIFIED., .F., .F.,
 ( 4, 3, 4 ),
 ( 7.287419555744632558E-17, 0.001246232571205270478, 0.002492492258783315755 ),
 .UNSPECIFIED. ) ;
#32267=CARTESIAN_POINT ( 'NONE',  ( -0.6561679790026240244, 0.1283753931104746893, -0.1820866141732285504 ) ) ;
#32268=ORIENTED_EDGE ( 'NONE', *, *, #20062, .T. ) ;
#32270=ORIENTED_EDGE ( 'NONE', *, *, #14233, .T. ) ;
#32271=CARTESIAN_POINT ( 'NONE',  ( -1.706036745406823485, 0.1283753931104748280, 0.1820866141732283561 ) ) ;
#32272=CARTESIAN_POINT ( 'NONE',  ( -1.253280839895012377, -0.3162353388693409650, -0.4822834645669289433 ) ) ;
#32273=CARTESIAN_POINT ( 'NONE',  ( -0.8136482939632537770, 0.2306618581243847221, -0.2411417322834647770 ) ) ;
#32275=CARTESIAN_POINT ( 'NONE',  ( -1.253280839895012377, -0.05778040916215522460, 0.4822834645669289988 ) ) ;
#32276=CARTESIAN_POINT ( 'NONE',  ( -1.377952755905511140, 0.2952755905511811885, 0.000000000000000000 ) ) ;
#32278=CARTESIAN_POINT ( 'NONE',  ( 0.6627296587926517768, -0.5511811023622048555, -0.09757992244046775898 ) ) ;
#32281=CARTESIAN_POINT ( 'NONE',  ( -0.3412073490813641308, -0.5023911411419708095, 0.1820866141732285504 ) ) ;
#32282=CARTESIAN_POINT ( 'NONE',  ( -0.7217847769028863381, -0.4281496062992124485, 0.4176697321401328655 ) ) ;
#32283=CARTESIAN_POINT ( 'NONE',  ( 1.286089238845145033, 0.2306618581243848609, 0.2411417322834645549 ) ) ;
#32284=CARTESIAN_POINT ( 'NONE',  ( -0.4461942257217840213, -0.6046776061558809534, -0.2411417322834644161 ) ) ;
#32288=CARTESIAN_POINT ( 'NONE',  ( -1.043307086614172041, -0.5400638737290844871, 0.3530559997133364547 ) ) ;
#32289=CARTESIAN_POINT ( 'NONE',  ( 1.128608923884514947, 0.2306618581243848609, 0.2411417322834645549 ) ) ;
#32290=CARTESIAN_POINT ( 'NONE',  ( -1.148293963254592542, -0.5511811023622048555, -0.09757992244046775898 ) ) ;
#32291=CARTESIAN_POINT ( 'NONE',  ( -1.240157480314959759, 0.1660481256975885056, 0.3530559997133364547 ) ) ;
#32296=CARTESIAN_POINT ( 'NONE',  ( 0.2755905511811031494, 0.2952755905511811885, 0.000000000000000000 ) ) ;
#32297=CARTESIAN_POINT ( 'NONE',  ( -0.9448818897637790704, -0.1870078740157480601, -0.3641732283464567677 ) ) ;
#32298=CARTESIAN_POINT ( 'NONE',  ( -0.5708661417322828946, 0.1660481256975883668, -0.3530559997133364547 ) ) ;
#32300=CARTESIAN_POINT ( 'NONE',  ( -1.108923884514435132, -0.3162353388693405765, 0.4822834645669290543 ) ) ;
#32301=CARTESIAN_POINT ( 'NONE',  ( -0.9448818897637790704, -0.1870078740157479769, 0.4822834645669291653 ) ) ;
#32302=CARTESIAN_POINT ( 'NONE',  ( 0.1181102362204730916, -0.6692913385826771977, 8.415575281601705876E-17 ) ) ;
#32304=CARTESIAN_POINT ( 'NONE',  ( 1.076115485564305141, -0.5023911411419708095, 0.1820866141732285504 ) ) ;
#32305=CARTESIAN_POINT ( 'NONE',  ( -0.5774278215223089816, 0.1283753931104746893, -0.1820866141732285504 ) ) ;
#32307=CARTESIAN_POINT ( 'NONE',  ( 0.6692913385826778638, -0.5511811023622047445, 6.969142054262312111E-17 ) ) ;
#32308=CARTESIAN_POINT ( 'NONE',  ( 1.541994750656168645, -0.5511811023622046335, 0.09757992244046803654 ) ) ;
#32309=CARTESIAN_POINT ( 'NONE',  ( 1.207349081364829990, -0.6046776061558809534, -0.2411417322834644161 ) ) ;
#32310=CARTESIAN_POINT ( 'NONE',  ( 0.1115485564304470323, 0.1771653543307087630, 0.09757992244046791164 ) ) ;
#32312=CARTESIAN_POINT ( 'NONE',  ( -1.003937007874014853, 0.1660481256975885056, 0.3530559997133364547 ) ) ;
#32313=CARTESIAN_POINT ( 'NONE',  ( 1.207349081364829990, -0.6046776061558809534, -0.2411417322834644161 ) ) ;
#32315=CARTESIAN_POINT ( 'NONE',  ( -0.3083989501312330295, -0.2845877964562161244, -0.3641732283464567121 ) ) ;
#32318=CARTESIAN_POINT ( 'NONE',  ( 0.1181102362204730916, 0.2952755905511811885, 0.000000000000000000 ) ) ;
#32320=CARTESIAN_POINT ( 'NONE',  ( 1.148293963254593653, 0.1771653543307087075, -0.09757992244046823083 ) ) ;
#32321=CARTESIAN_POINT ( 'NONE',  ( 0.3543307086614179147, 0.1771653543307087630, 0.000000000000000000 ) ) ;
#32322=CARTESIAN_POINT ( 'NONE',  ( 0.09186351706036827158, 0.05413385826771666132, 0.4176697321401328100 ) ) ;
#32323=CARTESIAN_POINT ( 'NONE',  ( -1.332020997375327642, -0.3162353388693409650, -0.4822834645669289433 ) ) ;
#32324=CARTESIAN_POINT ( 'NONE',  ( -0.6561679790026240244, 0.1283753931104746893, -0.1820866141732285504 ) ) ;
#32326=VECTOR ( 'NONE', #76085, 39.37007874015748143 ) ;
#32327=CARTESIAN_POINT ( 'NONE',  ( -0.8333333333333323711, 0.2952755905511811885, 0.1292274648535926551 ) ) ;
#32330=CARTESIAN_POINT ( 'NONE',  ( 0.3937007874015754361, -0.1870078740157480601, -0.3641732283464567677 ) ) ;
#32331=CARTESIAN_POINT ( 'NONE',  ( -0.9842519685039360366, 0.2952755905511811885, 0.000000000000000000 ) ) ;
#32332=CARTESIAN_POINT ( 'NONE',  ( -0.9711286089238838626, 0.2306618581243847221, -0.2411417322834647770 ) ) ;
#32333=CARTESIAN_POINT ( 'NONE',  ( -1.377952755905511140, -0.5511811023622047445, 6.969142054262312111E-17 ) ) ;
#32334=CARTESIAN_POINT ( 'NONE',  ( 1.561679790026247350, 0.05413385826771626580, -0.4176697321401330321 ) ) ;
#32335=CARTESIAN_POINT ( 'NONE',  ( -0.6299212598425188991, -0.1870078740157480879, -0.4822834645669291653 ) ) ;
#32336=CARTESIAN_POINT ( 'NONE',  ( -0.9120734908136475250, -0.5511811023622048555, -0.09757992244046775898 ) ) ;
#32337=CARTESIAN_POINT ( 'NONE',  ( -1.568241469816272105, -0.08942795157527998196, 0.3641732283464567121 ) ) ;
#32338=CARTESIAN_POINT ( 'NONE',  ( 1.463254593175853824, 0.2952755905511810774, -0.1292274648535930714 ) ) ;
#32342=CONICAL_SURFACE ( 'NONE', #1488, 1.220472440944881942, 0.7853981633974621568 ) ;
#32344=CARTESIAN_POINT ( 'NONE',  ( -1.227034120734907585, 0.2952755905511811885, 0.1292274648535926551 ) ) ;
#32345=CARTESIAN_POINT ( 'NONE',  ( -0.9383202099737524282, -0.05778040916215522460, 0.4822834645669289988 ) ) ;
#32346=CARTESIAN_POINT ( 'NONE',  ( -1.587926509186350810, 0.05413385826771626580, -0.4176697321401330321 ) ) ;
#32348=CARTESIAN_POINT ( 'NONE',  ( 1.614173228346457378, -0.5511811023622047445, 6.969142054262312111E-17 ) ) ;
#32349=CARTESIAN_POINT ( 'NONE',  ( 0.6561679790026253567, -0.6046776061558809534, -0.2411417322834644161 ) ) ;
#32350=CARTESIAN_POINT ( 'NONE',  ( -0.1115485564304453947, -0.6692913385826771977, 0.1292274648535927661 ) ) ;
#32353=CARTESIAN_POINT ( 'NONE',  ( 0.8595800524934390507, -0.08942795157528024563, -0.3641732283464568787 ) ) ;
#32358=CARTESIAN_POINT ( 'NONE',  ( -0.006561679790025524116, -0.3162353388693405765, 0.4822834645669290543 ) ) ;
#32359=CARTESIAN_POINT ( 'NONE',  ( -1.509186351706035767, -0.4281496062992124485, 0.4176697321401328655 ) ) ;
#32360=CARTESIAN_POINT ( 'NONE',  ( 0.8398950131233602345, -0.6046776061558807314, 0.2411417322834647770 ) ) ;
#32361=CARTESIAN_POINT ( 'NONE',  ( -1.646981627296586703, -0.08942795157527998196, 0.3641732283464567121 ) ) ;
#32362=CARTESIAN_POINT ( 'NONE',  ( 1.384514435695538337, -0.6692913385826771977, 0.1292274648535927661 ) ) ;
#32363=CARTESIAN_POINT ( 'NONE',  ( -0.2887139107611542133, -0.6046776061558809534, -0.2411417322834644161 ) ) ;
#32364=CARTESIAN_POINT ( 'NONE',  ( 0.4199475065616803948, -0.6046776061558809534, -0.2411417322834644161 ) ) ;
#32365=CARTESIAN_POINT ( 'NONE',  ( 1.548556430446194954, -0.6046776061558807314, 0.2411417322834647770 ) ) ;
#32366=CARTESIAN_POINT ( 'NONE',  ( 1.515748031496063186, -0.5400638737290845981, -0.3530559997133363437 ) ) ;
#32367=CARTESIAN_POINT ( 'NONE',  ( -0.2887139107611542133, 0.2306618581243848609, 0.2411417322834645549 ) ) ;
#32369=CARTESIAN_POINT ( 'NONE',  ( 0.3018372703412079971, -0.004921259842519870586, -0.3153832671262229437 ) ) ;
#32373=CARTESIAN_POINT ( 'NONE',  ( -0.5380577427821514602, -0.3690944881889765550, -0.3153832671262227771 ) ) ;
#32375=CARTESIAN_POINT ( 'NONE',  ( 0.3477690288713918276, 0.2952755905511811885, 0.1292274648535926551 ) ) ;
#32376=CARTESIAN_POINT ( 'NONE',  ( -0.1640419947506555343, -0.3162353388693405765, 0.4822834645669290543 ) ) ;
#32377=CARTESIAN_POINT ( 'NONE',  ( -1.017060367454067249, -0.3162353388693409650, -0.4822834645669289433 ) ) ;
#32379=CARTESIAN_POINT ( 'NONE',  ( -1.246719160104985846, -0.4281496062992127816, -0.4176697321401328100 ) ) ;
#32381=CARTESIAN_POINT ( 'NONE',  ( 0.7677165354330716118, -0.4536011799217367080, 0.2665933059059888421 ) ) ;
#32382=CARTESIAN_POINT ( 'NONE',  ( 0.3608923884514443348, -0.6692913385826771977, 0.1292274648535927661 ) ) ;
#32383=CARTESIAN_POINT ( 'NONE',  ( 0.6430446194225729606, -0.4281496062992127816, -0.4176697321401328100 ) ) ;
#32386=CARTESIAN_POINT ( 'NONE',  ( 0.3273801728231982566, 0.000000000000000000, 0.3464511005275205946 ) ) ;
#32389=CARTESIAN_POINT ( 'NONE',  ( -0.1181102362204717315, 0.2952755905511811885, 0.000000000000000000 ) ) ;
#32392=CARTESIAN_POINT ( 'NONE',  ( -1.207349081364828436, -0.5023911411419708095, 0.1820866141732285504 ) ) ;
#32393=CARTESIAN_POINT ( 'NONE',  ( 1.351706036745407458, -0.4281496062992127816, -0.4176697321401328100 ) ) ;
#32394=CARTESIAN_POINT ( 'NONE',  ( 1.279527559055118724, -0.5400638737290845981, -0.3530559997133363437 ) ) ;
#32395=CARTESIAN_POINT ( 'NONE',  ( 0.3149606299212606708, -0.1870078740157480601, -0.3641732283464567677 ) ) ;
#32396=CARTESIAN_POINT ( 'NONE',  ( 0.3083989501312343062, -0.3162353388693405765, 0.4822834645669290543 ) ) ;
#32398=CARTESIAN_POINT ( 'NONE',  ( 0.4199475065616805614, 0.1283753931104748280, 0.1820866141732283561 ) ) ;
#32399=CARTESIAN_POINT ( 'NONE',  ( -0.08530183727034056085, -0.05778040916215560624, -0.4822834645669293319 ) ) ;
#32401=CARTESIAN_POINT ( 'NONE',  ( -1.082677165354329896, 0.1660481256975885056, 0.3530559997133364547 ) ) ;
#32402=CARTESIAN_POINT ( 'NONE',  ( 0.4199475065616803948, -0.5023911411419708095, -0.1820866141732282451 ) ) ;
#32403=VECTOR ( 'NONE', #73321, 39.37007874015748854 ) ;
#32404=CARTESIAN_POINT ( 'NONE',  ( 0.3608923884514443348, 0.2066929133858267098, -0.1054918080437494132 ) ) ;
#32405=CARTESIAN_POINT ( 'NONE',  ( -0.5446194225721777693, -0.3162353388693409650, -0.4822834645669289433 ) ) ;
#32406=CARTESIAN_POINT ( 'NONE',  ( -0.4724409448818890911, -0.1870078740157480601, -0.3641732283464567677 ) ) ;
#32408=CARTESIAN_POINT ( 'NONE',  ( -0.4921259842519677963, -0.5400638737290844871, 0.3530559997133364547 ) ) ;
#32409=CARTESIAN_POINT ( 'NONE',  ( -0.1115485564304453947, -0.6692913385826771977, 0.1292274648535927661 ) ) ;
#32410=CARTESIAN_POINT ( 'NONE',  ( 0.3149606299212603933, -0.1870078740157479769, 0.3641732283464567677 ) ) ;
#32412=CARTESIAN_POINT ( 'NONE',  ( -0.1246719160104980823, -0.6692913385826773087, -0.1292274648535924053 ) ) ;
#32415=CARTESIAN_POINT ( 'NONE',  ( 0.6758530183727039509, -0.5511811023622046335, 0.09757992244046803654 ) ) ;
#32416=CARTESIAN_POINT ( 'NONE',  ( 1.515748031496063186, -0.5400638737290845981, -0.3530559997133363437 ) ) ;
#32417=CARTESIAN_POINT ( 'NONE',  ( -0.7874015748031489847, -0.1870078740157479769, 0.3641732283464567677 ) ) ;
#32418=CARTESIAN_POINT ( 'NONE',  ( -0.7217847769028863381, -0.004921259842519870586, -0.3153832671262229437 ) ) ;
#32419=CARTESIAN_POINT ( 'NONE',  ( -0.8595800524934373854, -0.05778040916215522460, 0.4822834645669289988 ) ) ;
#32420=CARTESIAN_POINT ( 'NONE',  ( -0.1443569553805768291, 0.05413385826771666132, 0.4176697321401328100 ) ) ;
#32421=CARTESIAN_POINT ( 'NONE',  ( 0.4658792650918641698, -0.08942795157528024563, -0.3641732283464568787 ) ) ;
#32423=CARTESIAN_POINT ( 'NONE',  ( 1.128608923884514947, 0.1283753931104748280, 0.1820866141732283561 ) ) ;
#32424=CARTESIAN_POINT ( 'NONE',  ( 0.8005249343832028242, -0.4281496062992127816, -0.4176697321401328100 ) ) ;
#32425=CARTESIAN_POINT ( 'NONE',  ( 1.614173228346456712, 0.7166040191147866611, 0.1372047244094478646 ) ) ;
#32426=CARTESIAN_POINT ( 'NONE',  ( -0.1115485564304456306, 0.2952755905511810774, -0.1292274648535930714 ) ) ;
#32428=CARTESIAN_POINT ( 'NONE',  ( 1.371391076115485719, -0.5511811023622048555, -0.09757992244046775898 ) ) ;
#32429=CARTESIAN_POINT ( 'NONE',  ( 0.6167979002624679463, 0.05413385826771626580, -0.4176697321401330321 ) ) ;
#32430=CARTESIAN_POINT ( 'NONE',  ( 0.2296587926509192634, -0.3162353388693405765, 0.4822834645669290543 ) ) ;
#32432=CARTESIAN_POINT ( 'NONE',  ( 0.2362204724409456558, -0.1870078740157479769, 0.3641732283464567677 ) ) ;
#32433=CARTESIAN_POINT ( 'NONE',  ( 0.7742782152230979209, 0.05413385826771626580, -0.4176697321401330321 ) ) ;
#32434=CARTESIAN_POINT ( 'NONE',  ( -0.1246719160104980823, 0.1771653543307087630, 0.09757992244046791164 ) ) ;
#32435=CARTESIAN_POINT ( 'NONE',  ( -0.5643044619422565855, -0.4281496062992124485, 0.4176697321401328655 ) ) ;
#32437=CARTESIAN_POINT ( 'NONE',  ( -0.1574803149606292529, -0.1870078740157479769, 0.4822834645669291653 ) ) ;
#32438=CARTESIAN_POINT ( 'NONE',  ( -1.410761154855641575, -0.3162353388693409650, -0.4822834645669289433 ) ) ;
#32439=CARTESIAN_POINT ( 'NONE',  ( -0.6036745406824141069, 0.1283753931104748280, 0.1820866141732283561 ) ) ;
#32441=CARTESIAN_POINT ( 'NONE',  ( 0.2034120734908142214, 0.2952755905511810774, -0.1292274648535930714 ) ) ;
#32442=CARTESIAN_POINT ( 'NONE',  ( -1.338582677165353729, -0.1870078740157480879, -0.4822834645669291653 ) ) ;
#32443=CARTESIAN_POINT ( 'NONE',  ( -0.4790026246719152336, -0.05778040916215560624, -0.4822834645669293319 ) ) ;
#32446=CARTESIAN_POINT ( 'NONE',  ( 1.207349081364829990, -0.6046776061558809534, -0.2411417322834644161 ) ) ;
#32447=CARTESIAN_POINT ( 'NONE',  ( 1.345144356955381593, -0.05778040916215522460, 0.4822834645669289988 ) ) ;
#32449=CARTESIAN_POINT ( 'NONE',  ( -1.646981627296586703, -0.05778040916215522460, 0.4822834645669289988 ) ) ;
#32450=CARTESIAN_POINT ( 'NONE',  ( -1.200787401574802349, 0.1660481256975883668, -0.3530559997133364547 ) ) ;
#32453=ORIENTED_EDGE ( 'NONE', *, *, #63059, .F. ) ;
#32454=CARTESIAN_POINT ( 'NONE',  ( 0.006561679790026889343, -0.2845877964562161244, -0.3641732283464567121 ) ) ;
#32456=VERTEX_POINT ( 'NONE', #75990 ) ;
#32457=CARTESIAN_POINT ( 'NONE',  ( 0.1049868766404206816, -0.6046776061558809534, -0.2411417322834644161 ) ) ;
#32458=CARTESIAN_POINT ( 'NONE',  ( 0.6036745406824153282, -0.6046776061558807314, 0.2411417322834647770 ) ) ;
#32460=CARTESIAN_POINT ( 'NONE',  ( 1.614173228346457378, 0.7794589730112001513, -0.1372047244094476148 ) ) ;
#32461=CARTESIAN_POINT ( 'NONE',  ( -0.2690288713910754526, -0.5511811023622046335, 0.09757992244046803654 ) ) ;
#32463=CARTESIAN_POINT ( 'NONE',  ( 0.8661417322834653598, -0.1870078740157479769, 0.4822834645669291653 ) ) ;
#32464=CARTESIAN_POINT ( 'NONE',  ( 1.030183727034121421, -0.2845877964562161244, -0.3641732283464567121 ) ) ;
#32465=CARTESIAN_POINT ( 'NONE',  ( -0.6167979002624665030, -0.4281496062992127816, -0.4176697321401328100 ) ) ;
#32467=CARTESIAN_POINT ( 'NONE',  ( -0.8202099737532799750, 0.2952755905511810774, -0.1292274648535930714 ) ) ;
#32468=CARTESIAN_POINT ( 'NONE',  ( -1.220472440944881054, 0.1771653543307087630, 0.000000000000000000 ) ) ;
#32469=CARTESIAN_POINT ( 'NONE',  ( -1.017060367454067249, -0.3162353388693409650, -0.4822834645669289433 ) ) ;
#32470=CARTESIAN_POINT ( 'NONE',  ( 1.194225721784777594, 0.05413385826771666132, 0.4176697321401328100 ) ) ;
#32474=CARTESIAN_POINT ( 'NONE',  ( 0.1640419947506569498, -0.3162353388693409650, -0.4822834645669289433 ) ) ;
#32475=VERTEX_POINT ( 'NONE', #63344 ) ;
#32476=CARTESIAN_POINT ( 'NONE',  ( -0.9251968503937002541, 0.1660481256975885056, 0.3530559997133364547 ) ) ;
#32477=CARTESIAN_POINT ( 'NONE',  ( 1.259842519685040019, -0.1870078740157479769, 0.4822834645669291653 ) ) ;
#32478=CARTESIAN_POINT ( 'NONE',  ( 1.220472440944882386, -0.6692913385826771977, 8.415575281601705876E-17 ) ) ;
#32479=CARTESIAN_POINT ( 'NONE',  ( 0.07217847769028949700, -0.05778040916215560624, -0.4822834645669293319 ) ) ;
#32480=CARTESIAN_POINT ( 'NONE',  ( 0.1181102362204730916, 0.2952755905511811885, 0.000000000000000000 ) ) ;
#32482=CARTESIAN_POINT ( 'NONE',  ( -1.187664041994750175, -0.05778040916215560624, -0.4822834645669293319 ) ) ;
#32483=CARTESIAN_POINT ( 'NONE',  ( -0.3149606299212590610, -0.1870078740157480879, -0.4822834645669291653 ) ) ;
#32484=CARTESIAN_POINT ( 'NONE',  ( -0.2362204724409440182, -0.1870078740157479769, 0.3641732283464567677 ) ) ;
#32486=CARTESIAN_POINT ( 'NONE',  ( 1.476377952755906442, -0.5400638737290844871, 0.3530559997133364547 ) ) ;
#32487=CARTESIAN_POINT ( 'NONE',  ( -0.4265091863517051496, 0.2952755905511810774, -0.1292274648535930714 ) ) ;
#32489=CARTESIAN_POINT ( 'NONE',  ( 1.069553805774278610, -0.6692913385826771977, 0.1292274648535927661 ) ) ;
#32490=CARTESIAN_POINT ( 'NONE',  ( 0.5380577427821529035, 0.009842519685039144428, -0.3409548833797004797 ) ) ;
#32493=CARTESIAN_POINT ( 'NONE',  ( 0.4133858267716541968, 0.1660481256975885056, 0.3530559997133364547 ) ) ;
#32494=CARTESIAN_POINT ( 'NONE',  ( -0.3215223097112853146, -0.2845877964562159024, 0.3641732283464567677 ) ) ;
#32495=CARTESIAN_POINT ( 'NONE',  ( 1.601049868766404982, -0.5023911411419708095, -0.1820866141732282451 ) ) ;
#32496=CARTESIAN_POINT ( 'NONE',  ( -1.220472440944881054, 0.2952755905511811885, 0.000000000000000000 ) ) ;
#32498=CARTESIAN_POINT ( 'NONE',  ( 1.673228346456693494, 0.07958543189024085140, 0.2665933059059887866 ) ) ;
#32499=CARTESIAN_POINT ( 'NONE',  ( 1.568241469816273437, -0.3162353388693405765, 0.4822834645669290543 ) ) ;
#32502=CARTESIAN_POINT ( 'NONE',  ( -0.1574803149606292529, -0.1870078740157479769, 0.4822834645669291653 ) ) ;
#32504=CARTESIAN_POINT ( 'NONE',  ( -1.594488188976377563, -0.5400638737290844871, 0.3530559997133364547 ) ) ;
#32505=CARTESIAN_POINT ( 'NONE',  ( 0.2952755905511816326, -0.5400638737290844871, 0.3530559997133364547 ) ) ;
#32507=CARTESIAN_POINT ( 'NONE',  ( -1.627296587926508442, 0.1283753931104748280, 0.1820866141732283561 ) ) ;
#32508=CARTESIAN_POINT ( 'NONE',  ( 0.8136482939632553313, 0.2306618581243848609, 0.2411417322834645549 ) ) ;
#32510=CARTESIAN_POINT ( 'NONE',  ( 1.062992125984252745, 0.1771653543307087630, 0.000000000000000000 ) ) ;
#32512=CARTESIAN_POINT ( 'NONE',  ( 1.017060367454068803, -0.2845877964562159024, 0.3641732283464567677 ) ) ;
#32513=CARTESIAN_POINT ( 'NONE',  ( -1.476377952755905110, 0.1660481256975885056, 0.3530559997133364547 ) ) ;
#32515=CARTESIAN_POINT ( 'NONE',  ( 0.9711286089238851948, -0.6046776061558809534, -0.2411417322834644161 ) ) ;
#32517=CARTESIAN_POINT ( 'NONE',  ( 0.6627296587926517768, -0.6692913385826773087, -0.1292274648535924053 ) ) ;
#32519=CARTESIAN_POINT ( 'NONE',  ( -1.581364829396324945, -0.2845877964562159024, 0.3641732283464567677 ) ) ;
#32520=CARTESIAN_POINT ( 'NONE',  ( 0.5774278215223103139, -0.5023911411419708095, -0.1820866141732282451 ) ) ;
#32521=CARTESIAN_POINT ( 'NONE',  ( 0.5052493438320218022, -0.6692913385826773087, -0.1292274648535924053 ) ) ;
#32523=CARTESIAN_POINT ( 'NONE',  ( -0.8792650918635160906, -0.004921259842519870586, -0.3153832671262229437 ) ) ;
#32524=CARTESIAN_POINT ( 'NONE',  ( -1.194225721784776262, 0.05413385826771626580, -0.4176697321401330321 ) ) ;
#32525=CARTESIAN_POINT ( 'NONE',  ( 1.522309711286089939, 0.2306618581243848609, 0.2411417322834645549 ) ) ;
#32526=CARTESIAN_POINT ( 'NONE',  ( -1.272965879265091305, -0.4281496062992124485, 0.4176697321401328655 ) ) ;
#32527=CARTESIAN_POINT ( 'NONE',  ( 0.7874015748031503170, -0.1870078740157480879, -0.4822834645669291653 ) ) ;
#32528=CARTESIAN_POINT ( 'NONE',  ( -1.253280839895012377, -0.2845877964562161244, -0.3641732283464567121 ) ) ;
#32530=CARTESIAN_POINT ( 'NONE',  ( 1.154855643044620184, 0.2306618581243847221, -0.2411417322834647770 ) ) ;
#32532=CARTESIAN_POINT ( 'NONE',  ( -1.430446194225721390, -0.4281496062992124485, 0.4176697321401328655 ) ) ;
#32533=CARTESIAN_POINT ( 'NONE',  ( 1.220472440944882608, 0.2952755905511811885, 0.000000000000000000 ) ) ;
#32534=CARTESIAN_POINT ( 'NONE',  ( -0.8727034120734901146, -0.08942795157528024563, -0.3641732283464568787 ) ) ;
#32535=CARTESIAN_POINT ( 'NONE',  ( 1.482939632545932307, -0.3690944881889763329, 0.3153832671262228327 ) ) ;
#32536=CARTESIAN_POINT ( 'NONE',  ( -1.207349081364828436, -0.5023911411419708095, 0.1820866141732285504 ) ) ;
#32537=CARTESIAN_POINT ( 'NONE',  ( -0.4986876640419939388, 0.1283753931104746893, -0.1820866141732285504 ) ) ;
#32538=CARTESIAN_POINT ( 'NONE',  ( -1.469816272965878357, -0.5023911411419708095, -0.1820866141732282451 ) ) ;
#32539=CARTESIAN_POINT ( 'NONE',  ( 0.8464566929133865436, 0.07958543189024071263, -0.2665933059059888421 ) ) ;
#32540=CARTESIAN_POINT ( 'NONE',  ( 0.3412073490813655186, -0.6046776061558809534, -0.2411417322834644161 ) ) ;
#32541=DIRECTION ( 'NONE',  ( 0.000000000000000000, 0.000000000000000000, -1.000000000000000000 ) ) ;
#32542=CARTESIAN_POINT ( 'NONE',  ( -0.1443569553805765515, -0.4281496062992127816, -0.4176697321401328100 ) ) ;
#32543=EDGE_CURVE ( 'NONE', #76877, #72166, #55997, .T. ) ;
#32544=CARTESIAN_POINT ( 'NONE',  ( 0.5839895013123367340, -0.5511811023622048555, -0.09757992244046775898 ) ) ;
#32545=CARTESIAN_POINT ( 'NONE',  ( -1.620734908136482577, 0.2952755905511811885, 0.1292274648535926551 ) ) ;
#32547=CARTESIAN_POINT ( 'NONE',  ( -1.384514435695537005, -0.6692913385826773087, -0.1292274648535924053 ) ) ;
#32548=CARTESIAN_POINT ( 'NONE',  ( -0.3477690288713905509, -0.6692913385826771977, 0.1292274648535927661 ) ) ;
#32551=CARTESIAN_POINT ( 'NONE',  ( -0.08530183727034056085, -0.05778040916215560624, -0.4822834645669293319 ) ) ;
#32552=CARTESIAN_POINT ( 'NONE',  ( 1.082677165354331228, -0.4536011799217367080, 0.2665933059059888421 ) ) ;
#32553=CARTESIAN_POINT ( 'NONE',  ( -0.3149606299212590610, -0.1870078740157480879, -0.4822834645669291653 ) ) ;
#32554=CARTESIAN_POINT ( 'NONE',  ( 0.2099737532808405305, 0.2306618581243847221, -0.2411417322834647770 ) ) ;
#32560=CARTESIAN_POINT ( 'NONE',  ( -1.154855643044618851, -0.5023911411419708095, -0.1820866141732282451 ) ) ;
#32562=CARTESIAN_POINT ( 'NONE',  ( -0.9580052493438311334, -0.4281496062992124485, 0.4176697321401328655 ) ) ;
#32565=CARTESIAN_POINT ( 'NONE',  ( 0.5380577427821529035, -0.4281496062992124485, 0.4176697321401328655 ) ) ;
#32567=CARTESIAN_POINT ( 'NONE',  ( 1.213910761154856299, -0.6692913385826773087, -0.1292274648535924053 ) ) ;
#32568=CARTESIAN_POINT ( 'NONE',  ( 0.5774278215223103139, -0.6046776061558809534, -0.2411417322834644161 ) ) ;
#32572=CARTESIAN_POINT ( 'NONE',  ( 1.154855643044620184, -0.6046776061558807314, 0.2411417322834647770 ) ) ;
#32573=CARTESIAN_POINT ( 'NONE',  ( 0.3740157480314966754, 0.1660481256975883668, -0.3530559997133364547 ) ) ;
#32574=CARTESIAN_POINT ( 'NONE',  ( 0.09186351706036799403, -0.4281496062992127816, -0.4176697321401328100 ) ) ;
#32575=CARTESIAN_POINT ( 'NONE',  ( 0.6233595800524939223, -0.2845877964562159024, 0.3641732283464567677 ) ) ;
#32576=CARTESIAN_POINT ( 'NONE',  ( 1.141732283464567788, -0.6692913385826771977, 8.415575281601705876E-17 ) ) ;
#32579=CARTESIAN_POINT ( 'NONE',  ( -0.07874015748031421014, -0.1870078740157480879, -0.4822834645669291653 ) ) ;
#32580=CARTESIAN_POINT ( 'NONE',  ( 0.8792650918635177559, 0.05413385826771666132, 0.4176697321401328100 ) ) ;
#32581=CARTESIAN_POINT ( 'NONE',  ( 0.4724409448818904789, -0.1870078740157480879, -0.4822834645669291653 ) ) ;
#32582=CARTESIAN_POINT ( 'NONE',  ( 1.266404199475066328, -0.2845877964562161244, -0.3641732283464567121 ) ) ;
#32583=CARTESIAN_POINT ( 'NONE',  ( -0.8202099737532801971, -0.6692913385826771977, 0.1292274648535927661 ) ) ;
#32584=CARTESIAN_POINT ( 'NONE',  ( -0.8333333333333323711, -0.6692913385826773087, -0.1292274648535924053 ) ) ;
#32585=CARTESIAN_POINT ( 'NONE',  ( 1.148293963254593653, 0.2952755905511810774, -0.1292274648535930714 ) ) ;
#32592=CARTESIAN_POINT ( 'NONE',  ( 1.587926509186352586, -0.4281496062992127816, -0.4176697321401328100 ) ) ;
#32593=CARTESIAN_POINT ( 'NONE',  ( 0.9448818897637802916, -0.1870078740157479769, 0.3641732283464567677 ) ) ;
#32595=DIRECTION ( 'NONE',  ( 1.000000000000000000, -0.000000000000000000, -0.000000000000000000 ) ) ;
#32599=CARTESIAN_POINT ( 'NONE',  ( -1.233595800524933894, -0.5023911411419708095, -0.1820866141732282451 ) ) ;
#32600=CARTESIAN_POINT ( 'NONE',  ( -1.515748031496062076, 0.07958543189024071263, -0.2665933059059888421 ) ) ;
#32601=CARTESIAN_POINT ( 'NONE',  ( -1.253280839895012377, -0.3162353388693409650, -0.4822834645669289433 ) ) ;
#32602=CARTESIAN_POINT ( 'NONE',  ( -0.4265091863517051496, 0.2952755905511810774, -0.1292274648535930714 ) ) ;
#32603=CARTESIAN_POINT ( 'NONE',  ( -1.646981627296586703, -0.05778040916215522460, 0.4822834645669289988 ) ) ;
#32609=CARTESIAN_POINT ( 'NONE',  ( -1.614173228346457378, 1.543375672658094944, 0.1372047244094476981 ) ) ;
#32610=CARTESIAN_POINT ( 'NONE',  ( -0.9186351706036736120, -0.5023911411419708095, -0.1820866141732282451 ) ) ;
#32611=CARTESIAN_POINT ( 'NONE',  ( 0.9186351706036752773, 0.1539470093639521697, -0.1968503937007875793 ) ) ;
#32612=CARTESIAN_POINT ( 'NONE',  ( 0.5446194225721792126, -0.3162353388693405765, 0.4822834645669290543 ) ) ;
#32613=ORIENTED_EDGE ( 'NONE', *, *, #54463, .T. ) ;
#32616=CARTESIAN_POINT ( 'NONE',  ( 1.279527559055118724, -0.5400638737290845981, -0.3530559997133363437 ) ) ;
#32617=CARTESIAN_POINT ( 'NONE',  ( -1.561679790026246017, 0.05413385826771666132, 0.4176697321401328100 ) ) ;
#32619=CARTESIAN_POINT ( 'NONE',  ( -0.4396325459317579898, 0.1771653543307087630, 0.09757992244046791164 ) ) ;
#32620=CARTESIAN_POINT ( 'NONE',  ( -1.627296587926508442, 0.1283753931104748280, 0.1820866141732283561 ) ) ;
#32622=CARTESIAN_POINT ( 'NONE',  ( -0.3805774278215216522, -0.004921259842519576551, 0.3153832671262227771 ) ) ;
#32623=CARTESIAN_POINT ( 'NONE',  ( 0.1968503937007881344, 0.1771653543307087630, 0.000000000000000000 ) ) ;
#32624=CARTESIAN_POINT ( 'NONE',  ( -0.07874015748031421014, -0.1870078740157480879, -0.4822834645669291653 ) ) ;
#32625=CARTESIAN_POINT ( 'NONE',  ( -1.148293963254592542, 0.1771653543307087630, 0.09757992244046791164 ) ) ;
#32627=CARTESIAN_POINT ( 'NONE',  ( 1.187664041994751285, -0.3162353388693409650, -0.4822834645669289433 ) ) ;
#32629=CARTESIAN_POINT ( 'NONE',  ( -1.515748031496062076, -0.5400638737290844871, 0.3530559997133364547 ) ) ;
#32631=CARTESIAN_POINT ( 'NONE',  ( -0.3412073490813641308, -0.6046776061558807314, 0.2411417322834647770 ) ) ;
#32632=CARTESIAN_POINT ( 'NONE',  ( 0.2230971128608929543, -0.004921259842519870586, -0.3153832671262229437 ) ) ;
#32633=CARTESIAN_POINT ( 'NONE',  ( -0.7939632545931750718, -0.05778040916215560624, -0.4822834645669293319 ) ) ;
#32634=CARTESIAN_POINT ( 'NONE',  ( 0.8202099737532814183, -0.5511811023622048555, -0.09757992244046775898 ) ) ;
#32635=CARTESIAN_POINT ( 'NONE',  ( -0.4461942257217840213, 0.1283753931104748280, 0.1820866141732283561 ) ) ;
#32636=CARTESIAN_POINT ( 'NONE',  ( -0.8333333333333323711, -0.6692913385826773087, -0.1292274648535924053 ) ) ;
#32637=CARTESIAN_POINT ( 'NONE',  ( -1.496062992125983815, -0.1870078740157479769, 0.4822834645669291653 ) ) ;
#32638=DIRECTION ( 'NONE',  ( -0.7119855458575206075, 0.7021941202331221099, 0.000000000000000000 ) ) ;
#32639=CARTESIAN_POINT ( 'NONE',  ( 1.351706036745407680, -0.004921259842519576551, 0.3153832671262227771 ) ) ;
#32640=CARTESIAN_POINT ( 'NONE',  ( -1.528871391076114250, -0.6692913385826771977, 0.1292274648535927661 ) ) ;
#32641=CARTESIAN_POINT ( 'NONE',  ( -1.640419947506561060, -0.4281496062992127816, -0.4176697321401328100 ) ) ;
#32644=CARTESIAN_POINT ( 'NONE',  ( -0.7152230971128602510, -0.2845877964562159024, 0.3641732283464567677 ) ) ;
#32645=CARTESIAN_POINT ( 'NONE',  ( 0.7283464566929140904, -0.5400638737290845981, -0.3530559997133363437 ) ) ;
#32646=CARTESIAN_POINT ( 'NONE',  ( -0.9251968503937002541, 0.07958543189024085140, 0.2665933059059887866 ) ) ;
#32648=CARTESIAN_POINT ( 'NONE',  ( -1.167979002624671470, -0.4281496062992127816, -0.4176697321401328100 ) ) ;
#32649=CARTESIAN_POINT ( 'NONE',  ( 0.6561679790026253567, -0.6046776061558809534, -0.2411417322834644161 ) ) ;
#32650=CARTESIAN_POINT ( 'NONE',  ( 0.3805774278215230400, -0.4281496062992124485, 0.4176697321401328655 ) ) ;
#32651=CARTESIAN_POINT ( 'NONE',  ( 1.614173228346457378, 0.2952755905511811885, 0.000000000000000000 ) ) ;
#32652=CARTESIAN_POINT ( 'NONE',  ( -1.660104986876639543, -0.08942795157528024563, -0.3641732283464568787 ) ) ;
#32657=CARTESIAN_POINT ( 'NONE',  ( 0.8858267716535438430, 0.07958543189024085140, 0.2665933059059887866 ) ) ;
#32658=CARTESIAN_POINT ( 'NONE',  ( 0.4790026246719167324, -0.08942795157527998196, 0.3641732283464567121 ) ) ;
#32659=CARTESIAN_POINT ( 'NONE',  ( -0.03937007874015669567, -0.6692913385826771977, 8.415575281601705876E-17 ) ) ;
#32660=CARTESIAN_POINT ( 'NONE',  ( 1.351706036745407458, -0.4281496062992127816, -0.4176697321401328100 ) ) ;
#32662=CARTESIAN_POINT ( 'NONE',  ( 0.4855643044619430415, -0.3690944881889765550, -0.3153832671262227771 ) ) ;
#32663=CARTESIAN_POINT ( 'NONE',  ( -0.7480314960629914633, -0.6692913385826771977, 8.415575281601705876E-17 ) ) ;
#32664=CARTESIAN_POINT ( 'NONE',  ( -1.135170603674539924, 0.2952755905511810774, -0.1292274648535930714 ) ) ;
#32665=CARTESIAN_POINT ( 'NONE',  ( 0.9055118110236227702, 0.2952755905511811885, 0.000000000000000000 ) ) ;
#32668=ORIENTED_EDGE ( 'NONE', *, *, #73267, .F. ) ;
#32671=CARTESIAN_POINT ( 'NONE',  ( -1.345144356955379816, -0.05778040916215560624, -0.4822834645669293319 ) ) ;
#32672=CARTESIAN_POINT ( 'NONE',  ( -0.5511811023622038563, -0.1870078740157479769, 0.4822834645669291653 ) ) ;
#32673=CARTESIAN_POINT ( 'NONE',  ( -0.9055118110236215490, -0.5511811023622047445, 6.969142054262312111E-17 ) ) ;
#32674=CARTESIAN_POINT ( 'NONE',  ( -0.8267716535433065062, 0.2952755905511811885, 0.000000000000000000 ) ) ;
#32677=CARTESIAN_POINT ( 'NONE',  ( -1.509186351706035767, -0.3690944881889763329, 0.3153832671262228327 ) ) ;
#32678=CARTESIAN_POINT ( 'NONE',  ( -1.036745406824146176, 0.05413385826771626580, -0.4176697321401330321 ) ) ;
#32679=CARTESIAN_POINT ( 'NONE',  ( 0.3871391076115492380, -0.05778040916215560624, -0.4822834645669293319 ) ) ;
#32680=CARTESIAN_POINT ( 'NONE',  ( -0.7808398950131222316, -0.3162353388693409650, -0.4822834645669289433 ) ) ;
#32681=CARTESIAN_POINT ( 'NONE',  ( 0.6496062992125991586, 0.1660481256975885056, 0.3530559997133364547 ) ) ;
#32683=CARTESIAN_POINT ( 'NONE',  ( -1.030183727034119867, -0.2845877964562159024, 0.3641732283464567677 ) ) ;
#32684=EDGE_LOOP ( 'NONE', ( #62214, #76697, #72568, #37421 ) ) ;
#32688=CARTESIAN_POINT ( 'NONE',  ( -1.253280839895012377, -0.05778040916215522460, 0.4822834645669289988 ) ) ;
#32689=CARTESIAN_POINT ( 'NONE',  ( -1.286089238845143479, 0.2306618581243847221, -0.2411417322834647770 ) ) ;
#32691=CARTESIAN_POINT ( 'NONE',  ( -1.259842519685038686, -0.1870078740157479769, 0.4822834645669291653 ) ) ;
#32692=CARTESIAN_POINT ( 'NONE',  ( -1.194225721784776262, 0.05413385826771626580, -0.4176697321401330321 ) ) ;
#32693=CARTESIAN_POINT ( 'NONE',  ( -1.371391076115484609, -0.6692913385826771977, 0.1292274648535927661 ) ) ;
#32697=CARTESIAN_POINT ( 'NONE',  ( 0.07217847769028949700, -0.2845877964562159024, 0.3641732283464567677 ) ) ;
#32700=CARTESIAN_POINT ( 'NONE',  ( -0.3937007874015740483, -0.1870078740157480601, -0.3641732283464567677 ) ) ;
#32701=CARTESIAN_POINT ( 'NONE',  ( -0.9186351706036736120, -0.6046776061558809534, -0.2411417322834644161 ) ) ;
#32703=CARTESIAN_POINT ( 'NONE',  ( 1.213910761154856299, -0.6692913385826773087, -0.1292274648535924053 ) ) ;
#32704=CARTESIAN_POINT ( 'NONE',  ( -0.6955380577427815458, 0.05413385826771666132, 0.4176697321401328100 ) ) ;
#32705=ORIENTED_EDGE ( 'NONE', *, *, #48920, .F. ) ;
#32708=CARTESIAN_POINT ( 'NONE',  ( -0.9776902887139098386, 0.2952755905511810774, -0.1292274648535930714 ) ) ;
#32709=CARTESIAN_POINT ( 'NONE',  ( 1.364829396325459854, -0.6046776061558809534, -0.2411417322834644161 ) ) ;
#32710=CARTESIAN_POINT ( 'NONE',  ( -1.568241469816272105, -0.08942795157527998196, 0.3641732283464567121 ) ) ;
#32711=CARTESIAN_POINT ( 'NONE',  ( -1.345144356955379816, -0.05778040916215560624, -0.4822834645669293319 ) ) ;
#32716=CARTESIAN_POINT ( 'NONE',  ( 0.2165354330708668673, -0.5400638737290844871, 0.3530559997133364547 ) ) ;
#32717=CARTESIAN_POINT ( 'NONE',  ( -1.299212598425196097, 0.1771653543307087630, 0.000000000000000000 ) ) ;
#32718=CARTESIAN_POINT ( 'NONE',  ( -0.8661417322834640276, -0.1870078740157480879, -0.4822834645669291653 ) ) ;
#32720=CARTESIAN_POINT ( 'NONE',  ( -1.443569553805773564, -0.6046776061558807314, 0.2411417322834647770 ) ) ;
#32722=CARTESIAN_POINT ( 'NONE',  ( -0.9186351706036736120, 0.2306618581243848609, 0.2411417322834645549 ) ) ;
#32723=CARTESIAN_POINT ( 'NONE',  ( -0.5314960629921254842, -0.5400638737290845981, -0.3530559997133363437 ) ) ;
#32725=CARTESIAN_POINT ( 'NONE',  ( 1.069553805774278610, -0.5511811023622046335, 0.09757992244046803654 ) ) ;
#32728=CARTESIAN_POINT ( 'NONE',  ( 0.6364829396325465405, -0.2845877964562161244, -0.3641732283464567121 ) ) ;
#32729=CARTESIAN_POINT ( 'NONE',  ( 1.404199475065617264, -0.3690944881889763329, 0.3153832671262228327 ) ) ;
#32730=CARTESIAN_POINT ( 'NONE',  ( 1.450131233595801428, 0.2952755905511811885, 0.1292274648535926551 ) ) ;
#32731=CARTESIAN_POINT ( 'NONE',  ( 0.2362204724409456558, -0.1870078740157479769, 0.3641732283464567677 ) ) ;
#32733=CARTESIAN_POINT ( 'NONE',  ( -0.8792650918635160906, -0.4281496062992124485, 0.4176697321401328655 ) ) ;
#32734=CARTESIAN_POINT ( 'NONE',  ( 1.174540682414699111, -0.05778040916215560624, -0.4822834645669293319 ) ) ;
#32736=CARTESIAN_POINT ( 'NONE',  ( -0.3543307086614165824, 0.1771653543307087630, 0.000000000000000000 ) ) ;
#32738=CARTESIAN_POINT ( 'NONE',  ( 0.2099737532808405305, -0.6046776061558807314, 0.2411417322834647770 ) ) ;
#32740=CIRCLE ( 'NONE', #71742, 3.543307086614173151 ) ;
#32741=CARTESIAN_POINT ( 'NONE',  ( 1.089238845144357537, -0.3690944881889763329, 0.3153832671262228327 ) ) ;
#32742=CARTESIAN_POINT ( 'NONE',  ( -0.01968503937007793844, -0.4536011799217367080, 0.2665933059059888421 ) ) ;
#32743=CARTESIAN_POINT ( 'NONE',  ( -0.2493438320209966919, -0.4281496062992124485, 0.4176697321401328655 ) ) ;
#32744=CARTESIAN_POINT ( 'NONE',  ( -1.286089238845143479, -0.6046776061558807314, 0.2411417322834647770 ) ) ;
#32745=CARTESIAN_POINT ( 'NONE',  ( -0.7545931758530176614, -0.5511811023622048555, -0.09757992244046775898 ) ) ;
#32747=CARTESIAN_POINT ( 'NONE',  ( 0.7086614173228353852, -0.1870078740157479769, 0.4822834645669291653 ) ) ;
#32748=CARTESIAN_POINT ( 'NONE',  ( -0.9120734908136475250, -0.6692913385826773087, -0.1292274648535924053 ) ) ;
#32751=CARTESIAN_POINT ( 'NONE',  ( 0.3018372703412079971, -0.3690944881889763329, 0.3153832671262228327 ) ) ;
#32752=CARTESIAN_POINT ( 'NONE',  ( -0.5905511811023613777, -0.6692913385826771977, 8.415575281601705876E-17 ) ) ;
#32753=CARTESIAN_POINT ( 'NONE',  ( -1.194225721784776262, -0.4281496062992124485, 0.4176697321401328655 ) ) ;
#32754=CARTESIAN_POINT ( 'NONE',  ( -1.423884514435694859, -0.08942795157528024563, -0.3641732283464568787 ) ) ;
#32756=CARTESIAN_POINT ( 'NONE',  ( -0.8595800524934373854, -0.08942795157527998196, 0.3641732283464567121 ) ) ;
#32757=CARTESIAN_POINT ( 'NONE',  ( -1.509186351706035767, -0.004921259842519870586, -0.3153832671262229437 ) ) ;
#32758=CARTESIAN_POINT ( 'NONE',  ( 1.115485564304462551, 0.05413385826771666132, 0.4176697321401328100 ) ) ;
#32763=CARTESIAN_POINT ( 'NONE',  ( 1.594488188976378673, 0.07958543189024085140, 0.2665933059059887866 ) ) ;
#32764=CARTESIAN_POINT ( 'NONE',  ( -1.482939632545930975, -0.4281496062992127816, -0.4176697321401328100 ) ) ;
#32765=CARTESIAN_POINT ( 'NONE',  ( 1.259842519685040019, -0.1870078740157479769, 0.4822834645669291653 ) ) ;
#32768=CARTESIAN_POINT ( 'NONE',  ( 0.7217847769028878924, 0.05413385826771666132, 0.4176697321401328100 ) ) ;
#32769=CARTESIAN_POINT ( 'NONE',  ( 0.01312335958005323398, -0.4281496062992127816, -0.4176697321401328100 ) ) ;
#32770=CARTESIAN_POINT ( 'NONE',  ( -0.6971652711706680661, 5.991678263669262536E-15, 0.3791483426435162674 ) ) ;
#32771=CARTESIAN_POINT ( 'NONE',  ( -0.6824146981627288167, 0.2306618581243848609, 0.2411417322834645549 ) ) ;
#32772=CARTESIAN_POINT ( 'NONE',  ( 0.8202099737532813073, 0.1771653543307087630, 0.09757992244046791164 ) ) ;
#32774=ORIENTED_EDGE ( 'NONE', *, *, #82598, .T. ) ;
#32776=ORIENTED_EDGE ( 'NONE', *, *, #2252, .T. ) ;
#32777=CARTESIAN_POINT ( 'NONE',  ( -0.2230971128608915943, -0.4281496062992127816, -0.4176697321401328100 ) ) ;
#32778=CARTESIAN_POINT ( 'NONE',  ( 1.587926509186352142, 0.05413385826771666132, 0.4176697321401328100 ) ) ;
#32779=CARTESIAN_POINT ( 'NONE',  ( 0.6036745406824154392, 0.2306618581243847221, -0.2411417322834647770 ) ) ;
#32781=CARTESIAN_POINT ( 'NONE',  ( 1.259842519685040019, -0.1870078740157480879, -0.4822834645669291653 ) ) ;
#32782=CARTESIAN_POINT ( 'NONE',  ( 1.601049868766404982, 0.2306618581243848609, 0.2411417322834645549 ) ) ;
#32783=CARTESIAN_POINT ( 'NONE',  ( -0.4593175853018364174, -0.4281496062992127816, -0.4176697321401328100 ) ) ;
#32784=CARTESIAN_POINT ( 'NONE',  ( 0.1902887139107617975, 0.2952755905511811885, 0.1292274648535926551 ) ) ;
#32785=CARTESIAN_POINT ( 'NONE',  ( -1.620734908136482577, 0.2952755905511811885, 0.1292274648535926551 ) ) ;
#32786=CARTESIAN_POINT ( 'NONE',  ( 1.371391076115485719, -0.6692913385826773087, -0.1292274648535924053 ) ) ;
#32787=CARTESIAN_POINT ( 'NONE',  ( 1.266404199475066328, -0.3162353388693409650, -0.4822834645669289433 ) ) ;
#32788=CARTESIAN_POINT ( 'NONE',  ( -0.2230971128608915943, -0.4281496062992127816, -0.4176697321401328100 ) ) ;
#32790=CARTESIAN_POINT ( 'NONE',  ( 0.3608923884514443348, -0.5511811023622046335, 0.09757992244046803654 ) ) ;
#32791=VERTEX_POINT ( 'NONE', #77646 ) ;
#32794=CARTESIAN_POINT ( 'NONE',  ( -0.2362204724409442680, -0.1870078740157480601, -0.3641732283464567677 ) ) ;
#32795=CARTESIAN_POINT ( 'NONE',  ( 0.03937007874015833325, -0.6692913385826771977, 8.415575281601705876E-17 ) ) ;
#32797=CARTESIAN_POINT ( 'NONE',  ( 0.03280839895013198948, 0.2952755905511811885, 0.1292274648535926551 ) ) ;
#32798=CARTESIAN_POINT ( 'NONE',  ( -0.01968503937007793844, -0.5400638737290844871, 0.3530559997133364547 ) ) ;
#32799=EDGE_CURVE ( 'NONE', #57471, #50964, #37851, .T. ) ;
#32800=CARTESIAN_POINT ( 'NONE',  ( -1.089238845144356427, 0.05413385826771666132, 0.4176697321401328100 ) ) ;
#32802=CARTESIAN_POINT ( 'NONE',  ( 1.469816272965879911, -0.5023911411419708095, 0.1820866141732285504 ) ) ;
#32803=CARTESIAN_POINT ( 'NONE',  ( -1.482939632545930975, 0.05413385826771666132, 0.4176697321401328100 ) ) ;
#32805=CARTESIAN_POINT ( 'NONE',  ( 0.7349081364829402885, -0.5023911411419708095, -0.1820866141732282451 ) ) ;
#32806=CARTESIAN_POINT ( 'NONE',  ( 0.5839895013123367340, 0.2952755905511811885, 0.1292274648535926551 ) ) ;
#32807=CARTESIAN_POINT ( 'NONE',  ( 0.7677165354330716118, 0.1660481256975883668, -0.3530559997133364547 ) ) ;
#32809=CARTESIAN_POINT ( 'NONE',  ( -1.666666666666665853, 0.05413385826771626580, -0.4176697321401330321 ) ) ;
#32812=CARTESIAN_POINT ( 'NONE',  ( 0.05249343832021075018, 0.2306618581243847221, -0.2411417322834647770 ) ) ;
#32815=CARTESIAN_POINT ( 'NONE',  ( -1.082677165354329896, -0.4536011799217368745, -0.2665933059059886201 ) ) ;
#32816=CARTESIAN_POINT ( 'NONE',  ( 1.443569553805774897, 0.2306618581243848609, 0.2411417322834645549 ) ) ;
#32817=CARTESIAN_POINT ( 'NONE',  ( 1.220472440944882608, 0.2952755905511811885, 0.000000000000000000 ) ) ;
#32818=CARTESIAN_POINT ( 'NONE',  ( -0.4133858267716528645, -0.4536011799217367080, 0.2665933059059888421 ) ) ;
#32819=CARTESIAN_POINT ( 'NONE',  ( 0.3215223097112867578, -0.05778040916215522460, 0.4822834645669289988 ) ) ;
#32821=CARTESIAN_POINT ( 'NONE',  ( 0.2755905511811031494, 0.1771653543307087630, 0.000000000000000000 ) ) ;
#32822=CARTESIAN_POINT ( 'NONE',  ( -0.03280839895013062252, -0.6692913385826771977, 0.1292274648535927661 ) ) ;
#32824=CARTESIAN_POINT ( 'NONE',  ( -1.227034120734907585, 0.2952755905511811885, 0.1292274648535926551 ) ) ;
#32825=CARTESIAN_POINT ( 'NONE',  ( 0.3740157480314966754, 0.07958543189024071263, -0.2665933059059888421 ) ) ;
#32826=CARTESIAN_POINT ( 'NONE',  ( 0.3809280630633196107, 0.004960608223778500969, -0.3437734562760191848 ) ) ;
#32827=CARTESIAN_POINT ( 'NONE',  ( -0.6758530183727028406, -0.6692913385826773087, -0.1292274648535924053 ) ) ;
#32828=CARTESIAN_POINT ( 'NONE',  ( -0.2690288713910754526, -0.5511811023622046335, 0.09757992244046803654 ) ) ;
#32830=CARTESIAN_POINT ( 'NONE',  ( -0.8070866141732276899, -0.5400638737290844871, 0.3530559997133364547 ) ) ;
#32831=CARTESIAN_POINT ( 'NONE',  ( -0.09842519685039295696, -0.5400638737290844871, 0.3530559997133364547 ) ) ;
#32832=CARTESIAN_POINT ( 'NONE',  ( 0.3937007874015754361, -0.1870078740157480601, -0.3641732283464567677 ) ) ;
#32834=CARTESIAN_POINT ( 'NONE',  ( -0.08530183727034056085, -0.3162353388693405765, 0.4822834645669290543 ) ) ;
#32837=CARTESIAN_POINT ( 'NONE',  ( 0.6627296587926517768, -0.5511811023622048555, -0.09757992244046775898 ) ) ;
#32838=CARTESIAN_POINT ( 'NONE',  ( 1.489501312335958172, -0.05778040916215560624, -0.4822834645669293319 ) ) ;
#32839=CARTESIAN_POINT ( 'NONE',  ( -1.010498687664041384, -0.3690944881889765550, -0.3153832671262227771 ) ) ;
#32840=CARTESIAN_POINT ( 'NONE',  ( -1.227034120734907585, 0.1771653543307087630, 0.09757992244046791164 ) ) ;
#32841=CARTESIAN_POINT ( 'NONE',  ( -0.5643044619422565855, -0.4281496062992124485, 0.4176697321401328655 ) ) ;
#32842=CARTESIAN_POINT ( 'NONE',  ( 0.03937007874015806264, 0.2952755905511811885, 0.000000000000000000 ) ) ;
#32843=CARTESIAN_POINT ( 'NONE',  ( 0.5577427821522316087, -0.08942795157527998196, 0.3641732283464567121 ) ) ;
#32845=CARTESIAN_POINT ( 'NONE',  ( 0.9776902887139113929, 0.1771653543307087630, 0.09757992244046791164 ) ) ;
#32846=CARTESIAN_POINT ( 'NONE',  ( 0.4527559055118117182, 0.1660481256975883668, -0.3530559997133364547 ) ) ;
#32848=CARTESIAN_POINT ( 'NONE',  ( -0.3740157480314953431, -0.5400638737290845981, -0.3530559997133363437 ) ) ;
#32850=CARTESIAN_POINT ( 'NONE',  ( 1.541994750656168645, -0.5511811023622046335, 0.09757992244046803654 ) ) ;
#32851=CARTESIAN_POINT ( 'NONE',  ( 0.6758530183727039509, -0.6692913385826771977, 0.1292274648535927661 ) ) ;
#32852=CARTESIAN_POINT ( 'NONE',  ( 0.1771653543307093182, -0.5400638737290845981, -0.3530559997133363437 ) ) ;
#32853=CARTESIAN_POINT ( 'NONE',  ( 1.112701331685804984, -9.595573933774993207E-16, 0.4281989832122458095 ) ) ;
#32854=CARTESIAN_POINT ( 'NONE',  ( -0.1181102362204717315, -0.5511811023622047445, 6.969142054262312111E-17 ) ) ;
#32855=CARTESIAN_POINT ( 'NONE',  ( 0.7545931758530189937, 0.2952755905511810774, -0.1292274648535930714 ) ) ;
#32856=CARTESIAN_POINT ( 'NONE',  ( -0.4724409448818890911, -0.1870078740157479769, 0.3641732283464567677 ) ) ;
#32858=CARTESIAN_POINT ( 'NONE',  ( -0.5183727034120726440, 0.2952755905511811885, 0.1292274648535926551 ) ) ;
#32859=CARTESIAN_POINT ( 'NONE',  ( 1.204164820379010070, 1.535433070866141447, 0.4915354330708652242 ) ) ;
#32860=CARTESIAN_POINT ( 'NONE',  ( -0.3215223097112853146, -0.3162353388693405765, 0.4822834645669290543 ) ) ;
#32862=CARTESIAN_POINT ( 'NONE',  ( -1.174540682414697335, -0.05778040916215522460, 0.4822834645669289988 ) ) ;
#32863=CARTESIAN_POINT ( 'NONE',  ( -0.8727034120734901146, -0.08942795157528024563, -0.3641732283464568787 ) ) ;
#32864=CARTESIAN_POINT ( 'NONE',  ( -0.006561679790025524116, -0.3162353388693405765, 0.4822834645669290543 ) ) ;
#32865=CARTESIAN_POINT ( 'NONE',  ( -1.450131233595799651, -0.6692913385826771977, 0.1292274648535927661 ) ) ;
#32866=CARTESIAN_POINT ( 'NONE',  ( -0.6758530183727028406, 0.2952755905511811885, 0.1292274648535926551 ) ) ;
#32868=CARTESIAN_POINT ( 'NONE',  ( -0.9348729704079935532, -2.191421614605370878E-15, 0.4445507791589071167 ) ) ;
#32869=CARTESIAN_POINT ( 'NONE',  ( 1.240157480314961314, -0.5400638737290844871, 0.3530559997133364547 ) ) ;
#32870=CARTESIAN_POINT ( 'NONE',  ( 1.115485564304462551, -0.4281496062992127816, -0.4176697321401328100 ) ) ;
#32873=CARTESIAN_POINT ( 'NONE',  ( -1.423884514435694859, -0.3162353388693405765, 0.4822834645669290543 ) ) ;
#32877=CARTESIAN_POINT ( 'NONE',  ( -0.2230971128608915943, -0.004921259842519576551, 0.3153832671262227771 ) ) ;
#32880=CARTESIAN_POINT ( 'NONE',  ( 0.2165354330708668673, 0.1660481256975883668, -0.3530559997133364547 ) ) ;
#32881=CARTESIAN_POINT ( 'NONE',  ( 0.3937007874015754361, -0.1870078740157480879, -0.4822834645669291653 ) ) ;
#32884=CARTESIAN_POINT ( 'NONE',  ( -0.8464566929133852113, 0.07958543189024085140, 0.2665933059059887866 ) ) ;
#32886=CARTESIAN_POINT ( 'NONE',  ( 0.7742782152230979209, 0.05413385826771626580, -0.4176697321401330321 ) ) ;
#32887=CARTESIAN_POINT ( 'NONE',  ( 0.8661417322834652488, -0.1870078740157480601, -0.3641732283464567677 ) ) ;
#32888=CARTESIAN_POINT ( 'NONE',  ( -0.3215223097112853146, -0.05778040916215560624, -0.4822834645669293319 ) ) ;
#32890=CARTESIAN_POINT ( 'NONE',  ( -0.7874015748031489847, -0.1870078740157480879, -0.4822834645669291653 ) ) ;
#32891=CARTESIAN_POINT ( 'NONE',  ( -1.692913385826770645, 0.1771653543307087630, 0.000000000000000000 ) ) ;
#32893=CARTESIAN_POINT ( 'NONE',  ( -0.8727034120734901146, -0.05778040916215560624, -0.4822834645669293319 ) ) ;
#32894=CARTESIAN_POINT ( 'NONE',  ( 1.213910761154856299, 0.2952755905511811885, 0.1292274648535926551 ) ) ;
#32898=CARTESIAN_POINT ( 'NONE',  ( -0.1181102362204717315, -0.6692913385826771977, 8.415575281601705876E-17 ) ) ;
#32900=CARTESIAN_POINT ( 'NONE',  ( -0.8202099737532801971, -0.6692913385826771977, 0.1292274648535927661 ) ) ;
#32901=CARTESIAN_POINT ( 'NONE',  ( 1.246719160104987623, -0.4281496062992124485, 0.4176697321401328655 ) ) ;
#32902=CARTESIAN_POINT ( 'NONE',  ( 1.089238845144357537, -0.4281496062992124485, 0.4176697321401328655 ) ) ;
#32903=CARTESIAN_POINT ( 'NONE',  ( 0.4527559055118117182, -0.5400638737290844871, 0.3530559997133364547 ) ) ;
#32904=EDGE_CURVE ( 'NONE', #62516, #25432, #16239, .T. ) ;
#32905=CARTESIAN_POINT ( 'NONE',  ( -0.3477690288713902178, 0.2952755905511810774, -0.1292274648535930714 ) ) ;
#32907=CARTESIAN_POINT ( 'NONE',  ( -1.286089238845143479, -0.6046776061558807314, 0.2411417322834647770 ) ) ;
#32908=CARTESIAN_POINT ( 'NONE',  ( -0.07874015748031421014, -0.1870078740157479769, 0.4822834645669291653 ) ) ;
#32910=CARTESIAN_POINT ( 'NONE',  ( -0.1837270341207340729, 0.1283753931104746893, -0.1820866141732285504 ) ) ;
#32911=CARTESIAN_POINT ( 'NONE',  ( 1.574803149606299746, -0.1870078740157480879, -0.4822834645669291653 ) ) ;
#32912=CARTESIAN_POINT ( 'NONE',  ( 1.371391076115485941, 0.2952755905511811885, 0.1292274648535926551 ) ) ;
#32913=CARTESIAN_POINT ( 'NONE',  ( -0.4002624671916004129, -0.05778040916215560624, -0.4822834645669293319 ) ) ;
#32915=CARTESIAN_POINT ( 'NONE',  ( 1.325459317585302665, 0.05413385826771626580, -0.4176697321401330321 ) ) ;
#32916=CARTESIAN_POINT ( 'NONE',  ( 0.4986876640419954376, 0.1539470093639523085, 0.1968503937007873850 ) ) ;
#32918=CARTESIAN_POINT ( 'NONE',  ( 0.3412073490813655186, -0.6046776061558809534, -0.2411417322834644161 ) ) ;
#32919=CARTESIAN_POINT ( 'NONE',  ( -0.4461942257217840213, 0.1283753931104748280, 0.1820866141732283561 ) ) ;
#32920=CARTESIAN_POINT ( 'NONE',  ( 1.555118110236221041, 0.07958543189024071263, -0.2665933059059888421 ) ) ;
#32921=CARTESIAN_POINT ( 'NONE',  ( -1.614173228346456712, 0.4410134679336886188, -0.1372047244094478091 ) ) ;
#32923=CARTESIAN_POINT ( 'NONE',  ( 1.568241469816273659, -0.08942795157528024563, -0.3641732283464568787 ) ) ;
#32924=CARTESIAN_POINT ( 'NONE',  ( 1.259842519685040019, -0.1870078740157479769, 0.4822834645669291653 ) ) ;
#32925=AXIS2_PLACEMENT_3D ( 'NONE', #41412, #46878, #21635 ) ;
#32927=CARTESIAN_POINT ( 'NONE',  ( -0.1115485564304456306, 0.2952755905511810774, -0.1292274648535930714 ) ) ;
#32928=CARTESIAN_POINT ( 'NONE',  ( -1.633858267716534529, 0.1660481256975885056, 0.3530559997133364547 ) ) ;
#32929=CARTESIAN_POINT ( 'NONE',  ( -1.732283464566928277, -0.1870078740157479769, 0.4822834645669291653 ) ) ;
#32930=CARTESIAN_POINT ( 'NONE',  ( -0.3412073490813641308, -0.6046776061558807314, 0.2411417322834647770 ) ) ;
#32932=CARTESIAN_POINT ( 'NONE',  ( 1.620734908136483465, -0.6692913385826771977, 0.1292274648535927661 ) ) ;
#32933=CARTESIAN_POINT ( 'NONE',  ( 0.6758530183727039509, 0.2952755905511810774, -0.1292274648535930714 ) ) ;
#32934=CARTESIAN_POINT ( 'NONE',  ( 1.043307086614173818, 0.07958543189024085140, 0.2665933059059887866 ) ) ;
#32936=CARTESIAN_POINT ( 'NONE',  ( 0.8136482939632553313, -0.5023911411419708095, -0.1820866141732282451 ) ) ;
#32937=CARTESIAN_POINT ( 'NONE',  ( -1.358267716535432434, -0.5400638737290844871, 0.3530559997133364547 ) ) ;
#32939=CARTESIAN_POINT ( 'NONE',  ( 1.141732283464567788, -0.6692913385826771977, 8.415575281601705876E-17 ) ) ;
#32941=CARTESIAN_POINT ( 'NONE',  ( 0.6561679790026253567, -0.6046776061558809534, -0.2411417322834644161 ) ) ;
#32943=DIRECTION ( 'NONE',  ( -3.096699300667737957E-16, 1.000000000000000000, -0.000000000000000000 ) ) ;
#32944=CARTESIAN_POINT ( 'NONE',  ( 0.2362204724409456558, -0.1870078740157480601, -0.3641732283464567677 ) ) ;
#32945=CARTESIAN_POINT ( 'NONE',  ( 0.4921259842519691285, -0.5400638737290845981, -0.3530559997133363437 ) ) ;
#32946=CARTESIAN_POINT ( 'NONE',  ( 1.686351706036745890, 0.1771653543307087630, 0.09757992244046791164 ) ) ;
#32947=CARTESIAN_POINT ( 'NONE',  ( -0.9776902887139098386, -0.5511811023622046335, 0.09757992244046803654 ) ) ;
#32948=CARTESIAN_POINT ( 'NONE',  ( -0.8202099737532801971, -0.6692913385826771977, 0.1292274648535927661 ) ) ;
#32949=CARTESIAN_POINT ( 'NONE',  ( -1.627296587926508442, -0.6046776061558809534, -0.2411417322834644161 ) ) ;
#32950=CARTESIAN_POINT ( 'NONE',  ( 1.082677165354331228, 0.1660481256975883668, -0.3530559997133364547 ) ) ;
#32951=CARTESIAN_POINT ( 'NONE',  ( 1.646981627296588035, -0.3162353388693405765, 0.4822834645669290543 ) ) ;
#32953=CARTESIAN_POINT ( 'NONE',  ( 0.9120734908136489683, -0.6692913385826771977, 0.1292274648535927661 ) ) ;
#32956=CARTESIAN_POINT ( 'NONE',  ( 1.568241469816273659, -0.05778040916215560624, -0.4822834645669293319 ) ) ;
#32957=CARTESIAN_POINT ( 'NONE',  ( -1.633858267716534529, -0.4536011799217368745, -0.2665933059059886201 ) ) ;
#32958=CARTESIAN_POINT ( 'NONE',  ( 1.069553805774278832, 0.1771653543307087075, -0.09757992244046823083 ) ) ;
#32959=CARTESIAN_POINT ( 'NONE',  ( -1.443569553805773564, 0.1283753931104746893, -0.1820866141732285504 ) ) ;
#32960=CARTESIAN_POINT ( 'NONE',  ( -0.5774278215223089816, -0.5023911411419708095, 0.1820866141732285504 ) ) ;
#32961=CARTESIAN_POINT ( 'NONE',  ( -1.594488188976377563, -0.4536011799217367080, 0.2665933059059888421 ) ) ;
#32962=CARTESIAN_POINT ( 'NONE',  ( 1.003937007874016185, 0.07958543189024071263, -0.2665933059059888421 ) ) ;
#32963=CARTESIAN_POINT ( 'NONE',  ( 0.5446194225721792126, -0.3162353388693405765, 0.4822834645669290543 ) ) ;
#32964=CARTESIAN_POINT ( 'NONE',  ( 1.003937007874016185, 0.1660481256975883668, -0.3530559997133364547 ) ) ;
#32965=CARTESIAN_POINT ( 'NONE',  ( 0.09842519685039434474, 0.1660481256975885056, 0.3530559997133364547 ) ) ;
#32966=CARTESIAN_POINT ( 'NONE',  ( 0.7480314960629927956, -0.5511811023622047445, 6.969142054262312111E-17 ) ) ;
#32967=CARTESIAN_POINT ( 'NONE',  ( 1.614173228346457378, 0.2952755905511811885, 0.000000000000000000 ) ) ;
#32969=CARTESIAN_POINT ( 'NONE',  ( -0.6824146981627291497, -0.6046776061558809534, -0.2411417322834644161 ) ) ;
#32972=CARTESIAN_POINT ( 'NONE',  ( 0.07874015748031558404, -0.1870078740157480879, -0.4822834645669291653 ) ) ;
#32973=CARTESIAN_POINT ( 'NONE',  ( -0.3805774278215216522, 0.05413385826771666132, 0.4176697321401328100 ) ) ;
#32975=CARTESIAN_POINT ( 'NONE',  ( -0.1837270341207343505, -0.6046776061558807314, 0.2411417322834647770 ) ) ;
#32981=CARTESIAN_POINT ( 'NONE',  ( -1.049868766404198794, 0.1283753931104746893, -0.1820866141732285504 ) ) ;
#32983=CARTESIAN_POINT ( 'NONE',  ( -1.240157480314959759, 0.1660481256975885056, 0.3530559997133364547 ) ) ;
#32985=CARTESIAN_POINT ( 'NONE',  ( 0.5446194225721792126, -0.3162353388693405765, 0.4822834645669290543 ) ) ;
#32986=CARTESIAN_POINT ( 'NONE',  ( -0.07874015748031421014, -0.1870078740157480601, -0.3641732283464567677 ) ) ;
#32987=CARTESIAN_POINT ( 'NONE',  ( 1.259842519685040019, -0.1870078740157479769, 0.4822834645669291653 ) ) ;
#32988=CARTESIAN_POINT ( 'NONE',  ( 0.4199475065616803948, -0.6046776061558809534, -0.2411417322834644161 ) ) ;
#32992=CARTESIAN_POINT ( 'NONE',  ( 1.076115485564305141, 0.2306618581243847221, -0.2411417322834647770 ) ) ;
#32993=CARTESIAN_POINT ( 'NONE',  ( 0.3018372703412079971, -0.4281496062992124485, 0.4176697321401328655 ) ) ;
#32994=CARTESIAN_POINT ( 'NONE',  ( 0.3412073490813655186, 0.2306618581243848609, 0.2411417322834645549 ) ) ;
#32995=CARTESIAN_POINT ( 'NONE',  ( 1.417322834645670104, -0.1870078740157480879, -0.4822834645669291653 ) ) ;
#32997=CARTESIAN_POINT ( 'NONE',  ( -0.09842519685039295696, 0.1660481256975883668, -0.3530559997133364547 ) ) ;
#32998=CARTESIAN_POINT ( 'NONE',  ( 1.141732283464567788, -0.6692913385826771977, 8.415575281601705876E-17 ) ) ;
#32999=CARTESIAN_POINT ( 'NONE',  ( 0.4921259842519691285, -0.5400638737290845981, -0.3530559997133363437 ) ) ;
#33000=CARTESIAN_POINT ( 'NONE',  ( 1.122047244094488860, -0.4536011799217368745, -0.2665933059059886201 ) ) ;
#33001=CARTESIAN_POINT ( 'NONE',  ( -1.089238845144356427, 0.05413385826771666132, 0.4176697321401328100 ) ) ;
#33002=CARTESIAN_POINT ( 'NONE',  ( -1.528871391076114250, 0.2952755905511810774, -0.1292274648535930714 ) ) ;
#33003=CARTESIAN_POINT ( 'NONE',  ( 0.7349081364829402885, -0.6046776061558809534, -0.2411417322834644161 ) ) ;
#33006=ORIENTED_EDGE ( 'NONE', *, *, #50269, .T. ) ;
#33009=CARTESIAN_POINT ( 'NONE',  ( 1.351706036745407680, 0.05413385826771666132, 0.4176697321401328100 ) ) ;
#33010=CARTESIAN_POINT ( 'NONE',  ( 1.043307086614173818, -0.4536011799217368745, -0.2665933059059886201 ) ) ;
#33015=CARTESIAN_POINT ( 'NONE',  ( -1.253280839895012377, -0.2845877964562161244, -0.3641732283464567121 ) ) ;
#33016=CARTESIAN_POINT ( 'NONE',  ( -1.653543307086613234, -0.1870078740157480601, -0.3641732283464567677 ) ) ;
#33018=CARTESIAN_POINT ( 'NONE',  ( -0.2296587926509179312, -0.3162353388693409650, -0.4822834645669289433 ) ) ;
#33019=CARTESIAN_POINT ( 'NONE',  ( 1.292650918635171564, 0.2952755905511811885, 0.1292274648535926551 ) ) ;
#33022=CARTESIAN_POINT ( 'NONE',  ( -1.482939632545930975, -0.4281496062992127816, -0.4176697321401328100 ) ) ;
#33023=CARTESIAN_POINT ( 'NONE',  ( -0.7201575634749992627, -5.642773921931522838E-15, -0.3791483426435192094 ) ) ;
#33027=CARTESIAN_POINT ( 'NONE',  ( -0.8070866141732276899, 0.07958543189024071263, -0.2665933059059888421 ) ) ;
#33028=CARTESIAN_POINT ( 'NONE',  ( -1.377952755905511140, -0.6692913385826771977, 8.415575281601705876E-17 ) ) ;
#33029=CARTESIAN_POINT ( 'NONE',  ( 0.6167979002624679463, 0.05413385826771626580, -0.4176697321401330321 ) ) ;
#33033=FACE_OUTER_BOUND ( 'NONE', #13035, .T. ) ;
#33034=CARTESIAN_POINT ( 'NONE',  ( 1.364829396325460076, 0.2306618581243848609, 0.2411417322834645549 ) ) ;
#33035=CARTESIAN_POINT ( 'NONE',  ( 1.528871391076116026, -0.5511811023622048555, -0.09757992244046775898 ) ) ;
#33037=CARTESIAN_POINT ( 'NONE',  ( -0.4068241469816267775, -0.004921259842519870586, -0.3153832671262229437 ) ) ;
#33038=CARTESIAN_POINT ( 'NONE',  ( -1.358267716535432434, -0.4536011799217367080, 0.2665933059059888421 ) ) ;
#33040=CARTESIAN_POINT ( 'NONE',  ( 0.4724409448818904789, -0.1870078740157479769, 0.4822834645669291653 ) ) ;
#33041=CARTESIAN_POINT ( 'NONE',  ( -0.9580052493438311334, -0.004921259842519870586, -0.3153832671262229437 ) ) ;
#33042=CARTESIAN_POINT ( 'NONE',  ( 0.2493438320209980519, -0.3690944881889765550, -0.3153832671262227771 ) ) ;
#33043=CARTESIAN_POINT ( 'NONE',  ( 0.1640419947506569498, -0.05778040916215522460, 0.4822834645669289988 ) ) ;
#33044=CARTESIAN_POINT ( 'NONE',  ( -0.9514435695538050464, -0.08942795157528024563, -0.3641732283464568787 ) ) ;
#33046=CARTESIAN_POINT ( 'NONE',  ( 0.9317585301837276734, -0.4281496062992124485, 0.4176697321401328655 ) ) ;
#33048=CARTESIAN_POINT ( 'NONE',  ( -1.253280839895012377, -0.3162353388693409650, -0.4822834645669289433 ) ) ;
#33050=CARTESIAN_POINT ( 'NONE',  ( -0.7677165354330699465, 0.1660481256975885056, 0.3530559997133364547 ) ) ;
#33051=CARTESIAN_POINT ( 'NONE',  ( -0.3149606299212590610, -0.1870078740157479769, 0.3641732283464567677 ) ) ;
#33052=CARTESIAN_POINT ( 'NONE',  ( -1.095800524934382292, -0.3162353388693409650, -0.4822834645669289433 ) ) ;
#33053=CARTESIAN_POINT ( 'NONE',  ( 0.8661417322834653598, -0.1870078740157479769, 0.3641732283464567677 ) ) ;
#33054=CARTESIAN_POINT ( 'NONE',  ( -0.2755905511811018171, 0.1771653543307087630, 0.000000000000000000 ) ) ;
#33055=CARTESIAN_POINT ( 'NONE',  ( -0.6233595800524928121, -0.05778040916215522460, 0.4822834645669289988 ) ) ;
#33056=CARTESIAN_POINT ( 'NONE',  ( -1.325459317585300889, -0.4281496062992127816, -0.4176697321401328100 ) ) ;
#33057=B_SPLINE_CURVE_WITH_KNOTS ( 'NONE', 3,
 ( #67128, #9458, #16202, #46497, #46913, #59966, #65885 ),
 .UNSPECIFIED., .F., .F.,
 ( 4, 3, 4 ),
 ( 3.469446951953614189E-17, 0.001246232571205268744, 0.002492492258783275856 ),
 .UNSPECIFIED. ) ;
#33058=CARTESIAN_POINT ( 'NONE',  ( -1.581364829396324945, -0.05778040916215560624, -0.4822834645669293319 ) ) ;
#33060=CARTESIAN_POINT ( 'NONE',  ( 1.384514435695538559, 0.1771653543307087075, -0.09757992244046823083 ) ) ;
#33061=CARTESIAN_POINT ( 'NONE',  ( 0.4396325459317593221, 0.2952755905511810774, -0.1292274648535930714 ) ) ;
#33062=CARTESIAN_POINT ( 'NONE',  ( 1.220472440944882386, 0.2952755905511811885, 0.000000000000000000 ) ) ;
#33063=CARTESIAN_POINT ( 'NONE',  ( -1.653543307086613234, -0.1870078740157480879, -0.4822834645669291653 ) ) ;
#33067=CARTESIAN_POINT ( 'NONE',  ( -1.062992125984250968, -0.5511811023622047445, 6.969142054262312111E-17 ) ) ;
#33068=CARTESIAN_POINT ( 'NONE',  ( 0.9383202099737536495, -0.3162353388693405765, 0.4822834645669290543 ) ) ;
#33070=CARTESIAN_POINT ( 'NONE',  ( -1.069553805774277722, 0.1771653543307087630, 0.09757992244046791164 ) ) ;
#33072=CARTESIAN_POINT ( 'NONE',  ( -1.095800524934382292, -0.05778040916215522460, 0.4822834645669289988 ) ) ;
#33074=VECTOR ( 'NONE', #66390, 39.37007874015748143 ) ;
#33075=CARTESIAN_POINT ( 'NONE',  ( 0.8530183727034128527, -0.4281496062992124485, 0.4176697321401328655 ) ) ;
#33076=CARTESIAN_POINT ( 'NONE',  ( 0.3018372703412079971, 0.05413385826771626580, -0.4176697321401330321 ) ) ;
#33077=CARTESIAN_POINT ( 'NONE',  ( 0.9973753280839902091, 0.2306618581243847221, -0.2411417322834647770 ) ) ;
#33078=CARTESIAN_POINT ( 'NONE',  ( -1.725721784776902190, -0.08942795157527998196, 0.3641732283464567121 ) ) ;
#33083=CARTESIAN_POINT ( 'NONE',  ( 0.9580052493438327987, -0.3690944881889765550, -0.3153832671262227771 ) ) ;
#33084=CARTESIAN_POINT ( 'NONE',  ( 0.1837270341207354329, 0.1283753931104748280, 0.1820866141732283561 ) ) ;
#33085=CARTESIAN_POINT ( 'NONE',  ( 0.1246719160104994284, -0.6692913385826771977, 0.1292274648535927661 ) ) ;
#33086=CARTESIAN_POINT ( 'NONE',  ( 1.423884514435696191, -0.05778040916215522460, 0.4822834645669289988 ) ) ;
#33088=CARTESIAN_POINT ( 'NONE',  ( 0.3608923884514443348, -0.5511811023622046335, 0.09757992244046803654 ) ) ;
#33089=CARTESIAN_POINT ( 'NONE',  ( -0.9383202099737524282, -0.3162353388693409650, -0.4822834645669289433 ) ) ;
#33090=CARTESIAN_POINT ( 'NONE',  ( 1.423884514435696191, -0.05778040916215522460, 0.4822834645669289988 ) ) ;
#33091=CARTESIAN_POINT ( 'NONE',  ( 0.9645669291338591078, -0.5400638737290845981, -0.3530559997133363437 ) ) ;
#33093=CARTESIAN_POINT ( 'NONE',  ( 1.614173228346457378, 1.330640075373405118, -0.1372047244094476148 ) ) ;
#33095=ORIENTED_EDGE ( 'NONE', *, *, #49331, .T. ) ;
#33096=ORIENTED_EDGE ( 'NONE', *, *, #19297, .T. ) ;
#33097=CARTESIAN_POINT ( 'NONE',  ( -1.437007874015747477, -0.5400638737290844871, 0.3530559997133364547 ) ) ;
#33098=CARTESIAN_POINT ( 'NONE',  ( -0.6758530183727028406, 0.1771653543307087630, 0.09757992244046791164 ) ) ;
#33099=CARTESIAN_POINT ( 'NONE',  ( -0.5511811023622038563, -0.1870078740157479769, 0.4822834645669291653 ) ) ;
#33102=CARTESIAN_POINT ( 'NONE',  ( -1.601049868766403650, 0.1283753931104746893, -0.1820866141732285504 ) ) ;
#33103=CARTESIAN_POINT ( 'NONE',  ( -1.220472440944881054, 0.2952755905511811885, 0.000000000000000000 ) ) ;
#33104=CARTESIAN_POINT ( 'NONE',  ( 0.1377952755905518800, -0.5400638737290844871, 0.3530559997133364547 ) ) ;
#33105=CARTESIAN_POINT ( 'NONE',  ( -1.410761154855641575, -0.3162353388693409650, -0.4822834645669289433 ) ) ;
#33108=CARTESIAN_POINT ( 'NONE',  ( 0.4593175853018379162, -0.4281496062992124485, 0.4176697321401328655 ) ) ;
#33110=CARTESIAN_POINT ( 'NONE',  ( -0.8333333333333323711, 0.1771653543307087630, 0.09757992244046791164 ) ) ;
#33111=VERTEX_POINT ( 'NONE', #206 ) ;
#33115=CARTESIAN_POINT ( 'NONE',  ( -1.167979002624671470, -0.4281496062992127816, -0.4176697321401328100 ) ) ;
#33116=CARTESIAN_POINT ( 'NONE',  ( -1.443569553805773564, 0.2306618581243847221, -0.2411417322834647770 ) ) ;
#33118=CARTESIAN_POINT ( 'NONE',  ( -1.089238845144356427, 0.05413385826771666132, 0.4176697321401328100 ) ) ;
#33119=CARTESIAN_POINT ( 'NONE',  ( -1.358267716535432434, 0.1660481256975883668, -0.3530559997133364547 ) ) ;
#33120=CARTESIAN_POINT ( 'NONE',  ( -1.286089238845143479, 0.2306618581243847221, -0.2411417322834647770 ) ) ;
#33121=CARTESIAN_POINT ( 'NONE',  ( -1.604771003085129655, 1.829390573268580455, 0.1466069496707748387 ) ) ;
#33123=CARTESIAN_POINT ( 'NONE',  ( 0.1706036745406830368, -0.3690944881889765550, -0.3153832671262227771 ) ) ;
#33126=CARTESIAN_POINT ( 'NONE',  ( -0.2624671916010490880, 0.1283753931104746893, -0.1820866141732285504 ) ) ;
#33127=CARTESIAN_POINT ( 'NONE',  ( -0.7020997375328074108, -0.05778040916215522460, 0.4822834645669289988 ) ) ;
#33128=CARTESIAN_POINT ( 'NONE',  ( 1.148293963254593653, 0.2952755905511810774, -0.1292274648535930714 ) ) ;
#33129=CARTESIAN_POINT ( 'NONE',  ( -0.5577427821522301654, -0.3162353388693405765, 0.4822834645669290543 ) ) ;
#33130=ORIENTED_EDGE ( 'NONE', *, *, #52141, .T. ) ;
#33133=CARTESIAN_POINT ( 'NONE',  ( -0.9711286089238838626, 0.2306618581243847221, -0.2411417322834647770 ) ) ;
#33134=CARTESIAN_POINT ( 'NONE',  ( 0.7349081364829402885, -0.6046776061558809534, -0.2411417322834644161 ) ) ;
#33135=CARTESIAN_POINT ( 'NONE',  ( -1.692913385826770645, 0.1771653543307087630, 0.000000000000000000 ) ) ;
#33139=AXIS2_PLACEMENT_3D ( 'NONE', #77981, #7695, #64502 ) ;
#33141=CARTESIAN_POINT ( 'NONE',  ( -0.1246719160104980823, -0.6692913385826773087, -0.1292274648535924053 ) ) ;
#33142=CARTESIAN_POINT ( 'NONE',  ( 1.679790026246720025, 0.2306618581243848609, 0.2411417322834645549 ) ) ;
#33143=AXIS2_PLACEMENT_3D ( 'NONE', #21373, #47857, #35244 ) ;
#33145=CARTESIAN_POINT ( 'NONE',  ( -0.7808398950131225646, -0.05778040916215522460, 0.4822834645669289988 ) ) ;
#33147=CARTESIAN_POINT ( 'NONE',  ( -1.246719160104986512, 0.05413385826771666132, 0.4176697321401328100 ) ) ;
#33149=CARTESIAN_POINT ( 'NONE',  ( -0.8792650918635160906, 0.05413385826771626580, -0.4176697321401330321 ) ) ;
#33150=CARTESIAN_POINT ( 'NONE',  ( -0.5905511811023615998, 0.2952755905511811885, 0.000000000000000000 ) ) ;
#33152=CARTESIAN_POINT ( 'NONE',  ( 0.8202099737532813073, 0.1771653543307087630, 0.09757992244046791164 ) ) ;
#33154=CARTESIAN_POINT ( 'NONE',  ( 0.5446194225721792126, -0.2845877964562159024, 0.3641732283464567677 ) ) ;
#33155=CARTESIAN_POINT ( 'NONE',  ( 1.207349081364829990, -0.5023911411419708095, -0.1820866141732282451 ) ) ;
#33156=CARTESIAN_POINT ( 'NONE',  ( 1.489501312335958172, -0.05778040916215560624, -0.4822834645669293319 ) ) ;
#33157=CARTESIAN_POINT ( 'NONE',  ( 0.02624671916010564918, -0.5023911411419708095, -0.1820866141732282451 ) ) ;
#33159=CARTESIAN_POINT ( 'NONE',  ( -1.404199475065615932, -0.4281496062992127816, -0.4176697321401328100 ) ) ;
#33160=CARTESIAN_POINT ( 'NONE',  ( 1.351706036745407458, -0.4281496062992127816, -0.4176697321401328100 ) ) ;
#33163=CARTESIAN_POINT ( 'NONE',  ( -0.5774278215223089816, -0.5023911411419708095, 0.1820866141732285504 ) ) ;
#33164=CARTESIAN_POINT ( 'NONE',  ( 1.614173228346457156, 1.929133858267716661, 0.5309055118110233007 ) ) ;
#33165=CARTESIAN_POINT ( 'NONE',  ( 0.2427821522309719648, -0.05778040916215522460, 0.4822834645669289988 ) ) ;
#33167=CARTESIAN_POINT ( 'NONE',  ( 0.7545931758530188826, -0.5511811023622046335, 0.09757992244046803654 ) ) ;
#33168=CARTESIAN_POINT ( 'NONE',  ( 0.09186351706036799403, -0.3690944881889765550, -0.3153832671262227771 ) ) ;
#33169=CARTESIAN_POINT ( 'NONE',  ( -0.2230971128608915943, 0.05413385826771666132, 0.4176697321401328100 ) ) ;
#33170=CARTESIAN_POINT ( 'NONE',  ( -1.371391076115484831, 0.2952755905511810774, -0.1292274648535930714 ) ) ;
#33171=CARTESIAN_POINT ( 'NONE',  ( -0.6824146981627288167, 0.1283753931104748280, 0.1820866141732283561 ) ) ;
#33173=CARTESIAN_POINT ( 'NONE',  ( 0.4199475065616805614, 0.2306618581243848609, 0.2411417322834645549 ) ) ;
#33174=CARTESIAN_POINT ( 'NONE',  ( -0.9186351706036736120, -0.6046776061558809534, -0.2411417322834644161 ) ) ;
#33177=CARTESIAN_POINT ( 'NONE',  ( 0.2952755905511816326, -0.4536011799217367080, 0.2665933059059888421 ) ) ;
#33178=CARTESIAN_POINT ( 'NONE',  ( -0.9973753280839886548, 0.2306618581243848609, 0.2411417322834645549 ) ) ;
#33179=CARTESIAN_POINT ( 'NONE',  ( -1.213910761154854745, -0.6692913385826771977, 0.1292274648535927661 ) ) ;
#33180=CARTESIAN_POINT ( 'NONE',  ( -1.305774278215222184, 0.1771653543307087630, 0.09757992244046791164 ) ) ;
#33181=CARTESIAN_POINT ( 'NONE',  ( 1.581364829396326277, -0.3162353388693409650, -0.4822834645669289433 ) ) ;
#33183=CARTESIAN_POINT ( 'NONE',  ( -0.9317585301837263412, -0.3690944881889765550, -0.3153832671262227771 ) ) ;
#33184=CARTESIAN_POINT ( 'NONE',  ( 1.227034120734908917, -0.6692913385826771977, 0.1292274648535927661 ) ) ;
#33190=CARTESIAN_POINT ( 'NONE',  ( -1.660104986876639543, -0.05778040916215560624, -0.4822834645669293319 ) ) ;
#33191=CARTESIAN_POINT ( 'NONE',  ( -1.292650918635170010, -0.6692913385826771977, 0.1292274648535927661 ) ) ;
#33193=CARTESIAN_POINT ( 'NONE',  ( 1.095800524934383846, -0.3162353388693405765, 0.4822834645669290543 ) ) ;
#33195=LINE ( 'NONE', #45381, #52524 ) ;
#33196=CARTESIAN_POINT ( 'NONE',  ( 0.4527559055118117182, 0.1660481256975883668, -0.3530559997133364547 ) ) ;
#33197=CARTESIAN_POINT ( 'NONE',  ( -0.2099737532808391705, 0.2306618581243848609, 0.2411417322834645549 ) ) ;
#33202=CARTESIAN_POINT ( 'NONE',  ( 0.06804098107080244762, 1.722984403643211298E-16, -0.4118484887281974594 ) ) ;
#33203=CARTESIAN_POINT ( 'NONE',  ( 0.9776902887139113929, 0.1771653543307087630, 0.09757992244046791164 ) ) ;
#33208=CARTESIAN_POINT ( 'NONE',  ( -0.03937007874015669567, -0.6692913385826771977, 8.415575281601705876E-17 ) ) ;
#33210=CARTESIAN_POINT ( 'NONE',  ( 1.437007874015748810, 0.1660481256975885056, 0.3530559997133364547 ) ) ;
#33211=CARTESIAN_POINT ( 'NONE',  ( 0.1312335958005257930, 0.2306618581243847221, -0.2411417322834647770 ) ) ;
#33212=CARTESIAN_POINT ( 'NONE',  ( 1.351706036745407680, 0.05413385826771666132, 0.4176697321401328100 ) ) ;
#33213=CARTESIAN_POINT ( 'NONE',  ( -0.3083989501312330295, -0.3162353388693409650, -0.4822834645669289433 ) ) ;
#33214=CARTESIAN_POINT ( 'NONE',  ( -0.05249343832020938322, -0.6046776061558809534, -0.2411417322834644161 ) ) ;
#33215=CARTESIAN_POINT ( 'NONE',  ( 1.568241469816273437, -0.3162353388693405765, 0.4822834645669290543 ) ) ;
#33216=CARTESIAN_POINT ( 'NONE',  ( 1.266404199475066328, -0.05778040916215522460, 0.4822834645669289988 ) ) ;
#33218=CARTESIAN_POINT ( 'NONE',  ( 1.161417322834646493, -0.5400638737290844871, 0.3530559997133364547 ) ) ;
#33220=CARTESIAN_POINT ( 'NONE',  ( 0.2362204724409456558, -0.1870078740157479769, 0.3641732283464567677 ) ) ;
#33221=VERTEX_POINT ( 'NONE', #79317 ) ;
#33224=CARTESIAN_POINT ( 'NONE',  ( -0.5249343832020990641, -0.5023911411419708095, -0.1820866141732282451 ) ) ;
#33225=CARTESIAN_POINT ( 'NONE',  ( -0.1837270341207340729, 0.2306618581243847221, -0.2411417322834647770 ) ) ;
#33227=CARTESIAN_POINT ( 'NONE',  ( 0.2296587926509192634, -0.05778040916215560624, -0.4822834645669293319 ) ) ;
#33228=CARTESIAN_POINT ( 'NONE',  ( 0.1246719160104994284, -0.6692913385826771977, 0.1292274648535927661 ) ) ;
#33229=CARTESIAN_POINT ( 'NONE',  ( -0.7677165354330699465, -0.5400638737290845981, -0.3530559997133363437 ) ) ;
#33230=CARTESIAN_POINT ( 'NONE',  ( -1.174540682414697335, -0.3162353388693409650, -0.4822834645669289433 ) ) ;
#33232=CARTESIAN_POINT ( 'NONE',  ( 1.568241469816273659, -0.08942795157528024563, -0.3641732283464568787 ) ) ;
#33233=CARTESIAN_POINT ( 'NONE',  ( 1.595398199321655497, 0.4619154201552252981, 0.1559797534342493852 ) ) ;
#33235=CARTESIAN_POINT ( 'NONE',  ( 0.8727034120734912248, -0.2845877964562161244, -0.3641732283464567121 ) ) ;
#33236=CARTESIAN_POINT ( 'NONE',  ( 0.6036745406824154392, 0.2306618581243847221, -0.2411417322834647770 ) ) ;
#33237=CARTESIAN_POINT ( 'NONE',  ( 0.8136482939632553313, -0.6046776061558809534, -0.2411417322834644161 ) ) ;
#33239=DIRECTION ( 'NONE',  ( 0.000000000000000000, 0.000000000000000000, 1.000000000000000000 ) ) ;
#33242=CARTESIAN_POINT ( 'NONE',  ( -0.4658792650918627265, -0.05778040916215522460, 0.4822834645669289988 ) ) ;
#33246=CARTESIAN_POINT ( 'NONE',  ( -1.010498687664041384, -0.004921259842519576551, 0.3153832671262227771 ) ) ;
#33247=CARTESIAN_POINT ( 'NONE',  ( 1.286089238845145033, 0.2306618581243848609, 0.2411417322834645549 ) ) ;
#33248=CARTESIAN_POINT ( 'NONE',  ( 0.9448818897637802916, -0.1870078740157480879, -0.4822834645669291653 ) ) ;
#33249=CARTESIAN_POINT ( 'NONE',  ( -0.3346456692913377662, 0.07958543189024071263, -0.2665933059059888421 ) ) ;
#33250=CARTESIAN_POINT ( 'NONE',  ( 0.3280839895013130669, 0.05413385826771666132, 0.4176697321401328100 ) ) ;
#33252=CARTESIAN_POINT ( 'NONE',  ( 0.2034120734908144990, -0.5511811023622046335, 0.09757992244046803654 ) ) ;
#33253=CARTESIAN_POINT ( 'NONE',  ( -0.2034120734908131112, -0.6692913385826773087, -0.1292274648535924053 ) ) ;
#33255=CARTESIAN_POINT ( 'NONE',  ( -1.207349081364828880, 0.2306618581243847221, -0.2411417322834647770 ) ) ;
#33256=CARTESIAN_POINT ( 'NONE',  ( 0.6955380577427828781, -0.004921259842519870586, -0.3153832671262229437 ) ) ;
#33258=CARTESIAN_POINT ( 'NONE',  ( -0.6036745406824141069, 0.2306618581243848609, 0.2411417322834645549 ) ) ;
#33259=CARTESIAN_POINT ( 'NONE',  ( -0.3543307086614165824, 0.1771653543307087630, 0.000000000000000000 ) ) ;
#33261=CARTESIAN_POINT ( 'NONE',  ( -0.8202099737532801971, -0.6692913385826771977, 0.1292274648535927661 ) ) ;
#33262=CARTESIAN_POINT ( 'NONE',  ( -0.7808398950131222316, -0.3162353388693409650, -0.4822834645669289433 ) ) ;
#33263=CARTESIAN_POINT ( 'NONE',  ( -0.08530183727034056085, -0.3162353388693405765, 0.4822834645669290543 ) ) ;
#33265=CARTESIAN_POINT ( 'NONE',  ( -0.1706036745406816491, 0.05413385826771626580, -0.4176697321401330321 ) ) ;
#33270=CARTESIAN_POINT ( 'NONE',  ( 0.7086614173228353852, -0.1870078740157479769, 0.3641732283464567677 ) ) ;
#33271=CARTESIAN_POINT ( 'NONE',  ( 1.246719160104987623, -0.4281496062992124485, 0.4176697321401328655 ) ) ;
#33272=CARTESIAN_POINT ( 'NONE',  ( -0.8267716535433065062, -0.5511811023622047445, 6.969142054262312111E-17 ) ) ;
#33273=CARTESIAN_POINT ( 'NONE',  ( -0.9973753280839886548, -0.5023911411419708095, -0.1820866141732282451 ) ) ;
#33274=CARTESIAN_POINT ( 'NONE',  ( -0.6758530183727028406, 0.2952755905511811885, 0.1292274648535926551 ) ) ;
#33275=CARTESIAN_POINT ( 'NONE',  ( -0.1377952755905504645, 0.1660481256975885056, 0.3530559997133364547 ) ) ;
#33276=CARTESIAN_POINT ( 'NONE',  ( 0.4330708661417329575, 0.1771653543307087630, 0.000000000000000000 ) ) ;
#33278=CARTESIAN_POINT ( 'NONE',  ( 0.8661417322834652488, -0.1870078740157480601, -0.3641732283464567677 ) ) ;
#33279=CARTESIAN_POINT ( 'NONE',  ( 0.3805774278215230400, -0.4281496062992124485, 0.4176697321401328655 ) ) ;
#33281=CARTESIAN_POINT ( 'NONE',  ( -0.7742782152230965886, 0.05413385826771666132, 0.4176697321401328100 ) ) ;
#33283=CARTESIAN_POINT ( 'NONE',  ( 1.279527559055118724, 0.07958543189024085140, 0.2665933059059887866 ) ) ;
#33284=CARTESIAN_POINT ( 'NONE',  ( 0.4724409448818904789, -0.1870078740157480879, -0.4822834645669291653 ) ) ;
#33285=CARTESIAN_POINT ( 'NONE',  ( 0.2755905511811031494, 0.2952755905511811885, 0.000000000000000000 ) ) ;
#33286=CARTESIAN_POINT ( 'NONE',  ( 0.2034120734908144990, -0.5511811023622046335, 0.09757992244046803654 ) ) ;
#33287=CARTESIAN_POINT ( 'NONE',  ( 0.6175017169405826456, 2.784432375088962958E-17, -0.3464511005275205946 ) ) ;
#33288=CARTESIAN_POINT ( 'NONE',  ( -0.1574803149606292529, -0.1870078740157480601, -0.3641732283464567677 ) ) ;
#33289=CARTESIAN_POINT ( 'NONE',  ( 0.8530183727034128527, -0.4281496062992124485, 0.4176697321401328655 ) ) ;
#33291=CARTESIAN_POINT ( 'NONE',  ( -0.7480314960629914633, 0.1771653543307087630, 0.000000000000000000 ) ) ;
#33292=CARTESIAN_POINT ( 'NONE',  ( -0.7545931758530176614, -0.6692913385826773087, -0.1292274648535924053 ) ) ;
#33294=ORIENTED_EDGE ( 'NONE', *, *, #12532, .F. ) ;
#33295=CARTESIAN_POINT ( 'NONE',  ( -1.292650918635170010, 0.2952755905511810774, -0.1292274648535930714 ) ) ;
#33296=CARTESIAN_POINT ( 'NONE',  ( -1.292650918635170010, -0.5511811023622046335, 0.09757992244046803654 ) ) ;
#33297=CARTESIAN_POINT ( 'NONE',  ( 0.08530183727034192087, -0.3162353388693409650, -0.4822834645669289433 ) ) ;
#33298=CARTESIAN_POINT ( 'NONE',  ( -1.496062992125983815, -0.1870078740157480879, -0.4822834645669291653 ) ) ;
#33299=CARTESIAN_POINT ( 'NONE',  ( -0.6233595800524928121, -0.3162353388693409650, -0.4822834645669289433 ) ) ;
#33300=DIRECTION ( 'NONE',  ( -1.000000000000000000, -3.412570772413389987E-16, 0.000000000000000000 ) ) ;
#33301=CARTESIAN_POINT ( 'NONE',  ( 1.076115485564305141, 0.2306618581243847221, -0.2411417322834647770 ) ) ;
#33302=CARTESIAN_POINT ( 'NONE',  ( 0.9973753280839902091, 0.2306618581243847221, -0.2411417322834647770 ) ) ;
#33303=CARTESIAN_POINT ( 'NONE',  ( 1.430446194225722500, -0.4281496062992127816, -0.4176697321401328100 ) ) ;
#33305=CARTESIAN_POINT ( 'NONE',  ( 1.548556430446194954, -0.6046776061558807314, 0.2411417322834647770 ) ) ;
#33306=CARTESIAN_POINT ( 'NONE',  ( -1.194225721784776262, 0.05413385826771626580, -0.4176697321401330321 ) ) ;
#33309=VERTEX_POINT ( 'NONE', #21636 ) ;
#33310=CARTESIAN_POINT ( 'NONE',  ( -0.1968503937007867743, 0.1771653543307087630, 0.000000000000000000 ) ) ;
#33313=CARTESIAN_POINT ( 'NONE',  ( 0.06561679790026316017, 0.05413385826771626580, -0.4176697321401330321 ) ) ;
#33314=CARTESIAN_POINT ( 'NONE',  ( 0.2296587926509192634, -0.05778040916215560624, -0.4822834645669293319 ) ) ;
#33315=CARTESIAN_POINT ( 'NONE',  ( -0.6167979002624665030, -0.4281496062992127816, -0.4176697321401328100 ) ) ;
#33317=CARTESIAN_POINT ( 'NONE',  ( -0.8070866141732276899, 0.07958543189024071263, -0.2665933059059888421 ) ) ;
#33319=CARTESIAN_POINT ( 'NONE',  ( 0.8005249343832028242, -0.4281496062992127816, -0.4176697321401328100 ) ) ;
#33320=CARTESIAN_POINT ( 'NONE',  ( 0.4790026246719167324, -0.08942795157527998196, 0.3641732283464567121 ) ) ;
#33321=CARTESIAN_POINT ( 'NONE',  ( -0.3412073490813641308, 0.2306618581243847221, -0.2411417322834647770 ) ) ;
#33323=CARTESIAN_POINT ( 'NONE',  ( -0.6430446194225712953, 0.05413385826771626580, -0.4176697321401330321 ) ) ;
#33324=CARTESIAN_POINT ( 'NONE',  ( -1.574803149606298636, -0.1870078740157479769, 0.3641732283464567677 ) ) ;
#33325=CARTESIAN_POINT ( 'NONE',  ( 1.167979002624672580, -0.4281496062992124485, 0.4176697321401328655 ) ) ;
#33326=CARTESIAN_POINT ( 'NONE',  ( 1.660104986876641320, -0.08942795157527998196, 0.3641732283464567121 ) ) ;
#33329=CARTESIAN_POINT ( 'NONE',  ( -0.1377952755905504645, -0.5400638737290845981, -0.3530559997133363437 ) ) ;
#33332=CARTESIAN_POINT ( 'NONE',  ( -0.8595800524934373854, -0.3162353388693409650, -0.4822834645669289433 ) ) ;
#33333=CARTESIAN_POINT ( 'NONE',  ( 1.548556430446194954, -0.6046776061558807314, 0.2411417322834647770 ) ) ;
#33334=CARTESIAN_POINT ( 'NONE',  ( 1.233595800524935227, -0.6046776061558807314, 0.2411417322834647770 ) ) ;
#33335=CARTESIAN_POINT ( 'NONE',  ( 0.1312335958005255154, -0.6046776061558807314, 0.2411417322834647770 ) ) ;
#33336=CARTESIAN_POINT ( 'NONE',  ( -0.2690288713910754526, -0.6692913385826771977, 0.1292274648535927661 ) ) ;
#33338=CARTESIAN_POINT ( 'NONE',  ( -1.207349081364828880, 0.2306618581243847221, -0.2411417322834647770 ) ) ;
#33339=CARTESIAN_POINT ( 'NONE',  ( -0.07217847769028787330, -0.05778040916215522460, 0.4822834645669289988 ) ) ;
#33340=CARTESIAN_POINT ( 'NONE',  ( 0.06561679790026316017, -0.3690944881889763329, 0.3153832671262228327 ) ) ;
#33341=DIRECTION ( 'NONE',  ( 0.000000000000000000, 0.000000000000000000, 1.000000000000000000 ) ) ;
#33342=CARTESIAN_POINT ( 'NONE',  ( -0.3937007874015740483, -0.1870078740157480879, -0.4822834645669291653 ) ) ;
#33344=CARTESIAN_POINT ( 'NONE',  ( 1.318897637795276356, 0.1660481256975883668, -0.3530559997133364547 ) ) ;
#33347=CARTESIAN_POINT ( 'NONE',  ( -0.1115485564304453947, -0.6692913385826771977, 0.1292274648535927661 ) ) ;
#33348=CARTESIAN_POINT ( 'NONE',  ( -0.1574803149606292529, -0.1870078740157479769, 0.3641732283464567677 ) ) ;
#33349=CARTESIAN_POINT ( 'NONE',  ( 0.9251968503937015864, 0.07958543189024071263, -0.2665933059059888421 ) ) ;
#33351=CARTESIAN_POINT ( 'NONE',  ( 1.220472440944882386, 0.000000000000000000, 0.4445507791589061175 ) ) ;
#33352=CARTESIAN_POINT ( 'NONE',  ( 1.299212598425197429, 0.2952755905511811885, 0.000000000000000000 ) ) ;
#33354=CARTESIAN_POINT ( 'NONE',  ( 0.1968503937007881344, 0.2952755905511811885, 0.000000000000000000 ) ) ;
#33356=CARTESIAN_POINT ( 'NONE',  ( -1.522309711286088607, 0.2306618581243847221, -0.2411417322834647770 ) ) ;
#33357=CARTESIAN_POINT ( 'NONE',  ( 0.02624671916010564918, 0.2306618581243848609, 0.2411417322834645549 ) ) ;
#33359=CARTESIAN_POINT ( 'NONE',  ( -1.587926509186350810, -0.004921259842519870586, -0.3153832671262229437 ) ) ;
#33360=CARTESIAN_POINT ( 'NONE',  ( 0.5380577427821529035, 0.05413385826771626580, -0.4176697321401330321 ) ) ;
#33361=CARTESIAN_POINT ( 'NONE',  ( 1.030183727034121421, -0.08942795157527998196, 0.3641732283464567121 ) ) ;
#33363=CARTESIAN_POINT ( 'NONE',  ( 0.5446194225721792126, -0.2845877964562159024, 0.3641732283464567677 ) ) ;
#33364=CARTESIAN_POINT ( 'NONE',  ( -1.069553805774277722, -0.6692913385826773087, -0.1292274648535924053 ) ) ;
#33366=CARTESIAN_POINT ( 'NONE',  ( 1.338582677165355062, -0.1870078740157479769, 0.4822834645669291653 ) ) ;
#33368=CARTESIAN_POINT ( 'NONE',  ( 0.5971128608923891301, 0.2952755905511810774, -0.1292274648535930714 ) ) ;
#33370=CARTESIAN_POINT ( 'NONE',  ( -0.7993346172249354842, -1.308147748527373767E-15, -0.3627985898453525704 ) ) ;
#33371=CARTESIAN_POINT ( 'NONE',  ( 0.3412073490813655186, 0.1283753931104748280, 0.1820866141732283561 ) ) ;
#33372=CARTESIAN_POINT ( 'NONE',  ( 0.6824146981627303710, -0.6046776061558807314, 0.2411417322834647770 ) ) ;
#33373=CARTESIAN_POINT ( 'NONE',  ( 1.646981627296588035, -0.2845877964562159024, 0.3641732283464567677 ) ) ;
#33374=CARTESIAN_POINT ( 'NONE',  ( -0.9120734908136475250, 0.1771653543307087630, 0.09757992244046791164 ) ) ;
#33375=CARTESIAN_POINT ( 'NONE',  ( -0.9580052493438311334, -0.4281496062992124485, 0.4176697321401328655 ) ) ;
#33376=CARTESIAN_POINT ( 'NONE',  ( -1.601049868766403650, -0.6046776061558807314, 0.2411417322834647770 ) ) ;
#33377=CARTESIAN_POINT ( 'NONE',  ( 1.108923884514436686, -0.3162353388693409650, -0.4822834645669289433 ) ) ;
#33378=CARTESIAN_POINT ( 'NONE',  ( 1.541994750656168645, 0.2952755905511810774, -0.1292274648535930714 ) ) ;
#33380=CARTESIAN_POINT ( 'NONE',  ( 0.7480314960629927956, -0.6692913385826771977, 8.415575281601705876E-17 ) ) ;
#33383=CARTESIAN_POINT ( 'NONE',  ( 1.646981627296588035, -0.3162353388693405765, 0.4822834645669290543 ) ) ;
#33384=CARTESIAN_POINT ( 'NONE',  ( 1.535433070866142558, 0.2952755905511811885, 0.000000000000000000 ) ) ;
#33385=CARTESIAN_POINT ( 'NONE',  ( -1.358267716535432434, 0.07958543189024071263, -0.2665933059059888421 ) ) ;
#33386=CARTESIAN_POINT ( 'NONE',  ( 1.266404199475066328, -0.2845877964562161244, -0.3641732283464567121 ) ) ;
#33387=CARTESIAN_POINT ( 'NONE',  ( -1.115485564304461219, -0.004921259842519870586, -0.3153832671262229437 ) ) ;
#33388=CARTESIAN_POINT ( 'NONE',  ( -0.5249343832020990641, 0.1283753931104748280, 0.1820866141732283561 ) ) ;
#33391=CARTESIAN_POINT ( 'NONE',  ( 1.069553805774278610, -0.5511811023622046335, 0.09757992244046803654 ) ) ;
#33392=CARTESIAN_POINT ( 'NONE',  ( 0.7086614173228353852, -0.1870078740157479769, 0.4822834645669291653 ) ) ;
#33393=CARTESIAN_POINT ( 'NONE',  ( 1.089238845144357537, -0.4281496062992124485, 0.4176697321401328655 ) ) ;
#33394=CARTESIAN_POINT ( 'NONE',  ( -0.01312335958005186876, 0.05413385826771626580, -0.4176697321401330321 ) ) ;
#33395=CARTESIAN_POINT ( 'NONE',  ( 0.4921259842519691285, 0.07958543189024085140, 0.2665933059059887866 ) ) ;
#33396=CARTESIAN_POINT ( 'NONE',  ( 1.305774278215223960, 0.2952755905511810774, -0.1292274648535930714 ) ) ;
#33397=CARTESIAN_POINT ( 'NONE',  ( -1.555118110236219930, -0.5400638737290845981, -0.3530559997133363437 ) ) ;
#33398=CARTESIAN_POINT ( 'NONE',  ( -0.4199475065616791736, 0.2306618581243847221, -0.2411417322834647770 ) ) ;
#33401=CARTESIAN_POINT ( 'NONE',  ( 0.2230971128608929543, 0.05413385826771626580, -0.4176697321401330321 ) ) ;
#33402=CARTESIAN_POINT ( 'NONE',  ( -0.6364829396325453192, -0.05778040916215560624, -0.4822834645669293319 ) ) ;
#33403=CARTESIAN_POINT ( 'NONE',  ( -0.09842519685039295696, 0.1660481256975883668, -0.3530559997133364547 ) ) ;
#33408=CARTESIAN_POINT ( 'NONE',  ( -1.003937007874015297, -0.4536011799217368745, -0.2665933059059886201 ) ) ;
#33410=CARTESIAN_POINT ( 'NONE',  ( -1.148293963254592542, -0.6692913385826773087, -0.1292274648535924053 ) ) ;
#33412=CARTESIAN_POINT ( 'NONE',  ( 0.5643044619422579178, 0.05413385826771666132, 0.4176697321401328100 ) ) ;
#33413=CARTESIAN_POINT ( 'NONE',  ( -0.5446194225721777693, -0.2845877964562161244, -0.3641732283464567121 ) ) ;
#33414=CARTESIAN_POINT ( 'NONE',  ( 1.423884514435696191, -0.05778040916215522460, 0.4822834645669289988 ) ) ;
#33415=CARTESIAN_POINT ( 'NONE',  ( 0.1706036745406830368, 0.05413385826771666132, 0.4176697321401328100 ) ) ;
#33419=CARTESIAN_POINT ( 'NONE',  ( 1.049868766404200349, 0.2306618581243848609, 0.2411417322834645549 ) ) ;
#33420=CARTESIAN_POINT ( 'NONE',  ( 0.6758530183727039509, 0.2952755905511810774, -0.1292274648535930714 ) ) ;
#33422=CARTESIAN_POINT ( 'NONE',  ( 0.2952755905511816326, -0.5400638737290844871, 0.3530559997133364547 ) ) ;
#33423=CARTESIAN_POINT ( 'NONE',  ( 1.450131233595801428, 0.2952755905511811885, 0.1292274648535926551 ) ) ;
#33424=CARTESIAN_POINT ( 'NONE',  ( 1.017060367454068803, -0.3162353388693405765, 0.4822834645669290543 ) ) ;
#33426=CARTESIAN_POINT ( 'NONE',  ( -0.1443569553805768291, 0.05413385826771666132, 0.4176697321401328100 ) ) ;
#33427=CARTESIAN_POINT ( 'NONE',  ( 0.8923884514435703741, 0.2306618581243848609, 0.2411417322834645549 ) ) ;
#33428=CARTESIAN_POINT ( 'NONE',  ( 0.4658792650918641698, -0.05778040916215560624, -0.4822834645669293319 ) ) ;
#33429=CARTESIAN_POINT ( 'NONE',  ( 1.141732283464567788, -0.5511811023622047445, 6.969142054262312111E-17 ) ) ;
#33430=CARTESIAN_POINT ( 'NONE',  ( -0.7742782152230965886, 0.05413385826771666132, 0.4176697321401328100 ) ) ;
#33431=CARTESIAN_POINT ( 'NONE',  ( -1.456692913385826182, -0.6692913385826771977, 8.415575281601705876E-17 ) ) ;
#33432=CARTESIAN_POINT ( 'NONE',  ( 0.5971128608923890191, -0.6692913385826771977, 0.1292274648535927661 ) ) ;
#33435=( BOUNDED_CURVE ( )  B_SPLINE_CURVE ( 1, ( #65951, #39003 ),
 .UNSPECIFIED., .F., .F. ) 
 B_SPLINE_CURVE_WITH_KNOTS ( ( 2, 2 ),
 ( 1.387778780781445676E-17, 0.001999999999999991368 ),
 .UNSPECIFIED. ) 
 CURVE ( )  GEOMETRIC_REPRESENTATION_ITEM ( )  RATIONAL_B_SPLINE_CURVE ( ( 0.9875488213027535656, 0.9875488213027535656 ) ) 
 REPRESENTATION_ITEM ( '' )  );
#33439=CARTESIAN_POINT ( 'NONE',  ( 1.522309711286089939, 0.2306618581243848609, 0.2411417322834645549 ) ) ;
#33440=CARTESIAN_POINT ( 'NONE',  ( 1.017060367454068581, -0.08942795157528024563, -0.3641732283464568787 ) ) ;
#33445=CARTESIAN_POINT ( 'NONE',  ( 1.115485564304462551, 0.05413385826771666132, 0.4176697321401328100 ) ) ;
#33447=CARTESIAN_POINT ( 'NONE',  ( -0.4724409448818890911, -0.1870078740157479769, 0.4822834645669291653 ) ) ;
#33448=CARTESIAN_POINT ( 'NONE',  ( 0.9908136482939640111, 0.2952755905511810774, -0.1292274648535930714 ) ) ;
#33450=CARTESIAN_POINT ( 'NONE',  ( -1.640419947506561060, -0.4281496062992127816, -0.4176697321401328100 ) ) ;
#33452=DIRECTION ( 'NONE',  ( -1.000000000000000000, -3.096699300667737464E-16, 1.692413147294446216E-16 ) ) ;
#33453=CARTESIAN_POINT ( 'NONE',  ( 2.795275590551181910, 1.726086921369709426, 0.000000000000000000 ) ) ;
#33454=CARTESIAN_POINT ( 'NONE',  ( -0.9251968503937002541, -0.4536011799217368745, -0.2665933059059886201 ) ) ;
#33455=CARTESIAN_POINT ( 'NONE',  ( 0.8989501312335963501, 0.2066929133858267931, 0.1054918080437490802 ) ) ;
#33456=CARTESIAN_POINT ( 'NONE',  ( 0.4068241469816281097, 0.05413385826771666132, 0.4176697321401328100 ) ) ;
#33459=CARTESIAN_POINT ( 'NONE',  ( -1.614173228346456712, 1.543375672658095610, -0.1372047244094478091 ) ) ;
#33460=CARTESIAN_POINT ( 'NONE',  ( 1.003937007874016407, -0.5400638737290844871, 0.3530559997133364547 ) ) ;
#33461=CARTESIAN_POINT ( 'NONE',  ( -1.725721784776902190, -0.05778040916215522460, 0.4822834645669289988 ) ) ;
#33463=CARTESIAN_POINT ( 'NONE',  ( -0.7742782152230965886, -0.004921259842519576551, 0.3153832671262227771 ) ) ;
#33464=CARTESIAN_POINT ( 'NONE',  ( 1.666666666666667185, 0.05413385826771666132, 0.4176697321401328100 ) ) ;
#33466=CARTESIAN_POINT ( 'NONE',  ( 0.2624671916010504757, -0.6046776061558809534, -0.2411417322834644161 ) ) ;
#33467=CARTESIAN_POINT ( 'NONE',  ( -0.8595800524934373854, -0.08942795157527998196, 0.3641732283464567121 ) ) ;
#33468=CARTESIAN_POINT ( 'NONE',  ( 0.1181102362204730916, -0.5511811023622047445, 6.969142054262312111E-17 ) ) ;
#33469=CARTESIAN_POINT ( 'NONE',  ( -0.3805774278215216522, -0.4281496062992127816, -0.4176697321401328100 ) ) ;
#33470=CARTESIAN_POINT ( 'NONE',  ( -1.108923884514435132, -0.08942795157528024563, -0.3641732283464568787 ) ) ;
#33472=CARTESIAN_POINT ( 'NONE',  ( 0.6233595800524939223, -0.3162353388693405765, 0.4822834645669290543 ) ) ;
#33474=CARTESIAN_POINT ( 'NONE',  ( -1.627296587926508442, 0.2306618581243848609, 0.2411417322834645549 ) ) ;
#33476=CARTESIAN_POINT ( 'NONE',  ( -0.7480314960629914633, 0.2952755905511811885, 0.000000000000000000 ) ) ;
#33477=CARTESIAN_POINT ( 'NONE',  ( -0.02624671916010428221, -0.5023911411419708095, 0.1820866141732285504 ) ) ;
#33478=CARTESIAN_POINT ( 'NONE',  ( -1.194225721784776262, -0.4281496062992124485, 0.4176697321401328655 ) ) ;
#33479=CARTESIAN_POINT ( 'NONE',  ( 1.023622047244095334, -0.1870078740157479769, 0.3641732283464567677 ) ) ;
#33480=CARTESIAN_POINT ( 'NONE',  ( -0.6102362204724400829, 0.07958543189024085140, 0.2665933059059887866 ) ) ;
#33481=CARTESIAN_POINT ( 'NONE',  ( -0.9514435695538050464, -0.3162353388693405765, 0.4822834645669290543 ) ) ;
#33482=CARTESIAN_POINT ( 'NONE',  ( -1.089238845144356427, 0.05413385826771666132, 0.4176697321401328100 ) ) ;
#33483=CARTESIAN_POINT ( 'NONE',  ( -1.601049868766403650, 0.2306618581243847221, -0.2411417322834647770 ) ) ;
#33486=CARTESIAN_POINT ( 'NONE',  ( 0.9514435695538062676, -0.2845877964562161244, -0.3641732283464567121 ) ) ;
#33487=CARTESIAN_POINT ( 'NONE',  ( 0.4790026246719168435, -0.3162353388693409650, -0.4822834645669289433 ) ) ;
#33488=CARTESIAN_POINT ( 'NONE',  ( -1.332020997375327642, -0.05778040916215522460, 0.4822834645669289988 ) ) ;
#33489=CARTESIAN_POINT ( 'NONE',  ( -1.476377952755905110, -0.5400638737290845981, -0.3530559997133363437 ) ) ;
#33492=CARTESIAN_POINT ( 'NONE',  ( -1.423884514435694859, -0.08942795157528024563, -0.3641732283464568787 ) ) ;
#33493=CARTESIAN_POINT ( 'NONE',  ( 0.5511811023622054106, -0.1870078740157480879, -0.4822834645669291653 ) ) ;
#33494=CARTESIAN_POINT ( 'NONE',  ( -1.266404199475064773, -0.2845877964562159024, 0.3641732283464567677 ) ) ;
#33496=CARTESIAN_POINT ( 'NONE',  ( -1.404199475065615932, 0.05413385826771666132, 0.4176697321401328100 ) ) ;
#33497=CARTESIAN_POINT ( 'NONE',  ( 0.8989501312335964611, 0.2952755905511811885, 0.1292274648535926551 ) ) ;
#33498=CARTESIAN_POINT ( 'NONE',  ( 0.6496062992125991586, -0.5400638737290845981, -0.3530559997133363437 ) ) ;
#33499=CARTESIAN_POINT ( 'NONE',  ( 1.358267716535433323, -0.5400638737290845981, -0.3530559997133363437 ) ) ;
#33504=CARTESIAN_POINT ( 'NONE',  ( 0.5118110236220478892, 0.1771653543307087630, 0.000000000000000000 ) ) ;
#33505=CARTESIAN_POINT ( 'NONE',  ( 0.1443569553805781891, -0.4281496062992124485, 0.4176697321401328655 ) ) ;
#33506=CARTESIAN_POINT ( 'NONE',  ( 1.456692913385827515, 0.2952755905511811885, 0.000000000000000000 ) ) ;
#33508=CARTESIAN_POINT ( 'NONE',  ( 0.1902887139107617975, -0.5511811023622048555, -0.09757992244046775898 ) ) ;
#33509=CARTESIAN_POINT ( 'NONE',  ( -0.7283464566929126471, -0.5400638737290844871, 0.3530559997133364547 ) ) ;
#33510=CARTESIAN_POINT ( 'NONE',  ( 1.607611548556431069, 0.2952755905511811885, 0.1292274648535926551 ) ) ;
#33511=CARTESIAN_POINT ( 'NONE',  ( 0.3805774278215230400, -0.4281496062992124485, 0.4176697321401328655 ) ) ;
#33514=ORIENTED_EDGE ( 'NONE', *, *, #82040, .F. ) ;
#33515=EDGE_LOOP ( 'NONE', ( #34985, #59531, #82567, #54018, #61967, #66798, #34882, #32270 ) ) ;
#33516=CARTESIAN_POINT ( 'NONE',  ( -1.187664041994750175, -0.05778040916215560624, -0.4822834645669293319 ) ) ;
#33517=CARTESIAN_POINT ( 'NONE',  ( -1.240157480314959759, -0.4536011799217368745, -0.2665933059059886201 ) ) ;
#33518=CARTESIAN_POINT ( 'NONE',  ( -1.056430446194224881, -0.6692913385826771977, 0.1292274648535927661 ) ) ;
#33520=CARTESIAN_POINT ( 'NONE',  ( -0.4621018179204942067, -4.378520898609941727E-15, 0.4281989832122470863 ) ) ;
#33521=CARTESIAN_POINT ( 'NONE',  ( 1.574803149606299746, -0.1870078740157480879, -0.4822834645669291653 ) ) ;
#33522=CARTESIAN_POINT ( 'NONE',  ( -1.227034120734907585, 0.2952755905511811885, 0.1292274648535926551 ) ) ;
#33523=CARTESIAN_POINT ( 'NONE',  ( 0.4199475065616803948, -0.6046776061558809534, -0.2411417322834644161 ) ) ;
#33524=CARTESIAN_POINT ( 'NONE',  ( -1.325459317585300889, 0.05413385826771666132, 0.4176697321401328100 ) ) ;
#33526=CARTESIAN_POINT ( 'NONE',  ( 0.8267716535433077274, 0.2952755905511811885, 0.000000000000000000 ) ) ;
#33528=CARTESIAN_POINT ( 'NONE',  ( -1.135170603674539924, 0.1771653543307087075, -0.09757992244046823083 ) ) ;
#33529=EDGE_LOOP ( 'NONE', ( #7953, #15431, #72647, #52365 ) ) ;
#33532=CARTESIAN_POINT ( 'NONE',  ( -0.6402603868039137280, -5.134928753749862370E-15, -0.4281989832122467532 ) ) ;
#33533=CARTESIAN_POINT ( 'NONE',  ( -0.9842519685039365918, -0.6692913385826771977, 8.415575281601705876E-17 ) ) ;
#33534=CARTESIAN_POINT ( 'NONE',  ( -1.259842519685038686, -0.1870078740157480879, -0.4822834645669291653 ) ) ;
#33536=CARTESIAN_POINT ( 'NONE',  ( -1.469816272965878357, -0.6046776061558809534, -0.2411417322834644161 ) ) ;
#33537=CARTESIAN_POINT ( 'NONE',  ( -1.699475065616797398, 0.2952755905511811885, 0.1292274648535926551 ) ) ;
#33538=CARTESIAN_POINT ( 'NONE',  ( -1.404199475065615932, -0.4281496062992127816, -0.4176697321401328100 ) ) ;
#33539=CARTESIAN_POINT ( 'NONE',  ( -1.586052503253846169, 1.850393700787402729, 0.1653254495020583248 ) ) ;
#33541=CARTESIAN_POINT ( 'NONE',  ( -0.03937007874015669567, 0.1771653543307087630, 0.000000000000000000 ) ) ;
#33544=CARTESIAN_POINT ( 'NONE',  ( -0.2296587926509179312, -0.2845877964562161244, -0.3641732283464567121 ) ) ;
#33545=CARTESIAN_POINT ( 'NONE',  ( -0.7874015748031489847, -0.1870078740157480879, -0.4822834645669291653 ) ) ;
#33546=CARTESIAN_POINT ( 'NONE',  ( 1.128608923884514947, 0.2306618581243848609, 0.2411417322834645549 ) ) ;
#33547=CARTESIAN_POINT ( 'NONE',  ( -0.8398950131233585692, 0.2306618581243848609, 0.2411417322834645549 ) ) ;
#33548=ORIENTED_EDGE ( 'NONE', *, *, #405, .F. ) ;
#33550=CARTESIAN_POINT ( 'NONE',  ( -0.8267716535433065062, 0.2952755905511811885, 0.000000000000000000 ) ) ;
#33551=CARTESIAN_POINT ( 'NONE',  ( 0.7020997375328090762, -0.05778040916215560624, -0.4822834645669293319 ) ) ;
#33552=CARTESIAN_POINT ( 'NONE',  ( -1.535433070866141225, 0.1771653543307087630, 0.000000000000000000 ) ) ;
#33557=CARTESIAN_POINT ( 'NONE',  ( -0.2821522309711278487, -0.6692913385826773087, -0.1292274648535924053 ) ) ;
#33558=CARTESIAN_POINT ( 'NONE',  ( -1.286089238845143479, 0.1283753931104746893, -0.1820866141732285504 ) ) ;
#33559=CARTESIAN_POINT ( 'NONE',  ( -0.8070866141732276899, -0.5400638737290844871, 0.3530559997133364547 ) ) ;
#33561=CARTESIAN_POINT ( 'NONE',  ( -1.469816272965878357, -0.6046776061558809534, -0.2411417322834644161 ) ) ;
#33562=CARTESIAN_POINT ( 'NONE',  ( 0.4330708661417324024, 2.793565526369266028, 0.000000000000000000 ) ) ;
#33563=CARTESIAN_POINT ( 'NONE',  ( -1.568241469816272105, -0.05778040916215522460, 0.4822834645669289988 ) ) ;
#33564=CARTESIAN_POINT ( 'NONE',  ( -0.4396325459317579898, 0.2952755905511811885, 0.1292274648535926551 ) ) ;
#33566=CARTESIAN_POINT ( 'NONE',  ( 0.5708661417322841158, -0.4536011799217368745, -0.2665933059059886201 ) ) ;
#33568=CARTESIAN_POINT ( 'NONE',  ( 0.2624671916010504757, 0.1283753931104748280, 0.1820866141732283561 ) ) ;
#33569=CARTESIAN_POINT ( 'NONE',  ( 1.253280839895013710, -0.2845877964562159024, 0.3641732283464567677 ) ) ;
#33570=CARTESIAN_POINT ( 'NONE',  ( 1.141732283464567566, 0.2952755905511811885, 0.000000000000000000 ) ) ;
#33571=CARTESIAN_POINT ( 'NONE',  ( 0.2559055118110243332, 0.07958543189024085140, 0.2665933059059887866 ) ) ;
#33573=CARTESIAN_POINT ( 'NONE',  ( -1.463254593175852492, 0.2952755905511811885, 0.1292274648535926551 ) ) ;
#33574=CARTESIAN_POINT ( 'NONE',  ( 0.01968503937007930540, 0.07958543189024085140, 0.2665933059059887866 ) ) ;
#33576=CARTESIAN_POINT ( 'NONE',  ( -0.5511811023622038563, -0.1870078740157479769, 0.3641732283464567677 ) ) ;
#33578=CARTESIAN_POINT ( 'NONE',  ( -0.3018372703412066094, -0.4281496062992127816, -0.4176697321401328100 ) ) ;
#33579=DIRECTION ( 'NONE',  ( 0.000000000000000000, 0.000000000000000000, -1.000000000000000000 ) ) ;
#33580=CARTESIAN_POINT ( 'NONE',  ( 1.056430446194226436, -0.5511811023622048555, -0.09757992244046775898 ) ) ;
#33581=CARTESIAN_POINT ( 'NONE',  ( -0.2034120734908131112, -0.5511811023622048555, -0.09757992244046775898 ) ) ;
#33582=CARTESIAN_POINT ( 'NONE',  ( -0.2559055118110227234, -0.5400638737290844871, 0.3530559997133364547 ) ) ;
#33584=CARTESIAN_POINT ( 'NONE',  ( -0.9317585301837263412, -0.3690944881889765550, -0.3153832671262227771 ) ) ;
#33586=CARTESIAN_POINT ( 'NONE',  ( 0.7611548556430454138, 0.2306618581243847221, -0.2411417322834647770 ) ) ;
#33587=CARTESIAN_POINT ( 'NONE',  ( -0.8989501312335946848, -0.6692913385826771977, 0.1292274648535927661 ) ) ;
#33590=CARTESIAN_POINT ( 'NONE',  ( 0.04593175853018440641, 0.1771653543307087075, -0.09757992244046823083 ) ) ;
#33591=CARTESIAN_POINT ( 'NONE',  ( -0.7742782152230962556, -0.4281496062992127816, -0.4176697321401328100 ) ) ;
#33592=CARTESIAN_POINT ( 'NONE',  ( -1.108923884514435132, -0.05778040916215560624, -0.4822834645669293319 ) ) ;
#33593=CARTESIAN_POINT ( 'NONE',  ( -1.391076115485563314, -0.5023911411419708095, -0.1820866141732282451 ) ) ;
#33594=CARTESIAN_POINT ( 'NONE',  ( 1.620734908136483465, -0.6692913385826771977, 0.1292274648535927661 ) ) ;
#33595=CARTESIAN_POINT ( 'NONE',  ( -1.076115485564303809, -0.5023911411419708095, -0.1820866141732282451 ) ) ;
#33596=CARTESIAN_POINT ( 'NONE',  ( -0.7217847769028863381, 0.009842519685039144428, -0.3409548833797004797 ) ) ;
#33597=CARTESIAN_POINT ( 'NONE',  ( 0.7414698162729663755, -0.6692913385826773087, -0.1292274648535924053 ) ) ;
#33603=CARTESIAN_POINT ( 'NONE',  ( 1.489501312335958172, -0.08942795157528024563, -0.3641732283464568787 ) ) ;
#33604=CARTESIAN_POINT ( 'NONE',  ( -1.305774278215222184, -0.6692913385826773087, -0.1292274648535924053 ) ) ;
#33605=CARTESIAN_POINT ( 'NONE',  ( 1.174540682414699111, -0.05778040916215560624, -0.4822834645669293319 ) ) ;
#33607=CARTESIAN_POINT ( 'NONE',  ( 1.515748031496063408, 0.07958543189024085140, 0.2665933059059887866 ) ) ;
#33609=CARTESIAN_POINT ( 'NONE',  ( 0.7283464566929143125, 0.1660481256975885056, 0.3530559997133364547 ) ) ;
#33610=CARTESIAN_POINT ( 'NONE',  ( -0.3608923884514428360, 0.2952755905511811885, 0.1292274648535926551 ) ) ;
#33613=CARTESIAN_POINT ( 'NONE',  ( 0.6167979002624678353, -0.3690944881889763329, 0.3153832671262228327 ) ) ;
#33615=ORIENTED_EDGE ( 'NONE', *, *, #54690, .T. ) ;
#33617=VERTEX_POINT ( 'NONE', #34272 ) ;
#33618=CARTESIAN_POINT ( 'NONE',  ( 0.01312335958005323398, 0.05413385826771666132, 0.4176697321401328100 ) ) ;
#33619=CARTESIAN_POINT ( 'NONE',  ( 1.253280839895013710, -0.3162353388693405765, 0.4822834645669290543 ) ) ;
#33620=CARTESIAN_POINT ( 'NONE',  ( 0.2493438320209980519, 0.05413385826771666132, 0.4176697321401328100 ) ) ;
#33621=CARTESIAN_POINT ( 'NONE',  ( -0.1640419947506553400, -0.08942795157528024563, -0.3641732283464568787 ) ) ;
#33622=CARTESIAN_POINT ( 'NONE',  ( 1.220472440944882608, 0.2952755905511811885, 0.000000000000000000 ) ) ;
#33623=CARTESIAN_POINT ( 'NONE',  ( -0.5971128608923877978, -0.6692913385826773087, -0.1292274648535924053 ) ) ;
#33624=CARTESIAN_POINT ( 'NONE',  ( -0.1377952755905504645, 0.1660481256975885056, 0.3530559997133364547 ) ) ;
#33625=CARTESIAN_POINT ( 'NONE',  ( -1.587926509186350810, 0.05413385826771626580, -0.4176697321401330321 ) ) ;
#33626=CARTESIAN_POINT ( 'NONE',  ( 1.450131233595801428, 0.2952755905511811885, 0.1292274648535926551 ) ) ;
#33627=CARTESIAN_POINT ( 'NONE',  ( 1.181102362204725198, -0.1870078740157479769, 0.4822834645669291653 ) ) ;
#33628=EDGE_CURVE ( 'NONE', #2588, #19450, #72120, .T. ) ;
#33630=CARTESIAN_POINT ( 'NONE',  ( 0.4855643044619430415, -0.3690944881889765550, -0.3153832671262227771 ) ) ;
#33633=ORIENTED_EDGE ( 'NONE', *, *, #36412, .F. ) ;
#33634=CARTESIAN_POINT ( 'NONE',  ( -0.5118110236220466680, -0.5511811023622047445, 6.969142054262312111E-17 ) ) ;
#33635=CARTESIAN_POINT ( 'NONE',  ( -0.2427821522309703550, -0.3162353388693405765, 0.4822834645669290543 ) ) ;
#33637=CARTESIAN_POINT ( 'NONE',  ( -0.1443569553805768291, 0.05413385826771666132, 0.4176697321401328100 ) ) ;
#33638=CARTESIAN_POINT ( 'NONE',  ( -0.06561679790026180015, -0.4281496062992127816, -0.4176697321401328100 ) ) ;
#33640=CARTESIAN_POINT ( 'NONE',  ( -0.9251968503937002541, -0.5400638737290845981, -0.3530559997133363437 ) ) ;
#33641=CARTESIAN_POINT ( 'NONE',  ( -0.9251968503937002541, 0.1660481256975885056, 0.3530559997133364547 ) ) ;
#33642=CARTESIAN_POINT ( 'NONE',  ( 1.161417322834646493, -0.4536011799217367080, 0.2665933059059888421 ) ) ;
#33643=CARTESIAN_POINT ( 'NONE',  ( -1.555118110236219930, -0.5400638737290845981, -0.3530559997133363437 ) ) ;
#33644=CARTESIAN_POINT ( 'NONE',  ( -0.1467811222005243055, -2.624320362099288585E-15, 0.4118477457933001906 ) ) ;
#33645=CARTESIAN_POINT ( 'NONE',  ( 0.8792650918635177559, -0.3690944881889765550, -0.3153832671262227771 ) ) ;
#33646=CARTESIAN_POINT ( 'NONE',  ( 0.4986876640419954376, -0.6046776061558809534, -0.2411417322834644161 ) ) ;
#33647=CARTESIAN_POINT ( 'NONE',  ( 0.3608923884514443348, -0.6692913385826771977, 0.1292274648535927661 ) ) ;
#33649=CARTESIAN_POINT ( 'NONE',  ( -1.646981627296586703, -0.3162353388693409650, -0.4822834645669289433 ) ) ;
#33652=CARTESIAN_POINT ( 'NONE',  ( -0.7152230971128602510, -0.05778040916215560624, -0.4822834645669293319 ) ) ;
#33655=CARTESIAN_POINT ( 'NONE',  ( -1.213910761154854745, -0.5511811023622046335, 0.09757992244046803654 ) ) ;
#33656=CARTESIAN_POINT ( 'NONE',  ( 0.9711286089238851948, 0.2306618581243848609, 0.2411417322834645549 ) ) ;
#33657=CARTESIAN_POINT ( 'NONE',  ( 0.9514435695538062676, -0.3162353388693409650, -0.4822834645669289433 ) ) ;
#33658=CARTESIAN_POINT ( 'NONE',  ( -0.1246719160104980823, -0.5511811023622048555, -0.09757992244046775898 ) ) ;
#33659=CARTESIAN_POINT ( 'NONE',  ( 0.5511811023622054106, -0.1870078740157480879, -0.4822834645669291653 ) ) ;
#33661=CARTESIAN_POINT ( 'NONE',  ( 0.07874015748031558404, -0.1870078740157479769, 0.3641732283464567677 ) ) ;
#33662=CARTESIAN_POINT ( 'NONE',  ( -0.05905511811023545637, -0.5400638737290845981, -0.3530559997133363437 ) ) ;
#33665=CARTESIAN_POINT ( 'NONE',  ( -1.679790026246718693, 0.2306618581243847221, -0.2411417322834647770 ) ) ;
#33666=CARTESIAN_POINT ( 'NONE',  ( 0.6167979002624678353, -0.3690944881889763329, 0.3153832671262228327 ) ) ;
#33667=CARTESIAN_POINT ( 'NONE',  ( 1.568241469816273659, -0.08942795157528024563, -0.3641732283464568787 ) ) ;
#33668=CARTESIAN_POINT ( 'NONE',  ( -0.5708661417322828946, 0.1660481256975883668, -0.3530559997133364547 ) ) ;
#33669=CARTESIAN_POINT ( 'NONE',  ( -0.1902887139107604098, 0.1771653543307087075, -0.09757992244046823083 ) ) ;
#33671=CARTESIAN_POINT ( 'NONE',  ( -0.7677165354330699465, 0.1660481256975885056, 0.3530559997133364547 ) ) ;
#33672=CARTESIAN_POINT ( 'NONE',  ( -0.8005249343832011588, 0.05413385826771626580, -0.4176697321401330321 ) ) ;
#33673=CARTESIAN_POINT ( 'NONE',  ( -0.1312335958005241554, -0.6046776061558809534, -0.2411417322834644161 ) ) ;
#33676=CARTESIAN_POINT ( 'NONE',  ( -1.666666666666665853, -0.004921259842519870586, -0.3153832671262229437 ) ) ;
#33677=CARTESIAN_POINT ( 'NONE',  ( 0.5577427821522316087, -0.08942795157527998196, 0.3641732283464567121 ) ) ;
#33678=CARTESIAN_POINT ( 'NONE',  ( 1.404199475065617264, -0.4281496062992124485, 0.4176697321401328655 ) ) ;
#33679=CARTESIAN_POINT ( 'NONE',  ( -0.7020997375328076329, -0.2845877964562161244, -0.3641732283464567121 ) ) ;
#33680=CARTESIAN_POINT ( 'NONE',  ( -1.135170603674539924, -0.5511811023622046335, 0.09757992244046803654 ) ) ;
#33681=CARTESIAN_POINT ( 'NONE',  ( -0.8070866141732276899, 0.1660481256975883668, -0.3530559997133364547 ) ) ;
#33682=CARTESIAN_POINT ( 'NONE',  ( -0.6758530183727028406, -0.6692913385826773087, -0.1292274648535924053 ) ) ;
#33683=CARTESIAN_POINT ( 'NONE',  ( 0.4461942257217856311, 0.1283753931104746893, -0.1820866141732285504 ) ) ;
#33685=CARTESIAN_POINT ( 'NONE',  ( 1.095800524934383846, -0.2845877964562159024, 0.3641732283464567677 ) ) ;
#33686=EDGE_CURVE ( 'NONE', #30580, #81796, #43913, .T. ) ;
#33687=CARTESIAN_POINT ( 'NONE',  ( 0.3412073490813655186, -0.6046776061558809534, -0.2411417322834644161 ) ) ;
#33689=CARTESIAN_POINT ( 'NONE',  ( -0.5380577427821514602, -0.4281496062992127816, -0.4176697321401328100 ) ) ;
#33691=CARTESIAN_POINT ( 'NONE',  ( -1.706036745406823485, 0.2306618581243848609, 0.2411417322834645549 ) ) ;
#33692=CARTESIAN_POINT ( 'NONE',  ( 0.5052493438320218022, -0.6692913385826773087, -0.1292274648535924053 ) ) ;
#33693=CARTESIAN_POINT ( 'NONE',  ( 0.2559055118110243332, 0.1660481256975885056, 0.3530559997133364547 ) ) ;
#33694=CARTESIAN_POINT ( 'NONE',  ( 0.1377952755905518800, 0.07958543189024071263, -0.2665933059059888421 ) ) ;
#33696=CARTESIAN_POINT ( 'NONE',  ( -0.1377952755905504645, -0.4536011799217368745, -0.2665933059059886201 ) ) ;
#33698=CARTESIAN_POINT ( 'NONE',  ( 0.8989501312335964611, 0.2952755905511811885, 0.1292274648535926551 ) ) ;
#33699=CARTESIAN_POINT ( 'NONE',  ( -0.6167979002624665030, -0.004921259842519576551, 0.3153832671262227771 ) ) ;
#33700=CARTESIAN_POINT ( 'NONE',  ( -1.069553805774277722, -0.6692913385826773087, -0.1292274648535924053 ) ) ;
#33703=CARTESIAN_POINT ( 'NONE',  ( -1.233595800524933894, -0.6046776061558809534, -0.2411417322834644161 ) ) ;
#33704=CARTESIAN_POINT ( 'NONE',  ( -1.062992125984250968, 0.1771653543307087630, 0.000000000000000000 ) ) ;
#33705=CARTESIAN_POINT ( 'NONE',  ( 0.01968503937007930540, 0.1660481256975885056, 0.3530559997133364547 ) ) ;
#33706=CARTESIAN_POINT ( 'NONE',  ( -1.555118110236219930, 0.1660481256975885056, 0.3530559997133364547 ) ) ;
#33707=CARTESIAN_POINT ( 'NONE',  ( -0.7611548556430438595, -0.6046776061558809534, -0.2411417322834644161 ) ) ;
#33709=CARTESIAN_POINT ( 'NONE',  ( 1.686351706036745890, 0.2952755905511811885, 0.1292274648535926551 ) ) ;
#33710=CARTESIAN_POINT ( 'NONE',  ( 0.7939632545931766261, -0.05778040916215522460, 0.4822834645669289988 ) ) ;
#33711=CARTESIAN_POINT ( 'NONE',  ( 0.7742782152230979209, 0.05413385826771626580, -0.4176697321401330321 ) ) ;
#33714=CARTESIAN_POINT ( 'NONE',  ( -1.259842519685038686, -0.1870078740157479769, 0.4822834645669291653 ) ) ;
#33716=ORIENTED_EDGE ( 'NONE', *, *, #57864, .T. ) ;
#33717=CARTESIAN_POINT ( 'NONE',  ( -0.3412073490813641308, 0.1283753931104746893, -0.1820866141732285504 ) ) ;
#33719=ORIENTED_EDGE ( 'NONE', *, *, #82527, .T. ) ;
#33720=CARTESIAN_POINT ( 'NONE',  ( 0.2362204724409456558, -0.1870078740157480879, -0.4822834645669291653 ) ) ;
#33721=CARTESIAN_POINT ( 'NONE',  ( 0.06561679790026316017, 0.05413385826771626580, -0.4176697321401330321 ) ) ;
#33722=CARTESIAN_POINT ( 'NONE',  ( -0.4921259842519677963, 0.1660481256975883668, -0.3530559997133364547 ) ) ;
#33723=CARTESIAN_POINT ( 'NONE',  ( 1.489501312335958172, -0.3162353388693405765, 0.4822834645669290543 ) ) ;
#33724=CARTESIAN_POINT ( 'NONE',  ( -1.017060367454067249, -0.08942795157527998196, 0.3641732283464567121 ) ) ;
#33726=CARTESIAN_POINT ( 'NONE',  ( 0.8989501312335964611, 0.2952755905511811885, 0.1292274648535926551 ) ) ;
#33727=CARTESIAN_POINT ( 'NONE',  ( 0.6233595800524939223, -0.2845877964562159024, 0.3641732283464567677 ) ) ;
#33729=CARTESIAN_POINT ( 'NONE',  ( -0.2624671916010490880, -0.6046776061558807314, 0.2411417322834647770 ) ) ;
#33731=CARTESIAN_POINT ( 'NONE',  ( -0.9514435695538050464, -0.05778040916215560624, -0.4822834645669293319 ) ) ;
#33732=CARTESIAN_POINT ( 'NONE',  ( -1.719160104986876103, -0.004921259842519576551, 0.3153832671262227771 ) ) ;
#33734=CARTESIAN_POINT ( 'NONE',  ( 1.266404199475066328, -0.3162353388693409650, -0.4822834645669289433 ) ) ;
#33735=CARTESIAN_POINT ( 'NONE',  ( 1.627296587926509996, -0.5023911411419708095, 0.1820866141732285504 ) ) ;
#33738=CARTESIAN_POINT ( 'NONE',  ( -0.01312335958005186876, 0.05413385826771626580, -0.4176697321401330321 ) ) ;
#33739=VERTEX_POINT ( 'NONE', #56507 ) ;
#33740=CARTESIAN_POINT ( 'NONE',  ( -1.266404199475064773, -0.3162353388693405765, 0.4822834645669290543 ) ) ;
#33741=CARTESIAN_POINT ( 'NONE',  ( 1.279527559055118724, 0.1660481256975885056, 0.3530559997133364547 ) ) ;
#33742=CARTESIAN_POINT ( 'NONE',  ( 1.351706036745407458, -0.4281496062992127816, -0.4176697321401328100 ) ) ;
#33743=CARTESIAN_POINT ( 'NONE',  ( 0.4658792650918640033, -0.3162353388693405765, 0.4822834645669290543 ) ) ;
#33744=CARTESIAN_POINT ( 'NONE',  ( -0.5183727034120726440, 0.2952755905511811885, 0.1292274648535926551 ) ) ;
#33746=CARTESIAN_POINT ( 'NONE',  ( -1.292650918635170010, -0.6692913385826771977, 0.1292274648535927661 ) ) ;
#33747=CARTESIAN_POINT ( 'NONE',  ( -0.5708661417322825615, -0.5400638737290844871, 0.3530559997133364547 ) ) ;
#33748=CARTESIAN_POINT ( 'NONE',  ( -0.5052493438320203589, 0.1771653543307087075, -0.09757992244046823083 ) ) ;
#33749=CARTESIAN_POINT ( 'NONE',  ( -1.603475055217291612, 0.7166759647713523140, 0.04573490813648251746 ) ) ;
#33751=CARTESIAN_POINT ( 'NONE',  ( -0.5839895013123351797, 0.2952755905511810774, -0.1292274648535930714 ) ) ;
#33753=CARTESIAN_POINT ( 'NONE',  ( 0.6627296587926515548, 0.2952755905511811885, 0.1292274648535926551 ) ) ;
#33755=CARTESIAN_POINT ( 'NONE',  ( -0.1443569553805765515, -0.4281496062992127816, -0.4176697321401328100 ) ) ;
#33756=CARTESIAN_POINT ( 'NONE',  ( -0.4199475065616791736, 0.1283753931104746893, -0.1820866141732285504 ) ) ;
#33757=CARTESIAN_POINT ( 'NONE',  ( 0.9317585301837276734, -0.004921259842519870586, -0.3153832671262229437 ) ) ;
#33758=CARTESIAN_POINT ( 'NONE',  ( -0.9251968503937002541, 0.1012011053420777407, 0.2882089793578257453 ) ) ;
#33760=CARTESIAN_POINT ( 'NONE',  ( 1.345144356955381593, -0.08942795157527998196, 0.3641732283464567121 ) ) ;
#33762=CARTESIAN_POINT ( 'NONE',  ( 1.423884514435696191, -0.05778040916215522460, 0.4822834645669289988 ) ) ;
#33764=CARTESIAN_POINT ( 'NONE',  ( 0.2034120734908142214, 0.2952755905511810774, -0.1292274648535930714 ) ) ;
#33766=CARTESIAN_POINT ( 'NONE',  ( -1.607611548556429737, -0.6692913385826771977, 0.1292274648535927661 ) ) ;
#33767=CARTESIAN_POINT ( 'NONE',  ( -0.01968503937007793844, -0.5400638737290844871, 0.3530559997133364547 ) ) ;
#33770=CARTESIAN_POINT ( 'NONE',  ( -1.561679790026246017, -0.3690944881889765550, -0.3153832671262227771 ) ) ;
#33771=CARTESIAN_POINT ( 'NONE',  ( 0.4133858267716541968, -0.5400638737290845981, -0.3530559997133363437 ) ) ;
#33772=CARTESIAN_POINT ( 'NONE',  ( 0.8267716535433078384, -0.5511811023622047445, 6.969142054262312111E-17 ) ) ;
#33774=CARTESIAN_POINT ( 'NONE',  ( 0.4527559055118117182, 0.07958543189024071263, -0.2665933059059888421 ) ) ;
#33775=CARTESIAN_POINT ( 'NONE',  ( -1.417322834645668772, -0.1870078740157480879, -0.4822834645669291653 ) ) ;
#33777=CARTESIAN_POINT ( 'NONE',  ( 1.181102362204725198, -0.1870078740157479769, 0.4822834645669291653 ) ) ;
#33779=CARTESIAN_POINT ( 'NONE',  ( 0.4724409448818904789, -0.1870078740157480879, -0.4822834645669291653 ) ) ;
#33781=CARTESIAN_POINT ( 'NONE',  ( -0.3273801728231969244, -2.609869883881465018E-15, -0.3464511005275220379 ) ) ;
#33782=CARTESIAN_POINT ( 'NONE',  ( 0.3674540682414705883, 0.1283753931104746893, -0.1820866141732285504 ) ) ;
#33783=CARTESIAN_POINT ( 'NONE',  ( 0.4002624671916016896, -0.05778040916215522460, 0.4822834645669289988 ) ) ;
#33785=CARTESIAN_POINT ( 'NONE',  ( -1.082677165354329896, 0.07958543189024085140, 0.2665933059059887866 ) ) ;
#33786=CARTESIAN_POINT ( 'NONE',  ( -0.8858267716535425107, 0.1660481256975883668, -0.3530559997133364547 ) ) ;
#33787=CARTESIAN_POINT ( 'NONE',  ( 1.614173228346457378, 0.1771653543307087630, 0.000000000000000000 ) ) ;
#33789=CARTESIAN_POINT ( 'NONE',  ( 0.7414698162729663755, 0.2952755905511811885, 0.1292274648535926551 ) ) ;
#33790=CARTESIAN_POINT ( 'NONE',  ( -1.633858267716534529, 0.07958543189024085140, 0.2665933059059887866 ) ) ;
#33792=CARTESIAN_POINT ( 'NONE',  ( 0.6824146981627303710, 0.2306618581243847221, -0.2411417322834647770 ) ) ;
#33794=CARTESIAN_POINT ( 'NONE',  ( 1.574803149606299746, -0.1870078740157480879, -0.4822834645669291653 ) ) ;
#33795=CARTESIAN_POINT ( 'NONE',  ( 1.528871391076116026, 0.2952755905511811885, 0.1292274648535926551 ) ) ;
#33796=CARTESIAN_POINT ( 'NONE',  ( -1.653543307086613234, -0.1870078740157480601, -0.3641732283464567677 ) ) ;
#33797=CARTESIAN_POINT ( 'NONE',  ( 1.017060367454068803, -0.2845877964562159024, 0.3641732283464567677 ) ) ;
#33798=CARTESIAN_POINT ( 'NONE',  ( -1.351706036745406347, -0.3690944881889763329, 0.3153832671262228327 ) ) ;
#33799=CARTESIAN_POINT ( 'NONE',  ( -0.6692913385826764205, 0.1771653543307087630, 0.000000000000000000 ) ) ;
#33801=CARTESIAN_POINT ( 'NONE',  ( 0.4527559055118117182, -0.4536011799217367080, 0.2665933059059888421 ) ) ;
#33802=CARTESIAN_POINT ( 'NONE',  ( 0.4527559055118117182, 0.1660481256975883668, -0.3530559997133364547 ) ) ;
#33803=CARTESIAN_POINT ( 'NONE',  ( 1.174540682414699111, -0.05778040916215560624, -0.4822834645669293319 ) ) ;
#33804=CARTESIAN_POINT ( 'NONE',  ( -0.1246719160104980823, -0.6692913385826773087, -0.1292274648535924053 ) ) ;
#33805=CARTESIAN_POINT ( 'NONE',  ( 0.2034120734908142214, 0.1771653543307087075, -0.09757992244046823083 ) ) ;
#33806=CARTESIAN_POINT ( 'NONE',  ( 1.299212598425197429, 0.2952755905511811885, 0.000000000000000000 ) ) ;
#33808=CARTESIAN_POINT ( 'NONE',  ( -0.7742782152230965886, 0.05413385826771666132, 0.4176697321401328100 ) ) ;
#33810=CARTESIAN_POINT ( 'NONE',  ( 0.02624671916010564918, 0.1539470093639523085, 0.1968503937007873850 ) ) ;
#33811=CARTESIAN_POINT ( 'NONE',  ( -0.02624671916010428221, -0.6046776061558807314, 0.2411417322834647770 ) ) ;
#33812=CARTESIAN_POINT ( 'NONE',  ( -0.9580052493438311334, 0.05413385826771626580, -0.4176697321401330321 ) ) ;
#33813=CARTESIAN_POINT ( 'NONE',  ( -0.1049868766404193215, 0.2306618581243847221, -0.2411417322834647770 ) ) ;
#33818=CARTESIAN_POINT ( 'NONE',  ( -1.017060367454067249, -0.2845877964562161244, -0.3641732283464567121 ) ) ;
#33820=CARTESIAN_POINT ( 'NONE',  ( -1.633858267716534529, -0.5400638737290845981, -0.3530559997133363437 ) ) ;
#33822=CARTESIAN_POINT ( 'NONE',  ( 0.6102362204724416372, 0.1660481256975883668, -0.3530559997133364547 ) ) ;
#33823=CARTESIAN_POINT ( 'NONE',  ( -0.4593175853018366950, -0.004921259842519576551, 0.3153832671262227771 ) ) ;
#33824=CARTESIAN_POINT ( 'NONE',  ( 0.7545931758530188826, -0.6692913385826771977, 0.1292274648535927661 ) ) ;
#33825=CARTESIAN_POINT ( 'NONE',  ( 0.4396325459317590445, -0.6692913385826771977, 0.1292274648535927661 ) ) ;
#33829=CARTESIAN_POINT ( 'NONE',  ( 1.174540682414699111, -0.3162353388693405765, 0.4822834645669290543 ) ) ;
#33830=CARTESIAN_POINT ( 'NONE',  ( 0.006561679790026889343, -0.05778040916215522460, 0.4822834645669289988 ) ) ;
#33831=CARTESIAN_POINT ( 'NONE',  ( 1.430446194225722500, 0.05413385826771666132, 0.4176697321401328100 ) ) ;
#33832=CARTESIAN_POINT ( 'NONE',  ( 0.7020997375328090762, -0.3162353388693405765, 0.4822834645669290543 ) ) ;
#33834=CARTESIAN_POINT ( 'NONE',  ( -0.05249343832020938322, -0.6046776061558809534, -0.2411417322834644161 ) ) ;
#33835=CARTESIAN_POINT ( 'NONE',  ( 0.5643044619422579178, 0.05413385826771666132, 0.4176697321401328100 ) ) ;
#33836=CARTESIAN_POINT ( 'NONE',  ( -0.2099737532808391705, 0.2306618581243848609, 0.2411417322834645549 ) ) ;
#33837=CARTESIAN_POINT ( 'NONE',  ( 1.154855643044620184, -0.5023911411419708095, 0.1820866141732285504 ) ) ;
#33838=CARTESIAN_POINT ( 'NONE',  ( -1.253280839895012377, -0.05778040916215522460, 0.4822834645669289988 ) ) ;
#33839=CARTESIAN_POINT ( 'NONE',  ( -1.502624671916009680, -0.05778040916215560624, -0.4822834645669293319 ) ) ;
#33841=CARTESIAN_POINT ( 'NONE',  ( 0.6758530183727039509, 0.2952755905511810774, -0.1292274648535930714 ) ) ;
#33844=ORIENTED_EDGE ( 'NONE', *, *, #63059, .T. ) ;
#33846=ORIENTED_EDGE ( 'NONE', *, *, #37456, .F. ) ;
#33847=CARTESIAN_POINT ( 'NONE',  ( 1.286089238845145033, -0.6046776061558809534, -0.2411417322834644161 ) ) ;
#33848=CARTESIAN_POINT ( 'NONE',  ( 0.9973753280839902091, 0.1283753931104746893, -0.1820866141732285504 ) ) ;
#33854=CARTESIAN_POINT ( 'NONE',  ( 1.371391076115485719, -0.6692913385826773087, -0.1292274648535924053 ) ) ;
#33855=CARTESIAN_POINT ( 'NONE',  ( -1.574803149606298192, -0.1870078740157480879, -0.4822834645669291653 ) ) ;
#33856=CARTESIAN_POINT ( 'NONE',  ( -0.5052493438320203589, -0.6692913385826771977, 0.1292274648535927661 ) ) ;
#33857=CARTESIAN_POINT ( 'NONE',  ( 0.9317585301837276734, -0.4281496062992124485, 0.4176697321401328655 ) ) ;
#33858=ORIENTED_EDGE ( 'NONE', *, *, #63918, .T. ) ;
#33859=CARTESIAN_POINT ( 'NONE',  ( -1.561679790026246017, 0.05413385826771666132, 0.4176697321401328100 ) ) ;
#33860=CARTESIAN_POINT ( 'NONE',  ( -0.09115970038225217065, 2.409604939980833412E-17, -0.3464511005275205946 ) ) ;
#33862=CARTESIAN_POINT ( 'NONE',  ( 1.686351706036745890, 0.1771653543307087630, 0.09757992244046791164 ) ) ;
#33863=CARTESIAN_POINT ( 'NONE',  ( -1.614173228346457378, 1.881821177735609085, 0.1372047244094476981 ) ) ;
#33864=CARTESIAN_POINT ( 'NONE',  ( -0.9908136482939626788, 0.1771653543307087630, 0.09757992244046791164 ) ) ;
#33865=CARTESIAN_POINT ( 'NONE',  ( -1.587926509186350810, 0.05413385826771626580, -0.4176697321401330321 ) ) ;
#33866=CARTESIAN_POINT ( 'NONE',  ( 0.8005249343832028242, -0.4281496062992127816, -0.4176697321401328100 ) ) ;
#33867=ORIENTED_EDGE ( 'NONE', *, *, #78524, .T. ) ;
#33868=CARTESIAN_POINT ( 'NONE',  ( 1.509186351706037543, 0.05413385826771666132, 0.4176697321401328100 ) ) ;
#33869=CARTESIAN_POINT ( 'NONE',  ( -0.4068241469816267775, 0.009842519685039144428, -0.3409548833797004797 ) ) ;
#33870=CARTESIAN_POINT ( 'NONE',  ( -0.5446194225721777693, -0.2845877964562161244, -0.3641732283464567121 ) ) ;
#33871=CARTESIAN_POINT ( 'NONE',  ( 0.6430446194225729606, -0.4281496062992127816, -0.4176697321401328100 ) ) ;
#33872=CARTESIAN_POINT ( 'NONE',  ( -1.614173228346456268, -0.6692913385826771977, 8.415575281601705876E-17 ) ) ;
#33874=CARTESIAN_POINT ( 'NONE',  ( -0.7283464566929126471, 0.07958543189024071263, -0.2665933059059888421 ) ) ;
#33875=CARTESIAN_POINT ( 'NONE',  ( 1.587926509186352586, -0.4281496062992127816, -0.4176697321401328100 ) ) ;
#33876=LINE ( 'NONE', #20001, #8872 ) ;
#33877=CARTESIAN_POINT ( 'NONE',  ( 0.6692913385826777528, 0.2952755905511811885, 0.000000000000000000 ) ) ;
#33878=CARTESIAN_POINT ( 'NONE',  ( -0.7611548556430438595, -0.5023911411419708095, -0.1820866141732282451 ) ) ;
#33879=CARTESIAN_POINT ( 'NONE',  ( -0.4199475065616791736, 0.1283753931104746893, -0.1820866141732285504 ) ) ;
#33880=CARTESIAN_POINT ( 'NONE',  ( -0.1902887139107604098, -0.6692913385826771977, 0.1292274648535927661 ) ) ;
#33881=CARTESIAN_POINT ( 'NONE',  ( -1.266404199475064773, -0.08942795157528024563, -0.3641732283464568787 ) ) ;
#33883=CARTESIAN_POINT ( 'NONE',  ( 0.6627296587926515548, 0.2952755905511811885, 0.1292274648535926551 ) ) ;
#33886=CARTESIAN_POINT ( 'NONE',  ( -0.9383202099737524282, -0.05778040916215522460, 0.4822834645669289988 ) ) ;
#33887=CARTESIAN_POINT ( 'NONE',  ( -0.2034120734908131112, -0.5511811023622048555, -0.09757992244046775898 ) ) ;
#33888=CARTESIAN_POINT ( 'NONE',  ( -1.397637795275589623, -0.5400638737290845981, -0.3530559997133363437 ) ) ;
#33889=CARTESIAN_POINT ( 'NONE',  ( 0.6627296587926517768, -0.5511811023622048555, -0.09757992244046775898 ) ) ;
#33890=CARTESIAN_POINT ( 'NONE',  ( -0.9317585301837263412, -0.004921259842519576551, 0.3153832671262227771 ) ) ;
#33891=CARTESIAN_POINT ( 'NONE',  ( -0.8858267716535425107, 0.1660481256975883668, -0.3530559997133364547 ) ) ;
#33892=CARTESIAN_POINT ( 'NONE',  ( -1.679790026246718693, 0.2306618581243847221, -0.2411417322834647770 ) ) ;
#33893=CARTESIAN_POINT ( 'NONE',  ( -1.541994750656167090, -0.6692913385826773087, -0.1292274648535924053 ) ) ;
#33894=CARTESIAN_POINT ( 'NONE',  ( -0.6743677364976040645, 1.919528099548696076, 0.5309055118110236338 ) ) ;
#33895=CARTESIAN_POINT ( 'NONE',  ( 0.9711286089238851948, -0.5023911411419708095, -0.1820866141732282451 ) ) ;
#33897=CARTESIAN_POINT ( 'NONE',  ( 0.6036745406824154392, 0.2306618581243847221, -0.2411417322834647770 ) ) ;
#33898=CARTESIAN_POINT ( 'NONE',  ( -1.456692913385826182, 0.2952755905511811885, 0.000000000000000000 ) ) ;
#33899=CARTESIAN_POINT ( 'NONE',  ( 1.548556430446194954, -0.5023911411419708095, 0.1820866141732285504 ) ) ;
#33901=ORIENTED_EDGE ( 'NONE', *, *, #61940, .F. ) ;
#33903=CARTESIAN_POINT ( 'NONE',  ( -1.167979002624671470, -0.004921259842519576551, 0.3153832671262227771 ) ) ;
#33904=CARTESIAN_POINT ( 'NONE',  ( -0.6758530183727028406, 0.2952755905511811885, 0.1292274648535926551 ) ) ;
#33905=CARTESIAN_POINT ( 'NONE',  ( 0.2230971128608929543, 0.05413385826771626580, -0.4176697321401330321 ) ) ;
#33906=CARTESIAN_POINT ( 'NONE',  ( -1.633858267716534529, -0.4536011799217368745, -0.2665933059059886201 ) ) ;
#33908=CARTESIAN_POINT ( 'NONE',  ( -1.292650918635170010, -0.6692913385826771977, 0.1292274648535927661 ) ) ;
#33909=CARTESIAN_POINT ( 'NONE',  ( 0.4461942257217856311, 0.2306618581243847221, -0.2411417322834647770 ) ) ;
#33910=CARTESIAN_POINT ( 'NONE',  ( 0.3083989501312343062, -0.05778040916215560624, -0.4822834645669293319 ) ) ;
#33911=CARTESIAN_POINT ( 'NONE',  ( 1.213910761154856299, -0.6692913385826773087, -0.1292274648535924053 ) ) ;
#33916=CARTESIAN_POINT ( 'NONE',  ( 0.5183727034120741983, 0.1771653543307087075, -0.09757992244046823083 ) ) ;
#33917=CARTESIAN_POINT ( 'NONE',  ( -0.4527559055118102749, 0.1660481256975885056, 0.3530559997133364547 ) ) ;
#33918=CARTESIAN_POINT ( 'NONE',  ( 1.246719160104987623, -0.4281496062992124485, 0.4176697321401328655 ) ) ;
#33920=CARTESIAN_POINT ( 'NONE',  ( 0.006561679790026889343, -0.2845877964562161244, -0.3641732283464567121 ) ) ;
#33921=( BOUNDED_CURVE ( )  B_SPLINE_CURVE ( 2, ( #51591, #38151, #70981, #19205, #82373, #18401, #31418, #13325, #58334, #7000, #696, #57082, #63823 ),
 .UNSPECIFIED., .F., .F. ) 
 B_SPLINE_CURVE_WITH_KNOTS ( ( 3, 2, 2, 2, 2, 2, 3 ),
 ( 0.6733310946348007864, 0.6742424242424241987, 0.6780303030303029832, 0.6818181818181817677, 0.6856060606060605522, 0.6893939393939394478, 0.6903052690015629711 ),
 .UNSPECIFIED. ) 
 CURVE ( )  GEOMETRIC_REPRESENTATION_ITEM ( )  RATIONAL_B_SPLINE_CURVE ( ( 0.9875488213027523443, 0.9918020599134680371, 1.000000000000000000, 0.9659258262890683122, 1.000000000000000000, 0.9659258262890683122, 1.000000000000000000, 0.9659258262890683122, 1.000000000000000000, 0.9659258262890683122, 1.000000000000000000, 0.9918020599134671489, 0.9875488213027514561 ) ) 
 REPRESENTATION_ITEM ( '' )  );
#33922=CARTESIAN_POINT ( 'NONE',  ( -1.095800524934382292, -0.3162353388693409650, -0.4822834645669289433 ) ) ;
#33923=CARTESIAN_POINT ( 'NONE',  ( 1.502624671916010790, -0.3162353388693409650, -0.4822834645669289433 ) ) ;
#33924=CARTESIAN_POINT ( 'NONE',  ( 0.3149606299212606708, -0.1870078740157480879, -0.4822834645669291653 ) ) ;
#33928=EDGE_LOOP ( 'NONE', ( #74235, #36716, #1721, #17508 ) ) ;
#33929=CARTESIAN_POINT ( 'NONE',  ( 1.568241469816273437, -0.2845877964562159024, 0.3641732283464567677 ) ) ;
#33930=CARTESIAN_POINT ( 'NONE',  ( -1.286089238845143479, 0.1283753931104746893, -0.1820866141732285504 ) ) ;
#33931=CARTESIAN_POINT ( 'NONE',  ( -1.325459317585300889, 0.05413385826771666132, 0.4176697321401328100 ) ) ;
#33933=CARTESIAN_POINT ( 'NONE',  ( 0.4848604877838280647, 0.000000000000000000, 0.3464511005275205946 ) ) ;
#33934=CARTESIAN_POINT ( 'NONE',  ( 1.194225721784777594, 0.05413385826771666132, 0.4176697321401328100 ) ) ;
#33935=CARTESIAN_POINT ( 'NONE',  ( -1.338582677165353729, -0.1870078740157480879, -0.4822834645669291653 ) ) ;
#33936=CARTESIAN_POINT ( 'NONE',  ( 0.01968503937007930540, 0.1660481256975885056, 0.3530559997133364547 ) ) ;
#33937=CARTESIAN_POINT ( 'NONE',  ( -1.253280839895012377, -0.3162353388693409650, -0.4822834645669289433 ) ) ;
#33940=CARTESIAN_POINT ( 'NONE',  ( 0.4658792650918640033, -0.3162353388693405765, 0.4822834645669290543 ) ) ;
#33942=CARTESIAN_POINT ( 'NONE',  ( -1.253280839895012377, -0.2845877964562161244, -0.3641732283464567121 ) ) ;
#33943=ORIENTED_EDGE ( 'NONE', *, *, #55305, .T. ) ;
#33946=LINE ( 'NONE', #73925, #16712 ) ;
#33947=CARTESIAN_POINT ( 'NONE',  ( -1.043307086614172707, 0.1660481256975883668, -0.3530559997133364547 ) ) ;
#33948=CARTESIAN_POINT ( 'NONE',  ( -1.187664041994749731, -0.3162353388693405765, 0.4822834645669290543 ) ) ;
#33950=CARTESIAN_POINT ( 'NONE',  ( -1.443569553805773564, -0.6046776061558807314, 0.2411417322834647770 ) ) ;
#33951=CARTESIAN_POINT ( 'NONE',  ( -1.541994750656167090, 0.2952755905511811885, 0.1292274648535926551 ) ) ;
#33952=CARTESIAN_POINT ( 'NONE',  ( -1.535433070866141225, -0.6692913385826771977, 8.415575281601705876E-17 ) ) ;
#33953=LINE ( 'NONE', #27635, #17637 ) ;
#33957=CARTESIAN_POINT ( 'NONE',  ( 0.2493438320209980519, -0.004921259842519576551, 0.3153832671262227771 ) ) ;
#33959=CARTESIAN_POINT ( 'NONE',  ( -0.6824146981627291497, -0.5023911411419708095, -0.1820866141732282451 ) ) ;
#33960=CARTESIAN_POINT ( 'NONE',  ( -1.272965879265091305, 0.05413385826771626580, -0.4176697321401330321 ) ) ;
#33961=CARTESIAN_POINT ( 'NONE',  ( 1.017060367454068581, -0.05778040916215560624, -0.4822834645669293319 ) ) ;
#33962=CARTESIAN_POINT ( 'NONE',  ( -0.9580052493438311334, 0.05413385826771626580, -0.4176697321401330321 ) ) ;
#33965=CARTESIAN_POINT ( 'NONE',  ( -0.7742782152230962556, -0.4281496062992127816, -0.4176697321401328100 ) ) ;
#33966=CARTESIAN_POINT ( 'NONE',  ( 0.7152230971128614723, -0.3162353388693409650, -0.4822834645669289433 ) ) ;
#33967=CARTESIAN_POINT ( 'NONE',  ( -1.706036745406823485, 0.1283753931104748280, 0.1820866141732283561 ) ) ;
#33973=CARTESIAN_POINT ( 'NONE',  ( -0.5052493438320203589, 0.2952755905511810774, -0.1292274648535930714 ) ) ;
#33974=CARTESIAN_POINT ( 'NONE',  ( 1.686351706036745890, 0.2952755905511811885, 0.1292274648535926551 ) ) ;
#33976=CARTESIAN_POINT ( 'NONE',  ( -1.325459317585300889, -0.4281496062992127816, -0.4176697321401328100 ) ) ;
#33978=CARTESIAN_POINT ( 'NONE',  ( -1.417322834645668772, -0.1870078740157479769, 0.4822834645669291653 ) ) ;
#33979=CARTESIAN_POINT ( 'NONE',  ( -0.3280839895013117347, -0.4281496062992124485, 0.4176697321401328655 ) ) ;
#33981=CARTESIAN_POINT ( 'NONE',  ( 0.5774278215223103139, -0.5023911411419708095, -0.1820866141732282451 ) ) ;
#33983=CARTESIAN_POINT ( 'NONE',  ( 0.2887139107611556010, 0.1283753931104746893, -0.1820866141732285504 ) ) ;
#33984=CARTESIAN_POINT ( 'NONE',  ( 1.410761154855643795, -0.2845877964562159024, 0.3641732283464567677 ) ) ;
#33985=CARTESIAN_POINT ( 'NONE',  ( 0.9580052493438326877, 0.05413385826771666132, 0.4176697321401328100 ) ) ;
#33986=CARTESIAN_POINT ( 'NONE',  ( 0.2230971128608932319, -0.3690944881889763329, 0.3153832671262228327 ) ) ;
#33988=CARTESIAN_POINT ( 'NONE',  ( -1.240157480314959759, -0.5400638737290845981, -0.3530559997133363437 ) ) ;
#33989=CARTESIAN_POINT ( 'NONE',  ( 0.006561679790026889343, -0.08942795157527998196, 0.3641732283464567121 ) ) ;
#33990=CARTESIAN_POINT ( 'NONE',  ( -1.161417322834644716, 0.07958543189024085140, 0.2665933059059887866 ) ) ;
#33992=CARTESIAN_POINT ( 'NONE',  ( -0.6299212598425188991, -0.1870078740157480601, -0.3641732283464567677 ) ) ;
#33994=CARTESIAN_POINT ( 'NONE',  ( -0.2362204724409440182, -0.1870078740157479769, 0.4822834645669291653 ) ) ;
#33995=CARTESIAN_POINT ( 'NONE',  ( -1.614173228346456712, 2.401574803149606474, 0.1372047244094477536 ) ) ;
#33996=CARTESIAN_POINT ( 'NONE',  ( 0.3805774278215230400, -0.004921259842519870586, -0.3153832671262229437 ) ) ;
#33997=CARTESIAN_POINT ( 'NONE',  ( -0.1312335958005241554, 0.1283753931104748280, 0.1820866141732283561 ) ) ;
#33998=CARTESIAN_POINT ( 'NONE',  ( -0.1443569553805765515, -0.4281496062992127816, -0.4176697321401328100 ) ) ;
#34000=CARTESIAN_POINT ( 'NONE',  ( -1.076115485564303809, -0.5023911411419708095, -0.1820866141732282451 ) ) ;
#34001=DIRECTION ( 'NONE',  ( -0.000000000000000000, -1.000000000000000000, -0.000000000000000000 ) ) ;
#34003=CARTESIAN_POINT ( 'NONE',  ( 0.5052493438320218022, -0.6692913385826773087, -0.1292274648535924053 ) ) ;
#34004=CARTESIAN_POINT ( 'NONE',  ( -0.9514435695538050464, -0.05778040916215560624, -0.4822834645669293319 ) ) ;
#34007=CARTESIAN_POINT ( 'NONE',  ( -0.1837270341207343505, -0.5023911411419708095, 0.1820866141732285504 ) ) ;
#34008=CARTESIAN_POINT ( 'NONE',  ( -1.364829396325458521, -0.6046776061558807314, 0.2411417322834647770 ) ) ;
#34009=CARTESIAN_POINT ( 'NONE',  ( 1.515748031496063408, 0.1660481256975885056, 0.3530559997133364547 ) ) ;
#34011=CARTESIAN_POINT ( 'NONE',  ( -0.5577427821522301654, -0.08942795157528024563, -0.3641732283464568787 ) ) ;
#34013=CARTESIAN_POINT ( 'NONE',  ( 0.6955380577427828781, 0.05413385826771626580, -0.4176697321401330321 ) ) ;
#34019=CARTESIAN_POINT ( 'NONE',  ( 1.535433070866142335, -0.5511811023622047445, 6.969142054262312111E-17 ) ) ;
#34020=CARTESIAN_POINT ( 'NONE',  ( -1.187664041994750175, -0.05778040916215560624, -0.4822834645669293319 ) ) ;
#34021=CARTESIAN_POINT ( 'NONE',  ( 1.364829396325459854, -0.6046776061558809534, -0.2411417322834644161 ) ) ;
#34023=CARTESIAN_POINT ( 'NONE',  ( 1.640419947506562393, -0.3690944881889763329, 0.3153832671262228327 ) ) ;
#34024=CARTESIAN_POINT ( 'NONE',  ( 0.6430446194225729606, -0.4281496062992127816, -0.4176697321401328100 ) ) ;
#34025=CARTESIAN_POINT ( 'NONE',  ( -0.5511811023622038563, -0.1870078740157479769, 0.4822834645669291653 ) ) ;
#34026=FACE_OUTER_BOUND ( 'NONE', #62373, .T. ) ;
#34028=CARTESIAN_POINT ( 'NONE',  ( 0.7677165354330716118, -0.4536011799217367080, 0.2665933059059888421 ) ) ;
#34029=ORIENTED_EDGE ( 'NONE', *, *, #16635, .T. ) ;
#34032=CARTESIAN_POINT ( 'NONE',  ( -0.4658792650918627265, -0.05778040916215522460, 0.4822834645669289988 ) ) ;
#34033=CARTESIAN_POINT ( 'NONE',  ( 1.194225721784777594, -0.4281496062992127816, -0.4176697321401328100 ) ) ;
#34034=CARTESIAN_POINT ( 'NONE',  ( 0.1640419947506569498, -0.3162353388693409650, -0.4822834645669289433 ) ) ;
#34035=CARTESIAN_POINT ( 'NONE',  ( -0.2099737532808391705, 0.1283753931104748280, 0.1820866141732283561 ) ) ;
#34036=CARTESIAN_POINT ( 'NONE',  ( 1.154855643044620184, -0.6046776061558807314, 0.2411417322834647770 ) ) ;
#34037=CARTESIAN_POINT ( 'NONE',  ( -0.8398950131233585692, 0.2306618581243848609, 0.2411417322834645549 ) ) ;
#34038=CARTESIAN_POINT ( 'NONE',  ( 0.006561679790026889343, -0.05778040916215522460, 0.4822834645669289988 ) ) ;
#34039=CARTESIAN_POINT ( 'NONE',  ( 1.135170603674541256, 0.2952755905511811885, 0.1292274648535926551 ) ) ;
#34040=CARTESIAN_POINT ( 'NONE',  ( 0.9317585301837276734, -0.4281496062992124485, 0.4176697321401328655 ) ) ;
#34041=CARTESIAN_POINT ( 'NONE',  ( 1.246719160104987623, 0.05413385826771626580, -0.4176697321401330321 ) ) ;
#34043=CARTESIAN_POINT ( 'NONE',  ( 0.05249343832021075018, -0.5023911411419708095, 0.1820866141732285504 ) ) ;
#34047=CARTESIAN_POINT ( 'NONE',  ( -0.2690288713910754526, 0.1771653543307087075, -0.09757992244046823083 ) ) ;
#34048=CARTESIAN_POINT ( 'NONE',  ( -0.05249343832020911260, 0.2306618581243848609, 0.2411417322834645549 ) ) ;
#34050=CARTESIAN_POINT ( 'NONE',  ( -0.2624671916010490880, 0.2306618581243847221, -0.2411417322834647770 ) ) ;
#34051=CARTESIAN_POINT ( 'NONE',  ( -0.3083989501312330295, -0.05778040916215522460, 0.4822834645669289988 ) ) ;
#34052=CARTESIAN_POINT ( 'NONE',  ( -0.9186351706036736120, -0.6046776061558809534, -0.2411417322834644161 ) ) ;
#34053=CARTESIAN_POINT ( 'NONE',  ( -0.9842519685039365918, -0.6692913385826771977, 8.415575281601705876E-17 ) ) ;
#34054=CARTESIAN_POINT ( 'NONE',  ( 1.561679790026247350, -0.004921259842519870586, -0.3153832671262229437 ) ) ;
#34057=CARTESIAN_POINT ( 'NONE',  ( 0.4790026246719167324, -0.08942795157527998196, 0.3641732283464567121 ) ) ;
#34058=AXIS2_PLACEMENT_3D ( 'NONE', #59248, #70207, #6235 ) ;
#34059=CARTESIAN_POINT ( 'NONE',  ( 0.5118110236220480003, -0.6692913385826771977, 8.415575281601705876E-17 ) ) ;
#34060=CARTESIAN_POINT ( 'NONE',  ( 0.5446194225721792126, -0.3162353388693405765, 0.4822834645669290543 ) ) ;
#34063=CARTESIAN_POINT ( 'NONE',  ( -1.601049868766403650, -0.6046776061558807314, 0.2411417322834647770 ) ) ;
#34066=CARTESIAN_POINT ( 'NONE',  ( -0.5643044619422565855, 0.05413385826771626580, -0.4176697321401330321 ) ) ;
#34069=CARTESIAN_POINT ( 'NONE',  ( -1.568241469816272105, -0.2845877964562161244, -0.3641732283464567121 ) ) ;
#34070=CARTESIAN_POINT ( 'NONE',  ( 0.7874015748031503170, -0.1870078740157479769, 0.4822834645669291653 ) ) ;
#34071=CARTESIAN_POINT ( 'NONE',  ( 1.122047244094488860, -0.5400638737290845981, -0.3530559997133363437 ) ) ;
#34072=CARTESIAN_POINT ( 'NONE',  ( -0.3937007874015740483, -0.1870078740157479769, 0.3641732283464567677 ) ) ;
#34073=CARTESIAN_POINT ( 'NONE',  ( 0.4396325459317590445, -0.6692913385826771977, 0.1292274648535927661 ) ) ;
#34075=CARTESIAN_POINT ( 'NONE',  ( 0.04593175853018440641, -0.5511811023622046335, 0.09757992244046803654 ) ) ;
#34076=CARTESIAN_POINT ( 'NONE',  ( 0.02624671916010564918, 0.2306618581243848609, 0.2411417322834645549 ) ) ;
#34079=CARTESIAN_POINT ( 'NONE',  ( 1.601049868766404982, 0.1283753931104748280, 0.1820866141732283561 ) ) ;
#34080=CARTESIAN_POINT ( 'NONE',  ( 0.03280839895013198948, 0.1771653543307087630, 0.09757992244046791164 ) ) ;
#34081=CARTESIAN_POINT ( 'NONE',  ( -0.8333333333333323711, -0.6692913385826773087, -0.1292274648535924053 ) ) ;
#34083=CARTESIAN_POINT ( 'NONE',  ( -0.7217847769028863381, -0.3690944881889763329, 0.3153832671262228327 ) ) ;
#34085=CARTESIAN_POINT ( 'NONE',  ( -0.7414698162729651543, 0.2952755905511810774, -0.1292274648535930714 ) ) ;
#34086=CARTESIAN_POINT ( 'NONE',  ( -0.4855643044619415427, 0.05413385826771626580, -0.4176697321401330321 ) ) ;
#34087=CARTESIAN_POINT ( 'NONE',  ( -0.1902887139107604098, 0.2952755905511810774, -0.1292274648535930714 ) ) ;
#34091=CARTESIAN_POINT ( 'NONE',  ( 0.8989501312335964611, 0.1771653543307087630, 0.09757992244046791164 ) ) ;
#34092=CARTESIAN_POINT ( 'NONE',  ( 1.476377952755906220, 0.1660481256975883668, -0.3530559997133364547 ) ) ;
#34093=CARTESIAN_POINT ( 'NONE',  ( -1.213910761154854745, 0.1771653543307087075, -0.09757992244046823083 ) ) ;
#34094=CARTESIAN_POINT ( 'NONE',  ( 1.122047244094488860, -0.5400638737290845981, -0.3530559997133363437 ) ) ;
#34095=CARTESIAN_POINT ( 'NONE',  ( -1.069553805774277722, 0.1771653543307087630, 0.09757992244046791164 ) ) ;
#34096=CARTESIAN_POINT ( 'NONE',  ( -0.5118110236220466680, -0.6692913385826771977, 8.415575281601705876E-17 ) ) ;
#34097=CARTESIAN_POINT ( 'NONE',  ( -0.05905511811023545637, 0.07958543189024085140, 0.2665933059059887866 ) ) ;
#34098=CARTESIAN_POINT ( 'NONE',  ( -1.614173228346456712, 0.4410134679336886188, -0.1372047244094478091 ) ) ;
#34099=CARTESIAN_POINT ( 'NONE',  ( 1.272965879265092637, -0.004921259842519576551, 0.3153832671262227771 ) ) ;
#34100=EDGE_CURVE ( 'NONE', #7120, #73064, #72066, .T. ) ;
#34102=CARTESIAN_POINT ( 'NONE',  ( 0.2362204724409456558, -0.1870078740157479769, 0.4822834645669291653 ) ) ;
#34105=CARTESIAN_POINT ( 'NONE',  ( -0.7545931758530177724, 0.2952755905511811885, 0.1292274648535926551 ) ) ;
#34107=CARTESIAN_POINT ( 'NONE',  ( 0.8333333333333340365, 0.1771653543307087075, -0.09757992244046823083 ) ) ;
#34108=CARTESIAN_POINT ( 'NONE',  ( 0.3346456692913393205, -0.5400638737290845981, -0.3530559997133363437 ) ) ;
#34109=CARTESIAN_POINT ( 'NONE',  ( 0.06561679790026316017, -0.4281496062992124485, 0.4176697321401328655 ) ) ;
#34110=CARTESIAN_POINT ( 'NONE',  ( -0.1640419947506553400, -0.08942795157528024563, -0.3641732283464568787 ) ) ;
#34112=CARTESIAN_POINT ( 'NONE',  ( -0.2230971128608915943, -0.004921259842519576551, 0.3153832671262227771 ) ) ;
#34113=CARTESIAN_POINT ( 'NONE',  ( 0.6889763779527566800, -0.5400638737290844871, 0.3530559997133364547 ) ) ;
#34114=CARTESIAN_POINT ( 'NONE',  ( -0.8661417322834640276, -0.1870078740157480601, -0.3641732283464567677 ) ) ;
#34116=CARTESIAN_POINT ( 'NONE',  ( -0.9514435695538050464, -0.05778040916215560624, -0.4822834645669293319 ) ) ;
#34117=DIRECTION ( 'NONE',  ( 0.7071067811865495711, -0.000000000000000000, -0.7071067811865454633 ) ) ;
#34118=VERTEX_POINT ( 'NONE', #26612 ) ;
#34120=CARTESIAN_POINT ( 'NONE',  ( -0.9055118110236215490, 0.1771653543307087630, 0.000000000000000000 ) ) ;
#34121=CARTESIAN_POINT ( 'NONE',  ( -0.09186351706036689768, 0.05413385826771626580, -0.4176697321401330321 ) ) ;
#34122=CARTESIAN_POINT ( 'NONE',  ( -1.509186351706035767, 0.05413385826771626580, -0.4176697321401330321 ) ) ;
#34123=CARTESIAN_POINT ( 'NONE',  ( -0.9186351706036736120, -0.6046776061558809534, -0.2411417322834644161 ) ) ;
#34126=CARTESIAN_POINT ( 'NONE',  ( 1.082677165354331228, -0.5400638737290844871, 0.3530559997133364547 ) ) ;
#34127=CARTESIAN_POINT ( 'NONE',  ( 0.8858267716535438430, 0.1660481256975885056, 0.3530559997133364547 ) ) ;
#34128=CARTESIAN_POINT ( 'NONE',  ( -0.2690288713910753970, 0.2066929133858267098, -0.1054918080437494132 ) ) ;
#34130=CARTESIAN_POINT ( 'NONE',  ( -1.325459317585300889, -0.4281496062992127816, -0.4176697321401328100 ) ) ;
#34133=CARTESIAN_POINT ( 'NONE',  ( -0.7086614173228339419, -0.1870078740157479769, 0.3641732283464567677 ) ) ;
#34136=VERTEX_POINT ( 'NONE', #45533 ) ;
#34137=CARTESIAN_POINT ( 'NONE',  ( 0.8923884514435701520, -0.6046776061558809534, -0.2411417322834644161 ) ) ;
#34138=CARTESIAN_POINT ( 'NONE',  ( 0.1968503937007881344, 0.2952755905511811885, 0.000000000000000000 ) ) ;
#34139=CARTESIAN_POINT ( 'NONE',  ( -0.7480314960629914633, -0.6692913385826771977, 8.415575281601705876E-17 ) ) ;
#34140=CARTESIAN_POINT ( 'NONE',  ( 1.509186351706037543, 0.05413385826771666132, 0.4176697321401328100 ) ) ;
#34141=CARTESIAN_POINT ( 'NONE',  ( -1.062992125984250968, -0.5511811023622047445, 6.969142054262312111E-17 ) ) ;
#34142=LINE ( 'NONE', #15628, #56073 ) ;
#34143=CARTESIAN_POINT ( 'NONE',  ( 0.6364829396325465405, -0.3162353388693409650, -0.4822834645669289433 ) ) ;
#34144=CARTESIAN_POINT ( 'NONE',  ( 0.3871391076115492380, -0.08942795157528024563, -0.3641732283464568787 ) ) ;
#34145=CARTESIAN_POINT ( 'NONE',  ( -0.5380577427821514602, 0.05413385826771666132, 0.4176697321401328100 ) ) ;
#34147=CARTESIAN_POINT ( 'NONE',  ( -1.115485564304461219, 0.05413385826771626580, -0.4176697321401330321 ) ) ;
#34148=CARTESIAN_POINT ( 'NONE',  ( -1.712598425196849572, 0.07958543189024085140, 0.2665933059059887866 ) ) ;
#34149=CARTESIAN_POINT ( 'NONE',  ( 1.535433070866142558, 0.2952755905511811885, 0.000000000000000000 ) ) ;
#34150=CARTESIAN_POINT ( 'NONE',  ( 1.299212598425197429, -0.5511811023622047445, 6.969142054262312111E-17 ) ) ;
#34153=CARTESIAN_POINT ( 'NONE',  ( 0.04593175853018440641, -0.6692913385826771977, 0.1292274648535927661 ) ) ;
#34155=CARTESIAN_POINT ( 'NONE',  ( 0.8858267716535438430, -0.4536011799217368745, -0.2665933059059886201 ) ) ;
#34156=CARTESIAN_POINT ( 'NONE',  ( -1.043307086614172707, 0.1660481256975883668, -0.3530559997133364547 ) ) ;
#34157=CARTESIAN_POINT ( 'NONE',  ( 1.141732283464567566, 0.2952755905511811885, 0.000000000000000000 ) ) ;
#34158=CARTESIAN_POINT ( 'NONE',  ( 0.6430446194225728496, 0.05413385826771666132, 0.4176697321401328100 ) ) ;
#34159=CARTESIAN_POINT ( 'NONE',  ( 0.3412073490813655186, 0.2306618581243848609, 0.2411417322834645549 ) ) ;
#34160=CARTESIAN_POINT ( 'NONE',  ( -0.4658792650918627265, -0.3162353388693409650, -0.4822834645669289433 ) ) ;
#34162=CARTESIAN_POINT ( 'NONE',  ( -1.377952755905511140, 0.2952755905511811885, 0.000000000000000000 ) ) ;
#34163=CARTESIAN_POINT ( 'NONE',  ( -0.5249343832020990641, 0.2306618581243848609, 0.2411417322834645549 ) ) ;
#34164=CARTESIAN_POINT ( 'NONE',  ( -0.3608923884514428360, 0.1771653543307087630, 0.09757992244046791164 ) ) ;
#34167=CARTESIAN_POINT ( 'NONE',  ( -0.4133858267716528645, 0.1660481256975883668, -0.3530559997133364547 ) ) ;
#34169=CARTESIAN_POINT ( 'NONE',  ( 0.7480314960629927956, -0.6692913385826771977, 8.415575281601705876E-17 ) ) ;
#34172=CARTESIAN_POINT ( 'NONE',  ( -0.3412073490813641308, 0.2306618581243847221, -0.2411417322834647770 ) ) ;
#34173=CARTESIAN_POINT ( 'NONE',  ( 1.082677165354331228, 0.07958543189024071263, -0.2665933059059888421 ) ) ;
#34174=LINE ( 'NONE', #16802, #50551 ) ;
#34176=CARTESIAN_POINT ( 'NONE',  ( 1.299212598425197429, -0.5511811023622047445, 6.969142054262312111E-17 ) ) ;
#34177=CARTESIAN_POINT ( 'NONE',  ( 1.227034120734908917, -0.6692913385826771977, 0.1292274648535927661 ) ) ;
#34179=CARTESIAN_POINT ( 'NONE',  ( -0.3412073490813641308, -0.6046776061558807314, 0.2411417322834647770 ) ) ;
#34180=CARTESIAN_POINT ( 'NONE',  ( -1.443569553805773564, 0.2306618581243847221, -0.2411417322834647770 ) ) ;
#34182=CARTESIAN_POINT ( 'NONE',  ( -1.679790026246718693, 0.2306618581243847221, -0.2411417322834647770 ) ) ;
#34183=CARTESIAN_POINT ( 'NONE',  ( -0.3280839895013117347, -0.4281496062992124485, 0.4176697321401328655 ) ) ;
#34185=CARTESIAN_POINT ( 'NONE',  ( 1.377952755905512472, 0.2952755905511811885, 0.000000000000000000 ) ) ;
#34186=CARTESIAN_POINT ( 'NONE',  ( 0.5708661417322841158, -0.5400638737290845981, -0.3530559997133363437 ) ) ;
#34187=CARTESIAN_POINT ( 'NONE',  ( 0.4790026246719168435, -0.2845877964562161244, -0.3641732283464567121 ) ) ;
#34189=CARTESIAN_POINT ( 'NONE',  ( 0.2887139107611556010, 0.1283753931104746893, -0.1820866141732285504 ) ) ;
#34192=CARTESIAN_POINT ( 'NONE',  ( 0.9645669291338591078, -0.5400638737290845981, -0.3530559997133363437 ) ) ;
#34195=CARTESIAN_POINT ( 'NONE',  ( -0.3280839895013117347, 0.009842519685039147898, -0.3409548833797004797 ) ) ;
#34196=CARTESIAN_POINT ( 'NONE',  ( -0.1049868766404193215, 0.1283753931104746893, -0.1820866141732285504 ) ) ;
#34197=CIRCLE ( 'NONE', #77198, 3.582677165354330562 ) ;
#34198=CARTESIAN_POINT ( 'NONE',  ( 0.3346456692913393205, -0.5400638737290845981, -0.3530559997133363437 ) ) ;
#34200=CARTESIAN_POINT ( 'NONE',  ( 1.450131233595801428, -0.5511811023622048555, -0.09757992244046775898 ) ) ;
#34201=CARTESIAN_POINT ( 'NONE',  ( -0.8136482939632537770, -0.5023911411419708095, 0.1820866141732285504 ) ) ;
#34202=CARTESIAN_POINT ( 'NONE',  ( -0.9776902887139098386, -0.6692913385826771977, 0.1292274648535927661 ) ) ;
#34203=CARTESIAN_POINT ( 'NONE',  ( -1.384514435695537005, 0.2952755905511811885, 0.1292274648535926551 ) ) ;
#34204=CARTESIAN_POINT ( 'NONE',  ( 0.3346456692913393205, -0.5400638737290845981, -0.3530559997133363437 ) ) ;
#34205=CARTESIAN_POINT ( 'NONE',  ( 1.423884514435696413, -0.3162353388693409650, -0.4822834645669289433 ) ) ;
#34207=CARTESIAN_POINT ( 'NONE',  ( 0.4133858267716541968, -0.5400638737290845981, -0.3530559997133363437 ) ) ;
#34209=CARTESIAN_POINT ( 'NONE',  ( 1.640419947506562393, -0.4281496062992124485, 0.4176697321401328655 ) ) ;
#34210=CARTESIAN_POINT ( 'NONE',  ( 1.318897637795276356, -0.5400638737290844871, 0.3530559997133364547 ) ) ;
#34211=CARTESIAN_POINT ( 'NONE',  ( -1.423884514435694859, -0.2845877964562159024, 0.3641732283464567677 ) ) ;
#34212=CARTESIAN_POINT ( 'NONE',  ( 1.148293963254593875, -0.5511811023622046335, 0.09757992244046803654 ) ) ;
#34213=CARTESIAN_POINT ( 'NONE',  ( -1.167979002624671470, -0.004921259842519576551, 0.3153832671262227771 ) ) ;
#34214=CARTESIAN_POINT ( 'NONE',  ( -0.8136482939632537770, 0.1283753931104746893, -0.1820866141732285504 ) ) ;
#34215=FACE_OUTER_BOUND ( 'NONE', #26775, .T. ) ;
#34216=CARTESIAN_POINT ( 'NONE',  ( 0.6299212598425204535, -0.1870078740157479769, 0.3641732283464567677 ) ) ;
#34217=CARTESIAN_POINT ( 'NONE',  ( 0.3280839895013130669, -0.4281496062992127816, -0.4176697321401328100 ) ) ;
#34218=CARTESIAN_POINT ( 'NONE',  ( 0.9383202099737536495, -0.3162353388693405765, 0.4822834645669290543 ) ) ;
#34219=ADVANCED_FACE ( 'NONE', ( #44686 ), #16733, .F. ) ;
#34220=CARTESIAN_POINT ( 'NONE',  ( 0.1115485564304470323, 0.2952755905511811885, 0.1292274648535926551 ) ) ;
#34221=CARTESIAN_POINT ( 'NONE',  ( 0.01312335958005323398, -0.004921259842519576551, 0.3153832671262227771 ) ) ;
#34222=B_SPLINE_CURVE_WITH_KNOTS ( 'NONE', 3,
 ( #43454, #23700, #68741, #69152 ),
 .UNSPECIFIED., .F., .F.,
 ( 4, 4 ),
 ( 3.210432057660995322E-07, 0.001287787053612077974 ),
 .UNSPECIFIED. ) ;
#34223=CARTESIAN_POINT ( 'NONE',  ( 1.384514435695538337, -0.6692913385826771977, 0.1292274648535927661 ) ) ;
#34224=DIRECTION ( 'NONE',  ( -1.000000000000000000, -3.469446951953613696E-16, 0.000000000000000000 ) ) ;
#34225=CARTESIAN_POINT ( 'NONE',  ( -1.003937007874015297, -0.5400638737290845981, -0.3530559997133363437 ) ) ;
#34228=CARTESIAN_POINT ( 'NONE',  ( -0.8398950131233585692, 0.2306618581243848609, 0.2411417322834645549 ) ) ;
#34229=CARTESIAN_POINT ( 'NONE',  ( -0.1706036745406816491, -0.4281496062992124485, 0.4176697321401328655 ) ) ;
#34237=CARTESIAN_POINT ( 'NONE',  ( -1.207349081364828880, 0.1283753931104746893, -0.1820866141732285504 ) ) ;
#34239=CARTESIAN_POINT ( 'NONE',  ( -1.581364829396324945, -0.3162353388693405765, 0.4822834645669290543 ) ) ;
#34241=CARTESIAN_POINT ( 'NONE',  ( 0.1377952755905518800, 0.1660481256975883668, -0.3530559997133364547 ) ) ;
#34242=CARTESIAN_POINT ( 'NONE',  ( -0.3608923884514428360, -0.5511811023622048555, -0.09757992244046775898 ) ) ;
#34243=CARTESIAN_POINT ( 'NONE',  ( 0.8661417322834652488, -0.1870078740157480879, -0.4822834645669291653 ) ) ;
#34244=CARTESIAN_POINT ( 'NONE',  ( 0.3805774278215230400, 0.05413385826771626580, -0.4176697321401330321 ) ) ;
#34248=CARTESIAN_POINT ( 'NONE',  ( 1.102362204724410155, -0.1870078740157480879, -0.4822834645669291653 ) ) ;
#34249=CARTESIAN_POINT ( 'NONE',  ( 0.1443569553805781891, -0.4281496062992124485, 0.4176697321401328655 ) ) ;
#34250=CARTESIAN_POINT ( 'NONE',  ( -1.194225721784776262, -0.4281496062992124485, 0.4176697321401328655 ) ) ;
#34252=CARTESIAN_POINT ( 'NONE',  ( 1.351706036745407458, -0.4281496062992127816, -0.4176697321401328100 ) ) ;
#34253=CARTESIAN_POINT ( 'NONE',  ( 1.089238845144357759, 0.05413385826771626580, -0.4176697321401330321 ) ) ;
#34255=CARTESIAN_POINT ( 'NONE',  ( 0.02624671916010564918, 0.2306618581243848609, 0.2411417322834645549 ) ) ;
#34256=CARTESIAN_POINT ( 'NONE',  ( 0.6167979002624679463, 0.05413385826771626580, -0.4176697321401330321 ) ) ;
#34257=CARTESIAN_POINT ( 'NONE',  ( 8.195543980992789655E-16, -0.1870078740157480879, -0.4822834645669291653 ) ) ;
#34258=CARTESIAN_POINT ( 'NONE',  ( 0.5577427821522316087, -0.08942795157527998196, 0.3641732283464567121 ) ) ;
#34259=CARTESIAN_POINT ( 'NONE',  ( -1.207349081364828880, 0.2306618581243847221, -0.2411417322834647770 ) ) ;
#34260=CARTESIAN_POINT ( 'NONE',  ( -1.338582677165353729, -0.1870078740157480879, -0.4822834645669291653 ) ) ;
#34261=CARTESIAN_POINT ( 'NONE',  ( 0.7742782152230978099, -0.4281496062992124485, 0.4176697321401328655 ) ) ;
#34265=ORIENTED_EDGE ( 'NONE', *, *, #31679, .T. ) ;
#34268=CARTESIAN_POINT ( 'NONE',  ( 1.128608923884515169, -0.6046776061558809534, -0.2411417322834644161 ) ) ;
#34269=CARTESIAN_POINT ( 'NONE',  ( 0.4790026246719167324, -0.08942795157527998196, 0.3641732283464567121 ) ) ;
#34270=CARTESIAN_POINT ( 'NONE',  ( -0.7763038905084325147, -3.623651218081290895E-15, 0.3954974714151467952 ) ) ;
#34271=CARTESIAN_POINT ( 'NONE',  ( 0.4581548248993063122, 1.775897345035375441, -0.5309055118110237448 ) ) ;
#34272=CARTESIAN_POINT ( 'NONE',  ( -1.614173228346457378, 0.5038684218300933937, -0.1372047244094477536 ) ) ;
#34276=CARTESIAN_POINT ( 'NONE',  ( -0.2230971128608915943, -0.4281496062992127816, -0.4176697321401328100 ) ) ;
#34277=CARTESIAN_POINT ( 'NONE',  ( 1.213910761154856299, -0.6692913385826773087, -0.1292274648535924053 ) ) ;
#34279=CARTESIAN_POINT ( 'NONE',  ( -1.371391076115484831, 0.2952755905511810774, -0.1292274648535930714 ) ) ;
#34283=CARTESIAN_POINT ( 'NONE',  ( -1.423884514435694859, -0.08942795157528024563, -0.3641732283464568787 ) ) ;
#34284=EDGE_CURVE ( 'NONE', #30161, #23065, #25288, .T. ) ;
#34285=CARTESIAN_POINT ( 'NONE',  ( -1.561679790026246017, -0.4281496062992127816, -0.4176697321401328100 ) ) ;
#34286=CARTESIAN_POINT ( 'NONE',  ( 0.2099737532808405305, -0.6046776061558807314, 0.2411417322834647770 ) ) ;
#34288=CARTESIAN_POINT ( 'NONE',  ( 1.640419947506562393, -0.4281496062992124485, 0.4176697321401328655 ) ) ;
#34289=CARTESIAN_POINT ( 'NONE',  ( -0.4527559055118102749, 0.1012011053420777407, 0.2882089793578257453 ) ) ;
#34290=CARTESIAN_POINT ( 'NONE',  ( -0.5511811023622041894, -0.1870078740157480601, -0.3641732283464567677 ) ) ;
#34291=( BOUNDED_CURVE ( )  B_SPLINE_CURVE ( 1, ( #65504, #26762 ),
 .UNSPECIFIED., .F., .F. ) 
 B_SPLINE_CURVE_WITH_KNOTS ( ( 2, 2 ),
 ( 0.000000000000000000, 0.002000000000000008715 ),
 .UNSPECIFIED. ) 
 CURVE ( )  GEOMETRIC_REPRESENTATION_ITEM ( )  RATIONAL_B_SPLINE_CURVE ( ( 0.9875488213027527884, 0.9875488213027527884 ) ) 
 REPRESENTATION_ITEM ( '' )  );
#34292=CARTESIAN_POINT ( 'NONE',  ( 0.7939632545931766261, -0.3162353388693409650, -0.4822834645669289433 ) ) ;
#34293=CARTESIAN_POINT ( 'NONE',  ( 1.574803149606299746, -0.1870078740157479769, 0.3641732283464567677 ) ) ;
#34295=CARTESIAN_POINT ( 'NONE',  ( -0.8727034120734901146, -0.08942795157528024563, -0.3641732283464568787 ) ) ;
#34296=CARTESIAN_POINT ( 'NONE',  ( -1.620734908136482577, 0.1771653543307087630, 0.09757992244046791164 ) ) ;
#34298=CARTESIAN_POINT ( 'NONE',  ( 0.5511811023622054106, -0.1870078740157480879, -0.4822834645669291653 ) ) ;
#34299=CARTESIAN_POINT ( 'NONE',  ( -0.7874015748031489847, -0.1870078740157480601, -0.3641732283464567677 ) ) ;
#34300=CARTESIAN_POINT ( 'NONE',  ( -0.1246719160104980823, 0.1771653543307087630, 0.09757992244046791164 ) ) ;
#34301=CARTESIAN_POINT ( 'NONE',  ( -0.1115485564304456306, 0.2952755905511810774, -0.1292274648535930714 ) ) ;
#34302=CARTESIAN_POINT ( 'NONE',  ( -1.515748031496062076, -0.4536011799217367080, 0.2665933059059888421 ) ) ;
#34304=CARTESIAN_POINT ( 'NONE',  ( 0.5708661417322841158, -0.5400638737290845981, -0.3530559997133363437 ) ) ;
#34305=CARTESIAN_POINT ( 'NONE',  ( -1.653543307086613234, -0.1870078740157479769, 0.4822834645669291653 ) ) ;
#34307=CARTESIAN_POINT ( 'NONE',  ( -0.6889763779527552368, -0.5400638737290845981, -0.3530559997133363437 ) ) ;
#34308=CARTESIAN_POINT ( 'NONE',  ( 0.01312335958005323398, -0.004921259842519576551, 0.3153832671262227771 ) ) ;
#34309=CARTESIAN_POINT ( 'NONE',  ( -1.469816272965878357, 0.2306618581243848609, 0.2411417322834645549 ) ) ;
#34310=CARTESIAN_POINT ( 'NONE',  ( 0.5708661417322842269, 0.07958543189024085140, 0.2665933059059887866 ) ) ;
#34311=CONICAL_SURFACE ( 'NONE', #26240, 1.220472440944881942, 0.7853981633974621568 ) ;
#34312=CARTESIAN_POINT ( 'NONE',  ( -0.7283464566929126471, 0.07958543189024071263, -0.2665933059059888421 ) ) ;
#34313=CARTESIAN_POINT ( 'NONE',  ( -1.174540682414697335, -0.3162353388693409650, -0.4822834645669289433 ) ) ;
#34314=CARTESIAN_POINT ( 'NONE',  ( -1.686351706036744558, 0.2952755905511810774, -0.1292274648535930714 ) ) ;
#34315=CARTESIAN_POINT ( 'NONE',  ( 1.437007874015748810, -0.5400638737290845981, -0.3530559997133363437 ) ) ;
#34317=CARTESIAN_POINT ( 'NONE',  ( 0.8858267716535438430, 0.07958543189024085140, 0.2665933059059887866 ) ) ;
#34318=CARTESIAN_POINT ( 'NONE',  ( 0.4068241469816281097, 0.05413385826771666132, 0.4176697321401328100 ) ) ;
#34319=CARTESIAN_POINT ( 'NONE',  ( -1.437007874015747477, 0.1660481256975883668, -0.3530559997133364547 ) ) ;
#34320=CARTESIAN_POINT ( 'NONE',  ( 1.364829396325459854, -0.5023911411419708095, -0.1820866141732282451 ) ) ;
#34321=VERTEX_POINT ( 'NONE', #15677 ) ;
#34323=CARTESIAN_POINT ( 'NONE',  ( -1.253280839895012377, -0.2845877964562161244, -0.3641732283464567121 ) ) ;
#34324=CARTESIAN_POINT ( 'NONE',  ( -0.2887139107611542133, -0.6046776061558809534, -0.2411417322834644161 ) ) ;
#34325=CARTESIAN_POINT ( 'NONE',  ( 0.4986876640419954376, 0.2306618581243848609, 0.2411417322834645549 ) ) ;
#34326=CARTESIAN_POINT ( 'NONE',  ( -1.377952755905511140, 0.1771653543307087630, 0.000000000000000000 ) ) ;
#34328=CARTESIAN_POINT ( 'NONE',  ( -1.227034120734907585, 0.2952755905511811885, 0.1292274648535926551 ) ) ;
#34329=CARTESIAN_POINT ( 'NONE',  ( 0.3280839895013130669, -0.4281496062992127816, -0.4176697321401328100 ) ) ;
#34330=CARTESIAN_POINT ( 'NONE',  ( 0.05905511811023709395, -0.5400638737290844871, 0.3530559997133364547 ) ) ;
#34331=CARTESIAN_POINT ( 'NONE',  ( 1.384514435695538337, -0.6692913385826771977, 0.1292274648535927661 ) ) ;
#34337=CARTESIAN_POINT ( 'NONE',  ( -0.3149606299212590610, -0.1870078740157479769, 0.3641732283464567677 ) ) ;
#34338=CARTESIAN_POINT ( 'NONE',  ( -0.3937007874015740483, -0.1870078740157480879, -0.4822834645669291653 ) ) ;
#34339=CARTESIAN_POINT ( 'NONE',  ( 1.036745406824147508, -0.4281496062992127816, -0.4176697321401328100 ) ) ;
#34341=CARTESIAN_POINT ( 'NONE',  ( 0.09186351706036827158, -0.004921259842519576551, 0.3153832671262227771 ) ) ;
#34342=CARTESIAN_POINT ( 'NONE',  ( -1.220472440944881054, -0.6692913385826771977, 8.415575281601705876E-17 ) ) ;
#34343=CARTESIAN_POINT ( 'NONE',  ( 1.548556430446194954, -0.6046776061558807314, 0.2411417322834647770 ) ) ;
#34347=ORIENTED_EDGE ( 'NONE', *, *, #51054, .F. ) ;
#34348=CARTESIAN_POINT ( 'NONE',  ( 1.253280839895013710, -0.3162353388693405765, 0.4822834645669290543 ) ) ;
#34349=CARTESIAN_POINT ( 'NONE',  ( 1.528871391076116026, -0.5511811023622048555, -0.09757992244046775898 ) ) ;
#34350=CARTESIAN_POINT ( 'NONE',  ( -1.377952755905511140, -0.5511811023622047445, 6.969142054262312111E-17 ) ) ;
#34351=CARTESIAN_POINT ( 'NONE',  ( -1.377952755905511140, -0.6692913385826771977, 8.415575281601705876E-17 ) ) ;
#34353=DIRECTION ( 'NONE',  ( 1.000000000000000000, -0.000000000000000000, -0.000000000000000000 ) ) ;
#34354=CARTESIAN_POINT ( 'NONE',  ( 1.128608923884515169, -0.6046776061558809534, -0.2411417322834644161 ) ) ;
#34355=CARTESIAN_POINT ( 'NONE',  ( -1.502624671916009680, -0.05778040916215560624, -0.4822834645669293319 ) ) ;
#34356=CARTESIAN_POINT ( 'NONE',  ( -0.2493438320209966919, 0.05413385826771626580, -0.4176697321401330321 ) ) ;
#34357=CARTESIAN_POINT ( 'NONE',  ( -0.03280839895013062252, -0.6692913385826771977, 0.1292274648535927661 ) ) ;
#34358=CARTESIAN_POINT ( 'NONE',  ( -1.240157480314959759, -0.5400638737290845981, -0.3530559997133363437 ) ) ;
#34360=CARTESIAN_POINT ( 'NONE',  ( 0.4133858267716541968, -0.5400638737290845981, -0.3530559997133363437 ) ) ;
#34362=CARTESIAN_POINT ( 'NONE',  ( -1.233595800524933894, -0.5023911411419708095, -0.1820866141732282451 ) ) ;
#34366=LINE ( 'NONE', #8696, #4545 ) ;
#34368=CARTESIAN_POINT ( 'NONE',  ( -1.102362204724408601, -0.1870078740157479769, 0.4822834645669291653 ) ) ;
#34369=CARTESIAN_POINT ( 'NONE',  ( -1.292650918635170010, 0.2952755905511810774, -0.1292274648535930714 ) ) ;
#34371=CARTESIAN_POINT ( 'NONE',  ( -1.541994750656167090, 0.2952755905511811885, 0.1292274648535926551 ) ) ;
#34374=CARTESIAN_POINT ( 'NONE',  ( -0.3265464962716608799, 0.02791078216816347476, -0.4328096321851898631 ) ) ;
#34376=CARTESIAN_POINT ( 'NONE',  ( -0.07874015748031421014, -0.1870078740157479769, 0.3641732283464567677 ) ) ;
#34377=CARTESIAN_POINT ( 'NONE',  ( -0.7939632545931754048, -0.2845877964562159024, 0.3641732283464567677 ) ) ;
#34378=CARTESIAN_POINT ( 'NONE',  ( -1.371391076115484609, -0.6692913385826771977, 0.1292274648535927661 ) ) ;
#34379=CARTESIAN_POINT ( 'NONE',  ( 1.108923884514436242, -0.05778040916215522460, 0.4822834645669289988 ) ) ;
#34380=CARTESIAN_POINT ( 'NONE',  ( -0.7283464566929126471, -0.5400638737290844871, 0.3530559997133364547 ) ) ;
#34382=ORIENTED_EDGE ( 'NONE', *, *, #76459, .F. ) ;
#34383=CARTESIAN_POINT ( 'NONE',  ( -1.496062992125983815, -0.1870078740157479769, 0.4822834645669291653 ) ) ;
#34384=CARTESIAN_POINT ( 'NONE',  ( -1.437007874015747477, -0.4536011799217367080, 0.2665933059059888421 ) ) ;
#34385=CARTESIAN_POINT ( 'NONE',  ( -1.666666666666665853, 0.05413385826771626580, -0.4176697321401330321 ) ) ;
#34390=CARTESIAN_POINT ( 'NONE',  ( -0.3083989501312330295, -0.3162353388693409650, -0.4822834645669289433 ) ) ;
#34391=CARTESIAN_POINT ( 'NONE',  ( -1.456692913385826182, 0.1771653543307087630, 0.000000000000000000 ) ) ;
#34393=CARTESIAN_POINT ( 'NONE',  ( -1.620734908136482577, -0.6692913385826773087, -0.1292274648535924053 ) ) ;
#34395=CARTESIAN_POINT ( 'NONE',  ( -1.502624671916009680, -0.05778040916215560624, -0.4822834645669293319 ) ) ;
#34396=CARTESIAN_POINT ( 'NONE',  ( -0.5577427821522301654, -0.05778040916215560624, -0.4822834645669293319 ) ) ;
#34398=CARTESIAN_POINT ( 'NONE',  ( 0.6627296587926515548, 0.1771653543307087630, 0.09757992244046791164 ) ) ;
#34400=CARTESIAN_POINT ( 'NONE',  ( 0.5314960629921267055, -0.4536011799217367080, 0.2665933059059888421 ) ) ;
#34401=CARTESIAN_POINT ( 'NONE',  ( 0.9776902887139113929, 0.1771653543307087630, 0.09757992244046791164 ) ) ;
#34402=CARTESIAN_POINT ( 'NONE',  ( 1.062992125984252745, -0.6692913385826771977, 8.415575281601705876E-17 ) ) ;
#34403=CARTESIAN_POINT ( 'NONE',  ( -0.4330708661417315697, -0.5511811023622047445, 6.969142054262312111E-17 ) ) ;
#34405=CARTESIAN_POINT ( 'NONE',  ( -1.200787401574802349, -0.5400638737290844871, 0.3530559997133364547 ) ) ;
#34406=CARTESIAN_POINT ( 'NONE',  ( 0.05905511811023681640, 0.07958543189024071263, -0.2665933059059888421 ) ) ;
#34407=CARTESIAN_POINT ( 'NONE',  ( -1.253280839895012377, -0.2845877964562161244, -0.3641732283464567121 ) ) ;
#34410=CARTESIAN_POINT ( 'NONE',  ( -1.128608923884513837, 0.1283753931104746893, -0.1820866141732285504 ) ) ;
#34411=CARTESIAN_POINT ( 'NONE',  ( -1.220472440944882386, 0.000000000000000000, 0.000000000000000000 ) ) ;
#34412=CARTESIAN_POINT ( 'NONE',  ( -0.2034120734908128059, 0.2952755905511811885, 0.1292274648535926551 ) ) ;
#34413=CARTESIAN_POINT ( 'NONE',  ( 1.581364829396326277, -0.2845877964562161244, -0.3641732283464567121 ) ) ;
#34414=CARTESIAN_POINT ( 'NONE',  ( 0.3871391076115492380, -0.08942795157528024563, -0.3641732283464568787 ) ) ;
#34415=CARTESIAN_POINT ( 'NONE',  ( -0.2230971128608915943, -0.3690944881889765550, -0.3153832671262227771 ) ) ;
#34416=CARTESIAN_POINT ( 'NONE',  ( -0.2296587926509179312, -0.05778040916215522460, 0.4822834645669289988 ) ) ;
#34417=CARTESIAN_POINT ( 'NONE',  ( -1.646981627296586703, -0.3162353388693409650, -0.4822834645669289433 ) ) ;
#34418=CARTESIAN_POINT ( 'NONE',  ( -1.010498687664041384, -0.004921259842519576551, 0.3153832671262227771 ) ) ;
#34420=CARTESIAN_POINT ( 'NONE',  ( 0.5249343832021005074, -0.6046776061558807314, 0.2411417322834647770 ) ) ;
#34421=ORIENTED_EDGE ( 'NONE', *, *, #39648, .F. ) ;
#34425=CARTESIAN_POINT ( 'NONE',  ( 1.397637795275591177, -0.5400638737290844871, 0.3530559997133364547 ) ) ;
#34426=CARTESIAN_POINT ( 'NONE',  ( -0.1771653543307080136, -0.4536011799217367080, 0.2665933059059888421 ) ) ;
#34428=CARTESIAN_POINT ( 'NONE',  ( -0.04593175853018302557, -0.6692913385826773087, -0.1292274648535924053 ) ) ;
#34429=CARTESIAN_POINT ( 'NONE',  ( -1.587926509186350810, 0.05413385826771626580, -0.4176697321401330321 ) ) ;
#34430=CARTESIAN_POINT ( 'NONE',  ( -1.496062992125983815, -0.1870078740157479769, 0.3641732283464567677 ) ) ;
#34431=CARTESIAN_POINT ( 'NONE',  ( 1.253280839895013710, -0.05778040916215560624, -0.4822834645669293319 ) ) ;
#34432=CARTESIAN_POINT ( 'NONE',  ( -0.5511811023622041894, -0.1870078740157480601, -0.3641732283464567677 ) ) ;
#34433=CARTESIAN_POINT ( 'NONE',  ( 0.4556365134843000653, 1.537493841523237759, 0.5309055118110234117 ) ) ;
#34437=CARTESIAN_POINT ( 'NONE',  ( 0.9973753280839902091, 0.1283753931104746893, -0.1820866141732285504 ) ) ;
#34438=CARTESIAN_POINT ( 'NONE',  ( -1.246719160104986512, 0.05413385826771666132, 0.4176697321401328100 ) ) ;
#34439=CARTESIAN_POINT ( 'NONE',  ( 1.279527559055118724, 0.1660481256975885056, 0.3530559997133364547 ) ) ;
#34441=CARTESIAN_POINT ( 'NONE',  ( 1.338582677165355062, -0.1870078740157479769, 0.3641732283464567677 ) ) ;
#34442=CARTESIAN_POINT ( 'NONE',  ( -0.03280839895013062252, 0.2952755905511810774, -0.1292274648535930714 ) ) ;
#34443=CARTESIAN_POINT ( 'NONE',  ( -0.3740157480314953431, 0.1660481256975885056, 0.3530559997133364547 ) ) ;
#34444=CARTESIAN_POINT ( 'NONE',  ( 1.594488188976378673, -0.5400638737290845981, -0.3530559997133363437 ) ) ;
#34446=CARTESIAN_POINT ( 'NONE',  ( 0.1837270341207354329, 0.1283753931104748280, 0.1820866141732283561 ) ) ;
#34450=CARTESIAN_POINT ( 'NONE',  ( -0.3937007874015740483, -0.1870078740157480879, -0.4822834645669291653 ) ) ;
#34451=CARTESIAN_POINT ( 'NONE',  ( 1.233595800524935227, -0.6046776061558807314, 0.2411417322834647770 ) ) ;
#34452=CARTESIAN_POINT ( 'NONE',  ( 0.4133858267716541968, 0.1660481256975885056, 0.3530559997133364547 ) ) ;
#34453=CARTESIAN_POINT ( 'NONE',  ( -0.3805774278215216522, -0.004921259842519576551, 0.3153832671262227771 ) ) ;
#34454=CARTESIAN_POINT ( 'NONE',  ( 0.6889763779527566800, -0.5400638737290844871, 0.3530559997133364547 ) ) ;
#34455=CARTESIAN_POINT ( 'NONE',  ( -0.8858267716535425107, -0.5400638737290844871, 0.3530559997133364547 ) ) ;
#34456=CARTESIAN_POINT ( 'NONE',  ( -0.6036745406824141069, 0.2306618581243848609, 0.2411417322834645549 ) ) ;
#34457=CARTESIAN_POINT ( 'NONE',  ( -0.6955380577427815458, -0.4281496062992127816, -0.4176697321401328100 ) ) ;
#34458=CARTESIAN_POINT ( 'NONE',  ( 1.122047244094488860, 0.1660481256975885056, 0.3530559997133364547 ) ) ;
#34459=CARTESIAN_POINT ( 'NONE',  ( 0.9251968503937015864, -0.5400638737290844871, 0.3530559997133364547 ) ) ;
#34460=CARTESIAN_POINT ( 'NONE',  ( 1.240157480314961314, 0.1660481256975883668, -0.3530559997133364547 ) ) ;
#34462=CARTESIAN_POINT ( 'NONE',  ( 0.2230971128608932319, -0.3690944881889763329, 0.3153832671262228327 ) ) ;
#34463=VERTEX_POINT ( 'NONE', #41734 ) ;
#34465=CONICAL_SURFACE ( 'NONE', #45178, 3.582677165354331450, 0.5235987755982945968 ) ;
#34467=CARTESIAN_POINT ( 'NONE',  ( -0.7742782152230965886, -0.004921259842519576551, 0.3153832671262227771 ) ) ;
#34470=CARTESIAN_POINT ( 'NONE',  ( -0.2230971128608915943, 0.05413385826771666132, 0.4176697321401328100 ) ) ;
#34472=CARTESIAN_POINT ( 'NONE',  ( -0.1837270341207343505, -0.6046776061558807314, 0.2411417322834647770 ) ) ;
#34473=CARTESIAN_POINT ( 'NONE',  ( -0.2624671916010490880, 0.2306618581243847221, -0.2411417322834647770 ) ) ;
#34474=CARTESIAN_POINT ( 'NONE',  ( -0.9580052493438311334, 0.05413385826771626580, -0.4176697321401330321 ) ) ;
#34475=CARTESIAN_POINT ( 'NONE',  ( -1.404199475065615932, 0.05413385826771666132, 0.4176697321401328100 ) ) ;
#34476=CARTESIAN_POINT ( 'NONE',  ( 1.358267716535433323, 0.07958543189024085140, 0.2665933059059887866 ) ) ;
#34479=CARTESIAN_POINT ( 'NONE',  ( 0.4330708661417329575, -0.5511811023622047445, 6.969142054262312111E-17 ) ) ;
#34480=CARTESIAN_POINT ( 'NONE',  ( -0.07217847769028787330, -0.05778040916215522460, 0.4822834645669289988 ) ) ;
#34481=CARTESIAN_POINT ( 'NONE',  ( 0.1640419947506569498, -0.3162353388693409650, -0.4822834645669289433 ) ) ;
#34484=CARTESIAN_POINT ( 'NONE',  ( -0.5971128608923876868, 0.2066929133858267931, 0.1054918080437490802 ) ) ;
#34487=CARTESIAN_POINT ( 'NONE',  ( -0.7480314960629914633, 0.2952755905511811885, 0.000000000000000000 ) ) ;
#34490=CARTESIAN_POINT ( 'NONE',  ( -1.450131233595799651, 0.1771653543307087075, -0.09757992244046823083 ) ) ;
#34491=CARTESIAN_POINT ( 'NONE',  ( 0.8727034120734912248, -0.3162353388693409650, -0.4822834645669289433 ) ) ;
#34493=CARTESIAN_POINT ( 'NONE',  ( 0.7742782152230979209, 0.05413385826771626580, -0.4176697321401330321 ) ) ;
#34494=CARTESIAN_POINT ( 'NONE',  ( -0.3412073490813641308, 0.1283753931104746893, -0.1820866141732285504 ) ) ;
#34495=CARTESIAN_POINT ( 'NONE',  ( 0.1049868766404206816, -0.6046776061558809534, -0.2411417322834644161 ) ) ;
#34497=CARTESIAN_POINT ( 'NONE',  ( -0.1902887139107604098, 0.1771653543307087075, -0.09757992244046823083 ) ) ;
#34498=CARTESIAN_POINT ( 'NONE',  ( -0.4068241469816267775, 0.05413385826771626580, -0.4176697321401330321 ) ) ;
#34500=CARTESIAN_POINT ( 'NONE',  ( -1.627296587926508442, -0.6046776061558809534, -0.2411417322834644161 ) ) ;
#34501=CARTESIAN_POINT ( 'NONE',  ( 0.3018372703412079971, -0.3690944881889763329, 0.3153832671262228327 ) ) ;
#34503=CARTESIAN_POINT ( 'NONE',  ( -1.049868766404198794, 0.2306618581243847221, -0.2411417322834647770 ) ) ;
#34504=CARTESIAN_POINT ( 'NONE',  ( -0.8595800524934373854, -0.08942795157527998196, 0.3641732283464567121 ) ) ;
#34506=CARTESIAN_POINT ( 'NONE',  ( -0.8005249343832013809, -0.4281496062992124485, 0.4176697321401328655 ) ) ;
#34507=CARTESIAN_POINT ( 'NONE',  ( -0.5905511811023613777, -0.6692913385826771977, 8.415575281601705876E-17 ) ) ;
#34508=CARTESIAN_POINT ( 'NONE',  ( 0.006561679790026889343, -0.3162353388693409650, -0.4822834645669289433 ) ) ;
#34512=CARTESIAN_POINT ( 'NONE',  ( 0.4658792650918641698, -0.08942795157528024563, -0.3641732283464568787 ) ) ;
#34513=CARTESIAN_POINT ( 'NONE',  ( 0.9317585301837276734, -0.4281496062992124485, 0.4176697321401328655 ) ) ;
#34514=CARTESIAN_POINT ( 'NONE',  ( -1.325459317585300889, -0.3690944881889765550, -0.3153832671262227771 ) ) ;
#34515=CARTESIAN_POINT ( 'NONE',  ( 1.345144356955381593, -0.05778040916215522460, 0.4822834645669289988 ) ) ;
#34516=CARTESIAN_POINT ( 'NONE',  ( -1.056430446194224881, 0.1771653543307087075, -0.09757992244046823083 ) ) ;
#34517=CARTESIAN_POINT ( 'NONE',  ( -0.7283464566929126471, 0.1660481256975883668, -0.3530559997133364547 ) ) ;
#34518=CARTESIAN_POINT ( 'NONE',  ( 0.1706036745406830368, -0.3690944881889765550, -0.3153832671262227771 ) ) ;
#34520=CARTESIAN_POINT ( 'NONE',  ( 0.8267716535433077274, 0.1771653543307087630, 0.000000000000000000 ) ) ;
#34521=CARTESIAN_POINT ( 'NONE',  ( 0.4790026246719168435, -0.3162353388693409650, -0.4822834645669289433 ) ) ;
#34523=EDGE_CURVE ( 'NONE', #82183, #25632, #26924, .T. ) ;
#34524=CARTESIAN_POINT ( 'NONE',  ( -0.8398950131233589023, -0.6046776061558809534, -0.2411417322834644161 ) ) ;
#34527=CARTESIAN_POINT ( 'NONE',  ( 1.207349081364829990, -0.5023911411419708095, -0.1820866141732282451 ) ) ;
#34528=AXIS2_PLACEMENT_3D ( 'NONE', #80029, #81258, #16461 ) ;
#34529=CARTESIAN_POINT ( 'NONE',  ( -0.02624671916010428221, 0.2306618581243847221, -0.2411417322834647770 ) ) ;
#34530=CARTESIAN_POINT ( 'NONE',  ( -0.1902887139107604098, 0.2952755905511810774, -0.1292274648535930714 ) ) ;
#34531=CARTESIAN_POINT ( 'NONE',  ( -0.2296587926509179312, -0.08942795157527998196, 0.3641732283464567121 ) ) ;
#34532=CARTESIAN_POINT ( 'NONE',  ( 0.1509186351706045259, -0.08942795157528024563, -0.3641732283464568787 ) ) ;
#34533=CARTESIAN_POINT ( 'NONE',  ( 0.5643044619422579178, 0.05413385826771666132, 0.4176697321401328100 ) ) ;
#34534=CARTESIAN_POINT ( 'NONE',  ( -0.5971128608923877978, 0.1771653543307087630, 0.09757992244046791164 ) ) ;
#34536=CARTESIAN_POINT ( 'NONE',  ( -1.036745406824146176, -0.4281496062992124485, 0.4176697321401328655 ) ) ;
#34539=CARTESIAN_POINT ( 'NONE',  ( -1.122047244094487306, -0.4536011799217367080, 0.2665933059059888421 ) ) ;
#34540=CARTESIAN_POINT ( 'NONE',  ( -0.2034120734908131112, -0.6692913385826773087, -0.1292274648535924053 ) ) ;
#34542=CARTESIAN_POINT ( 'NONE',  ( -0.6955380577427815458, 0.05413385826771666132, 0.4176697321401328100 ) ) ;
#34544=CARTESIAN_POINT ( 'NONE',  ( 1.213910761154856299, 0.2952755905511811885, 0.1292274648535926551 ) ) ;
#34545=CARTESIAN_POINT ( 'NONE',  ( 1.056430446194226658, 0.2952755905511811885, 0.1292274648535926551 ) ) ;
#34549=CARTESIAN_POINT ( 'NONE',  ( 1.443569553805774897, 0.1283753931104748280, 0.1820866141732283561 ) ) ;
#34551=ORIENTED_EDGE ( 'NONE', *, *, #78501, .T. ) ;
#34552=CARTESIAN_POINT ( 'NONE',  ( -0.3608923884514428360, 0.1771653543307087630, 0.09757992244046791164 ) ) ;
#34555=CARTESIAN_POINT ( 'NONE',  ( 0.7611548556430451917, -0.6046776061558807314, 0.2411417322834647770 ) ) ;
#34556=CARTESIAN_POINT ( 'NONE',  ( 0.1574803149606306130, -0.1870078740157479769, 0.4822834645669291653 ) ) ;
#34557=CARTESIAN_POINT ( 'NONE',  ( -0.8858267716535425107, -0.5400638737290844871, 0.3530559997133364547 ) ) ;
#34558=CARTESIAN_POINT ( 'NONE',  ( 1.476377952755906442, -0.5400638737290844871, 0.3530559997133364547 ) ) ;
#34559=CARTESIAN_POINT ( 'NONE',  ( -0.8005249343832011588, -0.004921259842519870586, -0.3153832671262229437 ) ) ;
#34561=CARTESIAN_POINT ( 'NONE',  ( 0.4068241469816281097, 0.05413385826771666132, 0.4176697321401328100 ) ) ;
#34562=EDGE_CURVE ( 'NONE', #76682, #5541, #10600, .T. ) ;
#34563=CARTESIAN_POINT ( 'NONE',  ( 0.4330708661417329575, -0.5511811023622047445, 6.969142054262312111E-17 ) ) ;
#34564=CARTESIAN_POINT ( 'NONE',  ( -1.043307086614172041, -0.5400638737290844871, 0.3530559997133364547 ) ) ;
#34566=CARTESIAN_POINT ( 'NONE',  ( -1.286089238845143479, 0.2306618581243847221, -0.2411417322834647770 ) ) ;
#34567=CARTESIAN_POINT ( 'NONE',  ( -1.594488188976377563, -0.4536011799217367080, 0.2665933059059888421 ) ) ;
#34568=CARTESIAN_POINT ( 'NONE',  ( 0.9645669291338591078, -0.5400638737290845981, -0.3530559997133363437 ) ) ;
#34569=CARTESIAN_POINT ( 'NONE',  ( 1.450131233595801428, -0.5511811023622048555, -0.09757992244046775898 ) ) ;
#34572=CARTESIAN_POINT ( 'NONE',  ( -0.3477690288713902178, 0.2952755905511810774, -0.1292274648535930714 ) ) ;
#34574=CARTESIAN_POINT ( 'NONE',  ( 0.5446194225721792126, -0.08942795157528024563, -0.3641732283464568787 ) ) ;
#34575=CARTESIAN_POINT ( 'NONE',  ( -1.391076115485563758, 0.2306618581243848609, 0.2411417322834645549 ) ) ;
#34576=CARTESIAN_POINT ( 'NONE',  ( 1.036745406824147508, -0.4281496062992127816, -0.4176697321401328100 ) ) ;
#34577=CARTESIAN_POINT ( 'NONE',  ( 0.7283464566929140904, -0.5400638737290845981, -0.3530559997133363437 ) ) ;
#34578=CARTESIAN_POINT ( 'NONE',  ( -0.3083989501312330295, -0.05778040916215522460, 0.4822834645669289988 ) ) ;
#34579=CARTESIAN_POINT ( 'NONE',  ( -0.2230971128608915943, 0.05413385826771666132, 0.4176697321401328100 ) ) ;
#34581=CARTESIAN_POINT ( 'NONE',  ( -1.699475065616797398, 0.2952755905511811885, 0.1292274648535926551 ) ) ;
#34582=CARTESIAN_POINT ( 'NONE',  ( -0.8136482939632537770, 0.2306618581243847221, -0.2411417322834647770 ) ) ;
#34583=CARTESIAN_POINT ( 'NONE',  ( -0.5118110236220466680, 0.1771653543307087630, 0.000000000000000000 ) ) ;
#34584=CARTESIAN_POINT ( 'NONE',  ( 1.299212598425197429, -0.6692913385826771977, 8.415575281601705876E-17 ) ) ;
#34585=FACE_OUTER_BOUND ( 'NONE', #40363, .T. ) ;
#34586=CARTESIAN_POINT ( 'NONE',  ( -1.076115485564303809, 0.2306618581243848609, 0.2411417322834645549 ) ) ;
#34589=CARTESIAN_POINT ( 'NONE',  ( 0.8464566929133865436, 0.1660481256975883668, -0.3530559997133364547 ) ) ;
#34594=CARTESIAN_POINT ( 'NONE',  ( -0.2427821522309703550, -0.3162353388693405765, 0.4822834645669290543 ) ) ;
#34595=CARTESIAN_POINT ( 'NONE',  ( -1.272965879265091305, -0.004921259842519870586, -0.3153832671262229437 ) ) ;
#34596=CARTESIAN_POINT ( 'NONE',  ( 1.227034120734908917, 0.1771653543307087075, -0.09757992244046823083 ) ) ;
#34599=CARTESIAN_POINT ( 'NONE',  ( 1.338582677165355062, -0.1870078740157479769, 0.3641732283464567677 ) ) ;
#34600=CARTESIAN_POINT ( 'NONE',  ( 1.404199475065617264, -0.4281496062992124485, 0.4176697321401328655 ) ) ;
#34602=CARTESIAN_POINT ( 'NONE',  ( -0.1706036745406816491, -0.4281496062992124485, 0.4176697321401328655 ) ) ;
#34604=CARTESIAN_POINT ( 'NONE',  ( 1.489501312335958172, -0.08942795157528024563, -0.3641732283464568787 ) ) ;
#34605=CARTESIAN_POINT ( 'NONE',  ( 0.03280839895013198948, 0.2952755905511811885, 0.1292274648535926551 ) ) ;
#34607=CARTESIAN_POINT ( 'NONE',  ( 1.194225721784777594, 0.05413385826771666132, 0.4176697321401328100 ) ) ;
#34608=CARTESIAN_POINT ( 'NONE',  ( 0.3608923884514443348, 0.2952755905511810774, -0.1292274648535930714 ) ) ;
#34609=CARTESIAN_POINT ( 'NONE',  ( 0.5446194225721792126, -0.2845877964562159024, 0.3641732283464567677 ) ) ;
#34610=DIRECTION ( 'NONE',  ( 0.000000000000000000, 0.000000000000000000, 1.000000000000000000 ) ) ;
#34611=CARTESIAN_POINT ( 'NONE',  ( 0.2821522309711292364, 0.1771653543307087075, -0.09757992244046823083 ) ) ;
#34614=CARTESIAN_POINT ( 'NONE',  ( 0.8858267716535438430, 0.1660481256975885056, 0.3530559997133364547 ) ) ;
#34619=CARTESIAN_POINT ( 'NONE',  ( 0.05905511811023681640, 0.07958543189024071263, -0.2665933059059888421 ) ) ;
#34620=CARTESIAN_POINT ( 'NONE',  ( 0.03937007874015833325, -0.6692913385826771977, 8.415575281601705876E-17 ) ) ;
#34621=CARTESIAN_POINT ( 'NONE',  ( 1.535433070866142558, 0.1771653543307087630, 0.000000000000000000 ) ) ;
#34622=CARTESIAN_POINT ( 'NONE',  ( -1.502624671916009680, -0.08942795157528024563, -0.3641732283464568787 ) ) ;
#34623=CARTESIAN_POINT ( 'NONE',  ( -1.469816272965878357, -0.6046776061558809534, -0.2411417322834644161 ) ) ;
#34624=CARTESIAN_POINT ( 'NONE',  ( 0.6758530183727039509, -0.6692913385826771977, 0.1292274648535927661 ) ) ;
#34625=CARTESIAN_POINT ( 'NONE',  ( 1.574803149606299746, -0.1870078740157480879, -0.4822834645669291653 ) ) ;
#34627=CARTESIAN_POINT ( 'NONE',  ( 0.4921259842519691285, 0.1660481256975885056, 0.3530559997133364547 ) ) ;
#34629=CARTESIAN_POINT ( 'NONE',  ( 1.541994750656168645, 0.2952755905511810774, -0.1292274648535930714 ) ) ;
#34630=CARTESIAN_POINT ( 'NONE',  ( 0.9317585301837276734, 0.05413385826771626580, -0.4176697321401330321 ) ) ;
#34631=CARTESIAN_POINT ( 'NONE',  ( -1.417322834645668772, -0.1870078740157479769, 0.3641732283464567677 ) ) ;
#34632=CARTESIAN_POINT ( 'NONE',  ( 1.286089238845145033, -0.5023911411419708095, -0.1820866141732282451 ) ) ;
#34633=CARTESIAN_POINT ( 'NONE',  ( 1.509186351706037543, 0.05413385826771666132, 0.4176697321401328100 ) ) ;
#34634=CARTESIAN_POINT ( 'NONE',  ( -0.9186351706036736120, -0.5023911411419708095, -0.1820866141732282451 ) ) ;
#34635=CARTESIAN_POINT ( 'NONE',  ( 1.614173228346457378, 0.2952755905511811885, 0.000000000000000000 ) ) ;
#34636=CARTESIAN_POINT ( 'NONE',  ( 0.5052493438320215802, 0.1771653543307087630, 0.09757992244046791164 ) ) ;
#34637=CARTESIAN_POINT ( 'NONE',  ( 0.1706036745406830368, -0.4281496062992127816, -0.4176697321401328100 ) ) ;
#34638=CARTESIAN_POINT ( 'NONE',  ( 1.135170603674541256, 0.2952755905511811885, 0.1292274648535926551 ) ) ;
#34639=CARTESIAN_POINT ( 'NONE',  ( -0.3346456692913377662, 0.1660481256975883668, -0.3530559997133364547 ) ) ;
#34640=CARTESIAN_POINT ( 'NONE',  ( 0.3083989501312343062, -0.2845877964562159024, 0.3641732283464567677 ) ) ;
#34641=CARTESIAN_POINT ( 'NONE',  ( 1.279527559055118724, 0.1660481256975885056, 0.3530559997133364547 ) ) ;
#34642=CARTESIAN_POINT ( 'NONE',  ( -1.528871391076114250, -0.6692913385826771977, 0.1292274648535927661 ) ) ;
#34643=CARTESIAN_POINT ( 'NONE',  ( -0.9580052493438311334, -0.4281496062992124485, 0.4176697321401328655 ) ) ;
#34644=CARTESIAN_POINT ( 'NONE',  ( -1.502624671916009680, -0.08942795157528024563, -0.3641732283464568787 ) ) ;
#34646=CARTESIAN_POINT ( 'NONE',  ( 1.012524390108117345, 2.412178165100495768E-16, -0.3954985857520057491 ) ) ;
#34648=CARTESIAN_POINT ( 'NONE',  ( -0.9514435695538050464, -0.05778040916215560624, -0.4822834645669293319 ) ) ;
#34649=CARTESIAN_POINT ( 'NONE',  ( 0.1443569553805781891, -0.4281496062992124485, 0.4176697321401328655 ) ) ;
#34653=CARTESIAN_POINT ( 'NONE',  ( 0.6955380577427828781, -0.3690944881889763329, 0.3153832671262228327 ) ) ;
#34655=CARTESIAN_POINT ( 'NONE',  ( 1.128608923884514947, 0.2306618581243848609, 0.2411417322834645549 ) ) ;
#34657=CARTESIAN_POINT ( 'NONE',  ( -1.391076115485563758, 0.1283753931104748280, 0.1820866141732283561 ) ) ;
#34660=CARTESIAN_POINT ( 'NONE',  ( -1.404199475065615932, 0.05413385826771666132, 0.4176697321401328100 ) ) ;
#34662=CARTESIAN_POINT ( 'NONE',  ( 0.1902887139107617975, -0.6692913385826773087, -0.1292274648535924053 ) ) ;
#34663=CARTESIAN_POINT ( 'NONE',  ( -0.5314960629921254842, -0.4536011799217368745, -0.2665933059059886201 ) ) ;
#34664=CARTESIAN_POINT ( 'NONE',  ( 0.9186351706036751663, -0.6046776061558807314, 0.2411417322834647770 ) ) ;
#34665=CARTESIAN_POINT ( 'NONE',  ( 0.05249343832021075018, 0.2306618581243847221, -0.2411417322834647770 ) ) ;
#34668=DIRECTION ( 'NONE',  ( -3.096699300667737957E-16, 1.000000000000000000, -0.000000000000000000 ) ) ;
#34670=CARTESIAN_POINT ( 'NONE',  ( 0.8989501312335964611, 0.2952755905511811885, 0.1292274648535926551 ) ) ;
#34671=CARTESIAN_POINT ( 'NONE',  ( 0.2165354330708668673, 0.1660481256975883668, -0.3530559997133364547 ) ) ;
#34672=CARTESIAN_POINT ( 'NONE',  ( -1.227034120734907141, -0.6692913385826773087, -0.1292274648535924053 ) ) ;
#34673=CARTESIAN_POINT ( 'NONE',  ( -1.568241469816272105, -0.3162353388693409650, -0.4822834645669289433 ) ) ;
#34674=CARTESIAN_POINT ( 'NONE',  ( 0.9120734908136490793, 0.2952755905511810774, -0.1292274648535930714 ) ) ;
#34676=CARTESIAN_POINT ( 'NONE',  ( -0.2362204724409442680, -0.1870078740157480879, -0.4822834645669291653 ) ) ;
#34677=CARTESIAN_POINT ( 'NONE',  ( 0.4986876640419954376, -0.6046776061558809534, -0.2411417322834644161 ) ) ;
#34678=CARTESIAN_POINT ( 'NONE',  ( -0.09186351706036663400, -0.4281496062992124485, 0.4176697321401328655 ) ) ;
#34679=CARTESIAN_POINT ( 'NONE',  ( 0.5446194225721792126, -0.2845877964562159024, 0.3641732283464567677 ) ) ;
#34680=CARTESIAN_POINT ( 'NONE',  ( -1.384514435695537005, 0.2952755905511811885, 0.1292274648535926551 ) ) ;
#34681=CARTESIAN_POINT ( 'NONE',  ( -1.371391076115484831, 0.2952755905511810774, -0.1292274648535930714 ) ) ;
#34682=CARTESIAN_POINT ( 'NONE',  ( 0.7283464566929140904, -0.5400638737290845981, -0.3530559997133363437 ) ) ;
#34685=ORIENTED_EDGE ( 'NONE', *, *, #74375, .T. ) ;
#34688=CARTESIAN_POINT ( 'NONE',  ( 1.187664041994751285, -0.05778040916215522460, 0.4822834645669289988 ) ) ;
#34689=CARTESIAN_POINT ( 'NONE',  ( 0.6824146981627303710, 0.1283753931104746893, -0.1820866141732285504 ) ) ;
#34690=CARTESIAN_POINT ( 'NONE',  ( 0.4849061582275022153, 1.726086921369708538, 0.4921425059946342717 ) ) ;
#34691=ADVANCED_FACE ( 'NONE', ( #55186 ), #80894, .T. ) ;
#34696=CARTESIAN_POINT ( 'NONE',  ( -0.9448818897637790704, -0.1870078740157479769, 0.4822834645669291653 ) ) ;
#34697=CARTESIAN_POINT ( 'NONE',  ( 1.017060367454068581, -0.05778040916215560624, -0.4822834645669293319 ) ) ;
#34699=CARTESIAN_POINT ( 'NONE',  ( -1.601049868766403650, -0.6046776061558807314, 0.2411417322834647770 ) ) ;
#34704=CARTESIAN_POINT ( 'NONE',  ( -1.528871391076114250, -0.5511811023622046335, 0.09757992244046803654 ) ) ;
#34706=CARTESIAN_POINT ( 'NONE',  ( 0.3543307086614181922, -0.6692913385826771977, 8.415575281601705876E-17 ) ) ;
#34708=CARTESIAN_POINT ( 'NONE',  ( 1.423884514435696413, -0.3162353388693409650, -0.4822834645669289433 ) ) ;
#34709=CARTESIAN_POINT ( 'NONE',  ( -0.4461942257217840213, 0.1539470093639523085, 0.1968503937007873850 ) ) ;
#34710=CARTESIAN_POINT ( 'NONE',  ( -0.8005249343832013809, -0.3690944881889763329, 0.3153832671262228327 ) ) ;
#34711=CARTESIAN_POINT ( 'NONE',  ( 0.6233595800524942554, -0.05778040916215560624, -0.4822834645669293319 ) ) ;
#34712=CARTESIAN_POINT ( 'NONE',  ( 1.364829396325459854, -0.5023911411419708095, -0.1820866141732282451 ) ) ;
#34714=CARTESIAN_POINT ( 'NONE',  ( -0.6364829396325453192, -0.2845877964562159024, 0.3641732283464567677 ) ) ;
#34715=CARTESIAN_POINT ( 'NONE',  ( 1.292650918635171564, -0.6692913385826773087, -0.1292274648535924053 ) ) ;
#34717=CARTESIAN_POINT ( 'NONE',  ( 0.3608923884514443348, 0.2952755905511810774, -0.1292274648535930714 ) ) ;
#34718=EDGE_CURVE ( 'NONE', #33221, #9295, #53913, .T. ) ;
#34719=CARTESIAN_POINT ( 'NONE',  ( -0.9776902887139098386, 0.1771653543307087075, -0.09757992244046823083 ) ) ;
#34720=CARTESIAN_POINT ( 'NONE',  ( -0.1312335958005241554, 0.1283753931104748280, 0.1820866141732283561 ) ) ;
#34721=CARTESIAN_POINT ( 'NONE',  ( -0.3412073490813641308, -0.6046776061558807314, 0.2411417322834647770 ) ) ;
#34722=CARTESIAN_POINT ( 'NONE',  ( 1.587926509186352586, -0.4281496062992127816, -0.4176697321401328100 ) ) ;
#34724=CARTESIAN_POINT ( 'NONE',  ( 0.2427821522309716595, -0.3162353388693409650, -0.4822834645669289433 ) ) ;
#34726=CARTESIAN_POINT ( 'NONE',  ( -1.646981627296586703, -0.05778040916215522460, 0.4822834645669289988 ) ) ;
#34728=CARTESIAN_POINT ( 'NONE',  ( -0.9842519685039365918, -0.6692913385826771977, 8.415575281601705876E-17 ) ) ;
#34729=CARTESIAN_POINT ( 'NONE',  ( -0.3083989501312330295, -0.08942795157527998196, 0.3641732283464567121 ) ) ;
#34730=CARTESIAN_POINT ( 'NONE',  ( -1.200787401574802349, -0.5400638737290844871, 0.3530559997133364547 ) ) ;
#34731=CARTESIAN_POINT ( 'NONE',  ( 0.3215223097112867578, -0.2845877964562161244, -0.3641732283464567121 ) ) ;
#34732=CARTESIAN_POINT ( 'NONE',  ( -0.6233595800524928121, -0.08942795157527998196, 0.3641732283464567121 ) ) ;
#34733=CARTESIAN_POINT ( 'NONE',  ( -0.8792650918635160906, 0.05413385826771626580, -0.4176697321401330321 ) ) ;
#34734=CARTESIAN_POINT ( 'NONE',  ( -1.482939632545930975, -0.4281496062992127816, -0.4176697321401328100 ) ) ;
#34735=CARTESIAN_POINT ( 'NONE',  ( 1.450131233595801428, -0.6692913385826773087, -0.1292274648535924053 ) ) ;
#34737=CARTESIAN_POINT ( 'NONE',  ( 0.8202099737532814183, -0.5511811023622048555, -0.09757992244046775898 ) ) ;
#34738=CARTESIAN_POINT ( 'NONE',  ( 0.5839895013123367340, 0.2952755905511811885, 0.1292274648535926551 ) ) ;
#34740=CARTESIAN_POINT ( 'NONE',  ( 1.614173228346457378, 0.1771653543307087630, 0.000000000000000000 ) ) ;
#34744=CARTESIAN_POINT ( 'NONE',  ( -1.240157480314959759, -0.4536011799217368745, -0.2665933059059886201 ) ) ;
#34745=CARTESIAN_POINT ( 'NONE',  ( -0.4527559055118102749, -0.5400638737290845981, -0.3530559997133363437 ) ) ;
#34746=CARTESIAN_POINT ( 'NONE',  ( 0.3280839895013130669, 0.05413385826771666132, 0.4176697321401328100 ) ) ;
#34747=CARTESIAN_POINT ( 'NONE',  ( -1.646981627296586703, -0.2845877964562161244, -0.3641732283464567121 ) ) ;
#34749=CARTESIAN_POINT ( 'NONE',  ( -1.437007874015747477, -0.5400638737290844871, 0.3530559997133364547 ) ) ;
#34750=CARTESIAN_POINT ( 'NONE',  ( 0.6102362204724416372, 0.1660481256975883668, -0.3530559997133364547 ) ) ;
#34751=CARTESIAN_POINT ( 'NONE',  ( 0.1181102362204730916, 0.2952755905511811885, 0.000000000000000000 ) ) ;
#34752=CARTESIAN_POINT ( 'NONE',  ( 1.391076115485564868, -0.6046776061558807314, 0.2411417322834647770 ) ) ;
#34757=CARTESIAN_POINT ( 'NONE',  ( -0.7426113562972000981, 2.401574803149605586, -0.5309055118110235227 ) ) ;
#34759=CARTESIAN_POINT ( 'NONE',  ( 0.06561679790026316017, -0.004921259842519870586, -0.3153832671262229437 ) ) ;
#34760=CARTESIAN_POINT ( 'NONE',  ( -0.5249343832020990641, -0.6046776061558809534, -0.2411417322834644161 ) ) ;
#34761=CARTESIAN_POINT ( 'NONE',  ( 0.8858267716535438430, -0.5400638737290845981, -0.3530559997133363437 ) ) ;
#34763=CARTESIAN_POINT ( 'NONE',  ( 0.09842519685039434474, 0.07958543189024085140, 0.2665933059059887866 ) ) ;
#34765=CARTESIAN_POINT ( 'NONE',  ( -1.154855643044618851, 0.2306618581243848609, 0.2411417322834645549 ) ) ;
#34766=CARTESIAN_POINT ( 'NONE',  ( -1.568241469816272105, -0.3162353388693409650, -0.4822834645669289433 ) ) ;
#34770=EDGE_LOOP ( 'NONE', ( #13444, #80431, #73879, #26748 ) ) ;
#34771=CARTESIAN_POINT ( 'NONE',  ( 1.017060367454068581, -0.05778040916215560624, -0.4822834645669293319 ) ) ;
#34772=CARTESIAN_POINT ( 'NONE',  ( 1.541994750656168645, -0.5511811023622046335, 0.09757992244046803654 ) ) ;
#34773=CARTESIAN_POINT ( 'NONE',  ( -1.102362204724408601, -0.1870078740157480601, -0.3641732283464567677 ) ) ;
#34774=CARTESIAN_POINT ( 'NONE',  ( -1.076115485564303809, -0.6046776061558809534, -0.2411417322834644161 ) ) ;
#34777=CARTESIAN_POINT ( 'NONE',  ( 1.358267716535433323, 0.1660481256975885056, 0.3530559997133364547 ) ) ;
#34778=CARTESIAN_POINT ( 'NONE',  ( -1.660104986876639543, -0.05778040916215560624, -0.4822834645669293319 ) ) ;
#34779=CARTESIAN_POINT ( 'NONE',  ( -0.06561679790026180015, -0.4281496062992127816, -0.4176697321401328100 ) ) ;
#34780=CARTESIAN_POINT ( 'NONE',  ( -0.07217847769028813698, -0.3162353388693409650, -0.4822834645669289433 ) ) ;
#34781=CARTESIAN_POINT ( 'NONE',  ( -1.358267716535432434, -0.5400638737290844871, 0.3530559997133364547 ) ) ;
#34783=CARTESIAN_POINT ( 'NONE',  ( 0.3215223097112867578, -0.05778040916215522460, 0.4822834645669289988 ) ) ;
#34785=CARTESIAN_POINT ( 'NONE',  ( -1.305774278215222184, 0.1771653543307087630, 0.09757992244046791164 ) ) ;
#34786=ORIENTED_EDGE ( 'NONE', *, *, #81347, .F. ) ;
#34790=CARTESIAN_POINT ( 'NONE',  ( -1.646981627296586703, -0.3162353388693409650, -0.4822834645669289433 ) ) ;
#34792=CARTESIAN_POINT ( 'NONE',  ( -1.332020997375327642, -0.3162353388693409650, -0.4822834645669289433 ) ) ;
#34795=CARTESIAN_POINT ( 'NONE',  ( -0.3740157480314952876, 0.1660481256975885056, 0.3530559997133364547 ) ) ;
#34797=( BOUNDED_SURFACE ( )  B_SPLINE_SURFACE ( 1, 2, ( 
 ( #9082, #15824, #43813, #79798, #22530, #50142, #73888, #73475, #62793, #24880, #2764, #5535, #69104, #82561, #82160, #81753, #31200, #50548, #75839, #16228, #69518, #11452, #37109, #5127, #41875, #62367, #76252, #30792, #28423, #54083, #24476, #58109, #51369, #64021, #39604, #19832, #77072, #13109, #77496, #38762, #33303, #63608, #7632, #1321, #65293, #58964, #7198, #18988, #19406, #58538, #12273, #77918, #70758, #32447, #64439, #25709, #904, #5945, #37931, #45481, #6775, #57693, #26970, #31614, #57275, #82973, #475, #12688, #52215, #26130, #51792, #45057, #25292, #71178, #13520, #52635, #78340, #44229, #64860, #50958, #76655, #39176, #6362, #70332, #44635, #55, #38347, #32034, #32870, #26561, #69919, #20249, #45898, #71595, #13947, #72435, #28639, #34545, #66536, #2142, #59372, #79180, #47570, #9701, #67367, #35371, #41271, #27387, #1731, #8867, #66121, #46743, #21084, #59788, #40030, #53048, #14373, #54297, #80011, #22326, #61036, #34960, #40441, #34127, #8457, #21495, #73688, #47989, #21908, #40851, #20671, #73264, #60211, #65718, #72017, #78759, #3386, #79593, #29048, #8049, #33711, #27810, #53470, #53878, #16028, #15612, #66957, #41675, #14785, #47154, #9289, #2561, #46324, #72845, #15193, #28219, #54720, #60623, #2973, #10120, #42493, #62691, #16858, #3799, #75329, #37429, #22737, #75743, #4608, #69421, #69004, #42901, #50049, #24377, #5033, #80829, #30701, #55943, #36593, #62271, #55120, #74511, #11776, #68596, #31102, #80426, #56365, #10936, #4203, #68197, #18084, #81658, #29867, #49222, #30280, #74928, #63102, #16442, #43719, #5441, #48396, #74096, #43306, #23143, #55529, #11355, #42087, #82064, #23554, #23969, #17273, #61862, #37013, #67782, #35782, #49636, #17676, #61451, #29462, #48812, #10535, #81238, #36191, #76154, #24784, #58011, #83287, #70233, #71497, #50453, #18494, #44137, #44957, #25199, #64760, #70653, #19305, #38246, #12178, #31936, #376, #45800, #20150, #13845, #77394, #63514, #37836, #13009, #18893, #82876, #57177, #12588, #69829, #5844, #31520, #7099, #32769, #58436, #39503, #71080, #76565, #63924, #44542, #57597, #26459, #798, #26031, #76975, #56769, #51691, #38664, #50865, #6258, #25610, #65191, #32350, #7527, #51273, #64342, #6678, #19726, #45384, #52112, #13423, #39079, #77820, #82469, #66022, #8769, #53369, #33197, #7948, #71919, #52532, #67266, #65617, #9188, #46223, #78660, #15508, #52946, #39928, #28121, #73584, #58865, #28534, #40750, #22223, #21803, #79080, #2871, #60522, #41167, #33610, #66856, #34443, #72744, #15092, #59273, #27288, #47879, #21397, #1223, #26872, #34860, #47052, #40341, #20981, #54191, #60110, #8358, #2041, #66433, #27706, #15929, #78240, #79907, #41576, #20572, #14269, #79488, #1629, #34025, #47467, #46641, #72336, #59686, #14684, #2463, #53776, #73159, #35679, #41984, #16341, #67678, #23870, #74826, #10838, #81552, #10014, #75232, #29362, #61345, #4512, #49948, #35267, #4932, #17170, #81962, #49537, #55431, #62590, #36914, #17575, #3697, #43208, #68498, #49120, #42804, #55022, #80730, #24277, #81140, #43622, #9599, #68904, #23455, #16753, #23044, #30600, #36498, #42392, #61764, #62173, #4104, #75646, #28947, #56266, #17986, #60932, #3282, #55843, #48711, #68091, #11256, #54612, #80321, #36093, #30181, #29770, #74409, #22637, #48297, #73994, #10436, #12484, #82774, #693, #63004, #37331, #5343, #57495, #37735, #77289, #83186, #31834, #50768, #24689, #44440, #12904, #58331, #32664, #26349, #6578, #76054, #50357, #25509, #31415, #12077, #69733, #25096, #31002, #18398, #56670, #19620, #45282, #70977, #52010, #274, #5744, #76469, #57079, #70133, #38975, #13322, #70549, #6159, #69324, #38563, #51174, #82370, #44040, #63409, #77715, #44851, #20045, #18796, #38148, #63820, #76870, #19202, #64658, #6997, #51588, #64243, #11674, #32249, #57910, #25929, #45697, #72643, #47370, #9093, #52425, #21298, #78135, #46951, #46121, #2364, #71816, #20468, #14993, #79810, #39823, #14166, #65511, #15410, #34766, #40650, #78977, #60425, #66334, #2776, #54095, #52848, #20885, #40238, #59587, #8672, #71393, #28020 ),
 ( #7843, #33510, #60008, #27606, #53267, #59172, #7420, #1530, #53679, #8258, #34343, #79387, #27184, #21706, #73060, #41070, #1944, #33923, #78559, #66759, #46536, #14585, #72236, #28436, #65921, #13742, #1119, #39399, #65082, #33090, #58757, #26770, #54931, #80638, #23776, #43117, #54512, #22542, #30088, #22950, #4013, #42713, #49447, #68814, #3186, #17076, #17486, #10749, #36819, #68409, #62494, #30507, #75141, #11160, #28850, #16658, #61672, #41485, #67171, #9500, #48617, #81459, #55751, #36406, #74311, #42298, #80226, #29677, #4829, #56169, #35173, #60834, #48205, #41888, #73900, #22127, #62081, #16241, #29267, #4421, #73487, #47785, #67995, #10341, #36002, #3602, #15837, #67581, #9913, #23360, #55340, #35585, #61248, #81048, #49031, #74727, #70038, #50264, #6483, #12392, #44347, #63315, #37235, #56984, #25413, #70882, #45176, #13231, #19107, #5246, #62913, #38049, #43944, #24596, #82278, #37638, #17892, #30910, #75553, #32153, #57809, #176, #38881, #12809, #18300, #11984, #69639, #82681, #51488, #25829, #83092, #18706, #81872, #51077, #63725, #43529, #49853, #56577, #64560, #57401, #6897, #69228, #11575, #5653, #31319, #31736, #77191, #76775, #44755, #19523, #75962, #24998, #70451, #6065, #24184, #50673, #76372, #38463, #32568, #64149, #46019, #40973, #597, #40555, #78037, #64984, #53163, #15310, #26253, #53582, #65827, #47269, #46854, #20784, #27924, #2258, #66236, #58656, #8574, #33825, #14489, #40142, #32988, #52331, #72959, #46440, #8992, #58230, #34244, #72130, #65413, #20367, #79292, #59491, #7750, #27088, #8160, #52751, #66655, #77619, #21609, #51912, #19952, #72548, #45602, #21199, #71296, #13644, #59906, #39297, #7319, #78459, #1845, #1023, #26676, #71713, #1432, #14068, #39721, #78875, #33415, #27506, #59077, #14895, #68315, #68714, #79710, #53998, #47686, #54415, #60738, #61983, #16975, #35485, #17389, #35071, #9401, #75043, #34665, #61573, #36307, #81359, #41387, #10237, #67068, #35904, #3089, #74632, #28753, #80126, #3916, #60329, #22445, #48106, #73804, #4320, #23672, #29577, #67899, #49343, #55240, #43020, #2677, #41787, #9814, #29167, #48513, #80946, #28337, #42615, #29985, #74214, #23262, #22026, #73381, #15731, #16140, #61149, #67479, #3501, #54836, #80541, #22853, #16559, #42204, #48931, #10652, #55649, #76273, #69124, #56066, #30812, #76676, #56888, #57295, #37951, #62814, #69940, #82993, #44657, #50569, #82581, #37130, #70353, #75859, #63216, #11888, #63628, #18201, #5965, #49754, #5148, #37541, #24900, #69538, #5556, #43836, #31220, #12708, #32054, #43427, #11473, #19009, #18607, #44250, #31635, #38367, #57714, #75454, #25314, #6382, #51391, #11055, #50978, #64043, #77, #17792, #12295, #56477, #25730, #82180, #77095, #24497, #50163, #19427, #45079, #36713, #62388, #4726, #30400, #81774, #24084, #34457, #54207, #60126, #47894, #73602, #59701, #27720, #21413, #40763, #79503, #15944, #15525, #60537, #66448, #2477, #70782, #13133, #6798, #45503, #79094, #38784, #19854, #71200, #39199, #64882, #13543, #7221, #32893, #66873, #28136, #53792, #2056, #499, #53387, #34876, #8784, #41183, #21819, #47066, #47482, #9203, #2888, #73175, #28550, #72758, #79923, #15107, #22239, #64461, #32469, #58131, #26153, #51814, #77519, #25704, #56860, #18983, #39599, #39171, #19401, #12683, #25286, #899, #64435, #38341, #57688, #38758, #50, #77913, #24875, #52209, #45893, #26556, #20244, #51787, #63603, #64016, #19826, #82557, #64855, #32029, #77068, #51364, #70327, #45476, #50543, #76247, #6770, #45052, #44631, #71590, #18581, #44224, #69914, #70753, #57270, #13514, #13104, #32442, #6357, #12268, #58104, #470, #13942, #5530, #31194, #26126, #37926, #5939, #31609, #77491, #82968, #71173, #7193, #50954, #32865, #58533, #76651, #8451, #46738, #21904, #1316, #33298, #66532, #34122, #78755, #80008, #58959, #26965, #52630, #53465, #33706, #73259, #79174, #27805, #72430, #20666, #40436, #8863, #54293, #28635, #22321, #2557, #72012, #46319, #21490, #27382, #8044, #65713, #21080, #78335, #14368, #40025, #15608, #41267, #66953, #47985, #79589, #1725 ) ),
 .UNSPECIFIED., .F., .F., .F. ) 
 B_SPLINE_SURFACE_WITH_KNOTS ( ( 2, 2 ),
 ( 3, 2, 2, 2, 2, 2, 2, 2, 2, 2, 2, 2, 2, 2, 2, 2, 2, 2, 2, 2, 2, 2, 2, 2, 2, 2, 2, 2, 2, 2, 2, 2, 2, 2, 2, 2, 2, 2, 2, 2, 2, 2, 2, 2, 2, 2, 2, 2, 2, 2, 2, 2, 2, 2, 2, 2, 2, 2, 2, 2, 2, 2, 2, 2, 2, 2, 2, 2, 2, 2, 2, 2, 2, 2, 2, 2, 2, 2, 2, 2, 2, 2, 2, 2, 2, 2, 2, 2, 2, 2, 2, 2, 2, 2, 2, 2, 2, 2, 2, 2, 2, 2, 2, 2, 2, 2, 2, 2, 2, 2, 2, 2, 2, 2, 2, 2, 2, 2, 2, 2, 2, 2, 2, 2, 2, 2, 2, 2, 2, 2, 2, 2, 2, 2, 2, 2, 2, 2, 2, 2, 2, 2, 2, 2, 2, 2, 2, 2, 2, 2, 2, 2, 2, 2, 2, 2, 2, 2, 2, 2, 2, 2, 2, 2, 2, 2, 2, 2, 2, 2, 2, 2, 2, 2, 2, 2, 2, 2, 2, 2, 2, 2, 2, 2, 2, 2, 2, 2, 2, 2, 2, 2, 2, 2, 2, 2, 2, 2, 2, 2, 2, 2, 2, 2, 2, 2, 2, 2, 2, 2, 2, 2, 2, 2, 2, 2, 2, 2, 2, 2, 2, 2, 2, 2, 2, 2, 2, 2, 2, 2, 2, 2, 2, 2, 2, 2, 2, 2, 2, 2, 2, 2, 2, 2, 2, 2, 2, 2, 2, 2, 2, 2, 2, 2, 2, 3 ),
 ( 0.000000000000000000, 1.000000000000000000 ),
 ( 0.000000000000000000, 0.003787878787878787984, 0.007575757575757575968, 0.01136363636363636395, 0.01515151515151515194, 0.01893939393939393992, 0.02272727272727272790, 0.02651515151515151589, 0.03030303030303030387, 0.03409090909090908839, 0.03787878787878787984, 0.04166666666666666435, 0.04545454545454545581, 0.04924242424242424032, 0.05303030303030303177, 0.05681818181818181629, 0.06060606060606060774, 0.06439393939393939226, 0.06818181818181817677, 0.07196969696969697516, 0.07575757575757575968, 0.07954545454545454419, 0.08333333333333332871, 0.08712121212121212710, 0.09090909090909091161, 0.09469696969696969613, 0.09848484848484848064, 0.1022727272727272790, 0.1060606060606060635, 0.1098484848484848481, 0.1136363636363636326, 0.1174242424242424310, 0.1212121212121212155, 0.1250000000000000000, 0.1287878787878787845, 0.1325757575757575690, 0.1363636363636363535, 0.1401515151515151381, 0.1439393939393939503, 0.1477272727272727348, 0.1515151515151515194, 0.1553030303030303039, 0.1590909090909090884, 0.1628787878787878729, 0.1666666666666666574, 0.1704545454545454419, 0.1742424242424242542, 0.1780303030303030387, 0.1818181818181818232, 0.1856060606060606077, 0.1893939393939393923, 0.1931818181818181768, 0.1969696969696969613, 0.2007575757575757458, 0.2045454545454545581, 0.2083333333333333426, 0.2121212121212121271, 0.2159090909090909116, 0.2196969696969696961, 0.2234848484848484806, 0.2272727272727272652, 0.2310606060606060497, 0.2348484848484848619, 0.2386363636363636465, 0.2424242424242424310, 0.2462121212121212155, 0.2500000000000000000, 0.2537878787878787845, 0.2575757575757575690, 0.2613636363636363535, 0.2651515151515151381, 0.2689393939393939226, 0.2727272727272727071, 0.2765151515151514916, 0.2803030303030302761, 0.2840909090909091161, 0.2878787878787879007, 0.2916666666666666852, 0.2954545454545454697, 0.2992424242424242542, 0.3030303030303030387, 0.3068181818181818232, 0.3106060606060606077, 0.3143939393939393923, 0.3181818181818181768, 0.3219696969696969613, 0.3257575757575757458, 0.3295454545454545303, 0.3333333333333333148, 0.3371212121212120993, 0.3409090909090908839, 0.3446969696969697239, 0.3484848484848485084, 0.3522727272727272929, 0.3560606060606060774, 0.3598484848484848619, 0.3636363636363636465, 0.3674242424242424310, 0.3712121212121212155, 0.3750000000000000000, 0.3787878787878787845, 0.3825757575757575690, 0.3863636363636363535, 0.3901515151515151381, 0.3939393939393939226, 0.3977272727272727071, 0.4015151515151514916, 0.4053030303030302761, 0.4090909090909091161, 0.4128787878787879007, 0.4166666666666666852, 0.4204545454545454697, 0.4242424242424242542, 0.4280303030303030387, 0.4318181818181818232, 0.4356060606060606077, 0.4393939393939393923, 0.4431818181818181768, 0.4469696969696969613, 0.4507575757575757458, 0.4545454545454545303, 0.4583333333333333148, 0.4621212121212120993, 0.4659090909090908839, 0.4696969696969697239, 0.4734848484848485084, 0.4772727272727272929, 0.4810606060606060774, 0.4848484848484848619, 0.4886363636363636465, 0.4924242424242424310, 0.4962121212121212155, 0.5000000000000000000, 0.5037878787878787845, 0.5075757575757575690, 0.5113636363636363535, 0.5151515151515151381, 0.5189393939393939226, 0.5227272727272727071, 0.5265151515151514916, 0.5303030303030302761, 0.5340909090909090606, 0.5378787878787878451, 0.5416666666666666297, 0.5454545454545454142, 0.5492424242424241987, 0.5530303030303029832, 0.5568181818181817677, 0.5606060606060605522, 0.5643939393939394478, 0.5681818181818182323, 0.5719696969696970168, 0.5757575757575758013, 0.5795454545454545858, 0.5833333333333333703, 0.5871212121212121549, 0.5909090909090909394, 0.5946969696969697239, 0.5984848484848485084, 0.6022727272727272929, 0.6060606060606060774, 0.6098484848484848619, 0.6136363636363636465, 0.6174242424242424310, 0.6212121212121212155, 0.6250000000000000000, 0.6287878787878787845, 0.6325757575757575690, 0.6363636363636363535, 0.6401515151515151381, 0.6439393939393939226, 0.6477272727272727071, 0.6515151515151514916, 0.6553030303030302761, 0.6590909090909090606, 0.6628787878787878451, 0.6666666666666666297, 0.6704545454545454142, 0.6742424242424241987, 0.6780303030303029832, 0.6818181818181817677, 0.6856060606060605522, 0.6893939393939394478, 0.6931818181818182323, 0.6969696969696970168, 0.7007575757575758013, 0.7045454545454545858, 0.7083333333333333703, 0.7121212121212121549, 0.7159090909090909394, 0.7196969696969697239, 0.7234848484848485084, 0.7272727272727272929, 0.7310606060606060774, 0.7348484848484848619, 0.7386363636363636465, 0.7424242424242424310, 0.7462121212121212155, 0.7500000000000000000, 0.7537878787878787845, 0.7575757575757575690, 0.7613636363636363535, 0.7651515151515151381, 0.7689393939393939226, 0.7727272727272727071, 0.7765151515151514916, 0.7803030303030302761, 0.7840909090909090606, 0.7878787878787878451, 0.7916666666666666297, 0.7954545454545454142, 0.7992424242424241987, 0.8030303030303029832, 0.8068181818181817677, 0.8106060606060605522, 0.8143939393939394478, 0.8181818181818182323, 0.8219696969696970168, 0.8257575757575758013, 0.8295454545454545858, 0.8333333333333333703, 0.8371212121212121549, 0.8409090909090909394, 0.8446969696969697239, 0.8484848484848485084, 0.8522727272727272929, 0.8560606060606060774, 0.8598484848484848619, 0.8636363636363636465, 0.8674242424242424310, 0.8712121212121212155, 0.8750000000000000000, 0.8787878787878787845, 0.8825757575757575690, 0.8863636363636363535, 0.8901515151515151381, 0.8939393939393939226, 0.8977272727272727071, 0.9015151515151514916, 0.9053030303030302761, 0.9090909090909090606, 0.9128787878787878451, 0.9166666666666666297, 0.9204545454545454142, 0.9242424242424241987, 0.9280303030303029832, 0.9318181818181817677, 0.9356060606060605522, 0.9393939393939394478, 0.9431818181818182323, 0.9469696969696970168, 0.9507575757575758013, 0.9545454545454545858, 0.9583333333333333703, 0.9621212121212121549, 0.9659090909090909394 ),
 .UNSPECIFIED. ) 
 GEOMETRIC_REPRESENTATION_ITEM ( )  RATIONAL_B_SPLINE_SURFACE ( (
 ( 1.000000000000000000, 0.9659258262890683122, 1.000000000000000000, 0.9659258262890683122, 1.000000000000000000, 0.9659258262890683122, 1.000000000000000000, 0.9659258262890683122, 1.000000000000000000, 0.9659258262890683122, 1.000000000000000000, 0.9659258262890683122, 1.000000000000000000, 0.9659258262890683122, 1.000000000000000000, 0.9659258262890683122, 1.000000000000000000, 0.9659258262890683122, 1.000000000000000000, 0.9659258262890683122, 1.000000000000000000, 0.9659258262890683122, 1.000000000000000000, 0.9659258262890683122, 1.000000000000000000, 0.9659258262890683122, 1.000000000000000000, 0.9659258262890683122, 1.000000000000000000, 0.9659258262890683122, 1.000000000000000000, 0.9659258262890683122, 1.000000000000000000, 0.9659258262890683122, 1.000000000000000000, 0.9659258262890683122, 1.000000000000000000, 0.9659258262890683122, 1.000000000000000000, 0.9659258262890683122, 1.000000000000000000, 0.9659258262890683122, 1.000000000000000000, 0.9659258262890683122, 1.000000000000000000, 0.9659258262890683122, 1.000000000000000000, 0.9659258262890683122, 1.000000000000000000, 0.9659258262890683122, 1.000000000000000000, 0.9659258262890683122, 1.000000000000000000, 0.9659258262890683122, 1.000000000000000000, 0.9659258262890683122, 1.000000000000000000, 0.9659258262890683122, 1.000000000000000000, 0.9659258262890683122, 1.000000000000000000, 0.9659258262890683122, 1.000000000000000000, 0.9659258262890683122, 1.000000000000000000, 0.9659258262890683122, 1.000000000000000000, 0.9659258262890683122, 1.000000000000000000, 0.9659258262890683122, 1.000000000000000000, 0.9659258262890683122, 1.000000000000000000, 0.9659258262890683122, 1.000000000000000000, 0.9659258262890683122, 1.000000000000000000, 0.9659258262890683122, 1.000000000000000000, 0.9659258262890683122, 1.000000000000000000, 0.9659258262890683122, 1.000000000000000000, 0.9659258262890683122, 1.000000000000000000, 0.9659258262890683122, 1.000000000000000000, 0.9659258262890683122, 1.000000000000000000, 0.9659258262890683122, 1.000000000000000000, 0.9659258262890683122, 1.000000000000000000, 0.9659258262890683122, 1.000000000000000000, 0.9659258262890683122, 1.000000000000000000, 0.9659258262890683122, 1.000000000000000000, 0.9659258262890683122, 1.000000000000000000, 0.9659258262890683122, 1.000000000000000000, 0.9659258262890683122, 1.000000000000000000, 0.9659258262890683122, 1.000000000000000000, 0.9659258262890683122, 1.000000000000000000, 0.9659258262890683122, 1.000000000000000000, 0.9659258262890683122, 1.000000000000000000, 0.9659258262890683122, 1.000000000000000000, 0.9659258262890683122, 1.000000000000000000, 0.9659258262890683122, 1.000000000000000000, 0.9659258262890683122, 1.000000000000000000, 0.9659258262890683122, 1.000000000000000000, 0.9659258262890683122, 1.000000000000000000, 0.9659258262890683122, 1.000000000000000000, 0.9659258262890683122, 1.000000000000000000, 0.9659258262890683122, 1.000000000000000000, 0.9659258262890683122, 1.000000000000000000, 0.9659258262890683122, 1.000000000000000000, 0.9659258262890683122, 1.000000000000000000, 0.9659258262890683122, 1.000000000000000000, 0.9659258262890683122, 1.000000000000000000, 0.9659258262890683122, 1.000000000000000000, 0.9659258262890683122, 1.000000000000000000, 0.9659258262890683122, 1.000000000000000000, 0.9659258262890683122, 1.000000000000000000, 0.9659258262890683122, 1.000000000000000000, 0.9659258262890683122, 1.000000000000000000, 0.9659258262890683122, 1.000000000000000000, 0.9659258262890683122, 1.000000000000000000, 0.9659258262890683122, 1.000000000000000000, 0.9659258262890683122, 1.000000000000000000, 0.9659258262890683122, 1.000000000000000000, 0.9659258262890683122, 1.000000000000000000, 0.9659258262890683122, 1.000000000000000000, 0.9659258262890683122, 1.000000000000000000, 0.9659258262890683122, 1.000000000000000000, 0.9659258262890683122, 1.000000000000000000, 0.9659258262890683122, 1.000000000000000000, 0.9659258262890683122, 1.000000000000000000, 0.9659258262890683122, 1.000000000000000000, 0.9659258262890683122, 1.000000000000000000, 0.9659258262890683122, 1.000000000000000000, 0.9659258262890683122, 1.000000000000000000, 0.9659258262890683122, 1.000000000000000000, 0.9659258262890683122, 1.000000000000000000, 0.9659258262890683122, 1.000000000000000000, 0.9659258262890683122, 1.000000000000000000, 0.9659258262890683122, 1.000000000000000000, 0.9659258262890683122, 1.000000000000000000, 0.9659258262890683122, 1.000000000000000000, 0.9659258262890683122, 1.000000000000000000, 0.9659258262890683122, 1.000000000000000000, 0.9659258262890683122, 1.000000000000000000, 0.9659258262890683122, 1.000000000000000000, 0.9659258262890683122, 1.000000000000000000, 0.9659258262890683122, 1.000000000000000000, 0.9659258262890683122, 1.000000000000000000, 0.9659258262890683122, 1.000000000000000000, 0.9659258262890683122, 1.000000000000000000, 0.9659258262890683122, 1.000000000000000000, 0.9659258262890683122, 1.000000000000000000, 0.9659258262890683122, 1.000000000000000000, 0.9659258262890683122, 1.000000000000000000, 0.9659258262890683122, 1.000000000000000000, 0.9659258262890683122, 1.000000000000000000, 0.9659258262890683122, 1.000000000000000000, 0.9659258262890683122, 1.000000000000000000, 0.9659258262890683122, 1.000000000000000000, 0.9659258262890683122, 1.000000000000000000, 0.9659258262890683122, 1.000000000000000000, 0.9659258262890683122, 1.000000000000000000, 0.9659258262890683122, 1.000000000000000000, 0.9659258262890683122, 1.000000000000000000, 0.9659258262890683122, 1.000000000000000000, 0.9659258262890683122, 1.000000000000000000, 0.9659258262890683122, 1.000000000000000000, 0.9659258262890683122, 1.000000000000000000, 0.9659258262890683122, 1.000000000000000000, 0.9659258262890683122, 1.000000000000000000, 0.9659258262890683122, 1.000000000000000000, 0.9659258262890683122, 1.000000000000000000, 0.9659258262890683122, 1.000000000000000000, 0.9659258262890683122, 1.000000000000000000, 0.9659258262890683122, 1.000000000000000000, 0.9659258262890683122, 1.000000000000000000, 0.9659258262890683122, 1.000000000000000000, 0.9659258262890683122, 1.000000000000000000, 0.9659258262890683122, 1.000000000000000000, 0.9659258262890683122, 1.000000000000000000, 0.9659258262890683122, 1.000000000000000000, 0.9659258262890683122, 1.000000000000000000, 0.9659258262890683122, 1.000000000000000000, 0.9659258262890683122, 1.000000000000000000, 0.9659258262890683122, 1.000000000000000000, 0.9659258262890683122, 1.000000000000000000, 0.9659258262890683122, 1.000000000000000000, 0.9659258262890683122, 1.000000000000000000, 0.9659258262890683122, 1.000000000000000000, 0.9659258262890683122, 1.000000000000000000, 0.9659258262890683122, 1.000000000000000000, 0.9659258262890683122, 1.000000000000000000, 0.9659258262890683122, 1.000000000000000000, 0.9659258262890683122, 1.000000000000000000, 0.9659258262890683122, 1.000000000000000000, 0.9659258262890683122, 1.000000000000000000, 0.9659258262890683122, 1.000000000000000000, 0.9659258262890683122, 1.000000000000000000, 0.9659258262890683122, 1.000000000000000000, 0.9659258262890683122, 1.000000000000000000, 0.9659258262890683122, 1.000000000000000000, 0.9659258262890683122, 1.000000000000000000, 0.9659258262890683122, 1.000000000000000000, 0.9659258262890683122, 1.000000000000000000, 0.9659258262890683122, 1.000000000000000000, 0.9659258262890683122, 1.000000000000000000, 0.9659258262890683122, 1.000000000000000000, 0.9659258262890683122, 1.000000000000000000, 0.9659258262890683122, 1.000000000000000000, 0.9659258262890683122, 1.000000000000000000, 0.9659258262890683122, 1.000000000000000000, 0.9659258262890683122, 1.000000000000000000, 0.9659258262890683122, 1.000000000000000000, 0.9659258262890683122, 1.000000000000000000, 0.9659258262890683122, 1.000000000000000000, 0.9659258262890683122, 1.000000000000000000, 0.9659258262890683122, 1.000000000000000000, 0.9659258262890683122, 1.000000000000000000, 0.9659258262890683122, 1.000000000000000000, 0.9659258262890683122, 1.000000000000000000, 0.9659258262890683122, 1.000000000000000000, 0.9659258262890683122, 1.000000000000000000, 0.9659258262890683122, 1.000000000000000000, 0.9659258262890683122, 1.000000000000000000, 0.9659258262890683122, 1.000000000000000000, 0.9659258262890683122, 1.000000000000000000, 0.9659258262890683122, 1.000000000000000000, 0.9659258262890683122, 1.000000000000000000, 0.9659258262890683122, 1.000000000000000000, 0.9659258262890683122, 1.000000000000000000, 0.9659258262890683122, 1.000000000000000000, 0.9659258262890683122, 1.000000000000000000, 0.9659258262890683122, 1.000000000000000000, 0.9659258262890683122, 1.000000000000000000, 0.9659258262890683122, 1.000000000000000000, 0.9659258262890683122, 1.000000000000000000, 0.9659258262890683122, 1.000000000000000000, 0.9659258262890683122, 1.000000000000000000, 0.9659258262890683122, 1.000000000000000000, 0.9659258262890683122, 1.000000000000000000, 0.9659258262890683122, 1.000000000000000000, 0.9659258262890683122, 1.000000000000000000, 0.9659258262890683122, 1.000000000000000000, 0.9659258262890683122, 1.000000000000000000, 0.9659258262890683122, 1.000000000000000000, 0.9659258262890683122, 1.000000000000000000, 0.9659258262890683122, 1.000000000000000000, 0.9659258262890683122, 1.000000000000000000, 0.9659258262890683122, 1.000000000000000000, 0.9659258262890683122, 1.000000000000000000, 0.9659258262890683122, 1.000000000000000000, 0.9659258262890683122, 1.000000000000000000, 0.9659258262890683122, 1.000000000000000000, 0.9659258262890683122, 1.000000000000000000, 0.9659258262890683122, 1.000000000000000000, 0.9659258262890683122, 1.000000000000000000, 0.9659258262890683122, 1.000000000000000000, 0.9659258262890683122, 1.000000000000000000, 0.9659258262890683122, 1.000000000000000000, 0.9659258262890683122, 1.000000000000000000, 0.9659258262890683122, 1.000000000000000000, 0.9659258262890683122, 1.000000000000000000, 0.9659258262890683122, 1.000000000000000000, 0.9659258262890683122, 1.000000000000000000, 0.9659258262890683122, 1.000000000000000000, 0.9659258262890683122, 1.000000000000000000, 0.9659258262890683122, 1.000000000000000000, 0.9659258262890683122, 1.000000000000000000, 0.9659258262890683122, 1.000000000000000000, 0.9659258262890683122, 1.000000000000000000, 0.9659258262890683122, 1.000000000000000000, 0.9659258262890683122, 1.000000000000000000, 0.9659258262890683122, 1.000000000000000000, 0.9659258262890683122, 1.000000000000000000, 0.9659258262890683122, 1.000000000000000000, 0.9659258262890683122, 1.000000000000000000, 0.9659258262890683122, 1.000000000000000000, 0.9659258262890683122, 1.000000000000000000, 0.9659258262890683122, 1.000000000000000000, 0.9659258262890683122, 1.000000000000000000, 0.9659258262890683122, 1.000000000000000000, 0.9659258262890683122, 1.000000000000000000, 0.9659258262890683122, 1.000000000000000000, 0.9659258262890683122, 1.000000000000000000, 0.9659258262890683122, 1.000000000000000000, 0.9659258262890683122, 1.000000000000000000, 0.9659258262890683122, 1.000000000000000000, 0.9659258262890683122, 1.000000000000000000, 0.9659258262890683122, 1.000000000000000000, 0.9659258262890683122, 1.000000000000000000, 0.9659258262890683122, 1.000000000000000000, 0.9659258262890683122, 1.000000000000000000, 0.9659258262890683122, 1.000000000000000000, 0.9659258262890683122, 1.000000000000000000, 0.9659258262890683122, 1.000000000000000000, 0.9659258262890683122, 1.000000000000000000, 0.9659258262890683122, 1.000000000000000000),
 ( 1.000000000000000000, 0.9659258262890683122, 1.000000000000000000, 0.9659258262890683122, 1.000000000000000000, 0.9659258262890683122, 1.000000000000000000, 0.9659258262890683122, 1.000000000000000000, 0.9659258262890683122, 1.000000000000000000, 0.9659258262890683122, 1.000000000000000000, 0.9659258262890683122, 1.000000000000000000, 0.9659258262890683122, 1.000000000000000000, 0.9659258262890683122, 1.000000000000000000, 0.9659258262890683122, 1.000000000000000000, 0.9659258262890683122, 1.000000000000000000, 0.9659258262890683122, 1.000000000000000000, 0.9659258262890683122, 1.000000000000000000, 0.9659258262890683122, 1.000000000000000000, 0.9659258262890683122, 1.000000000000000000, 0.9659258262890683122, 1.000000000000000000, 0.9659258262890683122, 1.000000000000000000, 0.9659258262890683122, 1.000000000000000000, 0.9659258262890683122, 1.000000000000000000, 0.9659258262890683122, 1.000000000000000000, 0.9659258262890683122, 1.000000000000000000, 0.9659258262890683122, 1.000000000000000000, 0.9659258262890683122, 1.000000000000000000, 0.9659258262890683122, 1.000000000000000000, 0.9659258262890683122, 1.000000000000000000, 0.9659258262890683122, 1.000000000000000000, 0.9659258262890683122, 1.000000000000000000, 0.9659258262890683122, 1.000000000000000000, 0.9659258262890683122, 1.000000000000000000, 0.9659258262890683122, 1.000000000000000000, 0.9659258262890683122, 1.000000000000000000, 0.9659258262890683122, 1.000000000000000000, 0.9659258262890683122, 1.000000000000000000, 0.9659258262890683122, 1.000000000000000000, 0.9659258262890683122, 1.000000000000000000, 0.9659258262890683122, 1.000000000000000000, 0.9659258262890683122, 1.000000000000000000, 0.9659258262890683122, 1.000000000000000000, 0.9659258262890683122, 1.000000000000000000, 0.9659258262890683122, 1.000000000000000000, 0.9659258262890683122, 1.000000000000000000, 0.9659258262890683122, 1.000000000000000000, 0.9659258262890683122, 1.000000000000000000, 0.9659258262890683122, 1.000000000000000000, 0.9659258262890683122, 1.000000000000000000, 0.9659258262890683122, 1.000000000000000000, 0.9659258262890683122, 1.000000000000000000, 0.9659258262890683122, 1.000000000000000000, 0.9659258262890683122, 1.000000000000000000, 0.9659258262890683122, 1.000000000000000000, 0.9659258262890683122, 1.000000000000000000, 0.9659258262890683122, 1.000000000000000000, 0.9659258262890683122, 1.000000000000000000, 0.9659258262890683122, 1.000000000000000000, 0.9659258262890683122, 1.000000000000000000, 0.9659258262890683122, 1.000000000000000000, 0.9659258262890683122, 1.000000000000000000, 0.9659258262890683122, 1.000000000000000000, 0.9659258262890683122, 1.000000000000000000, 0.9659258262890683122, 1.000000000000000000, 0.9659258262890683122, 1.000000000000000000, 0.9659258262890683122, 1.000000000000000000, 0.9659258262890683122, 1.000000000000000000, 0.9659258262890683122, 1.000000000000000000, 0.9659258262890683122, 1.000000000000000000, 0.9659258262890683122, 1.000000000000000000, 0.9659258262890683122, 1.000000000000000000, 0.9659258262890683122, 1.000000000000000000, 0.9659258262890683122, 1.000000000000000000, 0.9659258262890683122, 1.000000000000000000, 0.9659258262890683122, 1.000000000000000000, 0.9659258262890683122, 1.000000000000000000, 0.9659258262890683122, 1.000000000000000000, 0.9659258262890683122, 1.000000000000000000, 0.9659258262890683122, 1.000000000000000000, 0.9659258262890683122, 1.000000000000000000, 0.9659258262890683122, 1.000000000000000000, 0.9659258262890683122, 1.000000000000000000, 0.9659258262890683122, 1.000000000000000000, 0.9659258262890683122, 1.000000000000000000, 0.9659258262890683122, 1.000000000000000000, 0.9659258262890683122, 1.000000000000000000, 0.9659258262890683122, 1.000000000000000000, 0.9659258262890683122, 1.000000000000000000, 0.9659258262890683122, 1.000000000000000000, 0.9659258262890683122, 1.000000000000000000, 0.9659258262890683122, 1.000000000000000000, 0.9659258262890683122, 1.000000000000000000, 0.9659258262890683122, 1.000000000000000000, 0.9659258262890683122, 1.000000000000000000, 0.9659258262890683122, 1.000000000000000000, 0.9659258262890683122, 1.000000000000000000, 0.9659258262890683122, 1.000000000000000000, 0.9659258262890683122, 1.000000000000000000, 0.9659258262890683122, 1.000000000000000000, 0.9659258262890683122, 1.000000000000000000, 0.9659258262890683122, 1.000000000000000000, 0.9659258262890683122, 1.000000000000000000, 0.9659258262890683122, 1.000000000000000000, 0.9659258262890683122, 1.000000000000000000, 0.9659258262890683122, 1.000000000000000000, 0.9659258262890683122, 1.000000000000000000, 0.9659258262890683122, 1.000000000000000000, 0.9659258262890683122, 1.000000000000000000, 0.9659258262890683122, 1.000000000000000000, 0.9659258262890683122, 1.000000000000000000, 0.9659258262890683122, 1.000000000000000000, 0.9659258262890683122, 1.000000000000000000, 0.9659258262890683122, 1.000000000000000000, 0.9659258262890683122, 1.000000000000000000, 0.9659258262890683122, 1.000000000000000000, 0.9659258262890683122, 1.000000000000000000, 0.9659258262890683122, 1.000000000000000000, 0.9659258262890683122, 1.000000000000000000, 0.9659258262890683122, 1.000000000000000000, 0.9659258262890683122, 1.000000000000000000, 0.9659258262890683122, 1.000000000000000000, 0.9659258262890683122, 1.000000000000000000, 0.9659258262890683122, 1.000000000000000000, 0.9659258262890683122, 1.000000000000000000, 0.9659258262890683122, 1.000000000000000000, 0.9659258262890683122, 1.000000000000000000, 0.9659258262890683122, 1.000000000000000000, 0.9659258262890683122, 1.000000000000000000, 0.9659258262890683122, 1.000000000000000000, 0.9659258262890683122, 1.000000000000000000, 0.9659258262890683122, 1.000000000000000000, 0.9659258262890683122, 1.000000000000000000, 0.9659258262890683122, 1.000000000000000000, 0.9659258262890683122, 1.000000000000000000, 0.9659258262890683122, 1.000000000000000000, 0.9659258262890683122, 1.000000000000000000, 0.9659258262890683122, 1.000000000000000000, 0.9659258262890683122, 1.000000000000000000, 0.9659258262890683122, 1.000000000000000000, 0.9659258262890683122, 1.000000000000000000, 0.9659258262890683122, 1.000000000000000000, 0.9659258262890683122, 1.000000000000000000, 0.9659258262890683122, 1.000000000000000000, 0.9659258262890683122, 1.000000000000000000, 0.9659258262890683122, 1.000000000000000000, 0.9659258262890683122, 1.000000000000000000, 0.9659258262890683122, 1.000000000000000000, 0.9659258262890683122, 1.000000000000000000, 0.9659258262890683122, 1.000000000000000000, 0.9659258262890683122, 1.000000000000000000, 0.9659258262890683122, 1.000000000000000000, 0.9659258262890683122, 1.000000000000000000, 0.9659258262890683122, 1.000000000000000000, 0.9659258262890683122, 1.000000000000000000, 0.9659258262890683122, 1.000000000000000000, 0.9659258262890683122, 1.000000000000000000, 0.9659258262890683122, 1.000000000000000000, 0.9659258262890683122, 1.000000000000000000, 0.9659258262890683122, 1.000000000000000000, 0.9659258262890683122, 1.000000000000000000, 0.9659258262890683122, 1.000000000000000000, 0.9659258262890683122, 1.000000000000000000, 0.9659258262890683122, 1.000000000000000000, 0.9659258262890683122, 1.000000000000000000, 0.9659258262890683122, 1.000000000000000000, 0.9659258262890683122, 1.000000000000000000, 0.9659258262890683122, 1.000000000000000000, 0.9659258262890683122, 1.000000000000000000, 0.9659258262890683122, 1.000000000000000000, 0.9659258262890683122, 1.000000000000000000, 0.9659258262890683122, 1.000000000000000000, 0.9659258262890683122, 1.000000000000000000, 0.9659258262890683122, 1.000000000000000000, 0.9659258262890683122, 1.000000000000000000, 0.9659258262890683122, 1.000000000000000000, 0.9659258262890683122, 1.000000000000000000, 0.9659258262890683122, 1.000000000000000000, 0.9659258262890683122, 1.000000000000000000, 0.9659258262890683122, 1.000000000000000000, 0.9659258262890683122, 1.000000000000000000, 0.9659258262890683122, 1.000000000000000000, 0.9659258262890683122, 1.000000000000000000, 0.9659258262890683122, 1.000000000000000000, 0.9659258262890683122, 1.000000000000000000, 0.9659258262890683122, 1.000000000000000000, 0.9659258262890683122, 1.000000000000000000, 0.9659258262890683122, 1.000000000000000000, 0.9659258262890683122, 1.000000000000000000, 0.9659258262890683122, 1.000000000000000000, 0.9659258262890683122, 1.000000000000000000, 0.9659258262890683122, 1.000000000000000000, 0.9659258262890683122, 1.000000000000000000, 0.9659258262890683122, 1.000000000000000000, 0.9659258262890683122, 1.000000000000000000, 0.9659258262890683122, 1.000000000000000000, 0.9659258262890683122, 1.000000000000000000, 0.9659258262890683122, 1.000000000000000000, 0.9659258262890683122, 1.000000000000000000, 0.9659258262890683122, 1.000000000000000000, 0.9659258262890683122, 1.000000000000000000, 0.9659258262890683122, 1.000000000000000000, 0.9659258262890683122, 1.000000000000000000, 0.9659258262890683122, 1.000000000000000000, 0.9659258262890683122, 1.000000000000000000, 0.9659258262890683122, 1.000000000000000000, 0.9659258262890683122, 1.000000000000000000, 0.9659258262890683122, 1.000000000000000000, 0.9659258262890683122, 1.000000000000000000, 0.9659258262890683122, 1.000000000000000000, 0.9659258262890683122, 1.000000000000000000, 0.9659258262890683122, 1.000000000000000000, 0.9659258262890683122, 1.000000000000000000, 0.9659258262890683122, 1.000000000000000000, 0.9659258262890683122, 1.000000000000000000, 0.9659258262890683122, 1.000000000000000000, 0.9659258262890683122, 1.000000000000000000, 0.9659258262890683122, 1.000000000000000000, 0.9659258262890683122, 1.000000000000000000, 0.9659258262890683122, 1.000000000000000000, 0.9659258262890683122, 1.000000000000000000, 0.9659258262890683122, 1.000000000000000000, 0.9659258262890683122, 1.000000000000000000, 0.9659258262890683122, 1.000000000000000000, 0.9659258262890683122, 1.000000000000000000, 0.9659258262890683122, 1.000000000000000000, 0.9659258262890683122, 1.000000000000000000, 0.9659258262890683122, 1.000000000000000000, 0.9659258262890683122, 1.000000000000000000, 0.9659258262890683122, 1.000000000000000000, 0.9659258262890683122, 1.000000000000000000, 0.9659258262890683122, 1.000000000000000000, 0.9659258262890683122, 1.000000000000000000, 0.9659258262890683122, 1.000000000000000000, 0.9659258262890683122, 1.000000000000000000, 0.9659258262890683122, 1.000000000000000000, 0.9659258262890683122, 1.000000000000000000, 0.9659258262890683122, 1.000000000000000000, 0.9659258262890683122, 1.000000000000000000, 0.9659258262890683122, 1.000000000000000000, 0.9659258262890683122, 1.000000000000000000, 0.9659258262890683122, 1.000000000000000000, 0.9659258262890683122, 1.000000000000000000, 0.9659258262890683122, 1.000000000000000000, 0.9659258262890683122, 1.000000000000000000, 0.9659258262890683122, 1.000000000000000000, 0.9659258262890683122, 1.000000000000000000, 0.9659258262890683122, 1.000000000000000000, 0.9659258262890683122, 1.000000000000000000, 0.9659258262890683122, 1.000000000000000000, 0.9659258262890683122, 1.000000000000000000, 0.9659258262890683122, 1.000000000000000000, 0.9659258262890683122, 1.000000000000000000, 0.9659258262890683122, 1.000000000000000000, 0.9659258262890683122, 1.000000000000000000, 0.9659258262890683122, 1.000000000000000000, 0.9659258262890683122, 1.000000000000000000, 0.9659258262890683122, 1.000000000000000000, 0.9659258262890683122, 1.000000000000000000, 0.9659258262890683122, 1.000000000000000000) ) ) 
 REPRESENTATION_ITEM ( '' )  SURFACE ( )  );
#34798=CARTESIAN_POINT ( 'NONE',  ( -0.4068241469816264999, -0.3690944881889763329, 0.3153832671262228327 ) ) ;
#34799=CARTESIAN_POINT ( 'NONE',  ( -0.6955380577427815458, -0.3690944881889765550, -0.3153832671262227771 ) ) ;
#34800=CARTESIAN_POINT ( 'NONE',  ( -1.003937007874014853, 0.1660481256975885056, 0.3530559997133364547 ) ) ;
#34801=CARTESIAN_POINT ( 'NONE',  ( 1.089238845144357537, -0.4281496062992124485, 0.4176697321401328655 ) ) ;
#34802=CARTESIAN_POINT ( 'NONE',  ( -0.9186351706036736120, -0.6046776061558809534, -0.2411417322834644161 ) ) ;
#34805=CARTESIAN_POINT ( 'NONE',  ( -1.397637795275589623, -0.5400638737290845981, -0.3530559997133363437 ) ) ;
#34806=CARTESIAN_POINT ( 'NONE',  ( -1.606174037523448561, 0.2952824826768989941, 0.01137383275704648665 ) ) ;
#34807=CARTESIAN_POINT ( 'NONE',  ( -1.712598425196849572, 0.1660481256975885056, 0.3530559997133364547 ) ) ;
#34812=CARTESIAN_POINT ( 'NONE',  ( -0.5577427821522301654, -0.3162353388693405765, 0.4822834645669290543 ) ) ;
#34813=CARTESIAN_POINT ( 'NONE',  ( 1.253280839895013710, -0.05778040916215560624, -0.4822834645669293319 ) ) ;
#34815=CARTESIAN_POINT ( 'NONE',  ( -1.561679790026246017, 0.05413385826771666132, 0.4176697321401328100 ) ) ;
#34817=EDGE_CURVE ( 'NONE', #24575, #52448, #17739, .T. ) ;
#34818=CARTESIAN_POINT ( 'NONE',  ( -1.338582677165353729, -0.1870078740157480879, -0.4822834645669291653 ) ) ;
#34819=CARTESIAN_POINT ( 'NONE',  ( -0.9776902887139098386, -0.6692913385826771977, 0.1292274648535927661 ) ) ;
#34821=CARTESIAN_POINT ( 'NONE',  ( 0.4724409448818904789, -0.1870078740157479769, 0.3641732283464567677 ) ) ;
#34823=EDGE_CURVE ( 'NONE', #58545, #46767, #64953, .T. ) ;
#34824=CARTESIAN_POINT ( 'NONE',  ( 0.2296587926509192634, -0.2845877964562159024, 0.3641732283464567677 ) ) ;
#34825=CARTESIAN_POINT ( 'NONE',  ( 1.049868766404200127, -0.5023911411419708095, -0.1820866141732282451 ) ) ;
#34826=CARTESIAN_POINT ( 'NONE',  ( 1.108923884514436242, -0.05778040916215522460, 0.4822834645669289988 ) ) ;
#34827=CARTESIAN_POINT ( 'NONE',  ( -0.4790026246719152336, -0.08942795157528024563, -0.3641732283464568787 ) ) ;
#34829=CARTESIAN_POINT ( 'NONE',  ( -1.187664041994749731, -0.3162353388693405765, 0.4822834645669290543 ) ) ;
#34830=CARTESIAN_POINT ( 'NONE',  ( -1.102362204724408601, -0.1870078740157480601, -0.3641732283464567677 ) ) ;
#34832=CARTESIAN_POINT ( 'NONE',  ( -0.9514435695538050464, -0.08942795157528024563, -0.3641732283464568787 ) ) ;
#34833=CARTESIAN_POINT ( 'NONE',  ( -0.2690288713910754526, -0.6692913385826771977, 0.1292274648535927661 ) ) ;
#34835=CARTESIAN_POINT ( 'NONE',  ( 0.5839895013123367340, -0.5511811023622048555, -0.09757992244046775898 ) ) ;
#34836=CARTESIAN_POINT ( 'NONE',  ( -0.1115485564304456306, 0.1771653543307087075, -0.09757992244046823083 ) ) ;
#34837=CARTESIAN_POINT ( 'NONE',  ( -0.6496062992125976043, 0.1660481256975883668, -0.3530559997133364547 ) ) ;
#34838=CARTESIAN_POINT ( 'NONE',  ( -1.653543307086613234, -0.1870078740157480879, -0.4822834645669291653 ) ) ;
#34839=CARTESIAN_POINT ( 'NONE',  ( -1.646051170424378096, -0.1870078740157480046, 1.254653134982923898E-17 ) ) ;
#34840=CARTESIAN_POINT ( 'NONE',  ( -0.01312335958005186876, 0.05413385826771626580, -0.4176697321401330321 ) ) ;
#34842=CARTESIAN_POINT ( 'NONE',  ( 1.430446194225722500, 0.05413385826771666132, 0.4176697321401328100 ) ) ;
#34843=CARTESIAN_POINT ( 'NONE',  ( -0.4265091863517051496, 0.1771653543307087075, -0.09757992244046823083 ) ) ;
#34844=CARTESIAN_POINT ( 'NONE',  ( 0.006561679790026889343, -0.05778040916215522460, 0.4822834645669289988 ) ) ;
#34845=CARTESIAN_POINT ( 'NONE',  ( -1.568241469816272105, -0.3162353388693409650, -0.4822834645669289433 ) ) ;
#34846=CARTESIAN_POINT ( 'NONE',  ( -1.633858267716534529, 0.07958543189024085140, 0.2665933059059887866 ) ) ;
#34847=CARTESIAN_POINT ( 'NONE',  ( 1.338582677165355062, -0.1870078740157479769, 0.4822834645669291653 ) ) ;
#34848=CARTESIAN_POINT ( 'NONE',  ( -0.6627296587926503335, -0.5511811023622046335, 0.09757992244046803654 ) ) ;
#34854=CARTESIAN_POINT ( 'NONE',  ( 1.325459317585302665, -0.004921259842519870586, -0.3153832671262229437 ) ) ;
#34856=CARTESIAN_POINT ( 'NONE',  ( 0.6824146981627303710, 0.2306618581243847221, -0.2411417322834647770 ) ) ;
#34858=CARTESIAN_POINT ( 'NONE',  ( 1.318897637795276356, -0.4536011799217367080, 0.2665933059059888421 ) ) ;
#34859=CARTESIAN_POINT ( 'NONE',  ( 0.3083989501312343062, -0.05778040916215560624, -0.4822834645669293319 ) ) ;
#34860=CARTESIAN_POINT ( 'NONE',  ( -0.4330708661417315697, -0.6692913385826771977, 8.415575281601705876E-17 ) ) ;
#34861=CARTESIAN_POINT ( 'NONE',  ( 1.496062992125985147, -0.1870078740157479769, 0.4822834645669291653 ) ) ;
#34864=CARTESIAN_POINT ( 'NONE',  ( 0.2099737532808405305, 0.1283753931104746893, -0.1820866141732285504 ) ) ;
#34869=CARTESIAN_POINT ( 'NONE',  ( -0.4790026246719154557, -0.3162353388693405765, 0.4822834645669290543 ) ) ;
#34870=CARTESIAN_POINT ( 'NONE',  ( 1.154855643044620184, 0.2306618581243847221, -0.2411417322834647770 ) ) ;
#34871=CARTESIAN_POINT ( 'NONE',  ( 0.2034120734908144990, -0.6692913385826771977, 0.1292274648535927661 ) ) ;
#34872=CARTESIAN_POINT ( 'NONE',  ( -0.4593175853018364174, -0.3690944881889765550, -0.3153832671262227771 ) ) ;
#34873=CARTESIAN_POINT ( 'NONE',  ( 0.6299212598425204535, -0.1870078740157480879, -0.4822834645669291653 ) ) ;
#34874=CARTESIAN_POINT ( 'NONE',  ( -1.122047244094487306, 0.1660481256975883668, -0.3530559997133364547 ) ) ;
#34875=CARTESIAN_POINT ( 'NONE',  ( -0.5052493438320203589, -0.6692913385826771977, 0.1292274648535927661 ) ) ;
#34876=CARTESIAN_POINT ( 'NONE',  ( -0.9186351706036736120, 0.2306618581243848609, 0.2411417322834645549 ) ) ;
#34877=CARTESIAN_POINT ( 'NONE',  ( 1.049868766404200127, -0.6046776061558809534, -0.2411417322834644161 ) ) ;
#34878=CARTESIAN_POINT ( 'NONE',  ( 0.7349081364829402885, -0.6046776061558809534, -0.2411417322834644161 ) ) ;
#34879=CARTESIAN_POINT ( 'NONE',  ( 0.7742782152230979209, 0.05413385826771626580, -0.4176697321401330321 ) ) ;
#34881=CARTESIAN_POINT ( 'NONE',  ( -0.01968503937007793844, 0.07958543189024071263, -0.2665933059059888421 ) ) ;
#34882=ORIENTED_EDGE ( 'NONE', *, *, #21903, .F. ) ;
#34884=ORIENTED_EDGE ( 'NONE', *, *, #48192, .F. ) ;
#34885=CARTESIAN_POINT ( 'NONE',  ( -0.8792650918635160906, -0.004921259842519870586, -0.3153832671262229437 ) ) ;
#34886=CARTESIAN_POINT ( 'NONE',  ( -0.3215223097112853146, -0.05778040916215560624, -0.4822834645669293319 ) ) ;
#34888=CARTESIAN_POINT ( 'NONE',  ( -0.4527559055118102749, 0.1660481256975885056, 0.3530559997133364547 ) ) ;
#34889=CARTESIAN_POINT ( 'NONE',  ( -0.2690288713910754526, 0.2952755905511810774, -0.1292274648535930714 ) ) ;
#34890=CARTESIAN_POINT ( 'NONE',  ( -1.345144356955379816, -0.3162353388693405765, 0.4822834645669290543 ) ) ;
#34891=CARTESIAN_POINT ( 'NONE',  ( -1.430446194225721390, -0.4281496062992124485, 0.4176697321401328655 ) ) ;
#34892=CARTESIAN_POINT ( 'NONE',  ( 1.108923884514436686, -0.2845877964562161244, -0.3641732283464567121 ) ) ;
#34895=CARTESIAN_POINT ( 'NONE',  ( 0.6627296587926515548, 0.1771653543307087630, 0.09757992244046791164 ) ) ;
#34896=CARTESIAN_POINT ( 'NONE',  ( 0.03937007874015833325, -0.6692913385826771977, 8.415575281601705876E-17 ) ) ;
#34897=CARTESIAN_POINT ( 'NONE',  ( 0.1509186351706045259, -0.05778040916215560624, -0.4822834645669293319 ) ) ;
#34904=CARTESIAN_POINT ( 'NONE',  ( -0.5052493438320203589, -0.6692913385826771977, 0.1292274648535927661 ) ) ;
#34907=CARTESIAN_POINT ( 'NONE',  ( 1.660104986876641320, -0.05778040916215522460, 0.4822834645669289988 ) ) ;
#34908=CARTESIAN_POINT ( 'NONE',  ( 0.9448818897637802916, -0.1870078740157479769, 0.4822834645669291653 ) ) ;
#34909=CARTESIAN_POINT ( 'NONE',  ( 1.095800524934383846, -0.05778040916215560624, -0.4822834645669293319 ) ) ;
#34910=CARTESIAN_POINT ( 'NONE',  ( -0.7874015748031489847, -0.1870078740157480601, -0.3641732283464567677 ) ) ;
#34911=CARTESIAN_POINT ( 'NONE',  ( 5.463695987328526437E-16, -0.1870078740157479769, 0.4822834645669291653 ) ) ;
#34913=CARTESIAN_POINT ( 'NONE',  ( 8.195543980992789655E-16, -0.1870078740157480601, -0.3641732283464567677 ) ) ;
#34914=CARTESIAN_POINT ( 'NONE',  ( -0.3477690288713905509, -0.6692913385826771977, 0.1292274648535927661 ) ) ;
#34915=ADVANCED_FACE ( 'NONE', ( #78618 ), #14225, .F. ) ;
#34917=CARTESIAN_POINT ( 'NONE',  ( 1.548556430446194954, -0.5023911411419708095, 0.1820866141732285504 ) ) ;
#34918=CARTESIAN_POINT ( 'NONE',  ( 0.1968503937007881344, 0.1771653543307087630, 0.000000000000000000 ) ) ;
#34920=CARTESIAN_POINT ( 'NONE',  ( -1.174540682414697335, -0.3162353388693409650, -0.4822834645669289433 ) ) ;
#34921=CARTESIAN_POINT ( 'NONE',  ( -0.7020997375328074108, -0.08942795157527998196, 0.3641732283464567121 ) ) ;
#34923=CARTESIAN_POINT ( 'NONE',  ( -1.089238845144356427, 0.05413385826771666132, 0.4176697321401328100 ) ) ;
#34924=CARTESIAN_POINT ( 'NONE',  ( -0.1640419947506553400, -0.05778040916215560624, -0.4822834645669293319 ) ) ;
#34926=( BOUNDED_CURVE ( )  B_SPLINE_CURVE ( 1, ( #19976, #25856 ),
 .UNSPECIFIED., .F., .F. ) 
 B_SPLINE_CURVE_WITH_KNOTS ( ( 2, 2 ),
 ( 3.469446951953614189E-18, 0.002000000000000005246 ),
 .UNSPECIFIED. ) 
 CURVE ( )  GEOMETRIC_REPRESENTATION_ITEM ( )  RATIONAL_B_SPLINE_CURVE ( ( 0.9875488213027527884, 0.9875488213027527884 ) ) 
 REPRESENTATION_ITEM ( '' )  );
#34929=CARTESIAN_POINT ( 'NONE',  ( 0.2821522309711292364, 0.1771653543307087075, -0.09757992244046823083 ) ) ;
#34930=CARTESIAN_POINT ( 'NONE',  ( 1.161417322834646271, 0.1660481256975883668, -0.3530559997133364547 ) ) ;
#34931=CARTESIAN_POINT ( 'NONE',  ( -1.122047244094487306, -0.4536011799217367080, 0.2665933059059888421 ) ) ;
#34932=CARTESIAN_POINT ( 'NONE',  ( 1.128608923884515169, -0.6046776061558809534, -0.2411417322834644161 ) ) ;
#34933=CARTESIAN_POINT ( 'NONE',  ( -1.397637795275589623, 0.07958543189024085140, 0.2665933059059887866 ) ) ;
#34934=CARTESIAN_POINT ( 'NONE',  ( -0.5446194225721777693, -0.3162353388693409650, -0.4822834645669289433 ) ) ;
#34935=CARTESIAN_POINT ( 'NONE',  ( 0.3412073490813655186, -0.5023911411419708095, -0.1820866141732282451 ) ) ;
#34937=CARTESIAN_POINT ( 'NONE',  ( 0.8398950131233602345, 0.1283753931104746893, -0.1820866141732285504 ) ) ;
#34938=CARTESIAN_POINT ( 'NONE',  ( -0.01312335958005186876, 0.05413385826771626580, -0.4176697321401330321 ) ) ;
#34940=CARTESIAN_POINT ( 'NONE',  ( -0.8727034120734901146, -0.05778040916215560624, -0.4822834645669293319 ) ) ;
#34942=CARTESIAN_POINT ( 'NONE',  ( 0.9448818897637802916, -0.1870078740157479769, 0.3641732283464567677 ) ) ;
#34943=CARTESIAN_POINT ( 'NONE',  ( 0.2493438320209980519, 0.05413385826771666132, 0.4176697321401328100 ) ) ;
#34944=CARTESIAN_POINT ( 'NONE',  ( -0.1115485564304453947, -0.6692913385826771977, 0.1292274648535927661 ) ) ;
#34945=CARTESIAN_POINT ( 'NONE',  ( -0.5446194225721777693, -0.08942795157527998196, 0.3641732283464567121 ) ) ;
#34946=CARTESIAN_POINT ( 'NONE',  ( 1.010498687664042716, 0.009842519685039144428, -0.3409548833797004797 ) ) ;
#34947=CARTESIAN_POINT ( 'NONE',  ( -0.2952755905511803003, -0.4536011799217368745, -0.2665933059059886201 ) ) ;
#34948=CARTESIAN_POINT ( 'NONE',  ( 0.2887139107611556010, 0.2306618581243847221, -0.2411417322834647770 ) ) ;
#34949=CARTESIAN_POINT ( 'NONE',  ( -0.7283464566929126471, 0.07958543189024071263, -0.2665933059059888421 ) ) ;
#34951=CARTESIAN_POINT ( 'NONE',  ( -1.056430446194224881, -0.6692913385826771977, 0.1292274648535927661 ) ) ;
#34954=CARTESIAN_POINT ( 'NONE',  ( -1.207349081364828880, 0.1283753931104746893, -0.1820866141732285504 ) ) ;
#34955=CARTESIAN_POINT ( 'NONE',  ( -0.4330708661417315697, 0.2952755905511811885, 0.000000000000000000 ) ) ;
#34957=CARTESIAN_POINT ( 'NONE',  ( -1.207349081364828436, -0.6046776061558807314, 0.2411417322834647770 ) ) ;
#34959=CARTESIAN_POINT ( 'NONE',  ( 1.167979002624672580, -0.4281496062992124485, 0.4176697321401328655 ) ) ;
#34960=CARTESIAN_POINT ( 'NONE',  ( 0.8989501312335964611, 0.2952755905511811885, 0.1292274648535926551 ) ) ;
#34962=DIRECTION ( 'NONE',  ( -1.000000000000000000, -3.083952846180990281E-16, 0.000000000000000000 ) ) ;
#34963=CARTESIAN_POINT ( 'NONE',  ( 1.437007874015748810, 0.07958543189024085140, 0.2665933059059887866 ) ) ;
#34966=CARTESIAN_POINT ( 'NONE',  ( -0.6692913385826764205, 0.1771653543307087630, 0.000000000000000000 ) ) ;
#34968=ORIENTED_EDGE ( 'NONE', *, *, #35375, .F. ) ;
#34969=CARTESIAN_POINT ( 'NONE',  ( 0.8267716535433077274, 0.2952755905511811885, 0.000000000000000000 ) ) ;
#34970=CARTESIAN_POINT ( 'NONE',  ( -0.01312335958005186876, -0.4281496062992124485, 0.4176697321401328655 ) ) ;
#34971=CARTESIAN_POINT ( 'NONE',  ( -0.5183727034120726440, 0.2952755905511811885, 0.1292274648535926551 ) ) ;
#34972=CARTESIAN_POINT ( 'NONE',  ( 1.587926509186352586, -0.4281496062992127816, -0.4176697321401328100 ) ) ;
#34973=CARTESIAN_POINT ( 'NONE',  ( -1.299212598425196097, 0.1771653543307087630, 0.000000000000000000 ) ) ;
#34974=CARTESIAN_POINT ( 'NONE',  ( 0.5027385518334777093, 1.496062992125983815, -0.5309055118110237448 ) ) ;
#34975=CARTESIAN_POINT ( 'NONE',  ( 0.2952755905511819101, 0.1660481256975883668, -0.3530559997133364547 ) ) ;
#34976=CARTESIAN_POINT ( 'NONE',  ( -0.7545931758530176614, -0.6692913385826773087, -0.1292274648535924053 ) ) ;
#34978=CARTESIAN_POINT ( 'NONE',  ( -1.200787401574802349, -0.5400638737290844871, 0.3530559997133364547 ) ) ;
#34980=CARTESIAN_POINT ( 'NONE',  ( 1.108923884514436686, -0.3162353388693409650, -0.4822834645669289433 ) ) ;
#34981=CARTESIAN_POINT ( 'NONE',  ( 1.122047244094488860, -0.4536011799217368745, -0.2665933059059886201 ) ) ;
#34984=CARTESIAN_POINT ( 'NONE',  ( -0.6102362204724400829, -0.5400638737290845981, -0.3530559997133363437 ) ) ;
#34985=ORIENTED_EDGE ( 'NONE', *, *, #5920, .T. ) ;
#34986=CARTESIAN_POINT ( 'NONE',  ( 0.2624671916010504757, -0.5023911411419708095, -0.1820866141732282451 ) ) ;
#34987=CARTESIAN_POINT ( 'NONE',  ( -1.082677165354329896, 0.1660481256975885056, 0.3530559997133364547 ) ) ;
#34988=CARTESIAN_POINT ( 'NONE',  ( 1.167979002624672580, 0.05413385826771626580, -0.4176697321401330321 ) ) ;
#34989=CARTESIAN_POINT ( 'NONE',  ( 0.6627296587926515548, 0.2952755905511811885, 0.1292274648535926551 ) ) ;
#34990=CARTESIAN_POINT ( 'NONE',  ( -0.2099737532808391705, -0.6046776061558809534, -0.2411417322834644161 ) ) ;
#34991=CARTESIAN_POINT ( 'NONE',  ( -0.9842519685039360366, 0.2952755905511811885, 0.000000000000000000 ) ) ;
#34993=CARTESIAN_POINT ( 'NONE',  ( -1.522309711286088607, 0.2306618581243847221, -0.2411417322834647770 ) ) ;
#34994=CARTESIAN_POINT ( 'NONE',  ( -0.4330708661417315697, -0.6692913385826771977, 8.415575281601705876E-17 ) ) ;
#34995=CARTESIAN_POINT ( 'NONE',  ( -0.6692913385826764205, 0.1771653543307087630, 0.000000000000000000 ) ) ;
#34996=CARTESIAN_POINT ( 'NONE',  ( 1.272965879265092637, -0.4281496062992127816, -0.4176697321401328100 ) ) ;
#34997=CARTESIAN_POINT ( 'NONE',  ( 1.515748031496063408, 0.1660481256975885056, 0.3530559997133364547 ) ) ;
#34998=CARTESIAN_POINT ( 'NONE',  ( -0.9055118110236215490, 0.2952755905511811885, 0.000000000000000000 ) ) ;
#35000=CARTESIAN_POINT ( 'NONE',  ( 0.5511811023622054106, -0.1870078740157480879, -0.4822834645669291653 ) ) ;
#35004=CARTESIAN_POINT ( 'NONE',  ( -0.09842519685039295696, -0.5400638737290844871, 0.3530559997133364547 ) ) ;
#35005=CARTESIAN_POINT ( 'NONE',  ( -1.200787401574802349, -0.4536011799217367080, 0.2665933059059888421 ) ) ;
#35006=CARTESIAN_POINT ( 'NONE',  ( 0.9514435695538062676, -0.2845877964562161244, -0.3641732283464567121 ) ) ;
#35008=CARTESIAN_POINT ( 'NONE',  ( 1.318897637795276356, -0.4536011799217367080, 0.2665933059059888421 ) ) ;
#35009=CARTESIAN_POINT ( 'NONE',  ( 0.9842519685039375910, 0.2952755905511811885, 0.000000000000000000 ) ) ;
#35010=ADVANCED_FACE ( 'NONE', ( #40706 ), #54582, .F. ) ;
#35012=CARTESIAN_POINT ( 'NONE',  ( -0.4986876640419942164, -0.6046776061558807314, 0.2411417322834647770 ) ) ;
#35014=CARTESIAN_POINT ( 'NONE',  ( 1.430446194225722500, -0.004921259842519576551, 0.3153832671262227771 ) ) ;
#35015=CARTESIAN_POINT ( 'NONE',  ( -0.4855643044619415427, -0.4281496062992124485, 0.4176697321401328655 ) ) ;
#35017=CARTESIAN_POINT ( 'NONE',  ( 1.397637795275591177, 0.1660481256975883668, -0.3530559997133364547 ) ) ;
#35018=CARTESIAN_POINT ( 'NONE',  ( 0.01968503937007930540, 0.1660481256975885056, 0.3530559997133364547 ) ) ;
#35019=CARTESIAN_POINT ( 'NONE',  ( 0.5643044619422579178, -0.004921259842519576551, 0.3153832671262227771 ) ) ;
#35021=CARTESIAN_POINT ( 'NONE',  ( 0.4396325459317593221, 0.1771653543307087075, -0.09757992244046823083 ) ) ;
#35022=CARTESIAN_POINT ( 'NONE',  ( -1.515748031496062076, -0.5400638737290844871, 0.3530559997133364547 ) ) ;
#35024=CARTESIAN_POINT ( 'NONE',  ( 0.8333333333333340365, -0.6692913385826771977, 0.1292274648535927661 ) ) ;
#35026=CARTESIAN_POINT ( 'NONE',  ( 1.627296587926509996, -0.5023911411419708095, 0.1820866141732285504 ) ) ;
#35027=CARTESIAN_POINT ( 'NONE',  ( 0.09842519685039433086, 0.1660481256975885056, 0.3530559997133364547 ) ) ;
#35028=CARTESIAN_POINT ( 'NONE',  ( 0.1968503937007881344, 0.1771653543307087630, 0.000000000000000000 ) ) ;
#35029=CARTESIAN_POINT ( 'NONE',  ( -0.02624671916010428221, 0.2306618581243847221, -0.2411417322834647770 ) ) ;
#35030=CARTESIAN_POINT ( 'NONE',  ( 1.358267716535433323, 0.07958543189024085140, 0.2665933059059887866 ) ) ;
#35031=CARTESIAN_POINT ( 'NONE',  ( -1.410761154855642463, -0.08942795157527998196, 0.3641732283464567121 ) ) ;
#35032=CARTESIAN_POINT ( 'NONE',  ( -1.489501312335957062, -0.3162353388693409650, -0.4822834645669289433 ) ) ;
#35033=CARTESIAN_POINT ( 'NONE',  ( 0.4002624671916016896, -0.05778040916215522460, 0.4822834645669289988 ) ) ;
#35034=CARTESIAN_POINT ( 'NONE',  ( 1.069553805774278832, 0.2952755905511810774, -0.1292274648535930714 ) ) ;
#35036=CARTESIAN_POINT ( 'NONE',  ( 0.5774278215223103139, -0.6046776061558809534, -0.2411417322834644161 ) ) ;
#35037=CARTESIAN_POINT ( 'NONE',  ( 1.351706036745407680, 0.05413385826771666132, 0.4176697321401328100 ) ) ;
#35038=CARTESIAN_POINT ( 'NONE',  ( 1.043307086614173818, 0.1660481256975885056, 0.3530559997133364547 ) ) ;
#35040=CARTESIAN_POINT ( 'NONE',  ( 0.6430446194225729606, -0.3690944881889765550, -0.3153832671262227771 ) ) ;
#35041=CARTESIAN_POINT ( 'NONE',  ( 1.502624671916010790, -0.05778040916215522460, 0.4822834645669289988 ) ) ;
#35042=CARTESIAN_POINT ( 'NONE',  ( -0.9711286089238838626, 0.1283753931104746893, -0.1820866141732285504 ) ) ;
#35043=CARTESIAN_POINT ( 'NONE',  ( 0.7086614173228352742, -0.1870078740157480601, -0.3641732283464567677 ) ) ;
#35044=CARTESIAN_POINT ( 'NONE',  ( 0.07874015748031558404, -0.1870078740157479769, 0.4822834645669291653 ) ) ;
#35045=CARTESIAN_POINT ( 'NONE',  ( 0.6102362204724416372, -0.5400638737290844871, 0.3530559997133364547 ) ) ;
#35046=CARTESIAN_POINT ( 'NONE',  ( -0.3937007874015740483, -0.1870078740157479769, 0.4822834645669291653 ) ) ;
#35047=CARTESIAN_POINT ( 'NONE',  ( 0.2230971128608929543, -0.004921259842519870586, -0.3153832671262229437 ) ) ;
#35048=CARTESIAN_POINT ( 'NONE',  ( 0.9842519685039375910, 0.2952755905511811885, 0.000000000000000000 ) ) ;
#35050=CARTESIAN_POINT ( 'NONE',  ( -1.102362204724408601, -0.1870078740157479769, 0.4822834645669291653 ) ) ;
#35051=CARTESIAN_POINT ( 'NONE',  ( -1.035207913594495599, 0.02791078216816347476, -0.4328096321851898631 ) ) ;
#35054=CARTESIAN_POINT ( 'NONE',  ( -0.8923884514435688198, -0.6046776061558807314, 0.2411417322834647770 ) ) ;
#35055=CARTESIAN_POINT ( 'NONE',  ( -0.5183727034120726440, -0.6692913385826773087, -0.1292274648535924053 ) ) ;
#35059=CARTESIAN_POINT ( 'NONE',  ( 0.5839895013123367340, 0.1771653543307087630, 0.09757992244046791164 ) ) ;
#35061=CARTESIAN_POINT ( 'NONE',  ( 1.312335958005249825, 0.2306618581243847221, -0.2411417322834647770 ) ) ;
#35064=CARTESIAN_POINT ( 'NONE',  ( -1.364829396325458521, 0.1283753931104746893, -0.1820866141732285504 ) ) ;
#35065=CARTESIAN_POINT ( 'NONE',  ( 1.607611548556431069, -0.6692913385826773087, -0.1292274648535924053 ) ) ;
#35066=CARTESIAN_POINT ( 'NONE',  ( -1.666666666666665853, 0.05413385826771626580, -0.4176697321401330321 ) ) ;
#35068=CARTESIAN_POINT ( 'NONE',  ( -0.1640419947506553400, -0.05778040916215560624, -0.4822834645669293319 ) ) ;
#35069=CARTESIAN_POINT ( 'NONE',  ( -0.7808398950131225646, -0.08942795157527998196, 0.3641732283464567121 ) ) ;
#35070=CARTESIAN_POINT ( 'NONE',  ( 0.7349081364829402885, -0.6046776061558809534, -0.2411417322834644161 ) ) ;
#35071=CARTESIAN_POINT ( 'NONE',  ( 0.07217847769028949700, -0.05778040916215560624, -0.4822834645669293319 ) ) ;
#35075=CARTESIAN_POINT ( 'NONE',  ( 0.8267716535433078384, -0.6692913385826771977, 8.415575281601705876E-17 ) ) ;
#35076=CARTESIAN_POINT ( 'NONE',  ( 0.2493438320209980519, -0.4281496062992127816, -0.4176697321401328100 ) ) ;
#35077=CARTESIAN_POINT ( 'NONE',  ( -0.8661417322834640276, -0.1870078740157479769, 0.4822834645669291653 ) ) ;
#35078=CARTESIAN_POINT ( 'NONE',  ( 1.135170603674541256, 0.2952755905511811885, 0.1292274648535926551 ) ) ;
#35079=CARTESIAN_POINT ( 'NONE',  ( 0.7939632545931766261, -0.3162353388693409650, -0.4822834645669289433 ) ) ;
#35081=CARTESIAN_POINT ( 'NONE',  ( -0.4133858267716528645, 0.1660481256975883668, -0.3530559997133364547 ) ) ;
#35082=CARTESIAN_POINT ( 'NONE',  ( 0.7414698162729663755, 0.2952755905511811885, 0.1292274648535926551 ) ) ;
#35083=CARTESIAN_POINT ( 'NONE',  ( 0.006561679790026889343, -0.3162353388693409650, -0.4822834645669289433 ) ) ;
#35084=CARTESIAN_POINT ( 'NONE',  ( 0.6692913385826778638, -0.5511811023622047445, 6.969142054262312111E-17 ) ) ;
#35085=CARTESIAN_POINT ( 'NONE',  ( -1.410761154855642463, -0.05778040916215522460, 0.4822834645669289988 ) ) ;
#35087=CARTESIAN_POINT ( 'NONE',  ( 0.1246719160104994284, -0.6692913385826771977, 0.1292274648535927661 ) ) ;
#35090=ORIENTED_EDGE ( 'NONE', *, *, #82011, .T. ) ;
#35092=CARTESIAN_POINT ( 'NONE',  ( 0.9908136482939640111, -0.6692913385826771977, 0.1292274648535927661 ) ) ;
#35093=CARTESIAN_POINT ( 'NONE',  ( 0.6102362204724416372, -0.4536011799217367080, 0.2665933059059888421 ) ) ;
#35100=CARTESIAN_POINT ( 'NONE',  ( -0.9908136482939626788, 0.2952755905511811885, 0.1292274648535926551 ) ) ;
#35101=CARTESIAN_POINT ( 'NONE',  ( -0.6758530183727028406, -0.6692913385826773087, -0.1292274648535924053 ) ) ;
#35102=CARTESIAN_POINT ( 'NONE',  ( 0.6167979002624678353, -0.4281496062992124485, 0.4176697321401328655 ) ) ;
#35104=VECTOR ( 'NONE', #65113, 39.37007874015748143 ) ;
#35105=CARTESIAN_POINT ( 'NONE',  ( 1.384514435695538337, -0.6692913385826771977, 0.1292274648535927661 ) ) ;
#35106=FACE_OUTER_BOUND ( 'NONE', #54822, .T. ) ;
#35108=CARTESIAN_POINT ( 'NONE',  ( 1.614173228346457378, -0.5511811023622047445, 6.969142054262312111E-17 ) ) ;
#35110=CARTESIAN_POINT ( 'NONE',  ( -1.541994750656167090, -0.5511811023622048555, -0.09757992244046775898 ) ) ;
#35112=CARTESIAN_POINT ( 'NONE',  ( 0.1443569553805781891, 0.05413385826771626580, -0.4176697321401330321 ) ) ;
#35113=CARTESIAN_POINT ( 'NONE',  ( 1.594488188976378673, -0.5400638737290845981, -0.3530559997133363437 ) ) ;
#35114=DIRECTION ( 'NONE',  ( -0.000000000000000000, 0.000000000000000000, -1.000000000000000000 ) ) ;
#35115=CARTESIAN_POINT ( 'NONE',  ( -1.122047244094487306, -0.4536011799217367080, 0.2665933059059888421 ) ) ;
#35116=CARTESIAN_POINT ( 'NONE',  ( 0.9055118110236227702, 0.2952755905511811885, 0.000000000000000000 ) ) ;
#35117=CARTESIAN_POINT ( 'NONE',  ( 1.213910761154856299, -0.5511811023622048555, -0.09757992244046775898 ) ) ;
#35119=CARTESIAN_POINT ( 'NONE',  ( -1.417322834645668772, -0.1870078740157479769, 0.3641732283464567677 ) ) ;
#35120=CARTESIAN_POINT ( 'NONE',  ( 1.404199475065617708, 0.05413385826771626580, -0.4176697321401330321 ) ) ;
#35122=CARTESIAN_POINT ( 'NONE',  ( -0.1837270341207343505, -0.6046776061558807314, 0.2411417322834647770 ) ) ;
#35123=CARTESIAN_POINT ( 'NONE',  ( -1.312335958005248715, 0.1283753931104748280, 0.1820866141732283561 ) ) ;
#35124=CARTESIAN_POINT ( 'NONE',  ( -0.3149606299212590610, -0.1870078740157479769, 0.3641732283464567677 ) ) ;
#35127=CARTESIAN_POINT ( 'NONE',  ( -0.2755905511811018171, 0.2952755905511811885, 0.000000000000000000 ) ) ;
#35128=CARTESIAN_POINT ( 'NONE',  ( -1.476377952755905110, 0.07958543189024085140, 0.2665933059059887866 ) ) ;
#35130=CARTESIAN_POINT ( 'NONE',  ( 0.2624671916010504757, -0.6046776061558809534, -0.2411417322834644161 ) ) ;
#35131=EDGE_CURVE ( 'NONE', #24616, #66982, #78196, .T. ) ;
#35132=CARTESIAN_POINT ( 'NONE',  ( -1.646051170424378096, 0.000000000000000000, -0.3464511005275205946 ) ) ;
#35134=CARTESIAN_POINT ( 'NONE',  ( -1.279527559055116948, -0.5400638737290844871, 0.3530559997133364547 ) ) ;
#35135=CARTESIAN_POINT ( 'NONE',  ( -0.5905511811023615998, 0.1771653543307087630, 0.000000000000000000 ) ) ;
#35136=CARTESIAN_POINT ( 'NONE',  ( -1.555118110236219930, -0.5400638737290845981, -0.3530559997133363437 ) ) ;
#35137=CARTESIAN_POINT ( 'NONE',  ( 0.1706036745406830368, -0.4281496062992127816, -0.4176697321401328100 ) ) ;
#35138=CARTESIAN_POINT ( 'NONE',  ( 0.5577427821522316087, -0.08942795157527998196, 0.3641732283464567121 ) ) ;
#35139=CARTESIAN_POINT ( 'NONE',  ( -0.8530183727034112984, -0.3690944881889765550, -0.3153832671262227771 ) ) ;
#35140=CARTESIAN_POINT ( 'NONE',  ( -1.069553805774277722, 0.2952755905511811885, 0.1292274648535926551 ) ) ;
#35141=CARTESIAN_POINT ( 'NONE',  ( -1.417322834645668772, -0.1870078740157479769, 0.4822834645669291653 ) ) ;
#35142=CARTESIAN_POINT ( 'NONE',  ( 1.417322834645670104, -0.1870078740157480879, -0.4822834645669291653 ) ) ;
#35144=CARTESIAN_POINT ( 'NONE',  ( 0.8595800524934390507, -0.2845877964562159024, 0.3641732283464567677 ) ) ;
#35145=CARTESIAN_POINT ( 'NONE',  ( 0.8989501312335964611, 0.2952755905511811885, 0.1292274648535926551 ) ) ;
#35147=CARTESIAN_POINT ( 'NONE',  ( 1.312335958005249825, 0.1283753931104746893, -0.1820866141732285504 ) ) ;
#35149=CARTESIAN_POINT ( 'NONE',  ( -0.7677165354330699465, -0.5400638737290845981, -0.3530559997133363437 ) ) ;
#35150=B_SPLINE_CURVE_WITH_KNOTS ( 'NONE', 3,
 ( #68881, #48688, #43597, #10412 ),
 .UNSPECIFIED., .F., .F.,
 ( 4, 4 ),
 ( 3.593986969189856797E-07, 0.001287825409103300319 ),
 .UNSPECIFIED. ) ;
#35153=CARTESIAN_POINT ( 'NONE',  ( -1.384514435695537005, -0.5511811023622048555, -0.09757992244046775898 ) ) ;
#35154=CARTESIAN_POINT ( 'NONE',  ( -0.7742782152230962556, -0.4281496062992127816, -0.4176697321401328100 ) ) ;
#35155=CARTESIAN_POINT ( 'NONE',  ( 0.5118110236220478892, 0.2952755905511811885, 0.000000000000000000 ) ) ;
#35156=CARTESIAN_POINT ( 'NONE',  ( -1.541994750656167090, 0.1771653543307087630, 0.09757992244046791164 ) ) ;
#35158=CARTESIAN_POINT ( 'NONE',  ( -1.535433070866141225, 0.2952755905511811885, 0.000000000000000000 ) ) ;
#35159=CARTESIAN_POINT ( 'NONE',  ( 0.5446194225721792126, -0.3162353388693405765, 0.4822834645669290543 ) ) ;
#35160=CARTESIAN_POINT ( 'NONE',  ( -0.03280839895013062252, 0.2952755905511810774, -0.1292274648535930714 ) ) ;
#35161=CARTESIAN_POINT ( 'NONE',  ( 0.8595800524934390507, -0.05778040916215560624, -0.4822834645669293319 ) ) ;
#35165=CARTESIAN_POINT ( 'NONE',  ( -0.9548908091195642545, -2.567464376874931580E-15, -0.4445507791589072832 ) ) ;
#35167=CARTESIAN_POINT ( 'NONE',  ( -0.1443569553805768291, -0.004921259842519576551, 0.3153832671262227771 ) ) ;
#35168=CARTESIAN_POINT ( 'NONE',  ( -0.4461942257217840213, 0.2306618581243848609, 0.2411417322834645549 ) ) ;
#35169=CARTESIAN_POINT ( 'NONE',  ( 0.7020997375328090762, -0.05778040916215560624, -0.4822834645669293319 ) ) ;
#35171=CARTESIAN_POINT ( 'NONE',  ( 0.05249343832021075018, -0.5023911411419708095, 0.1820866141732285504 ) ) ;
#35172=CARTESIAN_POINT ( 'NONE',  ( -1.292650918635170010, 0.2952755905511810774, -0.1292274648535930714 ) ) ;
#35173=CARTESIAN_POINT ( 'NONE',  ( 1.154855643044620184, 0.2306618581243847221, -0.2411417322834647770 ) ) ;
#35178=ORIENTED_EDGE ( 'NONE', *, *, #67069, .F. ) ;
#35179=CARTESIAN_POINT ( 'NONE',  ( 1.049868766404200127, -0.6046776061558809534, -0.2411417322834644161 ) ) ;
#35180=CARTESIAN_POINT ( 'NONE',  ( -1.732283464566928277, -0.1870078740157479769, 0.4822834645669291653 ) ) ;
#35181=CARTESIAN_POINT ( 'NONE',  ( -1.069553805774277722, -0.5511811023622048555, -0.09757992244046775898 ) ) ;
#35182=CARTESIAN_POINT ( 'NONE',  ( -1.227034120734907141, -0.6692913385826773087, -0.1292274648535924053 ) ) ;
#35184=CARTESIAN_POINT ( 'NONE',  ( -0.9842519685039360366, 0.2066929133858268208, 0.000000000000000000 ) ) ;
#35185=CARTESIAN_POINT ( 'NONE',  ( 1.089238845144357759, 0.05413385826771626580, -0.4176697321401330321 ) ) ;
#35187=CARTESIAN_POINT ( 'NONE',  ( 0.05249343832021075018, 0.2306618581243847221, -0.2411417322834647770 ) ) ;
#35188=CARTESIAN_POINT ( 'NONE',  ( -0.5708661417322828946, 0.1660481256975883668, -0.3530559997133364547 ) ) ;
#35189=CARTESIAN_POINT ( 'NONE',  ( 1.581364829396326277, -0.05778040916215522460, 0.4822834645669289988 ) ) ;
#35191=CARTESIAN_POINT ( 'NONE',  ( 0.2427821522309716595, -0.3162353388693409650, -0.4822834645669289433 ) ) ;
#35193=CARTESIAN_POINT ( 'NONE',  ( -1.430446194225720724, -0.004921259842519870586, -0.3153832671262229437 ) ) ;
#35196=VERTEX_POINT ( 'NONE', #65876 ) ;
#35198=CARTESIAN_POINT ( 'NONE',  ( -1.581364829396324945, -0.3162353388693405765, 0.4822834645669290543 ) ) ;
#35200=CARTESIAN_POINT ( 'NONE',  ( -1.699475065616797398, 0.2952755905511811885, 0.1292274648535926551 ) ) ;
#35201=CARTESIAN_POINT ( 'NONE',  ( -1.587926509186350810, -0.4281496062992124485, 0.4176697321401328655 ) ) ;
#35202=CARTESIAN_POINT ( 'NONE',  ( -0.9580052493438311334, 0.05413385826771626580, -0.4176697321401330321 ) ) ;
#35205=CARTESIAN_POINT ( 'NONE',  ( -0.4724409448818890911, -0.1870078740157480601, -0.3641732283464567677 ) ) ;
#35206=CARTESIAN_POINT ( 'NONE',  ( -0.7874015748031489847, -0.1870078740157479769, 0.3641732283464567677 ) ) ;
#35207=CARTESIAN_POINT ( 'NONE',  ( -1.115485564304461219, 0.05413385826771626580, -0.4176697321401330321 ) ) ;
#35208=CARTESIAN_POINT ( 'NONE',  ( 0.4986876640419954376, 0.2306618581243848609, 0.2411417322834645549 ) ) ;
#35209=CARTESIAN_POINT ( 'NONE',  ( -1.003937007874014853, 0.1660481256975885056, 0.3530559997133364547 ) ) ;
#35212=CARTESIAN_POINT ( 'NONE',  ( -1.423884514435694859, -0.05778040916215560624, -0.4822834645669293319 ) ) ;
#35216=CARTESIAN_POINT ( 'NONE',  ( -1.614173228346457378, 1.055049524192299693, -0.1372047244094477536 ) ) ;
#35219=CARTESIAN_POINT ( 'NONE',  ( -0.8398950131233585692, 0.2306618581243848609, 0.2411417322834645549 ) ) ;
#35220=CARTESIAN_POINT ( 'NONE',  ( 1.240157480314961314, 0.1660481256975883668, -0.3530559997133364547 ) ) ;
#35223=CARTESIAN_POINT ( 'NONE',  ( -0.6889763779527551257, 0.1012011053420777407, 0.2882089793578256898 ) ) ;
#35224=CARTESIAN_POINT ( 'NONE',  ( -1.476377952755905110, -0.5400638737290845981, -0.3530559997133363437 ) ) ;
#35225=CARTESIAN_POINT ( 'NONE',  ( -0.6496062992125976043, -0.5400638737290844871, 0.3530559997133364547 ) ) ;
#35227=CARTESIAN_POINT ( 'NONE',  ( 0.3018372703412079971, -0.3690944881889763329, 0.3153832671262228327 ) ) ;
#35229=CARTESIAN_POINT ( 'NONE',  ( 0.1312335958005257930, 0.1283753931104746893, -0.1820866141732285504 ) ) ;
#35230=CARTESIAN_POINT ( 'NONE',  ( 1.036745406824147508, -0.3690944881889765550, -0.3153832671262227771 ) ) ;
#35231=CARTESIAN_POINT ( 'NONE',  ( 1.102362204724410155, -0.1870078740157479769, 0.4822834645669291653 ) ) ;
#35232=VECTOR ( 'NONE', #19404, 39.37007874015748854 ) ;
#35233=CARTESIAN_POINT ( 'NONE',  ( -0.2755905511811015396, -0.5511811023622047445, 6.969142054262312111E-17 ) ) ;
#35235=CARTESIAN_POINT ( 'NONE',  ( 1.509186351706037543, -0.4281496062992127816, -0.4176697321401328100 ) ) ;
#35236=CARTESIAN_POINT ( 'NONE',  ( -1.391076115485563314, -0.5023911411419708095, -0.1820866141732282451 ) ) ;
#35239=CARTESIAN_POINT ( 'NONE',  ( 0.05905511811023709395, -0.5400638737290844871, 0.3530559997133364547 ) ) ;
#35240=CARTESIAN_POINT ( 'NONE',  ( 1.541994750656168645, 0.1771653543307087075, -0.09757992244046823083 ) ) ;
#35241=CARTESIAN_POINT ( 'NONE',  ( 0.3543307086614179147, 0.1771653543307087630, 0.000000000000000000 ) ) ;
#35242=CARTESIAN_POINT ( 'NONE',  ( -0.3543307086614165824, -0.5511811023622047445, 6.969142054262312111E-17 ) ) ;
#35243=CARTESIAN_POINT ( 'NONE',  ( -0.9317585301837263412, -0.4281496062992127816, -0.4176697321401328100 ) ) ;
#35244=DIRECTION ( 'NONE',  ( -1.000000000000000000, -3.469446951953613696E-16, 0.000000000000000000 ) ) ;
#35246=CARTESIAN_POINT ( 'NONE',  ( 0.1246719160104994284, 0.2952755905511810774, -0.1292274648535930714 ) ) ;
#35249=CARTESIAN_POINT ( 'NONE',  ( 0.3049517105654749871, 8.471767977567108961E-16, -0.4445507791589058955 ) ) ;
#35250=CARTESIAN_POINT ( 'NONE',  ( -0.4133858267716528645, 0.07958543189024071263, -0.2665933059059888421 ) ) ;
#35251=CARTESIAN_POINT ( 'NONE',  ( -0.2624671916010490880, 0.2306618581243847221, -0.2411417322834647770 ) ) ;
#35252=CARTESIAN_POINT ( 'NONE',  ( -1.345144356955379816, -0.3162353388693405765, 0.4822834645669290543 ) ) ;
#35253=CARTESIAN_POINT ( 'NONE',  ( -1.541994750656167090, -0.5511811023622048555, -0.09757992244046775898 ) ) ;
#35254=CARTESIAN_POINT ( 'NONE',  ( 1.476377952755906442, -0.5400638737290844871, 0.3530559997133364547 ) ) ;
#35255=CARTESIAN_POINT ( 'NONE',  ( -1.286089238845143479, 0.2306618581243847221, -0.2411417322834647770 ) ) ;
#35256=CARTESIAN_POINT ( 'NONE',  ( -0.7283464566929126471, 0.07958543189024071263, -0.2665933059059888421 ) ) ;
#35260=DIRECTION ( 'NONE',  ( -1.000000000000000000, -3.096699300667737957E-16, 1.692413147294446216E-16 ) ) ;
#35261=CARTESIAN_POINT ( 'NONE',  ( 1.187664041994751285, -0.2845877964562161244, -0.3641732283464567121 ) ) ;
#35262=CARTESIAN_POINT ( 'NONE',  ( -1.535433070866141225, 0.2952755905511811885, 0.000000000000000000 ) ) ;
#35263=CARTESIAN_POINT ( 'NONE',  ( 0.7677165354330716118, -0.5400638737290844871, 0.3530559997133364547 ) ) ;
#35265=CARTESIAN_POINT ( 'NONE',  ( 1.292650918635171564, -0.5511811023622048555, -0.09757992244046775898 ) ) ;
#35266=CARTESIAN_POINT ( 'NONE',  ( 0.2230971128608932319, -0.4281496062992124485, 0.4176697321401328655 ) ) ;
#35267=CARTESIAN_POINT ( 'NONE',  ( -0.7020997375328074108, -0.05778040916215522460, 0.4822834645669289988 ) ) ;
#35271=CARTESIAN_POINT ( 'NONE',  ( 0.3608923884514443348, 0.1771653543307087075, -0.09757992244046823083 ) ) ;
#35276=CARTESIAN_POINT ( 'NONE',  ( -0.5249343832020990641, -0.6046776061558809534, -0.2411417322834644161 ) ) ;
#35278=CARTESIAN_POINT ( 'NONE',  ( -0.1837270341207340729, 0.2306618581243847221, -0.2411417322834647770 ) ) ;
#35279=CARTESIAN_POINT ( 'NONE',  ( -0.4790026246719152336, -0.08942795157528024563, -0.3641732283464568787 ) ) ;
#35280=CARTESIAN_POINT ( 'NONE',  ( 0.7086614173228353852, -0.1870078740157479769, 0.4822834645669291653 ) ) ;
#35281=EDGE_CURVE ( 'NONE', #61268, #49328, #53216, .T. ) ;
#35282=CARTESIAN_POINT ( 'NONE',  ( -0.7283464566929126471, -0.5400638737290844871, 0.3530559997133364547 ) ) ;
#35283=CARTESIAN_POINT ( 'NONE',  ( -0.2296587926509179312, -0.3162353388693409650, -0.4822834645669289433 ) ) ;
#35284=CARTESIAN_POINT ( 'NONE',  ( 1.207349081364829990, -0.6046776061558809534, -0.2411417322834644161 ) ) ;
#35286=CARTESIAN_POINT ( 'NONE',  ( 1.062992125984252745, -0.6692913385826771977, 8.415575281601705876E-17 ) ) ;
#35287=CARTESIAN_POINT ( 'NONE',  ( 0.7086614173228353852, -0.1870078740157479769, 0.4822834645669291653 ) ) ;
#35289=CARTESIAN_POINT ( 'NONE',  ( -0.1509186351706028884, -0.2845877964562161244, -0.3641732283464567121 ) ) ;
#35292=ORIENTED_EDGE ( 'NONE', *, *, #79015, .T. ) ;
#35293=CARTESIAN_POINT ( 'NONE',  ( -1.062992125984250968, 0.1771653543307087630, 0.000000000000000000 ) ) ;
#35294=CARTESIAN_POINT ( 'NONE',  ( -0.5511811023622038563, -0.1870078740157479769, 0.4822834645669291653 ) ) ;
#35296=CARTESIAN_POINT ( 'NONE',  ( -0.2230971128608915943, -0.4281496062992127816, -0.4176697321401328100 ) ) ;
#35297=CARTESIAN_POINT ( 'NONE',  ( -0.6102362204724400829, 0.1660481256975885056, 0.3530559997133364547 ) ) ;
#35298=CARTESIAN_POINT ( 'NONE',  ( -1.089238845144356427, -0.4281496062992127816, -0.4176697321401328100 ) ) ;
#35299=CARTESIAN_POINT ( 'NONE',  ( -1.299212598425196097, -0.6692913385826771977, 8.415575281601705876E-17 ) ) ;
#35300=CARTESIAN_POINT ( 'NONE',  ( 1.030183727034121421, -0.08942795157527998196, 0.3641732283464567121 ) ) ;
#35303=CARTESIAN_POINT ( 'NONE',  ( 0.3937007874015754361, -0.1870078740157480601, -0.3641732283464567677 ) ) ;
#35304=CARTESIAN_POINT ( 'NONE',  ( -0.02624671916010428221, 0.2306618581243847221, -0.2411417322834647770 ) ) ;
#35305=CARTESIAN_POINT ( 'NONE',  ( 0.4921259842519691285, -0.5400638737290845981, -0.3530559997133363437 ) ) ;
#35306=VERTEX_POINT ( 'NONE', #58283 ) ;
#35308=CARTESIAN_POINT ( 'NONE',  ( -0.6102362204724400829, 0.1660481256975885056, 0.3530559997133364547 ) ) ;
#35312=CARTESIAN_POINT ( 'NONE',  ( -0.7020997375328076329, -0.2845877964562161244, -0.3641732283464567121 ) ) ;
#35313=CARTESIAN_POINT ( 'NONE',  ( -1.089238845144356427, 0.05413385826771666132, 0.4176697321401328100 ) ) ;
#35316=CARTESIAN_POINT ( 'NONE',  ( 1.607611548556431069, -0.6692913385826773087, -0.1292274648535924053 ) ) ;
#35317=CARTESIAN_POINT ( 'NONE',  ( 1.069553805774278610, -0.6692913385826771977, 0.1292274648535927661 ) ) ;
#35318=CARTESIAN_POINT ( 'NONE',  ( 0.3083989501312343062, -0.05778040916215560624, -0.4822834645669293319 ) ) ;
#35319=CARTESIAN_POINT ( 'NONE',  ( -0.6299212598425188991, -0.1870078740157480601, -0.3641732283464567677 ) ) ;
#35320=CARTESIAN_POINT ( 'NONE',  ( 0.1246719160104994284, -0.6692913385826771977, 0.1292274648535927661 ) ) ;
#35322=CARTESIAN_POINT ( 'NONE',  ( 0.03280839895013198948, -0.5511811023622048555, -0.09757992244046775898 ) ) ;
#35323=CARTESIAN_POINT ( 'NONE',  ( -0.2559055118110230564, 0.1660481256975883668, -0.3530559997133364547 ) ) ;
#35324=EDGE_CURVE ( 'NONE', #1754, #64485, #40193, .T. ) ;
#35326=CARTESIAN_POINT ( 'NONE',  ( -1.614173228346456268, -0.6692913385826771977, 8.415575281601705876E-17 ) ) ;
#35327=CARTESIAN_POINT ( 'NONE',  ( 0.006561679790026889343, -0.08942795157527998196, 0.3641732283464567121 ) ) ;
#35328=CARTESIAN_POINT ( 'NONE',  ( 1.620734908136483465, -0.5511811023622046335, 0.09757992244046803654 ) ) ;
#35329=CARTESIAN_POINT ( 'NONE',  ( -1.095800524934382292, -0.05778040916215522460, 0.4822834645669289988 ) ) ;
#35330=CARTESIAN_POINT ( 'NONE',  ( -0.8398950131233585692, 0.1283753931104748280, 0.1820866141732283561 ) ) ;
#35332=CARTESIAN_POINT ( 'NONE',  ( -0.9514435695538050464, -0.3162353388693405765, 0.4822834645669290543 ) ) ;
#35333=CARTESIAN_POINT ( 'NONE',  ( -0.5511811023622038563, -0.1870078740157479769, 0.4822834645669291653 ) ) ;
#35334=CARTESIAN_POINT ( 'NONE',  ( 0.2099737532808405305, -0.6046776061558807314, 0.2411417322834647770 ) ) ;
#35337=CARTESIAN_POINT ( 'NONE',  ( 0.3740157480314966754, -0.4536011799217367080, 0.2665933059059888421 ) ) ;
#35338=CARTESIAN_POINT ( 'NONE',  ( 1.023622047244095112, -0.1870078740157480879, -0.4822834645669291653 ) ) ;
#35339=B_SPLINE_CURVE_WITH_KNOTS ( 'NONE', 3,
 ( #6452, #63695, #44316, #44724, #77588, #38849, #39266 ),
 .UNSPECIFIED., .F., .F.,
 ( 4, 3, 4 ),
 ( 1.908195823574487804E-17, 0.001246232571205249445, 0.002492492258783241595 ),
 .UNSPECIFIED. ) ;
#35340=CARTESIAN_POINT ( 'NONE',  ( -1.200787401574802349, 0.07958543189024071263, -0.2665933059059888421 ) ) ;
#35341=CARTESIAN_POINT ( 'NONE',  ( 1.003937007874016407, -0.5400638737290844871, 0.3530559997133364547 ) ) ;
#35342=CARTESIAN_POINT ( 'NONE',  ( -1.686351706036744558, 0.1771653543307087075, -0.09757992244046823083 ) ) ;
#35344=CARTESIAN_POINT ( 'NONE',  ( -0.4921259842519677963, -0.5400638737290844871, 0.3530559997133364547 ) ) ;
#35345=CARTESIAN_POINT ( 'NONE',  ( 0.2230971128608932319, -0.3690944881889763329, 0.3153832671262228327 ) ) ;
#35346=PLANE ( 'NONE',  #27321 ) ;
#35347=CARTESIAN_POINT ( 'NONE',  ( 0.7152230971128614723, -0.2845877964562161244, -0.3641732283464567121 ) ) ;
#35348=CARTESIAN_POINT ( 'NONE',  ( -0.1443569553805765515, -0.4281496062992127816, -0.4176697321401328100 ) ) ;
#35350=CARTESIAN_POINT ( 'NONE',  ( -1.043307086614172707, 0.1660481256975883668, -0.3530559997133364547 ) ) ;
#35352=CARTESIAN_POINT ( 'NONE',  ( 1.148293963254593653, 0.1771653543307087075, -0.09757992244046823083 ) ) ;
#35353=CARTESIAN_POINT ( 'NONE',  ( 0.03280839895013198948, -0.6692913385826773087, -0.1292274648535924053 ) ) ;
#35354=CARTESIAN_POINT ( 'NONE',  ( -0.2493438320209966919, -0.4281496062992124485, 0.4176697321401328655 ) ) ;
#35355=CARTESIAN_POINT ( 'NONE',  ( -0.2887139107611542133, -0.5023911411419708095, -0.1820866141732282451 ) ) ;
#35357=CARTESIAN_POINT ( 'NONE',  ( -0.4330708661417315697, -0.5511811023622047445, 6.969142054262312111E-17 ) ) ;
#35358=CARTESIAN_POINT ( 'NONE',  ( 0.3018372703412079971, 0.05413385826771626580, -0.4176697321401330321 ) ) ;
#35359=CARTESIAN_POINT ( 'NONE',  ( -1.318897637795274802, -0.4536011799217368745, -0.2665933059059886201 ) ) ;
#35361=CARTESIAN_POINT ( 'NONE',  ( -1.181102362204723644, -0.1870078740157479769, 0.4822834645669291653 ) ) ;
#35363=VERTEX_POINT ( 'NONE', #51964 ) ;
#35364=CARTESIAN_POINT ( 'NONE',  ( -1.364829396325458521, 0.1283753931104746893, -0.1820866141732285504 ) ) ;
#35365=CARTESIAN_POINT ( 'NONE',  ( -0.4527559055118102749, 0.1660481256975885056, 0.3530559997133364547 ) ) ;
#35367=CARTESIAN_POINT ( 'NONE',  ( -1.292650918635170010, 0.2952755905511810774, -0.1292274648535930714 ) ) ;
#35370=CARTESIAN_POINT ( 'NONE',  ( 1.397637795275591177, 0.1660481256975883668, -0.3530559997133364547 ) ) ;
#35371=CARTESIAN_POINT ( 'NONE',  ( 1.003937007874016407, -0.5400638737290844871, 0.3530559997133364547 ) ) ;
#35373=CARTESIAN_POINT ( 'NONE',  ( -0.7480314960629922405, 2.244094488188976388, 0.000000000000000000 ) ) ;
#35374=CARTESIAN_POINT ( 'NONE',  ( -1.581364829396324945, -0.3162353388693405765, 0.4822834645669290543 ) ) ;
#35375=EDGE_CURVE ( 'NONE', #17097, #3706, #33876, .T. ) ;
#35378=CARTESIAN_POINT ( 'NONE',  ( -0.5708661417322825615, -0.4536011799217367080, 0.2665933059059888421 ) ) ;
#35380=VERTEX_POINT ( 'NONE', #59542 ) ;
#35381=CARTESIAN_POINT ( 'NONE',  ( 0.8333333333333340365, 0.2952755905511810774, -0.1292274648535930714 ) ) ;
#35382=CARTESIAN_POINT ( 'NONE',  ( -0.2952755905511804668, 0.1660481256975885056, 0.3530559997133364547 ) ) ;
#35383=CARTESIAN_POINT ( 'NONE',  ( -1.154855643044618851, 0.2306618581243848609, 0.2411417322834645549 ) ) ;
#35384=CARTESIAN_POINT ( 'NONE',  ( 1.502624671916010790, -0.05778040916215522460, 0.4822834645669289988 ) ) ;
#35385=CARTESIAN_POINT ( 'NONE',  ( -1.371391076115484609, -0.5511811023622046335, 0.09757992244046803654 ) ) ;
#35387=CARTESIAN_POINT ( 'NONE',  ( 0.4396325459317593221, 0.2952755905511810774, -0.1292274648535930714 ) ) ;
#35388=CARTESIAN_POINT ( 'NONE',  ( -0.9055118110236215490, -0.6692913385826771977, 8.415575281601705876E-17 ) ) ;
#35390=CARTESIAN_POINT ( 'NONE',  ( -1.036745406824146176, -0.4281496062992124485, 0.4176697321401328655 ) ) ;
#35392=CARTESIAN_POINT ( 'NONE',  ( 1.115485564304462551, -0.4281496062992127816, -0.4176697321401328100 ) ) ;
#35393=CARTESIAN_POINT ( 'NONE',  ( 1.437007874015748810, -0.4536011799217368745, -0.2665933059059886201 ) ) ;
#35396=CARTESIAN_POINT ( 'NONE',  ( -0.4527559055118102749, -0.5400638737290845981, -0.3530559997133363437 ) ) ;
#35398=CARTESIAN_POINT ( 'NONE',  ( 0.4921259842519691285, 0.07958543189024085140, 0.2665933059059887866 ) ) ;
#35399=CARTESIAN_POINT ( 'NONE',  ( -1.292650918635170010, -0.6692913385826771977, 0.1292274648535927661 ) ) ;
#35400=CARTESIAN_POINT ( 'NONE',  ( 1.102362204724410155, -0.1870078740157479769, 0.4822834645669291653 ) ) ;
#35401=CARTESIAN_POINT ( 'NONE',  ( 0.8858267716535438430, -0.5400638737290845981, -0.3530559997133363437 ) ) ;
#35402=CARTESIAN_POINT ( 'NONE',  ( -0.3412073490813641308, -0.6046776061558807314, 0.2411417322834647770 ) ) ;
#35405=CARTESIAN_POINT ( 'NONE',  ( -0.8267716535433065062, 0.2952755905511811885, 0.000000000000000000 ) ) ;
#35407=CARTESIAN_POINT ( 'NONE',  ( -1.666666666666665853, 0.05413385826771626580, -0.4176697321401330321 ) ) ;
#35408=CARTESIAN_POINT ( 'NONE',  ( -0.8464566929133852113, 0.1660481256975885056, 0.3530559997133364547 ) ) ;
#35409=CARTESIAN_POINT ( 'NONE',  ( 1.174540682414699111, -0.3162353388693405765, 0.4822834645669290543 ) ) ;
#35410=CARTESIAN_POINT ( 'NONE',  ( 1.555118110236221041, 0.1660481256975883668, -0.3530559997133364547 ) ) ;
#35411=CARTESIAN_POINT ( 'NONE',  ( -0.9842519685039365918, -0.6692913385826771977, 8.415575281601705876E-17 ) ) ;
#35413=CARTESIAN_POINT ( 'NONE',  ( 0.3805774278215230400, 0.05413385826771626580, -0.4176697321401330321 ) ) ;
#35415=CARTESIAN_POINT ( 'NONE',  ( -0.5511811023622038563, -0.1870078740157479769, 0.4822834645669291653 ) ) ;
#35416=CARTESIAN_POINT ( 'NONE',  ( -1.456692913385826182, 0.1771653543307087630, 0.000000000000000000 ) ) ;
#35417=CARTESIAN_POINT ( 'NONE',  ( 0.7939632545931766261, -0.2845877964562161244, -0.3641732283464567121 ) ) ;
#35418=CARTESIAN_POINT ( 'NONE',  ( 1.391076115485564868, -0.6046776061558807314, 0.2411417322834647770 ) ) ;
#35420=CARTESIAN_POINT ( 'NONE',  ( 1.030183727034121421, -0.08942795157527998196, 0.3641732283464567121 ) ) ;
#35421=CARTESIAN_POINT ( 'NONE',  ( 0.8792650918635177559, -0.4281496062992127816, -0.4176697321401328100 ) ) ;
#35423=CARTESIAN_POINT ( 'NONE',  ( -0.3543307086614165824, -0.6692913385826771977, 8.415575281601705876E-17 ) ) ;
#35425=CARTESIAN_POINT ( 'NONE',  ( 1.371391076115485719, -0.5511811023622048555, -0.09757992244046775898 ) ) ;
#35426=CARTESIAN_POINT ( 'NONE',  ( -0.6233595800524928121, -0.05778040916215522460, 0.4822834645669289988 ) ) ;
#35428=CARTESIAN_POINT ( 'NONE',  ( 1.338582677165355062, -0.1870078740157479769, 0.4822834645669291653 ) ) ;
#35429=CARTESIAN_POINT ( 'NONE',  ( 0.2690288713910767848, -0.6692913385826773087, -0.1292274648535924053 ) ) ;
#35430=CARTESIAN_POINT ( 'NONE',  ( 0.4593175853018380828, -0.004921259842519870586, -0.3153832671262229437 ) ) ;
#35431=CARTESIAN_POINT ( 'NONE',  ( -1.646051170424378096, 0.8346805926620876059, -0.5309055118110233007 ) ) ;
#35432=CARTESIAN_POINT ( 'NONE',  ( -0.03937007874015669567, 0.1771653543307087630, 0.000000000000000000 ) ) ;
#35433=CARTESIAN_POINT ( 'NONE',  ( -1.568241469816272105, -0.3162353388693409650, -0.4822834645669289433 ) ) ;
#35435=CARTESIAN_POINT ( 'NONE',  ( 0.8792650918635177559, 0.05413385826771666132, 0.4176697321401328100 ) ) ;
#35437=CARTESIAN_POINT ( 'NONE',  ( 1.463254593175853824, -0.5511811023622046335, 0.09757992244046803654 ) ) ;
#35438=FACE_OUTER_BOUND ( 'NONE', #25950, .T. ) ;
#35439=CARTESIAN_POINT ( 'NONE',  ( 0.06561679790026316017, -0.004921259842519870586, -0.3153832671262229437 ) ) ;
#35440=CARTESIAN_POINT ( 'NONE',  ( 0.1049868766404206816, 0.2306618581243848609, 0.2411417322834645549 ) ) ;
#35441=CARTESIAN_POINT ( 'NONE',  ( 1.548556430446194954, 0.1283753931104746893, -0.1820866141732285504 ) ) ;
#35442=CARTESIAN_POINT ( 'NONE',  ( -1.167979002624671470, -0.3690944881889765550, -0.3153832671262227771 ) ) ;
#35443=CARTESIAN_POINT ( 'NONE',  ( -1.620734908136482577, -0.6692913385826773087, -0.1292274648535924053 ) ) ;
#35444=CONICAL_SURFACE ( 'NONE', #28712, 1.181102362204724310, 0.7853981633974621568 ) ;
#35445=CARTESIAN_POINT ( 'NONE',  ( 0.4265091863517067594, 0.2952755905511811885, 0.1292274648535926551 ) ) ;
#35446=CARTESIAN_POINT ( 'NONE',  ( 1.266404199475066328, -0.3162353388693409650, -0.4822834645669289433 ) ) ;
#35448=CARTESIAN_POINT ( 'NONE',  ( 0.1377952755905518800, -0.5400638737290844871, 0.3530559997133364547 ) ) ;
#35449=CARTESIAN_POINT ( 'NONE',  ( 1.141732283464567788, -0.6692913385826771977, 8.415575281601705876E-17 ) ) ;
#35450=CARTESIAN_POINT ( 'NONE',  ( 0.8727034120734913358, -0.05778040916215522460, 0.4822834645669289988 ) ) ;
#35451=LINE ( 'NONE', #29134, #69601 ) ;
#35452=CARTESIAN_POINT ( 'NONE',  ( 0.7939632545931766261, -0.2845877964562161244, -0.3641732283464567121 ) ) ;
#35453=CARTESIAN_POINT ( 'NONE',  ( 1.417322834645670104, -0.1870078740157480879, -0.4822834645669291653 ) ) ;
#35454=CARTESIAN_POINT ( 'NONE',  ( 0.4855643044619428750, -0.004921259842519576551, 0.3153832671262227771 ) ) ;
#35456=CARTESIAN_POINT ( 'NONE',  ( -0.03937007874015669567, 0.2952755905511811885, 0.000000000000000000 ) ) ;
#35457=CARTESIAN_POINT ( 'NONE',  ( 0.6627296587926515548, 0.2952755905511811885, 0.1292274648535926551 ) ) ;
#35458=CARTESIAN_POINT ( 'NONE',  ( -0.2493438320209966919, -0.4281496062992124485, 0.4176697321401328655 ) ) ;
#35459=CARTESIAN_POINT ( 'NONE',  ( -0.006561679790025524116, -0.2845877964562159024, 0.3641732283464567677 ) ) ;
#35460=CARTESIAN_POINT ( 'NONE',  ( 0.8202099737532813073, 0.2952755905511811885, 0.1292274648535926551 ) ) ;
#35463=CARTESIAN_POINT ( 'NONE',  ( -1.115485564304461219, -0.4281496062992124485, 0.4176697321401328655 ) ) ;
#35464=CARTESIAN_POINT ( 'NONE',  ( -1.090776338374007226, 0.02791078216816064370, 0.4328096321851915285 ) ) ;
#35467=CARTESIAN_POINT ( 'NONE',  ( -1.377952755905511140, -0.6692913385826771977, 8.415575281601705876E-17 ) ) ;
#35468=CARTESIAN_POINT ( 'NONE',  ( -0.4527559055118102749, 0.1660481256975885056, 0.3530559997133364547 ) ) ;
#35472=CARTESIAN_POINT ( 'NONE',  ( 0.6036745406824154392, 0.1283753931104746893, -0.1820866141732285504 ) ) ;
#35474=CARTESIAN_POINT ( 'NONE',  ( 0.9973753280839902091, 0.2306618581243847221, -0.2411417322834647770 ) ) ;
#35476=DIRECTION ( 'NONE',  ( -1.000000000000000000, -3.553564358545519864E-16, 0.000000000000000000 ) ) ;
#35477=CARTESIAN_POINT ( 'NONE',  ( -1.541994750656167090, 0.1771653543307087630, 0.09757992244046791164 ) ) ;
#35478=CARTESIAN_POINT ( 'NONE',  ( 1.673228346456693494, 0.1660481256975885056, 0.3530559997133364547 ) ) ;
#35479=CARTESIAN_POINT ( 'NONE',  ( -1.620734908136482577, -0.6692913385826773087, -0.1292274648535924053 ) ) ;
#35480=CARTESIAN_POINT ( 'NONE',  ( 0.2559055118110243332, 0.1660481256975885056, 0.3530559997133364547 ) ) ;
#35482=CARTESIAN_POINT ( 'NONE',  ( 0.01968503937007957949, -0.5400638737290845981, -0.3530559997133363437 ) ) ;
#35483=CARTESIAN_POINT ( 'NONE',  ( -0.7611548556430438595, 0.1283753931104748280, 0.1820866141732283561 ) ) ;
#35484=CARTESIAN_POINT ( 'NONE',  ( 0.8792650918635177559, -0.4281496062992127816, -0.4176697321401328100 ) ) ;
#35485=CARTESIAN_POINT ( 'NONE',  ( 0.08530183727034192087, -0.3162353388693409650, -0.4822834645669289433 ) ) ;
#35489=CARTESIAN_POINT ( 'NONE',  ( 0.9120734908136490793, 0.2952755905511810774, -0.1292274648535930714 ) ) ;
#35490=CARTESIAN_POINT ( 'NONE',  ( 0.05249343832021075018, 0.2306618581243847221, -0.2411417322834647770 ) ) ;
#35491=CARTESIAN_POINT ( 'NONE',  ( -0.8989501312335946848, -0.6692913385826771977, 0.1292274648535927661 ) ) ;
#35492=CARTESIAN_POINT ( 'NONE',  ( 1.043307086614173818, -0.5400638737290845981, -0.3530559997133363437 ) ) ;
#35493=CARTESIAN_POINT ( 'NONE',  ( 0.3543307086614181922, -0.6692913385826771977, 8.415575281601705876E-17 ) ) ;
#35495=CARTESIAN_POINT ( 'NONE',  ( -0.5052493438320203589, -0.6692913385826771977, 0.1292274648535927661 ) ) ;
#35496=CARTESIAN_POINT ( 'NONE',  ( 0.7480314960629927956, 0.2952755905511811885, 0.000000000000000000 ) ) ;
#35497=CARTESIAN_POINT ( 'NONE',  ( 0.1443569553805781891, 0.05413385826771626580, -0.4176697321401330321 ) ) ;
#35499=CARTESIAN_POINT ( 'NONE',  ( 0.6496062992125991586, -0.4536011799217368745, -0.2665933059059886201 ) ) ;
#35500=FACE_OUTER_BOUND ( 'NONE', #52403, .T. ) ;
#35501=CARTESIAN_POINT ( 'NONE',  ( -1.646981627296586703, -0.3162353388693409650, -0.4822834645669289433 ) ) ;
#35502=CARTESIAN_POINT ( 'NONE',  ( 0.4199475065616803948, -0.6046776061558809534, -0.2411417322834644161 ) ) ;
#35505=ORIENTED_EDGE ( 'NONE', *, *, #49907, .F. ) ;
#35507=CARTESIAN_POINT ( 'NONE',  ( 1.141732283464567788, -0.6692913385826771977, 8.415575281601705876E-17 ) ) ;
#35508=CARTESIAN_POINT ( 'NONE',  ( 0.4396325459317590445, -0.5511811023622046335, 0.09757992244046803654 ) ) ;
#35517=CARTESIAN_POINT ( 'NONE',  ( 0.9448818897637802916, -0.1870078740157479769, 0.4822834645669291653 ) ) ;
#35518=CARTESIAN_POINT ( 'NONE',  ( -0.9055118110236215490, -0.6692913385826771977, 8.415575281601705876E-17 ) ) ;
#35519=CARTESIAN_POINT ( 'NONE',  ( -0.6364829396325453192, -0.3162353388693405765, 0.4822834645669290543 ) ) ;
#35520=CARTESIAN_POINT ( 'NONE',  ( 0.5249343832021003964, 0.2306618581243847221, -0.2411417322834647770 ) ) ;
#35522=CARTESIAN_POINT ( 'NONE',  ( 1.246719160104987623, -0.4281496062992124485, 0.4176697321401328655 ) ) ;
#35523=CARTESIAN_POINT ( 'NONE',  ( -2.795275590551183686, 1.338582677165354395, -1.990688069879260956E-16 ) ) ;
#35524=CARTESIAN_POINT ( 'NONE',  ( 1.102362204724410155, -0.1870078740157480601, -0.3641732283464567677 ) ) ;
#35526=CARTESIAN_POINT ( 'NONE',  ( -1.286089238845143479, 0.1283753931104746893, -0.1820866141732285504 ) ) ;
#35528=CARTESIAN_POINT ( 'NONE',  ( 0.2755905511811031494, 0.2952755905511811885, 0.000000000000000000 ) ) ;
#35529=CARTESIAN_POINT ( 'NONE',  ( 1.686351706036745890, 0.2952755905511811885, 0.1292274648535926551 ) ) ;
#35530=CARTESIAN_POINT ( 'NONE',  ( -1.220472440944882386, -0.1870078740157480046, 1.254653134982923898E-17 ) ) ;
#35531=CARTESIAN_POINT ( 'NONE',  ( -1.082677165354329896, 0.07958543189024085140, 0.2665933059059887866 ) ) ;
#35532=CARTESIAN_POINT ( 'NONE',  ( 0.5708661417322842269, 0.1660481256975885056, 0.3530559997133364547 ) ) ;
#35533=CARTESIAN_POINT ( 'NONE',  ( 1.299212598425197429, 0.1771653543307087630, 0.000000000000000000 ) ) ;
#35535=CARTESIAN_POINT ( 'NONE',  ( -1.345144356955379816, -0.08942795157528024563, -0.3641732283464568787 ) ) ;
#35536=CARTESIAN_POINT ( 'NONE',  ( 1.227034120734908917, 0.2952755905511810774, -0.1292274648535930714 ) ) ;
#35538=CARTESIAN_POINT ( 'NONE',  ( 0.006561679790026889343, -0.05778040916215522460, 0.4822834645669289988 ) ) ;
#35539=CARTESIAN_POINT ( 'NONE',  ( -1.332020997375327642, -0.08942795157527998196, 0.3641732283464567121 ) ) ;
#35540=CARTESIAN_POINT ( 'NONE',  ( -0.5183727034120726440, -0.5511811023622048555, -0.09757992244046775898 ) ) ;
#35541=CARTESIAN_POINT ( 'NONE',  ( -0.8989501312335946848, 0.2952755905511810774, -0.1292274648535930714 ) ) ;
#35542=CARTESIAN_POINT ( 'NONE',  ( -1.601049868766403650, 0.1283753931104746893, -0.1820866141732285504 ) ) ;
#35544=CARTESIAN_POINT ( 'NONE',  ( 0.1443569553805781891, -0.4281496062992124485, 0.4176697321401328655 ) ) ;
#35545=FACE_OUTER_BOUND ( 'NONE', #29700, .T. ) ;
#35547=CARTESIAN_POINT ( 'NONE',  ( -1.220472440944881054, 0.2952755905511811885, 0.000000000000000000 ) ) ;
#35548=CARTESIAN_POINT ( 'NONE',  ( -0.6430446194225716283, -0.3690944881889763329, 0.3153832671262228327 ) ) ;
#35549=CARTESIAN_POINT ( 'NONE',  ( -1.646981627296586703, -0.05778040916215522460, 0.4822834645669289988 ) ) ;
#35550=CARTESIAN_POINT ( 'NONE',  ( 0.1640419947506569498, -0.3162353388693409650, -0.4822834645669289433 ) ) ;
#35551=CARTESIAN_POINT ( 'NONE',  ( 0.2362204724409456558, -0.1870078740157479769, 0.3641732283464567677 ) ) ;
#35552=CARTESIAN_POINT ( 'NONE',  ( -1.141732283464566011, -0.5511811023622047445, 6.969142054262312111E-17 ) ) ;
#35553=CARTESIAN_POINT ( 'NONE',  ( -1.489501312335957062, -0.3162353388693409650, -0.4822834645669289433 ) ) ;
#35554=CARTESIAN_POINT ( 'NONE',  ( -1.423884514435694859, -0.3162353388693405765, 0.4822834645669290543 ) ) ;
#35555=CARTESIAN_POINT ( 'NONE',  ( 1.555118110236221041, 0.1660481256975883668, -0.3530559997133364547 ) ) ;
#35557=CARTESIAN_POINT ( 'NONE',  ( 0.4593175853018380828, -0.004921259842519870586, -0.3153832671262229437 ) ) ;
#35559=CARTESIAN_POINT ( 'NONE',  ( 1.036745406824147731, 0.05413385826771666132, 0.4176697321401328100 ) ) ;
#35561=CARTESIAN_POINT ( 'NONE',  ( 1.391076115485564868, -0.5023911411419708095, 0.1820866141732285504 ) ) ;
#35563=CARTESIAN_POINT ( 'NONE',  ( -1.141732283464566011, 0.2952755905511811885, 0.000000000000000000 ) ) ;
#35565=CARTESIAN_POINT ( 'NONE',  ( -1.036745406824146176, -0.4281496062992124485, 0.4176697321401328655 ) ) ;
#35566=CARTESIAN_POINT ( 'NONE',  ( 0.3608923884514443348, 0.2952755905511810774, -0.1292274648535930714 ) ) ;
#35569=CARTESIAN_POINT ( 'NONE',  ( 0.9055118110236227702, -0.6692913385826771977, 8.415575281601705876E-17 ) ) ;
#35570=CARTESIAN_POINT ( 'NONE',  ( -1.679790026246718693, 0.2306618581243847221, -0.2411417322834647770 ) ) ;
#35571=CARTESIAN_POINT ( 'NONE',  ( 0.2624671916010504757, 0.2306618581243848609, 0.2411417322834645549 ) ) ;
#35572=CARTESIAN_POINT ( 'NONE',  ( 0.7611548556430451917, -0.6046776061558807314, 0.2411417322834647770 ) ) ;
#35574=AXIS2_PLACEMENT_3D ( 'NONE', #3515, #48528, #11070 ) ;
#35579=CARTESIAN_POINT ( 'NONE',  ( -0.1312335958005241554, 0.1283753931104748280, 0.1820866141732283561 ) ) ;
#35580=CARTESIAN_POINT ( 'NONE',  ( -0.4068241469816267775, 0.05413385826771626580, -0.4176697321401330321 ) ) ;
#35581=CARTESIAN_POINT ( 'NONE',  ( 0.8136482939632553313, 0.2306618581243848609, 0.2411417322834645549 ) ) ;
#35583=CARTESIAN_POINT ( 'NONE',  ( -0.1509186351706028884, -0.2845877964562161244, -0.3641732283464567121 ) ) ;
#35584=CARTESIAN_POINT ( 'NONE',  ( -1.200787401574802349, -0.5400638737290844871, 0.3530559997133364547 ) ) ;
#35585=CARTESIAN_POINT ( 'NONE',  ( 1.017060367454068581, -0.05778040916215560624, -0.4822834645669293319 ) ) ;
#35588=FACE_OUTER_BOUND ( 'NONE', #70999, .T. ) ;
#35589=VERTEX_POINT ( 'NONE', #73011 ) ;
#35590=CARTESIAN_POINT ( 'NONE',  ( 0.8070866141732288002, 0.1660481256975885056, 0.3530559997133364547 ) ) ;
#35591=CARTESIAN_POINT ( 'NONE',  ( 1.351706036745407458, -0.3690944881889765550, -0.3153832671262227771 ) ) ;
#35592=CARTESIAN_POINT ( 'NONE',  ( 1.541994750656168645, 0.2952755905511810774, -0.1292274648535930714 ) ) ;
#35593=CARTESIAN_POINT ( 'NONE',  ( 1.574803149606299746, -0.1870078740157479769, 0.4822834645669291653 ) ) ;
#35595=CARTESIAN_POINT ( 'NONE',  ( -1.220472440944882386, -3.283890673957456492E-15, 0.4445507791589070057 ) ) ;
#35596=CARTESIAN_POINT ( 'NONE',  ( 1.279527559055118724, -0.5400638737290845981, -0.3530559997133363437 ) ) ;
#35598=CARTESIAN_POINT ( 'NONE',  ( 0.07217847769028949700, -0.05778040916215560624, -0.4822834645669293319 ) ) ;
#35599=CARTESIAN_POINT ( 'NONE',  ( -0.7677165354330699465, 0.1660481256975885056, 0.3530559997133364547 ) ) ;
#35601=CARTESIAN_POINT ( 'NONE',  ( 1.443569553805774897, 0.2306618581243848609, 0.2411417322834645549 ) ) ;
#35603=CARTESIAN_POINT ( 'NONE',  ( 0.02624671916010564918, 0.2306618581243848609, 0.2411417322834645549 ) ) ;
#35605=CARTESIAN_POINT ( 'NONE',  ( -1.548556430446193399, -0.5023911411419708095, -0.1820866141732282451 ) ) ;
#35608=EDGE_LOOP ( 'NONE', ( #64333, #70059, #77927, #44046 ) ) ;
#35610=CARTESIAN_POINT ( 'NONE',  ( -1.692913385826770645, 0.2952755905511811885, 0.000000000000000000 ) ) ;
#35614=CARTESIAN_POINT ( 'NONE',  ( -0.9548908091195642545, -2.567464376874931580E-15, -0.4445507791589072832 ) ) ;
#35617=CARTESIAN_POINT ( 'NONE',  ( -0.1771653543307080136, 0.07958543189024071263, -0.2665933059059888421 ) ) ;
#35618=CARTESIAN_POINT ( 'NONE',  ( -0.9383202099737524282, -0.08942795157527998196, 0.3641732283464567121 ) ) ;
#35620=CARTESIAN_POINT ( 'NONE',  ( -1.292650918635170010, 0.2952755905511810774, -0.1292274648535930714 ) ) ;
#35621=CARTESIAN_POINT ( 'NONE',  ( 0.6692913385826777528, 0.2952755905511811885, 0.000000000000000000 ) ) ;
#35622=CARTESIAN_POINT ( 'NONE',  ( -1.207349081364828436, -0.6046776061558807314, 0.2411417322834647770 ) ) ;
#35625=CARTESIAN_POINT ( 'NONE',  ( -1.292650918635170010, 0.2952755905511810774, -0.1292274648535930714 ) ) ;
#35626=CARTESIAN_POINT ( 'NONE',  ( 1.220472440944881942, 2.401574803149606474, -0.5309055118110238558 ) ) ;
#35633=CARTESIAN_POINT ( 'NONE',  ( -0.8727034120734901146, -0.3162353388693405765, 0.4822834645669290543 ) ) ;
#35634=CARTESIAN_POINT ( 'NONE',  ( 1.574803149606299746, -0.1870078740157480879, -0.4822834645669291653 ) ) ;
#35635=CARTESIAN_POINT ( 'NONE',  ( -1.692913385826770645, 0.2952755905511811885, 0.000000000000000000 ) ) ;
#35636=CARTESIAN_POINT ( 'NONE',  ( -1.614173228346457378, 1.606230626554505658, -0.1372047244094477536 ) ) ;
#35637=CARTESIAN_POINT ( 'NONE',  ( 1.528871391076116026, 0.2952755905511811885, 0.1292274648535926551 ) ) ;
#35638=CARTESIAN_POINT ( 'NONE',  ( -0.6167979002624665030, 0.05413385826771666132, 0.4176697321401328100 ) ) ;
#35641=CARTESIAN_POINT ( 'NONE',  ( -0.05905511811023545637, -0.4536011799217368745, -0.2665933059059886201 ) ) ;
#35643=CARTESIAN_POINT ( 'NONE',  ( -0.1049868766404193215, -0.5023911411419708095, 0.1820866141732285504 ) ) ;
#35644=CARTESIAN_POINT ( 'NONE',  ( 1.089238845144357537, -0.3690944881889763329, 0.3153832671262228327 ) ) ;
#35645=CARTESIAN_POINT ( 'NONE',  ( 0.3937007874015754361, -0.1870078740157480879, -0.4822834645669291653 ) ) ;
#35646=CARTESIAN_POINT ( 'NONE',  ( -0.1312335958005241554, -0.5023911411419708095, -0.1820866141732282451 ) ) ;
#35648=CARTESIAN_POINT ( 'NONE',  ( -1.502624671916009680, -0.3162353388693405765, 0.4822834645669290543 ) ) ;
#35649=CARTESIAN_POINT ( 'NONE',  ( -1.266404199475064773, -0.08942795157528024563, -0.3641732283464568787 ) ) ;
#35651=CARTESIAN_POINT ( 'NONE',  ( 0.06561679790026316017, 0.05413385826771626580, -0.4176697321401330321 ) ) ;
#35652=CARTESIAN_POINT ( 'NONE',  ( -0.4068241469816264999, -0.4281496062992124485, 0.4176697321401328655 ) ) ;
#35653=CARTESIAN_POINT ( 'NONE',  ( 0.01000891935578606708, -2.191421614605370878E-15, 0.4445507791589071167 ) ) ;
#35654=CARTESIAN_POINT ( 'NONE',  ( 0.5183727034120741983, 0.1771653543307087075, -0.09757992244046823083 ) ) ;
#35655=CARTESIAN_POINT ( 'NONE',  ( -0.2427821522309703550, -0.05778040916215560624, -0.4822834645669293319 ) ) ;
#35656=CARTESIAN_POINT ( 'NONE',  ( -0.5839895013123351797, -0.6692913385826771977, 0.1292274648535927661 ) ) ;
#35659=CARTESIAN_POINT ( 'NONE',  ( -0.04593175853018302557, 0.2952755905511811885, 0.1292274648535926551 ) ) ;
#35661=CARTESIAN_POINT ( 'NONE',  ( 1.581364829396326277, -0.05778040916215522460, 0.4822834645669289988 ) ) ;
#35662=CARTESIAN_POINT ( 'NONE',  ( -0.1181102362204717315, 0.1771653543307087630, 0.000000000000000000 ) ) ;
#35663=CARTESIAN_POINT ( 'NONE',  ( -0.3805774278215216522, -0.4281496062992127816, -0.4176697321401328100 ) ) ;
#35664=CARTESIAN_POINT ( 'NONE',  ( -1.450131233595799651, 0.1771653543307087075, -0.09757992244046823083 ) ) ;
#35665=CARTESIAN_POINT ( 'NONE',  ( 1.194225721784777594, 0.05413385826771666132, 0.4176697321401328100 ) ) ;
#35666=CARTESIAN_POINT ( 'NONE',  ( -1.443569553805773564, 0.2306618581243847221, -0.2411417322834647770 ) ) ;
#35667=CARTESIAN_POINT ( 'NONE',  ( -0.7349081364829390672, 0.1283753931104746893, -0.1820866141732285504 ) ) ;
#35671=CARTESIAN_POINT ( 'NONE',  ( 1.410761154855643795, -0.08942795157528024563, -0.3641732283464568787 ) ) ;
#35672=CARTESIAN_POINT ( 'NONE',  ( 1.305774278215223960, 0.1771653543307087075, -0.09757992244046823083 ) ) ;
#35673=CARTESIAN_POINT ( 'NONE',  ( 0.8989501312335963501, -0.6692913385826773087, -0.1292274648535924053 ) ) ;
#35674=CARTESIAN_POINT ( 'NONE',  ( 0.4396325459317593221, 0.2066929133858267098, -0.1054918080437494132 ) ) ;
#35675=CARTESIAN_POINT ( 'NONE',  ( 0.9514435695538062676, -0.05778040916215522460, 0.4822834645669289988 ) ) ;
#35677=CARTESIAN_POINT ( 'NONE',  ( 1.266404199475066328, -0.2845877964562161244, -0.3641732283464567121 ) ) ;
#35678=CARTESIAN_POINT ( 'NONE',  ( 0.2493438320209980519, 0.05413385826771666132, 0.4176697321401328100 ) ) ;
#35679=CARTESIAN_POINT ( 'NONE',  ( -0.6102362204724400829, -0.5400638737290845981, -0.3530559997133363437 ) ) ;
#35680=CARTESIAN_POINT ( 'NONE',  ( 1.561679790026247350, 0.05413385826771626580, -0.4176697321401330321 ) ) ;
#35684=CARTESIAN_POINT ( 'NONE',  ( 0.4790026246719167324, -0.08942795157527998196, 0.3641732283464567121 ) ) ;
#35688=CARTESIAN_POINT ( 'NONE',  ( -0.4724409448818890911, -0.1870078740157479769, 0.4822834645669291653 ) ) ;
#35689=CARTESIAN_POINT ( 'NONE',  ( -0.1115485564304453947, -0.6692913385826771977, 0.1292274648535927661 ) ) ;
#35690=CARTESIAN_POINT ( 'NONE',  ( -0.4724409448818890911, -0.1870078740157480879, -0.4822834645669291653 ) ) ;
#35691=CARTESIAN_POINT ( 'NONE',  ( 0.6233595800524942554, -0.05778040916215560624, -0.4822834645669293319 ) ) ;
#35692=CARTESIAN_POINT ( 'NONE',  ( -0.8005249343832011588, 0.05413385826771626580, -0.4176697321401330321 ) ) ;
#35693=CARTESIAN_POINT ( 'NONE',  ( -0.4199475065616791736, 0.2306618581243847221, -0.2411417322834647770 ) ) ;
#35694=CARTESIAN_POINT ( 'NONE',  ( 1.043307086614173818, -0.5400638737290845981, -0.3530559997133363437 ) ) ;
#35695=CARTESIAN_POINT ( 'NONE',  ( 0.4790026246719167324, -0.05778040916215522460, 0.4822834645669289988 ) ) ;
#35696=CARTESIAN_POINT ( 'NONE',  ( 0.6824146981627303710, -0.6046776061558807314, 0.2411417322834647770 ) ) ;
#35698=CARTESIAN_POINT ( 'NONE',  ( -0.09842519685039295696, -0.4536011799217367080, 0.2665933059059888421 ) ) ;
#35699=ORIENTED_EDGE ( 'NONE', *, *, #40855, .F. ) ;
#35702=CARTESIAN_POINT ( 'NONE',  ( -0.6561679790026240244, -0.5023911411419708095, 0.1820866141732285504 ) ) ;
#35703=CARTESIAN_POINT ( 'NONE',  ( -0.5183727034120726440, 0.2952755905511811885, 0.1292274648535926551 ) ) ;
#35705=CARTESIAN_POINT ( 'NONE',  ( -0.8333333333333323711, -0.6692913385826773087, -0.1292274648535924053 ) ) ;
#35706=CARTESIAN_POINT ( 'NONE',  ( -0.3412073490813641308, -0.6046776061558807314, 0.2411417322834647770 ) ) ;
#35707=CARTESIAN_POINT ( 'NONE',  ( -1.115485564304461219, 0.05413385826771626580, -0.4176697321401330321 ) ) ;
#35708=CARTESIAN_POINT ( 'NONE',  ( -1.476377952755905110, -0.5400638737290845981, -0.3530559997133363437 ) ) ;
#35709=CARTESIAN_POINT ( 'NONE',  ( 0.8202099737532814183, -0.5511811023622048555, -0.09757992244046775898 ) ) ;
#35712=CARTESIAN_POINT ( 'NONE',  ( 0.4068241469816279987, -0.3690944881889765550, -0.3153832671262227771 ) ) ;
#35713=CARTESIAN_POINT ( 'NONE',  ( -0.1574803149606292529, -0.1870078740157480879, -0.4822834645669291653 ) ) ;
#35714=CARTESIAN_POINT ( 'NONE',  ( -0.1968503937007867743, 0.2952755905511811885, 0.000000000000000000 ) ) ;
#35721=CARTESIAN_POINT ( 'NONE',  ( -0.8989501312335946848, 0.1771653543307087075, -0.09757992244046823083 ) ) ;
#35722=CARTESIAN_POINT ( 'NONE',  ( -0.9251968503937002541, 0.1660481256975885056, 0.3530559997133364547 ) ) ;
#35725=CARTESIAN_POINT ( 'NONE',  ( 1.686351706036745890, 0.2952755905511811885, 0.1292274648535926551 ) ) ;
#35726=CARTESIAN_POINT ( 'NONE',  ( 0.3608923884514443348, 0.2952755905511810774, -0.1292274648535930714 ) ) ;
#35727=CARTESIAN_POINT ( 'NONE',  ( 0.5839895013123367340, 0.2952755905511811885, 0.1292274648535926551 ) ) ;
#35728=CARTESIAN_POINT ( 'NONE',  ( -0.7283464566929126471, -0.4536011799217367080, 0.2665933059059888421 ) ) ;
#35729=CARTESIAN_POINT ( 'NONE',  ( 0.08530183727034192087, -0.3162353388693409650, -0.4822834645669289433 ) ) ;
#35731=CARTESIAN_POINT ( 'NONE',  ( -0.5577427821522301654, -0.2845877964562159024, 0.3641732283464567677 ) ) ;
#35733=CARTESIAN_POINT ( 'NONE',  ( -0.5511811023622041894, -0.1870078740157480879, -0.4822834645669291653 ) ) ;
#35735=CARTESIAN_POINT ( 'NONE',  ( 1.122047244094488860, 0.07958543189024085140, 0.2665933059059887866 ) ) ;
#35736=CARTESIAN_POINT ( 'NONE',  ( 0.03937007874015806264, 0.1771653543307087630, 0.000000000000000000 ) ) ;
#35737=CARTESIAN_POINT ( 'NONE',  ( 1.279527559055118724, -0.4536011799217368745, -0.2665933059059886201 ) ) ;
#35738=CARTESIAN_POINT ( 'NONE',  ( -1.332020997375327642, -0.3162353388693409650, -0.4822834645669289433 ) ) ;
#35739=CARTESIAN_POINT ( 'NONE',  ( -0.9317585301837263412, -0.3690944881889765550, -0.3153832671262227771 ) ) ;
#35740=CARTESIAN_POINT ( 'NONE',  ( 1.586688153636164111, 1.522296263979924902, -0.1275903502784764554 ) ) ;
#35741=CARTESIAN_POINT ( 'NONE',  ( -1.108923884514435132, -0.3162353388693405765, 0.4822834645669290543 ) ) ;
#35742=CARTESIAN_POINT ( 'NONE',  ( -0.5905511811023613777, -0.6692913385826771977, 8.415575281601705876E-17 ) ) ;
#35743=CARTESIAN_POINT ( 'NONE',  ( 0.5052493438320218022, -0.6692913385826773087, -0.1292274648535924053 ) ) ;
#35747=CARTESIAN_POINT ( 'NONE',  ( 0.1640419947506569498, -0.2845877964562161244, -0.3641732283464567121 ) ) ;
#35748=CARTESIAN_POINT ( 'NONE',  ( 0.8923884514435701520, -0.6046776061558809534, -0.2411417322834644161 ) ) ;
#35749=CARTESIAN_POINT ( 'NONE',  ( -1.318897637795274802, -0.4536011799217368745, -0.2665933059059886201 ) ) ;
#35751=CARTESIAN_POINT ( 'NONE',  ( 1.036745406824147731, 0.05413385826771666132, 0.4176697321401328100 ) ) ;
#35752=CARTESIAN_POINT ( 'NONE',  ( -1.555118110236219930, 0.07958543189024085140, 0.2665933059059887866 ) ) ;
#35753=CARTESIAN_POINT ( 'NONE',  ( -1.371391076115484831, 0.2952755905511810774, -0.1292274648535930714 ) ) ;
#35754=CARTESIAN_POINT ( 'NONE',  ( -1.010498687664041384, -0.4281496062992127816, -0.4176697321401328100 ) ) ;
#35755=CARTESIAN_POINT ( 'NONE',  ( 0.02624671916010564918, -0.5023911411419708095, -0.1820866141732282451 ) ) ;
#35757=CARTESIAN_POINT ( 'NONE',  ( 0.8464566929133865436, 0.07958543189024071263, -0.2665933059059888421 ) ) ;
#35759=CARTESIAN_POINT ( 'NONE',  ( -0.2427821522309703550, -0.3162353388693405765, 0.4822834645669290543 ) ) ;
#35761=CARTESIAN_POINT ( 'NONE',  ( -1.108923884514435132, -0.3162353388693405765, 0.4822834645669290543 ) ) ;
#35763=CARTESIAN_POINT ( 'NONE',  ( 0.9251968503937015864, -0.4536011799217367080, 0.2665933059059888421 ) ) ;
#35764=CARTESIAN_POINT ( 'NONE',  ( -0.1377952755905504645, -0.5400638737290845981, -0.3530559997133363437 ) ) ;
#35765=CARTESIAN_POINT ( 'NONE',  ( -0.1377952755905504645, -0.5400638737290845981, -0.3530559997133363437 ) ) ;
#35766=CARTESIAN_POINT ( 'NONE',  ( -0.5314960629921250401, 0.07958543189024085140, 0.2665933059059887866 ) ) ;
#35768=CARTESIAN_POINT ( 'NONE',  ( -0.4855643044619415427, -0.004921259842519870586, -0.3153832671262229437 ) ) ;
#35769=CARTESIAN_POINT ( 'NONE',  ( 0.5052493438320218022, -0.6692913385826773087, -0.1292274648535924053 ) ) ;
#35770=CARTESIAN_POINT ( 'NONE',  ( -1.253280839895012377, -0.08942795157527998196, 0.3641732283464567121 ) ) ;
#35772=CARTESIAN_POINT ( 'NONE',  ( 1.587926509186352142, 0.05413385826771666132, 0.4176697321401328100 ) ) ;
#35775=CARTESIAN_POINT ( 'NONE',  ( -1.410761154855642463, -0.08942795157527998196, 0.3641732283464567121 ) ) ;
#35776=CARTESIAN_POINT ( 'NONE',  ( -0.5118110236220466680, -0.6692913385826771977, 8.415575281601705876E-17 ) ) ;
#35778=CARTESIAN_POINT ( 'NONE',  ( -1.305774278215222184, 0.2952755905511811885, 0.1292274648535926551 ) ) ;
#35781=CARTESIAN_POINT ( 'NONE',  ( 1.266404199475066328, -0.3162353388693409650, -0.4822834645669289433 ) ) ;
#35782=CARTESIAN_POINT ( 'NONE',  ( 0.2887139107611556010, 0.2306618581243847221, -0.2411417322834647770 ) ) ;
#35787=CARTESIAN_POINT ( 'NONE',  ( 1.587926509186352142, -0.004921259842519576551, 0.3153832671262227771 ) ) ;
#35791=CARTESIAN_POINT ( 'NONE',  ( -0.8333333333333323711, 0.1771653543307087630, 0.09757992244046791164 ) ) ;
#35794=CARTESIAN_POINT ( 'NONE',  ( 0.8989501312335963501, -0.6692913385826773087, -0.1292274648535924053 ) ) ;
#35795=CARTESIAN_POINT ( 'NONE',  ( -0.5249343832020990641, -0.6046776061558809534, -0.2411417322834644161 ) ) ;
#35796=CARTESIAN_POINT ( 'NONE',  ( -1.266404199475064773, -0.05778040916215560624, -0.4822834645669293319 ) ) ;
#35797=CARTESIAN_POINT ( 'NONE',  ( 1.082677165354331228, 0.1660481256975883668, -0.3530559997133364547 ) ) ;
#35798=CARTESIAN_POINT ( 'NONE',  ( -1.154855643044618851, 0.1283753931104748280, 0.1820866141732283561 ) ) ;
#35800=CARTESIAN_POINT ( 'NONE',  ( 0.2690288713910767848, 0.2952755905511811885, 0.1292274648535926551 ) ) ;
#35801=CARTESIAN_POINT ( 'NONE',  ( -0.6758530183727028406, 0.2952755905511811885, 0.1292274648535926551 ) ) ;
#35803=CARTESIAN_POINT ( 'NONE',  ( -1.049868766404198794, -0.6046776061558807314, 0.2411417322834647770 ) ) ;
#35805=EDGE_CURVE ( 'NONE', #69360, #83014, #18657, .T. ) ;
#35806=CARTESIAN_POINT ( 'NONE',  ( 1.102362204724410155, -0.1870078740157480879, -0.4822834645669291653 ) ) ;
#35808=CARTESIAN_POINT ( 'NONE',  ( 1.253280839895013710, -0.08942795157528024563, -0.3641732283464568787 ) ) ;
#35811=CARTESIAN_POINT ( 'NONE',  ( -0.3543307086614165824, 0.2952755905511811885, 0.000000000000000000 ) ) ;
#35813=CARTESIAN_POINT ( 'NONE',  ( 0.3543307086614179147, 0.1771653543307087630, 0.000000000000000000 ) ) ;
#35815=CARTESIAN_POINT ( 'NONE',  ( -1.614173228346456268, -0.6692913385826771977, 8.415575281601705876E-17 ) ) ;
#35816=CARTESIAN_POINT ( 'NONE',  ( 0.6889763779527563470, 0.1660481256975883668, -0.3530559997133364547 ) ) ;
#35817=CARTESIAN_POINT ( 'NONE',  ( 0.8923884514435701520, -0.6046776061558809534, -0.2411417322834644161 ) ) ;
#35818=CARTESIAN_POINT ( 'NONE',  ( -0.08530183727034056085, -0.05778040916215560624, -0.4822834645669293319 ) ) ;
#35820=CARTESIAN_POINT ( 'NONE',  ( -0.9120734908136475250, -0.6692913385826773087, -0.1292274648535924053 ) ) ;
#35822=CARTESIAN_POINT ( 'NONE',  ( -1.712598425196849572, 0.1660481256975885056, 0.3530559997133364547 ) ) ;
#35823=CARTESIAN_POINT ( 'NONE',  ( -1.095800524934382292, -0.3162353388693409650, -0.4822834645669289433 ) ) ;
#35824=CARTESIAN_POINT ( 'NONE',  ( 1.233595800524935227, 0.2306618581243847221, -0.2411417322834647770 ) ) ;
#35825=CARTESIAN_POINT ( 'NONE',  ( 1.601049868766404982, -0.6046776061558809534, -0.2411417322834644161 ) ) ;
#35827=CARTESIAN_POINT ( 'NONE',  ( -1.017060367454067249, -0.3162353388693409650, -0.4822834645669289433 ) ) ;
#35829=CARTESIAN_POINT ( 'NONE',  ( 0.1246719160104994284, -0.6692913385826771977, 0.1292274648535927661 ) ) ;
#35831=CARTESIAN_POINT ( 'NONE',  ( -0.5643044619422565855, -0.4281496062992124485, 0.4176697321401328655 ) ) ;
#35832=CARTESIAN_POINT ( 'NONE',  ( -1.594488188976377119, 0.07958543189024071263, -0.2665933059059888421 ) ) ;
#35833=CARTESIAN_POINT ( 'NONE',  ( 0.7414698162729663755, 0.1771653543307087630, 0.09757992244046791164 ) ) ;
#35834=CARTESIAN_POINT ( 'NONE',  ( 1.279527559055118724, 0.1660481256975885056, 0.3530559997133364547 ) ) ;
#35836=CARTESIAN_POINT ( 'NONE',  ( 0.7939632545931766261, -0.2845877964562161244, -0.3641732283464567121 ) ) ;
#35837=CARTESIAN_POINT ( 'NONE',  ( 0.6627296587926515548, 0.2952755905511811885, 0.1292274648535926551 ) ) ;
#35839=CARTESIAN_POINT ( 'NONE',  ( -0.4658792650918627265, -0.05778040916215522460, 0.4822834645669289988 ) ) ;
#35841=CARTESIAN_POINT ( 'NONE',  ( 1.325459317585302665, -0.004921259842519870586, -0.3153832671262229437 ) ) ;
#35842=CARTESIAN_POINT ( 'NONE',  ( -0.5708661417322828946, 0.1660481256975883668, -0.3530559997133364547 ) ) ;
#35843=CARTESIAN_POINT ( 'NONE',  ( 0.1574803149606306130, -0.1870078740157479769, 0.4822834645669291653 ) ) ;
#35844=CARTESIAN_POINT ( 'NONE',  ( 0.09151288181857175630, 0.004960608223780119466, 0.3437734562760182411 ) ) ;
#35845=CARTESIAN_POINT ( 'NONE',  ( -0.03280839895013062252, -0.6692913385826771977, 0.1292274648535927661 ) ) ;
#35846=CARTESIAN_POINT ( 'NONE',  ( 0.6430446194225729606, -0.3690944881889765550, -0.3153832671262227771 ) ) ;
#35848=CARTESIAN_POINT ( 'NONE',  ( -0.09186351706036663400, -0.3690944881889763329, 0.3153832671262228327 ) ) ;
#35849=CARTESIAN_POINT ( 'NONE',  ( 0.9317585301837276734, -0.3690944881889763329, 0.3153832671262228327 ) ) ;
#35850=CARTESIAN_POINT ( 'NONE',  ( -1.082677165354329896, 0.1012011053420777407, 0.2882089793578257453 ) ) ;
#35852=CARTESIAN_POINT ( 'NONE',  ( 0.7152230971128616943, -0.05778040916215522460, 0.4822834645669289988 ) ) ;
#35853=AXIS2_PLACEMENT_3D ( 'NONE', #19050, #22996, #49073 ) ;
#35857=CARTESIAN_POINT ( 'NONE',  ( 0.2258813529811906362, 4.257495641787552160E-16, -0.4281993546915526805 ) ) ;
#35859=CARTESIAN_POINT ( 'NONE',  ( -0.09186351706036689768, -0.004921259842519870586, -0.3153832671262229437 ) ) ;
#35861=CARTESIAN_POINT ( 'NONE',  ( 0.1443569553805781891, 0.05413385826771626580, -0.4176697321401330321 ) ) ;
#35862=CARTESIAN_POINT ( 'NONE',  ( 1.397637795275591177, 0.07958543189024071263, -0.2665933059059888421 ) ) ;
#35863=CARTESIAN_POINT ( 'NONE',  ( -1.174540682414697335, -0.2845877964562161244, -0.3641732283464567121 ) ) ;
#35864=CARTESIAN_POINT ( 'NONE',  ( -1.318897637795274802, -0.5400638737290845981, -0.3530559997133363437 ) ) ;
#35865=CARTESIAN_POINT ( 'NONE',  ( 0.2887139107611556010, 0.2306618581243847221, -0.2411417322834647770 ) ) ;
#35866=CARTESIAN_POINT ( 'NONE',  ( 1.003937007874016407, -0.5400638737290844871, 0.3530559997133364547 ) ) ;
#35867=CARTESIAN_POINT ( 'NONE',  ( 1.251578178566641997, 1.420967098491911607, -0.6060014054450971743 ) ) ;
#35868=CARTESIAN_POINT ( 'NONE',  ( 0.1443569553805781891, -0.4281496062992124485, 0.4176697321401328655 ) ) ;
#35869=CARTESIAN_POINT ( 'NONE',  ( 1.450131233595801428, -0.6692913385826773087, -0.1292274648535924053 ) ) ;
#35870=CARTESIAN_POINT ( 'NONE',  ( 1.062992125984252745, 0.2952755905511811885, 0.000000000000000000 ) ) ;
#35871=CARTESIAN_POINT ( 'NONE',  ( -1.604771003085129433, 2.146987379487327985, -0.1466069496707750608 ) ) ;
#35872=CARTESIAN_POINT ( 'NONE',  ( 0.7283464566929143125, 0.07958543189024085140, 0.2665933059059887866 ) ) ;
#35873=CARTESIAN_POINT ( 'NONE',  ( 1.614173228346457378, -0.6692913385826771977, 8.415575281601705876E-17 ) ) ;
#35874=CARTESIAN_POINT ( 'NONE',  ( 0.06561679790026316017, -0.004921259842519870586, -0.3153832671262229437 ) ) ;
#35875=CARTESIAN_POINT ( 'NONE',  ( 0.1246719160104994284, 0.2952755905511810774, -0.1292274648535930714 ) ) ;
#35876=CARTESIAN_POINT ( 'NONE',  ( 0.8727034120734912248, -0.3162353388693409650, -0.4822834645669289433 ) ) ;
#35877=CARTESIAN_POINT ( 'NONE',  ( -0.4396325459317577122, -0.6692913385826773087, -0.1292274648535924053 ) ) ;
#35878=CARTESIAN_POINT ( 'NONE',  ( -0.4002624671916004129, -0.08942795157528024563, -0.3641732283464568787 ) ) ;
#35879=CARTESIAN_POINT ( 'NONE',  ( 0.8398950131233602345, 0.2306618581243847221, -0.2411417322834647770 ) ) ;
#35880=CARTESIAN_POINT ( 'NONE',  ( 1.036745406824147731, -0.004921259842519576551, 0.3153832671262227771 ) ) ;
#35881=CYLINDRICAL_SURFACE ( 'NONE', #60811, 1.181102362204724310 ) ;
#35885=CARTESIAN_POINT ( 'NONE',  ( -1.154855643044618851, 0.2306618581243848609, 0.2411417322834645549 ) ) ;
#35886=CARTESIAN_POINT ( 'NONE',  ( -0.4658792650918627265, -0.05778040916215522460, 0.4822834645669289988 ) ) ;
#35889=ORIENTED_EDGE ( 'NONE', *, *, #75955, .T. ) ;
#35890=CARTESIAN_POINT ( 'NONE',  ( 0.1377952755905518800, 0.07958543189024071263, -0.2665933059059888421 ) ) ;
#35892=CARTESIAN_POINT ( 'NONE',  ( 0.9055118110236227702, -0.6692913385826771977, 8.415575281601705876E-17 ) ) ;
#35896=CARTESIAN_POINT ( 'NONE',  ( 1.476377952755906442, -0.5400638737290844871, 0.3530559997133364547 ) ) ;
#35897=CARTESIAN_POINT ( 'NONE',  ( 1.469816272965879911, 0.1283753931104746893, -0.1820866141732285504 ) ) ;
#35898=CARTESIAN_POINT ( 'NONE',  ( 0.4002624671916016896, -0.05778040916215522460, 0.4822834645669289988 ) ) ;
#35901=CARTESIAN_POINT ( 'NONE',  ( 0.02624671916010564918, -0.6046776061558809534, -0.2411417322834644161 ) ) ;
#35902=CARTESIAN_POINT ( 'NONE',  ( -1.069553805774277722, 0.1771653543307087630, 0.09757992244046791164 ) ) ;
#35903=CARTESIAN_POINT ( 'NONE',  ( 0.2952755905511816326, -0.5400638737290844871, 0.3530559997133364547 ) ) ;
#35904=CARTESIAN_POINT ( 'NONE',  ( 0.006561679790026889343, -0.05778040916215522460, 0.4822834645669289988 ) ) ;
#35906=CARTESIAN_POINT ( 'NONE',  ( 0.4855643044619428750, 0.05413385826771666132, 0.4176697321401328100 ) ) ;
#35910=CARTESIAN_POINT ( 'NONE',  ( 0.7414698162729663755, 0.2952755905511811885, 0.1292274648535926551 ) ) ;
#35912=CARTESIAN_POINT ( 'NONE',  ( -0.2493438320209966919, 0.05413385826771626580, -0.4176697321401330321 ) ) ;
#35913=CARTESIAN_POINT ( 'NONE',  ( -1.148293963254592542, 0.2952755905511811885, 0.1292274648535926551 ) ) ;
#35914=CARTESIAN_POINT ( 'NONE',  ( 1.062992125984252745, -0.6692913385826771977, 8.415575281601705876E-17 ) ) ;
#35915=CARTESIAN_POINT ( 'NONE',  ( 0.5905511811023629321, 0.2952755905511811885, 0.000000000000000000 ) ) ;
#35917=CARTESIAN_POINT ( 'NONE',  ( -0.5511811023622041894, -0.1870078740157480879, -0.4822834645669291653 ) ) ;
#35918=CARTESIAN_POINT ( 'NONE',  ( 0.3412073490813655186, -0.6046776061558809534, -0.2411417322834644161 ) ) ;
#35919=CARTESIAN_POINT ( 'NONE',  ( -0.5446194225721777693, -0.05778040916215522460, 0.4822834645669289988 ) ) ;
#35920=CARTESIAN_POINT ( 'NONE',  ( 0.3477690288713918276, -0.5511811023622048555, -0.09757992244046775898 ) ) ;
#35921=CARTESIAN_POINT ( 'NONE',  ( -1.594488188976377563, -0.5400638737290844871, 0.3530559997133364547 ) ) ;
#35922=CARTESIAN_POINT ( 'NONE',  ( -1.719160104986876103, 0.05413385826771666132, 0.4176697321401328100 ) ) ;
#35923=CARTESIAN_POINT ( 'NONE',  ( 0.3149606299212603933, -0.1870078740157479769, 0.4822834645669291653 ) ) ;
#35924=CARTESIAN_POINT ( 'NONE',  ( 1.384514435695538337, -0.6692913385826771977, 0.1292274648535927661 ) ) ;
#35928=CARTESIAN_POINT ( 'NONE',  ( 0.7283464566929143125, 0.1660481256975885056, 0.3530559997133364547 ) ) ;
#35929=CARTESIAN_POINT ( 'NONE',  ( 0.7480314960629927956, -0.5511811023622047445, 6.969142054262312111E-17 ) ) ;
#35931=DIRECTION ( 'NONE',  ( 1.000000000000000000, 3.469446951953613203E-16, 0.000000000000000000 ) ) ;
#35933=CARTESIAN_POINT ( 'NONE',  ( 0.4606732211678803424, 1.778019097314518016, -0.5309055118110237448 ) ) ;
#35936=CARTESIAN_POINT ( 'NONE',  ( 0.8136482939632553313, 0.2306618581243848609, 0.2411417322834645549 ) ) ;
#35937=CARTESIAN_POINT ( 'NONE',  ( -0.8595800524934373854, -0.05778040916215522460, 0.4822834645669289988 ) ) ;
#35938=CARTESIAN_POINT ( 'NONE',  ( -0.5905511811023615998, 0.2952755905511811885, 0.000000000000000000 ) ) ;
#35939=CARTESIAN_POINT ( 'NONE',  ( 0.7677165354330716118, -0.5400638737290844871, 0.3530559997133364547 ) ) ;
#35940=CARTESIAN_POINT ( 'NONE',  ( 1.345144356955381593, -0.3162353388693409650, -0.4822834645669289433 ) ) ;
#35942=CARTESIAN_POINT ( 'NONE',  ( 1.443569553805774897, -0.5023911411419708095, -0.1820866141732282451 ) ) ;
#35943=CARTESIAN_POINT ( 'NONE',  ( 1.614173228346456712, 2.401574803149606474, -0.1372047244094476703 ) ) ;
#35944=CARTESIAN_POINT ( 'NONE',  ( -1.325459317585300889, -0.004921259842519576551, 0.3153832671262227771 ) ) ;
#35945=CARTESIAN_POINT ( 'NONE',  ( -2.787279214012418738, 2.362204724409448620, 0.000000000000000000 ) ) ;
#35946=CARTESIAN_POINT ( 'NONE',  ( 0.05905511811023709395, -0.5400638737290844871, 0.3530559997133364547 ) ) ;
#35947=CARTESIAN_POINT ( 'NONE',  ( 1.174540682414699111, -0.3162353388693405765, 0.4822834645669290543 ) ) ;
#35949=CARTESIAN_POINT ( 'NONE',  ( -1.167979002624671470, -0.3690944881889765550, -0.3153832671262227771 ) ) ;
#35950=CARTESIAN_POINT ( 'NONE',  ( 0.3805774278215230400, -0.4281496062992124485, 0.4176697321401328655 ) ) ;
#35951=CARTESIAN_POINT ( 'NONE',  ( 1.174540682414699111, -0.08942795157528024563, -0.3641732283464568787 ) ) ;
#35952=EDGE_CURVE ( 'NONE', #41264, #66355, #18911, .T. ) ;
#35954=CARTESIAN_POINT ( 'NONE',  ( -1.043307086614172707, 0.07958543189024071263, -0.2665933059059888421 ) ) ;
#35955=CARTESIAN_POINT ( 'NONE',  ( 1.450131233595801428, -0.6692913385826773087, -0.1292274648535924053 ) ) ;
#35957=CARTESIAN_POINT ( 'NONE',  ( 0.07217847769028949700, -0.08942795157528024563, -0.3641732283464568787 ) ) ;
#35958=CARTESIAN_POINT ( 'NONE',  ( -0.1574803149606292529, -0.1870078740157479769, 0.4822834645669291653 ) ) ;
#35959=CARTESIAN_POINT ( 'NONE',  ( -1.194225721784776262, -0.3690944881889763329, 0.3153832671262228327 ) ) ;
#35960=CARTESIAN_POINT ( 'NONE',  ( -0.8923884514435688198, 0.2306618581243847221, -0.2411417322834647770 ) ) ;
#35961=CARTESIAN_POINT ( 'NONE',  ( 1.646981627296588035, -0.3162353388693405765, 0.4822834645669290543 ) ) ;
#35964=CARTESIAN_POINT ( 'NONE',  ( 1.614173228346457378, 0.2952755905511811885, 0.000000000000000000 ) ) ;
#35966=CARTESIAN_POINT ( 'NONE',  ( -1.404199475065615932, 0.05413385826771666132, 0.4176697321401328100 ) ) ;
#35967=CARTESIAN_POINT ( 'NONE',  ( -1.207349081364828436, -0.5023911411419708095, 0.1820866141732285504 ) ) ;
#35968=CARTESIAN_POINT ( 'NONE',  ( -0.7545931758530177724, 0.1771653543307087630, 0.09757992244046791164 ) ) ;
#35969=CARTESIAN_POINT ( 'NONE',  ( -1.653543307086613234, -0.1870078740157479769, 0.4822834645669291653 ) ) ;
#35970=CARTESIAN_POINT ( 'NONE',  ( 0.2034120734908144990, -0.6692913385826771977, 0.1292274648535927661 ) ) ;
#35971=CARTESIAN_POINT ( 'NONE',  ( 0.3871391076115493490, -0.2845877964562159024, 0.3641732283464567677 ) ) ;
#35972=CARTESIAN_POINT ( 'NONE',  ( -1.213910761154854745, 0.1771653543307087075, -0.09757992244046823083 ) ) ;
#35973=CARTESIAN_POINT ( 'NONE',  ( -1.299212598425196097, -0.6692913385826771977, 8.415575281601705876E-17 ) ) ;
#35974=CARTESIAN_POINT ( 'NONE',  ( 1.227034120734908917, -0.5511811023622046335, 0.09757992244046803654 ) ) ;
#35975=CARTESIAN_POINT ( 'NONE',  ( 1.404199475065617708, 0.05413385826771626580, -0.4176697321401330321 ) ) ;
#35977=CARTESIAN_POINT ( 'NONE',  ( 0.6364829396325465405, -0.2845877964562161244, -0.3641732283464567121 ) ) ;
#35978=CARTESIAN_POINT ( 'NONE',  ( 0.9711286089238851948, -0.6046776061558809534, -0.2411417322834644161 ) ) ;
#35979=LINE ( 'NONE', #50130, #39404 ) ;
#35980=CARTESIAN_POINT ( 'NONE',  ( 0.9645669291338588858, 0.07958543189024085140, 0.2665933059059887866 ) ) ;
#35982=CARTESIAN_POINT ( 'NONE',  ( -1.318897637795274802, 0.1660481256975885056, 0.3530559997133364547 ) ) ;
#35983=CARTESIAN_POINT ( 'NONE',  ( -0.7217847769028863381, -0.4281496062992124485, 0.4176697321401328655 ) ) ;
#35984=CARTESIAN_POINT ( 'NONE',  ( -0.1509186351706028884, -0.05778040916215522460, 0.4822834645669289988 ) ) ;
#35987=CARTESIAN_POINT ( 'NONE',  ( 0.9120734908136489683, -0.6692913385826771977, 0.1292274648535927661 ) ) ;
#35988=CARTESIAN_POINT ( 'NONE',  ( 1.417322834645670104, -0.1870078740157479769, 0.3641732283464567677 ) ) ;
#35989=CARTESIAN_POINT ( 'NONE',  ( -0.07217847769028787330, -0.05778040916215522460, 0.4822834645669289988 ) ) ;
#35990=CARTESIAN_POINT ( 'NONE',  ( 0.7414698162729663755, -0.6692913385826773087, -0.1292274648535924053 ) ) ;
#35994=CARTESIAN_POINT ( 'NONE',  ( -1.033630966599879297, -2.567464376874931580E-15, -0.4445507791589072832 ) ) ;
#35996=CARTESIAN_POINT ( 'NONE',  ( -0.2755905511811018171, 0.1771653543307087630, 0.000000000000000000 ) ) ;
#35997=CARTESIAN_POINT ( 'NONE',  ( -0.8267716535433065062, -0.6692913385826771977, 8.415575281601705876E-17 ) ) ;
#35998=CARTESIAN_POINT ( 'NONE',  ( 0.9383202099737536495, -0.3162353388693405765, 0.4822834645669290543 ) ) ;
#36000=CARTESIAN_POINT ( 'NONE',  ( -0.5380577427821514602, -0.004921259842519576551, 0.3153832671262227771 ) ) ;
#36001=CARTESIAN_POINT ( 'NONE',  ( 1.587926509186352142, 0.05413385826771666132, 0.4176697321401328100 ) ) ;
#36002=CARTESIAN_POINT ( 'NONE',  ( 1.062992125984252745, -0.6692913385826771977, 8.415575281601705876E-17 ) ) ;
#36005=CARTESIAN_POINT ( 'NONE',  ( 1.148293963254593653, 0.2952755905511810219, -0.1292274648535930437 ) ) ;
#36007=CARTESIAN_POINT ( 'NONE',  ( 1.200787401574803681, -0.5400638737290845981, -0.3530559997133363437 ) ) ;
#36008=CARTESIAN_POINT ( 'NONE',  ( 1.122047244094488860, 0.07958543189024085140, 0.2665933059059887866 ) ) ;
#36009=CARTESIAN_POINT ( 'NONE',  ( -1.574803149606298192, -0.1870078740157480601, -0.3641732283464567677 ) ) ;
#36010=CARTESIAN_POINT ( 'NONE',  ( -1.469816272965878357, 0.2306618581243848609, 0.2411417322834645549 ) ) ;
#36012=CARTESIAN_POINT ( 'NONE',  ( 0.9776902887139113929, -0.6692913385826773087, -0.1292274648535924053 ) ) ;
#36013=CARTESIAN_POINT ( 'NONE',  ( -1.482939632545930975, -0.4281496062992127816, -0.4176697321401328100 ) ) ;
#36014=CARTESIAN_POINT ( 'NONE',  ( -0.5380577427821514602, -0.4281496062992127816, -0.4176697321401328100 ) ) ;
#36015=CARTESIAN_POINT ( 'NONE',  ( -0.3740157480314953431, -0.5400638737290845981, -0.3530559997133363437 ) ) ;
#36016=CARTESIAN_POINT ( 'NONE',  ( 1.476377952755906220, 0.1660481256975883668, -0.3530559997133364547 ) ) ;
#36018=CARTESIAN_POINT ( 'NONE',  ( 0.2559055118110243332, -0.5400638737290845981, -0.3530559997133363437 ) ) ;
#36020=CARTESIAN_POINT ( 'NONE',  ( -1.555118110236219930, -0.4536011799217368745, -0.2665933059059886201 ) ) ;
#36024=CARTESIAN_POINT ( 'NONE',  ( -0.06632061457837669372, -2.294479370626195693E-15, 0.3464511005275217603 ) ) ;
#36025=CARTESIAN_POINT ( 'NONE',  ( -1.358267716535432434, 0.1660481256975883668, -0.3530559997133364547 ) ) ;
#36030=CARTESIAN_POINT ( 'NONE',  ( -0.5249343832020990641, 0.1283753931104748280, 0.1820866141732283561 ) ) ;
#36031=CARTESIAN_POINT ( 'NONE',  ( -1.174540682414697335, -0.2845877964562161244, -0.3641732283464567121 ) ) ;
#36032=CARTESIAN_POINT ( 'NONE',  ( -1.561679790026246017, -0.4281496062992127816, -0.4176697321401328100 ) ) ;
#36033=CARTESIAN_POINT ( 'NONE',  ( 0.7283464566929140904, -0.5400638737290845981, -0.3530559997133363437 ) ) ;
#36034=CARTESIAN_POINT ( 'NONE',  ( -1.502624671916009680, -0.3162353388693405765, 0.4822834645669290543 ) ) ;
#36037=B_SPLINE_CURVE_WITH_KNOTS ( 'NONE', 3,
 ( #67743, #59747, #35740, #14745 ),
 .UNSPECIFIED., .F., .F.,
 ( 4, 4 ),
 ( 0.000000000000000000, 0.001493228121701133202 ),
 .UNSPECIFIED. ) ;
#36038=CARTESIAN_POINT ( 'NONE',  ( -1.463254593175852492, 0.2952755905511811885, 0.1292274648535926551 ) ) ;
#36045=CARTESIAN_POINT ( 'NONE',  ( -0.8464566929133852113, 0.1660481256975885056, 0.3530559997133364547 ) ) ;
#36046=CARTESIAN_POINT ( 'NONE',  ( 1.305774278215223960, -0.6692913385826771977, 0.1292274648535927661 ) ) ;
#36047=CARTESIAN_POINT ( 'NONE',  ( -1.607611548556429737, -0.6692913385826771977, 0.1292274648535927661 ) ) ;
#36048=CARTESIAN_POINT ( 'NONE',  ( -1.603475055217291612, 1.606158680897942670, -0.04573490813648262154 ) ) ;
#36049=CARTESIAN_POINT ( 'NONE',  ( -1.719160104986876103, 0.05413385826771666132, 0.4176697321401328100 ) ) ;
#36050=CARTESIAN_POINT ( 'NONE',  ( -0.6233595800524928121, -0.05778040916215522460, 0.4822834645669289988 ) ) ;
#36052=B_SPLINE_CURVE_WITH_KNOTS ( 'NONE', 3,
 ( #52103, #51684, #31928, #25192, #83280, #45376, #57590 ),
 .UNSPECIFIED., .F., .F.,
 ( 4, 3, 4 ),
 ( 1.734723475976807094E-18, 0.001246232571205225159, 0.002492492258783242029 ),
 .UNSPECIFIED. ) ;
#36053=CARTESIAN_POINT ( 'NONE',  ( 0.1706036745406830368, -0.004921259842519576551, 0.3153832671262227771 ) ) ;
#36055=CARTESIAN_POINT ( 'NONE',  ( 0.09842519685039434474, 0.07958543189024085140, 0.2665933059059887866 ) ) ;
#36056=CARTESIAN_POINT ( 'NONE',  ( 1.095800524934383846, -0.2845877964562159024, 0.3641732283464567677 ) ) ;
#36057=CARTESIAN_POINT ( 'NONE',  ( 0.3608923884514443348, 0.2952755905511810774, -0.1292274648535930714 ) ) ;
#36058=CARTESIAN_POINT ( 'NONE',  ( -0.3149606299212590610, -0.1870078740157480601, -0.3641732283464567677 ) ) ;
#36060=CARTESIAN_POINT ( 'NONE',  ( 1.535433070866142335, -0.6692913385826771977, 8.415575281601705876E-17 ) ) ;
#36061=CARTESIAN_POINT ( 'NONE',  ( -0.8792650918635160906, -0.4281496062992124485, 0.4176697321401328655 ) ) ;
#36063=CARTESIAN_POINT ( 'NONE',  ( 0.1443569553805781891, -0.4281496062992124485, 0.4176697321401328655 ) ) ;
#36064=CARTESIAN_POINT ( 'NONE',  ( -0.5052493438320203589, 0.2952755905511810774, -0.1292274648535930714 ) ) ;
#36065=CARTESIAN_POINT ( 'NONE',  ( 1.574803149606299746, -0.1870078740157480601, -0.3641732283464567677 ) ) ;
#36066=CARTESIAN_POINT ( 'NONE',  ( 0.08530183727034192087, -0.2845877964562161244, -0.3641732283464567121 ) ) ;
#36067=CARTESIAN_POINT ( 'NONE',  ( -0.2755905511811018171, 0.2952755905511811885, 0.000000000000000000 ) ) ;
#36068=CARTESIAN_POINT ( 'NONE',  ( -0.8136482939632537770, 0.2306618581243847221, -0.2411417322834647770 ) ) ;
#36071=CARTESIAN_POINT ( 'NONE',  ( 0.1771653543307093182, -0.5400638737290845981, -0.3530559997133363437 ) ) ;
#36075=CARTESIAN_POINT ( 'NONE',  ( 1.417322834645670104, -0.1870078740157479769, 0.4822834645669291653 ) ) ;
#36076=CARTESIAN_POINT ( 'NONE',  ( -0.5314960629921254842, -0.4536011799217368745, -0.2665933059059886201 ) ) ;
#36077=CARTESIAN_POINT ( 'NONE',  ( -0.4855643044619415427, -0.4281496062992124485, 0.4176697321401328655 ) ) ;
#36078=CARTESIAN_POINT ( 'NONE',  ( 1.384514435695538559, 0.2952755905511810774, -0.1292274648535930714 ) ) ;
#36079=CARTESIAN_POINT ( 'NONE',  ( 1.174540682414699111, -0.3162353388693405765, 0.4822834645669290543 ) ) ;
#36080=CARTESIAN_POINT ( 'NONE',  ( -1.601049868766403650, 0.2306618581243847221, -0.2411417322834647770 ) ) ;
#36081=CARTESIAN_POINT ( 'NONE',  ( -0.9251968503937002541, 0.07958543189024085140, 0.2665933059059887866 ) ) ;
#36085=CARTESIAN_POINT ( 'NONE',  ( 1.679790026246720025, 0.1283753931104748280, 0.1820866141732283561 ) ) ;
#36086=CARTESIAN_POINT ( 'NONE',  ( 1.135170603674541256, 0.1771653543307087630, 0.09757992244046791164 ) ) ;
#36087=CARTESIAN_POINT ( 'NONE',  ( 0.8333333333333340365, 0.2952755905511810774, -0.1292274648535930714 ) ) ;
#36088=CARTESIAN_POINT ( 'NONE',  ( -1.646981627296586703, -0.3162353388693409650, -0.4822834645669289433 ) ) ;
#36089=CARTESIAN_POINT ( 'NONE',  ( 0.9580052493438326877, 0.05413385826771666132, 0.4176697321401328100 ) ) ;
#36091=CARTESIAN_POINT ( 'NONE',  ( 1.233595800524935227, 0.1283753931104746893, -0.1820866141732285504 ) ) ;
#36092=CARTESIAN_POINT ( 'NONE',  ( 0.2887139107611556010, 0.2306618581243847221, -0.2411417322834647770 ) ) ;
#36093=CARTESIAN_POINT ( 'NONE',  ( -0.9776902887139098386, 0.2952755905511810774, -0.1292274648535930714 ) ) ;
#36094=CARTESIAN_POINT ( 'NONE',  ( 1.213910761154856299, 0.2952755905511811885, 0.1292274648535926551 ) ) ;
#36097=CARTESIAN_POINT ( 'NONE',  ( 0.3871391076115492380, -0.08942795157528024563, -0.3641732283464568787 ) ) ;
#36098=VERTEX_POINT ( 'NONE', #82232 ) ;
#36100=ORIENTED_EDGE ( 'NONE', *, *, #23015, .F. ) ;
#36101=CARTESIAN_POINT ( 'NONE',  ( -0.9120734908136475250, 0.2952755905511811885, 0.1292274648535926551 ) ) ;
#36102=CARTESIAN_POINT ( 'NONE',  ( -0.2099737532808391705, 0.2306618581243848609, 0.2411417322834645549 ) ) ;
#36103=CARTESIAN_POINT ( 'NONE',  ( -0.5118110236220466680, 0.2952755905511811885, 0.000000000000000000 ) ) ;
#36104=CARTESIAN_POINT ( 'NONE',  ( 0.8136482939632553313, -0.6046776061558809534, -0.2411417322834644161 ) ) ;
#36105=CARTESIAN_POINT ( 'NONE',  ( -1.325459317585300889, 0.05413385826771666132, 0.4176697321401328100 ) ) ;
#36106=CARTESIAN_POINT ( 'NONE',  ( -0.2427821522309703550, -0.05778040916215560624, -0.4822834645669293319 ) ) ;
#36107=CARTESIAN_POINT ( 'NONE',  ( 0.5905511811023629321, -0.6692913385826771977, 8.415575281601705876E-17 ) ) ;
#36108=CARTESIAN_POINT ( 'NONE',  ( 0.3805774278215230400, 0.05413385826771626580, -0.4176697321401330321 ) ) ;
#36109=CARTESIAN_POINT ( 'NONE',  ( 0.8136482939632553313, -0.6046776061558809534, -0.2411417322834644161 ) ) ;
#36111=CARTESIAN_POINT ( 'NONE',  ( -0.3083989501312330295, -0.2845877964562161244, -0.3641732283464567121 ) ) ;
#36112=ORIENTED_EDGE ( 'NONE', *, *, #1873, .T. ) ;
#36114=ORIENTED_EDGE ( 'NONE', *, *, #45969, .T. ) ;
#36115=CARTESIAN_POINT ( 'NONE',  ( -0.6824146981627291497, -0.5023911411419708095, -0.1820866141732282451 ) ) ;
#36116=CARTESIAN_POINT ( 'NONE',  ( -0.3083989501312330295, -0.3162353388693409650, -0.4822834645669289433 ) ) ;
#36117=CARTESIAN_POINT ( 'NONE',  ( -0.8661417322834640276, -0.1870078740157480879, -0.4822834645669291653 ) ) ;
#36118=CARTESIAN_POINT ( 'NONE',  ( -0.9776902887139098386, -0.6692913385826771977, 0.1292274648535927661 ) ) ;
#36119=CARTESIAN_POINT ( 'NONE',  ( -1.325459317585300889, 0.05413385826771666132, 0.4176697321401328100 ) ) ;
#36120=CARTESIAN_POINT ( 'NONE',  ( -1.233595800524933894, 0.2306618581243848609, 0.2411417322834645549 ) ) ;
#36121=CARTESIAN_POINT ( 'NONE',  ( 0.9186351706036752773, 0.1283753931104746893, -0.1820866141732285504 ) ) ;
#36124=CARTESIAN_POINT ( 'NONE',  ( -0.06561679790026180015, -0.3690944881889765550, -0.3153832671262227771 ) ) ;
#36125=CARTESIAN_POINT ( 'NONE',  ( 0.1574803149606306130, -0.1870078740157480879, -0.4822834645669291653 ) ) ;
#36126=CARTESIAN_POINT ( 'NONE',  ( -0.2034120734908128059, 0.2952755905511811885, 0.1292274648535926551 ) ) ;
#36129=CARTESIAN_POINT ( 'NONE',  ( -0.5971128608923876868, 0.2952755905511811885, 0.1292274648535926551 ) ) ;
#36133=CARTESIAN_POINT ( 'NONE',  ( -0.5511811023622041894, -0.1870078740157480601, -0.3641732283464567677 ) ) ;
#36134=CARTESIAN_POINT ( 'NONE',  ( -0.8070866141732276899, -0.5400638737290844871, 0.3530559997133364547 ) ) ;
#36137=( BOUNDED_CURVE ( )  B_SPLINE_CURVE ( 2, ( #44191, #37067, #5088, #56418, #69881, #61513, #3858, #80888, #31991, #18948, #7155, #7585, #52170 ),
 .UNSPECIFIED., .F., .F. ) 
 B_SPLINE_CURVE_WITH_KNOTS ( ( 3, 2, 2, 2, 2, 2, 3 ),
 ( 0.8096947309984371399, 0.8106060606060605522, 0.8143939393939394478, 0.8181818181818182323, 0.8219696969696970168, 0.8257575757575758013, 0.8266689053651993246 ),
 .UNSPECIFIED. ) 
 CURVE ( )  GEOMETRIC_REPRESENTATION_ITEM ( )  RATIONAL_B_SPLINE_CURVE ( ( 0.9875488213027523443, 0.9918020599134680371, 1.000000000000000000, 0.9659258262890683122, 1.000000000000000000, 0.9659258262890683122, 1.000000000000000000, 0.9659258262890683122, 1.000000000000000000, 0.9659258262890683122, 1.000000000000000000, 0.9918020599134671489, 0.9875488213027514561 ) ) 
 REPRESENTATION_ITEM ( '' )  );
#36139=CARTESIAN_POINT ( 'NONE',  ( 1.102362204724410155, -0.1870078740157480879, -0.4822834645669291653 ) ) ;
#36140=CARTESIAN_POINT ( 'NONE',  ( 0.5446194225721792126, -0.05778040916215560624, -0.4822834645669293319 ) ) ;
#36141=CARTESIAN_POINT ( 'NONE',  ( 0.4527559055118117182, 0.1660481256975883668, -0.3530559997133364547 ) ) ;
#36142=CARTESIAN_POINT ( 'NONE',  ( -0.8202099737532799750, 0.1771653543307087075, -0.09757992244046823083 ) ) ;
#36143=CARTESIAN_POINT ( 'NONE',  ( 0.1640419947506569498, -0.05778040916215522460, 0.4822834645669289988 ) ) ;
#36145=CARTESIAN_POINT ( 'NONE',  ( -0.2624671916010490880, 0.2306618581243847221, -0.2411417322834647770 ) ) ;
#36147=CARTESIAN_POINT ( 'NONE',  ( 1.489501312335958172, -0.08942795157528024563, -0.3641732283464568787 ) ) ;
#36148=CARTESIAN_POINT ( 'NONE',  ( -0.4461942257217840213, 0.1283753931104748280, 0.1820866141732283561 ) ) ;
#36149=CARTESIAN_POINT ( 'NONE',  ( 1.135170603674541256, -0.5511811023622048555, -0.09757992244046775898 ) ) ;
#36150=CARTESIAN_POINT ( 'NONE',  ( -1.345144356955379816, -0.05778040916215560624, -0.4822834645669293319 ) ) ;
#36151=CARTESIAN_POINT ( 'NONE',  ( -0.9514435695538050464, -0.08942795157528024563, -0.3641732283464568787 ) ) ;
#36152=CARTESIAN_POINT ( 'NONE',  ( 0.4606732211678789546, 1.763126522798926343, 0.5309055118110234117 ) ) ;
#36153=CARTESIAN_POINT ( 'NONE',  ( -1.154855643044618851, -0.6046776061558809534, -0.2411417322834644161 ) ) ;
#36154=CARTESIAN_POINT ( 'NONE',  ( -0.6430446194225712953, 0.05413385826771626580, -0.4176697321401330321 ) ) ;
#36155=CARTESIAN_POINT ( 'NONE',  ( 0.3805774278215230400, -0.4281496062992124485, 0.4176697321401328655 ) ) ;
#36157=CARTESIAN_POINT ( 'NONE',  ( 0.3805774278215230400, -0.3690944881889763329, 0.3153832671262228327 ) ) ;
#36158=CARTESIAN_POINT ( 'NONE',  ( -1.535433070866141225, 0.1771653543307087630, 0.000000000000000000 ) ) ;
#36159=CARTESIAN_POINT ( 'NONE',  ( 0.7480314960629927956, 0.2952755905511811885, 0.000000000000000000 ) ) ;
#36160=CARTESIAN_POINT ( 'NONE',  ( -1.594488188976377563, -0.4536011799217367080, 0.2665933059059888421 ) ) ;
#36161=CARTESIAN_POINT ( 'NONE',  ( 1.509186351706037543, -0.3690944881889765550, -0.3153832671262227771 ) ) ;
#36162=CARTESIAN_POINT ( 'NONE',  ( -0.8333333333333323711, -0.6692913385826773087, -0.1292274648535924053 ) ) ;
#36163=CARTESIAN_POINT ( 'NONE',  ( -0.1443569553805765515, -0.3690944881889765550, -0.3153832671262227771 ) ) ;
#36164=CARTESIAN_POINT ( 'NONE',  ( -1.646051170424378096, 0.000000000000000000, 0.3464511005275205946 ) ) ;
#36165=CARTESIAN_POINT ( 'NONE',  ( 0.4986876640419954376, 0.1283753931104748280, 0.1820866141732283561 ) ) ;
#36167=CARTESIAN_POINT ( 'NONE',  ( -0.1049868766404193215, -0.6046776061558807314, 0.2411417322834647770 ) ) ;
#36171=CARTESIAN_POINT ( 'NONE',  ( 0.6430446194225728496, -0.004921259842519576551, 0.3153832671262227771 ) ) ;
#36172=CARTESIAN_POINT ( 'NONE',  ( 0.2034120734908144990, -0.6692913385826771977, 0.1292274648535927661 ) ) ;
#36173=CARTESIAN_POINT ( 'NONE',  ( -0.7217847769028863381, -0.4281496062992124485, 0.4176697321401328655 ) ) ;
#36174=CARTESIAN_POINT ( 'NONE',  ( -0.4461942257217840213, -0.5023911411419708095, -0.1820866141732282451 ) ) ;
#36176=CARTESIAN_POINT ( 'NONE',  ( -0.3149606299212590610, -0.1870078740157480601, -0.3641732283464567677 ) ) ;
#36177=CARTESIAN_POINT ( 'NONE',  ( 0.2755905511811031494, 0.2952755905511811885, 0.000000000000000000 ) ) ;
#36179=CARTESIAN_POINT ( 'NONE',  ( -1.023622047244094002, -0.1870078740157480601, -0.3641732283464567677 ) ) ;
#36181=CARTESIAN_POINT ( 'NONE',  ( 1.601049868766404982, 0.2306618581243848609, 0.2411417322834645549 ) ) ;
#36183=ORIENTED_EDGE ( 'NONE', *, *, #39193, .F. ) ;
#36184=CARTESIAN_POINT ( 'NONE',  ( -1.581364829396324945, -0.2845877964562159024, 0.3641732283464567677 ) ) ;
#36185=CARTESIAN_POINT ( 'NONE',  ( -0.6364829396325453192, -0.3162353388693405765, 0.4822834645669290543 ) ) ;
#36186=CARTESIAN_POINT ( 'NONE',  ( -1.312335958005248715, 0.2306618581243848609, 0.2411417322834645549 ) ) ;
#36190=CARTESIAN_POINT ( 'NONE',  ( 1.246719160104987623, 0.05413385826771626580, -0.4176697321401330321 ) ) ;
#36191=CARTESIAN_POINT ( 'NONE',  ( 0.2362204724409456558, -0.1870078740157479769, 0.4822834645669291653 ) ) ;
#36195=CARTESIAN_POINT ( 'NONE',  ( 1.482939632545932307, -0.004921259842519870586, -0.3153832671262229437 ) ) ;
#36197=ORIENTED_EDGE ( 'NONE', *, *, #53789, .F. ) ;
#36198=CARTESIAN_POINT ( 'NONE',  ( -0.7283464566929126471, -0.4536011799217367080, 0.2665933059059888421 ) ) ;
#36200=VERTEX_POINT ( 'NONE', #56529 ) ;
#36202=CARTESIAN_POINT ( 'NONE',  ( 0.3805774278215230400, 0.05413385826771626580, -0.4176697321401330321 ) ) ;
#36203=CARTESIAN_POINT ( 'NONE',  ( -0.5511811023622041894, -0.1870078740157480879, -0.4822834645669291653 ) ) ;
#36204=CARTESIAN_POINT ( 'NONE',  ( -0.9055118110236215490, -0.6692913385826771977, 8.415575281601705876E-17 ) ) ;
#36205=CARTESIAN_POINT ( 'NONE',  ( 0.9120734908136490793, 0.2952755905511810774, -0.1292274648535930714 ) ) ;
#36206=CARTESIAN_POINT ( 'NONE',  ( -1.338582677165353729, -0.1870078740157479769, 0.3641732283464567677 ) ) ;
#36207=CARTESIAN_POINT ( 'NONE',  ( 0.08983781461629372633, 7.699586553780600482E-16, 0.3954985857520059711 ) ) ;
#36208=CARTESIAN_POINT ( 'NONE',  ( 0.2559055118110243332, 0.1660481256975885056, 0.3530559997133364547 ) ) ;
#36209=CARTESIAN_POINT ( 'NONE',  ( -0.9645669291338575535, 0.1660481256975883668, -0.3530559997133364547 ) ) ;
#36211=CARTESIAN_POINT ( 'NONE',  ( -1.515748031496062076, -0.5400638737290844871, 0.3530559997133364547 ) ) ;
#36214=CARTESIAN_POINT ( 'NONE',  ( 0.9448818897637802916, -0.1870078740157480601, -0.3641732283464567677 ) ) ;
#36217=CARTESIAN_POINT ( 'NONE',  ( -0.3215223097112853146, -0.05778040916215560624, -0.4822834645669293319 ) ) ;
#36219=CARTESIAN_POINT ( 'NONE',  ( 0.5249343832021003964, 0.1283753931104746893, -0.1820866141732285504 ) ) ;
#36220=CARTESIAN_POINT ( 'NONE',  ( -1.410761154855642463, -0.05778040916215522460, 0.4822834645669289988 ) ) ;
#36221=CARTESIAN_POINT ( 'NONE',  ( 0.5380577427821529035, 0.05413385826771626580, -0.4176697321401330321 ) ) ;
#36222=CARTESIAN_POINT ( 'NONE',  ( 0.4396325459317590445, -0.6692913385826771977, 0.1292274648535927661 ) ) ;
#36223=CARTESIAN_POINT ( 'NONE',  ( -0.03280839895013062252, -0.6692913385826771977, 0.1292274648535927661 ) ) ;
#36225=CARTESIAN_POINT ( 'NONE',  ( -0.6036745406824141069, -0.6046776061558809534, -0.2411417322834644161 ) ) ;
#36227=CARTESIAN_POINT ( 'NONE',  ( 1.561679790026247350, -0.3690944881889763329, 0.3153832671262228327 ) ) ;
#36228=CARTESIAN_POINT ( 'NONE',  ( -1.017060367454067249, -0.05778040916215522460, 0.4822834645669289988 ) ) ;
#36229=CARTESIAN_POINT ( 'NONE',  ( 1.377952755905512472, 0.2952755905511811885, 0.000000000000000000 ) ) ;
#36230=CARTESIAN_POINT ( 'NONE',  ( 1.036745406824147731, 0.05413385826771666132, 0.4176697321401328100 ) ) ;
#36232=CARTESIAN_POINT ( 'NONE',  ( -0.9514435695538050464, -0.3162353388693405765, 0.4822834645669290543 ) ) ;
#36234=CARTESIAN_POINT ( 'NONE',  ( 0.3149606299212603933, -0.1870078740157479769, 0.4822834645669291653 ) ) ;
#36236=CARTESIAN_POINT ( 'NONE',  ( -0.5118110236220466680, 0.2952755905511811885, 0.000000000000000000 ) ) ;
#36237=CARTESIAN_POINT ( 'NONE',  ( 1.640419947506562393, -0.4281496062992124485, 0.4176697321401328655 ) ) ;
#36238=CARTESIAN_POINT ( 'NONE',  ( 0.5052493438320218022, -0.5511811023622048555, -0.09757992244046775898 ) ) ;
#36239=CARTESIAN_POINT ( 'NONE',  ( 1.469816272965879911, 0.2306618581243847221, -0.2411417322834647770 ) ) ;
#36241=CARTESIAN_POINT ( 'NONE',  ( 0.9580052493438327987, -0.3690944881889765550, -0.3153832671262227771 ) ) ;
#36243=CARTESIAN_POINT ( 'NONE',  ( 0.8202099737532813073, 0.2952755905511811885, 0.1292274648535926551 ) ) ;
#36245=CARTESIAN_POINT ( 'NONE',  ( -0.6233595800524928121, -0.05778040916215522460, 0.4822834645669289988 ) ) ;
#36247=CARTESIAN_POINT ( 'NONE',  ( 1.476377952755906220, 0.07958543189024071263, -0.2665933059059888421 ) ) ;
#36248=CARTESIAN_POINT ( 'NONE',  ( -0.7808398950131225646, -0.05778040916215522460, 0.4822834645669289988 ) ) ;
#36249=CARTESIAN_POINT ( 'NONE',  ( 0.03280839895013198948, 0.2952755905511811885, 0.1292274648535926551 ) ) ;
#36250=CARTESIAN_POINT ( 'NONE',  ( 0.4624320255261049062, 8.471767977567108961E-16, -0.4445507791589058955 ) ) ;
#36251=CARTESIAN_POINT ( 'NONE',  ( 0.08530183727034192087, -0.3162353388693409650, -0.4822834645669289433 ) ) ;
#36252=CARTESIAN_POINT ( 'NONE',  ( 0.03280839895013198948, -0.5511811023622048555, -0.09757992244046775898 ) ) ;
#36254=CARTESIAN_POINT ( 'NONE',  ( 8.195543980992789655E-16, -0.1870078740157480601, -0.3641732283464567677 ) ) ;
#36255=CARTESIAN_POINT ( 'NONE',  ( 0.5511811023622054106, -0.1870078740157480601, -0.3641732283464567677 ) ) ;
#36259=CARTESIAN_POINT ( 'NONE',  ( 0.5314960629921267055, -0.5400638737290844871, 0.3530559997133364547 ) ) ;
#36261=CARTESIAN_POINT ( 'NONE',  ( 1.561679790026247350, -0.004921259842519870586, -0.3153832671262229437 ) ) ;
#36263=CARTESIAN_POINT ( 'NONE',  ( -0.5774278215223089816, 0.1283753931104746893, -0.1820866141732285504 ) ) ;
#36264=CARTESIAN_POINT ( 'NONE',  ( -0.03937007874015669567, 0.2952755905511811885, 0.000000000000000000 ) ) ;
#36265=CARTESIAN_POINT ( 'NONE',  ( 1.161417322834646493, -0.4536011799217367080, 0.2665933059059888421 ) ) ;
#36266=CARTESIAN_POINT ( 'NONE',  ( -1.161417322834644716, -0.4536011799217368745, -0.2665933059059886201 ) ) ;
#36267=CARTESIAN_POINT ( 'NONE',  ( -1.450131233595799651, -0.6692913385826771977, 0.1292274648535927661 ) ) ;
#36268=CARTESIAN_POINT ( 'NONE',  ( 0.1115485564304470323, 0.2952755905511811885, 0.1292274648535926551 ) ) ;
#36269=CARTESIAN_POINT ( 'NONE',  ( 1.272965879265092637, -0.4281496062992127816, -0.4176697321401328100 ) ) ;
#36271=CARTESIAN_POINT ( 'NONE',  ( 0.08530183727034192087, -0.3162353388693409650, -0.4822834645669289433 ) ) ;
#36272=CARTESIAN_POINT ( 'NONE',  ( 1.305774278215223960, -0.6692913385826771977, 0.1292274648535927661 ) ) ;
#36273=CARTESIAN_POINT ( 'NONE',  ( 1.108923884514436686, -0.3162353388693409650, -0.4822834645669289433 ) ) ;
#36275=CARTESIAN_POINT ( 'NONE',  ( 0.8989501312335964611, 0.1771653543307087630, 0.09757992244046791164 ) ) ;
#36276=CARTESIAN_POINT ( 'NONE',  ( -1.548556430446193399, -0.5023911411419708095, -0.1820866141732282451 ) ) ;
#36277=CARTESIAN_POINT ( 'NONE',  ( 0.2624671916010504757, -0.5023911411419708095, -0.1820866141732282451 ) ) ;
#36278=CARTESIAN_POINT ( 'NONE',  ( -0.1902887139107604098, 0.2952755905511810774, -0.1292274648535930714 ) ) ;
#36279=CARTESIAN_POINT ( 'NONE',  ( 0.7283464566929140904, -0.5400638737290845981, -0.3530559997133363437 ) ) ;
#36280=CARTESIAN_POINT ( 'NONE',  ( -0.5643044619422565855, -0.4281496062992124485, 0.4176697321401328655 ) ) ;
#36282=CARTESIAN_POINT ( 'NONE',  ( -0.3608923884514428360, -0.5511811023622048555, -0.09757992244046775898 ) ) ;
#36283=CARTESIAN_POINT ( 'NONE',  ( 0.8727034120734912248, -0.3162353388693409650, -0.4822834645669289433 ) ) ;
#36284=CARTESIAN_POINT ( 'NONE',  ( 0.8792650918635177559, -0.004921259842519576551, 0.3153832671262227771 ) ) ;
#36286=CARTESIAN_POINT ( 'NONE',  ( -1.049868766404198794, 0.2306618581243847221, -0.2411417322834647770 ) ) ;
#36287=CARTESIAN_POINT ( 'NONE',  ( 1.601049868766404982, 0.2306618581243848609, 0.2411417322834645549 ) ) ;
#36289=CARTESIAN_POINT ( 'NONE',  ( -1.279527559055116948, 0.1660481256975883668, -0.3530559997133364547 ) ) ;
#36290=CARTESIAN_POINT ( 'NONE',  ( -0.3018372703412066094, 0.05413385826771666132, 0.4176697321401328100 ) ) ;
#36293=EDGE_LOOP ( 'NONE', ( #76981, #73591, #8039, #7442, #42811, #75353, #63929 ) ) ;
#36294=CARTESIAN_POINT ( 'NONE',  ( 0.3018372703412079971, -0.004921259842519870586, -0.3153832671262229437 ) ) ;
#36296=CARTESIAN_POINT ( 'NONE',  ( 1.043307086614173818, -0.5400638737290845981, -0.3530559997133363437 ) ) ;
#36300=CARTESIAN_POINT ( 'NONE',  ( 1.646981627296588035, -0.3162353388693405765, 0.4822834645669290543 ) ) ;
#36301=CARTESIAN_POINT ( 'NONE',  ( 1.541994750656168645, -0.5511811023622046335, 0.09757992244046803654 ) ) ;
#36302=CARTESIAN_POINT ( 'NONE',  ( 0.6102362204724416372, 0.1660481256975883668, -0.3530559997133364547 ) ) ;
#36304=CARTESIAN_POINT ( 'NONE',  ( -0.3805774278215216522, 0.05413385826771666132, 0.4176697321401328100 ) ) ;
#36305=CARTESIAN_POINT ( 'NONE',  ( -1.056430446194224881, 0.1771653543307087075, -0.09757992244046823083 ) ) ;
#36306=CARTESIAN_POINT ( 'NONE',  ( 0.6496062992125991586, 0.1660481256975885056, 0.3530559997133364547 ) ) ;
#36307=CARTESIAN_POINT ( 'NONE',  ( 0.03937007874015806264, 0.2952755905511811885, 0.000000000000000000 ) ) ;
#36311=CARTESIAN_POINT ( 'NONE',  ( 0.9251968503937015864, 0.1660481256975883668, -0.3530559997133364547 ) ) ;
#36312=CARTESIAN_POINT ( 'NONE',  ( -0.1771653543307080136, -0.5400638737290844871, 0.3530559997133364547 ) ) ;
#36313=CARTESIAN_POINT ( 'NONE',  ( -1.279527559055116948, 0.1660481256975883668, -0.3530559997133364547 ) ) ;
#36315=CARTESIAN_POINT ( 'NONE',  ( 1.049868766404200127, -0.6046776061558809534, -0.2411417322834644161 ) ) ;
#36316=CARTESIAN_POINT ( 'NONE',  ( 0.4396325459317593221, 0.2952755905511810774, -0.1292274648535930714 ) ) ;
#36318=CARTESIAN_POINT ( 'NONE',  ( -0.3608923884514428360, -0.6692913385826773087, -0.1292274648535924053 ) ) ;
#36319=CARTESIAN_POINT ( 'NONE',  ( 0.1049868766404206816, 0.2306618581243848609, 0.2411417322834645549 ) ) ;
#36320=CARTESIAN_POINT ( 'NONE',  ( -0.6299212598425188991, -0.1870078740157480879, -0.4822834645669291653 ) ) ;
#36322=CARTESIAN_POINT ( 'NONE',  ( 0.3608923884514443348, -0.5511811023622046335, 0.09757992244046803654 ) ) ;
#36323=CARTESIAN_POINT ( 'NONE',  ( 1.640419947506562393, -0.3690944881889763329, 0.3153832671262228327 ) ) ;
#36324=CARTESIAN_POINT ( 'NONE',  ( -1.673228346456691717, 0.1660481256975883668, -0.3530559997133364547 ) ) ;
#36325=CARTESIAN_POINT ( 'NONE',  ( 0.5052493438320215802, 0.2952755905511811885, 0.1292274648535926551 ) ) ;
#36326=FILL_AREA_STYLE ('',( #3936 ) ) ;
#36327=CARTESIAN_POINT ( 'NONE',  ( 1.561679790026247350, -0.4281496062992124485, 0.4176697321401328655 ) ) ;
#36329=EDGE_LOOP ( 'NONE', ( #5988, #15622, #38917 ) ) ;
#36330=ORIENTED_EDGE ( 'NONE', *, *, #50107, .T. ) ;
#36331=CARTESIAN_POINT ( 'NONE',  ( 0.6430446194225729606, -0.4281496062992127816, -0.4176697321401328100 ) ) ;
#36332=CARTESIAN_POINT ( 'NONE',  ( 0.1706036745406830368, -0.004921259842519576551, 0.3153832671262227771 ) ) ;
#36336=DIRECTION ( 'NONE',  ( 3.096699300667737957E-16, -1.000000000000000000, 0.000000000000000000 ) ) ;
#36339=CARTESIAN_POINT ( 'NONE',  ( 0.5839895013123367340, -0.6692913385826773087, -0.1292274648535924053 ) ) ;
#36340=CARTESIAN_POINT ( 'NONE',  ( -0.9317585301837263412, -0.4281496062992127816, -0.4176697321401328100 ) ) ;
#36341=CARTESIAN_POINT ( 'NONE',  ( -0.5511811023622041894, -0.1870078740157480879, -0.4822834645669291653 ) ) ;
#36342=CARTESIAN_POINT ( 'NONE',  ( 0.7349081364829402885, -0.6046776061558809534, -0.2411417322834644161 ) ) ;
#36343=CARTESIAN_POINT ( 'NONE',  ( 1.187664041994751285, -0.3162353388693409650, -0.4822834645669289433 ) ) ;
#36344=CARTESIAN_POINT ( 'NONE',  ( 1.627296587926509996, -0.5023911411419708095, 0.1820866141732285504 ) ) ;
#36346=CARTESIAN_POINT ( 'NONE',  ( 1.161417322834646493, -0.4536011799217367080, 0.2665933059059888421 ) ) ;
#36347=CARTESIAN_POINT ( 'NONE',  ( -0.8398950131233585692, 0.2306618581243848609, 0.2411417322834645549 ) ) ;
#36348=CARTESIAN_POINT ( 'NONE',  ( -1.653543307086613234, -0.1870078740157479769, 0.3641732283464567677 ) ) ;
#36350=CARTESIAN_POINT ( 'NONE',  ( -0.2887139107611542133, -0.6046776061558809534, -0.2411417322834644161 ) ) ;
#36351=CARTESIAN_POINT ( 'NONE',  ( 1.233595800524935227, 0.2306618581243847221, -0.2411417322834647770 ) ) ;
#36353=CARTESIAN_POINT ( 'NONE',  ( -0.9580052493438311334, -0.3690944881889763329, 0.3153832671262228327 ) ) ;
#36354=CARTESIAN_POINT ( 'NONE',  ( 0.3412073490813655186, -0.6046776061558809534, -0.2411417322834644161 ) ) ;
#36355=CARTESIAN_POINT ( 'NONE',  ( 1.181102362204724976, -0.1870078740157480601, -0.3641732283464567677 ) ) ;
#36357=B_SPLINE_CURVE_WITH_KNOTS ( 'NONE', 3,
 ( #33863, #45640, #1884, #58271 ),
 .UNSPECIFIED., .F., .F.,
 ( 4, 4 ),
 ( 1.999999999927407068E-07, 0.006970199999999936863 ),
 .UNSPECIFIED. ) ;
#36358=CARTESIAN_POINT ( 'NONE',  ( -1.246719160104986512, -0.004921259842519576551, 0.3153832671262227771 ) ) ;
#36359=CARTESIAN_POINT ( 'NONE',  ( 1.318897637795276356, -0.5400638737290844871, 0.3530559997133364547 ) ) ;
#36361=CARTESIAN_POINT ( 'NONE',  ( -0.01312335958005186876, -0.3690944881889763329, 0.3153832671262228327 ) ) ;
#36362=CARTESIAN_POINT ( 'NONE',  ( -0.2165354330708654795, -0.5400638737290845981, -0.3530559997133363437 ) ) ;
#36363=CARTESIAN_POINT ( 'NONE',  ( -1.404199475065615932, -0.3690944881889765550, -0.3153832671262227771 ) ) ;
#36364=CARTESIAN_POINT ( 'NONE',  ( -0.8858267716535425107, 0.1660481256975883668, -0.3530559997133364547 ) ) ;
#36366=CARTESIAN_POINT ( 'NONE',  ( 1.463254593175853824, -0.6692913385826771977, 0.1292274648535927661 ) ) ;
#36368=CARTESIAN_POINT ( 'NONE',  ( -0.8727034120734901146, -0.2845877964562159024, 0.3641732283464567677 ) ) ;
#36369=DIRECTION ( 'NONE',  ( 1.692413147294446216E-16, -0.000000000000000000, 1.000000000000000000 ) ) ;
#36370=CARTESIAN_POINT ( 'NONE',  ( 1.456692913385827515, 0.2952755905511811885, 0.000000000000000000 ) ) ;
#36372=CARTESIAN_POINT ( 'NONE',  ( -1.174540682414697335, -0.3162353388693409650, -0.4822834645669289433 ) ) ;
#36373=CARTESIAN_POINT ( 'NONE',  ( -1.194225721784776262, -0.3690944881889763329, 0.3153832671262228327 ) ) ;
#36374=CARTESIAN_POINT ( 'NONE',  ( -0.6889763779527552368, -0.4536011799217368745, -0.2665933059059886201 ) ) ;
#36375=CARTESIAN_POINT ( 'NONE',  ( -1.614173228346455824, 0.2952755905511811885, 0.000000000000000000 ) ) ;
#36376=CARTESIAN_POINT ( 'NONE',  ( 0.07217847769028949700, -0.3162353388693405765, 0.4822834645669290543 ) ) ;
#36377=CARTESIAN_POINT ( 'NONE',  ( -0.1574803149606292529, -0.1870078740157480601, -0.3641732283464567677 ) ) ;
#36378=CARTESIAN_POINT ( 'NONE',  ( -1.286089238845143479, -0.5023911411419708095, 0.1820866141732285504 ) ) ;
#36379=CARTESIAN_POINT ( 'NONE',  ( -1.272965879265091305, -0.4281496062992124485, 0.4176697321401328655 ) ) ;
#36380=CARTESIAN_POINT ( 'NONE',  ( 1.443569553805774897, 0.1283753931104748280, 0.1820866141732283561 ) ) ;
#36381=CARTESIAN_POINT ( 'NONE',  ( 0.8661417322834653598, -0.1870078740157479769, 0.4822834645669291653 ) ) ;
#36383=CARTESIAN_POINT ( 'NONE',  ( 0.5380577427821529035, -0.3690944881889763329, 0.3153832671262228327 ) ) ;
#36384=CARTESIAN_POINT ( 'NONE',  ( 0.8333333333333340365, -0.6692913385826771977, 0.1292274648535927661 ) ) ;
#36385=CARTESIAN_POINT ( 'NONE',  ( 1.161417322834646271, 0.07958543189024071263, -0.2665933059059888421 ) ) ;
#36387=CARTESIAN_POINT ( 'NONE',  ( -1.404199475065615932, -0.4281496062992127816, -0.4176697321401328100 ) ) ;
#36388=CARTESIAN_POINT ( 'NONE',  ( -1.076115485564303809, -0.6046776061558809534, -0.2411417322834644161 ) ) ;
#36389=CARTESIAN_POINT ( 'NONE',  ( -0.02624671916010428221, -0.6046776061558807314, 0.2411417322834647770 ) ) ;
#36392=CARTESIAN_POINT ( 'NONE',  ( 0.9776902887139113929, 0.2952755905511811885, 0.1292274648535926551 ) ) ;
#36393=CARTESIAN_POINT ( 'NONE',  ( 1.391076115485564868, -0.5023911411419708095, 0.1820866141732285504 ) ) ;
#36394=CARTESIAN_POINT ( 'NONE',  ( 0.1968503937007881344, -0.6692913385826771977, 8.415575281601705876E-17 ) ) ;
#36395=CARTESIAN_POINT ( 'NONE',  ( 0.7349081364829402885, -0.6046776061558809534, -0.2411417322834644161 ) ) ;
#36401=CARTESIAN_POINT ( 'NONE',  ( -0.4921259842519677963, -0.4536011799217367080, 0.2665933059059888421 ) ) ;
#36402=CARTESIAN_POINT ( 'NONE',  ( -0.6955380577427815458, -0.4281496062992127816, -0.4176697321401328100 ) ) ;
#36403=CARTESIAN_POINT ( 'NONE',  ( 0.2493438320209980519, -0.4281496062992127816, -0.4176697321401328100 ) ) ;
#36405=CARTESIAN_POINT ( 'NONE',  ( 1.535433070866142335, -0.6692913385826771977, 8.415575281601705876E-17 ) ) ;
#36406=CARTESIAN_POINT ( 'NONE',  ( 1.200787401574803681, -0.5400638737290845981, -0.3530559997133363437 ) ) ;
#36411=CARTESIAN_POINT ( 'NONE',  ( 0.9317585301837276734, -0.4281496062992124485, 0.4176697321401328655 ) ) ;
#36412=EDGE_CURVE ( 'NONE', #32791, #81796, #48417, .T. ) ;
#36413=CARTESIAN_POINT ( 'NONE',  ( 0.8267716535433077274, 0.2952755905511811885, 0.000000000000000000 ) ) ;
#36414=CARTESIAN_POINT ( 'NONE',  ( 1.135170603674541256, 0.1771653543307087630, 0.09757992244046791164 ) ) ;
#36415=CARTESIAN_POINT ( 'NONE',  ( -1.587926509186350810, -0.004921259842519870586, -0.3153832671262229437 ) ) ;
#36416=CARTESIAN_POINT ( 'NONE',  ( -1.620734908136482577, 0.2952755905511811885, 0.1292274648535926551 ) ) ;
#36419=CARTESIAN_POINT ( 'NONE',  ( 1.010498687664042716, -0.4281496062992124485, 0.4176697321401328655 ) ) ;
#36420=CARTESIAN_POINT ( 'NONE',  ( 1.476377952755906442, -0.4536011799217367080, 0.2665933059059888421 ) ) ;
#36421=CARTESIAN_POINT ( 'NONE',  ( -0.6299212598425188991, -0.1870078740157479769, 0.4822834645669291653 ) ) ;
#36422=CARTESIAN_POINT ( 'NONE',  ( -0.6167979002624665030, 0.05413385826771666132, 0.4176697321401328100 ) ) ;
#36423=CARTESIAN_POINT ( 'NONE',  ( -1.528871391076114250, -0.6692913385826771977, 0.1292274648535927661 ) ) ;
#36425=CARTESIAN_POINT ( 'NONE',  ( 0.3608923884514443348, 0.2952755905511810774, -0.1292274648535930714 ) ) ;
#36427=CARTESIAN_POINT ( 'NONE',  ( 1.587926509186352586, -0.4281496062992127816, -0.4176697321401328100 ) ) ;
#36428=ORIENTED_EDGE ( 'NONE', *, *, #23876, .T. ) ;
#36430=ORIENTED_EDGE ( 'NONE', *, *, #36782, .F. ) ;
#36431=CARTESIAN_POINT ( 'NONE',  ( -1.586052503253849499, 0.4724409448818907564, 0.1653254495020552439 ) ) ;
#36432=CARTESIAN_POINT ( 'NONE',  ( 1.200787401574803681, -0.4536011799217368745, -0.2665933059059886201 ) ) ;
#36437=CARTESIAN_POINT ( 'NONE',  ( 0.4531182788721078158, 1.771653543307086354, 0.5309055118110234117 ) ) ;
#36439=CARTESIAN_POINT ( 'NONE',  ( -0.1968503937007867743, 0.1771653543307087630, 0.000000000000000000 ) ) ;
#36440=CARTESIAN_POINT ( 'NONE',  ( -1.371391076115484831, 0.1771653543307087075, -0.09757992244046823083 ) ) ;
#36441=CARTESIAN_POINT ( 'NONE',  ( 1.469816272965879911, 0.2306618581243847221, -0.2411417322834647770 ) ) ;
#36442=CARTESIAN_POINT ( 'NONE',  ( 0.6233595800524939223, -0.3162353388693405765, 0.4822834645669290543 ) ) ;
#36443=CARTESIAN_POINT ( 'NONE',  ( -1.443569553805773564, 0.2306618581243847221, -0.2411417322834647770 ) ) ;
#36446=CARTESIAN_POINT ( 'NONE',  ( -1.646981627296586703, -0.05778040916215522460, 0.4822834645669289988 ) ) ;
#36451=CARTESIAN_POINT ( 'NONE',  ( -0.8267716535433065062, 0.2952755905511811885, 0.000000000000000000 ) ) ;
#36452=CARTESIAN_POINT ( 'NONE',  ( 1.364829396325460076, 0.2306618581243848609, 0.2411417322834645549 ) ) ;
#36453=FACE_OUTER_BOUND ( 'NONE', #49159, .T. ) ;
#36454=CARTESIAN_POINT ( 'NONE',  ( 1.603475055217291612, 0.9922665159524515222, 0.04573490813648272563 ) ) ;
#36455=CARTESIAN_POINT ( 'NONE',  ( 1.463254593175853824, -0.6692913385826771977, 0.1292274648535927661 ) ) ;
#36456=CARTESIAN_POINT ( 'NONE',  ( -0.8333333333333323711, -0.6692913385826773087, -0.1292274648535924053 ) ) ;
#36458=CARTESIAN_POINT ( 'NONE',  ( -0.1115485564304456306, 0.1771653543307087075, -0.09757992244046823083 ) ) ;
#36460=CARTESIAN_POINT ( 'NONE',  ( -0.07874015748031421014, -0.1870078740157479769, 0.3641732283464567677 ) ) ;
#36461=CARTESIAN_POINT ( 'NONE',  ( 0.5446194225721792126, -0.08942795157528024563, -0.3641732283464568787 ) ) ;
#36462=CARTESIAN_POINT ( 'NONE',  ( 0.3740157480314966754, 0.1660481256975883668, -0.3530559997133364547 ) ) ;
#36463=CARTESIAN_POINT ( 'NONE',  ( -0.8727034120734901146, -0.2845877964562159024, 0.3641732283464567677 ) ) ;
#36465=CARTESIAN_POINT ( 'NONE',  ( 1.443569553805774897, 0.2306618581243848609, 0.2411417322834645549 ) ) ;
#36466=CARTESIAN_POINT ( 'NONE',  ( -0.8070866141732276899, 0.1660481256975883668, -0.3530559997133364547 ) ) ;
#36468=CARTESIAN_POINT ( 'NONE',  ( -0.1115485564304456306, 0.2952755905511810774, -0.1292274648535930714 ) ) ;
#36469=CARTESIAN_POINT ( 'NONE',  ( -0.6430446194225712953, 0.05413385826771626580, -0.4176697321401330321 ) ) ;
#36470=CARTESIAN_POINT ( 'NONE',  ( 1.299212598425197429, -0.5511811023622047445, 6.969142054262312111E-17 ) ) ;
#36471=CARTESIAN_POINT ( 'NONE',  ( 0.2296587926509192634, -0.08942795157528024563, -0.3641732283464568787 ) ) ;
#36472=CARTESIAN_POINT ( 'NONE',  ( -0.1640419947506555343, -0.3162353388693405765, 0.4822834645669290543 ) ) ;
#36473=CARTESIAN_POINT ( 'NONE',  ( -0.8464566929133852113, 0.1660481256975885056, 0.3530559997133364547 ) ) ;
#36474=CARTESIAN_POINT ( 'NONE',  ( -0.6155095129758836325, 1.955395699586894409, -0.5046436704918447758 ) ) ;
#36475=CARTESIAN_POINT ( 'NONE',  ( 1.555118110236221041, 0.07958543189024071263, -0.2665933059059888421 ) ) ;
#36476=CARTESIAN_POINT ( 'NONE',  ( 0.1377952755905518800, 0.1660481256975883668, -0.3530559997133364547 ) ) ;
#36480=CARTESIAN_POINT ( 'NONE',  ( 1.233595800524935227, -0.6046776061558807314, 0.2411417322834647770 ) ) ;
#36481=CARTESIAN_POINT ( 'NONE',  ( -0.4658792650918627265, -0.08942795157527998196, 0.3641732283464567121 ) ) ;
#36482=CARTESIAN_POINT ( 'NONE',  ( -0.4330708661417315697, 0.2952755905511811885, 0.000000000000000000 ) ) ;
#36483=CARTESIAN_POINT ( 'NONE',  ( 1.404199475065617708, 0.05413385826771626580, -0.4176697321401330321 ) ) ;
#36484=CARTESIAN_POINT ( 'NONE',  ( 0.8202099737532814183, -0.6692913385826773087, -0.1292274648535924053 ) ) ;
#36485=CARTESIAN_POINT ( 'NONE',  ( -1.496062992125983815, -0.1870078740157479769, 0.4822834645669291653 ) ) ;
#36486=CARTESIAN_POINT ( 'NONE',  ( -1.030183727034119867, -0.08942795157528024563, -0.3641732283464568787 ) ) ;
#36490=CARTESIAN_POINT ( 'NONE',  ( 1.522309711286089939, 0.1283753931104748280, 0.1820866141732283561 ) ) ;
#36491=CARTESIAN_POINT ( 'NONE',  ( 0.6233595800524939223, -0.2845877964562159024, 0.3641732283464567677 ) ) ;
#36492=CARTESIAN_POINT ( 'NONE',  ( 0.4855643044619428750, 0.05413385826771666132, 0.4176697321401328100 ) ) ;
#36493=CARTESIAN_POINT ( 'NONE',  ( 2.795275590551181466, 0.5118110236220471121, -3.234977217930338483E-16 ) ) ;
#36495=CARTESIAN_POINT ( 'NONE',  ( 0.6824146981627303710, -0.5023911411419708095, 0.1820866141732285504 ) ) ;
#36497=CARTESIAN_POINT ( 'NONE',  ( -0.3805774278215216522, 0.05413385826771666132, 0.4176697321401328100 ) ) ;
#36498=CARTESIAN_POINT ( 'NONE',  ( -0.8661417322834640276, -0.1870078740157479769, 0.4822834645669291653 ) ) ;
#36499=CARTESIAN_POINT ( 'NONE',  ( 1.154855643044620184, -0.6046776061558807314, 0.2411417322834647770 ) ) ;
#36502=CARTESIAN_POINT ( 'NONE',  ( -0.006561679790025524116, -0.2845877964562159024, 0.3641732283464567677 ) ) ;
#36505=VERTEX_POINT ( 'NONE', #77149 ) ;
#36507=CARTESIAN_POINT ( 'NONE',  ( -1.036745406824146176, 0.05413385826771626580, -0.4176697321401330321 ) ) ;
#36508=CARTESIAN_POINT ( 'NONE',  ( -0.06561679790026180015, 0.05413385826771666132, 0.4176697321401328100 ) ) ;
#36509=CARTESIAN_POINT ( 'NONE',  ( -0.4658792650918627265, -0.3162353388693409650, -0.4822834645669289433 ) ) ;
#36510=CARTESIAN_POINT ( 'NONE',  ( 0.4133858267716541968, 0.1660481256975885056, 0.3530559997133364547 ) ) ;
#36511=CARTESIAN_POINT ( 'NONE',  ( -0.6167979002624665030, -0.4281496062992127816, -0.4176697321401328100 ) ) ;
#36512=CARTESIAN_POINT ( 'NONE',  ( -1.213910761154854745, -0.6692913385826771977, 0.1292274648535927661 ) ) ;
#36513=CARTESIAN_POINT ( 'NONE',  ( -0.9383202099737524282, -0.05778040916215522460, 0.4822834645669289988 ) ) ;
#36514=CARTESIAN_POINT ( 'NONE',  ( 0.9186351706036751663, -0.6046776061558807314, 0.2411417322834647770 ) ) ;
#36515=CARTESIAN_POINT ( 'NONE',  ( 0.4593175853018379162, -0.4281496062992124485, 0.4176697321401328655 ) ) ;
#36517=CARTESIAN_POINT ( 'NONE',  ( -0.5314960629921250401, 0.07958543189024085140, 0.2665933059059887866 ) ) ;
#36518=EDGE_LOOP ( 'NONE', ( #57058, #57199, #60031, #52553 ) ) ;
#36521=CARTESIAN_POINT ( 'NONE',  ( -1.272965879265091305, -0.3690944881889763329, 0.3153832671262228327 ) ) ;
#36522=CARTESIAN_POINT ( 'NONE',  ( -0.3018372703412066094, -0.4281496062992127816, -0.4176697321401328100 ) ) ;
#36524=CARTESIAN_POINT ( 'NONE',  ( -0.7349081364829390672, 0.2306618581243847221, -0.2411417322834647770 ) ) ;
#36525=CARTESIAN_POINT ( 'NONE',  ( -0.6561679790026240244, -0.6046776061558807314, 0.2411417322834647770 ) ) ;
#36527=CARTESIAN_POINT ( 'NONE',  ( -1.640419947506561060, 0.05413385826771666132, 0.4176697321401328100 ) ) ;
#36529=CARTESIAN_POINT ( 'NONE',  ( 1.062992125984252745, 0.1771653543307087630, 0.000000000000000000 ) ) ;
#36531=CARTESIAN_POINT ( 'NONE',  ( -0.006561679790025524116, -0.2845877964562159024, 0.3641732283464567677 ) ) ;
#36532=CARTESIAN_POINT ( 'NONE',  ( -0.3477690288713902178, 0.2952755905511810774, -0.1292274648535930714 ) ) ;
#36533=CARTESIAN_POINT ( 'NONE',  ( 1.614173228346457378, 0.2952755905511811885, 0.000000000000000000 ) ) ;
#36534=CARTESIAN_POINT ( 'NONE',  ( 0.06561679790026316017, -0.4281496062992124485, 0.4176697321401328655 ) ) ;
#36535=VERTEX_POINT ( 'NONE', #46395 ) ;
#36540=CARTESIAN_POINT ( 'NONE',  ( 1.013613127888309595, -4.408777212815537393E-16, -0.4445507791589063395 ) ) ;
#36541=CARTESIAN_POINT ( 'NONE',  ( -0.8005249343832013809, -0.3690944881889763329, 0.3153832671262228327 ) ) ;
#36542=CARTESIAN_POINT ( 'NONE',  ( -1.167979002624671470, -0.4281496062992127816, -0.4176697321401328100 ) ) ;
#36544=CARTESIAN_POINT ( 'NONE',  ( 1.220472440944879722, 0.000000000000000000, 0.5309055118110233007 ) ) ;
#36546=CARTESIAN_POINT ( 'NONE',  ( 1.174540682414699111, -0.3162353388693405765, 0.4822834645669290543 ) ) ;
#36547=CARTESIAN_POINT ( 'NONE',  ( 0.2887139107611556010, -0.6046776061558807314, 0.2411417322834647770 ) ) ;
#36548=CARTESIAN_POINT ( 'NONE',  ( 0.6561679790026253567, -0.6046776061558809534, -0.2411417322834644161 ) ) ;
#36549=CARTESIAN_POINT ( 'NONE',  ( -0.6889763779527552368, 0.07958543189024085140, 0.2665933059059887866 ) ) ;
#36550=CARTESIAN_POINT ( 'NONE',  ( -0.3018372703412066094, 0.05413385826771666132, 0.4176697321401328100 ) ) ;
#36552=CARTESIAN_POINT ( 'NONE',  ( -0.9645669291338575535, -0.5400638737290844871, 0.3530559997133364547 ) ) ;
#36554=CARTESIAN_POINT ( 'NONE',  ( 1.299212598425197429, 0.1771653543307087630, 0.000000000000000000 ) ) ;
#36555=CARTESIAN_POINT ( 'NONE',  ( -0.3543307086614165824, -0.5511811023622047445, 6.969142054262312111E-17 ) ) ;
#36556=CARTESIAN_POINT ( 'NONE',  ( 1.122047244094488860, -0.4536011799217368745, -0.2665933059059886201 ) ) ;
#36557=CARTESIAN_POINT ( 'NONE',  ( -1.725721784776902190, -0.05778040916215522460, 0.4822834645669289988 ) ) ;
#36558=CARTESIAN_POINT ( 'NONE',  ( -1.069553805774277722, -0.5511811023622048555, -0.09757992244046775898 ) ) ;
#36559=CARTESIAN_POINT ( 'NONE',  ( 1.607611548556431069, 0.2952755905511811885, 0.1292274648535926551 ) ) ;
#36560=CARTESIAN_POINT ( 'NONE',  ( -0.9842519685039365918, -0.6692913385826771977, 8.415575281601705876E-17 ) ) ;
#36561=CARTESIAN_POINT ( 'NONE',  ( -0.4593175853018364174, -0.4281496062992127816, -0.4176697321401328100 ) ) ;
#36562=CARTESIAN_POINT ( 'NONE',  ( 0.2690288713910768403, 0.2952755905511811885, 0.1292274648535926551 ) ) ;
#36563=CARTESIAN_POINT ( 'NONE',  ( -0.2099737532808391705, 0.1283753931104748280, 0.1820866141732283561 ) ) ;
#36564=CARTESIAN_POINT ( 'NONE',  ( -1.561679790026246017, -0.004921259842519576551, 0.3153832671262227771 ) ) ;
#36565=CARTESIAN_POINT ( 'NONE',  ( 0.9514435695538062676, -0.3162353388693409650, -0.4822834645669289433 ) ) ;
#36567=CARTESIAN_POINT ( 'NONE',  ( 1.292650918635171564, 0.1771653543307087630, 0.09757992244046791164 ) ) ;
#36568=CARTESIAN_POINT ( 'NONE',  ( -0.9055118110236215490, 0.2952755905511811885, 0.000000000000000000 ) ) ;
#36569=CARTESIAN_POINT ( 'NONE',  ( -0.1640419947506553400, -0.08942795157528024563, -0.3641732283464568787 ) ) ;
#36570=DIRECTION ( 'NONE',  ( 3.096699300667737957E-16, -1.000000000000000000, 0.000000000000000000 ) ) ;
#36571=CARTESIAN_POINT ( 'NONE',  ( 0.3871391076115492380, -0.08942795157528024563, -0.3641732283464568787 ) ) ;
#36572=CARTESIAN_POINT ( 'NONE',  ( -0.1902887139107604098, 0.2952755905511810774, -0.1292274648535930714 ) ) ;
#36575=CARTESIAN_POINT ( 'NONE',  ( 0.7874015748031503170, -0.1870078740157479769, 0.3641732283464567677 ) ) ;
#36576=CARTESIAN_POINT ( 'NONE',  ( -0.1706036745406816491, 0.05413385826771626580, -0.4176697321401330321 ) ) ;
#36577=CARTESIAN_POINT ( 'NONE',  ( -0.8202099737532799750, 0.2952755905511810774, -0.1292274648535930714 ) ) ;
#36578=CARTESIAN_POINT ( 'NONE',  ( -0.8464566929133852113, 0.07958543189024085140, 0.2665933059059887866 ) ) ;
#36580=CARTESIAN_POINT ( 'NONE',  ( -0.5839895013123351797, -0.5511811023622046335, 0.09757992244046803654 ) ) ;
#36581=CARTESIAN_POINT ( 'NONE',  ( -0.1049868766404193215, -0.6046776061558807314, 0.2411417322834647770 ) ) ;
#36582=CARTESIAN_POINT ( 'NONE',  ( -0.9842519685039365918, -0.5511811023622047445, 6.969142054262312111E-17 ) ) ;
#36583=CARTESIAN_POINT ( 'NONE',  ( -1.404199475065615932, -0.4281496062992127816, -0.4176697321401328100 ) ) ;
#36584=CARTESIAN_POINT ( 'NONE',  ( 0.2234477481026895529, 0.004960608223778500969, -0.3437734562760191848 ) ) ;
#36586=CARTESIAN_POINT ( 'NONE',  ( -1.371391076115484831, 0.1771653543307087075, -0.09757992244046823083 ) ) ;
#36588=CARTESIAN_POINT ( 'NONE',  ( -0.3083989501312330295, -0.05778040916215522460, 0.4822834645669289988 ) ) ;
#36589=CARTESIAN_POINT ( 'NONE',  ( -1.017060367454067249, -0.05778040916215522460, 0.4822834645669289988 ) ) ;
#36592=CARTESIAN_POINT ( 'NONE',  ( 0.8858267716535438430, 0.1660481256975885056, 0.3530559997133364547 ) ) ;
#36593=CARTESIAN_POINT ( 'NONE',  ( 0.5249343832021005074, -0.6046776061558807314, 0.2411417322834647770 ) ) ;
#36596=CARTESIAN_POINT ( 'NONE',  ( 0.9908136482939640111, 0.1771653543307087075, -0.09757992244046823083 ) ) ;
#36599=CARTESIAN_POINT ( 'NONE',  ( -0.9120734908136475250, -0.5511811023622048555, -0.09757992244046775898 ) ) ;
#36601=ORIENTED_EDGE ( 'NONE', *, *, #17740, .T. ) ;
#36602=CARTESIAN_POINT ( 'NONE',  ( 0.2362204724409456558, -0.1870078740157480879, -0.4822834645669291653 ) ) ;
#36603=CARTESIAN_POINT ( 'NONE',  ( -0.3215223097112853146, -0.3162353388693405765, 0.4822834645669290543 ) ) ;
#36604=CARTESIAN_POINT ( 'NONE',  ( -1.095800524934382292, -0.3162353388693409650, -0.4822834645669289433 ) ) ;
#36605=CARTESIAN_POINT ( 'NONE',  ( 1.227034120734908917, 0.2952755905511810774, -0.1292274648535930714 ) ) ;
#36606=CARTESIAN_POINT ( 'NONE',  ( -1.272965879265091305, -0.004921259842519870586, -0.3153832671262229437 ) ) ;
#36607=LINE ( 'NONE', #16456, #21185 ) ;
#36608=CARTESIAN_POINT ( 'NONE',  ( -0.07874015748031421014, -0.1870078740157479769, 0.4822834645669291653 ) ) ;
#36609=CARTESIAN_POINT ( 'NONE',  ( -1.181102362204723644, -0.1870078740157479769, 0.4822834645669291653 ) ) ;
#36615=CARTESIAN_POINT ( 'NONE',  ( 0.7939632545931766261, -0.2845877964562161244, -0.3641732283464567121 ) ) ;
#36616=VERTEX_POINT ( 'NONE', #45557 ) ;
#36618=CARTESIAN_POINT ( 'NONE',  ( -0.7414698162729651543, -0.6692913385826771977, 0.1292274648535927661 ) ) ;
#36620=CARTESIAN_POINT ( 'NONE',  ( -0.1902887139107604098, -0.5511811023622046335, 0.09757992244046803654 ) ) ;
#36621=CARTESIAN_POINT ( 'NONE',  ( -1.404199475065615932, 0.05413385826771666132, 0.4176697321401328100 ) ) ;
#36622=CARTESIAN_POINT ( 'NONE',  ( 0.7217847769028878924, -0.4281496062992127816, -0.4176697321401328100 ) ) ;
#36623=CLOSED_SHELL ( 'NONE', ( #64958, #7374, #25752, #54935, #70733, #51735, #1821, #47944, #25333, #76522, #26848, #19885, #69142, #11075, #28052, #16220, #70674, #39242, #832, #75662, #68040, #5147, #77950, #43611, #77659, #82379, #81980, #40748, #50614, #78792, #15751, #14196, #60182, #14522, #48146, #11046, #59035, #54292, #51886, #39068, #59857, #6339, #74921, #72851, #49593, #18277, #12501, #14127, #73582, #71804, #64091, #77573, #3078, #47044, #66647, #66049, #61028, #5709, #58286, #24472, #7053, #23813, #2977, #45457, #58343, #39934, #309, #28884, #32150, #73262, #35010, #24462, #57649, #44305, #76875, #11664, #76847, #5941, #34915, #41318, #31832, #7728, #23210, #5737, #25393, #67534, #57858, #55403, #57842, #76353, #25465, #11498, #55879, #38874, #2362, #74437, #72839, #31144, #17528, #13143, #79426, #34691, #77306, #66262, #2188, #67096, #66697, #36794, #62011, #30890, #77379, #12279, #10915, #25890, #52736, #14702, #58774, #42821, #82319, #43048, #55731, #17187, #65609, #42977, #61218, #5469, #71477, #75798, #54272, #29285, #72193, #21036, #26888, #66171, #67147, #31018, #62738, #498, #43515, #3646, #80808, #34219, #29759, #65220, #13620, #43768, #69699, #8530, #16801, #49553, #36730, #43829, #70097, #70096, #4241, #73139, #5762, #51057, #20883, #54303, #79323, #81613, #78731, #2287, #39454, #83155, #45513, #70149 ) ) ;
#36624=CARTESIAN_POINT ( 'NONE',  ( 0.5118110236220478892, 0.2952755905511811885, 0.000000000000000000 ) ) ;
#36625=CARTESIAN_POINT ( 'NONE',  ( -0.3740157480314953431, -0.5400638737290845981, -0.3530559997133363437 ) ) ;
#36627=CARTESIAN_POINT ( 'NONE',  ( -0.6102362204724400829, -0.5400638737290845981, -0.3530559997133363437 ) ) ;
#36629=CARTESIAN_POINT ( 'NONE',  ( 1.259842519685040019, -0.1870078740157479769, 0.3641732283464567677 ) ) ;
#36630=CARTESIAN_POINT ( 'NONE',  ( -1.174540682414697335, -0.05778040916215522460, 0.4822834645669289988 ) ) ;
#36631=CARTESIAN_POINT ( 'NONE',  ( 0.7677165354330716118, 0.1660481256975883668, -0.3530559997133364547 ) ) ;
#36632=CARTESIAN_POINT ( 'NONE',  ( 1.069553805774278832, 0.2952755905511810774, -0.1292274648535930714 ) ) ;
#36635=CARTESIAN_POINT ( 'NONE',  ( -1.482939632545930975, -0.4281496062992127816, -0.4176697321401328100 ) ) ;
#36637=CARTESIAN_POINT ( 'NONE',  ( 0.3477690288713918276, 0.2952755905511811885, 0.1292274648535926551 ) ) ;
#36639=CARTESIAN_POINT ( 'NONE',  ( -1.528871391076114250, -0.5511811023622046335, 0.09757992244046803654 ) ) ;
#36640=CARTESIAN_POINT ( 'NONE',  ( 0.6889763779527566800, -0.4536011799217367080, 0.2665933059059888421 ) ) ;
#36641=CARTESIAN_POINT ( 'NONE',  ( 1.030183727034121421, -0.3162353388693409650, -0.4822834645669289433 ) ) ;
#36643=CARTESIAN_POINT ( 'NONE',  ( 0.8530183727034128527, -0.3690944881889763329, 0.3153832671262228327 ) ) ;
#36644=CARTESIAN_POINT ( 'NONE',  ( 0.6561679790026253567, 0.2306618581243848609, 0.2411417322834645549 ) ) ;
#36647=CARTESIAN_POINT ( 'NONE',  ( -0.8530183727034112984, -0.4281496062992127816, -0.4176697321401328100 ) ) ;
#36649=CARTESIAN_POINT ( 'NONE',  ( 0.9908136482939640111, 0.1771653543307087075, -0.09757992244046823083 ) ) ;
#36650=CARTESIAN_POINT ( 'NONE',  ( -0.6299212598425188991, -0.1870078740157479769, 0.4822834645669291653 ) ) ;
#36651=CARTESIAN_POINT ( 'NONE',  ( -0.03280839895013062252, -0.6692913385826771977, 0.1292274648535927661 ) ) ;
#36653=CARTESIAN_POINT ( 'NONE',  ( -0.2493438320209966919, 0.05413385826771626580, -0.4176697321401330321 ) ) ;
#36654=CARTESIAN_POINT ( 'NONE',  ( 0.2624671916010504757, 0.1283753931104748280, 0.1820866141732283561 ) ) ;
#36656=CARTESIAN_POINT ( 'NONE',  ( 0.07217847769028949700, -0.2845877964562159024, 0.3641732283464567677 ) ) ;
#36657=CARTESIAN_POINT ( 'NONE',  ( 0.7939632545931766261, -0.08942795157527998196, 0.3641732283464567121 ) ) ;
#36660=CARTESIAN_POINT ( 'NONE',  ( 0.4527559055118117182, 0.1660481256975883668, -0.3530559997133364547 ) ) ;
#36663=CARTESIAN_POINT ( 'NONE',  ( 1.443569553805774897, -0.5023911411419708095, -0.1820866141732282451 ) ) ;
#36664=CARTESIAN_POINT ( 'NONE',  ( 0.4824498642376759960, 1.223219560026271499E-15, 0.4445507791589056734 ) ) ;
#36665=CARTESIAN_POINT ( 'NONE',  ( -0.2427821522309703550, -0.08942795157528024563, -0.3641732283464568787 ) ) ;
#36666=CARTESIAN_POINT ( 'NONE',  ( -0.1706036745406816491, 0.05413385826771626580, -0.4176697321401330321 ) ) ;
#36667=CARTESIAN_POINT ( 'NONE',  ( 1.174540682414699111, -0.2845877964562159024, 0.3641732283464567677 ) ) ;
#36669=CARTESIAN_POINT ( 'NONE',  ( 1.384514435695538337, -0.5511811023622046335, 0.09757992244046803654 ) ) ;
#36670=CARTESIAN_POINT ( 'NONE',  ( -0.06561679790026180015, 0.05413385826771666132, 0.4176697321401328100 ) ) ;
#36671=CARTESIAN_POINT ( 'NONE',  ( 1.312335958005250269, -0.6046776061558807314, 0.2411417322834647770 ) ) ;
#36673=CARTESIAN_POINT ( 'NONE',  ( 0.03937007874015806264, 0.2952755905511811885, 0.000000000000000000 ) ) ;
#36674=CARTESIAN_POINT ( 'NONE',  ( 1.489501312335958172, -0.3162353388693405765, 0.4822834645669290543 ) ) ;
#36675=CARTESIAN_POINT ( 'NONE',  ( 0.4330708661417329575, 0.2952755905511811885, 0.000000000000000000 ) ) ;
#36677=CARTESIAN_POINT ( 'NONE',  ( 0.8923884514435703741, 0.1283753931104748280, 0.1820866141732283561 ) ) ;
#36678=CARTESIAN_POINT ( 'NONE',  ( 1.364829396325460076, 0.2306618581243848609, 0.2411417322834645549 ) ) ;
#36679=B_SPLINE_CURVE_WITH_KNOTS ( 'NONE', 3,
 ( #47145, #72835, #15185, #15603, #40842, #67358, #78329 ),
 .UNSPECIFIED., .F., .F.,
 ( 4, 3, 4 ),
 ( 3.642919299551294898E-17, 0.001246232571205267226, 0.002492492258783278024 ),
 .UNSPECIFIED. ) ;
#36680=CARTESIAN_POINT ( 'NONE',  ( 0.02624671916010564918, 0.1283753931104748280, 0.1820866141732283561 ) ) ;
#36681=CARTESIAN_POINT ( 'NONE',  ( -0.2755905511811015396, -0.6692913385826771977, 8.415575281601705876E-17 ) ) ;
#36682=CARTESIAN_POINT ( 'NONE',  ( 0.6955380577427828781, 0.05413385826771626580, -0.4176697321401330321 ) ) ;
#36683=CARTESIAN_POINT ( 'NONE',  ( -0.6824146981627288167, 0.2306618581243848609, 0.2411417322834645549 ) ) ;
#36684=VECTOR ( 'NONE', #70106, 39.37007874015748143 ) ;
#36685=CARTESIAN_POINT ( 'NONE',  ( -0.3346456692913377662, -0.4536011799217367080, 0.2665933059059888421 ) ) ;
#36686=CARTESIAN_POINT ( 'NONE',  ( 0.5971128608923890191, -0.6692913385826771977, 0.1292274648535927661 ) ) ;
#36687=CARTESIAN_POINT ( 'NONE',  ( 1.017060367454068803, -0.2845877964562159024, 0.3641732283464567677 ) ) ;
#36688=CARTESIAN_POINT ( 'NONE',  ( 0.09186351706036827158, 0.05413385826771666132, 0.4176697321401328100 ) ) ;
#36692=CARTESIAN_POINT ( 'NONE',  ( -0.4624320255261038515, -2.191421614605370878E-15, 0.4445507791589071167 ) ) ;
#36694=CARTESIAN_POINT ( 'NONE',  ( -1.141732283464566011, 0.2952755905511811885, 0.000000000000000000 ) ) ;
#36695=CARTESIAN_POINT ( 'NONE',  ( -0.4921259842519677963, -0.5400638737290844871, 0.3530559997133364547 ) ) ;
#36698=ORIENTED_EDGE ( 'NONE', *, *, #815, .T. ) ;
#36699=CARTESIAN_POINT ( 'NONE',  ( 0.1968503937007881344, -0.5511811023622047445, 6.969142054262312111E-17 ) ) ;
#36702=CARTESIAN_POINT ( 'NONE',  ( 0.5249343832021003964, 0.2306618581243847221, -0.2411417322834647770 ) ) ;
#36705=CARTESIAN_POINT ( 'NONE',  ( -1.666666666666665853, -0.004921259842519870586, -0.3153832671262229437 ) ) ;
#36706=CARTESIAN_POINT ( 'NONE',  ( 1.076115485564305141, 0.2306618581243847221, -0.2411417322834647770 ) ) ;
#36707=CARTESIAN_POINT ( 'NONE',  ( 1.456692913385827515, 0.1771653543307087630, 0.000000000000000000 ) ) ;
#36708=CARTESIAN_POINT ( 'NONE',  ( 0.06561679790026316017, -0.4281496062992124485, 0.4176697321401328655 ) ) ;
#36710=CARTESIAN_POINT ( 'NONE',  ( -0.3412073490813641308, 0.2306618581243847221, -0.2411417322834647770 ) ) ;
#36711=CARTESIAN_POINT ( 'NONE',  ( -1.102362204724408601, -0.1870078740157479769, 0.3641732283464567677 ) ) ;
#36712=CARTESIAN_POINT ( 'NONE',  ( 0.5643044619422579178, -0.4281496062992127816, -0.4176697321401328100 ) ) ;
#36713=CARTESIAN_POINT ( 'NONE',  ( -0.6561679790026240244, -0.6046776061558807314, 0.2411417322834647770 ) ) ;
#36714=CARTESIAN_POINT ( 'NONE',  ( -1.191801538614237099, -5.582469467804009507E-15, -0.4118484887281986251 ) ) ;
#36716=ORIENTED_EDGE ( 'NONE', *, *, #47083, .F. ) ;
#36718=CARTESIAN_POINT ( 'NONE',  ( 0.3805774278215230400, -0.4281496062992124485, 0.4176697321401328655 ) ) ;
#36719=CARTESIAN_POINT ( 'NONE',  ( -0.1902887139107604098, -0.6692913385826771977, 0.1292274648535927661 ) ) ;
#36720=CARTESIAN_POINT ( 'NONE',  ( -1.443569553805773564, 0.2306618581243847221, -0.2411417322834647770 ) ) ;
#36721=CARTESIAN_POINT ( 'NONE',  ( 1.259842519685040019, -0.1870078740157479769, 0.4822834645669291653 ) ) ;
#36722=CARTESIAN_POINT ( 'NONE',  ( 0.3083989501312343062, -0.05778040916215560624, -0.4822834645669293319 ) ) ;
#36724=CARTESIAN_POINT ( 'NONE',  ( -0.8595800524934373854, -0.3162353388693409650, -0.4822834645669289433 ) ) ;
#36725=CARTESIAN_POINT ( 'NONE',  ( 0.3477690288713918276, -0.6692913385826773087, -0.1292274648535924053 ) ) ;
#36726=CARTESIAN_POINT ( 'NONE',  ( -0.4790026246719152336, -0.05778040916215560624, -0.4822834645669293319 ) ) ;
#36727=CARTESIAN_POINT ( 'NONE',  ( 0.4068241469816281097, -0.004921259842519576551, 0.3153832671262227771 ) ) ;
#36728=CARTESIAN_POINT ( 'NONE',  ( 1.574803149606299746, -0.1870078740157480601, -0.3641732283464567677 ) ) ;
#36730=ADVANCED_FACE ( 'NONE', ( #14854 ), #39821, .F. ) ;
#36731=CARTESIAN_POINT ( 'NONE',  ( 0.1509186351706042484, -0.3162353388693405765, 0.4822834645669290543 ) ) ;
#36733=CARTESIAN_POINT ( 'NONE',  ( 1.555118110236221041, -0.5400638737290844871, 0.3530559997133364547 ) ) ;
#36735=ORIENTED_EDGE ( 'NONE', *, *, #59271, .T. ) ;
#36737=CARTESIAN_POINT ( 'NONE',  ( 0.8595800524934390507, -0.3162353388693405765, 0.4822834645669290543 ) ) ;
#36738=CARTESIAN_POINT ( 'NONE',  ( 0.1771653543307093182, 0.07958543189024085140, 0.2665933059059887866 ) ) ;
#36743=CARTESIAN_POINT ( 'NONE',  ( 0.7201575634750010391, 1.521610601467410833E-15, 0.3791483426435167670 ) ) ;
#36745=CARTESIAN_POINT ( 'NONE',  ( 0.6036745406824153282, -0.6046776061558807314, 0.2411417322834647770 ) ) ;
#36746=CARTESIAN_POINT ( 'NONE',  ( -1.246719160104985846, -0.4281496062992127816, -0.4176697321401328100 ) ) ;
#36747=AXIS2_PLACEMENT_3D ( 'NONE', #71056, #39053, #77370 ) ;
#36748=CARTESIAN_POINT ( 'NONE',  ( -1.227034120734907585, 0.2952755905511811885, 0.1292274648535926551 ) ) ;
#36749=CARTESIAN_POINT ( 'NONE',  ( 0.8661417322834652488, -0.1870078740157480879, -0.4822834645669291653 ) ) ;
#36750=CARTESIAN_POINT ( 'NONE',  ( 1.423884514435696191, -0.05778040916215522460, 0.4822834645669289988 ) ) ;
#36751=CARTESIAN_POINT ( 'NONE',  ( 1.450131233595801428, -0.5511811023622048555, -0.09757992244046775898 ) ) ;
#36753=CARTESIAN_POINT ( 'NONE',  ( 1.135170603674541256, -0.5511811023622048555, -0.09757992244046775898 ) ) ;
#36754=CARTESIAN_POINT ( 'NONE',  ( -0.7874015748031489847, -0.1870078740157480879, -0.4822834645669291653 ) ) ;
#36756=CARTESIAN_POINT ( 'NONE',  ( 1.417322834645670104, -0.1870078740157480879, -0.4822834645669291653 ) ) ;
#36758=CARTESIAN_POINT ( 'NONE',  ( -0.3740157480314953431, 0.1660481256975885056, 0.3530559997133364547 ) ) ;
#36759=CARTESIAN_POINT ( 'NONE',  ( 1.325459317585302665, -0.4281496062992124485, 0.4176697321401328655 ) ) ;
#36760=CARTESIAN_POINT ( 'NONE',  ( 0.4768132735438215253, 1.796500554427757690, -0.5050878842330656093 ) ) ;
#36761=CARTESIAN_POINT ( 'NONE',  ( -1.069553805774277722, 0.1771653543307087630, 0.09757992244046791164 ) ) ;
#36762=CARTESIAN_POINT ( 'NONE',  ( 0.2887139107611556010, 0.2306618581243847221, -0.2411417322834647770 ) ) ;
#36763=CARTESIAN_POINT ( 'NONE',  ( 0.9120734908136489683, -0.5511811023622046335, 0.09757992244046803654 ) ) ;
#36766=CARTESIAN_POINT ( 'NONE',  ( -1.115485564304461219, -0.3690944881889763329, 0.3153832671262228327 ) ) ;
#36767=CARTESIAN_POINT ( 'NONE',  ( 0.7545931758530189937, 0.2952755905511810774, -0.1292274648535930714 ) ) ;
#36769=CARTESIAN_POINT ( 'NONE',  ( -0.4724409448818890911, -0.1870078740157479769, 0.3641732283464567677 ) ) ;
#36770=CARTESIAN_POINT ( 'NONE',  ( -0.2230971128608915943, -0.4281496062992127816, -0.4176697321401328100 ) ) ;
#36771=CARTESIAN_POINT ( 'NONE',  ( -1.482939632545930975, -0.004921259842519576551, 0.3153832671262227771 ) ) ;
#36772=CARTESIAN_POINT ( 'NONE',  ( -0.8333333333333323711, -0.6692913385826773087, -0.1292274648535924053 ) ) ;
#36773=CARTESIAN_POINT ( 'NONE',  ( 1.292650918635171564, -0.6692913385826773087, -0.1292274648535924053 ) ) ;
#36775=CARTESIAN_POINT ( 'NONE',  ( -0.7939632545931750718, -0.08942795157528024563, -0.3641732283464568787 ) ) ;
#36777=CARTESIAN_POINT ( 'NONE',  ( 1.430446194225722500, 0.05413385826771666132, 0.4176697321401328100 ) ) ;
#36779=CARTESIAN_POINT ( 'NONE',  ( -1.358267716535432434, 0.1660481256975883668, -0.3530559997133364547 ) ) ;
#36780=CARTESIAN_POINT ( 'NONE',  ( 1.686351706036745890, 0.2952755905511811885, 0.1292274648535926551 ) ) ;
#36781=CARTESIAN_POINT ( 'NONE',  ( -0.7874015748031489847, -0.1870078740157479769, 0.3641732283464567677 ) ) ;
#36782=EDGE_CURVE ( 'NONE', #6582, #17097, #73978, .T. ) ;
#36783=CARTESIAN_POINT ( 'NONE',  ( 0.4935044252197980930, 1.488513638086841118, 0.5309055118110234117 ) ) ;
#36784=CARTESIAN_POINT ( 'NONE',  ( -0.006561679790025524116, -0.05778040916215560624, -0.4822834645669293319 ) ) ;
#36785=CARTESIAN_POINT ( 'NONE',  ( 0.05905511811023709395, -0.4536011799217367080, 0.2665933059059888421 ) ) ;
#36786=CARTESIAN_POINT ( 'NONE',  ( -1.279527559055116948, -0.4536011799217367080, 0.2665933059059888421 ) ) ;
#36787=CARTESIAN_POINT ( 'NONE',  ( -1.358267716535432434, 0.1660481256975883668, -0.3530559997133364547 ) ) ;
#36788=CARTESIAN_POINT ( 'NONE',  ( 1.174540682414699111, -0.08942795157528024563, -0.3641732283464568787 ) ) ;
#36789=CARTESIAN_POINT ( 'NONE',  ( 1.036745406824147731, 0.05413385826771666132, 0.4176697321401328100 ) ) ;
#36791=CARTESIAN_POINT ( 'NONE',  ( 0.4199475065616805614, 0.1283753931104748280, 0.1820866141732283561 ) ) ;
#36793=CARTESIAN_POINT ( 'NONE',  ( 1.043307086614173818, 0.1660481256975885056, 0.3530559997133364547 ) ) ;
#36794=ADVANCED_FACE ( 'NONE', ( #40325 ), #80211, .F. ) ;
#36795=CARTESIAN_POINT ( 'NONE',  ( 0.8923884514435701520, -0.5023911411419708095, -0.1820866141732282451 ) ) ;
#36796=VERTEX_POINT ( 'NONE', #32609 ) ;
#36797=CARTESIAN_POINT ( 'NONE',  ( -1.410761154855641575, -0.3162353388693409650, -0.4822834645669289433 ) ) ;
#36798=CARTESIAN_POINT ( 'NONE',  ( -0.7349081364829387342, -0.6046776061558807314, 0.2411417322834647770 ) ) ;
#36799=CARTESIAN_POINT ( 'NONE',  ( -0.1706036745406816491, -0.4281496062992124485, 0.4176697321401328655 ) ) ;
#36802=CARTESIAN_POINT ( 'NONE',  ( 0.6561679790026253567, 0.2306618581243848609, 0.2411417322834645549 ) ) ;
#36803=CARTESIAN_POINT ( 'NONE',  ( 1.601049868766404982, 0.1283753931104748280, 0.1820866141732283561 ) ) ;
#36804=CARTESIAN_POINT ( 'NONE',  ( 0.05905511811023709395, -0.5400638737290844871, 0.3530559997133364547 ) ) ;
#36805=CARTESIAN_POINT ( 'NONE',  ( 0.9251968503937015864, -0.5400638737290844871, 0.3530559997133364547 ) ) ;
#36812=CARTESIAN_POINT ( 'NONE',  ( -0.5118110236220466680, -0.5511811023622047445, 6.969142054262312111E-17 ) ) ;
#36813=CARTESIAN_POINT ( 'NONE',  ( -0.8792650918635160906, 0.05413385826771626580, -0.4176697321401330321 ) ) ;
#36814=CARTESIAN_POINT ( 'NONE',  ( 0.3740157480314966754, 0.1660481256975883668, -0.3530559997133364547 ) ) ;
#36816=EDGE_CURVE ( 'NONE', #57928, #3606, #28310, .T. ) ;
#36817=CARTESIAN_POINT ( 'NONE',  ( 0.7742782152230979209, 0.05413385826771626580, -0.4176697321401330321 ) ) ;
#36818=CARTESIAN_POINT ( 'NONE',  ( 1.502624671916010790, -0.3162353388693409650, -0.4822834645669289433 ) ) ;
#36819=CARTESIAN_POINT ( 'NONE',  ( 1.299212598425197429, 0.2952755905511811885, 0.000000000000000000 ) ) ;
#36822=FACE_OUTER_BOUND ( 'NONE', #78598, .T. ) ;
#36823=CARTESIAN_POINT ( 'NONE',  ( 1.010498687664042716, 0.05413385826771626580, -0.4176697321401330321 ) ) ;
#36824=CARTESIAN_POINT ( 'NONE',  ( 0.5118110236220478892, 0.2952755905511811885, 0.000000000000000000 ) ) ;
#36825=EDGE_CURVE ( 'NONE', #20402, #1757, #49313, .T. ) ;
#36827=CARTESIAN_POINT ( 'NONE',  ( 1.253280839895013710, -0.2845877964562159024, 0.3641732283464567677 ) ) ;
#36828=CARTESIAN_POINT ( 'NONE',  ( -1.509186351706035767, -0.3690944881889763329, 0.3153832671262228327 ) ) ;
#36829=CARTESIAN_POINT ( 'NONE',  ( 1.515748031496063186, -0.5400638737290845981, -0.3530559997133363437 ) ) ;
#36832=CARTESIAN_POINT ( 'NONE',  ( 0.7086614173228353852, -0.1870078740157479769, 0.4822834645669291653 ) ) ;
#36833=CARTESIAN_POINT ( 'NONE',  ( 1.522309711286089939, 0.1283753931104748280, 0.1820866141732283561 ) ) ;
#36834=CARTESIAN_POINT ( 'NONE',  ( -0.4461942257217840213, 0.2306618581243848609, 0.2411417322834645549 ) ) ;
#36835=CARTESIAN_POINT ( 'NONE',  ( -0.7152230971128602510, -0.05778040916215560624, -0.4822834645669293319 ) ) ;
#36836=CARTESIAN_POINT ( 'NONE',  ( 1.384514435695538337, -0.6692913385826771977, 0.1292274648535927661 ) ) ;
#36841=CARTESIAN_POINT ( 'NONE',  ( 1.653543307086614789, -0.1870078740157479769, 0.4822834645669291653 ) ) ;
#36844=VERTEX_POINT ( 'NONE', #65454 ) ;
#36845=DIRECTION ( 'NONE',  ( -0.6427876096865343669, 0.7660444431189822323, 0.000000000000000000 ) ) ;
#36846=CARTESIAN_POINT ( 'NONE',  ( 1.423884514435696191, -0.08942795157527998196, 0.3641732283464567121 ) ) ;
#36853=CARTESIAN_POINT ( 'NONE',  ( -0.8398950131233585692, 0.1283753931104748280, 0.1820866141732283561 ) ) ;
#36854=CARTESIAN_POINT ( 'NONE',  ( -1.023622047244094002, -0.1870078740157480601, -0.3641732283464567677 ) ) ;
#36855=CARTESIAN_POINT ( 'NONE',  ( 0.7086614173228352742, -0.1870078740157480879, -0.4822834645669291653 ) ) ;
#36856=CARTESIAN_POINT ( 'NONE',  ( -1.148293963254592542, 0.2952755905511811885, 0.1292274648535926551 ) ) ;
#36859=CARTESIAN_POINT ( 'NONE',  ( 1.528871391076116026, -0.6692913385826773087, -0.1292274648535924053 ) ) ;
#36865=CARTESIAN_POINT ( 'NONE',  ( -1.076115485564303809, -0.6046776061558809534, -0.2411417322834644161 ) ) ;
#36866=CARTESIAN_POINT ( 'NONE',  ( 0.8136482939632553313, -0.6046776061558809534, -0.2411417322834644161 ) ) ;
#36868=CARTESIAN_POINT ( 'NONE',  ( 0.6627296587926515548, 0.2066929133858267931, 0.1054918080437490802 ) ) ;
#36870=CARTESIAN_POINT ( 'NONE',  ( -1.207349081364828880, 0.2306618581243847221, -0.2411417322834647770 ) ) ;
#36872=CARTESIAN_POINT ( 'NONE',  ( -0.04593175853018302557, -0.5511811023622048555, -0.09757992244046775898 ) ) ;
#36874=AXIS2_PLACEMENT_3D ( 'NONE', #17939, #75186, #17532 ) ;
#36875=CARTESIAN_POINT ( 'NONE',  ( -0.03280839895013062252, 0.1771653543307087075, -0.09757992244046823083 ) ) ;
#36876=CARTESIAN_POINT ( 'NONE',  ( 0.4396325459317590445, -0.5511811023622046335, 0.09757992244046803654 ) ) ;
#36877=CARTESIAN_POINT ( 'NONE',  ( 0.3805774278215230400, 0.05413385826771626580, -0.4176697321401330321 ) ) ;
#36878=CARTESIAN_POINT ( 'NONE',  ( -0.8989501312335946848, -0.5511811023622046335, 0.09757992244046803654 ) ) ;
#36880=CARTESIAN_POINT ( 'NONE',  ( 1.463254593175853824, 0.2952755905511810774, -0.1292274648535930714 ) ) ;
#36881=CARTESIAN_POINT ( 'NONE',  ( -1.056430446194224881, -0.6692913385826771977, 0.1292274648535927661 ) ) ;
#36883=CARTESIAN_POINT ( 'NONE',  ( -0.1574803149606292529, -0.1870078740157479769, 0.4822834645669291653 ) ) ;
#36885=CARTESIAN_POINT ( 'NONE',  ( -0.3674540682414689785, 0.2306618581243848609, 0.2411417322834645549 ) ) ;
#36886=CARTESIAN_POINT ( 'NONE',  ( 1.430446194225722500, -0.3690944881889765550, -0.3153832671262227771 ) ) ;
#36888=CARTESIAN_POINT ( 'NONE',  ( 0.1574803149606306130, -0.1870078740157479769, 0.3641732283464567677 ) ) ;
#36889=CARTESIAN_POINT ( 'NONE',  ( -0.1246719160104980823, 0.2952755905511811885, 0.1292274648535926551 ) ) ;
#36890=CARTESIAN_POINT ( 'NONE',  ( -1.351706036745406347, -0.4281496062992124485, 0.4176697321401328655 ) ) ;
#36891=CARTESIAN_POINT ( 'NONE',  ( -0.6575345472709128725, 1.929133858267715773, -0.5309055118110235227 ) ) ;
#36892=CARTESIAN_POINT ( 'NONE',  ( 1.633858267716535639, -0.4536011799217367080, 0.2665933059059888421 ) ) ;
#36893=CARTESIAN_POINT ( 'NONE',  ( -0.09186351706036663400, -0.4281496062992124485, 0.4176697321401328655 ) ) ;
#36896=CARTESIAN_POINT ( 'NONE',  ( 1.364829396325459854, -0.6046776061558809534, -0.2411417322834644161 ) ) ;
#36897=CARTESIAN_POINT ( 'NONE',  ( -0.7545931758530177724, 0.1771653543307087630, 0.09757992244046791164 ) ) ;
#36898=CARTESIAN_POINT ( 'NONE',  ( -0.4199475065616791736, 0.2306618581243847221, -0.2411417322834647770 ) ) ;
#36899=CARTESIAN_POINT ( 'NONE',  ( 1.318897637795276356, -0.5400638737290844871, 0.3530559997133364547 ) ) ;
#36900=CARTESIAN_POINT ( 'NONE',  ( 0.8464566929133866546, -0.5400638737290844871, 0.3530559997133364547 ) ) ;
#36901=CARTESIAN_POINT ( 'NONE',  ( -1.528871391076114250, -0.6692913385826771977, 0.1292274648535927661 ) ) ;
#36902=CARTESIAN_POINT ( 'NONE',  ( -1.167979002624671470, -0.3690944881889765550, -0.3153832671262227771 ) ) ;
#36907=CARTESIAN_POINT ( 'NONE',  ( 1.581364829396326277, -0.2845877964562161244, -0.3641732283464567121 ) ) ;
#36908=CARTESIAN_POINT ( 'NONE',  ( 0.9317585301837276734, -0.3690944881889763329, 0.3153832671262228327 ) ) ;
#36909=CARTESIAN_POINT ( 'NONE',  ( 0.3412073490813655186, 0.2306618581243848609, 0.2411417322834645549 ) ) ;
#36912=CARTESIAN_POINT ( 'NONE',  ( 0.6102362204724416372, 0.07958543189024071263, -0.2665933059059888421 ) ) ;
#36913=CARTESIAN_POINT ( 'NONE',  ( -0.3280839895013117347, 0.05413385826771626580, -0.4176697321401330321 ) ) ;
#36914=CARTESIAN_POINT ( 'NONE',  ( -0.7480314960629914633, -0.6692913385826771977, 8.415575281601705876E-17 ) ) ;
#36915=CARTESIAN_POINT ( 'NONE',  ( 1.227034120734908917, 0.2952755905511810774, -0.1292274648535930714 ) ) ;
#36918=CARTESIAN_POINT ( 'NONE',  ( 0.1377952755905518800, -0.4536011799217367080, 0.2665933059059888421 ) ) ;
#36919=ORIENTED_EDGE ( 'NONE', *, *, #60874, .F. ) ;
#36922=CARTESIAN_POINT ( 'NONE',  ( -1.062992125984250968, 0.2952755905511811885, 0.000000000000000000 ) ) ;
#36923=CARTESIAN_POINT ( 'NONE',  ( -0.2427821522309703550, -0.3162353388693405765, 0.4822834645669290543 ) ) ;
#36924=CARTESIAN_POINT ( 'NONE',  ( -0.4921259842519677963, 0.1660481256975883668, -0.3530559997133364547 ) ) ;
#36925=CARTESIAN_POINT ( 'NONE',  ( 0.6955380577427828781, -0.004921259842519870586, -0.3153832671262229437 ) ) ;
#36926=CARTESIAN_POINT ( 'NONE',  ( 0.2755905511811031494, 0.2952755905511811885, 0.000000000000000000 ) ) ;
#36927=CARTESIAN_POINT ( 'NONE',  ( -0.3543307086614165824, 0.2952755905511811885, 0.000000000000000000 ) ) ;
#36928=CARTESIAN_POINT ( 'NONE',  ( -1.266404199475064773, -0.05778040916215560624, -0.4822834645669293319 ) ) ;
#36929=CARTESIAN_POINT ( 'NONE',  ( -0.7677165354330699465, 0.1660481256975885056, 0.3530559997133364547 ) ) ;
#36930=CARTESIAN_POINT ( 'NONE',  ( 0.8398950131233602345, 0.2306618581243847221, -0.2411417322834647770 ) ) ;
#36932=CARTESIAN_POINT ( 'NONE',  ( -0.2427821522309703550, -0.2845877964562159024, 0.3641732283464567677 ) ) ;
#36935=ORIENTED_EDGE ( 'NONE', *, *, #31097, .F. ) ;
#36936=CARTESIAN_POINT ( 'NONE',  ( -1.397637795275589623, 0.07958543189024085140, 0.2665933059059887866 ) ) ;
#36937=CARTESIAN_POINT ( 'NONE',  ( -1.017060367454067249, -0.05778040916215522460, 0.4822834645669289988 ) ) ;
#36938=CARTESIAN_POINT ( 'NONE',  ( -0.9120734908136475250, -0.6692913385826773087, -0.1292274648535924053 ) ) ;
#36940=CARTESIAN_POINT ( 'NONE',  ( -0.6561679790026240244, -0.6046776061558807314, 0.2411417322834647770 ) ) ;
#36941=CARTESIAN_POINT ( 'NONE',  ( -0.7086614173228339419, -0.1870078740157480879, -0.4822834645669291653 ) ) ;
#36942=DIRECTION ( 'NONE',  ( -0.8479387356305996271, -2.625811289636364142E-16, -0.5300942374872417151 ) ) ;
#36943=CARTESIAN_POINT ( 'NONE',  ( 0.5411721830064198935, 8.471767977567108961E-16, -0.4445507791589058955 ) ) ;
#36945=CARTESIAN_POINT ( 'NONE',  ( 0.4790026246719168435, -0.2845877964562161244, -0.3641732283464567121 ) ) ;
#36946=CARTESIAN_POINT ( 'NONE',  ( 1.595398199321655275, 1.013096522517429987, -0.1559797534342494130 ) ) ;
#36948=CARTESIAN_POINT ( 'NONE',  ( 0.2362204724409456558, -0.1870078740157480601, -0.3641732283464567677 ) ) ;
#36949=CARTESIAN_POINT ( 'NONE',  ( -0.3543307086614165824, 0.2952755905511811885, 0.000000000000000000 ) ) ;
#36950=CARTESIAN_POINT ( 'NONE',  ( 1.581364829396326277, -0.05778040916215522460, 0.4822834645669289988 ) ) ;
#36951=CARTESIAN_POINT ( 'NONE',  ( 0.1115485564304470323, 0.2952755905511811885, 0.1292274648535926551 ) ) ;
#36957=CARTESIAN_POINT ( 'NONE',  ( 1.561679790026247350, -0.4281496062992124485, 0.4176697321401328655 ) ) ;
#36958=CARTESIAN_POINT ( 'NONE',  ( -0.9186351706036736120, 0.1283753931104748280, 0.1820866141732283561 ) ) ;
#36959=CARTESIAN_POINT ( 'NONE',  ( -0.9776902887139098386, -0.6692913385826771977, 0.1292274648535927661 ) ) ;
#36963=CARTESIAN_POINT ( 'NONE',  ( 1.377952755905512472, 0.2952755905511811885, 0.000000000000000000 ) ) ;
#36964=CARTESIAN_POINT ( 'NONE',  ( 0.2559055118110243332, -0.5400638737290845981, -0.3530559997133363437 ) ) ;
#36965=CARTESIAN_POINT ( 'NONE',  ( 0.3871391076115493490, -0.3162353388693405765, 0.4822834645669290543 ) ) ;
#36966=CARTESIAN_POINT ( 'NONE',  ( -1.227034120734907141, -0.5511811023622048555, -0.09757992244046775898 ) ) ;
#36967=CARTESIAN_POINT ( 'NONE',  ( -0.2165354330708654795, -0.5400638737290845981, -0.3530559997133363437 ) ) ;
#36969=CARTESIAN_POINT ( 'NONE',  ( -0.9383202099737524282, -0.05778040916215522460, 0.4822834645669289988 ) ) ;
#36971=CARTESIAN_POINT ( 'NONE',  ( 1.502624671916010790, -0.2845877964562161244, -0.3641732283464567121 ) ) ;
#36972=CARTESIAN_POINT ( 'NONE',  ( -0.4330708661417315697, 0.1771653543307087630, 0.000000000000000000 ) ) ;
#36973=CARTESIAN_POINT ( 'NONE',  ( 1.351706036745407680, -0.004921259842519576551, 0.3153832671262227771 ) ) ;
#36974=CARTESIAN_POINT ( 'NONE',  ( 1.581364829396326277, -0.08942795157527998196, 0.3641732283464567121 ) ) ;
#36975=CARTESIAN_POINT ( 'NONE',  ( -1.115485564304461219, -0.004921259842519870586, -0.3153832671262229437 ) ) ;
#36977=CARTESIAN_POINT ( 'NONE',  ( 0.7152230971128616943, -0.08942795157527998196, 0.3641732283464567121 ) ) ;
#36978=CARTESIAN_POINT ( 'NONE',  ( -0.5446194225721777693, -0.05778040916215522460, 0.4822834645669289988 ) ) ;
#36980=CARTESIAN_POINT ( 'NONE',  ( -0.2887139107611542133, -0.5023911411419708095, -0.1820866141732282451 ) ) ;
#36981=CARTESIAN_POINT ( 'NONE',  ( -1.614173228346456268, -0.5511811023622047445, 6.969142054262312111E-17 ) ) ;
#36982=( BOUNDED_CURVE ( )  B_SPLINE_CURVE ( 2, ( #65442, #25440, #58682, #51106, #6512, #38495, #76803, #13260, #39746, #32182, #71322, #39323, #7344 ),
 .UNSPECIFIED., .F., .F. ) 
 B_SPLINE_CURVE_WITH_KNOTS ( ( 3, 2, 2, 2, 2, 2, 3 ),
 ( 0.4915129128166190742, 0.4924242424242424310, 0.4962121212121212155, 0.5000000000000000000, 0.5037878787878787845, 0.5075757575757575690, 0.5084870871833810924 ),
 .UNSPECIFIED. ) 
 CURVE ( )  GEOMETRIC_REPRESENTATION_ITEM ( )  RATIONAL_B_SPLINE_CURVE ( ( 0.9875488213027530104, 0.9918020599134685922, 1.000000000000000000, 0.9659258262890683122, 1.000000000000000000, 0.9659258262890683122, 1.000000000000000000, 0.9659258262890683122, 1.000000000000000000, 0.9659258262890683122, 1.000000000000000000, 0.9918020599134671489, 0.9875488213027514561 ) ) 
 REPRESENTATION_ITEM ( '' )  );
#36984=CARTESIAN_POINT ( 'NONE',  ( 0.8989501312335964611, 0.2952755905511811885, 0.1292274648535926551 ) ) ;
#36985=CARTESIAN_POINT ( 'NONE',  ( 0.6955380577427828781, 0.05413385826771626580, -0.4176697321401330321 ) ) ;
#36986=CARTESIAN_POINT ( 'NONE',  ( 1.167979002624672580, -0.004921259842519870586, -0.3153832671262229437 ) ) ;
#36987=CARTESIAN_POINT ( 'NONE',  ( -1.102362204724408601, -0.1870078740157479769, 0.4822834645669291653 ) ) ;
#36988=CARTESIAN_POINT ( 'NONE',  ( -0.1706036745406816491, -0.004921259842519870586, -0.3153832671262229437 ) ) ;
#36989=CARTESIAN_POINT ( 'NONE',  ( -1.614173228346457378, 0.9921945702958913094, 0.1372047244094476981 ) ) ;
#36990=CARTESIAN_POINT ( 'NONE',  ( 0.3937007874015754361, -0.1870078740157480601, -0.3641732283464567677 ) ) ;
#36991=CARTESIAN_POINT ( 'NONE',  ( -0.3871391076115476282, -0.05778040916215522460, 0.4822834645669289988 ) ) ;
#36994=CARTESIAN_POINT ( 'NONE',  ( 0.5511811023622054106, -0.1870078740157480601, -0.3641732283464567677 ) ) ;
#36995=CARTESIAN_POINT ( 'NONE',  ( -0.2821522309711278487, -0.6692913385826773087, -0.1292274648535924053 ) ) ;
#36997=CARTESIAN_POINT ( 'NONE',  ( -0.6692913385826764205, 0.2952755905511811885, 0.000000000000000000 ) ) ;
#36998=CARTESIAN_POINT ( 'NONE',  ( -0.6430446194225712953, -0.004921259842519870586, -0.3153832671262229437 ) ) ;
#37000=CARTESIAN_POINT ( 'NONE',  ( 0.03937007874015833325, -0.6692913385826771977, 8.415575281601705876E-17 ) ) ;
#37001=CARTESIAN_POINT ( 'NONE',  ( -1.122047244094487306, -0.4536011799217367080, 0.2665933059059888421 ) ) ;
#37002=CONICAL_SURFACE ( 'NONE', #73318, 1.220472440944881942, 0.7853981633974621568 ) ;
#37003=CARTESIAN_POINT ( 'NONE',  ( -1.528871391076114250, -0.6692913385826771977, 0.1292274648535927661 ) ) ;
#37006=CARTESIAN_POINT ( 'NONE',  ( -1.692913385826770645, 0.1771653543307087630, 0.000000000000000000 ) ) ;
#37007=CARTESIAN_POINT ( 'NONE',  ( -1.568241469816272105, -0.05778040916215522460, 0.4822834645669289988 ) ) ;
#37008=CARTESIAN_POINT ( 'NONE',  ( -0.9514435695538050464, -0.3162353388693405765, 0.4822834645669290543 ) ) ;
#37009=CARTESIAN_POINT ( 'NONE',  ( -1.633858267716534529, 0.1660481256975885056, 0.3530559997133364547 ) ) ;
#37012=CARTESIAN_POINT ( 'NONE',  ( 0.8595800524934390507, -0.3162353388693405765, 0.4822834645669290543 ) ) ;
#37013=CARTESIAN_POINT ( 'NONE',  ( 0.3018372703412079971, 0.05413385826771626580, -0.4176697321401330321 ) ) ;
#37016=CARTESIAN_POINT ( 'NONE',  ( 1.299212598425197429, 0.1771653543307087630, 0.000000000000000000 ) ) ;
#37018=ORIENTED_EDGE ( 'NONE', *, *, #37700, .F. ) ;
#37019=CARTESIAN_POINT ( 'NONE',  ( -0.9055118110236215490, -0.5511811023622047445, 6.969142054262312111E-17 ) ) ;
#37022=CARTESIAN_POINT ( 'NONE',  ( 0.2427821522309716595, -0.3162353388693409650, -0.4822834645669289433 ) ) ;
#37023=CARTESIAN_POINT ( 'NONE',  ( -0.4265091863517051496, 0.2952755905511810774, -0.1292274648535930714 ) ) ;
#37024=CARTESIAN_POINT ( 'NONE',  ( -1.076115485564303809, -0.6046776061558809534, -0.2411417322834644161 ) ) ;
#37025=CARTESIAN_POINT ( 'NONE',  ( 0.8661417322834653598, -0.1870078740157479769, 0.4822834645669291653 ) ) ;
#37026=CARTESIAN_POINT ( 'NONE',  ( 1.594488188976378673, -0.5400638737290845981, -0.3530559997133363437 ) ) ;
#37028=CARTESIAN_POINT ( 'NONE',  ( -0.2034120734908128059, 0.2952755905511811885, 0.1292274648535926551 ) ) ;
#37029=CARTESIAN_POINT ( 'NONE',  ( -1.089238845144356427, -0.4281496062992127816, -0.4176697321401328100 ) ) ;
#37030=LINE ( 'NONE', #50469, #43355 ) ;
#37033=CARTESIAN_POINT ( 'NONE',  ( 0.6692913385826778638, -0.5511811023622047445, 6.969142054262312111E-17 ) ) ;
#37036=CARTESIAN_POINT ( 'NONE',  ( -0.6364829396325453192, -0.05778040916215560624, -0.4822834645669293319 ) ) ;
#37038=CARTESIAN_POINT ( 'NONE',  ( 0.1246719160104994284, -0.5511811023622046335, 0.09757992244046803654 ) ) ;
#37040=CARTESIAN_POINT ( 'NONE',  ( 0.7020997375328090762, -0.05778040916215560624, -0.4822834645669293319 ) ) ;
#37041=CARTESIAN_POINT ( 'NONE',  ( 0.4527559055118117182, -0.5400638737290844871, 0.3530559997133364547 ) ) ;
#37042=CARTESIAN_POINT ( 'NONE',  ( -0.4527559055118102749, 0.1660481256975885056, 0.3530559997133364547 ) ) ;
#37044=CARTESIAN_POINT ( 'NONE',  ( -1.384514435695537005, -0.6692913385826773087, -0.1292274648535924053 ) ) ;
#37046=CARTESIAN_POINT ( 'NONE',  ( 1.463254593175853824, 0.1771653543307087075, -0.09757992244046823083 ) ) ;
#37047=CARTESIAN_POINT ( 'NONE',  ( -1.220472440944881054, -0.6692913385826771977, 8.415575281601705876E-17 ) ) ;
#37048=CARTESIAN_POINT ( 'NONE',  ( 0.6889763779527566800, -0.5400638737290844871, 0.3530559997133364547 ) ) ;
#37049=CARTESIAN_POINT ( 'NONE',  ( 1.030183727034121421, -0.05778040916215522460, 0.4822834645669289988 ) ) ;
#37051=CARTESIAN_POINT ( 'NONE',  ( -1.154855643044618851, -0.6046776061558809534, -0.2411417322834644161 ) ) ;
#37053=CARTESIAN_POINT ( 'NONE',  ( 0.3674540682414705883, 0.2306618581243847221, -0.2411417322834647770 ) ) ;
#37056=CARTESIAN_POINT ( 'NONE',  ( -1.646981627296586703, -0.08942795157527998196, 0.3641732283464567121 ) ) ;
#37057=CARTESIAN_POINT ( 'NONE',  ( 0.7611548556430454138, 0.1283753931104746893, -0.1820866141732285504 ) ) ;
#37058=CARTESIAN_POINT ( 'NONE',  ( 1.089238845144357537, -0.4281496062992124485, 0.4176697321401328655 ) ) ;
#37060=CARTESIAN_POINT ( 'NONE',  ( 0.9514435695538062676, -0.2845877964562161244, -0.3641732283464567121 ) ) ;
#37061=CARTESIAN_POINT ( 'NONE',  ( 0.2493438320209980519, -0.4281496062992127816, -0.4176697321401328100 ) ) ;
#37063=CARTESIAN_POINT ( 'NONE',  ( -0.8661417322834640276, -0.1870078740157480879, -0.4822834645669291653 ) ) ;
#37064=CARTESIAN_POINT ( 'NONE',  ( -1.614173228346457378, 2.157411728916712068, -0.1372047244094477536 ) ) ;
#37065=CARTESIAN_POINT ( 'NONE',  ( 1.030183727034121421, -0.2845877964562161244, -0.3641732283464567121 ) ) ;
#37066=CARTESIAN_POINT ( 'NONE',  ( 0.2230971128608929543, 0.05413385826771626580, -0.4176697321401330321 ) ) ;
#37067=CARTESIAN_POINT ( 'NONE',  ( -1.113948071074810420, 0.02791078216816347476, -0.4328096321851898631 ) ) ;
#37068=CARTESIAN_POINT ( 'NONE',  ( -0.1049868766404193215, 0.2306618581243847221, -0.2411417322834647770 ) ) ;
#37069=CARTESIAN_POINT ( 'NONE',  ( -0.07874015748031421014, -0.1870078740157479769, 0.3641732283464567677 ) ) ;
#37071=CARTESIAN_POINT ( 'NONE',  ( -0.3805774278215216522, -0.4281496062992127816, -0.4176697321401328100 ) ) ;
#37072=CARTESIAN_POINT ( 'NONE',  ( 0.6299212598425204535, -0.1870078740157479769, 0.3641732283464567677 ) ) ;
#37073=CARTESIAN_POINT ( 'NONE',  ( 1.220472440944881942, 0.4405861044731111953, -0.5309055118110238558 ) ) ;
#37075=CARTESIAN_POINT ( 'NONE',  ( 0.4461942257217856311, 0.2306618581243847221, -0.2411417322834647770 ) ) ;
#37077=CARTESIAN_POINT ( 'NONE',  ( 1.227034120734908917, 0.1771653543307087075, -0.09757992244046823083 ) ) ;
#37079=CARTESIAN_POINT ( 'NONE',  ( -0.4527559055118102749, 0.07958543189024085140, 0.2665933059059887866 ) ) ;
#37080=CARTESIAN_POINT ( 'NONE',  ( -0.9251968503937002541, 0.07958543189024085140, 0.2665933059059887866 ) ) ;
#37081=B_SPLINE_CURVE_WITH_KNOTS ( 'NONE', 3,
 ( #1149, #64687, #20914, #77745, #71006, #51615, #26800 ),
 .UNSPECIFIED., .F., .F.,
 ( 4, 3, 4 ),
 ( 1.734723475976807094E-18, 0.001246232571205225159, 0.002492492258783241162 ),
 .UNSPECIFIED. ) ;
#37082=CARTESIAN_POINT ( 'NONE',  ( -0.2690288713910754526, -0.6692913385826771977, 0.1292274648535927661 ) ) ;
#37083=CARTESIAN_POINT ( 'NONE',  ( 0.4265091863517067039, -0.6692913385826773087, -0.1292274648535924053 ) ) ;
#37084=CARTESIAN_POINT ( 'NONE',  ( 0.9908136482939640111, -0.5511811023622046335, 0.09757992244046803654 ) ) ;
#37085=CARTESIAN_POINT ( 'NONE',  ( -1.673228346456691717, 0.07958543189024071263, -0.2665933059059888421 ) ) ;
#37086=CARTESIAN_POINT ( 'NONE',  ( 1.607611548556431069, 0.1771653543307087630, 0.09757992244046791164 ) ) ;
#37087=CARTESIAN_POINT ( 'NONE',  ( 0.7217847769028878924, 0.05413385826771666132, 0.4176697321401328100 ) ) ;
#37089=CARTESIAN_POINT ( 'NONE',  ( 0.1968503937007881344, 0.2952755905511811885, 0.000000000000000000 ) ) ;
#37091=CARTESIAN_POINT ( 'NONE',  ( 1.010498687664042716, -0.4281496062992124485, 0.4176697321401328655 ) ) ;
#37093=CARTESIAN_POINT ( 'NONE',  ( 0.6167979002624679463, 0.05413385826771626580, -0.4176697321401330321 ) ) ;
#37095=CARTESIAN_POINT ( 'NONE',  ( 0.5249343832021005074, -0.5023911411419708095, 0.1820866141732285504 ) ) ;
#37096=CARTESIAN_POINT ( 'NONE',  ( 1.082677165354331228, 0.1660481256975883668, -0.3530559997133364547 ) ) ;
#37097=CARTESIAN_POINT ( 'NONE',  ( 0.1706036745406830368, -0.004921259842519576551, 0.3153832671262227771 ) ) ;
#37098=CARTESIAN_POINT ( 'NONE',  ( -0.2493438320209966919, -0.4281496062992124485, 0.4176697321401328655 ) ) ;
#37099=CARTESIAN_POINT ( 'NONE',  ( 0.2690288713910767848, -0.6692913385826773087, -0.1292274648535924053 ) ) ;
#37100=CARTESIAN_POINT ( 'NONE',  ( -0.8070866141732276899, 0.1660481256975883668, -0.3530559997133364547 ) ) ;
#37101=CARTESIAN_POINT ( 'NONE',  ( -0.4790026246719154557, -0.2845877964562159024, 0.3641732283464567677 ) ) ;
#37102=CARTESIAN_POINT ( 'NONE',  ( 0.2230971128608929543, 0.05413385826771626580, -0.4176697321401330321 ) ) ;
#37103=CARTESIAN_POINT ( 'NONE',  ( 0.9711286089238851948, -0.5023911411419708095, -0.1820866141732282451 ) ) ;
#37104=CARTESIAN_POINT ( 'NONE',  ( -0.2362204724409440182, -0.1870078740157479769, 0.4822834645669291653 ) ) ;
#37106=CARTESIAN_POINT ( 'NONE',  ( 1.115134929062665980, 0.004960608223778823628, 0.3437734562760190182 ) ) ;
#37109=CARTESIAN_POINT ( 'NONE',  ( 1.548556430446194954, 0.2306618581243847221, -0.2411417322834647770 ) ) ;
#37111=CARTESIAN_POINT ( 'NONE',  ( -1.108923884514435132, -0.05778040916215560624, -0.4822834645669293319 ) ) ;
#37113=CARTESIAN_POINT ( 'NONE',  ( -0.8333333333333323711, -0.6692913385826773087, -0.1292274648535924053 ) ) ;
#37116=ORIENTED_EDGE ( 'NONE', *, *, #25485, .F. ) ;
#37117=CARTESIAN_POINT ( 'NONE',  ( 0.2559055118110243332, 0.07958543189024085140, 0.2665933059059887866 ) ) ;
#37119=CARTESIAN_POINT ( 'NONE',  ( 0.7086614173228352742, -0.1870078740157480879, -0.4822834645669291653 ) ) ;
#37122=CARTESIAN_POINT ( 'NONE',  ( -1.712598425196849572, 0.07958543189024085140, 0.2665933059059887866 ) ) ;
#37123=CARTESIAN_POINT ( 'NONE',  ( 1.148293963254593875, -0.6692913385826771977, 0.1292274648535927661 ) ) ;
#37124=CARTESIAN_POINT ( 'NONE',  ( 1.476377952755906220, 0.07958543189024071263, -0.2665933059059888421 ) ) ;
#37125=CARTESIAN_POINT ( 'NONE',  ( 0.006561679790026889343, -0.3162353388693409650, -0.4822834645669289433 ) ) ;
#37127=CARTESIAN_POINT ( 'NONE',  ( -0.4790026246719152336, -0.05778040916215560624, -0.4822834645669293319 ) ) ;
#37128=CARTESIAN_POINT ( 'NONE',  ( -1.528871391076114250, 0.1771653543307087075, -0.09757992244046823083 ) ) ;
#37129=CARTESIAN_POINT ( 'NONE',  ( 0.5905511811023629321, -0.6692913385826771977, 8.415575281601705876E-17 ) ) ;
#37130=CARTESIAN_POINT ( 'NONE',  ( -0.3674540682414692561, -0.6046776061558809534, -0.2411417322834644161 ) ) ;
#37131=CARTESIAN_POINT ( 'NONE',  ( 1.607611548556431069, -0.6692913385826773087, -0.1292274648535924053 ) ) ;
#37135=CARTESIAN_POINT ( 'NONE',  ( 0.5708661417322842269, 0.1660481256975885056, 0.3530559997133364547 ) ) ;
#37136=CARTESIAN_POINT ( 'NONE',  ( -0.2755905511811018171, 0.2952755905511811885, 0.000000000000000000 ) ) ;
#37137=CARTESIAN_POINT ( 'NONE',  ( -1.528871391076114250, -0.6692913385826771977, 0.1292274648535927661 ) ) ;
#37138=CARTESIAN_POINT ( 'NONE',  ( 0.8727034120734912248, -0.3162353388693409650, -0.4822834645669289433 ) ) ;
#37139=CARTESIAN_POINT ( 'NONE',  ( 0.6627296587926517768, -0.6692913385826773087, -0.1292274648535924053 ) ) ;
#37141=CARTESIAN_POINT ( 'NONE',  ( -0.6496062992125976043, -0.5400638737290844871, 0.3530559997133364547 ) ) ;
#37142=CARTESIAN_POINT ( 'NONE',  ( 0.04593175853018440641, -0.6692913385826771977, 0.1292274648535927661 ) ) ;
#37143=CARTESIAN_POINT ( 'NONE',  ( -0.5708661417322825615, -0.5400638737290844871, 0.3530559997133364547 ) ) ;
#37144=CARTESIAN_POINT ( 'NONE',  ( 0.2755905511811031494, 0.1771653543307087630, 0.000000000000000000 ) ) ;
#37145=CARTESIAN_POINT ( 'NONE',  ( -1.627296587926508442, -0.6046776061558809534, -0.2411417322834644161 ) ) ;
#37147=CARTESIAN_POINT ( 'NONE',  ( -0.2821522309711278487, 0.2952755905511811885, 0.1292274648535926551 ) ) ;
#37149=CARTESIAN_POINT ( 'NONE',  ( 1.358267716535433323, -0.5400638737290845981, -0.3530559997133363437 ) ) ;
#37151=ORIENTED_EDGE ( 'NONE', *, *, #45942, .F. ) ;
#37153=AXIS2_PLACEMENT_3D ( 'NONE', #81920, #10794, #68045 ) ;
#37154=CARTESIAN_POINT ( 'NONE',  ( 0.8464566929133866546, -0.5400638737290844871, 0.3530559997133364547 ) ) ;
#37155=CARTESIAN_POINT ( 'NONE',  ( 0.2624671916010504757, -0.5023911411419708095, -0.1820866141732282451 ) ) ;
#37157=VECTOR ( 'NONE', #55278, 39.37007874015748143 ) ;
#37164=CARTESIAN_POINT ( 'NONE',  ( 0.2952755905511816326, -0.5400638737290844871, 0.3530559997133364547 ) ) ;
#37165=CARTESIAN_POINT ( 'NONE',  ( -1.345144356955379816, -0.3162353388693405765, 0.4822834645669290543 ) ) ;
#37166=CARTESIAN_POINT ( 'NONE',  ( -0.9514435695538050464, -0.3162353388693405765, 0.4822834645669290543 ) ) ;
#37167=CARTESIAN_POINT ( 'NONE',  ( 0.2821522309711292364, -0.6692913385826771977, 0.1292274648535927661 ) ) ;
#37168=CARTESIAN_POINT ( 'NONE',  ( 1.049868766404200127, -0.6046776061558809534, -0.2411417322834644161 ) ) ;
#37169=CARTESIAN_POINT ( 'NONE',  ( 1.482939632545932307, -0.3690944881889763329, 0.3153832671262228327 ) ) ;
#37170=CARTESIAN_POINT ( 'NONE',  ( 1.318897637795276356, -0.4536011799217367080, 0.2665933059059888421 ) ) ;
#37171=CARTESIAN_POINT ( 'NONE',  ( -1.030183727034119867, -0.3162353388693405765, 0.4822834645669290543 ) ) ;
#37173=CARTESIAN_POINT ( 'NONE',  ( 1.594488188976378673, -0.5400638737290845981, -0.3530559997133363437 ) ) ;
#37175=CARTESIAN_POINT ( 'NONE',  ( -0.4133858267716528645, -0.5400638737290844871, 0.3530559997133364547 ) ) ;
#37177=CARTESIAN_POINT ( 'NONE',  ( 1.069553805774278832, 0.2952755905511810774, -0.1292274648535930714 ) ) ;
#37179=CARTESIAN_POINT ( 'NONE',  ( -1.430446194225721390, -0.3690944881889763329, 0.3153832671262228327 ) ) ;
#37180=CARTESIAN_POINT ( 'NONE',  ( 0.3149606299212606708, -0.1870078740157480879, -0.4822834645669291653 ) ) ;
#37181=CARTESIAN_POINT ( 'NONE',  ( 1.030183727034121421, -0.2845877964562161244, -0.3641732283464567121 ) ) ;
#37183=CARTESIAN_POINT ( 'NONE',  ( 0.7414698162729663755, 0.2952755905511811885, 0.1292274648535926551 ) ) ;
#37185=CARTESIAN_POINT ( 'NONE',  ( -0.6299212598425188991, -0.1870078740157479769, 0.3641732283464567677 ) ) ;
#37186=CARTESIAN_POINT ( 'NONE',  ( -0.5249343832020990641, -0.6046776061558809534, -0.2411417322834644161 ) ) ;
#37187=CARTESIAN_POINT ( 'NONE',  ( -1.568241469816272105, -0.2845877964562161244, -0.3641732283464567121 ) ) ;
#37188=CARTESIAN_POINT ( 'NONE',  ( -0.8530183727034112984, -0.4281496062992127816, -0.4176697321401328100 ) ) ;
#37189=CARTESIAN_POINT ( 'NONE',  ( 1.456692913385827515, -0.6692913385826771977, 8.415575281601705876E-17 ) ) ;
#37191=CARTESIAN_POINT ( 'NONE',  ( -1.036745406824146176, -0.3690944881889763329, 0.3153832671262228327 ) ) ;
#37193=CARTESIAN_POINT ( 'NONE',  ( 1.489501312335958172, -0.05778040916215560624, -0.4822834645669293319 ) ) ;
#37195=CARTESIAN_POINT ( 'NONE',  ( -1.673228346456691717, 0.1660481256975883668, -0.3530559997133364547 ) ) ;
#37196=CARTESIAN_POINT ( 'NONE',  ( -1.528871391076114250, -0.5511811023622046335, 0.09757992244046803654 ) ) ;
#37197=CARTESIAN_POINT ( 'NONE',  ( -0.8661417322834640276, -0.1870078740157480601, -0.3641732283464567677 ) ) ;
#37199=CARTESIAN_POINT ( 'NONE',  ( -0.2362204724409440182, -0.1870078740157479769, 0.4822834645669291653 ) ) ;
#37200=CARTESIAN_POINT ( 'NONE',  ( 0.1902887139107617975, -0.5511811023622048555, -0.09757992244046775898 ) ) ;
#37201=CARTESIAN_POINT ( 'NONE',  ( -1.154855643044618851, -0.5023911411419708095, -0.1820866141732282451 ) ) ;
#37202=CARTESIAN_POINT ( 'NONE',  ( 1.332020997375328974, -0.08942795157528024563, -0.3641732283464568787 ) ) ;
#37203=CARTESIAN_POINT ( 'NONE',  ( 0.8333333333333340365, -0.6692913385826771977, 0.1292274648535927661 ) ) ;
#37204=CARTESIAN_POINT ( 'NONE',  ( 1.561679790026247350, -0.4281496062992124485, 0.4176697321401328655 ) ) ;
#37205=CARTESIAN_POINT ( 'NONE',  ( 0.6496062992125991586, -0.4536011799217368745, -0.2665933059059886201 ) ) ;
#37206=CARTESIAN_POINT ( 'NONE',  ( 0.6627296587926517768, -0.6692913385826773087, -0.1292274648535924053 ) ) ;
#37208=CARTESIAN_POINT ( 'NONE',  ( 0.9711286089238851948, 0.1283753931104748280, 0.1820866141732283561 ) ) ;
#37211=CARTESIAN_POINT ( 'NONE',  ( -1.358267716535432434, -0.5400638737290844871, 0.3530559997133364547 ) ) ;
#37213=CARTESIAN_POINT ( 'NONE',  ( -1.312335958005248715, 0.2306618581243848609, 0.2411417322834645549 ) ) ;
#37214=CARTESIAN_POINT ( 'NONE',  ( 0.09842519685039434474, -0.5400638737290845981, -0.3530559997133363437 ) ) ;
#37217=CARTESIAN_POINT ( 'NONE',  ( 0.4986876640419954376, 0.2306618581243848609, 0.2411417322834645549 ) ) ;
#37218=CARTESIAN_POINT ( 'NONE',  ( 1.345144356955381593, -0.2845877964562161244, -0.3641732283464567121 ) ) ;
#37220=CONICAL_SURFACE ( 'NONE', #50659, 1.181102362204724310, 0.7853981633974621568 ) ;
#37221=CARTESIAN_POINT ( 'NONE',  ( 0.2296587926509192634, -0.3162353388693405765, 0.4822834645669290543 ) ) ;
#37222=CARTESIAN_POINT ( 'NONE',  ( 0.3346456692913390985, 0.1660481256975885056, 0.3530559997133364547 ) ) ;
#37228=CARTESIAN_POINT ( 'NONE',  ( -0.5839895013123351797, 0.1771653543307087075, -0.09757992244046823083 ) ) ;
#37229=CARTESIAN_POINT ( 'NONE',  ( -0.6102362204724400829, 0.1660481256975885056, 0.3530559997133364547 ) ) ;
#37230=CARTESIAN_POINT ( 'NONE',  ( 0.5446194225721792126, -0.05778040916215560624, -0.4822834645669293319 ) ) ;
#37232=CARTESIAN_POINT ( 'NONE',  ( 0.7152230971128616943, -0.05778040916215522460, 0.4822834645669289988 ) ) ;
#37233=EDGE_CURVE ( 'NONE', #79833, #32475, #49226, .T. ) ;
#37234=CARTESIAN_POINT ( 'NONE',  ( -1.502624671916009680, -0.3162353388693405765, 0.4822834645669290543 ) ) ;
#37235=CARTESIAN_POINT ( 'NONE',  ( 0.9448818897637802916, -0.1870078740157479769, 0.4822834645669291653 ) ) ;
#37236=CARTESIAN_POINT ( 'NONE',  ( -0.6192220670824142292, -3.724876541855331158E-15, 0.4118477457932994135 ) ) ;
#37238=CARTESIAN_POINT ( 'NONE',  ( 1.469816272965879911, -0.6046776061558807314, 0.2411417322834647770 ) ) ;
#37239=EDGE_CURVE ( 'NONE', #48621, #19643, #36357, .T. ) ;
#37240=CARTESIAN_POINT ( 'NONE',  ( 1.069553805774278610, -0.6692913385826771977, 0.1292274648535927661 ) ) ;
#37241=CARTESIAN_POINT ( 'NONE',  ( 0.4265091863517067039, -0.6692913385826773087, -0.1292274648535924053 ) ) ;
#37242=CARTESIAN_POINT ( 'NONE',  ( 1.082677165354331228, -0.4536011799217367080, 0.2665933059059888421 ) ) ;
#37244=CARTESIAN_POINT ( 'NONE',  ( -1.496062992125983815, -0.1870078740157479769, 0.3641732283464567677 ) ) ;
#37245=CARTESIAN_POINT ( 'NONE',  ( -1.397637795275589623, -0.5400638737290845981, -0.3530559997133363437 ) ) ;
#37247=DIRECTION ( 'NONE',  ( 0.000000000000000000, 0.000000000000000000, 1.000000000000000000 ) ) ;
#37248=CARTESIAN_POINT ( 'NONE',  ( 0.7874015748031503170, -0.1870078740157480879, -0.4822834645669291653 ) ) ;
#37249=DIRECTION ( 'NONE',  ( -3.096699300667737957E-16, 1.000000000000000000, -0.000000000000000000 ) ) ;
#37250=CARTESIAN_POINT ( 'NONE',  ( -0.6364829396325453192, -0.3162353388693405765, 0.4822834645669290543 ) ) ;
#37251=CARTESIAN_POINT ( 'NONE',  ( -0.9842519685039365918, -0.6692913385826771977, 8.415575281601705876E-17 ) ) ;
#37252=CARTESIAN_POINT ( 'NONE',  ( 1.128608923884514947, 0.2306618581243848609, 0.2411417322834645549 ) ) ;
#37256=CARTESIAN_POINT ( 'NONE',  ( 1.692913385826772421, 0.2952755905511811885, 0.000000000000000000 ) ) ;
#37259=ORIENTED_EDGE ( 'NONE', *, *, #54140, .F. ) ;
#37261=CARTESIAN_POINT ( 'NONE',  ( 1.522309711286089939, -0.5023911411419708095, -0.1820866141732282451 ) ) ;
#37263=CARTESIAN_POINT ( 'NONE',  ( 1.397637795275591177, 0.07958543189024071263, -0.2665933059059888421 ) ) ;
#37268=CARTESIAN_POINT ( 'NONE',  ( -0.9186351706036736120, -0.5023911411419708095, -0.1820866141732282451 ) ) ;
#37269=CARTESIAN_POINT ( 'NONE',  ( -1.272965879265091305, -0.3690944881889763329, 0.3153832671262228327 ) ) ;
#37270=CARTESIAN_POINT ( 'NONE',  ( -1.305774278215222184, 0.2952755905511811885, 0.1292274648535926551 ) ) ;
#37272=CARTESIAN_POINT ( 'NONE',  ( 0.1509186351706042484, -0.3162353388693405765, 0.4822834645669290543 ) ) ;
#37273=CARTESIAN_POINT ( 'NONE',  ( -1.410761154855641575, -0.3162353388693409650, -0.4822834645669289433 ) ) ;
#37274=EDGE_LOOP ( 'NONE', ( #16283, #50648, #73593, #53350 ) ) ;
#37275=CARTESIAN_POINT ( 'NONE',  ( 1.515748031496063186, -0.5400638737290845981, -0.3530559997133363437 ) ) ;
#37278=CARTESIAN_POINT ( 'NONE',  ( -0.7426113562972000981, 2.362204724409448620, -0.5309055118110235227 ) ) ;
#37279=CARTESIAN_POINT ( 'NONE',  ( -0.6561679790026240244, 0.1283753931104746893, -0.1820866141732285504 ) ) ;
#37281=CARTESIAN_POINT ( 'NONE',  ( -0.9776902887139098386, 0.2952755905511810774, -0.1292274648535930714 ) ) ;
#37282=CARTESIAN_POINT ( 'NONE',  ( 0.9317585301837276734, 0.05413385826771626580, -0.4176697321401330321 ) ) ;
#37283=ORIENTED_EDGE ( 'NONE', *, *, #19019, .T. ) ;
#37284=CARTESIAN_POINT ( 'NONE',  ( 0.7349081364829403995, 0.2306618581243848609, 0.2411417322834645549 ) ) ;
#37285=CARTESIAN_POINT ( 'NONE',  ( 1.603475055217291612, 0.9922665159524516332, -0.04573490813648244807 ) ) ;
#37286=CARTESIAN_POINT ( 'NONE',  ( -1.706036745406823485, 0.2306618581243848609, 0.2411417322834645549 ) ) ;
#37287=CARTESIAN_POINT ( 'NONE',  ( -1.410761154855642463, -0.05778040916215522460, 0.4822834645669289988 ) ) ;
#37289=CARTESIAN_POINT ( 'NONE',  ( 0.06561679790026316017, -0.004921259842519870586, -0.3153832671262229437 ) ) ;
#37291=CARTESIAN_POINT ( 'NONE',  ( -0.5380577427821514602, -0.004921259842519576551, 0.3153832671262227771 ) ) ;
#37292=CARTESIAN_POINT ( 'NONE',  ( 0.5708661417322841158, -0.4536011799217368745, -0.2665933059059886201 ) ) ;
#37293=CARTESIAN_POINT ( 'NONE',  ( 0.6692913385826777528, 0.2952755905511811885, 0.000000000000000000 ) ) ;
#37294=CARTESIAN_POINT ( 'NONE',  ( -0.7152230971128602510, -0.2845877964562159024, 0.3641732283464567677 ) ) ;
#37296=CARTESIAN_POINT ( 'NONE',  ( 1.122047244094488860, 0.1660481256975885056, 0.3530559997133364547 ) ) ;
#37298=CARTESIAN_POINT ( 'NONE',  ( -0.8136482939632537770, 0.2306618581243847221, -0.2411417322834647770 ) ) ;
#37300=CARTESIAN_POINT ( 'NONE',  ( 0.1574803149606306130, -0.1870078740157479769, 0.4822834645669291653 ) ) ;
#37301=CARTESIAN_POINT ( 'NONE',  ( -0.4855643044619415427, 0.05413385826771626580, -0.4176697321401330321 ) ) ;
#37302=CARTESIAN_POINT ( 'NONE',  ( 1.371391076115485941, 0.1771653543307087630, 0.09757992244046791164 ) ) ;
#37303=CARTESIAN_POINT ( 'NONE',  ( 0.2165354330708668673, 0.07958543189024071263, -0.2665933059059888421 ) ) ;
#37304=CARTESIAN_POINT ( 'NONE',  ( -0.3543307086614165824, -0.6692913385826771977, 8.415575281601705876E-17 ) ) ;
#37305=CARTESIAN_POINT ( 'NONE',  ( -1.253280839895012377, -0.3162353388693409650, -0.4822834645669289433 ) ) ;
#37307=CARTESIAN_POINT ( 'NONE',  ( 1.607611548556431069, -0.5511811023622048555, -0.09757992244046775898 ) ) ;
#37308=CARTESIAN_POINT ( 'NONE',  ( -0.07217847769028787330, -0.05778040916215522460, 0.4822834645669289988 ) ) ;
#37309=CARTESIAN_POINT ( 'NONE',  ( -0.9317585301837263412, 0.05413385826771666132, 0.4176697321401328100 ) ) ;
#37310=ORIENTED_EDGE ( 'NONE', *, *, #18464, .F. ) ;
#37312=EDGE_CURVE ( 'NONE', #54857, #34118, #218, .T. ) ;
#37313=CARTESIAN_POINT ( 'NONE',  ( 1.259842519685040019, -0.1870078740157479769, 0.4822834645669291653 ) ) ;
#37314=CARTESIAN_POINT ( 'NONE',  ( -0.4593175853018366950, -0.004921259842519576551, 0.3153832671262227771 ) ) ;
#37315=CARTESIAN_POINT ( 'NONE',  ( -0.5183727034120726440, -0.6692913385826773087, -0.1292274648535924053 ) ) ;
#37316=CARTESIAN_POINT ( 'NONE',  ( 1.279527559055118724, -0.5400638737290845981, -0.3530559997133363437 ) ) ;
#37317=CARTESIAN_POINT ( 'NONE',  ( 1.043307086614173818, 0.1660481256975885056, 0.3530559997133364547 ) ) ;
#37318=B_SPLINE_CURVE_WITH_KNOTS ( 'NONE', 3,
 ( #63193, #5533, #82559, #25707, #24878, #50546, #76250 ),
 .UNSPECIFIED., .F., .F.,
 ( 4, 3, 4 ),
 ( 1.561251128379126385E-17, 0.001246230184515585400, 0.002492489877932649398 ),
 .UNSPECIFIED. ) ;
#37319=CARTESIAN_POINT ( 'NONE',  ( 2.795275590551181466, 1.338582677165354395, -1.617488608965169241E-16 ) ) ;
#37320=CARTESIAN_POINT ( 'NONE',  ( -1.095800524934382292, -0.08942795157527998196, 0.3641732283464567121 ) ) ;
#37325=CARTESIAN_POINT ( 'NONE',  ( 1.154855643044620184, -0.5023911411419708095, 0.1820866141732285504 ) ) ;
#37326=CARTESIAN_POINT ( 'NONE',  ( 0.5774278215223103139, -0.5023911411419708095, -0.1820866141732282451 ) ) ;
#37327=CARTESIAN_POINT ( 'NONE',  ( 0.5708661417322841158, -0.5400638737290845981, -0.3530559997133363437 ) ) ;
#37329=CARTESIAN_POINT ( 'NONE',  ( 0.7283464566929143125, 0.07958543189024085140, 0.2665933059059887866 ) ) ;
#37330=CARTESIAN_POINT ( 'NONE',  ( -0.3018372703412066094, -0.4281496062992127816, -0.4176697321401328100 ) ) ;
#37331=CARTESIAN_POINT ( 'NONE',  ( -1.056430446194224881, -0.6692913385826771977, 0.1292274648535927661 ) ) ;
#37332=CARTESIAN_POINT ( 'NONE',  ( 1.062992125984252745, 0.2952755905511811885, 0.000000000000000000 ) ) ;
#37336=CARTESIAN_POINT ( 'NONE',  ( 0.1246719160104994284, -0.5511811023622046335, 0.09757992244046803654 ) ) ;
#37338=ORIENTED_EDGE ( 'NONE', *, *, #61119, .F. ) ;
#37339=CARTESIAN_POINT ( 'NONE',  ( -0.9908136482939626788, -0.6692913385826773087, -0.1292274648535924053 ) ) ;
#37340=CARTESIAN_POINT ( 'NONE',  ( -0.6889763779527552368, 0.1660481256975885056, 0.3530559997133364547 ) ) ;
#37341=CARTESIAN_POINT ( 'NONE',  ( -0.2821522309711278487, -0.6692913385826773087, -0.1292274648535924053 ) ) ;
#37343=CARTESIAN_POINT ( 'NONE',  ( 0.3608923884514443348, -0.6692913385826771977, 0.1292274648535927661 ) ) ;
#37344=CARTESIAN_POINT ( 'NONE',  ( -0.3608923884514428360, 0.2952755905511811885, 0.1292274648535926551 ) ) ;
#37345=CARTESIAN_POINT ( 'NONE',  ( -1.522309711286088607, -0.6046776061558807314, 0.2411417322834647770 ) ) ;
#37346=CARTESIAN_POINT ( 'NONE',  ( -0.9776902887139098386, -0.6692913385826771977, 0.1292274648535927661 ) ) ;
#37347=CARTESIAN_POINT ( 'NONE',  ( 0.9448818897637802916, -0.1870078740157479769, 0.4822834645669291653 ) ) ;
#37349=CARTESIAN_POINT ( 'NONE',  ( -0.4330708661417315697, -0.5511811023622047445, 6.969142054262312111E-17 ) ) ;
#37350=ORIENTED_EDGE ( 'NONE', *, *, #3392, .F. ) ;
#37352=VERTEX_POINT ( 'NONE', #19989 ) ;
#37353=CARTESIAN_POINT ( 'NONE',  ( -1.082677165354329896, 0.07958543189024085140, 0.2665933059059887866 ) ) ;
#37354=CARTESIAN_POINT ( 'NONE',  ( -0.9842519685039360366, 0.2952755905511811885, 0.000000000000000000 ) ) ;
#37355=CARTESIAN_POINT ( 'NONE',  ( -0.7283464566929126471, -0.5400638737290844871, 0.3530559997133364547 ) ) ;
#37357=CARTESIAN_POINT ( 'NONE',  ( -0.6496062992125976043, -0.5400638737290844871, 0.3530559997133364547 ) ) ;
#37358=CARTESIAN_POINT ( 'NONE',  ( -0.6627296587926503335, -0.6692913385826771977, 0.1292274648535927661 ) ) ;
#37362=CARTESIAN_POINT ( 'NONE',  ( 0.4658792650918641698, -0.08942795157528024563, -0.3641732283464568787 ) ) ;
#37363=CARTESIAN_POINT ( 'NONE',  ( 1.586052503253845281, 1.023622047244095556, -0.1653254495020587966 ) ) ;
#37365=CARTESIAN_POINT ( 'NONE',  ( -0.1312335958005241554, 0.1283753931104748280, 0.1820866141732283561 ) ) ;
#37366=CARTESIAN_POINT ( 'NONE',  ( -0.3740157480314953431, 0.1660481256975885056, 0.3530559997133364547 ) ) ;
#37368=CARTESIAN_POINT ( 'NONE',  ( 1.496062992125984703, -0.1870078740157480879, -0.4822834645669291653 ) ) ;
#37369=CARTESIAN_POINT ( 'NONE',  ( 0.1049868766404206816, 0.2306618581243848609, 0.2411417322834645549 ) ) ;
#37372=CARTESIAN_POINT ( 'NONE',  ( -0.8530183727034112984, 0.009842519685039467087, 0.3409548833797002021 ) ) ;
#37376=CARTESIAN_POINT ( 'NONE',  ( -1.003937007874015297, -0.4536011799217368745, -0.2665933059059886201 ) ) ;
#37377=CARTESIAN_POINT ( 'NONE',  ( -1.561679790026246017, 0.05413385826771666132, 0.4176697321401328100 ) ) ;
#37379=CARTESIAN_POINT ( 'NONE',  ( 1.586052503253845503, 0.7480314960629931287, 0.1653254495020587966 ) ) ;
#37381=CARTESIAN_POINT ( 'NONE',  ( 1.259842519685040019, -0.1870078740157480879, -0.4822834645669291653 ) ) ;
#37382=CARTESIAN_POINT ( 'NONE',  ( 0.4396325459317590445, -0.6692913385826771977, 0.1292274648535927661 ) ) ;
#37383=CARTESIAN_POINT ( 'NONE',  ( 0.1968503937007881344, -0.6692913385826771977, 8.415575281601705876E-17 ) ) ;
#37384=CARTESIAN_POINT ( 'NONE',  ( -0.8923884514435688198, -0.5023911411419708095, 0.1820866141732285504 ) ) ;
#37385=CARTESIAN_POINT ( 'NONE',  ( -0.2296587926509179312, -0.3162353388693409650, -0.4822834645669289433 ) ) ;
#37387=CARTESIAN_POINT ( 'NONE',  ( -1.030183727034119867, -0.05778040916215560624, -0.4822834645669293319 ) ) ;
#37389=CARTESIAN_POINT ( 'NONE',  ( 1.213910761154856299, -0.5511811023622048555, -0.09757992244046775898 ) ) ;
#37390=CARTESIAN_POINT ( 'NONE',  ( -0.3083989501312330295, -0.08942795157527998196, 0.3641732283464567121 ) ) ;
#37391=CARTESIAN_POINT ( 'NONE',  ( 1.371391076115485941, 0.1771653543307087630, 0.09757992244046791164 ) ) ;
#37392=CARTESIAN_POINT ( 'NONE',  ( -1.371391076115484831, 0.2952755905511810774, -0.1292274648535930714 ) ) ;
#37393=CARTESIAN_POINT ( 'NONE',  ( -1.220472440944881054, -0.5511811023622047445, 6.969142054262312111E-17 ) ) ;
#37395=CARTESIAN_POINT ( 'NONE',  ( 0.3477690288713918276, -0.5511811023622048555, -0.09757992244046775898 ) ) ;
#37396=CARTESIAN_POINT ( 'NONE',  ( -0.9776902887139098386, 0.2952755905511810774, -0.1292274648535930714 ) ) ;
#37399=CARTESIAN_POINT ( 'NONE',  ( -0.01968503937007793844, 0.07958543189024071263, -0.2665933059059888421 ) ) ;
#37400=CARTESIAN_POINT ( 'NONE',  ( -1.522309711286088607, 0.1283753931104746893, -0.1820866141732285504 ) ) ;
#37401=CARTESIAN_POINT ( 'NONE',  ( 0.6496062992125991586, -0.5400638737290845981, -0.3530559997133363437 ) ) ;
#37402=LINE ( 'NONE', #44925, #47849 ) ;
#37403=CARTESIAN_POINT ( 'NONE',  ( 1.332020997375328974, -0.08942795157528024563, -0.3641732283464568787 ) ) ;
#37404=CARTESIAN_POINT ( 'NONE',  ( -1.095800524934382292, -0.05778040916215522460, 0.4822834645669289988 ) ) ;
#37405=CARTESIAN_POINT ( 'NONE',  ( -0.3477690288713902178, 0.1771653543307087075, -0.09757992244046823083 ) ) ;
#37406=CARTESIAN_POINT ( 'NONE',  ( -1.603475055217291612, 0.9922665159524542977, -0.04573490813648263542 ) ) ;
#37407=CARTESIAN_POINT ( 'NONE',  ( 0.4068241469816279987, -0.3690944881889765550, -0.3153832671262227771 ) ) ;
#37408=CARTESIAN_POINT ( 'NONE',  ( -1.181102362204723644, -0.1870078740157480879, -0.4822834645669291653 ) ) ;
#37409=CARTESIAN_POINT ( 'NONE',  ( -0.5971128608923877978, -0.6692913385826773087, -0.1292274648535924053 ) ) ;
#37412=CARTESIAN_POINT ( 'NONE',  ( 0.5446194225721792126, -0.08942795157528024563, -0.3641732283464568787 ) ) ;
#37413=CARTESIAN_POINT ( 'NONE',  ( -0.1968503937007867743, 0.2952755905511811885, 0.000000000000000000 ) ) ;
#37414=CARTESIAN_POINT ( 'NONE',  ( -0.7874015748031489847, -0.1870078740157480879, -0.4822834645669291653 ) ) ;
#37415=CARTESIAN_POINT ( 'NONE',  ( -0.9973753280839886548, 0.1283753931104748280, 0.1820866141732283561 ) ) ;
#37417=CARTESIAN_POINT ( 'NONE',  ( -0.1837270341207340729, 0.2306618581243847221, -0.2411417322834647770 ) ) ;
#37418=CARTESIAN_POINT ( 'NONE',  ( -1.515748031496062076, 0.07958543189024071263, -0.2665933059059888421 ) ) ;
#37419=CARTESIAN_POINT ( 'NONE',  ( -1.351706036745406347, -0.4281496062992124485, 0.4176697321401328655 ) ) ;
#37421=ORIENTED_EDGE ( 'NONE', *, *, #36825, .F. ) ;
#37423=CARTESIAN_POINT ( 'NONE',  ( -1.443569553805773564, -0.6046776061558807314, 0.2411417322834647770 ) ) ;
#37424=CARTESIAN_POINT ( 'NONE',  ( -1.036745406824146176, 0.05413385826771626580, -0.4176697321401330321 ) ) ;
#37425=CARTESIAN_POINT ( 'NONE',  ( 1.515748031496063186, -0.5400638737290845981, -0.3530559997133363437 ) ) ;
#37428=CARTESIAN_POINT ( 'NONE',  ( 0.8530183727034128527, -0.4281496062992124485, 0.4176697321401328655 ) ) ;
#37429=CARTESIAN_POINT ( 'NONE',  ( 0.6102362204724416372, 0.1660481256975883668, -0.3530559997133364547 ) ) ;
#37432=CARTESIAN_POINT ( 'NONE',  ( 1.089238845144357537, -0.3690944881889763329, 0.3153832671262228327 ) ) ;
#37434=ORIENTED_EDGE ( 'NONE', *, *, #65412, .F. ) ;
#37437=CARTESIAN_POINT ( 'NONE',  ( 0.3937007874015754361, -0.1870078740157480879, -0.4822834645669291653 ) ) ;
#37438=CARTESIAN_POINT ( 'NONE',  ( -0.7480314960629914633, 0.2952755905511811885, 0.000000000000000000 ) ) ;
#37439=CARTESIAN_POINT ( 'NONE',  ( -1.410761154855641575, -0.3162353388693409650, -0.4822834645669289433 ) ) ;
#37440=CARTESIAN_POINT ( 'NONE',  ( 1.010498687664042716, -0.4281496062992124485, 0.4176697321401328655 ) ) ;
#37441=CARTESIAN_POINT ( 'NONE',  ( 1.601049868766404982, -0.6046776061558809534, -0.2411417322834644161 ) ) ;
#37443=CARTESIAN_POINT ( 'NONE',  ( -0.2362204724409440182, -0.1870078740157479769, 0.4822834645669291653 ) ) ;
#37444=CARTESIAN_POINT ( 'NONE',  ( -1.095800524934382292, -0.3162353388693409650, -0.4822834645669289433 ) ) ;
#37445=CARTESIAN_POINT ( 'NONE',  ( -1.541994750656167090, -0.6692913385826773087, -0.1292274648535924053 ) ) ;
#37448=CARTESIAN_POINT ( 'NONE',  ( 1.049868766404200349, 0.1283753931104748280, 0.1820866141732283561 ) ) ;
#37452=CARTESIAN_POINT ( 'NONE',  ( -0.1312335958005241554, 0.1283753931104748280, 0.1820866141732283561 ) ) ;
#37454=CARTESIAN_POINT ( 'NONE',  ( 0.5774278215223103139, -0.6046776061558809534, -0.2411417322834644161 ) ) ;
#37455=CARTESIAN_POINT ( 'NONE',  ( 0.2755905511811031494, -0.6692913385826771977, 8.415575281601705876E-17 ) ) ;
#37456=EDGE_CURVE ( 'NONE', #65086, #19973, #67518, .T. ) ;
#37457=CARTESIAN_POINT ( 'NONE',  ( -0.7086614173228339419, -0.1870078740157480879, -0.4822834645669291653 ) ) ;
#37459=CARTESIAN_POINT ( 'NONE',  ( -1.135170603674539924, 0.2952755905511810774, -0.1292274648535930714 ) ) ;
#37461=CARTESIAN_POINT ( 'NONE',  ( 1.286089238845145033, 0.1283753931104748280, 0.1820866141732283561 ) ) ;
#37462=CARTESIAN_POINT ( 'NONE',  ( -1.430446194225720724, 0.05413385826771626580, -0.4176697321401330321 ) ) ;
#37463=CARTESIAN_POINT ( 'NONE',  ( 0.9055118110236227702, 0.2952755905511811885, 0.000000000000000000 ) ) ;
#37464=CARTESIAN_POINT ( 'NONE',  ( 0.9842519685039378130, -0.6692913385826771977, 8.415575281601705876E-17 ) ) ;
#37466=CARTESIAN_POINT ( 'NONE',  ( -1.299212598425196097, -0.6692913385826771977, 8.415575281601705876E-17 ) ) ;
#37468=CARTESIAN_POINT ( 'NONE',  ( 0.006561679790026889343, -0.05778040916215522460, 0.4822834645669289988 ) ) ;
#37471=CARTESIAN_POINT ( 'NONE',  ( 1.541994750656168645, 0.2952755905511810774, -0.1292274648535930714 ) ) ;
#37472=CARTESIAN_POINT ( 'NONE',  ( 0.1968503937007881344, -0.5511811023622047445, 6.969142054262312111E-17 ) ) ;
#37473=CARTESIAN_POINT ( 'NONE',  ( 0.9514435695538062676, -0.05778040916215522460, 0.4822834645669289988 ) ) ;
#37475=CARTESIAN_POINT ( 'NONE',  ( 0.7349081364829403995, 0.1283753931104748280, 0.1820866141732283561 ) ) ;
#37476=( BOUNDED_CURVE ( )  B_SPLINE_CURVE ( 1, ( #29881, #81253 ),
 .UNSPECIFIED., .F., .F. ) 
 B_SPLINE_CURVE_WITH_KNOTS ( ( 2, 2 ),
 ( 6.938893903907228378E-18, 0.001999999999999994837 ),
 .UNSPECIFIED. ) 
 CURVE ( )  GEOMETRIC_REPRESENTATION_ITEM ( )  RATIONAL_B_SPLINE_CURVE ( ( 0.9875488213027535656, 0.9875488213027535656 ) ) 
 REPRESENTATION_ITEM ( '' )  );
#37477=CARTESIAN_POINT ( 'NONE',  ( 0.3280839895013130669, 0.05413385826771666132, 0.4176697321401328100 ) ) ;
#37479=CARTESIAN_POINT ( 'NONE',  ( -0.7677165354330699465, 0.1660481256975885056, 0.3530559997133364547 ) ) ;
#37481=CARTESIAN_POINT ( 'NONE',  ( 0.7611548556430451917, -0.5023911411419708095, 0.1820866141732285504 ) ) ;
#37483=CARTESIAN_POINT ( 'NONE',  ( -0.3083989501312330295, -0.05778040916215522460, 0.4822834645669289988 ) ) ;
#37484=CARTESIAN_POINT ( 'NONE',  ( 0.07874015748031558404, -0.1870078740157479769, 0.3641732283464567677 ) ) ;
#37486=CARTESIAN_POINT ( 'NONE',  ( -0.5118110236220466680, -0.6692913385826771977, 8.415575281601705876E-17 ) ) ;
#37487=CARTESIAN_POINT ( 'NONE',  ( 0.7152230971128614723, -0.2845877964562161244, -0.3641732283464567121 ) ) ;
#37489=CARTESIAN_POINT ( 'NONE',  ( 0.4658792650918641698, -0.05778040916215560624, -0.4822834645669293319 ) ) ;
#37490=CARTESIAN_POINT ( 'NONE',  ( 1.371391076115485941, 0.1771653543307087630, 0.09757992244046791164 ) ) ;
#37492=CARTESIAN_POINT ( 'NONE',  ( -0.5577427821522301654, -0.08942795157528024563, -0.3641732283464568787 ) ) ;
#37493=CARTESIAN_POINT ( 'NONE',  ( -0.5708661417322828946, 0.07958543189024071263, -0.2665933059059888421 ) ) ;
#37494=CARTESIAN_POINT ( 'NONE',  ( -0.4265091863517051496, -0.6692913385826771977, 0.1292274648535927661 ) ) ;
#37495=CARTESIAN_POINT ( 'NONE',  ( 0.1837270341207354329, 0.2306618581243848609, 0.2411417322834645549 ) ) ;
#37496=CARTESIAN_POINT ( 'NONE',  ( 0.8595800524934390507, -0.2845877964562159024, 0.3641732283464567677 ) ) ;
#37497=CARTESIAN_POINT ( 'NONE',  ( -1.627296587926508442, -0.5023911411419708095, -0.1820866141732282451 ) ) ;
#37498=CARTESIAN_POINT ( 'NONE',  ( 1.450131233595801428, 0.1771653543307087630, 0.09757992244046791164 ) ) ;
#37499=CARTESIAN_POINT ( 'NONE',  ( 0.7349081364829403995, 0.2306618581243848609, 0.2411417322834645549 ) ) ;
#37501=CARTESIAN_POINT ( 'NONE',  ( -0.4002624671916004129, -0.05778040916215560624, -0.4822834645669293319 ) ) ;
#37503=CARTESIAN_POINT ( 'NONE',  ( 0.8464566929133866546, -0.5400638737290844871, 0.3530559997133364547 ) ) ;
#37504=CARTESIAN_POINT ( 'NONE',  ( 0.5905511811023629321, 0.2952755905511811885, 0.000000000000000000 ) ) ;
#37506=CARTESIAN_POINT ( 'NONE',  ( 0.5839895013123367340, 0.1771653543307087630, 0.09757992244046791164 ) ) ;
#37507=CARTESIAN_POINT ( 'NONE',  ( 1.292650918635171564, -0.6692913385826773087, -0.1292274648535924053 ) ) ;
#37508=CARTESIAN_POINT ( 'NONE',  ( 0.08530183727034192087, -0.2845877964562161244, -0.3641732283464567121 ) ) ;
#37509=CARTESIAN_POINT ( 'NONE',  ( -0.4855643044619415427, 0.05413385826771626580, -0.4176697321401330321 ) ) ;
#37511=CARTESIAN_POINT ( 'NONE',  ( 0.4199475065616803948, -0.6046776061558809534, -0.2411417322834644161 ) ) ;
#37512=CARTESIAN_POINT ( 'NONE',  ( -0.5905511811023613777, -0.6692913385826771977, 8.415575281601705876E-17 ) ) ;
#37513=CARTESIAN_POINT ( 'NONE',  ( -0.4330708661417315697, 0.1771653543307087630, 0.000000000000000000 ) ) ;
#37514=CARTESIAN_POINT ( 'NONE',  ( 0.2821522309711292364, -0.6692913385826771977, 0.1292274648535927661 ) ) ;
#37515=CARTESIAN_POINT ( 'NONE',  ( 1.141732283464567788, -0.5511811023622047445, 6.969142054262312111E-17 ) ) ;
#37516=CARTESIAN_POINT ( 'NONE',  ( -0.4265091863517051496, -0.6692913385826771977, 0.1292274648535927661 ) ) ;
#37519=CARTESIAN_POINT ( 'NONE',  ( 1.456692913385827515, 0.2952755905511811885, 0.000000000000000000 ) ) ;
#37522=CARTESIAN_POINT ( 'NONE',  ( -1.541994750656167090, -0.6692913385826773087, -0.1292274648535924053 ) ) ;
#37523=CARTESIAN_POINT ( 'NONE',  ( -0.8989501312335946848, 0.2952755905511810774, -0.1292274648535930714 ) ) ;
#37527=CARTESIAN_POINT ( 'NONE',  ( 0.4658792650918641698, -0.08942795157528024563, -0.3641732283464568787 ) ) ;
#37529=CARTESIAN_POINT ( 'NONE',  ( 0.6955380577427828781, 0.05413385826771626580, -0.4176697321401330321 ) ) ;
#37531=CARTESIAN_POINT ( 'NONE',  ( -0.5618802787717172009, -5.582469467804009507E-15, -0.4118484887281986251 ) ) ;
#37532=CARTESIAN_POINT ( 'NONE',  ( -0.3937007874015740483, -0.1870078740157479769, 0.3641732283464567677 ) ) ;
#37533=CARTESIAN_POINT ( 'NONE',  ( -1.719160104986876103, -0.004921259842519576551, 0.3153832671262227771 ) ) ;
#37534=CARTESIAN_POINT ( 'NONE',  ( 1.240157480314961314, 0.1660481256975883668, -0.3530559997133364547 ) ) ;
#37535=CARTESIAN_POINT ( 'NONE',  ( 1.345144356955381593, -0.2845877964562161244, -0.3641732283464567121 ) ) ;
#37536=CARTESIAN_POINT ( 'NONE',  ( -0.1246719160104980823, -0.6692913385826773087, -0.1292274648535924053 ) ) ;
#37538=CARTESIAN_POINT ( 'NONE',  ( -0.5905511811023613777, -0.6692913385826771977, 8.415575281601705876E-17 ) ) ;
#37539=CARTESIAN_POINT ( 'NONE',  ( -1.305774278215222184, -0.5511811023622048555, -0.09757992244046775898 ) ) ;
#37540=EDGE_CURVE ( 'NONE', #36844, #44871, #25061, .T. ) ;
#37541=CARTESIAN_POINT ( 'NONE',  ( -0.4330708661417315697, 0.2952755905511811885, 0.000000000000000000 ) ) ;
#37542=CARTESIAN_POINT ( 'NONE',  ( 1.620734908136483465, -0.6692913385826771977, 0.1292274648535927661 ) ) ;
#37543=FACE_OUTER_BOUND ( 'NONE', #67605, .T. ) ;
#37544=ORIENTED_EDGE ( 'NONE', *, *, #44425, .F. ) ;
#37546=CARTESIAN_POINT ( 'NONE',  ( 0.5249343832021005074, -0.6046776061558807314, 0.2411417322834647770 ) ) ;
#37548=CARTESIAN_POINT ( 'NONE',  ( -0.5446194225721777693, -0.3162353388693409650, -0.4822834645669289433 ) ) ;
#37549=CARTESIAN_POINT ( 'NONE',  ( -1.646981627296586703, -0.05778040916215522460, 0.4822834645669289988 ) ) ;
#37550=CARTESIAN_POINT ( 'NONE',  ( 0.6955380577427828781, 0.05413385826771626580, -0.4176697321401330321 ) ) ;
#37552=CARTESIAN_POINT ( 'NONE',  ( -0.006561679790025524116, -0.05778040916215560624, -0.4822834645669293319 ) ) ;
#37554=CARTESIAN_POINT ( 'NONE',  ( -0.9448818897637790704, -0.1870078740157479769, 0.4822834645669291653 ) ) ;
#37555=CARTESIAN_POINT ( 'NONE',  ( 0.3937007874015754361, -0.1870078740157479769, 0.4822834645669291653 ) ) ;
#37556=CARTESIAN_POINT ( 'NONE',  ( -0.5511811023622038563, -0.1870078740157479769, 0.4822834645669291653 ) ) ;
#37557=CARTESIAN_POINT ( 'NONE',  ( 0.2690288713910767848, 0.1771653543307087630, 0.09757992244046791164 ) ) ;
#37559=CARTESIAN_POINT ( 'NONE',  ( -0.1902887139107604098, -0.6692913385826771977, 0.1292274648535927661 ) ) ;
#37561=CARTESIAN_POINT ( 'NONE',  ( 1.489501312335958172, -0.05778040916215560624, -0.4822834645669293319 ) ) ;
#37564=ORIENTED_EDGE ( 'NONE', *, *, #28626, .F. ) ;
#37565=CARTESIAN_POINT ( 'NONE',  ( 0.8202099737532814183, -0.6692913385826773087, -0.1292274648535924053 ) ) ;
#37566=CARTESIAN_POINT ( 'NONE',  ( 0.1246719160104994284, -0.5511811023622046335, 0.09757992244046803654 ) ) ;
#37567=CARTESIAN_POINT ( 'NONE',  ( 1.509186351706037543, -0.004921259842519576551, 0.3153832671262227771 ) ) ;
#37568=CARTESIAN_POINT ( 'NONE',  ( -0.06873123812452887338, -2.191421614605370878E-15, 0.4445507791589071167 ) ) ;
#37572=B_SPLINE_CURVE_WITH_KNOTS ( 'NONE', 3,
 ( #21591, #8972, #67460, #34646, #3068, #53567, #80107 ),
 .UNSPECIFIED., .F., .F.,
 ( 4, 3, 4 ),
 ( 7.703719777548943412E-34, 0.001246232571205258119, 0.002492492258783253305 ),
 .UNSPECIFIED. ) ;
#37574=CARTESIAN_POINT ( 'NONE',  ( 0.2887139107611556010, -0.6046776061558807314, 0.2411417322834647770 ) ) ;
#37575=CARTESIAN_POINT ( 'NONE',  ( -1.423884514435694859, -0.05778040916215560624, -0.4822834645669293319 ) ) ;
#37576=CARTESIAN_POINT ( 'NONE',  ( -1.332020997375327642, -0.3162353388693409650, -0.4822834645669289433 ) ) ;
#37577=CARTESIAN_POINT ( 'NONE',  ( 0.1706036745406830368, 0.05413385826771666132, 0.4176697321401328100 ) ) ;
#37578=CARTESIAN_POINT ( 'NONE',  ( 0.9711286089238851948, 0.2306618581243848609, 0.2411417322834645549 ) ) ;
#37579=CARTESIAN_POINT ( 'NONE',  ( 1.528871391076116026, 0.1771653543307087630, 0.09757992244046791164 ) ) ;
#37580=CARTESIAN_POINT ( 'NONE',  ( 0.7480314960629927956, 0.1771653543307087630, 0.000000000000000000 ) ) ;
#37581=CARTESIAN_POINT ( 'NONE',  ( -1.023622047244093558, -0.1870078740157479769, 0.4822834645669291653 ) ) ;
#37583=CARTESIAN_POINT ( 'NONE',  ( 1.561679790026247350, 0.05413385826771626580, -0.4176697321401330321 ) ) ;
#37585=CARTESIAN_POINT ( 'NONE',  ( 1.318897637795276356, -0.5400638737290844871, 0.3530559997133364547 ) ) ;
#37587=CARTESIAN_POINT ( 'NONE',  ( -1.633858267716534529, -0.4536011799217368745, -0.2665933059059886201 ) ) ;
#37588=CARTESIAN_POINT ( 'NONE',  ( 0.09842519685039434474, 0.1660481256975885056, 0.3530559997133364547 ) ) ;
#37589=CARTESIAN_POINT ( 'NONE',  ( 0.8923884514435701520, -0.5023911411419708095, -0.1820866141732282451 ) ) ;
#37590=CARTESIAN_POINT ( 'NONE',  ( -1.509186351706035767, -0.004921259842519870586, -0.3153832671262229437 ) ) ;
#37591=CARTESIAN_POINT ( 'NONE',  ( 0.8792650918635177559, 0.05413385826771666132, 0.4176697321401328100 ) ) ;
#37593=CARTESIAN_POINT ( 'NONE',  ( -0.4527559055118102749, 0.07958543189024085140, 0.2665933059059887866 ) ) ;
#37594=CARTESIAN_POINT ( 'NONE',  ( -0.4133858267716528645, 0.1660481256975883668, -0.3530559997133364547 ) ) ;
#37595=CARTESIAN_POINT ( 'NONE',  ( 1.437007874015748810, -0.5400638737290845981, -0.3530559997133363437 ) ) ;
#37596=CARTESIAN_POINT ( 'NONE',  ( -1.174540682414697335, -0.3162353388693409650, -0.4822834645669289433 ) ) ;
#37597=CARTESIAN_POINT ( 'NONE',  ( 1.489501312335958172, -0.3162353388693405765, 0.4822834645669290543 ) ) ;
#37599=CARTESIAN_POINT ( 'NONE',  ( -1.161417322834644716, 0.07958543189024085140, 0.2665933059059887866 ) ) ;
#37602=CARTESIAN_POINT ( 'NONE',  ( 0.8005249343832027131, 0.05413385826771666132, 0.4176697321401328100 ) ) ;
#37604=CARTESIAN_POINT ( 'NONE',  ( -1.509186351706035767, 0.05413385826771626580, -0.4176697321401330321 ) ) ;
#37605=CARTESIAN_POINT ( 'NONE',  ( -1.607611548556429737, 0.1771653543307087075, -0.09757992244046823083 ) ) ;
#37606=CARTESIAN_POINT ( 'NONE',  ( -0.9317585301837263412, -0.004921259842519576551, 0.3153832671262227771 ) ) ;
#37607=CARTESIAN_POINT ( 'NONE',  ( 1.614173228346457378, -0.5511811023622047445, 6.969142054262312111E-17 ) ) ;
#37608=CARTESIAN_POINT ( 'NONE',  ( -0.3937007874015740483, -0.1870078740157479769, 0.4822834645669291653 ) ) ;
#37609=CARTESIAN_POINT ( 'NONE',  ( 0.1509186351706045259, -0.08942795157528024563, -0.3641732283464568787 ) ) ;
#37610=CARTESIAN_POINT ( 'NONE',  ( -1.443569553805773564, -0.5023911411419708095, 0.1820866141732285504 ) ) ;
#37611=CARTESIAN_POINT ( 'NONE',  ( 1.318897637795276356, 0.07958543189024071263, -0.2665933059059888421 ) ) ;
#37612=CARTESIAN_POINT ( 'NONE',  ( 1.010498687664042716, -0.4281496062992124485, 0.4176697321401328655 ) ) ;
#37613=CARTESIAN_POINT ( 'NONE',  ( 1.410761154855643795, -0.3162353388693405765, 0.4822834645669290543 ) ) ;
#37614=CARTESIAN_POINT ( 'NONE',  ( 0.2296587926509192634, -0.2845877964562159024, 0.3641732283464567677 ) ) ;
#37616=CARTESIAN_POINT ( 'NONE',  ( 0.3018372703412079971, 0.05413385826771626580, -0.4176697321401330321 ) ) ;
#37617=CARTESIAN_POINT ( 'NONE',  ( 1.056430446194226436, -0.5511811023622048555, -0.09757992244046775898 ) ) ;
#37619=CARTESIAN_POINT ( 'NONE',  ( 1.437007874015748810, 0.1660481256975885056, 0.3530559997133364547 ) ) ;
#37620=CARTESIAN_POINT ( 'NONE',  ( -1.404199475065615932, -0.4281496062992127816, -0.4176697321401328100 ) ) ;
#37621=CARTESIAN_POINT ( 'NONE',  ( -0.3018372703412066094, 0.05413385826771666132, 0.4176697321401328100 ) ) ;
#37624=CARTESIAN_POINT ( 'NONE',  ( 0.4068241469816279987, -0.4281496062992127816, -0.4176697321401328100 ) ) ;
#37625=CARTESIAN_POINT ( 'NONE',  ( 1.076115485564305141, -0.5023911411419708095, 0.1820866141732285504 ) ) ;
#37626=CARTESIAN_POINT ( 'NONE',  ( -0.006561679790025524116, -0.05778040916215560624, -0.4822834645669293319 ) ) ;
#37627=CARTESIAN_POINT ( 'NONE',  ( 0.1706036745406830368, 0.05413385826771666132, 0.4176697321401328100 ) ) ;
#37633=CARTESIAN_POINT ( 'NONE',  ( -0.5774278215223089816, 0.1283753931104746893, -0.1820866141732285504 ) ) ;
#37634=CARTESIAN_POINT ( 'NONE',  ( -0.9514435695538050464, -0.3162353388693405765, 0.4822834645669290543 ) ) ;
#37636=CARTESIAN_POINT ( 'NONE',  ( 0.8202099737532814183, -0.6692913385826773087, -0.1292274648535924053 ) ) ;
#37637=CARTESIAN_POINT ( 'NONE',  ( -1.601049868766403650, 0.2306618581243847221, -0.2411417322834647770 ) ) ;
#37638=CARTESIAN_POINT ( 'NONE',  ( 0.8595800524934390507, -0.05778040916215560624, -0.4822834645669293319 ) ) ;
#37642=CARTESIAN_POINT ( 'NONE',  ( 0.9842519685039375910, 0.2952755905511811885, 0.000000000000000000 ) ) ;
#37643=CARTESIAN_POINT ( 'NONE',  ( 0.7677165354330716118, -0.5400638737290844871, 0.3530559997133364547 ) ) ;
#37644=CARTESIAN_POINT ( 'NONE',  ( 0.7020997375328090762, -0.08942795157528024563, -0.3641732283464568787 ) ) ;
#37645=CARTESIAN_POINT ( 'NONE',  ( 1.463254593175853824, -0.6692913385826771977, 0.1292274648535927661 ) ) ;
#37648=CARTESIAN_POINT ( 'NONE',  ( 0.7217847769028878924, 0.05413385826771666132, 0.4176697321401328100 ) ) ;
#37649=CARTESIAN_POINT ( 'NONE',  ( 1.574803149606299746, -0.1870078740157480601, -0.3641732283464567677 ) ) ;
#37650=CARTESIAN_POINT ( 'NONE',  ( -0.5183727034120726440, -0.6692913385826773087, -0.1292274648535924053 ) ) ;
#37651=CARTESIAN_POINT ( 'NONE',  ( -1.003937007874015297, -0.5400638737290845981, -0.3530559997133363437 ) ) ;
#37652=CARTESIAN_POINT ( 'NONE',  ( 1.292650918635171564, 0.2952755905511811885, 0.1292274648535926551 ) ) ;
#37656=CARTESIAN_POINT ( 'NONE',  ( 1.351706036745407680, 0.05413385826771666132, 0.4176697321401328100 ) ) ;
#37661=CARTESIAN_POINT ( 'NONE',  ( 1.371391076115485719, -0.5511811023622048555, -0.09757992244046775898 ) ) ;
#37663=CARTESIAN_POINT ( 'NONE',  ( 1.384514435695538559, 0.1771653543307087075, -0.09757992244046823083 ) ) ;
#37668=CARTESIAN_POINT ( 'NONE',  ( -0.7677165354330699465, -0.4536011799217368745, -0.2665933059059886201 ) ) ;
#37670=CARTESIAN_POINT ( 'NONE',  ( -1.397637795275589623, 0.07958543189024085140, 0.2665933059059887866 ) ) ;
#37671=CARTESIAN_POINT ( 'NONE',  ( -1.292650918635170010, 0.2952755905511810774, -0.1292274648535930714 ) ) ;
#37672=CARTESIAN_POINT ( 'NONE',  ( 0.09186351706036799403, -0.4281496062992127816, -0.4176697321401328100 ) ) ;
#37673=CARTESIAN_POINT ( 'NONE',  ( 1.450131233595801428, 0.2952755905511811885, 0.1292274648535926551 ) ) ;
#37674=EDGE_LOOP ( 'NONE', ( #13720, #67103, #4852, #44480 ) ) ;
#37675=EDGE_CURVE ( 'NONE', #59607, #41772, #42240, .T. ) ;
#37676=CARTESIAN_POINT ( 'NONE',  ( 1.338582677165355062, -0.1870078740157480879, -0.4822834645669291653 ) ) ;
#37677=CARTESIAN_POINT ( 'NONE',  ( -1.154855643044618629, 0.1539470093639523085, 0.1968503937007873850 ) ) ;
#37678=SHAPE_REPRESENTATION_RELATIONSHIP ( 'NONE' , 'NONE' ,  #48103, #60502 ) ;
#37681=CARTESIAN_POINT ( 'NONE',  ( -0.3608923884514428360, 0.1771653543307087630, 0.09757992244046791164 ) ) ;
#37683=CARTESIAN_POINT ( 'NONE',  ( -1.364829396325458521, -0.6046776061558807314, 0.2411417322834647770 ) ) ;
#37684=CARTESIAN_POINT ( 'NONE',  ( 0.8989501312335964611, 0.2952755905511811885, 0.1292274648535926551 ) ) ;
#37686=CARTESIAN_POINT ( 'NONE',  ( 0.7677165354330716118, 0.1660481256975883391, -0.3530559997133364547 ) ) ;
#37688=CARTESIAN_POINT ( 'NONE',  ( 1.108923884514436686, -0.3162353388693409650, -0.4822834645669289433 ) ) ;
#37689=CARTESIAN_POINT ( 'NONE',  ( -1.108923884514435132, -0.3162353388693405765, 0.4822834645669290543 ) ) ;
#37691=CARTESIAN_POINT ( 'NONE',  ( -0.1771653543307080136, -0.4536011799217367080, 0.2665933059059888421 ) ) ;
#37693=CARTESIAN_POINT ( 'NONE',  ( -0.6692913385826764205, 0.1771653543307087630, 0.000000000000000000 ) ) ;
#37694=CARTESIAN_POINT ( 'NONE',  ( 0.6955380577427828781, -0.004921259842519870586, -0.3153832671262229437 ) ) ;
#37695=CARTESIAN_POINT ( 'NONE',  ( 0.04593175853018440641, 0.2952755905511810774, -0.1292274648535930714 ) ) ;
#37696=CARTESIAN_POINT ( 'NONE',  ( -0.5380577427821514602, -0.004921259842519576551, 0.3153832671262227771 ) ) ;
#37698=CARTESIAN_POINT ( 'NONE',  ( 1.240157480314961314, -0.5400638737290844871, 0.3530559997133364547 ) ) ;
#37699=EDGE_CURVE ( 'NONE', #38952, #24575, #26033, .T. ) ;
#37700=EDGE_CURVE ( 'NONE', #13300, #71398, #9244, .T. ) ;
#37701=CARTESIAN_POINT ( 'NONE',  ( -0.8595800524934373854, -0.05778040916215522460, 0.4822834645669289988 ) ) ;
#37703=CARTESIAN_POINT ( 'NONE',  ( -0.4330708661417315697, 0.2952755905511811885, 0.000000000000000000 ) ) ;
#37704=CARTESIAN_POINT ( 'NONE',  ( -1.122047244094487306, 0.1660481256975883668, -0.3530559997133364547 ) ) ;
#37705=CARTESIAN_POINT ( 'NONE',  ( 1.108923884514436686, -0.2845877964562161244, -0.3641732283464567121 ) ) ;
#37706=CARTESIAN_POINT ( 'NONE',  ( 0.1771653543307093182, 0.07958543189024085140, 0.2665933059059887866 ) ) ;
#37707=CARTESIAN_POINT ( 'NONE',  ( -0.4330708661417315697, 0.2952755905511811885, 0.000000000000000000 ) ) ;
#37708=CARTESIAN_POINT ( 'NONE',  ( -1.233595800524933894, -0.6046776061558809534, -0.2411417322834644161 ) ) ;
#37710=CARTESIAN_POINT ( 'NONE',  ( 1.627296587926509996, -0.5023911411419708095, 0.1820866141732285504 ) ) ;
#37711=CARTESIAN_POINT ( 'NONE',  ( -0.3674540682414689785, 0.2306618581243848609, 0.2411417322834645549 ) ) ;
#37712=CARTESIAN_POINT ( 'NONE',  ( -1.076115485564303809, 0.2306618581243848609, 0.2411417322834645549 ) ) ;
#37713=VERTEX_POINT ( 'NONE', #76977 ) ;
#37715=CARTESIAN_POINT ( 'NONE',  ( 1.010498687664042716, 0.05413385826771626580, -0.4176697321401330321 ) ) ;
#37716=CARTESIAN_POINT ( 'NONE',  ( -0.6496062992125976043, -0.4536011799217367080, 0.2665933059059888421 ) ) ;
#37718=CARTESIAN_POINT ( 'NONE',  ( -0.8333333333333323711, -0.6692913385826773087, -0.1292274648535924053 ) ) ;
#37719=CARTESIAN_POINT ( 'NONE',  ( 1.292650918635171564, -0.6692913385826773087, -0.1292274648535924053 ) ) ;
#37720=CARTESIAN_POINT ( 'NONE',  ( 0.9251968503937015864, 0.1660481256975883668, -0.3530559997133364547 ) ) ;
#37722=CARTESIAN_POINT ( 'NONE',  ( -1.246719160104986512, -0.004921259842519576551, 0.3153832671262227771 ) ) ;
#37727=CARTESIAN_POINT ( 'NONE',  ( 1.069553805774278832, 0.1771653543307087075, -0.09757992244046823083 ) ) ;
#37728=CARTESIAN_POINT ( 'NONE',  ( 0.9186351706036751663, -0.5023911411419708095, 0.1820866141732285504 ) ) ;
#37730=CARTESIAN_POINT ( 'NONE',  ( 0.5314960629921264834, 0.1660481256975883668, -0.3530559997133364547 ) ) ;
#37731=CARTESIAN_POINT ( 'NONE',  ( 1.574803149606299746, -0.1870078740157479769, 0.4822834645669291653 ) ) ;
#37733=CARTESIAN_POINT ( 'NONE',  ( 0.7480314960629927956, 0.1771653543307087630, 0.000000000000000000 ) ) ;
#37734=CARTESIAN_POINT ( 'NONE',  ( -0.2559055118110227234, -0.5400638737290844871, 0.3530559997133364547 ) ) ;
#37735=CARTESIAN_POINT ( 'NONE',  ( -1.076115485564303809, -0.6046776061558809534, -0.2411417322834644161 ) ) ;
#37736=CARTESIAN_POINT ( 'NONE',  ( 1.358267716535433323, 0.1660481256975885056, 0.3530559997133364547 ) ) ;
#37739=CARTESIAN_POINT ( 'NONE',  ( -0.1968503937007867743, -0.5511811023622047445, 6.969142054262312111E-17 ) ) ;
#37742=CARTESIAN_POINT ( 'NONE',  ( -0.6692913385826764205, -0.6692913385826771977, 8.415575281601705876E-17 ) ) ;
#37743=CARTESIAN_POINT ( 'NONE',  ( -0.5839895013123351797, -0.6692913385826771977, 0.1292274648535927661 ) ) ;
#37744=CARTESIAN_POINT ( 'NONE',  ( -0.7086614173228339419, -0.1870078740157479769, 0.4822834645669291653 ) ) ;
#37745=CARTESIAN_POINT ( 'NONE',  ( 0.3477690288713918276, -0.6692913385826773087, -0.1292274648535924053 ) ) ;
#37746=CARTESIAN_POINT ( 'NONE',  ( -0.4986876640419939388, 0.2306618581243847221, -0.2411417322834647770 ) ) ;
#37747=CARTESIAN_POINT ( 'NONE',  ( -1.312335958005248715, 0.2306618581243848609, 0.2411417322834645549 ) ) ;
#37749=CARTESIAN_POINT ( 'NONE',  ( -0.8661417322834640276, -0.1870078740157480879, -0.4822834645669291653 ) ) ;
#37750=CARTESIAN_POINT ( 'NONE',  ( 0.6824146981627303710, 0.2306618581243847221, -0.2411417322834647770 ) ) ;
#37751=EDGE_CURVE ( 'NONE', #19878, #36616, #31938, .T. ) ;
#37753=CARTESIAN_POINT ( 'NONE',  ( -0.4658792650918627265, -0.2845877964562161244, -0.3641732283464567121 ) ) ;
#37757=CARTESIAN_POINT ( 'NONE',  ( -1.384514435695537005, 0.1771653543307087630, 0.09757992244046791164 ) ) ;
#37758=CARTESIAN_POINT ( 'NONE',  ( -1.233595800524933894, -0.6046776061558809534, -0.2411417322834644161 ) ) ;
#37759=CARTESIAN_POINT ( 'NONE',  ( -1.062992125984250968, -0.6692913385826771977, 8.415575281601705876E-17 ) ) ;
#37761=CARTESIAN_POINT ( 'NONE',  ( -1.318897637795274802, -0.5400638737290845981, -0.3530559997133363437 ) ) ;
#37762=CARTESIAN_POINT ( 'NONE',  ( -0.9842519685039365918, -0.6692913385826771977, 8.415575281601705876E-17 ) ) ;
#37764=CARTESIAN_POINT ( 'NONE',  ( -1.679790026246718693, 0.2306618581243847221, -0.2411417322834647770 ) ) ;
#37765=CARTESIAN_POINT ( 'NONE',  ( 0.3740157480314966754, -0.4536011799217367080, 0.2665933059059888421 ) ) ;
#37766=CARTESIAN_POINT ( 'NONE',  ( -1.646051170424378096, 0.000000000000000000, 0.3464511005275205946 ) ) ;
#37768=CARTESIAN_POINT ( 'NONE',  ( -0.1115485564304456306, 0.1771653543307087075, -0.09757992244046823083 ) ) ;
#37769=CARTESIAN_POINT ( 'NONE',  ( -0.5380577427821514602, 0.05413385826771666132, 0.4176697321401328100 ) ) ;
#37770=CARTESIAN_POINT ( 'NONE',  ( 1.541994750656168645, -0.6692913385826771977, 0.1292274648535927661 ) ) ;
#37771=CARTESIAN_POINT ( 'NONE',  ( -0.4396325459317577122, -0.6692913385826773087, -0.1292274648535924053 ) ) ;
#37774=LINE ( 'NONE', #31455, #56015 ) ;
#37777=CARTESIAN_POINT ( 'NONE',  ( -0.4986876640419939388, 0.2306618581243847221, -0.2411417322834647770 ) ) ;
#37778=CARTESIAN_POINT ( 'NONE',  ( 1.509186351706037543, -0.4281496062992127816, -0.4176697321401328100 ) ) ;
#37779=CARTESIAN_POINT ( 'NONE',  ( -1.030183727034119867, -0.08942795157528024563, -0.3641732283464568787 ) ) ;
#37780=CARTESIAN_POINT ( 'NONE',  ( -1.364829396325458521, 0.2306618581243847221, -0.2411417322834647770 ) ) ;
#37782=CARTESIAN_POINT ( 'NONE',  ( 0.4847769261806181285, 1.968503937007873850, -0.4915354330708656128 ) ) ;
#37784=CARTESIAN_POINT ( 'NONE',  ( 1.135170603674541256, -0.6692913385826773087, -0.1292274648535924053 ) ) ;
#37785=CARTESIAN_POINT ( 'NONE',  ( 1.220472440944881942, 0.8346805926620878280, -0.5309055118110238558 ) ) ;
#37786=CARTESIAN_POINT ( 'NONE',  ( 0.2427821522309719648, -0.05778040916215522460, 0.4822834645669289988 ) ) ;
#37787=CARTESIAN_POINT ( 'NONE',  ( -1.089238845144356427, -0.3690944881889765550, -0.3153832671262227771 ) ) ;
#37788=CARTESIAN_POINT ( 'NONE',  ( -0.3215223097112853146, -0.3162353388693405765, 0.4822834645669290543 ) ) ;
#37790=CARTESIAN_POINT ( 'NONE',  ( -0.9251968503937002541, 0.1660481256975885056, 0.3530559997133364547 ) ) ;
#37792=CARTESIAN_POINT ( 'NONE',  ( 0.6955380577427828781, -0.004921259842519870586, -0.3153832671262229437 ) ) ;
#37793=CARTESIAN_POINT ( 'NONE',  ( -0.3018372703412066094, -0.004921259842519576551, 0.3153832671262227771 ) ) ;
#37794=CARTESIAN_POINT ( 'NONE',  ( 0.7611548556430454138, 0.1283753931104746893, -0.1820866141732285504 ) ) ;
#37795=CARTESIAN_POINT ( 'NONE',  ( -1.430446194225721390, -0.4281496062992124485, 0.4176697321401328655 ) ) ;
#37798=CARTESIAN_POINT ( 'NONE',  ( 0.7283464566929143125, 0.07958543189024085140, 0.2665933059059887866 ) ) ;
#37799=CARTESIAN_POINT ( 'NONE',  ( -0.9580052493438311334, 0.05413385826771626580, -0.4176697321401330321 ) ) ;
#37800=CARTESIAN_POINT ( 'NONE',  ( 1.377952755905512472, -0.6692913385826771977, 8.415575281601705876E-17 ) ) ;
#37802=CARTESIAN_POINT ( 'NONE',  ( -0.08530183727034056085, -0.2845877964562159024, 0.3641732283464567677 ) ) ;
#37804=CARTESIAN_POINT ( 'NONE',  ( 0.5446194225721792126, -0.3162353388693405765, 0.4822834645669290543 ) ) ;
#37806=CARTESIAN_POINT ( 'NONE',  ( 1.358267716535433323, -0.4536011799217368745, -0.2665933059059886201 ) ) ;
#37807=CARTESIAN_POINT ( 'NONE',  ( -1.227034120734907585, 0.2952755905511811885, 0.1292274648535926551 ) ) ;
#37808=CARTESIAN_POINT ( 'NONE',  ( -0.4396325459317577122, -0.5511811023622048555, -0.09757992244046775898 ) ) ;
#37810=CARTESIAN_POINT ( 'NONE',  ( 0.4265091863517067039, -0.5511811023622048555, -0.09757992244046775898 ) ) ;
#37812=CARTESIAN_POINT ( 'NONE',  ( -0.9645669291338575535, -0.5400638737290844871, 0.3530559997133364547 ) ) ;
#37813=CARTESIAN_POINT ( 'NONE',  ( -0.3083989501312330295, -0.3162353388693409650, -0.4822834645669289433 ) ) ;
#37816=CARTESIAN_POINT ( 'NONE',  ( 0.8202099737532813073, 0.1771653543307087630, 0.09757992244046791164 ) ) ;
#37817=CARTESIAN_POINT ( 'NONE',  ( -0.4986876640419939388, 0.2306618581243847221, -0.2411417322834647770 ) ) ;
#37818=CARTESIAN_POINT ( 'NONE',  ( -0.8333333333333323711, 0.2952755905511811885, 0.1292274648535926551 ) ) ;
#37819=CARTESIAN_POINT ( 'NONE',  ( -0.8136482939632537770, 0.1283753931104746893, -0.1820866141732285504 ) ) ;
#37821=CARTESIAN_POINT ( 'NONE',  ( -0.09186351706036663400, -0.4281496062992124485, 0.4176697321401328655 ) ) ;
#37822=EDGE_CURVE ( 'NONE', #82322, #47058, #44139, .T. ) ;
#37823=CARTESIAN_POINT ( 'NONE',  ( -1.463254593175852492, -0.5511811023622048555, -0.09757992244046775898 ) ) ;
#37824=CARTESIAN_POINT ( 'NONE',  ( 1.102362204724410155, -0.1870078740157479769, 0.4822834645669291653 ) ) ;
#37825=DIRECTION ( 'NONE',  ( -3.096699300667737957E-16, 1.000000000000000000, -0.000000000000000000 ) ) ;
#37827=ORIENTED_EDGE ( 'NONE', *, *, #49490, .F. ) ;
#37828=EDGE_CURVE ( 'NONE', #41807, #57855, #31104, .T. ) ;
#37830=CARTESIAN_POINT ( 'NONE',  ( -1.253280839895012377, -0.05778040916215522460, 0.4822834645669289988 ) ) ;
#37831=CARTESIAN_POINT ( 'NONE',  ( -0.7480314960629914633, 0.2952755905511811885, 0.000000000000000000 ) ) ;
#37832=CARTESIAN_POINT ( 'NONE',  ( 1.476377952755906220, 0.1660481256975883668, -0.3530559997133364547 ) ) ;
#37835=CARTESIAN_POINT ( 'NONE',  ( 0.8202099737532814183, -0.6692913385826773087, -0.1292274648535924053 ) ) ;
#37836=CARTESIAN_POINT ( 'NONE',  ( 0.07874015748031558404, -0.1870078740157479769, 0.4822834645669291653 ) ) ;
#37838=CARTESIAN_POINT ( 'NONE',  ( -0.6627296587926501115, 0.2952755905511810219, -0.1292274648535930437 ) ) ;
#37839=CARTESIAN_POINT ( 'NONE',  ( 1.043307086614173818, -0.4536011799217368745, -0.2665933059059886201 ) ) ;
#37843=ORIENTED_EDGE ( 'NONE', *, *, #65705, .F. ) ;
#37844=CARTESIAN_POINT ( 'NONE',  ( 0.1968503937007881344, 0.2952755905511811885, 0.000000000000000000 ) ) ;
#37845=CARTESIAN_POINT ( 'NONE',  ( -0.8727034120734901146, -0.05778040916215560624, -0.4822834645669293319 ) ) ;
#37846=CARTESIAN_POINT ( 'NONE',  ( -1.640419947506561060, 0.05413385826771666132, 0.4176697321401328100 ) ) ;
#37847=CARTESIAN_POINT ( 'NONE',  ( 0.7742782152230979209, 0.05413385826771626580, -0.4176697321401330321 ) ) ;
#37848=CARTESIAN_POINT ( 'NONE',  ( 1.443569553805774897, -0.6046776061558809534, -0.2411417322834644161 ) ) ;
#37849=CARTESIAN_POINT ( 'NONE',  ( 1.515748031496063186, -0.5400638737290845981, -0.3530559997133363437 ) ) ;
#37850=CARTESIAN_POINT ( 'NONE',  ( -0.1837270341207340729, 0.2306618581243847221, -0.2411417322834647770 ) ) ;
#37851=CIRCLE ( 'NONE', #23080, 3.582677165354330562 ) ;
#37852=CARTESIAN_POINT ( 'NONE',  ( -1.456692913385826182, 0.2952755905511811885, 0.000000000000000000 ) ) ;
#37853=CARTESIAN_POINT ( 'NONE',  ( 1.614173228346457378, 0.2952755905511811885, 0.000000000000000000 ) ) ;
#37854=EDGE_CURVE ( 'NONE', #75665, #40053, #22125, .T. ) ;
#37855=CARTESIAN_POINT ( 'NONE',  ( 1.653543307086614789, -0.1870078740157479769, 0.4822834645669291653 ) ) ;
#37857=CARTESIAN_POINT ( 'NONE',  ( 0.9776902887139113929, -0.5511811023622048555, -0.09757992244046775898 ) ) ;
#37860=EDGE_LOOP ( 'NONE', ( #30288, #19331, #70138, #28986, #65300, #57699 ) ) ;
#37861=CARTESIAN_POINT ( 'NONE',  ( -0.2165354330708654795, -0.4536011799217368745, -0.2665933059059886201 ) ) ;
#37863=CARTESIAN_POINT ( 'NONE',  ( 5.463695987328526437E-16, -0.1870078740157479769, 0.4822834645669291653 ) ) ;
#37864=CARTESIAN_POINT ( 'NONE',  ( 0.4068241469816279987, -0.4281496062992127816, -0.4176697321401328100 ) ) ;
#37865=CARTESIAN_POINT ( 'NONE',  ( -0.6167979002624665030, 0.05413385826771666132, 0.4176697321401328100 ) ) ;
#37868=CARTESIAN_POINT ( 'NONE',  ( -1.017060367454067249, -0.05778040916215522460, 0.4822834645669289988 ) ) ;
#37870=CARTESIAN_POINT ( 'NONE',  ( 1.332020997375328974, -0.08942795157528024563, -0.3641732283464568787 ) ) ;
#37871=CARTESIAN_POINT ( 'NONE',  ( -1.266404199475064773, -0.05778040916215560624, -0.4822834645669293319 ) ) ;
#37872=CARTESIAN_POINT ( 'NONE',  ( 0.9120734908136490793, 0.2952755905511810774, -0.1292274648535930714 ) ) ;
#37873=CARTESIAN_POINT ( 'NONE',  ( 1.095800524934383846, -0.05778040916215560624, -0.4822834645669293319 ) ) ;
#37875=CARTESIAN_POINT ( 'NONE',  ( -1.161417322834644716, -0.5400638737290845981, -0.3530559997133363437 ) ) ;
#37878=CARTESIAN_POINT ( 'NONE',  ( -0.2755905511811018171, 0.2952755905511811885, 0.000000000000000000 ) ) ;
#37881=CARTESIAN_POINT ( 'NONE',  ( 1.312335958005249825, 0.2306618581243847221, -0.2411417322834647770 ) ) ;
#37882=CARTESIAN_POINT ( 'NONE',  ( 1.292650918635171564, -0.6692913385826773087, -0.1292274648535924053 ) ) ;
#37883=CARTESIAN_POINT ( 'NONE',  ( 0.02624671916010564918, -0.5023911411419708095, -0.1820866141732282451 ) ) ;
#37884=CARTESIAN_POINT ( 'NONE',  ( 0.9251968503937015864, -0.5400638737290844871, 0.3530559997133364547 ) ) ;
#37886=CARTESIAN_POINT ( 'NONE',  ( 0.4002624671916016896, -0.08942795157527998196, 0.3641732283464567121 ) ) ;
#37887=CARTESIAN_POINT ( 'NONE',  ( 0.2755905511811031494, -0.6692913385826771977, 8.415575281601705876E-17 ) ) ;
#37889=CARTESIAN_POINT ( 'NONE',  ( -0.9842519685039365918, -0.6692913385826771977, 8.415575281601705876E-17 ) ) ;
#37890=CARTESIAN_POINT ( 'NONE',  ( 0.9842519685039375910, 0.1771653543307087630, 0.000000000000000000 ) ) ;
#37891=CARTESIAN_POINT ( 'NONE',  ( 0.3812812444996376282, 2.409604939980833412E-17, -0.3464511005275205946 ) ) ;
#37892=CARTESIAN_POINT ( 'NONE',  ( -0.4133858267716528645, 0.1660481256975883668, -0.3530559997133364547 ) ) ;
#37893=CARTESIAN_POINT ( 'NONE',  ( 0.1312335958005257930, 0.1283753931104746893, -0.1820866141732285504 ) ) ;
#37895=CARTESIAN_POINT ( 'NONE',  ( -0.3018372703412066094, 0.05413385826771666132, 0.4176697321401328100 ) ) ;
#37896=CARTESIAN_POINT ( 'NONE',  ( 0.2690288713910767848, -0.5511811023622048555, -0.09757992244046775898 ) ) ;
#37898=CARTESIAN_POINT ( 'NONE',  ( 0.1640419947506569498, -0.3162353388693409650, -0.4822834645669289433 ) ) ;
#37899=CARTESIAN_POINT ( 'NONE',  ( 1.148293963254593875, -0.5511811023622046335, 0.09757992244046803654 ) ) ;
#37900=CARTESIAN_POINT ( 'NONE',  ( 0.3822046412494098377, 1.809133623825372073E-16, -0.3791483426435173776 ) ) ;
#37901=CARTESIAN_POINT ( 'NONE',  ( -0.2559055118110230564, 0.07958543189024071263, -0.2665933059059888421 ) ) ;
#37902=CARTESIAN_POINT ( 'NONE',  ( -0.7480314960629914633, 0.1771653543307087630, 0.000000000000000000 ) ) ;
#37903=CARTESIAN_POINT ( 'NONE',  ( -0.1640419947506553400, -0.05778040916215560624, -0.4822834645669293319 ) ) ;
#37904=CARTESIAN_POINT ( 'NONE',  ( -0.08530183727034056085, -0.05778040916215560624, -0.4822834645669293319 ) ) ;
#37905=CARTESIAN_POINT ( 'NONE',  ( 1.135170603674541256, -0.5511811023622048555, -0.09757992244046775898 ) ) ;
#37906=CARTESIAN_POINT ( 'NONE',  ( -1.646981627296586703, -0.2845877964562161244, -0.3641732283464567121 ) ) ;
#37907=CARTESIAN_POINT ( 'NONE',  ( -1.706036745406823485, 0.2306618581243848609, 0.2411417322834645549 ) ) ;
#37909=CARTESIAN_POINT ( 'NONE',  ( 0.6299212598425204535, -0.1870078740157480879, -0.4822834645669291653 ) ) ;
#37911=CARTESIAN_POINT ( 'NONE',  ( -0.1640419947506555343, -0.3162353388693405765, 0.4822834645669290543 ) ) ;
#37913=CARTESIAN_POINT ( 'NONE',  ( 0.9580052493438327987, -0.4281496062992127816, -0.4176697321401328100 ) ) ;
#37914=CARTESIAN_POINT ( 'NONE',  ( 0.6692913385826778638, -0.6692913385826771977, 8.415575281601705876E-17 ) ) ;
#37916=CARTESIAN_POINT ( 'NONE',  ( 0.4461942257217856311, 0.1283753931104746893, -0.1820866141732285504 ) ) ;
#37917=CARTESIAN_POINT ( 'NONE',  ( 1.089238845144357759, 0.05413385826771626580, -0.4176697321401330321 ) ) ;
#37919=CARTESIAN_POINT ( 'NONE',  ( -0.1574803149606292529, -0.1870078740157479769, 0.3641732283464567677 ) ) ;
#37920=CARTESIAN_POINT ( 'NONE',  ( -0.2230971128608915943, 0.05413385826771666132, 0.4176697321401328100 ) ) ;
#37921=CARTESIAN_POINT ( 'NONE',  ( 0.8267716535433077274, 0.2952755905511811885, 0.000000000000000000 ) ) ;
#37922=CARTESIAN_POINT ( 'NONE',  ( 0.4593175853018379162, -0.4281496062992124485, 0.4176697321401328655 ) ) ;
#37923=CARTESIAN_POINT ( 'NONE',  ( -0.7283464566929126471, -0.5400638737290844871, 0.3530559997133364547 ) ) ;
#37924=CARTESIAN_POINT ( 'NONE',  ( -0.8530183727034112984, -0.3690944881889765550, -0.3153832671262227771 ) ) ;
#37925=CARTESIAN_POINT ( 'NONE',  ( 0.4855643044619428750, 0.05413385826771666132, 0.4176697321401328100 ) ) ;
#37926=CARTESIAN_POINT ( 'NONE',  ( -1.397637795275589623, 0.1660481256975885056, 0.3530559997133364547 ) ) ;
#37927=CARTESIAN_POINT ( 'NONE',  ( -0.5380577427821514602, 0.05413385826771666132, 0.4176697321401328100 ) ) ;
#37928=CARTESIAN_POINT ( 'NONE',  ( 1.168682819302787168, 2.409604939980833412E-17, -0.3464511005275205946 ) ) ;
#37929=LINE ( 'NONE', #43402, #54015 ) ;
#37930=CARTESIAN_POINT ( 'NONE',  ( 1.463254593175853824, 0.2952755905511810774, -0.1292274648535930714 ) ) ;
#37931=CARTESIAN_POINT ( 'NONE',  ( 1.312335958005250269, -0.6046776061558807314, 0.2411417322834647770 ) ) ;
#37933=CARTESIAN_POINT ( 'NONE',  ( -1.522309711286088607, -0.6046776061558807314, 0.2411417322834647770 ) ) ;
#37934=CARTESIAN_POINT ( 'NONE',  ( -0.7677165354330699465, 0.1660481256975885056, 0.3530559997133364547 ) ) ;
#37938=CARTESIAN_POINT ( 'NONE',  ( -0.1640419947506553400, -0.08942795157528024563, -0.3641732283464568787 ) ) ;
#37940=CARTESIAN_POINT ( 'NONE',  ( 0.8595800524934390507, -0.05778040916215560624, -0.4822834645669293319 ) ) ;
#37942=DIRECTION ( 'NONE',  ( 1.000000000000000000, -0.000000000000000000, -0.000000000000000000 ) ) ;
#37943=CARTESIAN_POINT ( 'NONE',  ( -0.6430446194225712953, -0.004921259842519870586, -0.3153832671262229437 ) ) ;
#37945=CARTESIAN_POINT ( 'NONE',  ( 1.272965879265092637, -0.4281496062992127816, -0.4176697321401328100 ) ) ;
#37946=CARTESIAN_POINT ( 'NONE',  ( 0.7677165354330716118, -0.4536011799217367080, 0.2665933059059888421 ) ) ;
#37947=CARTESIAN_POINT ( 'NONE',  ( 0.2034120734908144990, -0.6692913385826771977, 0.1292274648535927661 ) ) ;
#37949=CARTESIAN_POINT ( 'NONE',  ( -0.4396325459317577122, -0.6692913385826773087, -0.1292274648535924053 ) ) ;
#37950=CARTESIAN_POINT ( 'NONE',  ( -1.430446194225721390, -0.3690944881889763329, 0.3153832671262228327 ) ) ;
#37951=CARTESIAN_POINT ( 'NONE',  ( -0.3215223097112853146, -0.3162353388693405765, 0.4822834645669290543 ) ) ;
#37952=CARTESIAN_POINT ( 'NONE',  ( 1.594488188976378673, -0.5400638737290845981, -0.3530559997133363437 ) ) ;
#37956=CARTESIAN_POINT ( 'NONE',  ( 0.3543307086614181922, -0.6692913385826771977, 8.415575281601705876E-17 ) ) ;
#37957=ORIENTED_EDGE ( 'NONE', *, *, #24432, .F. ) ;
#37958=CARTESIAN_POINT ( 'NONE',  ( -0.8333333333333323711, -0.6692913385826773087, -0.1292274648535924053 ) ) ;
#37959=CARTESIAN_POINT ( 'NONE',  ( -1.482939632545930975, 0.05413385826771666132, 0.4176697321401328100 ) ) ;
#37960=CARTESIAN_POINT ( 'NONE',  ( 0.7480314960629927956, -0.6692913385826771977, 8.415575281601705876E-17 ) ) ;
#37962=CARTESIAN_POINT ( 'NONE',  ( 0.07874015748031558404, -0.1870078740157479769, 0.4822834645669291653 ) ) ;
#37964=CARTESIAN_POINT ( 'NONE',  ( -0.7480314960629914633, 0.2952755905511811885, 0.000000000000000000 ) ) ;
#37965=CARTESIAN_POINT ( 'NONE',  ( -0.06561679790026180015, 0.05413385826771666132, 0.4176697321401328100 ) ) ;
#37966=CARTESIAN_POINT ( 'NONE',  ( -1.030183727034119867, -0.3162353388693405765, 0.4822834645669290543 ) ) ;
#37967=CARTESIAN_POINT ( 'NONE',  ( -0.06561679790026180015, -0.004921259842519576551, 0.3153832671262227771 ) ) ;
#37969=CARTESIAN_POINT ( 'NONE',  ( 0.1049868766404206816, -0.6046776061558809534, -0.2411417322834644161 ) ) ;
#37970=AXIS2_PLACEMENT_3D ( 'NONE', #55763, #37249, #50275 ) ;
#37972=CARTESIAN_POINT ( 'NONE',  ( 1.102362204724410155, -0.1870078740157479769, 0.4822834645669291653 ) ) ;
#37974=VERTEX_POINT ( 'NONE', #26874 ) ;
#37976=CARTESIAN_POINT ( 'NONE',  ( 0.2624671916010504757, 0.2306618581243848609, 0.2411417322834645549 ) ) ;
#37977=CARTESIAN_POINT ( 'NONE',  ( 0.2952755905511816326, -0.4536011799217367080, 0.2665933059059888421 ) ) ;
#37978=CARTESIAN_POINT ( 'NONE',  ( 1.430446194225722500, -0.3690944881889765550, -0.3153832671262227771 ) ) ;
#37982=CARTESIAN_POINT ( 'NONE',  ( 1.502624671916010790, -0.08942795157527998196, 0.3641732283464567121 ) ) ;
#37983=CARTESIAN_POINT ( 'NONE',  ( -1.640419947506561060, 0.05413385826771666132, 0.4176697321401328100 ) ) ;
#37985=CARTESIAN_POINT ( 'NONE',  ( 0.5183727034120741983, 0.2952755905511810774, -0.1292274648535930714 ) ) ;
#37986=CARTESIAN_POINT ( 'NONE',  ( -1.141732283464566011, 0.2952755905511811885, 0.000000000000000000 ) ) ;
#37987=CARTESIAN_POINT ( 'NONE',  ( -1.115485564304461219, -0.4281496062992124485, 0.4176697321401328655 ) ) ;
#37988=CARTESIAN_POINT ( 'NONE',  ( 0.3477690288713918276, 0.2952755905511811885, 0.1292274648535926551 ) ) ;
#37989=CARTESIAN_POINT ( 'NONE',  ( 0.8005249343832027131, 0.05413385826771666132, 0.4176697321401328100 ) ) ;
#37990=CARTESIAN_POINT ( 'NONE',  ( 1.338582677165355062, -0.1870078740157479769, 0.3641732283464567677 ) ) ;
#37991=CARTESIAN_POINT ( 'NONE',  ( 1.010498687664042716, -0.3690944881889763329, 0.3153832671262228327 ) ) ;
#37992=CARTESIAN_POINT ( 'NONE',  ( -0.9251968503937002541, -0.5400638737290845981, -0.3530559997133363437 ) ) ;
#37994=CARTESIAN_POINT ( 'NONE',  ( -1.574803149606298192, -0.1870078740157480601, -0.3641732283464567677 ) ) ;
#37996=CARTESIAN_POINT ( 'NONE',  ( 0.9317585301837276734, 0.05413385826771626580, -0.4176697321401330321 ) ) ;
#37998=CARTESIAN_POINT ( 'NONE',  ( -1.515748031496062076, 0.07958543189024071263, -0.2665933059059888421 ) ) ;
#37999=CARTESIAN_POINT ( 'NONE',  ( -0.05905511811023545637, 0.1660481256975885056, 0.3530559997133364547 ) ) ;
#38000=CARTESIAN_POINT ( 'NONE',  ( 0.9908136482939640111, 0.1771653543307087075, -0.09757992244046823083 ) ) ;
#38001=CARTESIAN_POINT ( 'NONE',  ( -1.679790026246718693, 0.1283753931104746893, -0.1820866141732285504 ) ) ;
#38002=CARTESIAN_POINT ( 'NONE',  ( 1.141732283464567788, -0.6692913385826771977, 8.415575281601705876E-17 ) ) ;
#38003=CARTESIAN_POINT ( 'NONE',  ( -0.4855643044619415427, 0.05413385826771626580, -0.4176697321401330321 ) ) ;
#38004=CARTESIAN_POINT ( 'NONE',  ( -0.6496062992125976043, -0.4536011799217367080, 0.2665933059059888421 ) ) ;
#38005=CARTESIAN_POINT ( 'NONE',  ( -0.6496062992125976043, -0.5400638737290844871, 0.3530559997133364547 ) ) ;
#38006=CARTESIAN_POINT ( 'NONE',  ( 1.640419947506562393, -0.4281496062992124485, 0.4176697321401328655 ) ) ;
#38007=CARTESIAN_POINT ( 'NONE',  ( -1.305774278215222184, -0.6692913385826773087, -0.1292274648535924053 ) ) ;
#38008=CARTESIAN_POINT ( 'NONE',  ( 1.574803149606299746, -0.1870078740157480879, -0.4822834645669291653 ) ) ;
#38010=CARTESIAN_POINT ( 'NONE',  ( -1.430446194225720724, -0.004921259842519870586, -0.3153832671262229437 ) ) ;
#38011=EDGE_CURVE ( 'NONE', #10560, #14996, #45273, .T. ) ;
#38013=B_SPLINE_CURVE_WITH_KNOTS ( 'NONE', 3,
 ( #1663, #45415, #13454, #39964, #33644, #46677, #19341 ),
 .UNSPECIFIED., .F., .F.,
 ( 4, 3, 4 ),
 ( 1.388456241783856658E-17, 0.001246230184515585400, 0.002492489877932651567 ),
 .UNSPECIFIED. ) ;
#38014=CARTESIAN_POINT ( 'NONE',  ( 1.148293963254593653, 0.2952755905511810774, -0.1292274648535930714 ) ) ;
#38016=CARTESIAN_POINT ( 'NONE',  ( -1.712598425196849572, 0.1660481256975885056, 0.3530559997133364547 ) ) ;
#38017=CARTESIAN_POINT ( 'NONE',  ( -1.640419947506561060, -0.004921259842519576551, 0.3153832671262227771 ) ) ;
#38018=CARTESIAN_POINT ( 'NONE',  ( -0.8464566929133852113, -0.4536011799217368745, -0.2665933059059886201 ) ) ;
#38020=CARTESIAN_POINT ( 'NONE',  ( -0.4790026246719152336, -0.05778040916215560624, -0.4822834645669293319 ) ) ;
#38021=CARTESIAN_POINT ( 'NONE',  ( -0.1771653543307080136, 0.07958543189024071263, -0.2665933059059888421 ) ) ;
#38022=CARTESIAN_POINT ( 'NONE',  ( -1.489501312335957062, -0.2845877964562161244, -0.3641732283464567121 ) ) ;
#38023=CARTESIAN_POINT ( 'NONE',  ( 1.141732283464567566, 0.1771653543307087630, 0.000000000000000000 ) ) ;
#38025=CARTESIAN_POINT ( 'NONE',  ( 0.9776902887139113929, -0.6692913385826773087, -0.1292274648535924053 ) ) ;
#38026=CARTESIAN_POINT ( 'NONE',  ( 1.587926509186352142, 0.05413385826771666132, 0.4176697321401328100 ) ) ;
#38027=CARTESIAN_POINT ( 'NONE',  ( 0.1115485564304470323, 0.1771653543307087630, 0.09757992244046791164 ) ) ;
#38028=CARTESIAN_POINT ( 'NONE',  ( 0.5708661417322842269, 0.1660481256975885056, 0.3530559997133364547 ) ) ;
#38029=CARTESIAN_POINT ( 'NONE',  ( 0.4855643044619428750, -0.004921259842519576551, 0.3153832671262227771 ) ) ;
#38030=CARTESIAN_POINT ( 'NONE',  ( 1.607611548556431069, 0.2952755905511811885, 0.1292274648535926551 ) ) ;
#38031=CARTESIAN_POINT ( 'NONE',  ( -1.246719160104985846, -0.4281496062992127816, -0.4176697321401328100 ) ) ;
#38032=CARTESIAN_POINT ( 'NONE',  ( -0.3280839895013117347, -0.4281496062992124485, 0.4176697321401328655 ) ) ;
#38035=CARTESIAN_POINT ( 'NONE',  ( 0.2952755905511816326, -0.5400638737290844871, 0.3530559997133364547 ) ) ;
#38036=CARTESIAN_POINT ( 'NONE',  ( 1.286089238845145033, 0.1283753931104748280, 0.1820866141732283561 ) ) ;
#38037=CARTESIAN_POINT ( 'NONE',  ( -0.3871391076115476282, -0.05778040916215522460, 0.4822834645669289988 ) ) ;
#38038=CARTESIAN_POINT ( 'NONE',  ( 0.5446194225721792126, -0.05778040916215560624, -0.4822834645669293319 ) ) ;
#38044=CARTESIAN_POINT ( 'NONE',  ( -0.3477690288713905509, -0.5511811023622046335, 0.09757992244046803654 ) ) ;
#38045=CARTESIAN_POINT ( 'NONE',  ( -1.227034120734907585, 0.2952755905511811885, 0.1292274648535926551 ) ) ;
#38047=CARTESIAN_POINT ( 'NONE',  ( 0.7349081364829403995, 0.2306618581243848609, 0.2411417322834645549 ) ) ;
#38048=CARTESIAN_POINT ( 'NONE',  ( 1.227034120734908917, -0.6692913385826771977, 0.1292274648535927661 ) ) ;
#38049=CARTESIAN_POINT ( 'NONE',  ( 0.8858267716535438430, -0.5400638737290845981, -0.3530559997133363437 ) ) ;
#38050=CARTESIAN_POINT ( 'NONE',  ( -0.6179882174207321777, -1.177125479915915794E-15, 0.3627985898453519598 ) ) ;
#38053=CARTESIAN_POINT ( 'NONE',  ( 0.3937007874015754361, -0.1870078740157480879, -0.4822834645669291653 ) ) ;
#38054=CARTESIAN_POINT ( 'NONE',  ( 0.7545931758530188826, -0.6692913385826771977, 0.1292274648535927661 ) ) ;
#38055=CARTESIAN_POINT ( 'NONE',  ( 0.6824146981627303710, 0.1283753931104746893, -0.1820866141732285504 ) ) ;
#38056=CARTESIAN_POINT ( 'NONE',  ( 1.207349081364829990, 0.2306618581243848609, 0.2411417322834645549 ) ) ;
#38058=CARTESIAN_POINT ( 'NONE',  ( 0.4658792650918640033, -0.3162353388693405765, 0.4822834645669290543 ) ) ;
#38059=CARTESIAN_POINT ( 'NONE',  ( 0.9973753280839902091, -0.6046776061558807314, 0.2411417322834647770 ) ) ;
#38060=CARTESIAN_POINT ( 'NONE',  ( 0.2624671916010504757, 0.2306618581243848609, 0.2411417322834645549 ) ) ;
#38062=CARTESIAN_POINT ( 'NONE',  ( 1.502624671916010790, -0.08942795157527998196, 0.3641732283464567121 ) ) ;
#38063=CARTESIAN_POINT ( 'NONE',  ( -0.8333333333333323711, -0.6692913385826773087, -0.1292274648535924053 ) ) ;
#38064=CARTESIAN_POINT ( 'NONE',  ( -1.194225721784776262, 0.05413385826771626580, -0.4176697321401330321 ) ) ;
#38065=CARTESIAN_POINT ( 'NONE',  ( 1.167979002624672580, 0.05413385826771626580, -0.4176697321401330321 ) ) ;
#38072=CARTESIAN_POINT ( 'NONE',  ( 1.574803149606299746, -0.1870078740157480879, -0.4822834645669291653 ) ) ;
#38073=CARTESIAN_POINT ( 'NONE',  ( 1.443569553805774897, 0.1283753931104748280, 0.1820866141732283561 ) ) ;
#38075=CARTESIAN_POINT ( 'NONE',  ( 1.253280839895013710, -0.08942795157528024563, -0.3641732283464568787 ) ) ;
#38077=CARTESIAN_POINT ( 'NONE',  ( 2.795275590551181910, 1.900312960331935086, 0.000000000000000000 ) ) ;
#38078=CARTESIAN_POINT ( 'NONE',  ( 0.4606732211678789546, 1.763126522798926343, 0.5309055118110234117 ) ) ;
#38081=CARTESIAN_POINT ( 'NONE',  ( -0.7480314960629914633, -0.5511811023622047445, 6.969142054262312111E-17 ) ) ;
#38082=CARTESIAN_POINT ( 'NONE',  ( -1.476377952755905110, -0.4536011799217368745, -0.2665933059059886201 ) ) ;
#38083=CARTESIAN_POINT ( 'NONE',  ( -1.115485564304461219, 0.05413385826771626580, -0.4176697321401330321 ) ) ;
#38084=CARTESIAN_POINT ( 'NONE',  ( 0.05905511811023681640, 0.1660481256975883668, -0.3530559997133364547 ) ) ;
#38085=CARTESIAN_POINT ( 'NONE',  ( -1.640419947506561060, 0.05413385826771666132, 0.4176697321401328100 ) ) ;
#38091=CARTESIAN_POINT ( 'NONE',  ( -0.2887139107611542133, -0.5023911411419708095, -0.1820866141732282451 ) ) ;
#38093=CARTESIAN_POINT ( 'NONE',  ( -0.9842519685039360366, 0.2952755905511811885, 0.000000000000000000 ) ) ;
#38094=CARTESIAN_POINT ( 'NONE',  ( 0.9383202099737538715, -0.05778040916215560624, -0.4822834645669293319 ) ) ;
#38095=ORIENTED_EDGE ( 'NONE', *, *, #45233, .F. ) ;
#38098=CARTESIAN_POINT ( 'NONE',  ( 1.154855643044620184, -0.6046776061558807314, 0.2411417322834647770 ) ) ;
#38099=CARTESIAN_POINT ( 'NONE',  ( -1.299212598425196097, -0.6692913385826771977, 8.415575281601705876E-17 ) ) ;
#38101=CARTESIAN_POINT ( 'NONE',  ( -0.4921259842519677963, -0.4536011799217367080, 0.2665933059059888421 ) ) ;
#38103=CARTESIAN_POINT ( 'NONE',  ( -0.6299212598425188991, -0.1870078740157480601, -0.3641732283464567677 ) ) ;
#38104=CARTESIAN_POINT ( 'NONE',  ( -0.07874015748031421014, -0.1870078740157480601, -0.3641732283464567677 ) ) ;
#38105=CARTESIAN_POINT ( 'NONE',  ( 0.1574803149606306130, -0.1870078740157479769, 0.4822834645669291653 ) ) ;
#38106=CARTESIAN_POINT ( 'NONE',  ( -0.7414698162729651543, -0.5511811023622046335, 0.09757992244046803654 ) ) ;
#38108=CARTESIAN_POINT ( 'NONE',  ( 1.043307086614173818, -0.5400638737290845981, -0.3530559997133363437 ) ) ;
#38109=B_SPLINE_CURVE_WITH_KNOTS ( 'NONE', 3,
 ( #57054, #63382, #64631, #58301 ),
 .UNSPECIFIED., .F., .F.,
 ( 4, 4 ),
 ( 0.000000000000000000, 0.001421551995671108343 ),
 .UNSPECIFIED. ) ;
#38111=CARTESIAN_POINT ( 'NONE',  ( -1.397637795275589623, -0.5400638737290845981, -0.3530559997133363437 ) ) ;
#38113=CARTESIAN_POINT ( 'NONE',  ( -0.3018372703412066094, 0.05413385826771666132, 0.4176697321401328100 ) ) ;
#38114=CARTESIAN_POINT ( 'NONE',  ( -1.017060367454067249, -0.05778040916215522460, 0.4822834645669289988 ) ) ;
#38115=CARTESIAN_POINT ( 'NONE',  ( 1.266404199475066328, -0.2845877964562161244, -0.3641732283464567121 ) ) ;
#38116=CARTESIAN_POINT ( 'NONE',  ( -0.1312335958005241554, 0.1283753931104748280, 0.1820866141732283561 ) ) ;
#38117=CARTESIAN_POINT ( 'NONE',  ( -0.8136482939632537770, -0.6046776061558807314, 0.2411417322834647770 ) ) ;
#38118=CARTESIAN_POINT ( 'NONE',  ( -0.9776902887139098386, 0.2952755905511810774, -0.1292274648535930714 ) ) ;
#38120=CARTESIAN_POINT ( 'NONE',  ( 1.345144356955381593, -0.08942795157527998196, 0.3641732283464567121 ) ) ;
#38122=CARTESIAN_POINT ( 'NONE',  ( -0.3805774278215216522, 0.05413385826771666132, 0.4176697321401328100 ) ) ;
#38123=CARTESIAN_POINT ( 'NONE',  ( -1.220472440944881054, 0.2952755905511811885, 0.000000000000000000 ) ) ;
#38124=ORIENTED_EDGE ( 'NONE', *, *, #51676, .F. ) ;
#38126=CARTESIAN_POINT ( 'NONE',  ( -0.8989501312335946848, -0.5511811023622046335, 0.09757992244046803654 ) ) ;
#38127=CARTESIAN_POINT ( 'NONE',  ( 0.9908136482939640111, 0.2952755905511810774, -0.1292274648535930714 ) ) ;
#38128=CARTESIAN_POINT ( 'NONE',  ( -1.010498687664041384, -0.3690944881889765550, -0.3153832671262227771 ) ) ;
#38130=CARTESIAN_POINT ( 'NONE',  ( -0.9448818897637790704, -0.1870078740157479769, 0.4822834645669291653 ) ) ;
#38131=CARTESIAN_POINT ( 'NONE',  ( 1.003937007874016407, -0.5400638737290844871, 0.3530559997133364547 ) ) ;
#38132=CARTESIAN_POINT ( 'NONE',  ( 0.9514435695538062676, -0.3162353388693409650, -0.4822834645669289433 ) ) ;
#38133=CARTESIAN_POINT ( 'NONE',  ( 1.522309711286089939, -0.6046776061558809534, -0.2411417322834644161 ) ) ;
#38134=CARTESIAN_POINT ( 'NONE',  ( -1.509186351706035767, -0.004921259842519870586, -0.3153832671262229437 ) ) ;
#38137=CIRCLE ( 'NONE', #27394, 1.220472440944883719 ) ;
#38140=CARTESIAN_POINT ( 'NONE',  ( 1.141732283464567788, -0.5511811023622047445, 6.969142054262312111E-17 ) ) ;
#38142=CARTESIAN_POINT ( 'NONE',  ( 0.7020997375328090762, -0.08942795157528024563, -0.3641732283464568787 ) ) ;
#38143=CARTESIAN_POINT ( 'NONE',  ( 0.01312335958005323398, 0.05413385826771666132, 0.4176697321401328100 ) ) ;
#38146=CARTESIAN_POINT ( 'NONE',  ( 0.9973753280839902091, -0.5023911411419708095, 0.1820866141732285504 ) ) ;
#38147=CARTESIAN_POINT ( 'NONE',  ( -0.4658792650918627265, -0.3162353388693409650, -0.4822834645669289433 ) ) ;
#38148=CARTESIAN_POINT ( 'NONE',  ( -1.371391076115484609, -0.6692913385826771977, 0.1292274648535927661 ) ) ;
#38149=CARTESIAN_POINT ( 'NONE',  ( 0.7742782152230979209, 0.05413385826771626580, -0.4176697321401330321 ) ) ;
#38151=CARTESIAN_POINT ( 'NONE',  ( -0.7202472836732357608, 0.02791078216816347476, -0.4328096321851898631 ) ) ;
#38153=EDGE_LOOP ( 'NONE', ( #28357, #42302, #25456, #31436 ) ) ;
#38154=CARTESIAN_POINT ( 'NONE',  ( -1.181102362204723644, -0.1870078740157480879, -0.4822834645669291653 ) ) ;
#38155=CARTESIAN_POINT ( 'NONE',  ( -0.7874015748031489847, -0.1870078740157480879, -0.4822834645669291653 ) ) ;
#38156=CARTESIAN_POINT ( 'NONE',  ( -0.8398950131233585692, 0.1283753931104748280, 0.1820866141732283561 ) ) ;
#38157=CARTESIAN_POINT ( 'NONE',  ( -0.7611548556430438595, -0.6046776061558809534, -0.2411417322834644161 ) ) ;
#38159=CARTESIAN_POINT ( 'NONE',  ( -0.2296587926509179312, -0.05778040916215522460, 0.4822834645669289988 ) ) ;
#38160=CARTESIAN_POINT ( 'NONE',  ( 1.443569553805774897, 0.2306618581243848609, 0.2411417322834645549 ) ) ;
#38161=CARTESIAN_POINT ( 'NONE',  ( -0.8267716535433065062, -0.6692913385826771977, 8.415575281601705876E-17 ) ) ;
#38162=CARTESIAN_POINT ( 'NONE',  ( 0.2559055118110243332, -0.5400638737290845981, -0.3530559997133363437 ) ) ;
#38165=CARTESIAN_POINT ( 'NONE',  ( -0.7283464566929126471, -0.4536011799217367080, 0.2665933059059888421 ) ) ;
#38169=CARTESIAN_POINT ( 'NONE',  ( -1.725721784776902190, -0.08942795157527998196, 0.3641732283464567121 ) ) ;
#38170=CARTESIAN_POINT ( 'NONE',  ( -1.030183727034119867, -0.3162353388693405765, 0.4822834645669290543 ) ) ;
#38171=CARTESIAN_POINT ( 'NONE',  ( -0.8333333333333323711, 0.2952755905511811885, 0.1292274648535926551 ) ) ;
#38173=CARTESIAN_POINT ( 'NONE',  ( -1.167979002624671470, -0.4281496062992127816, -0.4176697321401328100 ) ) ;
#38174=CARTESIAN_POINT ( 'NONE',  ( -1.338582677165353729, -0.1870078740157480879, -0.4822834645669291653 ) ) ;
#38175=CARTESIAN_POINT ( 'NONE',  ( -1.555118110236219930, -0.5400638737290845981, -0.3530559997133363437 ) ) ;
#38176=CARTESIAN_POINT ( 'NONE',  ( 0.6199123404867349363, 8.471767977567108961E-16, -0.4445507791589058955 ) ) ;
#38177=CARTESIAN_POINT ( 'NONE',  ( 0.6167979002624679463, -0.004921259842519870586, -0.3153832671262229437 ) ) ;
#38180=CARTESIAN_POINT ( 'NONE',  ( -0.5643044619422565855, -0.004921259842519870586, -0.3153832671262229437 ) ) ;
#38181=CARTESIAN_POINT ( 'NONE',  ( -0.8530183727034112984, 0.05413385826771666132, 0.4176697321401328100 ) ) ;
#38182=CARTESIAN_POINT ( 'NONE',  ( 1.384514435695538337, -0.6692913385826771977, 0.1292274648535927661 ) ) ;
#38183=CARTESIAN_POINT ( 'NONE',  ( -0.5052493438320203589, 0.2952755905511810774, -0.1292274648535930714 ) ) ;
#38184=VERTEX_POINT ( 'NONE', #15094 ) ;
#38187=CARTESIAN_POINT ( 'NONE',  ( -0.4658792650918627265, -0.3162353388693409650, -0.4822834645669289433 ) ) ;
#38188=CARTESIAN_POINT ( 'NONE',  ( 1.430446194225722500, 0.05413385826771666132, 0.4176697321401328100 ) ) ;
#38189=CARTESIAN_POINT ( 'NONE',  ( -1.253280839895012377, -0.08942795157527998196, 0.3641732283464567121 ) ) ;
#38190=CARTESIAN_POINT ( 'NONE',  ( -1.286089238845143479, -0.6046776061558807314, 0.2411417322834647770 ) ) ;
#38195=CARTESIAN_POINT ( 'NONE',  ( 0.2362204724409456558, -0.1870078740157479769, 0.4822834645669291653 ) ) ;
#38196=CARTESIAN_POINT ( 'NONE',  ( -0.8989501312335946848, -0.5511811023622046335, 0.09757992244046803654 ) ) ;
#38197=CARTESIAN_POINT ( 'NONE',  ( -0.4133858267716528645, 0.1660481256975883668, -0.3530559997133364547 ) ) ;
#38199=CARTESIAN_POINT ( 'NONE',  ( -0.6955380577427815458, -0.4281496062992127816, -0.4176697321401328100 ) ) ;
#38200=CARTESIAN_POINT ( 'NONE',  ( -0.8858267716535425107, 0.1660481256975883668, -0.3530559997133364547 ) ) ;
#38203=CARTESIAN_POINT ( 'NONE',  ( 1.017060367454068581, -0.08942795157528024563, -0.3641732283464568787 ) ) ;
#38204=CARTESIAN_POINT ( 'NONE',  ( -0.9120734908136475250, 0.1771653543307087630, 0.09757992244046791164 ) ) ;
#38205=CARTESIAN_POINT ( 'NONE',  ( 0.8464566929133866546, -0.4536011799217367080, 0.2665933059059888421 ) ) ;
#38206=CARTESIAN_POINT ( 'NONE',  ( -1.679790026246718693, 0.2306618581243847221, -0.2411417322834647770 ) ) ;
#38207=CARTESIAN_POINT ( 'NONE',  ( 1.502624671916010790, -0.3162353388693409650, -0.4822834645669289433 ) ) ;
#38208=CARTESIAN_POINT ( 'NONE',  ( 0.6889763779527566800, -0.4536011799217367080, 0.2665933059059888421 ) ) ;
#38210=CARTESIAN_POINT ( 'NONE',  ( -0.8398950131233585692, 0.2306618581243848609, 0.2411417322834645549 ) ) ;
#38211=CARTESIAN_POINT ( 'NONE',  ( 1.148293963254593653, 0.2952755905511810774, -0.1292274648535930714 ) ) ;
#38213=CARTESIAN_POINT ( 'NONE',  ( -0.2362204724409440182, -0.1870078740157479769, 0.3641732283464567677 ) ) ;
#38214=CARTESIAN_POINT ( 'NONE',  ( 0.6399301791983058596, -1.374501131054255944E-15, 0.4445507791589066726 ) ) ;
#38215=CARTESIAN_POINT ( 'NONE',  ( 0.3346456692913393205, -0.5400638737290845981, -0.3530559997133363437 ) ) ;
#38216=CARTESIAN_POINT ( 'NONE',  ( 0.6692913385826777528, 0.2952755905511811885, 0.000000000000000000 ) ) ;
#38217=CARTESIAN_POINT ( 'NONE',  ( 0.8923884514435701520, -0.5023911411419708095, -0.1820866141732282451 ) ) ;
#38218=CARTESIAN_POINT ( 'NONE',  ( 0.1771653543307093182, 0.07958543189024085140, 0.2665933059059887866 ) ) ;
#38219=CARTESIAN_POINT ( 'NONE',  ( 0.1246719160104994284, 0.2952755905511810774, -0.1292274648535930714 ) ) ;
#38220=CARTESIAN_POINT ( 'NONE',  ( -1.561679790026246017, 0.05413385826771666132, 0.4176697321401328100 ) ) ;
#38221=CARTESIAN_POINT ( 'NONE',  ( -0.5905511811023613777, -0.5511811023622047445, 6.969142054262312111E-17 ) ) ;
#38222=PLANE ( 'NONE',  #7190 ) ;
#38223=CARTESIAN_POINT ( 'NONE',  ( -0.3477690288713902178, 0.2952755905511810774, -0.1292274648535930714 ) ) ;
#38226=CARTESIAN_POINT ( 'NONE',  ( 0.07874015748031558404, -0.1870078740157480601, -0.3641732283464567677 ) ) ;
#38227=CARTESIAN_POINT ( 'NONE',  ( -0.4593175853018364174, -0.4281496062992127816, -0.4176697321401328100 ) ) ;
#38228=CARTESIAN_POINT ( 'NONE',  ( -1.122047244094487306, 0.1660481256975883668, -0.3530559997133364547 ) ) ;
#38229=CARTESIAN_POINT ( 'NONE',  ( -0.7283464566929126471, -0.4536011799217367080, 0.2665933059059888421 ) ) ;
#38231=CARTESIAN_POINT ( 'NONE',  ( -0.1312335958005241554, -0.6046776061558809534, -0.2411417322834644161 ) ) ;
#38232=CARTESIAN_POINT ( 'NONE',  ( -1.601049868766403650, -0.5023911411419708095, 0.1820866141732285504 ) ) ;
#38233=CARTESIAN_POINT ( 'NONE',  ( 1.200787401574803681, -0.5400638737290845981, -0.3530559997133363437 ) ) ;
#38237=VECTOR ( 'NONE', #48252, 39.37007874015748143 ) ;
#38240=CARTESIAN_POINT ( 'NONE',  ( -1.200787401574802349, 0.1660481256975883668, -0.3530559997133364547 ) ) ;
#38241=CARTESIAN_POINT ( 'NONE',  ( -0.8661417322834640276, -0.1870078740157480879, -0.4822834645669291653 ) ) ;
#38242=CARTESIAN_POINT ( 'NONE',  ( -1.555118110236219930, -0.5400638737290845981, -0.3530559997133363437 ) ) ;
#38245=CARTESIAN_POINT ( 'NONE',  ( 0.9251968503937015864, 0.1660481256975883668, -0.3530559997133364547 ) ) ;
#38246=CARTESIAN_POINT ( 'NONE',  ( 0.1377952755905518800, 0.1660481256975883668, -0.3530559997133364547 ) ) ;
#38249=CARTESIAN_POINT ( 'NONE',  ( 1.286089238845145033, 0.1283753931104748280, 0.1820866141732283561 ) ) ;
#38255=CARTESIAN_POINT ( 'NONE',  ( 0.1640419947506569498, -0.05778040916215522460, 0.4822834645669289988 ) ) ;
#38256=CARTESIAN_POINT ( 'NONE',  ( -0.8989501312335946848, 0.2952755905511810774, -0.1292274648535930714 ) ) ;
#38257=CARTESIAN_POINT ( 'NONE',  ( -1.594488188976377119, 0.1660481256975883668, -0.3530559997133364547 ) ) ;
#38258=CARTESIAN_POINT ( 'NONE',  ( 0.4396325459317593221, 0.2952755905511810774, -0.1292274648535930714 ) ) ;
#38259=CARTESIAN_POINT ( 'NONE',  ( 1.450131233595801428, -0.6692913385826773087, -0.1292274648535924053 ) ) ;
#38260=CARTESIAN_POINT ( 'NONE',  ( -0.1574803149606292529, -0.1870078740157480879, -0.4822834645669291653 ) ) ;
#38261=CARTESIAN_POINT ( 'NONE',  ( -1.167979002624671470, 0.05413385826771666132, 0.4176697321401328100 ) ) ;
#38262=CARTESIAN_POINT ( 'NONE',  ( 1.128608923884514947, 0.2306618581243848609, 0.2411417322834645549 ) ) ;
#38263=B_SPLINE_CURVE_WITH_KNOTS ( 'NONE', 3,
 ( #44241, #77510, #38775, #918, #19845, #64452, #13533 ),
 .UNSPECIFIED., .F., .F.,
 ( 4, 3, 4 ),
 ( 1.734723475976807094E-18, 0.001246232571205225159, 0.002492492258783242029 ),
 .UNSPECIFIED. ) ;
#38264=CARTESIAN_POINT ( 'NONE',  ( 1.561679790026247350, 0.05413385826771626580, -0.4176697321401330321 ) ) ;
#38265=CARTESIAN_POINT ( 'NONE',  ( -0.08530183727034056085, -0.05778040916215560624, -0.4822834645669293319 ) ) ;
#38267=CARTESIAN_POINT ( 'NONE',  ( 0.4068241469816281097, -0.004921259842519576551, 0.3153832671262227771 ) ) ;
#38268=VERTEX_POINT ( 'NONE', #32252 ) ;
#38270=ORIENTED_EDGE ( 'NONE', *, *, #69485, .T. ) ;
#38271=CARTESIAN_POINT ( 'NONE',  ( -0.03280839895013062252, -0.5511811023622046335, 0.09757992244046803654 ) ) ;
#38273=CARTESIAN_POINT ( 'NONE',  ( -0.03280839895013062252, -0.6692913385826771977, 0.1292274648535927661 ) ) ;
#38274=CARTESIAN_POINT ( 'NONE',  ( -0.1377952755905504645, 0.1660481256975885056, 0.3530559997133364547 ) ) ;
#38276=CARTESIAN_POINT ( 'NONE',  ( -0.7677165354330699465, 0.1660481256975885056, 0.3530559997133364547 ) ) ;
#38278=CARTESIAN_POINT ( 'NONE',  ( -1.030183727034119867, -0.3162353388693405765, 0.4822834645669290543 ) ) ;
#38281=CARTESIAN_POINT ( 'NONE',  ( 0.7283464566929140904, -0.4536011799217368745, -0.2665933059059886201 ) ) ;
#38282=CARTESIAN_POINT ( 'NONE',  ( 0.9580052493438327987, -0.4281496062992127816, -0.4176697321401328100 ) ) ;
#38283=CARTESIAN_POINT ( 'NONE',  ( 0.6889763779527566800, -0.5400638737290844871, 0.3530559997133364547 ) ) ;
#38285=CARTESIAN_POINT ( 'NONE',  ( -1.384514435695537005, 0.2952755905511811885, 0.1292274648535926551 ) ) ;
#38288=CARTESIAN_POINT ( 'NONE',  ( -0.2952755905511804668, 0.1660481256975885056, 0.3530559997133364547 ) ) ;
#38291=CARTESIAN_POINT ( 'NONE',  ( 1.259842519685040019, -0.1870078740157479769, 0.4822834645669291653 ) ) ;
#38292=CARTESIAN_POINT ( 'NONE',  ( 1.253280839895013710, -0.05778040916215560624, -0.4822834645669293319 ) ) ;
#38293=CARTESIAN_POINT ( 'NONE',  ( 0.2690288713910767848, 0.1771653543307087630, 0.09757992244046791164 ) ) ;
#38294=CARTESIAN_POINT ( 'NONE',  ( 0.9776902887139113929, 0.2952755905511811885, 0.1292274648535926551 ) ) ;
#38296=CARTESIAN_POINT ( 'NONE',  ( 0.1574803149606306130, -0.1870078740157480601, -0.3641732283464567677 ) ) ;
#38298=CARTESIAN_POINT ( 'NONE',  ( 0.4396325459317590445, -0.6692913385826771977, 0.1292274648535927661 ) ) ;
#38300=CARTESIAN_POINT ( 'NONE',  ( -1.154855643044618851, -0.6046776061558809534, -0.2411417322834644161 ) ) ;
#38302=CARTESIAN_POINT ( 'NONE',  ( 1.069553805774278610, -0.5511811023622046335, 0.09757992244046803654 ) ) ;
#38303=EDGE_CURVE ( 'NONE', #73526, #44157, #33921, .T. ) ;
#38304=CARTESIAN_POINT ( 'NONE',  ( 0.3543307086614179147, 0.2066929133858268208, 0.000000000000000000 ) ) ;
#38305=CARTESIAN_POINT ( 'NONE',  ( -0.4461942257217840213, 0.2306618581243848609, 0.2411417322834645549 ) ) ;
#38306=CARTESIAN_POINT ( 'NONE',  ( -0.3805774278215216522, -0.004921259842519576551, 0.3153832671262227771 ) ) ;
#38307=CARTESIAN_POINT ( 'NONE',  ( 0.4606732211678742361, 1.778019097314512686, 0.5309055118110234117 ) ) ;
#38308=CARTESIAN_POINT ( 'NONE',  ( -0.4133858267716528645, 0.1660481256975883668, -0.3530559997133364547 ) ) ;
#38309=CARTESIAN_POINT ( 'NONE',  ( 0.4790026246719167324, -0.08942795157527998196, 0.3641732283464567121 ) ) ;
#38311=CARTESIAN_POINT ( 'NONE',  ( -0.1181102362204717315, -0.6692913385826771977, 8.415575281601705876E-17 ) ) ;
#38313=CARTESIAN_POINT ( 'NONE',  ( 1.240157480314961314, 0.07958543189024071263, -0.2665933059059888421 ) ) ;
#38314=CARTESIAN_POINT ( 'NONE',  ( 0.3812812444996376282, 2.409604939980833412E-17, -0.3464511005275205946 ) ) ;
#38315=CARTESIAN_POINT ( 'NONE',  ( -0.6955380577427815458, -0.3690944881889765550, -0.3153832671262227771 ) ) ;
#38317=CARTESIAN_POINT ( 'NONE',  ( -0.7611548556430438595, 0.1283753931104748280, 0.1820866141732283561 ) ) ;
#38318=CARTESIAN_POINT ( 'NONE',  ( -0.3280839895013117347, 0.05413385826771626580, -0.4176697321401330321 ) ) ;
#38319=CARTESIAN_POINT ( 'NONE',  ( 0.07217847769028949700, -0.05778040916215560624, -0.4822834645669293319 ) ) ;
#38320=CARTESIAN_POINT ( 'NONE',  ( 0.4002624671916016896, -0.08942795157527998196, 0.3641732283464567121 ) ) ;
#38322=CARTESIAN_POINT ( 'NONE',  ( 1.404199475065617264, -0.3690944881889763329, 0.3153832671262228327 ) ) ;
#38324=CARTESIAN_POINT ( 'NONE',  ( 0.5708661417322842269, 0.1660481256975885056, 0.3530559997133364547 ) ) ;
#38326=CARTESIAN_POINT ( 'NONE',  ( -0.1968503937007867743, -0.6692913385826771977, 8.415575281601705876E-17 ) ) ;
#38328=CARTESIAN_POINT ( 'NONE',  ( -1.318897637795274802, -0.5400638737290845981, -0.3530559997133363437 ) ) ;
#38329=CARTESIAN_POINT ( 'NONE',  ( 0.9251968503937015864, 0.1660481256975883668, -0.3530559997133364547 ) ) ;
#38330=CARTESIAN_POINT ( 'NONE',  ( 0.4921259842519691285, -0.5400638737290845981, -0.3530559997133363437 ) ) ;
#38331=CARTESIAN_POINT ( 'NONE',  ( 0.4199475065616805614, 0.1283753931104748280, 0.1820866141732283561 ) ) ;
#38332=CARTESIAN_POINT ( 'NONE',  ( 1.312335958005250269, -0.6046776061558807314, 0.2411417322834647770 ) ) ;
#38334=CARTESIAN_POINT ( 'NONE',  ( -0.2821522309711278487, 0.1771653543307087630, 0.09757992244046791164 ) ) ;
#38335=CARTESIAN_POINT ( 'NONE',  ( -0.5839895013123351797, -0.6692913385826771977, 0.1292274648535927661 ) ) ;
#38337=CARTESIAN_POINT ( 'NONE',  ( 0.3937007874015754361, -0.1870078740157480879, -0.4822834645669291653 ) ) ;
#38338=CARTESIAN_POINT ( 'NONE',  ( -0.9055118110236215490, -0.6692913385826771977, 8.415575281601705876E-17 ) ) ;
#38339=CARTESIAN_POINT ( 'NONE',  ( -0.8005249343832013809, -0.3690944881889763329, 0.3153832671262228327 ) ) ;
#38340=CARTESIAN_POINT ( 'NONE',  ( 0.3412073490813655186, 0.2306618581243848609, 0.2411417322834645549 ) ) ;
#38341=CARTESIAN_POINT ( 'NONE',  ( -1.115485564304461219, -0.4281496062992124485, 0.4176697321401328655 ) ) ;
#38342=CARTESIAN_POINT ( 'NONE',  ( -0.2230971128608915943, 0.05413385826771666132, 0.4176697321401328100 ) ) ;
#38343=EDGE_CURVE ( 'NONE', #16885, #36844, #20471, .T. ) ;
#38345=CARTESIAN_POINT ( 'NONE',  ( -1.586052503253848611, 0.7480314960629931287, 0.1653254495020559378 ) ) ;
#38346=CARTESIAN_POINT ( 'NONE',  ( 1.174540682414699111, -0.05778040916215560624, -0.4822834645669293319 ) ) ;
#38347=CARTESIAN_POINT ( 'NONE',  ( 1.128608923884515169, -0.6046776061558809534, -0.2411417322834644161 ) ) ;
#38349=CARTESIAN_POINT ( 'NONE',  ( 0.4768059346183028957, 1.738380701482457269, -0.5050996235782325705 ) ) ;
#38350=CARTESIAN_POINT ( 'NONE',  ( -1.108923884514435132, -0.3162353388693405765, 0.4822834645669290543 ) ) ;
#38354=CARTESIAN_POINT ( 'NONE',  ( -0.1902887139107604098, 0.1771653543307087075, -0.09757992244046823083 ) ) ;
#38356=CARTESIAN_POINT ( 'NONE',  ( 0.6824146981627303710, 0.2306618581243847221, -0.2411417322834647770 ) ) ;
#38358=CARTESIAN_POINT ( 'NONE',  ( -1.595398199321655719, 1.860919225514068298, -0.1559797534342489689 ) ) ;
#38359=CARTESIAN_POINT ( 'NONE',  ( -0.5643044619422565855, -0.3690944881889763329, 0.3153832671262228327 ) ) ;
#38361=CARTESIAN_POINT ( 'NONE',  ( 1.266404199475066328, -0.3162353388693409650, -0.4822834645669289433 ) ) ;
#38362=CARTESIAN_POINT ( 'NONE',  ( 0.7545931758530188826, -0.5511811023622046335, 0.09757992244046803654 ) ) ;
#38363=CARTESIAN_POINT ( 'NONE',  ( -0.07874015748031421014, -0.1870078740157479769, 0.4822834645669291653 ) ) ;
#38365=CARTESIAN_POINT ( 'NONE',  ( -1.010498687664041384, 0.05413385826771666132, 0.4176697321401328100 ) ) ;
#38366=CARTESIAN_POINT ( 'NONE',  ( -1.253280839895012377, -0.08942795157527998196, 0.3641732283464567121 ) ) ;
#38367=CARTESIAN_POINT ( 'NONE',  ( -0.5249343832020990641, -0.6046776061558809534, -0.2411417322834644161 ) ) ;
#38370=VERTEX_POINT ( 'NONE', #15412 ) ;
#38372=CARTESIAN_POINT ( 'NONE',  ( 0.4396325459317593221, 0.2952755905511810774, -0.1292274648535930714 ) ) ;
#38375=CARTESIAN_POINT ( 'NONE',  ( -0.7152230971128602510, -0.05778040916215560624, -0.4822834645669293319 ) ) ;
#38376=CARTESIAN_POINT ( 'NONE',  ( 1.410761154855643795, -0.3162353388693405765, 0.4822834645669290543 ) ) ;
#38377=CARTESIAN_POINT ( 'NONE',  ( 0.6889763779527563470, 0.1660481256975883668, -0.3530559997133364547 ) ) ;
#38378=CARTESIAN_POINT ( 'NONE',  ( 0.1968503937007881344, -0.6692913385826771977, 8.415575281601705876E-17 ) ) ;
#38380=CARTESIAN_POINT ( 'NONE',  ( -0.7349081364829390672, 0.2306618581243847221, -0.2411417322834647770 ) ) ;
#38381=CARTESIAN_POINT ( 'NONE',  ( -0.3346456692913377662, 0.1660481256975883668, -0.3530559997133364547 ) ) ;
#38382=CARTESIAN_POINT ( 'NONE',  ( 0.07874015748031558404, -0.1870078740157479769, 0.3641732283464567677 ) ) ;
#38384=CARTESIAN_POINT ( 'NONE',  ( 0.05249343832021075018, 0.2306618581243847221, -0.2411417322834647770 ) ) ;
#38386=CARTESIAN_POINT ( 'NONE',  ( 0.9514435695538062676, -0.05778040916215522460, 0.4822834645669289988 ) ) ;
#38389=ORIENTED_EDGE ( 'NONE', *, *, #29541, .F. ) ;
#38390=CARTESIAN_POINT ( 'NONE',  ( 0.3477690288713918276, -0.6692913385826773087, -0.1292274648535924053 ) ) ;
#38391=CARTESIAN_POINT ( 'NONE',  ( -0.4921259842519677963, -0.4536011799217367080, 0.2665933059059888421 ) ) ;
#38392=CARTESIAN_POINT ( 'NONE',  ( 1.574803149606299746, -0.1870078740157480601, -0.3641732283464567677 ) ) ;
#38396=CARTESIAN_POINT ( 'NONE',  ( 1.443569553805774897, -0.5023911411419708095, -0.1820866141732282451 ) ) ;
#38397=EDGE_CURVE ( 'NONE', #33221, #34136, #25301, .T. ) ;
#38398=CARTESIAN_POINT ( 'NONE',  ( -1.450131233595799651, 0.2952755905511810774, -0.1292274648535930714 ) ) ;
#38400=CARTESIAN_POINT ( 'NONE',  ( -0.1049868766404193215, 0.2306618581243847221, -0.2411417322834647770 ) ) ;
#38401=CARTESIAN_POINT ( 'NONE',  ( -1.384514435695537005, -0.6692913385826773087, -0.1292274648535924053 ) ) ;
#38402=CARTESIAN_POINT ( 'NONE',  ( -1.325459317585300889, -0.4281496062992127816, -0.4176697321401328100 ) ) ;
#38403=CARTESIAN_POINT ( 'NONE',  ( 0.4199475065616803948, -0.6046776061558809534, -0.2411417322834644161 ) ) ;
#38405=CARTESIAN_POINT ( 'NONE',  ( 1.502624671916010790, -0.05778040916215522460, 0.4822834645669289988 ) ) ;
#38406=CARTESIAN_POINT ( 'NONE',  ( 0.7808398950131240079, -0.3162353388693405765, 0.4822834645669290543 ) ) ;
#38407=CARTESIAN_POINT ( 'NONE',  ( 1.253280839895013710, -0.08942795157528024563, -0.3641732283464568787 ) ) ;
#38408=CARTESIAN_POINT ( 'NONE',  ( 0.6299212598425204535, -0.1870078740157480601, -0.3641732283464567677 ) ) ;
#38409=CARTESIAN_POINT ( 'NONE',  ( -1.443569553805773564, 0.2306618581243847221, -0.2411417322834647770 ) ) ;
#38411=CARTESIAN_POINT ( 'NONE',  ( 1.062992125984252745, 0.2952755905511811885, 0.000000000000000000 ) ) ;
#38414=CARTESIAN_POINT ( 'NONE',  ( 0.5577427821522316087, -0.05778040916215522460, 0.4822834645669289988 ) ) ;
#38417=CARTESIAN_POINT ( 'NONE',  ( 0.1509186351706045259, -0.05778040916215560624, -0.4822834645669293319 ) ) ;
#38418=CARTESIAN_POINT ( 'NONE',  ( 0.6233595800524939223, -0.2845877964562159024, 0.3641732283464567677 ) ) ;
#38419=CARTESIAN_POINT ( 'NONE',  ( 1.003937007874016407, -0.5400638737290844871, 0.3530559997133364547 ) ) ;
#38421=CARTESIAN_POINT ( 'NONE',  ( -0.5971128608923877978, 0.1771653543307087630, 0.09757992244046791164 ) ) ;
#38422=CARTESIAN_POINT ( 'NONE',  ( -0.5314960629921254842, -0.5400638737290845981, -0.3530559997133363437 ) ) ;
#38423=CARTESIAN_POINT ( 'NONE',  ( 1.646981627296588035, -0.3162353388693405765, 0.4822834645669290543 ) ) ;
#38424=CARTESIAN_POINT ( 'NONE',  ( -0.9448818897637790704, -0.1870078740157479769, 0.4822834645669291653 ) ) ;
#38425=CARTESIAN_POINT ( 'NONE',  ( 0.9973753280839902091, -0.6046776061558807314, 0.2411417322834647770 ) ) ;
#38427=CARTESIAN_POINT ( 'NONE',  ( -1.548556430446193399, -0.5023911411419708095, -0.1820866141732282451 ) ) ;
#38429=CARTESIAN_POINT ( 'NONE',  ( 1.036745406824147508, -0.4281496062992127816, -0.4176697321401328100 ) ) ;
#38431=CARTESIAN_POINT ( 'NONE',  ( -1.633858267716534529, -0.5400638737290845981, -0.3530559997133363437 ) ) ;
#38432=CARTESIAN_POINT ( 'NONE',  ( -1.574803149606298192, -0.1870078740157480601, -0.3641732283464567677 ) ) ;
#38433=CARTESIAN_POINT ( 'NONE',  ( -1.148293963254592542, -0.5511811023622048555, -0.09757992244046775898 ) ) ;
#38435=CARTESIAN_POINT ( 'NONE',  ( -0.4068241469816264999, -0.4281496062992124485, 0.4176697321401328655 ) ) ;
#38436=CARTESIAN_POINT ( 'NONE',  ( -0.4396325459317577122, -0.5511811023622048555, -0.09757992244046775898 ) ) ;
#38437=CARTESIAN_POINT ( 'NONE',  ( -1.404199475065615932, -0.004921259842519576551, 0.3153832671262227771 ) ) ;
#38438=CARTESIAN_POINT ( 'NONE',  ( 0.9908136482939640111, 0.1771653543307087075, -0.09757992244046823083 ) ) ;
#38439=CARTESIAN_POINT ( 'NONE',  ( 0.3871391076115493490, -0.3162353388693405765, 0.4822834645669290543 ) ) ;
#38441=CARTESIAN_POINT ( 'NONE',  ( -0.1509186351706028884, -0.2845877964562161244, -0.3641732283464567121 ) ) ;
#38442=CARTESIAN_POINT ( 'NONE',  ( 0.3543307086614181922, -0.6692913385826771977, 8.415575281601705876E-17 ) ) ;
#38443=CARTESIAN_POINT ( 'NONE',  ( 0.6955380577427828781, -0.004921259842519870586, -0.3153832671262229437 ) ) ;
#38444=CARTESIAN_POINT ( 'NONE',  ( -1.627296587926508442, 0.2306618581243848609, 0.2411417322834645549 ) ) ;
#38445=CARTESIAN_POINT ( 'NONE',  ( -1.115485564304461219, 0.05413385826771626580, -0.4176697321401330321 ) ) ;
#38446=CARTESIAN_POINT ( 'NONE',  ( -0.6102362204724400829, 0.1660481256975885056, 0.3530559997133364547 ) ) ;
#38449=CARTESIAN_POINT ( 'NONE',  ( 0.4527559055118117182, -0.5400638737290844871, 0.3530559997133364547 ) ) ;
#38450=CARTESIAN_POINT ( 'NONE',  ( 1.056430446194226436, -0.5511811023622048555, -0.09757992244046775898 ) ) ;
#38451=CARTESIAN_POINT ( 'NONE',  ( -0.3937007874015740483, -0.1870078740157479769, 0.4822834645669291653 ) ) ;
#38452=CARTESIAN_POINT ( 'NONE',  ( 0.3477690288713918276, 0.2952755905511811885, 0.1292274648535926551 ) ) ;
#38458=CARTESIAN_POINT ( 'NONE',  ( -1.148293963254592542, -0.5511811023622048555, -0.09757992244046775898 ) ) ;
#38459=CARTESIAN_POINT ( 'NONE',  ( -1.082677165354329896, 0.1660481256975885056, 0.3530559997133364547 ) ) ;
#38461=CARTESIAN_POINT ( 'NONE',  ( 0.9973753280839902091, -0.6046776061558807314, 0.2411417322834647770 ) ) ;
#38462=CARTESIAN_POINT ( 'NONE',  ( 1.489501312335958172, -0.05778040916215560624, -0.4822834645669293319 ) ) ;
#38463=CARTESIAN_POINT ( 'NONE',  ( 0.5839895013123367340, -0.6692913385826773087, -0.1292274648535924053 ) ) ;
#38464=CARTESIAN_POINT ( 'NONE',  ( -0.6188235755478027622, -3.724876541855331158E-15, 0.3954974714151467396 ) ) ;
#38468=CARTESIAN_POINT ( 'NONE',  ( -0.7461015470515853787, 2.202998601811383850, 0.5309055118110236338 ) ) ;
#38471=CARTESIAN_POINT ( 'NONE',  ( 0.3543307086614179147, 0.2952755905511811885, 0.000000000000000000 ) ) ;
#38472=CARTESIAN_POINT ( 'NONE',  ( 0.08530183727034192087, -0.3162353388693409650, -0.4822834645669289433 ) ) ;
#38473=CARTESIAN_POINT ( 'NONE',  ( 0.7874015748031503170, -0.1870078740157479769, 0.3641732283464567677 ) ) ;
#38474=CARTESIAN_POINT ( 'NONE',  ( 1.200787401574803681, 0.1660481256975885056, 0.3530559997133364547 ) ) ;
#38476=CARTESIAN_POINT ( 'NONE',  ( 0.6561679790026253567, 0.2306618581243848609, 0.2411417322834645549 ) ) ;
#38477=CARTESIAN_POINT ( 'NONE',  ( 1.233595800524935227, 0.2306618581243847221, -0.2411417322834647770 ) ) ;
#38478=CARTESIAN_POINT ( 'NONE',  ( 0.5183727034120741983, -0.6692913385826771977, 0.1292274648535927661 ) ) ;
#38479=CARTESIAN_POINT ( 'NONE',  ( 1.332020997375329197, -0.2845877964562159024, 0.3641732283464567677 ) ) ;
#38480=CARTESIAN_POINT ( 'NONE',  ( -0.9842519685039365918, -0.6692913385826771977, 8.415575281601705876E-17 ) ) ;
#38481=CARTESIAN_POINT ( 'NONE',  ( -0.8858267716535425107, 0.1660481256975883668, -0.3530559997133364547 ) ) ;
#38482=CARTESIAN_POINT ( 'NONE',  ( 1.233595800524935227, -0.6046776061558807314, 0.2411417322834647770 ) ) ;
#38486=VERTEX_POINT ( 'NONE', #1533 ) ;
#38489=CARTESIAN_POINT ( 'NONE',  ( 1.456692913385827515, -0.6692913385826771977, 8.415575281601705876E-17 ) ) ;
#38491=CARTESIAN_POINT ( 'NONE',  ( 1.010498687664042716, -0.004921259842519870586, -0.3153832671262229437 ) ) ;
#38493=CARTESIAN_POINT ( 'NONE',  ( 1.266404199475066328, -0.2845877964562161244, -0.3641732283464567121 ) ) ;
#38495=CARTESIAN_POINT ( 'NONE',  ( -0.1115485564304456445, 0.2952755905511810219, -0.1292274648535930437 ) ) ;
#38499=CARTESIAN_POINT ( 'NONE',  ( -0.7020997375328074108, -0.08942795157527998196, 0.3641732283464567121 ) ) ;
#38500=CARTESIAN_POINT ( 'NONE',  ( -1.555118110236219930, 0.07958543189024085140, 0.2665933059059887866 ) ) ;
#38501=CARTESIAN_POINT ( 'NONE',  ( -1.220472440944881054, -0.6692913385826771977, 8.415575281601705876E-17 ) ) ;
#38502=CARTESIAN_POINT ( 'NONE',  ( 0.1443569553805781891, -0.4281496062992124485, 0.4176697321401328655 ) ) ;
#38503=CARTESIAN_POINT ( 'NONE',  ( 1.581364829396326277, -0.05778040916215522460, 0.4822834645669289988 ) ) ;
#38505=CARTESIAN_POINT ( 'NONE',  ( -1.609562092802257816, 0.2869345716361978438, 0.09226303723660828071 ) ) ;
#38509=CARTESIAN_POINT ( 'NONE',  ( -0.2952755905511803003, -0.4536011799217368745, -0.2665933059059886201 ) ) ;
#38510=CARTESIAN_POINT ( 'NONE',  ( -1.187664041994749731, -0.3162353388693405765, 0.4822834645669290543 ) ) ;
#38511=CARTESIAN_POINT ( 'NONE',  ( 0.8858267716535438430, 0.1660481256975885056, 0.3530559997133364547 ) ) ;
#38513=CARTESIAN_POINT ( 'NONE',  ( -1.603475055217291612, 0.5037964761735302943, -0.04573490813648262154 ) ) ;
#38514=CARTESIAN_POINT ( 'NONE',  ( -1.646051170424378096, -0.1870078740157480046, 1.254653134982923898E-17 ) ) ;
#38515=CARTESIAN_POINT ( 'NONE',  ( 1.023622047244095334, -0.1870078740157479769, 0.4822834645669291653 ) ) ;
#38516=CARTESIAN_POINT ( 'NONE',  ( -1.233595800524933894, 0.2306618581243848609, 0.2411417322834645549 ) ) ;
#38518=CARTESIAN_POINT ( 'NONE',  ( -0.4265091863517051496, 0.1771653543307087075, -0.09757992244046823083 ) ) ;
#38520=CARTESIAN_POINT ( 'NONE',  ( -0.4330708661417315697, -0.5511811023622047445, 6.969142054262312111E-17 ) ) ;
#38521=CARTESIAN_POINT ( 'NONE',  ( 0.1706036745406830368, -0.004921259842519576551, 0.3153832671262227771 ) ) ;
#38522=CARTESIAN_POINT ( 'NONE',  ( 0.1312335958005255154, -0.6046776061558807314, 0.2411417322834647770 ) ) ;
#38523=CARTESIAN_POINT ( 'NONE',  ( -0.9711286089238838626, 0.1283753931104746893, -0.1820866141732285504 ) ) ;
#38525=CARTESIAN_POINT ( 'NONE',  ( 1.272965879265092637, 0.05413385826771666132, 0.4176697321401328100 ) ) ;
#38526=AXIS2_PLACEMENT_3D ( 'NONE', #30032, #42245, #22487 ) ;
#38527=CARTESIAN_POINT ( 'NONE',  ( -1.410761154855641575, -0.3162353388693409650, -0.4822834645669289433 ) ) ;
#38528=AXIS2_PLACEMENT_3D ( 'NONE', #52236, #2582, #53491 ) ;
#38530=CARTESIAN_POINT ( 'NONE',  ( -0.5118110236220466680, -0.6692913385826771977, 8.415575281601705876E-17 ) ) ;
#38531=CARTESIAN_POINT ( 'NONE',  ( -0.9842519685039360366, 0.2952755905511811885, 0.000000000000000000 ) ) ;
#38532=CARTESIAN_POINT ( 'NONE',  ( 0.6364829396325465405, -0.2845877964562161244, -0.3641732283464567121 ) ) ;
#38533=CARTESIAN_POINT ( 'NONE',  ( -0.4921259842519677963, -0.4536011799217367080, 0.2665933059059888421 ) ) ;
#38534=CARTESIAN_POINT ( 'NONE',  ( -0.5511811023622041894, -0.1870078740157480879, -0.4822834645669291653 ) ) ;
#38535=CARTESIAN_POINT ( 'NONE',  ( -0.9908136482939626788, 0.2952755905511811885, 0.1292274648535926551 ) ) ;
#38537=CARTESIAN_POINT ( 'NONE',  ( 1.122047244094488860, -0.4536011799217368745, -0.2665933059059886201 ) ) ;
#38539=CARTESIAN_POINT ( 'NONE',  ( -0.1574803149606292529, -0.1870078740157480879, -0.4822834645669291653 ) ) ;
#38540=CARTESIAN_POINT ( 'NONE',  ( -1.391076115485563758, 0.2306618581243848609, 0.2411417322834645549 ) ) ;
#38543=CARTESIAN_POINT ( 'NONE',  ( -1.003937007874014853, 0.07958543189024085140, 0.2665933059059887866 ) ) ;
#38544=CARTESIAN_POINT ( 'NONE',  ( 0.8923884514435701520, -0.6046776061558809534, -0.2411417322834644161 ) ) ;
#38545=CARTESIAN_POINT ( 'NONE',  ( -0.9711286089238838626, -0.5023911411419708095, 0.1820866141732285504 ) ) ;
#38547=CARTESIAN_POINT ( 'NONE',  ( -0.8661417322834640276, -0.1870078740157480879, -0.4822834645669291653 ) ) ;
#38548=CARTESIAN_POINT ( 'NONE',  ( 0.7283464566929143125, 0.1660481256975885056, 0.3530559997133364547 ) ) ;
#38549=CARTESIAN_POINT ( 'NONE',  ( 0.6758530183727039509, -0.6692913385826771977, 0.1292274648535927661 ) ) ;
#38550=CARTESIAN_POINT ( 'NONE',  ( 1.568241469816273437, -0.3162353388693405765, 0.4822834645669290543 ) ) ;
#38551=CARTESIAN_POINT ( 'NONE',  ( -1.482939632545930975, -0.3690944881889765550, -0.3153832671262227771 ) ) ;
#38556=CARTESIAN_POINT ( 'NONE',  ( 1.062992125984252745, 0.1771653543307087630, 0.000000000000000000 ) ) ;
#38557=CARTESIAN_POINT ( 'NONE',  ( 0.4396325459317590445, -0.5511811023622046335, 0.09757992244046803654 ) ) ;
#38558=CARTESIAN_POINT ( 'NONE',  ( 0.09842519685039434474, -0.5400638737290845981, -0.3530559997133363437 ) ) ;
#38559=CARTESIAN_POINT ( 'NONE',  ( 1.325459317585302665, 0.05413385826771626580, -0.4176697321401330321 ) ) ;
#38561=CARTESIAN_POINT ( 'NONE',  ( 0.4396325459317593221, 0.1771653543307087075, -0.09757992244046823083 ) ) ;
#38562=CARTESIAN_POINT ( 'NONE',  ( -0.5905511811023613777, -0.6692913385826771977, 8.415575281601705876E-17 ) ) ;
#38563=CARTESIAN_POINT ( 'NONE',  ( -1.312335958005248715, 0.2306618581243848609, 0.2411417322834645549 ) ) ;
#38564=CARTESIAN_POINT ( 'NONE',  ( 0.8005249343832028242, -0.4281496062992127816, -0.4176697321401328100 ) ) ;
#38568=ORIENTED_EDGE ( 'NONE', *, *, #10106, .T. ) ;
#38569=CARTESIAN_POINT ( 'NONE',  ( -1.384514435695537005, 0.2952755905511811885, 0.1292274648535926551 ) ) ;
#38570=CARTESIAN_POINT ( 'NONE',  ( -0.6102362204724400829, -0.5400638737290845981, -0.3530559997133363437 ) ) ;
#38571=CARTESIAN_POINT ( 'NONE',  ( -0.5905511811023613777, -0.5511811023622047445, 6.969142054262312111E-17 ) ) ;
#38572=CARTESIAN_POINT ( 'NONE',  ( -0.7677165354330699465, -0.5400638737290845981, -0.3530559997133363437 ) ) ;
#38575=CARTESIAN_POINT ( 'NONE',  ( -1.587926509186350810, -0.004921259842519870586, -0.3153832671262229437 ) ) ;
#38576=CARTESIAN_POINT ( 'NONE',  ( -1.332020997375327642, -0.3162353388693409650, -0.4822834645669289433 ) ) ;
#38577=CARTESIAN_POINT ( 'NONE',  ( 0.2690288713910767848, -0.6692913385826773087, -0.1292274648535924053 ) ) ;
#38578=CARTESIAN_POINT ( 'NONE',  ( -0.9580052493438311334, 0.05413385826771626580, -0.4176697321401330321 ) ) ;
#38582=CARTESIAN_POINT ( 'NONE',  ( -0.9448818897637790704, -0.1870078740157480601, -0.3641732283464567677 ) ) ;
#38587=CARTESIAN_POINT ( 'NONE',  ( 0.9348729704079946634, -8.644661201599092366E-16, -0.4445507791589066171 ) ) ;
#38588=CARTESIAN_POINT ( 'NONE',  ( -1.115485564304461219, 0.05413385826771626580, -0.4176697321401330321 ) ) ;
#38589=CARTESIAN_POINT ( 'NONE',  ( -0.8858267716535425107, -0.5400638737290844871, 0.3530559997133364547 ) ) ;
#38591=CARTESIAN_POINT ( 'NONE',  ( -1.115485564304461219, -0.4281496062992124485, 0.4176697321401328655 ) ) ;
#38592=CARTESIAN_POINT ( 'NONE',  ( -1.253280839895012377, -0.05778040916215522460, 0.4822834645669289988 ) ) ;
#38594=CARTESIAN_POINT ( 'NONE',  ( 0.5643044619422579178, -0.004921259842519576551, 0.3153832671262227771 ) ) ;
#38595=CARTESIAN_POINT ( 'NONE',  ( -1.646051170424378096, -0.1870078740157480046, 1.254653134982923898E-17 ) ) ;
#38597=CARTESIAN_POINT ( 'NONE',  ( -0.3871391076115479057, -0.2845877964562161244, -0.3641732283464567121 ) ) ;
#38598=CARTESIAN_POINT ( 'NONE',  ( -0.9448818897637790704, -0.1870078740157480879, -0.4822834645669291653 ) ) ;
#38599=CARTESIAN_POINT ( 'NONE',  ( 1.443569553805774897, 0.2306618581243848609, 0.2411417322834645549 ) ) ;
#38600=CARTESIAN_POINT ( 'NONE',  ( -0.6102362204724400829, -0.5400638737290845981, -0.3530559997133363437 ) ) ;
#38602=ORIENTED_EDGE ( 'NONE', *, *, #72224, .T. ) ;
#38604=CARTESIAN_POINT ( 'NONE',  ( -1.049868766404198794, -0.6046776061558807314, 0.2411417322834647770 ) ) ;
#38605=CARTESIAN_POINT ( 'NONE',  ( 1.194225721784777594, -0.4281496062992127816, -0.4176697321401328100 ) ) ;
#38606=CARTESIAN_POINT ( 'NONE',  ( -0.9383202099737524282, -0.08942795157527998196, 0.3641732283464567121 ) ) ;
#38607=CARTESIAN_POINT ( 'NONE',  ( -1.574803149606298636, -0.1870078740157479769, 0.4822834645669291653 ) ) ;
#38612=CARTESIAN_POINT ( 'NONE',  ( 0.03937007874015833325, -0.6692913385826771977, 8.415575281601705876E-17 ) ) ;
#38613=CARTESIAN_POINT ( 'NONE',  ( -0.8727034120734901146, -0.2845877964562159024, 0.3641732283464567677 ) ) ;
#38614=CARTESIAN_POINT ( 'NONE',  ( -0.7611548556430438595, 0.2306618581243848609, 0.2411417322834645549 ) ) ;
#38616=CARTESIAN_POINT ( 'NONE',  ( -1.135170603674539924, -0.6692913385826771977, 0.1292274648535927661 ) ) ;
#38617=CARTESIAN_POINT ( 'NONE',  ( -0.9645669291338575535, -0.5400638737290844871, 0.3530559997133364547 ) ) ;
#38618=CARTESIAN_POINT ( 'NONE',  ( -0.04593175853018302557, -0.6692913385826773087, -0.1292274648535924053 ) ) ;
#38620=CARTESIAN_POINT ( 'NONE',  ( 0.9973753280839902091, 0.1283753931104746893, -0.1820866141732285504 ) ) ;
#38621=CARTESIAN_POINT ( 'NONE',  ( -0.5905511811023615998, 0.1771653543307087630, 0.000000000000000000 ) ) ;
#38623=CARTESIAN_POINT ( 'NONE',  ( 0.5905511811023629321, 0.1771653543307087630, 0.000000000000000000 ) ) ;
#38624=CARTESIAN_POINT ( 'NONE',  ( 1.154855643044620184, 0.1283753931104746893, -0.1820866141732285504 ) ) ;
#38625=CARTESIAN_POINT ( 'NONE',  ( 1.377952755905512472, -0.6692913385826771977, 8.415575281601705876E-17 ) ) ;
#38626=CARTESIAN_POINT ( 'NONE',  ( 0.4199475065616805614, 0.1283753931104748280, 0.1820866141732283561 ) ) ;
#38628=CARTESIAN_POINT ( 'NONE',  ( -0.9514435695538050464, -0.05778040916215560624, -0.4822834645669293319 ) ) ;
#38629=CARTESIAN_POINT ( 'NONE',  ( 1.259842519685040019, -0.1870078740157479769, 0.4822834645669291653 ) ) ;
#38631=CARTESIAN_POINT ( 'NONE',  ( -0.4986876640419939388, 0.1283753931104746893, -0.1820866141732285504 ) ) ;
#38632=CARTESIAN_POINT ( 'NONE',  ( -0.7137454485294950635, 2.362204724409448620, -0.4917280318828581298 ) ) ;
#38633=CARTESIAN_POINT ( 'NONE',  ( 0.3740157480314966754, -0.5400638737290844871, 0.3530559997133364547 ) ) ;
#38635=CARTESIAN_POINT ( 'NONE',  ( 1.023622047244095112, -0.1870078740157480601, -0.3641732283464567677 ) ) ;
#38636=CARTESIAN_POINT ( 'NONE',  ( 0.2296587926509192634, -0.08942795157528024563, -0.3641732283464568787 ) ) ;
#38637=CARTESIAN_POINT ( 'NONE',  ( 0.1049868766404206816, 0.2306618581243848609, 0.2411417322834645549 ) ) ;
#38638=CARTESIAN_POINT ( 'NONE',  ( -1.568241469816272105, -0.05778040916215522460, 0.4822834645669289988 ) ) ;
#38639=CARTESIAN_POINT ( 'NONE',  ( -0.7414698162729651543, -0.5511811023622046335, 0.09757992244046803654 ) ) ;
#38640=CYLINDRICAL_SURFACE ( 'NONE', #36747, 0.3937007874015748254 ) ;
#38641=CARTESIAN_POINT ( 'NONE',  ( -0.4133858267716528645, -0.5400638737290844871, 0.3530559997133364547 ) ) ;
#38644=CARTESIAN_POINT ( 'NONE',  ( 0.3412073490813655186, 0.1283753931104748280, 0.1820866141732283561 ) ) ;
#38645=CARTESIAN_POINT ( 'NONE',  ( -0.9580052493438311334, 0.05413385826771626580, -0.4176697321401330321 ) ) ;
#38647=CARTESIAN_POINT ( 'NONE',  ( -1.030183727034119867, -0.3162353388693405765, 0.4822834645669290543 ) ) ;
#38648=CARTESIAN_POINT ( 'NONE',  ( -1.325459317585300889, -0.004921259842519576551, 0.3153832671262227771 ) ) ;
#38649=DIRECTION ( 'NONE',  ( -1.000000000000000000, 0.000000000000000000, 0.000000000000000000 ) ) ;
#38650=CARTESIAN_POINT ( 'NONE',  ( -0.5052493438320203589, 0.2952755905511810774, -0.1292274648535930714 ) ) ;
#38651=CARTESIAN_POINT ( 'NONE',  ( -0.7742782152230962556, -0.3690944881889765550, -0.3153832671262227771 ) ) ;
#38652=CARTESIAN_POINT ( 'NONE',  ( -1.706036745406823485, 0.1283753931104748280, 0.1820866141732283561 ) ) ;
#38653=CARTESIAN_POINT ( 'NONE',  ( 1.469816272965879911, 0.2306618581243847221, -0.2411417322834647770 ) ) ;
#38656=VERTEX_POINT ( 'NONE', #14169 ) ;
#38657=CARTESIAN_POINT ( 'NONE',  ( 0.4061203303035133549, 3.421639014772782816E-16, 0.3464511005275203726 ) ) ;
#38658=CARTESIAN_POINT ( 'NONE',  ( -1.292650918635170010, -0.6692913385826771977, 0.1292274648535927661 ) ) ;
#38659=CARTESIAN_POINT ( 'NONE',  ( -0.8398950131233589023, -0.6046776061558809534, -0.2411417322834644161 ) ) ;
#38660=CARTESIAN_POINT ( 'NONE',  ( -1.548556430446193399, -0.6046776061558809534, -0.2411417322834644161 ) ) ;
#38662=CARTESIAN_POINT ( 'NONE',  ( 1.443569553805774897, -0.5023911411419708095, -0.1820866141732282451 ) ) ;
#38663=CARTESIAN_POINT ( 'NONE',  ( 0.6758530183727039509, -0.6692913385826771977, 0.1292274648535927661 ) ) ;
#38664=CARTESIAN_POINT ( 'NONE',  ( -0.07874015748031421014, -0.1870078740157479769, 0.4822834645669291653 ) ) ;
#38666=CARTESIAN_POINT ( 'NONE',  ( 1.614173228346456712, 2.401574803149606474, 0.1372047244094478646 ) ) ;
#38667=CARTESIAN_POINT ( 'NONE',  ( 0.7020997375328090762, -0.08942795157528024563, -0.3641732283464568787 ) ) ;
#38672=CARTESIAN_POINT ( 'NONE',  ( -0.1115485564304456306, 0.2952755905511810774, -0.1292274648535930714 ) ) ;
#38673=CARTESIAN_POINT ( 'NONE',  ( -0.8464566929133852113, -0.5400638737290845981, -0.3530559997133363437 ) ) ;
#38674=CARTESIAN_POINT ( 'NONE',  ( -1.620734908136482577, 0.2952755905511811885, 0.1292274648535926551 ) ) ;
#38675=CARTESIAN_POINT ( 'NONE',  ( 0.6496062992125991586, -0.5400638737290845981, -0.3530559997133363437 ) ) ;
#38676=CARTESIAN_POINT ( 'NONE',  ( -1.594488188976377119, 0.07958543189024071263, -0.2665933059059888421 ) ) ;
#38677=CARTESIAN_POINT ( 'NONE',  ( 1.332020997375328974, -0.05778040916215560624, -0.4822834645669293319 ) ) ;
#38678=CARTESIAN_POINT ( 'NONE',  ( -0.5052493438320203589, 0.2952755905511810774, -0.1292274648535930714 ) ) ;
#38679=CARTESIAN_POINT ( 'NONE',  ( 0.6299212598425204535, -0.1870078740157479769, 0.4822834645669291653 ) ) ;
#38680=CARTESIAN_POINT ( 'NONE',  ( 1.581364829396326277, -0.05778040916215522460, 0.4822834645669289988 ) ) ;
#38681=CARTESIAN_POINT ( 'NONE',  ( 1.115485564304462551, 0.05413385826771666132, 0.4176697321401328100 ) ) ;
#38683=CARTESIAN_POINT ( 'NONE',  ( -0.2034120734908131112, -0.6692913385826773087, -0.1292274648535924053 ) ) ;
#38685=CARTESIAN_POINT ( 'NONE',  ( 0.3215223097112867578, -0.2845877964562161244, -0.3641732283464567121 ) ) ;
#38689=CARTESIAN_POINT ( 'NONE',  ( -0.4986876640419942164, -0.5023911411419708095, 0.1820866141732285504 ) ) ;
#38691=CARTESIAN_POINT ( 'NONE',  ( 0.1771653543307093182, 0.1660481256975885056, 0.3530559997133364547 ) ) ;
#38692=CARTESIAN_POINT ( 'NONE',  ( 0.1377952755905518800, -0.5400638737290844871, 0.3530559997133364547 ) ) ;
#38693=CARTESIAN_POINT ( 'NONE',  ( -0.8070866141732276899, -0.5400638737290844871, 0.3530559997133364547 ) ) ;
#38695=CARTESIAN_POINT ( 'NONE',  ( -1.194225721784776262, -0.4281496062992124485, 0.4176697321401328655 ) ) ;
#38697=CARTESIAN_POINT ( 'NONE',  ( 0.7742782152230978099, -0.3690944881889763329, 0.3153832671262228327 ) ) ;
#38698=CARTESIAN_POINT ( 'NONE',  ( 0.3674540682414705883, -0.6046776061558807314, 0.2411417322834647770 ) ) ;
#38699=CARTESIAN_POINT ( 'NONE',  ( 0.7742782152230979209, 0.05413385826771626580, -0.4176697321401330321 ) ) ;
#38701=CARTESIAN_POINT ( 'NONE',  ( -1.725721784776902190, -0.05778040916215522460, 0.4822834645669289988 ) ) ;
#38704=CARTESIAN_POINT ( 'NONE',  ( -0.2230971128608915943, -0.4281496062992127816, -0.4176697321401328100 ) ) ;
#38707=CARTESIAN_POINT ( 'NONE',  ( -1.312335958005248715, 0.1283753931104748280, 0.1820866141732283561 ) ) ;
#38708=CARTESIAN_POINT ( 'NONE',  ( 1.161417322834646271, 0.1660481256975883668, -0.3530559997133364547 ) ) ;
#38710=CARTESIAN_POINT ( 'NONE',  ( 1.489501312335958172, -0.3162353388693405765, 0.4822834645669290543 ) ) ;
#38711=CARTESIAN_POINT ( 'NONE',  ( 0.3937007874015754361, -0.1870078740157479769, 0.3641732283464567677 ) ) ;
#38712=CARTESIAN_POINT ( 'NONE',  ( 0.4068241469816279987, -0.4281496062992127816, -0.4176697321401328100 ) ) ;
#38714=CARTESIAN_POINT ( 'NONE',  ( 0.3543307086614181922, -0.5511811023622047445, 6.969142054262312111E-17 ) ) ;
#38715=CARTESIAN_POINT ( 'NONE',  ( 0.4068241469816279987, -0.4281496062992127816, -0.4176697321401328100 ) ) ;
#38717=CARTESIAN_POINT ( 'NONE',  ( -1.023622047244094002, -0.1870078740157480879, -0.4822834645669291653 ) ) ;
#38718=CARTESIAN_POINT ( 'NONE',  ( 0.5774278215223103139, -0.5023911411419708095, -0.1820866141732282451 ) ) ;
#38720=CARTESIAN_POINT ( 'NONE',  ( -0.6496062992125976043, -0.5400638737290844871, 0.3530559997133364547 ) ) ;
#38721=EDGE_CURVE ( 'NONE', #71398, #18593, #59175, .T. ) ;
#38722=CARTESIAN_POINT ( 'NONE',  ( -0.4527559055118102749, -0.4536011799217368745, -0.2665933059059886201 ) ) ;
#38724=CARTESIAN_POINT ( 'NONE',  ( -0.2821522309711278487, 0.2952755905511811885, 0.1292274648535926551 ) ) ;
#38725=CARTESIAN_POINT ( 'NONE',  ( -0.2362204724409440182, -0.1870078740157479769, 0.4822834645669291653 ) ) ;
#38726=CARTESIAN_POINT ( 'NONE',  ( 0.1246719160104994284, -0.5511811023622046335, 0.09757992244046803654 ) ) ;
#38728=CARTESIAN_POINT ( 'NONE',  ( -0.1377952755905504645, -0.5400638737290845981, -0.3530559997133363437 ) ) ;
#38731=CARTESIAN_POINT ( 'NONE',  ( 1.089238845144357759, -0.004921259842519870586, -0.3153832671262229437 ) ) ;
#38732=CARTESIAN_POINT ( 'NONE',  ( 1.509186351706037543, -0.4281496062992127816, -0.4176697321401328100 ) ) ;
#38733=CARTESIAN_POINT ( 'NONE',  ( -0.6561679790026240244, -0.5023911411419708095, 0.1820866141732285504 ) ) ;
#38734=CARTESIAN_POINT ( 'NONE',  ( -0.5905511811023615998, 0.1771653543307087630, 0.000000000000000000 ) ) ;
#38735=CARTESIAN_POINT ( 'NONE',  ( -0.5577427821522301654, -0.3162353388693405765, 0.4822834645669290543 ) ) ;
#38736=CARTESIAN_POINT ( 'NONE',  ( 0.05249343832021075018, 0.2306618581243847221, -0.2411417322834647770 ) ) ;
#38737=CARTESIAN_POINT ( 'NONE',  ( 0.4921259842519691285, -0.4536011799217368745, -0.2665933059059886201 ) ) ;
#38739=CARTESIAN_POINT ( 'NONE',  ( 1.213910761154856299, -0.5511811023622048555, -0.09757992244046775898 ) ) ;
#38740=CARTESIAN_POINT ( 'NONE',  ( 0.6364829396325465405, -0.3162353388693409650, -0.4822834645669289433 ) ) ;
#38741=EDGE_CURVE ( 'NONE', #27293, #10557, #47928, .T. ) ;
#38743=CARTESIAN_POINT ( 'NONE',  ( -0.1574803149606292529, -0.1870078740157479769, 0.4822834645669291653 ) ) ;
#38745=CARTESIAN_POINT ( 'NONE',  ( 1.391076115485564868, -0.5023911411419708095, 0.1820866141732285504 ) ) ;
#38746=CARTESIAN_POINT ( 'NONE',  ( 1.043307086614173818, 0.1660481256975885056, 0.3530559997133364547 ) ) ;
#38747=CARTESIAN_POINT ( 'NONE',  ( 0.1968503937007881344, -0.6692913385826771977, 8.415575281601705876E-17 ) ) ;
#38749=CARTESIAN_POINT ( 'NONE',  ( 0.4002624671916016896, -0.08942795157527998196, 0.3641732283464567121 ) ) ;
#38750=CARTESIAN_POINT ( 'NONE',  ( 0.6036745406824154392, 0.2306618581243847221, -0.2411417322834647770 ) ) ;
#38751=CARTESIAN_POINT ( 'NONE',  ( -0.2493438320209966919, -0.004921259842519870586, -0.3153832671262229437 ) ) ;
#38752=CARTESIAN_POINT ( 'NONE',  ( -0.8661417322834640276, -0.1870078740157479769, 0.4822834645669291653 ) ) ;
#38754=CARTESIAN_POINT ( 'NONE',  ( -0.1968503937007867743, -0.6692913385826771977, 8.415575281601705876E-17 ) ) ;
#38755=CARTESIAN_POINT ( 'NONE',  ( -1.397637795275589623, -0.5400638737290845981, -0.3530559997133363437 ) ) ;
#38756=CARTESIAN_POINT ( 'NONE',  ( -0.6167979002624665030, -0.004921259842519576551, 0.3153832671262227771 ) ) ;
#38757=CARTESIAN_POINT ( 'NONE',  ( 0.2296587926509192634, -0.05778040916215560624, -0.4822834645669293319 ) ) ;
#38758=CARTESIAN_POINT ( 'NONE',  ( -1.128608923884513837, -0.6046776061558807314, 0.2411417322834647770 ) ) ;
#38759=CARTESIAN_POINT ( 'NONE',  ( -0.4199475065616791736, -0.6046776061558807314, 0.2411417322834647770 ) ) ;
#38761=CARTESIAN_POINT ( 'NONE',  ( 1.469816272965879911, 0.2306618581243847221, -0.2411417322834647770 ) ) ;
#38762=CARTESIAN_POINT ( 'NONE',  ( 1.437007874015748810, -0.5400638737290845981, -0.3530559997133363437 ) ) ;
#38765=CARTESIAN_POINT ( 'NONE',  ( -1.082677165354329896, 0.1660481256975885056, 0.3530559997133364547 ) ) ;
#38769=CARTESIAN_POINT ( 'NONE',  ( -0.2362204724409440182, -0.1870078740157479769, 0.3641732283464567677 ) ) ;
#38771=VERTEX_POINT ( 'NONE', #3605 ) ;
#38772=CARTESIAN_POINT ( 'NONE',  ( 0.2034120734908142214, 0.2952755905511810774, -0.1292274648535930714 ) ) ;
#38773=CARTESIAN_POINT ( 'NONE',  ( 0.6233595800524939223, -0.3162353388693405765, 0.4822834645669290543 ) ) ;
#38775=CARTESIAN_POINT ( 'NONE',  ( -0.5404819259526909558, -4.992347309556208597E-15, 0.4118484887281982920 ) ) ;
#38776=CARTESIAN_POINT ( 'NONE',  ( -0.3280839895013117347, -0.004921259842519870586, -0.3153832671262229437 ) ) ;
#38777=CARTESIAN_POINT ( 'NONE',  ( 0.3821149210511736727, 0.02791078216816508459, -0.4328096321851889194 ) ) ;
#38778=CARTESIAN_POINT ( 'NONE',  ( 0.6627296587926517768, -0.6692913385826773087, -0.1292274648535924053 ) ) ;
#38779=CARTESIAN_POINT ( 'NONE',  ( 0.9514435695538062676, -0.08942795157527998196, 0.3641732283464567121 ) ) ;
#38780=CARTESIAN_POINT ( 'NONE',  ( -0.5971128608923877978, -0.6692913385826773087, -0.1292274648535924053 ) ) ;
#38782=CARTESIAN_POINT ( 'NONE',  ( -0.6299212598425188991, -0.1870078740157480879, -0.4822834645669291653 ) ) ;
#38783=CARTESIAN_POINT ( 'NONE',  ( -1.318897637795274802, -0.4536011799217368745, -0.2665933059059886201 ) ) ;
#38784=CARTESIAN_POINT ( 'NONE',  ( -0.8267716535433065062, -0.6692913385826771977, 8.415575281601705876E-17 ) ) ;
#38785=CARTESIAN_POINT ( 'NONE',  ( 1.640419947506562393, -0.4281496062992124485, 0.4176697321401328655 ) ) ;
#38789=CARTESIAN_POINT ( 'NONE',  ( 0.2034120734908144990, -0.6692913385826771977, 0.1292274648535927661 ) ) ;
#38791=CARTESIAN_POINT ( 'NONE',  ( -0.8661417322834640276, -0.1870078740157480879, -0.4822834645669291653 ) ) ;
#38793=CARTESIAN_POINT ( 'NONE',  ( 1.325459317585302665, 0.05413385826771626580, -0.4176697321401330321 ) ) ;
#38794=CARTESIAN_POINT ( 'NONE',  ( 1.128608923884514947, 0.2306618581243848609, 0.2411417322834645549 ) ) ;
#38795=CARTESIAN_POINT ( 'NONE',  ( 0.6102362204724416372, -0.5400638737290844871, 0.3530559997133364547 ) ) ;
#38796=CARTESIAN_POINT ( 'NONE',  ( 0.2296587926509192634, -0.3162353388693405765, 0.4822834645669290543 ) ) ;
#38798=CARTESIAN_POINT ( 'NONE',  ( -1.122047244094487306, -0.5400638737290844871, 0.3530559997133364547 ) ) ;
#38799=CARTESIAN_POINT ( 'NONE',  ( -0.02624671916010428221, 0.2306618581243847221, -0.2411417322834647770 ) ) ;
#38800=CARTESIAN_POINT ( 'NONE',  ( -0.2165354330708654795, 0.07958543189024085140, 0.2665933059059887866 ) ) ;
#38801=FACE_OUTER_BOUND ( 'NONE', #82349, .T. ) ;
#38802=CARTESIAN_POINT ( 'NONE',  ( -0.05249343832020938322, -0.6046776061558809534, -0.2411417322834644161 ) ) ;
#38803=LINE ( 'NONE', #14824, #27858 ) ;
#38805=CARTESIAN_POINT ( 'NONE',  ( 1.332020997375328974, -0.05778040916215560624, -0.4822834645669293319 ) ) ;
#38808=ORIENTED_EDGE ( 'NONE', *, *, #27035, .T. ) ;
#38809=CARTESIAN_POINT ( 'NONE',  ( 0.4461942257217856311, 0.2306618581243847221, -0.2411417322834647770 ) ) ;
#38810=CARTESIAN_POINT ( 'NONE',  ( -0.3083989501312330295, -0.08942795157527998196, 0.3641732283464567121 ) ) ;
#38811=CARTESIAN_POINT ( 'NONE',  ( 1.633858267716535639, -0.4536011799217367080, 0.2665933059059888421 ) ) ;
#38814=CARTESIAN_POINT ( 'NONE',  ( 1.614173228346457378, 0.2952755905511811885, 0.000000000000000000 ) ) ;
#38816=CARTESIAN_POINT ( 'NONE',  ( -0.1509186351706028884, -0.05778040916215522460, 0.4822834645669289988 ) ) ;
#38818=CARTESIAN_POINT ( 'NONE',  ( -1.397637795275589623, 0.1660481256975885056, 0.3530559997133364547 ) ) ;
#38819=CARTESIAN_POINT ( 'NONE',  ( 0.3543307086614179147, 0.2952755905511811885, 0.000000000000000000 ) ) ;
#38821=CARTESIAN_POINT ( 'NONE',  ( 1.535433070866142558, 0.2952755905511811885, 0.000000000000000000 ) ) ;
#38822=CARTESIAN_POINT ( 'NONE',  ( 0.8333333333333340365, 0.2952755905511810774, -0.1292274648535930714 ) ) ;
#38823=CARTESIAN_POINT ( 'NONE',  ( 0.9908136482939640111, -0.5511811023622046335, 0.09757992244046803654 ) ) ;
#38824=CARTESIAN_POINT ( 'NONE',  ( -0.02624671916010428221, 0.2306618581243847221, -0.2411417322834647770 ) ) ;
#38825=CARTESIAN_POINT ( 'NONE',  ( 0.7874015748031503170, -0.1870078740157480601, -0.3641732283464567677 ) ) ;
#38826=CARTESIAN_POINT ( 'NONE',  ( -1.384514435695537005, -0.6692913385826773087, -0.1292274648535924053 ) ) ;
#38828=CARTESIAN_POINT ( 'NONE',  ( 1.003937007874016407, -0.5400638737290844871, 0.3530559997133364547 ) ) ;
#38829=( BOUNDED_SURFACE ( )  B_SPLINE_SURFACE ( 1, 2, ( 
 ( #60772, #61185, #15347, #54451, #27957, #80163, #22480, #48141, #74668, #3539, #36344, #47304, #72994, #41008, #68349, #66692, #9027, #30440, #83032, #68752, #18238, #24936, #69978, #75898, #11513, #37579, #50606, #63666, #11094, #24535, #51017, #4764, #37169, #63252, #62849, #69162, #5592, #36751, #6006, #17424, #49790, #12333, #24121, #62427, #82620, #25355, #44288, #31258, #69576, #76716, #76313, #50201, #57336, #31675, #37990, #56105, #19049, #56926, #43878, #11924, #81809, #75492, #18644, #17831, #44696, #70393, #12748, #38407, #4355, #30023, #43465, #5185, #55687, #30849, #56514, #81394, #23710, #49381, #75077, #82217, #43055, #46802, #65356, #52693, #70826, #64501, #46383, #26622, #27031, #7694, #13173, #6839, #26194, #78400, #20310, #52276, #32510, #40087, #45543, #32934, #64924, #33361, #71241, #59024, #19468, #58172, #77980, #38823, #45961, #71657, #13585, #39240, #65774, #1788, #45118, #19896, #14009, #25771, #7262, #51855, #20732, #968, #541, #1380, #59434, #72076, #27448, #53109, #21147, #77562, #14435, #58599, #33772, #39666, #8106, #78818, #72493, #51432, #14842, #64087, #6424, #32093, #57754, #116, #77135, #29520, #74156, #74574, #2203, #59851, #28698, #53942, #9759, #48874, #15257, #2624, #60274, #73750, #73327, #41335, #35846, #8520, #67425, #28280, #27871, #79655, #16086, #3033, #15674, #79239, #40916, #29110, #35019, #40502, #22389, #34609, #53531, #21554, #55181, #54780, #3446, #67015, #47215, #10181, #66184, #34187, #54360, #72905, #35430, #66598, #9348, #8932, #80072, #21971, #61515, #47633, #48049, #61095, #22796, #41731, #60683, #80483, #48456, #16504, #42147, #67842, #3860, #80890, #23203, #75799, #49694, #81716, #18141, #49284, #76212, #29926, #62329, #82523, #36654, #23615, #11831, #12237, #56826, #50102, #82120, #5904, #5497, #62754, #69883, #44193, #24841, #17332, #50508, #43775, #56420, #24435, #74987, #18548, #37893, #69478, #55589, #50919, #63569, #30758, #24026, #4666, #37484, #30339, #31576, #5090, #56005, #42962, #57232, #36252, #82933, #25255, #16919, #68656, #75389, #42556, #68260, #10994, #4263, #10596, #61922, #81301, #17735, #43364, #69064, #11414, #37069, #63158, #31159, #52590, #46280, #70292, #64816, #12644, #7157, #45016, #1280, #59331, #16, #435, #1688, #71976, #57654, #33669, #19366, #13478, #25670, #26929, #65678, #13903, #18950, #65250, #14330, #26090, #78297, #32828, #77453, #77034, #6317, #20629, #13067, #58496, #63980, #51750, #76619, #19788, #45440, #71136, #33259, #860, #27346, #44597, #38306, #39988, #8005, #31994, #6735, #51330, #39136, #70716, #52172, #26517, #58921, #38722, #64399, #7587, #32406, #77875, #20206, #45856, #58069, #71554, #39561, #3342, #3756, #14744, #72394, #41230, #66493, #22284, #61407, #27765, #15151, #72802, #2934, #2522, #53838, #48355, #21042, #79971, #40808, #40398, #8827, #28598, #15571, #28180, #8415, #53430, #41636, #47529, #53004, #34921, #47113, #66079, #34083, #42046, #67327, #15989, #79551, #59746, #22696, #78717, #46701, #66917, #2100, #47945, #79138, #60584, #21455, #67742, #9660, #29006, #35330, #54255, #74053, #34504, #21864, #10075, #60168, #73220, #60993, #54672, #73647, #9249, #80384, #16400, #35739, #30664, #18048, #36151, #29828, #11738, #75294, #75707, #56327, #61824, #55491, #74888, #43681, #68967, #17638, #81201, #5402, #10900, #81619, #30244, #82026, #36558, #24340, #68153, #23516, #43270, #4164, #11316, #36975, #62235, #4573, #31065, #51542, #10497, #68557, #62655, #74470, #55907, #17234, #69384, #49600, #49185, #50009, #25881, #37393, #42864, #63065, #4996, #56733, #230, #23933, #77245, #19575, #45235, #70935, #64612, #13280, #38932, #29421, #55079, #80788, #23103, #48771, #16817, #42453, #33038, #40603, #26305, #53631, #47319, #2312, #13693, #52379, #72598, #14944, #58707, #77670, #73010, #58282, #27973, #39348, #647, #26725, #46903, #79339, #1072, #14117, #66286, #59957, #51963, #78511, #20000, #20834, #78088, #8625, #15361, #65033, #39770, #41022, #21659, #71346, #6949, #20419, #27137, #7368, #34296, #32620, #27556, #45651, #78926, #46072 ),
 ( #53215, #65465, #71764, #7799, #33464, #59126, #52802, #1483, #1896, #46487, #72182, #14540, #40192, #21248, #65875, #8210, #33875, #59540, #41435, #41839, #55701, #47735, #73852, #74681, #48982, #10288, #29220, #60786, #9041, #49397, #67946, #55289, #73433, #67118, #17027, #54887, #29629, #35955, #15783, #9449, #28802, #80999, #22900, #80592, #35120, #42666, #48157, #68365, #23313, #74265, #4370, #3139, #67529, #81409, #54466, #16193, #10703, #36359, #61624, #48567, #80179, #34715, #75091, #3966, #62034, #22494, #9867, #30039, #16608, #23726, #17439, #35536, #61198, #3555, #66708, #42251, #60376, #2724, #28385, #54045, #79759, #22076, #69991, #24550, #38002, #81825, #69175, #56938, #17845, #5605, #82635, #75912, #18251, #44709, #64101, #24135, #82231, #24948, #4779, #69590, #30863, #31690, #63264, #49805, #63680, #38419, #57348, #6436, #32107, #128, #56528, #51030, #50216, #12762, #18656, #76326, #25367, #75506, #30455, #83044, #76729, #11936, #31273, #43893, #37591, #50621, #57766, #19061, #77148, #56119, #62443, #44300, #12346, #6018, #51444, #43479, #5199, #62862, #70406, #25783, #43069, #68766, #11110, #36767, #11526, #37183, #39252, #52704, #65370, #77993, #58183, #19906, #8118, #38835, #33372, #6851, #52288, #19480, #45974, #71669, #20321, #59447, #7705, #2215, #70837, #13186, #53541, #14021, #64514, #59036, #45556, #14853, #553, #1390, #40097, #64934, #7274, #78415, #39678, #27044, #40514, #32521, #46394, #32945, #26206, #58611, #20744, #72088, #14446, #51868, #21157, #77574, #979, #71252, #65785, #13598, #26634, #33783, #8531, #1799, #27462, #53120, #78831, #72504, #45133, #46813, #66194, #34198, #59862, #27881, #61106, #47644, #10607, #42159, #55194, #10192, #3458, #16930, #53952, #54372, #68272, #60284, #3043, #3872, #61526, #22810, #41741, #73339, #21564, #61933, #80494, #67854, #2634, #79665, #29531, #67435, #35861, #48467, #28290, #21982, #41345, #80901, #35440, #9769, #15687, #23215, #60693, #48059, #80082, #74168, #28708, #16515, #34620, #67025, #29123, #9358, #54791, #48885, #22402, #73761, #74586, #42570, #35029, #16096, #36264, #40928, #4276, #29937, #79249, #47226, #72916, #15267, #66608, #8944, #18960, #44608, #12657, #69077, #63580, #62768, #25265, #31170, #5507, #37903, #36666, #42972, #69893, #5914, #82132, #18154, #30769, #11427, #11841, #70304, #31588, #6333, #17344, #74998, #43786, #37082, #24852, #63992, #30351, #12247, #63169, #76629, #56020, #56430, #38318, #62341, #5102, #57243, #82947, #82534, #69492, #49707, #81313, #55601, #56836, #44203, #4680, #81728, #50931, #37494, #18559, #50520, #24037, #75402, #17748, #23626, #76226, #49297, #43377, #68668, #24446, #50114, #75811, #11007, #77466, #13918, #45029, #6747, #873, #38735, #32841, #26532, #45452, #71150, #78310, #71989, #70728, #51764, #52185, #51341, #13491, #26102, #7600, #7170, #13082, #39574, #14342, #33274, #40002, #65690, #8018, #19803, #1292, #39147, #20641, #20220, #77889, #58934, #64412, #77045, #26942, #52603, #64832, #58510, #45869, #71567, #65264, #33681, #46294, #59343, #19377, #25681, #32006, #57666, #28, #32419, #58081, #447, #43643, #57101, #56694, #24711, #19225, #75256, #50790, #69346, #11278, #11700, #82796, #69754, #82393, #62615, #25532, #81987, #37354, #49971, #5769, #18009, #68929, #36937, #12928, #38170, #70156, #50379, #4957, #76895, #23896, #17600, #12100, #30625, #18818, #56290, #31438, #75669, #38588, #12509, #83210, #24301, #63027, #25120, #5365, #76077, #31026, #63844, #44062, #18421, #44465, #44875, #6182, #70574, #64266, #6600, #37758, #31860, #63433, #32272, #76491, #57519, #51197, #57932, #49562, #43232, #59563, #65489, #21272, #14968, #38950, #33488, #64634, #59150, #13718, #53238, #27996, #51986, #52401, #53655, #40626, #26324, #2339, #71368, #7821, #77691, #78954, #34319, #65897, #70953, #33898, #66308, #78110, #46927, #1507, #46096, #52823, #39371, #13298, #6969, #27160, #32640, #20442, #45257, #71788, #14142, #39794, #1919, #78535, #79363, #58304, #669, #20021, #20858, #45672, #46510, #65057, #8648, #7394, #72211, #8233 ) ),
 .UNSPECIFIED., .F., .F., .F. ) 
 B_SPLINE_SURFACE_WITH_KNOTS ( ( 2, 2 ),
 ( 3, 2, 2, 2, 2, 2, 2, 2, 2, 2, 2, 2, 2, 2, 2, 2, 2, 2, 2, 2, 2, 2, 2, 2, 2, 2, 2, 2, 2, 2, 2, 2, 2, 2, 2, 2, 2, 2, 2, 2, 2, 2, 2, 2, 2, 2, 2, 2, 2, 2, 2, 2, 2, 2, 2, 2, 2, 2, 2, 2, 2, 2, 2, 2, 2, 2, 2, 2, 2, 2, 2, 2, 2, 2, 2, 2, 2, 2, 2, 2, 2, 2, 2, 2, 2, 2, 2, 2, 2, 2, 2, 2, 2, 2, 2, 2, 2, 2, 2, 2, 2, 2, 2, 2, 2, 2, 2, 2, 2, 2, 2, 2, 2, 2, 2, 2, 2, 2, 2, 2, 2, 2, 2, 2, 2, 2, 2, 2, 2, 2, 2, 2, 2, 2, 2, 2, 2, 2, 2, 2, 2, 2, 2, 2, 2, 2, 2, 2, 2, 2, 2, 2, 2, 2, 2, 2, 2, 2, 2, 2, 2, 2, 2, 2, 2, 2, 2, 2, 2, 2, 2, 2, 2, 2, 2, 2, 2, 2, 2, 2, 2, 2, 2, 2, 2, 2, 2, 2, 2, 2, 2, 2, 2, 2, 2, 2, 2, 2, 2, 2, 2, 2, 2, 2, 2, 2, 2, 2, 2, 2, 2, 2, 2, 2, 2, 2, 2, 2, 2, 2, 2, 2, 2, 2, 2, 2, 2, 2, 2, 2, 2, 2, 2, 2, 2, 2, 2, 2, 2, 2, 2, 2, 2, 2, 2, 2, 2, 2, 2, 2, 2, 2, 2, 2, 2, 3 ),
 ( 0.000000000000000000, 1.000000000000000000 ),
 ( 0.000000000000000000, 0.003787878787878787984, 0.007575757575757575968, 0.01136363636363636395, 0.01515151515151515194, 0.01893939393939393992, 0.02272727272727272790, 0.02651515151515151589, 0.03030303030303030387, 0.03409090909090908839, 0.03787878787878787984, 0.04166666666666666435, 0.04545454545454545581, 0.04924242424242424032, 0.05303030303030303177, 0.05681818181818181629, 0.06060606060606060774, 0.06439393939393939226, 0.06818181818181817677, 0.07196969696969697516, 0.07575757575757575968, 0.07954545454545454419, 0.08333333333333332871, 0.08712121212121212710, 0.09090909090909091161, 0.09469696969696969613, 0.09848484848484848064, 0.1022727272727272790, 0.1060606060606060635, 0.1098484848484848481, 0.1136363636363636326, 0.1174242424242424310, 0.1212121212121212155, 0.1250000000000000000, 0.1287878787878787845, 0.1325757575757575690, 0.1363636363636363535, 0.1401515151515151381, 0.1439393939393939503, 0.1477272727272727348, 0.1515151515151515194, 0.1553030303030303039, 0.1590909090909090884, 0.1628787878787878729, 0.1666666666666666574, 0.1704545454545454419, 0.1742424242424242542, 0.1780303030303030387, 0.1818181818181818232, 0.1856060606060606077, 0.1893939393939393923, 0.1931818181818181768, 0.1969696969696969613, 0.2007575757575757458, 0.2045454545454545581, 0.2083333333333333426, 0.2121212121212121271, 0.2159090909090909116, 0.2196969696969696961, 0.2234848484848484806, 0.2272727272727272652, 0.2310606060606060497, 0.2348484848484848619, 0.2386363636363636465, 0.2424242424242424310, 0.2462121212121212155, 0.2500000000000000000, 0.2537878787878787845, 0.2575757575757575690, 0.2613636363636363535, 0.2651515151515151381, 0.2689393939393939226, 0.2727272727272727071, 0.2765151515151514916, 0.2803030303030302761, 0.2840909090909091161, 0.2878787878787879007, 0.2916666666666666852, 0.2954545454545454697, 0.2992424242424242542, 0.3030303030303030387, 0.3068181818181818232, 0.3106060606060606077, 0.3143939393939393923, 0.3181818181818181768, 0.3219696969696969613, 0.3257575757575757458, 0.3295454545454545303, 0.3333333333333333148, 0.3371212121212120993, 0.3409090909090908839, 0.3446969696969697239, 0.3484848484848485084, 0.3522727272727272929, 0.3560606060606060774, 0.3598484848484848619, 0.3636363636363636465, 0.3674242424242424310, 0.3712121212121212155, 0.3750000000000000000, 0.3787878787878787845, 0.3825757575757575690, 0.3863636363636363535, 0.3901515151515151381, 0.3939393939393939226, 0.3977272727272727071, 0.4015151515151514916, 0.4053030303030302761, 0.4090909090909091161, 0.4128787878787879007, 0.4166666666666666852, 0.4204545454545454697, 0.4242424242424242542, 0.4280303030303030387, 0.4318181818181818232, 0.4356060606060606077, 0.4393939393939393923, 0.4431818181818181768, 0.4469696969696969613, 0.4507575757575757458, 0.4545454545454545303, 0.4583333333333333148, 0.4621212121212120993, 0.4659090909090908839, 0.4696969696969697239, 0.4734848484848485084, 0.4772727272727272929, 0.4810606060606060774, 0.4848484848484848619, 0.4886363636363636465, 0.4924242424242424310, 0.4962121212121212155, 0.5000000000000000000, 0.5037878787878787845, 0.5075757575757575690, 0.5113636363636363535, 0.5151515151515151381, 0.5189393939393939226, 0.5227272727272727071, 0.5265151515151514916, 0.5303030303030302761, 0.5340909090909090606, 0.5378787878787878451, 0.5416666666666666297, 0.5454545454545454142, 0.5492424242424241987, 0.5530303030303029832, 0.5568181818181817677, 0.5606060606060605522, 0.5643939393939394478, 0.5681818181818182323, 0.5719696969696970168, 0.5757575757575758013, 0.5795454545454545858, 0.5833333333333333703, 0.5871212121212121549, 0.5909090909090909394, 0.5946969696969697239, 0.5984848484848485084, 0.6022727272727272929, 0.6060606060606060774, 0.6098484848484848619, 0.6136363636363636465, 0.6174242424242424310, 0.6212121212121212155, 0.6250000000000000000, 0.6287878787878787845, 0.6325757575757575690, 0.6363636363636363535, 0.6401515151515151381, 0.6439393939393939226, 0.6477272727272727071, 0.6515151515151514916, 0.6553030303030302761, 0.6590909090909090606, 0.6628787878787878451, 0.6666666666666666297, 0.6704545454545454142, 0.6742424242424241987, 0.6780303030303029832, 0.6818181818181817677, 0.6856060606060605522, 0.6893939393939394478, 0.6931818181818182323, 0.6969696969696970168, 0.7007575757575758013, 0.7045454545454545858, 0.7083333333333333703, 0.7121212121212121549, 0.7159090909090909394, 0.7196969696969697239, 0.7234848484848485084, 0.7272727272727272929, 0.7310606060606060774, 0.7348484848484848619, 0.7386363636363636465, 0.7424242424242424310, 0.7462121212121212155, 0.7500000000000000000, 0.7537878787878787845, 0.7575757575757575690, 0.7613636363636363535, 0.7651515151515151381, 0.7689393939393939226, 0.7727272727272727071, 0.7765151515151514916, 0.7803030303030302761, 0.7840909090909090606, 0.7878787878787878451, 0.7916666666666666297, 0.7954545454545454142, 0.7992424242424241987, 0.8030303030303029832, 0.8068181818181817677, 0.8106060606060605522, 0.8143939393939394478, 0.8181818181818182323, 0.8219696969696970168, 0.8257575757575758013, 0.8295454545454545858, 0.8333333333333333703, 0.8371212121212121549, 0.8409090909090909394, 0.8446969696969697239, 0.8484848484848485084, 0.8522727272727272929, 0.8560606060606060774, 0.8598484848484848619, 0.8636363636363636465, 0.8674242424242424310, 0.8712121212121212155, 0.8750000000000000000, 0.8787878787878787845, 0.8825757575757575690, 0.8863636363636363535, 0.8901515151515151381, 0.8939393939393939226, 0.8977272727272727071, 0.9015151515151514916, 0.9053030303030302761, 0.9090909090909090606, 0.9128787878787878451, 0.9166666666666666297, 0.9204545454545454142, 0.9242424242424241987, 0.9280303030303029832, 0.9318181818181817677, 0.9356060606060605522, 0.9393939393939394478, 0.9431818181818182323, 0.9469696969696970168, 0.9507575757575758013, 0.9545454545454545858, 0.9583333333333333703, 0.9621212121212121549, 0.9659090909090909394 ),
 .UNSPECIFIED. ) 
 GEOMETRIC_REPRESENTATION_ITEM ( )  RATIONAL_B_SPLINE_SURFACE ( (
 ( 1.000000000000000000, 0.9659258262890683122, 1.000000000000000000, 0.9659258262890683122, 1.000000000000000000, 0.9659258262890683122, 1.000000000000000000, 0.9659258262890683122, 1.000000000000000000, 0.9659258262890683122, 1.000000000000000000, 0.9659258262890683122, 1.000000000000000000, 0.9659258262890683122, 1.000000000000000000, 0.9659258262890683122, 1.000000000000000000, 0.9659258262890683122, 1.000000000000000000, 0.9659258262890683122, 1.000000000000000000, 0.9659258262890683122, 1.000000000000000000, 0.9659258262890683122, 1.000000000000000000, 0.9659258262890683122, 1.000000000000000000, 0.9659258262890683122, 1.000000000000000000, 0.9659258262890683122, 1.000000000000000000, 0.9659258262890683122, 1.000000000000000000, 0.9659258262890683122, 1.000000000000000000, 0.9659258262890683122, 1.000000000000000000, 0.9659258262890683122, 1.000000000000000000, 0.9659258262890683122, 1.000000000000000000, 0.9659258262890683122, 1.000000000000000000, 0.9659258262890683122, 1.000000000000000000, 0.9659258262890683122, 1.000000000000000000, 0.9659258262890683122, 1.000000000000000000, 0.9659258262890683122, 1.000000000000000000, 0.9659258262890683122, 1.000000000000000000, 0.9659258262890683122, 1.000000000000000000, 0.9659258262890683122, 1.000000000000000000, 0.9659258262890683122, 1.000000000000000000, 0.9659258262890683122, 1.000000000000000000, 0.9659258262890683122, 1.000000000000000000, 0.9659258262890683122, 1.000000000000000000, 0.9659258262890683122, 1.000000000000000000, 0.9659258262890683122, 1.000000000000000000, 0.9659258262890683122, 1.000000000000000000, 0.9659258262890683122, 1.000000000000000000, 0.9659258262890683122, 1.000000000000000000, 0.9659258262890683122, 1.000000000000000000, 0.9659258262890683122, 1.000000000000000000, 0.9659258262890683122, 1.000000000000000000, 0.9659258262890683122, 1.000000000000000000, 0.9659258262890683122, 1.000000000000000000, 0.9659258262890683122, 1.000000000000000000, 0.9659258262890683122, 1.000000000000000000, 0.9659258262890683122, 1.000000000000000000, 0.9659258262890683122, 1.000000000000000000, 0.9659258262890683122, 1.000000000000000000, 0.9659258262890683122, 1.000000000000000000, 0.9659258262890683122, 1.000000000000000000, 0.9659258262890683122, 1.000000000000000000, 0.9659258262890683122, 1.000000000000000000, 0.9659258262890683122, 1.000000000000000000, 0.9659258262890683122, 1.000000000000000000, 0.9659258262890683122, 1.000000000000000000, 0.9659258262890683122, 1.000000000000000000, 0.9659258262890683122, 1.000000000000000000, 0.9659258262890683122, 1.000000000000000000, 0.9659258262890683122, 1.000000000000000000, 0.9659258262890683122, 1.000000000000000000, 0.9659258262890683122, 1.000000000000000000, 0.9659258262890683122, 1.000000000000000000, 0.9659258262890683122, 1.000000000000000000, 0.9659258262890683122, 1.000000000000000000, 0.9659258262890683122, 1.000000000000000000, 0.9659258262890683122, 1.000000000000000000, 0.9659258262890683122, 1.000000000000000000, 0.9659258262890683122, 1.000000000000000000, 0.9659258262890683122, 1.000000000000000000, 0.9659258262890683122, 1.000000000000000000, 0.9659258262890683122, 1.000000000000000000, 0.9659258262890683122, 1.000000000000000000, 0.9659258262890683122, 1.000000000000000000, 0.9659258262890683122, 1.000000000000000000, 0.9659258262890683122, 1.000000000000000000, 0.9659258262890683122, 1.000000000000000000, 0.9659258262890683122, 1.000000000000000000, 0.9659258262890683122, 1.000000000000000000, 0.9659258262890683122, 1.000000000000000000, 0.9659258262890683122, 1.000000000000000000, 0.9659258262890683122, 1.000000000000000000, 0.9659258262890683122, 1.000000000000000000, 0.9659258262890683122, 1.000000000000000000, 0.9659258262890683122, 1.000000000000000000, 0.9659258262890683122, 1.000000000000000000, 0.9659258262890683122, 1.000000000000000000, 0.9659258262890683122, 1.000000000000000000, 0.9659258262890683122, 1.000000000000000000, 0.9659258262890683122, 1.000000000000000000, 0.9659258262890683122, 1.000000000000000000, 0.9659258262890683122, 1.000000000000000000, 0.9659258262890683122, 1.000000000000000000, 0.9659258262890683122, 1.000000000000000000, 0.9659258262890683122, 1.000000000000000000, 0.9659258262890683122, 1.000000000000000000, 0.9659258262890683122, 1.000000000000000000, 0.9659258262890683122, 1.000000000000000000, 0.9659258262890683122, 1.000000000000000000, 0.9659258262890683122, 1.000000000000000000, 0.9659258262890683122, 1.000000000000000000, 0.9659258262890683122, 1.000000000000000000, 0.9659258262890683122, 1.000000000000000000, 0.9659258262890683122, 1.000000000000000000, 0.9659258262890683122, 1.000000000000000000, 0.9659258262890683122, 1.000000000000000000, 0.9659258262890683122, 1.000000000000000000, 0.9659258262890683122, 1.000000000000000000, 0.9659258262890683122, 1.000000000000000000, 0.9659258262890683122, 1.000000000000000000, 0.9659258262890683122, 1.000000000000000000, 0.9659258262890683122, 1.000000000000000000, 0.9659258262890683122, 1.000000000000000000, 0.9659258262890683122, 1.000000000000000000, 0.9659258262890683122, 1.000000000000000000, 0.9659258262890683122, 1.000000000000000000, 0.9659258262890683122, 1.000000000000000000, 0.9659258262890683122, 1.000000000000000000, 0.9659258262890683122, 1.000000000000000000, 0.9659258262890683122, 1.000000000000000000, 0.9659258262890683122, 1.000000000000000000, 0.9659258262890683122, 1.000000000000000000, 0.9659258262890683122, 1.000000000000000000, 0.9659258262890683122, 1.000000000000000000, 0.9659258262890683122, 1.000000000000000000, 0.9659258262890683122, 1.000000000000000000, 0.9659258262890683122, 1.000000000000000000, 0.9659258262890683122, 1.000000000000000000, 0.9659258262890683122, 1.000000000000000000, 0.9659258262890683122, 1.000000000000000000, 0.9659258262890683122, 1.000000000000000000, 0.9659258262890683122, 1.000000000000000000, 0.9659258262890683122, 1.000000000000000000, 0.9659258262890683122, 1.000000000000000000, 0.9659258262890683122, 1.000000000000000000, 0.9659258262890683122, 1.000000000000000000, 0.9659258262890683122, 1.000000000000000000, 0.9659258262890683122, 1.000000000000000000, 0.9659258262890683122, 1.000000000000000000, 0.9659258262890683122, 1.000000000000000000, 0.9659258262890683122, 1.000000000000000000, 0.9659258262890683122, 1.000000000000000000, 0.9659258262890683122, 1.000000000000000000, 0.9659258262890683122, 1.000000000000000000, 0.9659258262890683122, 1.000000000000000000, 0.9659258262890683122, 1.000000000000000000, 0.9659258262890683122, 1.000000000000000000, 0.9659258262890683122, 1.000000000000000000, 0.9659258262890683122, 1.000000000000000000, 0.9659258262890683122, 1.000000000000000000, 0.9659258262890683122, 1.000000000000000000, 0.9659258262890683122, 1.000000000000000000, 0.9659258262890683122, 1.000000000000000000, 0.9659258262890683122, 1.000000000000000000, 0.9659258262890683122, 1.000000000000000000, 0.9659258262890683122, 1.000000000000000000, 0.9659258262890683122, 1.000000000000000000, 0.9659258262890683122, 1.000000000000000000, 0.9659258262890683122, 1.000000000000000000, 0.9659258262890683122, 1.000000000000000000, 0.9659258262890683122, 1.000000000000000000, 0.9659258262890683122, 1.000000000000000000, 0.9659258262890683122, 1.000000000000000000, 0.9659258262890683122, 1.000000000000000000, 0.9659258262890683122, 1.000000000000000000, 0.9659258262890683122, 1.000000000000000000, 0.9659258262890683122, 1.000000000000000000, 0.9659258262890683122, 1.000000000000000000, 0.9659258262890683122, 1.000000000000000000, 0.9659258262890683122, 1.000000000000000000, 0.9659258262890683122, 1.000000000000000000, 0.9659258262890683122, 1.000000000000000000, 0.9659258262890683122, 1.000000000000000000, 0.9659258262890683122, 1.000000000000000000, 0.9659258262890683122, 1.000000000000000000, 0.9659258262890683122, 1.000000000000000000, 0.9659258262890683122, 1.000000000000000000, 0.9659258262890683122, 1.000000000000000000, 0.9659258262890683122, 1.000000000000000000, 0.9659258262890683122, 1.000000000000000000, 0.9659258262890683122, 1.000000000000000000, 0.9659258262890683122, 1.000000000000000000, 0.9659258262890683122, 1.000000000000000000, 0.9659258262890683122, 1.000000000000000000, 0.9659258262890683122, 1.000000000000000000, 0.9659258262890683122, 1.000000000000000000, 0.9659258262890683122, 1.000000000000000000, 0.9659258262890683122, 1.000000000000000000, 0.9659258262890683122, 1.000000000000000000, 0.9659258262890683122, 1.000000000000000000, 0.9659258262890683122, 1.000000000000000000, 0.9659258262890683122, 1.000000000000000000, 0.9659258262890683122, 1.000000000000000000, 0.9659258262890683122, 1.000000000000000000, 0.9659258262890683122, 1.000000000000000000, 0.9659258262890683122, 1.000000000000000000, 0.9659258262890683122, 1.000000000000000000, 0.9659258262890683122, 1.000000000000000000, 0.9659258262890683122, 1.000000000000000000, 0.9659258262890683122, 1.000000000000000000, 0.9659258262890683122, 1.000000000000000000, 0.9659258262890683122, 1.000000000000000000, 0.9659258262890683122, 1.000000000000000000, 0.9659258262890683122, 1.000000000000000000, 0.9659258262890683122, 1.000000000000000000, 0.9659258262890683122, 1.000000000000000000, 0.9659258262890683122, 1.000000000000000000, 0.9659258262890683122, 1.000000000000000000, 0.9659258262890683122, 1.000000000000000000, 0.9659258262890683122, 1.000000000000000000, 0.9659258262890683122, 1.000000000000000000, 0.9659258262890683122, 1.000000000000000000, 0.9659258262890683122, 1.000000000000000000, 0.9659258262890683122, 1.000000000000000000, 0.9659258262890683122, 1.000000000000000000, 0.9659258262890683122, 1.000000000000000000, 0.9659258262890683122, 1.000000000000000000, 0.9659258262890683122, 1.000000000000000000, 0.9659258262890683122, 1.000000000000000000, 0.9659258262890683122, 1.000000000000000000, 0.9659258262890683122, 1.000000000000000000, 0.9659258262890683122, 1.000000000000000000, 0.9659258262890683122, 1.000000000000000000, 0.9659258262890683122, 1.000000000000000000, 0.9659258262890683122, 1.000000000000000000, 0.9659258262890683122, 1.000000000000000000, 0.9659258262890683122, 1.000000000000000000, 0.9659258262890683122, 1.000000000000000000, 0.9659258262890683122, 1.000000000000000000, 0.9659258262890683122, 1.000000000000000000, 0.9659258262890683122, 1.000000000000000000, 0.9659258262890683122, 1.000000000000000000, 0.9659258262890683122, 1.000000000000000000, 0.9659258262890683122, 1.000000000000000000, 0.9659258262890683122, 1.000000000000000000, 0.9659258262890683122, 1.000000000000000000, 0.9659258262890683122, 1.000000000000000000, 0.9659258262890683122, 1.000000000000000000, 0.9659258262890683122, 1.000000000000000000, 0.9659258262890683122, 1.000000000000000000, 0.9659258262890683122, 1.000000000000000000, 0.9659258262890683122, 1.000000000000000000, 0.9659258262890683122, 1.000000000000000000, 0.9659258262890683122, 1.000000000000000000, 0.9659258262890683122, 1.000000000000000000, 0.9659258262890683122, 1.000000000000000000, 0.9659258262890683122, 1.000000000000000000, 0.9659258262890683122, 1.000000000000000000, 0.9659258262890683122, 1.000000000000000000, 0.9659258262890683122, 1.000000000000000000, 0.9659258262890683122, 1.000000000000000000, 0.9659258262890683122, 1.000000000000000000, 0.9659258262890683122, 1.000000000000000000, 0.9659258262890683122, 1.000000000000000000, 0.9659258262890683122, 1.000000000000000000, 0.9659258262890683122, 1.000000000000000000, 0.9659258262890683122, 1.000000000000000000),
 ( 1.000000000000000000, 0.9659258262890683122, 1.000000000000000000, 0.9659258262890683122, 1.000000000000000000, 0.9659258262890683122, 1.000000000000000000, 0.9659258262890683122, 1.000000000000000000, 0.9659258262890683122, 1.000000000000000000, 0.9659258262890683122, 1.000000000000000000, 0.9659258262890683122, 1.000000000000000000, 0.9659258262890683122, 1.000000000000000000, 0.9659258262890683122, 1.000000000000000000, 0.9659258262890683122, 1.000000000000000000, 0.9659258262890683122, 1.000000000000000000, 0.9659258262890683122, 1.000000000000000000, 0.9659258262890683122, 1.000000000000000000, 0.9659258262890683122, 1.000000000000000000, 0.9659258262890683122, 1.000000000000000000, 0.9659258262890683122, 1.000000000000000000, 0.9659258262890683122, 1.000000000000000000, 0.9659258262890683122, 1.000000000000000000, 0.9659258262890683122, 1.000000000000000000, 0.9659258262890683122, 1.000000000000000000, 0.9659258262890683122, 1.000000000000000000, 0.9659258262890683122, 1.000000000000000000, 0.9659258262890683122, 1.000000000000000000, 0.9659258262890683122, 1.000000000000000000, 0.9659258262890683122, 1.000000000000000000, 0.9659258262890683122, 1.000000000000000000, 0.9659258262890683122, 1.000000000000000000, 0.9659258262890683122, 1.000000000000000000, 0.9659258262890683122, 1.000000000000000000, 0.9659258262890683122, 1.000000000000000000, 0.9659258262890683122, 1.000000000000000000, 0.9659258262890683122, 1.000000000000000000, 0.9659258262890683122, 1.000000000000000000, 0.9659258262890683122, 1.000000000000000000, 0.9659258262890683122, 1.000000000000000000, 0.9659258262890683122, 1.000000000000000000, 0.9659258262890683122, 1.000000000000000000, 0.9659258262890683122, 1.000000000000000000, 0.9659258262890683122, 1.000000000000000000, 0.9659258262890683122, 1.000000000000000000, 0.9659258262890683122, 1.000000000000000000, 0.9659258262890683122, 1.000000000000000000, 0.9659258262890683122, 1.000000000000000000, 0.9659258262890683122, 1.000000000000000000, 0.9659258262890683122, 1.000000000000000000, 0.9659258262890683122, 1.000000000000000000, 0.9659258262890683122, 1.000000000000000000, 0.9659258262890683122, 1.000000000000000000, 0.9659258262890683122, 1.000000000000000000, 0.9659258262890683122, 1.000000000000000000, 0.9659258262890683122, 1.000000000000000000, 0.9659258262890683122, 1.000000000000000000, 0.9659258262890683122, 1.000000000000000000, 0.9659258262890683122, 1.000000000000000000, 0.9659258262890683122, 1.000000000000000000, 0.9659258262890683122, 1.000000000000000000, 0.9659258262890683122, 1.000000000000000000, 0.9659258262890683122, 1.000000000000000000, 0.9659258262890683122, 1.000000000000000000, 0.9659258262890683122, 1.000000000000000000, 0.9659258262890683122, 1.000000000000000000, 0.9659258262890683122, 1.000000000000000000, 0.9659258262890683122, 1.000000000000000000, 0.9659258262890683122, 1.000000000000000000, 0.9659258262890683122, 1.000000000000000000, 0.9659258262890683122, 1.000000000000000000, 0.9659258262890683122, 1.000000000000000000, 0.9659258262890683122, 1.000000000000000000, 0.9659258262890683122, 1.000000000000000000, 0.9659258262890683122, 1.000000000000000000, 0.9659258262890683122, 1.000000000000000000, 0.9659258262890683122, 1.000000000000000000, 0.9659258262890683122, 1.000000000000000000, 0.9659258262890683122, 1.000000000000000000, 0.9659258262890683122, 1.000000000000000000, 0.9659258262890683122, 1.000000000000000000, 0.9659258262890683122, 1.000000000000000000, 0.9659258262890683122, 1.000000000000000000, 0.9659258262890683122, 1.000000000000000000, 0.9659258262890683122, 1.000000000000000000, 0.9659258262890683122, 1.000000000000000000, 0.9659258262890683122, 1.000000000000000000, 0.9659258262890683122, 1.000000000000000000, 0.9659258262890683122, 1.000000000000000000, 0.9659258262890683122, 1.000000000000000000, 0.9659258262890683122, 1.000000000000000000, 0.9659258262890683122, 1.000000000000000000, 0.9659258262890683122, 1.000000000000000000, 0.9659258262890683122, 1.000000000000000000, 0.9659258262890683122, 1.000000000000000000, 0.9659258262890683122, 1.000000000000000000, 0.9659258262890683122, 1.000000000000000000, 0.9659258262890683122, 1.000000000000000000, 0.9659258262890683122, 1.000000000000000000, 0.9659258262890683122, 1.000000000000000000, 0.9659258262890683122, 1.000000000000000000, 0.9659258262890683122, 1.000000000000000000, 0.9659258262890683122, 1.000000000000000000, 0.9659258262890683122, 1.000000000000000000, 0.9659258262890683122, 1.000000000000000000, 0.9659258262890683122, 1.000000000000000000, 0.9659258262890683122, 1.000000000000000000, 0.9659258262890683122, 1.000000000000000000, 0.9659258262890683122, 1.000000000000000000, 0.9659258262890683122, 1.000000000000000000, 0.9659258262890683122, 1.000000000000000000, 0.9659258262890683122, 1.000000000000000000, 0.9659258262890683122, 1.000000000000000000, 0.9659258262890683122, 1.000000000000000000, 0.9659258262890683122, 1.000000000000000000, 0.9659258262890683122, 1.000000000000000000, 0.9659258262890683122, 1.000000000000000000, 0.9659258262890683122, 1.000000000000000000, 0.9659258262890683122, 1.000000000000000000, 0.9659258262890683122, 1.000000000000000000, 0.9659258262890683122, 1.000000000000000000, 0.9659258262890683122, 1.000000000000000000, 0.9659258262890683122, 1.000000000000000000, 0.9659258262890683122, 1.000000000000000000, 0.9659258262890683122, 1.000000000000000000, 0.9659258262890683122, 1.000000000000000000, 0.9659258262890683122, 1.000000000000000000, 0.9659258262890683122, 1.000000000000000000, 0.9659258262890683122, 1.000000000000000000, 0.9659258262890683122, 1.000000000000000000, 0.9659258262890683122, 1.000000000000000000, 0.9659258262890683122, 1.000000000000000000, 0.9659258262890683122, 1.000000000000000000, 0.9659258262890683122, 1.000000000000000000, 0.9659258262890683122, 1.000000000000000000, 0.9659258262890683122, 1.000000000000000000, 0.9659258262890683122, 1.000000000000000000, 0.9659258262890683122, 1.000000000000000000, 0.9659258262890683122, 1.000000000000000000, 0.9659258262890683122, 1.000000000000000000, 0.9659258262890683122, 1.000000000000000000, 0.9659258262890683122, 1.000000000000000000, 0.9659258262890683122, 1.000000000000000000, 0.9659258262890683122, 1.000000000000000000, 0.9659258262890683122, 1.000000000000000000, 0.9659258262890683122, 1.000000000000000000, 0.9659258262890683122, 1.000000000000000000, 0.9659258262890683122, 1.000000000000000000, 0.9659258262890683122, 1.000000000000000000, 0.9659258262890683122, 1.000000000000000000, 0.9659258262890683122, 1.000000000000000000, 0.9659258262890683122, 1.000000000000000000, 0.9659258262890683122, 1.000000000000000000, 0.9659258262890683122, 1.000000000000000000, 0.9659258262890683122, 1.000000000000000000, 0.9659258262890683122, 1.000000000000000000, 0.9659258262890683122, 1.000000000000000000, 0.9659258262890683122, 1.000000000000000000, 0.9659258262890683122, 1.000000000000000000, 0.9659258262890683122, 1.000000000000000000, 0.9659258262890683122, 1.000000000000000000, 0.9659258262890683122, 1.000000000000000000, 0.9659258262890683122, 1.000000000000000000, 0.9659258262890683122, 1.000000000000000000, 0.9659258262890683122, 1.000000000000000000, 0.9659258262890683122, 1.000000000000000000, 0.9659258262890683122, 1.000000000000000000, 0.9659258262890683122, 1.000000000000000000, 0.9659258262890683122, 1.000000000000000000, 0.9659258262890683122, 1.000000000000000000, 0.9659258262890683122, 1.000000000000000000, 0.9659258262890683122, 1.000000000000000000, 0.9659258262890683122, 1.000000000000000000, 0.9659258262890683122, 1.000000000000000000, 0.9659258262890683122, 1.000000000000000000, 0.9659258262890683122, 1.000000000000000000, 0.9659258262890683122, 1.000000000000000000, 0.9659258262890683122, 1.000000000000000000, 0.9659258262890683122, 1.000000000000000000, 0.9659258262890683122, 1.000000000000000000, 0.9659258262890683122, 1.000000000000000000, 0.9659258262890683122, 1.000000000000000000, 0.9659258262890683122, 1.000000000000000000, 0.9659258262890683122, 1.000000000000000000, 0.9659258262890683122, 1.000000000000000000, 0.9659258262890683122, 1.000000000000000000, 0.9659258262890683122, 1.000000000000000000, 0.9659258262890683122, 1.000000000000000000, 0.9659258262890683122, 1.000000000000000000, 0.9659258262890683122, 1.000000000000000000, 0.9659258262890683122, 1.000000000000000000, 0.9659258262890683122, 1.000000000000000000, 0.9659258262890683122, 1.000000000000000000, 0.9659258262890683122, 1.000000000000000000, 0.9659258262890683122, 1.000000000000000000, 0.9659258262890683122, 1.000000000000000000, 0.9659258262890683122, 1.000000000000000000, 0.9659258262890683122, 1.000000000000000000, 0.9659258262890683122, 1.000000000000000000, 0.9659258262890683122, 1.000000000000000000, 0.9659258262890683122, 1.000000000000000000, 0.9659258262890683122, 1.000000000000000000, 0.9659258262890683122, 1.000000000000000000, 0.9659258262890683122, 1.000000000000000000, 0.9659258262890683122, 1.000000000000000000, 0.9659258262890683122, 1.000000000000000000, 0.9659258262890683122, 1.000000000000000000, 0.9659258262890683122, 1.000000000000000000, 0.9659258262890683122, 1.000000000000000000, 0.9659258262890683122, 1.000000000000000000, 0.9659258262890683122, 1.000000000000000000, 0.9659258262890683122, 1.000000000000000000, 0.9659258262890683122, 1.000000000000000000, 0.9659258262890683122, 1.000000000000000000, 0.9659258262890683122, 1.000000000000000000, 0.9659258262890683122, 1.000000000000000000, 0.9659258262890683122, 1.000000000000000000, 0.9659258262890683122, 1.000000000000000000, 0.9659258262890683122, 1.000000000000000000, 0.9659258262890683122, 1.000000000000000000, 0.9659258262890683122, 1.000000000000000000, 0.9659258262890683122, 1.000000000000000000, 0.9659258262890683122, 1.000000000000000000, 0.9659258262890683122, 1.000000000000000000, 0.9659258262890683122, 1.000000000000000000, 0.9659258262890683122, 1.000000000000000000, 0.9659258262890683122, 1.000000000000000000, 0.9659258262890683122, 1.000000000000000000, 0.9659258262890683122, 1.000000000000000000, 0.9659258262890683122, 1.000000000000000000, 0.9659258262890683122, 1.000000000000000000, 0.9659258262890683122, 1.000000000000000000, 0.9659258262890683122, 1.000000000000000000, 0.9659258262890683122, 1.000000000000000000, 0.9659258262890683122, 1.000000000000000000, 0.9659258262890683122, 1.000000000000000000, 0.9659258262890683122, 1.000000000000000000, 0.9659258262890683122, 1.000000000000000000, 0.9659258262890683122, 1.000000000000000000, 0.9659258262890683122, 1.000000000000000000, 0.9659258262890683122, 1.000000000000000000, 0.9659258262890683122, 1.000000000000000000, 0.9659258262890683122, 1.000000000000000000, 0.9659258262890683122, 1.000000000000000000, 0.9659258262890683122, 1.000000000000000000, 0.9659258262890683122, 1.000000000000000000, 0.9659258262890683122, 1.000000000000000000, 0.9659258262890683122, 1.000000000000000000, 0.9659258262890683122, 1.000000000000000000, 0.9659258262890683122, 1.000000000000000000, 0.9659258262890683122, 1.000000000000000000, 0.9659258262890683122, 1.000000000000000000, 0.9659258262890683122, 1.000000000000000000, 0.9659258262890683122, 1.000000000000000000, 0.9659258262890683122, 1.000000000000000000, 0.9659258262890683122, 1.000000000000000000, 0.9659258262890683122, 1.000000000000000000, 0.9659258262890683122, 1.000000000000000000, 0.9659258262890683122, 1.000000000000000000, 0.9659258262890683122, 1.000000000000000000) ) ) 
 REPRESENTATION_ITEM ( '' )  SURFACE ( )  );
#38831=CARTESIAN_POINT ( 'NONE',  ( 0.8661417322834653598, -0.1870078740157479769, 0.4822834645669291653 ) ) ;
#38833=CARTESIAN_POINT ( 'NONE',  ( -1.699475065616797398, 0.1771653543307087630, 0.09757992244046791164 ) ) ;
#38834=CARTESIAN_POINT ( 'NONE',  ( 0.3871391076115492380, -0.08942795157528024563, -0.3641732283464568787 ) ) ;
#38835=CARTESIAN_POINT ( 'NONE',  ( 0.6889763779527566800, -0.5400638737290844871, 0.3530559997133364547 ) ) ;
#38837=CARTESIAN_POINT ( 'NONE',  ( -1.010498687664041384, -0.3690944881889765550, -0.3153832671262227771 ) ) ;
#38838=CARTESIAN_POINT ( 'NONE',  ( -0.5905511811023615998, 0.2952755905511811885, 0.000000000000000000 ) ) ;
#38839=CARTESIAN_POINT ( 'NONE',  ( -1.653543307086613234, -0.1870078740157479769, 0.3641732283464567677 ) ) ;
#38840=CARTESIAN_POINT ( 'NONE',  ( -1.227034120734907585, 0.2952755905511811885, 0.1292274648535926551 ) ) ;
#38841=CARTESIAN_POINT ( 'NONE',  ( 0.9645669291338591078, -0.5400638737290845981, -0.3530559997133363437 ) ) ;
#38842=CARTESIAN_POINT ( 'NONE',  ( -1.148293963254592542, 0.1771653543307087630, 0.09757992244046791164 ) ) ;
#38844=CARTESIAN_POINT ( 'NONE',  ( 1.194225721784777594, -0.4281496062992127816, -0.4176697321401328100 ) ) ;
#38847=CARTESIAN_POINT ( 'NONE',  ( 1.377952755905512472, 0.2952755905511811885, 0.000000000000000000 ) ) ;
#38848=CARTESIAN_POINT ( 'NONE',  ( -1.108923884514435132, -0.2845877964562159024, 0.3641732283464567677 ) ) ;
#38849=CARTESIAN_POINT ( 'NONE',  ( 1.169169330835494014, -5.140490538625777863E-17, -0.3627989612356145588 ) ) ;
#38850=CARTESIAN_POINT ( 'NONE',  ( -1.423884514435694859, -0.08942795157528024563, -0.3641732283464568787 ) ) ;
#38851=CARTESIAN_POINT ( 'NONE',  ( -0.4790026246719152336, -0.08942795157528024563, -0.3641732283464568787 ) ) ;
#38852=CARTESIAN_POINT ( 'NONE',  ( -1.587926509186350810, -0.3690944881889763329, 0.3153832671262228327 ) ) ;
#38853=CARTESIAN_POINT ( 'NONE',  ( 0.7808398950131240079, -0.2845877964562159024, 0.3641732283464567677 ) ) ;
#38854=CARTESIAN_POINT ( 'NONE',  ( 0.3608923884514443348, -0.6692913385826771977, 0.1292274648535927661 ) ) ;
#38855=CARTESIAN_POINT ( 'NONE',  ( 1.318897637795276356, 0.1660481256975883668, -0.3530559997133364547 ) ) ;
#38856=CARTESIAN_POINT ( 'NONE',  ( 0.5511811023622055217, -0.1870078740157479769, 0.4822834645669291653 ) ) ;
#38857=CARTESIAN_POINT ( 'NONE',  ( 0.3608923884514443348, 0.1771653543307087075, -0.09757992244046823083 ) ) ;
#38858=CARTESIAN_POINT ( 'NONE',  ( -1.423884514435694859, -0.05778040916215560624, -0.4822834645669293319 ) ) ;
#38859=CARTESIAN_POINT ( 'NONE',  ( -1.305774278215222184, 0.2952755905511811885, 0.1292274648535926551 ) ) ;
#38860=CARTESIAN_POINT ( 'NONE',  ( -0.6561679790026240244, -0.6046776061558807314, 0.2411417322834647770 ) ) ;
#38863=CARTESIAN_POINT ( 'NONE',  ( -0.07874015748031421014, -0.1870078740157480879, -0.4822834645669291653 ) ) ;
#38864=CARTESIAN_POINT ( 'NONE',  ( 1.122047244094488860, 0.07958543189024085140, 0.2665933059059887866 ) ) ;
#38865=CARTESIAN_POINT ( 'NONE',  ( -0.2230971128608915943, 0.05413385826771666132, 0.4176697321401328100 ) ) ;
#38866=CARTESIAN_POINT ( 'NONE',  ( 0.3608923884514443348, 0.2952755905511810774, -0.1292274648535930714 ) ) ;
#38874=ADVANCED_FACE ( 'NONE', ( #67998 ), #73903, .F. ) ;
#38875=CARTESIAN_POINT ( 'NONE',  ( -1.023622047244094002, -0.1870078740157480601, -0.3641732283464567677 ) ) ;
#38877=CARTESIAN_POINT ( 'NONE',  ( -1.174540682414697335, -0.3162353388693409650, -0.4822834645669289433 ) ) ;
#38879=CARTESIAN_POINT ( 'NONE',  ( 0.6036745406824154392, 0.2306618581243847221, -0.2411417322834647770 ) ) ;
#38880=CARTESIAN_POINT ( 'NONE',  ( 1.154855643044620184, 0.2306618581243847221, -0.2411417322834647770 ) ) ;
#38881=CARTESIAN_POINT ( 'NONE',  ( 0.8136482939632553313, 0.2306618581243848609, 0.2411417322834645549 ) ) ;
#38886=CARTESIAN_POINT ( 'NONE',  ( 0.4461942257217855201, -0.6046776061558807314, 0.2411417322834647770 ) ) ;
#38887=CARTESIAN_POINT ( 'NONE',  ( 0.3083989501312343062, -0.3162353388693405765, 0.4822834645669290543 ) ) ;
#38888=CARTESIAN_POINT ( 'NONE',  ( 0.9973753280839902091, 0.1283753931104746893, -0.1820866141732285504 ) ) ;
#38889=CARTESIAN_POINT ( 'NONE',  ( 1.161417322834646493, -0.5400638737290844871, 0.3530559997133364547 ) ) ;
#38891=CARTESIAN_POINT ( 'NONE',  ( 0.1837270341207354329, 0.2306618581243848609, 0.2411417322834645549 ) ) ;
#38892=CARTESIAN_POINT ( 'NONE',  ( 0.9317585301837276734, 0.05413385826771626580, -0.4176697321401330321 ) ) ;
#38893=CARTESIAN_POINT ( 'NONE',  ( 0.3215223097112867578, -0.3162353388693409650, -0.4822834645669289433 ) ) ;
#38894=CARTESIAN_POINT ( 'NONE',  ( 1.312335958005250269, -0.5023911411419708095, 0.1820866141732285504 ) ) ;
#38895=CARTESIAN_POINT ( 'NONE',  ( -1.095800524934382292, -0.05778040916215522460, 0.4822834645669289988 ) ) ;
#38896=CARTESIAN_POINT ( 'NONE',  ( -1.010498687664041384, -0.4281496062992127816, -0.4176697321401328100 ) ) ;
#38897=CARTESIAN_POINT ( 'NONE',  ( 1.220472440944882386, -0.6692913385826771977, 8.415575281601705876E-17 ) ) ;
#38901=ORIENTED_EDGE ( 'NONE', *, *, #65412, .T. ) ;
#38903=VERTEX_POINT ( 'NONE', #60837 ) ;
#38904=CARTESIAN_POINT ( 'NONE',  ( 1.601049868766404982, -0.6046776061558809534, -0.2411417322834644161 ) ) ;
#38905=CARTESIAN_POINT ( 'NONE',  ( 1.049868766404200127, -0.5023911411419708095, -0.1820866141732282451 ) ) ;
#38907=CARTESIAN_POINT ( 'NONE',  ( 1.174540682414699111, -0.2845877964562159024, 0.3641732283464567677 ) ) ;
#38908=CARTESIAN_POINT ( 'NONE',  ( 2.795275590551181466, 2.001539355558160871, 0.000000000000000000 ) ) ;
#38912=CARTESIAN_POINT ( 'NONE',  ( -1.076115485564303809, -0.5023911411419708095, -0.1820866141732282451 ) ) ;
#38913=CARTESIAN_POINT ( 'NONE',  ( 1.601049868766404982, 0.2306618581243848609, 0.2411417322834645549 ) ) ;
#38914=CARTESIAN_POINT ( 'NONE',  ( -1.318897637795274802, 0.1660481256975885056, 0.3530559997133364547 ) ) ;
#38915=CARTESIAN_POINT ( 'NONE',  ( 0.2362204724409456558, -0.1870078740157480879, -0.4822834645669291653 ) ) ;
#38916=CARTESIAN_POINT ( 'NONE',  ( 1.332020997375328974, -0.05778040916215560624, -0.4822834645669293319 ) ) ;
#38917=ORIENTED_EDGE ( 'NONE', *, *, #59271, .F. ) ;
#38922=CARTESIAN_POINT ( 'NONE',  ( -1.023622047244093558, -0.1870078740157479769, 0.3641732283464567677 ) ) ;
#38923=DIRECTION ( 'NONE',  ( 3.096699300667737957E-16, -1.000000000000000000, 0.000000000000000000 ) ) ;
#38924=CARTESIAN_POINT ( 'NONE',  ( 0.6824146981627303710, -0.6046776061558807314, 0.2411417322834647770 ) ) ;
#38926=CARTESIAN_POINT ( 'NONE',  ( -1.603475055217291612, 0.5037964761735302943, 0.04573490813648253134 ) ) ;
#38928=CARTESIAN_POINT ( 'NONE',  ( 1.391076115485564868, 0.2306618581243847221, -0.2411417322834647770 ) ) ;
#38929=CARTESIAN_POINT ( 'NONE',  ( -1.528871391076114250, 0.2952755905511810774, -0.1292274648535930714 ) ) ;
#38931=CARTESIAN_POINT ( 'NONE',  ( -0.2362204724409442680, -0.1870078740157480601, -0.3641732283464567677 ) ) ;
#38932=CARTESIAN_POINT ( 'NONE',  ( -1.305774278215222184, 0.1771653543307087630, 0.09757992244046791164 ) ) ;
#38934=CARTESIAN_POINT ( 'NONE',  ( -0.5183727034120726440, 0.1771653543307087630, 0.09757992244046791164 ) ) ;
#38935=CARTESIAN_POINT ( 'NONE',  ( 0.2690288713910767848, -0.5511811023622048555, -0.09757992244046775898 ) ) ;
#38936=CARTESIAN_POINT ( 'NONE',  ( 0.1246719160104994284, -0.6692913385826771977, 0.1292274648535927661 ) ) ;
#38937=CARTESIAN_POINT ( 'NONE',  ( -1.049868766404198794, -0.5023911411419708095, 0.1820866141732285504 ) ) ;
#38939=CARTESIAN_POINT ( 'NONE',  ( 0.9973753280839902091, 0.2306618581243847221, -0.2411417322834647770 ) ) ;
#38940=CARTESIAN_POINT ( 'NONE',  ( -1.240157480314959759, -0.5400638737290845981, -0.3530559997133363437 ) ) ;
#38942=CARTESIAN_POINT ( 'NONE',  ( -0.3937007874015740483, -0.1870078740157480879, -0.4822834645669291653 ) ) ;
#38943=CARTESIAN_POINT ( 'NONE',  ( -0.9120734908136475250, -0.6692913385826773087, -0.1292274648535924053 ) ) ;
#38944=CARTESIAN_POINT ( 'NONE',  ( 0.7480314960629927956, 0.1771653543307087630, 0.000000000000000000 ) ) ;
#38945=CARTESIAN_POINT ( 'NONE',  ( -0.3083989501312330295, -0.08942795157527998196, 0.3641732283464567121 ) ) ;
#38946=CARTESIAN_POINT ( 'NONE',  ( -0.4658792650918627265, -0.05778040916215522460, 0.4822834645669289988 ) ) ;
#38947=CARTESIAN_POINT ( 'NONE',  ( -1.515748031496062076, -0.5400638737290844871, 0.3530559997133364547 ) ) ;
#38948=DIRECTION ( 'NONE',  ( 0.6236670536615140925, 0.6323634944239162614, 0.4595169388576875180 ) ) ;
#38949=CARTESIAN_POINT ( 'NONE',  ( 1.476377952755906442, -0.4536011799217367080, 0.2665933059059888421 ) ) ;
#38950=CARTESIAN_POINT ( 'NONE',  ( -1.325459317585300889, 0.05413385826771666132, 0.4176697321401328100 ) ) ;
#38951=CARTESIAN_POINT ( 'NONE',  ( -1.318897637795274802, -0.5400638737290845981, -0.3530559997133363437 ) ) ;
#38952=VERTEX_POINT ( 'NONE', #48620 ) ;
#38954=CARTESIAN_POINT ( 'NONE',  ( -1.030183727034119867, -0.2845877964562159024, 0.3641732283464567677 ) ) ;
#38955=CARTESIAN_POINT ( 'NONE',  ( 0.8202099737532813073, 0.2952755905511811885, 0.1292274648535926551 ) ) ;
#38956=CARTESIAN_POINT ( 'NONE',  ( -0.8923884514435688198, 0.1283753931104746893, -0.1820866141732285504 ) ) ;
#38958=CARTESIAN_POINT ( 'NONE',  ( -0.9842519685039365918, -0.6692913385826771977, 8.415575281601705876E-17 ) ) ;
#38959=CARTESIAN_POINT ( 'NONE',  ( 0.7874015748031503170, -0.1870078740157480879, -0.4822834645669291653 ) ) ;
#38960=CARTESIAN_POINT ( 'NONE',  ( 0.6889763779527566800, -0.5400638737290844871, 0.3530559997133364547 ) ) ;
#38961=DIRECTION ( 'NONE',  ( -0.7071067811865472397, 0.000000000000000000, -0.7071067811865476838 ) ) ;
#38962=CARTESIAN_POINT ( 'NONE',  ( -1.640419947506561060, -0.3690944881889765550, -0.3153832671262227771 ) ) ;
#38968=CARTESIAN_POINT ( 'NONE',  ( 0.9908136482939640111, -0.5511811023622046335, 0.09757992244046803654 ) ) ;
#38969=CARTESIAN_POINT ( 'NONE',  ( 0.3740157480314966754, 0.07958543189024071263, -0.2665933059059888421 ) ) ;
#38970=CARTESIAN_POINT ( 'NONE',  ( 0.2887139107611556010, -0.6046776061558807314, 0.2411417322834647770 ) ) ;
#38971=CARTESIAN_POINT ( 'NONE',  ( 1.266404199475066328, -0.05778040916215522460, 0.4822834645669289988 ) ) ;
#38973=CARTESIAN_POINT ( 'NONE',  ( 0.4921259842519691285, -0.4536011799217368745, -0.2665933059059886201 ) ) ;
#38974=CARTESIAN_POINT ( 'NONE',  ( -0.6889763779527552368, 0.1660481256975885056, 0.3530559997133364547 ) ) ;
#38975=CARTESIAN_POINT ( 'NONE',  ( -1.279527559055116948, 0.1660481256975883668, -0.3530559997133364547 ) ) ;
#38976=CARTESIAN_POINT ( 'NONE',  ( 0.6430446194225729606, -0.4281496062992127816, -0.4176697321401328100 ) ) ;
#38980=VERTEX_POINT ( 'NONE', #80229 ) ;
#38981=CARTESIAN_POINT ( 'NONE',  ( -1.246719160104986512, 0.05413385826771666132, 0.4176697321401328100 ) ) ;
#38982=CARTESIAN_POINT ( 'NONE',  ( -0.6430446194225712953, 0.05413385826771626580, -0.4176697321401330321 ) ) ;
#38983=CARTESIAN_POINT ( 'NONE',  ( -0.8989501312335946848, -0.5511811023622046335, 0.09757992244046803654 ) ) ;
#38984=CARTESIAN_POINT ( 'NONE',  ( -0.9251968503937002541, -0.5400638737290845981, -0.3530559997133363437 ) ) ;
#38987=CARTESIAN_POINT ( 'NONE',  ( 1.607611548556431069, -0.6692913385826773087, -0.1292274648535924053 ) ) ;
#38988=CARTESIAN_POINT ( 'NONE',  ( -1.115485564304461219, -0.4281496062992124485, 0.4176697321401328655 ) ) ;
#38989=CARTESIAN_POINT ( 'NONE',  ( 0.1706036745406830368, 0.05413385826771666132, 0.4176697321401328100 ) ) ;
#38990=CARTESIAN_POINT ( 'NONE',  ( -0.6430446194225712953, 0.05413385826771626580, -0.4176697321401330321 ) ) ;
#38991=( BOUNDED_CURVE ( )  B_SPLINE_CURVE ( 2, ( #74335, #17917, #30530, #31341, #69662, #23798, #25022, #49877, #57007, #68020, #4036, #17100, #36024 ),
 .UNSPECIFIED., .F., .F. ) 
 B_SPLINE_CURVE_WITH_KNOTS ( ( 3, 2, 2, 2, 2, 2, 3 ),
 ( 0.4922150842069599741, 0.4924242424242424310, 0.4962121212121212155, 0.5000000000000000000, 0.5037878787878787845, 0.5075757575757575690, 0.5077849157930400814 ),
 .UNSPECIFIED. ) 
 CURVE ( )  GEOMETRIC_REPRESENTATION_ITEM ( )  RATIONAL_B_SPLINE_CURVE ( ( 0.9964447847208428577, 0.9981185001348096275, 1.000000000000000000, 0.9659258262890683122, 1.000000000000000000, 0.9659258262890683122, 1.000000000000000000, 0.9659258262890683122, 1.000000000000000000, 0.9659258262890683122, 1.000000000000000000, 0.9981185001348091834, 0.9964447847208420805 ) ) 
 REPRESENTATION_ITEM ( '' )  );
#38993=CARTESIAN_POINT ( 'NONE',  ( -0.9383202099737524282, -0.2845877964562161244, -0.3641732283464567121 ) ) ;
#38994=VERTEX_POINT ( 'NONE', #22545 ) ;
#38997=CARTESIAN_POINT ( 'NONE',  ( -1.548556430446193399, 0.1283753931104748280, 0.1820866141732283561 ) ) ;
#38998=CARTESIAN_POINT ( 'NONE',  ( -1.095800524934382292, -0.05778040916215522460, 0.4822834645669289988 ) ) ;
#38999=CARTESIAN_POINT ( 'NONE',  ( -1.364829396325458521, -0.6046776061558807314, 0.2411417322834647770 ) ) ;
#39001=CARTESIAN_POINT ( 'NONE',  ( -1.246719160104986512, 0.05413385826771666132, 0.4176697321401328100 ) ) ;
#39002=CARTESIAN_POINT ( 'NONE',  ( -1.259842519685038686, -0.1870078740157479769, 0.4822834645669291653 ) ) ;
#39003=CARTESIAN_POINT ( 'NONE',  ( -0.6986524979670485358, -2.191421614605370878E-15, 0.4445507791589071167 ) ) ;
#39004=CARTESIAN_POINT ( 'NONE',  ( -0.8005249343832011588, 0.05413385826771626580, -0.4176697321401330321 ) ) ;
#39005=CARTESIAN_POINT ( 'NONE',  ( 0.09842519685039434474, 0.07958543189024085140, 0.2665933059059887866 ) ) ;
#39008=CARTESIAN_POINT ( 'NONE',  ( -0.2690288713910754526, 0.1771653543307087075, -0.09757992244046823083 ) ) ;
#39009=CARTESIAN_POINT ( 'NONE',  ( -0.8858267716535425107, -0.5400638737290844871, 0.3530559997133364547 ) ) ;
#39010=CARTESIAN_POINT ( 'NONE',  ( 1.437007874015748810, 0.1660481256975885056, 0.3530559997133364547 ) ) ;
#39011=CARTESIAN_POINT ( 'NONE',  ( -0.3740157480314953431, 0.1660481256975885056, 0.3530559997133364547 ) ) ;
#39015=CARTESIAN_POINT ( 'NONE',  ( -1.167979002624671470, 0.05413385826771666132, 0.4176697321401328100 ) ) ;
#39016=CARTESIAN_POINT ( 'NONE',  ( 1.391076115485564868, -0.6046776061558807314, 0.2411417322834647770 ) ) ;
#39017=CARTESIAN_POINT ( 'NONE',  ( -1.515748031496062076, 0.07958543189024071263, -0.2665933059059888421 ) ) ;
#39018=CARTESIAN_POINT ( 'NONE',  ( -1.496062992125983815, -0.1870078740157480879, -0.4822834645669291653 ) ) ;
#39023=CARTESIAN_POINT ( 'NONE',  ( -0.06561679790026180015, 0.05413385826771666132, 0.4176697321401328100 ) ) ;
#39024=CARTESIAN_POINT ( 'NONE',  ( -1.535433070866141225, -0.5511811023622047445, 6.969142054262312111E-17 ) ) ;
#39025=CARTESIAN_POINT ( 'NONE',  ( -0.6758530183727028406, -0.6692913385826773087, -0.1292274648535924053 ) ) ;
#39027=CARTESIAN_POINT ( 'NONE',  ( -1.174540682414697335, -0.3162353388693409650, -0.4822834645669289433 ) ) ;
#39028=CARTESIAN_POINT ( 'NONE',  ( -0.2246346060905426156, 0.02791078216816064370, 0.4328096321851915285 ) ) ;
#39029=CARTESIAN_POINT ( 'NONE',  ( -1.017060367454067249, -0.3162353388693409650, -0.4822834645669289433 ) ) ;
#39030=CARTESIAN_POINT ( 'NONE',  ( -0.2296587926509179312, -0.3162353388693409650, -0.4822834645669289433 ) ) ;
#39032=CARTESIAN_POINT ( 'NONE',  ( 0.9842519685039375910, 0.1771653543307087630, 0.000000000000000000 ) ) ;
#39033=CARTESIAN_POINT ( 'NONE',  ( -0.7086614173228339419, -0.1870078740157480601, -0.3641732283464567677 ) ) ;
#39035=CARTESIAN_POINT ( 'NONE',  ( 0.7939632545931766261, -0.2845877964562161244, -0.3641732283464567121 ) ) ;
#39036=CARTESIAN_POINT ( 'NONE',  ( 1.332020997375328974, -0.08942795157528024563, -0.3641732283464568787 ) ) ;
#39037=CARTESIAN_POINT ( 'NONE',  ( 1.522309711286089939, -0.6046776061558809534, -0.2411417322834644161 ) ) ;
#39038=CARTESIAN_POINT ( 'NONE',  ( 0.2624671916010504757, 0.1283753931104748280, 0.1820866141732283561 ) ) ;
#39040=CARTESIAN_POINT ( 'NONE',  ( -0.8727034120734901146, -0.3162353388693405765, 0.4822834645669290543 ) ) ;
#39041=CARTESIAN_POINT ( 'NONE',  ( 1.397637795275591177, -0.5400638737290844871, 0.3530559997133364547 ) ) ;
#39042=B_SPLINE_CURVE_WITH_KNOTS ( 'NONE', 3,
 ( #2786, #59598, #21716, #1953 ),
 .UNSPECIFIED., .F., .F.,
 ( 4, 4 ),
 ( 1.999999999897049408E-07, 0.006970199999999935128 ),
 .UNSPECIFIED. ) ;
#39044=CARTESIAN_POINT ( 'NONE',  ( -0.4461942257217840213, -0.5023911411419708095, -0.1820866141732282451 ) ) ;
#39045=CARTESIAN_POINT ( 'NONE',  ( 0.06561679790026316017, 0.05413385826771626580, -0.4176697321401330321 ) ) ;
#39046=CARTESIAN_POINT ( 'NONE',  ( 0.3608923884514443348, -0.6692913385826771977, 0.1292274648535927661 ) ) ;
#39047=FACE_OUTER_BOUND ( 'NONE', #63519, .T. ) ;
#39048=CARTESIAN_POINT ( 'NONE',  ( 0.9055118110236227702, -0.5511811023622047445, 6.969142054262312111E-17 ) ) ;
#39049=CARTESIAN_POINT ( 'NONE',  ( 0.2755905511811031494, -0.5511811023622047445, 6.969142054262312111E-17 ) ) ;
#39050=CARTESIAN_POINT ( 'NONE',  ( -0.1968503937007867743, 0.2952755905511811885, 0.000000000000000000 ) ) ;
#39051=CARTESIAN_POINT ( 'NONE',  ( -1.515748031496062076, 0.1660481256975883668, -0.3530559997133364547 ) ) ;
#39052=CARTESIAN_POINT ( 'NONE',  ( -0.8398950131233585692, 0.1283753931104748280, 0.1820866141732283561 ) ) ;
#39053=DIRECTION ( 'NONE',  ( 1.000000000000000000, -0.000000000000000000, -0.000000000000000000 ) ) ;
#39054=AXIS2_PLACEMENT_3D ( 'NONE', #65547, #305, #59204 ) ;
#39055=CARTESIAN_POINT ( 'NONE',  ( -0.8464566929133852113, 0.1660481256975885056, 0.3530559997133364547 ) ) ;
#39059=CARTESIAN_POINT ( 'NONE',  ( 5.463695987328526437E-16, -0.1870078740157479769, 0.3641732283464567677 ) ) ;
#39060=CARTESIAN_POINT ( 'NONE',  ( -0.8595800524934373854, -0.05778040916215522460, 0.4822834645669289988 ) ) ;
#39061=CARTESIAN_POINT ( 'NONE',  ( -1.246719160104985846, -0.4281496062992127816, -0.4176697321401328100 ) ) ;
#39062=CARTESIAN_POINT ( 'NONE',  ( -1.089238845144356427, -0.3690944881889765550, -0.3153832671262227771 ) ) ;
#39064=CARTESIAN_POINT ( 'NONE',  ( -1.017060367454067249, -0.08942795157527998196, 0.3641732283464567121 ) ) ;
#39065=CARTESIAN_POINT ( 'NONE',  ( -1.535433070866141225, 0.1771653543307087630, 0.000000000000000000 ) ) ;
#39066=CARTESIAN_POINT ( 'NONE',  ( 1.194225721784777594, -0.4281496062992127816, -0.4176697321401328100 ) ) ;
#39068=ADVANCED_FACE ( 'NONE', ( #35588 ), #16244, .F. ) ;
#39073=CARTESIAN_POINT ( 'NONE',  ( -1.732283464566928277, -0.1870078740157479769, 0.4822834645669291653 ) ) ;
#39074=CARTESIAN_POINT ( 'NONE',  ( -1.476377952755905110, -0.5400638737290845981, -0.3530559997133363437 ) ) ;
#39075=CARTESIAN_POINT ( 'NONE',  ( 1.154855643044620184, 0.2306618581243847221, -0.2411417322834647770 ) ) ;
#39078=CARTESIAN_POINT ( 'NONE',  ( 0.4133858267716541968, 0.1660481256975885056, 0.3530559997133364547 ) ) ;
#39079=CARTESIAN_POINT ( 'NONE',  ( -0.1706036745406816491, 0.05413385826771626580, -0.4176697321401330321 ) ) ;
#39080=CARTESIAN_POINT ( 'NONE',  ( -0.3273801728231969244, -2.609869883881465018E-15, -0.3464511005275220379 ) ) ;
#39081=CARTESIAN_POINT ( 'NONE',  ( -0.6399301791983041943, -2.567464376874931580E-15, -0.4445507791589072832 ) ) ;
#39082=CARTESIAN_POINT ( 'NONE',  ( 0.9317585301837276734, -0.3690944881889763329, 0.3153832671262228327 ) ) ;
#39084=VERTEX_POINT ( 'NONE', #55343 ) ;
#39086=ORIENTED_EDGE ( 'NONE', *, *, #27581, .T. ) ;
#39087=CARTESIAN_POINT ( 'NONE',  ( 0.09186351706036799403, -0.4281496062992127816, -0.4176697321401328100 ) ) ;
#39088=CARTESIAN_POINT ( 'NONE',  ( -1.653543307086613234, -0.1870078740157479769, 0.4822834645669291653 ) ) ;
#39089=CARTESIAN_POINT ( 'NONE',  ( 0.7677165354330716118, 0.1660481256975883668, -0.3530559997133364547 ) ) ;
#39090=CARTESIAN_POINT ( 'NONE',  ( 1.010498687664042716, -0.4281496062992124485, 0.4176697321401328655 ) ) ;
#39091=CARTESIAN_POINT ( 'NONE',  ( 1.220472440944882386, -0.6692913385826771977, 8.415575281601705876E-17 ) ) ;
#39092=CARTESIAN_POINT ( 'NONE',  ( -0.6692913385826764205, 0.2952755905511811885, 0.000000000000000000 ) ) ;
#39093=CARTESIAN_POINT ( 'NONE',  ( -0.02624671916010428221, -0.6046776061558807314, 0.2411417322834647770 ) ) ;
#39094=CARTESIAN_POINT ( 'NONE',  ( 1.404199475065617264, -0.4281496062992124485, 0.4176697321401328655 ) ) ;
#39095=CARTESIAN_POINT ( 'NONE',  ( 1.430446194225722500, 0.05413385826771666132, 0.4176697321401328100 ) ) ;
#39096=CARTESIAN_POINT ( 'NONE',  ( 1.174540682414699111, -0.3162353388693405765, 0.4822834645669290543 ) ) ;
#39097=CARTESIAN_POINT ( 'NONE',  ( -0.3215223097112853146, -0.3162353388693405765, 0.4822834645669290543 ) ) ;
#39099=CARTESIAN_POINT ( 'NONE',  ( 0.2493438320209980519, -0.004921259842519576551, 0.3153832671262227771 ) ) ;
#39100=ORIENTED_EDGE ( 'NONE', *, *, #76855, .T. ) ;
#39103=CARTESIAN_POINT ( 'NONE',  ( -0.6496062992125976043, -0.4536011799217367080, 0.2665933059059888421 ) ) ;
#39104=DIRECTION ( 'NONE',  ( -1.692413147294446216E-16, 0.000000000000000000, -1.000000000000000000 ) ) ;
#39105=CARTESIAN_POINT ( 'NONE',  ( 0.06561679790026316017, 0.05413385826771626580, -0.4176697321401330321 ) ) ;
#39106=CARTESIAN_POINT ( 'NONE',  ( -0.1312335958005241554, 0.2306618581243848609, 0.2411417322834645549 ) ) ;
#39107=CARTESIAN_POINT ( 'NONE',  ( -1.036745406824146176, 0.05413385826771626580, -0.4176697321401330321 ) ) ;
#39109=CARTESIAN_POINT ( 'NONE',  ( -1.423884514435694859, -0.05778040916215560624, -0.4822834645669293319 ) ) ;
#39111=CARTESIAN_POINT ( 'NONE',  ( 0.8005249343832027131, -0.004921259842519576551, 0.3153832671262227771 ) ) ;
#39112=CARTESIAN_POINT ( 'NONE',  ( 0.3412073490813655186, -0.6046776061558809534, -0.2411417322834644161 ) ) ;
#39113=CARTESIAN_POINT ( 'NONE',  ( 0.9120734908136490793, 0.2952755905511810774, -0.1292274648535930714 ) ) ;
#39114=AXIS2_PLACEMENT_3D ( 'NONE', #41569, #49113, #35260 ) ;
#39119=CARTESIAN_POINT ( 'NONE',  ( 0.01312335958005323398, 0.05413385826771666132, 0.4176697321401328100 ) ) ;
#39122=CARTESIAN_POINT ( 'NONE',  ( -1.141732283464566011, 0.1771653543307087630, 0.000000000000000000 ) ) ;
#39123=CARTESIAN_POINT ( 'NONE',  ( 1.154855643044620184, 0.2306618581243847221, -0.2411417322834647770 ) ) ;
#39124=CARTESIAN_POINT ( 'NONE',  ( 1.207349081364829990, 0.2306618581243848609, 0.2411417322834645549 ) ) ;
#39125=CARTESIAN_POINT ( 'NONE',  ( 0.2230971128608932319, -0.3690944881889763329, 0.3153832671262228327 ) ) ;
#39126=CARTESIAN_POINT ( 'NONE',  ( 0.4658792650918640033, -0.3162353388693405765, 0.4822834645669290543 ) ) ;
#39128=CARTESIAN_POINT ( 'NONE',  ( 0.2952755905511819101, 0.07958543189024071263, -0.2665933059059888421 ) ) ;
#39129=CARTESIAN_POINT ( 'NONE',  ( -0.1312335958005241554, 0.2306618581243848609, 0.2411417322834645549 ) ) ;
#39131=CARTESIAN_POINT ( 'NONE',  ( -1.417322834645668772, -0.1870078740157479769, 0.4822834645669291653 ) ) ;
#39132=CARTESIAN_POINT ( 'NONE',  ( 0.3871391076115492380, -0.08942795157528024563, -0.3641732283464568787 ) ) ;
#39135=CARTESIAN_POINT ( 'NONE',  ( -0.6824146981627291497, -0.6046776061558809534, -0.2411417322834644161 ) ) ;
#39136=CARTESIAN_POINT ( 'NONE',  ( -0.4199475065616791736, -0.5023911411419708095, 0.1820866141732285504 ) ) ;
#39137=CARTESIAN_POINT ( 'NONE',  ( -0.9317585301837263412, 0.05413385826771666132, 0.4176697321401328100 ) ) ;
#39138=CARTESIAN_POINT ( 'NONE',  ( -0.1706036745406816491, 0.05413385826771626580, -0.4176697321401330321 ) ) ;
#39139=CARTESIAN_POINT ( 'NONE',  ( 0.2493438320209980519, -0.3690944881889765550, -0.3153832671262227771 ) ) ;
#39141=CARTESIAN_POINT ( 'NONE',  ( 0.006561679790026889343, -0.3162353388693409650, -0.4822834645669289433 ) ) ;
#39143=CARTESIAN_POINT ( 'NONE',  ( 0.6824146981627303710, -0.5023911411419708095, 0.1820866141732285504 ) ) ;
#39144=CARTESIAN_POINT ( 'NONE',  ( 1.502624671916010790, -0.3162353388693409650, -0.4822834645669289433 ) ) ;
#39145=CARTESIAN_POINT ( 'NONE',  ( -0.7611548556430438595, 0.1283753931104748280, 0.1820866141732283561 ) ) ;
#39146=CARTESIAN_POINT ( 'NONE',  ( -1.345144356955379816, -0.08942795157528024563, -0.3641732283464568787 ) ) ;
#39147=CARTESIAN_POINT ( 'NONE',  ( -0.7152230971128602510, -0.3162353388693405765, 0.4822834645669290543 ) ) ;
#39148=CARTESIAN_POINT ( 'NONE',  ( -0.05905511811023545637, -0.5400638737290845981, -0.3530559997133363437 ) ) ;
#39149=CARTESIAN_POINT ( 'NONE',  ( 0.5511811023622055217, -0.1870078740157479769, 0.3641732283464567677 ) ) ;
#39151=CARTESIAN_POINT ( 'NONE',  ( 1.010498687664042716, -0.004921259842519870586, -0.3153832671262229437 ) ) ;
#39152=CARTESIAN_POINT ( 'NONE',  ( 0.2493438320209980519, 0.05413385826771666132, 0.4176697321401328100 ) ) ;
#39154=CARTESIAN_POINT ( 'NONE',  ( -0.2099737532808391705, -0.6046776061558809534, -0.2411417322834644161 ) ) ;
#39156=CARTESIAN_POINT ( 'NONE',  ( 1.509186351706037543, -0.3690944881889765550, -0.3153832671262227771 ) ) ;
#39157=CARTESIAN_POINT ( 'NONE',  ( 0.4265091863517067594, 0.2952755905511811885, 0.1292274648535926551 ) ) ;
#39158=CARTESIAN_POINT ( 'NONE',  ( 0.03937007874015833325, -0.6692913385826771977, 8.415575281601705876E-17 ) ) ;
#39159=CARTESIAN_POINT ( 'NONE',  ( 0.6167979002624679463, 0.009842519685039147898, -0.3409548833797004797 ) ) ;
#39160=CARTESIAN_POINT ( 'NONE',  ( 0.1049868766404206816, 0.1283753931104748280, 0.1820866141732283561 ) ) ;
#39161=CARTESIAN_POINT ( 'NONE',  ( 0.6299212598425204535, -0.1870078740157480879, -0.4822834645669291653 ) ) ;
#39162=CARTESIAN_POINT ( 'NONE',  ( -0.4265091863517051496, 0.1771653543307087075, -0.09757992244046823083 ) ) ;
#39163=CARTESIAN_POINT ( 'NONE',  ( -0.7086614173228339419, -0.1870078740157479769, 0.4822834645669291653 ) ) ;
#39165=CARTESIAN_POINT ( 'NONE',  ( -0.3083989501312330295, -0.05778040916215522460, 0.4822834645669289988 ) ) ;
#39166=VERTEX_POINT ( 'NONE', #73489 ) ;
#39167=CARTESIAN_POINT ( 'NONE',  ( -1.115485564304461219, 0.05413385826771626580, -0.4176697321401330321 ) ) ;
#39168=CARTESIAN_POINT ( 'NONE',  ( -0.6561679790026240244, -0.5023911411419708095, 0.1820866141732285504 ) ) ;
#39169=VECTOR ( 'NONE', #6829, 39.37007874015748143 ) ;
#39170=CARTESIAN_POINT ( 'NONE',  ( 0.1312335958005255154, -0.6046776061558807314, 0.2411417322834647770 ) ) ;
#39171=CARTESIAN_POINT ( 'NONE',  ( -1.076115485564303809, 0.2306618581243848609, 0.2411417322834645549 ) ) ;
#39172=CARTESIAN_POINT ( 'NONE',  ( -0.9120734908136475250, -0.6692913385826773087, -0.1292274648535924053 ) ) ;
#39173=FACE_OUTER_BOUND ( 'NONE', #734, .T. ) ;
#39175=CARTESIAN_POINT ( 'NONE',  ( 1.423884514435696191, -0.05778040916215522460, 0.4822834645669289988 ) ) ;
#39176=CARTESIAN_POINT ( 'NONE',  ( 1.161417322834646493, -0.5400638737290844871, 0.3530559997133364547 ) ) ;
#39178=CARTESIAN_POINT ( 'NONE',  ( 2.795275590551181466, 2.244094488188977277, 0.000000000000000000 ) ) ;
#39179=CARTESIAN_POINT ( 'NONE',  ( -1.489501312335957062, -0.3162353388693409650, -0.4822834645669289433 ) ) ;
#39183=CARTESIAN_POINT ( 'NONE',  ( -0.02624671916010428221, 0.1283753931104746893, -0.1820866141732285504 ) ) ;
#39186=CARTESIAN_POINT ( 'NONE',  ( 0.3018372703412079971, -0.4281496062992124485, 0.4176697321401328655 ) ) ;
#39187=CARTESIAN_POINT ( 'NONE',  ( 0.3412073490813655186, 0.2306618581243848609, 0.2411417322834645549 ) ) ;
#39188=CARTESIAN_POINT ( 'NONE',  ( -1.614173228346456712, 2.401574803149606474, -0.1372047244094478091 ) ) ;
#39189=FACE_OUTER_BOUND ( 'NONE', #18994, .T. ) ;
#39190=CARTESIAN_POINT ( 'NONE',  ( -0.9580052493438311334, -0.004921259842519870586, -0.3153832671262229437 ) ) ;
#39192=CARTESIAN_POINT ( 'NONE',  ( 0.6889763779527566800, -0.5400638737290844871, 0.3530559997133364547 ) ) ;
#39193=EDGE_CURVE ( 'NONE', #21404, #14171, #42031, .T. ) ;
#39194=CARTESIAN_POINT ( 'NONE',  ( 0.9842519685039375910, 0.1771653543307087630, 0.000000000000000000 ) ) ;
#39195=CARTESIAN_POINT ( 'NONE',  ( -0.2755905511811015396, -0.6692913385826771977, 8.415575281601705876E-17 ) ) ;
#39197=CARTESIAN_POINT ( 'NONE',  ( -0.8661417322834640276, -0.1870078740157479769, 0.4822834645669291653 ) ) ;
#39199=CARTESIAN_POINT ( 'NONE',  ( -0.8464566929133852113, -0.5400638737290845981, -0.3530559997133363437 ) ) ;
#39200=CARTESIAN_POINT ( 'NONE',  ( 1.332020997375329197, -0.3162353388693405765, 0.4822834645669290543 ) ) ;
#39201=CARTESIAN_POINT ( 'NONE',  ( 1.607611548556431069, -0.5511811023622048555, -0.09757992244046775898 ) ) ;
#39202=EDGE_LOOP ( 'NONE', ( #53378, #45526, #38095, #28854 ) ) ;
#39204=CARTESIAN_POINT ( 'NONE',  ( -0.08530183727034056085, -0.3162353388693405765, 0.4822834645669290543 ) ) ;
#39206=CARTESIAN_POINT ( 'NONE',  ( -0.7217847769028863381, 0.05413385826771626580, -0.4176697321401330321 ) ) ;
#39207=CARTESIAN_POINT ( 'NONE',  ( 1.430446194225722500, 0.05413385826771666132, 0.4176697321401328100 ) ) ;
#39208=CARTESIAN_POINT ( 'NONE',  ( 1.141732283464567566, 0.2952755905511811885, 0.000000000000000000 ) ) ;
#39209=CARTESIAN_POINT ( 'NONE',  ( 0.3346456692913390985, 0.1660481256975885056, 0.3530559997133364547 ) ) ;
#39210=CARTESIAN_POINT ( 'NONE',  ( 0.2230971128608932319, -0.4281496062992124485, 0.4176697321401328655 ) ) ;
#39212=CARTESIAN_POINT ( 'NONE',  ( -1.338582677165353729, -0.1870078740157480879, -0.4822834645669291653 ) ) ;
#39213=CARTESIAN_POINT ( 'NONE',  ( -0.3937007874015740483, -0.1870078740157479769, 0.4822834645669291653 ) ) ;
#39214=CARTESIAN_POINT ( 'NONE',  ( -0.2493438320209966919, -0.3690944881889763329, 0.3153832671262228327 ) ) ;
#39215=CARTESIAN_POINT ( 'NONE',  ( 1.607611548556431069, -0.6692913385826773087, -0.1292274648535924053 ) ) ;
#39216=CARTESIAN_POINT ( 'NONE',  ( 1.345144356955381593, -0.05778040916215522460, 0.4822834645669289988 ) ) ;
#39217=CARTESIAN_POINT ( 'NONE',  ( -0.4527559055118102749, 0.1660481256975885056, 0.3530559997133364547 ) ) ;
#39218=DIRECTION ( 'NONE',  ( -1.000000000000000000, 0.000000000000000000, 0.000000000000000000 ) ) ;
#39219=CARTESIAN_POINT ( 'NONE',  ( 1.003937007874016185, 0.1660481256975883668, -0.3530559997133364547 ) ) ;
#39224=CARTESIAN_POINT ( 'NONE',  ( 0.1509186351706045259, -0.05778040916215560624, -0.4822834645669293319 ) ) ;
#39225=CARTESIAN_POINT ( 'NONE',  ( -0.2165354330708654795, -0.4536011799217368745, -0.2665933059059886201 ) ) ;
#39226=CARTESIAN_POINT ( 'NONE',  ( 1.351706036745407680, -0.004921259842519576551, 0.3153832671262227771 ) ) ;
#39227=CARTESIAN_POINT ( 'NONE',  ( 1.603475055217291612, 0.5037964761735347352, 0.04573490813648269093 ) ) ;
#39229=CARTESIAN_POINT ( 'NONE',  ( 1.528871391076116026, 0.1771653543307087630, 0.09757992244046791164 ) ) ;
#39230=CARTESIAN_POINT ( 'NONE',  ( 1.154855643044620184, 0.2306618581243847221, -0.2411417322834647770 ) ) ;
#39232=CARTESIAN_POINT ( 'NONE',  ( 0.1049868766404206816, -0.6046776061558809534, -0.2411417322834644161 ) ) ;
#39233=CARTESIAN_POINT ( 'NONE',  ( -1.522309711286088607, -0.6046776061558807314, 0.2411417322834647770 ) ) ;
#39234=CARTESIAN_POINT ( 'NONE',  ( -1.725721784776902190, -0.05778040916215522460, 0.4822834645669289988 ) ) ;
#39235=CARTESIAN_POINT ( 'NONE',  ( -0.2427821522309703550, -0.05778040916215560624, -0.4822834645669293319 ) ) ;
#39237=CARTESIAN_POINT ( 'NONE',  ( -1.640419947506561060, -0.004921259842519576551, 0.3153832671262227771 ) ) ;
#39238=CARTESIAN_POINT ( 'NONE',  ( 0.4986876640419954376, 0.2306618581243848609, 0.2411417322834645549 ) ) ;
#39240=CARTESIAN_POINT ( 'NONE',  ( 0.9645669291338591078, -0.4536011799217368745, -0.2665933059059886201 ) ) ;
#39242=ADVANCED_FACE ( 'NONE', ( #36822 ), #41487, .F. ) ;
#39243=CARTESIAN_POINT ( 'NONE',  ( 0.7020997375328090762, -0.2845877964562159024, 0.3641732283464567677 ) ) ;
#39244=CARTESIAN_POINT ( 'NONE',  ( -1.207349081364828436, -0.6046776061558807314, 0.2411417322834647770 ) ) ;
#39246=CARTESIAN_POINT ( 'NONE',  ( 1.102362204724410155, -0.1870078740157480879, -0.4822834645669291653 ) ) ;
#39248=CARTESIAN_POINT ( 'NONE',  ( 0.7545931758530189937, 0.2952755905511810774, -0.1292274648535930714 ) ) ;
#39250=CARTESIAN_POINT ( 'NONE',  ( -0.3805774278215216522, 0.009842519685039467087, 0.3409548833797002021 ) ) ;
#39251=CARTESIAN_POINT ( 'NONE',  ( 0.5511811023622054106, -0.1870078740157480601, -0.3641732283464567677 ) ) ;
#39252=CARTESIAN_POINT ( 'NONE',  ( 0.7349081364829403995, 0.2306618581243848609, 0.2411417322834645549 ) ) ;
#39254=CARTESIAN_POINT ( 'NONE',  ( -1.128608923884513837, -0.5023911411419708095, 0.1820866141732285504 ) ) ;
#39255=CARTESIAN_POINT ( 'NONE',  ( -0.9383202099737524282, -0.05778040916215522460, 0.4822834645669289988 ) ) ;
#39256=CARTESIAN_POINT ( 'NONE',  ( 0.9580052493438327987, -0.4281496062992127816, -0.4176697321401328100 ) ) ;
#39257=CARTESIAN_POINT ( 'NONE',  ( -0.9383202099737524282, -0.05778040916215522460, 0.4822834645669289988 ) ) ;
#39258=CARTESIAN_POINT ( 'NONE',  ( 0.9908136482939640111, -0.6692913385826771977, 0.1292274648535927661 ) ) ;
#39259=CARTESIAN_POINT ( 'NONE',  ( -1.443569553805773564, 0.1283753931104746893, -0.1820866141732285504 ) ) ;
#39261=CARTESIAN_POINT ( 'NONE',  ( 0.9776902887139113929, 0.2952755905511811885, 0.1292274648535926551 ) ) ;
#39264=CARTESIAN_POINT ( 'NONE',  ( 1.194225721784777594, 0.05413385826771666132, 0.4176697321401328100 ) ) ;
#39265=CARTESIAN_POINT ( 'NONE',  ( -1.627296587926508442, -0.5023911411419708095, -0.1820866141732282451 ) ) ;
#39266=CARTESIAN_POINT ( 'NONE',  ( 1.168682819302787168, 2.409604939980833412E-17, -0.3464511005275205946 ) ) ;
#39267=CARTESIAN_POINT ( 'NONE',  ( -1.272965879265091305, -0.004921259842519870586, -0.3153832671262229437 ) ) ;
#39268=CARTESIAN_POINT ( 'NONE',  ( -0.5577427821522301654, -0.2845877964562159024, 0.3641732283464567677 ) ) ;
#39269=CARTESIAN_POINT ( 'NONE',  ( -1.397637795275589623, 0.07958543189024085140, 0.2665933059059887866 ) ) ;
#39270=CARTESIAN_POINT ( 'NONE',  ( 0.8727034120734912248, -0.2845877964562161244, -0.3641732283464567121 ) ) ;
#39271=CARTESIAN_POINT ( 'NONE',  ( 0.5839895013123367340, 0.2952755905511811885, 0.1292274648535926551 ) ) ;
#39272=CARTESIAN_POINT ( 'NONE',  ( 1.200787401574803681, -0.5400638737290845981, -0.3530559997133363437 ) ) ;
#39273=CARTESIAN_POINT ( 'NONE',  ( -0.05905511811023545637, 0.1660481256975885056, 0.3530559997133364547 ) ) ;
#39274=CARTESIAN_POINT ( 'NONE',  ( 0.5380577427821529035, -0.004921259842519870586, -0.3153832671262229437 ) ) ;
#39275=CARTESIAN_POINT ( 'NONE',  ( 1.555118110236221041, -0.5400638737290844871, 0.3530559997133364547 ) ) ;
#39277=CARTESIAN_POINT ( 'NONE',  ( -0.5708661417322828946, 0.1660481256975883668, -0.3530559997133364547 ) ) ;
#39280=CARTESIAN_POINT ( 'NONE',  ( 0.1312335958005255154, -0.6046776061558807314, 0.2411417322834647770 ) ) ;
#39281=CARTESIAN_POINT ( 'NONE',  ( -0.5774278215223089816, -0.6046776061558807314, 0.2411417322834647770 ) ) ;
#39282=CARTESIAN_POINT ( 'NONE',  ( 0.06561679790026316017, 0.05413385826771626580, -0.4176697321401330321 ) ) ;
#39286=CARTESIAN_POINT ( 'NONE',  ( 1.363814626685859954, 0.1354692512615922884, 0.3875633260700433458 ) ) ;
#39289=CARTESIAN_POINT ( 'NONE',  ( -0.7874015748031489847, -0.1870078740157479769, 0.3641732283464567677 ) ) ;
#39291=CARTESIAN_POINT ( 'NONE',  ( -1.253280839895012377, -0.05778040916215522460, 0.4822834645669289988 ) ) ;
#39292=CONICAL_SURFACE ( 'NONE', #54071, 1.181102362204724310, 0.7853981633974621568 ) ;
#39294=CARTESIAN_POINT ( 'NONE',  ( 0.5249343832021005074, -0.6046776061558807314, 0.2411417322834647770 ) ) ;
#39295=CARTESIAN_POINT ( 'NONE',  ( -0.05905511811023545637, -0.4536011799217368745, -0.2665933059059886201 ) ) ;
#39296=CARTESIAN_POINT ( 'NONE',  ( 1.476377952755906220, 0.1660481256975883668, -0.3530559997133364547 ) ) ;
#39297=CARTESIAN_POINT ( 'NONE',  ( 0.2427821522309716595, -0.3162353388693409650, -0.4822834645669289433 ) ) ;
#39301=CARTESIAN_POINT ( 'NONE',  ( 1.089238845144357759, 0.05413385826771626580, -0.4176697321401330321 ) ) ;
#39302=CARTESIAN_POINT ( 'NONE',  ( 0.3280839895013130669, 0.05413385826771666132, 0.4176697321401328100 ) ) ;
#39303=CARTESIAN_POINT ( 'NONE',  ( 0.1443569553805781891, -0.4281496062992124485, 0.4176697321401328655 ) ) ;
#39304=CARTESIAN_POINT ( 'NONE',  ( 1.456692913385827515, -0.6692913385826771977, 8.415575281601705876E-17 ) ) ;
#39306=CARTESIAN_POINT ( 'NONE',  ( -0.06561679790026180015, -0.4281496062992127816, -0.4176697321401328100 ) ) ;
#39307=CARTESIAN_POINT ( 'NONE',  ( 1.272965879265092637, -0.4281496062992127816, -0.4176697321401328100 ) ) ;
#39308=CARTESIAN_POINT ( 'NONE',  ( 0.5118110236220480003, -0.6692913385826771977, 8.415575281601705876E-17 ) ) ;
#39309=CARTESIAN_POINT ( 'NONE',  ( 0.9973753280839902091, -0.5023911411419708095, 0.1820866141732285504 ) ) ;
#39310=CARTESIAN_POINT ( 'NONE',  ( -0.8923884514435688198, 0.2306618581243847221, -0.2411417322834647770 ) ) ;
#39311=CARTESIAN_POINT ( 'NONE',  ( -1.364829396325458521, 0.2306618581243847221, -0.2411417322834647770 ) ) ;
#39312=CARTESIAN_POINT ( 'NONE',  ( 0.9186351706036751663, -0.6046776061558807314, 0.2411417322834647770 ) ) ;
#39315=( BOUNDED_CURVE ( )  B_SPLINE_CURVE ( 2, ( #8808, #47092, #72782, #15132, #40788, #34484, #28161, #60562, #2913, #23495, #49161, #25135, #11295 ),
 .UNSPECIFIED., .F., .F. ) 
 B_SPLINE_CURVE_WITH_KNOTS ( ( 3, 2, 2, 2, 2, 2, 3 ),
 ( 0.3217605387524145044, 0.3219696969696970168, 0.3257575757575758013, 0.3295454545454545858, 0.3333333333333333703, 0.3371212121212121549, 0.3373303703384946672 ),
 .UNSPECIFIED. ) 
 CURVE ( )  GEOMETRIC_REPRESENTATION_ITEM ( )  RATIONAL_B_SPLINE_CURVE ( ( 0.9964447847208419695, 0.9981185001348091834, 1.000000000000000000, 0.9659258262890683122, 1.000000000000000000, 0.9659258262890683122, 1.000000000000000000, 0.9659258262890683122, 1.000000000000000000, 0.9659258262890683122, 1.000000000000000000, 0.9981185001348091834, 0.9964447847208420805 ) ) 
 REPRESENTATION_ITEM ( '' )  );
#39316=CARTESIAN_POINT ( 'NONE',  ( 1.574803149606299746, -0.1870078740157480879, -0.4822834645669291653 ) ) ;
#39317=ORIENTED_EDGE ( 'NONE', *, *, #5285, .F. ) ;
#39320=CARTESIAN_POINT ( 'NONE',  ( 1.555118110236221041, 0.1660481256975883668, -0.3530559997133364547 ) ) ;
#39321=CARTESIAN_POINT ( 'NONE',  ( 0.9120734908136489683, -0.5511811023622046335, 0.09757992244046803654 ) ) ;
#39323=CARTESIAN_POINT ( 'NONE',  ( -0.1458944486102277671, 0.02791078216816064370, 0.4328096321851915285 ) ) ;
#39324=CARTESIAN_POINT ( 'NONE',  ( 2.795275590551181466, 2.204724409448820310, 0.000000000000000000 ) ) ;
#39326=CARTESIAN_POINT ( 'NONE',  ( -1.082677165354329896, -0.4536011799217368745, -0.2665933059059886201 ) ) ;
#39327=CARTESIAN_POINT ( 'NONE',  ( -1.725721784776902190, -0.08942795157527998196, 0.3641732283464567121 ) ) ;
#39329=CARTESIAN_POINT ( 'NONE',  ( -0.2690288713910754526, 0.2952755905511810774, -0.1292274648535930714 ) ) ;
#39330=CARTESIAN_POINT ( 'NONE',  ( -1.568241469816272105, -0.3162353388693409650, -0.4822834645669289433 ) ) ;
#39332=CARTESIAN_POINT ( 'NONE',  ( -1.391076115485563758, 0.2306618581243848609, 0.2411417322834645549 ) ) ;
#39334=CARTESIAN_POINT ( 'NONE',  ( -0.3273801728231969244, -2.609869883881465018E-15, -0.3464511005275220379 ) ) ;
#39335=CARTESIAN_POINT ( 'NONE',  ( -0.3046215029598641766, -4.378520898609941727E-15, 0.4281989832122466977 ) ) ;
#39336=CARTESIAN_POINT ( 'NONE',  ( -0.7086614173228339419, -0.1870078740157479769, 0.3641732283464567677 ) ) ;
#39337=CARTESIAN_POINT ( 'NONE',  ( -1.627296587926508442, 0.2306618581243848609, 0.2411417322834645549 ) ) ;
#39338=CARTESIAN_POINT ( 'NONE',  ( 0.5118110236220480003, -0.6692913385826771977, 8.415575281601705876E-17 ) ) ;
#39341=CARTESIAN_POINT ( 'NONE',  ( 0.7998211177050879028, 0.000000000000000000, 0.3464511005275205946 ) ) ;
#39343=CARTESIAN_POINT ( 'NONE',  ( 1.404199475065617708, 0.05413385826771626580, -0.4176697321401330321 ) ) ;
#39344=CARTESIAN_POINT ( 'NONE',  ( 1.614173228346457378, 0.1771653543307087630, 0.000000000000000000 ) ) ;
#39347=CARTESIAN_POINT ( 'NONE',  ( -0.4527559055118102749, 0.07958543189024085140, 0.2665933059059887866 ) ) ;
#39348=CARTESIAN_POINT ( 'NONE',  ( -1.456692913385826182, 0.1771653543307087630, 0.000000000000000000 ) ) ;
#39350=CARTESIAN_POINT ( 'NONE',  ( 0.3018372703412079971, -0.4281496062992124485, 0.4176697321401328655 ) ) ;
#39352=CARTESIAN_POINT ( 'NONE',  ( -0.7939632545931750718, -0.08942795157528024563, -0.3641732283464568787 ) ) ;
#39353=CARTESIAN_POINT ( 'NONE',  ( -0.006561679790025524116, -0.2845877964562159024, 0.3641732283464567677 ) ) ;
#39354=CARTESIAN_POINT ( 'NONE',  ( 0.3018372703412079971, -0.4281496062992124485, 0.4176697321401328655 ) ) ;
#39355=CARTESIAN_POINT ( 'NONE',  ( -1.056430446194224881, -0.5511811023622046335, 0.09757992244046803654 ) ) ;
#39357=CARTESIAN_POINT ( 'NONE',  ( 0.7677165354330716118, -0.5400638737290844871, 0.3530559997133364547 ) ) ;
#39358=CARTESIAN_POINT ( 'NONE',  ( -1.620734908136482577, 0.2952755905511811885, 0.1292274648535926551 ) ) ;
#39360=CARTESIAN_POINT ( 'NONE',  ( -0.4790026246719154557, -0.3162353388693405765, 0.4822834645669290543 ) ) ;
#39361=CARTESIAN_POINT ( 'NONE',  ( 0.1771653543307093182, 0.07958543189024085140, 0.2665933059059887866 ) ) ;
#39362=CARTESIAN_POINT ( 'NONE',  ( -0.9383202099737524282, -0.3162353388693409650, -0.4822834645669289433 ) ) ;
#39363=CARTESIAN_POINT ( 'NONE',  ( 0.8792650918635177559, -0.004921259842519576551, 0.3153832671262227771 ) ) ;
#39364=CARTESIAN_POINT ( 'NONE',  ( -0.1837270341207343505, -0.5023911411419708095, 0.1820866141732285504 ) ) ;
#39365=CARTESIAN_POINT ( 'NONE',  ( -0.4724409448818890911, -0.1870078740157479769, 0.4822834645669291653 ) ) ;
#39366=CARTESIAN_POINT ( 'NONE',  ( -1.312335958005248715, -0.6046776061558809534, -0.2411417322834644161 ) ) ;
#39367=CARTESIAN_POINT ( 'NONE',  ( -1.574803149606298192, -0.1870078740157480879, -0.4822834645669291653 ) ) ;
#39369=CARTESIAN_POINT ( 'NONE',  ( 1.463254593175853824, -0.5511811023622046335, 0.09757992244046803654 ) ) ;
#39370=CARTESIAN_POINT ( 'NONE',  ( 0.3149606299212606708, -0.1870078740157480879, -0.4822834645669291653 ) ) ;
#39371=CARTESIAN_POINT ( 'NONE',  ( -1.502624671916009680, -0.3162353388693405765, 0.4822834645669290543 ) ) ;
#39372=CARTESIAN_POINT ( 'NONE',  ( -1.548556430446193399, 0.2306618581243848609, 0.2411417322834645549 ) ) ;
#39376=CARTESIAN_POINT ( 'NONE',  ( -1.056430446194224881, -0.5511811023622046335, 0.09757992244046803654 ) ) ;
#39377=CARTESIAN_POINT ( 'NONE',  ( 0.6692913385826777528, 0.2952755905511811885, 0.000000000000000000 ) ) ;
#39378=CARTESIAN_POINT ( 'NONE',  ( -0.9776902887139098386, -0.5511811023622046335, 0.09757992244046803654 ) ) ;
#39380=CARTESIAN_POINT ( 'NONE',  ( -1.010498687664041384, -0.4281496062992127816, -0.4176697321401328100 ) ) ;
#39381=CARTESIAN_POINT ( 'NONE',  ( 0.8267716535433078384, -0.6692913385826771977, 8.415575281601705876E-17 ) ) ;
#39382=CARTESIAN_POINT ( 'NONE',  ( 0.4330708661417329575, 0.2952755905511811885, 0.000000000000000000 ) ) ;
#39383=LINE ( 'NONE', #51997, #72136 ) ;
#39384=CARTESIAN_POINT ( 'NONE',  ( -1.706036745406823485, 0.1283753931104748280, 0.1820866141732283561 ) ) ;
#39390=DIRECTION ( 'NONE',  ( -1.000000000000000000, -3.096699300667737957E-16, 1.692413147294446216E-16 ) ) ;
#39391=CARTESIAN_POINT ( 'NONE',  ( 0.5446194225721792126, -0.2845877964562159024, 0.3641732283464567677 ) ) ;
#39392=CARTESIAN_POINT ( 'NONE',  ( 0.2362204724409456558, -0.1870078740157480601, -0.3641732283464567677 ) ) ;
#39393=CARTESIAN_POINT ( 'NONE',  ( -0.03280839895013062252, -0.6692913385826771977, 0.1292274648535927661 ) ) ;
#39394=CARTESIAN_POINT ( 'NONE',  ( 1.122047244094488860, 0.1660481256975885056, 0.3530559997133364547 ) ) ;
#39396=CARTESIAN_POINT ( 'NONE',  ( 0.5249343832021005074, -0.5023911411419708095, 0.1820866141732285504 ) ) ;
#39397=EDGE_CURVE ( 'NONE', #7338, #78564, #78414, .T. ) ;
#39398=CARTESIAN_POINT ( 'NONE',  ( -0.9120734908136475250, -0.6692913385826773087, -0.1292274648535924053 ) ) ;
#39399=CARTESIAN_POINT ( 'NONE',  ( 1.437007874015748810, 0.1660481256975885056, 0.3530559997133364547 ) ) ;
#39400=CARTESIAN_POINT ( 'NONE',  ( 1.043307086614173818, 0.1660481256975885056, 0.3530559997133364547 ) ) ;
#39404=VECTOR ( 'NONE', #9890, 39.37007874015748143 ) ;
#39405=CARTESIAN_POINT ( 'NONE',  ( -1.227034120734907585, 0.2952755905511811885, 0.1292274648535926551 ) ) ;
#39406=CARTESIAN_POINT ( 'NONE',  ( -0.8464566929133852113, 0.1660481256975885056, 0.3530559997133364547 ) ) ;
#39407=CARTESIAN_POINT ( 'NONE',  ( -0.7152230971128602510, -0.2845877964562159024, 0.3641732283464567677 ) ) ;
#39408=CARTESIAN_POINT ( 'NONE',  ( -0.5643044619422565855, -0.4281496062992124485, 0.4176697321401328655 ) ) ;
#39411=CARTESIAN_POINT ( 'NONE',  ( 1.528871391076116026, 0.2952755905511811885, 0.1292274648535926551 ) ) ;
#39412=CARTESIAN_POINT ( 'NONE',  ( -1.430446194225721390, -0.4281496062992124485, 0.4176697321401328655 ) ) ;
#39413=CARTESIAN_POINT ( 'NONE',  ( 0.4790026246719167324, -0.05778040916215522460, 0.4822834645669289988 ) ) ;
#39414=CARTESIAN_POINT ( 'NONE',  ( -0.9645669291338575535, 0.1660481256975883668, -0.3530559997133364547 ) ) ;
#39416=CARTESIAN_POINT ( 'NONE',  ( 0.5183727034120741983, 0.2952755905511810774, -0.1292274648535930714 ) ) ;
#39418=CARTESIAN_POINT ( 'NONE',  ( -0.7939632545931750718, -0.08942795157528024563, -0.3641732283464568787 ) ) ;
#39421=ORIENTED_EDGE ( 'NONE', *, *, #32070, .F. ) ;
#39422=CARTESIAN_POINT ( 'NONE',  ( -1.541994750656167090, 0.1771653543307087630, 0.09757992244046791164 ) ) ;
#39423=CARTESIAN_POINT ( 'NONE',  ( -1.161417322834644716, -0.5400638737290845981, -0.3530559997133363437 ) ) ;
#39424=CARTESIAN_POINT ( 'NONE',  ( -1.141732283464566011, 0.2952755905511811885, 0.000000000000000000 ) ) ;
#39426=CARTESIAN_POINT ( 'NONE',  ( -1.069553805774277722, 0.2952755905511811885, 0.1292274648535926551 ) ) ;
#39427=CARTESIAN_POINT ( 'NONE',  ( -1.076115485564303809, 0.2306618581243848609, 0.2411417322834645549 ) ) ;
#39428=CARTESIAN_POINT ( 'NONE',  ( -1.620734908136482577, 0.2952755905511811885, 0.1292274648535926551 ) ) ;
#39429=CARTESIAN_POINT ( 'NONE',  ( -1.595398199321656829, 0.7375059713363286695, -0.1559797534342474701 ) ) ;
#39430=CARTESIAN_POINT ( 'NONE',  ( 0.2165354330708668673, -0.4536011799217367080, 0.2665933059059888421 ) ) ;
#39431=CARTESIAN_POINT ( 'NONE',  ( 1.595398199321655497, 0.4829664696085563258, 0.1559797534342492742 ) ) ;
#39433=CARTESIAN_POINT ( 'NONE',  ( -0.3083989501312330295, -0.08942795157527998196, 0.3641732283464567121 ) ) ;
#39434=CARTESIAN_POINT ( 'NONE',  ( -0.6561679790026240244, 0.2306618581243847221, -0.2411417322834647770 ) ) ;
#39435=CARTESIAN_POINT ( 'NONE',  ( 0.7742782152230978099, -0.4281496062992124485, 0.4176697321401328655 ) ) ;
#39436=CARTESIAN_POINT ( 'NONE',  ( -0.5249343832020990641, 0.2306618581243848609, 0.2411417322834645549 ) ) ;
#39437=ORIENTED_EDGE ( 'NONE', *, *, #52610, .T. ) ;
#39438=EDGE_LOOP ( 'NONE', ( #18224, #33867, #79331, #47472, #73713 ) ) ;
#39440=CARTESIAN_POINT ( 'NONE',  ( -0.8989501312335946848, -0.6692913385826771977, 0.1292274648535927661 ) ) ;
#39441=CARTESIAN_POINT ( 'NONE',  ( 1.213910761154856299, -0.6692913385826773087, -0.1292274648535924053 ) ) ;
#39442=CARTESIAN_POINT ( 'NONE',  ( -1.469816272965878357, -0.5023911411419708095, -0.1820866141732282451 ) ) ;
#39448=CARTESIAN_POINT ( 'NONE',  ( -0.1509186351706028884, -0.3162353388693409650, -0.4822834645669289433 ) ) ;
#39449=CARTESIAN_POINT ( 'NONE',  ( -1.522309711286088607, -0.5023911411419708095, 0.1820866141732285504 ) ) ;
#39450=CARTESIAN_POINT ( 'NONE',  ( -0.8923884514435688198, 0.2306618581243847221, -0.2411417322834647770 ) ) ;
#39452=CARTESIAN_POINT ( 'NONE',  ( -1.095800524934382292, -0.05778040916215522460, 0.4822834645669289988 ) ) ;
#39454=ADVANCED_FACE ( 'NONE', ( #49856 ), #27525, .F. ) ;
#39455=CARTESIAN_POINT ( 'NONE',  ( -0.9711286089238838626, -0.6046776061558807314, 0.2411417322834647770 ) ) ;
#39456=CARTESIAN_POINT ( 'NONE',  ( -0.3346456692913377662, -0.5400638737290844871, 0.3530559997133364547 ) ) ;
#39458=CARTESIAN_POINT ( 'NONE',  ( 0.8267716535433077274, 0.1771653543307087630, 0.000000000000000000 ) ) ;
#39460=CIRCLE ( 'NONE', #70387, 1.220472440944881942 ) ;
#39461=CARTESIAN_POINT ( 'NONE',  ( 0.6561679790026253567, -0.5023911411419708095, -0.1820866141732282451 ) ) ;
#39462=CARTESIAN_POINT ( 'NONE',  ( 1.384514435695538337, -0.5511811023622046335, 0.09757992244046803654 ) ) ;
#39463=CARTESIAN_POINT ( 'NONE',  ( 1.541994750656168645, -0.6692913385826771977, 0.1292274648535927661 ) ) ;
#39465=CARTESIAN_POINT ( 'NONE',  ( 0.1640419947506569498, -0.2845877964562161244, -0.3641732283464567121 ) ) ;
#39467=CARTESIAN_POINT ( 'NONE',  ( -1.377952755905511140, -0.6692913385826771977, 8.415575281601705876E-17 ) ) ;
#39468=CARTESIAN_POINT ( 'NONE',  ( 1.417322834645670104, -0.1870078740157479769, 0.4822834645669291653 ) ) ;
#39470=CARTESIAN_POINT ( 'NONE',  ( -0.6233595800524928121, -0.2845877964562161244, -0.3641732283464567121 ) ) ;
#39471=CARTESIAN_POINT ( 'NONE',  ( -0.4527559055118102749, 0.1660481256975885056, 0.3530559997133364547 ) ) ;
#39472=CARTESIAN_POINT ( 'NONE',  ( 0.5118110236220480003, -0.6692913385826771977, 8.415575281601705876E-17 ) ) ;
#39475=CARTESIAN_POINT ( 'NONE',  ( 0.7939632545931766261, -0.08942795157527998196, 0.3641732283464567121 ) ) ;
#39476=CARTESIAN_POINT ( 'NONE',  ( -0.03937007874015669567, -0.5511811023622047445, 6.969142054262312111E-17 ) ) ;
#39477=CARTESIAN_POINT ( 'NONE',  ( -0.4527559055118102749, -0.5400638737290845981, -0.3530559997133363437 ) ) ;
#39478=CARTESIAN_POINT ( 'NONE',  ( -1.423884514435694859, -0.3162353388693405765, 0.4822834645669290543 ) ) ;
#39479=CARTESIAN_POINT ( 'NONE',  ( -0.5971128608923877978, -0.5511811023622048555, -0.09757992244046775898 ) ) ;
#39481=CARTESIAN_POINT ( 'NONE',  ( 0.6299212598425204535, -0.1870078740157480879, -0.4822834645669291653 ) ) ;
#39482=CARTESIAN_POINT ( 'NONE',  ( -0.8661417322834640276, -0.1870078740157479769, 0.4822834645669291653 ) ) ;
#39485=CARTESIAN_POINT ( 'NONE',  ( 0.2493438320209980519, -0.3690944881889765550, -0.3153832671262227771 ) ) ;
#39486=CARTESIAN_POINT ( 'NONE',  ( -0.9711286089238838626, 0.2306618581243847221, -0.2411417322834647770 ) ) ;
#39487=CARTESIAN_POINT ( 'NONE',  ( -1.279527559055116948, 0.1660481256975883668, -0.3530559997133364547 ) ) ;
#39488=CARTESIAN_POINT ( 'NONE',  ( -1.292650918635170010, 0.1771653543307087075, -0.09757992244046823083 ) ) ;
#39490=CARTESIAN_POINT ( 'NONE',  ( -0.8530183727034112984, -0.004921259842519576551, 0.3153832671262227771 ) ) ;
#39492=CARTESIAN_POINT ( 'NONE',  ( 1.430446194225722500, 0.05413385826771666132, 0.4176697321401328100 ) ) ;
#39497=CARTESIAN_POINT ( 'NONE',  ( -1.574803149606298636, -0.1870078740157479769, 0.4822834645669291653 ) ) ;
#39498=CARTESIAN_POINT ( 'NONE',  ( -1.502624671916009680, -0.05778040916215560624, -0.4822834645669293319 ) ) ;
#39499=CARTESIAN_POINT ( 'NONE',  ( 1.076115485564305141, -0.6046776061558807314, 0.2411417322834647770 ) ) ;
#39502=CARTESIAN_POINT ( 'NONE',  ( 0.3674540682414705883, -0.6046776061558807314, 0.2411417322834647770 ) ) ;
#39503=CARTESIAN_POINT ( 'NONE',  ( 8.195543980992789655E-16, -0.1870078740157480879, -0.4822834645669291653 ) ) ;
#39506=CARTESIAN_POINT ( 'NONE',  ( 0.7939632545931766261, -0.08942795157527998196, 0.3641732283464567121 ) ) ;
#39511=CARTESIAN_POINT ( 'NONE',  ( -0.01968503937007793844, -0.5400638737290844871, 0.3530559997133364547 ) ) ;
#39512=CARTESIAN_POINT ( 'NONE',  ( 1.259842519685040019, -0.1870078740157479769, 0.4822834645669291653 ) ) ;
#39513=CARTESIAN_POINT ( 'NONE',  ( 0.5249343832021005074, -0.6046776061558807314, 0.2411417322834647770 ) ) ;
#39515=CARTESIAN_POINT ( 'NONE',  ( 1.246719160104987623, 0.05413385826771626580, -0.4176697321401330321 ) ) ;
#39516=CARTESIAN_POINT ( 'NONE',  ( -0.5183727034120726440, 0.2952755905511811885, 0.1292274648535926551 ) ) ;
#39517=CARTESIAN_POINT ( 'NONE',  ( -0.05905511811023545637, -0.5400638737290845981, -0.3530559997133363437 ) ) ;
#39518=CARTESIAN_POINT ( 'NONE',  ( 1.450131233595801428, 0.2952755905511811885, 0.1292274648535926551 ) ) ;
#39519=CARTESIAN_POINT ( 'NONE',  ( 1.482939632545932307, 0.05413385826771626580, -0.4176697321401330321 ) ) ;
#39520=CARTESIAN_POINT ( 'NONE',  ( 1.292650918635171564, -0.6692913385826773087, -0.1292274648535924053 ) ) ;
#39522=CARTESIAN_POINT ( 'NONE',  ( 0.2952755905511819101, 0.07958543189024071263, -0.2665933059059888421 ) ) ;
#39526=CARTESIAN_POINT ( 'NONE',  ( -0.2887139107611542133, 0.1283753931104748280, 0.1820866141732283561 ) ) ;
#39527=CARTESIAN_POINT ( 'NONE',  ( -0.1640419947506553400, -0.05778040916215560624, -0.4822834645669293319 ) ) ;
#39529=CARTESIAN_POINT ( 'NONE',  ( -0.03937007874015669567, -0.6692913385826771977, 8.415575281601705876E-17 ) ) ;
#39530=CARTESIAN_POINT ( 'NONE',  ( 0.01312335958005323398, 0.05413385826771666132, 0.4176697321401328100 ) ) ;
#39531=CARTESIAN_POINT ( 'NONE',  ( -0.9842519685039360366, 0.2952755905511811885, 0.000000000000000000 ) ) ;
#39532=CARTESIAN_POINT ( 'NONE',  ( -1.135170603674539924, -0.6692913385826771977, 0.1292274648535927661 ) ) ;
#39534=CARTESIAN_POINT ( 'NONE',  ( 1.463254593175853824, -0.5511811023622046335, 0.09757992244046803654 ) ) ;
#39535=CARTESIAN_POINT ( 'NONE',  ( -1.430446194225720724, 0.05413385826771626580, -0.4176697321401330321 ) ) ;
#39537=CARTESIAN_POINT ( 'NONE',  ( 1.095800524934383846, -0.2845877964562159024, 0.3641732283464567677 ) ) ;
#39538=CARTESIAN_POINT ( 'NONE',  ( 0.2887139107611556010, 0.2306618581243847221, -0.2411417322834647770 ) ) ;
#39539=CARTESIAN_POINT ( 'NONE',  ( 0.7874015748031503170, -0.1870078740157480879, -0.4822834645669291653 ) ) ;
#39541=CARTESIAN_POINT ( 'NONE',  ( -1.712598425196849572, 0.1660481256975885056, 0.3530559997133364547 ) ) ;
#39544=CARTESIAN_POINT ( 'NONE',  ( -0.6692913385826764205, -0.6692913385826771977, 8.415575281601705876E-17 ) ) ;
#39547=CARTESIAN_POINT ( 'NONE',  ( -1.076115485564303809, -0.5023911411419708095, -0.1820866141732282451 ) ) ;
#39548=CARTESIAN_POINT ( 'NONE',  ( 1.108923884514436242, -0.05778040916215522460, 0.4822834645669289988 ) ) ;
#39549=CARTESIAN_POINT ( 'NONE',  ( 0.8858267716535438430, 0.1660481256975885056, 0.3530559997133364547 ) ) ;
#39550=CARTESIAN_POINT ( 'NONE',  ( -0.1771653543307080136, 0.07958543189024071263, -0.2665933059059888421 ) ) ;
#39551=CARTESIAN_POINT ( 'NONE',  ( 0.5183727034120741983, 0.2952755905511810774, -0.1292274648535930714 ) ) ;
#39553=CARTESIAN_POINT ( 'NONE',  ( 0.3937007874015754361, -0.1870078740157479769, 0.3641732283464567677 ) ) ;
#39554=CARTESIAN_POINT ( 'NONE',  ( 0.1312335958005255154, -0.6046776061558807314, 0.2411417322834647770 ) ) ;
#39557=CARTESIAN_POINT ( 'NONE',  ( -1.240157480314959759, 0.1660481256975885056, 0.3530559997133364547 ) ) ;
#39558=CARTESIAN_POINT ( 'NONE',  ( 0.3280839895013130669, -0.004921259842519576551, 0.3153832671262227771 ) ) ;
#39560=CARTESIAN_POINT ( 'NONE',  ( -0.8005249343832013809, -0.4281496062992124485, 0.4176697321401328655 ) ) ;
#39561=CARTESIAN_POINT ( 'NONE',  ( -0.5118110236220466680, 0.1771653543307087630, 0.000000000000000000 ) ) ;
#39563=CARTESIAN_POINT ( 'NONE',  ( -0.7874015748031489847, -0.1870078740157479769, 0.4822834645669291653 ) ) ;
#39564=CARTESIAN_POINT ( 'NONE',  ( -0.7283464566929126471, -0.5400638737290844871, 0.3530559997133364547 ) ) ;
#39565=CARTESIAN_POINT ( 'NONE',  ( 0.4330708661417329575, -0.5511811023622047445, 6.969142054262312111E-17 ) ) ;
#39567=CARTESIAN_POINT ( 'NONE',  ( -0.1574803149606292529, -0.1870078740157480879, -0.4822834645669291653 ) ) ;
#39569=CARTESIAN_POINT ( 'NONE',  ( -1.437007874015747477, -0.4536011799217367080, 0.2665933059059888421 ) ) ;
#39570=CARTESIAN_POINT ( 'NONE',  ( 0.8398950131233602345, -0.5023911411419708095, 0.1820866141732285504 ) ) ;
#39571=CARTESIAN_POINT ( 'NONE',  ( 1.272965879265092637, 0.05413385826771666132, 0.4176697321401328100 ) ) ;
#39572=CARTESIAN_POINT ( 'NONE',  ( -0.6889763779527552368, -0.4536011799217368745, -0.2665933059059886201 ) ) ;
#39573=CARTESIAN_POINT ( 'NONE',  ( -1.364829396325458521, 0.1283753931104746893, -0.1820866141732285504 ) ) ;
#39574=CARTESIAN_POINT ( 'NONE',  ( -0.6627296587926501115, 0.2952755905511810774, -0.1292274648535930714 ) ) ;
#39575=CARTESIAN_POINT ( 'NONE',  ( -0.2887139107611542133, 0.2306618581243848609, 0.2411417322834645549 ) ) ;
#39576=CARTESIAN_POINT ( 'NONE',  ( 0.7217847769028878924, -0.004921259842519576551, 0.3153832671262227771 ) ) ;
#39578=CARTESIAN_POINT ( 'NONE',  ( 1.161417322834646271, 0.07958543189024071263, -0.2665933059059888421 ) ) ;
#39580=CARTESIAN_POINT ( 'NONE',  ( 0.5118110236220480003, -0.6692913385826771977, 8.415575281601705876E-17 ) ) ;
#39582=CARTESIAN_POINT ( 'NONE',  ( -0.7086614173228339419, -0.1870078740157480879, -0.4822834645669291653 ) ) ;
#39584=CARTESIAN_POINT ( 'NONE',  ( 1.292650918635171564, 0.1771653543307087630, 0.09757992244046791164 ) ) ;
#39585=CARTESIAN_POINT ( 'NONE',  ( 0.6364829396325465405, -0.3162353388693409650, -0.4822834645669289433 ) ) ;
#39586=CARTESIAN_POINT ( 'NONE',  ( 0.3018372703412079971, 0.05413385826771626580, -0.4176697321401330321 ) ) ;
#39588=CARTESIAN_POINT ( 'NONE',  ( 0.1312335958005257930, 0.1283753931104746893, -0.1820866141732285504 ) ) ;
#39589=CARTESIAN_POINT ( 'NONE',  ( 0.8070866141732289112, -0.5400638737290845981, -0.3530559997133363437 ) ) ;
#39590=CARTESIAN_POINT ( 'NONE',  ( -0.2034120734908131112, -0.5511811023622048555, -0.09757992244046775898 ) ) ;
#39591=AXIS2_PLACEMENT_3D ( 'NONE', #10369, #3217, #72674 ) ;
#39592=CARTESIAN_POINT ( 'NONE',  ( -0.5905511811023613777, -0.6692913385826771977, 8.415575281601705876E-17 ) ) ;
#39594=CARTESIAN_POINT ( 'NONE',  ( -0.3477690288713905509, -0.6692913385826771977, 0.1292274648535927661 ) ) ;
#39596=CARTESIAN_POINT ( 'NONE',  ( -1.167979002624671470, 0.05413385826771666132, 0.4176697321401328100 ) ) ;
#39597=CARTESIAN_POINT ( 'NONE',  ( -0.5905511811023615998, 0.1771653543307087630, 0.000000000000000000 ) ) ;
#39598=CARTESIAN_POINT ( 'NONE',  ( -0.1181102362204717315, 0.2952755905511811885, 0.000000000000000000 ) ) ;
#39599=CARTESIAN_POINT ( 'NONE',  ( -1.069553805774277722, 0.2952755905511811885, 0.1292274648535926551 ) ) ;
#39600=CARTESIAN_POINT ( 'NONE',  ( -0.5839895013123351797, -0.6692913385826771977, 0.1292274648535927661 ) ) ;
#39602=CARTESIAN_POINT ( 'NONE',  ( -0.8989501312335947958, 0.2952755905511810219, -0.1292274648535930437 ) ) ;
#39603=CARTESIAN_POINT ( 'NONE',  ( 0.7349081364829402885, -0.6046776061558809534, -0.2411417322834644161 ) ) ;
#39604=CARTESIAN_POINT ( 'NONE',  ( 1.469816272965879911, -0.6046776061558807314, 0.2411417322834647770 ) ) ;
#39606=B_SPLINE_CURVE_WITH_KNOTS ( 'NONE', 3,
 ( #32103, #76321, #44295, #549 ),
 .UNSPECIFIED., .F., .F.,
 ( 4, 4 ),
 ( 3.210432057656183116E-07, 0.001287787053612148448 ),
 .UNSPECIFIED. ) ;
#39608=CARTESIAN_POINT ( 'NONE',  ( -1.312335958005248715, -0.6046776061558809534, -0.2411417322834644161 ) ) ;
#39612=CARTESIAN_POINT ( 'NONE',  ( -0.1509186351706028884, -0.2845877964562161244, -0.3641732283464567121 ) ) ;
#39615=CARTESIAN_POINT ( 'NONE',  ( 0.1968503937007881344, 0.2952755905511811885, 0.000000000000000000 ) ) ;
#39616=CARTESIAN_POINT ( 'NONE',  ( -0.1377952755905504645, 0.1660481256975885056, 0.3530559997133364547 ) ) ;
#39617=CARTESIAN_POINT ( 'NONE',  ( -0.5839895013123351797, -0.6692913385826771977, 0.1292274648535927661 ) ) ;
#39619=CARTESIAN_POINT ( 'NONE',  ( -0.6955380577427815458, -0.004921259842519576551, 0.3153832671262227771 ) ) ;
#39620=CARTESIAN_POINT ( 'NONE',  ( 0.5839895013123367340, 0.2952755905511811885, 0.1292274648535926551 ) ) ;
#39621=CARTESIAN_POINT ( 'NONE',  ( 0.5905511811023629321, -0.5511811023622047445, 6.969142054262312111E-17 ) ) ;
#39622=CARTESIAN_POINT ( 'NONE',  ( -0.4658792650918627265, -0.3162353388693409650, -0.4822834645669289433 ) ) ;
#39623=B_SPLINE_CURVE_WITH_KNOTS ( 'NONE', 3,
 ( #23252, #56056, #81350, #10643 ),
 .UNSPECIFIED., .F., .F.,
 ( 4, 4 ),
 ( 1.999999999910059834E-07, 0.006970199999999935996 ),
 .UNSPECIFIED. ) ;
#39625=CARTESIAN_POINT ( 'NONE',  ( -0.7283464566929126471, -0.5400638737290844871, 0.3530559997133364547 ) ) ;
#39627=CARTESIAN_POINT ( 'NONE',  ( 1.417322834645670104, -0.1870078740157480879, -0.4822834645669291653 ) ) ;
#39631=CARTESIAN_POINT ( 'NONE',  ( 0.1377952755905518800, 0.1660481256975883668, -0.3530559997133364547 ) ) ;
#39633=CARTESIAN_POINT ( 'NONE',  ( -0.7677165354330699465, 0.1660481256975885056, 0.3530559997133364547 ) ) ;
#39634=CARTESIAN_POINT ( 'NONE',  ( 1.515748031496063186, -0.5400638737290845981, -0.3530559997133363437 ) ) ;
#39635=CARTESIAN_POINT ( 'NONE',  ( 1.450131233595801428, 0.2952755905511811885, 0.1292274648535926551 ) ) ;
#39636=CARTESIAN_POINT ( 'NONE',  ( 0.1574803149606306130, -0.1870078740157479769, 0.4822834645669291653 ) ) ;
#39637=CARTESIAN_POINT ( 'NONE',  ( -0.1706036745406816491, 0.05413385826771626580, -0.4176697321401330321 ) ) ;
#39639=CARTESIAN_POINT ( 'NONE',  ( -1.371391076115484831, 0.2952755905511810774, -0.1292274648535930714 ) ) ;
#39640=CARTESIAN_POINT ( 'NONE',  ( -0.1640419947506553400, -0.05778040916215560624, -0.4822834645669293319 ) ) ;
#39641=CARTESIAN_POINT ( 'NONE',  ( -0.3149606299212590610, -0.1870078740157480601, -0.3641732283464567677 ) ) ;
#39642=CARTESIAN_POINT ( 'NONE',  ( 1.548556430446194954, 0.2306618581243847221, -0.2411417322834647770 ) ) ;
#39643=CARTESIAN_POINT ( 'NONE',  ( 1.423884514435696413, -0.3162353388693409650, -0.4822834645669289433 ) ) ;
#39644=CARTESIAN_POINT ( 'NONE',  ( -0.3740157480314953431, -0.5400638737290845981, -0.3530559997133363437 ) ) ;
#39645=CARTESIAN_POINT ( 'NONE',  ( -0.6299212598425201204, 1.968503937007873628, 0.4915354330708656128 ) ) ;
#39646=CARTESIAN_POINT ( 'NONE',  ( 1.167979002624672580, 0.05413385826771626580, -0.4176697321401330321 ) ) ;
#39648=EDGE_CURVE ( 'NONE', #71206, #29072, #73539, .T. ) ;
#39650=CARTESIAN_POINT ( 'NONE',  ( 0.02624671916010564918, -0.6046776061558809534, -0.2411417322834644161 ) ) ;
#39651=CARTESIAN_POINT ( 'NONE',  ( -0.2034120734908131112, -0.5511811023622048555, -0.09757992244046775898 ) ) ;
#39652=CARTESIAN_POINT ( 'NONE',  ( 0.8923884514435703741, 0.1283753931104748280, 0.1820866141732283561 ) ) ;
#39653=CARTESIAN_POINT ( 'NONE',  ( -0.7137454485294948414, 2.165354330708661124, 0.4917280318828577412 ) ) ;
#39655=CARTESIAN_POINT ( 'NONE',  ( 1.587926509186352586, -0.3690944881889765550, -0.3153832671262227771 ) ) ;
#39656=CARTESIAN_POINT ( 'NONE',  ( 1.043307086614173818, -0.5400638737290845981, -0.3530559997133363437 ) ) ;
#39659=CARTESIAN_POINT ( 'NONE',  ( 0.2362204724409456558, -0.1870078740157480879, -0.4822834645669291653 ) ) ;
#39660=CARTESIAN_POINT ( 'NONE',  ( -1.614173228346455824, 0.2952755905511811885, 0.000000000000000000 ) ) ;
#39661=CARTESIAN_POINT ( 'NONE',  ( -1.509186351706035767, 0.05413385826771626580, -0.4176697321401330321 ) ) ;
#39662=CARTESIAN_POINT ( 'NONE',  ( -0.2821522309711278487, 0.2952755905511811885, 0.1292274648535926551 ) ) ;
#39664=CARTESIAN_POINT ( 'NONE',  ( 1.489501312335958172, -0.3162353388693405765, 0.4822834645669290543 ) ) ;
#39665=CARTESIAN_POINT ( 'NONE',  ( 0.5643044619422579178, -0.4281496062992127816, -0.4176697321401328100 ) ) ;
#39666=CARTESIAN_POINT ( 'NONE',  ( 0.8202099737532814183, -0.5511811023622048555, -0.09757992244046775898 ) ) ;
#39668=CARTESIAN_POINT ( 'NONE',  ( 0.2296587926509192634, -0.2845877964562159024, 0.3641732283464567677 ) ) ;
#39669=CARTESIAN_POINT ( 'NONE',  ( -1.187664041994749731, -0.3162353388693405765, 0.4822834645669290543 ) ) ;
#39671=CARTESIAN_POINT ( 'NONE',  ( 0.9973753280839902091, -0.6046776061558807314, 0.2411417322834647770 ) ) ;
#39673=CARTESIAN_POINT ( 'NONE',  ( 0.9251968503937015864, 0.1660481256975883668, -0.3530559997133364547 ) ) ;
#39675=CARTESIAN_POINT ( 'NONE',  ( -0.3740157480314952876, 0.1012011053420777407, 0.2882089793578256898 ) ) ;
#39676=B_SPLINE_CURVE_WITH_KNOTS ( 'NONE', 3,
 ( #23263, #9815, #74633, #42616 ),
 .UNSPECIFIED., .F., .F.,
 ( 4, 4 ),
 ( 1.999999999897049408E-07, 0.006970199999999935128 ),
 .UNSPECIFIED. ) ;
#39677=CARTESIAN_POINT ( 'NONE',  ( 0.4986876640419954376, 0.1283753931104748280, 0.1820866141732283561 ) ) ;
#39678=CARTESIAN_POINT ( 'NONE',  ( 0.5249343832021005074, -0.6046776061558807314, 0.2411417322834647770 ) ) ;
#39680=CARTESIAN_POINT ( 'NONE',  ( -1.089238845144356427, -0.004921259842519576551, 0.3153832671262227771 ) ) ;
#39681=CARTESIAN_POINT ( 'NONE',  ( -1.207349081364828880, 0.2306618581243847221, -0.2411417322834647770 ) ) ;
#39682=CARTESIAN_POINT ( 'NONE',  ( -1.581364829396324945, -0.3162353388693405765, 0.4822834645669290543 ) ) ;
#39683=CARTESIAN_POINT ( 'NONE',  ( 1.161417322834646493, -0.5400638737290844871, 0.3530559997133364547 ) ) ;
#39684=CARTESIAN_POINT ( 'NONE',  ( 1.528871391076116026, 0.2952755905511811885, 0.1292274648535926551 ) ) ;
#39686=CARTESIAN_POINT ( 'NONE',  ( 0.5314960629921264834, 0.1660481256975883668, -0.3530559997133364547 ) ) ;
#39689=CARTESIAN_POINT ( 'NONE',  ( 1.456692913385827515, -0.6692913385826771977, 8.415575281601705876E-17 ) ) ;
#39690=CARTESIAN_POINT ( 'NONE',  ( -1.509186351706035767, -0.004921259842519870586, -0.3153832671262229437 ) ) ;
#39692=CARTESIAN_POINT ( 'NONE',  ( 1.377952755905512472, 0.1771653543307087630, 0.000000000000000000 ) ) ;
#39693=CARTESIAN_POINT ( 'NONE',  ( -1.325459317585300889, -0.004921259842519576551, 0.3153832671262227771 ) ) ;
#39694=CARTESIAN_POINT ( 'NONE',  ( -0.3280839895013117347, -0.004921259842519870586, -0.3153832671262229437 ) ) ;
#39696=CARTESIAN_POINT ( 'NONE',  ( 1.043307086614173818, -0.4536011799217368745, -0.2665933059059886201 ) ) ;
#39697=CARTESIAN_POINT ( 'NONE',  ( 0.6364829396325465405, -0.3162353388693409650, -0.4822834645669289433 ) ) ;
#39698=CARTESIAN_POINT ( 'NONE',  ( 0.9186351706036751663, -0.6046776061558807314, 0.2411417322834647770 ) ) ;
#39699=CARTESIAN_POINT ( 'NONE',  ( 0.1902887139107617975, -0.6692913385826773087, -0.1292274648535924053 ) ) ;
#39700=CARTESIAN_POINT ( 'NONE',  ( 0.5511811023622054106, -0.1870078740157480601, -0.3641732283464567677 ) ) ;
#39701=CARTESIAN_POINT ( 'NONE',  ( 1.141732283464567566, 0.2952755905511811885, 0.000000000000000000 ) ) ;
#39703=CARTESIAN_POINT ( 'NONE',  ( -0.5643044619422565855, 0.05413385826771626580, -0.4176697321401330321 ) ) ;
#39706=CARTESIAN_POINT ( 'NONE',  ( 0.1377952755905518800, -0.5400638737290844871, 0.3530559997133364547 ) ) ;
#39707=CARTESIAN_POINT ( 'NONE',  ( -0.3215223097112853146, -0.05778040916215560624, -0.4822834645669293319 ) ) ;
#39709=CARTESIAN_POINT ( 'NONE',  ( -0.06561679790026180015, -0.4281496062992127816, -0.4176697321401328100 ) ) ;
#39714=CARTESIAN_POINT ( 'NONE',  ( -0.7742782152230965886, -0.004921259842519576551, 0.3153832671262227771 ) ) ;
#39716=CARTESIAN_POINT ( 'NONE',  ( -1.194225721784776262, 0.05413385826771626580, -0.4176697321401330321 ) ) ;
#39718=CARTESIAN_POINT ( 'NONE',  ( 0.4724409448818904789, -0.1870078740157480879, -0.4822834645669291653 ) ) ;
#39719=CARTESIAN_POINT ( 'NONE',  ( -0.6299212598425188991, -0.1870078740157479769, 0.3641732283464567677 ) ) ;
#39720=CARTESIAN_POINT ( 'NONE',  ( 1.076115485564305141, -0.6046776061558807314, 0.2411417322834647770 ) ) ;
#39721=CARTESIAN_POINT ( 'NONE',  ( 0.1837270341207354329, 0.2306618581243848609, 0.2411417322834645549 ) ) ;
#39725=CARTESIAN_POINT ( 'NONE',  ( 1.463254593175853824, -0.6692913385826771977, 0.1292274648535927661 ) ) ;
#39726=CARTESIAN_POINT ( 'NONE',  ( 0.4593175853018379162, -0.4281496062992124485, 0.4176697321401328655 ) ) ;
#39727=CARTESIAN_POINT ( 'NONE',  ( 0.1246719160104994284, -0.6692913385826771977, 0.1292274648535927661 ) ) ;
#39728=CARTESIAN_POINT ( 'NONE',  ( 1.541994750656168645, -0.6692913385826771977, 0.1292274648535927661 ) ) ;
#39729=CARTESIAN_POINT ( 'NONE',  ( 1.069553805774278832, 0.2952755905511810774, -0.1292274648535930714 ) ) ;
#39731=CARTESIAN_POINT ( 'NONE',  ( -0.1312335958005241554, 0.2306618581243848609, 0.2411417322834645549 ) ) ;
#39732=CARTESIAN_POINT ( 'NONE',  ( 1.122047244094488860, -0.5400638737290845981, -0.3530559997133363437 ) ) ;
#39733=CARTESIAN_POINT ( 'NONE',  ( 0.5380577427821529035, -0.4281496062992124485, 0.4176697321401328655 ) ) ;
#39734=CARTESIAN_POINT ( 'NONE',  ( 1.167979002624672580, -0.3690944881889763329, 0.3153832671262228327 ) ) ;
#39735=CARTESIAN_POINT ( 'NONE',  ( -1.115485564304461219, -0.4281496062992124485, 0.4176697321401328655 ) ) ;
#39736=CARTESIAN_POINT ( 'NONE',  ( -1.450131233595799651, -0.6692913385826771977, 0.1292274648535927661 ) ) ;
#39737=CARTESIAN_POINT ( 'NONE',  ( 0.8727034120734912248, -0.3162353388693409650, -0.4822834645669289433 ) ) ;
#39740=ORIENTED_EDGE ( 'NONE', *, *, #38741, .T. ) ;
#39743=CARTESIAN_POINT ( 'NONE',  ( 1.443569553805774897, -0.6046776061558809534, -0.2411417322834644161 ) ) ;
#39744=CARTESIAN_POINT ( 'NONE',  ( 0.7939632545931766261, -0.08942795157527998196, 0.3641732283464567121 ) ) ;
#39746=CARTESIAN_POINT ( 'NONE',  ( -0.1312335958005241554, 0.2306618581243848609, 0.2411417322834645549 ) ) ;
#39749=CARTESIAN_POINT ( 'NONE',  ( 1.384514435695538337, -0.6692913385826771977, 0.1292274648535927661 ) ) ;
#39751=CARTESIAN_POINT ( 'NONE',  ( -0.1968503937007867743, -0.6692913385826771977, 8.415575281601705876E-17 ) ) ;
#39752=CARTESIAN_POINT ( 'NONE',  ( 0.9973753280839902091, 0.2306618581243847221, -0.2411417322834647770 ) ) ;
#39754=CARTESIAN_POINT ( 'NONE',  ( -1.541994750656167090, 0.2952755905511811885, 0.1292274648535926551 ) ) ;
#39759=CARTESIAN_POINT ( 'NONE',  ( -0.9383202099737524282, -0.2845877964562161244, -0.3641732283464567121 ) ) ;
#39760=CARTESIAN_POINT ( 'NONE',  ( 0.9324623468618423727, 2.784432375088962958E-17, -0.3464511005275205946 ) ) ;
#39761=CARTESIAN_POINT ( 'NONE',  ( 0.4199475065616805614, 0.2306618581243848609, 0.2411417322834645549 ) ) ;
#39763=EDGE_LOOP ( 'NONE', ( #19223, #15433, #83192, #9505 ) ) ;
#39766=CARTESIAN_POINT ( 'NONE',  ( 0.7808398950131241190, -0.05778040916215560624, -0.4822834645669293319 ) ) ;
#39767=CARTESIAN_POINT ( 'NONE',  ( -1.489501312335957062, -0.3162353388693409650, -0.4822834645669289433 ) ) ;
#39769=CARTESIAN_POINT ( 'NONE',  ( -0.8005249343832013809, -0.3690944881889763329, 0.3153832671262228327 ) ) ;
#39770=CARTESIAN_POINT ( 'NONE',  ( -1.568241469816272105, -0.2845877964562161244, -0.3641732283464567121 ) ) ;
#39772=CARTESIAN_POINT ( 'NONE',  ( 0.4002624671916016896, -0.3162353388693409650, -0.4822834645669289433 ) ) ;
#39773=CARTESIAN_POINT ( 'NONE',  ( -0.7545931758530176614, -0.5511811023622048555, -0.09757992244046775898 ) ) ;
#39774=CARTESIAN_POINT ( 'NONE',  ( 0.2952755905511816326, -0.4536011799217367080, 0.2665933059059888421 ) ) ;
#39775=EDGE_CURVE ( 'NONE', #20676, #24808, #24114, .T. ) ;
#39776=CARTESIAN_POINT ( 'NONE',  ( -0.1771653543307080136, -0.5400638737290844871, 0.3530559997133364547 ) ) ;
#39777=CARTESIAN_POINT ( 'NONE',  ( -1.292650918635170010, 0.1771653543307087075, -0.09757992244046823083 ) ) ;
#39779=CARTESIAN_POINT ( 'NONE',  ( 0.9055118110236227702, -0.6692913385826771977, 8.415575281601705876E-17 ) ) ;
#39780=EDGE_CURVE ( 'NONE', #14171, #17097, #51730, .T. ) ;
#39781=CARTESIAN_POINT ( 'NONE',  ( -1.535433070866141225, -0.6692913385826771977, 8.415575281601705876E-17 ) ) ;
#39783=CARTESIAN_POINT ( 'NONE',  ( -0.7217847769028863381, 0.05413385826771626580, -0.4176697321401330321 ) ) ;
#39784=CARTESIAN_POINT ( 'NONE',  ( -0.2690288713910754526, 0.1771653543307087075, -0.09757992244046823083 ) ) ;
#39785=CARTESIAN_POINT ( 'NONE',  ( -1.181102362204723644, -0.1870078740157479769, 0.4822834645669291653 ) ) ;
#39786=CARTESIAN_POINT ( 'NONE',  ( 0.9842519685039378130, -0.5511811023622047445, 6.969142054262312111E-17 ) ) ;
#39787=CARTESIAN_POINT ( 'NONE',  ( -0.4199475065616791736, 0.1283753931104746893, -0.1820866141732285504 ) ) ;
#39788=CARTESIAN_POINT ( 'NONE',  ( -1.181102362204723644, -0.1870078740157480879, -0.4822834645669291653 ) ) ;
#39789=CARTESIAN_POINT ( 'NONE',  ( -1.148293963254592542, -0.6692913385826773087, -0.1292274648535924053 ) ) ;
#39790=CARTESIAN_POINT ( 'NONE',  ( 1.692913385826772421, 0.2952755905511811885, 0.000000000000000000 ) ) ;
#39792=CARTESIAN_POINT ( 'NONE',  ( 1.437007874015748810, -0.4536011799217368745, -0.2665933059059886201 ) ) ;
#39793=CARTESIAN_POINT ( 'NONE',  ( 0.2165354330708668673, -0.5400638737290844871, 0.3530559997133364547 ) ) ;
#39794=CARTESIAN_POINT ( 'NONE',  ( -1.561679790026246017, -0.4281496062992127816, -0.4176697321401328100 ) ) ;
#39795=CARTESIAN_POINT ( 'NONE',  ( -1.469816272965878357, -0.6046776061558809534, -0.2411417322834644161 ) ) ;
#39796=ORIENTED_EDGE ( 'NONE', *, *, #12583, .T. ) ;
#39799=CARTESIAN_POINT ( 'NONE',  ( -0.7939632545931750718, -0.08942795157528024563, -0.3641732283464568787 ) ) ;
#39800=CARTESIAN_POINT ( 'NONE',  ( 0.8858267716535438430, -0.5400638737290845981, -0.3530559997133363437 ) ) ;
#39802=CARTESIAN_POINT ( 'NONE',  ( -1.253280839895012377, -0.08942795157527998196, 0.3641732283464567121 ) ) ;
#39804=CARTESIAN_POINT ( 'NONE',  ( -1.568241469816272105, -0.05778040916215522460, 0.4822834645669289988 ) ) ;
#39805=CIRCLE ( 'NONE', #50529, 1.220472440944881942 ) ;
#39807=CARTESIAN_POINT ( 'NONE',  ( 0.8858267716535438430, 0.1660481256975885056, 0.3530559997133364547 ) ) ;
#39808=CARTESIAN_POINT ( 'NONE',  ( 0.4461942257217856311, 0.2306618581243847221, -0.2411417322834647770 ) ) ;
#39809=EDGE_CURVE ( 'NONE', #78537, #31856, #79176, .T. ) ;
#39810=CARTESIAN_POINT ( 'NONE',  ( 1.069553805774278610, -0.6692913385826771977, 0.1292274648535927661 ) ) ;
#39815=CARTESIAN_POINT ( 'NONE',  ( 0.9055118110236227702, 0.1771653543307087630, 0.000000000000000000 ) ) ;
#39816=CARTESIAN_POINT ( 'NONE',  ( 0.1968503937007881344, 0.1771653543307087630, 0.000000000000000000 ) ) ;
#39817=CARTESIAN_POINT ( 'NONE',  ( 5.463695987328526437E-16, -0.1870078740157479769, 0.4822834645669291653 ) ) ;
#39818=CARTESIAN_POINT ( 'NONE',  ( 1.095800524934383846, -0.3162353388693405765, 0.4822834645669290543 ) ) ;
#39820=CARTESIAN_POINT ( 'NONE',  ( 0.4068241469816281097, -0.004921259842519576551, 0.3153832671262227771 ) ) ;
#39821=( BOUNDED_SURFACE ( )  B_SPLINE_SURFACE ( 1, 2, ( 
 ( #40515, #32946, #26635, #26207, #58612, #66195, #52289, #33373, #129, #51445, #1391, #52705, #70838, #79666, #28292, #53953, #41742, #22811, #72917, #74169, #54373, #54792, #35441, #15268, #34621, #21983, #80495, #73340, #47227, #22403, #10193, #15688, #60694, #9359, #61107, #16516, #3873, #34200, #42160, #48060, #66609, #80083, #73762, #41346, #67027, #35862, #29532, #55195, #42571, #28709, #2216, #35030, #47645, #48468, #16097, #3459, #59863, #40929, #3044, #67855, #61527, #80902, #53542, #67436, #9770, #29124, #23216, #21565, #48886, #74587, #16931, #2635, #8532, #27882, #79250, #8945, #60285, #4277, #56432, #36667, #76228, #36265, #75403, #24448, #29938, #37905, #49298, #25267, #11008, #5104, #17345, #18562, #57245, #50933, #43378, #12249, #31590, #17749, #44205, #50116, #69078, #74999, #63582, #5916, #11429, #82134, #55602, #37084, #68273, #62770, #30771, #75813, #24854, #18156, #76631, #61934, #81314, #18962, #43788, #23627, #69494, #62342, #82949, #42973, #11843, #69895, #4681, #37496, #63171, #5509, #31172, #10608, #68669, #56838, #30352, #56021, #82536, #81729, #50522, #24038, #49708, #77468, #19379, #44610, #26104, #26944, #64414, #51343, #39576, #40004, #1294, #77891, #26534, #78733, #58936, #70730, #25683, #71991, #52605, #45031, #78312, #19805, #32008, #59345, #58083, #20643, #14344, #45871, #30, #70306, #46296, #58512, #51766, #32843, #39149, #65266, #27359, #875, #6749, #13084, #65692, #52187, #7602, #38737, #63994, #8020, #20222, #32421, #6335, #57668, #33683, #1702, #33276, #45454, #77047, #53018, #12659, #38320, #7172, #449, #71152, #13493, #71569, #64834, #13920, #67341, #34935, #80398, #79565, #15585, #79153, #21880, #10090, #2115, #28194, #29021, #3356, #47958, #21469, #60598, #8842, #40823, #66508, #54269, #35345, #27781, #54687, #66931, #9674, #73662, #53444, #47127, #34518, #61007, #2536, #59760, #2947, #22711, #53852, #73234, #47544, #16003, #48369, #16414, #46716, #74068, #28612, #72817, #9264, #79984, #41244, #22297, #42061, #67756, #35755, #55094, #41650, #14757, #61421, #60184, #3771, #29435, #21056, #72408, #40412, #66093, #8429, #34097, #15167, #10911, #68167, #5007, #61837, #63077, #30677, #55505, #43692, #18469, #31076, #80802, #36163, #82037, #55919, #36569, #36988, #69804, #56744, #31491, #42467, #16831, #17649, #42876, #69397, #18059, #81213, #68569, #17247, #56338, #30255, #81632, #76127, #48787, #75305, #24351, #74484, #50020, #75719, #43281, #23943, #4178, #49610, #37405, #11328, #82442, #62247, #68980, #62667, #11749, #5415, #44112, #23119, #24759, #50427, #23528, #12152, #37808, #63486, #5820, #10510, #29841, #49198, #74899, #4584, #50841, #351, #44930, #45773, #77369, #26433, #19701, #14244, #57152, #20546, #46198, #39902, #70627, #44518, #64737, #38221, #39479, #7075, #31910, #20126, #78214, #7502, #82851, #12563, #58412, #32324, #12983, #13399, #71893, #33171, #7923, #18869, #76541, #45358, #19279, #71472, #77793, #57571, #38639, #76951, #32745, #6651, #57986, #52505, #25172, #51665, #771, #70206, #52084, #13820, #71055, #26008, #63896, #39052, #65166, #6234, #58839, #1197, #51249, #83263, #25585, #65590, #26846, #64317, #8747, #72313, #4384, #33584, #27262, #79464, #20960, #29642, #14660, #15487, #2018, #49412, #81011, #47443, #10716, #34418, #28098, #8334, #60086, #23739, #40317, #40724, #42679, #17039, #61637, #34000, #73137, #21374, #53347, #79057, #67959, #48995, #65996, #68377, #21781, #23325, #3978, #59662, #27682, #47029, #74694, #15068, #72721, #36373, #62047, #35967, #66410, #68779, #30052, #41144, #2440, #10301, #53754, #55303, #17452, #55714, #81424, #75105, #43082, #59247, #1606, #52922, #78636, #46618, #56543, #76744, #19074, #57778, #56133, #82244, #69604, #76339, #50634, #24149, #82648, #75925, #12359, #5212, #51457, #70420, #64115, #4792, #24963, #30469, #18669, #62877, #44722, #62456, #18265, #44314, #81838, #6450, #75519, #77160, #37196, #31286, #43493, #12775, #141, #19492, #11950, #38432, #25797, #43906, #32120, #70004, #37605, #17858, #45146, #11123, #63279, #38017, #49819, #5620 ),
 ( #30876, #36780, #57362, #63693, #69189, #56951, #6032, #11540, #31704, #24563, #50229, #83058, #25380, #51043, #14457, #45569, #27057, #58623, #7286, #32956, #20755, #1811, #51881, #53131, #33384, #33795, #40109, #77586, #13610, #990, #59460, #52299, #26218, #1401, #72515, #78005, #39689, #71681, #65796, #78842, #66205, #13200, #20333, #65381, #14033, #8130, #21168, #8544, #38847, #46824, #52716, #71263, #59047, #78427, #45985, #7716, #14864, #34210, #59873, #21575, #46405, #64527, #72099, #26645, #27473, #40526, #2227, #27892, #53552, #70849, #79260, #6864, #32533, #58197, #565, #19920, #39264, #64946, #54800, #21992, #10201, #68281, #80911, #47237, #2644, #48477, #22412, #3052, #3467, #36273, #23224, #81322, #8956, #66618, #67445, #9367, #35870, #67864, #47653, #35038, #67035, #80503, #80091, #48068, #42580, #15278, #41750, #22819, #40939, #16524, #74178, #9778, #73771, #28301, #16105, #3881, #34630, #48894, #29133, #41354, #60294, #53963, #61944, #61536, #29540, #35450, #79675, #16939, #72926, #73349, #61115, #15697, #42169, #60703, #55203, #28718, #4285, #74596, #10616, #29947, #55611, #54381, #81738, #82143, #12670, #4689, #30779, #31598, #5926, #50532, #24047, #63179, #11437, #43388, #69089, #56847, #37914, #30363, #57257, #69502, #69903, #76236, #56030, #49718, #37093, #12257, #5112, #62351, #37504, #25275, #18570, #82545, #11851, #24458, #75414, #50124, #63591, #42982, #50943, #5517, #17758, #68677, #11018, #38330, #82957, #76640, #75823, #62778, #18971, #23636, #17354, #31182, #36675, #44213, #56440, #24863, #18165, #64005, #44620, #70315, #6345, #43798, #32017, #57677, #49306, #75007, #64424, #7181, #8030, #65700, #26953, #58093, #39586, #71162, #19815, #45464, #33285, #14356, #6758, #33693, #45880, #46306, #52616, #32430, #26114, #13502, #72000, #64843, #38747, #13929, #1713, #32852, #52197, #887, #78322, #59354, #78742, #25692, #27368, #65275, #458, #71578, #7614, #58521, #26544, #53029, #21067, #46725, #34109, #20232, #77056, #77901, #39158, #40013, #58946, #20653, #1304, #40422, #39, #72417, #14766, #66103, #8439, #70742, #51353, #51775, #19389, #45041, #77480, #13094, #80813, #10101, #59770, #15177, #61016, #34944, #15595, #16013, #48796, #35765, #10519, #21478, #79161, #79995, #21890, #48379, #80408, #34530, #47554, #79574, #9683, #9273, #60607, #55104, #27793, #54279, #35354, #53453, #3782, #3367, #40834, #2125, #61435, #73671, #66941, #47972, #22309, #22720, #42475, #41659, #73246, #2545, #29445, #67350, #54702, #60194, #47136, #66519, #41255, #42070, #67765, #23128, #72827, #2956, #28621, #29031, #74078, #8851, #16424, #74494, #16841, #53862, #68180, #28203, #5828, #29850, #24361, #55513, #50031, #4592, #44121, #4187, #43291, #75728, #81221, #31501, #17256, #76549, #62256, #56347, #68579, #69813, #25182, #18877, #11337, #63494, #82860, #68988, #12162, #18068, #36997, #42884, #57161, #50849, #62676, #43703, #23537, #5018, #36173, #30686, #82048, #69406, #76138, #11760, #44526, #49206, #74910, #70214, #37414, #10920, #63086, #30263, #61846, #36577, #5424, #37818, #55927, #31086, #56753, #82453, #24768, #81643, #23951, #50437, #49619, #75313, #18479, #17660, #64744, #7082, #77802, #45367, #70635, #12570, #77377, #78222, #32332, #19286, #7511, #7931, #52514, #45782, #20134, #46625, #26855, #38647, #76958, #39911, #20555, #12991, #46207, #71062, #83270, #27270, #26015, #71901, #58848, #33592, #14253, #38228, #51256, #13828, #13406, #51673, #52094, #1614, #65599, #63905, #57579, #31918, #32753, #57994, #1205, #33179, #64324, #358, #19708, #71481, #39061, #58420, #59257, #6241, #780, #39487, #25593, #65174, #52931, #26441, #78643, #44937, #20966, #6660, #8342, #35252, #66840, #72729, #34008, #59670, #80306, #73569, #22208, #28107, #2025, #60916, #72321, #27691, #15494, #53354, #79890, #79065, #9174, #15075, #48280, #47865, #41152, #3267, #53761, #47450, #21381, #79472, #22621, #47035, #2449, #67251, #9583, #54176, #40733, #34845, #8753, #66417, #34429, #60508, #15914, #60094, #28928, #2856, #41562, #28520, #21788, #73145, #54597 ) ),
 .UNSPECIFIED., .F., .F., .F. ) 
 B_SPLINE_SURFACE_WITH_KNOTS ( ( 2, 2 ),
 ( 3, 2, 2, 2, 2, 2, 2, 2, 2, 2, 2, 2, 2, 2, 2, 2, 2, 2, 2, 2, 2, 2, 2, 2, 2, 2, 2, 2, 2, 2, 2, 2, 2, 2, 2, 2, 2, 2, 2, 2, 2, 2, 2, 2, 2, 2, 2, 2, 2, 2, 2, 2, 2, 2, 2, 2, 2, 2, 2, 2, 2, 2, 2, 2, 2, 2, 2, 2, 2, 2, 2, 2, 2, 2, 2, 2, 2, 2, 2, 2, 2, 2, 2, 2, 2, 2, 2, 2, 2, 2, 2, 2, 2, 2, 2, 2, 2, 2, 2, 2, 2, 2, 2, 2, 2, 2, 2, 2, 2, 2, 2, 2, 2, 2, 2, 2, 2, 2, 2, 2, 2, 2, 2, 2, 2, 2, 2, 2, 2, 2, 2, 2, 2, 2, 2, 2, 2, 2, 2, 2, 2, 2, 2, 2, 2, 2, 2, 2, 2, 2, 2, 2, 2, 2, 2, 2, 2, 2, 2, 2, 2, 2, 2, 2, 2, 2, 2, 2, 2, 2, 2, 2, 2, 2, 2, 2, 2, 2, 2, 2, 2, 2, 2, 2, 2, 2, 2, 2, 2, 2, 2, 2, 2, 2, 2, 2, 2, 2, 2, 2, 2, 2, 2, 2, 2, 2, 2, 2, 2, 2, 2, 2, 2, 2, 2, 2, 2, 2, 2, 2, 2, 2, 2, 2, 2, 2, 2, 2, 2, 2, 2, 2, 2, 2, 2, 2, 2, 2, 2, 2, 2, 2, 2, 2, 2, 2, 2, 2, 2, 2, 2, 2, 2, 2, 2, 3 ),
 ( 0.000000000000000000, 1.000000000000000000 ),
 ( 0.000000000000000000, 0.003787878787878787984, 0.007575757575757575968, 0.01136363636363636395, 0.01515151515151515194, 0.01893939393939393992, 0.02272727272727272790, 0.02651515151515151589, 0.03030303030303030387, 0.03409090909090908839, 0.03787878787878787984, 0.04166666666666666435, 0.04545454545454545581, 0.04924242424242424032, 0.05303030303030303177, 0.05681818181818181629, 0.06060606060606060774, 0.06439393939393939226, 0.06818181818181817677, 0.07196969696969697516, 0.07575757575757575968, 0.07954545454545454419, 0.08333333333333332871, 0.08712121212121212710, 0.09090909090909091161, 0.09469696969696969613, 0.09848484848484848064, 0.1022727272727272790, 0.1060606060606060635, 0.1098484848484848481, 0.1136363636363636326, 0.1174242424242424310, 0.1212121212121212155, 0.1250000000000000000, 0.1287878787878787845, 0.1325757575757575690, 0.1363636363636363535, 0.1401515151515151381, 0.1439393939393939503, 0.1477272727272727348, 0.1515151515151515194, 0.1553030303030303039, 0.1590909090909090884, 0.1628787878787878729, 0.1666666666666666574, 0.1704545454545454419, 0.1742424242424242542, 0.1780303030303030387, 0.1818181818181818232, 0.1856060606060606077, 0.1893939393939393923, 0.1931818181818181768, 0.1969696969696969613, 0.2007575757575757458, 0.2045454545454545581, 0.2083333333333333426, 0.2121212121212121271, 0.2159090909090909116, 0.2196969696969696961, 0.2234848484848484806, 0.2272727272727272652, 0.2310606060606060497, 0.2348484848484848619, 0.2386363636363636465, 0.2424242424242424310, 0.2462121212121212155, 0.2500000000000000000, 0.2537878787878787845, 0.2575757575757575690, 0.2613636363636363535, 0.2651515151515151381, 0.2689393939393939226, 0.2727272727272727071, 0.2765151515151514916, 0.2803030303030302761, 0.2840909090909091161, 0.2878787878787879007, 0.2916666666666666852, 0.2954545454545454697, 0.2992424242424242542, 0.3030303030303030387, 0.3068181818181818232, 0.3106060606060606077, 0.3143939393939393923, 0.3181818181818181768, 0.3219696969696969613, 0.3257575757575757458, 0.3295454545454545303, 0.3333333333333333148, 0.3371212121212120993, 0.3409090909090908839, 0.3446969696969697239, 0.3484848484848485084, 0.3522727272727272929, 0.3560606060606060774, 0.3598484848484848619, 0.3636363636363636465, 0.3674242424242424310, 0.3712121212121212155, 0.3750000000000000000, 0.3787878787878787845, 0.3825757575757575690, 0.3863636363636363535, 0.3901515151515151381, 0.3939393939393939226, 0.3977272727272727071, 0.4015151515151514916, 0.4053030303030302761, 0.4090909090909091161, 0.4128787878787879007, 0.4166666666666666852, 0.4204545454545454697, 0.4242424242424242542, 0.4280303030303030387, 0.4318181818181818232, 0.4356060606060606077, 0.4393939393939393923, 0.4431818181818181768, 0.4469696969696969613, 0.4507575757575757458, 0.4545454545454545303, 0.4583333333333333148, 0.4621212121212120993, 0.4659090909090908839, 0.4696969696969697239, 0.4734848484848485084, 0.4772727272727272929, 0.4810606060606060774, 0.4848484848484848619, 0.4886363636363636465, 0.4924242424242424310, 0.4962121212121212155, 0.5000000000000000000, 0.5037878787878787845, 0.5075757575757575690, 0.5113636363636363535, 0.5151515151515151381, 0.5189393939393939226, 0.5227272727272727071, 0.5265151515151514916, 0.5303030303030302761, 0.5340909090909090606, 0.5378787878787878451, 0.5416666666666666297, 0.5454545454545454142, 0.5492424242424241987, 0.5530303030303029832, 0.5568181818181817677, 0.5606060606060605522, 0.5643939393939394478, 0.5681818181818182323, 0.5719696969696970168, 0.5757575757575758013, 0.5795454545454545858, 0.5833333333333333703, 0.5871212121212121549, 0.5909090909090909394, 0.5946969696969697239, 0.5984848484848485084, 0.6022727272727272929, 0.6060606060606060774, 0.6098484848484848619, 0.6136363636363636465, 0.6174242424242424310, 0.6212121212121212155, 0.6250000000000000000, 0.6287878787878787845, 0.6325757575757575690, 0.6363636363636363535, 0.6401515151515151381, 0.6439393939393939226, 0.6477272727272727071, 0.6515151515151514916, 0.6553030303030302761, 0.6590909090909090606, 0.6628787878787878451, 0.6666666666666666297, 0.6704545454545454142, 0.6742424242424241987, 0.6780303030303029832, 0.6818181818181817677, 0.6856060606060605522, 0.6893939393939394478, 0.6931818181818182323, 0.6969696969696970168, 0.7007575757575758013, 0.7045454545454545858, 0.7083333333333333703, 0.7121212121212121549, 0.7159090909090909394, 0.7196969696969697239, 0.7234848484848485084, 0.7272727272727272929, 0.7310606060606060774, 0.7348484848484848619, 0.7386363636363636465, 0.7424242424242424310, 0.7462121212121212155, 0.7500000000000000000, 0.7537878787878787845, 0.7575757575757575690, 0.7613636363636363535, 0.7651515151515151381, 0.7689393939393939226, 0.7727272727272727071, 0.7765151515151514916, 0.7803030303030302761, 0.7840909090909090606, 0.7878787878787878451, 0.7916666666666666297, 0.7954545454545454142, 0.7992424242424241987, 0.8030303030303029832, 0.8068181818181817677, 0.8106060606060605522, 0.8143939393939394478, 0.8181818181818182323, 0.8219696969696970168, 0.8257575757575758013, 0.8295454545454545858, 0.8333333333333333703, 0.8371212121212121549, 0.8409090909090909394, 0.8446969696969697239, 0.8484848484848485084, 0.8522727272727272929, 0.8560606060606060774, 0.8598484848484848619, 0.8636363636363636465, 0.8674242424242424310, 0.8712121212121212155, 0.8750000000000000000, 0.8787878787878787845, 0.8825757575757575690, 0.8863636363636363535, 0.8901515151515151381, 0.8939393939393939226, 0.8977272727272727071, 0.9015151515151514916, 0.9053030303030302761, 0.9090909090909090606, 0.9128787878787878451, 0.9166666666666666297, 0.9204545454545454142, 0.9242424242424241987, 0.9280303030303029832, 0.9318181818181817677, 0.9356060606060605522, 0.9393939393939394478, 0.9431818181818182323, 0.9469696969696970168, 0.9507575757575758013, 0.9545454545454545858, 0.9583333333333333703, 0.9621212121212121549, 0.9659090909090909394 ),
 .UNSPECIFIED. ) 
 GEOMETRIC_REPRESENTATION_ITEM ( )  RATIONAL_B_SPLINE_SURFACE ( (
 ( 1.000000000000000000, 0.9659258262890683122, 1.000000000000000000, 0.9659258262890683122, 1.000000000000000000, 0.9659258262890683122, 1.000000000000000000, 0.9659258262890683122, 1.000000000000000000, 0.9659258262890683122, 1.000000000000000000, 0.9659258262890683122, 1.000000000000000000, 0.9659258262890683122, 1.000000000000000000, 0.9659258262890683122, 1.000000000000000000, 0.9659258262890683122, 1.000000000000000000, 0.9659258262890683122, 1.000000000000000000, 0.9659258262890683122, 1.000000000000000000, 0.9659258262890683122, 1.000000000000000000, 0.9659258262890683122, 1.000000000000000000, 0.9659258262890683122, 1.000000000000000000, 0.9659258262890683122, 1.000000000000000000, 0.9659258262890683122, 1.000000000000000000, 0.9659258262890683122, 1.000000000000000000, 0.9659258262890683122, 1.000000000000000000, 0.9659258262890683122, 1.000000000000000000, 0.9659258262890683122, 1.000000000000000000, 0.9659258262890683122, 1.000000000000000000, 0.9659258262890683122, 1.000000000000000000, 0.9659258262890683122, 1.000000000000000000, 0.9659258262890683122, 1.000000000000000000, 0.9659258262890683122, 1.000000000000000000, 0.9659258262890683122, 1.000000000000000000, 0.9659258262890683122, 1.000000000000000000, 0.9659258262890683122, 1.000000000000000000, 0.9659258262890683122, 1.000000000000000000, 0.9659258262890683122, 1.000000000000000000, 0.9659258262890683122, 1.000000000000000000, 0.9659258262890683122, 1.000000000000000000, 0.9659258262890683122, 1.000000000000000000, 0.9659258262890683122, 1.000000000000000000, 0.9659258262890683122, 1.000000000000000000, 0.9659258262890683122, 1.000000000000000000, 0.9659258262890683122, 1.000000000000000000, 0.9659258262890683122, 1.000000000000000000, 0.9659258262890683122, 1.000000000000000000, 0.9659258262890683122, 1.000000000000000000, 0.9659258262890683122, 1.000000000000000000, 0.9659258262890683122, 1.000000000000000000, 0.9659258262890683122, 1.000000000000000000, 0.9659258262890683122, 1.000000000000000000, 0.9659258262890683122, 1.000000000000000000, 0.9659258262890683122, 1.000000000000000000, 0.9659258262890683122, 1.000000000000000000, 0.9659258262890683122, 1.000000000000000000, 0.9659258262890683122, 1.000000000000000000, 0.9659258262890683122, 1.000000000000000000, 0.9659258262890683122, 1.000000000000000000, 0.9659258262890683122, 1.000000000000000000, 0.9659258262890683122, 1.000000000000000000, 0.9659258262890683122, 1.000000000000000000, 0.9659258262890683122, 1.000000000000000000, 0.9659258262890683122, 1.000000000000000000, 0.9659258262890683122, 1.000000000000000000, 0.9659258262890683122, 1.000000000000000000, 0.9659258262890683122, 1.000000000000000000, 0.9659258262890683122, 1.000000000000000000, 0.9659258262890683122, 1.000000000000000000, 0.9659258262890683122, 1.000000000000000000, 0.9659258262890683122, 1.000000000000000000, 0.9659258262890683122, 1.000000000000000000, 0.9659258262890683122, 1.000000000000000000, 0.9659258262890683122, 1.000000000000000000, 0.9659258262890683122, 1.000000000000000000, 0.9659258262890683122, 1.000000000000000000, 0.9659258262890683122, 1.000000000000000000, 0.9659258262890683122, 1.000000000000000000, 0.9659258262890683122, 1.000000000000000000, 0.9659258262890683122, 1.000000000000000000, 0.9659258262890683122, 1.000000000000000000, 0.9659258262890683122, 1.000000000000000000, 0.9659258262890683122, 1.000000000000000000, 0.9659258262890683122, 1.000000000000000000, 0.9659258262890683122, 1.000000000000000000, 0.9659258262890683122, 1.000000000000000000, 0.9659258262890683122, 1.000000000000000000, 0.9659258262890683122, 1.000000000000000000, 0.9659258262890683122, 1.000000000000000000, 0.9659258262890683122, 1.000000000000000000, 0.9659258262890683122, 1.000000000000000000, 0.9659258262890683122, 1.000000000000000000, 0.9659258262890683122, 1.000000000000000000, 0.9659258262890683122, 1.000000000000000000, 0.9659258262890683122, 1.000000000000000000, 0.9659258262890683122, 1.000000000000000000, 0.9659258262890683122, 1.000000000000000000, 0.9659258262890683122, 1.000000000000000000, 0.9659258262890683122, 1.000000000000000000, 0.9659258262890683122, 1.000000000000000000, 0.9659258262890683122, 1.000000000000000000, 0.9659258262890683122, 1.000000000000000000, 0.9659258262890683122, 1.000000000000000000, 0.9659258262890683122, 1.000000000000000000, 0.9659258262890683122, 1.000000000000000000, 0.9659258262890683122, 1.000000000000000000, 0.9659258262890683122, 1.000000000000000000, 0.9659258262890683122, 1.000000000000000000, 0.9659258262890683122, 1.000000000000000000, 0.9659258262890683122, 1.000000000000000000, 0.9659258262890683122, 1.000000000000000000, 0.9659258262890683122, 1.000000000000000000, 0.9659258262890683122, 1.000000000000000000, 0.9659258262890683122, 1.000000000000000000, 0.9659258262890683122, 1.000000000000000000, 0.9659258262890683122, 1.000000000000000000, 0.9659258262890683122, 1.000000000000000000, 0.9659258262890683122, 1.000000000000000000, 0.9659258262890683122, 1.000000000000000000, 0.9659258262890683122, 1.000000000000000000, 0.9659258262890683122, 1.000000000000000000, 0.9659258262890683122, 1.000000000000000000, 0.9659258262890683122, 1.000000000000000000, 0.9659258262890683122, 1.000000000000000000, 0.9659258262890683122, 1.000000000000000000, 0.9659258262890683122, 1.000000000000000000, 0.9659258262890683122, 1.000000000000000000, 0.9659258262890683122, 1.000000000000000000, 0.9659258262890683122, 1.000000000000000000, 0.9659258262890683122, 1.000000000000000000, 0.9659258262890683122, 1.000000000000000000, 0.9659258262890683122, 1.000000000000000000, 0.9659258262890683122, 1.000000000000000000, 0.9659258262890683122, 1.000000000000000000, 0.9659258262890683122, 1.000000000000000000, 0.9659258262890683122, 1.000000000000000000, 0.9659258262890683122, 1.000000000000000000, 0.9659258262890683122, 1.000000000000000000, 0.9659258262890683122, 1.000000000000000000, 0.9659258262890683122, 1.000000000000000000, 0.9659258262890683122, 1.000000000000000000, 0.9659258262890683122, 1.000000000000000000, 0.9659258262890683122, 1.000000000000000000, 0.9659258262890683122, 1.000000000000000000, 0.9659258262890683122, 1.000000000000000000, 0.9659258262890683122, 1.000000000000000000, 0.9659258262890683122, 1.000000000000000000, 0.9659258262890683122, 1.000000000000000000, 0.9659258262890683122, 1.000000000000000000, 0.9659258262890683122, 1.000000000000000000, 0.9659258262890683122, 1.000000000000000000, 0.9659258262890683122, 1.000000000000000000, 0.9659258262890683122, 1.000000000000000000, 0.9659258262890683122, 1.000000000000000000, 0.9659258262890683122, 1.000000000000000000, 0.9659258262890683122, 1.000000000000000000, 0.9659258262890683122, 1.000000000000000000, 0.9659258262890683122, 1.000000000000000000, 0.9659258262890683122, 1.000000000000000000, 0.9659258262890683122, 1.000000000000000000, 0.9659258262890683122, 1.000000000000000000, 0.9659258262890683122, 1.000000000000000000, 0.9659258262890683122, 1.000000000000000000, 0.9659258262890683122, 1.000000000000000000, 0.9659258262890683122, 1.000000000000000000, 0.9659258262890683122, 1.000000000000000000, 0.9659258262890683122, 1.000000000000000000, 0.9659258262890683122, 1.000000000000000000, 0.9659258262890683122, 1.000000000000000000, 0.9659258262890683122, 1.000000000000000000, 0.9659258262890683122, 1.000000000000000000, 0.9659258262890683122, 1.000000000000000000, 0.9659258262890683122, 1.000000000000000000, 0.9659258262890683122, 1.000000000000000000, 0.9659258262890683122, 1.000000000000000000, 0.9659258262890683122, 1.000000000000000000, 0.9659258262890683122, 1.000000000000000000, 0.9659258262890683122, 1.000000000000000000, 0.9659258262890683122, 1.000000000000000000, 0.9659258262890683122, 1.000000000000000000, 0.9659258262890683122, 1.000000000000000000, 0.9659258262890683122, 1.000000000000000000, 0.9659258262890683122, 1.000000000000000000, 0.9659258262890683122, 1.000000000000000000, 0.9659258262890683122, 1.000000000000000000, 0.9659258262890683122, 1.000000000000000000, 0.9659258262890683122, 1.000000000000000000, 0.9659258262890683122, 1.000000000000000000, 0.9659258262890683122, 1.000000000000000000, 0.9659258262890683122, 1.000000000000000000, 0.9659258262890683122, 1.000000000000000000, 0.9659258262890683122, 1.000000000000000000, 0.9659258262890683122, 1.000000000000000000, 0.9659258262890683122, 1.000000000000000000, 0.9659258262890683122, 1.000000000000000000, 0.9659258262890683122, 1.000000000000000000, 0.9659258262890683122, 1.000000000000000000, 0.9659258262890683122, 1.000000000000000000, 0.9659258262890683122, 1.000000000000000000, 0.9659258262890683122, 1.000000000000000000, 0.9659258262890683122, 1.000000000000000000, 0.9659258262890683122, 1.000000000000000000, 0.9659258262890683122, 1.000000000000000000, 0.9659258262890683122, 1.000000000000000000, 0.9659258262890683122, 1.000000000000000000, 0.9659258262890683122, 1.000000000000000000, 0.9659258262890683122, 1.000000000000000000, 0.9659258262890683122, 1.000000000000000000, 0.9659258262890683122, 1.000000000000000000, 0.9659258262890683122, 1.000000000000000000, 0.9659258262890683122, 1.000000000000000000, 0.9659258262890683122, 1.000000000000000000, 0.9659258262890683122, 1.000000000000000000, 0.9659258262890683122, 1.000000000000000000, 0.9659258262890683122, 1.000000000000000000, 0.9659258262890683122, 1.000000000000000000, 0.9659258262890683122, 1.000000000000000000, 0.9659258262890683122, 1.000000000000000000, 0.9659258262890683122, 1.000000000000000000, 0.9659258262890683122, 1.000000000000000000, 0.9659258262890683122, 1.000000000000000000, 0.9659258262890683122, 1.000000000000000000, 0.9659258262890683122, 1.000000000000000000, 0.9659258262890683122, 1.000000000000000000, 0.9659258262890683122, 1.000000000000000000, 0.9659258262890683122, 1.000000000000000000, 0.9659258262890683122, 1.000000000000000000, 0.9659258262890683122, 1.000000000000000000, 0.9659258262890683122, 1.000000000000000000, 0.9659258262890683122, 1.000000000000000000, 0.9659258262890683122, 1.000000000000000000, 0.9659258262890683122, 1.000000000000000000, 0.9659258262890683122, 1.000000000000000000, 0.9659258262890683122, 1.000000000000000000, 0.9659258262890683122, 1.000000000000000000, 0.9659258262890683122, 1.000000000000000000, 0.9659258262890683122, 1.000000000000000000, 0.9659258262890683122, 1.000000000000000000, 0.9659258262890683122, 1.000000000000000000, 0.9659258262890683122, 1.000000000000000000, 0.9659258262890683122, 1.000000000000000000, 0.9659258262890683122, 1.000000000000000000, 0.9659258262890683122, 1.000000000000000000, 0.9659258262890683122, 1.000000000000000000, 0.9659258262890683122, 1.000000000000000000, 0.9659258262890683122, 1.000000000000000000, 0.9659258262890683122, 1.000000000000000000, 0.9659258262890683122, 1.000000000000000000, 0.9659258262890683122, 1.000000000000000000, 0.9659258262890683122, 1.000000000000000000, 0.9659258262890683122, 1.000000000000000000, 0.9659258262890683122, 1.000000000000000000, 0.9659258262890683122, 1.000000000000000000, 0.9659258262890683122, 1.000000000000000000, 0.9659258262890683122, 1.000000000000000000, 0.9659258262890683122, 1.000000000000000000, 0.9659258262890683122, 1.000000000000000000, 0.9659258262890683122, 1.000000000000000000, 0.9659258262890683122, 1.000000000000000000, 0.9659258262890683122, 1.000000000000000000, 0.9659258262890683122, 1.000000000000000000, 0.9659258262890683122, 1.000000000000000000, 0.9659258262890683122, 1.000000000000000000),
 ( 1.000000000000000000, 0.9659258262890683122, 1.000000000000000000, 0.9659258262890683122, 1.000000000000000000, 0.9659258262890683122, 1.000000000000000000, 0.9659258262890683122, 1.000000000000000000, 0.9659258262890683122, 1.000000000000000000, 0.9659258262890683122, 1.000000000000000000, 0.9659258262890683122, 1.000000000000000000, 0.9659258262890683122, 1.000000000000000000, 0.9659258262890683122, 1.000000000000000000, 0.9659258262890683122, 1.000000000000000000, 0.9659258262890683122, 1.000000000000000000, 0.9659258262890683122, 1.000000000000000000, 0.9659258262890683122, 1.000000000000000000, 0.9659258262890683122, 1.000000000000000000, 0.9659258262890683122, 1.000000000000000000, 0.9659258262890683122, 1.000000000000000000, 0.9659258262890683122, 1.000000000000000000, 0.9659258262890683122, 1.000000000000000000, 0.9659258262890683122, 1.000000000000000000, 0.9659258262890683122, 1.000000000000000000, 0.9659258262890683122, 1.000000000000000000, 0.9659258262890683122, 1.000000000000000000, 0.9659258262890683122, 1.000000000000000000, 0.9659258262890683122, 1.000000000000000000, 0.9659258262890683122, 1.000000000000000000, 0.9659258262890683122, 1.000000000000000000, 0.9659258262890683122, 1.000000000000000000, 0.9659258262890683122, 1.000000000000000000, 0.9659258262890683122, 1.000000000000000000, 0.9659258262890683122, 1.000000000000000000, 0.9659258262890683122, 1.000000000000000000, 0.9659258262890683122, 1.000000000000000000, 0.9659258262890683122, 1.000000000000000000, 0.9659258262890683122, 1.000000000000000000, 0.9659258262890683122, 1.000000000000000000, 0.9659258262890683122, 1.000000000000000000, 0.9659258262890683122, 1.000000000000000000, 0.9659258262890683122, 1.000000000000000000, 0.9659258262890683122, 1.000000000000000000, 0.9659258262890683122, 1.000000000000000000, 0.9659258262890683122, 1.000000000000000000, 0.9659258262890683122, 1.000000000000000000, 0.9659258262890683122, 1.000000000000000000, 0.9659258262890683122, 1.000000000000000000, 0.9659258262890683122, 1.000000000000000000, 0.9659258262890683122, 1.000000000000000000, 0.9659258262890683122, 1.000000000000000000, 0.9659258262890683122, 1.000000000000000000, 0.9659258262890683122, 1.000000000000000000, 0.9659258262890683122, 1.000000000000000000, 0.9659258262890683122, 1.000000000000000000, 0.9659258262890683122, 1.000000000000000000, 0.9659258262890683122, 1.000000000000000000, 0.9659258262890683122, 1.000000000000000000, 0.9659258262890683122, 1.000000000000000000, 0.9659258262890683122, 1.000000000000000000, 0.9659258262890683122, 1.000000000000000000, 0.9659258262890683122, 1.000000000000000000, 0.9659258262890683122, 1.000000000000000000, 0.9659258262890683122, 1.000000000000000000, 0.9659258262890683122, 1.000000000000000000, 0.9659258262890683122, 1.000000000000000000, 0.9659258262890683122, 1.000000000000000000, 0.9659258262890683122, 1.000000000000000000, 0.9659258262890683122, 1.000000000000000000, 0.9659258262890683122, 1.000000000000000000, 0.9659258262890683122, 1.000000000000000000, 0.9659258262890683122, 1.000000000000000000, 0.9659258262890683122, 1.000000000000000000, 0.9659258262890683122, 1.000000000000000000, 0.9659258262890683122, 1.000000000000000000, 0.9659258262890683122, 1.000000000000000000, 0.9659258262890683122, 1.000000000000000000, 0.9659258262890683122, 1.000000000000000000, 0.9659258262890683122, 1.000000000000000000, 0.9659258262890683122, 1.000000000000000000, 0.9659258262890683122, 1.000000000000000000, 0.9659258262890683122, 1.000000000000000000, 0.9659258262890683122, 1.000000000000000000, 0.9659258262890683122, 1.000000000000000000, 0.9659258262890683122, 1.000000000000000000, 0.9659258262890683122, 1.000000000000000000, 0.9659258262890683122, 1.000000000000000000, 0.9659258262890683122, 1.000000000000000000, 0.9659258262890683122, 1.000000000000000000, 0.9659258262890683122, 1.000000000000000000, 0.9659258262890683122, 1.000000000000000000, 0.9659258262890683122, 1.000000000000000000, 0.9659258262890683122, 1.000000000000000000, 0.9659258262890683122, 1.000000000000000000, 0.9659258262890683122, 1.000000000000000000, 0.9659258262890683122, 1.000000000000000000, 0.9659258262890683122, 1.000000000000000000, 0.9659258262890683122, 1.000000000000000000, 0.9659258262890683122, 1.000000000000000000, 0.9659258262890683122, 1.000000000000000000, 0.9659258262890683122, 1.000000000000000000, 0.9659258262890683122, 1.000000000000000000, 0.9659258262890683122, 1.000000000000000000, 0.9659258262890683122, 1.000000000000000000, 0.9659258262890683122, 1.000000000000000000, 0.9659258262890683122, 1.000000000000000000, 0.9659258262890683122, 1.000000000000000000, 0.9659258262890683122, 1.000000000000000000, 0.9659258262890683122, 1.000000000000000000, 0.9659258262890683122, 1.000000000000000000, 0.9659258262890683122, 1.000000000000000000, 0.9659258262890683122, 1.000000000000000000, 0.9659258262890683122, 1.000000000000000000, 0.9659258262890683122, 1.000000000000000000, 0.9659258262890683122, 1.000000000000000000, 0.9659258262890683122, 1.000000000000000000, 0.9659258262890683122, 1.000000000000000000, 0.9659258262890683122, 1.000000000000000000, 0.9659258262890683122, 1.000000000000000000, 0.9659258262890683122, 1.000000000000000000, 0.9659258262890683122, 1.000000000000000000, 0.9659258262890683122, 1.000000000000000000, 0.9659258262890683122, 1.000000000000000000, 0.9659258262890683122, 1.000000000000000000, 0.9659258262890683122, 1.000000000000000000, 0.9659258262890683122, 1.000000000000000000, 0.9659258262890683122, 1.000000000000000000, 0.9659258262890683122, 1.000000000000000000, 0.9659258262890683122, 1.000000000000000000, 0.9659258262890683122, 1.000000000000000000, 0.9659258262890683122, 1.000000000000000000, 0.9659258262890683122, 1.000000000000000000, 0.9659258262890683122, 1.000000000000000000, 0.9659258262890683122, 1.000000000000000000, 0.9659258262890683122, 1.000000000000000000, 0.9659258262890683122, 1.000000000000000000, 0.9659258262890683122, 1.000000000000000000, 0.9659258262890683122, 1.000000000000000000, 0.9659258262890683122, 1.000000000000000000, 0.9659258262890683122, 1.000000000000000000, 0.9659258262890683122, 1.000000000000000000, 0.9659258262890683122, 1.000000000000000000, 0.9659258262890683122, 1.000000000000000000, 0.9659258262890683122, 1.000000000000000000, 0.9659258262890683122, 1.000000000000000000, 0.9659258262890683122, 1.000000000000000000, 0.9659258262890683122, 1.000000000000000000, 0.9659258262890683122, 1.000000000000000000, 0.9659258262890683122, 1.000000000000000000, 0.9659258262890683122, 1.000000000000000000, 0.9659258262890683122, 1.000000000000000000, 0.9659258262890683122, 1.000000000000000000, 0.9659258262890683122, 1.000000000000000000, 0.9659258262890683122, 1.000000000000000000, 0.9659258262890683122, 1.000000000000000000, 0.9659258262890683122, 1.000000000000000000, 0.9659258262890683122, 1.000000000000000000, 0.9659258262890683122, 1.000000000000000000, 0.9659258262890683122, 1.000000000000000000, 0.9659258262890683122, 1.000000000000000000, 0.9659258262890683122, 1.000000000000000000, 0.9659258262890683122, 1.000000000000000000, 0.9659258262890683122, 1.000000000000000000, 0.9659258262890683122, 1.000000000000000000, 0.9659258262890683122, 1.000000000000000000, 0.9659258262890683122, 1.000000000000000000, 0.9659258262890683122, 1.000000000000000000, 0.9659258262890683122, 1.000000000000000000, 0.9659258262890683122, 1.000000000000000000, 0.9659258262890683122, 1.000000000000000000, 0.9659258262890683122, 1.000000000000000000, 0.9659258262890683122, 1.000000000000000000, 0.9659258262890683122, 1.000000000000000000, 0.9659258262890683122, 1.000000000000000000, 0.9659258262890683122, 1.000000000000000000, 0.9659258262890683122, 1.000000000000000000, 0.9659258262890683122, 1.000000000000000000, 0.9659258262890683122, 1.000000000000000000, 0.9659258262890683122, 1.000000000000000000, 0.9659258262890683122, 1.000000000000000000, 0.9659258262890683122, 1.000000000000000000, 0.9659258262890683122, 1.000000000000000000, 0.9659258262890683122, 1.000000000000000000, 0.9659258262890683122, 1.000000000000000000, 0.9659258262890683122, 1.000000000000000000, 0.9659258262890683122, 1.000000000000000000, 0.9659258262890683122, 1.000000000000000000, 0.9659258262890683122, 1.000000000000000000, 0.9659258262890683122, 1.000000000000000000, 0.9659258262890683122, 1.000000000000000000, 0.9659258262890683122, 1.000000000000000000, 0.9659258262890683122, 1.000000000000000000, 0.9659258262890683122, 1.000000000000000000, 0.9659258262890683122, 1.000000000000000000, 0.9659258262890683122, 1.000000000000000000, 0.9659258262890683122, 1.000000000000000000, 0.9659258262890683122, 1.000000000000000000, 0.9659258262890683122, 1.000000000000000000, 0.9659258262890683122, 1.000000000000000000, 0.9659258262890683122, 1.000000000000000000, 0.9659258262890683122, 1.000000000000000000, 0.9659258262890683122, 1.000000000000000000, 0.9659258262890683122, 1.000000000000000000, 0.9659258262890683122, 1.000000000000000000, 0.9659258262890683122, 1.000000000000000000, 0.9659258262890683122, 1.000000000000000000, 0.9659258262890683122, 1.000000000000000000, 0.9659258262890683122, 1.000000000000000000, 0.9659258262890683122, 1.000000000000000000, 0.9659258262890683122, 1.000000000000000000, 0.9659258262890683122, 1.000000000000000000, 0.9659258262890683122, 1.000000000000000000, 0.9659258262890683122, 1.000000000000000000, 0.9659258262890683122, 1.000000000000000000, 0.9659258262890683122, 1.000000000000000000, 0.9659258262890683122, 1.000000000000000000, 0.9659258262890683122, 1.000000000000000000, 0.9659258262890683122, 1.000000000000000000, 0.9659258262890683122, 1.000000000000000000, 0.9659258262890683122, 1.000000000000000000, 0.9659258262890683122, 1.000000000000000000, 0.9659258262890683122, 1.000000000000000000, 0.9659258262890683122, 1.000000000000000000, 0.9659258262890683122, 1.000000000000000000, 0.9659258262890683122, 1.000000000000000000, 0.9659258262890683122, 1.000000000000000000, 0.9659258262890683122, 1.000000000000000000, 0.9659258262890683122, 1.000000000000000000, 0.9659258262890683122, 1.000000000000000000, 0.9659258262890683122, 1.000000000000000000, 0.9659258262890683122, 1.000000000000000000, 0.9659258262890683122, 1.000000000000000000, 0.9659258262890683122, 1.000000000000000000, 0.9659258262890683122, 1.000000000000000000, 0.9659258262890683122, 1.000000000000000000, 0.9659258262890683122, 1.000000000000000000, 0.9659258262890683122, 1.000000000000000000, 0.9659258262890683122, 1.000000000000000000, 0.9659258262890683122, 1.000000000000000000, 0.9659258262890683122, 1.000000000000000000, 0.9659258262890683122, 1.000000000000000000, 0.9659258262890683122, 1.000000000000000000, 0.9659258262890683122, 1.000000000000000000, 0.9659258262890683122, 1.000000000000000000, 0.9659258262890683122, 1.000000000000000000, 0.9659258262890683122, 1.000000000000000000, 0.9659258262890683122, 1.000000000000000000, 0.9659258262890683122, 1.000000000000000000, 0.9659258262890683122, 1.000000000000000000, 0.9659258262890683122, 1.000000000000000000, 0.9659258262890683122, 1.000000000000000000, 0.9659258262890683122, 1.000000000000000000, 0.9659258262890683122, 1.000000000000000000, 0.9659258262890683122, 1.000000000000000000, 0.9659258262890683122, 1.000000000000000000, 0.9659258262890683122, 1.000000000000000000, 0.9659258262890683122, 1.000000000000000000, 0.9659258262890683122, 1.000000000000000000, 0.9659258262890683122, 1.000000000000000000) ) ) 
 REPRESENTATION_ITEM ( '' )  SURFACE ( )  );
#39822=CARTESIAN_POINT ( 'NONE',  ( -0.5380577427821514602, 0.05413385826771666132, 0.4176697321401328100 ) ) ;
#39823=CARTESIAN_POINT ( 'NONE',  ( -1.541994750656167090, -0.6692913385826773087, -0.1292274648535924053 ) ) ;
#39824=CARTESIAN_POINT ( 'NONE',  ( 0.8398950131233602345, -0.6046776061558807314, 0.2411417322834647770 ) ) ;
#39826=CARTESIAN_POINT ( 'NONE',  ( -0.7426113562971992099, 2.401574803149605586, -0.5309055118110235227 ) ) ;
#39827=VECTOR ( 'NONE', #75595, 39.37007874015748143 ) ;
#39830=CARTESIAN_POINT ( 'NONE',  ( -1.358267716535432434, 0.1660481256975883668, -0.3530559997133364547 ) ) ;
#39831=CARTESIAN_POINT ( 'NONE',  ( -1.338582677165353729, -0.1870078740157479769, 0.3641732283464567677 ) ) ;
#39832=CARTESIAN_POINT ( 'NONE',  ( -1.259842519685038686, -0.1870078740157480879, -0.4822834645669291653 ) ) ;
#39834=CARTESIAN_POINT ( 'NONE',  ( 1.614173228346457378, 1.267785121476991073, -0.1372047244094476148 ) ) ;
#39835=CARTESIAN_POINT ( 'NONE',  ( -1.502624671916009680, -0.2845877964562159024, 0.3641732283464567677 ) ) ;
#39836=CARTESIAN_POINT ( 'NONE',  ( -1.154855643044618851, -0.6046776061558809534, -0.2411417322834644161 ) ) ;
#39837=CARTESIAN_POINT ( 'NONE',  ( 0.4068241469816279987, -0.4281496062992127816, -0.4176697321401328100 ) ) ;
#39838=CARTESIAN_POINT ( 'NONE',  ( -1.318897637795274802, 0.1660481256975885056, 0.3530559997133364547 ) ) ;
#39840=CARTESIAN_POINT ( 'NONE',  ( 0.4724409448818904789, -0.1870078740157479769, 0.4822834645669291653 ) ) ;
#39842=CARTESIAN_POINT ( 'NONE',  ( -0.6364829396325453192, -0.08942795157528024563, -0.3641732283464568787 ) ) ;
#39846=CARTESIAN_POINT ( 'NONE',  ( -1.581364829396324945, -0.2845877964562159024, 0.3641732283464567677 ) ) ;
#39847=CARTESIAN_POINT ( 'NONE',  ( -1.056430446194224881, 0.2952755905511810774, -0.1292274648535930714 ) ) ;
#39848=CARTESIAN_POINT ( 'NONE',  ( -1.496062992125983815, -0.1870078740157479769, 0.4822834645669291653 ) ) ;
#39850=CARTESIAN_POINT ( 'NONE',  ( -1.404199475065615932, 0.05413385826771666132, 0.4176697321401328100 ) ) ;
#39851=CARTESIAN_POINT ( 'NONE',  ( -1.397637795275589623, 0.1660481256975885056, 0.3530559997133364547 ) ) ;
#39852=CARTESIAN_POINT ( 'NONE',  ( -1.384514435695537005, -0.6692913385826773087, -0.1292274648535924053 ) ) ;
#39854=DIRECTION ( 'NONE',  ( -0.5931762764595015502, 3.423560842947300903E-15, -0.8050726085550551359 ) ) ;
#39855=CARTESIAN_POINT ( 'NONE',  ( 8.195543980992789655E-16, -0.1870078740157480601, -0.3641732283464567677 ) ) ;
#39858=CARTESIAN_POINT ( 'NONE',  ( -0.5052493438320203589, -0.5511811023622046335, 0.09757992244046803654 ) ) ;
#39859=CARTESIAN_POINT ( 'NONE',  ( -0.6955380577427815458, 0.05413385826771666132, 0.4176697321401328100 ) ) ;
#39860=CARTESIAN_POINT ( 'NONE',  ( 1.023622047244095112, -0.1870078740157480879, -0.4822834645669291653 ) ) ;
#39861=CARTESIAN_POINT ( 'NONE',  ( -1.095800524934382292, -0.3162353388693409650, -0.4822834645669289433 ) ) ;
#39863=VERTEX_POINT ( 'NONE', #79530 ) ;
#39864=CARTESIAN_POINT ( 'NONE',  ( -1.102362204724408601, -0.1870078740157480879, -0.4822834645669291653 ) ) ;
#39865=CARTESIAN_POINT ( 'NONE',  ( 0.9186351706036751663, -0.6046776061558807314, 0.2411417322834647770 ) ) ;
#39866=CARTESIAN_POINT ( 'NONE',  ( -1.463254593175852492, -0.5511811023622048555, -0.09757992244046775898 ) ) ;
#39869=EDGE_CURVE ( 'NONE', #62181, #64347, #66325, .T. ) ;
#39873=CARTESIAN_POINT ( 'NONE',  ( -0.2887139107611542133, -0.6046776061558809534, -0.2411417322834644161 ) ) ;
#39874=CARTESIAN_POINT ( 'NONE',  ( -1.633858267716534529, 0.07958543189024085140, 0.2665933059059887866 ) ) ;
#39877=CARTESIAN_POINT ( 'NONE',  ( -0.8398950131233589023, -0.6046776061558809534, -0.2411417322834644161 ) ) ;
#39879=CARTESIAN_POINT ( 'NONE',  ( -1.292650918635170010, -0.6692913385826771977, 0.1292274648535927661 ) ) ;
#39881=CARTESIAN_POINT ( 'NONE',  ( -1.108923884514435132, -0.3162353388693405765, 0.4822834645669290543 ) ) ;
#39882=CARTESIAN_POINT ( 'NONE',  ( -0.2887139107611542133, 0.2306618581243848609, 0.2411417322834645549 ) ) ;
#39884=CARTESIAN_POINT ( 'NONE',  ( 0.2690288713910767848, -0.5511811023622048555, -0.09757992244046775898 ) ) ;
#39885=CARTESIAN_POINT ( 'NONE',  ( -1.112701331685803652, -5.134928753749862370E-15, -0.4281989832122463091 ) ) ;
#39886=CARTESIAN_POINT ( 'NONE',  ( 0.1574803149606306130, -0.1870078740157480601, -0.3641732283464567677 ) ) ;
#39887=CARTESIAN_POINT ( 'NONE',  ( 1.187664041994751285, -0.2845877964562161244, -0.3641732283464567121 ) ) ;
#39888=CARTESIAN_POINT ( 'NONE',  ( 0.7874015748031503170, -0.1870078740157479769, 0.4822834645669291653 ) ) ;
#39889=CARTESIAN_POINT ( 'NONE',  ( 0.3018372703412079971, -0.004921259842519870586, -0.3153832671262229437 ) ) ;
#39891=CARTESIAN_POINT ( 'NONE',  ( -1.102362204724408601, -0.1870078740157480879, -0.4822834645669291653 ) ) ;
#39892=CARTESIAN_POINT ( 'NONE',  ( -0.09186351706036689768, -0.004921259842519870586, -0.3153832671262229437 ) ) ;
#39894=CARTESIAN_POINT ( 'NONE',  ( -0.6036745406824141069, -0.5023911411419708095, -0.1820866141732282451 ) ) ;
#39896=CARTESIAN_POINT ( 'NONE',  ( -0.03280839895013062252, 0.2952755905511810774, -0.1292274648535930714 ) ) ;
#39898=CARTESIAN_POINT ( 'NONE',  ( 0.8202099737532813073, 0.1771653543307087630, 0.09757992244046791164 ) ) ;
#39899=CARTESIAN_POINT ( 'NONE',  ( 0.1706036745406830368, -0.004921259842519576551, 0.3153832671262227771 ) ) ;
#39900=CARTESIAN_POINT ( 'NONE',  ( -0.2165354330708654795, 0.1660481256975885056, 0.3530559997133364547 ) ) ;
#39902=CARTESIAN_POINT ( 'NONE',  ( -0.5643044619422565855, -0.3690944881889763329, 0.3153832671262228327 ) ) ;
#39904=CARTESIAN_POINT ( 'NONE',  ( 0.7808398950131241190, -0.05778040916215560624, -0.4822834645669293319 ) ) ;
#39905=CARTESIAN_POINT ( 'NONE',  ( -0.7217847769028863381, -0.4281496062992124485, 0.4176697321401328655 ) ) ;
#39909=CARTESIAN_POINT ( 'NONE',  ( 0.08530183727034192087, -0.2845877964562161244, -0.3641732283464567121 ) ) ;
#39910=CARTESIAN_POINT ( 'NONE',  ( -0.7349081364829387342, -0.6046776061558807314, 0.2411417322834647770 ) ) ;
#39911=CARTESIAN_POINT ( 'NONE',  ( -1.043307086614172041, -0.5400638737290844871, 0.3530559997133364547 ) ) ;
#39912=CARTESIAN_POINT ( 'NONE',  ( -1.364829396325458521, -0.5023911411419708095, 0.1820866141732285504 ) ) ;
#39914=CARTESIAN_POINT ( 'NONE',  ( -1.056430446194224881, -0.5511811023622046335, 0.09757992244046803654 ) ) ;
#39915=DIRECTION ( 'NONE',  ( -0.000000000000000000, 1.000000000000000000, -0.000000000000000000 ) ) ;
#39916=CARTESIAN_POINT ( 'NONE',  ( 0.8989501312335963501, -0.6692913385826773087, -0.1292274648535924053 ) ) ;
#39921=CARTESIAN_POINT ( 'NONE',  ( -1.706036745406823485, 0.2306618581243848609, 0.2411417322834645549 ) ) ;
#39922=CARTESIAN_POINT ( 'NONE',  ( -1.200787401574802349, 0.1660481256975883668, -0.3530559997133364547 ) ) ;
#39924=CARTESIAN_POINT ( 'NONE',  ( 1.036745406824147508, -0.4281496062992127816, -0.4176697321401328100 ) ) ;
#39926=CARTESIAN_POINT ( 'NONE',  ( 1.574803149606299746, -0.1870078740157480601, -0.3641732283464567677 ) ) ;
#39927=CARTESIAN_POINT ( 'NONE',  ( 0.5249343832021005074, -0.6046776061558807314, 0.2411417322834647770 ) ) ;
#39928=CARTESIAN_POINT ( 'NONE',  ( -0.2821522309711278487, -0.6692913385826773087, -0.1292274648535924053 ) ) ;
#39933=CARTESIAN_POINT ( 'NONE',  ( 0.6430446194225728496, -0.004921259842519576551, 0.3153832671262227771 ) ) ;
#39934=ADVANCED_FACE ( 'NONE', ( #61387 ), #37220, .F. ) ;
#39939=CARTESIAN_POINT ( 'NONE',  ( 0.01968503937007930540, 0.1660481256975885056, 0.3530559997133364547 ) ) ;
#39940=CARTESIAN_POINT ( 'NONE',  ( 1.312335958005249825, 0.2306618581243847221, -0.2411417322834647770 ) ) ;
#39941=CARTESIAN_POINT ( 'NONE',  ( 0.2821522309711292364, 0.2952755905511810774, -0.1292274648535930714 ) ) ;
#39942=CARTESIAN_POINT ( 'NONE',  ( -0.4461942257217840213, -0.5023911411419708095, -0.1820866141732282451 ) ) ;
#39943=CARTESIAN_POINT ( 'NONE',  ( 1.272965879265092637, -0.4281496062992127816, -0.4176697321401328100 ) ) ;
#39945=CARTESIAN_POINT ( 'NONE',  ( -0.7020997375328074108, -0.05778040916215522460, 0.4822834645669289988 ) ) ;
#39946=CARTESIAN_POINT ( 'NONE',  ( -0.1049868766404193215, 0.2306618581243847221, -0.2411417322834647770 ) ) ;
#39947=CARTESIAN_POINT ( 'NONE',  ( 1.496062992125984703, -0.1870078740157480879, -0.4822834645669291653 ) ) ;
#39948=CARTESIAN_POINT ( 'NONE',  ( 1.167979002624672580, 0.05413385826771626580, -0.4176697321401330321 ) ) ;
#39949=CARTESIAN_POINT ( 'NONE',  ( 1.095800524934383846, -0.05778040916215560624, -0.4822834645669293319 ) ) ;
#39951=CARTESIAN_POINT ( 'NONE',  ( 0.5577427821522316087, -0.08942795157527998196, 0.3641732283464567121 ) ) ;
#39952=ORIENTED_EDGE ( 'NONE', *, *, #7540, .T. ) ;
#39955=CARTESIAN_POINT ( 'NONE',  ( -0.5971128608923877978, 0.1771653543307087630, 0.09757992244046791164 ) ) ;
#39956=CARTESIAN_POINT ( 'NONE',  ( -0.1312335958005241554, -0.6046776061558809534, -0.2411417322834644161 ) ) ;
#39958=CARTESIAN_POINT ( 'NONE',  ( -0.1049868766404193215, 0.2306618581243847221, -0.2411417322834647770 ) ) ;
#39959=CARTESIAN_POINT ( 'NONE',  ( -0.01312335958005186876, -0.4281496062992124485, 0.4176697321401328655 ) ) ;
#39960=CARTESIAN_POINT ( 'NONE',  ( -0.7611548556430438595, -0.6046776061558809534, -0.2411417322834644161 ) ) ;
#39961=CARTESIAN_POINT ( 'NONE',  ( -1.194225721784776262, 0.05413385826771626580, -0.4176697321401330321 ) ) ;
#39962=CARTESIAN_POINT ( 'NONE',  ( 1.515748031496063408, 0.07958543189024085140, 0.2665933059059887866 ) ) ;
#39963=CARTESIAN_POINT ( 'NONE',  ( -1.653543307086613234, -0.1870078740157479769, 0.4822834645669291653 ) ) ;
#39964=CARTESIAN_POINT ( 'NONE',  ( -0.1463826306659128940, -2.624320362099288585E-15, 0.3954974714151479054 ) ) ;
#39965=CARTESIAN_POINT ( 'NONE',  ( 1.023622047244095112, -0.1870078740157480601, -0.3641732283464567677 ) ) ;
#39966=CARTESIAN_POINT ( 'NONE',  ( 0.4593175853018380828, 0.05413385826771626580, -0.4176697321401330321 ) ) ;
#39967=CARTESIAN_POINT ( 'NONE',  ( 0.7939632545931766261, -0.3162353388693409650, -0.4822834645669289433 ) ) ;
#39972=CARTESIAN_POINT ( 'NONE',  ( -0.5183727034120726440, -0.6692913385826773087, -0.1292274648535924053 ) ) ;
#39975=CARTESIAN_POINT ( 'NONE',  ( -1.220472440944881054, -0.5511811023622047445, 6.969142054262312111E-17 ) ) ;
#39976=CARTESIAN_POINT ( 'NONE',  ( 1.076115485564305141, -0.6046776061558807314, 0.2411417322834647770 ) ) ;
#39977=CARTESIAN_POINT ( 'NONE',  ( 1.069553805774278832, 0.2952755905511810774, -0.1292274648535930714 ) ) ;
#39978=CARTESIAN_POINT ( 'NONE',  ( -0.2624671916010490880, -0.5023911411419708095, 0.1820866141732285504 ) ) ;
#39979=CARTESIAN_POINT ( 'NONE',  ( 0.3018372703412079971, -0.4281496062992124485, 0.4176697321401328655 ) ) ;
#39981=CARTESIAN_POINT ( 'NONE',  ( -0.2559055118110227234, -0.4536011799217367080, 0.2665933059059888421 ) ) ;
#39982=CARTESIAN_POINT ( 'NONE',  ( 0.1706036745406830368, 0.05413385826771666132, 0.4176697321401328100 ) ) ;
#39984=CARTESIAN_POINT ( 'NONE',  ( -1.299212598425196097, -0.6692913385826771977, 8.415575281601705876E-17 ) ) ;
#39985=CARTESIAN_POINT ( 'NONE',  ( 0.6889763779527563470, 0.07958543189024071263, -0.2665933059059888421 ) ) ;
#39986=CARTESIAN_POINT ( 'NONE',  ( 1.443569553805774897, -0.5023911411419708095, -0.1820866141732282451 ) ) ;
#39987=CARTESIAN_POINT ( 'NONE',  ( -0.7742782152230965886, 0.05413385826771666132, 0.4176697321401328100 ) ) ;
#39988=CARTESIAN_POINT ( 'NONE',  ( -0.3871391076115476282, -0.08942795157527998196, 0.3641732283464567121 ) ) ;
#39990=CARTESIAN_POINT ( 'NONE',  ( -0.8464566929133852113, -0.5400638737290845981, -0.3530559997133363437 ) ) ;
#39991=CARTESIAN_POINT ( 'NONE',  ( -0.7414698162729651543, -0.6692913385826771977, 0.1292274648535927661 ) ) ;
#39992=CARTESIAN_POINT ( 'NONE',  ( -0.07874015748031421014, -0.1870078740157479769, 0.4822834645669291653 ) ) ;
#39998=CARTESIAN_POINT ( 'NONE',  ( 0.5708661417322842269, 0.07958543189024085140, 0.2665933059059887866 ) ) ;
#39999=CARTESIAN_POINT ( 'NONE',  ( 1.318897637795276356, 0.1660481256975883668, -0.3530559997133364547 ) ) ;
#40000=CARTESIAN_POINT ( 'NONE',  ( -0.6824146981627291497, -0.5023911411419708095, -0.1820866141732282451 ) ) ;
#40001=CARTESIAN_POINT ( 'NONE',  ( -1.187664041994750175, -0.08942795157528024563, -0.3641732283464568787 ) ) ;
#40002=CARTESIAN_POINT ( 'NONE',  ( -0.6824146981627288167, 0.2306618581243848609, 0.2411417322834645549 ) ) ;
#40003=CARTESIAN_POINT ( 'NONE',  ( -0.3412073490813641308, -0.6046776061558807314, 0.2411417322834647770 ) ) ;
#40004=CARTESIAN_POINT ( 'NONE',  ( 0.7152230971128616943, -0.08942795157527998196, 0.3641732283464567121 ) ) ;
#40006=CARTESIAN_POINT ( 'NONE',  ( 1.003937007874016185, 0.07958543189024071263, -0.2665933059059888421 ) ) ;
#40007=CARTESIAN_POINT ( 'NONE',  ( 0.4593175853018380828, 0.05413385826771626580, -0.4176697321401330321 ) ) ;
#40009=CARTESIAN_POINT ( 'NONE',  ( -0.7939632545931754048, -0.3162353388693405765, 0.4822834645669290543 ) ) ;
#40011=CARTESIAN_POINT ( 'NONE',  ( 1.574803149606299746, -0.1870078740157479769, 0.3641732283464567677 ) ) ;
#40012=CARTESIAN_POINT ( 'NONE',  ( 0.3215223097112867578, -0.3162353388693409650, -0.4822834645669289433 ) ) ;
#40013=CARTESIAN_POINT ( 'NONE',  ( 0.03280839895013198948, -0.6692913385826773087, -0.1292274648535924053 ) ) ;
#40014=CARTESIAN_POINT ( 'NONE',  ( 0.09842519685039434474, 0.07958543189024085140, 0.2665933059059887866 ) ) ;
#40015=CARTESIAN_POINT ( 'NONE',  ( 0.5636006452641431075, 3.421639014772782816E-16, 0.3464511005275203726 ) ) ;
#40016=CARTESIAN_POINT ( 'NONE',  ( -0.1902887139107604098, 0.1771653543307087075, -0.09757992244046823083 ) ) ;
#40017=CARTESIAN_POINT ( 'NONE',  ( 0.5839895013123367340, 0.2952755905511811885, 0.1292274648535926551 ) ) ;
#40018=CARTESIAN_POINT ( 'NONE',  ( -0.5905511811023615998, 0.1771653543307087630, 0.000000000000000000 ) ) ;
#40019=CARTESIAN_POINT ( 'NONE',  ( -0.8923884514435688198, -0.6046776061558807314, 0.2411417322834647770 ) ) ;
#40021=ORIENTED_EDGE ( 'NONE', *, *, #56065, .T. ) ;
#40022=CARTESIAN_POINT ( 'NONE',  ( -1.062992125984250968, -0.6692913385826771977, 8.415575281601705876E-17 ) ) ;
#40023=CARTESIAN_POINT ( 'NONE',  ( -0.9973753280839886548, -0.5023911411419708095, -0.1820866141732282451 ) ) ;
#40024=CARTESIAN_POINT ( 'NONE',  ( -0.09842519685039295696, 0.1660481256975883668, -0.3530559997133364547 ) ) ;
#40025=CARTESIAN_POINT ( 'NONE',  ( -1.692913385826770645, 0.2952755905511811885, 0.000000000000000000 ) ) ;
#40026=CARTESIAN_POINT ( 'NONE',  ( -0.7480314960629914633, -0.6692913385826771977, 8.415575281601705876E-17 ) ) ;
#40028=CARTESIAN_POINT ( 'NONE',  ( -0.9251968503937002541, 0.1660481256975885056, 0.3530559997133364547 ) ) ;
#40029=CARTESIAN_POINT ( 'NONE',  ( 1.049868766404200127, -0.6046776061558809534, -0.2411417322834644161 ) ) ;
#40030=CARTESIAN_POINT ( 'NONE',  ( 0.9448818897637802916, -0.1870078740157480879, -0.4822834645669291653 ) ) ;
#40033=CARTESIAN_POINT ( 'NONE',  ( -1.227034120734907585, 0.2952755905511811885, 0.1292274648535926551 ) ) ;
#40037=CARTESIAN_POINT ( 'NONE',  ( -0.4527559055118102749, -0.4536011799217368745, -0.2665933059059886201 ) ) ;
#40040=CARTESIAN_POINT ( 'NONE',  ( 0.4068241469816279987, -0.4281496062992127816, -0.4176697321401328100 ) ) ;
#40041=CARTESIAN_POINT ( 'NONE',  ( -0.1246719160104980823, 0.2952755905511811885, 0.1292274648535926551 ) ) ;
#40042=CARTESIAN_POINT ( 'NONE',  ( -0.5643044619422565855, -0.4281496062992124485, 0.4176697321401328655 ) ) ;
#40043=CARTESIAN_POINT ( 'NONE',  ( 1.640419947506562393, -0.4281496062992124485, 0.4176697321401328655 ) ) ;
#40044=CARTESIAN_POINT ( 'NONE',  ( -0.9908136482939626788, 0.1771653543307087630, 0.09757992244046791164 ) ) ;
#40046=CARTESIAN_POINT ( 'NONE',  ( 0.7545931758530189937, 0.2952755905511810774, -0.1292274648535930714 ) ) ;
#40047=CARTESIAN_POINT ( 'NONE',  ( 0.6036745406824153282, -0.5023911411419708095, 0.1820866141732285504 ) ) ;
#40048=CARTESIAN_POINT ( 'NONE',  ( -0.3937007874015740483, -0.1870078740157479769, 0.4822834645669291653 ) ) ;
#40050=CARTESIAN_POINT ( 'NONE',  ( -0.8530183727034112984, 0.05413385826771666132, 0.4176697321401328100 ) ) ;
#40051=CARTESIAN_POINT ( 'NONE',  ( 1.614173228346456712, 0.7166040191147866611, 0.1372047244094478646 ) ) ;
#40052=CARTESIAN_POINT ( 'NONE',  ( 1.371391076115485941, 0.2952755905511811885, 0.1292274648535926551 ) ) ;
#40053=VERTEX_POINT ( 'NONE', #48334 ) ;
#40055=CARTESIAN_POINT ( 'NONE',  ( 0.1771653543307093182, -0.5400638737290845981, -0.3530559997133363437 ) ) ;
#40057=CARTESIAN_POINT ( 'NONE',  ( -1.371391076115484831, 0.2952755905511810774, -0.1292274648535930714 ) ) ;
#40058=CARTESIAN_POINT ( 'NONE',  ( 1.601049868766404982, 0.2306618581243848609, 0.2411417322834645549 ) ) ;
#40059=CARTESIAN_POINT ( 'NONE',  ( 1.325459317585302665, 0.05413385826771626580, -0.4176697321401330321 ) ) ;
#40060=CARTESIAN_POINT ( 'NONE',  ( 0.4199475065616803948, -0.6046776061558809534, -0.2411417322834644161 ) ) ;
#40061=CARTESIAN_POINT ( 'NONE',  ( -0.2493438320209966919, -0.4281496062992124485, 0.4176697321401328655 ) ) ;
#40063=CARTESIAN_POINT ( 'NONE',  ( -1.135170603674539924, -0.6692913385826771977, 0.1292274648535927661 ) ) ;
#40064=CARTESIAN_POINT ( 'NONE',  ( -0.4790026246719152336, -0.05778040916215560624, -0.4822834645669293319 ) ) ;
#40065=CARTESIAN_POINT ( 'NONE',  ( -0.5905511811023613777, -0.5511811023622047445, 6.969142054262312111E-17 ) ) ;
#40067=CARTESIAN_POINT ( 'NONE',  ( -0.6233595800524928121, -0.05778040916215522460, 0.4822834645669289988 ) ) ;
#40069=CARTESIAN_POINT ( 'NONE',  ( 0.7808398950131240079, -0.3162353388693405765, 0.4822834645669290543 ) ) ;
#40071=CARTESIAN_POINT ( 'NONE',  ( 0.04593175853018440641, -0.6692913385826771977, 0.1292274648535927661 ) ) ;
#40072=CARTESIAN_POINT ( 'NONE',  ( -0.4133858267716528645, 0.07958543189024071263, -0.2665933059059888421 ) ) ;
#40073=CARTESIAN_POINT ( 'NONE',  ( 0.8661417322834653598, -0.1870078740157479769, 0.3641732283464567677 ) ) ;
#40074=CARTESIAN_POINT ( 'NONE',  ( -0.8923884514435688198, 0.1539470093639521697, -0.1968503937007875793 ) ) ;
#40076=CARTESIAN_POINT ( 'NONE',  ( 0.9842519685039378130, -0.5511811023622047445, 6.969142054262312111E-17 ) ) ;
#40077=CARTESIAN_POINT ( 'NONE',  ( 1.213910761154856299, -0.6692913385826773087, -0.1292274648535924053 ) ) ;
#40080=CARTESIAN_POINT ( 'NONE',  ( 0.2296587926509192634, -0.05778040916215560624, -0.4822834645669293319 ) ) ;
#40081=CARTESIAN_POINT ( 'NONE',  ( -1.502624671916009680, -0.3162353388693405765, 0.4822834645669290543 ) ) ;
#40082=CARTESIAN_POINT ( 'NONE',  ( -1.450131233595799651, -0.6692913385826771977, 0.1292274648535927661 ) ) ;
#40083=CARTESIAN_POINT ( 'NONE',  ( -0.06561679790026180015, -0.4281496062992127816, -0.4176697321401328100 ) ) ;
#40085=CARTESIAN_POINT ( 'NONE',  ( -1.463254593175852492, 0.1771653543307087630, 0.09757992244046791164 ) ) ;
#40086=CARTESIAN_POINT ( 'NONE',  ( 0.4527559055118117182, -0.5400638737290844871, 0.3530559997133364547 ) ) ;
#40087=CARTESIAN_POINT ( 'NONE',  ( 1.056430446194226658, 0.1771653543307087630, 0.09757992244046791164 ) ) ;
#40088=CARTESIAN_POINT ( 'NONE',  ( 0.8001742991414061423, 0.004960608223778823628, 0.3437734562760190182 ) ) ;
#40089=CARTESIAN_POINT ( 'NONE',  ( 0.2624671916010504757, 0.1283753931104748280, 0.1820866141732283561 ) ) ;
#40090=CARTESIAN_POINT ( 'NONE',  ( -1.213910761154854745, -0.6692913385826771977, 0.1292274648535927661 ) ) ;
#40092=CARTESIAN_POINT ( 'NONE',  ( 1.233595800524935227, 0.2306618581243847221, -0.2411417322834647770 ) ) ;
#40094=CARTESIAN_POINT ( 'NONE',  ( 0.5183727034120741983, -0.6692913385826771977, 0.1292274648535927661 ) ) ;
#40095=CARTESIAN_POINT ( 'NONE',  ( -0.7988977408164217309, -3.187520833735697382E-15, -0.3791475997938244524 ) ) ;
#40096=CARTESIAN_POINT ( 'NONE',  ( 0.5380577427821529035, -0.004921259842519870586, -0.3153832671262229437 ) ) ;
#40097=CARTESIAN_POINT ( 'NONE',  ( 0.5511811023622055217, -0.1870078740157479769, 0.4822834645669291653 ) ) ;
#40099=CARTESIAN_POINT ( 'NONE',  ( -1.036745406824146176, -0.004921259842519870586, -0.3153832671262229437 ) ) ;
#40100=CARTESIAN_POINT ( 'NONE',  ( -1.141732283464566011, -0.6692913385826771977, 8.415575281601705876E-17 ) ) ;
#40101=CARTESIAN_POINT ( 'NONE',  ( -1.653543307086613234, -0.1870078740157480879, -0.4822834645669291653 ) ) ;
#40102=CARTESIAN_POINT ( 'NONE',  ( 0.9186351706036752773, 0.2306618581243847221, -0.2411417322834647770 ) ) ;
#40103=CARTESIAN_POINT ( 'NONE',  ( 1.601049868766404982, -0.6046776061558809534, -0.2411417322834644161 ) ) ;
#40105=CARTESIAN_POINT ( 'NONE',  ( 0.6758530183727039509, 0.2952755905511810774, -0.1292274648535930714 ) ) ;
#40109=CARTESIAN_POINT ( 'NONE',  ( 1.522309711286089939, 0.2306618581243848609, 0.2411417322834645549 ) ) ;
#40110=CARTESIAN_POINT ( 'NONE',  ( -1.587926509186350810, -0.3690944881889763329, 0.3153832671262228327 ) ) ;
#40111=CARTESIAN_POINT ( 'NONE',  ( 1.384514435695538559, 0.1771653543307087075, -0.09757992244046823083 ) ) ;
#40112=CARTESIAN_POINT ( 'NONE',  ( -1.404199475065615932, -0.3690944881889765550, -0.3153832671262227771 ) ) ;
#40113=CARTESIAN_POINT ( 'NONE',  ( -0.4199475065616791736, -0.5023911411419708095, 0.1820866141732285504 ) ) ;
#40114=CARTESIAN_POINT ( 'NONE',  ( 1.594488188976378673, 0.1660481256975885056, 0.3530559997133364547 ) ) ;
#40115=CARTESIAN_POINT ( 'NONE',  ( 0.3149606299212603933, -0.1870078740157479769, 0.3641732283464567677 ) ) ;
#40116=CARTESIAN_POINT ( 'NONE',  ( 0.4593175853018380828, 0.05413385826771626580, -0.4176697321401330321 ) ) ;
#40117=CARTESIAN_POINT ( 'NONE',  ( 0.8989501312335963501, -0.6692913385826773087, -0.1292274648535924053 ) ) ;
#40118=CARTESIAN_POINT ( 'NONE',  ( -0.1115485564304453947, -0.6692913385826771977, 0.1292274648535927661 ) ) ;
#40119=CARTESIAN_POINT ( 'NONE',  ( 0.2427821522309716595, -0.2845877964562161244, -0.3641732283464567121 ) ) ;
#40120=CARTESIAN_POINT ( 'NONE',  ( 1.253280839895013710, -0.3162353388693405765, 0.4822834645669290543 ) ) ;
#40122=CARTESIAN_POINT ( 'NONE',  ( -1.601049868766403650, 0.2306618581243847221, -0.2411417322834647770 ) ) ;
#40123=CARTESIAN_POINT ( 'NONE',  ( -0.7480314960629914633, 0.2952755905511811885, 0.000000000000000000 ) ) ;
#40124=B_SPLINE_CURVE_WITH_KNOTS ( 'NONE', 3,
 ( #80761, #22257, #23075, #67298 ),
 .UNSPECIFIED., .F., .F.,
 ( 4, 4 ),
 ( 0.000000000000000000, 0.001493228121701169198 ),
 .UNSPECIFIED. ) ;
#40127=CARTESIAN_POINT ( 'NONE',  ( 0.05905511811023681640, 0.1660481256975883668, -0.3530559997133364547 ) ) ;
#40128=CARTESIAN_POINT ( 'NONE',  ( -0.8792650918635160906, -0.4281496062992124485, 0.4176697321401328655 ) ) ;
#40129=CARTESIAN_POINT ( 'NONE',  ( 5.463695987328526437E-16, -0.1870078740157479769, 0.4822834645669291653 ) ) ;
#40135=CARTESIAN_POINT ( 'NONE',  ( -1.010498687664041384, -0.3690944881889765550, -0.3153832671262227771 ) ) ;
#40137=CARTESIAN_POINT ( 'NONE',  ( -1.725721784776902190, -0.05778040916215522460, 0.4822834645669289988 ) ) ;
#40139=CARTESIAN_POINT ( 'NONE',  ( 0.6430446194225729606, -0.4281496062992127816, -0.4176697321401328100 ) ) ;
#40140=CARTESIAN_POINT ( 'NONE',  ( -0.2952755905511804668, 0.07958543189024085140, 0.2665933059059887866 ) ) ;
#40141=CARTESIAN_POINT ( 'NONE',  ( 0.7020997375328090762, -0.05778040916215560624, -0.4822834645669293319 ) ) ;
#40142=CARTESIAN_POINT ( 'NONE',  ( 0.4265091863517067039, -0.6692913385826773087, -0.1292274648535924053 ) ) ;
#40146=CARTESIAN_POINT ( 'NONE',  ( 1.167979002624672580, -0.4281496062992124485, 0.4176697321401328655 ) ) ;
#40147=CARTESIAN_POINT ( 'NONE',  ( -0.09186351706036689768, 0.05413385826771626580, -0.4176697321401330321 ) ) ;
#40148=CARTESIAN_POINT ( 'NONE',  ( 0.3018372703412079971, -0.4281496062992124485, 0.4176697321401328655 ) ) ;
#40149=CARTESIAN_POINT ( 'NONE',  ( -1.607611548556429737, 0.2952755905511810774, -0.1292274648535930714 ) ) ;
#40150=CARTESIAN_POINT ( 'NONE',  ( 1.049868766404200349, 0.2306618581243848609, 0.2411417322834645549 ) ) ;
#40152=CARTESIAN_POINT ( 'NONE',  ( 0.01312335958005323398, 0.05413385826771666132, 0.4176697321401328100 ) ) ;
#40153=CARTESIAN_POINT ( 'NONE',  ( 0.5380577427821529035, -0.4281496062992124485, 0.4176697321401328655 ) ) ;
#40154=CARTESIAN_POINT ( 'NONE',  ( 0.09842519685039434474, 0.1660481256975885056, 0.3530559997133364547 ) ) ;
#40155=CARTESIAN_POINT ( 'NONE',  ( 1.174540682414699111, -0.2845877964562159024, 0.3641732283464567677 ) ) ;
#40156=CARTESIAN_POINT ( 'NONE',  ( -1.279527559055116948, -0.5400638737290844871, 0.3530559997133364547 ) ) ;
#40157=CARTESIAN_POINT ( 'NONE',  ( -1.233595800524933894, 0.2306618581243848609, 0.2411417322834645549 ) ) ;
#40158=CARTESIAN_POINT ( 'NONE',  ( 0.9120734908136489683, -0.6692913385826771977, 0.1292274648535927661 ) ) ;
#40161=ORIENTED_EDGE ( 'NONE', *, *, #40891, .F. ) ;
#40164=CARTESIAN_POINT ( 'NONE',  ( 1.003937007874016407, -0.5400638737290844871, 0.3530559997133364547 ) ) ;
#40165=CARTESIAN_POINT ( 'NONE',  ( 0.9514435695538062676, -0.08942795157527998196, 0.3641732283464567121 ) ) ;
#40170=CARTESIAN_POINT ( 'NONE',  ( 1.404199475065617264, -0.4281496062992124485, 0.4176697321401328655 ) ) ;
#40172=CARTESIAN_POINT ( 'NONE',  ( -0.4002624671916004129, -0.05778040916215560624, -0.4822834645669293319 ) ) ;
#40173=CARTESIAN_POINT ( 'NONE',  ( 1.253280839895013710, -0.3162353388693405765, 0.4822834645669290543 ) ) ;
#40175=CARTESIAN_POINT ( 'NONE',  ( -1.456692913385826182, -0.6692913385826771977, 8.415575281601705876E-17 ) ) ;
#40176=CARTESIAN_POINT ( 'NONE',  ( 1.614173228346456712, 1.496062992125984481, 0.1372047244094478646 ) ) ;
#40178=CARTESIAN_POINT ( 'NONE',  ( -1.646051170424378096, -0.1870078740157480046, 1.254653134982923898E-17 ) ) ;
#40180=CARTESIAN_POINT ( 'NONE',  ( -0.9120734908136475250, -0.5511811023622048555, -0.09757992244046775898 ) ) ;
#40181=CARTESIAN_POINT ( 'NONE',  ( -1.463254593175852492, 0.2952755905511811885, 0.1292274648535926551 ) ) ;
#40182=CARTESIAN_POINT ( 'NONE',  ( 0.6758530183727039509, -0.6692913385826771977, 0.1292274648535927661 ) ) ;
#40186=( BOUNDED_CURVE ( )  B_SPLINE_CURVE ( 1, ( #36692, #43404 ),
 .UNSPECIFIED., .F., .F. ) 
 B_SPLINE_CURVE_WITH_KNOTS ( ( 2, 2 ),
 ( 0.000000000000000000, 0.002000000000000003511 ),
 .UNSPECIFIED. ) 
 CURVE ( )  GEOMETRIC_REPRESENTATION_ITEM ( )  RATIONAL_B_SPLINE_CURVE ( ( 0.9875488213027523443, 0.9875488213027523443 ) ) 
 REPRESENTATION_ITEM ( '' )  );
#40187=CARTESIAN_POINT ( 'NONE',  ( 0.9580052493438327987, -0.4281496062992127816, -0.4176697321401328100 ) ) ;
#40188=CARTESIAN_POINT ( 'NONE',  ( -1.581364829396324945, -0.3162353388693405765, 0.4822834645669290543 ) ) ;
#40190=CARTESIAN_POINT ( 'NONE',  ( -0.6430446194225716283, -0.3690944881889763329, 0.3153832671262228327 ) ) ;
#40192=CARTESIAN_POINT ( 'NONE',  ( 1.614173228346457378, -0.6692913385826771977, 8.415575281601705876E-17 ) ) ;
#40193=LINE ( 'NONE', #14118, #6143 ) ;
#40194=CARTESIAN_POINT ( 'NONE',  ( 0.6627296587926515548, 0.2952755905511811885, 0.1292274648535926551 ) ) ;
#40195=CARTESIAN_POINT ( 'NONE',  ( -0.8923884514435688198, -0.5023911411419708095, 0.1820866141732285504 ) ) ;
#40196=CARTESIAN_POINT ( 'NONE',  ( -0.4855643044619415427, -0.3690944881889763329, 0.3153832671262228327 ) ) ;
#40197=CARTESIAN_POINT ( 'NONE',  ( -0.3346456692913377662, -0.5400638737290844871, 0.3530559997133364547 ) ) ;
#40198=CARTESIAN_POINT ( 'NONE',  ( -1.069553805774277722, -0.5511811023622048555, -0.09757992244046775898 ) ) ;
#40200=CARTESIAN_POINT ( 'NONE',  ( 0.8136482939632553313, 0.2306618581243848609, 0.2411417322834645549 ) ) ;
#40201=CARTESIAN_POINT ( 'NONE',  ( 0.8761506516392508770, -4.927456884911482678E-16, 0.4445507791589062840 ) ) ;
#40203=CARTESIAN_POINT ( 'NONE',  ( -0.7742782152230965886, 0.05413385826771666132, 0.4176697321401328100 ) ) ;
#40205=CARTESIAN_POINT ( 'NONE',  ( -0.05249343832020938322, -0.5023911411419708095, -0.1820866141732282451 ) ) ;
#40206=CARTESIAN_POINT ( 'NONE',  ( -1.345144356955379816, -0.3162353388693405765, 0.4822834645669290543 ) ) ;
#40207=CARTESIAN_POINT ( 'NONE',  ( 0.6758530183727039509, -0.5511811023622046335, 0.09757992244046803654 ) ) ;
#40208=CARTESIAN_POINT ( 'NONE',  ( -0.6955380577427815458, -0.3690944881889765550, -0.3153832671262227771 ) ) ;
#40209=CARTESIAN_POINT ( 'NONE',  ( -1.161417322834644716, -0.5400638737290845981, -0.3530559997133363437 ) ) ;
#40210=CARTESIAN_POINT ( 'NONE',  ( -1.653543307086613234, -0.1870078740157480879, -0.4822834645669291653 ) ) ;
#40211=CARTESIAN_POINT ( 'NONE',  ( -1.391076115485563314, -0.6046776061558809534, -0.2411417322834644161 ) ) ;
#40212=CARTESIAN_POINT ( 'NONE',  ( 1.076115485564305141, 0.1539470093639521697, -0.1968503937007875793 ) ) ;
#40213=CARTESIAN_POINT ( 'NONE',  ( 1.023622047244095334, -0.1870078740157479769, 0.3641732283464567677 ) ) ;
#40214=CARTESIAN_POINT ( 'NONE',  ( 0.3937007874015754361, -0.1870078740157479769, 0.4822834645669291653 ) ) ;
#40216=CARTESIAN_POINT ( 'NONE',  ( 1.266404199475066328, -0.08942795157527998196, 0.3641732283464567121 ) ) ;
#40217=ORIENTED_EDGE ( 'NONE', *, *, #43371, .T. ) ;
#40219=CARTESIAN_POINT ( 'NONE',  ( -1.332020997375327642, -0.08942795157527998196, 0.3641732283464567121 ) ) ;
#40220=CARTESIAN_POINT ( 'NONE',  ( -0.5839895013123351797, -0.6692913385826771977, 0.1292274648535927661 ) ) ;
#40221=CARTESIAN_POINT ( 'NONE',  ( 0.8267716535433077274, 0.2952755905511811885, 0.000000000000000000 ) ) ;
#40222=CARTESIAN_POINT ( 'NONE',  ( -1.548556430446193399, 0.1283753931104748280, 0.1820866141732283561 ) ) ;
#40224=CARTESIAN_POINT ( 'NONE',  ( -1.614173228346456268, -0.6692913385826771977, 8.415575281601705876E-17 ) ) ;
#40225=CARTESIAN_POINT ( 'NONE',  ( 0.6364829396325465405, -0.3162353388693409650, -0.4822834645669289433 ) ) ;
#40226=CARTESIAN_POINT ( 'NONE',  ( 0.3412073490813655186, -0.6046776061558809534, -0.2411417322834644161 ) ) ;
#40227=CARTESIAN_POINT ( 'NONE',  ( 1.030183727034121421, -0.3162353388693409650, -0.4822834645669289433 ) ) ;
#40232=CARTESIAN_POINT ( 'NONE',  ( 0.1706036745406830368, -0.004921259842519576551, 0.3153832671262227771 ) ) ;
#40233=CARTESIAN_POINT ( 'NONE',  ( -0.4133858267716528645, 0.1660481256975883668, -0.3530559997133364547 ) ) ;
#40234=CARTESIAN_POINT ( 'NONE',  ( 1.279527559055118724, 0.1660481256975885056, 0.3530559997133364547 ) ) ;
#40236=CARTESIAN_POINT ( 'NONE',  ( 0.2821522309711292364, 0.1771653543307087075, -0.09757992244046823083 ) ) ;
#40237=CARTESIAN_POINT ( 'NONE',  ( -0.7217847769028863381, -0.4281496062992124485, 0.4176697321401328655 ) ) ;
#40238=CARTESIAN_POINT ( 'NONE',  ( -1.627296587926508442, 0.2306618581243848609, 0.2411417322834645549 ) ) ;
#40239=CARTESIAN_POINT ( 'NONE',  ( 0.3674540682414705883, -0.6046776061558807314, 0.2411417322834647770 ) ) ;
#40241=CARTESIAN_POINT ( 'NONE',  ( 1.614173228346457378, 1.330640075373405118, 0.1372047244094478369 ) ) ;
#40244=CARTESIAN_POINT ( 'NONE',  ( 1.581364829396326277, -0.08942795157527998196, 0.3641732283464567121 ) ) ;
#40245=CARTESIAN_POINT ( 'NONE',  ( -1.082677165354329896, -0.4536011799217368745, -0.2665933059059886201 ) ) ;
#40246=CARTESIAN_POINT ( 'NONE',  ( -0.9711286089238838626, 0.2306618581243847221, -0.2411417322834647770 ) ) ;
#40248=LINE ( 'NONE', #65931, #51762 ) ;
#40249=CARTESIAN_POINT ( 'NONE',  ( 1.686351706036745890, 0.2952755905511811885, 0.1292274648535926551 ) ) ;
#40250=CARTESIAN_POINT ( 'NONE',  ( -1.377952755905511140, 0.2952755905511811885, 0.000000000000000000 ) ) ;
#40251=CARTESIAN_POINT ( 'NONE',  ( -0.08530183727034056085, -0.05778040916215560624, -0.4822834645669293319 ) ) ;
#40253=CARTESIAN_POINT ( 'NONE',  ( -1.187664041994749731, -0.3162353388693405765, 0.4822834645669290543 ) ) ;
#40255=CARTESIAN_POINT ( 'NONE',  ( 0.6430446194225728496, 0.05413385826771666132, 0.4176697321401328100 ) ) ;
#40257=CARTESIAN_POINT ( 'NONE',  ( -1.246719160104985846, -0.3690944881889765550, -0.3153832671262227771 ) ) ;
#40262=CARTESIAN_POINT ( 'NONE',  ( -0.9776902887139098386, -0.6692913385826771977, 0.1292274648535927661 ) ) ;
#40263=CARTESIAN_POINT ( 'NONE',  ( -1.489501312335957062, -0.05778040916215522460, 0.4822834645669289988 ) ) ;
#40265=CARTESIAN_POINT ( 'NONE',  ( -1.725721784776902190, -0.05778040916215522460, 0.4822834645669289988 ) ) ;
#40266=CARTESIAN_POINT ( 'NONE',  ( -0.7276493853111294374, 2.362204724409448620, 0.5105987775586408040 ) ) ;
#40267=CARTESIAN_POINT ( 'NONE',  ( -1.489501312335957062, -0.05778040916215522460, 0.4822834645669289988 ) ) ;
#40270=CARTESIAN_POINT ( 'NONE',  ( 0.03280839895013198948, -0.5511811023622048555, -0.09757992244046775898 ) ) ;
#40272=CARTESIAN_POINT ( 'NONE',  ( -0.8333333333333323711, -0.5511811023622048555, -0.09757992244046775898 ) ) ;
#40273=CARTESIAN_POINT ( 'NONE',  ( -1.154855643044618851, 0.2306618581243848609, 0.2411417322834645549 ) ) ;
#40274=CARTESIAN_POINT ( 'NONE',  ( 0.9645669291338588858, 0.1660481256975885056, 0.3530559997133364547 ) ) ;
#40275=CARTESIAN_POINT ( 'NONE',  ( -0.9842519685039360366, 0.2952755905511811885, 0.000000000000000000 ) ) ;
#40278=CARTESIAN_POINT ( 'NONE',  ( -0.8136482939632537770, 0.2306618581243847221, -0.2411417322834647770 ) ) ;
#40279=CARTESIAN_POINT ( 'NONE',  ( 1.069553805774278610, -0.6692913385826771977, 0.1292274648535927661 ) ) ;
#40280=EDGE_CURVE ( 'NONE', #33111, #40878, #39315, .T. ) ;
#40281=CARTESIAN_POINT ( 'NONE',  ( -1.653543307086613234, -0.1870078740157480601, -0.3641732283464567677 ) ) ;
#40282=CARTESIAN_POINT ( 'NONE',  ( -1.660104986876639543, -0.05778040916215560624, -0.4822834645669293319 ) ) ;
#40285=EDGE_CURVE ( 'NONE', #50981, #29775, #59237, .T. ) ;
#40288=CARTESIAN_POINT ( 'NONE',  ( -0.4921259842519677963, 0.1660481256975883668, -0.3530559997133364547 ) ) ;
#40289=CARTESIAN_POINT ( 'NONE',  ( -1.528871391076114250, -0.5511811023622046335, 0.09757992244046803654 ) ) ;
#40291=CARTESIAN_POINT ( 'NONE',  ( -1.240157480314959759, 0.1660481256975885056, 0.3530559997133364547 ) ) ;
#40292=DIRECTION ( 'NONE',  ( 0.000000000000000000, 0.000000000000000000, 1.000000000000000000 ) ) ;
#40293=CARTESIAN_POINT ( 'NONE',  ( -1.456692913385826182, -0.6692913385826771977, 8.415575281601705876E-17 ) ) ;
#40294=CARTESIAN_POINT ( 'NONE',  ( -0.5708661417322828946, 0.1660481256975883668, -0.3530559997133364547 ) ) ;
#40296=CARTESIAN_POINT ( 'NONE',  ( 0.4986876640419954376, 0.1283753931104748280, 0.1820866141732283561 ) ) ;
#40297=CARTESIAN_POINT ( 'NONE',  ( -1.113061397484513604, -4.850200619981615293E-15, -0.4118477457932993024 ) ) ;
#40298=CARTESIAN_POINT ( 'NONE',  ( 0.2493438320209980519, -0.004921259842519576551, 0.3153832671262227771 ) ) ;
#40299=CARTESIAN_POINT ( 'NONE',  ( 1.430446194225722500, -0.004921259842519576551, 0.3153832671262227771 ) ) ;
#40300=CARTESIAN_POINT ( 'NONE',  ( 0.7677165354330716118, -0.5400638737290844871, 0.3530559997133364547 ) ) ;
#40302=CARTESIAN_POINT ( 'NONE',  ( -0.03280839895013062252, 0.1771653543307087075, -0.09757992244046823083 ) ) ;
#40304=CARTESIAN_POINT ( 'NONE',  ( -1.161417322834644716, 0.1660481256975885056, 0.3530559997133364547 ) ) ;
#40305=CARTESIAN_POINT ( 'NONE',  ( 5.463695987328526437E-16, -0.1870078740157479769, 0.3641732283464567677 ) ) ;
#40306=CARTESIAN_POINT ( 'NONE',  ( -1.489501312335957062, -0.08942795157527998196, 0.3641732283464567121 ) ) ;
#40308=CARTESIAN_POINT ( 'NONE',  ( -0.3608923884514428360, 0.1771653543307087630, 0.09757992244046791164 ) ) ;
#40311=CARTESIAN_POINT ( 'NONE',  ( -0.1968503937007867743, 0.2952755905511811885, 0.000000000000000000 ) ) ;
#40313=CARTESIAN_POINT ( 'NONE',  ( 0.3674540682414705883, 0.1283753931104746893, -0.1820866141732285504 ) ) ;
#40314=CARTESIAN_POINT ( 'NONE',  ( -0.2821522309711278487, 0.1771653543307087630, 0.09757992244046791164 ) ) ;
#40315=CARTESIAN_POINT ( 'NONE',  ( -0.3674540682414689785, 0.2306618581243848609, 0.2411417322834645549 ) ) ;
#40317=CARTESIAN_POINT ( 'NONE',  ( -1.043307086614172041, -0.4536011799217367080, 0.2665933059059888421 ) ) ;
#40319=CARTESIAN_POINT ( 'NONE',  ( 0.7545931758530189937, 0.2952755905511810774, -0.1292274648535930714 ) ) ;
#40320=CARTESIAN_POINT ( 'NONE',  ( -0.8792650918635160906, -0.4281496062992124485, 0.4176697321401328655 ) ) ;
#40324=CARTESIAN_POINT ( 'NONE',  ( -0.3740157480314953431, -0.4536011799217368745, -0.2665933059059886201 ) ) ;
#40325=FACE_OUTER_BOUND ( 'NONE', #3287, .T. ) ;
#40326=CARTESIAN_POINT ( 'NONE',  ( -1.076115485564303809, -0.5023911411419708095, -0.1820866141732282451 ) ) ;
#40328=CARTESIAN_POINT ( 'NONE',  ( -0.8858267716535425107, 0.07958543189024071263, -0.2665933059059888421 ) ) ;
#40329=CARTESIAN_POINT ( 'NONE',  ( -1.091264520429692464, -2.570477104772672414E-15, 0.3954974714151479609 ) ) ;
#40330=CARTESIAN_POINT ( 'NONE',  ( 0.9317585301837276734, -0.4281496062992124485, 0.4176697321401328655 ) ) ;
#40334=CARTESIAN_POINT ( 'NONE',  ( 1.430446194225722500, -0.004921259842519576551, 0.3153832671262227771 ) ) ;
#40335=CARTESIAN_POINT ( 'NONE',  ( -1.423884514435694859, -0.3162353388693405765, 0.4822834645669290543 ) ) ;
#40337=CARTESIAN_POINT ( 'NONE',  ( 1.292650918635171564, 0.2952755905511811885, 0.1292274648535926551 ) ) ;
#40339=CARTESIAN_POINT ( 'NONE',  ( 1.568241469816273659, -0.08942795157528024563, -0.3641732283464568787 ) ) ;
#40340=CARTESIAN_POINT ( 'NONE',  ( 0.6627296587926517768, -0.6692913385826773087, -0.1292274648535924053 ) ) ;
#40341=CARTESIAN_POINT ( 'NONE',  ( -0.4461942257217840213, -0.6046776061558809534, -0.2411417322834644161 ) ) ;
#40342=CARTESIAN_POINT ( 'NONE',  ( 1.528871391076116026, 0.2952755905511811885, 0.1292274648535926551 ) ) ;
#40344=CARTESIAN_POINT ( 'NONE',  ( 0.5643044619422579178, -0.3690944881889765550, -0.3153832671262227771 ) ) ;
#40346=EDGE_LOOP ( 'NONE', ( #36735, #37259, #13156, #1948, #25514 ) ) ;
#40349=CARTESIAN_POINT ( 'NONE',  ( -0.4855643044619415427, -0.4281496062992124485, 0.4176697321401328655 ) ) ;
#40350=CARTESIAN_POINT ( 'NONE',  ( 1.325459317585302665, 0.05413385826771626580, -0.4176697321401330321 ) ) ;
#40351=CARTESIAN_POINT ( 'NONE',  ( 0.1771653543307093182, -0.5400638737290845981, -0.3530559997133363437 ) ) ;
#40352=CARTESIAN_POINT ( 'NONE',  ( -0.4855643044619415427, -0.004921259842519870586, -0.3153832671262229437 ) ) ;
#40353=CARTESIAN_POINT ( 'NONE',  ( 1.318897637795276356, -0.5400638737290844871, 0.3530559997133364547 ) ) ;
#40354=CARTESIAN_POINT ( 'NONE',  ( -1.095800524934382292, -0.3162353388693409650, -0.4822834645669289433 ) ) ;
#40355=CARTESIAN_POINT ( 'NONE',  ( 0.07874015748031558404, -0.1870078740157480879, -0.4822834645669291653 ) ) ;
#40356=CARTESIAN_POINT ( 'NONE',  ( -1.469816272965878357, 0.2306618581243848609, 0.2411417322834645549 ) ) ;
#40357=CARTESIAN_POINT ( 'NONE',  ( 0.9120734908136489683, -0.6692913385826771977, 0.1292274648535927661 ) ) ;
#40358=CARTESIAN_POINT ( 'NONE',  ( 1.325459317585302665, -0.4281496062992124485, 0.4176697321401328655 ) ) ;
#40360=CARTESIAN_POINT ( 'NONE',  ( -0.03280839895013062252, 0.1771653543307087075, -0.09757992244046823083 ) ) ;
#40361=EDGE_LOOP ( 'NONE', ( #14692, #36114, #51214, #33095 ) ) ;
#40363=EDGE_LOOP ( 'NONE', ( #17681, #6784, #49050, #70137 ) ) ;
#40364=CARTESIAN_POINT ( 'NONE',  ( -0.3412073490813641308, -0.5023911411419708095, 0.1820866141732285504 ) ) ;
#40365=CARTESIAN_POINT ( 'NONE',  ( 0.08530183727034192087, -0.05778040916215522460, 0.4822834645669289988 ) ) ;
#40367=CARTESIAN_POINT ( 'NONE',  ( -0.1640419947506555343, -0.3162353388693405765, 0.4822834645669290543 ) ) ;
#40368=CARTESIAN_POINT ( 'NONE',  ( -0.2952755905511804668, 0.1660481256975885056, 0.3530559997133364547 ) ) ;
#40369=CARTESIAN_POINT ( 'NONE',  ( -1.036745406824146176, -0.4281496062992124485, 0.4176697321401328655 ) ) ;
#40370=CARTESIAN_POINT ( 'NONE',  ( -0.9055118110236215490, 0.2952755905511811885, 0.000000000000000000 ) ) ;
#40371=CARTESIAN_POINT ( 'NONE',  ( 1.541994750656168645, 0.1771653543307087075, -0.09757992244046823083 ) ) ;
#40372=CARTESIAN_POINT ( 'NONE',  ( -1.627296587926508442, 0.2306618581243848609, 0.2411417322834645549 ) ) ;
#40373=CARTESIAN_POINT ( 'NONE',  ( 0.3215223097112867578, -0.08942795157527998196, 0.3641732283464567121 ) ) ;
#40374=CARTESIAN_POINT ( 'NONE',  ( 0.6496062992125991586, -0.5400638737290845981, -0.3530559997133363437 ) ) ;
#40375=CARTESIAN_POINT ( 'NONE',  ( 0.5052493438320218022, -0.6692913385826773087, -0.1292274648535924053 ) ) ;
#40377=CARTESIAN_POINT ( 'NONE',  ( -1.699475065616797398, 0.2952755905511811885, 0.1292274648535926551 ) ) ;
#40380=CARTESIAN_POINT ( 'NONE',  ( -0.5314960629921254842, -0.5400638737290845981, -0.3530559997133363437 ) ) ;
#40383=CARTESIAN_POINT ( 'NONE',  ( -1.358267716535432434, -0.4536011799217367080, 0.2665933059059888421 ) ) ;
#40384=CARTESIAN_POINT ( 'NONE',  ( 0.8333333333333340365, 0.2952755905511810774, -0.1292274648535930714 ) ) ;
#40385=CARTESIAN_POINT ( 'NONE',  ( 0.8727034120734913358, -0.05778040916215522460, 0.4822834645669289988 ) ) ;
#40386=CARTESIAN_POINT ( 'NONE',  ( -0.1902887139107604098, 0.1771653543307087075, -0.09757992244046823083 ) ) ;
#40387=CARTESIAN_POINT ( 'NONE',  ( 0.6561679790026253567, 0.2306618581243848609, 0.2411417322834645549 ) ) ;
#40389=CARTESIAN_POINT ( 'NONE',  ( -0.1115485564304453947, -0.5511811023622046335, 0.09757992244046803654 ) ) ;
#40390=CARTESIAN_POINT ( 'NONE',  ( 0.1049868766404206816, -0.6046776061558809534, -0.2411417322834644161 ) ) ;
#40393=CARTESIAN_POINT ( 'NONE',  ( -1.509186351706035767, 0.05413385826771626580, -0.4176697321401330321 ) ) ;
#40394=CARTESIAN_POINT ( 'NONE',  ( 0.5052493438320215802, 0.1771653543307087630, 0.09757992244046791164 ) ) ;
#40395=CARTESIAN_POINT ( 'NONE',  ( 1.640419947506562393, -0.3690944881889763329, 0.3153832671262228327 ) ) ;
#40396=CARTESIAN_POINT ( 'NONE',  ( -0.7480314960629914633, 0.2952755905511811885, 0.000000000000000000 ) ) ;
#40397=AXIS2_PLACEMENT_3D ( 'NONE', #72607, #2736, #14955 ) ;
#40398=CARTESIAN_POINT ( 'NONE',  ( -0.6364829396325453192, -0.08942795157528024563, -0.3641732283464568787 ) ) ;
#40400=CARTESIAN_POINT ( 'NONE',  ( -0.8661417322834640276, -0.1870078740157480879, -0.4822834645669291653 ) ) ;
#40401=CARTESIAN_POINT ( 'NONE',  ( -0.6955380577427815458, 0.05413385826771666132, 0.4176697321401328100 ) ) ;
#40402=CARTESIAN_POINT ( 'NONE',  ( -0.07217847769028787330, -0.05778040916215522460, 0.4822834645669289988 ) ) ;
#40406=CARTESIAN_POINT ( 'NONE',  ( 0.6692913385826778638, -0.5511811023622047445, 6.969142054262312111E-17 ) ) ;
#40407=CARTESIAN_POINT ( 'NONE',  ( 1.358267716535433323, -0.5400638737290845981, -0.3530559997133363437 ) ) ;
#40408=CARTESIAN_POINT ( 'NONE',  ( -1.181102362204723644, -0.1870078740157480601, -0.3641732283464567677 ) ) ;
#40410=CARTESIAN_POINT ( 'NONE',  ( -0.9645669291338575535, -0.4536011799217367080, 0.2665933059059888421 ) ) ;
#40411=CARTESIAN_POINT ( 'NONE',  ( -0.6167979002624665030, 0.05413385826771666132, 0.4176697321401328100 ) ) ;
#40412=CARTESIAN_POINT ( 'NONE',  ( -0.03937007874015669567, 0.1771653543307087630, 0.000000000000000000 ) ) ;
#40414=CARTESIAN_POINT ( 'NONE',  ( 0.9055118110236227702, -0.5511811023622047445, 6.969142054262312111E-17 ) ) ;
#40416=CARTESIAN_POINT ( 'NONE',  ( 0.3018372703412079971, 0.05413385826771626580, -0.4176697321401330321 ) ) ;
#40418=CARTESIAN_POINT ( 'NONE',  ( -0.7349081364829390672, 0.2306618581243847221, -0.2411417322834647770 ) ) ;
#40420=CARTESIAN_POINT ( 'NONE',  ( 1.528871391076116026, -0.5511811023622048555, -0.09757992244046775898 ) ) ;
#40421=CARTESIAN_POINT ( 'NONE',  ( 0.3740157480314966754, -0.5400638737290844871, 0.3530559997133364547 ) ) ;
#40422=CARTESIAN_POINT ( 'NONE',  ( 0.006561679790026889343, -0.3162353388693409650, -0.4822834645669289433 ) ) ;
#40423=CARTESIAN_POINT ( 'NONE',  ( 0.1509186351706045259, -0.08942795157528024563, -0.3641732283464568787 ) ) ;
#40424=CARTESIAN_POINT ( 'NONE',  ( 1.614173228346456712, 0.9921945702958890889, 0.1372047244094478646 ) ) ;
#40425=CARTESIAN_POINT ( 'NONE',  ( -0.2427821522309703550, -0.2845877964562159024, 0.3641732283464567677 ) ) ;
#40426=CARTESIAN_POINT ( 'NONE',  ( 0.7217847769028878924, 0.05413385826771666132, 0.4176697321401328100 ) ) ;
#40427=CARTESIAN_POINT ( 'NONE',  ( -0.6889763779527552368, -0.4536011799217368745, -0.2665933059059886201 ) ) ;
#40429=CARTESIAN_POINT ( 'NONE',  ( -1.102362204724408601, -0.1870078740157480879, -0.4822834645669291653 ) ) ;
#40431=EDGE_LOOP ( 'NONE', ( #82884, #52468, #33844, #50572 ) ) ;
#40432=CARTESIAN_POINT ( 'NONE',  ( -1.194225721784776262, -0.4281496062992124485, 0.4176697321401328655 ) ) ;
#40433=CARTESIAN_POINT ( 'NONE',  ( -0.9842519685039365918, -0.5511811023622047445, 6.969142054262312111E-17 ) ) ;
#40434=CARTESIAN_POINT ( 'NONE',  ( 0.05905511811023681640, 0.1660481256975883668, -0.3530559997133364547 ) ) ;
#40435=EDGE_CURVE ( 'NONE', #9917, #58735, #26205, .T. ) ;
#40436=CARTESIAN_POINT ( 'NONE',  ( -1.594488188976377563, -0.5400638737290844871, 0.3530559997133364547 ) ) ;
#40437=CARTESIAN_POINT ( 'NONE',  ( -0.8989501312335946848, -0.6692913385826771977, 0.1292274648535927661 ) ) ;
#40439=CARTESIAN_POINT ( 'NONE',  ( 1.673228346456693494, 0.1660481256975885056, 0.3530559997133364547 ) ) ;
#40440=CARTESIAN_POINT ( 'NONE',  ( 1.076115485564305141, -0.6046776061558807314, 0.2411417322834647770 ) ) ;
#40441=CARTESIAN_POINT ( 'NONE',  ( 0.8923884514435703741, 0.2306618581243848609, 0.2411417322834645549 ) ) ;
#40443=CARTESIAN_POINT ( 'NONE',  ( 1.515748031496063186, -0.5400638737290845981, -0.3530559997133363437 ) ) ;
#40444=CARTESIAN_POINT ( 'NONE',  ( -1.181102362204723644, -0.1870078740157480879, -0.4822834645669291653 ) ) ;
#40448=CARTESIAN_POINT ( 'NONE',  ( -0.6036745406824141069, -0.5023911411419708095, -0.1820866141732282451 ) ) ;
#40451=CARTESIAN_POINT ( 'NONE',  ( 0.1902887139107617975, 0.2952755905511811885, 0.1292274648535926551 ) ) ;
#40452=CARTESIAN_POINT ( 'NONE',  ( 0.07217847769028949700, -0.05778040916215560624, -0.4822834645669293319 ) ) ;
#40453=CARTESIAN_POINT ( 'NONE',  ( -0.8333333333333323711, 0.2952755905511811885, 0.1292274648535926551 ) ) ;
#40454=CARTESIAN_POINT ( 'NONE',  ( 1.338582677165355062, -0.1870078740157479769, 0.4822834645669291653 ) ) ;
#40455=CARTESIAN_POINT ( 'NONE',  ( -0.8727034120734901146, -0.2845877964562159024, 0.3641732283464567677 ) ) ;
#40456=CARTESIAN_POINT ( 'NONE',  ( -0.7461015470515859338, 2.206450217086253218, -0.5309055118110235227 ) ) ;
#40457=CARTESIAN_POINT ( 'NONE',  ( 0.5971128608923891301, 0.2952755905511810774, -0.1292274648535930714 ) ) ;
#40458=CARTESIAN_POINT ( 'NONE',  ( 0.6364829396325465405, -0.08942795157527998196, 0.3641732283464567121 ) ) ;
#40460=CARTESIAN_POINT ( 'NONE',  ( -0.5249343832020990641, 0.2306618581243848609, 0.2411417322834645549 ) ) ;
#40462=CARTESIAN_POINT ( 'NONE',  ( -1.364829396325458521, -0.6046776061558807314, 0.2411417322834647770 ) ) ;
#40463=CARTESIAN_POINT ( 'NONE',  ( -1.732283464566928277, -0.1870078740157479769, 0.3641732283464567677 ) ) ;
#40465=CARTESIAN_POINT ( 'NONE',  ( 1.397637795275591177, 0.1660481256975883668, -0.3530559997133364547 ) ) ;
#40466=CARTESIAN_POINT ( 'NONE',  ( 1.522309711286089939, 0.1283753931104748280, 0.1820866141732283561 ) ) ;
#40469=CARTESIAN_POINT ( 'NONE',  ( -0.1115485564304453947, -0.6692913385826771977, 0.1292274648535927661 ) ) ;
#40471=CARTESIAN_POINT ( 'NONE',  ( 1.003937007874016185, 0.07958543189024071263, -0.2665933059059888421 ) ) ;
#40472=CARTESIAN_POINT ( 'NONE',  ( -1.220472440944881054, 0.2952755905511811885, 0.000000000000000000 ) ) ;
#40473=CARTESIAN_POINT ( 'NONE',  ( 1.095800524934383846, -0.3162353388693405765, 0.4822834645669290543 ) ) ;
#40474=CARTESIAN_POINT ( 'NONE',  ( 1.332020997375328974, -0.05778040916215560624, -0.4822834645669293319 ) ) ;
#40475=CARTESIAN_POINT ( 'NONE',  ( 0.1246719160104994284, -0.6692913385826771977, 0.1292274648535927661 ) ) ;
#40476=CARTESIAN_POINT ( 'NONE',  ( -0.1902887139107604098, 0.2952755905511810774, -0.1292274648535930714 ) ) ;
#40478=CARTESIAN_POINT ( 'NONE',  ( -1.220472440944881054, 0.2952755905511811885, 0.000000000000000000 ) ) ;
#40479=CARTESIAN_POINT ( 'NONE',  ( -0.4396325459317577122, -0.6692913385826773087, -0.1292274648535924053 ) ) ;
#40480=CARTESIAN_POINT ( 'NONE',  ( -0.4396325459317577122, -0.5511811023622048555, -0.09757992244046775898 ) ) ;
#40481=CARTESIAN_POINT ( 'NONE',  ( 1.436417322834645294, 2.401574803149606474, -0.3149606299212598381 ) ) ;
#40483=CARTESIAN_POINT ( 'NONE',  ( -0.3346456692913377662, -0.5400638737290844871, 0.3530559997133364547 ) ) ;
#40485=CARTESIAN_POINT ( 'NONE',  ( 0.9120734908136489683, -0.6692913385826771977, 0.1292274648535927661 ) ) ;
#40488=CARTESIAN_POINT ( 'NONE',  ( -0.3280839895013117347, 0.05413385826771626580, -0.4176697321401330321 ) ) ;
#40489=CARTESIAN_POINT ( 'NONE',  ( 0.9711286089238851948, -0.5023911411419708095, -0.1820866141732282451 ) ) ;
#40492=CARTESIAN_POINT ( 'NONE',  ( 1.043307086614173818, 0.07958543189024085140, 0.2665933059059887866 ) ) ;
#40493=CARTESIAN_POINT ( 'NONE',  ( 1.220472440944882386, -0.6692913385826771977, 8.415575281601705876E-17 ) ) ;
#40495=CARTESIAN_POINT ( 'NONE',  ( -0.4921259842519677963, -0.5400638737290844871, 0.3530559997133364547 ) ) ;
#40497=CARTESIAN_POINT ( 'NONE',  ( -1.456692913385826182, -0.6692913385826771977, 8.415575281601705876E-17 ) ) ;
#40498=CARTESIAN_POINT ( 'NONE',  ( -0.1771653543307080136, -0.5400638737290844871, 0.3530559997133364547 ) ) ;
#40500=CARTESIAN_POINT ( 'NONE',  ( 1.148293963254593875, -0.6692913385826771977, 0.1292274648535927661 ) ) ;
#40501=CARTESIAN_POINT ( 'NONE',  ( 0.5774278215223103139, -0.6046776061558809534, -0.2411417322834644161 ) ) ;
#40502=CARTESIAN_POINT ( 'NONE',  ( 0.5577427821522316087, -0.08942795157527998196, 0.3641732283464567121 ) ) ;
#40504=CARTESIAN_POINT ( 'NONE',  ( 0.4921259842519691285, -0.4536011799217368745, -0.2665933059059886201 ) ) ;
#40505=CARTESIAN_POINT ( 'NONE',  ( -1.581364829396324945, -0.05778040916215560624, -0.4822834645669293319 ) ) ;
#40507=CARTESIAN_POINT ( 'NONE',  ( 0.7677165354330716118, 0.1660481256975883668, -0.3530559997133364547 ) ) ;
#40509=CARTESIAN_POINT ( 'NONE',  ( 0.3083989501312343062, -0.05778040916215560624, -0.4822834645669293319 ) ) ;
#40511=CARTESIAN_POINT ( 'NONE',  ( -0.7981007675632535436, -3.187520833735697382E-15, -0.4118477457933005237 ) ) ;
#40512=CARTESIAN_POINT ( 'NONE',  ( 0.03937007874015806264, 0.1771653543307087630, 0.000000000000000000 ) ) ;
#40513=EDGE_CURVE ( 'NONE', #44077, #68837, #37774, .T. ) ;
#40514=CARTESIAN_POINT ( 'NONE',  ( 0.5118110236220480003, -0.6692913385826771977, 8.415575281601705876E-17 ) ) ;
#40515=CARTESIAN_POINT ( 'NONE',  ( 1.692913385826772421, 0.1771653543307087630, 0.000000000000000000 ) ) ;
#40516=CARTESIAN_POINT ( 'NONE',  ( -1.095800524934382292, -0.08942795157527998196, 0.3641732283464567121 ) ) ;
#40517=CARTESIAN_POINT ( 'NONE',  ( -1.095800524934382292, -0.05778040916215522460, 0.4822834645669289988 ) ) ;
#40518=CARTESIAN_POINT ( 'NONE',  ( -1.587926509186350810, -0.4281496062992124485, 0.4176697321401328655 ) ) ;
#40520=CARTESIAN_POINT ( 'NONE',  ( 0.3412073490813655186, -0.6046776061558809534, -0.2411417322834644161 ) ) ;
#40521=CARTESIAN_POINT ( 'NONE',  ( 1.555118110236221041, 0.1660481256975883668, -0.3530559997133364547 ) ) ;
#40523=CARTESIAN_POINT ( 'NONE',  ( 0.5905511811023629321, -0.6692913385826771977, 8.415575281601705876E-17 ) ) ;
#40526=CARTESIAN_POINT ( 'NONE',  ( 1.266404199475066328, -0.3162353388693409650, -0.4822834645669289433 ) ) ;
#40527=CARTESIAN_POINT ( 'NONE',  ( -1.384514435695537005, 0.1771653543307087630, 0.09757992244046791164 ) ) ;
#40528=CARTESIAN_POINT ( 'NONE',  ( 1.404199475065617708, -0.004921259842519870586, -0.3153832671262229437 ) ) ;
#40529=CARTESIAN_POINT ( 'NONE',  ( -1.266404199475064773, -0.08942795157528024563, -0.3641732283464568787 ) ) ;
#40530=CARTESIAN_POINT ( 'NONE',  ( -0.7611548556430438595, -0.5023911411419708095, -0.1820866141732282451 ) ) ;
#40531=CARTESIAN_POINT ( 'NONE',  ( 1.541994750656168645, -0.6692913385826771977, 0.1292274648535927661 ) ) ;
#40532=CARTESIAN_POINT ( 'NONE',  ( 0.4396325459317590445, -0.5511811023622046335, 0.09757992244046803654 ) ) ;
#40533=CARTESIAN_POINT ( 'NONE',  ( -0.06561679790026180015, 0.05413385826771666132, 0.4176697321401328100 ) ) ;
#40534=CARTESIAN_POINT ( 'NONE',  ( 0.9645669291338588858, 0.1660481256975885056, 0.3530559997133364547 ) ) ;
#40535=CARTESIAN_POINT ( 'NONE',  ( 0.006561679790026889343, -0.3162353388693409650, -0.4822834645669289433 ) ) ;
#40536=CARTESIAN_POINT ( 'NONE',  ( 0.08530183727034192087, -0.2845877964562161244, -0.3641732283464567121 ) ) ;
#40537=CARTESIAN_POINT ( 'NONE',  ( 1.161417322834646271, 0.1660481256975883668, -0.3530559997133364547 ) ) ;
#40539=CARTESIAN_POINT ( 'NONE',  ( -0.7939632545931754048, -0.3162353388693405765, 0.4822834645669290543 ) ) ;
#40541=CARTESIAN_POINT ( 'NONE',  ( 0.06561679790026316017, 0.009842519685039144428, -0.3409548833797004797 ) ) ;
#40542=CARTESIAN_POINT ( 'NONE',  ( -0.7480314960629914633, -0.6692913385826771977, 8.415575281601705876E-17 ) ) ;
#40543=CARTESIAN_POINT ( 'NONE',  ( 0.1049868766404206816, -0.6046776061558809534, -0.2411417322834644161 ) ) ;
#40548=CARTESIAN_POINT ( 'NONE',  ( -1.489501312335957062, -0.2845877964562161244, -0.3641732283464567121 ) ) ;
#40550=CARTESIAN_POINT ( 'NONE',  ( -1.522309711286088607, 0.2306618581243847221, -0.2411417322834647770 ) ) ;
#40552=CARTESIAN_POINT ( 'NONE',  ( 0.3543307086614181922, -0.6692913385826771977, 8.415575281601705876E-17 ) ) ;
#40553=CARTESIAN_POINT ( 'NONE',  ( -0.5511811023622041894, -0.1870078740157480601, -0.3641732283464567677 ) ) ;
#40554=CARTESIAN_POINT ( 'NONE',  ( 0.8136482939632553313, 0.2306618581243848609, 0.2411417322834645549 ) ) ;
#40555=CARTESIAN_POINT ( 'NONE',  ( 0.5446194225721792126, -0.05778040916215560624, -0.4822834645669293319 ) ) ;
#40559=CARTESIAN_POINT ( 'NONE',  ( 1.338582677165355062, -0.1870078740157479769, 0.4822834645669291653 ) ) ;
#40560=CARTESIAN_POINT ( 'NONE',  ( -0.07217847769028813698, -0.3162353388693409650, -0.4822834645669289433 ) ) ;
#40561=CARTESIAN_POINT ( 'NONE',  ( -1.574803149606298192, -0.1870078740157480879, -0.4822834645669291653 ) ) ;
#40562=CARTESIAN_POINT ( 'NONE',  ( 0.9973753280839902091, -0.6046776061558807314, 0.2411417322834647770 ) ) ;
#40564=CARTESIAN_POINT ( 'NONE',  ( 0.07874015748031558404, -0.1870078740157480879, -0.4822834645669291653 ) ) ;
#40565=CARTESIAN_POINT ( 'NONE',  ( 0.5118110236220480003, -0.6692913385826771977, 8.415575281601705876E-17 ) ) ;
#40566=CARTESIAN_POINT ( 'NONE',  ( -0.2362204724409440182, -0.1870078740157479769, 0.4822834645669291653 ) ) ;
#40567=CARTESIAN_POINT ( 'NONE',  ( 0.7611548556430454138, 0.1283753931104746893, -0.1820866141732285504 ) ) ;
#40568=CARTESIAN_POINT ( 'NONE',  ( -1.148293963254592542, -0.6692913385826773087, -0.1292274648535924053 ) ) ;
#40569=CARTESIAN_POINT ( 'NONE',  ( -1.410761154855642463, -0.05778040916215522460, 0.4822834645669289988 ) ) ;
#40570=CARTESIAN_POINT ( 'NONE',  ( 0.8923884514435701520, -0.6046776061558809534, -0.2411417322834644161 ) ) ;
#40571=CARTESIAN_POINT ( 'NONE',  ( -0.7535225988626923499, 2.401574803149606474, -0.4915354330708644470 ) ) ;
#40576=CARTESIAN_POINT ( 'NONE',  ( 0.9645669291338591078, -0.5400638737290845981, -0.3530559997133363437 ) ) ;
#40577=CARTESIAN_POINT ( 'NONE',  ( 0.3608923884514443348, 0.1771653543307087075, -0.09757992244046823083 ) ) ;
#40582=CARTESIAN_POINT ( 'NONE',  ( 1.476377952755906220, 0.1660481256975883668, -0.3530559997133364547 ) ) ;
#40583=CARTESIAN_POINT ( 'NONE',  ( -1.568241469816272105, -0.3162353388693409650, -0.4822834645669289433 ) ) ;
#40584=CARTESIAN_POINT ( 'NONE',  ( -0.2887139107611542133, 0.2306618581243848609, 0.2411417322834645549 ) ) ;
#40585=CARTESIAN_POINT ( 'NONE',  ( 1.069553805774278610, -0.6692913385826771977, 0.1292274648535927661 ) ) ;
#40587=CARTESIAN_POINT ( 'NONE',  ( -1.725721784776902190, -0.05778040916215522460, 0.4822834645669289988 ) ) ;
#40590=CARTESIAN_POINT ( 'NONE',  ( 1.673228346456693494, 0.07958543189024085140, 0.2665933059059887866 ) ) ;
#40592=CARTESIAN_POINT ( 'NONE',  ( -1.496062992125983815, -0.1870078740157479769, 0.3641732283464567677 ) ) ;
#40593=CARTESIAN_POINT ( 'NONE',  ( -1.640419947506561060, 0.05413385826771666132, 0.4176697321401328100 ) ) ;
#40594=CARTESIAN_POINT ( 'NONE',  ( 0.7086614173228353852, -0.1870078740157479769, 0.4822834645669291653 ) ) ;
#40596=CARTESIAN_POINT ( 'NONE',  ( 1.417322834645670104, -0.1870078740157480879, -0.4822834645669291653 ) ) ;
#40598=CARTESIAN_POINT ( 'NONE',  ( -0.5971128608923877978, 0.1771653543307087630, 0.09757992244046791164 ) ) ;
#40599=CARTESIAN_POINT ( 'NONE',  ( 0.8464566929133866546, -0.5400638737290844871, 0.3530559997133364547 ) ) ;
#40600=CARTESIAN_POINT ( 'NONE',  ( -1.522309711286088607, 0.2306618581243847221, -0.2411417322834647770 ) ) ;
#40602=CARTESIAN_POINT ( 'NONE',  ( -0.9448818897637790704, -0.1870078740157479769, 0.3641732283464567677 ) ) ;
#40603=CARTESIAN_POINT ( 'NONE',  ( -1.364829396325458521, -0.5023911411419708095, 0.1820866141732285504 ) ) ;
#40605=CARTESIAN_POINT ( 'NONE',  ( 0.5774278215223103139, -0.6046776061558809534, -0.2411417322834644161 ) ) ;
#40606=CARTESIAN_POINT ( 'NONE',  ( -1.049868766404198794, -0.5023911411419708095, 0.1820866141732285504 ) ) ;
#40607=CARTESIAN_POINT ( 'NONE',  ( -0.1902887139107604098, -0.5511811023622046335, 0.09757992244046803654 ) ) ;
#40608=CARTESIAN_POINT ( 'NONE',  ( -0.4658792650918627265, -0.05778040916215522460, 0.4822834645669289988 ) ) ;
#40609=CARTESIAN_POINT ( 'NONE',  ( 1.607611548556431069, -0.6692913385826773087, -0.1292274648535924053 ) ) ;
#40611=CARTESIAN_POINT ( 'NONE',  ( 0.5971128608923890191, -0.6692913385826771977, 0.1292274648535927661 ) ) ;
#40612=CARTESIAN_POINT ( 'NONE',  ( -1.572991167713776672, 2.401574803149606474, -0.1227090857360982196 ) ) ;
#40614=CARTESIAN_POINT ( 'NONE',  ( -0.8136482939632537770, -0.6046776061558807314, 0.2411417322834647770 ) ) ;
#40615=CARTESIAN_POINT ( 'NONE',  ( -0.3412073490813641308, -0.5023911411419708095, 0.1820866141732285504 ) ) ;
#40616=CARTESIAN_POINT ( 'NONE',  ( -1.489501312335957062, -0.05778040916215522460, 0.4822834645669289988 ) ) ;
#40617=CARTESIAN_POINT ( 'NONE',  ( 0.5380577427821529035, -0.3690944881889763329, 0.3153832671262228327 ) ) ;
#40618=CARTESIAN_POINT ( 'NONE',  ( -0.8858267716535425107, 0.07958543189024071263, -0.2665933059059888421 ) ) ;
#40619=CARTESIAN_POINT ( 'NONE',  ( -1.003937007874015297, -0.5400638737290845981, -0.3530559997133363437 ) ) ;
#40620=CARTESIAN_POINT ( 'NONE',  ( -1.640419947506561060, -0.4281496062992127816, -0.4176697321401328100 ) ) ;
#40621=CARTESIAN_POINT ( 'NONE',  ( -1.653543307086613234, -0.1870078740157479769, 0.4822834645669291653 ) ) ;
#40622=DIRECTION ( 'NONE',  ( 0.000000000000000000, 0.000000000000000000, 1.000000000000000000 ) ) ;
#40623=CARTESIAN_POINT ( 'NONE',  ( 0.7414698162729663755, 0.1771653543307087630, 0.09757992244046791164 ) ) ;
#40625=CARTESIAN_POINT ( 'NONE',  ( 0.4330708661417329575, 0.2952755905511811885, 0.000000000000000000 ) ) ;
#40626=CARTESIAN_POINT ( 'NONE',  ( -1.391076115485563314, -0.6046776061558809534, -0.2411417322834644161 ) ) ;
#40627=CARTESIAN_POINT ( 'NONE',  ( 1.410761154855643795, -0.2845877964562159024, 0.3641732283464567677 ) ) ;
#40631=CARTESIAN_POINT ( 'NONE',  ( -1.351706036745406347, -0.3690944881889763329, 0.3153832671262228327 ) ) ;
#40632=CARTESIAN_POINT ( 'NONE',  ( -0.5446194225721777693, -0.05778040916215522460, 0.4822834645669289988 ) ) ;
#40633=CARTESIAN_POINT ( 'NONE',  ( 0.3477690288713918276, 0.2952755905511811885, 0.1292274648535926551 ) ) ;
#40634=CARTESIAN_POINT ( 'NONE',  ( -1.450131233595799651, -0.5511811023622046335, 0.09757992244046803654 ) ) ;
#40636=CARTESIAN_POINT ( 'NONE',  ( -1.450131233595799651, -0.6692913385826771977, 0.1292274648535927661 ) ) ;
#40637=CARTESIAN_POINT ( 'NONE',  ( 0.5183727034120741983, -0.6692913385826771977, 0.1292274648535927661 ) ) ;
#40638=CARTESIAN_POINT ( 'NONE',  ( 0.2493438320209980519, 0.05413385826771666132, 0.4176697321401328100 ) ) ;
#40639=CARTESIAN_POINT ( 'NONE',  ( 1.253280839895013710, -0.3162353388693405765, 0.4822834645669290543 ) ) ;
#40644=CARTESIAN_POINT ( 'NONE',  ( 0.08530183727034192087, -0.2845877964562161244, -0.3641732283464567121 ) ) ;
#40645=CARTESIAN_POINT ( 'NONE',  ( -0.1640419947506555343, -0.3162353388693405765, 0.4822834645669290543 ) ) ;
#40646=CARTESIAN_POINT ( 'NONE',  ( 0.8464566929133865436, 0.1660481256975883668, -0.3530559997133364547 ) ) ;
#40648=CARTESIAN_POINT ( 'NONE',  ( -0.1574803149606292529, -0.1870078740157480601, -0.3641732283464567677 ) ) ;
#40649=CARTESIAN_POINT ( 'NONE',  ( -1.246719160104985846, -0.4281496062992127816, -0.4176697321401328100 ) ) ;
#40650=CARTESIAN_POINT ( 'NONE',  ( -1.574803149606298192, -0.1870078740157480879, -0.4822834645669291653 ) ) ;
#40653=ORIENTED_EDGE ( 'NONE', *, *, #68271, .T. ) ;
#40654=ORIENTED_EDGE ( 'NONE', *, *, #79843, .F. ) ;
#40655=CARTESIAN_POINT ( 'NONE',  ( 1.312335958005249825, 0.2306618581243847221, -0.2411417322834647770 ) ) ;
#40656=CARTESIAN_POINT ( 'NONE',  ( -1.666666666666665853, 0.05413385826771626580, -0.4176697321401330321 ) ) ;
#40657=CARTESIAN_POINT ( 'NONE',  ( -1.325459317585300889, -0.004921259842519576551, 0.3153832671262227771 ) ) ;
#40658=CARTESIAN_POINT ( 'NONE',  ( -1.364829396325458521, -0.6046776061558807314, 0.2411417322834647770 ) ) ;
#40660=CYLINDRICAL_SURFACE ( 'NONE', #66588, 0.4822834645669291653 ) ;
#40661=CARTESIAN_POINT ( 'NONE',  ( 1.423884514435696413, -0.3162353388693409650, -0.4822834645669289433 ) ) ;
#40662=CARTESIAN_POINT ( 'NONE',  ( -1.719160104986876103, 0.05413385826771666132, 0.4176697321401328100 ) ) ;
#40663=CARTESIAN_POINT ( 'NONE',  ( -0.2362204724409442680, -0.1870078740157480879, -0.4822834645669291653 ) ) ;
#40664=CARTESIAN_POINT ( 'NONE',  ( -0.2493438320209966919, 0.05413385826771626580, -0.4176697321401330321 ) ) ;
#40665=CARTESIAN_POINT ( 'NONE',  ( -1.181102362204723644, -0.1870078740157479769, 0.4822834645669291653 ) ) ;
#40667=CARTESIAN_POINT ( 'NONE',  ( 0.4986876640419954376, 0.2306618581243848609, 0.2411417322834645549 ) ) ;
#40669=CARTESIAN_POINT ( 'NONE',  ( -1.325459317585300889, -0.004921259842519576551, 0.3153832671262227771 ) ) ;
#40674=CARTESIAN_POINT ( 'NONE',  ( -1.194225721784776262, 0.05413385826771626580, -0.4176697321401330321 ) ) ;
#40675=CARTESIAN_POINT ( 'NONE',  ( -1.220472440944881054, -0.6692913385826771977, 8.415575281601705876E-17 ) ) ;
#40677=CARTESIAN_POINT ( 'NONE',  ( -1.338582677165353729, -0.1870078740157480879, -0.4822834645669291653 ) ) ;
#40678=CARTESIAN_POINT ( 'NONE',  ( -1.666666666666665853, 0.05413385826771626580, -0.4176697321401330321 ) ) ;
#40682=CARTESIAN_POINT ( 'NONE',  ( 0.1049868766404206816, 0.1283753931104748280, 0.1820866141732283561 ) ) ;
#40683=CARTESIAN_POINT ( 'NONE',  ( -0.7808398950131225646, -0.08942795157527998196, 0.3641732283464567121 ) ) ;
#40684=CARTESIAN_POINT ( 'NONE',  ( -1.082677165354329896, -0.5400638737290845981, -0.3530559997133363437 ) ) ;
#40685=CARTESIAN_POINT ( 'NONE',  ( 0.8398950131233602345, 0.2306618581243847221, -0.2411417322834647770 ) ) ;
#40686=CARTESIAN_POINT ( 'NONE',  ( -0.9514435695538050464, -0.05778040916215560624, -0.4822834645669293319 ) ) ;
#40689=CARTESIAN_POINT ( 'NONE',  ( -1.272965879265091305, 0.05413385826771626580, -0.4176697321401330321 ) ) ;
#40690=CARTESIAN_POINT ( 'NONE',  ( -1.482939632545930975, -0.3690944881889765550, -0.3153832671262227771 ) ) ;
#40697=CARTESIAN_POINT ( 'NONE',  ( -0.2362204724409440182, -0.1870078740157479769, 0.4822834645669291653 ) ) ;
#40698=CARTESIAN_POINT ( 'NONE',  ( -1.397637795275589623, -0.4536011799217368745, -0.2665933059059886201 ) ) ;
#40700=CARTESIAN_POINT ( 'NONE',  ( -1.646981627296586703, -0.3162353388693409650, -0.4822834645669289433 ) ) ;
#40702=CARTESIAN_POINT ( 'NONE',  ( -1.371391076115484831, 0.2952755905511810774, -0.1292274648535930714 ) ) ;
#40703=CARTESIAN_POINT ( 'NONE',  ( -0.4593175853018366950, 0.05413385826771666132, 0.4176697321401328100 ) ) ;
#40705=CARTESIAN_POINT ( 'NONE',  ( 0.3740157480314966754, 0.07958543189024071263, -0.2665933059059888421 ) ) ;
#40706=FACE_OUTER_BOUND ( 'NONE', #1312, .T. ) ;
#40707=CARTESIAN_POINT ( 'NONE',  ( 0.4593175853018380828, -0.004921259842519870586, -0.3153832671262229437 ) ) ;
#40708=CARTESIAN_POINT ( 'NONE',  ( 0.8661417322834652488, -0.1870078740157480601, -0.3641732283464567677 ) ) ;
#40709=CARTESIAN_POINT ( 'NONE',  ( 1.023622047244095112, -0.1870078740157480879, -0.4822834645669291653 ) ) ;
#40710=CARTESIAN_POINT ( 'NONE',  ( -0.3674540682414689785, 0.1283753931104748280, 0.1820866141732283561 ) ) ;
#40712=CARTESIAN_POINT ( 'NONE',  ( -1.213910761154854745, -0.6692913385826771977, 0.1292274648535927661 ) ) ;
#40713=CARTESIAN_POINT ( 'NONE',  ( 0.09186351706036799403, -0.3690944881889765550, -0.3153832671262227771 ) ) ;
#40714=CARTESIAN_POINT ( 'NONE',  ( -1.371391076115484609, -0.5511811023622046335, 0.09757992244046803654 ) ) ;
#40716=CARTESIAN_POINT ( 'NONE',  ( -0.9383202099737524282, -0.2845877964562161244, -0.3641732283464567121 ) ) ;
#40718=CARTESIAN_POINT ( 'NONE',  ( -0.05249343832020911260, 0.2306618581243848609, 0.2411417322834645549 ) ) ;
#40719=CARTESIAN_POINT ( 'NONE',  ( 1.673228346456693494, 0.07958543189024085140, 0.2665933059059887866 ) ) ;
#40720=CARTESIAN_POINT ( 'NONE',  ( 0.7283464566929140904, -0.4536011799217368745, -0.2665933059059886201 ) ) ;
#40721=CARTESIAN_POINT ( 'NONE',  ( -0.2296587926509179312, -0.2845877964562161244, -0.3641732283464567121 ) ) ;
#40722=CARTESIAN_POINT ( 'NONE',  ( -0.4986876640419939388, 0.2306618581243847221, -0.2411417322834647770 ) ) ;
#40723=CARTESIAN_POINT ( 'NONE',  ( -1.673228346456691717, 0.1660481256975883668, -0.3530559997133364547 ) ) ;
#40724=CARTESIAN_POINT ( 'NONE',  ( -1.049868766404198794, -0.5023911411419708095, 0.1820866141732285504 ) ) ;
#40726=AXIS2_PLACEMENT_3D ( 'NONE', #5319, #38948, #32638 ) ;
#40728=CARTESIAN_POINT ( 'NONE',  ( 0.6430446194225729606, -0.4281496062992127816, -0.4176697321401328100 ) ) ;
#40731=DIRECTION ( 'NONE',  ( -3.096699300667737957E-16, 1.000000000000000000, -0.000000000000000000 ) ) ;
#40732=CARTESIAN_POINT ( 'NONE',  ( -0.1902887139107604098, -0.5511811023622046335, 0.09757992244046803654 ) ) ;
#40733=CARTESIAN_POINT ( 'NONE',  ( -1.561679790026246017, -0.4281496062992127816, -0.4176697321401328100 ) ) ;
#40734=CARTESIAN_POINT ( 'NONE',  ( -1.489501312335957062, -0.08942795157527998196, 0.3641732283464567121 ) ) ;
#40735=CARTESIAN_POINT ( 'NONE',  ( 1.397637795275591177, 0.1660481256975883668, -0.3530559997133364547 ) ) ;
#40736=CARTESIAN_POINT ( 'NONE',  ( -0.5118110236220466680, -0.5511811023622047445, 6.969142054262312111E-17 ) ) ;
#40738=CARTESIAN_POINT ( 'NONE',  ( 1.062992125984252745, -0.6692913385826771977, 8.415575281601705876E-17 ) ) ;
#40743=CARTESIAN_POINT ( 'NONE',  ( 1.423884514435696191, -0.08942795157527998196, 0.3641732283464567121 ) ) ;
#40744=CARTESIAN_POINT ( 'NONE',  ( -1.115485564304461219, -0.4281496062992124485, 0.4176697321401328655 ) ) ;
#40745=CARTESIAN_POINT ( 'NONE',  ( 1.299212598425197429, 0.2952755905511811885, 0.000000000000000000 ) ) ;
#40747=CARTESIAN_POINT ( 'NONE',  ( 1.167979002624672580, -0.3690944881889763329, 0.3153832671262228327 ) ) ;
#40748=ADVANCED_FACE ( 'NONE', ( #41477 ), #54087, .F. ) ;
#40749=CARTESIAN_POINT ( 'NONE',  ( 0.2755905511811031494, 0.2952755905511811885, 0.000000000000000000 ) ) ;
#40750=CARTESIAN_POINT ( 'NONE',  ( -0.3149606299212590610, -0.1870078740157480879, -0.4822834645669291653 ) ) ;
#40752=CARTESIAN_POINT ( 'NONE',  ( 0.2887139107611556010, -0.5023911411419708095, 0.1820866141732285504 ) ) ;
#40753=ORIENTED_EDGE ( 'NONE', *, *, #63106, .T. ) ;
#40755=ORIENTED_EDGE ( 'NONE', *, *, #72350, .T. ) ;
#40756=CARTESIAN_POINT ( 'NONE',  ( -0.4199475065616791736, 0.2306618581243847221, -0.2411417322834647770 ) ) ;
#40757=CARTESIAN_POINT ( 'NONE',  ( 1.364829396325459854, -0.6046776061558809534, -0.2411417322834644161 ) ) ;
#40758=CARTESIAN_POINT ( 'NONE',  ( 0.06561679790026316017, -0.4281496062992124485, 0.4176697321401328655 ) ) ;
#40759=CARTESIAN_POINT ( 'NONE',  ( -0.2755905511811015396, -0.5511811023622047445, 6.969142054262312111E-17 ) ) ;
#40760=CARTESIAN_POINT ( 'NONE',  ( 1.108923884514436686, -0.3162353388693409650, -0.4822834645669289433 ) ) ;
#40761=CARTESIAN_POINT ( 'NONE',  ( -1.023622047244093558, -0.1870078740157479769, 0.4822834645669291653 ) ) ;
#40762=CARTESIAN_POINT ( 'NONE',  ( -0.1181102362204717315, 0.2952755905511811885, 0.000000000000000000 ) ) ;
#40763=CARTESIAN_POINT ( 'NONE',  ( -0.7480314960629914633, 0.2952755905511811885, 0.000000000000000000 ) ) ;
#40764=CARTESIAN_POINT ( 'NONE',  ( 1.233595800524935227, -0.6046776061558807314, 0.2411417322834647770 ) ) ;
#40765=CARTESIAN_POINT ( 'NONE',  ( 0.7939632545931766261, -0.05778040916215522460, 0.4822834645669289988 ) ) ;
#40766=CARTESIAN_POINT ( 'NONE',  ( 1.023622047244095334, -0.1870078740157479769, 0.4822834645669291653 ) ) ;
#40768=CARTESIAN_POINT ( 'NONE',  ( 0.1443569553805781891, -0.004921259842519870586, -0.3153832671262229437 ) ) ;
#40772=CARTESIAN_POINT ( 'NONE',  ( -0.9842519685039365918, -0.5511811023622047445, 6.969142054262312111E-17 ) ) ;
#40773=CARTESIAN_POINT ( 'NONE',  ( 0.1509186351706045259, -0.05778040916215560624, -0.4822834645669293319 ) ) ;
#40775=CARTESIAN_POINT ( 'NONE',  ( -0.1181102362204717315, 0.2952755905511811885, 0.000000000000000000 ) ) ;
#40776=CARTESIAN_POINT ( 'NONE',  ( -0.3477690288713905509, -0.6692913385826771977, 0.1292274648535927661 ) ) ;
#40777=CARTESIAN_POINT ( 'NONE',  ( -0.8595800524934373854, -0.05778040916215522460, 0.4822834645669289988 ) ) ;
#40778=CARTESIAN_POINT ( 'NONE',  ( -1.246719160104986512, 0.05413385826771666132, 0.4176697321401328100 ) ) ;
#40779=CARTESIAN_POINT ( 'NONE',  ( 1.338582677165355062, -0.1870078740157479769, 0.3641732283464567677 ) ) ;
#40782=CARTESIAN_POINT ( 'NONE',  ( 0.3018372703412079971, -0.3690944881889763329, 0.3153832671262228327 ) ) ;
#40783=VECTOR ( 'NONE', #59663, 39.37007874015748143 ) ;
#40784=CARTESIAN_POINT ( 'NONE',  ( -0.006561679790025524116, -0.05778040916215560624, -0.4822834645669293319 ) ) ;
#40785=CARTESIAN_POINT ( 'NONE',  ( 0.4658792650918641698, -0.05778040916215560624, -0.4822834645669293319 ) ) ;
#40788=CARTESIAN_POINT ( 'NONE',  ( -0.6036745406824141069, 0.1539470093639523085, 0.1968503937007873850 ) ) ;
#40791=CARTESIAN_POINT ( 'NONE',  ( -0.5380577427821514602, -0.4281496062992127816, -0.4176697321401328100 ) ) ;
#40794=CARTESIAN_POINT ( 'NONE',  ( -1.548556430446193399, -0.5023911411419708095, -0.1820866141732282451 ) ) ;
#40795=CARTESIAN_POINT ( 'NONE',  ( 0.7020997375328090762, -0.05778040916215560624, -0.4822834645669293319 ) ) ;
#40796=CARTESIAN_POINT ( 'NONE',  ( 0.8923884514435703741, 0.2306618581243848609, 0.2411417322834645549 ) ) ;
#40797=CARTESIAN_POINT ( 'NONE',  ( -0.2690288713910754526, -0.5511811023622046335, 0.09757992244046803654 ) ) ;
#40798=CARTESIAN_POINT ( 'NONE',  ( 0.2165354330708668673, 0.1660481256975883668, -0.3530559997133364547 ) ) ;
#40800=CARTESIAN_POINT ( 'NONE',  ( -0.02624671916010428221, 0.1283753931104746893, -0.1820866141732285504 ) ) ;
#40801=CARTESIAN_POINT ( 'NONE',  ( -0.3608923884514428360, -0.6692913385826773087, -0.1292274648535924053 ) ) ;
#40804=CARTESIAN_POINT ( 'NONE',  ( -1.515748031496062076, 0.1660481256975883668, -0.3530559997133364547 ) ) ;
#40805=CARTESIAN_POINT ( 'NONE',  ( 0.05905511811023681640, 0.07958543189024071263, -0.2665933059059888421 ) ) ;
#40806=CARTESIAN_POINT ( 'NONE',  ( 1.384514435695538559, 0.1771653543307087075, -0.09757992244046823083 ) ) ;
#40807=CARTESIAN_POINT ( 'NONE',  ( -0.9645669291338575535, -0.5400638737290844871, 0.3530559997133364547 ) ) ;
#40808=CARTESIAN_POINT ( 'NONE',  ( -0.6299212598425188991, -0.1870078740157480601, -0.3641732283464567677 ) ) ;
#40809=FACE_OUTER_BOUND ( 'NONE', #24903, .T. ) ;
#40810=CARTESIAN_POINT ( 'NONE',  ( -0.6561679790026240244, -0.6046776061558807314, 0.2411417322834647770 ) ) ;
#40811=CARTESIAN_POINT ( 'NONE',  ( -0.7742782152230962556, -0.4281496062992127816, -0.4176697321401328100 ) ) ;
#40812=CARTESIAN_POINT ( 'NONE',  ( 0.1574803149606306130, -0.1870078740157480879, -0.4822834645669291653 ) ) ;
#40814=( BOUNDED_CURVE ( )  B_SPLINE_CURVE ( 1, ( #4997, #50417 ),
 .UNSPECIFIED., .F., .F. ) 
 B_SPLINE_CURVE_WITH_KNOTS ( ( 2, 2 ),
 ( 3.469446951953614189E-18, 0.002000000000000005246 ),
 .UNSPECIFIED. ) 
 CURVE ( )  GEOMETRIC_REPRESENTATION_ITEM ( )  RATIONAL_B_SPLINE_CURVE ( ( 0.9875488213027527884, 0.9875488213027527884 ) ) 
 REPRESENTATION_ITEM ( '' )  );
#40817=CARTESIAN_POINT ( 'NONE',  ( 0.3346456692913393205, -0.4536011799217368745, -0.2665933059059886201 ) ) ;
#40818=CARTESIAN_POINT ( 'NONE',  ( 1.095800524934383846, -0.3162353388693405765, 0.4822834645669290543 ) ) ;
#40819=CARTESIAN_POINT ( 'NONE',  ( -1.108923884514435132, -0.2845877964562159024, 0.3641732283464567677 ) ) ;
#40820=CARTESIAN_POINT ( 'NONE',  ( 1.141732283464567788, -0.6692913385826771977, 8.415575281601705876E-17 ) ) ;
#40821=CARTESIAN_POINT ( 'NONE',  ( -1.213910761154854745, 0.1771653543307087075, -0.09757992244046823083 ) ) ;
#40822=CARTESIAN_POINT ( 'NONE',  ( -0.4133858267716528645, 0.1660481256975883668, -0.3530559997133364547 ) ) ;
#40823=CARTESIAN_POINT ( 'NONE',  ( 0.2427821522309719648, -0.08942795157527998196, 0.3641732283464567121 ) ) ;
#40825=CARTESIAN_POINT ( 'NONE',  ( 0.7086614173228352742, -0.1870078740157480601, -0.3641732283464567677 ) ) ;
#40827=CARTESIAN_POINT ( 'NONE',  ( 0.1574803149606306130, -0.1870078740157480879, -0.4822834645669291653 ) ) ;
#40829=EDGE_CURVE ( 'NONE', #21005, #36505, #52287, .T. ) ;
#40830=CARTESIAN_POINT ( 'NONE',  ( -0.8333333333333323711, -0.6692913385826773087, -0.1292274648535924053 ) ) ;
#40832=CARTESIAN_POINT ( 'NONE',  ( 1.076115485564305141, -0.5023911411419708095, 0.1820866141732285504 ) ) ;
#40833=CARTESIAN_POINT ( 'NONE',  ( 0.5708661417322842269, 0.1660481256975885056, 0.3530559997133364547 ) ) ;
#40834=CARTESIAN_POINT ( 'NONE',  ( -0.2755905511811015396, -0.6692913385826771977, 8.415575281601705876E-17 ) ) ;
#40835=CARTESIAN_POINT ( 'NONE',  ( -0.2559055118110227234, -0.4536011799217367080, 0.2665933059059888421 ) ) ;
#40836=LINE ( 'NONE', #21069, #48084 ) ;
#40837=CARTESIAN_POINT ( 'NONE',  ( 0.1574803149606306130, -0.1870078740157480601, -0.3641732283464567677 ) ) ;
#40838=CARTESIAN_POINT ( 'NONE',  ( 0.2493438320209980519, 0.05413385826771666132, 0.4176697321401328100 ) ) ;
#40839=CARTESIAN_POINT ( 'NONE',  ( -0.5511811023622041894, -0.1870078740157480601, -0.3641732283464567677 ) ) ;
#40841=CARTESIAN_POINT ( 'NONE',  ( -1.227034120734907141, -0.6692913385826773087, -0.1292274648535924053 ) ) ;
#40842=CARTESIAN_POINT ( 'NONE',  ( 0.8546455861312993729, 1.722984403643211298E-16, -0.3791483426435174331 ) ) ;
#40843=ORIENTED_EDGE ( 'NONE', *, *, #15427, .F. ) ;
#40844=CARTESIAN_POINT ( 'NONE',  ( -1.246719160104986512, -0.004921259842519576551, 0.3153832671262227771 ) ) ;
#40845=CARTESIAN_POINT ( 'NONE',  ( -0.2296587926509179312, -0.3162353388693409650, -0.4822834645669289433 ) ) ;
#40847=CARTESIAN_POINT ( 'NONE',  ( -0.9711286089238838626, 0.2306618581243847221, -0.2411417322834647770 ) ) ;
#40848=DIRECTION ( 'NONE',  ( 1.000000000000000000, -0.000000000000000000, -0.000000000000000000 ) ) ;
#40849=EDGE_CURVE ( 'NONE', #25966, #5694, #9491, .T. ) ;
#40850=CARTESIAN_POINT ( 'NONE',  ( -0.9186351706036736120, 0.2306618581243848609, 0.2411417322834645549 ) ) ;
#40851=CARTESIAN_POINT ( 'NONE',  ( 0.8464566929133866546, -0.5400638737290844871, 0.3530559997133364547 ) ) ;
#40852=DIRECTION ( 'NONE',  ( 0.000000000000000000, 0.000000000000000000, 1.000000000000000000 ) ) ;
#40853=CARTESIAN_POINT ( 'NONE',  ( 1.528871391076116026, -0.6692913385826773087, -0.1292274648535924053 ) ) ;
#40855=EDGE_CURVE ( 'NONE', #37713, #72462, #74255, .T. ) ;
#40856=CARTESIAN_POINT ( 'NONE',  ( -1.266404199475064773, -0.3162353388693405765, 0.4822834645669290543 ) ) ;
#40859=CARTESIAN_POINT ( 'NONE',  ( -0.5118110236220466680, 0.1771653543307087630, 0.000000000000000000 ) ) ;
#40862=ORIENTED_EDGE ( 'NONE', *, *, #64032, .T. ) ;
#40863=CARTESIAN_POINT ( 'NONE',  ( 0.8136482939632553313, 0.2306618581243848609, 0.2411417322834645549 ) ) ;
#40865=CARTESIAN_POINT ( 'NONE',  ( -0.04593175853018302557, -0.6692913385826773087, -0.1292274648535924053 ) ) ;
#40866=CARTESIAN_POINT ( 'NONE',  ( -0.8727034120734901146, -0.3162353388693405765, 0.4822834645669290543 ) ) ;
#40867=CARTESIAN_POINT ( 'NONE',  ( 1.555118110236221041, 0.1660481256975883668, -0.3530559997133364547 ) ) ;
#40868=CARTESIAN_POINT ( 'NONE',  ( -0.8530183727034112984, -0.004921259842519576551, 0.3153832671262227771 ) ) ;
#40870=CARTESIAN_POINT ( 'NONE',  ( 0.5314960629921267055, -0.5400638737290844871, 0.3530559997133364547 ) ) ;
#40871=CARTESIAN_POINT ( 'NONE',  ( 0.5577427821522314977, -0.2845877964562161244, -0.3641732283464567121 ) ) ;
#40872=CARTESIAN_POINT ( 'NONE',  ( -1.023622047244093558, -0.1870078740157479769, 0.4822834645669291653 ) ) ;
#40874=CARTESIAN_POINT ( 'NONE',  ( -1.443569553805773564, 0.2306618581243847221, -0.2411417322834647770 ) ) ;
#40875=CARTESIAN_POINT ( 'NONE',  ( -1.699475065616797398, 0.1771653543307087630, 0.09757992244046791164 ) ) ;
#40876=CARTESIAN_POINT ( 'NONE',  ( 0.8661417322834653598, -0.1870078740157479769, 0.4822834645669291653 ) ) ;
#40877=CARTESIAN_POINT ( 'NONE',  ( 1.325459317585302665, -0.3690944881889763329, 0.3153832671262228327 ) ) ;
#40878=VERTEX_POINT ( 'NONE', #81451 ) ;
#40880=CARTESIAN_POINT ( 'NONE',  ( -0.3346456692913377662, 0.1660481256975883668, -0.3530559997133364547 ) ) ;
#40882=CARTESIAN_POINT ( 'NONE',  ( 0.4330708661417329575, -0.5511811023622047445, 6.969142054262312111E-17 ) ) ;
#40883=CARTESIAN_POINT ( 'NONE',  ( -1.358267716535432434, 0.1660481256975883668, -0.3530559997133364547 ) ) ;
#40884=CARTESIAN_POINT ( 'NONE',  ( 0.8530183727034126306, 0.05413385826771626580, -0.4176697321401330321 ) ) ;
#40885=CARTESIAN_POINT ( 'NONE',  ( 1.023622047244095112, -0.1870078740157480879, -0.4822834645669291653 ) ) ;
#40886=CARTESIAN_POINT ( 'NONE',  ( 0.09842519685039434474, -0.5400638737290845981, -0.3530559997133363437 ) ) ;
#40887=CARTESIAN_POINT ( 'NONE',  ( -0.3608923884514428360, 0.2952755905511811885, 0.1292274648535926551 ) ) ;
#40889=CARTESIAN_POINT ( 'NONE',  ( -1.482939632545930975, -0.4281496062992127816, -0.4176697321401328100 ) ) ;
#40890=CARTESIAN_POINT ( 'NONE',  ( -0.8005249343832011588, 0.05413385826771626580, -0.4176697321401330321 ) ) ;
#40891=EDGE_CURVE ( 'NONE', #18593, #18898, #10129, .T. ) ;
#40892=CARTESIAN_POINT ( 'NONE',  ( -0.3543307086614165824, 0.1771653543307087630, 0.000000000000000000 ) ) ;
#40893=CARTESIAN_POINT ( 'NONE',  ( 1.161417322834646493, -0.5400638737290844871, 0.3530559997133364547 ) ) ;
#40894=CARTESIAN_POINT ( 'NONE',  ( 1.456692913385827515, -0.6692913385826771977, 8.415575281601705876E-17 ) ) ;
#40895=CARTESIAN_POINT ( 'NONE',  ( -0.5708661417322828946, 0.1660481256975883668, -0.3530559997133364547 ) ) ;
#40897=CARTESIAN_POINT ( 'NONE',  ( 0.6561679790026253567, 0.2306618581243848609, 0.2411417322834645549 ) ) ;
#40899=CARTESIAN_POINT ( 'NONE',  ( 1.595398199321655275, 1.034147571970761126, 0.1559797534342493575 ) ) ;
#40900=CARTESIAN_POINT ( 'NONE',  ( -0.05249343832020911260, 0.2306618581243848609, 0.2411417322834645549 ) ) ;
#40901=CARTESIAN_POINT ( 'NONE',  ( -1.115485564304461219, -0.004921259842519870586, -0.3153832671262229437 ) ) ;
#40902=CARTESIAN_POINT ( 'NONE',  ( 1.135170603674541256, -0.5511811023622048555, -0.09757992244046775898 ) ) ;
#40905=CARTESIAN_POINT ( 'NONE',  ( 1.220472440944882608, 0.1771653543307087630, 0.000000000000000000 ) ) ;
#40906=CARTESIAN_POINT ( 'NONE',  ( 1.266404199475066328, -0.05778040916215522460, 0.4822834645669289988 ) ) ;
#40908=CARTESIAN_POINT ( 'NONE',  ( -0.2034120734908131112, -0.6692913385826773087, -0.1292274648535924053 ) ) ;
#40911=CARTESIAN_POINT ( 'NONE',  ( 1.227034120734908917, -0.5511811023622046335, 0.09757992244046803654 ) ) ;
#40912=CARTESIAN_POINT ( 'NONE',  ( -0.1968503937007867743, -0.6692913385826771977, 8.415575281601705876E-17 ) ) ;
#40914=CARTESIAN_POINT ( 'NONE',  ( 1.082677165354331228, 0.1660481256975883668, -0.3530559997133364547 ) ) ;
#40915=CARTESIAN_POINT ( 'NONE',  ( 0.3740157480314966754, 0.1660481256975883668, -0.3530559997133364547 ) ) ;
#40916=CARTESIAN_POINT ( 'NONE',  ( 0.5774278215223104249, 0.1283753931104748280, 0.1820866141732283561 ) ) ;
#40917=DIRECTION ( 'NONE',  ( 0.000000000000000000, 1.000000000000000000, -0.000000000000000000 ) ) ;
#40918=CARTESIAN_POINT ( 'NONE',  ( 0.6167979002624679463, -0.004921259842519870586, -0.3153832671262229437 ) ) ;
#40919=CARTESIAN_POINT ( 'NONE',  ( -2.795275590551183242, 1.574803149606300412, -1.327125379919507468E-16 ) ) ;
#40922=CARTESIAN_POINT ( 'NONE',  ( 0.6102362204724416372, 0.1660481256975883668, -0.3530559997133364547 ) ) ;
#40924=CARTESIAN_POINT ( 'NONE',  ( 0.4606732211678791766, 2.793565526369266028, 0.5309055118110233007 ) ) ;
#40926=CARTESIAN_POINT ( 'NONE',  ( 0.07874015748031558404, -0.1870078740157480601, -0.3641732283464567677 ) ) ;
#40928=CARTESIAN_POINT ( 'NONE',  ( -0.04593175853018302557, 0.2952755905511811885, 0.1292274648535926551 ) ) ;
#40929=CARTESIAN_POINT ( 'NONE',  ( 1.318897637795276356, -0.4536011799217367080, 0.2665933059059888421 ) ) ;
#40930=CARTESIAN_POINT ( 'NONE',  ( -1.496062992125983815, -0.1870078740157480601, -0.3641732283464567677 ) ) ;
#40931=CARTESIAN_POINT ( 'NONE',  ( -1.148293963254592542, -0.6692913385826773087, -0.1292274648535924053 ) ) ;
#40932=CARTESIAN_POINT ( 'NONE',  ( 0.6167979002624679463, 0.05413385826771626580, -0.4176697321401330321 ) ) ;
#40933=CARTESIAN_POINT ( 'NONE',  ( 1.627296587926509996, -0.6046776061558807314, 0.2411417322834647770 ) ) ;
#40936=CARTESIAN_POINT ( 'NONE',  ( 0.4593175853018379162, -0.4281496062992124485, 0.4176697321401328655 ) ) ;
#40938=CARTESIAN_POINT ( 'NONE',  ( 1.587926509186352586, -0.4281496062992127816, -0.4176697321401328100 ) ) ;
#40939=CARTESIAN_POINT ( 'NONE',  ( 0.9842519685039378130, -0.6692913385826771977, 8.415575281601705876E-17 ) ) ;
#40940=CARTESIAN_POINT ( 'NONE',  ( -1.391076115485563758, 0.1283753931104748280, 0.1820866141732283561 ) ) ;
#40941=CARTESIAN_POINT ( 'NONE',  ( 1.259842519685040019, -0.1870078740157480601, -0.3641732283464567677 ) ) ;
#40942=CARTESIAN_POINT ( 'NONE',  ( -1.614173228346455824, 0.1771653543307087630, 0.000000000000000000 ) ) ;
#40943=CARTESIAN_POINT ( 'NONE',  ( -0.7480314960629914633, -0.5511811023622047445, 6.969142054262312111E-17 ) ) ;
#40944=CARTESIAN_POINT ( 'NONE',  ( 1.509186351706037543, -0.4281496062992127816, -0.4176697321401328100 ) ) ;
#40945=CARTESIAN_POINT ( 'NONE',  ( 0.6496062992125991586, 0.07958543189024085140, 0.2665933059059887866 ) ) ;
#40946=CARTESIAN_POINT ( 'NONE',  ( 0.3215223097112867578, -0.3162353388693409650, -0.4822834645669289433 ) ) ;
#40947=CARTESIAN_POINT ( 'NONE',  ( 1.082677165354331228, -0.5400638737290844871, 0.3530559997133364547 ) ) ;
#40948=CARTESIAN_POINT ( 'NONE',  ( -0.4330708661417315697, -0.6692913385826771977, 8.415575281601705876E-17 ) ) ;
#40949=CARTESIAN_POINT ( 'NONE',  ( 0.3412073490813655186, 0.1283753931104748280, 0.1820866141732283561 ) ) ;
#40950=CARTESIAN_POINT ( 'NONE',  ( 1.036745406824147508, -0.4281496062992127816, -0.4176697321401328100 ) ) ;
#40951=CARTESIAN_POINT ( 'NONE',  ( -1.561679790026246017, -0.4281496062992127816, -0.4176697321401328100 ) ) ;
#40952=CARTESIAN_POINT ( 'NONE',  ( -1.030183727034119867, -0.05778040916215560624, -0.4822834645669293319 ) ) ;
#40953=CARTESIAN_POINT ( 'NONE',  ( -1.391076115485563758, 0.1283753931104748280, 0.1820866141732283561 ) ) ;
#40955=CARTESIAN_POINT ( 'NONE',  ( -1.207349081364828880, 0.1539470093639521697, -0.1968503937007875793 ) ) ;
#40956=CARTESIAN_POINT ( 'NONE',  ( -0.6758530183727028406, 0.2952755905511811885, 0.1292274648535926551 ) ) ;
#40957=CARTESIAN_POINT ( 'NONE',  ( 0.05905511811023681640, 0.1660481256975883668, -0.3530559997133364547 ) ) ;
#40963=CARTESIAN_POINT ( 'NONE',  ( 1.135170603674541256, 0.2952755905511811885, 0.1292274648535926551 ) ) ;
#40965=CARTESIAN_POINT ( 'NONE',  ( -0.2465595919006988435, -1.283732188437465593E-15, -0.4281993546915532911 ) ) ;
#40966=CARTESIAN_POINT ( 'NONE',  ( -1.187664041994750175, -0.08942795157528024563, -0.3641732283464568787 ) ) ;
#40967=CARTESIAN_POINT ( 'NONE',  ( 1.423884514435696413, -0.3162353388693409650, -0.4822834645669289433 ) ) ;
#40968=CARTESIAN_POINT ( 'NONE',  ( -1.469816272965878357, -0.6046776061558809534, -0.2411417322834644161 ) ) ;
#40970=CARTESIAN_POINT ( 'NONE',  ( 0.1115485564304470323, 0.2952755905511811885, 0.1292274648535926551 ) ) ;
#40971=CARTESIAN_POINT ( 'NONE',  ( -0.4265091863517051496, 0.1771653543307087075, -0.09757992244046823083 ) ) ;
#40972=CARTESIAN_POINT ( 'NONE',  ( 0.6627296587926515548, 0.2952755905511811885, 0.1292274648535926551 ) ) ;
#40973=CARTESIAN_POINT ( 'NONE',  ( 0.5577427821522314977, -0.3162353388693409650, -0.4822834645669289433 ) ) ;
#40977=CARTESIAN_POINT ( 'NONE',  ( 0.8398950131233602345, -0.6046776061558807314, 0.2411417322834647770 ) ) ;
#40978=CARTESIAN_POINT ( 'NONE',  ( -0.05249343832020938322, -0.6046776061558809534, -0.2411417322834644161 ) ) ;
#40979=CARTESIAN_POINT ( 'NONE',  ( -0.9842519685039360366, 0.2952755905511811885, 0.000000000000000000 ) ) ;
#40982=CARTESIAN_POINT ( 'NONE',  ( -1.640419947506561060, 0.05413385826771666132, 0.4176697321401328100 ) ) ;
#40983=CARTESIAN_POINT ( 'NONE',  ( 0.6889763779527566800, -0.5400638737290844871, 0.3530559997133364547 ) ) ;
#40985=CARTESIAN_POINT ( 'NONE',  ( -0.1509186351706028884, -0.05778040916215522460, 0.4822834645669289988 ) ) ;
#40986=CARTESIAN_POINT ( 'NONE',  ( 0.4724409448818904789, -0.1870078740157480879, -0.4822834645669291653 ) ) ;
#40987=CARTESIAN_POINT ( 'NONE',  ( 0.1640419947506569498, -0.3162353388693409650, -0.4822834645669289433 ) ) ;
#40989=CARTESIAN_POINT ( 'NONE',  ( 0.7939632545931766261, -0.2845877964562161244, -0.3641732283464567121 ) ) ;
#40990=CARTESIAN_POINT ( 'NONE',  ( -1.541994750656167090, 0.2952755905511811885, 0.1292274648535926551 ) ) ;
#40991=CARTESIAN_POINT ( 'NONE',  ( -1.581364829396324945, -0.3162353388693405765, 0.4822834645669290543 ) ) ;
#40992=CARTESIAN_POINT ( 'NONE',  ( 0.5577427821522314977, -0.3162353388693409650, -0.4822834645669289433 ) ) ;
#40995=EDGE_LOOP ( 'NONE', ( #39952, #69524, #27836, #42826 ) ) ;
#40998=CARTESIAN_POINT ( 'NONE',  ( 1.227034120734908917, 0.2952755905511810774, -0.1292274648535930714 ) ) ;
#40999=CARTESIAN_POINT ( 'NONE',  ( 0.4461942257217855201, -0.5023911411419708095, 0.1820866141732285504 ) ) ;
#41000=CARTESIAN_POINT ( 'NONE',  ( 0.6102362204724416372, 0.1660481256975883391, -0.3530559997133364547 ) ) ;
#41004=CARTESIAN_POINT ( 'NONE',  ( -1.601049868766403650, 0.2306618581243847221, -0.2411417322834647770 ) ) ;
#41005=CARTESIAN_POINT ( 'NONE',  ( -0.3805774278215216522, -0.4281496062992127816, -0.4176697321401328100 ) ) ;
#41006=CARTESIAN_POINT ( 'NONE',  ( 1.102362204724410155, -0.1870078740157479769, 0.4822834645669291653 ) ) ;
#41008=CARTESIAN_POINT ( 'NONE',  ( 1.607611548556431069, -0.5511811023622048555, -0.09757992244046775898 ) ) ;
#41010=CARTESIAN_POINT ( 'NONE',  ( 1.620734908136483465, -0.5511811023622046335, 0.09757992244046803654 ) ) ;
#41012=CARTESIAN_POINT ( 'NONE',  ( -1.135170603674539924, 0.1771653543307087075, -0.09757992244046823083 ) ) ;
#41014=CARTESIAN_POINT ( 'NONE',  ( 0.05249343832021075018, -0.6046776061558807314, 0.2411417322834647770 ) ) ;
#41015=CARTESIAN_POINT ( 'NONE',  ( 1.489501312335958172, -0.3162353388693405765, 0.4822834645669290543 ) ) ;
#41017=CARTESIAN_POINT ( 'NONE',  ( -0.7611548556430438595, 0.1283753931104748280, 0.1820866141732283561 ) ) ;
#41018=CARTESIAN_POINT ( 'NONE',  ( 0.6561679790026253567, -0.6046776061558809534, -0.2411417322834644161 ) ) ;
#41019=CARTESIAN_POINT ( 'NONE',  ( 1.482939632545932307, -0.004921259842519870586, -0.3153832671262229437 ) ) ;
#41021=CARTESIAN_POINT ( 'NONE',  ( -0.8858267716535425107, 0.07958543189024071263, -0.2665933059059888421 ) ) ;
#41022=CARTESIAN_POINT ( 'NONE',  ( -1.574803149606298192, -0.1870078740157480601, -0.3641732283464567677 ) ) ;
#41024=CARTESIAN_POINT ( 'NONE',  ( 0.4133858267716541968, -0.5400638737290845981, -0.3530559997133363437 ) ) ;
#41025=CARTESIAN_POINT ( 'NONE',  ( -1.089238845144356427, -0.3690944881889765550, -0.3153832671262227771 ) ) ;
#41026=CARTESIAN_POINT ( 'NONE',  ( -0.4265091863517051496, 0.1771653543307087075, -0.09757992244046823083 ) ) ;
#41027=CARTESIAN_POINT ( 'NONE',  ( -0.5052493438320203589, -0.6692913385826771977, 0.1292274648535927661 ) ) ;
#41028=CARTESIAN_POINT ( 'NONE',  ( 1.660104986876641320, -0.05778040916215522460, 0.4822834645669289988 ) ) ;
#41030=CARTESIAN_POINT ( 'NONE',  ( 0.7480314960629927956, -0.6692913385826771977, 8.415575281601705876E-17 ) ) ;
#41033=CARTESIAN_POINT ( 'NONE',  ( -0.5905511811023615998, 0.2952755905511811885, 0.000000000000000000 ) ) ;
#41034=CARTESIAN_POINT ( 'NONE',  ( -0.2887139107611542133, 0.1283753931104748280, 0.1820866141732283561 ) ) ;
#41035=CARTESIAN_POINT ( 'NONE',  ( -1.325459317585300889, 0.05413385826771666132, 0.4176697321401328100 ) ) ;
#41036=CARTESIAN_POINT ( 'NONE',  ( 0.4527559055118117182, 0.07958543189024071263, -0.2665933059059888421 ) ) ;
#41038=CARTESIAN_POINT ( 'NONE',  ( -0.5249343832020990641, -0.5023911411419708095, -0.1820866141732282451 ) ) ;
#41039=CARTESIAN_POINT ( 'NONE',  ( -0.9908136482939626788, -0.6692913385826773087, -0.1292274648535924053 ) ) ;
#41040=CARTESIAN_POINT ( 'NONE',  ( -1.377952755905511140, 0.2952755905511811885, 0.000000000000000000 ) ) ;
#41041=CARTESIAN_POINT ( 'NONE',  ( 1.391076115485564868, 0.2306618581243847221, -0.2411417322834647770 ) ) ;
#41043=CARTESIAN_POINT ( 'NONE',  ( 1.036745406824147731, -0.004921259842519576551, 0.3153832671262227771 ) ) ;
#41044=CARTESIAN_POINT ( 'NONE',  ( 0.4461942257217856311, 0.2306618581243847221, -0.2411417322834647770 ) ) ;
#41046=CARTESIAN_POINT ( 'NONE',  ( 1.345144356955381593, -0.2845877964562161244, -0.3641732283464567121 ) ) ;
#41047=ORIENTED_EDGE ( 'NONE', *, *, #3407, .T. ) ;
#41049=CARTESIAN_POINT ( 'NONE',  ( -1.148293963254592542, 0.1771653543307087630, 0.09757992244046791164 ) ) ;
#41050=CARTESIAN_POINT ( 'NONE',  ( -0.4265091863517051496, -0.6692913385826771977, 0.1292274648535927661 ) ) ;
#41051=CARTESIAN_POINT ( 'NONE',  ( 0.3740157480314966754, 0.1660481256975883668, -0.3530559997133364547 ) ) ;
#41052=CARTESIAN_POINT ( 'NONE',  ( -1.653543307086613234, -0.1870078740157480601, -0.3641732283464567677 ) ) ;
#41054=CARTESIAN_POINT ( 'NONE',  ( -1.410761154855642463, -0.05778040916215522460, 0.4822834645669289988 ) ) ;
#41055=CARTESIAN_POINT ( 'NONE',  ( 0.4002624671916016896, -0.05778040916215522460, 0.4822834645669289988 ) ) ;
#41056=CARTESIAN_POINT ( 'NONE',  ( 0.03280839895013198948, -0.6692913385826773087, -0.1292274648535924053 ) ) ;
#41057=CARTESIAN_POINT ( 'NONE',  ( 1.246719160104987623, -0.4281496062992124485, 0.4176697321401328655 ) ) ;
#41062=DIRECTION ( 'NONE',  ( 3.114085624724525612E-16, -1.000000000000000000, -5.270319453084425600E-32 ) ) ;
#41064=CARTESIAN_POINT ( 'NONE',  ( -0.1181102362204717315, 0.1771653543307087630, 0.000000000000000000 ) ) ;
#41065=CARTESIAN_POINT ( 'NONE',  ( -0.3805774278215216522, -0.4281496062992127816, -0.4176697321401328100 ) ) ;
#41066=CARTESIAN_POINT ( 'NONE',  ( 0.9055118110236227702, -0.6692913385826771977, 8.415575281601705876E-17 ) ) ;
#41068=CARTESIAN_POINT ( 'NONE',  ( -0.1640419947506553400, -0.08942795157528024563, -0.3641732283464568787 ) ) ;
#41069=CARTESIAN_POINT ( 'NONE',  ( -1.174540682414697335, -0.05778040916215522460, 0.4822834645669289988 ) ) ;
#41070=CARTESIAN_POINT ( 'NONE',  ( 1.515748031496063186, -0.5400638737290845981, -0.3530559997133363437 ) ) ;
#41074=EDGE_CURVE ( 'NONE', #24808, #24707, #68354, .T. ) ;
#41076=CARTESIAN_POINT ( 'NONE',  ( 1.010498687664042716, 0.05413385826771626580, -0.4176697321401330321 ) ) ;
#41077=CARTESIAN_POINT ( 'NONE',  ( 1.509186351706037543, -0.3690944881889765550, -0.3153832671262227771 ) ) ;
#41078=CARTESIAN_POINT ( 'NONE',  ( -1.003937007874014853, 0.07958543189024085140, 0.2665933059059887866 ) ) ;
#41079=CARTESIAN_POINT ( 'NONE',  ( -1.003937007874014853, 0.1660481256975885056, 0.3530559997133364547 ) ) ;
#41082=CARTESIAN_POINT ( 'NONE',  ( 1.391076115485564868, 0.2306618581243847221, -0.2411417322834647770 ) ) ;
#41083=CARTESIAN_POINT ( 'NONE',  ( -1.548556430446193399, 0.2306618581243848609, 0.2411417322834645549 ) ) ;
#41084=CARTESIAN_POINT ( 'NONE',  ( -0.2755905511811018171, 0.2952755905511811885, 0.000000000000000000 ) ) ;
#41085=CARTESIAN_POINT ( 'NONE',  ( -0.01968503937007793844, -0.5400638737290844871, 0.3530559997133364547 ) ) ;
#41086=CARTESIAN_POINT ( 'NONE',  ( -1.056430446194224881, -0.6692913385826771977, 0.1292274648535927661 ) ) ;
#41088=CARTESIAN_POINT ( 'NONE',  ( -0.006561679790025524116, -0.3162353388693405765, 0.4822834645669290543 ) ) ;
#41090=CARTESIAN_POINT ( 'NONE',  ( -1.299212598425196097, 0.1771653543307087630, 0.000000000000000000 ) ) ;
#41091=ORIENTED_EDGE ( 'NONE', *, *, #10113, .T. ) ;
#41094=DIRECTION ( 'NONE',  ( -0.7071067811865472397, -0.000000000000000000, -0.7071067811865476838 ) ) ;
#41096=CARTESIAN_POINT ( 'NONE',  ( -1.443569553805773564, -0.6046776061558807314, 0.2411417322834647770 ) ) ;
#41097=CARTESIAN_POINT ( 'NONE',  ( 1.391076115485564868, -0.6046776061558807314, 0.2411417322834647770 ) ) ;
#41099=CARTESIAN_POINT ( 'NONE',  ( -1.535433070866141225, 0.2952755905511811885, 0.000000000000000000 ) ) ;
#41101=CARTESIAN_POINT ( 'NONE',  ( 2.795275590551181466, 2.362204724409448620, 0.000000000000000000 ) ) ;
#41104=CARTESIAN_POINT ( 'NONE',  ( -0.2952755905511803003, -0.4536011799217368745, -0.2665933059059886201 ) ) ;
#41105=CARTESIAN_POINT ( 'NONE',  ( -0.9711286089238838626, -0.5023911411419708095, 0.1820866141732285504 ) ) ;
#41106=CARTESIAN_POINT ( 'NONE',  ( -1.102362204724408601, -0.1870078740157480879, -0.4822834645669291653 ) ) ;
#41107=CARTESIAN_POINT ( 'NONE',  ( 1.036745406824147508, -0.4281496062992127816, -0.4176697321401328100 ) ) ;
#41108=CARTESIAN_POINT ( 'NONE',  ( -1.030183727034119867, -0.3162353388693405765, 0.4822834645669290543 ) ) ;
#41110=ORIENTED_EDGE ( 'NONE', *, *, #61921, .T. ) ;
#41111=CARTESIAN_POINT ( 'NONE',  ( -1.404199475065615932, -0.4281496062992127816, -0.4176697321401328100 ) ) ;
#41112=CARTESIAN_POINT ( 'NONE',  ( -1.606188285223383527, 0.2952475903453252171, -0.04693825581093245825 ) ) ;
#41117=CARTESIAN_POINT ( 'NONE',  ( -0.3608923884514428360, 0.2952755905511811885, 0.1292274648535926551 ) ) ;
#41118=CARTESIAN_POINT ( 'NONE',  ( 1.594488188976378673, -0.5400638737290845981, -0.3530559997133363437 ) ) ;
#41120=CYLINDRICAL_SURFACE ( 'NONE', #19382, 1.181102362204724310 ) ;
#41122=CARTESIAN_POINT ( 'NONE',  ( -1.279527559055116948, -0.5400638737290844871, 0.3530559997133364547 ) ) ;
#41123=CARTESIAN_POINT ( 'NONE',  ( -0.8661417322834640276, -0.1870078740157480879, -0.4822834645669291653 ) ) ;
#41125=CARTESIAN_POINT ( 'NONE',  ( 0.4330708661417329575, -0.5511811023622047445, 6.969142054262312111E-17 ) ) ;
#41127=CARTESIAN_POINT ( 'NONE',  ( 0.2034120734908144990, -0.5511811023622046335, 0.09757992244046803654 ) ) ;
#41128=CARTESIAN_POINT ( 'NONE',  ( 0.8858267716535438430, -0.4536011799217368745, -0.2665933059059886201 ) ) ;
#41129=CARTESIAN_POINT ( 'NONE',  ( 0.9776902887139113929, 0.2952755905511811885, 0.1292274648535926551 ) ) ;
#41130=CARTESIAN_POINT ( 'NONE',  ( -0.2099737532808391705, 0.1283753931104748280, 0.1820866141732283561 ) ) ;
#41132=CARTESIAN_POINT ( 'NONE',  ( -1.391076115485563314, -0.6046776061558809534, -0.2411417322834644161 ) ) ;
#41133=CARTESIAN_POINT ( 'NONE',  ( -0.03937007874015669567, -0.5511811023622047445, 6.969142054262312111E-17 ) ) ;
#41134=CARTESIAN_POINT ( 'NONE',  ( -1.213910761154854745, -0.5511811023622046335, 0.09757992244046803654 ) ) ;
#41137=CARTESIAN_POINT ( 'NONE',  ( -0.9251968503937002541, -0.4536011799217368745, -0.2665933059059886201 ) ) ;
#41138=CARTESIAN_POINT ( 'NONE',  ( -0.04593175853018302557, 0.2952755905511811885, 0.1292274648535926551 ) ) ;
#41140=CARTESIAN_POINT ( 'NONE',  ( 0.3346456692913390985, 0.07958543189024085140, 0.2665933059059887866 ) ) ;
#41141=CARTESIAN_POINT ( 'NONE',  ( -0.3412073490813641308, -0.5023911411419708095, 0.1820866141732285504 ) ) ;
#41142=CARTESIAN_POINT ( 'NONE',  ( -0.8595800524934373854, -0.05778040916215522460, 0.4822834645669289988 ) ) ;
#41143=CARTESIAN_POINT ( 'NONE',  ( -1.699475065616797398, 0.2952755905511811885, 0.1292274648535926551 ) ) ;
#41144=CARTESIAN_POINT ( 'NONE',  ( -1.233595800524933894, -0.5023911411419708095, -0.1820866141732282451 ) ) ;
#41146=CARTESIAN_POINT ( 'NONE',  ( 0.6364829396325465405, -0.3162353388693409650, -0.4822834645669289433 ) ) ;
#41148=CARTESIAN_POINT ( 'NONE',  ( 1.476377952755906220, 0.1660481256975883668, -0.3530559997133364547 ) ) ;
#41149=CARTESIAN_POINT ( 'NONE',  ( -0.3871391076115479057, -0.2845877964562161244, -0.3641732283464567121 ) ) ;
#41151=CARTESIAN_POINT ( 'NONE',  ( -0.1443569553805768291, 0.05413385826771666132, 0.4176697321401328100 ) ) ;
#41152=CARTESIAN_POINT ( 'NONE',  ( -1.482939632545930975, 0.05413385826771666132, 0.4176697321401328100 ) ) ;
#41153=CARTESIAN_POINT ( 'NONE',  ( -1.640419947506561060, -0.004921259842519576551, 0.3153832671262227771 ) ) ;
#41154=CARTESIAN_POINT ( 'NONE',  ( 1.181102362204725198, -0.1870078740157479769, 0.4822834645669291653 ) ) ;
#41155=CARTESIAN_POINT ( 'NONE',  ( -0.4790026246719154557, -0.2845877964562159024, 0.3641732283464567677 ) ) ;
#41160=CARTESIAN_POINT ( 'NONE',  ( 1.332020997375328974, -0.08942795157528024563, -0.3641732283464568787 ) ) ;
#41161=CARTESIAN_POINT ( 'NONE',  ( -1.581364829396324945, -0.3162353388693405765, 0.4822834645669290543 ) ) ;
#41162=CARTESIAN_POINT ( 'NONE',  ( 0.6889763779527563470, 0.1660481256975883668, -0.3530559997133364547 ) ) ;
#41164=CARTESIAN_POINT ( 'NONE',  ( 1.213910761154856299, 0.1771653543307087630, 0.09757992244046791164 ) ) ;
#41166=CARTESIAN_POINT ( 'NONE',  ( 0.03937007874015833325, -0.6692913385826771977, 8.415575281601705876E-17 ) ) ;
#41167=CARTESIAN_POINT ( 'NONE',  ( -0.3543307086614165824, 0.2952755905511811885, 0.000000000000000000 ) ) ;
#41168=DIRECTION ( 'NONE',  ( -0.000000000000000000, -1.000000000000000000, -0.000000000000000000 ) ) ;
#41171=CARTESIAN_POINT ( 'NONE',  ( 0.1640419947506569498, -0.08942795157527998196, 0.3641732283464567121 ) ) ;
#41176=CARTESIAN_POINT ( 'NONE',  ( -0.6167979002624665030, 0.05413385826771666132, 0.4176697321401328100 ) ) ;
#41177=CARTESIAN_POINT ( 'NONE',  ( 1.167979002624672580, 0.05413385826771626580, -0.4176697321401330321 ) ) ;
#41178=CARTESIAN_POINT ( 'NONE',  ( 0.3543307086614181922, -0.6692913385826771977, 8.415575281601705876E-17 ) ) ;
#41179=CARTESIAN_POINT ( 'NONE',  ( -0.4527559055118102749, -0.4536011799217368745, -0.2665933059059886201 ) ) ;
#41180=CARTESIAN_POINT ( 'NONE',  ( 0.9842519685039378130, -0.6692913385826771977, 8.415575281601705876E-17 ) ) ;
#41181=CARTESIAN_POINT ( 'NONE',  ( -1.062992125984250968, -0.6692913385826771977, 8.415575281601705876E-17 ) ) ;
#41182=CARTESIAN_POINT ( 'NONE',  ( -0.2165354330708654795, -0.5400638737290845981, -0.3530559997133363437 ) ) ;
#41183=CARTESIAN_POINT ( 'NONE',  ( -0.9317585301837263412, 0.05413385826771666132, 0.4176697321401328100 ) ) ;
#41184=CARTESIAN_POINT ( 'NONE',  ( 1.318897637795276356, 0.1660481256975883668, -0.3530559997133364547 ) ) ;
#41185=CARTESIAN_POINT ( 'NONE',  ( 0.7742782152230978099, -0.4281496062992124485, 0.4176697321401328655 ) ) ;
#41186=CARTESIAN_POINT ( 'NONE',  ( 0.7545931758530189937, 0.2952755905511810774, -0.1292274648535930714 ) ) ;
#41188=CARTESIAN_POINT ( 'NONE',  ( -0.1181102362204717315, -0.5511811023622047445, 6.969142054262312111E-17 ) ) ;
#41192=CARTESIAN_POINT ( 'NONE',  ( -0.8005249343832013809, -0.3690944881889763329, 0.3153832671262228327 ) ) ;
#41195=CARTESIAN_POINT ( 'NONE',  ( 0.06561679790026316017, -0.4281496062992124485, 0.4176697321401328655 ) ) ;
#41197=CARTESIAN_POINT ( 'NONE',  ( -0.3805774278215216522, -0.4281496062992127816, -0.4176697321401328100 ) ) ;
#41198=CARTESIAN_POINT ( 'NONE',  ( -0.3740157480314953431, -0.5400638737290845981, -0.3530559997133363437 ) ) ;
#41199=CARTESIAN_POINT ( 'NONE',  ( -1.259842519685038686, -0.1870078740157480879, -0.4822834645669291653 ) ) ;
#41200=CARTESIAN_POINT ( 'NONE',  ( -1.515748031496062076, 0.1660481256975883668, -0.3530559997133364547 ) ) ;
#41201=CARTESIAN_POINT ( 'NONE',  ( 1.555118110236221041, 0.07958543189024071263, -0.2665933059059888421 ) ) ;
#41204=CARTESIAN_POINT ( 'NONE',  ( 0.6824146981627303710, 0.1283753931104746893, -0.1820866141732285504 ) ) ;
#41205=CARTESIAN_POINT ( 'NONE',  ( -0.1181102362204717315, -0.6692913385826771977, 8.415575281601705876E-17 ) ) ;
#41206=CARTESIAN_POINT ( 'NONE',  ( 0.5249343832021005074, -0.6046776061558807314, 0.2411417322834647770 ) ) ;
#41213=CARTESIAN_POINT ( 'NONE',  ( -0.5905511811023615998, 0.2952755905511811885, 0.000000000000000000 ) ) ;
#41216=CARTESIAN_POINT ( 'NONE',  ( -1.653543307086613234, -0.1870078740157479769, 0.3641732283464567677 ) ) ;
#41217=CARTESIAN_POINT ( 'NONE',  ( 0.7611548556430451917, -0.6046776061558807314, 0.2411417322834647770 ) ) ;
#41219=CARTESIAN_POINT ( 'NONE',  ( 0.9711286089238851948, -0.6046776061558809534, -0.2411417322834644161 ) ) ;
#41220=CARTESIAN_POINT ( 'NONE',  ( -0.4068241469816264999, -0.3690944881889763329, 0.3153832671262228327 ) ) ;
#41221=CARTESIAN_POINT ( 'NONE',  ( -0.1312335958005241554, 0.2306618581243848609, 0.2411417322834645549 ) ) ;
#41223=CARTESIAN_POINT ( 'NONE',  ( 0.1181102362204730916, 0.1771653543307087630, 0.000000000000000000 ) ) ;
#41224=CARTESIAN_POINT ( 'NONE',  ( -0.5839895013123351797, 0.2952755905511810774, -0.1292274648535930714 ) ) ;
#41226=CARTESIAN_POINT ( 'NONE',  ( -1.633858267716534529, -0.5400638737290845981, -0.3530559997133363437 ) ) ;
#41227=CARTESIAN_POINT ( 'NONE',  ( -0.01312335958005186876, -0.3690944881889763329, 0.3153832671262228327 ) ) ;
#41228=CARTESIAN_POINT ( 'NONE',  ( 1.515748031496063408, 0.07958543189024085140, 0.2665933059059887866 ) ) ;
#41229=CARTESIAN_POINT ( 'NONE',  ( -1.076115485564303809, 0.2306618581243848609, 0.2411417322834645549 ) ) ;
#41230=CARTESIAN_POINT ( 'NONE',  ( -0.5446194225721777693, -0.08942795157527998196, 0.3641732283464567121 ) ) ;
#41231=CARTESIAN_POINT ( 'NONE',  ( -1.586052503253848389, 0.7480314960629931287, -0.1653254495020559933 ) ) ;
#41232=CARTESIAN_POINT ( 'NONE',  ( -1.364829396325458521, 0.2306618581243847221, -0.2411417322834647770 ) ) ;
#41233=CARTESIAN_POINT ( 'NONE',  ( 0.1509186351706045259, -0.05778040916215560624, -0.4822834645669293319 ) ) ;
#41237=CARTESIAN_POINT ( 'NONE',  ( 0.2887139107611556010, 0.1283753931104746893, -0.1820866141732285504 ) ) ;
#41238=CARTESIAN_POINT ( 'NONE',  ( 0.8792650918635177559, -0.4281496062992127816, -0.4176697321401328100 ) ) ;
#41239=CARTESIAN_POINT ( 'NONE',  ( -1.056430446194224881, 0.1771653543307087075, -0.09757992244046823083 ) ) ;
#41240=CARTESIAN_POINT ( 'NONE',  ( 1.292650918635171564, -0.6692913385826773087, -0.1292274648535924053 ) ) ;
#41241=CARTESIAN_POINT ( 'NONE',  ( -1.371391076115484831, 0.1771653543307087075, -0.09757992244046823083 ) ) ;
#41243=CARTESIAN_POINT ( 'NONE',  ( -0.5249343832020990641, -0.6046776061558809534, -0.2411417322834644161 ) ) ;
#41244=CARTESIAN_POINT ( 'NONE',  ( 0.05249343832021075018, -0.5023911411419708095, 0.1820866141732285504 ) ) ;
#41245=CARTESIAN_POINT ( 'NONE',  ( 1.608925997164302624, 0.2886606758775757675, -0.09234068394397736135 ) ) ;
#41246=CARTESIAN_POINT ( 'NONE',  ( 0.7874015748031503170, -0.1870078740157479769, 0.3641732283464567677 ) ) ;
#41247=CARTESIAN_POINT ( 'NONE',  ( 0.03937007874015833325, -0.6692913385826771977, 8.415575281601705876E-17 ) ) ;
#41249=CARTESIAN_POINT ( 'NONE',  ( -0.7152230971128602510, -0.05778040916215560624, -0.4822834645669293319 ) ) ;
#41250=VECTOR ( 'NONE', #44491, 39.37007874015748854 ) ;
#41252=CARTESIAN_POINT ( 'NONE',  ( 0.9383202099737536495, -0.2845877964562159024, 0.3641732283464567677 ) ) ;
#41253=CARTESIAN_POINT ( 'NONE',  ( 0.1902887139107617975, -0.6692913385826773087, -0.1292274648535924053 ) ) ;
#41254=CONICAL_SURFACE ( 'NONE', #43931, 2.362204724409449508, 0.8582239808723030050 ) ;
#41255=CARTESIAN_POINT ( 'NONE',  ( -0.3937007874015740483, -0.1870078740157479769, 0.4822834645669291653 ) ) ;
#41256=CARTESIAN_POINT ( 'NONE',  ( -0.2952755905511803003, -0.4536011799217368745, -0.2665933059059886201 ) ) ;
#41258=CARTESIAN_POINT ( 'NONE',  ( -0.6299212598425188991, -0.1870078740157480601, -0.3641732283464567677 ) ) ;
#41259=CARTESIAN_POINT ( 'NONE',  ( 0.5577427821522316087, -0.05778040916215522460, 0.4822834645669289988 ) ) ;
#41260=CARTESIAN_POINT ( 'NONE',  ( -0.8858267716535425107, 0.07958543189024071263, -0.2665933059059888421 ) ) ;
#41262=CARTESIAN_POINT ( 'NONE',  ( -1.305774278215222184, 0.2952755905511811885, 0.1292274648535926551 ) ) ;
#41263=CARTESIAN_POINT ( 'NONE',  ( -0.8554425558739509050, -4.966502543501560364E-15, 0.4118484887281982920 ) ) ;
#41264=VERTEX_POINT ( 'NONE', #63307 ) ;
#41265=CARTESIAN_POINT ( 'NONE',  ( -0.9776902887139098386, -0.5511811023622046335, 0.09757992244046803654 ) ) ;
#41266=CARTESIAN_POINT ( 'NONE',  ( -0.2821522309711278487, 0.2952755905511811885, 0.1292274648535926551 ) ) ;
#41267=CARTESIAN_POINT ( 'NONE',  ( -1.706036745406823485, 0.2306618581243848609, 0.2411417322834645549 ) ) ;
#41268=CARTESIAN_POINT ( 'NONE',  ( -1.181102362204723644, -0.1870078740157479769, 0.4822834645669291653 ) ) ;
#41269=CARTESIAN_POINT ( 'NONE',  ( 1.614173228346456712, 2.401574803149606474, 0.1372047244094478646 ) ) ;
#41270=CARTESIAN_POINT ( 'NONE',  ( 1.456692913385827515, -0.6692913385826771977, 8.415575281601705876E-17 ) ) ;
#41271=CARTESIAN_POINT ( 'NONE',  ( 0.9973753280839902091, -0.6046776061558807314, 0.2411417322834647770 ) ) ;
#41272=FACE_OUTER_BOUND ( 'NONE', #16266, .T. ) ;
#41273=CARTESIAN_POINT ( 'NONE',  ( -1.436417322834643739, 0.4405861044731112508, -0.3149606299212598381 ) ) ;
#41274=CARTESIAN_POINT ( 'NONE',  ( 1.489501312335958172, -0.08942795157528024563, -0.3641732283464568787 ) ) ;
#41277=CARTESIAN_POINT ( 'NONE',  ( -0.4330708661417315697, -0.5511811023622047445, 6.969142054262312111E-17 ) ) ;
#41279=ORIENTED_EDGE ( 'NONE', *, *, #21598, .F. ) ;
#41280=CARTESIAN_POINT ( 'NONE',  ( 0.9776902887139113929, 0.2952755905511811885, 0.1292274648535926551 ) ) ;
#41281=CARTESIAN_POINT ( 'NONE',  ( 0.01312335958005323398, 0.05413385826771666132, 0.4176697321401328100 ) ) ;
#41282=CARTESIAN_POINT ( 'NONE',  ( -0.6496062992125976043, 0.1660481256975883668, -0.3530559997133364547 ) ) ;
#41283=CARTESIAN_POINT ( 'NONE',  ( 1.397637795275591177, 0.1660481256975883668, -0.3530559997133364547 ) ) ;
#41284=CARTESIAN_POINT ( 'NONE',  ( -1.305774278215222184, 0.1771653543307087630, 0.09757992244046791164 ) ) ;
#41286=CARTESIAN_POINT ( 'NONE',  ( 0.5118110236220480003, -0.6692913385826771977, 8.415575281601705876E-17 ) ) ;
#41287=CARTESIAN_POINT ( 'NONE',  ( 0.7086614173228352742, -0.1870078740157480601, -0.3641732283464567677 ) ) ;
#41288=CARTESIAN_POINT ( 'NONE',  ( -0.7086614173228339419, -0.1870078740157479769, 0.4822834645669291653 ) ) ;
#41290=CARTESIAN_POINT ( 'NONE',  ( -1.338582677165353729, -0.1870078740157479769, 0.4822834645669291653 ) ) ;
#41292=CARTESIAN_POINT ( 'NONE',  ( 1.017060367454068803, -0.3162353388693405765, 0.4822834645669290543 ) ) ;
#41293=CARTESIAN_POINT ( 'NONE',  ( 1.213910761154856299, 0.1771653543307087630, 0.09757992244046791164 ) ) ;
#41294=VERTEX_POINT ( 'NONE', #19099 ) ;
#41296=CARTESIAN_POINT ( 'NONE',  ( -0.2624671916010490880, -0.6046776061558807314, 0.2411417322834647770 ) ) ;
#41298=CARTESIAN_POINT ( 'NONE',  ( 0.2690288713910767848, -0.5511811023622048555, -0.09757992244046775898 ) ) ;
#41299=CARTESIAN_POINT ( 'NONE',  ( -1.181102362204723644, -0.1870078740157480879, -0.4822834645669291653 ) ) ;
#41300=CARTESIAN_POINT ( 'NONE',  ( 0.8923884514435701520, -0.6046776061558809534, -0.2411417322834644161 ) ) ;
#41301=CARTESIAN_POINT ( 'NONE',  ( 0.9776902887139113929, 0.2952755905511811885, 0.1292274648535926551 ) ) ;
#41302=CARTESIAN_POINT ( 'NONE',  ( -0.1902887139107604098, -0.6692913385826771977, 0.1292274648535927661 ) ) ;
#41303=CARTESIAN_POINT ( 'NONE',  ( -0.8858267716535425107, -0.5400638737290844871, 0.3530559997133364547 ) ) ;
#41305=CARTESIAN_POINT ( 'NONE',  ( -1.555118110236219930, 0.1660481256975885056, 0.3530559997133364547 ) ) ;
#41306=CARTESIAN_POINT ( 'NONE',  ( -0.6167979002624665030, -0.4281496062992127816, -0.4176697321401328100 ) ) ;
#41307=CARTESIAN_POINT ( 'NONE',  ( -0.4002624671916004129, -0.2845877964562159024, 0.3641732283464567677 ) ) ;
#41308=CARTESIAN_POINT ( 'NONE',  ( 1.450131233595801428, -0.6692913385826773087, -0.1292274648535924053 ) ) ;
#41309=CARTESIAN_POINT ( 'NONE',  ( 1.443569553805774897, -0.6046776061558809534, -0.2411417322834644161 ) ) ;
#41311=CARTESIAN_POINT ( 'NONE',  ( -0.9186351706036736120, 0.2306618581243848609, 0.2411417322834645549 ) ) ;
#41312=DIRECTION ( 'NONE',  ( 1.000000000000000000, 3.096699300667737957E-16, -1.692413147294446216E-16 ) ) ;
#41315=CARTESIAN_POINT ( 'NONE',  ( 0.5052493438320215802, 0.2952755905511811885, 0.1292274648535926551 ) ) ;
#41318=ADVANCED_FACE ( 'NONE', ( #43519 ), #41254, .F. ) ;
#41319=CARTESIAN_POINT ( 'NONE',  ( -0.03280839895013062252, 0.2952755905511810774, -0.1292274648535930714 ) ) ;
#41320=AXIS2_PLACEMENT_3D ( 'NONE', #41559, #54173, #21379 ) ;
#41321=CARTESIAN_POINT ( 'NONE',  ( -1.062992125984250968, -0.5511811023622047445, 6.969142054262312111E-17 ) ) ;
#41322=CARTESIAN_POINT ( 'NONE',  ( 1.036745406824147731, -0.004921259842519576551, 0.3153832671262227771 ) ) ;
#41324=CARTESIAN_POINT ( 'NONE',  ( 1.233595800524935227, 0.1283753931104746893, -0.1820866141732285504 ) ) ;
#41325=CARTESIAN_POINT ( 'NONE',  ( 0.7545931758530188826, -0.6692913385826771977, 0.1292274648535927661 ) ) ;
#41328=CARTESIAN_POINT ( 'NONE',  ( -0.5052493438320203589, -0.6692913385826771977, 0.1292274648535927661 ) ) ;
#41330=CARTESIAN_POINT ( 'NONE',  ( 1.377952755905512472, -0.5511811023622047445, 6.969142054262312111E-17 ) ) ;
#41331=CARTESIAN_POINT ( 'NONE',  ( -0.4265091863517051496, 0.2952755905511810774, -0.1292274648535930714 ) ) ;
#41333=CARTESIAN_POINT ( 'NONE',  ( 1.456692913385827515, -0.6692913385826771977, 8.415575281601705876E-17 ) ) ;
#41334=CARTESIAN_POINT ( 'NONE',  ( 0.1312335958005255154, -0.6046776061558807314, 0.2411417322834647770 ) ) ;
#41335=CARTESIAN_POINT ( 'NONE',  ( 0.6496062992125991586, -0.4536011799217368745, -0.2665933059059886201 ) ) ;
#41337=CARTESIAN_POINT ( 'NONE',  ( 0.5905511811023629321, 0.1771653543307087630, 0.000000000000000000 ) ) ;
#41338=CARTESIAN_POINT ( 'NONE',  ( -1.653543307086613234, -0.1870078740157479769, 0.4822834645669291653 ) ) ;
#41340=CARTESIAN_POINT ( 'NONE',  ( 0.6692913385826778638, -0.6692913385826771977, 8.415575281601705876E-17 ) ) ;
#41343=CARTESIAN_POINT ( 'NONE',  ( 1.581364829396326277, -0.2845877964562161244, -0.3641732283464567121 ) ) ;
#41344=CARTESIAN_POINT ( 'NONE',  ( -0.1574803149606292529, -0.1870078740157479769, 0.3641732283464567677 ) ) ;
#41345=CARTESIAN_POINT ( 'NONE',  ( 0.1181102362204730916, 0.2952755905511811885, 0.000000000000000000 ) ) ;
#41346=CARTESIAN_POINT ( 'NONE',  ( 1.410761154855643795, -0.08942795157528024563, -0.3641732283464568787 ) ) ;
#41347=CARTESIAN_POINT ( 'NONE',  ( -1.541994750656167090, 0.1771653543307087630, 0.09757992244046791164 ) ) ;
#41348=CARTESIAN_POINT ( 'NONE',  ( -1.312335958005248715, -0.6046776061558809534, -0.2411417322834644161 ) ) ;
#41349=CARTESIAN_POINT ( 'NONE',  ( 0.6889763779527566800, -0.5400638737290844871, 0.3530559997133364547 ) ) ;
#41350=CARTESIAN_POINT ( 'NONE',  ( 1.633858267716535639, -0.5400638737290844871, 0.3530559997133364547 ) ) ;
#41352=CARTESIAN_POINT ( 'NONE',  ( 0.6299212598425204535, -0.1870078740157479769, 0.4822834645669291653 ) ) ;
#41353=CARTESIAN_POINT ( 'NONE',  ( 1.437007874015748810, -0.5400638737290845981, -0.3530559997133363437 ) ) ;
#41354=CARTESIAN_POINT ( 'NONE',  ( 0.9120734908136490793, 0.2952755905511810774, -0.1292274648535930714 ) ) ;
#41355=CARTESIAN_POINT ( 'NONE',  ( -1.692913385826770645, 0.1771653543307087630, 0.000000000000000000 ) ) ;
#41356=CARTESIAN_POINT ( 'NONE',  ( 0.9317585301837276734, -0.004921259842519870586, -0.3153832671262229437 ) ) ;
#41357=CARTESIAN_POINT ( 'NONE',  ( 1.679790026246720025, 0.2306618581243848609, 0.2411417322834645549 ) ) ;
#41358=CARTESIAN_POINT ( 'NONE',  ( -0.9055118110236215490, -0.5511811023622047445, 6.969142054262312111E-17 ) ) ;
#41359=CARTESIAN_POINT ( 'NONE',  ( 0.6692913385826777528, 0.1771653543307087630, 0.000000000000000000 ) ) ;
#41360=CARTESIAN_POINT ( 'NONE',  ( 0.2559055118110243332, 0.1660481256975885056, 0.3530559997133364547 ) ) ;
#41361=CARTESIAN_POINT ( 'NONE',  ( 0.7480314960629927956, -0.6692913385826771977, 8.415575281601705876E-17 ) ) ;
#41362=CARTESIAN_POINT ( 'NONE',  ( -0.1837270341207340729, 0.2306618581243847221, -0.2411417322834647770 ) ) ;
#41363=CARTESIAN_POINT ( 'NONE',  ( 0.1115485564304467270, -0.5511811023622048555, -0.09757992244046775898 ) ) ;
#41364=CARTESIAN_POINT ( 'NONE',  ( 1.207349081364829990, -0.6046776061558809534, -0.2411417322834644161 ) ) ;
#41366=CARTESIAN_POINT ( 'NONE',  ( -1.043307086614172707, 0.1660481256975883668, -0.3530559997133364547 ) ) ;
#41369=AXIS2_PLACEMENT_3D ( 'NONE', #14768, #71579, #13930 ) ;
#41370=CARTESIAN_POINT ( 'NONE',  ( -0.6824146981627288167, 0.2306618581243848609, 0.2411417322834645549 ) ) ;
#41371=CARTESIAN_POINT ( 'NONE',  ( -0.5971128608923877978, 0.2952755905511811885, 0.1292274648535926551 ) ) ;
#41374=ORIENTED_EDGE ( 'NONE', *, *, #5920, .F. ) ;
#41375=CARTESIAN_POINT ( 'NONE',  ( 0.7611548556430454138, 0.1283753931104746893, -0.1820866141732285504 ) ) ;
#41377=CARTESIAN_POINT ( 'NONE',  ( 1.122047244094488860, 0.1660481256975885056, 0.3530559997133364547 ) ) ;
#41378=CARTESIAN_POINT ( 'NONE',  ( -1.646051170424378096, 0.8346805926620876059, -0.3149606299212598381 ) ) ;
#41379=CARTESIAN_POINT ( 'NONE',  ( -1.332020997375327642, -0.2845877964562161244, -0.3641732283464567121 ) ) ;
#41381=CARTESIAN_POINT ( 'NONE',  ( 1.607611548556431069, 0.1771653543307087630, 0.09757992244046791164 ) ) ;
#41384=CARTESIAN_POINT ( 'NONE',  ( -0.05249343832020911260, 0.2306618581243848609, 0.2411417322834645549 ) ) ;
#41385=CARTESIAN_POINT ( 'NONE',  ( -0.3412073490813641308, -0.5023911411419708095, 0.1820866141732285504 ) ) ;
#41386=CARTESIAN_POINT ( 'NONE',  ( 0.7742782152230978099, -0.4281496062992124485, 0.4176697321401328655 ) ) ;
#41387=CARTESIAN_POINT ( 'NONE',  ( 0.02624671916010564918, 0.2306618581243848609, 0.2411417322834645549 ) ) ;
#41389=CARTESIAN_POINT ( 'NONE',  ( -0.01149616601327268020, 1.490381362800744269E-15, -0.3791475997938222320 ) ) ;
#41391=CARTESIAN_POINT ( 'NONE',  ( 0.8595800524934390507, -0.3162353388693405765, 0.4822834645669290543 ) ) ;
#41392=CARTESIAN_POINT ( 'NONE',  ( 0.1837270341207354329, 0.2306618581243848609, 0.2411417322834645549 ) ) ;
#41393=CARTESIAN_POINT ( 'NONE',  ( -1.167979002624671470, 0.05413385826771666132, 0.4176697321401328100 ) ) ;
#41394=CARTESIAN_POINT ( 'NONE',  ( 0.9186351706036751663, -0.6046776061558807314, 0.2411417322834647770 ) ) ;
#41395=CARTESIAN_POINT ( 'NONE',  ( 0.9186351706036752773, 0.2306618581243847221, -0.2411417322834647770 ) ) ;
#41397=CARTESIAN_POINT ( 'NONE',  ( -0.2493438320209966919, 0.05413385826771626580, -0.4176697321401330321 ) ) ;
#41398=CARTESIAN_POINT ( 'NONE',  ( 0.7808398950131241190, -0.05778040916215560624, -0.4822834645669293319 ) ) ;
#41399=CARTESIAN_POINT ( 'NONE',  ( -0.04593175853018302557, 0.2952755905511811885, 0.1292274648535926551 ) ) ;
#41400=CARTESIAN_POINT ( 'NONE',  ( 0.6824146981627303710, -0.5023911411419708095, 0.1820866141732285504 ) ) ;
#41401=CARTESIAN_POINT ( 'NONE',  ( -1.364829396325458521, 0.2306618581243847221, -0.2411417322834647770 ) ) ;
#41402=CARTESIAN_POINT ( 'NONE',  ( -1.679790026246718693, 0.2306618581243847221, -0.2411417322834647770 ) ) ;
#41403=CARTESIAN_POINT ( 'NONE',  ( 0.1377952755905518800, -0.5400638737290844871, 0.3530559997133364547 ) ) ;
#41408=CARTESIAN_POINT ( 'NONE',  ( 0.9711286089238851948, -0.6046776061558809534, -0.2411417322834644161 ) ) ;
#41409=CARTESIAN_POINT ( 'NONE',  ( 0.5971128608923890191, -0.5511811023622046335, 0.09757992244046803654 ) ) ;
#41412=CARTESIAN_POINT ( 'NONE',  ( 2.795275590551181466, 2.204724409448820310, 0.000000000000000000 ) ) ;
#41416=CARTESIAN_POINT ( 'NONE',  ( -0.7939632545931750718, -0.05778040916215560624, -0.4822834645669293319 ) ) ;
#41417=CARTESIAN_POINT ( 'NONE',  ( -0.7808398950131225646, -0.05778040916215522460, 0.4822834645669289988 ) ) ;
#41418=CARTESIAN_POINT ( 'NONE',  ( 1.089238845144357537, -0.4281496062992124485, 0.4176697321401328655 ) ) ;
#41420=CARTESIAN_POINT ( 'NONE',  ( 1.161417322834646271, 0.1660481256975883668, -0.3530559997133364547 ) ) ;
#41422=CARTESIAN_POINT ( 'NONE',  ( 1.666666666666667185, -0.004921259842519576551, 0.3153832671262227771 ) ) ;
#41424=CARTESIAN_POINT ( 'NONE',  ( -1.351706036745406347, -0.3690944881889763329, 0.3153832671262228327 ) ) ;
#41426=CARTESIAN_POINT ( 'NONE',  ( 0.09186351706036827158, 0.05413385826771666132, 0.4176697321401328100 ) ) ;
#41429=CARTESIAN_POINT ( 'NONE',  ( -1.646051170424378096, 0.8346805926620876059, 0.3149606299212598381 ) ) ;
#41430=CARTESIAN_POINT ( 'NONE',  ( -0.9645669291338575535, -0.4536011799217367080, 0.2665933059059888421 ) ) ;
#41431=CARTESIAN_POINT ( 'NONE',  ( 0.7480314960629927956, 0.2952755905511811885, 0.000000000000000000 ) ) ;
#41432=CARTESIAN_POINT ( 'NONE',  ( 1.279527559055118724, 0.07958543189024085140, 0.2665933059059887866 ) ) ;
#41434=CARTESIAN_POINT ( 'NONE',  ( -0.9186351706036736120, 0.1283753931104748280, 0.1820866141732283561 ) ) ;
#41435=CARTESIAN_POINT ( 'NONE',  ( 1.574803149606299746, -0.1870078740157480879, -0.4822834645669291653 ) ) ;
#41437=CARTESIAN_POINT ( 'NONE',  ( -0.2690288713910754526, 0.2952755905511810774, -0.1292274648535930714 ) ) ;
#41438=CARTESIAN_POINT ( 'NONE',  ( -1.397637795275589623, -0.4536011799217368745, -0.2665933059059886201 ) ) ;
#41439=CARTESIAN_POINT ( 'NONE',  ( -0.2690288713910754526, 0.1771653543307087075, -0.09757992244046823083 ) ) ;
#41440=CARTESIAN_POINT ( 'NONE',  ( -0.4724409448818890911, -0.1870078740157479769, 0.4822834645669291653 ) ) ;
#41441=CARTESIAN_POINT ( 'NONE',  ( -1.581364829396324945, -0.08942795157528024563, -0.3641732283464568787 ) ) ;
#41443=CARTESIAN_POINT ( 'NONE',  ( 0.3149606299212603933, -0.1870078740157479769, 0.4822834645669291653 ) ) ;
#41446=CARTESIAN_POINT ( 'NONE',  ( -0.5971128608923877978, 0.2952755905511811885, 0.1292274648535926551 ) ) ;
#41447=CARTESIAN_POINT ( 'NONE',  ( -0.2493438320209966919, -0.004921259842519870586, -0.3153832671262229437 ) ) ;
#41449=CARTESIAN_POINT ( 'NONE',  ( -1.279527559055116948, 0.1660481256975883668, -0.3530559997133364547 ) ) ;
#41450=CARTESIAN_POINT ( 'NONE',  ( -0.1574803149606292529, -0.1870078740157480879, -0.4822834645669291653 ) ) ;
#41451=CARTESIAN_POINT ( 'NONE',  ( 0.4724409448818904789, -0.1870078740157480601, -0.3641732283464567677 ) ) ;
#41452=CARTESIAN_POINT ( 'NONE',  ( -0.8464566929133852113, -0.4536011799217368745, -0.2665933059059886201 ) ) ;
#41453=CARTESIAN_POINT ( 'NONE',  ( -0.9120734908136475250, 0.2952755905511811885, 0.1292274648535926551 ) ) ;
#41454=CARTESIAN_POINT ( 'NONE',  ( -1.706036745406823485, 0.2306618581243848609, 0.2411417322834645549 ) ) ;
#41455=CARTESIAN_POINT ( 'NONE',  ( 1.496062992125985147, -0.1870078740157479769, 0.4822834645669291653 ) ) ;
#41457=CARTESIAN_POINT ( 'NONE',  ( 0.7152230971128616943, -0.08942795157527998196, 0.3641732283464567121 ) ) ;
#41458=CARTESIAN_POINT ( 'NONE',  ( 0.6889763779527566800, -0.5400638737290844871, 0.3530559997133364547 ) ) ;
#41460=CARTESIAN_POINT ( 'NONE',  ( 1.200787401574803681, -0.4536011799217368745, -0.2665933059059886201 ) ) ;
#41461=VERTEX_POINT ( 'NONE', #75133 ) ;
#41462=CARTESIAN_POINT ( 'NONE',  ( -0.7545931758530176614, -0.6692913385826773087, -0.1292274648535924053 ) ) ;
#41464=CARTESIAN_POINT ( 'NONE',  ( -1.377952755905511140, -0.5511811023622047445, 6.969142054262312111E-17 ) ) ;
#41465=CARTESIAN_POINT ( 'NONE',  ( -0.9908136482939626788, 0.2952755905511811885, 0.1292274648535926551 ) ) ;
#41466=CARTESIAN_POINT ( 'NONE',  ( 0.1574803149606306130, -0.1870078740157479769, 0.4822834645669291653 ) ) ;
#41467=CARTESIAN_POINT ( 'NONE',  ( -1.345144356955379816, -0.08942795157528024563, -0.3641732283464568787 ) ) ;
#41469=CARTESIAN_POINT ( 'NONE',  ( -1.397637795275589623, 0.1660481256975885056, 0.3530559997133364547 ) ) ;
#41470=CARTESIAN_POINT ( 'NONE',  ( 0.5052493438320218022, -0.6692913385826773087, -0.1292274648535924053 ) ) ;
#41471=CARTESIAN_POINT ( 'NONE',  ( 0.2755905511811031494, 0.2952755905511811885, 0.000000000000000000 ) ) ;
#41472=CARTESIAN_POINT ( 'NONE',  ( 1.305774278215223960, 0.2952755905511810774, -0.1292274648535930714 ) ) ;
#41473=CARTESIAN_POINT ( 'NONE',  ( 0.4531182788721078158, 1.535433070866141447, 0.5309055118110234117 ) ) ;
#41477=FACE_OUTER_BOUND ( 'NONE', #32174, .T. ) ;
#41479=CARTESIAN_POINT ( 'NONE',  ( -0.2099737532808391705, -0.5023911411419708095, -0.1820866141732282451 ) ) ;
#41480=CARTESIAN_POINT ( 'NONE',  ( -0.2690288713910754526, 0.2952755905511810774, -0.1292274648535930714 ) ) ;
#41481=CARTESIAN_POINT ( 'NONE',  ( 0.7086614173228352742, -0.1870078740157480879, -0.4822834645669291653 ) ) ;
#41483=CARTESIAN_POINT ( 'NONE',  ( -0.06561679790026180015, -0.004921259842519576551, 0.3153832671262227771 ) ) ;
#41484=CARTESIAN_POINT ( 'NONE',  ( -1.023622047244093558, -0.1870078740157479769, 0.4822834645669291653 ) ) ;
#41485=CARTESIAN_POINT ( 'NONE',  ( 1.240157480314961314, -0.5400638737290844871, 0.3530559997133364547 ) ) ;
#41487=CYLINDRICAL_SURFACE ( 'NONE', #45183, 0.3937007874015748254 ) ;
#41489=ORIENTED_EDGE ( 'NONE', *, *, #43698, .F. ) ;
#41490=CARTESIAN_POINT ( 'NONE',  ( 0.9776902887139113929, 0.2952755905511811885, 0.1292274648535926551 ) ) ;
#41492=CARTESIAN_POINT ( 'NONE',  ( -1.561679790026246017, 0.05413385826771666132, 0.4176697321401328100 ) ) ;
#41493=CARTESIAN_POINT ( 'NONE',  ( -1.181102362204723644, -0.1870078740157479769, 0.3641732283464567677 ) ) ;
#41494=CARTESIAN_POINT ( 'NONE',  ( -1.049868766404198794, -0.6046776061558807314, 0.2411417322834647770 ) ) ;
#41497=CARTESIAN_POINT ( 'NONE',  ( 1.154855643044620184, -0.6046776061558807314, 0.2411417322834647770 ) ) ;
#41498=CARTESIAN_POINT ( 'NONE',  ( 1.220472440944881054, 0.4405861044731111953, -0.5309055118110239668 ) ) ;
#41499=CARTESIAN_POINT ( 'NONE',  ( -0.2821522309711278487, 0.2952755905511811885, 0.1292274648535926551 ) ) ;
#41500=CARTESIAN_POINT ( 'NONE',  ( -0.4921259842519677963, -0.5400638737290844871, 0.3530559997133364547 ) ) ;
#41501=CARTESIAN_POINT ( 'NONE',  ( -1.115485564304461219, 0.05413385826771626580, -0.4176697321401330321 ) ) ;
#41503=CARTESIAN_POINT ( 'NONE',  ( 0.1377952755905518800, -0.5400638737290844871, 0.3530559997133364547 ) ) ;
#41505=CARTESIAN_POINT ( 'NONE',  ( -1.404199475065615932, -0.3690944881889765550, -0.3153832671262227771 ) ) ;
#41508=ORIENTED_EDGE ( 'NONE', *, *, #2607, .F. ) ;
#41510=CARTESIAN_POINT ( 'NONE',  ( 1.594488188976378673, 0.07958543189024085140, 0.2665933059059887866 ) ) ;
#41512=CARTESIAN_POINT ( 'NONE',  ( -1.686351706036744558, 0.2952755905511810774, -0.1292274648535930714 ) ) ;
#41514=CARTESIAN_POINT ( 'NONE',  ( -0.9842519685039360366, 0.2952755905511811885, 0.000000000000000000 ) ) ;
#41515=CARTESIAN_POINT ( 'NONE',  ( 2.795275590551181910, 1.771653543307087242, 0.000000000000000000 ) ) ;
#41517=CARTESIAN_POINT ( 'NONE',  ( -0.3346456692913377662, 0.07958543189024071263, -0.2665933059059888421 ) ) ;
#41518=CARTESIAN_POINT ( 'NONE',  ( -0.7545931758530177724, 0.1771653543307087630, 0.09757992244046791164 ) ) ;
#41519=CARTESIAN_POINT ( 'NONE',  ( -1.017060367454067249, -0.05778040916215522460, 0.4822834645669289988 ) ) ;
#41520=CARTESIAN_POINT ( 'NONE',  ( 0.4002624671916016896, -0.3162353388693409650, -0.4822834645669289433 ) ) ;
#41521=CARTESIAN_POINT ( 'NONE',  ( -0.8136482939632537770, 0.2306618581243847221, -0.2411417322834647770 ) ) ;
#41523=ORIENTED_EDGE ( 'NONE', *, *, #51624, .T. ) ;
#41524=CARTESIAN_POINT ( 'NONE',  ( -1.187664041994749731, -0.3162353388693405765, 0.4822834645669290543 ) ) ;
#41525=DIRECTION ( 'NONE',  ( 1.000000000000000000, -0.000000000000000000, -0.000000000000000000 ) ) ;
#41527=DIRECTION ( 'NONE',  ( 1.000000000000000000, 3.469446951953613203E-16, 0.000000000000000000 ) ) ;
#41530=CARTESIAN_POINT ( 'NONE',  ( -0.6955380577427815458, 0.05413385826771666132, 0.4176697321401328100 ) ) ;
#41531=CARTESIAN_POINT ( 'NONE',  ( 1.417322834645670104, -0.1870078740157480879, -0.4822834645669291653 ) ) ;
#41533=CARTESIAN_POINT ( 'NONE',  ( -0.6399301791983041943, -2.567464376874931580E-15, -0.4445507791589072832 ) ) ;
#41534=CARTESIAN_POINT ( 'NONE',  ( -0.6423408027444563739, -2.609869883881465018E-15, -0.3464511005275220379 ) ) ;
#41535=CARTESIAN_POINT ( 'NONE',  ( -1.469816272965878357, -0.6046776061558809534, -0.2411417322834644161 ) ) ;
#41536=CARTESIAN_POINT ( 'NONE',  ( -0.7480314960629914633, 0.2952755905511811885, 0.000000000000000000 ) ) ;
#41538=CARTESIAN_POINT ( 'NONE',  ( 0.5971128608923890191, -0.5511811023622046335, 0.09757992244046803654 ) ) ;
#41540=CARTESIAN_POINT ( 'NONE',  ( 0.3543307086614181922, -0.5511811023622047445, 6.969142054262312111E-17 ) ) ;
#41541=CARTESIAN_POINT ( 'NONE',  ( 1.141732283464567566, 0.1771653543307087630, 0.000000000000000000 ) ) ;
#41542=CARTESIAN_POINT ( 'NONE',  ( 1.167979002624672580, 0.05413385826771626580, -0.4176697321401330321 ) ) ;
#41543=CARTESIAN_POINT ( 'NONE',  ( -0.1115485564304453947, -0.5511811023622046335, 0.09757992244046803654 ) ) ;
#41545=CARTESIAN_POINT ( 'NONE',  ( -1.601049868766403650, 0.2306618581243847221, -0.2411417322834647770 ) ) ;
#41546=CARTESIAN_POINT ( 'NONE',  ( -1.089238845144356427, -0.3690944881889765550, -0.3153832671262227771 ) ) ;
#41548=CARTESIAN_POINT ( 'NONE',  ( -1.030183727034119867, -0.2845877964562159024, 0.3641732283464567677 ) ) ;
#41550=CARTESIAN_POINT ( 'NONE',  ( -0.02624671916010428221, 0.2306618581243847221, -0.2411417322834647770 ) ) ;
#41552=CARTESIAN_POINT ( 'NONE',  ( 0.7217847769028878924, -0.3690944881889765550, -0.3153832671262227771 ) ) ;
#41553=CARTESIAN_POINT ( 'NONE',  ( -0.1246719160104980823, 0.1771653543307087630, 0.09757992244046791164 ) ) ;
#41554=CARTESIAN_POINT ( 'NONE',  ( -0.9120734908136475250, -0.6692913385826773087, -0.1292274648535924053 ) ) ;
#41555=CARTESIAN_POINT ( 'NONE',  ( -2.795275590551185907, 0.5118110236220471121, -3.981376139758521912E-16 ) ) ;
#41557=CARTESIAN_POINT ( 'NONE',  ( 0.2887139107611556010, 0.2306618581243847221, -0.2411417322834647770 ) ) ;
#41559=CARTESIAN_POINT ( 'NONE',  ( 1.220472440944882386, -0.1870078740157480046, 1.254653134982923898E-17 ) ) ;
#41560=CARTESIAN_POINT ( 'NONE',  ( -0.3543307086614165824, -0.5511811023622047445, 6.969142054262312111E-17 ) ) ;
#41561=CARTESIAN_POINT ( 'NONE',  ( -0.2427821522309703550, -0.05778040916215560624, -0.4822834645669293319 ) ) ;
#41562=CARTESIAN_POINT ( 'NONE',  ( -1.627296587926508442, 0.2306618581243848609, 0.2411417322834645549 ) ) ;
#41563=CARTESIAN_POINT ( 'NONE',  ( 1.502624671916010790, -0.05778040916215522460, 0.4822834645669289988 ) ) ;
#41564=CARTESIAN_POINT ( 'NONE',  ( 1.122047244094488860, -0.5400638737290845981, -0.3530559997133363437 ) ) ;
#41565=CARTESIAN_POINT ( 'NONE',  ( -0.5708661417322828946, 0.07958543189024071263, -0.2665933059059888421 ) ) ;
#41569=CARTESIAN_POINT ( 'NONE',  ( 1.614173228346457156, 1.496062992125984037, 0.5309055118110233007 ) ) ;
#41570=CARTESIAN_POINT ( 'NONE',  ( 1.174540682414699111, -0.08942795157528024563, -0.3641732283464568787 ) ) ;
#41571=CARTESIAN_POINT ( 'NONE',  ( -1.522309711286088607, 0.2306618581243847221, -0.2411417322834647770 ) ) ;
#41572=CARTESIAN_POINT ( 'NONE',  ( 0.9120734908136489683, -0.6692913385826771977, 0.1292274648535927661 ) ) ;
#41574=CARTESIAN_POINT ( 'NONE',  ( 1.115485564304462551, -0.3690944881889765550, -0.3153832671262227771 ) ) ;
#41575=CARTESIAN_POINT ( 'NONE',  ( -0.09186351706036663400, -0.4281496062992124485, 0.4176697321401328655 ) ) ;
#41576=CARTESIAN_POINT ( 'NONE',  ( -0.5183727034120726440, 0.2952755905511811885, 0.1292274648535926551 ) ) ;
#41577=DIRECTION ( 'NONE',  ( 0.000000000000000000, 0.000000000000000000, 1.000000000000000000 ) ) ;
#41580=CARTESIAN_POINT ( 'NONE',  ( 0.4396325459317590445, -0.5511811023622046335, 0.09757992244046803654 ) ) ;
#41581=ORIENTED_EDGE ( 'NONE', *, *, #56862, .F. ) ;
#41584=CARTESIAN_POINT ( 'NONE',  ( -0.5446194225721777693, -0.3162353388693409650, -0.4822834645669289433 ) ) ;
#41585=CARTESIAN_POINT ( 'NONE',  ( 1.049868766404200127, -0.6046776061558809534, -0.2411417322834644161 ) ) ;
#41586=CARTESIAN_POINT ( 'NONE',  ( 0.09186351706036827158, 0.05413385826771666132, 0.4176697321401328100 ) ) ;
#41587=CARTESIAN_POINT ( 'NONE',  ( -0.4396325459317577122, -0.5511811023622048555, -0.09757992244046775898 ) ) ;
#41588=CARTESIAN_POINT ( 'NONE',  ( 0.7349081364829403995, 0.2306618581243848609, 0.2411417322834645549 ) ) ;
#41589=CARTESIAN_POINT ( 'NONE',  ( -0.9383202099737524282, -0.3162353388693409650, -0.4822834645669289433 ) ) ;
#41590=CARTESIAN_POINT ( 'NONE',  ( -0.4461942257217840213, 0.2306618581243848609, 0.2411417322834645549 ) ) ;
#41591=CARTESIAN_POINT ( 'NONE',  ( 1.076115485564305141, -0.6046776061558807314, 0.2411417322834647770 ) ) ;
#41592=CARTESIAN_POINT ( 'NONE',  ( 0.9908136482939640111, 0.2952755905511810774, -0.1292274648535930714 ) ) ;
#41593=CARTESIAN_POINT ( 'NONE',  ( 0.9645669291338591078, -0.5400638737290845981, -0.3530559997133363437 ) ) ;
#41595=CARTESIAN_POINT ( 'NONE',  ( 0.03937007874015833325, -0.5511811023622047445, 6.969142054262312111E-17 ) ) ;
#41599=CARTESIAN_POINT ( 'NONE',  ( -0.8727034120734901146, -0.08942795157528024563, -0.3641732283464568787 ) ) ;
#41600=CARTESIAN_POINT ( 'NONE',  ( -0.5577427821522301654, -0.3162353388693405765, 0.4822834645669290543 ) ) ;
#41602=CARTESIAN_POINT ( 'NONE',  ( -0.3674540682414692561, -0.6046776061558809534, -0.2411417322834644161 ) ) ;
#41603=CARTESIAN_POINT ( 'NONE',  ( -0.4724409448818890911, -0.1870078740157479769, 0.4822834645669291653 ) ) ;
#41605=CARTESIAN_POINT ( 'NONE',  ( -1.482939632545930975, 0.05413385826771666132, 0.4176697321401328100 ) ) ;
#41606=CARTESIAN_POINT ( 'NONE',  ( -1.456692913385826182, -0.6692913385826771977, 8.415575281601705876E-17 ) ) ;
#41607=CARTESIAN_POINT ( 'NONE',  ( 0.9580052493438327987, -0.3690944881889765550, -0.3153832671262227771 ) ) ;
#41610=CARTESIAN_POINT ( 'NONE',  ( 0.4265091863517067039, -0.5511811023622048555, -0.09757992244046775898 ) ) ;
#41611=CARTESIAN_POINT ( 'NONE',  ( 0.05905511811023709395, -0.5400638737290844871, 0.3530559997133364547 ) ) ;
#41612=CARTESIAN_POINT ( 'NONE',  ( 0.2230971128608932319, -0.4281496062992124485, 0.4176697321401328655 ) ) ;
#41615=CARTESIAN_POINT ( 'NONE',  ( -1.586052503253848167, 1.023622047244095556, 0.1653254495020564929 ) ) ;
#41619=CARTESIAN_POINT ( 'NONE',  ( -0.5708661417322828946, 0.07958543189024071263, -0.2665933059059888421 ) ) ;
#41620=CARTESIAN_POINT ( 'NONE',  ( -0.8792650918635160906, 0.05413385826771626580, -0.4176697321401330321 ) ) ;
#41623=CARTESIAN_POINT ( 'NONE',  ( 1.627296587926509996, -0.6046776061558807314, 0.2411417322834647770 ) ) ;
#41624=CARTESIAN_POINT ( 'NONE',  ( 1.023622047244095112, -0.1870078740157480879, -0.4822834645669291653 ) ) ;
#41625=CARTESIAN_POINT ( 'NONE',  ( 0.3280839895013130669, -0.4281496062992127816, -0.4176697321401328100 ) ) ;
#41626=CARTESIAN_POINT ( 'NONE',  ( -0.5249343832020990641, 0.1283753931104748280, 0.1820866141732283561 ) ) ;
#41627=CARTESIAN_POINT ( 'NONE',  ( 0.1706036745406830368, 0.05413385826771666132, 0.4176697321401328100 ) ) ;
#41629=CARTESIAN_POINT ( 'NONE',  ( -0.2034120734908128059, 0.1771653543307087630, 0.09757992244046791164 ) ) ;
#41630=CARTESIAN_POINT ( 'NONE',  ( -0.6036745406824141069, 0.2306618581243848609, 0.2411417322834645549 ) ) ;
#41632=CARTESIAN_POINT ( 'NONE',  ( -1.496062992125983815, -0.1870078740157480879, -0.4822834645669291653 ) ) ;
#41633=CARTESIAN_POINT ( 'NONE',  ( 0.2099737532808405305, 0.1283753931104746893, -0.1820866141732285504 ) ) ;
#41635=CARTESIAN_POINT ( 'NONE',  ( -0.9908136482939626788, -0.6692913385826773087, -0.1292274648535924053 ) ) ;
#41636=CARTESIAN_POINT ( 'NONE',  ( -0.6824146981627288167, 0.1283753931104748280, 0.1820866141732283561 ) ) ;
#41638=CARTESIAN_POINT ( 'NONE',  ( -1.023622047244094002, -0.1870078740157480879, -0.4822834645669291653 ) ) ;
#41639=CARTESIAN_POINT ( 'NONE',  ( 0.1640419947506569498, -0.3162353388693409650, -0.4822834645669289433 ) ) ;
#41644=CARTESIAN_POINT ( 'NONE',  ( 0.2296587926509192634, -0.2845877964562159024, 0.3641732283464567677 ) ) ;
#41645=CARTESIAN_POINT ( 'NONE',  ( 1.167979002624672580, 0.05413385826771626580, -0.4176697321401330321 ) ) ;
#41646=CARTESIAN_POINT ( 'NONE',  ( -1.391076115485563758, 0.1283753931104748280, 0.1820866141732283561 ) ) ;
#41647=CARTESIAN_POINT ( 'NONE',  ( 1.167979002624672580, -0.4281496062992124485, 0.4176697321401328655 ) ) ;
#41648=CARTESIAN_POINT ( 'NONE',  ( -1.660104986876639543, -0.08942795157528024563, -0.3641732283464568787 ) ) ;
#41649=CARTESIAN_POINT ( 'NONE',  ( -0.4855643044619415427, -0.4281496062992124485, 0.4176697321401328655 ) ) ;
#41650=CARTESIAN_POINT ( 'NONE',  ( 0.01312335958005323398, -0.3690944881889765550, -0.3153832671262227771 ) ) ;
#41651=CARTESIAN_POINT ( 'NONE',  ( 1.306827173596999403, 0.000000000000000000, -0.4445507791589060620 ) ) ;
#41652=CARTESIAN_POINT ( 'NONE',  ( 0.5905511811023629321, -0.5511811023622047445, 6.969142054262312111E-17 ) ) ;
#41653=CARTESIAN_POINT ( 'NONE',  ( -0.07874015748031421014, -0.1870078740157479769, 0.4822834645669291653 ) ) ;
#41655=CARTESIAN_POINT ( 'NONE',  ( -1.272965879265091305, -0.4281496062992124485, 0.4176697321401328655 ) ) ;
#41657=CARTESIAN_POINT ( 'NONE',  ( 1.082677165354331228, -0.4536011799217367080, 0.2665933059059888421 ) ) ;
#41658=CARTESIAN_POINT ( 'NONE',  ( 0.2165354330708668673, -0.5400638737290844871, 0.3530559997133364547 ) ) ;
#41659=CARTESIAN_POINT ( 'NONE',  ( -0.3346456692913377662, 0.1660481256975883668, -0.3530559997133364547 ) ) ;
#41660=CARTESIAN_POINT ( 'NONE',  ( -0.2165354330708654795, 0.07958543189024085140, 0.2665933059059887866 ) ) ;
#41662=CARTESIAN_POINT ( 'NONE',  ( -0.4068241469816264999, -0.3690944881889763329, 0.3153832671262228327 ) ) ;
#41663=CARTESIAN_POINT ( 'NONE',  ( 0.3346456692913393205, -0.5400638737290845981, -0.3530559997133363437 ) ) ;
#41664=CARTESIAN_POINT ( 'NONE',  ( -1.220472440944881054, 0.1771653543307087630, 0.000000000000000000 ) ) ;
#41666=CARTESIAN_POINT ( 'NONE',  ( -0.9842519685039360366, 0.2952755905511811885, 0.000000000000000000 ) ) ;
#41667=CARTESIAN_POINT ( 'NONE',  ( 0.4606732211678803424, 1.778019097314518016, -0.5309055118110237448 ) ) ;
#41669=CARTESIAN_POINT ( 'NONE',  ( -1.706036745406823485, 0.1283753931104748280, 0.1820866141732283561 ) ) ;
#41670=CARTESIAN_POINT ( 'NONE',  ( -0.5511811023622041894, -0.1870078740157480879, -0.4822834645669291653 ) ) ;
#41672=CARTESIAN_POINT ( 'NONE',  ( -1.233595800524933894, -0.6046776061558809534, -0.2411417322834644161 ) ) ;
#41674=CARTESIAN_POINT ( 'NONE',  ( 1.377952755905512472, 0.2952755905511811885, 0.000000000000000000 ) ) ;
#41675=CARTESIAN_POINT ( 'NONE',  ( 0.7283464566929143125, 0.1660481256975885056, 0.3530559997133364547 ) ) ;
#41677=CARTESIAN_POINT ( 'NONE',  ( 1.548556430446194954, -0.5023911411419708095, 0.1820866141732285504 ) ) ;
#41679=ORIENTED_EDGE ( 'NONE', *, *, #35281, .F. ) ;
#41680=CARTESIAN_POINT ( 'NONE',  ( -0.4199475065616791736, -0.5023911411419708095, 0.1820866141732285504 ) ) ;
#41683=CARTESIAN_POINT ( 'NONE',  ( 0.7283464566929140904, -0.5400638737290845981, -0.3530559997133363437 ) ) ;
#41684=CARTESIAN_POINT ( 'NONE',  ( -0.1968503937007867743, -0.6692913385826771977, 8.415575281601705876E-17 ) ) ;
#41685=CARTESIAN_POINT ( 'NONE',  ( -0.9251968503937002541, -0.5400638737290845981, -0.3530559997133363437 ) ) ;
#41686=CARTESIAN_POINT ( 'NONE',  ( 1.312335958005250269, -0.6046776061558807314, 0.2411417322834647770 ) ) ;
#41687=CARTESIAN_POINT ( 'NONE',  ( -1.325459317585300889, -0.004921259842519576551, 0.3153832671262227771 ) ) ;
#41689=CARTESIAN_POINT ( 'NONE',  ( 0.3215223097112867578, -0.3162353388693409650, -0.4822834645669289433 ) ) ;
#41690=CARTESIAN_POINT ( 'NONE',  ( -0.8989501312335946848, -0.6692913385826771977, 0.1292274648535927661 ) ) ;
#41692=CARTESIAN_POINT ( 'NONE',  ( -1.279527559055116948, 0.1660481256975883668, -0.3530559997133364547 ) ) ;
#41693=DIRECTION ( 'NONE',  ( -1.000000000000000000, 0.000000000000000000, 1.692413147294446216E-16 ) ) ;
#41694=CARTESIAN_POINT ( 'NONE',  ( 0.8136482939632553313, -0.6046776061558809534, -0.2411417322834644161 ) ) ;
#41695=CARTESIAN_POINT ( 'NONE',  ( 1.482939632545932307, -0.3690944881889763329, 0.3153832671262228327 ) ) ;
#41698=CARTESIAN_POINT ( 'NONE',  ( -0.2887139107611542133, -0.6046776061558809534, -0.2411417322834644161 ) ) ;
#41700=CARTESIAN_POINT ( 'NONE',  ( 0.3608923884514443348, 0.1771653543307087075, -0.09757992244046823083 ) ) ;
#41701=CARTESIAN_POINT ( 'NONE',  ( -1.207349081364828880, 0.2306618581243847221, -0.2411417322834647770 ) ) ;
#41702=CARTESIAN_POINT ( 'NONE',  ( 1.010498687664042716, 0.05413385826771626580, -0.4176697321401330321 ) ) ;
#41703=CARTESIAN_POINT ( 'NONE',  ( 1.003937007874016185, 0.1660481256975883668, -0.3530559997133364547 ) ) ;
#41704=CARTESIAN_POINT ( 'NONE',  ( -0.3215223097112853146, -0.3162353388693405765, 0.4822834645669290543 ) ) ;
#41707=CARTESIAN_POINT ( 'NONE',  ( -0.7414698162729651543, -0.6692913385826771977, 0.1292274648535927661 ) ) ;
#41709=CARTESIAN_POINT ( 'NONE',  ( -1.417322834645668772, -0.1870078740157479769, 0.4822834645669291653 ) ) ;
#41710=CARTESIAN_POINT ( 'NONE',  ( -0.5052493438320203589, 0.2952755905511810774, -0.1292274648535930714 ) ) ;
#41711=CARTESIAN_POINT ( 'NONE',  ( 1.240157480314961314, 0.1660481256975883668, -0.3530559997133364547 ) ) ;
#41712=CARTESIAN_POINT ( 'NONE',  ( 1.417322834645670104, -0.1870078740157480879, -0.4822834645669291653 ) ) ;
#41713=CARTESIAN_POINT ( 'NONE',  ( -0.9645669291338575535, -0.5400638737290844871, 0.3530559997133364547 ) ) ;
#41715=CARTESIAN_POINT ( 'NONE',  ( 0.8661417322834652488, -0.1870078740157480879, -0.4822834645669291653 ) ) ;
#41717=CARTESIAN_POINT ( 'NONE',  ( -0.6627296587926501115, 0.2952755905511810774, -0.1292274648535930714 ) ) ;
#41718=CARTESIAN_POINT ( 'NONE',  ( -1.089238845144356427, -0.3690944881889765550, -0.3153832671262227771 ) ) ;
#41719=CARTESIAN_POINT ( 'NONE',  ( 0.8070866141732289112, -0.4536011799217368745, -0.2665933059059886201 ) ) ;
#41721=CARTESIAN_POINT ( 'NONE',  ( 1.062992125984252745, 0.1771653543307087630, 0.000000000000000000 ) ) ;
#41722=CARTESIAN_POINT ( 'NONE',  ( 0.9514435695538062676, -0.05778040916215522460, 0.4822834645669289988 ) ) ;
#41724=CARTESIAN_POINT ( 'NONE',  ( -0.4330708661417315697, 0.2952755905511811885, 0.000000000000000000 ) ) ;
#41726=CARTESIAN_POINT ( 'NONE',  ( 1.541994750656168645, -0.5511811023622046335, 0.09757992244046803654 ) ) ;
#41727=CARTESIAN_POINT ( 'NONE',  ( -0.4002624671916004129, -0.05778040916215560624, -0.4822834645669293319 ) ) ;
#41729=CARTESIAN_POINT ( 'NONE',  ( 1.404199475065617708, 0.05413385826771626580, -0.4176697321401330321 ) ) ;
#41730=CARTESIAN_POINT ( 'NONE',  ( -0.05249343832020938322, -0.6046776061558809534, -0.2411417322834644161 ) ) ;
#41731=CARTESIAN_POINT ( 'NONE',  ( 0.3871391076115493490, -0.2845877964562159024, 0.3641732283464567677 ) ) ;
#41733=CARTESIAN_POINT ( 'NONE',  ( -0.006561679790025524116, -0.08942795157528024563, -0.3641732283464568787 ) ) ;
#41734=CARTESIAN_POINT ( 'NONE',  ( 1.220472440944882164, 0.000000000000000000, 0.3464511005275205946 ) ) ;
#41736=CARTESIAN_POINT ( 'NONE',  ( 0.5577427821522316087, -0.05778040916215522460, 0.4822834645669289988 ) ) ;
#41738=CARTESIAN_POINT ( 'NONE',  ( 1.509186351706037543, -0.004921259842519576551, 0.3153832671262227771 ) ) ;
#41739=CARTESIAN_POINT ( 'NONE',  ( 0.09186351706036827158, 0.05413385826771666132, 0.4176697321401328100 ) ) ;
#41740=CARTESIAN_POINT ( 'NONE',  ( -0.06561679790026180015, -0.3690944881889765550, -0.3153832671262227771 ) ) ;
#41741=CARTESIAN_POINT ( 'NONE',  ( 0.2099737532808405305, -0.6046776061558807314, 0.2411417322834647770 ) ) ;
#41742=CARTESIAN_POINT ( 'NONE',  ( 1.587926509186352586, -0.3690944881889765550, -0.3153832671262227771 ) ) ;
#41743=CARTESIAN_POINT ( 'NONE',  ( -1.561679790026246017, -0.004921259842519576551, 0.3153832671262227771 ) ) ;
#41744=CARTESIAN_POINT ( 'NONE',  ( -1.410761154855642463, -0.05778040916215522460, 0.4822834645669289988 ) ) ;
#41745=CARTESIAN_POINT ( 'NONE',  ( 0.5839895013123367340, 0.2952755905511811885, 0.1292274648535926551 ) ) ;
#41746=CARTESIAN_POINT ( 'NONE',  ( 1.325459317585302665, -0.4281496062992124485, 0.4176697321401328655 ) ) ;
#41748=CARTESIAN_POINT ( 'NONE',  ( -0.01968503937007793844, -0.5400638737290844871, 0.3530559997133364547 ) ) ;
#41749=CARTESIAN_POINT ( 'NONE',  ( 1.213910761154856299, 0.2952755905511811885, 0.1292274648535926551 ) ) ;
#41750=CARTESIAN_POINT ( 'NONE',  ( 0.9973753280839902091, -0.6046776061558807314, 0.2411417322834647770 ) ) ;
#41752=CARTESIAN_POINT ( 'NONE',  ( 0.9842519685039378130, -0.5511811023622047445, 6.969142054262312111E-17 ) ) ;
#41753=CARTESIAN_POINT ( 'NONE',  ( 1.601049868766404982, -0.6046776061558809534, -0.2411417322834644161 ) ) ;
#41754=CARTESIAN_POINT ( 'NONE',  ( -0.6627296587926501115, 0.1771653543307087075, -0.09757992244046823083 ) ) ;
#41755=CARTESIAN_POINT ( 'NONE',  ( 0.4593175853018379162, -0.3690944881889763329, 0.3153832671262228327 ) ) ;
#41756=CARTESIAN_POINT ( 'NONE',  ( 0.07217847769028949700, -0.3162353388693405765, 0.4822834645669290543 ) ) ;
#41757=CARTESIAN_POINT ( 'NONE',  ( 0.5905511811023629321, -0.6692913385826771977, 8.415575281601705876E-17 ) ) ;
#41758=CARTESIAN_POINT ( 'NONE',  ( -0.5183727034120726440, 0.2952755905511811885, 0.1292274648535926551 ) ) ;
#41760=CARTESIAN_POINT ( 'NONE',  ( 0.06561679790026316017, -0.004921259842519870586, -0.3153832671262229437 ) ) ;
#41762=CARTESIAN_POINT ( 'NONE',  ( 0.7939632545931766261, -0.05778040916215522460, 0.4822834645669289988 ) ) ;
#41764=CARTESIAN_POINT ( 'NONE',  ( -0.9776902887139098386, -0.6692913385826771977, 0.1292274648535927661 ) ) ;
#41768=CARTESIAN_POINT ( 'NONE',  ( -0.6692913385826764205, 0.2952755905511811885, 0.000000000000000000 ) ) ;
#41769=CARTESIAN_POINT ( 'NONE',  ( -0.6036745406824141069, 0.2306618581243848609, 0.2411417322834645549 ) ) ;
#41772=VERTEX_POINT ( 'NONE', #41273 ) ;
#41773=CARTESIAN_POINT ( 'NONE',  ( 0.7874015748031503170, -0.1870078740157480601, -0.3641732283464567677 ) ) ;
#41775=CARTESIAN_POINT ( 'NONE',  ( 1.174540682414699111, -0.05778040916215560624, -0.4822834645669293319 ) ) ;
#41776=CARTESIAN_POINT ( 'NONE',  ( -0.1698998578625667832, -2.609869883881465018E-15, -0.3464511005275220379 ) ) ;
#41777=CARTESIAN_POINT ( 'NONE',  ( -1.279527559055116948, -0.4536011799217367080, 0.2665933059059888421 ) ) ;
#41778=AXIS2_PLACEMENT_3D ( 'NONE', #71592, #46740, #33300 ) ;
#41779=CARTESIAN_POINT ( 'NONE',  ( 1.397637795275591177, 0.1660481256975883668, -0.3530559997133364547 ) ) ;
#41780=CARTESIAN_POINT ( 'NONE',  ( -1.509186351706035767, 0.05413385826771626580, -0.4176697321401330321 ) ) ;
#41781=CARTESIAN_POINT ( 'NONE',  ( 0.4855643044619430415, -0.4281496062992127816, -0.4176697321401328100 ) ) ;
#41783=CARTESIAN_POINT ( 'NONE',  ( 0.006561679790026889343, -0.3162353388693409650, -0.4822834645669289433 ) ) ;
#41784=CARTESIAN_POINT ( 'NONE',  ( -0.9055118110236215490, 0.1771653543307087630, 0.000000000000000000 ) ) ;
#41785=EDGE_CURVE ( 'NONE', #30946, #21487, #7679, .T. ) ;
#41786=CARTESIAN_POINT ( 'NONE',  ( 1.023622047244095112, -0.1870078740157480879, -0.4822834645669291653 ) ) ;
#41787=CARTESIAN_POINT ( 'NONE',  ( -0.1115485564304456306, 0.2952755905511810774, -0.1292274648535930714 ) ) ;
#41788=( BOUNDED_SURFACE ( )  B_SPLINE_SURFACE ( 1, 2, ( 
 ( #36533, #54344, #18022, #48032, #11291, #36950, #56302, #57532, #82808, #310, #70168, #37770, #51211, #50392, #82405, #25964, #12521, #52047, #37368, #63857, #56706, #63039, #6194, #51622, #63445, #76089, #38599, #39010, #77327, #76907, #25544, #5377, #83223, #44477, #25132, #38182, #19656, #31872, #19237, #44888, #69358, #64694, #24724, #11712, #70587, #50802, #7033, #18433, #31038, #57943, #32283, #44075, #76503, #45318, #12941, #26389, #71013, #69768, #58369, #12112, #731, #32703, #64277, #5781, #31451, #77752, #57114, #43656, #18832, #6612, #13357, #33128, #45735, #65957, #33546, #7458, #15029, #34379, #71854, #66371, #34801, #1569, #8293, #27641, #53715, #60461, #8708, #15448, #41107, #59208, #39860, #33961, #59623, #13778, #2811, #28058, #66795, #46158, #78596, #40274, #14204, #9130, #28470, #72681, #21742, #65551, #47407, #1978, #21335, #58798, #7882, #53303, #46987, #1156, #54131, #26807, #65123, #79016, #40685, #46575, #71431, #20504, #52465, #27223, #60044, #52884, #2400, #20920, #39435, #79422, #73096, #20085, #78173, #72272, #14620, #36033, #43151, #68848, #36855, #9948, #67205, #4047, #60870, #62115, #35621, #54966, #22579, #11196, #42333, #62529, #9538, #36442, #55787, #81493, #4867, #68442, #75175, #48240, #80263, #61284, #30540, #4458, #47822, #17519, #67618, #30123, #3223, #29712, #55375, #23809, #35208, #79846, #49482, #81081, #74349, #22163, #3636, #28888, #73936, #54548, #73523, #23398, #15872, #49065, #42747, #41520, #16279, #29304, #41925, #74763, #80673, #22986, #17112, #48652, #16693, #68031, #10376, #61707, #10782, #11612, #43977, #63758, #69265, #6931, #70916, #57434, #51112, #76809, #82714, #82311, #38915, #18337, #49888, #64595, #44379, #83127, #69674, #45215, #24631, #50297, #70071, #56204, #13265, #37272, #38502, #18737, #19140, #25447, #62947, #75995, #12017, #44790, #37672, #70486, #6099, #12426, #56611, #38084, #81905, #63349, #32188, #5684, #24217, #77227, #17928, #31773, #211, #5282, #75589, #31353, #25034, #30944, #12843, #64184, #6518, #57844, #57019, #50707, #76406, #25864, #51524, #19556, #43564, #27119, #58265, #27953, #71329, #629, #14519, #71746, #53612, #13677, #26285, #46883, #21228, #51946, #39751, #72577, #59107, #15343, #34276, #33018, #47300, #77651, #72990, #79320, #72164, #39329, #78069, #14924, #40584, #21640, #19984, #20400, #7779, #45634, #65015, #78492, #46052, #7350, #27537, #66266, #1053, #78907, #41005, #14099, #20815, #40172, #8605, #66688, #59937, #32602, #58688, #65447, #52363, #46470, #65856, #26707, #33447, #2293, #1463, #52783, #8189, #33856, #59520, #1877, #53194, #61607, #10686, #3119, #36341, #22885, #10270, #47718, #28785, #48549, #35938, #73416, #81391, #15765, #54028, #16590, #42235, #35519, #60359, #9432, #22056, #54447, #74247, #35101, #74665, #80159, #2706, #67929, #3950, #60768, #55271, #29611, #67101, #80982, #48137, #48965, #61182, #22476, #23295, #41417, #73834, #17009, #3536, #17421, #28366, #29203, #16174, #79740, #54869, #42649, #41820, #67511, #68346, #4352, #62015, #30020, #55684, #9848, #23707, #80575, #49378, #75074, #43052, #9023, #34696, #37166, #31672, #111, #50198, #56923, #76310, #19044, #25766, #57333, #64082, #6419, #82213, #5182, #31255, #82617, #62424, #51427, #76711, #32088, #11510, #43875, #5588, #62846, #57749, #77130, #37987, #70388, #30846, #12743, #24933, #69975, #24118, #56511, #50603, #12329, #49787, #19463, #75488, #30437, #18641, #44285, #11921, #36748, #69159, #81806, #24532, #63663, #75895, #51012, #18235, #4761, #6003, #83027, #69573, #25350, #44691, #43462, #38402, #37576, #68748, #63249, #11091, #56102, #17828, #536, #1783, #14004, #53526, #38818, #65351, #58167, #64496, #7689, #27443, #64919, #51850, #40082, #40497, #53104, #78395, #27026, #6834, #1374, #45955, #963, #39661, #78813, #33356, #52687, #59019, #70820, #66177, #26189, #13168, #20727, #26617, #8515, #77557, #32504, #59428, #33766, #19890, #52270, #21142, #71652, #27866, #46797, #45538, #59846, #71236, #2198, #34182, #46378, #13580, #7257, #72488, #14837, #79234, #39234, #32929 ),
 ( #14430, #8101, #45113, #58594, #77975, #20305, #72071, #65769, #8927, #42142, #80885, #41726, #55584, #47627, #67010, #22791, #60269, #9343, #29104, #34604, #21549, #36247, #48451, #16498, #67837, #48044, #73322, #4258, #35014, #15251, #29921, #9753, #74151, #60678, #10590, #15668, #41330, #35425, #47210, #61916, #2619, #3855, #67420, #10176, #35841, #28275, #3027, #28693, #61509, #54355, #29515, #54775, #61090, #21966, #3441, #72900, #80066, #23198, #22384, #40911, #42552, #66592, #80478, #48869, #53937, #79649, #73745, #16081, #55176, #74569, #16914, #68255, #63154, #81712, #82116, #50916, #11828, #69060, #42956, #75383, #68650, #44594, #70289, #38302, #11410, #10988, #5494, #62324, #63566, #37065, #56417, #24022, #12641, #43772, #63977, #36649, #37890, #57229, #82930, #6313, #69880, #76616, #49690, #17731, #62750, #31990, #5900, #49279, #18946, #5086, #31573, #4662, #31156, #56822, #25252, #30335, #81296, #43359, #30754, #23610, #74982, #17327, #56001, #24431, #50099, #75795, #82520, #24837, #18138, #69475, #37481, #50505, #76209, #18546, #44190, #12233, #45013, #58065, #6732, #59328, #33256, #39985, #26926, #20626, #78714, #70712, #64813, #65675, #1277, #77031, #13064, #78294, #33666, #77872, #8412, #432, #19784, #58918, #38718, #45437, #65247, #64396, #57651, #72391, #52585, #46277, #71973, #857, #26087, #40394, #71132, #51327, #66076, #45852, #14327, #13475, #46698, #51747, #77450, #71551, #13, #14741, #32402, #8002, #20202, #1684, #27343, #39132, #7154, #32825, #53001, #58493, #21039, #7584, #13900, #26514, #39558, #25666, #52168, #19363, #34501, #74467, #55076, #79135, #9657, #61404, #66489, #42450, #53834, #2931, #8824, #73644, #15986, #80380, #41633, #60166, #34918, #3753, #47941, #21861, #21452, #28177, #47109, #80784, #23100, #16814, #47526, #72799, #67323, #15148, #16397, #73217, #9246, #2519, #48768, #79968, #68150, #40805, #74049, #10072, #35736, #34080, #22693, #29417, #79548, #35327, #15567, #42043, #41227, #60580, #66914, #59743, #22281, #2097, #28595, #67739, #27762, #53427, #54252, #48352, #60990, #3339, #29003, #54669, #25156, #50414, #61820, #31476, #81616, #44098, #17231, #18045, #43678, #69791, #81198, #5805, #76114, #11735, #4993, #63471, #23930, #23513, #10895, #42861, #12137, #69381, #18455, #63062, #56730, #57137, #49182, #17634, #37793, #37390, #29825, #74885, #31062, #82834, #30661, #44501, #36555, #55904, #5399, #68554, #49597, #82427, #62231, #10494, #50824, #24747, #76526, #18854, #36972, #4570, #36148, #75291, #4160, #55487, #82023, #30241, #43266, #68963, #11313, #62652, #24336, #56324, #50006, #75703, #53626, #33870, #34290, #14939, #76932, #12964, #32305, #59952, #38621, #40598, #21243, #27551, #70609, #53210, #70191, #25987, #47314, #64299, #28379, #9036, #31893, #46898, #15356, #19259, #79753, #6633, #39033, #44912, #78921, #72592, #2307, #66280, #57966, #71036, #41017, #1891, #333, #57554, #51646, #83245, #34710, #60371, #54040, #77350, #25568, #6217, #8620, #13380, #19682, #65870, #27968, #8205, #79334, #59534, #12545, #66703, #51233, #38204, #21654, #45340, #2719, #73004, #63878, #22070, #36353, #41430, #54882, #62029, #74260, #30450, #49392, #48152, #62437, #67113, #4774, #11105, #3961, #54460, #9861, #30033, #55696, #36761, #9444, #35531, #22894, #60781, #73428, #10283, #61193, #35115, #42661, #4365, #16187, #10698, #56114, #29215, #35949, #55284, #81404, #81820, #23721, #43064, #68761, #3549, #67524, #61619, #29624, #3133, #47730, #75086, #15778, #73847, #48562, #67941, #41834, #28797, #80174, #17022, #17433, #80587, #22488, #80994, #48977, #16601, #42246, #23307, #74676, #68359, #13183, #62858, #69171, #31686, #57345, #50617, #75501, #24546, #37179, #43889, #63674, #50210, #6433, #18247, #17840, #83041, #25364, #75908, #70402, #44706, #82226, #37998, #63260, #64097, #76322, #69586, #51027, #30859, #5194, #32104, #18652, #32519, #43475, #44296, #56524, #11522, #69987, #57763, #11932, #37587, #19058, #19477, #125, #76726, #6015, #5601, #31268, #56934, #70835, #38833, #64512, #82630, #24944, #12758, #12342 ) ),
 .UNSPECIFIED., .F., .F., .F. ) 
 B_SPLINE_SURFACE_WITH_KNOTS ( ( 2, 2 ),
 ( 3, 2, 2, 2, 2, 2, 2, 2, 2, 2, 2, 2, 2, 2, 2, 2, 2, 2, 2, 2, 2, 2, 2, 2, 2, 2, 2, 2, 2, 2, 2, 2, 2, 2, 2, 2, 2, 2, 2, 2, 2, 2, 2, 2, 2, 2, 2, 2, 2, 2, 2, 2, 2, 2, 2, 2, 2, 2, 2, 2, 2, 2, 2, 2, 2, 2, 2, 2, 2, 2, 2, 2, 2, 2, 2, 2, 2, 2, 2, 2, 2, 2, 2, 2, 2, 2, 2, 2, 2, 2, 2, 2, 2, 2, 2, 2, 2, 2, 2, 2, 2, 2, 2, 2, 2, 2, 2, 2, 2, 2, 2, 2, 2, 2, 2, 2, 2, 2, 2, 2, 2, 2, 2, 2, 2, 2, 2, 2, 2, 2, 2, 2, 2, 2, 2, 2, 2, 2, 2, 2, 2, 2, 2, 2, 2, 2, 2, 2, 2, 2, 2, 2, 2, 2, 2, 2, 2, 2, 2, 2, 2, 2, 2, 2, 2, 2, 2, 2, 2, 2, 2, 2, 2, 2, 2, 2, 2, 2, 2, 2, 2, 2, 2, 2, 2, 2, 2, 2, 2, 2, 2, 2, 2, 2, 2, 2, 2, 2, 2, 2, 2, 2, 2, 2, 2, 2, 2, 2, 2, 2, 2, 2, 2, 2, 2, 2, 2, 2, 2, 2, 2, 2, 2, 2, 2, 2, 2, 2, 2, 2, 2, 2, 2, 2, 2, 2, 2, 2, 2, 2, 2, 2, 2, 2, 2, 2, 2, 2, 2, 2, 2, 2, 2, 2, 2, 3 ),
 ( 0.000000000000000000, 1.000000000000000000 ),
 ( 0.000000000000000000, 0.003787878787878787984, 0.007575757575757575968, 0.01136363636363636395, 0.01515151515151515194, 0.01893939393939393992, 0.02272727272727272790, 0.02651515151515151589, 0.03030303030303030387, 0.03409090909090908839, 0.03787878787878787984, 0.04166666666666666435, 0.04545454545454545581, 0.04924242424242424032, 0.05303030303030303177, 0.05681818181818181629, 0.06060606060606060774, 0.06439393939393939226, 0.06818181818181817677, 0.07196969696969697516, 0.07575757575757575968, 0.07954545454545454419, 0.08333333333333332871, 0.08712121212121212710, 0.09090909090909091161, 0.09469696969696969613, 0.09848484848484848064, 0.1022727272727272790, 0.1060606060606060635, 0.1098484848484848481, 0.1136363636363636326, 0.1174242424242424310, 0.1212121212121212155, 0.1250000000000000000, 0.1287878787878787845, 0.1325757575757575690, 0.1363636363636363535, 0.1401515151515151381, 0.1439393939393939503, 0.1477272727272727348, 0.1515151515151515194, 0.1553030303030303039, 0.1590909090909090884, 0.1628787878787878729, 0.1666666666666666574, 0.1704545454545454419, 0.1742424242424242542, 0.1780303030303030387, 0.1818181818181818232, 0.1856060606060606077, 0.1893939393939393923, 0.1931818181818181768, 0.1969696969696969613, 0.2007575757575757458, 0.2045454545454545581, 0.2083333333333333426, 0.2121212121212121271, 0.2159090909090909116, 0.2196969696969696961, 0.2234848484848484806, 0.2272727272727272652, 0.2310606060606060497, 0.2348484848484848619, 0.2386363636363636465, 0.2424242424242424310, 0.2462121212121212155, 0.2500000000000000000, 0.2537878787878787845, 0.2575757575757575690, 0.2613636363636363535, 0.2651515151515151381, 0.2689393939393939226, 0.2727272727272727071, 0.2765151515151514916, 0.2803030303030302761, 0.2840909090909091161, 0.2878787878787879007, 0.2916666666666666852, 0.2954545454545454697, 0.2992424242424242542, 0.3030303030303030387, 0.3068181818181818232, 0.3106060606060606077, 0.3143939393939393923, 0.3181818181818181768, 0.3219696969696969613, 0.3257575757575757458, 0.3295454545454545303, 0.3333333333333333148, 0.3371212121212120993, 0.3409090909090908839, 0.3446969696969697239, 0.3484848484848485084, 0.3522727272727272929, 0.3560606060606060774, 0.3598484848484848619, 0.3636363636363636465, 0.3674242424242424310, 0.3712121212121212155, 0.3750000000000000000, 0.3787878787878787845, 0.3825757575757575690, 0.3863636363636363535, 0.3901515151515151381, 0.3939393939393939226, 0.3977272727272727071, 0.4015151515151514916, 0.4053030303030302761, 0.4090909090909091161, 0.4128787878787879007, 0.4166666666666666852, 0.4204545454545454697, 0.4242424242424242542, 0.4280303030303030387, 0.4318181818181818232, 0.4356060606060606077, 0.4393939393939393923, 0.4431818181818181768, 0.4469696969696969613, 0.4507575757575757458, 0.4545454545454545303, 0.4583333333333333148, 0.4621212121212120993, 0.4659090909090908839, 0.4696969696969697239, 0.4734848484848485084, 0.4772727272727272929, 0.4810606060606060774, 0.4848484848484848619, 0.4886363636363636465, 0.4924242424242424310, 0.4962121212121212155, 0.5000000000000000000, 0.5037878787878787845, 0.5075757575757575690, 0.5113636363636363535, 0.5151515151515151381, 0.5189393939393939226, 0.5227272727272727071, 0.5265151515151514916, 0.5303030303030302761, 0.5340909090909090606, 0.5378787878787878451, 0.5416666666666666297, 0.5454545454545454142, 0.5492424242424241987, 0.5530303030303029832, 0.5568181818181817677, 0.5606060606060605522, 0.5643939393939394478, 0.5681818181818182323, 0.5719696969696970168, 0.5757575757575758013, 0.5795454545454545858, 0.5833333333333333703, 0.5871212121212121549, 0.5909090909090909394, 0.5946969696969697239, 0.5984848484848485084, 0.6022727272727272929, 0.6060606060606060774, 0.6098484848484848619, 0.6136363636363636465, 0.6174242424242424310, 0.6212121212121212155, 0.6250000000000000000, 0.6287878787878787845, 0.6325757575757575690, 0.6363636363636363535, 0.6401515151515151381, 0.6439393939393939226, 0.6477272727272727071, 0.6515151515151514916, 0.6553030303030302761, 0.6590909090909090606, 0.6628787878787878451, 0.6666666666666666297, 0.6704545454545454142, 0.6742424242424241987, 0.6780303030303029832, 0.6818181818181817677, 0.6856060606060605522, 0.6893939393939394478, 0.6931818181818182323, 0.6969696969696970168, 0.7007575757575758013, 0.7045454545454545858, 0.7083333333333333703, 0.7121212121212121549, 0.7159090909090909394, 0.7196969696969697239, 0.7234848484848485084, 0.7272727272727272929, 0.7310606060606060774, 0.7348484848484848619, 0.7386363636363636465, 0.7424242424242424310, 0.7462121212121212155, 0.7500000000000000000, 0.7537878787878787845, 0.7575757575757575690, 0.7613636363636363535, 0.7651515151515151381, 0.7689393939393939226, 0.7727272727272727071, 0.7765151515151514916, 0.7803030303030302761, 0.7840909090909090606, 0.7878787878787878451, 0.7916666666666666297, 0.7954545454545454142, 0.7992424242424241987, 0.8030303030303029832, 0.8068181818181817677, 0.8106060606060605522, 0.8143939393939394478, 0.8181818181818182323, 0.8219696969696970168, 0.8257575757575758013, 0.8295454545454545858, 0.8333333333333333703, 0.8371212121212121549, 0.8409090909090909394, 0.8446969696969697239, 0.8484848484848485084, 0.8522727272727272929, 0.8560606060606060774, 0.8598484848484848619, 0.8636363636363636465, 0.8674242424242424310, 0.8712121212121212155, 0.8750000000000000000, 0.8787878787878787845, 0.8825757575757575690, 0.8863636363636363535, 0.8901515151515151381, 0.8939393939393939226, 0.8977272727272727071, 0.9015151515151514916, 0.9053030303030302761, 0.9090909090909090606, 0.9128787878787878451, 0.9166666666666666297, 0.9204545454545454142, 0.9242424242424241987, 0.9280303030303029832, 0.9318181818181817677, 0.9356060606060605522, 0.9393939393939394478, 0.9431818181818182323, 0.9469696969696970168, 0.9507575757575758013, 0.9545454545454545858, 0.9583333333333333703, 0.9621212121212121549, 0.9659090909090909394 ),
 .UNSPECIFIED. ) 
 GEOMETRIC_REPRESENTATION_ITEM ( )  RATIONAL_B_SPLINE_SURFACE ( (
 ( 1.000000000000000000, 0.9659258262890683122, 1.000000000000000000, 0.9659258262890683122, 1.000000000000000000, 0.9659258262890683122, 1.000000000000000000, 0.9659258262890683122, 1.000000000000000000, 0.9659258262890683122, 1.000000000000000000, 0.9659258262890683122, 1.000000000000000000, 0.9659258262890683122, 1.000000000000000000, 0.9659258262890683122, 1.000000000000000000, 0.9659258262890683122, 1.000000000000000000, 0.9659258262890683122, 1.000000000000000000, 0.9659258262890683122, 1.000000000000000000, 0.9659258262890683122, 1.000000000000000000, 0.9659258262890683122, 1.000000000000000000, 0.9659258262890683122, 1.000000000000000000, 0.9659258262890683122, 1.000000000000000000, 0.9659258262890683122, 1.000000000000000000, 0.9659258262890683122, 1.000000000000000000, 0.9659258262890683122, 1.000000000000000000, 0.9659258262890683122, 1.000000000000000000, 0.9659258262890683122, 1.000000000000000000, 0.9659258262890683122, 1.000000000000000000, 0.9659258262890683122, 1.000000000000000000, 0.9659258262890683122, 1.000000000000000000, 0.9659258262890683122, 1.000000000000000000, 0.9659258262890683122, 1.000000000000000000, 0.9659258262890683122, 1.000000000000000000, 0.9659258262890683122, 1.000000000000000000, 0.9659258262890683122, 1.000000000000000000, 0.9659258262890683122, 1.000000000000000000, 0.9659258262890683122, 1.000000000000000000, 0.9659258262890683122, 1.000000000000000000, 0.9659258262890683122, 1.000000000000000000, 0.9659258262890683122, 1.000000000000000000, 0.9659258262890683122, 1.000000000000000000, 0.9659258262890683122, 1.000000000000000000, 0.9659258262890683122, 1.000000000000000000, 0.9659258262890683122, 1.000000000000000000, 0.9659258262890683122, 1.000000000000000000, 0.9659258262890683122, 1.000000000000000000, 0.9659258262890683122, 1.000000000000000000, 0.9659258262890683122, 1.000000000000000000, 0.9659258262890683122, 1.000000000000000000, 0.9659258262890683122, 1.000000000000000000, 0.9659258262890683122, 1.000000000000000000, 0.9659258262890683122, 1.000000000000000000, 0.9659258262890683122, 1.000000000000000000, 0.9659258262890683122, 1.000000000000000000, 0.9659258262890683122, 1.000000000000000000, 0.9659258262890683122, 1.000000000000000000, 0.9659258262890683122, 1.000000000000000000, 0.9659258262890683122, 1.000000000000000000, 0.9659258262890683122, 1.000000000000000000, 0.9659258262890683122, 1.000000000000000000, 0.9659258262890683122, 1.000000000000000000, 0.9659258262890683122, 1.000000000000000000, 0.9659258262890683122, 1.000000000000000000, 0.9659258262890683122, 1.000000000000000000, 0.9659258262890683122, 1.000000000000000000, 0.9659258262890683122, 1.000000000000000000, 0.9659258262890683122, 1.000000000000000000, 0.9659258262890683122, 1.000000000000000000, 0.9659258262890683122, 1.000000000000000000, 0.9659258262890683122, 1.000000000000000000, 0.9659258262890683122, 1.000000000000000000, 0.9659258262890683122, 1.000000000000000000, 0.9659258262890683122, 1.000000000000000000, 0.9659258262890683122, 1.000000000000000000, 0.9659258262890683122, 1.000000000000000000, 0.9659258262890683122, 1.000000000000000000, 0.9659258262890683122, 1.000000000000000000, 0.9659258262890683122, 1.000000000000000000, 0.9659258262890683122, 1.000000000000000000, 0.9659258262890683122, 1.000000000000000000, 0.9659258262890683122, 1.000000000000000000, 0.9659258262890683122, 1.000000000000000000, 0.9659258262890683122, 1.000000000000000000, 0.9659258262890683122, 1.000000000000000000, 0.9659258262890683122, 1.000000000000000000, 0.9659258262890683122, 1.000000000000000000, 0.9659258262890683122, 1.000000000000000000, 0.9659258262890683122, 1.000000000000000000, 0.9659258262890683122, 1.000000000000000000, 0.9659258262890683122, 1.000000000000000000, 0.9659258262890683122, 1.000000000000000000, 0.9659258262890683122, 1.000000000000000000, 0.9659258262890683122, 1.000000000000000000, 0.9659258262890683122, 1.000000000000000000, 0.9659258262890683122, 1.000000000000000000, 0.9659258262890683122, 1.000000000000000000, 0.9659258262890683122, 1.000000000000000000, 0.9659258262890683122, 1.000000000000000000, 0.9659258262890683122, 1.000000000000000000, 0.9659258262890683122, 1.000000000000000000, 0.9659258262890683122, 1.000000000000000000, 0.9659258262890683122, 1.000000000000000000, 0.9659258262890683122, 1.000000000000000000, 0.9659258262890683122, 1.000000000000000000, 0.9659258262890683122, 1.000000000000000000, 0.9659258262890683122, 1.000000000000000000, 0.9659258262890683122, 1.000000000000000000, 0.9659258262890683122, 1.000000000000000000, 0.9659258262890683122, 1.000000000000000000, 0.9659258262890683122, 1.000000000000000000, 0.9659258262890683122, 1.000000000000000000, 0.9659258262890683122, 1.000000000000000000, 0.9659258262890683122, 1.000000000000000000, 0.9659258262890683122, 1.000000000000000000, 0.9659258262890683122, 1.000000000000000000, 0.9659258262890683122, 1.000000000000000000, 0.9659258262890683122, 1.000000000000000000, 0.9659258262890683122, 1.000000000000000000, 0.9659258262890683122, 1.000000000000000000, 0.9659258262890683122, 1.000000000000000000, 0.9659258262890683122, 1.000000000000000000, 0.9659258262890683122, 1.000000000000000000, 0.9659258262890683122, 1.000000000000000000, 0.9659258262890683122, 1.000000000000000000, 0.9659258262890683122, 1.000000000000000000, 0.9659258262890683122, 1.000000000000000000, 0.9659258262890683122, 1.000000000000000000, 0.9659258262890683122, 1.000000000000000000, 0.9659258262890683122, 1.000000000000000000, 0.9659258262890683122, 1.000000000000000000, 0.9659258262890683122, 1.000000000000000000, 0.9659258262890683122, 1.000000000000000000, 0.9659258262890683122, 1.000000000000000000, 0.9659258262890683122, 1.000000000000000000, 0.9659258262890683122, 1.000000000000000000, 0.9659258262890683122, 1.000000000000000000, 0.9659258262890683122, 1.000000000000000000, 0.9659258262890683122, 1.000000000000000000, 0.9659258262890683122, 1.000000000000000000, 0.9659258262890683122, 1.000000000000000000, 0.9659258262890683122, 1.000000000000000000, 0.9659258262890683122, 1.000000000000000000, 0.9659258262890683122, 1.000000000000000000, 0.9659258262890683122, 1.000000000000000000, 0.9659258262890683122, 1.000000000000000000, 0.9659258262890683122, 1.000000000000000000, 0.9659258262890683122, 1.000000000000000000, 0.9659258262890683122, 1.000000000000000000, 0.9659258262890683122, 1.000000000000000000, 0.9659258262890683122, 1.000000000000000000, 0.9659258262890683122, 1.000000000000000000, 0.9659258262890683122, 1.000000000000000000, 0.9659258262890683122, 1.000000000000000000, 0.9659258262890683122, 1.000000000000000000, 0.9659258262890683122, 1.000000000000000000, 0.9659258262890683122, 1.000000000000000000, 0.9659258262890683122, 1.000000000000000000, 0.9659258262890683122, 1.000000000000000000, 0.9659258262890683122, 1.000000000000000000, 0.9659258262890683122, 1.000000000000000000, 0.9659258262890683122, 1.000000000000000000, 0.9659258262890683122, 1.000000000000000000, 0.9659258262890683122, 1.000000000000000000, 0.9659258262890683122, 1.000000000000000000, 0.9659258262890683122, 1.000000000000000000, 0.9659258262890683122, 1.000000000000000000, 0.9659258262890683122, 1.000000000000000000, 0.9659258262890683122, 1.000000000000000000, 0.9659258262890683122, 1.000000000000000000, 0.9659258262890683122, 1.000000000000000000, 0.9659258262890683122, 1.000000000000000000, 0.9659258262890683122, 1.000000000000000000, 0.9659258262890683122, 1.000000000000000000, 0.9659258262890683122, 1.000000000000000000, 0.9659258262890683122, 1.000000000000000000, 0.9659258262890683122, 1.000000000000000000, 0.9659258262890683122, 1.000000000000000000, 0.9659258262890683122, 1.000000000000000000, 0.9659258262890683122, 1.000000000000000000, 0.9659258262890683122, 1.000000000000000000, 0.9659258262890683122, 1.000000000000000000, 0.9659258262890683122, 1.000000000000000000, 0.9659258262890683122, 1.000000000000000000, 0.9659258262890683122, 1.000000000000000000, 0.9659258262890683122, 1.000000000000000000, 0.9659258262890683122, 1.000000000000000000, 0.9659258262890683122, 1.000000000000000000, 0.9659258262890683122, 1.000000000000000000, 0.9659258262890683122, 1.000000000000000000, 0.9659258262890683122, 1.000000000000000000, 0.9659258262890683122, 1.000000000000000000, 0.9659258262890683122, 1.000000000000000000, 0.9659258262890683122, 1.000000000000000000, 0.9659258262890683122, 1.000000000000000000, 0.9659258262890683122, 1.000000000000000000, 0.9659258262890683122, 1.000000000000000000, 0.9659258262890683122, 1.000000000000000000, 0.9659258262890683122, 1.000000000000000000, 0.9659258262890683122, 1.000000000000000000, 0.9659258262890683122, 1.000000000000000000, 0.9659258262890683122, 1.000000000000000000, 0.9659258262890683122, 1.000000000000000000, 0.9659258262890683122, 1.000000000000000000, 0.9659258262890683122, 1.000000000000000000, 0.9659258262890683122, 1.000000000000000000, 0.9659258262890683122, 1.000000000000000000, 0.9659258262890683122, 1.000000000000000000, 0.9659258262890683122, 1.000000000000000000, 0.9659258262890683122, 1.000000000000000000, 0.9659258262890683122, 1.000000000000000000, 0.9659258262890683122, 1.000000000000000000, 0.9659258262890683122, 1.000000000000000000, 0.9659258262890683122, 1.000000000000000000, 0.9659258262890683122, 1.000000000000000000, 0.9659258262890683122, 1.000000000000000000, 0.9659258262890683122, 1.000000000000000000, 0.9659258262890683122, 1.000000000000000000, 0.9659258262890683122, 1.000000000000000000, 0.9659258262890683122, 1.000000000000000000, 0.9659258262890683122, 1.000000000000000000, 0.9659258262890683122, 1.000000000000000000, 0.9659258262890683122, 1.000000000000000000, 0.9659258262890683122, 1.000000000000000000, 0.9659258262890683122, 1.000000000000000000, 0.9659258262890683122, 1.000000000000000000, 0.9659258262890683122, 1.000000000000000000, 0.9659258262890683122, 1.000000000000000000, 0.9659258262890683122, 1.000000000000000000, 0.9659258262890683122, 1.000000000000000000, 0.9659258262890683122, 1.000000000000000000, 0.9659258262890683122, 1.000000000000000000, 0.9659258262890683122, 1.000000000000000000, 0.9659258262890683122, 1.000000000000000000, 0.9659258262890683122, 1.000000000000000000, 0.9659258262890683122, 1.000000000000000000, 0.9659258262890683122, 1.000000000000000000, 0.9659258262890683122, 1.000000000000000000, 0.9659258262890683122, 1.000000000000000000, 0.9659258262890683122, 1.000000000000000000, 0.9659258262890683122, 1.000000000000000000, 0.9659258262890683122, 1.000000000000000000, 0.9659258262890683122, 1.000000000000000000, 0.9659258262890683122, 1.000000000000000000, 0.9659258262890683122, 1.000000000000000000, 0.9659258262890683122, 1.000000000000000000, 0.9659258262890683122, 1.000000000000000000, 0.9659258262890683122, 1.000000000000000000, 0.9659258262890683122, 1.000000000000000000, 0.9659258262890683122, 1.000000000000000000, 0.9659258262890683122, 1.000000000000000000, 0.9659258262890683122, 1.000000000000000000, 0.9659258262890683122, 1.000000000000000000, 0.9659258262890683122, 1.000000000000000000, 0.9659258262890683122, 1.000000000000000000, 0.9659258262890683122, 1.000000000000000000, 0.9659258262890683122, 1.000000000000000000, 0.9659258262890683122, 1.000000000000000000, 0.9659258262890683122, 1.000000000000000000, 0.9659258262890683122, 1.000000000000000000, 0.9659258262890683122, 1.000000000000000000, 0.9659258262890683122, 1.000000000000000000, 0.9659258262890683122, 1.000000000000000000),
 ( 1.000000000000000000, 0.9659258262890683122, 1.000000000000000000, 0.9659258262890683122, 1.000000000000000000, 0.9659258262890683122, 1.000000000000000000, 0.9659258262890683122, 1.000000000000000000, 0.9659258262890683122, 1.000000000000000000, 0.9659258262890683122, 1.000000000000000000, 0.9659258262890683122, 1.000000000000000000, 0.9659258262890683122, 1.000000000000000000, 0.9659258262890683122, 1.000000000000000000, 0.9659258262890683122, 1.000000000000000000, 0.9659258262890683122, 1.000000000000000000, 0.9659258262890683122, 1.000000000000000000, 0.9659258262890683122, 1.000000000000000000, 0.9659258262890683122, 1.000000000000000000, 0.9659258262890683122, 1.000000000000000000, 0.9659258262890683122, 1.000000000000000000, 0.9659258262890683122, 1.000000000000000000, 0.9659258262890683122, 1.000000000000000000, 0.9659258262890683122, 1.000000000000000000, 0.9659258262890683122, 1.000000000000000000, 0.9659258262890683122, 1.000000000000000000, 0.9659258262890683122, 1.000000000000000000, 0.9659258262890683122, 1.000000000000000000, 0.9659258262890683122, 1.000000000000000000, 0.9659258262890683122, 1.000000000000000000, 0.9659258262890683122, 1.000000000000000000, 0.9659258262890683122, 1.000000000000000000, 0.9659258262890683122, 1.000000000000000000, 0.9659258262890683122, 1.000000000000000000, 0.9659258262890683122, 1.000000000000000000, 0.9659258262890683122, 1.000000000000000000, 0.9659258262890683122, 1.000000000000000000, 0.9659258262890683122, 1.000000000000000000, 0.9659258262890683122, 1.000000000000000000, 0.9659258262890683122, 1.000000000000000000, 0.9659258262890683122, 1.000000000000000000, 0.9659258262890683122, 1.000000000000000000, 0.9659258262890683122, 1.000000000000000000, 0.9659258262890683122, 1.000000000000000000, 0.9659258262890683122, 1.000000000000000000, 0.9659258262890683122, 1.000000000000000000, 0.9659258262890683122, 1.000000000000000000, 0.9659258262890683122, 1.000000000000000000, 0.9659258262890683122, 1.000000000000000000, 0.9659258262890683122, 1.000000000000000000, 0.9659258262890683122, 1.000000000000000000, 0.9659258262890683122, 1.000000000000000000, 0.9659258262890683122, 1.000000000000000000, 0.9659258262890683122, 1.000000000000000000, 0.9659258262890683122, 1.000000000000000000, 0.9659258262890683122, 1.000000000000000000, 0.9659258262890683122, 1.000000000000000000, 0.9659258262890683122, 1.000000000000000000, 0.9659258262890683122, 1.000000000000000000, 0.9659258262890683122, 1.000000000000000000, 0.9659258262890683122, 1.000000000000000000, 0.9659258262890683122, 1.000000000000000000, 0.9659258262890683122, 1.000000000000000000, 0.9659258262890683122, 1.000000000000000000, 0.9659258262890683122, 1.000000000000000000, 0.9659258262890683122, 1.000000000000000000, 0.9659258262890683122, 1.000000000000000000, 0.9659258262890683122, 1.000000000000000000, 0.9659258262890683122, 1.000000000000000000, 0.9659258262890683122, 1.000000000000000000, 0.9659258262890683122, 1.000000000000000000, 0.9659258262890683122, 1.000000000000000000, 0.9659258262890683122, 1.000000000000000000, 0.9659258262890683122, 1.000000000000000000, 0.9659258262890683122, 1.000000000000000000, 0.9659258262890683122, 1.000000000000000000, 0.9659258262890683122, 1.000000000000000000, 0.9659258262890683122, 1.000000000000000000, 0.9659258262890683122, 1.000000000000000000, 0.9659258262890683122, 1.000000000000000000, 0.9659258262890683122, 1.000000000000000000, 0.9659258262890683122, 1.000000000000000000, 0.9659258262890683122, 1.000000000000000000, 0.9659258262890683122, 1.000000000000000000, 0.9659258262890683122, 1.000000000000000000, 0.9659258262890683122, 1.000000000000000000, 0.9659258262890683122, 1.000000000000000000, 0.9659258262890683122, 1.000000000000000000, 0.9659258262890683122, 1.000000000000000000, 0.9659258262890683122, 1.000000000000000000, 0.9659258262890683122, 1.000000000000000000, 0.9659258262890683122, 1.000000000000000000, 0.9659258262890683122, 1.000000000000000000, 0.9659258262890683122, 1.000000000000000000, 0.9659258262890683122, 1.000000000000000000, 0.9659258262890683122, 1.000000000000000000, 0.9659258262890683122, 1.000000000000000000, 0.9659258262890683122, 1.000000000000000000, 0.9659258262890683122, 1.000000000000000000, 0.9659258262890683122, 1.000000000000000000, 0.9659258262890683122, 1.000000000000000000, 0.9659258262890683122, 1.000000000000000000, 0.9659258262890683122, 1.000000000000000000, 0.9659258262890683122, 1.000000000000000000, 0.9659258262890683122, 1.000000000000000000, 0.9659258262890683122, 1.000000000000000000, 0.9659258262890683122, 1.000000000000000000, 0.9659258262890683122, 1.000000000000000000, 0.9659258262890683122, 1.000000000000000000, 0.9659258262890683122, 1.000000000000000000, 0.9659258262890683122, 1.000000000000000000, 0.9659258262890683122, 1.000000000000000000, 0.9659258262890683122, 1.000000000000000000, 0.9659258262890683122, 1.000000000000000000, 0.9659258262890683122, 1.000000000000000000, 0.9659258262890683122, 1.000000000000000000, 0.9659258262890683122, 1.000000000000000000, 0.9659258262890683122, 1.000000000000000000, 0.9659258262890683122, 1.000000000000000000, 0.9659258262890683122, 1.000000000000000000, 0.9659258262890683122, 1.000000000000000000, 0.9659258262890683122, 1.000000000000000000, 0.9659258262890683122, 1.000000000000000000, 0.9659258262890683122, 1.000000000000000000, 0.9659258262890683122, 1.000000000000000000, 0.9659258262890683122, 1.000000000000000000, 0.9659258262890683122, 1.000000000000000000, 0.9659258262890683122, 1.000000000000000000, 0.9659258262890683122, 1.000000000000000000, 0.9659258262890683122, 1.000000000000000000, 0.9659258262890683122, 1.000000000000000000, 0.9659258262890683122, 1.000000000000000000, 0.9659258262890683122, 1.000000000000000000, 0.9659258262890683122, 1.000000000000000000, 0.9659258262890683122, 1.000000000000000000, 0.9659258262890683122, 1.000000000000000000, 0.9659258262890683122, 1.000000000000000000, 0.9659258262890683122, 1.000000000000000000, 0.9659258262890683122, 1.000000000000000000, 0.9659258262890683122, 1.000000000000000000, 0.9659258262890683122, 1.000000000000000000, 0.9659258262890683122, 1.000000000000000000, 0.9659258262890683122, 1.000000000000000000, 0.9659258262890683122, 1.000000000000000000, 0.9659258262890683122, 1.000000000000000000, 0.9659258262890683122, 1.000000000000000000, 0.9659258262890683122, 1.000000000000000000, 0.9659258262890683122, 1.000000000000000000, 0.9659258262890683122, 1.000000000000000000, 0.9659258262890683122, 1.000000000000000000, 0.9659258262890683122, 1.000000000000000000, 0.9659258262890683122, 1.000000000000000000, 0.9659258262890683122, 1.000000000000000000, 0.9659258262890683122, 1.000000000000000000, 0.9659258262890683122, 1.000000000000000000, 0.9659258262890683122, 1.000000000000000000, 0.9659258262890683122, 1.000000000000000000, 0.9659258262890683122, 1.000000000000000000, 0.9659258262890683122, 1.000000000000000000, 0.9659258262890683122, 1.000000000000000000, 0.9659258262890683122, 1.000000000000000000, 0.9659258262890683122, 1.000000000000000000, 0.9659258262890683122, 1.000000000000000000, 0.9659258262890683122, 1.000000000000000000, 0.9659258262890683122, 1.000000000000000000, 0.9659258262890683122, 1.000000000000000000, 0.9659258262890683122, 1.000000000000000000, 0.9659258262890683122, 1.000000000000000000, 0.9659258262890683122, 1.000000000000000000, 0.9659258262890683122, 1.000000000000000000, 0.9659258262890683122, 1.000000000000000000, 0.9659258262890683122, 1.000000000000000000, 0.9659258262890683122, 1.000000000000000000, 0.9659258262890683122, 1.000000000000000000, 0.9659258262890683122, 1.000000000000000000, 0.9659258262890683122, 1.000000000000000000, 0.9659258262890683122, 1.000000000000000000, 0.9659258262890683122, 1.000000000000000000, 0.9659258262890683122, 1.000000000000000000, 0.9659258262890683122, 1.000000000000000000, 0.9659258262890683122, 1.000000000000000000, 0.9659258262890683122, 1.000000000000000000, 0.9659258262890683122, 1.000000000000000000, 0.9659258262890683122, 1.000000000000000000, 0.9659258262890683122, 1.000000000000000000, 0.9659258262890683122, 1.000000000000000000, 0.9659258262890683122, 1.000000000000000000, 0.9659258262890683122, 1.000000000000000000, 0.9659258262890683122, 1.000000000000000000, 0.9659258262890683122, 1.000000000000000000, 0.9659258262890683122, 1.000000000000000000, 0.9659258262890683122, 1.000000000000000000, 0.9659258262890683122, 1.000000000000000000, 0.9659258262890683122, 1.000000000000000000, 0.9659258262890683122, 1.000000000000000000, 0.9659258262890683122, 1.000000000000000000, 0.9659258262890683122, 1.000000000000000000, 0.9659258262890683122, 1.000000000000000000, 0.9659258262890683122, 1.000000000000000000, 0.9659258262890683122, 1.000000000000000000, 0.9659258262890683122, 1.000000000000000000, 0.9659258262890683122, 1.000000000000000000, 0.9659258262890683122, 1.000000000000000000, 0.9659258262890683122, 1.000000000000000000, 0.9659258262890683122, 1.000000000000000000, 0.9659258262890683122, 1.000000000000000000, 0.9659258262890683122, 1.000000000000000000, 0.9659258262890683122, 1.000000000000000000, 0.9659258262890683122, 1.000000000000000000, 0.9659258262890683122, 1.000000000000000000, 0.9659258262890683122, 1.000000000000000000, 0.9659258262890683122, 1.000000000000000000, 0.9659258262890683122, 1.000000000000000000, 0.9659258262890683122, 1.000000000000000000, 0.9659258262890683122, 1.000000000000000000, 0.9659258262890683122, 1.000000000000000000, 0.9659258262890683122, 1.000000000000000000, 0.9659258262890683122, 1.000000000000000000, 0.9659258262890683122, 1.000000000000000000, 0.9659258262890683122, 1.000000000000000000, 0.9659258262890683122, 1.000000000000000000, 0.9659258262890683122, 1.000000000000000000, 0.9659258262890683122, 1.000000000000000000, 0.9659258262890683122, 1.000000000000000000, 0.9659258262890683122, 1.000000000000000000, 0.9659258262890683122, 1.000000000000000000, 0.9659258262890683122, 1.000000000000000000, 0.9659258262890683122, 1.000000000000000000, 0.9659258262890683122, 1.000000000000000000, 0.9659258262890683122, 1.000000000000000000, 0.9659258262890683122, 1.000000000000000000, 0.9659258262890683122, 1.000000000000000000, 0.9659258262890683122, 1.000000000000000000, 0.9659258262890683122, 1.000000000000000000, 0.9659258262890683122, 1.000000000000000000, 0.9659258262890683122, 1.000000000000000000, 0.9659258262890683122, 1.000000000000000000, 0.9659258262890683122, 1.000000000000000000, 0.9659258262890683122, 1.000000000000000000, 0.9659258262890683122, 1.000000000000000000, 0.9659258262890683122, 1.000000000000000000, 0.9659258262890683122, 1.000000000000000000, 0.9659258262890683122, 1.000000000000000000, 0.9659258262890683122, 1.000000000000000000, 0.9659258262890683122, 1.000000000000000000, 0.9659258262890683122, 1.000000000000000000, 0.9659258262890683122, 1.000000000000000000, 0.9659258262890683122, 1.000000000000000000, 0.9659258262890683122, 1.000000000000000000, 0.9659258262890683122, 1.000000000000000000, 0.9659258262890683122, 1.000000000000000000, 0.9659258262890683122, 1.000000000000000000, 0.9659258262890683122, 1.000000000000000000, 0.9659258262890683122, 1.000000000000000000, 0.9659258262890683122, 1.000000000000000000, 0.9659258262890683122, 1.000000000000000000, 0.9659258262890683122, 1.000000000000000000, 0.9659258262890683122, 1.000000000000000000, 0.9659258262890683122, 1.000000000000000000, 0.9659258262890683122, 1.000000000000000000) ) ) 
 REPRESENTATION_ITEM ( '' )  SURFACE ( )  );
#41789=CARTESIAN_POINT ( 'NONE',  ( -1.193521905106661674, 2.660739321503277841E-15, -0.3464511005275191513 ) ) ;
#41792=CARTESIAN_POINT ( 'NONE',  ( 0.9317585301837276734, 0.05413385826771626580, -0.4176697321401330321 ) ) ;
#41793=CARTESIAN_POINT ( 'NONE',  ( 0.07217847769028949700, -0.05778040916215560624, -0.4822834645669293319 ) ) ;
#41794=CARTESIAN_POINT ( 'NONE',  ( -0.9711286089238838626, 0.2306618581243847221, -0.2411417322834647770 ) ) ;
#41795=CARTESIAN_POINT ( 'NONE',  ( 1.069553805774278610, -0.6692913385826771977, 0.1292274648535927661 ) ) ;
#41796=CARTESIAN_POINT ( 'NONE',  ( 0.4199475065616805614, 0.2306618581243848609, 0.2411417322834645549 ) ) ;
#41798=CARTESIAN_POINT ( 'NONE',  ( -0.4527559055118102749, 0.1660481256975885056, 0.3530559997133364547 ) ) ;
#41799=CARTESIAN_POINT ( 'NONE',  ( 0.7742782152230979209, 0.05413385826771626580, -0.4176697321401330321 ) ) ;
#41800=CARTESIAN_POINT ( 'NONE',  ( -0.05905511811023545637, 0.1660481256975885056, 0.3530559997133364547 ) ) ;
#41801=CARTESIAN_POINT ( 'NONE',  ( 0.7545931758530189937, 0.1771653543307087075, -0.09757992244046823083 ) ) ;
#41802=CARTESIAN_POINT ( 'NONE',  ( -1.430446194225721390, -0.4281496062992124485, 0.4176697321401328655 ) ) ;
#41803=CARTESIAN_POINT ( 'NONE',  ( -1.686351706036744558, 0.2952755905511810774, -0.1292274648535930714 ) ) ;
#41804=CARTESIAN_POINT ( 'NONE',  ( 0.4527559055118117182, -0.5400638737290844871, 0.3530559997133364547 ) ) ;
#41805=EDGE_CURVE ( 'NONE', #71856, #73064, #4911, .T. ) ;
#41807=VERTEX_POINT ( 'NONE', #35373 ) ;
#41809=CARTESIAN_POINT ( 'NONE',  ( 1.161417322834646493, -0.5400638737290844871, 0.3530559997133364547 ) ) ;
#41810=CARTESIAN_POINT ( 'NONE',  ( 0.4527559055118117182, -0.4536011799217367080, 0.2665933059059888421 ) ) ;
#41818=CARTESIAN_POINT ( 'NONE',  ( 0.9973753280839902091, 0.2306618581243847221, -0.2411417322834647770 ) ) ;
#41819=CARTESIAN_POINT ( 'NONE',  ( -0.7020997375328074108, -0.05778040916215522460, 0.4822834645669289988 ) ) ;
#41820=CARTESIAN_POINT ( 'NONE',  ( -0.8530183727034112984, -0.4281496062992127816, -0.4176697321401328100 ) ) ;
#41821=CARTESIAN_POINT ( 'NONE',  ( 0.6758530183727039509, 0.2952755905511810774, -0.1292274648535930714 ) ) ;
#41822=ORIENTED_EDGE ( 'NONE', *, *, #38303, .F. ) ;
#41824=CARTESIAN_POINT ( 'NONE',  ( 1.259842519685040019, -0.1870078740157479769, 0.4822834645669291653 ) ) ;
#41826=PRODUCT_CONTEXT ( 'NONE', #9492, 'mechanical' ) ;
#41829=CARTESIAN_POINT ( 'NONE',  ( -1.187664041994749731, -0.2845877964562159024, 0.3641732283464567677 ) ) ;
#41831=CARTESIAN_POINT ( 'NONE',  ( 0.1181102362204730916, 0.2952755905511811885, 0.000000000000000000 ) ) ;
#41832=CARTESIAN_POINT ( 'NONE',  ( 1.555118110236221041, 0.1660481256975883668, -0.3530559997133364547 ) ) ;
#41834=CARTESIAN_POINT ( 'NONE',  ( -1.286089238845143479, -0.5023911411419708095, 0.1820866141732285504 ) ) ;
#41835=CARTESIAN_POINT ( 'NONE',  ( 0.2230971128608932319, -0.4281496062992124485, 0.4176697321401328655 ) ) ;
#41836=CARTESIAN_POINT ( 'NONE',  ( 1.167979002624672580, -0.004921259842519870586, -0.3153832671262229437 ) ) ;
#41838=CARTESIAN_POINT ( 'NONE',  ( -1.266404199475064773, -0.2845877964562159024, 0.3641732283464567677 ) ) ;
#41839=CARTESIAN_POINT ( 'NONE',  ( 1.568241469816273659, -0.05778040916215560624, -0.4822834645669293319 ) ) ;
#41841=CARTESIAN_POINT ( 'NONE',  ( -0.3477690288713905509, -0.6692913385826771977, 0.1292274648535927661 ) ) ;
#41842=CARTESIAN_POINT ( 'NONE',  ( -1.456692913385826182, 0.1771653543307087630, 0.000000000000000000 ) ) ;
#41843=CARTESIAN_POINT ( 'NONE',  ( -0.5118110236220466680, -0.5511811023622047445, 6.969142054262312111E-17 ) ) ;
#41844=VECTOR ( 'NONE', #7052, 39.37007874015748143 ) ;
#41845=CARTESIAN_POINT ( 'NONE',  ( -0.6496062992125976043, -0.5400638737290844871, 0.3530559997133364547 ) ) ;
#41846=CARTESIAN_POINT ( 'NONE',  ( -1.574803149606298192, -0.1870078740157480601, -0.3641732283464567677 ) ) ;
#41848=CARTESIAN_POINT ( 'NONE',  ( 0.3477690288713918276, 0.2952755905511811885, 0.1292274648535926551 ) ) ;
#41851=CARTESIAN_POINT ( 'NONE',  ( -1.154855643044618851, -0.6046776061558809534, -0.2411417322834644161 ) ) ;
#41852=CARTESIAN_POINT ( 'NONE',  ( -0.6561679790026240244, -0.5023911411419708095, 0.1820866141732285504 ) ) ;
#41853=CARTESIAN_POINT ( 'NONE',  ( 1.171093442848939681, -8.644661201599092366E-16, -0.4445507791589066171 ) ) ;
#41854=CARTESIAN_POINT ( 'NONE',  ( 0.2230971128608932319, -0.4281496062992124485, 0.4176697321401328655 ) ) ;
#41855=CARTESIAN_POINT ( 'NONE',  ( 0.2624671916010504757, 0.1283753931104748280, 0.1820866141732283561 ) ) ;
#41856=CARTESIAN_POINT ( 'NONE',  ( -0.6430446194225716283, -0.3690944881889763329, 0.3153832671262228327 ) ) ;
#41857=CARTESIAN_POINT ( 'NONE',  ( -1.332020997375327642, -0.3162353388693409650, -0.4822834645669289433 ) ) ;
#41858=CARTESIAN_POINT ( 'NONE',  ( -1.397637795275589623, 0.1660481256975885056, 0.3530559997133364547 ) ) ;
#41859=CARTESIAN_POINT ( 'NONE',  ( 1.318897637795276356, -0.5400638737290844871, 0.3530559997133364547 ) ) ;
#41861=CARTESIAN_POINT ( 'NONE',  ( 0.5314960629921267055, -0.4536011799217367080, 0.2665933059059888421 ) ) ;
#41862=CARTESIAN_POINT ( 'NONE',  ( 0.9645669291338591078, -0.5400638737290845981, -0.3530559997133363437 ) ) ;
#41864=CARTESIAN_POINT ( 'NONE',  ( 1.377952755905512472, -0.5511811023622047445, 6.969142054262312111E-17 ) ) ;
#41866=CARTESIAN_POINT ( 'NONE',  ( -1.056430446194224881, -0.6692913385826771977, 0.1292274648535927661 ) ) ;
#41867=B_SPLINE_CURVE_WITH_KNOTS ( 'NONE', 3,
 ( #58980, #19847, #3401, #34974 ),
 .UNSPECIFIED., .F., .F.,
 ( 4, 4 ),
 ( 0.02793953716399259421, 0.02824248980525632252 ),
 .UNSPECIFIED. ) ;
#41868=CARTESIAN_POINT ( 'NONE',  ( -0.8398950131233585692, 0.2306618581243848609, 0.2411417322834645549 ) ) ;
#41869=CARTESIAN_POINT ( 'NONE',  ( 0.1902887139107617975, 0.2952755905511811885, 0.1292274648535926551 ) ) ;
#41870=CARTESIAN_POINT ( 'NONE',  ( -1.279527559055116948, -0.4536011799217367080, 0.2665933059059888421 ) ) ;
#41872=CARTESIAN_POINT ( 'NONE',  ( 1.535433070866142335, -0.5511811023622047445, 6.969142054262312111E-17 ) ) ;
#41873=CARTESIAN_POINT ( 'NONE',  ( 0.5577427821522316087, -0.05778040916215522460, 0.4822834645669289988 ) ) ;
#41874=CARTESIAN_POINT ( 'NONE',  ( 0.7152230971128614723, -0.3162353388693409650, -0.4822834645669289433 ) ) ;
#41875=CARTESIAN_POINT ( 'NONE',  ( 1.535433070866142558, 0.2952755905511811885, 0.000000000000000000 ) ) ;
#41881=CARTESIAN_POINT ( 'NONE',  ( -0.1837270341207343505, -0.5023911411419708095, 0.1820866141732285504 ) ) ;
#41883=CARTESIAN_POINT ( 'NONE',  ( -0.1771653543307080136, -0.5400638737290844871, 0.3530559997133364547 ) ) ;
#41884=CARTESIAN_POINT ( 'NONE',  ( 0.8792650918635177559, -0.4281496062992127816, -0.4176697321401328100 ) ) ;
#41886=CARTESIAN_POINT ( 'NONE',  ( -0.1902887139107604098, 0.1771653543307087075, -0.09757992244046823083 ) ) ;
#41887=CARTESIAN_POINT ( 'NONE',  ( -1.259842519685038686, -0.1870078740157480879, -0.4822834645669291653 ) ) ;
#41888=CARTESIAN_POINT ( 'NONE',  ( 1.135170603674541256, 0.2952755905511811885, 0.1292274648535926551 ) ) ;
#41893=VERTEX_POINT ( 'NONE', #45169 ) ;
#41894=CARTESIAN_POINT ( 'NONE',  ( 0.8530183727034126306, 0.05413385826771626580, -0.4176697321401330321 ) ) ;
#41895=CARTESIAN_POINT ( 'NONE',  ( 1.614173228346457378, 0.1771653543307087630, 0.000000000000000000 ) ) ;
#41896=CARTESIAN_POINT ( 'NONE',  ( -1.469816272965878357, 0.1283753931104748280, 0.1820866141732283561 ) ) ;
#41897=CARTESIAN_POINT ( 'NONE',  ( -1.633858267716534529, 0.1660481256975885056, 0.3530559997133364547 ) ) ;
#41899=FACE_OUTER_BOUND ( 'NONE', #2999, .T. ) ;
#41900=CARTESIAN_POINT ( 'NONE',  ( 1.325459317585302665, -0.4281496062992124485, 0.4176697321401328655 ) ) ;
#41901=CARTESIAN_POINT ( 'NONE',  ( -1.456692913385826182, -0.6692913385826771977, 8.415575281601705876E-17 ) ) ;
#41902=CARTESIAN_POINT ( 'NONE',  ( 0.04593175853018440641, 0.2952755905511810774, -0.1292274648535930714 ) ) ;
#41903=CARTESIAN_POINT ( 'NONE',  ( -0.7349081364829390672, 0.2306618581243847221, -0.2411417322834647770 ) ) ;
#41904=CARTESIAN_POINT ( 'NONE',  ( -1.614173228346455824, 0.2952755905511811885, 0.000000000000000000 ) ) ;
#41906=CARTESIAN_POINT ( 'NONE',  ( 0.03937007874015806264, 0.2952755905511811885, 0.000000000000000000 ) ) ;
#41908=CARTESIAN_POINT ( 'NONE',  ( -1.174540682414697335, -0.08942795157527998196, 0.3641732283464567121 ) ) ;
#41913=CARTESIAN_POINT ( 'NONE',  ( -1.568241469816272105, -0.05778040916215522460, 0.4822834645669289988 ) ) ;
#41915=CARTESIAN_POINT ( 'NONE',  ( 1.646981627296588035, -0.2845877964562159024, 0.3641732283464567677 ) ) ;
#41916=CARTESIAN_POINT ( 'NONE',  ( -1.706036745406823485, 0.2306618581243848609, 0.2411417322834645549 ) ) ;
#41921=CARTESIAN_POINT ( 'NONE',  ( -0.1312335958005241554, -0.5023911411419708095, -0.1820866141732282451 ) ) ;
#41922=CARTESIAN_POINT ( 'NONE',  ( -0.8858267716535425107, 0.07958543189024071263, -0.2665933059059888421 ) ) ;
#41923=CARTESIAN_POINT ( 'NONE',  ( -1.358267716535432434, -0.5400638737290844871, 0.3530559997133364547 ) ) ;
#41924=EDGE_CURVE ( 'NONE', #1065, #20923, #2072, .T. ) ;
#41925=CARTESIAN_POINT ( 'NONE',  ( 0.3805774278215230400, 0.05413385826771626580, -0.4176697321401330321 ) ) ;
#41926=CARTESIAN_POINT ( 'NONE',  ( -1.430446194225720724, 0.05413385826771626580, -0.4176697321401330321 ) ) ;
#41928=ORIENTED_EDGE ( 'NONE', *, *, #79506, .T. ) ;
#41929=CARTESIAN_POINT ( 'NONE',  ( -1.574803149606298192, -0.1870078740157480879, -0.4822834645669291653 ) ) ;
#41930=CARTESIAN_POINT ( 'NONE',  ( -1.646051170424378096, 0.000000000000000000, 0.3464511005275205946 ) ) ;
#41935=CARTESIAN_POINT ( 'NONE',  ( -0.7020997375328074108, -0.05778040916215522460, 0.4822834645669289988 ) ) ;
#41936=CARTESIAN_POINT ( 'NONE',  ( 1.535433070866142558, 0.2952755905511811885, 0.000000000000000000 ) ) ;
#41937=CARTESIAN_POINT ( 'NONE',  ( -1.686351706036744558, 0.2952755905511810774, -0.1292274648535930714 ) ) ;
#41939=CARTESIAN_POINT ( 'NONE',  ( -1.561679790026246017, 0.05413385826771666132, 0.4176697321401328100 ) ) ;
#41940=CARTESIAN_POINT ( 'NONE',  ( -1.003937007874015297, -0.5400638737290845981, -0.3530559997133363437 ) ) ;
#41942=CARTESIAN_POINT ( 'NONE',  ( 0.03937007874015806264, 0.1771653543307087630, 0.000000000000000000 ) ) ;
#41944=CARTESIAN_POINT ( 'NONE',  ( 0.01968503937007957949, -0.4536011799217368745, -0.2665933059059886201 ) ) ;
#41945=CARTESIAN_POINT ( 'NONE',  ( 0.9186351706036751663, -0.5023911411419708095, 0.1820866141732285504 ) ) ;
#41946=CARTESIAN_POINT ( 'NONE',  ( 0.4986876640419954376, 0.2306618581243848609, 0.2411417322834645549 ) ) ;
#41948=CARTESIAN_POINT ( 'NONE',  ( -0.3543307086614165824, 0.1771653543307087630, 0.000000000000000000 ) ) ;
#41950=CARTESIAN_POINT ( 'NONE',  ( 1.601049868766404982, 0.2306618581243848609, 0.2411417322834645549 ) ) ;
#41951=EDGE_CURVE ( 'NONE', #8180, #55534, #13516, .T. ) ;
#41952=CARTESIAN_POINT ( 'NONE',  ( -1.423884514435694859, -0.08942795157528024563, -0.3641732283464568787 ) ) ;
#41954=CARTESIAN_POINT ( 'NONE',  ( 0.2034120734908142214, 0.2952755905511810774, -0.1292274648535930714 ) ) ;
#41955=CARTESIAN_POINT ( 'NONE',  ( -0.6299212598425188991, -0.1870078740157480879, -0.4822834645669291653 ) ) ;
#41958=CARTESIAN_POINT ( 'NONE',  ( 0.5446194225721792126, -0.08942795157528024563, -0.3641732283464568787 ) ) ;
#41959=CARTESIAN_POINT ( 'NONE',  ( -0.07874015748031421014, -0.1870078740157480601, -0.3641732283464567677 ) ) ;
#41960=CARTESIAN_POINT ( 'NONE',  ( -0.5249343832020990641, 0.2306618581243848609, 0.2411417322834645549 ) ) ;
#41963=CARTESIAN_POINT ( 'NONE',  ( 0.2624671916010504757, 0.2306618581243848609, 0.2411417322834645549 ) ) ;
#41966=CARTESIAN_POINT ( 'NONE',  ( 1.496062992125984703, -0.1870078740157480879, -0.4822834645669291653 ) ) ;
#41967=CARTESIAN_POINT ( 'NONE',  ( -0.2690288713910754526, 0.1771653543307087075, -0.09757992244046823083 ) ) ;
#41968=CARTESIAN_POINT ( 'NONE',  ( -0.6036745406824141069, 0.2306618581243848609, 0.2411417322834645549 ) ) ;
#41969=CARTESIAN_POINT ( 'NONE',  ( -1.581364829396324945, -0.08942795157528024563, -0.3641732283464568787 ) ) ;
#41970=CARTESIAN_POINT ( 'NONE',  ( 1.286089238845145033, -0.6046776061558809534, -0.2411417322834644161 ) ) ;
#41972=CARTESIAN_POINT ( 'NONE',  ( -0.7939632545931754048, -0.2845877964562159024, 0.3641732283464567677 ) ) ;
#41976=CARTESIAN_POINT ( 'NONE',  ( 1.614173228346457378, -0.5511811023622047445, 6.969142054262312111E-17 ) ) ;
#41977=CARTESIAN_POINT ( 'NONE',  ( 1.069553805774278610, -0.5511811023622046335, 0.09757992244046803654 ) ) ;
#41978=CARTESIAN_POINT ( 'NONE',  ( 0.9908136482939640111, 0.2952755905511810774, -0.1292274648535930714 ) ) ;
#41979=CARTESIAN_POINT ( 'NONE',  ( 0.4596682205436344870, 0.004960608223779807216, -0.3437734562760184631 ) ) ;
#41980=CARTESIAN_POINT ( 'NONE',  ( 0.9317585301837276734, -0.4281496062992124485, 0.4176697321401328655 ) ) ;
#41982=CARTESIAN_POINT ( 'NONE',  ( 1.023622047244095334, -0.1870078740157479769, 0.3641732283464567677 ) ) ;
#41983=CARTESIAN_POINT ( 'NONE',  ( 0.2099737532808405305, -0.6046776061558807314, 0.2411417322834647770 ) ) ;
#41984=CARTESIAN_POINT ( 'NONE',  ( -0.6167979002624665030, -0.4281496062992127816, -0.4176697321401328100 ) ) ;
#41985=CARTESIAN_POINT ( 'NONE',  ( 1.607611548556431069, -0.6692913385826773087, -0.1292274648535924053 ) ) ;
#41988=CARTESIAN_POINT ( 'NONE',  ( 0.4921259842519691285, 0.07958543189024085140, 0.2665933059059887866 ) ) ;
#41989=ORIENTED_EDGE ( 'NONE', *, *, #76459, .T. ) ;
#41993=CARTESIAN_POINT ( 'NONE',  ( -0.5118110236220466680, -0.6692913385826771977, 8.415575281601705876E-17 ) ) ;
#41994=CARTESIAN_POINT ( 'NONE',  ( -0.2296587926509179312, -0.05778040916215522460, 0.4822834645669289988 ) ) ;
#41995=CARTESIAN_POINT ( 'NONE',  ( -0.4199475065616791736, -0.6046776061558807314, 0.2411417322834647770 ) ) ;
#41996=CARTESIAN_POINT ( 'NONE',  ( 0.5905511811023629321, 0.2952755905511811885, 0.000000000000000000 ) ) ;
#41997=CARTESIAN_POINT ( 'NONE',  ( -0.9120734908136475250, -0.6692913385826773087, -0.1292274648535924053 ) ) ;
#41998=CARTESIAN_POINT ( 'NONE',  ( -0.2099737532808391705, -0.6046776061558809534, -0.2411417322834644161 ) ) ;
#41999=CARTESIAN_POINT ( 'NONE',  ( 1.220472440944882386, -0.6692913385826771977, 8.415575281601705876E-17 ) ) ;
#42001=CARTESIAN_POINT ( 'NONE',  ( 0.9645669291338588858, 0.1660481256975885056, 0.3530559997133364547 ) ) ;
#42002=CARTESIAN_POINT ( 'NONE',  ( 0.6758530183727039509, -0.6692913385826771977, 0.1292274648535927661 ) ) ;
#42004=CARTESIAN_POINT ( 'NONE',  ( -0.04593175853018302557, 0.1771653543307087630, 0.09757992244046791164 ) ) ;
#42005=EDGE_LOOP ( 'NONE', ( #32268, #44777, #53240, #31043 ) ) ;
#42008=CARTESIAN_POINT ( 'NONE',  ( -0.6758530183727028406, -0.5511811023622048555, -0.09757992244046775898 ) ) ;
#42009=CARTESIAN_POINT ( 'NONE',  ( -0.6692913385826764205, 0.2952755905511811885, 0.000000000000000000 ) ) ;
#42011=CARTESIAN_POINT ( 'NONE',  ( -0.7414698162729651543, 0.2952755905511810774, -0.1292274648535930714 ) ) ;
#42012=CARTESIAN_POINT ( 'NONE',  ( -0.4396325459317579898, 0.2952755905511811885, 0.1292274648535926551 ) ) ;
#42013=CARTESIAN_POINT ( 'NONE',  ( -1.187664041994749731, -0.3162353388693405765, 0.4822834645669290543 ) ) ;
#42014=EDGE_CURVE ( 'NONE', #15840, #4749, #64136, .T. ) ;
#42015=CARTESIAN_POINT ( 'NONE',  ( -1.312335958005248715, -0.6046776061558809534, -0.2411417322834644161 ) ) ;
#42016=CARTESIAN_POINT ( 'NONE',  ( 0.8923884514435703741, 0.1283753931104748280, 0.1820866141732283561 ) ) ;
#42017=DIRECTION ( 'NONE',  ( 1.000000000000000000, -0.000000000000000000, -0.000000000000000000 ) ) ;
#42019=CARTESIAN_POINT ( 'NONE',  ( 0.2755905511811031494, -0.5511811023622047445, 6.969142054262312111E-17 ) ) ;
#42020=CARTESIAN_POINT ( 'NONE',  ( -0.09186351706036663400, -0.4281496062992124485, 0.4176697321401328655 ) ) ;
#42021=CARTESIAN_POINT ( 'NONE',  ( -0.1246719160104980823, -0.6692913385826773087, -0.1292274648535924053 ) ) ;
#42027=CARTESIAN_POINT ( 'NONE',  ( 1.522309711286089939, -0.6046776061558809534, -0.2411417322834644161 ) ) ;
#42028=CARTESIAN_POINT ( 'NONE',  ( -0.8595800524934373854, -0.2845877964562161244, -0.3641732283464567121 ) ) ;
#42029=CARTESIAN_POINT ( 'NONE',  ( -1.003937007874015297, -0.5400638737290845981, -0.3530559997133363437 ) ) ;
#42031=( BOUNDED_CURVE ( )  B_SPLINE_CURVE ( 3, ( #23779, #22129, #22953, #49034 ),
 .UNSPECIFIED., .F., .F. ) 
 B_SPLINE_CURVE_WITH_KNOTS ( ( 4, 4 ),
 ( 1.780411317419258177, 1.780674070178078994 ),
 .UNSPECIFIED. ) 
 CURVE ( )  GEOMETRIC_REPRESENTATION_ITEM ( )  RATIONAL_B_SPLINE_CURVE ( ( 1.000000000000000000, 0.9999999942467490133, 0.9999999942467490133, 1.000000000000000000 ) ) 
 REPRESENTATION_ITEM ( '' )  );
#42033=CARTESIAN_POINT ( 'NONE',  ( -1.482939632545930975, -0.004921259842519576551, 0.3153832671262227771 ) ) ;
#42034=CARTESIAN_POINT ( 'NONE',  ( 0.3477690288713918276, 0.2952755905511811885, 0.1292274648535926551 ) ) ;
#42035=CARTESIAN_POINT ( 'NONE',  ( 0.6299212598425204535, -0.1870078740157480879, -0.4822834645669291653 ) ) ;
#42036=CARTESIAN_POINT ( 'NONE',  ( -0.7152230971128602510, -0.2845877964562159024, 0.3641732283464567677 ) ) ;
#42037=CARTESIAN_POINT ( 'NONE',  ( -0.03280839895013062252, -0.6692913385826771977, 0.1292274648535927661 ) ) ;
#42039=CARTESIAN_POINT ( 'NONE',  ( -0.4396325459317577122, -0.5511811023622048555, -0.09757992244046775898 ) ) ;
#42040=CARTESIAN_POINT ( 'NONE',  ( -0.5249343832020990641, -0.6046776061558809534, -0.2411417322834644161 ) ) ;
#42042=CARTESIAN_POINT ( 'NONE',  ( -1.522309711286088607, 0.2306618581243847221, -0.2411417322834647770 ) ) ;
#42043=CARTESIAN_POINT ( 'NONE',  ( -0.006561679790025524116, -0.2845877964562159024, 0.3641732283464567677 ) ) ;
#42044=CARTESIAN_POINT ( 'NONE',  ( 1.148293963254593875, -0.5511811023622046335, 0.09757992244046803654 ) ) ;
#42045=CARTESIAN_POINT ( 'NONE',  ( -1.312335958005248715, -0.6046776061558809534, -0.2411417322834644161 ) ) ;
#42046=CARTESIAN_POINT ( 'NONE',  ( -0.7283464566929126471, -0.4536011799217367080, 0.2665933059059888421 ) ) ;
#42048=CARTESIAN_POINT ( 'NONE',  ( -0.9711286089238838626, -0.6046776061558807314, 0.2411417322834647770 ) ) ;
#42049=CARTESIAN_POINT ( 'NONE',  ( -0.5774278215223089816, -0.6046776061558807314, 0.2411417322834647770 ) ) ;
#42050=CARTESIAN_POINT ( 'NONE',  ( 0.2755905511811031494, 0.2952755905511811885, 0.000000000000000000 ) ) ;
#42053=CARTESIAN_POINT ( 'NONE',  ( 0.4855643044619430415, -0.3690944881889765550, -0.3153832671262227771 ) ) ;
#42054=CARTESIAN_POINT ( 'NONE',  ( 1.062992125984252745, -0.6692913385826771977, 8.415575281601705876E-17 ) ) ;
#42055=CARTESIAN_POINT ( 'NONE',  ( -1.141732283464566011, -0.5511811023622047445, 6.969142054262312111E-17 ) ) ;
#42056=CARTESIAN_POINT ( 'NONE',  ( 1.154855643044620184, -0.6046776061558807314, 0.2411417322834647770 ) ) ;
#42057=CARTESIAN_POINT ( 'NONE',  ( -1.679790026246718693, 0.1283753931104746893, -0.1820866141732285504 ) ) ;
#42059=CARTESIAN_POINT ( 'NONE',  ( 1.601049868766404982, 0.1283753931104748280, 0.1820866141732283561 ) ) ;
#42060=CARTESIAN_POINT ( 'NONE',  ( -1.003937007874015297, -0.5400638737290845981, -0.3530559997133363437 ) ) ;
#42061=CARTESIAN_POINT ( 'NONE',  ( 0.03937007874015833325, -0.5511811023622047445, 6.969142054262312111E-17 ) ) ;
#42062=FACE_OUTER_BOUND ( 'NONE', #66545, .T. ) ;
#42063=CARTESIAN_POINT ( 'NONE',  ( 0.6233595800524939223, -0.2845877964562159024, 0.3641732283464567677 ) ) ;
#42064=CARTESIAN_POINT ( 'NONE',  ( -0.06561679790026180015, 0.05413385826771666132, 0.4176697321401328100 ) ) ;
#42066=CARTESIAN_POINT ( 'NONE',  ( -1.233595800524933894, 0.2306618581243848609, 0.2411417322834645549 ) ) ;
#42068=CARTESIAN_POINT ( 'NONE',  ( 1.062992125984252745, -0.5511811023622047445, 6.969142054262312111E-17 ) ) ;
#42069=CARTESIAN_POINT ( 'NONE',  ( -0.09186351706036663400, -0.4281496062992124485, 0.4176697321401328655 ) ) ;
#42070=CARTESIAN_POINT ( 'NONE',  ( -0.4002624671916004129, -0.3162353388693405765, 0.4822834645669290543 ) ) ;
#42071=CARTESIAN_POINT ( 'NONE',  ( -0.3346456692913377662, 0.07958543189024071263, -0.2665933059059888421 ) ) ;
#42073=CARTESIAN_POINT ( 'NONE',  ( -0.2755905511811015396, -0.5511811023622047445, 6.969142054262312111E-17 ) ) ;
#42074=CARTESIAN_POINT ( 'NONE',  ( 0.3543307086614181922, -0.6692913385826771977, 8.415575281601705876E-17 ) ) ;
#42075=CARTESIAN_POINT ( 'NONE',  ( -1.062992125984250968, 0.1771653543307087630, 0.000000000000000000 ) ) ;
#42077=CARTESIAN_POINT ( 'NONE',  ( -1.345144356955379816, -0.3162353388693405765, 0.4822834645669290543 ) ) ;
#42079=ORIENTED_EDGE ( 'NONE', *, *, #82598, .F. ) ;
#42080=CARTESIAN_POINT ( 'NONE',  ( -1.686351706036744558, 0.1771653543307087075, -0.09757992244046823083 ) ) ;
#42081=CARTESIAN_POINT ( 'NONE',  ( -0.6299212598425188991, -0.1870078740157479769, 0.4822834645669291653 ) ) ;
#42083=CARTESIAN_POINT ( 'NONE',  ( -1.384514435695537005, -0.6692913385826773087, -0.1292274648535924053 ) ) ;
#42086=CARTESIAN_POINT ( 'NONE',  ( 1.305774278215223960, -0.6692913385826771977, 0.1292274648535927661 ) ) ;
#42087=CARTESIAN_POINT ( 'NONE',  ( 0.3412073490813655186, -0.6046776061558809534, -0.2411417322834644161 ) ) ;
#42088=CARTESIAN_POINT ( 'NONE',  ( -0.3018372703412066094, 0.009842519685039463617, 0.3409548833797002576 ) ) ;
#42090=CARTESIAN_POINT ( 'NONE',  ( -1.541994750656167090, 0.2952755905511811885, 0.1292274648535926551 ) ) ;
#42092=VERTEX_POINT ( 'NONE', #36250 ) ;
#42093=CARTESIAN_POINT ( 'NONE',  ( -0.7349081364829387342, -0.5023911411419708095, 0.1820866141732285504 ) ) ;
#42096=CARTESIAN_POINT ( 'NONE',  ( 0.9383202099737536495, -0.3162353388693405765, 0.4822834645669290543 ) ) ;
#42097=CARTESIAN_POINT ( 'NONE',  ( -0.2821522309711278487, 0.2952755905511811885, 0.1292274648535926551 ) ) ;
#42098=CARTESIAN_POINT ( 'NONE',  ( -1.141732283464566011, 0.2952755905511811885, 0.000000000000000000 ) ) ;
#42099=CARTESIAN_POINT ( 'NONE',  ( 1.161417322834646493, -0.5400638737290844871, 0.3530559997133364547 ) ) ;
#42100=CARTESIAN_POINT ( 'NONE',  ( -1.292650918635170010, 0.1771653543307087075, -0.09757992244046823083 ) ) ;
#42101=DIRECTION ( 'NONE',  ( -0.4043106043482690426, -0.6467352376403840974, -0.6467352376403910919 ) ) ;
#42102=CARTESIAN_POINT ( 'NONE',  ( 0.4921259842519691285, -0.5400638737290845981, -0.3530559997133363437 ) ) ;
#42103=CARTESIAN_POINT ( 'NONE',  ( -0.8464566929133852113, 0.1660481256975885056, 0.3530559997133364547 ) ) ;
#42105=CARTESIAN_POINT ( 'NONE',  ( -1.266404199475064773, -0.05778040916215560624, -0.4822834645669293319 ) ) ;
#42106=LINE ( 'NONE', #48831, #70808 ) ;
#42107=CARTESIAN_POINT ( 'NONE',  ( 0.9514435695538062676, -0.3162353388693409650, -0.4822834645669289433 ) ) ;
#42109=CARTESIAN_POINT ( 'NONE',  ( 1.456692913385827515, -0.5511811023622047445, 6.969142054262312111E-17 ) ) ;
#42110=ORIENTED_EDGE ( 'NONE', *, *, #39780, .F. ) ;
#42112=CARTESIAN_POINT ( 'NONE',  ( -0.2690288713910754526, -0.6692913385826771977, 0.1292274648535927661 ) ) ;
#42114=CARTESIAN_POINT ( 'NONE',  ( 0.3346456692913390985, 0.07958543189024085140, 0.2665933059059887866 ) ) ;
#42115=CARTESIAN_POINT ( 'NONE',  ( -1.482939632545930975, -0.4281496062992127816, -0.4176697321401328100 ) ) ;
#42116=CARTESIAN_POINT ( 'NONE',  ( 1.161417322834646271, 0.1660481256975883668, -0.3530559997133364547 ) ) ;
#42117=CARTESIAN_POINT ( 'NONE',  ( 0.8530183727034126306, 0.05413385826771626580, -0.4176697321401330321 ) ) ;
#42119=CARTESIAN_POINT ( 'NONE',  ( -0.07217847769028813698, -0.3162353388693409650, -0.4822834645669289433 ) ) ;
#42122=CARTESIAN_POINT ( 'NONE',  ( -0.7939632545931750718, -0.05778040916215560624, -0.4822834645669293319 ) ) ;
#42124=CARTESIAN_POINT ( 'NONE',  ( 1.607611548556431069, 0.1771653543307087630, 0.09757992244046791164 ) ) ;
#42125=CARTESIAN_POINT ( 'NONE',  ( -1.115485564304461219, 0.05413385826771626580, -0.4176697321401330321 ) ) ;
#42126=CARTESIAN_POINT ( 'NONE',  ( 1.443569553805774897, -0.6046776061558809534, -0.2411417322834644161 ) ) ;
#42128=CARTESIAN_POINT ( 'NONE',  ( -0.8727034120734901146, -0.05778040916215560624, -0.4822834645669293319 ) ) ;
#42130=CARTESIAN_POINT ( 'NONE',  ( 0.2887139107611556010, -0.6046776061558807314, 0.2411417322834647770 ) ) ;
#42132=CARTESIAN_POINT ( 'NONE',  ( -0.3543307086614165824, 0.2952755905511811885, 0.000000000000000000 ) ) ;
#42133=CARTESIAN_POINT ( 'NONE',  ( -1.463254593175852492, 0.1771653543307087630, 0.09757992244046791164 ) ) ;
#42134=CARTESIAN_POINT ( 'NONE',  ( 0.7545931758530189937, 0.1771653543307087075, -0.09757992244046823083 ) ) ;
#42135=CARTESIAN_POINT ( 'NONE',  ( 1.318897637795276356, 0.1660481256975883668, -0.3530559997133364547 ) ) ;
#42137=CARTESIAN_POINT ( 'NONE',  ( 0.6102362204724416372, 0.07958543189024071263, -0.2665933059059888421 ) ) ;
#42138=CARTESIAN_POINT ( 'NONE',  ( 1.010498687664042716, 0.05413385826771626580, -0.4176697321401330321 ) ) ;
#42140=CARTESIAN_POINT ( 'NONE',  ( -0.5643044619422565855, 0.05413385826771626580, -0.4176697321401330321 ) ) ;
#42142=CARTESIAN_POINT ( 'NONE',  ( 1.555118110236221041, -0.4536011799217367080, 0.2665933059059888421 ) ) ;
#42143=CARTESIAN_POINT ( 'NONE',  ( -0.7217847769028863381, 0.05413385826771626580, -0.4176697321401330321 ) ) ;
#42145=CARTESIAN_POINT ( 'NONE',  ( 1.299212598425197429, -0.6692913385826771977, 8.415575281601705876E-17 ) ) ;
#42146=CARTESIAN_POINT ( 'NONE',  ( 0.2230971128608929543, 0.05413385826771626580, -0.4176697321401330321 ) ) ;
#42147=CARTESIAN_POINT ( 'NONE',  ( 0.3543307086614181922, -0.5511811023622047445, 6.969142054262312111E-17 ) ) ;
#42149=CARTESIAN_POINT ( 'NONE',  ( -0.1377952755905504645, -0.4536011799217368745, -0.2665933059059886201 ) ) ;
#42150=CARTESIAN_POINT ( 'NONE',  ( 0.9055118110236227702, -0.5511811023622047445, 6.969142054262312111E-17 ) ) ;
#42153=CARTESIAN_POINT ( 'NONE',  ( 0.7480314960629927956, 0.2952755905511811885, 0.000000000000000000 ) ) ;
#42155=CARTESIAN_POINT ( 'NONE',  ( 1.469816272965879911, -0.5023911411419708095, 0.1820866141732285504 ) ) ;
#42157=CARTESIAN_POINT ( 'NONE',  ( -0.1246719160104980823, 0.1771653543307087630, 0.09757992244046791164 ) ) ;
#42159=CARTESIAN_POINT ( 'NONE',  ( 0.2952755905511819101, 0.1660481256975883668, -0.3530559997133364547 ) ) ;
#42160=CARTESIAN_POINT ( 'NONE',  ( 1.443569553805774897, -0.5023911411419708095, -0.1820866141732282451 ) ) ;
#42161=CARTESIAN_POINT ( 'NONE',  ( -1.476377952755905110, -0.4536011799217368745, -0.2665933059059886201 ) ) ;
#42162=CARTESIAN_POINT ( 'NONE',  ( -1.384514435695537005, 0.2952755905511811885, 0.1292274648535926551 ) ) ;
#42164=CARTESIAN_POINT ( 'NONE',  ( 0.2034120734908144990, -0.6692913385826771977, 0.1292274648535927661 ) ) ;
#42165=CARTESIAN_POINT ( 'NONE',  ( 1.043307086614173818, 0.1660481256975885056, 0.3530559997133364547 ) ) ;
#42167=CARTESIAN_POINT ( 'NONE',  ( -0.05249343832020938322, -0.6046776061558809534, -0.2411417322834644161 ) ) ;
#42168=CARTESIAN_POINT ( 'NONE',  ( 1.115485564304462551, -0.4281496062992127816, -0.4176697321401328100 ) ) ;
#42169=CARTESIAN_POINT ( 'NONE',  ( 0.8267716535433078384, -0.6692913385826771977, 8.415575281601705876E-17 ) ) ;
#42171=CARTESIAN_POINT ( 'NONE',  ( 0.6167979002624679463, -0.004921259842519870586, -0.3153832671262229437 ) ) ;
#42172=CARTESIAN_POINT ( 'NONE',  ( 1.620734908136483465, -0.6692913385826771977, 0.1292274648535927661 ) ) ;
#42173=CARTESIAN_POINT ( 'NONE',  ( -0.03937007874015669567, -0.5511811023622047445, 6.969142054262312111E-17 ) ) ;
#42175=CARTESIAN_POINT ( 'NONE',  ( -0.05905511811023545637, 0.1660481256975885056, 0.3530559997133364547 ) ) ;
#42176=CARTESIAN_POINT ( 'NONE',  ( 0.8333333333333340365, 0.2952755905511810774, -0.1292274648535930714 ) ) ;
#42177=CARTESIAN_POINT ( 'NONE',  ( -0.1771653543307080136, 0.1660481256975883668, -0.3530559997133364547 ) ) ;
#42178=CARTESIAN_POINT ( 'NONE',  ( -0.2034120734908131112, -0.5511811023622048555, -0.09757992244046775898 ) ) ;
#42179=CARTESIAN_POINT ( 'NONE',  ( 1.003937007874016185, 0.1660481256975883668, -0.3530559997133364547 ) ) ;
#42180=CARTESIAN_POINT ( 'NONE',  ( 0.7545931758530189937, 0.1771653543307087075, -0.09757992244046823083 ) ) ;
#42181=CARTESIAN_POINT ( 'NONE',  ( 0.4606732211678742361, 1.778019097314512686, 0.5309055118110234117 ) ) ;
#42185=CARTESIAN_POINT ( 'NONE',  ( -1.148293963254592542, 0.2952755905511811885, 0.1292274648535926551 ) ) ;
#42186=CARTESIAN_POINT ( 'NONE',  ( -0.4461942257217840213, 0.2306618581243848609, 0.2411417322834645549 ) ) ;
#42190=CARTESIAN_POINT ( 'NONE',  ( 0.8661417322834653598, -0.1870078740157479769, 0.3641732283464567677 ) ) ;
#42192=CARTESIAN_POINT ( 'NONE',  ( 1.187664041994751285, -0.3162353388693409650, -0.4822834645669289433 ) ) ;
#42195=CARTESIAN_POINT ( 'NONE',  ( -1.371391076115484831, 0.1771653543307087075, -0.09757992244046823083 ) ) ;
#42196=CARTESIAN_POINT ( 'NONE',  ( -2.795275590551184131, 1.023622047244095556, -2.654250759839014936E-16 ) ) ;
#42197=CARTESIAN_POINT ( 'NONE',  ( 1.338582677165355062, -0.1870078740157480601, -0.3641732283464567677 ) ) ;
#42198=CARTESIAN_POINT ( 'NONE',  ( 0.2427821522309719648, -0.05778040916215522460, 0.4822834645669289988 ) ) ;
#42200=CARTESIAN_POINT ( 'NONE',  ( 0.1640419947506569498, -0.3162353388693409650, -0.4822834645669289433 ) ) ;
#42201=CARTESIAN_POINT ( 'NONE',  ( -0.8989501312335946848, 0.1771653543307087075, -0.09757992244046823083 ) ) ;
#42202=CARTESIAN_POINT ( 'NONE',  ( 0.6167979002624678353, -0.4281496062992124485, 0.4176697321401328655 ) ) ;
#42204=CARTESIAN_POINT ( 'NONE',  ( -0.2493438320209966919, 0.05413385826771626580, -0.4176697321401330321 ) ) ;
#42205=CARTESIAN_POINT ( 'NONE',  ( 0.5411721830064198935, 8.471767977567108961E-16, -0.4445507791589058955 ) ) ;
#42208=CARTESIAN_POINT ( 'NONE',  ( 0.8858267716535438430, 0.1660481256975885056, 0.3530559997133364547 ) ) ;
#42209=CARTESIAN_POINT ( 'NONE',  ( -0.1574803149606292529, -0.1870078740157479769, 0.4822834645669291653 ) ) ;
#42210=CARTESIAN_POINT ( 'NONE',  ( -1.108923884514435132, -0.05778040916215560624, -0.4822834645669293319 ) ) ;
#42211=CARTESIAN_POINT ( 'NONE',  ( 1.272965879265092637, 0.05413385826771666132, 0.4176697321401328100 ) ) ;
#42212=CARTESIAN_POINT ( 'NONE',  ( 0.3346456692913393205, -0.5400638737290845981, -0.3530559997133363437 ) ) ;
#42214=CARTESIAN_POINT ( 'NONE',  ( -0.5380577427821514602, -0.4281496062992127816, -0.4176697321401328100 ) ) ;
#42215=CARTESIAN_POINT ( 'NONE',  ( 0.2755905511811031494, 0.2952755905511811885, 0.000000000000000000 ) ) ;
#42216=CARTESIAN_POINT ( 'NONE',  ( -0.3608923884514428360, 0.2952755905511811885, 0.1292274648535926551 ) ) ;
#42218=CARTESIAN_POINT ( 'NONE',  ( 0.8464566929133866546, -0.4536011799217367080, 0.2665933059059888421 ) ) ;
#42219=CARTESIAN_POINT ( 'NONE',  ( -1.712598425196849572, 0.1660481256975885056, 0.3530559997133364547 ) ) ;
#42220=CARTESIAN_POINT ( 'NONE',  ( 0.4855643044619428750, 0.05413385826771666132, 0.4176697321401328100 ) ) ;
#42221=SURFACE_STYLE_FILL_AREA ( #36326 ) ;
#42223=ORIENTED_EDGE ( 'NONE', *, *, #56444, .F. ) ;
#42225=CARTESIAN_POINT ( 'NONE',  ( 0.8727034120734913358, -0.05778040916215522460, 0.4822834645669289988 ) ) ;
#42226=CARTESIAN_POINT ( 'NONE',  ( 0.6036745406824153282, -0.5023911411419708095, 0.1820866141732285504 ) ) ;
#42227=CARTESIAN_POINT ( 'NONE',  ( 0.9552210167251751205, -9.595573933774993207E-16, 0.4281989832122458095 ) ) ;
#42228=DIRECTION ( 'NONE',  ( 0.000000000000000000, 0.000000000000000000, -1.000000000000000000 ) ) ;
#42233=CARTESIAN_POINT ( 'NONE',  ( 0.8070866141732288002, 0.1660481256975885056, 0.3530559997133364547 ) ) ;
#42234=CARTESIAN_POINT ( 'NONE',  ( -0.8267716535433065062, 0.2952755905511811885, 0.000000000000000000 ) ) ;
#42235=CARTESIAN_POINT ( 'NONE',  ( -0.6299212598425188991, -0.1870078740157479769, 0.4822834645669291653 ) ) ;
#42236=CARTESIAN_POINT ( 'NONE',  ( 0.6692913385826777528, 0.2952755905511811885, 0.000000000000000000 ) ) ;
#42237=CARTESIAN_POINT ( 'NONE',  ( 1.410761154855643795, -0.3162353388693405765, 0.4822834645669290543 ) ) ;
#42239=CARTESIAN_POINT ( 'NONE',  ( 1.404199475065617708, -0.004921259842519870586, -0.3153832671262229437 ) ) ;
#42240=LINE ( 'NONE', #47724, #37157 ) ;
#42241=CARTESIAN_POINT ( 'NONE',  ( -1.318897637795274802, 0.07958543189024085140, 0.2665933059059887866 ) ) ;
#42243=CARTESIAN_POINT ( 'NONE',  ( -0.02624671916010428221, 0.2306618581243847221, -0.2411417322834647770 ) ) ;
#42244=CARTESIAN_POINT ( 'NONE',  ( 1.220472440944882608, 0.2952755905511811885, 0.000000000000000000 ) ) ;
#42245=DIRECTION ( 'NONE',  ( 0.000000000000000000, 1.000000000000000000, 0.000000000000000000 ) ) ;
#42246=CARTESIAN_POINT ( 'NONE',  ( -1.351706036745406347, -0.004921259842519870586, -0.3153832671262229437 ) ) ;
#42247=CARTESIAN_POINT ( 'NONE',  ( 0.4790026246719168435, -0.3162353388693409650, -0.4822834645669289433 ) ) ;
#42248=CARTESIAN_POINT ( 'NONE',  ( 1.305774278215223960, 0.1771653543307087075, -0.09757992244046823083 ) ) ;
#42250=CARTESIAN_POINT ( 'NONE',  ( -1.233595800524933894, 0.1283753931104748280, 0.1820866141732283561 ) ) ;
#42251=CARTESIAN_POINT ( 'NONE',  ( 1.200787401574803681, 0.1660481256975885056, 0.3530559997133364547 ) ) ;
#42253=CARTESIAN_POINT ( 'NONE',  ( -0.3740157480314953431, -0.5400638737290845981, -0.3530559997133363437 ) ) ;
#42254=CARTESIAN_POINT ( 'NONE',  ( -1.528871391076114250, -0.5511811023622046335, 0.09757992244046803654 ) ) ;
#42255=CARTESIAN_POINT ( 'NONE',  ( -0.8070866141732276899, -0.5400638737290844871, 0.3530559997133364547 ) ) ;
#42256=CARTESIAN_POINT ( 'NONE',  ( -1.364829396325458521, -0.5023911411419708095, 0.1820866141732285504 ) ) ;
#42258=CARTESIAN_POINT ( 'NONE',  ( 0.3280839895013130669, 0.05413385826771666132, 0.4176697321401328100 ) ) ;
#42260=CARTESIAN_POINT ( 'NONE',  ( 1.482939632545932307, 0.05413385826771626580, -0.4176697321401330321 ) ) ;
#42262=CARTESIAN_POINT ( 'NONE',  ( -1.049868766404198794, 0.2306618581243847221, -0.2411417322834647770 ) ) ;
#42263=CARTESIAN_POINT ( 'NONE',  ( -0.5249343832020990641, -0.5023911411419708095, -0.1820866141732282451 ) ) ;
#42264=CARTESIAN_POINT ( 'NONE',  ( -0.4986876640419939388, 0.1539470093639521697, -0.1968503937007875793 ) ) ;
#42265=CARTESIAN_POINT ( 'NONE',  ( 0.1377952755905518800, 0.1660481256975883668, -0.3530559997133364547 ) ) ;
#42266=CARTESIAN_POINT ( 'NONE',  ( 0.2034120734908144990, -0.5511811023622046335, 0.09757992244046803654 ) ) ;
#42267=CARTESIAN_POINT ( 'NONE',  ( -1.128608923884513837, -0.5023911411419708095, 0.1820866141732285504 ) ) ;
#42268=CARTESIAN_POINT ( 'NONE',  ( -1.522309711286088607, 0.2306618581243847221, -0.2411417322834647770 ) ) ;
#42269=CARTESIAN_POINT ( 'NONE',  ( 1.200787401574803681, -0.4536011799217368745, -0.2665933059059886201 ) ) ;
#42270=CARTESIAN_POINT ( 'NONE',  ( 1.528871391076116026, 0.2952755905511811885, 0.1292274648535926551 ) ) ;
#42271=CARTESIAN_POINT ( 'NONE',  ( -0.2262115530851587786, -2.191421614605370878E-15, 0.4445507791589071167 ) ) ;
#42272=CARTESIAN_POINT ( 'NONE',  ( 0.3215223097112867578, -0.2845877964562161244, -0.3641732283464567121 ) ) ;
#42273=CARTESIAN_POINT ( 'NONE',  ( 1.017060367454068803, -0.3162353388693405765, 0.4822834645669290543 ) ) ;
#42274=CARTESIAN_POINT ( 'NONE',  ( 0.1474713956048451791, 8.471767977567108961E-16, -0.4445507791589058955 ) ) ;
#42275=CARTESIAN_POINT ( 'NONE',  ( 1.010498687664042716, -0.004921259842519870586, -0.3153832671262229437 ) ) ;
#42277=CARTESIAN_POINT ( 'NONE',  ( -1.161417322834644716, 0.1660481256975885056, 0.3530559997133364547 ) ) ;
#42278=CARTESIAN_POINT ( 'NONE',  ( -0.9251968503937002541, -0.5400638737290845981, -0.3530559997133363437 ) ) ;
#42279=CARTESIAN_POINT ( 'NONE',  ( 0.1706036745406830368, 0.05413385826771666132, 0.4176697321401328100 ) ) ;
#42280=CARTESIAN_POINT ( 'NONE',  ( 0.5404819259526921771, 1.809133623825372073E-16, -0.4118484887281974038 ) ) ;
#42282=CARTESIAN_POINT ( 'NONE',  ( 0.7939632545931766261, -0.05778040916215522460, 0.4822834645669289988 ) ) ;
#42283=CARTESIAN_POINT ( 'NONE',  ( -1.712598425196849572, 0.1660481256975885056, 0.3530559997133364547 ) ) ;
#42284=CARTESIAN_POINT ( 'NONE',  ( -0.01312335958005186876, 0.05413385826771626580, -0.4176697321401330321 ) ) ;
#42285=CARTESIAN_POINT ( 'NONE',  ( 0.8136482939632553313, 0.2306618581243848609, 0.2411417322834645549 ) ) ;
#42292=CARTESIAN_POINT ( 'NONE',  ( -0.2296587926509179312, -0.2845877964562161244, -0.3641732283464567121 ) ) ;
#42293=CARTESIAN_POINT ( 'NONE',  ( -0.7349081364829390672, 0.2306618581243847221, -0.2411417322834647770 ) ) ;
#42294=CARTESIAN_POINT ( 'NONE',  ( 0.7480314960629927956, -0.6692913385826771977, 8.415575281601705876E-17 ) ) ;
#42296=CARTESIAN_POINT ( 'NONE',  ( 0.1312335958005257930, 0.1283753931104746893, -0.1820866141732285504 ) ) ;
#42297=CARTESIAN_POINT ( 'NONE',  ( -1.338582677165353729, -0.1870078740157479769, 0.4822834645669291653 ) ) ;
#42298=CARTESIAN_POINT ( 'NONE',  ( 1.187664041994751285, -0.3162353388693409650, -0.4822834645669289433 ) ) ;
#42301=CARTESIAN_POINT ( 'NONE',  ( -0.7426113562972000981, 2.793565526369265584, 0.5309055118110235227 ) ) ;
#42302=ORIENTED_EDGE ( 'NONE', *, *, #45132, .F. ) ;
#42303=CARTESIAN_POINT ( 'NONE',  ( 1.167979002624672580, 0.05413385826771626580, -0.4176697321401330321 ) ) ;
#42304=CARTESIAN_POINT ( 'NONE',  ( 1.207349081364829990, -0.5023911411419708095, -0.1820866141732282451 ) ) ;
#42305=CARTESIAN_POINT ( 'NONE',  ( -1.515748031496062076, -0.4536011799217367080, 0.2665933059059888421 ) ) ;
#42306=CARTESIAN_POINT ( 'NONE',  ( -1.653543307086613234, -0.1870078740157479769, 0.4822834645669291653 ) ) ;
#42308=CARTESIAN_POINT ( 'NONE',  ( 1.192200019340703188, 4.598214627222820490E-16, 0.3954985857520057491 ) ) ;
#42309=CARTESIAN_POINT ( 'NONE',  ( 1.377952755905512472, 0.2952755905511811885, 0.000000000000000000 ) ) ;
#42310=CARTESIAN_POINT ( 'NONE',  ( -1.706036745406823485, 0.2306618581243848609, 0.2411417322834645549 ) ) ;
#42311=CARTESIAN_POINT ( 'NONE',  ( -0.4199475065616791736, 0.2306618581243847221, -0.2411417322834647770 ) ) ;
#42312=CARTESIAN_POINT ( 'NONE',  ( -0.7217847769028863381, 0.05413385826771626580, -0.4176697321401330321 ) ) ;
#42313=CARTESIAN_POINT ( 'NONE',  ( 1.574803149606299746, -0.1870078740157479769, 0.4822834645669291653 ) ) ;
#42315=CARTESIAN_POINT ( 'NONE',  ( 0.07874015748031558404, -0.1870078740157480879, -0.4822834645669291653 ) ) ;
#42317=CARTESIAN_POINT ( 'NONE',  ( -1.620734908136482577, 0.1771653543307087630, 0.09757992244046791164 ) ) ;
#42318=VERTEX_POINT ( 'NONE', #29924 ) ;
#42322=CARTESIAN_POINT ( 'NONE',  ( -1.706036745406823485, 0.2306618581243848609, 0.2411417322834645549 ) ) ;
#42324=CARTESIAN_POINT ( 'NONE',  ( 1.653543307086614789, -0.1870078740157479769, 0.3641732283464567677 ) ) ;
#42327=CARTESIAN_POINT ( 'NONE',  ( -0.6199123404867337150, -2.191421614605370878E-15, 0.4445507791589071167 ) ) ;
#42329=CARTESIAN_POINT ( 'NONE',  ( -0.5183727034120726440, 0.1771653543307087630, 0.09757992244046791164 ) ) ;
#42330=CARTESIAN_POINT ( 'NONE',  ( -1.043307086614172707, 0.07958543189024071263, -0.2665933059059888421 ) ) ;
#42332=CARTESIAN_POINT ( 'NONE',  ( -1.469816272965878357, 0.2306618581243848609, 0.2411417322834645549 ) ) ;
#42333=CARTESIAN_POINT ( 'NONE',  ( 0.6430446194225728496, 0.05413385826771666132, 0.4176697321401328100 ) ) ;
#42334=CARTESIAN_POINT ( 'NONE',  ( -1.305774278215222184, 0.2952755905511811885, 0.1292274648535926551 ) ) ;
#42338=CARTESIAN_POINT ( 'NONE',  ( -1.443569553805773564, 0.2306618581243847221, -0.2411417322834647770 ) ) ;
#42344=CARTESIAN_POINT ( 'NONE',  ( -0.5708661417322825615, -0.5400638737290844871, 0.3530559997133364547 ) ) ;
#42345=CARTESIAN_POINT ( 'NONE',  ( 1.614173228346457378, -0.6692913385826771977, 8.415575281601705876E-17 ) ) ;
#42347=PLANE ( 'NONE',  #37153 ) ;
#42348=CARTESIAN_POINT ( 'NONE',  ( 1.601049868766404982, -0.6046776061558809534, -0.2411417322834644161 ) ) ;
#42349=CARTESIAN_POINT ( 'NONE',  ( -0.8464566929133852113, -0.5400638737290845981, -0.3530559997133363437 ) ) ;
#42351=CARTESIAN_POINT ( 'NONE',  ( -0.006561679790025524116, -0.2845877964562159024, 0.3641732283464567677 ) ) ;
#42353=CARTESIAN_POINT ( 'NONE',  ( -0.1181102362204717315, -0.5511811023622047445, 6.969142054262312111E-17 ) ) ;
#42354=CARTESIAN_POINT ( 'NONE',  ( 0.7808398950131240079, -0.2845877964562159024, 0.3641732283464567677 ) ) ;
#42355=CARTESIAN_POINT ( 'NONE',  ( 0.5839895013123367340, -0.6692913385826773087, -0.1292274648535924053 ) ) ;
#42356=CARTESIAN_POINT ( 'NONE',  ( -0.1902887139107604098, 0.1771653543307087075, -0.09757992244046823083 ) ) ;
#42358=CARTESIAN_POINT ( 'NONE',  ( -1.653543307086613234, -0.1870078740157479769, 0.4822834645669291653 ) ) ;
#42359=EDGE_CURVE ( 'NONE', #46767, #36200, #36137, .T. ) ;
#42360=CARTESIAN_POINT ( 'NONE',  ( -1.043307086614172041, -0.5400638737290844871, 0.3530559997133364547 ) ) ;
#42362=CARTESIAN_POINT ( 'NONE',  ( -0.05905511811023545637, -0.5400638737290845981, -0.3530559997133363437 ) ) ;
#42363=EDGE_CURVE ( 'NONE', #20676, #69946, #31196, .T. ) ;
#42364=CARTESIAN_POINT ( 'NONE',  ( -0.3937007874015740483, -0.1870078740157479769, 0.4822834645669291653 ) ) ;
#42366=CARTESIAN_POINT ( 'NONE',  ( 0.1377952755905518800, -0.4536011799217367080, 0.2665933059059888421 ) ) ;
#42367=CARTESIAN_POINT ( 'NONE',  ( -0.3346456692913377662, -0.5400638737290844871, 0.3530559997133364547 ) ) ;
#42368=CARTESIAN_POINT ( 'NONE',  ( -0.5446194225721777693, -0.05778040916215522460, 0.4822834645669289988 ) ) ;
#42369=DIRECTION ( 'NONE',  ( -0.7071067811865461294, -0.000000000000000000, -0.7071067811865490160 ) ) ;
#42370=CARTESIAN_POINT ( 'NONE',  ( 1.620734908136483465, -0.5511811023622046335, 0.09757992244046803654 ) ) ;
#42371=CARTESIAN_POINT ( 'NONE',  ( 0.3215223097112867578, -0.3162353388693409650, -0.4822834645669289433 ) ) ;
#42372=VERTEX_POINT ( 'NONE', #26927 ) ;
#42375=CARTESIAN_POINT ( 'NONE',  ( -0.7808398950131225646, -0.08942795157527998196, 0.3641732283464567121 ) ) ;
#42376=CARTESIAN_POINT ( 'NONE',  ( -0.4921259842519677963, -0.5400638737290844871, 0.3530559997133364547 ) ) ;
#42377=CARTESIAN_POINT ( 'NONE',  ( 1.587926509186352586, -0.4281496062992127816, -0.4176697321401328100 ) ) ;
#42378=CARTESIAN_POINT ( 'NONE',  ( 1.535433070866142558, 0.2952755905511811885, 0.000000000000000000 ) ) ;
#42380=CARTESIAN_POINT ( 'NONE',  ( -1.305774278215222184, -0.5511811023622048555, -0.09757992244046775898 ) ) ;
#42384=PLANE ( 'NONE',  #39114 ) ;
#42385=CARTESIAN_POINT ( 'NONE',  ( 1.082677165354331228, -0.4536011799217367080, 0.2665933059059888421 ) ) ;
#42386=CARTESIAN_POINT ( 'NONE',  ( 1.030183727034121421, -0.3162353388693409650, -0.4822834645669289433 ) ) ;
#42388=CARTESIAN_POINT ( 'NONE',  ( 0.7217847769028878924, -0.4281496062992127816, -0.4176697321401328100 ) ) ;
#42390=CARTESIAN_POINT ( 'NONE',  ( 1.351706036745407680, -0.004921259842519576551, 0.3153832671262227771 ) ) ;
#42391=CARTESIAN_POINT ( 'NONE',  ( 0.1443569553805781891, 0.05413385826771626580, -0.4176697321401330321 ) ) ;
#42392=CARTESIAN_POINT ( 'NONE',  ( -0.8727034120734901146, -0.3162353388693405765, 0.4822834645669290543 ) ) ;
#42393=CARTESIAN_POINT ( 'NONE',  ( 1.469816272965879911, -0.6046776061558807314, 0.2411417322834647770 ) ) ;
#42396=CIRCLE ( 'NONE', #66637, 1.220472440944881942 ) ;
#42397=CARTESIAN_POINT ( 'NONE',  ( 0.5446194225721792126, -0.08942795157528024563, -0.3641732283464568787 ) ) ;
#42401=CARTESIAN_POINT ( 'NONE',  ( -0.9055118110236215490, 0.2952755905511811885, 0.000000000000000000 ) ) ;
#42402=CARTESIAN_POINT ( 'NONE',  ( 0.006561679790026889343, -0.3162353388693409650, -0.4822834645669289433 ) ) ;
#42403=CARTESIAN_POINT ( 'NONE',  ( -0.4855643044619415427, 0.05413385826771626580, -0.4176697321401330321 ) ) ;
#42404=CARTESIAN_POINT ( 'NONE',  ( 0.9973753280839902091, -0.6046776061558807314, 0.2411417322834647770 ) ) ;
#42405=CARTESIAN_POINT ( 'NONE',  ( -1.272965879265091305, 0.05413385826771626580, -0.4176697321401330321 ) ) ;
#42406=CARTESIAN_POINT ( 'NONE',  ( -0.3149606299212590610, -0.1870078740157479769, 0.4822834645669291653 ) ) ;
#42407=CARTESIAN_POINT ( 'NONE',  ( 1.148293963254593653, 0.2952755905511810774, -0.1292274648535930714 ) ) ;
#42408=CARTESIAN_POINT ( 'NONE',  ( 0.4986876640419954376, 0.2306618581243848609, 0.2411417322834645549 ) ) ;
#42410=CARTESIAN_POINT ( 'NONE',  ( 0.6627296587926517768, -0.6692913385826773087, -0.1292274648535924053 ) ) ;
#42412=CARTESIAN_POINT ( 'NONE',  ( -0.5971128608923877978, -0.5511811023622048555, -0.09757992244046775898 ) ) ;
#42416=CARTESIAN_POINT ( 'NONE',  ( -0.7020997375328076329, -0.2845877964562161244, -0.3641732283464567121 ) ) ;
#42417=CARTESIAN_POINT ( 'NONE',  ( -0.5774278215223089816, -0.6046776061558807314, 0.2411417322834647770 ) ) ;
#42419=CARTESIAN_POINT ( 'NONE',  ( -0.8595800524934373854, -0.3162353388693409650, -0.4822834645669289433 ) ) ;
#42420=CARTESIAN_POINT ( 'NONE',  ( -0.7742782152230965886, 0.05413385826771666132, 0.4176697321401328100 ) ) ;
#42421=CARTESIAN_POINT ( 'NONE',  ( -1.161417322834644716, 0.1660481256975885056, 0.3530559997133364547 ) ) ;
#42422=CARTESIAN_POINT ( 'NONE',  ( -1.463254593175852492, -0.6692913385826773087, -0.1292274648535924053 ) ) ;
#42423=CARTESIAN_POINT ( 'NONE',  ( 1.148293963254593875, -0.5511811023622046335, 0.09757992244046803654 ) ) ;
#42426=CARTESIAN_POINT ( 'NONE',  ( -0.01968503937007793844, -0.4536011799217367080, 0.2665933059059888421 ) ) ;
#42427=CARTESIAN_POINT ( 'NONE',  ( 0.05249343832021075018, -0.6046776061558807314, 0.2411417322834647770 ) ) ;
#42428=CARTESIAN_POINT ( 'NONE',  ( -0.2296587926509179312, -0.05778040916215522460, 0.4822834645669289988 ) ) ;
#42434=CARTESIAN_POINT ( 'NONE',  ( 1.581364829396326277, -0.05778040916215522460, 0.4822834645669289988 ) ) ;
#42435=CARTESIAN_POINT ( 'NONE',  ( -0.8727034120734901146, -0.08942795157528024563, -0.3641732283464568787 ) ) ;
#42436=CARTESIAN_POINT ( 'NONE',  ( -1.076115485564303809, 0.2306618581243848609, 0.2411417322834645549 ) ) ;
#42438=CARTESIAN_POINT ( 'NONE',  ( 0.6983222978630806432, 4.257495641787552160E-16, -0.4281993546915526805 ) ) ;
#42440=CARTESIAN_POINT ( 'NONE',  ( 1.646981627296588035, -0.3162353388693405765, 0.4822834645669290543 ) ) ;
#42441=CARTESIAN_POINT ( 'NONE',  ( 0.4133858267716541968, -0.5400638737290845981, -0.3530559997133363437 ) ) ;
#42442=CARTESIAN_POINT ( 'NONE',  ( 0.4593175853018380828, 0.05413385826771626580, -0.4176697321401330321 ) ) ;
#42443=CARTESIAN_POINT ( 'NONE',  ( -0.8005249343832011588, -0.004921259842519870586, -0.3153832671262229437 ) ) ;
#42445=CARTESIAN_POINT ( 'NONE',  ( -0.08530183727034056085, -0.05778040916215560624, -0.4822834645669293319 ) ) ;
#42447=CARTESIAN_POINT ( 'NONE',  ( -0.5971128608923877978, 0.2952755905511811885, 0.1292274648535926551 ) ) ;
#42449=CARTESIAN_POINT ( 'NONE',  ( 1.246719160104987623, -0.3690944881889763329, 0.3153832671262228327 ) ) ;
#42450=CARTESIAN_POINT ( 'NONE',  ( 0.2559055118110243332, -0.4536011799217368745, -0.2665933059059886201 ) ) ;
#42451=CARTESIAN_POINT ( 'NONE',  ( 0.9973753280839902091, -0.5023911411419708095, 0.1820866141732285504 ) ) ;
#42452=CARTESIAN_POINT ( 'NONE',  ( -1.233595800524933894, 0.2306618581243848609, 0.2411417322834645549 ) ) ;
#42453=CARTESIAN_POINT ( 'NONE',  ( -1.351706036745406347, -0.3690944881889763329, 0.3153832671262228327 ) ) ;
#42455=CARTESIAN_POINT ( 'NONE',  ( -1.102362204724408601, -0.1870078740157479769, 0.4822834645669291653 ) ) ;
#42456=CARTESIAN_POINT ( 'NONE',  ( -0.6102362204724400829, -0.5400638737290845981, -0.3530559997133363437 ) ) ;
#42457=CARTESIAN_POINT ( 'NONE',  ( 0.5118110236220480003, -0.6692913385826771977, 8.415575281601705876E-17 ) ) ;
#42461=CARTESIAN_POINT ( 'NONE',  ( 0.2165354330708668673, -0.4536011799217367080, 0.2665933059059888421 ) ) ;
#42462=CARTESIAN_POINT ( 'NONE',  ( -1.555118110236219930, 0.07958543189024085140, 0.2665933059059887866 ) ) ;
#42463=CARTESIAN_POINT ( 'NONE',  ( 0.8792650918635177559, 0.05413385826771666132, 0.4176697321401328100 ) ) ;
#42465=CARTESIAN_POINT ( 'NONE',  ( 1.299212598425197429, 0.1771653543307087630, 0.000000000000000000 ) ) ;
#42466=CARTESIAN_POINT ( 'NONE',  ( -0.9842519685039365918, -0.6692913385826771977, 8.415575281601705876E-17 ) ) ;
#42467=CARTESIAN_POINT ( 'NONE',  ( -0.1968503937007867743, 0.1771653543307087630, 0.000000000000000000 ) ) ;
#42468=LINE ( 'NONE', #36164, #81173 ) ;
#42469=CARTESIAN_POINT ( 'NONE',  ( 0.5446194225721792126, -0.08942795157528024563, -0.3641732283464568787 ) ) ;
#42470=CARTESIAN_POINT ( 'NONE',  ( -0.2034120734908128059, 0.2952755905511811885, 0.1292274648535926551 ) ) ;
#42473=CARTESIAN_POINT ( 'NONE',  ( 1.049868766404200127, -0.5023911411419708095, -0.1820866141732282451 ) ) ;
#42474=CARTESIAN_POINT ( 'NONE',  ( 0.01968503937007957949, -0.5400638737290845981, -0.3530559997133363437 ) ) ;
#42475=CARTESIAN_POINT ( 'NONE',  ( -0.3280839895013117347, 0.05413385826771626580, -0.4176697321401330321 ) ) ;
#42476=CARTESIAN_POINT ( 'NONE',  ( -0.3608923884514428360, 0.1771653543307087630, 0.09757992244046791164 ) ) ;
#42478=CARTESIAN_POINT ( 'NONE',  ( -0.4986876640419939388, 0.1283753931104746893, -0.1820866141732285504 ) ) ;
#42479=CARTESIAN_POINT ( 'NONE',  ( 0.4724409448818904789, -0.1870078740157480879, -0.4822834645669291653 ) ) ;
#42481=CARTESIAN_POINT ( 'NONE',  ( -0.9645669291338575535, -0.4536011799217367080, 0.2665933059059888421 ) ) ;
#42483=CARTESIAN_POINT ( 'NONE',  ( -1.548556430446193399, -0.6046776061558809534, -0.2411417322834644161 ) ) ;
#42486=EDGE_CURVE ( 'NONE', #9936, #6582, #143, .T. ) ;
#42487=CARTESIAN_POINT ( 'NONE',  ( -1.476377952755905110, -0.4536011799217368745, -0.2665933059059886201 ) ) ;
#42488=CARTESIAN_POINT ( 'NONE',  ( -0.5052493438320203589, -0.6692913385826771977, 0.1292274648535927661 ) ) ;
#42489=CARTESIAN_POINT ( 'NONE',  ( -1.318897637795274802, 0.1660481256975885056, 0.3530559997133364547 ) ) ;
#42492=CARTESIAN_POINT ( 'NONE',  ( 1.259842519685040019, -0.1870078740157480879, -0.4822834645669291653 ) ) ;
#42493=CARTESIAN_POINT ( 'NONE',  ( 0.6430446194225729606, -0.4281496062992127816, -0.4176697321401328100 ) ) ;
#42499=CARTESIAN_POINT ( 'NONE',  ( -1.673228346456691717, 0.1660481256975883668, -0.3530559997133364547 ) ) ;
#42502=CARTESIAN_POINT ( 'NONE',  ( -0.9448818897637790704, -0.1870078740157480601, -0.3641732283464567677 ) ) ;
#42504=ORIENTED_EDGE ( 'NONE', *, *, #28103, .F. ) ;
#42505=CARTESIAN_POINT ( 'NONE',  ( 0.6561679790026253567, 0.2306618581243848609, 0.2411417322834645549 ) ) ;
#42506=CARTESIAN_POINT ( 'NONE',  ( -0.3871391076115479057, -0.3162353388693409650, -0.4822834645669289433 ) ) ;
#42507=CARTESIAN_POINT ( 'NONE',  ( -1.187664041994749731, -0.3162353388693405765, 0.4822834645669290543 ) ) ;
#42508=CARTESIAN_POINT ( 'NONE',  ( 1.023622047244095334, -0.1870078740157479769, 0.4822834645669291653 ) ) ;
#42509=CARTESIAN_POINT ( 'NONE',  ( -1.200787401574802349, -0.4536011799217367080, 0.2665933059059888421 ) ) ;
#42511=CARTESIAN_POINT ( 'NONE',  ( 0.4724409448818904789, -0.1870078740157480879, -0.4822834645669291653 ) ) ;
#42512=CARTESIAN_POINT ( 'NONE',  ( -0.8923884514435688198, -0.6046776061558807314, 0.2411417322834647770 ) ) ;
#42514=CARTESIAN_POINT ( 'NONE',  ( 1.541994750656168645, -0.6692913385826771977, 0.1292274648535927661 ) ) ;
#42515=FACE_OUTER_BOUND ( 'NONE', #73681, .T. ) ;
#42516=( BOUNDED_CURVE ( )  B_SPLINE_CURVE ( 1, ( #72168, #77230 ),
 .UNSPECIFIED., .F., .F. ) 
 B_SPLINE_CURVE_WITH_KNOTS ( ( 2, 2 ),
 ( 5.204170427930421283E-18, 0.002000000000000006981 ),
 .UNSPECIFIED. ) 
 CURVE ( )  GEOMETRIC_REPRESENTATION_ITEM ( )  RATIONAL_B_SPLINE_CURVE ( ( 0.9875488213027530104, 0.9875488213027530104 ) ) 
 REPRESENTATION_ITEM ( '' )  );
#42517=CARTESIAN_POINT ( 'NONE',  ( 1.003937007874016407, -0.5400638737290844871, 0.3530559997133364547 ) ) ;
#42519=CARTESIAN_POINT ( 'NONE',  ( 1.397637795275591177, 0.07958543189024071263, -0.2665933059059888421 ) ) ;
#42520=ORIENTED_EDGE ( 'NONE', *, *, #49112, .F. ) ;
#42522=CARTESIAN_POINT ( 'NONE',  ( -0.3083989501312330295, -0.3162353388693409650, -0.4822834645669289433 ) ) ;
#42523=ORIENTED_EDGE ( 'NONE', *, *, #64962, .F. ) ;
#42524=CARTESIAN_POINT ( 'NONE',  ( 0.5380577427821529035, -0.004921259842519870586, -0.3153832671262229437 ) ) ;
#42525=AXIS2_PLACEMENT_3D ( 'NONE', #76002, #69681, #18344 ) ;
#42526=CARTESIAN_POINT ( 'NONE',  ( -1.699475065616797398, 0.2952755905511811885, 0.1292274648535926551 ) ) ;
#42527=CARTESIAN_POINT ( 'NONE',  ( 0.6561679790026253567, 0.2306618581243848609, 0.2411417322834645549 ) ) ;
#42528=CARTESIAN_POINT ( 'NONE',  ( 0.4855643044619428750, 0.05413385826771666132, 0.4176697321401328100 ) ) ;
#42529=CARTESIAN_POINT ( 'NONE',  ( 0.006561679790026889343, -0.05778040916215522460, 0.4822834645669289988 ) ) ;
#42531=CARTESIAN_POINT ( 'NONE',  ( -0.8202099737532799750, 0.2952755905511810774, -0.1292274648535930714 ) ) ;
#42533=CARTESIAN_POINT ( 'NONE',  ( -1.646981627296586703, -0.3162353388693409650, -0.4822834645669289433 ) ) ;
#42534=CARTESIAN_POINT ( 'NONE',  ( -1.135170603674539924, 0.2952755905511810774, -0.1292274648535930714 ) ) ;
#42535=CARTESIAN_POINT ( 'NONE',  ( 1.312335958005250269, -0.6046776061558807314, 0.2411417322834647770 ) ) ;
#42536=CARTESIAN_POINT ( 'NONE',  ( 1.207349081364829990, 0.2306618581243848609, 0.2411417322834645549 ) ) ;
#42538=CARTESIAN_POINT ( 'NONE',  ( -0.8530183727034112984, -0.4281496062992127816, -0.4176697321401328100 ) ) ;
#42540=CARTESIAN_POINT ( 'NONE',  ( 0.4855643044619428750, 0.05413385826771666132, 0.4176697321401328100 ) ) ;
#42542=CARTESIAN_POINT ( 'NONE',  ( -0.4790026246719152336, -0.05778040916215560624, -0.4822834645669293319 ) ) ;
#42543=CARTESIAN_POINT ( 'NONE',  ( -1.410761154855641575, -0.2845877964562161244, -0.3641732283464567121 ) ) ;
#42544=CARTESIAN_POINT ( 'NONE',  ( 0.7217847769028878924, -0.004921259842519576551, 0.3153832671262227771 ) ) ;
#42545=CARTESIAN_POINT ( 'NONE',  ( 1.194225721784777594, -0.4281496062992127816, -0.4176697321401328100 ) ) ;
#42547=CARTESIAN_POINT ( 'NONE',  ( 0.5708661417322842269, 0.07958543189024085140, 0.2665933059059887866 ) ) ;
#42548=CARTESIAN_POINT ( 'NONE',  ( 0.6167979002624678353, -0.4281496062992124485, 0.4176697321401328655 ) ) ;
#42550=CARTESIAN_POINT ( 'NONE',  ( -0.6692913385826764205, -0.6692913385826771977, 8.415575281601705876E-17 ) ) ;
#42552=CARTESIAN_POINT ( 'NONE',  ( 1.220472440944882386, -0.5511811023622047445, 6.969142054262312111E-17 ) ) ;
#42553=CARTESIAN_POINT ( 'NONE',  ( -0.6889763779527552368, -0.5400638737290845981, -0.3530559997133363437 ) ) ;
#42554=CARTESIAN_POINT ( 'NONE',  ( 0.04593175853018440641, 0.2952755905511810774, -0.1292274648535930714 ) ) ;
#42555=CARTESIAN_POINT ( 'NONE',  ( 0.2887139107611556010, -0.6046776061558807314, 0.2411417322834647770 ) ) ;
#42556=CARTESIAN_POINT ( 'NONE',  ( -0.006561679790025524116, -0.08942795157528024563, -0.3641732283464568787 ) ) ;
#42558=CARTESIAN_POINT ( 'NONE',  ( 0.1443569553805781891, -0.004921259842519870586, -0.3153832671262229437 ) ) ;
#42559=CARTESIAN_POINT ( 'NONE',  ( 0.8661417322834652488, -0.1870078740157480601, -0.3641732283464567677 ) ) ;
#42562=CARTESIAN_POINT ( 'NONE',  ( 0.2952755905511819101, 0.1660481256975883668, -0.3530559997133364547 ) ) ;
#42567=CARTESIAN_POINT ( 'NONE',  ( 1.404199475065617708, -0.004921259842519870586, -0.3153832671262229437 ) ) ;
#42568=CARTESIAN_POINT ( 'NONE',  ( 0.1049868766404206816, 0.2306618581243848609, 0.2411417322834645549 ) ) ;
#42569=CARTESIAN_POINT ( 'NONE',  ( -0.5446194225721777693, -0.2845877964562161244, -0.3641732283464567121 ) ) ;
#42570=CARTESIAN_POINT ( 'NONE',  ( -0.01968503937007793844, 0.1660481256975883668, -0.3530559997133364547 ) ) ;
#42571=CARTESIAN_POINT ( 'NONE',  ( 1.377952755905512472, 0.1771653543307087630, 0.000000000000000000 ) ) ;
#42572=CARTESIAN_POINT ( 'NONE',  ( -1.417322834645668772, -0.1870078740157479769, 0.3641732283464567677 ) ) ;
#42573=CARTESIAN_POINT ( 'NONE',  ( -1.594488188976377563, -0.5400638737290844871, 0.3530559997133364547 ) ) ;
#42574=CARTESIAN_POINT ( 'NONE',  ( 0.1968503937007881344, -0.6692913385826771977, 8.415575281601705876E-17 ) ) ;
#42575=CARTESIAN_POINT ( 'NONE',  ( 1.345144356955381593, -0.05778040916215522460, 0.4822834645669289988 ) ) ;
#42576=LINE ( 'NONE', #35867, #59890 ) ;
#42577=CARTESIAN_POINT ( 'NONE',  ( 0.1574803149606306130, -0.1870078740157479769, 0.4822834645669291653 ) ) ;
#42578=B_SPLINE_CURVE_WITH_KNOTS ( 'NONE', 3,
 ( #33459, #30449, #3548, #68358 ),
 .UNSPECIFIED., .F., .F.,
 ( 4, 4 ),
 ( 1.999999999897049408E-07, 0.006970199999999935128 ),
 .UNSPECIFIED. ) ;
#42579=CARTESIAN_POINT ( 'NONE',  ( 1.496062992125985147, -0.1870078740157479769, 0.4822834645669291653 ) ) ;
#42580=CARTESIAN_POINT ( 'NONE',  ( 1.010498687664042716, -0.4281496062992124485, 0.4176697321401328655 ) ) ;
#42582=CARTESIAN_POINT ( 'NONE',  ( 0.8136482939632553313, -0.5023911411419708095, -0.1820866141732282451 ) ) ;
#42583=CARTESIAN_POINT ( 'NONE',  ( 1.450131233595801428, -0.6692913385826773087, -0.1292274648535924053 ) ) ;
#42585=CARTESIAN_POINT ( 'NONE',  ( -0.09842519685039295696, 0.07958543189024071263, -0.2665933059059888421 ) ) ;
#42586=CARTESIAN_POINT ( 'NONE',  ( -0.1377952755905504645, -0.5400638737290845981, -0.3530559997133363437 ) ) ;
#42587=CARTESIAN_POINT ( 'NONE',  ( 0.8070866141732288002, 0.1660481256975885056, 0.3530559997133364547 ) ) ;
#42588=CARTESIAN_POINT ( 'NONE',  ( -0.5380577427821514602, 0.05413385826771666132, 0.4176697321401328100 ) ) ;
#42590=CARTESIAN_POINT ( 'NONE',  ( -0.2690288713910754526, 0.1771653543307087075, -0.09757992244046823083 ) ) ;
#42591=CARTESIAN_POINT ( 'NONE',  ( 0.7480314960629927956, -0.6692913385826771977, 8.415575281601705876E-17 ) ) ;
#42592=CARTESIAN_POINT ( 'NONE',  ( 1.102362204724410155, -0.1870078740157480601, -0.3641732283464567677 ) ) ;
#42596=CARTESIAN_POINT ( 'NONE',  ( -1.253280839895012377, -0.3162353388693409650, -0.4822834645669289433 ) ) ;
#42597=CARTESIAN_POINT ( 'NONE',  ( -0.5118110236220466680, -0.6692913385826771977, 8.415575281601705876E-17 ) ) ;
#42600=ORIENTED_EDGE ( 'NONE', *, *, #46038, .T. ) ;
#42601=CARTESIAN_POINT ( 'NONE',  ( 0.3083989501312343062, -0.08942795157528024563, -0.3641732283464568787 ) ) ;
#42603=CARTESIAN_POINT ( 'NONE',  ( 1.220472440944882386, -0.6692913385826771977, 8.415575281601705876E-17 ) ) ;
#42605=CARTESIAN_POINT ( 'NONE',  ( -1.220472440944882830, 0.2066929133858268208, 2.389277853677468338E-14 ) ) ;
#42606=CARTESIAN_POINT ( 'NONE',  ( -1.601049868766403650, -0.5023911411419708095, 0.1820866141732285504 ) ) ;
#42607=CARTESIAN_POINT ( 'NONE',  ( 1.627296587926509996, -0.6046776061558807314, 0.2411417322834647770 ) ) ;
#42608=CARTESIAN_POINT ( 'NONE',  ( 1.318897637795276356, 0.07958543189024071263, -0.2665933059059888421 ) ) ;
#42609=CARTESIAN_POINT ( 'NONE',  ( 0.5249343832021005074, -0.6046776061558807314, 0.2411417322834647770 ) ) ;
#42610=CIRCLE ( 'NONE', #64126, 2.306288321832234978 ) ;
#42612=CARTESIAN_POINT ( 'NONE',  ( -0.1049868766404193215, -0.6046776061558807314, 0.2411417322834647770 ) ) ;
#42613=CARTESIAN_POINT ( 'NONE',  ( -0.9514435695538050464, -0.2845877964562159024, 0.3641732283464567677 ) ) ;
#42614=CARTESIAN_POINT ( 'NONE',  ( 0.3805774278215230400, 0.05413385826771626580, -0.4176697321401330321 ) ) ;
#42615=CARTESIAN_POINT ( 'NONE',  ( -0.1509186351706028884, -0.05778040916215522460, 0.4822834645669289988 ) ) ;
#42616=CARTESIAN_POINT ( 'NONE',  ( -1.614173228346457378, 2.094556775020298023, 0.1372047244094476981 ) ) ;
#42617=VECTOR ( 'NONE', #18863, 39.37007874015748143 ) ;
#42620=CARTESIAN_POINT ( 'NONE',  ( 0.6824146981627303710, -0.6046776061558807314, 0.2411417322834647770 ) ) ;
#42623=CARTESIAN_POINT ( 'NONE',  ( -0.3477690288713905509, -0.6692913385826771977, 0.1292274648535927661 ) ) ;
#42624=CARTESIAN_POINT ( 'NONE',  ( -1.272965879265091305, 0.05413385826771626580, -0.4176697321401330321 ) ) ;
#42625=CARTESIAN_POINT ( 'NONE',  ( 0.9908136482939640111, 0.2952755905511810774, -0.1292274648535930714 ) ) ;
#42626=CARTESIAN_POINT ( 'NONE',  ( 0.6758530183727039509, -0.6692913385826771977, 0.1292274648535927661 ) ) ;
#42628=CARTESIAN_POINT ( 'NONE',  ( -0.2165354330708654795, -0.5400638737290845981, -0.3530559997133363437 ) ) ;
#42629=CARTESIAN_POINT ( 'NONE',  ( 0.1246719160104994284, 0.2952755905511810774, -0.1292274648535930714 ) ) ;
#42630=CARTESIAN_POINT ( 'NONE',  ( -0.5314960629921250401, 0.1660481256975885056, 0.3530559997133364547 ) ) ;
#42631=CARTESIAN_POINT ( 'NONE',  ( 0.1377952755905518800, 0.07958543189024071263, -0.2665933059059888421 ) ) ;
#42632=CARTESIAN_POINT ( 'NONE',  ( 1.601049868766404982, -0.5023911411419708095, -0.1820866141732282451 ) ) ;
#42633=CARTESIAN_POINT ( 'NONE',  ( -0.7210809602247715278, -2.613618158232546091E-15, -0.3464511005275220379 ) ) ;
#42634=CARTESIAN_POINT ( 'NONE',  ( 0.4790026246719167324, -0.05778040916215522460, 0.4822834645669289988 ) ) ;
#42635=CARTESIAN_POINT ( 'NONE',  ( 1.450131233595801428, 0.2952755905511811885, 0.1292274648535926551 ) ) ;
#42637=EDGE_LOOP ( 'NONE', ( #72684, #41374, #33615, #75178 ) ) ;
#42639=CARTESIAN_POINT ( 'NONE',  ( 0.8989501312335964611, 0.2952755905511811885, 0.1292274648535926551 ) ) ;
#42640=CARTESIAN_POINT ( 'NONE',  ( 0.03280839895013198948, 0.1771653543307087630, 0.09757992244046791164 ) ) ;
#42644=CARTESIAN_POINT ( 'NONE',  ( -0.9559795740584949852, -3.764720552277026557E-15, -0.3954974714151476278 ) ) ;
#42645=CARTESIAN_POINT ( 'NONE',  ( 0.3049517105654749871, 8.471767977567108961E-16, -0.4445507791589058955 ) ) ;
#42647=CARTESIAN_POINT ( 'NONE',  ( 1.076115485564305141, -0.6046776061558807314, 0.2411417322834647770 ) ) ;
#42648=CARTESIAN_POINT ( 'NONE',  ( -0.7414698162729651543, -0.6692913385826771977, 0.1292274648535927661 ) ) ;
#42649=CARTESIAN_POINT ( 'NONE',  ( -0.8464566929133852113, -0.5400638737290845981, -0.3530559997133363437 ) ) ;
#42650=CARTESIAN_POINT ( 'NONE',  ( 0.7020997375328090762, -0.05778040916215560624, -0.4822834645669293319 ) ) ;
#42651=CARTESIAN_POINT ( 'NONE',  ( 1.469816272965879911, 0.2306618581243847221, -0.2411417322834647770 ) ) ;
#42652=CARTESIAN_POINT ( 'NONE',  ( 1.194225721784777594, 0.009842519685039467087, 0.3409548833797002021 ) ) ;
#42654=CARTESIAN_POINT ( 'NONE',  ( 1.174540682414699111, -0.2845877964562159024, 0.3641732283464567677 ) ) ;
#42655=CARTESIAN_POINT ( 'NONE',  ( -0.7020997375328074108, -0.05778040916215522460, 0.4822834645669289988 ) ) ;
#42656=CARTESIAN_POINT ( 'NONE',  ( 1.581364829396326277, -0.3162353388693409650, -0.4822834645669289433 ) ) ;
#42658=CARTESIAN_POINT ( 'NONE',  ( 0.01968503937007957949, -0.5400638737290845981, -0.3530559997133363437 ) ) ;
#42659=CARTESIAN_POINT ( 'NONE',  ( 1.030183727034121421, -0.05778040916215522460, 0.4822834645669289988 ) ) ;
#42661=CARTESIAN_POINT ( 'NONE',  ( -1.128608923884513837, -0.5023911411419708095, 0.1820866141732285504 ) ) ;
#42662=CARTESIAN_POINT ( 'NONE',  ( 0.2165354330708668673, -0.5400638737290844871, 0.3530559997133364547 ) ) ;
#42663=CARTESIAN_POINT ( 'NONE',  ( 1.417322834645670104, -0.1870078740157479769, 0.3641732283464567677 ) ) ;
#42665=CARTESIAN_POINT ( 'NONE',  ( -1.397637795275589623, 0.07958543189024085140, 0.2665933059059887866 ) ) ;
#42666=CARTESIAN_POINT ( 'NONE',  ( 1.397637795275591177, 0.1660481256975883668, -0.3530559997133364547 ) ) ;
#42668=CARTESIAN_POINT ( 'NONE',  ( -0.006561679790025524116, -0.2845877964562159024, 0.3641732283464567677 ) ) ;
#42669=CARTESIAN_POINT ( 'NONE',  ( 0.01968503937007930540, 0.1660481256975885056, 0.3530559997133364547 ) ) ;
#42670=CARTESIAN_POINT ( 'NONE',  ( -1.371391076115484609, -0.5511811023622046335, 0.09757992244046803654 ) ) ;
#42671=CARTESIAN_POINT ( 'NONE',  ( -0.5774278215223089816, 0.2306618581243847221, -0.2411417322834647770 ) ) ;
#42672=CARTESIAN_POINT ( 'NONE',  ( 1.437007874015748810, -0.5400638737290845981, -0.3530559997133363437 ) ) ;
#42674=EDGE_CURVE ( 'NONE', #70238, #60047, #53373, .T. ) ;
#42676=CARTESIAN_POINT ( 'NONE',  ( 1.404199475065617264, -0.4281496062992124485, 0.4176697321401328655 ) ) ;
#42678=CARTESIAN_POINT ( 'NONE',  ( -1.200787401574802349, 0.1660481256975883668, -0.3530559997133364547 ) ) ;
#42679=CARTESIAN_POINT ( 'NONE',  ( -1.056430446194224881, -0.5511811023622046335, 0.09757992244046803654 ) ) ;
#42680=CARTESIAN_POINT ( 'NONE',  ( -0.4921259842519677963, -0.4536011799217367080, 0.2665933059059888421 ) ) ;
#42681=CARTESIAN_POINT ( 'NONE',  ( -1.204164820379008294, 2.401574803149606474, -0.4915354330708643360 ) ) ;
#42682=CARTESIAN_POINT ( 'NONE',  ( -0.1049868766404193215, -0.6046776061558807314, 0.2411417322834647770 ) ) ;
#42683=CARTESIAN_POINT ( 'NONE',  ( -0.1115485564304453947, -0.5511811023622046335, 0.09757992244046803654 ) ) ;
#42684=CARTESIAN_POINT ( 'NONE',  ( -1.069553805774277722, 0.1771653543307087630, 0.09757992244046791164 ) ) ;
#42685=CARTESIAN_POINT ( 'NONE',  ( -1.679790026246718693, 0.2306618581243847221, -0.2411417322834647770 ) ) ;
#42686=CARTESIAN_POINT ( 'NONE',  ( 1.502624671916010790, -0.2845877964562161244, -0.3641732283464567121 ) ) ;
#42688=CARTESIAN_POINT ( 'NONE',  ( 1.305774278215223960, -0.6692913385826771977, 0.1292274648535927661 ) ) ;
#42690=CARTESIAN_POINT ( 'NONE',  ( 0.5905511811023629321, 0.1771653543307087630, 0.000000000000000000 ) ) ;
#42691=CARTESIAN_POINT ( 'NONE',  ( 0.8858267716535438430, 0.1660481256975885056, 0.3530559997133364547 ) ) ;
#42692=CARTESIAN_POINT ( 'NONE',  ( 1.095800524934383846, -0.2845877964562159024, 0.3641732283464567677 ) ) ;
#42694=CARTESIAN_POINT ( 'NONE',  ( -1.108923884514435132, -0.05778040916215560624, -0.4822834645669293319 ) ) ;
#42695=CARTESIAN_POINT ( 'NONE',  ( -1.056430446194224881, -0.6692913385826771977, 0.1292274648535927661 ) ) ;
#42696=CARTESIAN_POINT ( 'NONE',  ( 0.05905511811023681640, 0.1660481256975883668, -0.3530559997133364547 ) ) ;
#42699=CARTESIAN_POINT ( 'NONE',  ( 0.7808398950131240079, -0.3162353388693405765, 0.4822834645669290543 ) ) ;
#42700=CARTESIAN_POINT ( 'NONE',  ( -1.653543307086613234, -0.1870078740157480879, -0.4822834645669291653 ) ) ;
#42701=CARTESIAN_POINT ( 'NONE',  ( -0.09186351706036663400, -0.4281496062992124485, 0.4176697321401328655 ) ) ;
#42702=CARTESIAN_POINT ( 'NONE',  ( 0.8530183727034126306, 0.05413385826771626580, -0.4176697321401330321 ) ) ;
#42708=CARTESIAN_POINT ( 'NONE',  ( -0.4068241469816267775, -0.004921259842519870586, -0.3153832671262229437 ) ) ;
#42709=CARTESIAN_POINT ( 'NONE',  ( -0.7742782152230965886, 0.05413385826771666132, 0.4176697321401328100 ) ) ;
#42710=CARTESIAN_POINT ( 'NONE',  ( 0.4527559055118117182, -0.5400638737290844871, 0.3530559997133364547 ) ) ;
#42712=CARTESIAN_POINT ( 'NONE',  ( 1.548556430446194954, -0.6046776061558807314, 0.2411417322834647770 ) ) ;
#42713=CARTESIAN_POINT ( 'NONE',  ( 1.345144356955381593, -0.3162353388693409650, -0.4822834645669289433 ) ) ;
#42717=CARTESIAN_POINT ( 'NONE',  ( 0.9317585301837276734, -0.4281496062992124485, 0.4176697321401328655 ) ) ;
#42718=CARTESIAN_POINT ( 'NONE',  ( 1.410761154855643795, -0.2845877964562159024, 0.3641732283464567677 ) ) ;
#42719=CARTESIAN_POINT ( 'NONE',  ( 1.528871391076116026, 0.2952755905511811885, 0.1292274648535926551 ) ) ;
#42720=CARTESIAN_POINT ( 'NONE',  ( -1.384514435695537005, -0.6692913385826773087, -0.1292274648535924053 ) ) ;
#42723=CARTESIAN_POINT ( 'NONE',  ( 0.8858267716535438430, 0.1660481256975885056, 0.3530559997133364547 ) ) ;
#42724=CARTESIAN_POINT ( 'NONE',  ( 1.469816272965879911, -0.5023911411419708095, 0.1820866141732285504 ) ) ;
#42725=CARTESIAN_POINT ( 'NONE',  ( -0.4593175853018366950, 0.05413385826771666132, 0.4176697321401328100 ) ) ;
#42726=CARTESIAN_POINT ( 'NONE',  ( -0.6036745406824141069, 0.2306618581243848609, 0.2411417322834645549 ) ) ;
#42727=CARTESIAN_POINT ( 'NONE',  ( 1.463254593175853824, 0.2952755905511810774, -0.1292274648535930714 ) ) ;
#42729=CARTESIAN_POINT ( 'NONE',  ( 0.2493438320209980519, -0.4281496062992127816, -0.4176697321401328100 ) ) ;
#42731=CARTESIAN_POINT ( 'NONE',  ( 1.633858267716535639, -0.5400638737290844871, 0.3530559997133364547 ) ) ;
#42736=CARTESIAN_POINT ( 'NONE',  ( -1.410761154855642463, -0.05778040916215522460, 0.4822834645669289988 ) ) ;
#42743=CARTESIAN_POINT ( 'NONE',  ( -0.3083989501312330295, -0.2845877964562161244, -0.3641732283464567121 ) ) ;
#42745=CARTESIAN_POINT ( 'NONE',  ( -1.332020997375327642, -0.2845877964562161244, -0.3641732283464567121 ) ) ;
#42746=CARTESIAN_POINT ( 'NONE',  ( -1.620734908136482577, 0.2952755905511811885, 0.1292274648535926551 ) ) ;
#42747=CARTESIAN_POINT ( 'NONE',  ( 0.4068241469816279987, -0.4281496062992127816, -0.4176697321401328100 ) ) ;
#42748=CARTESIAN_POINT ( 'NONE',  ( -1.358267716535432434, -0.5400638737290844871, 0.3530559997133364547 ) ) ;
#42750=ORIENTED_EDGE ( 'NONE', *, *, #39775, .F. ) ;
#42751=CARTESIAN_POINT ( 'NONE',  ( 1.482939632545932307, 0.05413385826771626580, -0.4176697321401330321 ) ) ;
#42756=FACE_OUTER_BOUND ( 'NONE', #75938, .T. ) ;
#42757=CARTESIAN_POINT ( 'NONE',  ( -0.6824146981627288167, 0.2306618581243848609, 0.2411417322834645549 ) ) ;
#42758=CARTESIAN_POINT ( 'NONE',  ( 1.476377952755906442, -0.5400638737290844871, 0.3530559997133364547 ) ) ;
#42759=CARTESIAN_POINT ( 'NONE',  ( 0.7186703366786206804, -1.374501131054255944E-15, 0.4445507791589066726 ) ) ;
#42760=CARTESIAN_POINT ( 'NONE',  ( 0.6496062992125991586, 0.1012011053420777407, 0.2882089793578257453 ) ) ;
#42761=CARTESIAN_POINT ( 'NONE',  ( 1.489501312335958172, -0.3162353388693405765, 0.4822834645669290543 ) ) ;
#42762=CARTESIAN_POINT ( 'NONE',  ( -0.6824146981627291497, -0.6046776061558809534, -0.2411417322834644161 ) ) ;
#42764=CARTESIAN_POINT ( 'NONE',  ( -0.08530183727034056085, -0.08942795157528024563, -0.3641732283464568787 ) ) ;
#42766=CARTESIAN_POINT ( 'NONE',  ( -0.006561679790025524116, -0.08942795157528024563, -0.3641732283464568787 ) ) ;
#42767=CARTESIAN_POINT ( 'NONE',  ( 0.5380577427821529035, -0.004921259842519870586, -0.3153832671262229437 ) ) ;
#42768=CARTESIAN_POINT ( 'NONE',  ( 0.4658792650918640033, -0.3162353388693405765, 0.4822834645669290543 ) ) ;
#42769=CARTESIAN_POINT ( 'NONE',  ( -0.7020997375328074108, -0.08942795157527998196, 0.3641732283464567121 ) ) ;
#42771=CARTESIAN_POINT ( 'NONE',  ( -1.541994750656167090, -0.6692913385826773087, -0.1292274648535924053 ) ) ;
#42772=CARTESIAN_POINT ( 'NONE',  ( -0.9251968503937002541, -0.5400638737290845981, -0.3530559997133363437 ) ) ;
#42774=CARTESIAN_POINT ( 'NONE',  ( 0.1968503937007881344, 0.2952755905511811885, 0.000000000000000000 ) ) ;
#42775=CARTESIAN_POINT ( 'NONE',  ( -0.6561679790026240244, 0.2306618581243847221, -0.2411417322834647770 ) ) ;
#42776=CARTESIAN_POINT ( 'NONE',  ( 1.141732283464567788, -0.5511811023622047445, 6.969142054262312111E-17 ) ) ;
#42777=CARTESIAN_POINT ( 'NONE',  ( 0.06561679790026316017, -0.004921259842519870586, -0.3153832671262229437 ) ) ;
#42778=CARTESIAN_POINT ( 'NONE',  ( -0.09842519685039295696, 0.1660481256975883668, -0.3530559997133364547 ) ) ;
#42779=CARTESIAN_POINT ( 'NONE',  ( -0.7611548556430438595, -0.6046776061558809534, -0.2411417322834644161 ) ) ;
#42780=CARTESIAN_POINT ( 'NONE',  ( -0.5944687039322197331, 1.968503937007873850, -0.4915354330708654462 ) ) ;
#42781=CARTESIAN_POINT ( 'NONE',  ( -1.011202504342156416, -2.294479370626195693E-15, 0.3464511005275217603 ) ) ;
#42783=CARTESIAN_POINT ( 'NONE',  ( 0.1312335958005257930, 0.2306618581243847221, -0.2411417322834647770 ) ) ;
#42786=CARTESIAN_POINT ( 'NONE',  ( 1.135170603674541256, 0.2952755905511811885, 0.1292274648535926551 ) ) ;
#42787=CARTESIAN_POINT ( 'NONE',  ( -0.7414698162729651543, 0.1771653543307087075, -0.09757992244046823083 ) ) ;
#42788=CARTESIAN_POINT ( 'NONE',  ( -0.4002624671916004129, -0.05778040916215560624, -0.4822834645669293319 ) ) ;
#42789=CARTESIAN_POINT ( 'NONE',  ( 1.253280839895013710, -0.05778040916215560624, -0.4822834645669293319 ) ) ;
#42790=CARTESIAN_POINT ( 'NONE',  ( 0.9776902887139113929, -0.6692913385826773087, -0.1292274648535924053 ) ) ;
#42791=CARTESIAN_POINT ( 'NONE',  ( -1.509186351706035767, -0.4281496062992124485, 0.4176697321401328655 ) ) ;
#42792=CARTESIAN_POINT ( 'NONE',  ( -1.043307086614172707, 0.07958543189024071263, -0.2665933059059888421 ) ) ;
#42796=CARTESIAN_POINT ( 'NONE',  ( 1.607611548556431069, -0.5511811023622048555, -0.09757992244046775898 ) ) ;
#42798=CARTESIAN_POINT ( 'NONE',  ( 1.010498687664042716, -0.004921259842519870586, -0.3153832671262229437 ) ) ;
#42799=CARTESIAN_POINT ( 'NONE',  ( 0.3608923884514443348, 0.2952755905511810774, -0.1292274648535930714 ) ) ;
#42800=CARTESIAN_POINT ( 'NONE',  ( -1.666666666666665853, 0.05413385826771626580, -0.4176697321401330321 ) ) ;
#42802=CARTESIAN_POINT ( 'NONE',  ( 0.8727034120734913358, -0.08942795157527998196, 0.3641732283464567121 ) ) ;
#42803=CARTESIAN_POINT ( 'NONE',  ( -0.4133858267716528645, -0.5400638737290844871, 0.3530559997133364547 ) ) ;
#42804=CARTESIAN_POINT ( 'NONE',  ( -0.7874015748031489847, -0.1870078740157480879, -0.4822834645669291653 ) ) ;
#42805=CARTESIAN_POINT ( 'NONE',  ( 1.266404199475066328, -0.3162353388693409650, -0.4822834645669289433 ) ) ;
#42808=CARTESIAN_POINT ( 'NONE',  ( 0.1049868766404206816, -0.5023911411419708095, -0.1820866141732282451 ) ) ;
#42811=ORIENTED_EDGE ( 'NONE', *, *, #1873, .F. ) ;
#42812=CARTESIAN_POINT ( 'NONE',  ( -1.010498687664041384, -0.4281496062992127816, -0.4176697321401328100 ) ) ;
#42813=CARTESIAN_POINT ( 'NONE',  ( -0.2559055118110227234, -0.5400638737290844871, 0.3530559997133364547 ) ) ;
#42814=CARTESIAN_POINT ( 'NONE',  ( -0.4593175853018364174, -0.4281496062992127816, -0.4176697321401328100 ) ) ;
#42815=CARTESIAN_POINT ( 'NONE',  ( 0.8530183727034128527, -0.4281496062992124485, 0.4176697321401328655 ) ) ;
#42816=CARTESIAN_POINT ( 'NONE',  ( -0.3871391076115476282, -0.05778040916215522460, 0.4822834645669289988 ) ) ;
#42817=CARTESIAN_POINT ( 'NONE',  ( -1.259842519685038686, -0.1870078740157480879, -0.4822834645669291653 ) ) ;
#42818=CARTESIAN_POINT ( 'NONE',  ( -0.5249343832020990641, -0.6046776061558809534, -0.2411417322834644161 ) ) ;
#42819=CARTESIAN_POINT ( 'NONE',  ( 0.8595800524934390507, -0.05778040916215560624, -0.4822834645669293319 ) ) ;
#42820=CARTESIAN_POINT ( 'NONE',  ( 0.5314960629921264834, 0.1660481256975883668, -0.3530559997133364547 ) ) ;
#42821=ADVANCED_FACE ( 'NONE', ( #57652 ), #14, .T. ) ;
#42823=CARTESIAN_POINT ( 'NONE',  ( -0.2296587926509179312, -0.08942795157527998196, 0.3641732283464567121 ) ) ;
#42824=ORIENTED_EDGE ( 'NONE', *, *, #23015, .T. ) ;
#42826=ORIENTED_EDGE ( 'NONE', *, *, #36816, .T. ) ;
#42827=CARTESIAN_POINT ( 'NONE',  ( -1.463254593175852492, -0.5511811023622048555, -0.09757992244046775898 ) ) ;
#42828=CARTESIAN_POINT ( 'NONE',  ( -0.4461942257217840213, -0.6046776061558809534, -0.2411417322834644161 ) ) ;
#42829=CARTESIAN_POINT ( 'NONE',  ( 0.7773926554473647998, 8.471767977567108961E-16, -0.4445507791589058955 ) ) ;
#42830=CARTESIAN_POINT ( 'NONE',  ( -0.8202099737532801971, -0.6692913385826771977, 0.1292274648535927661 ) ) ;
#42831=CARTESIAN_POINT ( 'NONE',  ( -0.9317585301837263412, 0.05413385826771666132, 0.4176697321401328100 ) ) ;
#42832=CARTESIAN_POINT ( 'NONE',  ( -1.456692913385826182, 0.2952755905511811885, 0.000000000000000000 ) ) ;
#42833=CARTESIAN_POINT ( 'NONE',  ( -1.646981627296586703, -0.3162353388693409650, -0.4822834645669289433 ) ) ;
#42834=CARTESIAN_POINT ( 'NONE',  ( 1.069553805774278832, 0.1771653543307087075, -0.09757992244046823083 ) ) ;
#42835=CARTESIAN_POINT ( 'NONE',  ( 1.171093442848939681, -8.644661201599092366E-16, -0.4445507791589066171 ) ) ;
#42837=CARTESIAN_POINT ( 'NONE',  ( 0.2034120734908142214, 0.1771653543307087075, -0.09757992244046823083 ) ) ;
#42838=CARTESIAN_POINT ( 'NONE',  ( -0.3674540682414689785, 0.2306618581243848609, 0.2411417322834645549 ) ) ;
#42840=CARTESIAN_POINT ( 'NONE',  ( -0.2362204724409440182, -0.1870078740157479769, 0.4822834645669291653 ) ) ;
#42847=CARTESIAN_POINT ( 'NONE',  ( -0.7283464566929126471, 0.07958543189024071263, -0.2665933059059888421 ) ) ;
#42848=CARTESIAN_POINT ( 'NONE',  ( -0.9842519685039365918, -0.6692913385826771977, 8.415575281601705876E-17 ) ) ;
#42852=CARTESIAN_POINT ( 'NONE',  ( 1.410761154855643795, -0.05778040916215560624, -0.4822834645669293319 ) ) ;
#42853=CARTESIAN_POINT ( 'NONE',  ( 0.3215223097112867578, -0.05778040916215522460, 0.4822834645669289988 ) ) ;
#42854=CARTESIAN_POINT ( 'NONE',  ( 0.4855643044619430415, -0.4281496062992127816, -0.4176697321401328100 ) ) ;
#42855=CARTESIAN_POINT ( 'NONE',  ( -0.4986876640419939388, 0.1283753931104746893, -0.1820866141732285504 ) ) ;
#42856=CARTESIAN_POINT ( 'NONE',  ( -0.5118110236220466680, -0.6692913385826771977, 8.415575281601705876E-17 ) ) ;
#42858=CARTESIAN_POINT ( 'NONE',  ( -0.9580052493438311334, -0.4281496062992124485, 0.4176697321401328655 ) ) ;
#42860=CARTESIAN_POINT ( 'NONE',  ( 1.364829396325459854, -0.5023911411419708095, -0.1820866141732282451 ) ) ;
#42861=CARTESIAN_POINT ( 'NONE',  ( -0.2427821522309703550, -0.08942795157528024563, -0.3641732283464568787 ) ) ;
#42862=CARTESIAN_POINT ( 'NONE',  ( 1.141732283464567788, -0.5511811023622047445, 6.969142054262312111E-17 ) ) ;
#42863=CARTESIAN_POINT ( 'NONE',  ( -1.377952755905511140, 0.2952755905511811885, 0.000000000000000000 ) ) ;
#42864=CARTESIAN_POINT ( 'NONE',  ( -1.227034120734907141, -0.5511811023622048555, -0.09757992244046775898 ) ) ;
#42866=CARTESIAN_POINT ( 'NONE',  ( -1.312335958005248715, -0.6046776061558809534, -0.2411417322834644161 ) ) ;
#42867=CARTESIAN_POINT ( 'NONE',  ( -0.4461942257217840213, -0.6046776061558809534, -0.2411417322834644161 ) ) ;
#42869=CARTESIAN_POINT ( 'NONE',  ( 0.03280839895013198948, -0.5511811023622048555, -0.09757992244046775898 ) ) ;
#42870=CARTESIAN_POINT ( 'NONE',  ( -1.601049868766403650, -0.5023911411419708095, 0.1820866141732285504 ) ) ;
#42871=( BOUNDED_CURVE ( )  B_SPLINE_CURVE ( 2, ( #61564, #80936, #29975, #55639, #17783, #75850, #43417, #5139, #43825, #48922, #17380, #69115, #4716 ),
 .UNSPECIFIED., .F., .F. ) 
 B_SPLINE_CURVE_WITH_KNOTS ( ( 3, 2, 2, 2, 2, 2, 3 ),
 ( 0.1733310946348008696, 0.1742424242424242542, 0.1780303030303030387, 0.1818181818181818232, 0.1856060606060606077, 0.1893939393939393923, 0.1903052690015628601 ),
 .UNSPECIFIED. ) 
 CURVE ( )  GEOMETRIC_REPRESENTATION_ITEM ( )  RATIONAL_B_SPLINE_CURVE ( ( 0.9875488213027527884, 0.9918020599134683701, 1.000000000000000000, 0.9659258262890683122, 1.000000000000000000, 0.9659258262890683122, 1.000000000000000000, 0.9659258262890683122, 1.000000000000000000, 0.9659258262890683122, 1.000000000000000000, 0.9918020599134675930, 0.9875488213027519002 ) ) 
 REPRESENTATION_ITEM ( '' )  );
#42872=CARTESIAN_POINT ( 'NONE',  ( 0.5905511811023629321, 0.2952755905511811885, 0.000000000000000000 ) ) ;
#42874=CARTESIAN_POINT ( 'NONE',  ( 1.535433070866142335, -0.5511811023622047445, 6.969142054262312111E-17 ) ) ;
#42875=CARTESIAN_POINT ( 'NONE',  ( -0.8398950131233589023, -0.6046776061558809534, -0.2411417322834644161 ) ) ;
#42876=CARTESIAN_POINT ( 'NONE',  ( -0.2165354330708654795, 0.07958543189024085140, 0.2665933059059887866 ) ) ;
#42878=CARTESIAN_POINT ( 'NONE',  ( 0.1377952755905518800, -0.4536011799217367080, 0.2665933059059888421 ) ) ;
#42879=CARTESIAN_POINT ( 'NONE',  ( -0.2755905511811015396, -0.6692913385826771977, 8.415575281601705876E-17 ) ) ;
#42882=CARTESIAN_POINT ( 'NONE',  ( 0.6889763779527563470, 0.07958543189024071263, -0.2665933059059888421 ) ) ;
#42883=CARTESIAN_POINT ( 'NONE',  ( 0.07874015748031558404, -0.1870078740157479769, 0.4822834645669291653 ) ) ;
#42884=CARTESIAN_POINT ( 'NONE',  ( -0.6758530183727028406, 0.2952755905511811885, 0.1292274648535926551 ) ) ;
#42885=CARTESIAN_POINT ( 'NONE',  ( -0.7677165354330699465, -0.4536011799217368745, -0.2665933059059886201 ) ) ;
#42887=CARTESIAN_POINT ( 'NONE',  ( -0.4921259842519677963, 0.07958543189024071263, -0.2665933059059888421 ) ) ;
#42888=CARTESIAN_POINT ( 'NONE',  ( 0.1049868766404206816, 0.2306618581243848609, 0.2411417322834645549 ) ) ;
#42890=CARTESIAN_POINT ( 'NONE',  ( -1.345144356955379816, -0.08942795157528024563, -0.3641732283464568787 ) ) ;
#42892=CARTESIAN_POINT ( 'NONE',  ( -1.476377952755905110, 0.1660481256975885056, 0.3530559997133364547 ) ) ;
#42895=CARTESIAN_POINT ( 'NONE',  ( -1.673228346456691717, 0.07958543189024071263, -0.2665933059059888421 ) ) ;
#42896=CARTESIAN_POINT ( 'NONE',  ( -0.3543307086614165824, -0.6692913385826771977, 8.415575281601705876E-17 ) ) ;
#42897=CARTESIAN_POINT ( 'NONE',  ( -1.049868766404198794, -0.6046776061558807314, 0.2411417322834647770 ) ) ;
#42900=CARTESIAN_POINT ( 'NONE',  ( 0.9383202099737538715, -0.05778040916215560624, -0.4822834645669293319 ) ) ;
#42901=CARTESIAN_POINT ( 'NONE',  ( 0.5708661417322842269, 0.1660481256975885056, 0.3530559997133364547 ) ) ;
#42904=CARTESIAN_POINT ( 'NONE',  ( -1.706036745406823485, 0.2306618581243848609, 0.2411417322834645549 ) ) ;
#42907=CARTESIAN_POINT ( 'NONE',  ( -0.8070866141732276899, 0.07958543189024071263, -0.2665933059059888421 ) ) ;
#42910=CARTESIAN_POINT ( 'NONE',  ( 0.2559055118110243332, -0.5400638737290845981, -0.3530559997133363437 ) ) ;
#42911=CARTESIAN_POINT ( 'NONE',  ( -0.5839895013123351797, 0.2952755905511810774, -0.1292274648535930714 ) ) ;
#42912=CARTESIAN_POINT ( 'NONE',  ( -1.246719160104985846, -0.4281496062992127816, -0.4176697321401328100 ) ) ;
#42913=CARTESIAN_POINT ( 'NONE',  ( 1.102362204724410155, -0.1870078740157480879, -0.4822834645669291653 ) ) ;
#42914=CARTESIAN_POINT ( 'NONE',  ( -1.148293963254592542, 0.1771653543307087630, 0.09757992244046791164 ) ) ;
#42916=CARTESIAN_POINT ( 'NONE',  ( 0.09186351706036827158, 0.05413385826771666132, 0.4176697321401328100 ) ) ;
#42917=CARTESIAN_POINT ( 'NONE',  ( -1.122047244094487306, 0.1660481256975883668, -0.3530559997133364547 ) ) ;
#42919=CARTESIAN_POINT ( 'NONE',  ( -1.528871391076114250, -0.6692913385826771977, 0.1292274648535927661 ) ) ;
#42920=CARTESIAN_POINT ( 'NONE',  ( -1.614173228346456712, 0.7166040191147899918, -0.1372047244094478091 ) ) ;
#42922=CARTESIAN_POINT ( 'NONE',  ( 0.8333333333333340365, -0.5511811023622046335, 0.09757992244046803654 ) ) ;
#42925=CARTESIAN_POINT ( 'NONE',  ( -1.023622047244093558, -0.1870078740157479769, 0.4822834645669291653 ) ) ;
#42927=CARTESIAN_POINT ( 'NONE',  ( 0.09186351706036799403, -0.3690944881889765550, -0.3153832671262227771 ) ) ;
#42929=CARTESIAN_POINT ( 'NONE',  ( 0.4068241469816279987, -0.4281496062992127816, -0.4176697321401328100 ) ) ;
#42930=CARTESIAN_POINT ( 'NONE',  ( 0.6299212598425204535, -0.1870078740157479769, 0.4822834645669291653 ) ) ;
#42931=CARTESIAN_POINT ( 'NONE',  ( -0.7808398950131225646, -0.05778040916215522460, 0.4822834645669289988 ) ) ;
#42933=CARTESIAN_POINT ( 'NONE',  ( -0.9055118110236215490, -0.6692913385826771977, 8.415575281601705876E-17 ) ) ;
#42934=EDGE_CURVE ( 'NONE', #18593, #949, #3132, .T. ) ;
#42936=CARTESIAN_POINT ( 'NONE',  ( 1.384514435695538337, -0.5511811023622046335, 0.09757992244046803654 ) ) ;
#42937=CARTESIAN_POINT ( 'NONE',  ( -1.167979002624671470, 0.05413385826771666132, 0.4176697321401328100 ) ) ;
#42938=CARTESIAN_POINT ( 'NONE',  ( 0.9251968503937015864, 0.1660481256975883668, -0.3530559997133364547 ) ) ;
#42939=CARTESIAN_POINT ( 'NONE',  ( 1.023622047244095334, -0.1870078740157479769, 0.4822834645669291653 ) ) ;
#42941=CARTESIAN_POINT ( 'NONE',  ( -1.003937007874015297, -0.5400638737290845981, -0.3530559997133363437 ) ) ;
#42943=CARTESIAN_POINT ( 'NONE',  ( 0.2165354330708668673, 0.1660481256975883668, -0.3530559997133364547 ) ) ;
#42945=CARTESIAN_POINT ( 'NONE',  ( -0.6102362204724400829, -0.5400638737290845981, -0.3530559997133363437 ) ) ;
#42946=CARTESIAN_POINT ( 'NONE',  ( -1.384514435695537005, -0.5511811023622048555, -0.09757992244046775898 ) ) ;
#42947=CARTESIAN_POINT ( 'NONE',  ( 0.4724409448818904789, -0.1870078740157480601, -0.3641732283464567677 ) ) ;
#42948=CARTESIAN_POINT ( 'NONE',  ( 0.9186351706036751663, -0.6046776061558807314, 0.2411417322834647770 ) ) ;
#42950=CARTESIAN_POINT ( 'NONE',  ( 0.9120734908136490793, 0.1771653543307087075, -0.09757992244046823083 ) ) ;
#42952=CARTESIAN_POINT ( 'NONE',  ( 0.7217847769028878924, -0.4281496062992127816, -0.4176697321401328100 ) ) ;
#42954=CARTESIAN_POINT ( 'NONE',  ( -0.6430446194225716283, -0.4281496062992124485, 0.4176697321401328655 ) ) ;
#42956=CARTESIAN_POINT ( 'NONE',  ( 1.102362204724410155, -0.1870078740157479769, 0.3641732283464567677 ) ) ;
#42957=CARTESIAN_POINT ( 'NONE',  ( -0.4199475065616791736, 0.2306618581243847221, -0.2411417322834647770 ) ) ;
#42958=EDGE_CURVE ( 'NONE', #18885, #58371, #21628, .T. ) ;
#42959=CARTESIAN_POINT ( 'NONE',  ( -0.09842519685039295696, 0.1660481256975883668, -0.3530559997133364547 ) ) ;
#42961=CARTESIAN_POINT ( 'NONE',  ( 0.3018372703412079971, -0.4281496062992124485, 0.4176697321401328655 ) ) ;
#42962=CARTESIAN_POINT ( 'NONE',  ( 0.04593175853018440641, -0.5511811023622046335, 0.09757992244046803654 ) ) ;
#42964=CARTESIAN_POINT ( 'NONE',  ( -0.1115485564304453947, -0.5511811023622046335, 0.09757992244046803654 ) ) ;
#42965=CARTESIAN_POINT ( 'NONE',  ( 0.9448818897637802916, -0.1870078740157479769, 0.3641732283464567677 ) ) ;
#42968=CARTESIAN_POINT ( 'NONE',  ( 0.1968503937007881344, -0.6692913385826771977, 8.415575281601705876E-17 ) ) ;
#42971=CARTESIAN_POINT ( 'NONE',  ( -0.4265091863517051496, 0.1771653543307087075, -0.09757992244046823083 ) ) ;
#42972=CARTESIAN_POINT ( 'NONE',  ( -0.1771653543307080136, 0.1660481256975883668, -0.3530559997133364547 ) ) ;
#42973=CARTESIAN_POINT ( 'NONE',  ( 0.8858267716535438430, 0.07958543189024085140, 0.2665933059059887866 ) ) ;
#42975=CARTESIAN_POINT ( 'NONE',  ( 1.325459317585302665, -0.004921259842519870586, -0.3153832671262229437 ) ) ;
#42976=CARTESIAN_POINT ( 'NONE',  ( -0.03937007874015669567, 0.2952755905511811885, 0.000000000000000000 ) ) ;
#42977=ADVANCED_FACE ( 'NONE', ( #21453 ), #24803, .F. ) ;
#42978=CARTESIAN_POINT ( 'NONE',  ( 0.9776902887139113929, -0.6692913385826773087, -0.1292274648535924053 ) ) ;
#42980=CARTESIAN_POINT ( 'NONE',  ( 0.2099737532808405305, 0.2306618581243847221, -0.2411417322834647770 ) ) ;
#42981=CARTESIAN_POINT ( 'NONE',  ( 1.259842519685040019, -0.1870078740157480879, -0.4822834645669291653 ) ) ;
#42982=CARTESIAN_POINT ( 'NONE',  ( 0.5314960629921267055, -0.5400638737290844871, 0.3530559997133364547 ) ) ;
#42984=CARTESIAN_POINT ( 'NONE',  ( 0.7874015748031503170, -0.1870078740157480601, -0.3641732283464567677 ) ) ;
#42985=CARTESIAN_POINT ( 'NONE',  ( 1.108923884514436686, -0.3162353388693409650, -0.4822834645669289433 ) ) ;
#42986=EDGE_CURVE ( 'NONE', #11874, #37974, #44233, .T. ) ;
#42987=CARTESIAN_POINT ( 'NONE',  ( 0.05905511811023681640, 0.07958543189024071263, -0.2665933059059888421 ) ) ;
#42988=CARTESIAN_POINT ( 'NONE',  ( -0.2559055118110227234, -0.5400638737290844871, 0.3530559997133364547 ) ) ;
#42989=CARTESIAN_POINT ( 'NONE',  ( 0.4855643044619428750, 0.05413385826771666132, 0.4176697321401328100 ) ) ;
#42990=CARTESIAN_POINT ( 'NONE',  ( -0.7677165354330699465, -0.5400638737290845981, -0.3530559997133363437 ) ) ;
#42991=CARTESIAN_POINT ( 'NONE',  ( -0.2230971128608915943, -0.3690944881889765550, -0.3153832671262227771 ) ) ;
#42992=CARTESIAN_POINT ( 'NONE',  ( 0.7086614173228352742, -0.1870078740157480879, -0.4822834645669291653 ) ) ;
#42993=CARTESIAN_POINT ( 'NONE',  ( 1.154855643044620184, -0.5023911411419708095, 0.1820866141732285504 ) ) ;
#42994=CARTESIAN_POINT ( 'NONE',  ( -0.006561679790025524116, -0.05778040916215560624, -0.4822834645669293319 ) ) ;
#42995=( BOUNDED_SURFACE ( )  B_SPLINE_SURFACE ( 1, 2, ( 
 ( #53949, #28287, #79662, #73335, #48056, #10189, #3453, #16512, #73758, #61523, #35026, #67022, #29120, #68665, #29934, #54788, #48464, #41343, #21978, #74165, #36261, #16093, #60690, #23212, #11004, #61930, #3869, #29528, #41738, #28705, #22807, #9766, #55191, #80898, #42155, #35437, #67850, #80079, #36663, #61102, #48882, #74582, #47640, #16927, #42567, #4273, #55598, #11837, #81724, #37490, #18956, #31165, #70724, #6329, #5098, #19373, #69889, #82943, #30765, #30347, #11422, #50110, #70300, #12652, #51337, #49702, #75807, #63165, #69073, #38313, #25261, #37077, #13078, #63988, #43373, #5503, #62765, #32002, #56016, #17744, #57661, #43782, #77041, #37899, #45023, #24, #56427, #24848, #63575, #82127, #24442, #18149, #38731, #25677, #75398, #69488, #50926, #4675, #18555, #57239, #56832, #5910, #82530, #50515, #24033, #76625, #44604, #76223, #31583, #44199, #12243, #21051, #71563, #13913, #47121, #78305, #15159, #59754, #58929, #1696, #19799, #34091, #1288, #2109, #64408, #58077, #443, #65686, #71145, #20637, #39570, #26098, #65260, #78727, #7596, #72810, #66087, #64827, #79146, #46289, #59339, #7166, #6743, #13487, #26527, #46711, #72403, #27774, #51759, #52181, #33270, #45448, #14752, #27354, #39143, #32415, #40406, #32837, #26937, #58506, #8423, #77461, #869, #53438, #20216, #21463, #14338, #77884, #45865, #52599, #71985, #39998, #8013, #33677, #53013, #29835, #10504, #28188, #60591, #61414, #74477, #54680, #10083, #66925, #42053, #15579, #2530, #34512, #29428, #55086, #47537, #74061, #28605, #53846, #80795, #47952, #73655, #23522, #80392, #74893, #36157, #35337, #3764, #79559, #61831, #61001, #4171, #40817, #60177, #21872, #67749, #73228, #66501, #8836, #41237, #34929, #22704, #15997, #29015, #2941, #48362, #9257, #54262, #41644, #55498, #42461, #67335, #3349, #79978, #22291, #16407, #23112, #9668, #35747, #48778, #81207, #16824, #68160, #49192, #30671, #75299, #11743, #56332, #50421, #24753, #31069, #62661, #75712, #4578, #31902, #82031, #12145, #24345, #42869, #76121, #51241, #50833, #18462, #82435, #50014, #17643, #37399, #18053, #44106, #69798, #56738, #5001, #43686, #30249, #57563, #69390, #37802, #63071, #68563, #63480, #17241, #76534, #5814, #5408, #10905, #31484, #57145, #82844, #83254, #18862, #43275, #25577, #25164, #44511, #68972, #36563, #23937, #70199, #12554, #38213, #63888, #62240, #6227, #55913, #81625, #49605, #11322, #36980, #59654, #27254, #32315, #26425, #343, #59239, #44922, #6643, #1599, #32736, #40308, #26839, #8326, #52913, #19693, #13811, #52497, #77361, #13391, #51657, #65988, #46609, #64309, #39044, #14235, #78627, #7494, #46188, #45350, #78206, #71047, #38631, #70619, #65581, #7915, #26000, #20537, #64728, #57978, #33576, #763, #52077, #2010, #33163, #27673, #72305, #71464, #39894, #7067, #14651, #39470, #33992, #76943, #12975, #58404, #71885, #77785, #19269, #20118, #45765, #65157, #58831, #1189, #20952, #47436, #62042, #60077, #8739, #54162, #69183, #56127, #28504, #73556, #66401, #47020, #15900, #36775, #73129, #2432, #49405, #49814, #11118, #15480, #28089, #75099, #75514, #62451, #4379, #36368, #66827, #53746, #47852, #9159, #30047, #55709, #67237, #41137, #79876, #40716, #11534, #34832, #17447, #60491, #79048, #81418, #5207, #4787, #10711, #2841, #72713, #22194, #68774, #41548, #37191, #81833, #79455, #62871, #23734, #43077, #21774, #21366, #30464, #24143, #17853, #43487, #53339, #15060, #34410, #6027, #11945, #38842, #51452, #37599, #13605, #64522, #69598, #63688, #63274, #13193, #82239, #43901, #6859, #69999, #77581, #64109, #45563, #32528, #56946, #51038, #6444, #31281, #50629, #5613, #19913, #560, #18259, #76334, #77155, #58192, #44717, #136, #82643, #32115, #24956, #75920, #24558, #19487, #45140, #18664, #57773, #44309, #12354, #70844, #38010, #31697, #39259, #70414, #64941, #26213, #25375, #51875, #57356, #71259, #76739, #30871, #56537, #50224, #83052, #25791, #19069, #12770, #38427, #52294, #1396, #72510, #65791, #78837, #27051, #14859, #14027, #45980, #8124, #21988, #8950, #33790, #27468, #20328, #985 ),
 ( #52710, #59454, #77999, #47649, #20750, #2221, #46400, #32951, #66200, #41350, #40933, #21163, #14452, #26640, #40103, #21570, #1806, #73344, #34625, #7711, #15692, #40521, #27887, #33378, #58617, #39684, #78422, #72921, #15273, #53958, #71676, #72093, #53126, #65376, #66613, #53547, #59042, #7281, #60289, #46819, #8538, #34205, #2639, #59868, #79255, #28296, #47232, #79670, #16935, #81733, #75003, #9774, #3877, #42575, #67441, #3463, #41746, #56025, #36671, #54377, #29129, #4281, #17350, #80907, #36269, #35446, #68277, #61111, #28714, #60699, #55607, #81318, #73766, #10613, #54796, #80087, #23631, #74174, #16520, #49713, #23220, #17753, #62347, #61532, #29943, #22407, #4685, #29536, #30356, #67031, #3048, #48064, #61938, #16101, #9363, #35034, #80499, #22815, #48890, #42165, #55199, #48472, #74591, #67859, #10197, #35866, #24042, #68673, #49302, #42978, #11013, #75409, #63586, #25686, #63174, #50119, #26108, #77050, #82138, #76231, #75817, #51347, #11432, #56435, #19383, #82540, #6752, #76634, #58087, #45035, #69497, #5921, #18965, #43791, #5512, #18160, #32424, #13088, #30774, #31177, #63997, #70734, #57248, #12664, #11846, #44614, #37499, #5107, #37087, #32011, #57671, #56842, #70309, #24857, #24453, #33, #50525, #18565, #51769, #82952, #77472, #38740, #37909, #6338, #44208, #64417, #31593, #452, #43382, #62773, #69898, #38324, #12252, #69084, #25270, #50937, #13923, #1706, #78316, #8024, #39580, #27362, #26538, #58515, #20646, #34521, #21472, #46300, #40007, #32846, #13496, #65694, #2118, #65269, #52191, #14760, #15171, #59764, #53022, #78736, #33279, #77895, #14347, #58940, #21059, #46719, #33687, #7605, #71994, #7175, #60188, #1298, #40416, #26947, #45458, #72411, #53856, #53447, #59348, #52609, #39152, #66097, #34102, #8433, #2539, #47130, #20225, #28197, #27784, #79155, #45874, #71155, #71572, #72821, #40827, #66512, #8845, #64837, #19809, #878, #60601, #4182, #16835, #2950, #49201, #79568, #73239, #15588, #80806, #28615, #21884, #30258, #41247, #73665, #61426, #54692, #67759, #16006, #3775, #54273, #34938, #80401, #10914, #81216, #22714, #16417, #9267, #66934, #42064, #61840, #41653, #79989, #74488, #74902, #36167, #29438, #55098, #9677, #22301, #74072, #35348, #23122, #48790, #10094, #67344, #48372, #47962, #36572, #61010, #42470, #3361, #47548, #68172, #29025, #29844, #35759, #10514, #55508, #23532, #17251, #42879, #62250, #68573, #4587, #70629, #37813, #50844, #56342, #81636, #62671, #18063, #38223, #63899, #19281, #17654, #43696, #31081, #36991, #6236, #76544, #5011, #38641, #31912, #11331, #5419, #30681, #57573, #23946, #68983, #83265, #11753, #44932, #5823, #12986, #25588, #82042, #76131, #31495, #24356, #75723, #50025, #64319, #51251, #43285, #69401, #18872, #76953, #69808, #25175, #37409, #57155, #63081, #56748, #49614, #44521, #70209, #82447, #82855, #24763, #50431, #12565, #18473, #44116, #6653, #12157, #55922, #75308, #63489, #39905, #45361, #20962, #65169, #65593, #71057, #78217, #7926, #46621, #1609, #13401, #774, #14247, #59252, #72316, #57988, #27265, #32327, #26436, #39055, #7505, #13823, #39482, #14663, #40320, #20549, #46201, #33587, #71896, #32748, #33174, #65999, #52509, #52925, #58842, #34004, #353, #8338, #59666, #26010, #71475, #64739, #78639, #7077, #51668, #77371, #19703, #58415, #52087, #77797, #20129, #45777, #1200, #26850, #44789, #18336, #11611, #30943, #6930, #5281, #38083, #32187, #49887, #77226, #45214, #18736, #64594, #69673, #44378, #63348, #82713, #25446, #70070, #43976, #75588, #19139, #38501, #64183, #70915, #5683, #19555, #32601, #56610, #13264, #43563, #31352, #69264, #37671, #58264, #37270, #57018, #38914, #6098, #24216, #57433, #76405, #82310, #12425, #17927, #12016, #76808, #31772, #6517, #24630, #63757, #62946, #50296, #210, #75994, #57843, #83126, #25033, #50706, #51111, #70485, #12842, #25863, #51523, #2292, #59106, #20814, #13676, #77650, #46469, #66264, #20399, #7349, #78906, #79319, #40583, #33855, #14518, #53193, #72163, #41004, #628, #47299, #72988, #66687, #14098, #71328, #8188, #65014 ) ),
 .UNSPECIFIED., .F., .F., .F. ) 
 B_SPLINE_SURFACE_WITH_KNOTS ( ( 2, 2 ),
 ( 3, 2, 2, 2, 2, 2, 2, 2, 2, 2, 2, 2, 2, 2, 2, 2, 2, 2, 2, 2, 2, 2, 2, 2, 2, 2, 2, 2, 2, 2, 2, 2, 2, 2, 2, 2, 2, 2, 2, 2, 2, 2, 2, 2, 2, 2, 2, 2, 2, 2, 2, 2, 2, 2, 2, 2, 2, 2, 2, 2, 2, 2, 2, 2, 2, 2, 2, 2, 2, 2, 2, 2, 2, 2, 2, 2, 2, 2, 2, 2, 2, 2, 2, 2, 2, 2, 2, 2, 2, 2, 2, 2, 2, 2, 2, 2, 2, 2, 2, 2, 2, 2, 2, 2, 2, 2, 2, 2, 2, 2, 2, 2, 2, 2, 2, 2, 2, 2, 2, 2, 2, 2, 2, 2, 2, 2, 2, 2, 2, 2, 2, 2, 2, 2, 2, 2, 2, 2, 2, 2, 2, 2, 2, 2, 2, 2, 2, 2, 2, 2, 2, 2, 2, 2, 2, 2, 2, 2, 2, 2, 2, 2, 2, 2, 2, 2, 2, 2, 2, 2, 2, 2, 2, 2, 2, 2, 2, 2, 2, 2, 2, 2, 2, 2, 2, 2, 2, 2, 2, 2, 2, 2, 2, 2, 2, 2, 2, 2, 2, 2, 2, 2, 2, 2, 2, 2, 2, 2, 2, 2, 2, 2, 2, 2, 2, 2, 2, 2, 2, 2, 2, 2, 2, 2, 2, 2, 2, 2, 2, 2, 2, 2, 2, 2, 2, 2, 2, 2, 2, 2, 2, 2, 2, 2, 2, 2, 2, 2, 2, 2, 2, 2, 2, 2, 2, 3 ),
 ( 0.000000000000000000, 1.000000000000000000 ),
 ( 0.000000000000000000, 0.003787878787878787984, 0.007575757575757575968, 0.01136363636363636395, 0.01515151515151515194, 0.01893939393939393992, 0.02272727272727272790, 0.02651515151515151589, 0.03030303030303030387, 0.03409090909090908839, 0.03787878787878787984, 0.04166666666666666435, 0.04545454545454545581, 0.04924242424242424032, 0.05303030303030303177, 0.05681818181818181629, 0.06060606060606060774, 0.06439393939393939226, 0.06818181818181817677, 0.07196969696969697516, 0.07575757575757575968, 0.07954545454545454419, 0.08333333333333332871, 0.08712121212121212710, 0.09090909090909091161, 0.09469696969696969613, 0.09848484848484848064, 0.1022727272727272790, 0.1060606060606060635, 0.1098484848484848481, 0.1136363636363636326, 0.1174242424242424310, 0.1212121212121212155, 0.1250000000000000000, 0.1287878787878787845, 0.1325757575757575690, 0.1363636363636363535, 0.1401515151515151381, 0.1439393939393939503, 0.1477272727272727348, 0.1515151515151515194, 0.1553030303030303039, 0.1590909090909090884, 0.1628787878787878729, 0.1666666666666666574, 0.1704545454545454419, 0.1742424242424242542, 0.1780303030303030387, 0.1818181818181818232, 0.1856060606060606077, 0.1893939393939393923, 0.1931818181818181768, 0.1969696969696969613, 0.2007575757575757458, 0.2045454545454545581, 0.2083333333333333426, 0.2121212121212121271, 0.2159090909090909116, 0.2196969696969696961, 0.2234848484848484806, 0.2272727272727272652, 0.2310606060606060497, 0.2348484848484848619, 0.2386363636363636465, 0.2424242424242424310, 0.2462121212121212155, 0.2500000000000000000, 0.2537878787878787845, 0.2575757575757575690, 0.2613636363636363535, 0.2651515151515151381, 0.2689393939393939226, 0.2727272727272727071, 0.2765151515151514916, 0.2803030303030302761, 0.2840909090909091161, 0.2878787878787879007, 0.2916666666666666852, 0.2954545454545454697, 0.2992424242424242542, 0.3030303030303030387, 0.3068181818181818232, 0.3106060606060606077, 0.3143939393939393923, 0.3181818181818181768, 0.3219696969696969613, 0.3257575757575757458, 0.3295454545454545303, 0.3333333333333333148, 0.3371212121212120993, 0.3409090909090908839, 0.3446969696969697239, 0.3484848484848485084, 0.3522727272727272929, 0.3560606060606060774, 0.3598484848484848619, 0.3636363636363636465, 0.3674242424242424310, 0.3712121212121212155, 0.3750000000000000000, 0.3787878787878787845, 0.3825757575757575690, 0.3863636363636363535, 0.3901515151515151381, 0.3939393939393939226, 0.3977272727272727071, 0.4015151515151514916, 0.4053030303030302761, 0.4090909090909091161, 0.4128787878787879007, 0.4166666666666666852, 0.4204545454545454697, 0.4242424242424242542, 0.4280303030303030387, 0.4318181818181818232, 0.4356060606060606077, 0.4393939393939393923, 0.4431818181818181768, 0.4469696969696969613, 0.4507575757575757458, 0.4545454545454545303, 0.4583333333333333148, 0.4621212121212120993, 0.4659090909090908839, 0.4696969696969697239, 0.4734848484848485084, 0.4772727272727272929, 0.4810606060606060774, 0.4848484848484848619, 0.4886363636363636465, 0.4924242424242424310, 0.4962121212121212155, 0.5000000000000000000, 0.5037878787878787845, 0.5075757575757575690, 0.5113636363636363535, 0.5151515151515151381, 0.5189393939393939226, 0.5227272727272727071, 0.5265151515151514916, 0.5303030303030302761, 0.5340909090909090606, 0.5378787878787878451, 0.5416666666666666297, 0.5454545454545454142, 0.5492424242424241987, 0.5530303030303029832, 0.5568181818181817677, 0.5606060606060605522, 0.5643939393939394478, 0.5681818181818182323, 0.5719696969696970168, 0.5757575757575758013, 0.5795454545454545858, 0.5833333333333333703, 0.5871212121212121549, 0.5909090909090909394, 0.5946969696969697239, 0.5984848484848485084, 0.6022727272727272929, 0.6060606060606060774, 0.6098484848484848619, 0.6136363636363636465, 0.6174242424242424310, 0.6212121212121212155, 0.6250000000000000000, 0.6287878787878787845, 0.6325757575757575690, 0.6363636363636363535, 0.6401515151515151381, 0.6439393939393939226, 0.6477272727272727071, 0.6515151515151514916, 0.6553030303030302761, 0.6590909090909090606, 0.6628787878787878451, 0.6666666666666666297, 0.6704545454545454142, 0.6742424242424241987, 0.6780303030303029832, 0.6818181818181817677, 0.6856060606060605522, 0.6893939393939394478, 0.6931818181818182323, 0.6969696969696970168, 0.7007575757575758013, 0.7045454545454545858, 0.7083333333333333703, 0.7121212121212121549, 0.7159090909090909394, 0.7196969696969697239, 0.7234848484848485084, 0.7272727272727272929, 0.7310606060606060774, 0.7348484848484848619, 0.7386363636363636465, 0.7424242424242424310, 0.7462121212121212155, 0.7500000000000000000, 0.7537878787878787845, 0.7575757575757575690, 0.7613636363636363535, 0.7651515151515151381, 0.7689393939393939226, 0.7727272727272727071, 0.7765151515151514916, 0.7803030303030302761, 0.7840909090909090606, 0.7878787878787878451, 0.7916666666666666297, 0.7954545454545454142, 0.7992424242424241987, 0.8030303030303029832, 0.8068181818181817677, 0.8106060606060605522, 0.8143939393939394478, 0.8181818181818182323, 0.8219696969696970168, 0.8257575757575758013, 0.8295454545454545858, 0.8333333333333333703, 0.8371212121212121549, 0.8409090909090909394, 0.8446969696969697239, 0.8484848484848485084, 0.8522727272727272929, 0.8560606060606060774, 0.8598484848484848619, 0.8636363636363636465, 0.8674242424242424310, 0.8712121212121212155, 0.8750000000000000000, 0.8787878787878787845, 0.8825757575757575690, 0.8863636363636363535, 0.8901515151515151381, 0.8939393939393939226, 0.8977272727272727071, 0.9015151515151514916, 0.9053030303030302761, 0.9090909090909090606, 0.9128787878787878451, 0.9166666666666666297, 0.9204545454545454142, 0.9242424242424241987, 0.9280303030303029832, 0.9318181818181817677, 0.9356060606060605522, 0.9393939393939394478, 0.9431818181818182323, 0.9469696969696970168, 0.9507575757575758013, 0.9545454545454545858, 0.9583333333333333703, 0.9621212121212121549, 0.9659090909090909394 ),
 .UNSPECIFIED. ) 
 GEOMETRIC_REPRESENTATION_ITEM ( )  RATIONAL_B_SPLINE_SURFACE ( (
 ( 1.000000000000000000, 0.9659258262890683122, 1.000000000000000000, 0.9659258262890683122, 1.000000000000000000, 0.9659258262890683122, 1.000000000000000000, 0.9659258262890683122, 1.000000000000000000, 0.9659258262890683122, 1.000000000000000000, 0.9659258262890683122, 1.000000000000000000, 0.9659258262890683122, 1.000000000000000000, 0.9659258262890683122, 1.000000000000000000, 0.9659258262890683122, 1.000000000000000000, 0.9659258262890683122, 1.000000000000000000, 0.9659258262890683122, 1.000000000000000000, 0.9659258262890683122, 1.000000000000000000, 0.9659258262890683122, 1.000000000000000000, 0.9659258262890683122, 1.000000000000000000, 0.9659258262890683122, 1.000000000000000000, 0.9659258262890683122, 1.000000000000000000, 0.9659258262890683122, 1.000000000000000000, 0.9659258262890683122, 1.000000000000000000, 0.9659258262890683122, 1.000000000000000000, 0.9659258262890683122, 1.000000000000000000, 0.9659258262890683122, 1.000000000000000000, 0.9659258262890683122, 1.000000000000000000, 0.9659258262890683122, 1.000000000000000000, 0.9659258262890683122, 1.000000000000000000, 0.9659258262890683122, 1.000000000000000000, 0.9659258262890683122, 1.000000000000000000, 0.9659258262890683122, 1.000000000000000000, 0.9659258262890683122, 1.000000000000000000, 0.9659258262890683122, 1.000000000000000000, 0.9659258262890683122, 1.000000000000000000, 0.9659258262890683122, 1.000000000000000000, 0.9659258262890683122, 1.000000000000000000, 0.9659258262890683122, 1.000000000000000000, 0.9659258262890683122, 1.000000000000000000, 0.9659258262890683122, 1.000000000000000000, 0.9659258262890683122, 1.000000000000000000, 0.9659258262890683122, 1.000000000000000000, 0.9659258262890683122, 1.000000000000000000, 0.9659258262890683122, 1.000000000000000000, 0.9659258262890683122, 1.000000000000000000, 0.9659258262890683122, 1.000000000000000000, 0.9659258262890683122, 1.000000000000000000, 0.9659258262890683122, 1.000000000000000000, 0.9659258262890683122, 1.000000000000000000, 0.9659258262890683122, 1.000000000000000000, 0.9659258262890683122, 1.000000000000000000, 0.9659258262890683122, 1.000000000000000000, 0.9659258262890683122, 1.000000000000000000, 0.9659258262890683122, 1.000000000000000000, 0.9659258262890683122, 1.000000000000000000, 0.9659258262890683122, 1.000000000000000000, 0.9659258262890683122, 1.000000000000000000, 0.9659258262890683122, 1.000000000000000000, 0.9659258262890683122, 1.000000000000000000, 0.9659258262890683122, 1.000000000000000000, 0.9659258262890683122, 1.000000000000000000, 0.9659258262890683122, 1.000000000000000000, 0.9659258262890683122, 1.000000000000000000, 0.9659258262890683122, 1.000000000000000000, 0.9659258262890683122, 1.000000000000000000, 0.9659258262890683122, 1.000000000000000000, 0.9659258262890683122, 1.000000000000000000, 0.9659258262890683122, 1.000000000000000000, 0.9659258262890683122, 1.000000000000000000, 0.9659258262890683122, 1.000000000000000000, 0.9659258262890683122, 1.000000000000000000, 0.9659258262890683122, 1.000000000000000000, 0.9659258262890683122, 1.000000000000000000, 0.9659258262890683122, 1.000000000000000000, 0.9659258262890683122, 1.000000000000000000, 0.9659258262890683122, 1.000000000000000000, 0.9659258262890683122, 1.000000000000000000, 0.9659258262890683122, 1.000000000000000000, 0.9659258262890683122, 1.000000000000000000, 0.9659258262890683122, 1.000000000000000000, 0.9659258262890683122, 1.000000000000000000, 0.9659258262890683122, 1.000000000000000000, 0.9659258262890683122, 1.000000000000000000, 0.9659258262890683122, 1.000000000000000000, 0.9659258262890683122, 1.000000000000000000, 0.9659258262890683122, 1.000000000000000000, 0.9659258262890683122, 1.000000000000000000, 0.9659258262890683122, 1.000000000000000000, 0.9659258262890683122, 1.000000000000000000, 0.9659258262890683122, 1.000000000000000000, 0.9659258262890683122, 1.000000000000000000, 0.9659258262890683122, 1.000000000000000000, 0.9659258262890683122, 1.000000000000000000, 0.9659258262890683122, 1.000000000000000000, 0.9659258262890683122, 1.000000000000000000, 0.9659258262890683122, 1.000000000000000000, 0.9659258262890683122, 1.000000000000000000, 0.9659258262890683122, 1.000000000000000000, 0.9659258262890683122, 1.000000000000000000, 0.9659258262890683122, 1.000000000000000000, 0.9659258262890683122, 1.000000000000000000, 0.9659258262890683122, 1.000000000000000000, 0.9659258262890683122, 1.000000000000000000, 0.9659258262890683122, 1.000000000000000000, 0.9659258262890683122, 1.000000000000000000, 0.9659258262890683122, 1.000000000000000000, 0.9659258262890683122, 1.000000000000000000, 0.9659258262890683122, 1.000000000000000000, 0.9659258262890683122, 1.000000000000000000, 0.9659258262890683122, 1.000000000000000000, 0.9659258262890683122, 1.000000000000000000, 0.9659258262890683122, 1.000000000000000000, 0.9659258262890683122, 1.000000000000000000, 0.9659258262890683122, 1.000000000000000000, 0.9659258262890683122, 1.000000000000000000, 0.9659258262890683122, 1.000000000000000000, 0.9659258262890683122, 1.000000000000000000, 0.9659258262890683122, 1.000000000000000000, 0.9659258262890683122, 1.000000000000000000, 0.9659258262890683122, 1.000000000000000000, 0.9659258262890683122, 1.000000000000000000, 0.9659258262890683122, 1.000000000000000000, 0.9659258262890683122, 1.000000000000000000, 0.9659258262890683122, 1.000000000000000000, 0.9659258262890683122, 1.000000000000000000, 0.9659258262890683122, 1.000000000000000000, 0.9659258262890683122, 1.000000000000000000, 0.9659258262890683122, 1.000000000000000000, 0.9659258262890683122, 1.000000000000000000, 0.9659258262890683122, 1.000000000000000000, 0.9659258262890683122, 1.000000000000000000, 0.9659258262890683122, 1.000000000000000000, 0.9659258262890683122, 1.000000000000000000, 0.9659258262890683122, 1.000000000000000000, 0.9659258262890683122, 1.000000000000000000, 0.9659258262890683122, 1.000000000000000000, 0.9659258262890683122, 1.000000000000000000, 0.9659258262890683122, 1.000000000000000000, 0.9659258262890683122, 1.000000000000000000, 0.9659258262890683122, 1.000000000000000000, 0.9659258262890683122, 1.000000000000000000, 0.9659258262890683122, 1.000000000000000000, 0.9659258262890683122, 1.000000000000000000, 0.9659258262890683122, 1.000000000000000000, 0.9659258262890683122, 1.000000000000000000, 0.9659258262890683122, 1.000000000000000000, 0.9659258262890683122, 1.000000000000000000, 0.9659258262890683122, 1.000000000000000000, 0.9659258262890683122, 1.000000000000000000, 0.9659258262890683122, 1.000000000000000000, 0.9659258262890683122, 1.000000000000000000, 0.9659258262890683122, 1.000000000000000000, 0.9659258262890683122, 1.000000000000000000, 0.9659258262890683122, 1.000000000000000000, 0.9659258262890683122, 1.000000000000000000, 0.9659258262890683122, 1.000000000000000000, 0.9659258262890683122, 1.000000000000000000, 0.9659258262890683122, 1.000000000000000000, 0.9659258262890683122, 1.000000000000000000, 0.9659258262890683122, 1.000000000000000000, 0.9659258262890683122, 1.000000000000000000, 0.9659258262890683122, 1.000000000000000000, 0.9659258262890683122, 1.000000000000000000, 0.9659258262890683122, 1.000000000000000000, 0.9659258262890683122, 1.000000000000000000, 0.9659258262890683122, 1.000000000000000000, 0.9659258262890683122, 1.000000000000000000, 0.9659258262890683122, 1.000000000000000000, 0.9659258262890683122, 1.000000000000000000, 0.9659258262890683122, 1.000000000000000000, 0.9659258262890683122, 1.000000000000000000, 0.9659258262890683122, 1.000000000000000000, 0.9659258262890683122, 1.000000000000000000, 0.9659258262890683122, 1.000000000000000000, 0.9659258262890683122, 1.000000000000000000, 0.9659258262890683122, 1.000000000000000000, 0.9659258262890683122, 1.000000000000000000, 0.9659258262890683122, 1.000000000000000000, 0.9659258262890683122, 1.000000000000000000, 0.9659258262890683122, 1.000000000000000000, 0.9659258262890683122, 1.000000000000000000, 0.9659258262890683122, 1.000000000000000000, 0.9659258262890683122, 1.000000000000000000, 0.9659258262890683122, 1.000000000000000000, 0.9659258262890683122, 1.000000000000000000, 0.9659258262890683122, 1.000000000000000000, 0.9659258262890683122, 1.000000000000000000, 0.9659258262890683122, 1.000000000000000000, 0.9659258262890683122, 1.000000000000000000, 0.9659258262890683122, 1.000000000000000000, 0.9659258262890683122, 1.000000000000000000, 0.9659258262890683122, 1.000000000000000000, 0.9659258262890683122, 1.000000000000000000, 0.9659258262890683122, 1.000000000000000000, 0.9659258262890683122, 1.000000000000000000, 0.9659258262890683122, 1.000000000000000000, 0.9659258262890683122, 1.000000000000000000, 0.9659258262890683122, 1.000000000000000000, 0.9659258262890683122, 1.000000000000000000, 0.9659258262890683122, 1.000000000000000000, 0.9659258262890683122, 1.000000000000000000, 0.9659258262890683122, 1.000000000000000000, 0.9659258262890683122, 1.000000000000000000, 0.9659258262890683122, 1.000000000000000000, 0.9659258262890683122, 1.000000000000000000, 0.9659258262890683122, 1.000000000000000000, 0.9659258262890683122, 1.000000000000000000, 0.9659258262890683122, 1.000000000000000000, 0.9659258262890683122, 1.000000000000000000, 0.9659258262890683122, 1.000000000000000000, 0.9659258262890683122, 1.000000000000000000, 0.9659258262890683122, 1.000000000000000000, 0.9659258262890683122, 1.000000000000000000, 0.9659258262890683122, 1.000000000000000000, 0.9659258262890683122, 1.000000000000000000, 0.9659258262890683122, 1.000000000000000000, 0.9659258262890683122, 1.000000000000000000, 0.9659258262890683122, 1.000000000000000000, 0.9659258262890683122, 1.000000000000000000, 0.9659258262890683122, 1.000000000000000000, 0.9659258262890683122, 1.000000000000000000, 0.9659258262890683122, 1.000000000000000000, 0.9659258262890683122, 1.000000000000000000, 0.9659258262890683122, 1.000000000000000000, 0.9659258262890683122, 1.000000000000000000, 0.9659258262890683122, 1.000000000000000000, 0.9659258262890683122, 1.000000000000000000, 0.9659258262890683122, 1.000000000000000000, 0.9659258262890683122, 1.000000000000000000, 0.9659258262890683122, 1.000000000000000000, 0.9659258262890683122, 1.000000000000000000, 0.9659258262890683122, 1.000000000000000000, 0.9659258262890683122, 1.000000000000000000, 0.9659258262890683122, 1.000000000000000000, 0.9659258262890683122, 1.000000000000000000, 0.9659258262890683122, 1.000000000000000000, 0.9659258262890683122, 1.000000000000000000, 0.9659258262890683122, 1.000000000000000000, 0.9659258262890683122, 1.000000000000000000, 0.9659258262890683122, 1.000000000000000000, 0.9659258262890683122, 1.000000000000000000, 0.9659258262890683122, 1.000000000000000000, 0.9659258262890683122, 1.000000000000000000, 0.9659258262890683122, 1.000000000000000000, 0.9659258262890683122, 1.000000000000000000, 0.9659258262890683122, 1.000000000000000000, 0.9659258262890683122, 1.000000000000000000, 0.9659258262890683122, 1.000000000000000000, 0.9659258262890683122, 1.000000000000000000, 0.9659258262890683122, 1.000000000000000000, 0.9659258262890683122, 1.000000000000000000, 0.9659258262890683122, 1.000000000000000000, 0.9659258262890683122, 1.000000000000000000, 0.9659258262890683122, 1.000000000000000000, 0.9659258262890683122, 1.000000000000000000, 0.9659258262890683122, 1.000000000000000000, 0.9659258262890683122, 1.000000000000000000, 0.9659258262890683122, 1.000000000000000000, 0.9659258262890683122, 1.000000000000000000, 0.9659258262890683122, 1.000000000000000000),
 ( 1.000000000000000000, 0.9659258262890683122, 1.000000000000000000, 0.9659258262890683122, 1.000000000000000000, 0.9659258262890683122, 1.000000000000000000, 0.9659258262890683122, 1.000000000000000000, 0.9659258262890683122, 1.000000000000000000, 0.9659258262890683122, 1.000000000000000000, 0.9659258262890683122, 1.000000000000000000, 0.9659258262890683122, 1.000000000000000000, 0.9659258262890683122, 1.000000000000000000, 0.9659258262890683122, 1.000000000000000000, 0.9659258262890683122, 1.000000000000000000, 0.9659258262890683122, 1.000000000000000000, 0.9659258262890683122, 1.000000000000000000, 0.9659258262890683122, 1.000000000000000000, 0.9659258262890683122, 1.000000000000000000, 0.9659258262890683122, 1.000000000000000000, 0.9659258262890683122, 1.000000000000000000, 0.9659258262890683122, 1.000000000000000000, 0.9659258262890683122, 1.000000000000000000, 0.9659258262890683122, 1.000000000000000000, 0.9659258262890683122, 1.000000000000000000, 0.9659258262890683122, 1.000000000000000000, 0.9659258262890683122, 1.000000000000000000, 0.9659258262890683122, 1.000000000000000000, 0.9659258262890683122, 1.000000000000000000, 0.9659258262890683122, 1.000000000000000000, 0.9659258262890683122, 1.000000000000000000, 0.9659258262890683122, 1.000000000000000000, 0.9659258262890683122, 1.000000000000000000, 0.9659258262890683122, 1.000000000000000000, 0.9659258262890683122, 1.000000000000000000, 0.9659258262890683122, 1.000000000000000000, 0.9659258262890683122, 1.000000000000000000, 0.9659258262890683122, 1.000000000000000000, 0.9659258262890683122, 1.000000000000000000, 0.9659258262890683122, 1.000000000000000000, 0.9659258262890683122, 1.000000000000000000, 0.9659258262890683122, 1.000000000000000000, 0.9659258262890683122, 1.000000000000000000, 0.9659258262890683122, 1.000000000000000000, 0.9659258262890683122, 1.000000000000000000, 0.9659258262890683122, 1.000000000000000000, 0.9659258262890683122, 1.000000000000000000, 0.9659258262890683122, 1.000000000000000000, 0.9659258262890683122, 1.000000000000000000, 0.9659258262890683122, 1.000000000000000000, 0.9659258262890683122, 1.000000000000000000, 0.9659258262890683122, 1.000000000000000000, 0.9659258262890683122, 1.000000000000000000, 0.9659258262890683122, 1.000000000000000000, 0.9659258262890683122, 1.000000000000000000, 0.9659258262890683122, 1.000000000000000000, 0.9659258262890683122, 1.000000000000000000, 0.9659258262890683122, 1.000000000000000000, 0.9659258262890683122, 1.000000000000000000, 0.9659258262890683122, 1.000000000000000000, 0.9659258262890683122, 1.000000000000000000, 0.9659258262890683122, 1.000000000000000000, 0.9659258262890683122, 1.000000000000000000, 0.9659258262890683122, 1.000000000000000000, 0.9659258262890683122, 1.000000000000000000, 0.9659258262890683122, 1.000000000000000000, 0.9659258262890683122, 1.000000000000000000, 0.9659258262890683122, 1.000000000000000000, 0.9659258262890683122, 1.000000000000000000, 0.9659258262890683122, 1.000000000000000000, 0.9659258262890683122, 1.000000000000000000, 0.9659258262890683122, 1.000000000000000000, 0.9659258262890683122, 1.000000000000000000, 0.9659258262890683122, 1.000000000000000000, 0.9659258262890683122, 1.000000000000000000, 0.9659258262890683122, 1.000000000000000000, 0.9659258262890683122, 1.000000000000000000, 0.9659258262890683122, 1.000000000000000000, 0.9659258262890683122, 1.000000000000000000, 0.9659258262890683122, 1.000000000000000000, 0.9659258262890683122, 1.000000000000000000, 0.9659258262890683122, 1.000000000000000000, 0.9659258262890683122, 1.000000000000000000, 0.9659258262890683122, 1.000000000000000000, 0.9659258262890683122, 1.000000000000000000, 0.9659258262890683122, 1.000000000000000000, 0.9659258262890683122, 1.000000000000000000, 0.9659258262890683122, 1.000000000000000000, 0.9659258262890683122, 1.000000000000000000, 0.9659258262890683122, 1.000000000000000000, 0.9659258262890683122, 1.000000000000000000, 0.9659258262890683122, 1.000000000000000000, 0.9659258262890683122, 1.000000000000000000, 0.9659258262890683122, 1.000000000000000000, 0.9659258262890683122, 1.000000000000000000, 0.9659258262890683122, 1.000000000000000000, 0.9659258262890683122, 1.000000000000000000, 0.9659258262890683122, 1.000000000000000000, 0.9659258262890683122, 1.000000000000000000, 0.9659258262890683122, 1.000000000000000000, 0.9659258262890683122, 1.000000000000000000, 0.9659258262890683122, 1.000000000000000000, 0.9659258262890683122, 1.000000000000000000, 0.9659258262890683122, 1.000000000000000000, 0.9659258262890683122, 1.000000000000000000, 0.9659258262890683122, 1.000000000000000000, 0.9659258262890683122, 1.000000000000000000, 0.9659258262890683122, 1.000000000000000000, 0.9659258262890683122, 1.000000000000000000, 0.9659258262890683122, 1.000000000000000000, 0.9659258262890683122, 1.000000000000000000, 0.9659258262890683122, 1.000000000000000000, 0.9659258262890683122, 1.000000000000000000, 0.9659258262890683122, 1.000000000000000000, 0.9659258262890683122, 1.000000000000000000, 0.9659258262890683122, 1.000000000000000000, 0.9659258262890683122, 1.000000000000000000, 0.9659258262890683122, 1.000000000000000000, 0.9659258262890683122, 1.000000000000000000, 0.9659258262890683122, 1.000000000000000000, 0.9659258262890683122, 1.000000000000000000, 0.9659258262890683122, 1.000000000000000000, 0.9659258262890683122, 1.000000000000000000, 0.9659258262890683122, 1.000000000000000000, 0.9659258262890683122, 1.000000000000000000, 0.9659258262890683122, 1.000000000000000000, 0.9659258262890683122, 1.000000000000000000, 0.9659258262890683122, 1.000000000000000000, 0.9659258262890683122, 1.000000000000000000, 0.9659258262890683122, 1.000000000000000000, 0.9659258262890683122, 1.000000000000000000, 0.9659258262890683122, 1.000000000000000000, 0.9659258262890683122, 1.000000000000000000, 0.9659258262890683122, 1.000000000000000000, 0.9659258262890683122, 1.000000000000000000, 0.9659258262890683122, 1.000000000000000000, 0.9659258262890683122, 1.000000000000000000, 0.9659258262890683122, 1.000000000000000000, 0.9659258262890683122, 1.000000000000000000, 0.9659258262890683122, 1.000000000000000000, 0.9659258262890683122, 1.000000000000000000, 0.9659258262890683122, 1.000000000000000000, 0.9659258262890683122, 1.000000000000000000, 0.9659258262890683122, 1.000000000000000000, 0.9659258262890683122, 1.000000000000000000, 0.9659258262890683122, 1.000000000000000000, 0.9659258262890683122, 1.000000000000000000, 0.9659258262890683122, 1.000000000000000000, 0.9659258262890683122, 1.000000000000000000, 0.9659258262890683122, 1.000000000000000000, 0.9659258262890683122, 1.000000000000000000, 0.9659258262890683122, 1.000000000000000000, 0.9659258262890683122, 1.000000000000000000, 0.9659258262890683122, 1.000000000000000000, 0.9659258262890683122, 1.000000000000000000, 0.9659258262890683122, 1.000000000000000000, 0.9659258262890683122, 1.000000000000000000, 0.9659258262890683122, 1.000000000000000000, 0.9659258262890683122, 1.000000000000000000, 0.9659258262890683122, 1.000000000000000000, 0.9659258262890683122, 1.000000000000000000, 0.9659258262890683122, 1.000000000000000000, 0.9659258262890683122, 1.000000000000000000, 0.9659258262890683122, 1.000000000000000000, 0.9659258262890683122, 1.000000000000000000, 0.9659258262890683122, 1.000000000000000000, 0.9659258262890683122, 1.000000000000000000, 0.9659258262890683122, 1.000000000000000000, 0.9659258262890683122, 1.000000000000000000, 0.9659258262890683122, 1.000000000000000000, 0.9659258262890683122, 1.000000000000000000, 0.9659258262890683122, 1.000000000000000000, 0.9659258262890683122, 1.000000000000000000, 0.9659258262890683122, 1.000000000000000000, 0.9659258262890683122, 1.000000000000000000, 0.9659258262890683122, 1.000000000000000000, 0.9659258262890683122, 1.000000000000000000, 0.9659258262890683122, 1.000000000000000000, 0.9659258262890683122, 1.000000000000000000, 0.9659258262890683122, 1.000000000000000000, 0.9659258262890683122, 1.000000000000000000, 0.9659258262890683122, 1.000000000000000000, 0.9659258262890683122, 1.000000000000000000, 0.9659258262890683122, 1.000000000000000000, 0.9659258262890683122, 1.000000000000000000, 0.9659258262890683122, 1.000000000000000000, 0.9659258262890683122, 1.000000000000000000, 0.9659258262890683122, 1.000000000000000000, 0.9659258262890683122, 1.000000000000000000, 0.9659258262890683122, 1.000000000000000000, 0.9659258262890683122, 1.000000000000000000, 0.9659258262890683122, 1.000000000000000000, 0.9659258262890683122, 1.000000000000000000, 0.9659258262890683122, 1.000000000000000000, 0.9659258262890683122, 1.000000000000000000, 0.9659258262890683122, 1.000000000000000000, 0.9659258262890683122, 1.000000000000000000, 0.9659258262890683122, 1.000000000000000000, 0.9659258262890683122, 1.000000000000000000, 0.9659258262890683122, 1.000000000000000000, 0.9659258262890683122, 1.000000000000000000, 0.9659258262890683122, 1.000000000000000000, 0.9659258262890683122, 1.000000000000000000, 0.9659258262890683122, 1.000000000000000000, 0.9659258262890683122, 1.000000000000000000, 0.9659258262890683122, 1.000000000000000000, 0.9659258262890683122, 1.000000000000000000, 0.9659258262890683122, 1.000000000000000000, 0.9659258262890683122, 1.000000000000000000, 0.9659258262890683122, 1.000000000000000000, 0.9659258262890683122, 1.000000000000000000, 0.9659258262890683122, 1.000000000000000000, 0.9659258262890683122, 1.000000000000000000, 0.9659258262890683122, 1.000000000000000000, 0.9659258262890683122, 1.000000000000000000, 0.9659258262890683122, 1.000000000000000000, 0.9659258262890683122, 1.000000000000000000, 0.9659258262890683122, 1.000000000000000000, 0.9659258262890683122, 1.000000000000000000, 0.9659258262890683122, 1.000000000000000000, 0.9659258262890683122, 1.000000000000000000, 0.9659258262890683122, 1.000000000000000000, 0.9659258262890683122, 1.000000000000000000, 0.9659258262890683122, 1.000000000000000000, 0.9659258262890683122, 1.000000000000000000, 0.9659258262890683122, 1.000000000000000000, 0.9659258262890683122, 1.000000000000000000, 0.9659258262890683122, 1.000000000000000000, 0.9659258262890683122, 1.000000000000000000, 0.9659258262890683122, 1.000000000000000000, 0.9659258262890683122, 1.000000000000000000, 0.9659258262890683122, 1.000000000000000000, 0.9659258262890683122, 1.000000000000000000, 0.9659258262890683122, 1.000000000000000000, 0.9659258262890683122, 1.000000000000000000, 0.9659258262890683122, 1.000000000000000000, 0.9659258262890683122, 1.000000000000000000, 0.9659258262890683122, 1.000000000000000000, 0.9659258262890683122, 1.000000000000000000, 0.9659258262890683122, 1.000000000000000000, 0.9659258262890683122, 1.000000000000000000, 0.9659258262890683122, 1.000000000000000000, 0.9659258262890683122, 1.000000000000000000, 0.9659258262890683122, 1.000000000000000000, 0.9659258262890683122, 1.000000000000000000, 0.9659258262890683122, 1.000000000000000000, 0.9659258262890683122, 1.000000000000000000, 0.9659258262890683122, 1.000000000000000000, 0.9659258262890683122, 1.000000000000000000, 0.9659258262890683122, 1.000000000000000000, 0.9659258262890683122, 1.000000000000000000, 0.9659258262890683122, 1.000000000000000000, 0.9659258262890683122, 1.000000000000000000, 0.9659258262890683122, 1.000000000000000000, 0.9659258262890683122, 1.000000000000000000, 0.9659258262890683122, 1.000000000000000000, 0.9659258262890683122, 1.000000000000000000, 0.9659258262890683122, 1.000000000000000000, 0.9659258262890683122, 1.000000000000000000) ) ) 
 REPRESENTATION_ITEM ( '' )  SURFACE ( )  );
#42996=EDGE_CURVE ( 'NONE', #19860, #69770, #17454, .T. ) ;
#43001=CARTESIAN_POINT ( 'NONE',  ( -1.437007874015747477, 0.1660481256975883668, -0.3530559997133364547 ) ) ;
#43002=CARTESIAN_POINT ( 'NONE',  ( -0.2887139107611542133, 0.2306618581243848609, 0.2411417322834645549 ) ) ;
#43006=CARTESIAN_POINT ( 'NONE',  ( 0.3477690288713918276, -0.5511811023622048555, -0.09757992244046775898 ) ) ;
#43008=CARTESIAN_POINT ( 'NONE',  ( 0.6430446194225728496, 0.05413385826771666132, 0.4176697321401328100 ) ) ;
#43011=CARTESIAN_POINT ( 'NONE',  ( -1.679790026246718693, 0.1283753931104746893, -0.1820866141732285504 ) ) ;
#43012=CARTESIAN_POINT ( 'NONE',  ( 1.338582677165355062, -0.1870078740157479769, 0.4822834645669291653 ) ) ;
#43013=CARTESIAN_POINT ( 'NONE',  ( 1.161417322834646271, 0.07958543189024071263, -0.2665933059059888421 ) ) ;
#43014=CARTESIAN_POINT ( 'NONE',  ( 0.5314960629921267055, -0.5400638737290844871, 0.3530559997133364547 ) ) ;
#43017=CARTESIAN_POINT ( 'NONE',  ( -0.1968503937007867743, 0.2952755905511811885, 0.000000000000000000 ) ) ;
#43018=CARTESIAN_POINT ( 'NONE',  ( -1.043307086614172707, 0.07958543189024071263, -0.2665933059059888421 ) ) ;
#43019=CARTESIAN_POINT ( 'NONE',  ( 0.2493438320209980519, -0.4281496062992127816, -0.4176697321401328100 ) ) ;
#43020=CARTESIAN_POINT ( 'NONE',  ( -0.09842519685039295696, 0.1660481256975883668, -0.3530559997133364547 ) ) ;
#43022=CARTESIAN_POINT ( 'NONE',  ( 0.6406204526026253454, -2.592014407703319119E-15, 0.4118477457932993580 ) ) ;
#43024=CARTESIAN_POINT ( 'NONE',  ( 0.3937007874015754361, -0.1870078740157479769, 0.4822834645669291653 ) ) ;
#43025=CARTESIAN_POINT ( 'NONE',  ( -0.4396325459317579898, 0.2952755905511811885, 0.1292274648535926551 ) ) ;
#43026=CARTESIAN_POINT ( 'NONE',  ( -1.286089238845143479, 0.2306618581243847221, -0.2411417322834647770 ) ) ;
#43027=CARTESIAN_POINT ( 'NONE',  ( 1.213910761154856299, -0.6692913385826773087, -0.1292274648535924053 ) ) ;
#43028=CARTESIAN_POINT ( 'NONE',  ( 0.3608923884514443348, -0.6692913385826771977, 0.1292274648535927661 ) ) ;
#43030=CARTESIAN_POINT ( 'NONE',  ( -0.9251968503937002541, 0.1660481256975885056, 0.3530559997133364547 ) ) ;
#43031=CARTESIAN_POINT ( 'NONE',  ( 0.4396325459317593221, 0.2952755905511810774, -0.1292274648535930714 ) ) ;
#43032=CARTESIAN_POINT ( 'NONE',  ( -0.4133858267716528645, -0.5400638737290844871, 0.3530559997133364547 ) ) ;
#43033=CARTESIAN_POINT ( 'NONE',  ( 0.4133858267716541968, 0.07958543189024085140, 0.2665933059059887866 ) ) ;
#43034=CARTESIAN_POINT ( 'NONE',  ( -1.686351706036744558, 0.2952755905511810774, -0.1292274648535930714 ) ) ;
#43035=LINE ( 'NONE', #60344, #55725 ) ;
#43036=CARTESIAN_POINT ( 'NONE',  ( 0.2230971128608929543, 0.05413385826771626580, -0.4176697321401330321 ) ) ;
#43038=CARTESIAN_POINT ( 'NONE',  ( 1.404199475065617264, -0.4281496062992124485, 0.4176697321401328655 ) ) ;
#43042=CARTESIAN_POINT ( 'NONE',  ( 0.7742782152230979209, 0.05413385826771626580, -0.4176697321401330321 ) ) ;
#43043=CARTESIAN_POINT ( 'NONE',  ( 0.09842519685039434474, -0.4536011799217368745, -0.2665933059059886201 ) ) ;
#43044=DIRECTION ( 'NONE',  ( 0.000000000000000000, -1.000000000000000000, 0.000000000000000000 ) ) ;
#43045=DIRECTION ( 'NONE',  ( 1.000000000000000000, 0.000000000000000000, 0.000000000000000000 ) ) ;
#43047=CARTESIAN_POINT ( 'NONE',  ( -0.9563780557770518165, -3.764720552277026557E-15, -0.3791475997938235643 ) ) ;
#43048=ADVANCED_FACE ( 'NONE', ( #68781 ), #22509, .F. ) ;
#43050=CARTESIAN_POINT ( 'NONE',  ( 0.4658792650918640033, -0.3162353388693405765, 0.4822834645669290543 ) ) ;
#43051=CARTESIAN_POINT ( 'NONE',  ( -0.6496062992125976043, 0.1660481256975883668, -0.3530559997133364547 ) ) ;
#43052=CARTESIAN_POINT ( 'NONE',  ( -0.9317585301837263412, 0.05413385826771666132, 0.4176697321401328100 ) ) ;
#43053=CARTESIAN_POINT ( 'NONE',  ( 0.6824146981627303710, 0.2306618581243847221, -0.2411417322834647770 ) ) ;
#43054=CARTESIAN_POINT ( 'NONE',  ( 1.430446194225722500, 0.05413385826771666132, 0.4176697321401328100 ) ) ;
#43055=CARTESIAN_POINT ( 'NONE',  ( 1.167979002624672580, -0.3690944881889763329, 0.3153832671262228327 ) ) ;
#43056=CARTESIAN_POINT ( 'NONE',  ( 1.095800524934383846, -0.08942795157528024563, -0.3641732283464568787 ) ) ;
#43057=CARTESIAN_POINT ( 'NONE',  ( -0.6692913385826764205, 0.2952755905511811885, 0.000000000000000000 ) ) ;
#43059=CARTESIAN_POINT ( 'NONE',  ( 1.528871391076116026, 0.2952755905511811885, 0.1292274648535926551 ) ) ;
#43061=CARTESIAN_POINT ( 'NONE',  ( -0.2427821522309703550, -0.3162353388693405765, 0.4822834645669290543 ) ) ;
#43062=CARTESIAN_POINT ( 'NONE',  ( 0.9776902887139113929, -0.6692913385826773087, -0.1292274648535924053 ) ) ;
#43063=DIRECTION ( 'NONE',  ( 1.000000000000000000, 0.000000000000000000, 0.000000000000000000 ) ) ;
#43064=CARTESIAN_POINT ( 'NONE',  ( -1.200787401574802349, 0.07958543189024071263, -0.2665933059059888421 ) ) ;
#43065=CARTESIAN_POINT ( 'NONE',  ( 0.3543307086614181922, -0.6692913385826771977, 8.415575281601705876E-17 ) ) ;
#43066=CARTESIAN_POINT ( 'NONE',  ( 1.023622047244095112, -0.1870078740157480601, -0.3641732283464567677 ) ) ;
#43068=CARTESIAN_POINT ( 'NONE',  ( -1.227034120734907585, 0.1771653543307087630, 0.09757992244046791164 ) ) ;
#43069=CARTESIAN_POINT ( 'NONE',  ( 0.7742782152230979209, 0.05413385826771626580, -0.4176697321401330321 ) ) ;
#43071=CARTESIAN_POINT ( 'NONE',  ( -0.3871391076115479057, -0.2845877964562161244, -0.3641732283464567121 ) ) ;
#43072=CARTESIAN_POINT ( 'NONE',  ( -0.2362204724409442680, -0.1870078740157480879, -0.4822834645669291653 ) ) ;
#43073=CARTESIAN_POINT ( 'NONE',  ( -1.200787401574802349, -0.4536011799217367080, 0.2665933059059888421 ) ) ;
#43074=CARTESIAN_POINT ( 'NONE',  ( -0.7939632545931754048, -0.3162353388693405765, 0.4822834645669290543 ) ) ;
#43075=CARTESIAN_POINT ( 'NONE',  ( 1.358267716535433323, 0.1660481256975885056, 0.3530559997133364547 ) ) ;
#43077=CARTESIAN_POINT ( 'NONE',  ( -1.069553805774277722, -0.5511811023622048555, -0.09757992244046775898 ) ) ;
#43079=CARTESIAN_POINT ( 'NONE',  ( 1.351706036745407458, -0.4281496062992127816, -0.4176697321401328100 ) ) ;
#43081=CARTESIAN_POINT ( 'NONE',  ( -1.292650918635170010, -0.6692913385826771977, 0.1292274648535927661 ) ) ;
#43082=CARTESIAN_POINT ( 'NONE',  ( -1.292650918635170010, 0.1771653543307087075, -0.09757992244046823083 ) ) ;
#43083=CARTESIAN_POINT ( 'NONE',  ( -0.4396325459317579898, 0.1771653543307087630, 0.09757992244046791164 ) ) ;
#43084=CARTESIAN_POINT ( 'NONE',  ( -1.607611548556429737, 0.2952755905511810774, -0.1292274648535930714 ) ) ;
#43085=CARTESIAN_POINT ( 'NONE',  ( 0.04593175853018440641, -0.6692913385826771977, 0.1292274648535927661 ) ) ;
#43086=CARTESIAN_POINT ( 'NONE',  ( 0.08530183727034192087, -0.08942795157527998196, 0.3641732283464567121 ) ) ;
#43087=CARTESIAN_POINT ( 'NONE',  ( -1.207349081364828880, 0.1283753931104746893, -0.1820866141732285504 ) ) ;
#43088=CARTESIAN_POINT ( 'NONE',  ( -1.397637795275589623, 0.1660481256975885056, 0.3530559997133364547 ) ) ;
#43089=CARTESIAN_POINT ( 'NONE',  ( 1.207349081364829990, -0.5023911411419708095, -0.1820866141732282451 ) ) ;
#43090=CARTESIAN_POINT ( 'NONE',  ( 1.017060367454068803, -0.3162353388693405765, 0.4822834645669290543 ) ) ;
#43091=CARTESIAN_POINT ( 'NONE',  ( -1.595398199321657939, 0.4829664696085548825, -0.1559797534342468039 ) ) ;
#43092=CARTESIAN_POINT ( 'NONE',  ( 0.6233595800524942554, -0.08942795157528024563, -0.3641732283464568787 ) ) ;
#43093=CARTESIAN_POINT ( 'NONE',  ( 0.9383202099737538715, -0.05778040916215560624, -0.4822834645669293319 ) ) ;
#43095=CARTESIAN_POINT ( 'NONE',  ( 1.069553805774278610, -0.5511811023622046335, 0.09757992244046803654 ) ) ;
#43097=CARTESIAN_POINT ( 'NONE',  ( -1.095800524934382292, -0.3162353388693409650, -0.4822834645669289433 ) ) ;
#43098=CARTESIAN_POINT ( 'NONE',  ( -0.8333333333333323711, 0.2952755905511811885, 0.1292274648535926551 ) ) ;
#43099=CARTESIAN_POINT ( 'NONE',  ( -0.1246719160104980823, 0.2952755905511811885, 0.1292274648535926551 ) ) ;
#43100=CARTESIAN_POINT ( 'NONE',  ( 0.5396849562100397568, 1.809133623825372073E-16, -0.3791483426435173776 ) ) ;
#43102=CARTESIAN_POINT ( 'NONE',  ( 0.6627296587926515548, 0.2952755905511811885, 0.1292274648535926551 ) ) ;
#43103=CARTESIAN_POINT ( 'NONE',  ( 1.312335958005249825, 0.1283753931104746893, -0.1820866141732285504 ) ) ;
#43104=CARTESIAN_POINT ( 'NONE',  ( -0.05905511811023545637, 0.1660481256975885056, 0.3530559997133364547 ) ) ;
#43105=CARTESIAN_POINT ( 'NONE',  ( 0.7874015748031503170, -0.1870078740157479769, 0.4822834645669291653 ) ) ;
#43109=CARTESIAN_POINT ( 'NONE',  ( 0.4037097067573611753, 1.223219560026271499E-15, 0.4445507791589056734 ) ) ;
#43111=CARTESIAN_POINT ( 'NONE',  ( -0.6036745406824141069, 0.1283753931104748280, 0.1820866141732283561 ) ) ;
#43112=CARTESIAN_POINT ( 'NONE',  ( -0.8989501312335946848, 0.2952755905511810774, -0.1292274648535930714 ) ) ;
#43113=CARTESIAN_POINT ( 'NONE',  ( 0.5380577427821529035, 0.05413385826771626580, -0.4176697321401330321 ) ) ;
#43115=CARTESIAN_POINT ( 'NONE',  ( 0.9645669291338591078, -0.5400638737290845981, -0.3530559997133363437 ) ) ;
#43116=CARTESIAN_POINT ( 'NONE',  ( -1.476377952755905110, 0.1660481256975885056, 0.3530559997133364547 ) ) ;
#43117=CARTESIAN_POINT ( 'NONE',  ( 1.384514435695538337, -0.6692913385826771977, 0.1292274648535927661 ) ) ;
#43121=CARTESIAN_POINT ( 'NONE',  ( 0.9514435695538062676, -0.05778040916215522460, 0.4822834645669289988 ) ) ;
#43122=CARTESIAN_POINT ( 'NONE',  ( 0.5446194225721792126, -0.05778040916215560624, -0.4822834645669293319 ) ) ;
#43123=CARTESIAN_POINT ( 'NONE',  ( 1.181102362204724976, -0.1870078740157480601, -0.3641732283464567677 ) ) ;
#43124=CARTESIAN_POINT ( 'NONE',  ( 1.646981627296588035, -0.3162353388693405765, 0.4822834645669290543 ) ) ;
#43125=CARTESIAN_POINT ( 'NONE',  ( 1.541994750656168645, -0.6692913385826771977, 0.1292274648535927661 ) ) ;
#43127=CARTESIAN_POINT ( 'NONE',  ( 0.7414698162729663755, 0.2952755905511811885, 0.1292274648535926551 ) ) ;
#43128=CARTESIAN_POINT ( 'NONE',  ( 1.640419947506562393, -0.3690944881889763329, 0.3153832671262228327 ) ) ;
#43129=CARTESIAN_POINT ( 'NONE',  ( -0.7086614173228339419, -0.1870078740157480879, -0.4822834645669291653 ) ) ;
#43130=CARTESIAN_POINT ( 'NONE',  ( -0.4593175853018366950, 0.05413385826771666132, 0.4176697321401328100 ) ) ;
#43132=CARTESIAN_POINT ( 'NONE',  ( 1.548556430446194954, -0.6046776061558807314, 0.2411417322834647770 ) ) ;
#43133=B_SPLINE_CURVE_WITH_KNOTS ( 'NONE', 3,
 ( #63356, #4053, #30130, #30951 ),
 .UNSPECIFIED., .F., .F.,
 ( 4, 4 ),
 ( 3.210432057656183116E-07, 0.001287787053612145412 ),
 .UNSPECIFIED. ) ;
#43137=CARTESIAN_POINT ( 'NONE',  ( -1.456692913385826182, 0.1771653543307087630, 0.000000000000000000 ) ) ;
#43140=VERTEX_POINT ( 'NONE', #36783 ) ;
#43142=CARTESIAN_POINT ( 'NONE',  ( 1.587926509186352142, -0.004921259842519576551, 0.3153832671262227771 ) ) ;
#43144=CARTESIAN_POINT ( 'NONE',  ( 0.5636006452641431075, 3.421639014772782816E-16, 0.3464511005275203726 ) ) ;
#43149=CARTESIAN_POINT ( 'NONE',  ( -0.6102362204724400829, -0.4536011799217368745, -0.2665933059059886201 ) ) ;
#43150=CARTESIAN_POINT ( 'NONE',  ( -1.345144356955379816, -0.08942795157528024563, -0.3641732283464568787 ) ) ;
#43151=CARTESIAN_POINT ( 'NONE',  ( 0.7217847769028878924, -0.4281496062992127816, -0.4176697321401328100 ) ) ;
#43152=CARTESIAN_POINT ( 'NONE',  ( -1.259842519685038686, -0.1870078740157480879, -0.4822834645669291653 ) ) ;
#43155=VERTEX_POINT ( 'NONE', #29644 ) ;
#43156=CARTESIAN_POINT ( 'NONE',  ( 1.587926509186352142, 0.05413385826771666132, 0.4176697321401328100 ) ) ;
#43161=CARTESIAN_POINT ( 'NONE',  ( -0.5971128608923877978, -0.6692913385826773087, -0.1292274648535924053 ) ) ;
#43162=CARTESIAN_POINT ( 'NONE',  ( 0.8202099737532814183, -0.6692913385826773087, -0.1292274648535924053 ) ) ;
#43165=CARTESIAN_POINT ( 'NONE',  ( 1.646981627296588035, -0.3162353388693405765, 0.4822834645669290543 ) ) ;
#43166=CARTESIAN_POINT ( 'NONE',  ( -1.122047244094487306, -0.5400638737290844871, 0.3530559997133364547 ) ) ;
#43168=CARTESIAN_POINT ( 'NONE',  ( 0.2099737532808405305, 0.1283753931104746893, -0.1820866141732285504 ) ) ;
#43170=CARTESIAN_POINT ( 'NONE',  ( 8.195543980992789655E-16, -0.1870078740157480601, -0.3641732283464567677 ) ) ;
#43171=CARTESIAN_POINT ( 'NONE',  ( 0.4330708661417329575, -0.5511811023622047445, 6.969142054262312111E-17 ) ) ;
#43172=CARTESIAN_POINT ( 'NONE',  ( 0.5971128608923890191, -0.6692913385826771977, 0.1292274648535927661 ) ) ;
#43173=CARTESIAN_POINT ( 'NONE',  ( -0.6299212598425188991, -0.1870078740157480601, -0.3641732283464567677 ) ) ;
#43175=CARTESIAN_POINT ( 'NONE',  ( 1.502624671916010790, -0.3162353388693409650, -0.4822834645669289433 ) ) ;
#43176=CARTESIAN_POINT ( 'NONE',  ( -1.036745406824146176, -0.4281496062992124485, 0.4176697321401328655 ) ) ;
#43178=CARTESIAN_POINT ( 'NONE',  ( -0.1377952755905504645, 0.1660481256975885056, 0.3530559997133364547 ) ) ;
#43179=CARTESIAN_POINT ( 'NONE',  ( -0.6955380577427815458, 0.05413385826771666132, 0.4176697321401328100 ) ) ;
#43180=CARTESIAN_POINT ( 'NONE',  ( 1.279527559055118724, -0.4536011799217368745, -0.2665933059059886201 ) ) ;
#43181=CARTESIAN_POINT ( 'NONE',  ( 0.07874015748031558404, -0.1870078740157480601, -0.3641732283464567677 ) ) ;
#43182=CARTESIAN_POINT ( 'NONE',  ( -0.3018372703412066094, 0.05413385826771666132, 0.4176697321401328100 ) ) ;
#43183=CARTESIAN_POINT ( 'NONE',  ( -1.318897637795274802, 0.1660481256975885056, 0.3530559997133364547 ) ) ;
#43184=CARTESIAN_POINT ( 'NONE',  ( 1.586334378693442959, 1.535433070866141447, 0.1093658747564338618 ) ) ;
#43185=DIRECTION ( 'NONE',  ( -0.6537823813707712706, 0.7566826268715064474, 0.000000000000000000 ) ) ;
#43186=CARTESIAN_POINT ( 'NONE',  ( 0.05905511811023709395, -0.5400638737290844871, 0.3530559997133364547 ) ) ;
#43190=CARTESIAN_POINT ( 'NONE',  ( 0.9645669291338588858, 0.1660481256975885056, 0.3530559997133364547 ) ) ;
#43191=CARTESIAN_POINT ( 'NONE',  ( -0.5839895013123351797, 0.1771653543307087075, -0.09757992244046823083 ) ) ;
#43192=CARTESIAN_POINT ( 'NONE',  ( -0.5118110236220466680, -0.6692913385826771977, 8.415575281601705876E-17 ) ) ;
#43193=CARTESIAN_POINT ( 'NONE',  ( 1.246719160104987623, 0.05413385826771626580, -0.4176697321401330321 ) ) ;
#43194=CARTESIAN_POINT ( 'NONE',  ( 1.030183727034121421, -0.05778040916215522460, 0.4822834645669289988 ) ) ;
#43195=B_SPLINE_CURVE_WITH_KNOTS ( 'NONE', 3,
 ( #59981, #60400, #56854, #56447 ),
 .UNSPECIFIED., .F., .F.,
 ( 4, 4 ),
 ( 4.906538933386797396E-18, 0.001730108991777465225 ),
 .UNSPECIFIED. ) ;
#43196=CARTESIAN_POINT ( 'NONE',  ( -1.568241469816272105, -0.3162353388693409650, -0.4822834645669289433 ) ) ;
#43197=CARTESIAN_POINT ( 'NONE',  ( -0.9120734908136475250, 0.1771653543307087630, 0.09757992244046791164 ) ) ;
#43201=FACE_OUTER_BOUND ( 'NONE', #39202, .T. ) ;
#43202=CARTESIAN_POINT ( 'NONE',  ( 0.5380577427821529035, -0.004921259842519870586, -0.3153832671262229437 ) ) ;
#43203=CARTESIAN_POINT ( 'NONE',  ( 0.3805774278215230400, 0.05413385826771626580, -0.4176697321401330321 ) ) ;
#43206=CARTESIAN_POINT ( 'NONE',  ( 0.8792650918635177559, -0.004921259842519576551, 0.3153832671262227771 ) ) ;
#43207=CARTESIAN_POINT ( 'NONE',  ( -0.5052493438320203589, 0.2952755905511810774, -0.1292274648535930714 ) ) ;
#43208=CARTESIAN_POINT ( 'NONE',  ( -0.7677165354330699465, -0.5400638737290845981, -0.3530559997133363437 ) ) ;
#43209=CARTESIAN_POINT ( 'NONE',  ( 1.384514435695538559, 0.2952755905511810774, -0.1292274648535930714 ) ) ;
#43212=CARTESIAN_POINT ( 'NONE',  ( -0.2624671916010490880, 0.1283753931104746893, -0.1820866141732285504 ) ) ;
#43216=CARTESIAN_POINT ( 'NONE',  ( -0.9842519685039365918, -0.6692913385826771977, 8.415575281601705876E-17 ) ) ;
#43217=CARTESIAN_POINT ( 'NONE',  ( -0.09186351706036663400, -0.4281496062992124485, 0.4176697321401328655 ) ) ;
#43218=CARTESIAN_POINT ( 'NONE',  ( -0.3477690288713902178, 0.2952755905511810774, -0.1292274648535930714 ) ) ;
#43219=CARTESIAN_POINT ( 'NONE',  ( 0.3215223097112867578, -0.3162353388693409650, -0.4822834645669289433 ) ) ;
#43220=CARTESIAN_POINT ( 'NONE',  ( -0.4068241469816264999, -0.4281496062992124485, 0.4176697321401328655 ) ) ;
#43221=CARTESIAN_POINT ( 'NONE',  ( -1.135170603674539924, 0.2952755905511810774, -0.1292274648535930714 ) ) ;
#43222=CARTESIAN_POINT ( 'NONE',  ( -0.8530183727034112984, -0.4281496062992127816, -0.4176697321401328100 ) ) ;
#43223=CARTESIAN_POINT ( 'NONE',  ( 0.8858267716535438430, -0.5400638737290845981, -0.3530559997133363437 ) ) ;
#43224=CARTESIAN_POINT ( 'NONE',  ( 0.4461942257217855201, -0.6046776061558807314, 0.2411417322834647770 ) ) ;
#43227=CARTESIAN_POINT ( 'NONE',  ( -0.1968503937007867743, 0.1771653543307087630, 0.000000000000000000 ) ) ;
#43230=VERTEX_POINT ( 'NONE', #49414 ) ;
#43231=CARTESIAN_POINT ( 'NONE',  ( -1.364829396325458521, 0.1283753931104746893, -0.1820866141732285504 ) ) ;
#43232=CARTESIAN_POINT ( 'NONE',  ( -1.292650918635170010, 0.2952755905511810774, -0.1292274648535930714 ) ) ;
#43233=CARTESIAN_POINT ( 'NONE',  ( -0.5314960629921250401, 0.1660481256975885056, 0.3530559997133364547 ) ) ;
#43235=CARTESIAN_POINT ( 'NONE',  ( -0.6167979002624665030, 0.05413385826771666132, 0.4176697321401328100 ) ) ;
#43236=CARTESIAN_POINT ( 'NONE',  ( -1.023622047244094002, -0.1870078740157480879, -0.4822834645669291653 ) ) ;
#43239=CARTESIAN_POINT ( 'NONE',  ( 0.5183727034120741983, -0.5511811023622046335, 0.09757992244046803654 ) ) ;
#43240=CARTESIAN_POINT ( 'NONE',  ( 0.4768139191967642465, 1.559564387633134874, 0.5050868514466244630 ) ) ;
#43241=CARTESIAN_POINT ( 'NONE',  ( -0.03280839895013062252, -0.5511811023622046335, 0.09757992244046803654 ) ) ;
#43242=CARTESIAN_POINT ( 'NONE',  ( -0.3280839895013117347, 0.05413385826771626580, -0.4176697321401330321 ) ) ;
#43243=DIRECTION ( 'NONE',  ( 0.8479387356305982948, 2.625811289636359704E-16, -0.5300942374872437135 ) ) ;
#43244=CARTESIAN_POINT ( 'NONE',  ( -0.01312335958005186876, 0.05413385826771626580, -0.4176697321401330321 ) ) ;
#43247=CARTESIAN_POINT ( 'NONE',  ( -0.8267716535433065062, 0.2066929133858268208, 0.000000000000000000 ) ) ;
#43251=CARTESIAN_POINT ( 'NONE',  ( 1.587926509186352142, 0.05413385826771666132, 0.4176697321401328100 ) ) ;
#43252=CARTESIAN_POINT ( 'NONE',  ( -0.7742782152230965886, -0.004921259842519576551, 0.3153832671262227771 ) ) ;
#43253=CARTESIAN_POINT ( 'NONE',  ( -0.9383202099737524282, -0.05778040916215522460, 0.4822834645669289988 ) ) ;
#43257=CARTESIAN_POINT ( 'NONE',  ( 1.469816272965879911, -0.6046776061558807314, 0.2411417322834647770 ) ) ;
#43258=CARTESIAN_POINT ( 'NONE',  ( 0.6036745406824153282, -0.6046776061558807314, 0.2411417322834647770 ) ) ;
#43259=CARTESIAN_POINT ( 'NONE',  ( 0.4396325459317593221, 0.2952755905511810774, -0.1292274648535930714 ) ) ;
#43260=CARTESIAN_POINT ( 'NONE',  ( -0.8070866141732276899, 0.07958543189024071263, -0.2665933059059888421 ) ) ;
#43261=CARTESIAN_POINT ( 'NONE',  ( -0.2559055118110230564, 0.1660481256975883668, -0.3530559997133364547 ) ) ;
#43263=CARTESIAN_POINT ( 'NONE',  ( -0.7808398950131225646, -0.05778040916215522460, 0.4822834645669289988 ) ) ;
#43265=CARTESIAN_POINT ( 'NONE',  ( 1.141732283464567566, 0.1771653543307087630, 0.000000000000000000 ) ) ;
#43266=CARTESIAN_POINT ( 'NONE',  ( -0.4855643044619415427, -0.3690944881889763329, 0.3153832671262228327 ) ) ;
#43267=CARTESIAN_POINT ( 'NONE',  ( 1.240157480314961314, 0.07958543189024071263, -0.2665933059059888421 ) ) ;
#43268=CARTESIAN_POINT ( 'NONE',  ( -1.646981627296586703, -0.3162353388693409650, -0.4822834645669289433 ) ) ;
#43270=CARTESIAN_POINT ( 'NONE',  ( -1.095800524934382292, -0.2845877964562161244, -0.3641732283464567121 ) ) ;
#43271=CARTESIAN_POINT ( 'NONE',  ( 0.1450607720586929161, 2.784432375088962958E-17, -0.3464511005275205946 ) ) ;
#43272=CARTESIAN_POINT ( 'NONE',  ( 0.5511811023622055217, -0.1870078740157479769, 0.3641732283464567677 ) ) ;
#43273=CARTESIAN_POINT ( 'NONE',  ( -0.3018372703412066094, -0.4281496062992127816, -0.4176697321401328100 ) ) ;
#43275=CARTESIAN_POINT ( 'NONE',  ( -0.1771653543307080136, 0.07958543189024071263, -0.2665933059059888421 ) ) ;
#43277=CARTESIAN_POINT ( 'NONE',  ( 0.5511811023622055217, -0.1870078740157479769, 0.4822834645669291653 ) ) ;
#43278=CARTESIAN_POINT ( 'NONE',  ( 0.4849061582275016602, 2.793565526369266028, 0.4921425059946344382 ) ) ;
#43279=CARTESIAN_POINT ( 'NONE',  ( 1.266404199475066328, -0.08942795157527998196, 0.3641732283464567121 ) ) ;
#43280=CARTESIAN_POINT ( 'NONE',  ( -1.023622047244094002, -0.1870078740157480879, -0.4822834645669291653 ) ) ;
#43281=CARTESIAN_POINT ( 'NONE',  ( -0.3215223097112853146, -0.08942795157528024563, -0.3641732283464568787 ) ) ;
#43283=CARTESIAN_POINT ( 'NONE',  ( 0.07874015748031558404, -0.1870078740157480601, -0.3641732283464567677 ) ) ;
#43284=B_SPLINE_CURVE_WITH_KNOTS ( 'NONE', 3,
 ( #27434, #42438, #78388, #53096, #72064, #8094, #59838 ),
 .UNSPECIFIED., .F., .F.,
 ( 4, 3, 4 ),
 ( 1.540743955509788682E-33, 0.001246232571205247927, 0.002492492258783241162 ),
 .UNSPECIFIED. ) ;
#43285=CARTESIAN_POINT ( 'NONE',  ( -0.5577427821522301654, -0.3162353388693405765, 0.4822834645669290543 ) ) ;
#43289=CARTESIAN_POINT ( 'NONE',  ( 0.7939632545931766261, -0.08942795157527998196, 0.3641732283464567121 ) ) ;
#43290=CARTESIAN_POINT ( 'NONE',  ( -0.4133858267716528645, -0.5400638737290844871, 0.3530559997133364547 ) ) ;
#43291=CARTESIAN_POINT ( 'NONE',  ( -0.5511811023622038563, -0.1870078740157479769, 0.4822834645669291653 ) ) ;
#43292=CARTESIAN_POINT ( 'NONE',  ( -0.9317585301837263412, -0.3690944881889765550, -0.3153832671262227771 ) ) ;
#43294=CARTESIAN_POINT ( 'NONE',  ( 0.08530183727034192087, -0.05778040916215522460, 0.4822834645669289988 ) ) ;
#43295=CARTESIAN_POINT ( 'NONE',  ( -1.043307086614172707, 0.07958543189024071263, -0.2665933059059888421 ) ) ;
#43296=CARTESIAN_POINT ( 'NONE',  ( -1.489501312335957062, -0.05778040916215522460, 0.4822834645669289988 ) ) ;
#43298=ORIENTED_EDGE ( 'NONE', *, *, #10620, .F. ) ;
#43299=CARTESIAN_POINT ( 'NONE',  ( -1.679790026246718693, 0.1283753931104746893, -0.1820866141732285504 ) ) ;
#43300=CARTESIAN_POINT ( 'NONE',  ( -1.161417322834644716, -0.5400638737290845981, -0.3530559997133363437 ) ) ;
#43301=CARTESIAN_POINT ( 'NONE',  ( -0.8136482939632537770, -0.6046776061558807314, 0.2411417322834647770 ) ) ;
#43302=CARTESIAN_POINT ( 'NONE',  ( -1.450131233595799651, 0.2952755905511810774, -0.1292274648535930714 ) ) ;
#43305=CARTESIAN_POINT ( 'NONE',  ( 1.122047244094488860, -0.5400638737290845981, -0.3530559997133363437 ) ) ;
#43306=CARTESIAN_POINT ( 'NONE',  ( 0.3674540682414705883, -0.6046776061558807314, 0.2411417322834647770 ) ) ;
#43309=CARTESIAN_POINT ( 'NONE',  ( 1.141732283464567566, 0.1771653543307087630, 0.000000000000000000 ) ) ;
#43312=CARTESIAN_POINT ( 'NONE',  ( -1.003937007874014853, 0.07958543189024085140, 0.2665933059059887866 ) ) ;
#43315=CARTESIAN_POINT ( 'NONE',  ( 0.3346456692913390985, 0.1660481256975885056, 0.3530559997133364547 ) ) ;
#43316=CARTESIAN_POINT ( 'NONE',  ( -0.3280839895013117347, -0.4281496062992124485, 0.4176697321401328655 ) ) ;
#43317=CARTESIAN_POINT ( 'NONE',  ( -0.9645669291338575535, 0.1660481256975883668, -0.3530559997133364547 ) ) ;
#43318=CARTESIAN_POINT ( 'NONE',  ( 0.9317585301837276734, 0.05413385826771626580, -0.4176697321401330321 ) ) ;
#43319=CARTESIAN_POINT ( 'NONE',  ( 1.541994750656168645, 0.2952755905511810774, -0.1292274648535930714 ) ) ;
#43320=CARTESIAN_POINT ( 'NONE',  ( 0.07217847769028949700, -0.3162353388693405765, 0.4822834645669290543 ) ) ;
#43321=CARTESIAN_POINT ( 'NONE',  ( -1.233595800524933894, -0.6046776061558809534, -0.2411417322834644161 ) ) ;
#43322=CARTESIAN_POINT ( 'NONE',  ( -1.522309711286088607, -0.6046776061558807314, 0.2411417322834647770 ) ) ;
#43325=CARTESIAN_POINT ( 'NONE',  ( 0.8267716535433078384, -0.5511811023622047445, 6.969142054262312111E-17 ) ) ;
#43326=VERTEX_POINT ( 'NONE', #42681 ) ;
#43328=CARTESIAN_POINT ( 'NONE',  ( -0.6627296587926501115, 0.2952755905511810774, -0.1292274648535930714 ) ) ;
#43330=CARTESIAN_POINT ( 'NONE',  ( -0.01968503937007793844, -0.4536011799217367080, 0.2665933059059888421 ) ) ;
#43331=CARTESIAN_POINT ( 'NONE',  ( -1.653543307086613234, -0.1870078740157480879, -0.4822834645669291653 ) ) ;
#43332=CARTESIAN_POINT ( 'NONE',  ( 0.4396325459317590445, -0.6692913385826771977, 0.1292274648535927661 ) ) ;
#43333=CARTESIAN_POINT ( 'NONE',  ( 0.4724409448818904789, -0.1870078740157479769, 0.4822834645669291653 ) ) ;
#43334=CARTESIAN_POINT ( 'NONE',  ( -0.5577427821522301654, -0.05778040916215560624, -0.4822834645669293319 ) ) ;
#43336=CARTESIAN_POINT ( 'NONE',  ( -1.358267716535432434, -0.5400638737290844871, 0.3530559997133364547 ) ) ;
#43338=CARTESIAN_POINT ( 'NONE',  ( 1.246719160104987623, -0.3690944881889763329, 0.3153832671262228327 ) ) ;
#43339=CARTESIAN_POINT ( 'NONE',  ( -1.200787401574802349, -0.5400638737290844871, 0.3530559997133364547 ) ) ;
#43340=CARTESIAN_POINT ( 'NONE',  ( 1.043307086614173818, 0.1660481256975885056, 0.3530559997133364547 ) ) ;
#43341=CARTESIAN_POINT ( 'NONE',  ( 1.213910761154856299, 0.2952755905511811885, 0.1292274648535926551 ) ) ;
#43343=CARTESIAN_POINT ( 'NONE',  ( -1.259842519685038686, -0.1870078740157479769, 0.4822834645669291653 ) ) ;
#43345=CARTESIAN_POINT ( 'NONE',  ( 0.2755905511811031494, -0.6692913385826771977, 8.415575281601705876E-17 ) ) ;
#43348=CARTESIAN_POINT ( 'NONE',  ( -1.620734908136482577, 0.1771653543307087630, 0.09757992244046791164 ) ) ;
#43349=CARTESIAN_POINT ( 'NONE',  ( 0.5183727034120741983, -0.5511811023622046335, 0.09757992244046803654 ) ) ;
#43350=CARTESIAN_POINT ( 'NONE',  ( 0.9580052493438326877, 0.05413385826771666132, 0.4176697321401328100 ) ) ;
#43352=CARTESIAN_POINT ( 'NONE',  ( 0.8070866141732289112, -0.4536011799217368745, -0.2665933059059886201 ) ) ;
#43354=CARTESIAN_POINT ( 'NONE',  ( 0.4133858267716541968, -0.5400638737290845981, -0.3530559997133363437 ) ) ;
#43355=VECTOR ( 'NONE', #76173, 39.37007874015748854 ) ;
#43357=CARTESIAN_POINT ( 'NONE',  ( -0.6102362204724400829, 0.1660481256975885056, 0.3530559997133364547 ) ) ;
#43359=CARTESIAN_POINT ( 'NONE',  ( 0.8464566929133865436, 0.07958543189024071263, -0.2665933059059888421 ) ) ;
#43360=CARTESIAN_POINT ( 'NONE',  ( -0.01312335958005186876, -0.4281496062992124485, 0.4176697321401328655 ) ) ;
#43361=CARTESIAN_POINT ( 'NONE',  ( 0.1377952755905518245, 0.1012011053420775880, -0.2882089793578256898 ) ) ;
#43362=CARTESIAN_POINT ( 'NONE',  ( -0.3543307086614165824, -0.6692913385826771977, 8.415575281601705876E-17 ) ) ;
#43363=EDGE_CURVE ( 'NONE', #3487, #27293, #70527, .T. ) ;
#43364=CARTESIAN_POINT ( 'NONE',  ( -0.05905511811023545637, 0.07958543189024085140, 0.2665933059059887866 ) ) ;
#43366=CARTESIAN_POINT ( 'NONE',  ( -0.4986876640419942164, -0.6046776061558807314, 0.2411417322834647770 ) ) ;
#43367=CARTESIAN_POINT ( 'NONE',  ( 0.8267716535433077274, 0.1771653543307087630, 0.000000000000000000 ) ) ;
#43368=CARTESIAN_POINT ( 'NONE',  ( -0.7535225988626923499, 2.401574803149606474, 0.4915354330708645025 ) ) ;
#43370=CARTESIAN_POINT ( 'NONE',  ( 0.5183727034120741983, -0.6692913385826771977, 0.1292274648535927661 ) ) ;
#43371=EDGE_CURVE ( 'NONE', #41294, #46160, #71045, .T. ) ;
#43373=CARTESIAN_POINT ( 'NONE',  ( 1.207349081364829990, 0.1283753931104748280, 0.1820866141732283561 ) ) ;
#43374=CARTESIAN_POINT ( 'NONE',  ( -1.191111281560509383, -2.567464376874931580E-15, -0.4445507791589072832 ) ) ;
#43375=CARTESIAN_POINT ( 'NONE',  ( -0.2034120734908131112, -0.5511811023622048555, -0.09757992244046775898 ) ) ;
#43376=CARTESIAN_POINT ( 'NONE',  ( -0.7939632545931754048, -0.2845877964562159024, 0.3641732283464567677 ) ) ;
#43377=CARTESIAN_POINT ( 'NONE',  ( -0.4855643044619415427, 0.05413385826771626580, -0.4176697321401330321 ) ) ;
#43378=CARTESIAN_POINT ( 'NONE',  ( 1.076115485564305141, 0.1283753931104746893, -0.1820866141732285504 ) ) ;
#43380=CARTESIAN_POINT ( 'NONE',  ( 1.581364829396326277, -0.08942795157527998196, 0.3641732283464567121 ) ) ;
#43381=CARTESIAN_POINT ( 'NONE',  ( 0.2165354330708668673, -0.5400638737290844871, 0.3530559997133364547 ) ) ;
#43382=CARTESIAN_POINT ( 'NONE',  ( 0.5905511811023629321, 0.2952755905511811885, 0.000000000000000000 ) ) ;
#43385=CARTESIAN_POINT ( 'NONE',  ( 0.3543307086614179147, 0.2952755905511811885, 0.000000000000000000 ) ) ;
#43387=CARTESIAN_POINT ( 'NONE',  ( 0.6889763779527566800, -0.5400638737290844871, 0.3530559997133364547 ) ) ;
#43388=CARTESIAN_POINT ( 'NONE',  ( 0.6889763779527566800, -0.5400638737290844871, 0.3530559997133364547 ) ) ;
#43391=CARTESIAN_POINT ( 'NONE',  ( 0.4133858267716541968, 0.07958543189024085140, 0.2665933059059887866 ) ) ;
#43392=CARTESIAN_POINT ( 'NONE',  ( 1.069553805774278832, 0.2952755905511810774, -0.1292274648535930714 ) ) ;
#43393=CARTESIAN_POINT ( 'NONE',  ( 0.09842519685039434474, -0.4536011799217368745, -0.2665933059059886201 ) ) ;
#43394=CARTESIAN_POINT ( 'NONE',  ( -0.1771653543307080136, 0.1660481256975883668, -0.3530559997133364547 ) ) ;
#43395=CARTESIAN_POINT ( 'NONE',  ( 0.3871391076115492380, -0.05778040916215560624, -0.4822834645669293319 ) ) ;
#43396=CARTESIAN_POINT ( 'NONE',  ( -0.5971128608923877978, -0.6692913385826773087, -0.1292274648535924053 ) ) ;
#43398=CARTESIAN_POINT ( 'NONE',  ( -0.4593175853018366950, -0.004921259842519576551, 0.3153832671262227771 ) ) ;
#43399=CARTESIAN_POINT ( 'NONE',  ( 0.9383202099737536495, -0.3162353388693405765, 0.4822834645669290543 ) ) ;
#43400=CARTESIAN_POINT ( 'NONE',  ( 1.023622047244095334, -0.1870078740157479769, 0.3641732283464567677 ) ) ;
#43401=CARTESIAN_POINT ( 'NONE',  ( 0.006561679790026889343, -0.3162353388693409650, -0.4822834645669289433 ) ) ;
#43402=CARTESIAN_POINT ( 'NONE',  ( 1.220472440944879722, 2.401574803149606474, 0.5309055118110233007 ) ) ;
#43404=CARTESIAN_POINT ( 'NONE',  ( -0.3836918680457887532, -2.191421614605370878E-15, 0.4445507791589071167 ) ) ;
#43406=CARTESIAN_POINT ( 'NONE',  ( -1.030183727034119867, -0.3162353388693405765, 0.4822834645669290543 ) ) ;
#43407=B_SPLINE_CURVE_WITH_KNOTS ( 'NONE', 3,
 ( #25678, #24443, #12653, #11423, #37900, #63576, #38314 ),
 .UNSPECIFIED., .F., .F.,
 ( 4, 3, 4 ),
 ( 3.642919299551295515E-17, 0.001246232571205268744, 0.002492492258783277591 ),
 .UNSPECIFIED. ) ;
#43408=CARTESIAN_POINT ( 'NONE',  ( -0.7874015748031489847, -0.1870078740157479769, 0.4822834645669291653 ) ) ;
#43412=CARTESIAN_POINT ( 'NONE',  ( 0.2690288713910767848, 0.1771653543307087630, 0.09757992244046791164 ) ) ;
#43415=CARTESIAN_POINT ( 'NONE',  ( 0.4921259842519691285, 0.1660481256975885056, 0.3530559997133364547 ) ) ;
#43417=CARTESIAN_POINT ( 'NONE',  ( 0.9842519685039375910, 0.2952755905511811885, 0.000000000000000000 ) ) ;
#43420=CARTESIAN_POINT ( 'NONE',  ( 1.371391076115485941, 0.2952755905511811885, 0.1292274648535926551 ) ) ;
#43421=CARTESIAN_POINT ( 'NONE',  ( 1.502624671916010790, -0.2845877964562161244, -0.3641732283464567121 ) ) ;
#43422=CARTESIAN_POINT ( 'NONE',  ( -0.08530183727034056085, -0.3162353388693405765, 0.4822834645669290543 ) ) ;
#43424=CARTESIAN_POINT ( 'NONE',  ( -0.4002624671916004129, -0.3162353388693405765, 0.4822834645669290543 ) ) ;
#43425=CARTESIAN_POINT ( 'NONE',  ( -0.8005249343832013809, -0.3690944881889763329, 0.3153832671262228327 ) ) ;
#43426=CARTESIAN_POINT ( 'NONE',  ( 0.5511811023622054106, -0.1870078740157480879, -0.4822834645669291653 ) ) ;
#43427=CARTESIAN_POINT ( 'NONE',  ( -0.4855643044619415427, -0.4281496062992124485, 0.4176697321401328655 ) ) ;
#43428=DIRECTION ( 'NONE',  ( 0.000000000000000000, 1.000000000000000000, 0.000000000000000000 ) ) ;
#43432=CARTESIAN_POINT ( 'NONE',  ( 0.3477690288713918276, -0.6692913385826773087, -0.1292274648535924053 ) ) ;
#43433=CARTESIAN_POINT ( 'NONE',  ( -0.5183727034120726440, -0.6692913385826773087, -0.1292274648535924053 ) ) ;
#43434=CARTESIAN_POINT ( 'NONE',  ( -1.627296587926508442, 0.2306618581243848609, 0.2411417322834645549 ) ) ;
#43435=CARTESIAN_POINT ( 'NONE',  ( 0.6233595800524939223, -0.3162353388693405765, 0.4822834645669290543 ) ) ;
#43436=CARTESIAN_POINT ( 'NONE',  ( 0.4133858267716541968, 0.1660481256975885056, 0.3530559997133364547 ) ) ;
#43438=CARTESIAN_POINT ( 'NONE',  ( -0.9645669291338575535, -0.5400638737290844871, 0.3530559997133364547 ) ) ;
#43439=CARTESIAN_POINT ( 'NONE',  ( 0.1837270341207357105, -0.6046776061558809534, -0.2411417322834644161 ) ) ;
#43440=CARTESIAN_POINT ( 'NONE',  ( -0.4658792650918627265, -0.3162353388693409650, -0.4822834645669289433 ) ) ;
#43441=CARTESIAN_POINT ( 'NONE',  ( 0.4593175853018380828, -0.004921259842519870586, -0.3153832671262229437 ) ) ;
#43442=CARTESIAN_POINT ( 'NONE',  ( -1.679790026246718693, 0.2306618581243847221, -0.2411417322834647770 ) ) ;
#43444=CARTESIAN_POINT ( 'NONE',  ( 0.03937007874015806264, 0.2952755905511811885, 0.000000000000000000 ) ) ;
#43447=CARTESIAN_POINT ( 'NONE',  ( -1.548556430446193399, -0.6046776061558809534, -0.2411417322834644161 ) ) ;
#43451=CARTESIAN_POINT ( 'NONE',  ( 0.8923884514435703741, 0.2306618581243848609, 0.2411417322834645549 ) ) ;
#43452=CARTESIAN_POINT ( 'NONE',  ( 0.1181102362204730916, -0.5511811023622047445, 6.969142054262312111E-17 ) ) ;
#43454=CARTESIAN_POINT ( 'NONE',  ( -1.586052503253847057, 1.574803149606300412, 0.1653254495020574921 ) ) ;
#43456=CARTESIAN_POINT ( 'NONE',  ( -0.9573014326657163231, -2.609869883881465018E-15, -0.3464511005275220379 ) ) ;
#43457=CARTESIAN_POINT ( 'NONE',  ( 0.3025410870193226964, 2.784432375088962958E-17, -0.3464511005275205946 ) ) ;
#43459=CARTESIAN_POINT ( 'NONE',  ( 0.6692913385826777528, 0.2952755905511811885, 0.000000000000000000 ) ) ;
#43460=CARTESIAN_POINT ( 'NONE',  ( -1.292650918635170010, 0.2952755905511810774, -0.1292274648535930714 ) ) ;
#43461=AXIS2_PLACEMENT_3D ( 'NONE', #1198, #44519, #51250 ) ;
#43462=CARTESIAN_POINT ( 'NONE',  ( -1.318897637795274802, -0.5400638737290845981, -0.3530559997133363437 ) ) ;
#43463=CARTESIAN_POINT ( 'NONE',  ( 0.3937007874015754361, -0.1870078740157480879, -0.4822834645669291653 ) ) ;
#43464=CARTESIAN_POINT ( 'NONE',  ( 1.135170603674541256, 0.2952755905511811885, 0.1292274648535926551 ) ) ;
#43465=CARTESIAN_POINT ( 'NONE',  ( 1.233595800524935227, 0.1283753931104746893, -0.1820866141732285504 ) ) ;
#43466=CARTESIAN_POINT ( 'NONE',  ( 1.384514435695538559, 0.1771653543307087075, -0.09757992244046823083 ) ) ;
#43467=CARTESIAN_POINT ( 'NONE',  ( -0.9908136482939626788, 0.2952755905511811885, 0.1292274648535926551 ) ) ;
#43469=CARTESIAN_POINT ( 'NONE',  ( 1.640419947506562393, -0.4281496062992124485, 0.4176697321401328655 ) ) ;
#43470=EDGE_CURVE ( 'NONE', #27293, #65491, #35339, .T. ) ;
#43472=CARTESIAN_POINT ( 'NONE',  ( -0.2099737532808391705, 0.2306618581243848609, 0.2411417322834645549 ) ) ;
#43473=CARTESIAN_POINT ( 'NONE',  ( 1.141732283464567788, -0.6692913385826771977, 8.415575281601705876E-17 ) ) ;
#43475=CARTESIAN_POINT ( 'NONE',  ( -1.587926509186350810, -0.3690944881889763329, 0.3153832671262228327 ) ) ;
#43476=CARTESIAN_POINT ( 'NONE',  ( 0.5774278215223104249, 0.2306618581243848609, 0.2411417322834645549 ) ) ;
#43477=CARTESIAN_POINT ( 'NONE',  ( 0.9186351706036751663, -0.5023911411419708095, 0.1820866141732285504 ) ) ;
#43478=CARTESIAN_POINT ( 'NONE',  ( -1.377952755905511140, 0.1771653543307087630, 0.000000000000000000 ) ) ;
#43479=CARTESIAN_POINT ( 'NONE',  ( 0.8070866141732289112, -0.5400638737290845981, -0.3530559997133363437 ) ) ;
#43480=CARTESIAN_POINT ( 'NONE',  ( -0.5118110236220466680, 0.2952755905511811885, 0.000000000000000000 ) ) ;
#43481=CARTESIAN_POINT ( 'NONE',  ( -0.5314960629921254842, -0.4536011799217368745, -0.2665933059059886201 ) ) ;
#43482=CARTESIAN_POINT ( 'NONE',  ( -0.6758530183727028406, -0.6692913385826773087, -0.1292274648535924053 ) ) ;
#43483=CARTESIAN_POINT ( 'NONE',  ( 1.463254593175853824, -0.6692913385826771977, 0.1292274648535927661 ) ) ;
#43484=CARTESIAN_POINT ( 'NONE',  ( -0.8398950131233589023, -0.6046776061558809534, -0.2411417322834644161 ) ) ;
#43485=CARTESIAN_POINT ( 'NONE',  ( 1.568241469816273659, -0.05778040916215560624, -0.4822834645669293319 ) ) ;
#43487=CARTESIAN_POINT ( 'NONE',  ( -1.108923884514435132, -0.08942795157528024563, -0.3641732283464568787 ) ) ;
#43490=CARTESIAN_POINT ( 'NONE',  ( 1.397637795275591177, -0.5400638737290844871, 0.3530559997133364547 ) ) ;
#43492=CARTESIAN_POINT ( 'NONE',  ( -0.08983781461629233855, 1.809133623825372073E-16, -0.3954985857520062487 ) ) ;
#43493=CARTESIAN_POINT ( 'NONE',  ( -1.541994750656167090, -0.5511811023622048555, -0.09757992244046775898 ) ) ;
#43494=CARTESIAN_POINT ( 'NONE',  ( -0.4724409448818890911, -0.1870078740157479769, 0.3641732283464567677 ) ) ;
#43495=CARTESIAN_POINT ( 'NONE',  ( -1.587926509186350810, 0.05413385826771626580, -0.4176697321401330321 ) ) ;
#43496=CARTESIAN_POINT ( 'NONE',  ( -0.5314960629921250401, 0.1660481256975885056, 0.3530559997133364547 ) ) ;
#43497=CARTESIAN_POINT ( 'NONE',  ( 0.06561679790026316017, -0.3690944881889763329, 0.3153832671262228327 ) ) ;
#43498=CARTESIAN_POINT ( 'NONE',  ( -1.108923884514435132, -0.2845877964562159024, 0.3641732283464567677 ) ) ;
#43499=CARTESIAN_POINT ( 'NONE',  ( 1.456692913385827515, 0.1771653543307087630, 0.000000000000000000 ) ) ;
#43500=CARTESIAN_POINT ( 'NONE',  ( 0.9186351706036752773, 0.2306618581243847221, -0.2411417322834647770 ) ) ;
#43502=CARTESIAN_POINT ( 'NONE',  ( 0.5577427821522316087, -0.08942795157527998196, 0.3641732283464567121 ) ) ;
#43503=CARTESIAN_POINT ( 'NONE',  ( 0.2624671916010504757, 0.2306618581243848609, 0.2411417322834645549 ) ) ;
#43504=CARTESIAN_POINT ( 'NONE',  ( 0.8136482939632553313, 0.1283753931104748280, 0.1820866141732283561 ) ) ;
#43505=EDGE_LOOP ( 'NONE', ( #27726, #39100, #6529, #75981 ) ) ;
#43506=CARTESIAN_POINT ( 'NONE',  ( -1.417322834645668772, -0.1870078740157480879, -0.4822834645669291653 ) ) ;
#43507=CARTESIAN_POINT ( 'NONE',  ( -1.266404199475064773, -0.05778040916215560624, -0.4822834645669293319 ) ) ;
#43508=CARTESIAN_POINT ( 'NONE',  ( -0.09842519685039295696, 0.1660481256975883668, -0.3530559997133364547 ) ) ;
#43511=CARTESIAN_POINT ( 'NONE',  ( 0.6496062992125991586, 0.1660481256975885056, 0.3530559997133364547 ) ) ;
#43512=CARTESIAN_POINT ( 'NONE',  ( 1.450131233595801428, 0.1771653543307087630, 0.09757992244046791164 ) ) ;
#43513=CARTESIAN_POINT ( 'NONE',  ( -0.1443569553805765515, -0.4281496062992127816, -0.4176697321401328100 ) ) ;
#43514=CARTESIAN_POINT ( 'NONE',  ( 0.5380577427821529035, 0.05413385826771626580, -0.4176697321401330321 ) ) ;
#43515=ADVANCED_FACE ( 'NONE', ( #30878 ), #5406, .F. ) ;
#43519=FACE_OUTER_BOUND ( 'NONE', #53478, .T. ) ;
#43523=CARTESIAN_POINT ( 'NONE',  ( -0.4593175853018366950, -0.004921259842519576551, 0.3153832671262227771 ) ) ;
#43524=CARTESIAN_POINT ( 'NONE',  ( -0.7480314960629914633, 0.2952755905511811885, 0.000000000000000000 ) ) ;
#43525=CARTESIAN_POINT ( 'NONE',  ( 0.2887139107611556010, -0.6046776061558807314, 0.2411417322834647770 ) ) ;
#43527=CARTESIAN_POINT ( 'NONE',  ( 0.7874015748031503170, -0.1870078740157480879, -0.4822834645669291653 ) ) ;
#43528=CARTESIAN_POINT ( 'NONE',  ( 1.522309711286089939, -0.6046776061558809534, -0.2411417322834644161 ) ) ;
#43529=CARTESIAN_POINT ( 'NONE',  ( 0.7283464566929140904, -0.5400638737290845981, -0.3530559997133363437 ) ) ;
#43532=CARTESIAN_POINT ( 'NONE',  ( 1.476377952755906442, -0.5400638737290844871, 0.3530559997133364547 ) ) ;
#43533=CARTESIAN_POINT ( 'NONE',  ( 0.8005249343832027131, 0.05413385826771666132, 0.4176697321401328100 ) ) ;
#43534=CARTESIAN_POINT ( 'NONE',  ( 0.5839895013123367340, -0.6692913385826773087, -0.1292274648535924053 ) ) ;
#43536=CARTESIAN_POINT ( 'NONE',  ( 1.043307086614173818, -0.4536011799217368745, -0.2665933059059886201 ) ) ;
#43537=CARTESIAN_POINT ( 'NONE',  ( -1.646981627296586703, -0.08942795157527998196, 0.3641732283464567121 ) ) ;
#43538=CARTESIAN_POINT ( 'NONE',  ( 1.522309711286089939, -0.6046776061558809534, -0.2411417322834644161 ) ) ;
#43540=FACE_OUTER_BOUND ( 'NONE', #56500, .T. ) ;
#43541=CARTESIAN_POINT ( 'NONE',  ( 0.8464566929133866546, -0.5400638737290844871, 0.3530559997133364547 ) ) ;
#43542=CARTESIAN_POINT ( 'NONE',  ( 1.482939632545932307, -0.3690944881889763329, 0.3153832671262228327 ) ) ;
#43543=CARTESIAN_POINT ( 'NONE',  ( -0.5577427821522301654, -0.05778040916215560624, -0.4822834645669293319 ) ) ;
#43544=CARTESIAN_POINT ( 'NONE',  ( -0.8923884514435688198, 0.2306618581243847221, -0.2411417322834647770 ) ) ;
#43545=CARTESIAN_POINT ( 'NONE',  ( 1.076115485564305141, -0.6046776061558807314, 0.2411417322834647770 ) ) ;
#43549=CARTESIAN_POINT ( 'NONE',  ( 1.607611548556431069, -0.6692913385826773087, -0.1292274648535924053 ) ) ;
#43550=ORIENTED_EDGE ( 'NONE', *, *, #30143, .T. ) ;
#43554=CARTESIAN_POINT ( 'NONE',  ( 1.509186351706037543, -0.3690944881889765550, -0.3153832671262227771 ) ) ;
#43561=CARTESIAN_POINT ( 'NONE',  ( -0.8989501312335946848, -0.5511811023622046335, 0.09757992244046803654 ) ) ;
#43562=CARTESIAN_POINT ( 'NONE',  ( -1.200787401574802349, 0.07958543189024071263, -0.2665933059059888421 ) ) ;
#43563=CARTESIAN_POINT ( 'NONE',  ( -1.272965879265091305, 0.05413385826771626580, -0.4176697321401330321 ) ) ;
#43564=CARTESIAN_POINT ( 'NONE',  ( -0.1049868766404193215, 0.2306618581243847221, -0.2411417322834647770 ) ) ;
#43565=CARTESIAN_POINT ( 'NONE',  ( -1.391076115485563314, -0.6046776061558809534, -0.2411417322834644161 ) ) ;
#43566=EDGE_LOOP ( 'NONE', ( #631, #82072, #31838, #53075 ) ) ;
#43567=CARTESIAN_POINT ( 'NONE',  ( 1.614173228346457378, 0.2952755905511811885, 0.000000000000000000 ) ) ;
#43568=CARTESIAN_POINT ( 'NONE',  ( -1.148293963254592542, 0.2066929133858267931, 0.1054918080437490802 ) ) ;
#43571=CARTESIAN_POINT ( 'NONE',  ( -0.3674540682414689785, 0.1283753931104748280, 0.1820866141732283561 ) ) ;
#43572=CARTESIAN_POINT ( 'NONE',  ( -1.082677165354329896, -0.5400638737290845981, -0.3530559997133363437 ) ) ;
#43573=CARTESIAN_POINT ( 'NONE',  ( 1.141732283464567788, -0.6692913385826771977, 8.415575281601705876E-17 ) ) ;
#43574=ORIENTED_EDGE ( 'NONE', *, *, #50670, .F. ) ;
#43577=CARTESIAN_POINT ( 'NONE',  ( 1.679790026246720025, 0.2306618581243848609, 0.2411417322834645549 ) ) ;
#43578=CARTESIAN_POINT ( 'NONE',  ( -1.194225721784776262, 0.05413385826771626580, -0.4176697321401330321 ) ) ;
#43580=CARTESIAN_POINT ( 'NONE',  ( -0.03280839895013062252, -0.5511811023622046335, 0.09757992244046803654 ) ) ;
#43583=CARTESIAN_POINT ( 'NONE',  ( 0.07874015748031558404, -0.1870078740157479769, 0.3641732283464567677 ) ) ;
#43584=CARTESIAN_POINT ( 'NONE',  ( 0.3937007874015754361, -0.1870078740157480601, -0.3641732283464567677 ) ) ;
#43585=CARTESIAN_POINT ( 'NONE',  ( 0.4461942257217855201, -0.6046776061558807314, 0.2411417322834647770 ) ) ;
#43586=CARTESIAN_POINT ( 'NONE',  ( -0.7677165354330699465, -0.4536011799217368745, -0.2665933059059886201 ) ) ;
#43588=CARTESIAN_POINT ( 'NONE',  ( 1.358267716535433323, -0.5400638737290845981, -0.3530559997133363437 ) ) ;
#43589=CARTESIAN_POINT ( 'NONE',  ( -1.076115485564303809, -0.6046776061558809534, -0.2411417322834644161 ) ) ;
#43591=CARTESIAN_POINT ( 'NONE',  ( 0.1246719160104994284, -0.6692913385826771977, 0.1292274648535927661 ) ) ;
#43592=CARTESIAN_POINT ( 'NONE',  ( -0.5839895013123351797, -0.6692913385826771977, 0.1292274648535927661 ) ) ;
#43593=CARTESIAN_POINT ( 'NONE',  ( 1.128608923884515169, -0.5023911411419708095, -0.1820866141732282451 ) ) ;
#43594=CARTESIAN_POINT ( 'NONE',  ( -0.07217847769028813698, -0.2845877964562161244, -0.3641732283464567121 ) ) ;
#43595=CARTESIAN_POINT ( 'NONE',  ( -0.3412073490813641308, -0.6046776061558807314, 0.2411417322834647770 ) ) ;
#43596=CARTESIAN_POINT ( 'NONE',  ( -1.003937007874014853, 0.1660481256975885056, 0.3530559997133364547 ) ) ;
#43597=CARTESIAN_POINT ( 'NONE',  ( 1.595398199321655275, 0.7375059713363275593, -0.1559797534342494130 ) ) ;
#43598=CARTESIAN_POINT ( 'NONE',  ( 1.568241469816273659, -0.08942795157528024563, -0.3641732283464568787 ) ) ;
#43599=CARTESIAN_POINT ( 'NONE',  ( -0.2034120734908128059, 0.2952755905511811885, 0.1292274648535926551 ) ) ;
#43600=CARTESIAN_POINT ( 'NONE',  ( -1.095800524934382292, -0.05778040916215522460, 0.4822834645669289988 ) ) ;
#43603=CARTESIAN_POINT ( 'NONE',  ( 1.049868766404200127, -0.6046776061558809534, -0.2411417322834644161 ) ) ;
#43604=CARTESIAN_POINT ( 'NONE',  ( -0.5708661417322828946, 0.07958543189024071263, -0.2665933059059888421 ) ) ;
#43605=CARTESIAN_POINT ( 'NONE',  ( -0.4986876640419942164, -0.6046776061558807314, 0.2411417322834647770 ) ) ;
#43606=CARTESIAN_POINT ( 'NONE',  ( 1.469816272965879911, -0.6046776061558807314, 0.2411417322834647770 ) ) ;
#43607=CARTESIAN_POINT ( 'NONE',  ( 0.8923884514435703741, 0.2306618581243848609, 0.2411417322834645549 ) ) ;
#43608=CARTESIAN_POINT ( 'NONE',  ( -1.437007874015747477, 0.1660481256975883668, -0.3530559997133364547 ) ) ;
#43609=CARTESIAN_POINT ( 'NONE',  ( -0.9580052493438311334, -0.3690944881889763329, 0.3153832671262228327 ) ) ;
#43611=ADVANCED_FACE ( 'NONE', ( #23572 ), #69845, .F. ) ;
#43615=CARTESIAN_POINT ( 'NONE',  ( 1.167979002624672580, -0.3690944881889763329, 0.3153832671262228327 ) ) ;
#43616=CARTESIAN_POINT ( 'NONE',  ( 0.6496062992125991586, 0.07958543189024085140, 0.2665933059059887866 ) ) ;
#43617=CARTESIAN_POINT ( 'NONE',  ( 0.5511811023622054106, -0.1870078740157480879, -0.4822834645669291653 ) ) ;
#43618=FACE_OUTER_BOUND ( 'NONE', #18486, .T. ) ;
#43620=CARTESIAN_POINT ( 'NONE',  ( 1.010498687664042716, -0.3690944881889763329, 0.3153832671262228327 ) ) ;
#43621=CARTESIAN_POINT ( 'NONE',  ( -0.3477690288713902178, 0.2952755905511810774, -0.1292274648535930714 ) ) ;
#43622=CARTESIAN_POINT ( 'NONE',  ( -0.8202099737532799750, 0.2952755905511810774, -0.1292274648535930714 ) ) ;
#43623=CARTESIAN_POINT ( 'NONE',  ( 1.194225721784777594, 0.05413385826771666132, 0.4176697321401328100 ) ) ;
#43625=CARTESIAN_POINT ( 'NONE',  ( -0.03280839895013062252, -0.5511811023622046335, 0.09757992244046803654 ) ) ;
#43627=ORIENTED_EDGE ( 'NONE', *, *, #3457, .T. ) ;
#43628=CARTESIAN_POINT ( 'NONE',  ( -0.9448818897637790704, -0.1870078740157479769, 0.4822834645669291653 ) ) ;
#43629=CARTESIAN_POINT ( 'NONE',  ( -0.3215223097112853146, -0.05778040916215560624, -0.4822834645669293319 ) ) ;
#43630=CARTESIAN_POINT ( 'NONE',  ( -0.4068241469816264999, -0.4281496062992124485, 0.4176697321401328655 ) ) ;
#43632=CARTESIAN_POINT ( 'NONE',  ( 0.5052493438320218022, -0.6692913385826773087, -0.1292274648535924053 ) ) ;
#43633=CARTESIAN_POINT ( 'NONE',  ( -0.4724409448818890911, -0.1870078740157480879, -0.4822834645669291653 ) ) ;
#43634=CARTESIAN_POINT ( 'NONE',  ( -1.496062992125983815, -0.1870078740157479769, 0.4822834645669291653 ) ) ;
#43635=CARTESIAN_POINT ( 'NONE',  ( -0.9645669291338575535, -0.5400638737290844871, 0.3530559997133364547 ) ) ;
#43636=CARTESIAN_POINT ( 'NONE',  ( 0.7283464566929140904, -0.5400638737290845981, -0.3530559997133363437 ) ) ;
#43638=CARTESIAN_POINT ( 'NONE',  ( -0.2034120734908128059, 0.1771653543307087630, 0.09757992244046791164 ) ) ;
#43639=ORIENTED_EDGE ( 'NONE', *, *, #31494, .F. ) ;
#43642=CARTESIAN_POINT ( 'NONE',  ( -1.141732283464566011, -0.5511811023622047445, 6.969142054262312111E-17 ) ) ;
#43643=CARTESIAN_POINT ( 'NONE',  ( -0.8792650918635160906, -0.4281496062992124485, 0.4176697321401328655 ) ) ;
#43644=CARTESIAN_POINT ( 'NONE',  ( -0.9842519685039360366, 0.2952755905511811885, 0.000000000000000000 ) ) ;
#43646=CARTESIAN_POINT ( 'NONE',  ( -0.6364829396325453192, -0.3162353388693405765, 0.4822834645669290543 ) ) ;
#43647=CARTESIAN_POINT ( 'NONE',  ( -0.9055118110236215490, 0.2952755905511811885, 0.000000000000000000 ) ) ;
#43648=DIRECTION ( 'NONE',  ( -3.096699300667737957E-16, 1.000000000000000000, -0.000000000000000000 ) ) ;
#43649=CARTESIAN_POINT ( 'NONE',  ( -0.7137454485294953965, 2.001539355558159983, -0.4917280318828584074 ) ) ;
#43651=CARTESIAN_POINT ( 'NONE',  ( 0.4199475065616805614, 0.1283753931104748280, 0.1820866141732283561 ) ) ;
#43654=CARTESIAN_POINT ( 'NONE',  ( -0.1246719160104980823, 0.1771653543307087630, 0.09757992244046791164 ) ) ;
#43655=CARTESIAN_POINT ( 'NONE',  ( -0.2034120734908128059, 0.2952755905511811885, 0.1292274648535926551 ) ) ;
#43656=CARTESIAN_POINT ( 'NONE',  ( 1.174540682414699111, -0.05778040916215560624, -0.4822834645669293319 ) ) ;
#43657=CARTESIAN_POINT ( 'NONE',  ( -0.2099737532808391705, 0.2306618581243848609, 0.2411417322834645549 ) ) ;
#43664=CARTESIAN_POINT ( 'NONE',  ( -1.049868766404198794, 0.1283753931104746893, -0.1820866141732285504 ) ) ;
#43665=CARTESIAN_POINT ( 'NONE',  ( -1.541994750656167090, 0.2952755905511811885, 0.1292274648535926551 ) ) ;
#43667=DIRECTION ( 'NONE',  ( 0.000000000000000000, -1.000000000000000000, 0.000000000000000000 ) ) ;
#43669=CARTESIAN_POINT ( 'NONE',  ( 1.456692913385827515, -0.6692913385826771977, 8.415575281601705876E-17 ) ) ;
#43670=CARTESIAN_POINT ( 'NONE',  ( 0.3805774278215230400, 0.05413385826771626580, -0.4176697321401330321 ) ) ;
#43671=CARTESIAN_POINT ( 'NONE',  ( 0.2099737532808405305, -0.6046776061558807314, 0.2411417322834647770 ) ) ;
#43672=CARTESIAN_POINT ( 'NONE',  ( -0.9973753280839886548, 0.1283753931104748280, 0.1820866141732283561 ) ) ;
#43673=CARTESIAN_POINT ( 'NONE',  ( -0.2099737532808391705, -0.6046776061558809534, -0.2411417322834644161 ) ) ;
#43675=CARTESIAN_POINT ( 'NONE',  ( -0.9055118110236215490, 0.2952755905511811885, 0.000000000000000000 ) ) ;
#43677=CARTESIAN_POINT ( 'NONE',  ( 1.233595800524935227, -0.5023911411419708095, 0.1820866141732285504 ) ) ;
#43678=CARTESIAN_POINT ( 'NONE',  ( -0.1706036745406816491, -0.3690944881889763329, 0.3153832671262228327 ) ) ;
#43679=CARTESIAN_POINT ( 'NONE',  ( 1.102362204724410155, -0.1870078740157480601, -0.3641732283464567677 ) ) ;
#43680=CARTESIAN_POINT ( 'NONE',  ( -1.555118110236219930, 0.1660481256975885056, 0.3530559997133364547 ) ) ;
#43681=CARTESIAN_POINT ( 'NONE',  ( -1.010498687664041384, -0.004921259842519576551, 0.3153832671262227771 ) ) ;
#43683=CARTESIAN_POINT ( 'NONE',  ( 0.3543307086614181922, -0.5511811023622047445, 6.969142054262312111E-17 ) ) ;
#43684=CARTESIAN_POINT ( 'NONE',  ( -0.4921259842519677963, 0.1660481256975883668, -0.3530559997133364547 ) ) ;
#43685=CARTESIAN_POINT ( 'NONE',  ( 0.2952755905511819101, 0.1660481256975883391, -0.3530559997133364547 ) ) ;
#43686=CARTESIAN_POINT ( 'NONE',  ( -0.05905511811023545637, 0.07958543189024085140, 0.2665933059059887866 ) ) ;
#43688=CARTESIAN_POINT ( 'NONE',  ( 0.7217847769028878924, 0.05413385826771666132, 0.4176697321401328100 ) ) ;
#43690=CARTESIAN_POINT ( 'NONE',  ( 1.489501312335958172, -0.08942795157528024563, -0.3641732283464568787 ) ) ;
#43691=CARTESIAN_POINT ( 'NONE',  ( -1.135170603674539924, -0.6692913385826771977, 0.1292274648535927661 ) ) ;
#43692=CARTESIAN_POINT ( 'NONE',  ( -0.1181102362204717315, -0.5511811023622047445, 6.969142054262312111E-17 ) ) ;
#43694=CARTESIAN_POINT ( 'NONE',  ( 0.2099737532808405305, 0.1283753931104746893, -0.1820866141732285504 ) ) ;
#43695=CARTESIAN_POINT ( 'NONE',  ( -1.036745406824146176, 0.05413385826771626580, -0.4176697321401330321 ) ) ;
#43696=CARTESIAN_POINT ( 'NONE',  ( -0.3740157480314953431, 0.1660481256975885056, 0.3530559997133364547 ) ) ;
#43698=EDGE_CURVE ( 'NONE', #19860, #38268, #37030, .T. ) ;
#43700=CARTESIAN_POINT ( 'NONE',  ( 0.6758530183727039509, 0.1771653543307087075, -0.09757992244046823083 ) ) ;
#43701=CARTESIAN_POINT ( 'NONE',  ( -0.3412073490813641308, 0.2306618581243847221, -0.2411417322834647770 ) ) ;
#43703=CARTESIAN_POINT ( 'NONE',  ( -0.7020997375328074108, -0.05778040916215522460, 0.4822834645669289988 ) ) ;
#43704=CARTESIAN_POINT ( 'NONE',  ( -0.9842519685039360366, 0.1771653543307087630, 0.000000000000000000 ) ) ;
#43706=CARTESIAN_POINT ( 'NONE',  ( -0.2034120734908128059, 0.2952755905511811885, 0.1292274648535926551 ) ) ;
#43707=DIRECTION ( 'NONE',  ( -3.096699300667737957E-16, 1.000000000000000000, -0.000000000000000000 ) ) ;
#43708=CARTESIAN_POINT ( 'NONE',  ( -1.437007874015747477, 0.1660481256975883668, -0.3530559997133364547 ) ) ;
#43712=CARTESIAN_POINT ( 'NONE',  ( -1.614173228346456712, 2.401574803149606474, -0.1372047244094478091 ) ) ;
#43713=CARTESIAN_POINT ( 'NONE',  ( -1.423884514435694859, -0.3162353388693405765, 0.4822834645669290543 ) ) ;
#43714=CARTESIAN_POINT ( 'NONE',  ( -0.7611548556430438595, 0.2306618581243848609, 0.2411417322834645549 ) ) ;
#43715=CARTESIAN_POINT ( 'NONE',  ( 1.555118110236221041, -0.5400638737290844871, 0.3530559997133364547 ) ) ;
#43718=CARTESIAN_POINT ( 'NONE',  ( 0.9120734908136490793, 0.2952755905511810774, -0.1292274648535930714 ) ) ;
#43719=CARTESIAN_POINT ( 'NONE',  ( 0.3937007874015754361, -0.1870078740157479769, 0.4822834645669291653 ) ) ;
#43722=CARTESIAN_POINT ( 'NONE',  ( 1.272965879265092637, -0.004921259842519576551, 0.3153832671262227771 ) ) ;
#43726=ORIENTED_EDGE ( 'NONE', *, *, #58635, .F. ) ;
#43727=CARTESIAN_POINT ( 'NONE',  ( 0.4199475065616803948, -0.6046776061558809534, -0.2411417322834644161 ) ) ;
#43728=CARTESIAN_POINT ( 'NONE',  ( -0.7152230971128602510, -0.05778040916215560624, -0.4822834645669293319 ) ) ;
#43729=CARTESIAN_POINT ( 'NONE',  ( -1.568241469816272105, -0.3162353388693409650, -0.4822834645669289433 ) ) ;
#43730=CARTESIAN_POINT ( 'NONE',  ( 0.9580052493438327987, -0.4281496062992127816, -0.4176697321401328100 ) ) ;
#43731=CARTESIAN_POINT ( 'NONE',  ( 1.522309711286089939, 0.2306618581243848609, 0.2411417322834645549 ) ) ;
#43733=CARTESIAN_POINT ( 'NONE',  ( -0.03937007874015669567, 0.2952755905511811885, 0.000000000000000000 ) ) ;
#43734=CARTESIAN_POINT ( 'NONE',  ( -1.371391076115484609, -0.6692913385826771977, 0.1292274648535927661 ) ) ;
#43735=CARTESIAN_POINT ( 'NONE',  ( -1.653543307086613234, -0.1870078740157479769, 0.4822834645669291653 ) ) ;
#43736=CARTESIAN_POINT ( 'NONE',  ( 1.410761154855643795, -0.05778040916215560624, -0.4822834645669293319 ) ) ;
#43738=CARTESIAN_POINT ( 'NONE',  ( 0.9055118110236227702, 0.1771653543307087630, 0.000000000000000000 ) ) ;
#43739=VERTEX_POINT ( 'NONE', #30719 ) ;
#43741=ORIENTED_EDGE ( 'NONE', *, *, #24425, .F. ) ;
#43742=CARTESIAN_POINT ( 'NONE',  ( -0.2099737532808391705, -0.5023911411419708095, -0.1820866141732282451 ) ) ;
#43743=CARTESIAN_POINT ( 'NONE',  ( -1.686351706036744558, 0.2952755905511810774, -0.1292274648535930714 ) ) ;
#43744=CARTESIAN_POINT ( 'NONE',  ( 0.4002624671916016896, -0.3162353388693409650, -0.4822834645669289433 ) ) ;
#43745=CARTESIAN_POINT ( 'NONE',  ( 0.5511811023622054106, -0.1870078740157480879, -0.4822834645669291653 ) ) ;
#43746=CARTESIAN_POINT ( 'NONE',  ( -0.7349081364829390672, 0.2306618581243847221, -0.2411417322834647770 ) ) ;
#43748=CARTESIAN_POINT ( 'NONE',  ( -1.351706036745406347, -0.4281496062992124485, 0.4176697321401328655 ) ) ;
#43750=CARTESIAN_POINT ( 'NONE',  ( 1.377952755905512472, -0.5511811023622047445, 6.969142054262312111E-17 ) ) ;
#43751=CARTESIAN_POINT ( 'NONE',  ( -0.8923884514435688198, -0.6046776061558807314, 0.2411417322834647770 ) ) ;
#43752=CARTESIAN_POINT ( 'NONE',  ( 0.9842519685039378130, -0.6692913385826771977, 8.415575281601705876E-17 ) ) ;
#43753=CARTESIAN_POINT ( 'NONE',  ( 1.049868766404200349, 0.2306618581243848609, 0.2411417322834645549 ) ) ;
#43755=CARTESIAN_POINT ( 'NONE',  ( -1.253280839895012377, -0.05778040916215522460, 0.4822834645669289988 ) ) ;
#43757=CARTESIAN_POINT ( 'NONE',  ( 0.4068241469816279987, -0.4281496062992127816, -0.4176697321401328100 ) ) ;
#43761=CARTESIAN_POINT ( 'NONE',  ( -1.371391076115484609, -0.5511811023622046335, 0.09757992244046803654 ) ) ;
#43762=CARTESIAN_POINT ( 'NONE',  ( 0.2821522309711292364, 0.1771653543307087075, -0.09757992244046823083 ) ) ;
#43763=CARTESIAN_POINT ( 'NONE',  ( 0.8202099737532813073, 0.2952755905511811885, 0.1292274648535926551 ) ) ;
#43765=CARTESIAN_POINT ( 'NONE',  ( 0.6167979002624679463, -0.004921259842519870586, -0.3153832671262229437 ) ) ;
#43766=CARTESIAN_POINT ( 'NONE',  ( 0.3412073490813655186, 0.2306618581243848609, 0.2411417322834645549 ) ) ;
#43768=ADVANCED_FACE ( 'NONE', ( #16877 ), #28018, .F. ) ;
#43769=CARTESIAN_POINT ( 'NONE',  ( -0.6955380577427815458, -0.4281496062992127816, -0.4176697321401328100 ) ) ;
#43772=CARTESIAN_POINT ( 'NONE',  ( 1.003937007874016185, 0.07958543189024071263, -0.2665933059059888421 ) ) ;
#43774=CARTESIAN_POINT ( 'NONE',  ( -0.2165354330708654795, -0.5400638737290845981, -0.3530559997133363437 ) ) ;
#43775=CARTESIAN_POINT ( 'NONE',  ( 0.1640419947506569498, -0.2845877964562161244, -0.3641732283464567121 ) ) ;
#43777=CARTESIAN_POINT ( 'NONE',  ( -0.4724409448818890911, -0.1870078740157479769, 0.4822834645669291653 ) ) ;
#43778=CARTESIAN_POINT ( 'NONE',  ( 0.8005249343832027131, -0.004921259842519576551, 0.3153832671262227771 ) ) ;
#43779=B_SPLINE_CURVE_WITH_KNOTS ( 'NONE', 3,
 ( #2860, #34433, #47455, #8346 ),
 .UNSPECIFIED., .F., .F.,
 ( 4, 4 ),
 ( 0.02918618983606361197, 0.02943414011348784165 ),
 .UNSPECIFIED. ) ;
#43781=CARTESIAN_POINT ( 'NONE',  ( 0.2493438320209980519, 0.05413385826771666132, 0.4176697321401328100 ) ) ;
#43782=CARTESIAN_POINT ( 'NONE',  ( 1.161417322834646493, -0.4536011799217367080, 0.2665933059059888421 ) ) ;
#43784=CARTESIAN_POINT ( 'NONE',  ( -0.2362204724409442680, -0.1870078740157480601, -0.3641732283464567677 ) ) ;
#43785=CARTESIAN_POINT ( 'NONE',  ( -0.6692913385826764205, -0.5511811023622047445, 6.969142054262312111E-17 ) ) ;
#43786=CARTESIAN_POINT ( 'NONE',  ( -0.2624671916010490880, -0.6046776061558807314, 0.2411417322834647770 ) ) ;
#43787=CARTESIAN_POINT ( 'NONE',  ( 0.4921259842519691285, 0.1660481256975885056, 0.3530559997133364547 ) ) ;
#43788=CARTESIAN_POINT ( 'NONE',  ( 0.9186351706036752773, 0.1283753931104746893, -0.1820866141732285504 ) ) ;
#43789=CARTESIAN_POINT ( 'NONE',  ( -1.666666666666665853, -0.004921259842519870586, -0.3153832671262229437 ) ) ;
#43790=CARTESIAN_POINT ( 'NONE',  ( -1.686351706036744558, 0.2952755905511810774, -0.1292274648535930714 ) ) ;
#43791=CARTESIAN_POINT ( 'NONE',  ( 0.8202099737532814183, -0.6692913385826773087, -0.1292274648535924053 ) ) ;
#43793=CARTESIAN_POINT ( 'NONE',  ( -0.06561679790026180015, -0.4281496062992127816, -0.4176697321401328100 ) ) ;
#43796=CARTESIAN_POINT ( 'NONE',  ( 0.8989501312335964611, 0.2952755905511811885, 0.1292274648535926551 ) ) ;
#43798=CARTESIAN_POINT ( 'NONE',  ( 0.3740157480314966754, -0.5400638737290844871, 0.3530559997133364547 ) ) ;
#43800=CARTESIAN_POINT ( 'NONE',  ( 0.4527559055118117182, 0.07958543189024071263, -0.2665933059059888421 ) ) ;
#43801=CARTESIAN_POINT ( 'NONE',  ( 1.003937007874016407, -0.5400638737290844871, 0.3530559997133364547 ) ) ;
#43802=CARTESIAN_POINT ( 'NONE',  ( 0.1049868766404206816, -0.5023911411419708095, -0.1820866141732282451 ) ) ;
#43803=CARTESIAN_POINT ( 'NONE',  ( -0.4724409448818890911, -0.1870078740157480879, -0.4822834645669291653 ) ) ;
#43805=CARTESIAN_POINT ( 'NONE',  ( 0.06561679790026316017, 0.05413385826771626580, -0.4176697321401330321 ) ) ;
#43806=CARTESIAN_POINT ( 'NONE',  ( -0.9186351706036736120, -0.6046776061558809534, -0.2411417322834644161 ) ) ;
#43807=CARTESIAN_POINT ( 'NONE',  ( -0.3412073490813641308, -0.5023911411419708095, 0.1820866141732285504 ) ) ;
#43808=CARTESIAN_POINT ( 'NONE',  ( 0.3018372703412079971, -0.4281496062992124485, 0.4176697321401328655 ) ) ;
#43809=CARTESIAN_POINT ( 'NONE',  ( 0.8070866141732289112, -0.4536011799217368745, -0.2665933059059886201 ) ) ;
#43810=CARTESIAN_POINT ( 'NONE',  ( -0.2690288713910754526, -0.6692913385826771977, 0.1292274648535927661 ) ) ;
#43812=CARTESIAN_POINT ( 'NONE',  ( 1.417322834645670104, -0.1870078740157479769, 0.4822834645669291653 ) ) ;
#43813=CARTESIAN_POINT ( 'NONE',  ( 1.679790026246720025, 0.2306618581243848609, 0.2411417322834645549 ) ) ;
#43815=CARTESIAN_POINT ( 'NONE',  ( -1.056430446194224881, -0.6692913385826771977, 0.1292274648535927661 ) ) ;
#43817=CARTESIAN_POINT ( 'NONE',  ( -0.7414698162729651543, 0.2952755905511810774, -0.1292274648535930714 ) ) ;
#43820=ORIENTED_EDGE ( 'NONE', *, *, #52674, .F. ) ;
#43821=CARTESIAN_POINT ( 'NONE',  ( 0.4265091863517067594, 0.1771653543307087630, 0.09757992244046791164 ) ) ;
#43823=CARTESIAN_POINT ( 'NONE',  ( 0.7874015748031503170, -0.1870078740157479769, 0.4822834645669291653 ) ) ;
#43825=CARTESIAN_POINT ( 'NONE',  ( 0.9711286089238851948, 0.2306618581243848609, 0.2411417322834645549 ) ) ;
#43826=CARTESIAN_POINT ( 'NONE',  ( -0.5118110236220466680, 0.1771653543307087630, 0.000000000000000000 ) ) ;
#43828=CARTESIAN_POINT ( 'NONE',  ( 1.003937007874016407, -0.5400638737290844871, 0.3530559997133364547 ) ) ;
#43829=ADVANCED_FACE ( 'NONE', ( #76807 ), #19403, .F. ) ;
#43830=CARTESIAN_POINT ( 'NONE',  ( 1.509186351706037543, -0.3690944881889765550, -0.3153832671262227771 ) ) ;
#43831=CARTESIAN_POINT ( 'NONE',  ( 0.1902887139107617975, -0.6692913385826773087, -0.1292274648535924053 ) ) ;
#43834=CARTESIAN_POINT ( 'NONE',  ( -0.5708661417322825615, -0.5400638737290844871, 0.3530559997133364547 ) ) ;
#43835=CARTESIAN_POINT ( 'NONE',  ( -1.299212598425196097, -0.5511811023622047445, 6.969142054262312111E-17 ) ) ;
#43836=CARTESIAN_POINT ( 'NONE',  ( -0.4593175853018366950, 0.05413385826771666132, 0.4176697321401328100 ) ) ;
#43837=EDGE_CURVE ( 'NONE', #71206, #65960, #75436, .T. ) ;
#43842=CARTESIAN_POINT ( 'NONE',  ( 0.3149606299212606708, -0.1870078740157480879, -0.4822834645669291653 ) ) ;
#43844=CARTESIAN_POINT ( 'NONE',  ( -0.2952755905511804668, 0.1660481256975885056, 0.3530559997133364547 ) ) ;
#43845=CARTESIAN_POINT ( 'NONE',  ( -1.489501312335957062, -0.05778040916215522460, 0.4822834645669289988 ) ) ;
#43846=CARTESIAN_POINT ( 'NONE',  ( 0.5643044619422579178, -0.4281496062992127816, -0.4176697321401328100 ) ) ;
#43847=CARTESIAN_POINT ( 'NONE',  ( 0.1049868766404206816, 0.2306618581243848609, 0.2411417322834645549 ) ) ;
#43849=CARTESIAN_POINT ( 'NONE',  ( -0.9514435695538050464, -0.3162353388693405765, 0.4822834645669290543 ) ) ;
#43850=CARTESIAN_POINT ( 'NONE',  ( 0.3149606299212606708, -0.1870078740157480879, -0.4822834645669291653 ) ) ;
#43851=CARTESIAN_POINT ( 'NONE',  ( -0.2821522309711278487, -0.6692913385826773087, -0.1292274648535924053 ) ) ;
#43852=CARTESIAN_POINT ( 'NONE',  ( 0.1968503937007881344, -0.5511811023622047445, 6.969142054262312111E-17 ) ) ;
#43854=CARTESIAN_POINT ( 'NONE',  ( -0.1181102362204717315, 0.2952755905511811885, 0.000000000000000000 ) ) ;
#43855=CARTESIAN_POINT ( 'NONE',  ( 1.614173228346457378, 0.2753471884572480932, -0.1372047244094471152 ) ) ;
#43856=CARTESIAN_POINT ( 'NONE',  ( -1.587926509186350810, 0.05413385826771626580, -0.4176697321401330321 ) ) ;
#43860=ORIENTED_EDGE ( 'NONE', *, *, #47547, .F. ) ;
#43862=CARTESIAN_POINT ( 'NONE',  ( 0.8005249343832028242, -0.4281496062992127816, -0.4176697321401328100 ) ) ;
#43863=CARTESIAN_POINT ( 'NONE',  ( 0.01312335958005323398, -0.004921259842519576551, 0.3153832671262227771 ) ) ;
#43864=AXIS2_PLACEMENT_3D ( 'NONE', #41555, #65589, #79883 ) ;
#43866=CARTESIAN_POINT ( 'NONE',  ( 1.279527559055118724, -0.4536011799217368745, -0.2665933059059886201 ) ) ;
#43867=DIRECTION ( 'NONE',  ( 0.000000000000000000, 0.000000000000000000, -1.000000000000000000 ) ) ;
#43873=CARTESIAN_POINT ( 'NONE',  ( 0.4133858267716541968, -0.5400638737290845981, -0.3530559997133363437 ) ) ;
#43874=CARTESIAN_POINT ( 'NONE',  ( -1.082677165354329896, -0.5400638737290845981, -0.3530559997133363437 ) ) ;
#43875=CARTESIAN_POINT ( 'NONE',  ( -1.082677165354329896, 0.1660481256975885056, 0.3530559997133364547 ) ) ;
#43876=CARTESIAN_POINT ( 'NONE',  ( 0.2165354330708668673, 0.1660481256975883668, -0.3530559997133364547 ) ) ;
#43877=CARTESIAN_POINT ( 'NONE',  ( 1.030183727034121421, -0.3162353388693409650, -0.4822834645669289433 ) ) ;
#43878=CARTESIAN_POINT ( 'NONE',  ( 1.312335958005250269, -0.5023911411419708095, 0.1820866141732285504 ) ) ;
#43880=CARTESIAN_POINT ( 'NONE',  ( 1.154855643044620184, -0.5023911411419708095, 0.1820866141732285504 ) ) ;
#43881=CARTESIAN_POINT ( 'NONE',  ( -0.8792650918635160906, -0.4281496062992124485, 0.4176697321401328655 ) ) ;
#43883=CARTESIAN_POINT ( 'NONE',  ( -1.581364829396324945, -0.08942795157528024563, -0.3641732283464568787 ) ) ;
#43885=CARTESIAN_POINT ( 'NONE',  ( -0.07217847769028787330, -0.05778040916215522460, 0.4822834645669289988 ) ) ;
#43887=CARTESIAN_POINT ( 'NONE',  ( 1.358267716535433323, 0.1660481256975885056, 0.3530559997133364547 ) ) ;
#43889=CARTESIAN_POINT ( 'NONE',  ( -1.437007874015747477, -0.4536011799217367080, 0.2665933059059888421 ) ) ;
#43890=CARTESIAN_POINT ( 'NONE',  ( 8.195543980992789655E-16, -0.1870078740157480879, -0.4822834645669291653 ) ) ;
#43891=CARTESIAN_POINT ( 'NONE',  ( 0.6824146981627303710, 0.1283753931104746893, -0.1820866141732285504 ) ) ;
#43892=CARTESIAN_POINT ( 'NONE',  ( -1.614173228346456268, -0.5511811023622047445, 6.969142054262312111E-17 ) ) ;
#43893=CARTESIAN_POINT ( 'NONE',  ( 0.8858267716535438430, 0.1660481256975885056, 0.3530559997133364547 ) ) ;
#43895=CARTESIAN_POINT ( 'NONE',  ( -0.6561679790026240244, -0.5023911411419708095, 0.1820866141732285504 ) ) ;
#43896=CARTESIAN_POINT ( 'NONE',  ( -0.7217847769028863381, 0.05413385826771626580, -0.4176697321401330321 ) ) ;
#43897=CARTESIAN_POINT ( 'NONE',  ( 1.482939632545932307, -0.4281496062992124485, 0.4176697321401328655 ) ) ;
#43898=CARTESIAN_POINT ( 'NONE',  ( -1.292650918635170010, -0.6692913385826771977, 0.1292274648535927661 ) ) ;
#43899=CARTESIAN_POINT ( 'NONE',  ( 1.200787401574803681, 0.1660481256975885056, 0.3530559997133364547 ) ) ;
#43901=CARTESIAN_POINT ( 'NONE',  ( -1.213910761154854745, -0.5511811023622046335, 0.09757992244046803654 ) ) ;
#43902=CARTESIAN_POINT ( 'NONE',  ( -1.646051170424378096, 0.8346805926620876059, -0.5309055118110233007 ) ) ;
#43903=CARTESIAN_POINT ( 'NONE',  ( 1.259842519685040019, -0.1870078740157479769, 0.4822834645669291653 ) ) ;
#43905=CARTESIAN_POINT ( 'NONE',  ( -1.476377952755905110, -0.5400638737290845981, -0.3530559997133363437 ) ) ;
#43906=CARTESIAN_POINT ( 'NONE',  ( -1.587926509186350810, -0.004921259842519870586, -0.3153832671262229437 ) ) ;
#43907=CARTESIAN_POINT ( 'NONE',  ( -1.056430446194224881, 0.1771653543307087075, -0.09757992244046823083 ) ) ;
#43909=CARTESIAN_POINT ( 'NONE',  ( -0.3346456692913377662, 0.1660481256975883668, -0.3530559997133364547 ) ) ;
#43910=CARTESIAN_POINT ( 'NONE',  ( -0.05249343832020911260, 0.1283753931104748280, 0.1820866141732283561 ) ) ;
#43911=CARTESIAN_POINT ( 'NONE',  ( -1.358267716535432434, 0.07958543189024071263, -0.2665933059059888421 ) ) ;
#43912=CARTESIAN_POINT ( 'NONE',  ( 1.292650918635171564, 0.1771653543307087630, 0.09757992244046791164 ) ) ;
#43913=B_SPLINE_CURVE_WITH_KNOTS ( 'NONE', 3,
 ( #11086, #61601, #30433, #56098, #36743, #18231, #12324 ),
 .UNSPECIFIED., .F., .F.,
 ( 4, 3, 4 ),
 ( 0.000000000000000000, 0.001246232571205272213, 0.002492492258783270652 ),
 .UNSPECIFIED. ) ;
#43914=CARTESIAN_POINT ( 'NONE',  ( 1.056430446194226658, 0.2952755905511811885, 0.1292274648535926551 ) ) ;
#43915=FACE_OUTER_BOUND ( 'NONE', #71821, .T. ) ;
#43916=CARTESIAN_POINT ( 'NONE',  ( 0.07217847769028949700, -0.2845877964562159024, 0.3641732283464567677 ) ) ;
#43917=CARTESIAN_POINT ( 'NONE',  ( 0.4724409448818904789, -0.1870078740157480879, -0.4822834645669291653 ) ) ;
#43918=CARTESIAN_POINT ( 'NONE',  ( 1.108923884514436242, -0.08942795157527998196, 0.3641732283464567121 ) ) ;
#43921=CARTESIAN_POINT ( 'NONE',  ( 1.469816272965879911, 0.2306618581243847221, -0.2411417322834647770 ) ) ;
#43922=EDGE_CURVE ( 'NONE', #29775, #44273, #3641, .T. ) ;
#43923=CARTESIAN_POINT ( 'NONE',  ( -1.391076115485563314, -0.6046776061558809534, -0.2411417322834644161 ) ) ;
#43924=CARTESIAN_POINT ( 'NONE',  ( -0.2559055118110230564, 0.1660481256975883668, -0.3530559997133364547 ) ) ;
#43925=AXIS2_PLACEMENT_3D ( 'NONE', #27255, #48576, #20953 ) ;
#43928=CARTESIAN_POINT ( 'NONE',  ( 0.5839895013123367340, -0.6692913385826773087, -0.1292274648535924053 ) ) ;
#43929=CARTESIAN_POINT ( 'NONE',  ( 1.089238845144357537, -0.3690944881889763329, 0.3153832671262228327 ) ) ;
#43931=AXIS2_PLACEMENT_3D ( 'NONE', #63717, #69219, #18698 ) ;
#43932=CARTESIAN_POINT ( 'NONE',  ( -0.1049868766404193215, -0.6046776061558807314, 0.2411417322834647770 ) ) ;
#43933=CARTESIAN_POINT ( 'NONE',  ( 0.4658792650918640033, -0.3162353388693405765, 0.4822834645669290543 ) ) ;
#43939=CARTESIAN_POINT ( 'NONE',  ( -0.5183727034120726440, -0.5511811023622048555, -0.09757992244046775898 ) ) ;
#43940=CARTESIAN_POINT ( 'NONE',  ( -0.9186351706036736120, 0.2306618581243848609, 0.2411417322834645549 ) ) ;
#43942=CARTESIAN_POINT ( 'NONE',  ( 0.7086614173228353852, -0.1870078740157479769, 0.4822834645669291653 ) ) ;
#43943=CARTESIAN_POINT ( 'NONE',  ( -1.489501312335957062, -0.05778040916215522460, 0.4822834645669289988 ) ) ;
#43944=CARTESIAN_POINT ( 'NONE',  ( 0.8792650918635177559, -0.4281496062992127816, -0.4176697321401328100 ) ) ;
#43947=CARTESIAN_POINT ( 'NONE',  ( 1.509186351706037543, 0.05413385826771666132, 0.4176697321401328100 ) ) ;
#43948=CARTESIAN_POINT ( 'NONE',  ( 1.056430446194226436, -0.6692913385826773087, -0.1292274648535924053 ) ) ;
#43949=CARTESIAN_POINT ( 'NONE',  ( 0.4133858267716541968, -0.5400638737290845981, -0.3530559997133363437 ) ) ;
#43950=CARTESIAN_POINT ( 'NONE',  ( 1.417322834645670104, -0.1870078740157479769, 0.3641732283464567677 ) ) ;
#43951=CARTESIAN_POINT ( 'NONE',  ( 1.279527559055118724, -0.5400638737290845981, -0.3530559997133363437 ) ) ;
#43954=CARTESIAN_POINT ( 'NONE',  ( 1.003937007874016407, -0.5400638737290844871, 0.3530559997133364547 ) ) ;
#43955=CARTESIAN_POINT ( 'NONE',  ( 1.646981627296588035, -0.2845877964562159024, 0.3641732283464567677 ) ) ;
#43956=CARTESIAN_POINT ( 'NONE',  ( -0.4658792650918627265, -0.05778040916215522460, 0.4822834645669289988 ) ) ;
#43957=CARTESIAN_POINT ( 'NONE',  ( -1.122047244094487306, -0.5400638737290844871, 0.3530559997133364547 ) ) ;
#43958=CARTESIAN_POINT ( 'NONE',  ( 1.305774278215223960, 0.2952755905511810774, -0.1292274648535930714 ) ) ;
#43962=CARTESIAN_POINT ( 'NONE',  ( 1.614173228346457378, -0.6692913385826771977, 8.415575281601705876E-17 ) ) ;
#43963=ORIENTED_EDGE ( 'NONE', *, *, #76698, .T. ) ;
#43966=CARTESIAN_POINT ( 'NONE',  ( -1.614173228346457378, 0.4410134679336882302, 0.1372047244094476981 ) ) ;
#43967=CARTESIAN_POINT ( 'NONE',  ( 1.404199475065617264, -0.3690944881889763329, 0.3153832671262228327 ) ) ;
#43969=CARTESIAN_POINT ( 'NONE',  ( 1.469816272965879911, -0.5023911411419708095, 0.1820866141732285504 ) ) ;
#43970=CARTESIAN_POINT ( 'NONE',  ( 0.6195821328811250694, 1.702998256715020864E-15, -0.4281989832122452544 ) ) ;
#43971=CARTESIAN_POINT ( 'NONE',  ( 0.4665770185116075996, 1.519790403714398552, 0.5309055118110234117 ) ) ;
#43974=CARTESIAN_POINT ( 'NONE',  ( -0.6955380577427815458, -0.004921259842519576551, 0.3153832671262227771 ) ) ;
#43975=CARTESIAN_POINT ( 'NONE',  ( -1.246719160104986512, -0.004921259842519576551, 0.3153832671262227771 ) ) ;
#43976=CARTESIAN_POINT ( 'NONE',  ( -1.200787401574802349, -0.5400638737290844871, 0.3530559997133364547 ) ) ;
#43977=CARTESIAN_POINT ( 'NONE',  ( 0.3018372703412079971, -0.4281496062992124485, 0.4176697321401328655 ) ) ;
#43978=CARTESIAN_POINT ( 'NONE',  ( 1.574803149606299746, -0.1870078740157479769, 0.4822834645669291653 ) ) ;
#43979=ORIENTED_EDGE ( 'NONE', *, *, #26454, .F. ) ;
#43980=CARTESIAN_POINT ( 'NONE',  ( 1.318897637795276356, 0.1660481256975883668, -0.3530559997133364547 ) ) ;
#43984=CARTESIAN_POINT ( 'NONE',  ( -1.586052503253848167, 1.023622047244095556, -0.1653254495020564929 ) ) ;
#43985=CARTESIAN_POINT ( 'NONE',  ( -0.5511811023622038563, -0.1870078740157479769, 0.3641732283464567677 ) ) ;
#43987=CARTESIAN_POINT ( 'NONE',  ( -1.030183727034119867, -0.3162353388693405765, 0.4822834645669290543 ) ) ;
#43988=CARTESIAN_POINT ( 'NONE',  ( 1.167979002624672580, -0.4281496062992124485, 0.4176697321401328655 ) ) ;
#43990=ORIENTED_EDGE ( 'NONE', *, *, #4442, .F. ) ;
#43991=DIRECTION ( 'NONE',  ( -1.000000000000000000, 0.000000000000000000, 0.000000000000000000 ) ) ;
#43994=CARTESIAN_POINT ( 'NONE',  ( -1.586052503253848167, 1.023622047244095556, -0.1653254495020564929 ) ) ;
#43995=CARTESIAN_POINT ( 'NONE',  ( -1.056430446194224881, 0.2952755905511810774, -0.1292274648535930714 ) ) ;
#43997=CARTESIAN_POINT ( 'NONE',  ( -0.5314960629921254842, -0.4536011799217368745, -0.2665933059059886201 ) ) ;
#44000=CARTESIAN_POINT ( 'NONE',  ( -0.3871391076115476282, -0.08942795157527998196, 0.3641732283464567121 ) ) ;
#44001=CARTESIAN_POINT ( 'NONE',  ( 0.3608923884514443348, 0.1771653543307087075, -0.09757992244046823083 ) ) ;
#44002=CARTESIAN_POINT ( 'NONE',  ( 0.05249343832021075018, 0.2306618581243847221, -0.2411417322834647770 ) ) ;
#44003=CARTESIAN_POINT ( 'NONE',  ( -0.5839895013123351797, -0.5511811023622046335, 0.09757992244046803654 ) ) ;
#44005=CARTESIAN_POINT ( 'NONE',  ( 0.9711286089238851948, 0.2306618581243848609, 0.2411417322834645549 ) ) ;
#44006=CARTESIAN_POINT ( 'NONE',  ( -1.135170603674539924, 0.2952755905511810774, -0.1292274648535930714 ) ) ;
#44008=CARTESIAN_POINT ( 'NONE',  ( -0.5511811023622041894, -0.1870078740157480879, -0.4822834645669291653 ) ) ;
#44009=CARTESIAN_POINT ( 'NONE',  ( -0.8136482939632537770, 0.2306618581243847221, -0.2411417322834647770 ) ) ;
#44010=CARTESIAN_POINT ( 'NONE',  ( 1.194225721784777594, -0.004921259842519576551, 0.3153832671262227771 ) ) ;
#44011=CARTESIAN_POINT ( 'NONE',  ( 0.1837270341207354329, 0.1283753931104748280, 0.1820866141732283561 ) ) ;
#44012=CARTESIAN_POINT ( 'NONE',  ( -0.7677165354330699465, 0.1660481256975885056, 0.3530559997133364547 ) ) ;
#44013=CARTESIAN_POINT ( 'NONE',  ( -1.200787401574802349, -0.5400638737290844871, 0.3530559997133364547 ) ) ;
#44014=CARTESIAN_POINT ( 'NONE',  ( -0.7974104941589342799, -2.567464376874931580E-15, -0.4445507791589072832 ) ) ;
#44016=CARTESIAN_POINT ( 'NONE',  ( -0.3871391076115476282, -0.05778040916215522460, 0.4822834645669289988 ) ) ;
#44017=CARTESIAN_POINT ( 'NONE',  ( -1.030183727034119867, -0.05778040916215560624, -0.4822834645669293319 ) ) ;
#44021=CARTESIAN_POINT ( 'NONE',  ( 1.213910761154856299, -0.6692913385826773087, -0.1292274648535924053 ) ) ;
#44022=CARTESIAN_POINT ( 'NONE',  ( -0.4921259842519677963, -0.4536011799217367080, 0.2665933059059888421 ) ) ;
#44023=CARTESIAN_POINT ( 'NONE',  ( -0.7874015748031489847, -0.1870078740157479769, 0.4822834645669291653 ) ) ;
#44024=CARTESIAN_POINT ( 'NONE',  ( 1.095800524934383846, -0.05778040916215560624, -0.4822834645669293319 ) ) ;
#44025=CARTESIAN_POINT ( 'NONE',  ( 0.7349081364829403995, 0.2306618581243848609, 0.2411417322834645549 ) ) ;
#44027=CARTESIAN_POINT ( 'NONE',  ( -0.9186351706036736120, 0.1283753931104748280, 0.1820866141732283561 ) ) ;
#44033=CARTESIAN_POINT ( 'NONE',  ( 1.148293963254593875, -0.5511811023622046335, 0.09757992244046803654 ) ) ;
#44034=CARTESIAN_POINT ( 'NONE',  ( 0.7414698162729663755, -0.5511811023622048555, -0.09757992244046775898 ) ) ;
#44035=CARTESIAN_POINT ( 'NONE',  ( 0.6364829396325465405, -0.05778040916215522460, 0.4822834645669289988 ) ) ;
#44038=CARTESIAN_POINT ( 'NONE',  ( 0.9055118110236227702, 0.1771653543307087630, 0.000000000000000000 ) ) ;
#44039=CARTESIAN_POINT ( 'NONE',  ( -0.3937007874015740483, -0.1870078740157479769, 0.4822834645669291653 ) ) ;
#44040=CARTESIAN_POINT ( 'NONE',  ( -1.332020997375327642, -0.05778040916215522460, 0.4822834645669289988 ) ) ;
#44041=CARTESIAN_POINT ( 'NONE',  ( 1.417322834645670104, -0.1870078740157480879, -0.4822834645669291653 ) ) ;
#44045=CARTESIAN_POINT ( 'NONE',  ( -0.02624671916010428221, -0.5023911411419708095, 0.1820866141732285504 ) ) ;
#44046=ORIENTED_EDGE ( 'NONE', *, *, #42996, .F. ) ;
#44048=CARTESIAN_POINT ( 'NONE',  ( -0.8202099737532801971, -0.6692913385826771977, 0.1292274648535927661 ) ) ;
#44049=CARTESIAN_POINT ( 'NONE',  ( -0.5183727034120726440, 0.2952755905511811885, 0.1292274648535926551 ) ) ;
#44050=CARTESIAN_POINT ( 'NONE',  ( -0.7020997375328074108, -0.05778040916215522460, 0.4822834645669289988 ) ) ;
#44051=CARTESIAN_POINT ( 'NONE',  ( 0.3871391076115493490, -0.3162353388693405765, 0.4822834645669290543 ) ) ;
#44052=CARTESIAN_POINT ( 'NONE',  ( -0.3083989501312330295, -0.3162353388693409650, -0.4822834645669289433 ) ) ;
#44053=CARTESIAN_POINT ( 'NONE',  ( -1.535433070866141225, -0.6692913385826771977, 8.415575281601705876E-17 ) ) ;
#44054=CARTESIAN_POINT ( 'NONE',  ( -0.6955380577427815458, -0.4281496062992127816, -0.4176697321401328100 ) ) ;
#44055=CARTESIAN_POINT ( 'NONE',  ( 0.8464566929133865436, 0.1660481256975883668, -0.3530559997133364547 ) ) ;
#44057=CARTESIAN_POINT ( 'NONE',  ( -0.4921259842519677963, 0.07958543189024071263, -0.2665933059059888421 ) ) ;
#44060=ORIENTED_EDGE ( 'NONE', *, *, #81623, .T. ) ;
#44061=CARTESIAN_POINT ( 'NONE',  ( -1.259842519685038686, -0.1870078740157479769, 0.3641732283464567677 ) ) ;
#44062=CARTESIAN_POINT ( 'NONE',  ( -1.181102362204723644, -0.1870078740157479769, 0.4822834645669291653 ) ) ;
#44063=CARTESIAN_POINT ( 'NONE',  ( -0.8989501312335946848, -0.6692913385826771977, 0.1292274648535927661 ) ) ;
#44065=CARTESIAN_POINT ( 'NONE',  ( -1.272965879265091305, -0.4281496062992124485, 0.4176697321401328655 ) ) ;
#44066=CARTESIAN_POINT ( 'NONE',  ( -0.9448818897637790704, -0.1870078740157479769, 0.4822834645669291653 ) ) ;
#44070=CARTESIAN_POINT ( 'NONE',  ( 0.5708661417322842269, 0.07958543189024085140, 0.2665933059059887866 ) ) ;
#44071=FACE_OUTER_BOUND ( 'NONE', #78580, .T. ) ;
#44073=CARTESIAN_POINT ( 'NONE',  ( 0.2559055118110243332, -0.4536011799217368745, -0.2665933059059886201 ) ) ;
#44074=CARTESIAN_POINT ( 'NONE',  ( -0.4002624671916004129, -0.3162353388693405765, 0.4822834645669290543 ) ) ;
#44075=CARTESIAN_POINT ( 'NONE',  ( 1.279527559055118724, 0.1660481256975885056, 0.3530559997133364547 ) ) ;
#44076=CARTESIAN_POINT ( 'NONE',  ( -0.6692913385826764205, 0.2952755905511811885, 0.000000000000000000 ) ) ;
#44077=VERTEX_POINT ( 'NONE', #54553 ) ;
#44079=CARTESIAN_POINT ( 'NONE',  ( -0.8202099737532798640, 0.2066929133858267098, -0.1054918080437494132 ) ) ;
#44080=ORIENTED_EDGE ( 'NONE', *, *, #33686, .T. ) ;
#44082=CARTESIAN_POINT ( 'NONE',  ( 1.108923884514436242, -0.05778040916215522460, 0.4822834645669289988 ) ) ;
#44083=CARTESIAN_POINT ( 'NONE',  ( -0.9448818897637790704, -0.1870078740157479769, 0.3641732283464567677 ) ) ;
#44084=CARTESIAN_POINT ( 'NONE',  ( -1.187664041994750175, -0.05778040916215560624, -0.4822834645669293319 ) ) ;
#44088=CARTESIAN_POINT ( 'NONE',  ( 1.509186351706037543, 0.05413385826771666132, 0.4176697321401328100 ) ) ;
#44090=CARTESIAN_POINT ( 'NONE',  ( 0.1312335958005257930, 0.2306618581243847221, -0.2411417322834647770 ) ) ;
#44091=CARTESIAN_POINT ( 'NONE',  ( -0.9776902887139098386, 0.1771653543307087075, -0.09757992244046823083 ) ) ;
#44092=CARTESIAN_POINT ( 'NONE',  ( -0.3674540682414692561, -0.6046776061558809534, -0.2411417322834644161 ) ) ;
#44094=CARTESIAN_POINT ( 'NONE',  ( -0.7677165354330699465, 0.1660481256975885056, 0.3530559997133364547 ) ) ;
#44097=CARTESIAN_POINT ( 'NONE',  ( 1.102362204724410155, -0.1870078740157479769, 0.3641732283464567677 ) ) ;
#44098=CARTESIAN_POINT ( 'NONE',  ( -0.1509186351706028884, -0.08942795157527998196, 0.3641732283464567121 ) ) ;
#44099=CARTESIAN_POINT ( 'NONE',  ( 0.9383202099737538715, -0.08942795157528024563, -0.3641732283464568787 ) ) ;
#44100=CARTESIAN_POINT ( 'NONE',  ( -1.502624671916009680, -0.05778040916215560624, -0.4822834645669293319 ) ) ;
#44102=CARTESIAN_POINT ( 'NONE',  ( 0.5708661417322842269, 0.07958543189024085140, 0.2665933059059887866 ) ) ;
#44103=CARTESIAN_POINT ( 'NONE',  ( -0.9055118110236215490, -0.6692913385826771977, 8.415575281601705876E-17 ) ) ;
#44106=CARTESIAN_POINT ( 'NONE',  ( -0.03280839895013062252, 0.1771653543307087075, -0.09757992244046823083 ) ) ;
#44107=CARTESIAN_POINT ( 'NONE',  ( -1.699475065616797398, 0.1771653543307087630, 0.09757992244046791164 ) ) ;
#44108=CARTESIAN_POINT ( 'NONE',  ( 0.6758530183727039509, -0.6692913385826771977, 0.1292274648535927661 ) ) ;
#44110=CARTESIAN_POINT ( 'NONE',  ( 1.325459317585302665, -0.004921259842519870586, -0.3153832671262229437 ) ) ;
#44111=CARTESIAN_POINT ( 'NONE',  ( -1.410761154855642463, -0.05778040916215522460, 0.4822834645669289988 ) ) ;
#44112=CARTESIAN_POINT ( 'NONE',  ( -0.4002624671916004129, -0.2845877964562159024, 0.3641732283464567677 ) ) ;
#44113=CYLINDRICAL_SURFACE ( 'NONE', #67713, 0.3937007874015748254 ) ;
#44114=CARTESIAN_POINT ( 'NONE',  ( 0.02624671916010564918, 0.1283753931104748280, 0.1820866141732283561 ) ) ;
#44115=CARTESIAN_POINT ( 'NONE',  ( -1.253280839895012377, -0.05778040916215522460, 0.4822834645669289988 ) ) ;
#44116=CARTESIAN_POINT ( 'NONE',  ( -0.6824146981627288167, 0.2306618581243848609, 0.2411417322834645549 ) ) ;
#44119=CARTESIAN_POINT ( 'NONE',  ( 0.6955380577427828781, -0.004921259842519870586, -0.3153832671262229437 ) ) ;
#44120=CARTESIAN_POINT ( 'NONE',  ( -0.5380577427821514602, 0.05413385826771666132, 0.4176697321401328100 ) ) ;
#44121=CARTESIAN_POINT ( 'NONE',  ( -0.5380577427821514602, 0.05413385826771666132, 0.4176697321401328100 ) ) ;
#44122=CARTESIAN_POINT ( 'NONE',  ( -0.8070866141732276899, 0.07958543189024071263, -0.2665933059059888421 ) ) ;
#44124=CARTESIAN_POINT ( 'NONE',  ( 0.1443569553805781891, 0.05413385826771626580, -0.4176697321401330321 ) ) ;
#44125=CARTESIAN_POINT ( 'NONE',  ( 1.614173228346457156, 1.929133858267716661, -0.5309055118110239668 ) ) ;
#44126=CARTESIAN_POINT ( 'NONE',  ( -1.430446194225720724, 0.05413385826771626580, -0.4176697321401330321 ) ) ;
#44130=CARTESIAN_POINT ( 'NONE',  ( 1.614173228346457378, 1.055049524192302579, -0.1372047244094476148 ) ) ;
#44131=CARTESIAN_POINT ( 'NONE',  ( -1.154855643044618851, -0.6046776061558809534, -0.2411417322834644161 ) ) ;
#44132=CARTESIAN_POINT ( 'NONE',  ( -1.023622047244094002, -0.1870078740157480879, -0.4822834645669291653 ) ) ;
#44133=CARTESIAN_POINT ( 'NONE',  ( -1.607611548556429737, 0.2952755905511810774, -0.1292274648535930714 ) ) ;
#44136=CARTESIAN_POINT ( 'NONE',  ( 0.7480314960629927956, 0.2952755905511811885, 0.000000000000000000 ) ) ;
#44137=CARTESIAN_POINT ( 'NONE',  ( 0.1771653543307093182, -0.5400638737290845981, -0.3530559997133363437 ) ) ;
#44139=LINE ( 'NONE', #12180, #8940 ) ;
#44140=CARTESIAN_POINT ( 'NONE',  ( 1.397637795275591177, -0.4536011799217367080, 0.2665933059059888421 ) ) ;
#44145=CARTESIAN_POINT ( 'NONE',  ( 0.2624671916010504757, -0.6046776061558809534, -0.2411417322834644161 ) ) ;
#44146=CARTESIAN_POINT ( 'NONE',  ( -0.8136482939632537770, -0.6046776061558807314, 0.2411417322834647770 ) ) ;
#44147=CARTESIAN_POINT ( 'NONE',  ( -1.430446194225720724, 0.05413385826771626580, -0.4176697321401330321 ) ) ;
#44148=CARTESIAN_POINT ( 'NONE',  ( 0.5314960629921267055, -0.5400638737290844871, 0.3530559997133364547 ) ) ;
#44149=CARTESIAN_POINT ( 'NONE',  ( 1.463254593175853824, -0.6692913385826771977, 0.1292274648535927661 ) ) ;
#44150=CARTESIAN_POINT ( 'NONE',  ( 1.541994750656168645, -0.6692913385826771977, 0.1292274648535927661 ) ) ;
#44151=CARTESIAN_POINT ( 'NONE',  ( 0.01968503937007957949, -0.5400638737290845981, -0.3530559997133363437 ) ) ;
#44152=CARTESIAN_POINT ( 'NONE',  ( -1.279527559055116948, 0.1660481256975883668, -0.3530559997133364547 ) ) ;
#44153=CARTESIAN_POINT ( 'NONE',  ( 1.594488188976378673, 0.1660481256975885056, 0.3530559997133364547 ) ) ;
#44154=CARTESIAN_POINT ( 'NONE',  ( 1.633858267716535639, -0.5400638737290844871, 0.3530559997133364547 ) ) ;
#44156=CARTESIAN_POINT ( 'NONE',  ( 1.030183727034121421, -0.08942795157527998196, 0.3641732283464567121 ) ) ;
#44157=VERTEX_POINT ( 'NONE', #9135 ) ;
#44159=ORIENTED_EDGE ( 'NONE', *, *, #16637, .F. ) ;
#44160=CARTESIAN_POINT ( 'NONE',  ( 0.1640419947506569498, -0.08942795157527998196, 0.3641732283464567121 ) ) ;
#44161=DIRECTION ( 'NONE',  ( -1.000000000000000000, 0.000000000000000000, 1.692413147294446216E-16 ) ) ;
#44162=CARTESIAN_POINT ( 'NONE',  ( 0.4330708661417329575, -0.6692913385826771977, 8.415575281601705876E-17 ) ) ;
#44163=CARTESIAN_POINT ( 'NONE',  ( 0.2165354330708668673, 0.1660481256975883668, -0.3530559997133364547 ) ) ;
#44164=CARTESIAN_POINT ( 'NONE',  ( -0.4724409448818890911, -0.1870078740157479769, 0.4822834645669291653 ) ) ;
#44166=CARTESIAN_POINT ( 'NONE',  ( -1.305774278215222184, 0.2952755905511811885, 0.1292274648535926551 ) ) ;
#44168=CARTESIAN_POINT ( 'NONE',  ( 1.364829396325459854, -0.5023911411419708095, -0.1820866141732282451 ) ) ;
#44169=CARTESIAN_POINT ( 'NONE',  ( -1.410761154855641575, -0.3162353388693409650, -0.4822834645669289433 ) ) ;
#44170=CARTESIAN_POINT ( 'NONE',  ( 0.7611548556430454138, 0.2306618581243847221, -0.2411417322834647770 ) ) ;
#44171=CARTESIAN_POINT ( 'NONE',  ( 1.174540682414699111, -0.3162353388693405765, 0.4822834645669290543 ) ) ;
#44173=CARTESIAN_POINT ( 'NONE',  ( -1.410761154855642463, -0.05778040916215522460, 0.4822834645669289988 ) ) ;
#44176=CARTESIAN_POINT ( 'NONE',  ( -0.2690288713910754526, 0.2952755905511810774, -0.1292274648535930714 ) ) ;
#44180=CARTESIAN_POINT ( 'NONE',  ( 1.535433070866142558, 0.2952755905511811885, 0.000000000000000000 ) ) ;
#44181=CARTESIAN_POINT ( 'NONE',  ( -0.01312335958005186876, -0.004921259842519870586, -0.3153832671262229437 ) ) ;
#44182=CARTESIAN_POINT ( 'NONE',  ( 0.7283464566929140904, -0.5400638737290845981, -0.3530559997133363437 ) ) ;
#44184=CARTESIAN_POINT ( 'NONE',  ( 0.4855643044619430415, -0.3690944881889765550, -0.3153832671262227771 ) ) ;
#44185=CARTESIAN_POINT ( 'NONE',  ( 0.5446194225721792126, -0.05778040916215560624, -0.4822834645669293319 ) ) ;
#44186=EDGE_CURVE ( 'NONE', #5541, #82322, #9955, .T. ) ;
#44188=CARTESIAN_POINT ( 'NONE',  ( -0.9776902887139098386, -0.6692913385826771977, 0.1292274648535927661 ) ) ;
#44190=CARTESIAN_POINT ( 'NONE',  ( 0.7349081364829402885, -0.5023911411419708095, -0.1820866141732282451 ) ) ;
#44191=CARTESIAN_POINT ( 'NONE',  ( -1.112371124080194340, -2.567464376874931580E-15, -0.4445507791589072832 ) ) ;
#44192=CARTESIAN_POINT ( 'NONE',  ( -0.3740157480314953431, -0.5400638737290845981, -0.3530559997133363437 ) ) ;
#44193=CARTESIAN_POINT ( 'NONE',  ( 0.1902887139107617975, -0.5511811023622048555, -0.09757992244046775898 ) ) ;
#44195=CARTESIAN_POINT ( 'NONE',  ( -0.1377952755905504645, 0.1660481256975885056, 0.3530559997133364547 ) ) ;
#44196=CARTESIAN_POINT ( 'NONE',  ( 0.2952755905511816326, -0.4536011799217367080, 0.2665933059059888421 ) ) ;
#44198=CARTESIAN_POINT ( 'NONE',  ( 0.2559055118110243332, 0.1660481256975885056, 0.3530559997133364547 ) ) ;
#44199=CARTESIAN_POINT ( 'NONE',  ( 0.9776902887139113929, -0.5511811023622048555, -0.09757992244046775898 ) ) ;
#44201=CARTESIAN_POINT ( 'NONE',  ( -0.2887139107611542133, 0.1283753931104748280, 0.1820866141732283561 ) ) ;
#44202=CARTESIAN_POINT ( 'NONE',  ( -0.8530183727034112984, -0.3690944881889765550, -0.3153832671262227771 ) ) ;
#44203=CARTESIAN_POINT ( 'NONE',  ( -0.4002624671916004129, -0.3162353388693405765, 0.4822834645669290543 ) ) ;
#44204=CARTESIAN_POINT ( 'NONE',  ( 0.2230971128608929543, 0.05413385826771626580, -0.4176697321401330321 ) ) ;
#44205=CARTESIAN_POINT ( 'NONE',  ( 1.049868766404200349, 0.1283753931104748280, 0.1820866141732283561 ) ) ;
#44207=CARTESIAN_POINT ( 'NONE',  ( -1.732283464566928277, -0.1870078740157479769, 0.4822834645669291653 ) ) ;
#44208=CARTESIAN_POINT ( 'NONE',  ( 0.6167979002624679463, 0.05413385826771626580, -0.4176697321401330321 ) ) ;
#44209=CARTESIAN_POINT ( 'NONE',  ( -1.614173228346456712, 1.818966223839196816, -0.1372047244094478091 ) ) ;
#44210=CARTESIAN_POINT ( 'NONE',  ( -0.4396325459317579898, 0.2952755905511811885, 0.1292274648535926551 ) ) ;
#44212=CARTESIAN_POINT ( 'NONE',  ( 0.8661417322834653598, -0.1870078740157479769, 0.4822834645669291653 ) ) ;
#44213=CARTESIAN_POINT ( 'NONE',  ( 0.4265091863517067594, 0.2952755905511811885, 0.1292274648535926551 ) ) ;
#44215=CARTESIAN_POINT ( 'NONE',  ( 0.3149606299212606708, -0.1870078740157480601, -0.3641732283464567677 ) ) ;
#44216=CARTESIAN_POINT ( 'NONE',  ( 1.220472440944882608, 0.2952755905511811885, 0.000000000000000000 ) ) ;
#44217=CARTESIAN_POINT ( 'NONE',  ( -0.4461942257217840213, 0.1283753931104748280, 0.1820866141732283561 ) ) ;
#44218=CARTESIAN_POINT ( 'NONE',  ( -0.2165354330708654795, 0.1660481256975885056, 0.3530559997133364547 ) ) ;
#44220=CARTESIAN_POINT ( 'NONE',  ( 0.3543307086614179147, 0.2952755905511811885, 0.000000000000000000 ) ) ;
#44221=CARTESIAN_POINT ( 'NONE',  ( -0.6299212598425188991, -0.1870078740157480879, -0.4822834645669291653 ) ) ;
#44222=CARTESIAN_POINT ( 'NONE',  ( -0.6824146981627291497, -0.5023911411419708095, -0.1820866141732282451 ) ) ;
#44223=CARTESIAN_POINT ( 'NONE',  ( 0.5905511811023629321, -0.6692913385826771977, 8.415575281601705876E-17 ) ) ;
#44224=CARTESIAN_POINT ( 'NONE',  ( -1.299212598425196097, -0.6692913385826771977, 8.415575281601705876E-17 ) ) ;
#44225=CARTESIAN_POINT ( 'NONE',  ( -0.1640419947506553400, -0.05778040916215560624, -0.4822834645669293319 ) ) ;
#44226=CARTESIAN_POINT ( 'NONE',  ( 1.128608923884514947, 0.1539470093639523085, 0.1968503937007873850 ) ) ;
#44228=CARTESIAN_POINT ( 'NONE',  ( 1.246719160104987623, -0.4281496062992124485, 0.4176697321401328655 ) ) ;
#44229=CARTESIAN_POINT ( 'NONE',  ( 1.187664041994751285, -0.05778040916215522460, 0.4822834645669289988 ) ) ;
#44232=CARTESIAN_POINT ( 'NONE',  ( -0.9973753280839886548, -0.6046776061558809534, -0.2411417322834644161 ) ) ;
#44233=B_SPLINE_CURVE_WITH_KNOTS ( 'NONE', 3,
 ( #69193, #62459, #62879, #73866, #48170, #48997, #74278 ),
 .UNSPECIFIED., .F., .F.,
 ( 4, 3, 4 ),
 ( 3.469446951953614189E-18, 0.001246230184515571739, 0.002492489877932648097 ),
 .UNSPECIFIED. ) ;
#44237=CARTESIAN_POINT ( 'NONE',  ( -0.2887139107611542133, -0.5023911411419708095, -0.1820866141732282451 ) ) ;
#44239=CARTESIAN_POINT ( 'NONE',  ( 0.5314960629921264834, 0.1660481256975883668, -0.3530559997133364547 ) ) ;
#44241=CARTESIAN_POINT ( 'NONE',  ( -0.5411721830064186722, -2.191421614605370878E-15, 0.4445507791589071167 ) ) ;
#44242=CARTESIAN_POINT ( 'NONE',  ( -0.5249343832020990641, 0.1283753931104748280, 0.1820866141732283561 ) ) ;
#44244=CARTESIAN_POINT ( 'NONE',  ( 1.161417322834646493, -0.5400638737290844871, 0.3530559997133364547 ) ) ;
#44245=CARTESIAN_POINT ( 'NONE',  ( 0.7874015748031503170, -0.1870078740157479769, 0.3641732283464567677 ) ) ;
#44246=CARTESIAN_POINT ( 'NONE',  ( -0.1837270341207340729, 0.2306618581243847221, -0.2411417322834647770 ) ) ;
#44248=CARTESIAN_POINT ( 'NONE',  ( -0.3608923884514428360, 0.2952755905511811885, 0.1292274648535926551 ) ) ;
#44249=CARTESIAN_POINT ( 'NONE',  ( -1.515748031496062076, 0.07958543189024071263, -0.2665933059059888421 ) ) ;
#44250=CARTESIAN_POINT ( 'NONE',  ( -0.5118110236220466680, -0.6692913385826771977, 8.415575281601705876E-17 ) ) ;
#44251=CARTESIAN_POINT ( 'NONE',  ( 1.666666666666667185, 0.05413385826771666132, 0.4176697321401328100 ) ) ;
#44253=ORIENTED_EDGE ( 'NONE', *, *, #61823, .F. ) ;
#44255=CARTESIAN_POINT ( 'NONE',  ( 0.6102362204724416372, 0.1660481256975883668, -0.3530559997133364547 ) ) ;
#44257=CARTESIAN_POINT ( 'NONE',  ( -0.9711286089238838626, -0.6046776061558807314, 0.2411417322834647770 ) ) ;
#44258=CARTESIAN_POINT ( 'NONE',  ( 1.614173228346457378, 0.2952755905511811885, 0.000000000000000000 ) ) ;
#44259=CARTESIAN_POINT ( 'NONE',  ( 0.5052493438320215802, 0.2952755905511811885, 0.1292274648535926551 ) ) ;
#44260=CARTESIAN_POINT ( 'NONE',  ( -0.09842519685039295696, -0.5400638737290844871, 0.3530559997133364547 ) ) ;
#44262=CARTESIAN_POINT ( 'NONE',  ( -0.7020997375328076329, -0.3162353388693409650, -0.4822834645669289433 ) ) ;
#44263=CARTESIAN_POINT ( 'NONE',  ( -0.1509186351706028884, -0.3162353388693409650, -0.4822834645669289433 ) ) ;
#44264=CARTESIAN_POINT ( 'NONE',  ( -0.8136482939632537770, 0.2306618581243847221, -0.2411417322834647770 ) ) ;
#44265=CARTESIAN_POINT ( 'NONE',  ( 0.2624671916010504757, 0.1283753931104748280, 0.1820866141732283561 ) ) ;
#44267=CARTESIAN_POINT ( 'NONE',  ( -0.03280839895013062252, -0.6692913385826771977, 0.1292274648535927661 ) ) ;
#44269=CARTESIAN_POINT ( 'NONE',  ( 1.312335958005249825, 0.2306618581243847221, -0.2411417322834647770 ) ) ;
#44273=VERTEX_POINT ( 'NONE', #49487 ) ;
#44274=CARTESIAN_POINT ( 'NONE',  ( 0.2165354330708668673, -0.5400638737290844871, 0.3530559997133364547 ) ) ;
#44275=CARTESIAN_POINT ( 'NONE',  ( 0.1968503937007881344, 0.1771653543307087630, 0.000000000000000000 ) ) ;
#44276=CARTESIAN_POINT ( 'NONE',  ( 1.469816272965879911, -0.5023911411419708095, 0.1820866141732285504 ) ) ;
#44281=CARTESIAN_POINT ( 'NONE',  ( 1.548556430446194954, -0.6046776061558807314, 0.2411417322834647770 ) ) ;
#44283=CARTESIAN_POINT ( 'NONE',  ( 0.5249343832021003964, 0.2306618581243847221, -0.2411417322834647770 ) ) ;
#44284=CARTESIAN_POINT ( 'NONE',  ( -1.036745406824146176, -0.4281496062992124485, 0.4176697321401328655 ) ) ;
#44285=CARTESIAN_POINT ( 'NONE',  ( -1.213910761154854745, 0.2952755905511810774, -0.1292274648535930714 ) ) ;
#44286=CARTESIAN_POINT ( 'NONE',  ( 0.2099737532808405305, 0.2306618581243847221, -0.2411417322834647770 ) ) ;
#44287=CARTESIAN_POINT ( 'NONE',  ( 1.082677165354331228, -0.5400638737290844871, 0.3530559997133364547 ) ) ;
#44288=CARTESIAN_POINT ( 'NONE',  ( 1.391076115485564868, 0.1283753931104746893, -0.1820866141732285504 ) ) ;
#44289=CARTESIAN_POINT ( 'NONE',  ( 0.6364829396325465405, -0.2845877964562161244, -0.3641732283464567121 ) ) ;
#44290=CARTESIAN_POINT ( 'NONE',  ( -0.9580052493438311334, 0.05413385826771626580, -0.4176697321401330321 ) ) ;
#44292=CARTESIAN_POINT ( 'NONE',  ( 1.463254593175853824, -0.6692913385826771977, 0.1292274648535927661 ) ) ;
#44294=CARTESIAN_POINT ( 'NONE',  ( 0.8202099737532814183, -0.6692913385826773087, -0.1292274648535924053 ) ) ;
#44295=CARTESIAN_POINT ( 'NONE',  ( 1.604771003085129433, 0.7690346235818160681, -0.1466069496707749498 ) ) ;
#44296=CARTESIAN_POINT ( 'NONE',  ( -1.594488188976377563, -0.4536011799217367080, 0.2665933059059888421 ) ) ;
#44297=CARTESIAN_POINT ( 'NONE',  ( 0.07217847769028949700, -0.3162353388693405765, 0.4822834645669290543 ) ) ;
#44298=CARTESIAN_POINT ( 'NONE',  ( 1.062992125984252745, -0.5511811023622047445, 6.969142054262312111E-17 ) ) ;
#44299=CARTESIAN_POINT ( 'NONE',  ( -1.732283464566928277, -0.1870078740157479769, 0.3641732283464567677 ) ) ;
#44300=CARTESIAN_POINT ( 'NONE',  ( 0.8333333333333340365, -0.6692913385826771977, 0.1292274648535927661 ) ) ;
#44302=CARTESIAN_POINT ( 'NONE',  ( -0.6889763779527552368, -0.4536011799217368745, -0.2665933059059886201 ) ) ;
#44303=CARTESIAN_POINT ( 'NONE',  ( -0.6167979002624665030, 0.05413385826771666132, 0.4176697321401328100 ) ) ;
#44304=CARTESIAN_POINT ( 'NONE',  ( 1.515748031496063408, 0.1660481256975885056, 0.3530559997133364547 ) ) ;
#44305=ADVANCED_FACE ( 'NONE', ( #73528 ), #48245, .F. ) ;
#44306=CARTESIAN_POINT ( 'NONE',  ( -1.325459317585300889, -0.4281496062992127816, -0.4176697321401328100 ) ) ;
#44307=CARTESIAN_POINT ( 'NONE',  ( 1.351706036745407680, 0.05413385826771666132, 0.4176697321401328100 ) ) ;
#44309=CARTESIAN_POINT ( 'NONE',  ( -1.410761154855641575, -0.2845877964562161244, -0.3641732283464567121 ) ) ;
#44311=CARTESIAN_POINT ( 'NONE',  ( 1.135170603674541256, 0.2952755905511811885, 0.1292274648535926551 ) ) ;
#44313=CARTESIAN_POINT ( 'NONE',  ( -1.614173228346456268, -0.6692913385826771977, 8.415575281601705876E-17 ) ) ;
#44314=CARTESIAN_POINT ( 'NONE',  ( -1.496062992125983815, -0.1870078740157479769, 0.3641732283464567677 ) ) ;
#44315=CARTESIAN_POINT ( 'NONE',  ( -0.9908136482939626788, -0.5511811023622048555, -0.09757992244046775898 ) ) ;
#44316=CARTESIAN_POINT ( 'NONE',  ( 1.170403185795211742, -4.479759449472349425E-16, -0.4118484887281964046 ) ) ;
#44317=CARTESIAN_POINT ( 'NONE',  ( -0.5774278215223089816, -0.6046776061558807314, 0.2411417322834647770 ) ) ;
#44318=CARTESIAN_POINT ( 'NONE',  ( -0.1246719160104980823, -0.5511811023622048555, -0.09757992244046775898 ) ) ;
#44319=CARTESIAN_POINT ( 'NONE',  ( -1.627296587926508442, -0.5023911411419708095, -0.1820866141732282451 ) ) ;
#44320=CARTESIAN_POINT ( 'NONE',  ( 0.9120734908136489683, -0.5511811023622046335, 0.09757992244046803654 ) ) ;
#44321=CARTESIAN_POINT ( 'NONE',  ( 0.7808398950131241190, -0.05778040916215560624, -0.4822834645669293319 ) ) ;
#44322=CARTESIAN_POINT ( 'NONE',  ( 1.541994750656168645, -0.6692913385826771977, 0.1292274648535927661 ) ) ;
#44323=CARTESIAN_POINT ( 'NONE',  ( 0.1312335958005257930, 0.1283753931104746893, -0.1820866141732285504 ) ) ;
#44324=CARTESIAN_POINT ( 'NONE',  ( 0.4921259842519691285, -0.5400638737290845981, -0.3530559997133363437 ) ) ;
#44325=CARTESIAN_POINT ( 'NONE',  ( 0.3937007874015754361, -0.1870078740157480601, -0.3641732283464567677 ) ) ;
#44326=ORIENTED_EDGE ( 'NONE', *, *, #35131, .T. ) ;
#44327=CARTESIAN_POINT ( 'NONE',  ( -1.568241469816272105, -0.3162353388693409650, -0.4822834645669289433 ) ) ;
#44328=EDGE_CURVE ( 'NONE', #66982, #69770, #17117, .T. ) ;
#44329=CARTESIAN_POINT ( 'NONE',  ( -1.325459317585300889, 0.05413385826771666132, 0.4176697321401328100 ) ) ;
#44330=CARTESIAN_POINT ( 'NONE',  ( -0.5839895013123351797, 0.2952755905511810774, -0.1292274648535930714 ) ) ;
#44333=CARTESIAN_POINT ( 'NONE',  ( 0.4002624671916016896, -0.3162353388693409650, -0.4822834645669289433 ) ) ;
#44334=CARTESIAN_POINT ( 'NONE',  ( 0.9711286089238851948, 0.1283753931104748280, 0.1820866141732283561 ) ) ;
#44335=CARTESIAN_POINT ( 'NONE',  ( -0.3477690288713902178, 0.2952755905511810774, -0.1292274648535930714 ) ) ;
#44336=CARTESIAN_POINT ( 'NONE',  ( 0.1509186351706042484, -0.3162353388693405765, 0.4822834645669290543 ) ) ;
#44342=CARTESIAN_POINT ( 'NONE',  ( -0.7349081364829390672, 0.1283753931104746893, -0.1820866141732285504 ) ) ;
#44343=CARTESIAN_POINT ( 'NONE',  ( -1.161417322834644716, -0.5400638737290845981, -0.3530559997133363437 ) ) ;
#44345=CARTESIAN_POINT ( 'NONE',  ( 0.6627296587926517768, -0.6692913385826773087, -0.1292274648535924053 ) ) ;
#44346=CARTESIAN_POINT ( 'NONE',  ( 1.286089238845145033, 0.2306618581243848609, 0.2411417322834645549 ) ) ;
#44347=CARTESIAN_POINT ( 'NONE',  ( 0.9580052493438326877, 0.05413385826771666132, 0.4176697321401328100 ) ) ;
#44350=CARTESIAN_POINT ( 'NONE',  ( 1.515748031496063408, 0.1660481256975885056, 0.3530559997133364547 ) ) ;
#44351=CARTESIAN_POINT ( 'NONE',  ( 0.7742782152230978099, -0.4281496062992124485, 0.4176697321401328655 ) ) ;
#44352=CARTESIAN_POINT ( 'NONE',  ( 0.4593175853018379162, -0.4281496062992124485, 0.4176697321401328655 ) ) ;
#44353=CARTESIAN_POINT ( 'NONE',  ( 0.7545931758530188826, -0.5511811023622046335, 0.09757992244046803654 ) ) ;
#44354=CARTESIAN_POINT ( 'NONE',  ( 1.135170603674541256, -0.6692913385826773087, -0.1292274648535924053 ) ) ;
#44357=CARTESIAN_POINT ( 'NONE',  ( 0.6036745406824154392, 0.2306618581243847221, -0.2411417322834647770 ) ) ;
#44358=CARTESIAN_POINT ( 'NONE',  ( 1.660104986876641320, -0.08942795157527998196, 0.3641732283464567121 ) ) ;
#44359=CARTESIAN_POINT ( 'NONE',  ( -0.7939632545931754048, -0.3162353388693405765, 0.4822834645669290543 ) ) ;
#44360=CARTESIAN_POINT ( 'NONE',  ( -0.9711286089238838626, -0.6046776061558807314, 0.2411417322834647770 ) ) ;
#44361=CARTESIAN_POINT ( 'NONE',  ( 1.240157480314961314, -0.5400638737290844871, 0.3530559997133364547 ) ) ;
#44367=ORIENTED_EDGE ( 'NONE', *, *, #14488, .T. ) ;
#44368=CARTESIAN_POINT ( 'NONE',  ( 1.594488188976378673, -0.5400638737290845981, -0.3530559997133363437 ) ) ;
#44369=CARTESIAN_POINT ( 'NONE',  ( 1.430446194225722500, -0.004921259842519576551, 0.3153832671262227771 ) ) ;
#44371=CARTESIAN_POINT ( 'NONE',  ( 1.259842519685040019, -0.1870078740157480601, -0.3641732283464567677 ) ) ;
#44372=CARTESIAN_POINT ( 'NONE',  ( 0.4606732211678798428, 1.541615089183433485, -0.5309055118110237448 ) ) ;
#44373=DIRECTION ( 'NONE',  ( -3.096699300667737957E-16, 1.000000000000000000, -0.000000000000000000 ) ) ;
#44376=CARTESIAN_POINT ( 'NONE',  ( -0.5774278215223089816, -0.5023911411419708095, 0.1820866141732285504 ) ) ;
#44377=CARTESIAN_POINT ( 'NONE',  ( -1.561679790026246017, -0.004921259842519576551, 0.3153832671262227771 ) ) ;
#44378=CARTESIAN_POINT ( 'NONE',  ( -1.167979002624671470, 0.05413385826771666132, 0.4176697321401328100 ) ) ;
#44379=CARTESIAN_POINT ( 'NONE',  ( 0.2099737532808405305, 0.2306618581243847221, -0.2411417322834647770 ) ) ;
#44380=CARTESIAN_POINT ( 'NONE',  ( 1.358267716535433323, -0.5400638737290845981, -0.3530559997133363437 ) ) ;
#44385=( BOUNDED_SURFACE ( )  B_SPLINE_SURFACE ( 1, 2, ( 
 ( #57786, #11548, #24571, #6040, #38026, #18677, #31295, #6458, #37204, #62885, #51051, #44322, #63288, #64535, #5220, #56551, #82252, #63701, #69612, #150, #57372, #12367, #56959, #50237, #573, #83067, #11958, #75933, #70857, #24971, #32128, #37613, #25388, #5628, #50643, #70012, #70427, #19082, #44731, #12783, #51466, #58206, #19500, #13208, #45154, #38855, #8138, #27899, #45578, #79268, #27481, #72524, #46413, #26226, #53139, #65805, #66626, #21583, #59055, #60302, #1820, #8964, #19928, #39272, #52307, #71271, #1409, #33803, #47246, #78013, #20341, #65389, #78850, #34638, #7724, #58631, #51890, #27065, #59881, #77594, #33393, #40947, #53560, #21177, #72935, #20763, #13618, #64956, #59468, #7294, #46832, #52724, #15287, #32964, #999, #14873, #26653, #45993, #71690, #40534, #8552, #66213, #14041, #34218, #2235, #78436, #39698, #72107, #14465, #40117, #48901, #53971, #68287, #35876, #73777, #2652, #10623, #79684, #60710, #42176, #74184, #29140, #67452, #42587, #22001, #47661, #3887, #54806, #16113, #17360, #73356, #15704, #41361, #16531, #54388, #36279, #67870, #48483, #9786, #67042, #36682, #10208, #80099, #9374, #23642, #35457, #16945, #28727, #61543, #48075, #22418, #3059, #23230, #35045, #28309, #74602, #41757, #11025, #61122, #49312, #29547, #3473, #55209, #4291, #80510, #55618, #80917, #61951, #22825, #29953, #81328, #75014, #42989, #68683, #11858, #13100, #37922, #45048, #56036, #75421, #5118, #24054, #37511, #5525, #12264, #82964, #38337, #43395, #70323, #31190, #63186, #62358, #44220, #63598, #18978, #46, #82150, #5935, #56855, #31605, #69095, #44627, #11443, #64012, #25699, #37099, #57265, #4695, #62784, #50131, #50539, #76243, #24871, #18577, #30369, #69910, #30785, #25282, #19397, #81744, #70749, #77063, #56448, #50950, #49724, #17764, #69509, #24466, #75831, #82553, #51360, #18172, #12678, #32024, #76647, #6353, #43805, #57684, #60915, #13509, #13936, #28927, #19822, #28519, #73568, #34844, #60507, #79889, #54175, #28106, #15493, #3266, #6765, #34428, #60093, #77908, #45887, #79471, #48279, #21787, #47449, #80305, #54596, #7621, #2855, #77487, #53760, #73144, #41151, #15913, #32437, #66839, #22207, #73977, #9582, #22620, #38754, #58100, #894, #26122, #9173, #67250, #47864, #41561, #45471, #64431, #35251, #71169, #64850, #52204, #465, #20239, #51783, #39165, #7187, #32860, #58528, #26551, #71585, #39594, #65282, #2448, #55828, #81536, #35663, #61327, #3681, #42788, #75630, #24259, #36898, #74810, #36482, #80713, #23855, #49932, #50340, #29346, #55005, #23028, #36077, #42376, #43605, #17968, #43192, #37315, #10822, #16323, #82354, #49522, #48694, #75215, #81123, #62988, #74392, #69307, #68888, #67661, #41968, #9998, #4916, #81946, #17560, #24672, #11238, #11657, #17155, #5327, #16736, #62574, #62157, #30584, #68075, #30985, #56250, #4085, #10419, #56653, #61748, #29753, #55416, #4498, #68483, #23440, #49104, #30165, #44023, #77273, #19185, #6142, #7403, #69716, #12060, #37718, #64227, #44422, #678, #6561, #38547, #57477, #31398, #26754, #57891, #70117, #63392, #13726, #83171, #6979, #18779, #32233, #38130, #12468, #76452, #13306, #57063, #76037, #38958, #18382, #1103, #5727, #39380, #258, #82756, #25910, #77699, #25078, #45680, #19602, #64642, #12887, #50752, #45265, #51570, #33072, #71376, #25491, #63804, #70961, #58741, #31817, #51157, #76852, #44834, #70532, #32648, #58313, #26332, #51994, #20029, #65065, #78963, #53249, #52409, #34328, #28005, #9078, #59991, #47770, #20869, #46520, #8242, #53665, #60818, #33908, #1516, #78118, #21282, #2760, #3170, #59572, #67154, #22110, #66318, #21691, #1928, #46937, #73469, #27170, #27591, #41469, #33496, #41054, #28419, #47354, #73043, #34749, #66740, #40636, #79372, #15820, #20451, #72629, #14977, #8657, #2349, #15392, #46104, #60409, #54079, #9483, #35158, #79794, #71797, #7829, #14150, #39804, #65497, #59158, #52832, #78544, #72221, #14572, #40224, #65906, #69212, #80210, #74297, #16225, #42700, #56155, #68799, #75127, #35570, #49839, #30074, #61233, #54917, #42283, #81858, #67981, #30490 ),
 ( #55325, #4814, #36803, #49433, #3999, #49017, #9898, #68397, #62479, #62897, #73885, #48188, #41872, #48601, #80623, #24170, #75538, #16643, #55737, #29663, #81445, #3587, #11144, #29253, #17878, #43512, #22935, #4406, #54498, #10324, #35988, #17061, #10736, #74714, #36393, #28834, #62067, #61658, #23760, #11561, #22526, #37218, #67566, #81034, #17472, #23346, #43103, #76359, #24582, #5639, #38036, #70868, #6882, #32138, #18286, #76763, #50657, #13218, #50249, #51475, #44742, #30896, #5232, #75945, #57795, #162, #51063, #56563, #19093, #77178, #63711, #45163, #82264, #19509, #70437, #38864, #69625, #64545, #6468, #6051, #43929, #32552, #37625, #18691, #64134, #38450, #12794, #57384, #11970, #56970, #31306, #63301, #25815, #82668, #24983, #12378, #70025, #31723, #44334, #83078, #25399, #10997, #42965, #61925, #35849, #31162, #62332, #74577, #42150, #18144, #4267, #11417, #23206, #68659, #42559, #48877, #80893, #17738, #61518, #80486, #43367, #22800, #5500, #16507, #43778, #36657, #48459, #4669, #82123, #67845, #50105, #81719, #69067, #17335, #74159, #24029, #30342, #37487, #75802, #29929, #10184, #56008, #63161, #3863, #29523, #16922, #55185, #55592, #23618, #49697, #37072, #56423, #68263, #5093, #49287, #81304, #10599, #75393, #62757, #30761, #24438, #69481, #36255, #74990, #11834, #58073, #65254, #12647, #5907, #82526, #57657, #7161, #7591, #38309, #71558, #58500, #439, #77879, #51333, #56829, #39565, #64403, #63983, #31579, #24844, #19, #32832, #50511, #6320, #13907, #864, #26094, #20210, #77037, #76215, #18551, #6739, #12240, #32410, #31997, #45860, #44196, #26521, #51754, #69886, #37896, #63572, #45444, #39139, #13071, #57235, #77457, #64820, #25673, #52176, #82936, #19792, #19369, #71140, #25258, #50922, #13482, #44600, #76622, #18953, #70295, #45019, #38726, #70719, #79451, #8323, #66398, #40713, #74683, #23315, #35957, #72710, #34406, #78625, #53743, #48984, #49399, #59236, #33574, #27252, #33989, #40305, #42668, #36361, #59651, #15476, #15057, #41133, #20949, #81001, #46606, #17029, #62036, #72302, #73126, #39892, #14648, #2007, #2429, #28085, #60074, #21771, #14232, #47433, #65985, #66824, #55703, #65579, #81411, #30041, #27669, #10290, #23728, #7913, #21363, #1597, #53335, #8736, #4373, #52911, #55292, #68367, #61626, #3968, #79044, #29631, #47016, #10705, #50218, #64103, #56121, #63682, #25369, #69993, #12348, #31691, #6020, #63266, #50623, #12764, #43071, #69592, #11938, #30865, #82233, #68768, #49807, #31275, #24552, #75508, #37593, #70408, #11112, #36769, #76328, #18253, #5201, #6438, #62445, #4781, #30457, #5607, #43481, #83046, #56940, #82637, #56530, #81827, #25785, #24950, #69177, #24137, #38421, #75914, #57350, #17847, #18658, #37185, #11528, #62864, #38004, #43895, #75093, #51032, #17441, #130, #44302, #32110, #76731, #19063, #44711, #57768, #70839, #21159, #52706, #14448, #71671, #51446, #78417, #7707, #8533, #46815, #980, #2217, #27046, #34201, #45135, #64516, #77576, #13188, #26636, #77995, #1392, #72089, #27464, #32523, #59449, #20323, #52290, #77150, #33374, #20746, #8120, #59038, #72506, #19908, #45558, #7276, #46396, #59864, #32947, #555, #19482, #45976, #1801, #38837, #58613, #66196, #53122, #40099, #14855, #14023, #6853, #58185, #65787, #26208, #33785, #39680, #40516, #51870, #78833, #71254, #13600, #39254, #64936, #65372, #10194, #67437, #36266, #35442, #35863, #3045, #55196, #61935, #74170, #22404, #16517, #79251, #61528, #61108, #15689, #27883, #3874, #48469, #29533, #8946, #80903, #54374, #28710, #53543, #9771, #3460, #67856, #29125, #23217, #79667, #21984, #67028, #54793, #21566, #9360, #60286, #47228, #80084, #48887, #72918, #35031, #42572, #74588, #80496, #16932, #48061, #15269, #10609, #22812, #66610, #42161, #60695, #68274, #40930, #34622, #2636, #28293, #53954, #47646, #73341, #41347, #73763, #16098, #41743, #12250, #62771, #31591, #12660, #50523, #82135, #76229, #55603, #69896, #37497, #75404, #4278, #37906, #81315, #62343, #43789, #37085, #4682, #50117, #82950, #23628, #49299, #5510, #30772, #17750, #18963 ) ),
 .UNSPECIFIED., .F., .F., .F. ) 
 B_SPLINE_SURFACE_WITH_KNOTS ( ( 2, 2 ),
 ( 3, 2, 2, 2, 2, 2, 2, 2, 2, 2, 2, 2, 2, 2, 2, 2, 2, 2, 2, 2, 2, 2, 2, 2, 2, 2, 2, 2, 2, 2, 2, 2, 2, 2, 2, 2, 2, 2, 2, 2, 2, 2, 2, 2, 2, 2, 2, 2, 2, 2, 2, 2, 2, 2, 2, 2, 2, 2, 2, 2, 2, 2, 2, 2, 2, 2, 2, 2, 2, 2, 2, 2, 2, 2, 2, 2, 2, 2, 2, 2, 2, 2, 2, 2, 2, 2, 2, 2, 2, 2, 2, 2, 2, 2, 2, 2, 2, 2, 2, 2, 2, 2, 2, 2, 2, 2, 2, 2, 2, 2, 2, 2, 2, 2, 2, 2, 2, 2, 2, 2, 2, 2, 2, 2, 2, 2, 2, 2, 2, 2, 2, 2, 2, 2, 2, 2, 2, 2, 2, 2, 2, 2, 2, 2, 2, 2, 2, 2, 2, 2, 2, 2, 2, 2, 2, 2, 2, 2, 2, 2, 2, 2, 2, 2, 2, 2, 2, 2, 2, 2, 2, 2, 2, 2, 2, 2, 2, 2, 2, 2, 2, 2, 2, 2, 2, 2, 2, 2, 2, 2, 2, 2, 2, 2, 2, 2, 2, 2, 2, 2, 2, 2, 2, 2, 2, 2, 2, 2, 2, 2, 2, 2, 2, 2, 2, 2, 2, 2, 2, 2, 2, 2, 2, 2, 2, 2, 2, 2, 2, 2, 2, 2, 2, 2, 2, 2, 2, 2, 2, 2, 2, 2, 2, 2, 2, 2, 2, 2, 2, 2, 2, 2, 2, 2, 2, 3 ),
 ( 0.000000000000000000, 1.000000000000000000 ),
 ( 0.000000000000000000, 0.003787878787878787984, 0.007575757575757575968, 0.01136363636363636395, 0.01515151515151515194, 0.01893939393939393992, 0.02272727272727272790, 0.02651515151515151589, 0.03030303030303030387, 0.03409090909090908839, 0.03787878787878787984, 0.04166666666666666435, 0.04545454545454545581, 0.04924242424242424032, 0.05303030303030303177, 0.05681818181818181629, 0.06060606060606060774, 0.06439393939393939226, 0.06818181818181817677, 0.07196969696969697516, 0.07575757575757575968, 0.07954545454545454419, 0.08333333333333332871, 0.08712121212121212710, 0.09090909090909091161, 0.09469696969696969613, 0.09848484848484848064, 0.1022727272727272790, 0.1060606060606060635, 0.1098484848484848481, 0.1136363636363636326, 0.1174242424242424310, 0.1212121212121212155, 0.1250000000000000000, 0.1287878787878787845, 0.1325757575757575690, 0.1363636363636363535, 0.1401515151515151381, 0.1439393939393939503, 0.1477272727272727348, 0.1515151515151515194, 0.1553030303030303039, 0.1590909090909090884, 0.1628787878787878729, 0.1666666666666666574, 0.1704545454545454419, 0.1742424242424242542, 0.1780303030303030387, 0.1818181818181818232, 0.1856060606060606077, 0.1893939393939393923, 0.1931818181818181768, 0.1969696969696969613, 0.2007575757575757458, 0.2045454545454545581, 0.2083333333333333426, 0.2121212121212121271, 0.2159090909090909116, 0.2196969696969696961, 0.2234848484848484806, 0.2272727272727272652, 0.2310606060606060497, 0.2348484848484848619, 0.2386363636363636465, 0.2424242424242424310, 0.2462121212121212155, 0.2500000000000000000, 0.2537878787878787845, 0.2575757575757575690, 0.2613636363636363535, 0.2651515151515151381, 0.2689393939393939226, 0.2727272727272727071, 0.2765151515151514916, 0.2803030303030302761, 0.2840909090909091161, 0.2878787878787879007, 0.2916666666666666852, 0.2954545454545454697, 0.2992424242424242542, 0.3030303030303030387, 0.3068181818181818232, 0.3106060606060606077, 0.3143939393939393923, 0.3181818181818181768, 0.3219696969696969613, 0.3257575757575757458, 0.3295454545454545303, 0.3333333333333333148, 0.3371212121212120993, 0.3409090909090908839, 0.3446969696969697239, 0.3484848484848485084, 0.3522727272727272929, 0.3560606060606060774, 0.3598484848484848619, 0.3636363636363636465, 0.3674242424242424310, 0.3712121212121212155, 0.3750000000000000000, 0.3787878787878787845, 0.3825757575757575690, 0.3863636363636363535, 0.3901515151515151381, 0.3939393939393939226, 0.3977272727272727071, 0.4015151515151514916, 0.4053030303030302761, 0.4090909090909091161, 0.4128787878787879007, 0.4166666666666666852, 0.4204545454545454697, 0.4242424242424242542, 0.4280303030303030387, 0.4318181818181818232, 0.4356060606060606077, 0.4393939393939393923, 0.4431818181818181768, 0.4469696969696969613, 0.4507575757575757458, 0.4545454545454545303, 0.4583333333333333148, 0.4621212121212120993, 0.4659090909090908839, 0.4696969696969697239, 0.4734848484848485084, 0.4772727272727272929, 0.4810606060606060774, 0.4848484848484848619, 0.4886363636363636465, 0.4924242424242424310, 0.4962121212121212155, 0.5000000000000000000, 0.5037878787878787845, 0.5075757575757575690, 0.5113636363636363535, 0.5151515151515151381, 0.5189393939393939226, 0.5227272727272727071, 0.5265151515151514916, 0.5303030303030302761, 0.5340909090909090606, 0.5378787878787878451, 0.5416666666666666297, 0.5454545454545454142, 0.5492424242424241987, 0.5530303030303029832, 0.5568181818181817677, 0.5606060606060605522, 0.5643939393939394478, 0.5681818181818182323, 0.5719696969696970168, 0.5757575757575758013, 0.5795454545454545858, 0.5833333333333333703, 0.5871212121212121549, 0.5909090909090909394, 0.5946969696969697239, 0.5984848484848485084, 0.6022727272727272929, 0.6060606060606060774, 0.6098484848484848619, 0.6136363636363636465, 0.6174242424242424310, 0.6212121212121212155, 0.6250000000000000000, 0.6287878787878787845, 0.6325757575757575690, 0.6363636363636363535, 0.6401515151515151381, 0.6439393939393939226, 0.6477272727272727071, 0.6515151515151514916, 0.6553030303030302761, 0.6590909090909090606, 0.6628787878787878451, 0.6666666666666666297, 0.6704545454545454142, 0.6742424242424241987, 0.6780303030303029832, 0.6818181818181817677, 0.6856060606060605522, 0.6893939393939394478, 0.6931818181818182323, 0.6969696969696970168, 0.7007575757575758013, 0.7045454545454545858, 0.7083333333333333703, 0.7121212121212121549, 0.7159090909090909394, 0.7196969696969697239, 0.7234848484848485084, 0.7272727272727272929, 0.7310606060606060774, 0.7348484848484848619, 0.7386363636363636465, 0.7424242424242424310, 0.7462121212121212155, 0.7500000000000000000, 0.7537878787878787845, 0.7575757575757575690, 0.7613636363636363535, 0.7651515151515151381, 0.7689393939393939226, 0.7727272727272727071, 0.7765151515151514916, 0.7803030303030302761, 0.7840909090909090606, 0.7878787878787878451, 0.7916666666666666297, 0.7954545454545454142, 0.7992424242424241987, 0.8030303030303029832, 0.8068181818181817677, 0.8106060606060605522, 0.8143939393939394478, 0.8181818181818182323, 0.8219696969696970168, 0.8257575757575758013, 0.8295454545454545858, 0.8333333333333333703, 0.8371212121212121549, 0.8409090909090909394, 0.8446969696969697239, 0.8484848484848485084, 0.8522727272727272929, 0.8560606060606060774, 0.8598484848484848619, 0.8636363636363636465, 0.8674242424242424310, 0.8712121212121212155, 0.8750000000000000000, 0.8787878787878787845, 0.8825757575757575690, 0.8863636363636363535, 0.8901515151515151381, 0.8939393939393939226, 0.8977272727272727071, 0.9015151515151514916, 0.9053030303030302761, 0.9090909090909090606, 0.9128787878787878451, 0.9166666666666666297, 0.9204545454545454142, 0.9242424242424241987, 0.9280303030303029832, 0.9318181818181817677, 0.9356060606060605522, 0.9393939393939394478, 0.9431818181818182323, 0.9469696969696970168, 0.9507575757575758013, 0.9545454545454545858, 0.9583333333333333703, 0.9621212121212121549, 0.9659090909090909394 ),
 .UNSPECIFIED. ) 
 GEOMETRIC_REPRESENTATION_ITEM ( )  RATIONAL_B_SPLINE_SURFACE ( (
 ( 1.000000000000000000, 0.9659258262890683122, 1.000000000000000000, 0.9659258262890683122, 1.000000000000000000, 0.9659258262890683122, 1.000000000000000000, 0.9659258262890683122, 1.000000000000000000, 0.9659258262890683122, 1.000000000000000000, 0.9659258262890683122, 1.000000000000000000, 0.9659258262890683122, 1.000000000000000000, 0.9659258262890683122, 1.000000000000000000, 0.9659258262890683122, 1.000000000000000000, 0.9659258262890683122, 1.000000000000000000, 0.9659258262890683122, 1.000000000000000000, 0.9659258262890683122, 1.000000000000000000, 0.9659258262890683122, 1.000000000000000000, 0.9659258262890683122, 1.000000000000000000, 0.9659258262890683122, 1.000000000000000000, 0.9659258262890683122, 1.000000000000000000, 0.9659258262890683122, 1.000000000000000000, 0.9659258262890683122, 1.000000000000000000, 0.9659258262890683122, 1.000000000000000000, 0.9659258262890683122, 1.000000000000000000, 0.9659258262890683122, 1.000000000000000000, 0.9659258262890683122, 1.000000000000000000, 0.9659258262890683122, 1.000000000000000000, 0.9659258262890683122, 1.000000000000000000, 0.9659258262890683122, 1.000000000000000000, 0.9659258262890683122, 1.000000000000000000, 0.9659258262890683122, 1.000000000000000000, 0.9659258262890683122, 1.000000000000000000, 0.9659258262890683122, 1.000000000000000000, 0.9659258262890683122, 1.000000000000000000, 0.9659258262890683122, 1.000000000000000000, 0.9659258262890683122, 1.000000000000000000, 0.9659258262890683122, 1.000000000000000000, 0.9659258262890683122, 1.000000000000000000, 0.9659258262890683122, 1.000000000000000000, 0.9659258262890683122, 1.000000000000000000, 0.9659258262890683122, 1.000000000000000000, 0.9659258262890683122, 1.000000000000000000, 0.9659258262890683122, 1.000000000000000000, 0.9659258262890683122, 1.000000000000000000, 0.9659258262890683122, 1.000000000000000000, 0.9659258262890683122, 1.000000000000000000, 0.9659258262890683122, 1.000000000000000000, 0.9659258262890683122, 1.000000000000000000, 0.9659258262890683122, 1.000000000000000000, 0.9659258262890683122, 1.000000000000000000, 0.9659258262890683122, 1.000000000000000000, 0.9659258262890683122, 1.000000000000000000, 0.9659258262890683122, 1.000000000000000000, 0.9659258262890683122, 1.000000000000000000, 0.9659258262890683122, 1.000000000000000000, 0.9659258262890683122, 1.000000000000000000, 0.9659258262890683122, 1.000000000000000000, 0.9659258262890683122, 1.000000000000000000, 0.9659258262890683122, 1.000000000000000000, 0.9659258262890683122, 1.000000000000000000, 0.9659258262890683122, 1.000000000000000000, 0.9659258262890683122, 1.000000000000000000, 0.9659258262890683122, 1.000000000000000000, 0.9659258262890683122, 1.000000000000000000, 0.9659258262890683122, 1.000000000000000000, 0.9659258262890683122, 1.000000000000000000, 0.9659258262890683122, 1.000000000000000000, 0.9659258262890683122, 1.000000000000000000, 0.9659258262890683122, 1.000000000000000000, 0.9659258262890683122, 1.000000000000000000, 0.9659258262890683122, 1.000000000000000000, 0.9659258262890683122, 1.000000000000000000, 0.9659258262890683122, 1.000000000000000000, 0.9659258262890683122, 1.000000000000000000, 0.9659258262890683122, 1.000000000000000000, 0.9659258262890683122, 1.000000000000000000, 0.9659258262890683122, 1.000000000000000000, 0.9659258262890683122, 1.000000000000000000, 0.9659258262890683122, 1.000000000000000000, 0.9659258262890683122, 1.000000000000000000, 0.9659258262890683122, 1.000000000000000000, 0.9659258262890683122, 1.000000000000000000, 0.9659258262890683122, 1.000000000000000000, 0.9659258262890683122, 1.000000000000000000, 0.9659258262890683122, 1.000000000000000000, 0.9659258262890683122, 1.000000000000000000, 0.9659258262890683122, 1.000000000000000000, 0.9659258262890683122, 1.000000000000000000, 0.9659258262890683122, 1.000000000000000000, 0.9659258262890683122, 1.000000000000000000, 0.9659258262890683122, 1.000000000000000000, 0.9659258262890683122, 1.000000000000000000, 0.9659258262890683122, 1.000000000000000000, 0.9659258262890683122, 1.000000000000000000, 0.9659258262890683122, 1.000000000000000000, 0.9659258262890683122, 1.000000000000000000, 0.9659258262890683122, 1.000000000000000000, 0.9659258262890683122, 1.000000000000000000, 0.9659258262890683122, 1.000000000000000000, 0.9659258262890683122, 1.000000000000000000, 0.9659258262890683122, 1.000000000000000000, 0.9659258262890683122, 1.000000000000000000, 0.9659258262890683122, 1.000000000000000000, 0.9659258262890683122, 1.000000000000000000, 0.9659258262890683122, 1.000000000000000000, 0.9659258262890683122, 1.000000000000000000, 0.9659258262890683122, 1.000000000000000000, 0.9659258262890683122, 1.000000000000000000, 0.9659258262890683122, 1.000000000000000000, 0.9659258262890683122, 1.000000000000000000, 0.9659258262890683122, 1.000000000000000000, 0.9659258262890683122, 1.000000000000000000, 0.9659258262890683122, 1.000000000000000000, 0.9659258262890683122, 1.000000000000000000, 0.9659258262890683122, 1.000000000000000000, 0.9659258262890683122, 1.000000000000000000, 0.9659258262890683122, 1.000000000000000000, 0.9659258262890683122, 1.000000000000000000, 0.9659258262890683122, 1.000000000000000000, 0.9659258262890683122, 1.000000000000000000, 0.9659258262890683122, 1.000000000000000000, 0.9659258262890683122, 1.000000000000000000, 0.9659258262890683122, 1.000000000000000000, 0.9659258262890683122, 1.000000000000000000, 0.9659258262890683122, 1.000000000000000000, 0.9659258262890683122, 1.000000000000000000, 0.9659258262890683122, 1.000000000000000000, 0.9659258262890683122, 1.000000000000000000, 0.9659258262890683122, 1.000000000000000000, 0.9659258262890683122, 1.000000000000000000, 0.9659258262890683122, 1.000000000000000000, 0.9659258262890683122, 1.000000000000000000, 0.9659258262890683122, 1.000000000000000000, 0.9659258262890683122, 1.000000000000000000, 0.9659258262890683122, 1.000000000000000000, 0.9659258262890683122, 1.000000000000000000, 0.9659258262890683122, 1.000000000000000000, 0.9659258262890683122, 1.000000000000000000, 0.9659258262890683122, 1.000000000000000000, 0.9659258262890683122, 1.000000000000000000, 0.9659258262890683122, 1.000000000000000000, 0.9659258262890683122, 1.000000000000000000, 0.9659258262890683122, 1.000000000000000000, 0.9659258262890683122, 1.000000000000000000, 0.9659258262890683122, 1.000000000000000000, 0.9659258262890683122, 1.000000000000000000, 0.9659258262890683122, 1.000000000000000000, 0.9659258262890683122, 1.000000000000000000, 0.9659258262890683122, 1.000000000000000000, 0.9659258262890683122, 1.000000000000000000, 0.9659258262890683122, 1.000000000000000000, 0.9659258262890683122, 1.000000000000000000, 0.9659258262890683122, 1.000000000000000000, 0.9659258262890683122, 1.000000000000000000, 0.9659258262890683122, 1.000000000000000000, 0.9659258262890683122, 1.000000000000000000, 0.9659258262890683122, 1.000000000000000000, 0.9659258262890683122, 1.000000000000000000, 0.9659258262890683122, 1.000000000000000000, 0.9659258262890683122, 1.000000000000000000, 0.9659258262890683122, 1.000000000000000000, 0.9659258262890683122, 1.000000000000000000, 0.9659258262890683122, 1.000000000000000000, 0.9659258262890683122, 1.000000000000000000, 0.9659258262890683122, 1.000000000000000000, 0.9659258262890683122, 1.000000000000000000, 0.9659258262890683122, 1.000000000000000000, 0.9659258262890683122, 1.000000000000000000, 0.9659258262890683122, 1.000000000000000000, 0.9659258262890683122, 1.000000000000000000, 0.9659258262890683122, 1.000000000000000000, 0.9659258262890683122, 1.000000000000000000, 0.9659258262890683122, 1.000000000000000000, 0.9659258262890683122, 1.000000000000000000, 0.9659258262890683122, 1.000000000000000000, 0.9659258262890683122, 1.000000000000000000, 0.9659258262890683122, 1.000000000000000000, 0.9659258262890683122, 1.000000000000000000, 0.9659258262890683122, 1.000000000000000000, 0.9659258262890683122, 1.000000000000000000, 0.9659258262890683122, 1.000000000000000000, 0.9659258262890683122, 1.000000000000000000, 0.9659258262890683122, 1.000000000000000000, 0.9659258262890683122, 1.000000000000000000, 0.9659258262890683122, 1.000000000000000000, 0.9659258262890683122, 1.000000000000000000, 0.9659258262890683122, 1.000000000000000000, 0.9659258262890683122, 1.000000000000000000, 0.9659258262890683122, 1.000000000000000000, 0.9659258262890683122, 1.000000000000000000, 0.9659258262890683122, 1.000000000000000000, 0.9659258262890683122, 1.000000000000000000, 0.9659258262890683122, 1.000000000000000000, 0.9659258262890683122, 1.000000000000000000, 0.9659258262890683122, 1.000000000000000000, 0.9659258262890683122, 1.000000000000000000, 0.9659258262890683122, 1.000000000000000000, 0.9659258262890683122, 1.000000000000000000, 0.9659258262890683122, 1.000000000000000000, 0.9659258262890683122, 1.000000000000000000, 0.9659258262890683122, 1.000000000000000000, 0.9659258262890683122, 1.000000000000000000, 0.9659258262890683122, 1.000000000000000000, 0.9659258262890683122, 1.000000000000000000, 0.9659258262890683122, 1.000000000000000000, 0.9659258262890683122, 1.000000000000000000, 0.9659258262890683122, 1.000000000000000000, 0.9659258262890683122, 1.000000000000000000, 0.9659258262890683122, 1.000000000000000000, 0.9659258262890683122, 1.000000000000000000, 0.9659258262890683122, 1.000000000000000000, 0.9659258262890683122, 1.000000000000000000, 0.9659258262890683122, 1.000000000000000000, 0.9659258262890683122, 1.000000000000000000, 0.9659258262890683122, 1.000000000000000000, 0.9659258262890683122, 1.000000000000000000, 0.9659258262890683122, 1.000000000000000000, 0.9659258262890683122, 1.000000000000000000, 0.9659258262890683122, 1.000000000000000000, 0.9659258262890683122, 1.000000000000000000, 0.9659258262890683122, 1.000000000000000000, 0.9659258262890683122, 1.000000000000000000, 0.9659258262890683122, 1.000000000000000000, 0.9659258262890683122, 1.000000000000000000, 0.9659258262890683122, 1.000000000000000000, 0.9659258262890683122, 1.000000000000000000, 0.9659258262890683122, 1.000000000000000000, 0.9659258262890683122, 1.000000000000000000, 0.9659258262890683122, 1.000000000000000000, 0.9659258262890683122, 1.000000000000000000, 0.9659258262890683122, 1.000000000000000000, 0.9659258262890683122, 1.000000000000000000, 0.9659258262890683122, 1.000000000000000000, 0.9659258262890683122, 1.000000000000000000, 0.9659258262890683122, 1.000000000000000000, 0.9659258262890683122, 1.000000000000000000, 0.9659258262890683122, 1.000000000000000000, 0.9659258262890683122, 1.000000000000000000, 0.9659258262890683122, 1.000000000000000000, 0.9659258262890683122, 1.000000000000000000, 0.9659258262890683122, 1.000000000000000000, 0.9659258262890683122, 1.000000000000000000, 0.9659258262890683122, 1.000000000000000000, 0.9659258262890683122, 1.000000000000000000, 0.9659258262890683122, 1.000000000000000000, 0.9659258262890683122, 1.000000000000000000, 0.9659258262890683122, 1.000000000000000000, 0.9659258262890683122, 1.000000000000000000, 0.9659258262890683122, 1.000000000000000000, 0.9659258262890683122, 1.000000000000000000, 0.9659258262890683122, 1.000000000000000000, 0.9659258262890683122, 1.000000000000000000, 0.9659258262890683122, 1.000000000000000000, 0.9659258262890683122, 1.000000000000000000, 0.9659258262890683122, 1.000000000000000000, 0.9659258262890683122, 1.000000000000000000, 0.9659258262890683122, 1.000000000000000000, 0.9659258262890683122, 1.000000000000000000, 0.9659258262890683122, 1.000000000000000000),
 ( 1.000000000000000000, 0.9659258262890683122, 1.000000000000000000, 0.9659258262890683122, 1.000000000000000000, 0.9659258262890683122, 1.000000000000000000, 0.9659258262890683122, 1.000000000000000000, 0.9659258262890683122, 1.000000000000000000, 0.9659258262890683122, 1.000000000000000000, 0.9659258262890683122, 1.000000000000000000, 0.9659258262890683122, 1.000000000000000000, 0.9659258262890683122, 1.000000000000000000, 0.9659258262890683122, 1.000000000000000000, 0.9659258262890683122, 1.000000000000000000, 0.9659258262890683122, 1.000000000000000000, 0.9659258262890683122, 1.000000000000000000, 0.9659258262890683122, 1.000000000000000000, 0.9659258262890683122, 1.000000000000000000, 0.9659258262890683122, 1.000000000000000000, 0.9659258262890683122, 1.000000000000000000, 0.9659258262890683122, 1.000000000000000000, 0.9659258262890683122, 1.000000000000000000, 0.9659258262890683122, 1.000000000000000000, 0.9659258262890683122, 1.000000000000000000, 0.9659258262890683122, 1.000000000000000000, 0.9659258262890683122, 1.000000000000000000, 0.9659258262890683122, 1.000000000000000000, 0.9659258262890683122, 1.000000000000000000, 0.9659258262890683122, 1.000000000000000000, 0.9659258262890683122, 1.000000000000000000, 0.9659258262890683122, 1.000000000000000000, 0.9659258262890683122, 1.000000000000000000, 0.9659258262890683122, 1.000000000000000000, 0.9659258262890683122, 1.000000000000000000, 0.9659258262890683122, 1.000000000000000000, 0.9659258262890683122, 1.000000000000000000, 0.9659258262890683122, 1.000000000000000000, 0.9659258262890683122, 1.000000000000000000, 0.9659258262890683122, 1.000000000000000000, 0.9659258262890683122, 1.000000000000000000, 0.9659258262890683122, 1.000000000000000000, 0.9659258262890683122, 1.000000000000000000, 0.9659258262890683122, 1.000000000000000000, 0.9659258262890683122, 1.000000000000000000, 0.9659258262890683122, 1.000000000000000000, 0.9659258262890683122, 1.000000000000000000, 0.9659258262890683122, 1.000000000000000000, 0.9659258262890683122, 1.000000000000000000, 0.9659258262890683122, 1.000000000000000000, 0.9659258262890683122, 1.000000000000000000, 0.9659258262890683122, 1.000000000000000000, 0.9659258262890683122, 1.000000000000000000, 0.9659258262890683122, 1.000000000000000000, 0.9659258262890683122, 1.000000000000000000, 0.9659258262890683122, 1.000000000000000000, 0.9659258262890683122, 1.000000000000000000, 0.9659258262890683122, 1.000000000000000000, 0.9659258262890683122, 1.000000000000000000, 0.9659258262890683122, 1.000000000000000000, 0.9659258262890683122, 1.000000000000000000, 0.9659258262890683122, 1.000000000000000000, 0.9659258262890683122, 1.000000000000000000, 0.9659258262890683122, 1.000000000000000000, 0.9659258262890683122, 1.000000000000000000, 0.9659258262890683122, 1.000000000000000000, 0.9659258262890683122, 1.000000000000000000, 0.9659258262890683122, 1.000000000000000000, 0.9659258262890683122, 1.000000000000000000, 0.9659258262890683122, 1.000000000000000000, 0.9659258262890683122, 1.000000000000000000, 0.9659258262890683122, 1.000000000000000000, 0.9659258262890683122, 1.000000000000000000, 0.9659258262890683122, 1.000000000000000000, 0.9659258262890683122, 1.000000000000000000, 0.9659258262890683122, 1.000000000000000000, 0.9659258262890683122, 1.000000000000000000, 0.9659258262890683122, 1.000000000000000000, 0.9659258262890683122, 1.000000000000000000, 0.9659258262890683122, 1.000000000000000000, 0.9659258262890683122, 1.000000000000000000, 0.9659258262890683122, 1.000000000000000000, 0.9659258262890683122, 1.000000000000000000, 0.9659258262890683122, 1.000000000000000000, 0.9659258262890683122, 1.000000000000000000, 0.9659258262890683122, 1.000000000000000000, 0.9659258262890683122, 1.000000000000000000, 0.9659258262890683122, 1.000000000000000000, 0.9659258262890683122, 1.000000000000000000, 0.9659258262890683122, 1.000000000000000000, 0.9659258262890683122, 1.000000000000000000, 0.9659258262890683122, 1.000000000000000000, 0.9659258262890683122, 1.000000000000000000, 0.9659258262890683122, 1.000000000000000000, 0.9659258262890683122, 1.000000000000000000, 0.9659258262890683122, 1.000000000000000000, 0.9659258262890683122, 1.000000000000000000, 0.9659258262890683122, 1.000000000000000000, 0.9659258262890683122, 1.000000000000000000, 0.9659258262890683122, 1.000000000000000000, 0.9659258262890683122, 1.000000000000000000, 0.9659258262890683122, 1.000000000000000000, 0.9659258262890683122, 1.000000000000000000, 0.9659258262890683122, 1.000000000000000000, 0.9659258262890683122, 1.000000000000000000, 0.9659258262890683122, 1.000000000000000000, 0.9659258262890683122, 1.000000000000000000, 0.9659258262890683122, 1.000000000000000000, 0.9659258262890683122, 1.000000000000000000, 0.9659258262890683122, 1.000000000000000000, 0.9659258262890683122, 1.000000000000000000, 0.9659258262890683122, 1.000000000000000000, 0.9659258262890683122, 1.000000000000000000, 0.9659258262890683122, 1.000000000000000000, 0.9659258262890683122, 1.000000000000000000, 0.9659258262890683122, 1.000000000000000000, 0.9659258262890683122, 1.000000000000000000, 0.9659258262890683122, 1.000000000000000000, 0.9659258262890683122, 1.000000000000000000, 0.9659258262890683122, 1.000000000000000000, 0.9659258262890683122, 1.000000000000000000, 0.9659258262890683122, 1.000000000000000000, 0.9659258262890683122, 1.000000000000000000, 0.9659258262890683122, 1.000000000000000000, 0.9659258262890683122, 1.000000000000000000, 0.9659258262890683122, 1.000000000000000000, 0.9659258262890683122, 1.000000000000000000, 0.9659258262890683122, 1.000000000000000000, 0.9659258262890683122, 1.000000000000000000, 0.9659258262890683122, 1.000000000000000000, 0.9659258262890683122, 1.000000000000000000, 0.9659258262890683122, 1.000000000000000000, 0.9659258262890683122, 1.000000000000000000, 0.9659258262890683122, 1.000000000000000000, 0.9659258262890683122, 1.000000000000000000, 0.9659258262890683122, 1.000000000000000000, 0.9659258262890683122, 1.000000000000000000, 0.9659258262890683122, 1.000000000000000000, 0.9659258262890683122, 1.000000000000000000, 0.9659258262890683122, 1.000000000000000000, 0.9659258262890683122, 1.000000000000000000, 0.9659258262890683122, 1.000000000000000000, 0.9659258262890683122, 1.000000000000000000, 0.9659258262890683122, 1.000000000000000000, 0.9659258262890683122, 1.000000000000000000, 0.9659258262890683122, 1.000000000000000000, 0.9659258262890683122, 1.000000000000000000, 0.9659258262890683122, 1.000000000000000000, 0.9659258262890683122, 1.000000000000000000, 0.9659258262890683122, 1.000000000000000000, 0.9659258262890683122, 1.000000000000000000, 0.9659258262890683122, 1.000000000000000000, 0.9659258262890683122, 1.000000000000000000, 0.9659258262890683122, 1.000000000000000000, 0.9659258262890683122, 1.000000000000000000, 0.9659258262890683122, 1.000000000000000000, 0.9659258262890683122, 1.000000000000000000, 0.9659258262890683122, 1.000000000000000000, 0.9659258262890683122, 1.000000000000000000, 0.9659258262890683122, 1.000000000000000000, 0.9659258262890683122, 1.000000000000000000, 0.9659258262890683122, 1.000000000000000000, 0.9659258262890683122, 1.000000000000000000, 0.9659258262890683122, 1.000000000000000000, 0.9659258262890683122, 1.000000000000000000, 0.9659258262890683122, 1.000000000000000000, 0.9659258262890683122, 1.000000000000000000, 0.9659258262890683122, 1.000000000000000000, 0.9659258262890683122, 1.000000000000000000, 0.9659258262890683122, 1.000000000000000000, 0.9659258262890683122, 1.000000000000000000, 0.9659258262890683122, 1.000000000000000000, 0.9659258262890683122, 1.000000000000000000, 0.9659258262890683122, 1.000000000000000000, 0.9659258262890683122, 1.000000000000000000, 0.9659258262890683122, 1.000000000000000000, 0.9659258262890683122, 1.000000000000000000, 0.9659258262890683122, 1.000000000000000000, 0.9659258262890683122, 1.000000000000000000, 0.9659258262890683122, 1.000000000000000000, 0.9659258262890683122, 1.000000000000000000, 0.9659258262890683122, 1.000000000000000000, 0.9659258262890683122, 1.000000000000000000, 0.9659258262890683122, 1.000000000000000000, 0.9659258262890683122, 1.000000000000000000, 0.9659258262890683122, 1.000000000000000000, 0.9659258262890683122, 1.000000000000000000, 0.9659258262890683122, 1.000000000000000000, 0.9659258262890683122, 1.000000000000000000, 0.9659258262890683122, 1.000000000000000000, 0.9659258262890683122, 1.000000000000000000, 0.9659258262890683122, 1.000000000000000000, 0.9659258262890683122, 1.000000000000000000, 0.9659258262890683122, 1.000000000000000000, 0.9659258262890683122, 1.000000000000000000, 0.9659258262890683122, 1.000000000000000000, 0.9659258262890683122, 1.000000000000000000, 0.9659258262890683122, 1.000000000000000000, 0.9659258262890683122, 1.000000000000000000, 0.9659258262890683122, 1.000000000000000000, 0.9659258262890683122, 1.000000000000000000, 0.9659258262890683122, 1.000000000000000000, 0.9659258262890683122, 1.000000000000000000, 0.9659258262890683122, 1.000000000000000000, 0.9659258262890683122, 1.000000000000000000, 0.9659258262890683122, 1.000000000000000000, 0.9659258262890683122, 1.000000000000000000, 0.9659258262890683122, 1.000000000000000000, 0.9659258262890683122, 1.000000000000000000, 0.9659258262890683122, 1.000000000000000000, 0.9659258262890683122, 1.000000000000000000, 0.9659258262890683122, 1.000000000000000000, 0.9659258262890683122, 1.000000000000000000, 0.9659258262890683122, 1.000000000000000000, 0.9659258262890683122, 1.000000000000000000, 0.9659258262890683122, 1.000000000000000000, 0.9659258262890683122, 1.000000000000000000, 0.9659258262890683122, 1.000000000000000000, 0.9659258262890683122, 1.000000000000000000, 0.9659258262890683122, 1.000000000000000000, 0.9659258262890683122, 1.000000000000000000, 0.9659258262890683122, 1.000000000000000000, 0.9659258262890683122, 1.000000000000000000, 0.9659258262890683122, 1.000000000000000000, 0.9659258262890683122, 1.000000000000000000, 0.9659258262890683122, 1.000000000000000000, 0.9659258262890683122, 1.000000000000000000, 0.9659258262890683122, 1.000000000000000000, 0.9659258262890683122, 1.000000000000000000, 0.9659258262890683122, 1.000000000000000000, 0.9659258262890683122, 1.000000000000000000, 0.9659258262890683122, 1.000000000000000000, 0.9659258262890683122, 1.000000000000000000, 0.9659258262890683122, 1.000000000000000000, 0.9659258262890683122, 1.000000000000000000, 0.9659258262890683122, 1.000000000000000000, 0.9659258262890683122, 1.000000000000000000, 0.9659258262890683122, 1.000000000000000000, 0.9659258262890683122, 1.000000000000000000, 0.9659258262890683122, 1.000000000000000000, 0.9659258262890683122, 1.000000000000000000, 0.9659258262890683122, 1.000000000000000000, 0.9659258262890683122, 1.000000000000000000, 0.9659258262890683122, 1.000000000000000000, 0.9659258262890683122, 1.000000000000000000, 0.9659258262890683122, 1.000000000000000000, 0.9659258262890683122, 1.000000000000000000, 0.9659258262890683122, 1.000000000000000000, 0.9659258262890683122, 1.000000000000000000, 0.9659258262890683122, 1.000000000000000000, 0.9659258262890683122, 1.000000000000000000, 0.9659258262890683122, 1.000000000000000000, 0.9659258262890683122, 1.000000000000000000, 0.9659258262890683122, 1.000000000000000000, 0.9659258262890683122, 1.000000000000000000, 0.9659258262890683122, 1.000000000000000000, 0.9659258262890683122, 1.000000000000000000, 0.9659258262890683122, 1.000000000000000000, 0.9659258262890683122, 1.000000000000000000) ) ) 
 REPRESENTATION_ITEM ( '' )  SURFACE ( )  );
#44386=CARTESIAN_POINT ( 'NONE',  ( -0.4527559055118102749, -0.4536011799217368745, -0.2665933059059886201 ) ) ;
#44387=CARTESIAN_POINT ( 'NONE',  ( -1.003937007874014853, 0.1660481256975885056, 0.3530559997133364547 ) ) ;
#44388=CARTESIAN_POINT ( 'NONE',  ( 0.9711286089238851948, -0.6046776061558809534, -0.2411417322834644161 ) ) ;
#44390=PLANE ( 'NONE',  #46299 ) ;
#44392=B_SPLINE_CURVE_WITH_KNOTS ( 'NONE', 3,
 ( #63925, #13424, #52947, #52533, #32770, #26032, #64343 ),
 .UNSPECIFIED., .F., .F.,
 ( 4, 3, 4 ),
 ( 7.459310946700270506E-17, 0.001246232571205254649, 0.002492492258783168303 ),
 .UNSPECIFIED. ) ;
#44393=CARTESIAN_POINT ( 'NONE',  ( 1.240157480314961314, 0.1660481256975883668, -0.3530559997133364547 ) ) ;
#44394=CARTESIAN_POINT ( 'NONE',  ( -1.181102362204723644, -0.1870078740157480879, -0.4822834645669291653 ) ) ;
#44396=CARTESIAN_POINT ( 'NONE',  ( -0.4593175853018366950, -0.004921259842519576551, 0.3153832671262227771 ) ) ;
#44398=CARTESIAN_POINT ( 'NONE',  ( -0.3018372703412066094, -0.3690944881889765550, -0.3153832671262227771 ) ) ;
#44399=CARTESIAN_POINT ( 'NONE',  ( 0.5643044619422579178, -0.3690944881889765550, -0.3153832671262227771 ) ) ;
#44400=CARTESIAN_POINT ( 'NONE',  ( 0.1902887139107617975, 0.2952755905511811885, 0.1292274648535926551 ) ) ;
#44401=CARTESIAN_POINT ( 'NONE',  ( -0.7611548556430438595, -0.5023911411419708095, -0.1820866141732282451 ) ) ;
#44403=CARTESIAN_POINT ( 'NONE',  ( 1.017060367454068581, -0.05778040916215560624, -0.4822834645669293319 ) ) ;
#44404=CARTESIAN_POINT ( 'NONE',  ( -1.233595800524933894, -0.6046776061558809534, -0.2411417322834644161 ) ) ;
#44406=CARTESIAN_POINT ( 'NONE',  ( -0.5708661417322828946, 0.1660481256975883668, -0.3530559997133364547 ) ) ;
#44407=CARTESIAN_POINT ( 'NONE',  ( -0.9580052493438311334, 0.05413385826771626580, -0.4176697321401330321 ) ) ;
#44408=CARTESIAN_POINT ( 'NONE',  ( 1.272965879265092637, -0.3690944881889765550, -0.3153832671262227771 ) ) ;
#44409=CARTESIAN_POINT ( 'NONE',  ( -0.09842519685039295696, 0.07958543189024071263, -0.2665933059059888421 ) ) ;
#44410=CARTESIAN_POINT ( 'NONE',  ( -0.6692913385826764205, -0.6692913385826771977, 8.415575281601705876E-17 ) ) ;
#44411=CARTESIAN_POINT ( 'NONE',  ( -1.299212598425196097, 0.2952755905511811885, 0.000000000000000000 ) ) ;
#44413=CARTESIAN_POINT ( 'NONE',  ( 1.489501312335958172, -0.2845877964562159024, 0.3641732283464567677 ) ) ;
#44414=CARTESIAN_POINT ( 'NONE',  ( -0.4658792650918627265, -0.3162353388693409650, -0.4822834645669289433 ) ) ;
#44415=CARTESIAN_POINT ( 'NONE',  ( -1.200787401574802349, 0.1660481256975883668, -0.3530559997133364547 ) ) ;
#44418=CARTESIAN_POINT ( 'NONE',  ( -0.8661417322834640276, -0.1870078740157479769, 0.3641732283464567677 ) ) ;
#44419=CARTESIAN_POINT ( 'NONE',  ( 1.220472440944882386, -0.6692913385826771977, 8.415575281601705876E-17 ) ) ;
#44420=CARTESIAN_POINT ( 'NONE',  ( -1.056430446194224881, 0.1771653543307087075, -0.09757992244046823083 ) ) ;
#44422=CARTESIAN_POINT ( 'NONE',  ( -0.8464566929133852113, -0.5400638737290845981, -0.3530559997133363437 ) ) ;
#44423=CARTESIAN_POINT ( 'NONE',  ( 0.9383202099737538715, -0.05778040916215560624, -0.4822834645669293319 ) ) ;
#44424=CARTESIAN_POINT ( 'NONE',  ( 0.9580052493438327987, -0.4281496062992127816, -0.4176697321401328100 ) ) ;
#44425=EDGE_CURVE ( 'NONE', #25432, #30707, #80521, .T. ) ;
#44426=CARTESIAN_POINT ( 'NONE',  ( 1.443569553805774897, 0.2306618581243848609, 0.2411417322834645549 ) ) ;
#44427=CARTESIAN_POINT ( 'NONE',  ( -1.345144356955379816, -0.08942795157528024563, -0.3641732283464568787 ) ) ;
#44432=CARTESIAN_POINT ( 'NONE',  ( 1.187664041994751285, -0.08942795157527998196, 0.3641732283464567121 ) ) ;
#44433=CARTESIAN_POINT ( 'NONE',  ( 0.9383202099737536495, -0.2845877964562159024, 0.3641732283464567677 ) ) ;
#44435=CARTESIAN_POINT ( 'NONE',  ( 0.4133858267716541968, -0.5400638737290845981, -0.3530559997133363437 ) ) ;
#44438=CARTESIAN_POINT ( 'NONE',  ( 0.7152230971128616943, -0.08942795157527998196, 0.3641732283464567121 ) ) ;
#44439=CARTESIAN_POINT ( 'NONE',  ( -0.4330708661417315697, -0.6692913385826771977, 8.415575281601705876E-17 ) ) ;
#44440=CARTESIAN_POINT ( 'NONE',  ( -1.115485564304461219, 0.05413385826771626580, -0.4176697321401330321 ) ) ;
#44441=CARTESIAN_POINT ( 'NONE',  ( 0.9448818897637802916, -0.1870078740157480879, -0.4822834645669291653 ) ) ;
#44445=VERTEX_POINT ( 'NONE', #70489 ) ;
#44446=ORIENTED_EDGE ( 'NONE', *, *, #60654, .F. ) ;
#44447=CARTESIAN_POINT ( 'NONE',  ( -1.128608923884513837, -0.6046776061558807314, 0.2411417322834647770 ) ) ;
#44448=CARTESIAN_POINT ( 'NONE',  ( -0.4133858267716528645, -0.5400638737290844871, 0.3530559997133364547 ) ) ;
#44449=CARTESIAN_POINT ( 'NONE',  ( -0.8005249343832011588, -0.004921259842519870586, -0.3153832671262229437 ) ) ;
#44450=CARTESIAN_POINT ( 'NONE',  ( -0.8989501312335946848, -0.6692913385826771977, 0.1292274648535927661 ) ) ;
#44452=CARTESIAN_POINT ( 'NONE',  ( 0.4527559055118117182, 0.1660481256975883668, -0.3530559997133364547 ) ) ;
#44454=CARTESIAN_POINT ( 'NONE',  ( -0.2427821522309703550, -0.3162353388693405765, 0.4822834645669290543 ) ) ;
#44455=CARTESIAN_POINT ( 'NONE',  ( 1.384514435695538337, -0.6692913385826771977, 0.1292274648535927661 ) ) ;
#44457=CARTESIAN_POINT ( 'NONE',  ( -0.7545931758530177724, 0.2952755905511811885, 0.1292274648535926551 ) ) ;
#44458=CARTESIAN_POINT ( 'NONE',  ( 0.6430446194225728496, 0.05413385826771666132, 0.4176697321401328100 ) ) ;
#44460=CARTESIAN_POINT ( 'NONE',  ( -0.8267716535433065062, 0.1771653543307087630, 0.000000000000000000 ) ) ;
#44464=CARTESIAN_POINT ( 'NONE',  ( -1.430446194225721390, -0.3690944881889763329, 0.3153832671262228327 ) ) ;
#44465=CARTESIAN_POINT ( 'NONE',  ( -1.194225721784776262, -0.4281496062992124485, 0.4176697321401328655 ) ) ;
#44466=CARTESIAN_POINT ( 'NONE',  ( -0.8005249343832011588, 0.05413385826771626580, -0.4176697321401330321 ) ) ;
#44468=CARTESIAN_POINT ( 'NONE',  ( -1.023622047244094002, -0.1870078740157480879, -0.4822834645669291653 ) ) ;
#44469=CARTESIAN_POINT ( 'NONE',  ( -1.450131233595799651, -0.6692913385826771977, 0.1292274648535927661 ) ) ;
#44471=DIRECTION ( 'NONE',  ( 0.000000000000000000, 0.000000000000000000, -1.000000000000000000 ) ) ;
#44472=CARTESIAN_POINT ( 'NONE',  ( 0.3346456692913393205, -0.4536011799217368745, -0.2665933059059886201 ) ) ;
#44475=CARTESIAN_POINT ( 'NONE',  ( -0.5511811023622041894, -0.1870078740157480601, -0.3641732283464567677 ) ) ;
#44476=CARTESIAN_POINT ( 'NONE',  ( -0.2230971128608915943, 0.05413385826771666132, 0.4176697321401328100 ) ) ;
#44477=CARTESIAN_POINT ( 'NONE',  ( 1.397637795275591177, -0.5400638737290844871, 0.3530559997133364547 ) ) ;
#44478=CARTESIAN_POINT ( 'NONE',  ( -0.4790026246719152336, -0.05778040916215560624, -0.4822834645669293319 ) ) ;
#44480=ORIENTED_EDGE ( 'NONE', *, *, #68203, .F. ) ;
#44482=CARTESIAN_POINT ( 'NONE',  ( -0.3674540682414689785, 0.2306618581243848609, 0.2411417322834645549 ) ) ;
#44483=CARTESIAN_POINT ( 'NONE',  ( 1.102362204724410155, -0.1870078740157479769, 0.4822834645669291653 ) ) ;
#44484=CARTESIAN_POINT ( 'NONE',  ( -1.062992125984250968, 0.1771653543307087630, 0.000000000000000000 ) ) ;
#44485=CARTESIAN_POINT ( 'NONE',  ( -1.515748031496062076, 0.1660481256975883668, -0.3530559997133364547 ) ) ;
#44487=EDGE_CURVE ( 'NONE', #7970, #56774, #76940, .T. ) ;
#44490=CARTESIAN_POINT ( 'NONE',  ( 1.515748031496063408, 0.1660481256975885056, 0.3530559997133364547 ) ) ;
#44491=DIRECTION ( 'NONE',  ( 0.7071067811865462405, -0.000000000000000000, 0.7071067811865486830 ) ) ;
#44492=CARTESIAN_POINT ( 'NONE',  ( 0.07874015748031558404, -0.1870078740157479769, 0.4822834645669291653 ) ) ;
#44493=CARTESIAN_POINT ( 'NONE',  ( -0.9842519685039360366, 0.1771653543307087630, 0.000000000000000000 ) ) ;
#44494=CARTESIAN_POINT ( 'NONE',  ( -0.3805774278215216522, -0.4281496062992127816, -0.4176697321401328100 ) ) ;
#44496=CARTESIAN_POINT ( 'NONE',  ( -0.7349081364829390672, 0.2306618581243847221, -0.2411417322834647770 ) ) ;
#44497=CARTESIAN_POINT ( 'NONE',  ( -1.082677165354329896, 0.1660481256975885056, 0.3530559997133364547 ) ) ;
#44498=EDGE_CURVE ( 'NONE', #58545, #16126, #56519, .T. ) ;
#44500=CARTESIAN_POINT ( 'NONE',  ( 0.8727034120734912248, -0.2845877964562161244, -0.3641732283464567121 ) ) ;
#44501=CARTESIAN_POINT ( 'NONE',  ( -0.3477690288713905509, -0.5511811023622046335, 0.09757992244046803654 ) ) ;
#44502=CARTESIAN_POINT ( 'NONE',  ( 0.8923884514435703741, 0.1283753931104748280, 0.1820866141732283561 ) ) ;
#44503=CARTESIAN_POINT ( 'NONE',  ( -1.633858267716534529, -0.5400638737290845981, -0.3530559997133363437 ) ) ;
#44505=CARTESIAN_POINT ( 'NONE',  ( 1.312335958005249825, 0.2306618581243847221, -0.2411417322834647770 ) ) ;
#44506=CARTESIAN_POINT ( 'NONE',  ( 0.6561679790026253567, -0.5023911411419708095, -0.1820866141732282451 ) ) ;
#44507=CARTESIAN_POINT ( 'NONE',  ( -0.6561679790026240244, 0.2306618581243847221, -0.2411417322834647770 ) ) ;
#44508=CARTESIAN_POINT ( 'NONE',  ( 1.181102362204724976, -0.1870078740157480879, -0.4822834645669291653 ) ) ;
#44511=CARTESIAN_POINT ( 'NONE',  ( -0.1968503937007867743, 0.1771653543307087630, 0.000000000000000000 ) ) ;
#44513=CARTESIAN_POINT ( 'NONE',  ( 0.4593175853018380828, 0.05413385826771626580, -0.4176697321401330321 ) ) ;
#44514=CARTESIAN_POINT ( 'NONE',  ( 0.6415071261929219393, 0.02791078216816263863, 0.4328096321851903627 ) ) ;
#44515=CARTESIAN_POINT ( 'NONE',  ( 0.9842519685039375910, 0.1771653543307087630, 0.000000000000000000 ) ) ;
#44516=CARTESIAN_POINT ( 'NONE',  ( 0.08530183727034192087, -0.2845877964562161244, -0.3641732283464567121 ) ) ;
#44517=CARTESIAN_POINT ( 'NONE',  ( -1.528871391076114250, 0.2952755905511810774, -0.1292274648535930714 ) ) ;
#44518=CARTESIAN_POINT ( 'NONE',  ( -0.5774278215223089816, -0.5023911411419708095, 0.1820866141732285504 ) ) ;
#44519=DIRECTION ( 'NONE',  ( 0.8479387356305982948, 2.625811289636359704E-16, -0.5300942374872437135 ) ) ;
#44520=CARTESIAN_POINT ( 'NONE',  ( -1.010498687664041384, -0.4281496062992127816, -0.4176697321401328100 ) ) ;
#44521=CARTESIAN_POINT ( 'NONE',  ( -0.6299212598425188991, -0.1870078740157480879, -0.4822834645669291653 ) ) ;
#44524=CARTESIAN_POINT ( 'NONE',  ( 0.5643044619422579178, -0.3690944881889765550, -0.3153832671262227771 ) ) ;
#44525=CARTESIAN_POINT ( 'NONE',  ( -0.4265091863517051496, -0.6692913385826771977, 0.1292274648535927661 ) ) ;
#44526=CARTESIAN_POINT ( 'NONE',  ( -0.7611548556430438595, -0.6046776061558809534, -0.2411417322834644161 ) ) ;
#44527=CARTESIAN_POINT ( 'NONE',  ( -0.8858267716535425107, -0.4536011799217367080, 0.2665933059059888421 ) ) ;
#44528=CYLINDRICAL_SURFACE ( 'NONE', #27964, 3.543307086614173151 ) ;
#44529=CARTESIAN_POINT ( 'NONE',  ( -0.05905511811023545637, 0.1660481256975885056, 0.3530559997133364547 ) ) ;
#44530=CARTESIAN_POINT ( 'NONE',  ( -1.587926509186350810, -0.3690944881889763329, 0.3153832671262228327 ) ) ;
#44531=CARTESIAN_POINT ( 'NONE',  ( 1.213910761154856299, -0.6692913385826773087, -0.1292274648535924053 ) ) ;
#44535=CARTESIAN_POINT ( 'NONE',  ( -1.089942661822471459, 0.000000000000000000, 0.3464511005275205946 ) ) ;
#44536=CARTESIAN_POINT ( 'NONE',  ( -1.469816272965878357, -0.6046776061558809534, -0.2411417322834644161 ) ) ;
#44537=CARTESIAN_POINT ( 'NONE',  ( -0.9842519685039365918, -0.6692913385826771977, 8.415575281601705876E-17 ) ) ;
#44538=CARTESIAN_POINT ( 'NONE',  ( -1.410761154855641575, -0.3162353388693409650, -0.4822834645669289433 ) ) ;
#44540=LINE ( 'NONE', #10934, #57867 ) ;
#44541=CARTESIAN_POINT ( 'NONE',  ( 1.128608923884515169, -0.6046776061558809534, -0.2411417322834644161 ) ) ;
#44542=CARTESIAN_POINT ( 'NONE',  ( -0.02624671916010428221, 0.2306618581243847221, -0.2411417322834647770 ) ) ;
#44543=CARTESIAN_POINT ( 'NONE',  ( -0.3268936723430463931, 1.297973861003007810E-15, -0.3627985898453513491 ) ) ;
#44544=CARTESIAN_POINT ( 'NONE',  ( -0.6970755509724322341, 0.02791078216816064370, 0.4328096321851915285 ) ) ;
#44545=CARTESIAN_POINT ( 'NONE',  ( 1.207349081364829990, -0.5023911411419708095, -0.1820866141732282451 ) ) ;
#44551=CARTESIAN_POINT ( 'NONE',  ( 0.4133858267716541968, -0.5400638737290845981, -0.3530559997133363437 ) ) ;
#44552=CARTESIAN_POINT ( 'NONE',  ( -0.6955380577427815458, -0.4281496062992127816, -0.4176697321401328100 ) ) ;
#44553=CARTESIAN_POINT ( 'NONE',  ( -1.358267716535432434, -0.5400638737290844871, 0.3530559997133364547 ) ) ;
#44554=CARTESIAN_POINT ( 'NONE',  ( 0.5839895013123367340, 0.2952755905511811885, 0.1292274648535926551 ) ) ;
#44555=CARTESIAN_POINT ( 'NONE',  ( -1.515748031496062076, -0.4536011799217367080, 0.2665933059059888421 ) ) ;
#44556=CARTESIAN_POINT ( 'NONE',  ( 1.496062992125984703, -0.1870078740157480879, -0.4822834645669291653 ) ) ;
#44557=CARTESIAN_POINT ( 'NONE',  ( -0.02624671916010428221, 0.2306618581243847221, -0.2411417322834647770 ) ) ;
#44559=CARTESIAN_POINT ( 'NONE',  ( -1.338582677165353729, -0.1870078740157479769, 0.4822834645669291653 ) ) ;
#44560=CARTESIAN_POINT ( 'NONE',  ( 1.148293963254593653, 0.2952755905511810774, -0.1292274648535930714 ) ) ;
#44561=CARTESIAN_POINT ( 'NONE',  ( 1.574803149606299746, -0.1870078740157480879, -0.4822834645669291653 ) ) ;
#44563=CARTESIAN_POINT ( 'NONE',  ( 0.3280839895013130669, -0.3690944881889765550, -0.3153832671262227771 ) ) ;
#44564=ORIENTED_EDGE ( 'NONE', *, *, #31972, .F. ) ;
#44566=VERTEX_POINT ( 'NONE', #57023 ) ;
#44567=CARTESIAN_POINT ( 'NONE',  ( 0.07874015748031558404, -0.1870078740157480601, -0.3641732283464567677 ) ) ;
#44569=CARTESIAN_POINT ( 'NONE',  ( 0.2099737532808405305, 0.2306618581243847221, -0.2411417322834647770 ) ) ;
#44570=CARTESIAN_POINT ( 'NONE',  ( -0.006561679790025524116, -0.3162353388693405765, 0.4822834645669290543 ) ) ;
#44571=CARTESIAN_POINT ( 'NONE',  ( -0.4461942257217840213, 0.2306618581243848609, 0.2411417322834645549 ) ) ;
#44573=CARTESIAN_POINT ( 'NONE',  ( -1.272965879265091305, 0.05413385826771626580, -0.4176697321401330321 ) ) ;
#44575=CARTESIAN_POINT ( 'NONE',  ( 1.443569553805774897, 0.1283753931104748280, 0.1820866141732283561 ) ) ;
#44576=CARTESIAN_POINT ( 'NONE',  ( 0.9383202099737538715, -0.05778040916215560624, -0.4822834645669293319 ) ) ;
#44577=CARTESIAN_POINT ( 'NONE',  ( 0.8005249343832028242, -0.4281496062992127816, -0.4176697321401328100 ) ) ;
#44579=CARTESIAN_POINT ( 'NONE',  ( -1.187664041994750175, -0.05778040916215560624, -0.4822834645669293319 ) ) ;
#44582=CARTESIAN_POINT ( 'NONE',  ( -0.09842519685039295696, 0.1660481256975883668, -0.3530559997133364547 ) ) ;
#44585=CARTESIAN_POINT ( 'NONE',  ( 1.253280839895013710, -0.3162353388693405765, 0.4822834645669290543 ) ) ;
#44586=CARTESIAN_POINT ( 'NONE',  ( 1.476377952755906442, -0.5400638737290844871, 0.3530559997133364547 ) ) ;
#44587=CARTESIAN_POINT ( 'NONE',  ( 0.03280839895013198948, -0.5511811023622048555, -0.09757992244046775898 ) ) ;
#44588=CARTESIAN_POINT ( 'NONE',  ( 0.8595800524934390507, -0.05778040916215560624, -0.4822834645669293319 ) ) ;
#44590=CARTESIAN_POINT ( 'NONE',  ( 0.4133858267716541968, 0.07958543189024085140, 0.2665933059059887866 ) ) ;
#44591=CARTESIAN_POINT ( 'NONE',  ( 0.3674540682414705883, 0.2306618581243847221, -0.2411417322834647770 ) ) ;
#44593=CARTESIAN_POINT ( 'NONE',  ( -1.253280839895012377, -0.05778040916215522460, 0.4822834645669289988 ) ) ;
#44594=CARTESIAN_POINT ( 'NONE',  ( 1.082677165354331228, -0.4536011799217367080, 0.2665933059059888421 ) ) ;
#44595=CARTESIAN_POINT ( 'NONE',  ( 0.3674540682414705883, 0.1539470093639521697, -0.1968503937007875793 ) ) ;
#44596=CARTESIAN_POINT ( 'NONE',  ( -0.4068241469816267775, 0.05413385826771626580, -0.4176697321401330321 ) ) ;
#44597=CARTESIAN_POINT ( 'NONE',  ( -0.3740157480314953431, 0.07958543189024085140, 0.2665933059059887866 ) ) ;
#44599=CARTESIAN_POINT ( 'NONE',  ( -0.3937007874015740483, -0.1870078740157480879, -0.4822834645669291653 ) ) ;
#44600=CARTESIAN_POINT ( 'NONE',  ( 0.1574803149606306130, -0.1870078740157479769, 0.3641732283464567677 ) ) ;
#44602=CARTESIAN_POINT ( 'NONE',  ( 0.1049868766404206816, 0.2306618581243848609, 0.2411417322834645549 ) ) ;
#44604=CARTESIAN_POINT ( 'NONE',  ( 0.9973753280839902091, -0.5023911411419708095, 0.1820866141732285504 ) ) ;
#44606=CARTESIAN_POINT ( 'NONE',  ( -0.7480314960629914633, 0.1771653543307087630, 0.000000000000000000 ) ) ;
#44607=CARTESIAN_POINT ( 'NONE',  ( -0.6496062992125976043, -0.4536011799217367080, 0.2665933059059888421 ) ) ;
#44608=CARTESIAN_POINT ( 'NONE',  ( -0.1115485564304453947, -0.6692913385826771977, 0.1292274648535927661 ) ) ;
#44609=CARTESIAN_POINT ( 'NONE',  ( -0.07874015748031421014, -0.1870078740157480879, -0.4822834645669291653 ) ) ;
#44610=CARTESIAN_POINT ( 'NONE',  ( 0.7545931758530189937, 0.1771653543307087075, -0.09757992244046823083 ) ) ;
#44612=CARTESIAN_POINT ( 'NONE',  ( 1.463254593175853824, 0.1771653543307087075, -0.09757992244046823083 ) ) ;
#44614=CARTESIAN_POINT ( 'NONE',  ( 0.7414698162729663755, 0.2952755905511811885, 0.1292274648535926551 ) ) ;
#44616=CARTESIAN_POINT ( 'NONE',  ( -0.4724409448818890911, -0.1870078740157479769, 0.4822834645669291653 ) ) ;
#44618=CARTESIAN_POINT ( 'NONE',  ( -1.463254593175852492, -0.6692913385826773087, -0.1292274648535924053 ) ) ;
#44619=CARTESIAN_POINT ( 'NONE',  ( 0.9448818897637802916, -0.1870078740157480879, -0.4822834645669291653 ) ) ;
#44620=CARTESIAN_POINT ( 'NONE',  ( 0.3937007874015754361, -0.1870078740157479769, 0.4822834645669291653 ) ) ;
#44622=CARTESIAN_POINT ( 'NONE',  ( 0.2559055118110243332, 0.07958543189024085140, 0.2665933059059887866 ) ) ;
#44623=CARTESIAN_POINT ( 'NONE',  ( 1.207349081364829990, 0.2306618581243848609, 0.2411417322834645549 ) ) ;
#44624=CARTESIAN_POINT ( 'NONE',  ( -0.4986876640419942164, -0.5023911411419708095, 0.1820866141732285504 ) ) ;
#44625=CARTESIAN_POINT ( 'NONE',  ( -0.7480314960629914633, -0.6692913385826771977, 8.415575281601705876E-17 ) ) ;
#44626=CARTESIAN_POINT ( 'NONE',  ( 0.8202099737532814183, 0.2952755905511811885, 0.1292274648535926551 ) ) ;
#44627=CARTESIAN_POINT ( 'NONE',  ( 0.2952755905511816326, -0.5400638737290844871, 0.3530559997133364547 ) ) ;
#44628=CARTESIAN_POINT ( 'NONE',  ( -0.8136482939632537770, 0.2306618581243847221, -0.2411417322834647770 ) ) ;
#44629=CARTESIAN_POINT ( 'NONE',  ( -0.6364829396325453192, -0.2845877964562159024, 0.3641732283464567677 ) ) ;
#44630=CARTESIAN_POINT ( 'NONE',  ( 0.5774278215223103139, -0.6046776061558809534, -0.2411417322834644161 ) ) ;
#44631=CARTESIAN_POINT ( 'NONE',  ( -1.279527559055116948, -0.5400638737290844871, 0.3530559997133364547 ) ) ;
#44632=CARTESIAN_POINT ( 'NONE',  ( -0.4855643044619415427, 0.05413385826771626580, -0.4176697321401330321 ) ) ;
#44634=CARTESIAN_POINT ( 'NONE',  ( 1.345144356955381593, -0.3162353388693409650, -0.4822834645669289433 ) ) ;
#44635=CARTESIAN_POINT ( 'NONE',  ( 1.141732283464567788, -0.6692913385826771977, 8.415575281601705876E-17 ) ) ;
#44639=CARTESIAN_POINT ( 'NONE',  ( -0.9448818897637790704, -0.1870078740157479769, 0.4822834645669291653 ) ) ;
#44644=CARTESIAN_POINT ( 'NONE',  ( -0.03280839895013062252, 0.1771653543307087075, -0.09757992244046823083 ) ) ;
#44646=CARTESIAN_POINT ( 'NONE',  ( 0.8727034120734912248, -0.3162353388693409650, -0.4822834645669289433 ) ) ;
#44649=CARTESIAN_POINT ( 'NONE',  ( -0.4986876640419939388, 0.1283753931104746893, -0.1820866141732285504 ) ) ;
#44651=CARTESIAN_POINT ( 'NONE',  ( 0.9842519685039378130, -0.6692913385826771977, 8.415575281601705876E-17 ) ) ;
#44652=CARTESIAN_POINT ( 'NONE',  ( 0.8333333333333340365, 0.1771653543307087075, -0.09757992244046823083 ) ) ;
#44653=CARTESIAN_POINT ( 'NONE',  ( 0.09842519685039434474, 0.1660481256975885056, 0.3530559997133364547 ) ) ;
#44655=CARTESIAN_POINT ( 'NONE',  ( -0.3346456692913377662, 0.1660481256975883668, -0.3530559997133364547 ) ) ;
#44656=CARTESIAN_POINT ( 'NONE',  ( -1.167979002624671470, -0.3690944881889765550, -0.3153832671262227771 ) ) ;
#44657=CARTESIAN_POINT ( 'NONE',  ( -0.3477690288713905509, -0.6692913385826771977, 0.1292274648535927661 ) ) ;
#44658=CARTESIAN_POINT ( 'NONE',  ( 1.561679790026247350, 0.05413385826771626580, -0.4176697321401330321 ) ) ;
#44662=CARTESIAN_POINT ( 'NONE',  ( 0.6233595800524942554, -0.05778040916215560624, -0.4822834645669293319 ) ) ;
#44664=CARTESIAN_POINT ( 'NONE',  ( -0.6889763779527552368, -0.5400638737290845981, -0.3530559997133363437 ) ) ;
#44665=CARTESIAN_POINT ( 'NONE',  ( 1.469816272965879911, 0.2306618581243847221, -0.2411417322834647770 ) ) ;
#44666=CARTESIAN_POINT ( 'NONE',  ( 0.7152230971128614723, -0.3162353388693409650, -0.4822834645669289433 ) ) ;
#44667=VECTOR ( 'NONE', #11542, 39.37007874015748143 ) ;
#44668=CARTESIAN_POINT ( 'NONE',  ( 0.05905511811023709395, -0.5400638737290844871, 0.3530559997133364547 ) ) ;
#44670=CARTESIAN_POINT ( 'NONE',  ( -0.7086614173228339419, -0.1870078740157480879, -0.4822834645669291653 ) ) ;
#44671=CARTESIAN_POINT ( 'NONE',  ( -0.2493438320209966919, -0.4281496062992124485, 0.4176697321401328655 ) ) ;
#44672=CARTESIAN_POINT ( 'NONE',  ( -0.6627296587926501115, 0.2952755905511810774, -0.1292274648535930714 ) ) ;
#44673=CARTESIAN_POINT ( 'NONE',  ( -0.01968503937007793844, 0.07958543189024071263, -0.2665933059059888421 ) ) ;
#44674=CARTESIAN_POINT ( 'NONE',  ( -0.5944687039322197331, 1.968503937007873850, 0.4915354330708656128 ) ) ;
#44675=CARTESIAN_POINT ( 'NONE',  ( -0.2362204724409442680, -0.1870078740157480879, -0.4822834645669291653 ) ) ;
#44677=CARTESIAN_POINT ( 'NONE',  ( 1.266404199475066328, -0.05778040916215522460, 0.4822834645669289988 ) ) ;
#44678=ORIENTED_EDGE ( 'NONE', *, *, #14066, .F. ) ;
#44680=CARTESIAN_POINT ( 'NONE',  ( 0.4396325459317593221, 0.2952755905511810774, -0.1292274648535930714 ) ) ;
#44681=CARTESIAN_POINT ( 'NONE',  ( -0.4396325459317579898, 0.1771653543307087630, 0.09757992244046791164 ) ) ;
#44682=CARTESIAN_POINT ( 'NONE',  ( 1.561679790026247350, -0.004921259842519870586, -0.3153832671262229437 ) ) ;
#44686=FACE_OUTER_BOUND ( 'NONE', #2064, .T. ) ;
#44687=CARTESIAN_POINT ( 'NONE',  ( 1.541994750656168645, -0.6692913385826771977, 0.1292274648535927661 ) ) ;
#44689=CARTESIAN_POINT ( 'NONE',  ( -0.04593175853018302557, -0.6692913385826773087, -0.1292274648535924053 ) ) ;
#44690=CARTESIAN_POINT ( 'NONE',  ( -1.115485564304461219, 0.05413385826771626580, -0.4176697321401330321 ) ) ;
#44691=CARTESIAN_POINT ( 'NONE',  ( -1.312335958005248715, -0.6046776061558809534, -0.2411417322834644161 ) ) ;
#44692=CARTESIAN_POINT ( 'NONE',  ( 0.4593175853018379162, -0.4281496062992124485, 0.4176697321401328655 ) ) ;
#44694=CARTESIAN_POINT ( 'NONE',  ( 1.692913385826772421, 0.2952755905511811885, 0.000000000000000000 ) ) ;
#44695=CARTESIAN_POINT ( 'NONE',  ( 1.095800524934383846, -0.3162353388693405765, 0.4822834645669290543 ) ) ;
#44696=CARTESIAN_POINT ( 'NONE',  ( 1.272965879265092637, -0.3690944881889765550, -0.3153832671262227771 ) ) ;
#44698=CARTESIAN_POINT ( 'NONE',  ( 0.8858267716535438430, 0.07958543189024085140, 0.2665933059059887866 ) ) ;
#44699=CARTESIAN_POINT ( 'NONE',  ( -1.272965879265091305, 0.05413385826771626580, -0.4176697321401330321 ) ) ;
#44701=CARTESIAN_POINT ( 'NONE',  ( 1.095800524934383846, -0.05778040916215560624, -0.4822834645669293319 ) ) ;
#44704=CARTESIAN_POINT ( 'NONE',  ( 0.7874015748031503170, -0.1870078740157480879, -0.4822834645669291653 ) ) ;
#44706=CARTESIAN_POINT ( 'NONE',  ( -1.502624671916009680, -0.08942795157528024563, -0.3641732283464568787 ) ) ;
#44707=CARTESIAN_POINT ( 'NONE',  ( -0.1115485564304453947, -0.6692913385826771977, 0.1292274648535927661 ) ) ;
#44708=CARTESIAN_POINT ( 'NONE',  ( 0.9973753280839902091, 0.1283753931104746893, -0.1820866141732285504 ) ) ;
#44709=CARTESIAN_POINT ( 'NONE',  ( 1.082677165354331228, 0.1660481256975883668, -0.3530559997133364547 ) ) ;
#44711=CARTESIAN_POINT ( 'NONE',  ( -0.7152230971128602510, -0.08942795157528024563, -0.3641732283464568787 ) ) ;
#44712=CARTESIAN_POINT ( 'NONE',  ( -0.7480314960629914633, 0.2952755905511811885, 0.000000000000000000 ) ) ;
#44713=CARTESIAN_POINT ( 'NONE',  ( -1.574803149606298192, -0.1870078740157480601, -0.3641732283464567677 ) ) ;
#44714=CARTESIAN_POINT ( 'NONE',  ( -1.122047244094487306, -0.5400638737290844871, 0.3530559997133364547 ) ) ;
#44715=CARTESIAN_POINT ( 'NONE',  ( 0.9317585301837276734, 0.05413385826771626580, -0.4176697321401330321 ) ) ;
#44717=CARTESIAN_POINT ( 'NONE',  ( -1.338582677165353729, -0.1870078740157479769, 0.3641732283464567677 ) ) ;
#44719=CARTESIAN_POINT ( 'NONE',  ( 1.049868766404200127, -0.6046776061558809534, -0.2411417322834644161 ) ) ;
#44721=CARTESIAN_POINT ( 'NONE',  ( -1.496062992125983815, -0.1870078740157480879, -0.4822834645669291653 ) ) ;
#44722=CARTESIAN_POINT ( 'NONE',  ( -1.476377952755905110, 0.07958543189024085140, 0.2665933059059887866 ) ) ;
#44723=CARTESIAN_POINT ( 'NONE',  ( -1.207349081364828880, 0.1283753931104746893, -0.1820866141732285504 ) ) ;
#44724=CARTESIAN_POINT ( 'NONE',  ( 1.170004705068746986, -4.479759449472349425E-16, -0.3954985857520055825 ) ) ;
#44725=CARTESIAN_POINT ( 'NONE',  ( -0.4986876640419939388, 0.2306618581243847221, -0.2411417322834647770 ) ) ;
#44726=CARTESIAN_POINT ( 'NONE',  ( -0.2559055118110227234, -0.4536011799217367080, 0.2665933059059888421 ) ) ;
#44727=CARTESIAN_POINT ( 'NONE',  ( -1.515748031496062076, 0.07958543189024071263, -0.2665933059059888421 ) ) ;
#44728=CARTESIAN_POINT ( 'NONE',  ( 1.010498687664042716, -0.004921259842519870586, -0.3153832671262229437 ) ) ;
#44730=CARTESIAN_POINT ( 'NONE',  ( 0.4002624671916016896, -0.05778040916215522460, 0.4822834645669289988 ) ) ;
#44731=CARTESIAN_POINT ( 'NONE',  ( 1.364829396325459854, -0.6046776061558809534, -0.2411417322834644161 ) ) ;
#44732=CARTESIAN_POINT ( 'NONE',  ( -0.1312335958005241554, -0.5023911411419708095, -0.1820866141732282451 ) ) ;
#44733=CARTESIAN_POINT ( 'NONE',  ( 0.5052493438320218022, -0.6692913385826773087, -0.1292274648535924053 ) ) ;
#44734=CARTESIAN_POINT ( 'NONE',  ( 0.4330708661417329575, -0.5511811023622047445, 6.969142054262312111E-17 ) ) ;
#44735=CARTESIAN_POINT ( 'NONE',  ( -1.581364829396324945, -0.05778040916215560624, -0.4822834645669293319 ) ) ;
#44737=CARTESIAN_POINT ( 'NONE',  ( -1.502624671916009680, -0.3162353388693405765, 0.4822834645669290543 ) ) ;
#44738=CARTESIAN_POINT ( 'NONE',  ( -0.6036745406824141069, 0.2306618581243848609, 0.2411417322834645549 ) ) ;
#44741=CARTESIAN_POINT ( 'NONE',  ( 0.2755905511811031494, -0.6692913385826771977, 8.415575281601705876E-17 ) ) ;
#44742=CARTESIAN_POINT ( 'NONE',  ( 1.220472440944882386, -0.5511811023622047445, 6.969142054262312111E-17 ) ) ;
#44743=CARTESIAN_POINT ( 'NONE',  ( -0.5708661417322825615, -0.5400638737290844871, 0.3530559997133364547 ) ) ;
#44744=CARTESIAN_POINT ( 'NONE',  ( 0.3674540682414705883, 0.2306618581243847221, -0.2411417322834647770 ) ) ;
#44750=CARTESIAN_POINT ( 'NONE',  ( -1.062992125984250968, 0.1771653543307087630, 0.000000000000000000 ) ) ;
#44751=CARTESIAN_POINT ( 'NONE',  ( -1.200787401574802349, 0.1660481256975883668, -0.3530559997133364547 ) ) ;
#44753=CARTESIAN_POINT ( 'NONE',  ( 0.8398950131233602345, -0.6046776061558807314, 0.2411417322834647770 ) ) ;
#44754=CARTESIAN_POINT ( 'NONE',  ( 1.450131233595801428, 0.2952755905511811885, 0.1292274648535926551 ) ) ;
#44755=CARTESIAN_POINT ( 'NONE',  ( 0.6430446194225728496, 0.05413385826771666132, 0.4176697321401328100 ) ) ;
#44760=CARTESIAN_POINT ( 'NONE',  ( 0.5643044619422579178, -0.4281496062992127816, -0.4176697321401328100 ) ) ;
#44761=CARTESIAN_POINT ( 'NONE',  ( 0.6102362204724416372, -0.5400638737290844871, 0.3530559997133364547 ) ) ;
#44762=CARTESIAN_POINT ( 'NONE',  ( 0.6692913385826777528, 0.1771653543307087630, 0.000000000000000000 ) ) ;
#44763=CARTESIAN_POINT ( 'NONE',  ( 1.128608923884515169, -0.6046776061558809534, -0.2411417322834644161 ) ) ;
#44765=CARTESIAN_POINT ( 'NONE',  ( 0.5380577427821529035, 0.05413385826771626580, -0.4176697321401330321 ) ) ;
#44766=CARTESIAN_POINT ( 'NONE',  ( 0.9842519685039378130, -0.6692913385826771977, 8.415575281601705876E-17 ) ) ;
#44767=CARTESIAN_POINT ( 'NONE',  ( 0.4133858267716541968, 0.1660481256975885056, 0.3530559997133364547 ) ) ;
#44768=CARTESIAN_POINT ( 'NONE',  ( 1.161417322834646493, -0.4536011799217367080, 0.2665933059059888421 ) ) ;
#44769=CARTESIAN_POINT ( 'NONE',  ( -0.9711286089238838626, -0.6046776061558807314, 0.2411417322834647770 ) ) ;
#44770=CARTESIAN_POINT ( 'NONE',  ( -1.200787401574802349, 0.1660481256975883668, -0.3530559997133364547 ) ) ;
#44771=CARTESIAN_POINT ( 'NONE',  ( 1.122047244094488860, 0.1660481256975885056, 0.3530559997133364547 ) ) ;
#44777=ORIENTED_EDGE ( 'NONE', *, *, #11980, .T. ) ;
#44778=CARTESIAN_POINT ( 'NONE',  ( 1.482939632545932307, -0.4281496062992124485, 0.4176697321401328655 ) ) ;
#44779=CARTESIAN_POINT ( 'NONE',  ( 1.213910761154856299, -0.5511811023622048555, -0.09757992244046775898 ) ) ;
#44781=CARTESIAN_POINT ( 'NONE',  ( 1.437007874015748810, -0.4536011799217368745, -0.2665933059059886201 ) ) ;
#44782=CARTESIAN_POINT ( 'NONE',  ( -0.2462293917967295909, -2.567464376874931580E-15, -0.4445507791589072832 ) ) ;
#44787=CARTESIAN_POINT ( 'NONE',  ( -0.5577427821522301654, -0.2845877964562159024, 0.3641732283464567677 ) ) ;
#44788=CARTESIAN_POINT ( 'NONE',  ( -1.417322834645668772, -0.1870078740157479769, 0.3641732283464567677 ) ) ;
#44789=CARTESIAN_POINT ( 'NONE',  ( -1.076115485564303809, -0.6046776061558809534, -0.2411417322834644161 ) ) ;
#44790=CARTESIAN_POINT ( 'NONE',  ( 0.09842519685039434474, -0.5400638737290845981, -0.3530559997133363437 ) ) ;
#44791=CARTESIAN_POINT ( 'NONE',  ( -1.555118110236219930, -0.5400638737290845981, -0.3530559997133363437 ) ) ;
#44794=LENGTH_MEASURE_WITH_UNIT ( LENGTH_MEASURE( 0.02539999999999999897 ), #70076 );
#44797=CARTESIAN_POINT ( 'NONE',  ( -0.6627296587926501115, 0.1771653543307087075, -0.09757992244046823083 ) ) ;
#44799=CARTESIAN_POINT ( 'NONE',  ( -1.207349081364828436, -0.6046776061558807314, 0.2411417322834647770 ) ) ;
#44800=CARTESIAN_POINT ( 'NONE',  ( 1.128608923884515169, -0.6046776061558809534, -0.2411417322834644161 ) ) ;
#44804=CARTESIAN_POINT ( 'NONE',  ( 1.128608923884515169, -0.6046776061558809534, -0.2411417322834644161 ) ) ;
#44805=CARTESIAN_POINT ( 'NONE',  ( -1.332020997375327642, -0.3162353388693409650, -0.4822834645669289433 ) ) ;
#44807=CARTESIAN_POINT ( 'NONE',  ( -0.2034120734908131112, -0.5511811023622048555, -0.09757992244046775898 ) ) ;
#44809=CARTESIAN_POINT ( 'NONE',  ( -0.4986876640419939388, 0.1283753931104746893, -0.1820866141732285504 ) ) ;
#44810=CARTESIAN_POINT ( 'NONE',  ( -0.01968503937007793844, -0.4536011799217367080, 0.2665933059059888421 ) ) ;
#44811=CARTESIAN_POINT ( 'NONE',  ( -0.07217847769028813698, -0.3162353388693409650, -0.4822834645669289433 ) ) ;
#44812=CARTESIAN_POINT ( 'NONE',  ( -1.325459317585300889, -0.004921259842519576551, 0.3153832671262227771 ) ) ;
#44814=CARTESIAN_POINT ( 'NONE',  ( 1.082677165354331228, -0.5400638737290844871, 0.3530559997133364547 ) ) ;
#44815=CARTESIAN_POINT ( 'NONE',  ( -1.299212598425196097, 0.2952755905511811885, 0.000000000000000000 ) ) ;
#44817=CARTESIAN_POINT ( 'NONE',  ( -0.5052493438320203589, -0.6692913385826771977, 0.1292274648535927661 ) ) ;
#44818=CARTESIAN_POINT ( 'NONE',  ( -0.7808398950131222316, -0.3162353388693409650, -0.4822834645669289433 ) ) ;
#44819=CARTESIAN_POINT ( 'NONE',  ( 1.003937007874016407, -0.4536011799217367080, 0.2665933059059888421 ) ) ;
#44820=CARTESIAN_POINT ( 'NONE',  ( -0.3871391076115479057, -0.2845877964562161244, -0.3641732283464567121 ) ) ;
#44821=CARTESIAN_POINT ( 'NONE',  ( -0.5118110236220466680, -0.6692913385826771977, 8.415575281601705876E-17 ) ) ;
#44822=CARTESIAN_POINT ( 'NONE',  ( -1.207349081364828436, -0.6046776061558807314, 0.2411417322834647770 ) ) ;
#44824=CARTESIAN_POINT ( 'NONE',  ( 1.318897637795276356, -0.4536011799217367080, 0.2665933059059888421 ) ) ;
#44826=CARTESIAN_POINT ( 'NONE',  ( -0.1509186351706028884, -0.3162353388693409650, -0.4822834645669289433 ) ) ;
#44827=CARTESIAN_POINT ( 'NONE',  ( -1.456692913385826182, -0.6692913385826771977, 8.415575281601705876E-17 ) ) ;
#44830=CARTESIAN_POINT ( 'NONE',  ( -0.7808398950131222316, -0.2845877964562161244, -0.3641732283464567121 ) ) ;
#44831=CARTESIAN_POINT ( 'NONE',  ( 0.6233595800524939223, -0.3162353388693405765, 0.4822834645669290543 ) ) ;
#44832=CARTESIAN_POINT ( 'NONE',  ( -0.9908136482939626788, -0.5511811023622048555, -0.09757992244046775898 ) ) ;
#44834=CARTESIAN_POINT ( 'NONE',  ( -1.154855643044618851, -0.6046776061558809534, -0.2411417322834644161 ) ) ;
#44835=CARTESIAN_POINT ( 'NONE',  ( 0.7480314960629927956, 0.2952755905511811885, 0.000000000000000000 ) ) ;
#44836=CARTESIAN_POINT ( 'NONE',  ( 0.3346456692913393205, -0.5400638737290845981, -0.3530559997133363437 ) ) ;
#44837=CARTESIAN_POINT ( 'NONE',  ( 1.437007874015748810, 0.1660481256975885056, 0.3530559997133364547 ) ) ;
#44838=CARTESIAN_POINT ( 'NONE',  ( -1.561679790026246017, -0.004921259842519576551, 0.3153832671262227771 ) ) ;
#44841=AXIS2_PLACEMENT_3D ( 'NONE', #16443, #40852, #66537 ) ;
#44844=CARTESIAN_POINT ( 'NONE',  ( 1.102362204724410155, -0.1870078740157480601, -0.3641732283464567677 ) ) ;
#44845=CARTESIAN_POINT ( 'NONE',  ( 0.8792650918635177559, -0.3690944881889765550, -0.3153832671262227771 ) ) ;
#44846=CARTESIAN_POINT ( 'NONE',  ( 0.2427821522309716595, -0.3162353388693409650, -0.4822834645669289433 ) ) ;
#44849=CARTESIAN_POINT ( 'NONE',  ( 0.3018372703412079971, -0.004921259842519870586, -0.3153832671262229437 ) ) ;
#44850=CARTESIAN_POINT ( 'NONE',  ( -0.8792650918635160906, -0.4281496062992124485, 0.4176697321401328655 ) ) ;
#44851=CARTESIAN_POINT ( 'NONE',  ( -1.351706036745406347, -0.4281496062992124485, 0.4176697321401328655 ) ) ;
#44852=CARTESIAN_POINT ( 'NONE',  ( 0.6889763779527566800, -0.5400638737290844871, 0.3530559997133364547 ) ) ;
#44857=CARTESIAN_POINT ( 'NONE',  ( -1.476377952755905110, -0.5400638737290845981, -0.3530559997133363437 ) ) ;
#44858=CARTESIAN_POINT ( 'NONE',  ( -0.5643044619422565855, -0.4281496062992124485, 0.4176697321401328655 ) ) ;
#44859=CARTESIAN_POINT ( 'NONE',  ( -0.8530183727034112984, -0.004921259842519576551, 0.3153832671262227771 ) ) ;
#44860=CARTESIAN_POINT ( 'NONE',  ( -0.8595800524934373854, -0.05778040916215522460, 0.4822834645669289988 ) ) ;
#44863=CARTESIAN_POINT ( 'NONE',  ( -1.515748031496062076, -0.4536011799217367080, 0.2665933059059888421 ) ) ;
#44864=CARTESIAN_POINT ( 'NONE',  ( -0.8792650918635160906, 0.05413385826771626580, -0.4176697321401330321 ) ) ;
#44865=CARTESIAN_POINT ( 'NONE',  ( 0.3083989501312343062, -0.3162353388693405765, 0.4822834645669290543 ) ) ;
#44867=CARTESIAN_POINT ( 'NONE',  ( -0.8464566929133852113, 0.1660481256975885056, 0.3530559997133364547 ) ) ;
#44870=CARTESIAN_POINT ( 'NONE',  ( -1.003937007874014853, 0.07958543189024085140, 0.2665933059059887866 ) ) ;
#44871=VERTEX_POINT ( 'NONE', #40176 ) ;
#44873=ORIENTED_EDGE ( 'NONE', *, *, #24294, .T. ) ;
#44874=CARTESIAN_POINT ( 'NONE',  ( -1.574803149606298636, -0.1870078740157479769, 0.3641732283464567677 ) ) ;
#44875=CARTESIAN_POINT ( 'NONE',  ( -1.200787401574802349, -0.5400638737290844871, 0.3530559997133364547 ) ) ;
#44876=CARTESIAN_POINT ( 'NONE',  ( -1.089238845144356427, -0.4281496062992127816, -0.4176697321401328100 ) ) ;
#44878=CARTESIAN_POINT ( 'NONE',  ( -1.233595800524933894, 0.2306618581243848609, 0.2411417322834645549 ) ) ;
#44879=CARTESIAN_POINT ( 'NONE',  ( -1.200787401574802349, 0.1660481256975883668, -0.3530559997133364547 ) ) ;
#44882=CARTESIAN_POINT ( 'NONE',  ( 0.5905511811023629321, 0.1771653543307087630, 0.000000000000000000 ) ) ;
#44883=CARTESIAN_POINT ( 'NONE',  ( -0.4824498642376744417, -2.567464376874931580E-15, -0.4445507791589072832 ) ) ;
#44885=CARTESIAN_POINT ( 'NONE',  ( -0.2165354330708654795, -0.4536011799217368745, -0.2665933059059886201 ) ) ;
#44887=CARTESIAN_POINT ( 'NONE',  ( -0.6430446194225712953, 0.05413385826771626580, -0.4176697321401330321 ) ) ;
#44888=CARTESIAN_POINT ( 'NONE',  ( 1.358267716535433323, -0.5400638737290845981, -0.3530559997133363437 ) ) ;
#44889=CARTESIAN_POINT ( 'NONE',  ( -0.5708661417322825615, -0.5400638737290844871, 0.3530559997133364547 ) ) ;
#44890=VERTEX_POINT ( 'NONE', #20404 ) ;
#44891=VERTEX_POINT ( 'NONE', #33860 ) ;
#44893=CARTESIAN_POINT ( 'NONE',  ( -0.9580052493438311334, 0.05413385826771626580, -0.4176697321401330321 ) ) ;
#44894=CARTESIAN_POINT ( 'NONE',  ( 1.154855643044620184, 0.2306618581243847221, -0.2411417322834647770 ) ) ;
#44895=CARTESIAN_POINT ( 'NONE',  ( -1.194225721784776262, -0.004921259842519870586, -0.3153832671262229437 ) ) ;
#44896=CARTESIAN_POINT ( 'NONE',  ( -1.404199475065615932, 0.05413385826771666132, 0.4176697321401328100 ) ) ;
#44901=LINE ( 'NONE', #37785, #41250 ) ;
#44902=CARTESIAN_POINT ( 'NONE',  ( 0.07217847769028949700, -0.3162353388693405765, 0.4822834645669290543 ) ) ;
#44903=CARTESIAN_POINT ( 'NONE',  ( -0.9251968503937002541, -0.4536011799217368745, -0.2665933059059886201 ) ) ;
#44904=CARTESIAN_POINT ( 'NONE',  ( -0.7086614173228339419, -0.1870078740157480879, -0.4822834645669291653 ) ) ;
#44906=CARTESIAN_POINT ( 'NONE',  ( -1.305774278215222184, -0.6692913385826773087, -0.1292274648535924053 ) ) ;
#44907=CARTESIAN_POINT ( 'NONE',  ( -1.174540682414697335, -0.3162353388693409650, -0.4822834645669289433 ) ) ;
#44908=CARTESIAN_POINT ( 'NONE',  ( -0.1181102362204717315, 0.2952755905511811885, 0.000000000000000000 ) ) ;
#44911=CARTESIAN_POINT ( 'NONE',  ( 0.9186351706036751663, -0.5023911411419708095, 0.1820866141732285504 ) ) ;
#44912=CARTESIAN_POINT ( 'NONE',  ( -0.7152230971128602510, -0.08942795157528024563, -0.3641732283464568787 ) ) ;
#44913=CARTESIAN_POINT ( 'NONE',  ( -1.113459889019125182, -4.850200619981615293E-15, -0.3954974714151464621 ) ) ;
#44914=CARTESIAN_POINT ( 'NONE',  ( 0.9317585301837276734, -0.004921259842519870586, -0.3153832671262229437 ) ) ;
#44915=CARTESIAN_POINT ( 'NONE',  ( 1.200787401574803681, -0.4536011799217368745, -0.2665933059059886201 ) ) ;
#44916=CARTESIAN_POINT ( 'NONE',  ( 1.253280839895013710, -0.3162353388693405765, 0.4822834645669290543 ) ) ;
#44917=CARTESIAN_POINT ( 'NONE',  ( 0.5183727034120741983, -0.5511811023622046335, 0.09757992244046803654 ) ) ;
#44919=CARTESIAN_POINT ( 'NONE',  ( -0.8923884514435688198, -0.6046776061558807314, 0.2411417322834647770 ) ) ;
#44920=CARTESIAN_POINT ( 'NONE',  ( 1.167979002624672580, 0.05413385826771626580, -0.4176697321401330321 ) ) ;
#44922=CARTESIAN_POINT ( 'NONE',  ( -0.3346456692913377662, 0.07958543189024071263, -0.2665933059059888421 ) ) ;
#44923=CARTESIAN_POINT ( 'NONE',  ( 0.7186703366786207914, -1.374501131054255944E-15, 0.4445507791589066726 ) ) ;
#44924=CARTESIAN_POINT ( 'NONE',  ( 0.3215223097112867578, -0.3162353388693409650, -0.4822834645669289433 ) ) ;
#44925=CARTESIAN_POINT ( 'NONE',  ( -1.614173228346456712, 2.401574803149606474, -0.1372047244094478091 ) ) ;
#44926=CARTESIAN_POINT ( 'NONE',  ( 0.8727034120734912248, -0.2845877964562161244, -0.3641732283464567121 ) ) ;
#44927=CARTESIAN_POINT ( 'NONE',  ( 0.2887139107611556010, -0.5023911411419708095, 0.1820866141732285504 ) ) ;
#44928=CARTESIAN_POINT ( 'NONE',  ( 0.1574803149606306130, -0.1870078740157480879, -0.4822834645669291653 ) ) ;
#44929=CARTESIAN_POINT ( 'NONE',  ( -1.154855643044618851, -0.6046776061558809534, -0.2411417322834644161 ) ) ;
#44930=CARTESIAN_POINT ( 'NONE',  ( -0.5052493438320203589, 0.1771653543307087075, -0.09757992244046823083 ) ) ;
#44932=CARTESIAN_POINT ( 'NONE',  ( -0.4790026246719152336, -0.05778040916215560624, -0.4822834645669293319 ) ) ;
#44935=CARTESIAN_POINT ( 'NONE',  ( 0.03280839895013198948, 0.1771653543307087630, 0.09757992244046791164 ) ) ;
#44936=CARTESIAN_POINT ( 'NONE',  ( -0.6561679790026240244, 0.2306618581243847221, -0.2411417322834647770 ) ) ;
#44937=CARTESIAN_POINT ( 'NONE',  ( -1.318897637795274802, 0.1660481256975885056, 0.3530559997133364547 ) ) ;
#44938=CARTESIAN_POINT ( 'NONE',  ( -1.213910761154854745, -0.5511811023622046335, 0.09757992244046803654 ) ) ;
#44941=CARTESIAN_POINT ( 'NONE',  ( -0.5577427821522301654, -0.3162353388693405765, 0.4822834645669290543 ) ) ;
#44942=CARTESIAN_POINT ( 'NONE',  ( -0.8661417322834640276, -0.1870078740157479769, 0.3641732283464567677 ) ) ;
#44943=CARTESIAN_POINT ( 'NONE',  ( -1.633858267716534529, -0.4536011799217368745, -0.2665933059059886201 ) ) ;
#44944=CARTESIAN_POINT ( 'NONE',  ( 1.358267716535433323, -0.5400638737290845981, -0.3530559997133363437 ) ) ;
#44947=ORIENTED_EDGE ( 'NONE', *, *, #53708, .F. ) ;
#44950=CARTESIAN_POINT ( 'NONE',  ( -1.279527559055116948, -0.5400638737290844871, 0.3530559997133364547 ) ) ;
#44951=CARTESIAN_POINT ( 'NONE',  ( -0.8333333333333323711, -0.6692913385826773087, -0.1292274648535924053 ) ) ;
#44953=CARTESIAN_POINT ( 'NONE',  ( -1.522309711286088607, -0.6046776061558807314, 0.2411417322834647770 ) ) ;
#44955=CARTESIAN_POINT ( 'NONE',  ( 1.482939632545932307, -0.3690944881889763329, 0.3153832671262228327 ) ) ;
#44956=CARTESIAN_POINT ( 'NONE',  ( 0.4790026246719168435, -0.3162353388693409650, -0.4822834645669289433 ) ) ;
#44957=CARTESIAN_POINT ( 'NONE',  ( 0.1706036745406830368, -0.4281496062992127816, -0.4176697321401328100 ) ) ;
#44958=CARTESIAN_POINT ( 'NONE',  ( -0.3256598226813641195, -3.773335473449285555E-15, -0.4118477457933000796 ) ) ;
#44960=CARTESIAN_POINT ( 'NONE',  ( 0.8727034120734912248, -0.2845877964562161244, -0.3641732283464567121 ) ) ;
#44966=CARTESIAN_POINT ( 'NONE',  ( -0.2034120734908131112, -0.6692913385826773087, -0.1292274648535924053 ) ) ;
#44967=CARTESIAN_POINT ( 'NONE',  ( -0.8202099737532801971, -0.6692913385826771977, 0.1292274648535927661 ) ) ;
#44968=CARTESIAN_POINT ( 'NONE',  ( -1.325459317585300889, 0.05413385826771666132, 0.4176697321401328100 ) ) ;
#44969=CARTESIAN_POINT ( 'NONE',  ( 0.6299212598425204535, -0.1870078740157480879, -0.4822834645669291653 ) ) ;
#44970=CARTESIAN_POINT ( 'NONE',  ( -1.581364829396324945, -0.08942795157528024563, -0.3641732283464568787 ) ) ;
#44971=CARTESIAN_POINT ( 'NONE',  ( 1.568241469816273437, -0.3162353388693405765, 0.4822834645669290543 ) ) ;
#44972=CARTESIAN_POINT ( 'NONE',  ( -0.3740157480314953431, 0.1660481256975885056, 0.3530559997133364547 ) ) ;
#44973=CARTESIAN_POINT ( 'NONE',  ( 0.4855643044619428750, 0.05413385826771666132, 0.4176697321401328100 ) ) ;
#44974=CARTESIAN_POINT ( 'NONE',  ( -1.574803149606298192, -0.1870078740157480879, -0.4822834645669291653 ) ) ;
#44975=CARTESIAN_POINT ( 'NONE',  ( 1.141732283464567566, 0.2952755905511811885, 0.000000000000000000 ) ) ;
#44976=B_SPLINE_CURVE_WITH_KNOTS ( 'NONE', 3,
 ( #49040, #25010, #76381, #18715 ),
 .UNSPECIFIED., .F., .F.,
 ( 4, 4 ),
 ( 3.593986969187450165E-07, 0.001287825409103291428 ),
 .UNSPECIFIED. ) ;
#44977=CARTESIAN_POINT ( 'NONE',  ( 1.627296587926509996, -0.6046776061558807314, 0.2411417322834647770 ) ) ;
#44978=CARTESIAN_POINT ( 'NONE',  ( 0.04593175853018440641, 0.2952755905511810774, -0.1292274648535930714 ) ) ;
#44980=CARTESIAN_POINT ( 'NONE',  ( 0.4724409448818904789, -0.1870078740157480601, -0.3641732283464567677 ) ) ;
#44983=ORIENTED_EDGE ( 'NONE', *, *, #69760, .F. ) ;
#44984=CARTESIAN_POINT ( 'NONE',  ( -0.2427821522309703550, -0.08942795157528024563, -0.3641732283464568787 ) ) ;
#44986=CARTESIAN_POINT ( 'NONE',  ( 0.2821522309711292364, -0.6692913385826771977, 0.1292274648535927661 ) ) ;
#44987=CARTESIAN_POINT ( 'NONE',  ( 0.07874015748031558404, -0.1870078740157480879, -0.4822834645669291653 ) ) ;
#44988=CARTESIAN_POINT ( 'NONE',  ( -0.8661417322834640276, -0.1870078740157480879, -0.4822834645669291653 ) ) ;
#44990=CARTESIAN_POINT ( 'NONE',  ( -1.266404199475064773, -0.05778040916215560624, -0.4822834645669293319 ) ) ;
#44992=CARTESIAN_POINT ( 'NONE',  ( 0.8989501312335963501, -0.5511811023622048555, -0.09757992244046775898 ) ) ;
#44993=CARTESIAN_POINT ( 'NONE',  ( 0.4527559055118117182, 0.1660481256975883668, -0.3530559997133364547 ) ) ;
#44994=CARTESIAN_POINT ( 'NONE',  ( 0.8792650918635177559, 0.05413385826771666132, 0.4176697321401328100 ) ) ;
#44996=CARTESIAN_POINT ( 'NONE',  ( -1.561679790026246017, 0.05413385826771666132, 0.4176697321401328100 ) ) ;
#44999=CARTESIAN_POINT ( 'NONE',  ( -0.1377952755905504645, 0.1660481256975885056, 0.3530559997133364547 ) ) ;
#45002=CARTESIAN_POINT ( 'NONE',  ( -1.227034120734907141, -0.5511811023622048555, -0.09757992244046775898 ) ) ;
#45003=CARTESIAN_POINT ( 'NONE',  ( 1.220472440944882386, -0.6692913385826771977, 8.415575281601705876E-17 ) ) ;
#45004=CARTESIAN_POINT ( 'NONE',  ( 1.227034120734908917, 0.2952755905511810774, -0.1292274648535930714 ) ) ;
#45005=CARTESIAN_POINT ( 'NONE',  ( 0.006561679790026889343, -0.2845877964562161244, -0.3641732283464567121 ) ) ;
#45006=CARTESIAN_POINT ( 'NONE',  ( 0.4921259842519691285, 0.1660481256975885056, 0.3530559997133364547 ) ) ;
#45008=CARTESIAN_POINT ( 'NONE',  ( 0.4986876640419954376, -0.5023911411419708095, -0.1820866141732282451 ) ) ;
#45009=CARTESIAN_POINT ( 'NONE',  ( 0.2427821522309716595, -0.3162353388693409650, -0.4822834645669289433 ) ) ;
#45011=CARTESIAN_POINT ( 'NONE',  ( -1.351706036745406347, 0.05413385826771626580, -0.4176697321401330321 ) ) ;
#45012=CARTESIAN_POINT ( 'NONE',  ( -1.128608923884513837, 0.2306618581243847221, -0.2411417322834647770 ) ) ;
#45013=CARTESIAN_POINT ( 'NONE',  ( 0.7217847769028878924, -0.3690944881889765550, -0.3153832671262227771 ) ) ;
#45014=DIRECTION ( 'NONE',  ( -1.000000000000000000, -0.000000000000000000, -0.000000000000000000 ) ) ;
#45015=CARTESIAN_POINT ( 'NONE',  ( -0.2099737532808391705, -0.6046776061558809534, -0.2411417322834644161 ) ) ;
#45016=CARTESIAN_POINT ( 'NONE',  ( -0.1377952755905504645, -0.4536011799217368745, -0.2665933059059886201 ) ) ;
#45018=CARTESIAN_POINT ( 'NONE',  ( -0.2755905511811018171, 0.2952755905511811885, 0.000000000000000000 ) ) ;
#45019=CARTESIAN_POINT ( 'NONE',  ( 0.1312335958005255154, -0.5023911411419708095, 0.1820866141732285504 ) ) ;
#45021=CARTESIAN_POINT ( 'NONE',  ( 0.1181102362204730916, 0.2952755905511811885, 0.000000000000000000 ) ) ;
#45023=CARTESIAN_POINT ( 'NONE',  ( 1.141732283464567788, -0.5511811023622047445, 6.969142054262312111E-17 ) ) ;
#45024=CARTESIAN_POINT ( 'NONE',  ( 0.4843739873036773669, 1.677687439461655404E-16, 0.3627985898453510716 ) ) ;
#45025=CARTESIAN_POINT ( 'NONE',  ( -0.9645669291338575535, -0.4536011799217367080, 0.2665933059059888421 ) ) ;
#45028=CARTESIAN_POINT ( 'NONE',  ( -0.6824146981627291497, -0.5023911411419708095, -0.1820866141732282451 ) ) ;
#45029=CARTESIAN_POINT ( 'NONE',  ( -0.5380577427821514602, 0.05413385826771666132, 0.4176697321401328100 ) ) ;
#45030=CARTESIAN_POINT ( 'NONE',  ( -0.1706036745406816491, -0.4281496062992124485, 0.4176697321401328655 ) ) ;
#45031=CARTESIAN_POINT ( 'NONE',  ( 0.6496062992125991586, -0.4536011799217368745, -0.2665933059059886201 ) ) ;
#45033=CARTESIAN_POINT ( 'NONE',  ( 0.9645669291338588858, 0.07958543189024085140, 0.2665933059059887866 ) ) ;
#45035=CARTESIAN_POINT ( 'NONE',  ( 0.8464566929133866546, -0.5400638737290844871, 0.3530559997133364547 ) ) ;
#45037=CARTESIAN_POINT ( 'NONE',  ( -0.3083989501312330295, -0.05778040916215522460, 0.4822834645669289988 ) ) ;
#45039=CARTESIAN_POINT ( 'NONE',  ( 1.555118110236221041, -0.4536011799217367080, 0.2665933059059888421 ) ) ;
#45040=CARTESIAN_POINT ( 'NONE',  ( 1.017060367454068803, -0.3162353388693405765, 0.4822834645669290543 ) ) ;
#45041=CARTESIAN_POINT ( 'NONE',  ( -0.05905511811023545637, 0.1660481256975885056, 0.3530559997133364547 ) ) ;
#45042=CARTESIAN_POINT ( 'NONE',  ( -1.586688153636163001, 2.388437996263389707, -0.1275903502784763444 ) ) ;
#45043=CARTESIAN_POINT ( 'NONE',  ( 0.3543307086614181922, -0.5511811023622047445, 6.969142054262312111E-17 ) ) ;
#45044=CARTESIAN_POINT ( 'NONE',  ( 0.9120734908136490793, 0.2952755905511810774, -0.1292274648535930714 ) ) ;
#45045=CARTESIAN_POINT ( 'NONE',  ( -0.3477690288713905509, -0.5511811023622046335, 0.09757992244046803654 ) ) ;
#45046=CARTESIAN_POINT ( 'NONE',  ( -0.9120734908136475250, -0.6692913385826773087, -0.1292274648535924053 ) ) ;
#45048=CARTESIAN_POINT ( 'NONE',  ( 0.4527559055118117182, -0.5400638737290844871, 0.3530559997133364547 ) ) ;
#45049=CARTESIAN_POINT ( 'NONE',  ( -1.082677165354329896, -0.5400638737290845981, -0.3530559997133363437 ) ) ;
#45050=CARTESIAN_POINT ( 'NONE',  ( -0.6430446194225716283, -0.3690944881889763329, 0.3153832671262228327 ) ) ;
#45051=CARTESIAN_POINT ( 'NONE',  ( 0.4921259842519691285, 0.1660481256975885056, 0.3530559997133364547 ) ) ;
#45052=CARTESIAN_POINT ( 'NONE',  ( -1.272965879265091305, -0.4281496062992124485, 0.4176697321401328655 ) ) ;
#45053=CARTESIAN_POINT ( 'NONE',  ( -0.3280839895013117347, 0.05413385826771626580, -0.4176697321401330321 ) ) ;
#45054=CARTESIAN_POINT ( 'NONE',  ( 1.135170603674541256, 0.2066929133858267931, 0.1054918080437490802 ) ) ;
#45056=CARTESIAN_POINT ( 'NONE',  ( 1.358267716535433323, -0.5400638737290845981, -0.3530559997133363437 ) ) ;
#45057=CARTESIAN_POINT ( 'NONE',  ( 1.227034120734908917, 0.2952755905511810774, -0.1292274648535930714 ) ) ;
#45059=CARTESIAN_POINT ( 'NONE',  ( -1.456692913385826182, 0.2952755905511811885, 0.000000000000000000 ) ) ;
#45060=CARTESIAN_POINT ( 'NONE',  ( -1.030183727034119867, -0.05778040916215560624, -0.4822834645669293319 ) ) ;
#45064=CARTESIAN_POINT ( 'NONE',  ( 0.1115485564304470323, 0.1771653543307087630, 0.09757992244046791164 ) ) ;
#45067=CARTESIAN_POINT ( 'NONE',  ( 0.4265091863517067039, -0.6692913385826773087, -0.1292274648535924053 ) ) ;
#45068=CARTESIAN_POINT ( 'NONE',  ( 0.4921259842519691285, 0.1660481256975885056, 0.3530559997133364547 ) ) ;
#45071=CARTESIAN_POINT ( 'NONE',  ( -0.4658792650918627265, -0.2845877964562161244, -0.3641732283464567121 ) ) ;
#45073=CARTESIAN_POINT ( 'NONE',  ( 0.8792650918635177559, 0.05413385826771666132, 0.4176697321401328100 ) ) ;
#45074=CARTESIAN_POINT ( 'NONE',  ( 1.003937007874016185, 0.07958543189024071263, -0.2665933059059888421 ) ) ;
#45075=CARTESIAN_POINT ( 'NONE',  ( -0.5774278215223089816, -0.6046776061558807314, 0.2411417322834647770 ) ) ;
#45077=CARTESIAN_POINT ( 'NONE',  ( -0.6758530183727028406, 0.2952755905511811885, 0.1292274648535926551 ) ) ;
#45078=CARTESIAN_POINT ( 'NONE',  ( -1.181102362204723644, -0.1870078740157480601, -0.3641732283464567677 ) ) ;
#45079=CARTESIAN_POINT ( 'NONE',  ( -0.6496062992125976043, -0.5400638737290844871, 0.3530559997133364547 ) ) ;
#45081=ORIENTED_EDGE ( 'NONE', *, *, #17343, .F. ) ;
#45083=CARTESIAN_POINT ( 'NONE',  ( -0.1640419947506553400, -0.05778040916215560624, -0.4822834645669293319 ) ) ;
#45085=CARTESIAN_POINT ( 'NONE',  ( -0.7086614173228339419, -0.1870078740157480879, -0.4822834645669291653 ) ) ;
#45086=CARTESIAN_POINT ( 'NONE',  ( 1.345144356955381593, -0.3162353388693409650, -0.4822834645669289433 ) ) ;
#45087=CARTESIAN_POINT ( 'NONE',  ( 1.338582677165355062, -0.1870078740157480879, -0.4822834645669291653 ) ) ;
#45088=CARTESIAN_POINT ( 'NONE',  ( 0.6561679790026253567, 0.2306618581243848609, 0.2411417322834645549 ) ) ;
#45089=CARTESIAN_POINT ( 'NONE',  ( 0.1246719160104994284, 0.2952755905511810774, -0.1292274648535930714 ) ) ;
#45091=CARTESIAN_POINT ( 'NONE',  ( -1.404199475065615932, 0.05413385826771666132, 0.4176697321401328100 ) ) ;
#45092=CARTESIAN_POINT ( 'NONE',  ( 0.01968503937007957949, -0.5400638737290845981, -0.3530559997133363437 ) ) ;
#45093=CARTESIAN_POINT ( 'NONE',  ( 0.05249343832021075018, -0.5023911411419708095, 0.1820866141732285504 ) ) ;
#45095=CARTESIAN_POINT ( 'NONE',  ( -0.2165354330708654795, -0.5400638737290845981, -0.3530559997133363437 ) ) ;
#45096=CARTESIAN_POINT ( 'NONE',  ( 0.2887139107611556010, 0.1539470093639521697, -0.1968503937007875793 ) ) ;
#45098=CARTESIAN_POINT ( 'NONE',  ( 0.9317585301837276734, -0.4281496062992124485, 0.4176697321401328655 ) ) ;
#45101=ORIENTED_EDGE ( 'NONE', *, *, #72340, .F. ) ;
#45102=CARTESIAN_POINT ( 'NONE',  ( 0.2559055118110243332, 0.1660481256975885056, 0.3530559997133364547 ) ) ;
#45103=CARTESIAN_POINT ( 'NONE',  ( -0.4724409448818890911, -0.1870078740157479769, 0.3641732283464567677 ) ) ;
#45104=CARTESIAN_POINT ( 'NONE',  ( 1.312335958005250269, -0.5023911411419708095, 0.1820866141732285504 ) ) ;
#45108=CARTESIAN_POINT ( 'NONE',  ( 1.397637795275591177, 0.07958543189024071263, -0.2665933059059888421 ) ) ;
#45109=CARTESIAN_POINT ( 'NONE',  ( -1.489501312335957062, -0.05778040916215522460, 0.4822834645669289988 ) ) ;
#45111=CARTESIAN_POINT ( 'NONE',  ( 0.1640419947506569498, -0.05778040916215522460, 0.4822834645669289988 ) ) ;
#45112=CARTESIAN_POINT ( 'NONE',  ( -1.194225721784776262, -0.4281496062992124485, 0.4176697321401328655 ) ) ;
#45113=CARTESIAN_POINT ( 'NONE',  ( 1.601049868766404982, 0.1283753931104748280, 0.1820866141732283561 ) ) ;
#45114=CARTESIAN_POINT ( 'NONE',  ( 0.2624671916010504757, -0.6046776061558809534, -0.2411417322834644161 ) ) ;
#45116=CARTESIAN_POINT ( 'NONE',  ( 1.587926509186352586, -0.4281496062992127816, -0.4176697321401328100 ) ) ;
#45117=CARTESIAN_POINT ( 'NONE',  ( 1.010498687664042716, 0.05413385826771626580, -0.4176697321401330321 ) ) ;
#45118=CARTESIAN_POINT ( 'NONE',  ( 0.9448818897637802916, -0.1870078740157480601, -0.3641732283464567677 ) ) ;
#45119=CARTESIAN_POINT ( 'NONE',  ( 0.8398950131233602345, 0.1539470093639521697, -0.1968503937007875793 ) ) ;
#45120=CARTESIAN_POINT ( 'NONE',  ( 0.9317585301837276734, -0.004921259842519870586, -0.3153832671262229437 ) ) ;
#45121=CARTESIAN_POINT ( 'NONE',  ( -1.161417322834644716, 0.1660481256975885056, 0.3530559997133364547 ) ) ;
#45123=CARTESIAN_POINT ( 'NONE',  ( 1.023622047244095334, -0.1870078740157479769, 0.4822834645669291653 ) ) ;
#45127=CARTESIAN_POINT ( 'NONE',  ( 0.7677165354330716118, 0.1660481256975883668, -0.3530559997133364547 ) ) ;
#45129=CARTESIAN_POINT ( 'NONE',  ( -1.614173228346457378, 1.055049524192299693, -0.1372047244094477536 ) ) ;
#45130=CARTESIAN_POINT ( 'NONE',  ( -0.06561679790026180015, 0.05413385826771666132, 0.4176697321401328100 ) ) ;
#45131=CARTESIAN_POINT ( 'NONE',  ( 0.6299212598425204535, -0.1870078740157479769, 0.3641732283464567677 ) ) ;
#45132=EDGE_CURVE ( 'NONE', #73526, #81026, #53357, .T. ) ;
#45133=CARTESIAN_POINT ( 'NONE',  ( 0.3543307086614181922, -0.6692913385826771977, 8.415575281601705876E-17 ) ) ;
#45135=CARTESIAN_POINT ( 'NONE',  ( -0.8202099737532801971, -0.5511811023622046335, 0.09757992244046803654 ) ) ;
#45136=CARTESIAN_POINT ( 'NONE',  ( -0.6955380577427815458, -0.4281496062992127816, -0.4176697321401328100 ) ) ;
#45137=CARTESIAN_POINT ( 'NONE',  ( 1.679790026246720025, 0.2306618581243848609, 0.2411417322834645549 ) ) ;
#45138=CARTESIAN_POINT ( 'NONE',  ( -1.213910761154854745, 0.2952755905511810774, -0.1292274648535930714 ) ) ;
#45139=CARTESIAN_POINT ( 'NONE',  ( 0.8727034120734913358, -0.05778040916215522460, 0.4822834645669289988 ) ) ;
#45140=CARTESIAN_POINT ( 'NONE',  ( -1.391076115485563314, -0.5023911411419708095, -0.1820866141732282451 ) ) ;
#45142=CARTESIAN_POINT ( 'NONE',  ( 0.9711286089238851948, 0.2306618581243848609, 0.2411417322834645549 ) ) ;
#45145=CARTESIAN_POINT ( 'NONE',  ( -1.666666666666665853, 0.05413385826771626580, -0.4176697321401330321 ) ) ;
#45146=CARTESIAN_POINT ( 'NONE',  ( -1.620734908136482577, 0.1771653543307087630, 0.09757992244046791164 ) ) ;
#45147=CARTESIAN_POINT ( 'NONE',  ( -1.076115485564303809, 0.1283753931104748280, 0.1820866141732283561 ) ) ;
#45149=CARTESIAN_POINT ( 'NONE',  ( -0.2624671916010490880, -0.6046776061558807314, 0.2411417322834647770 ) ) ;
#45150=CARTESIAN_POINT ( 'NONE',  ( -0.2887139107611542133, -0.5023911411419708095, -0.1820866141732282451 ) ) ;
#45151=CARTESIAN_POINT ( 'NONE',  ( -1.646981627296586703, -0.2845877964562161244, -0.3641732283464567121 ) ) ;
#45152=CARTESIAN_POINT ( 'NONE',  ( 0.7939632545931766261, -0.08942795157527998196, 0.3641732283464567121 ) ) ;
#45153=CARTESIAN_POINT ( 'NONE',  ( 0.5577427821522316087, -0.05778040916215522460, 0.4822834645669289988 ) ) ;
#45154=CARTESIAN_POINT ( 'NONE',  ( 1.325459317585302665, 0.05413385826771626580, -0.4176697321401330321 ) ) ;
#45155=CARTESIAN_POINT ( 'NONE',  ( 0.5577427821522316087, -0.05778040916215522460, 0.4822834645669289988 ) ) ;
#45156=CARTESIAN_POINT ( 'NONE',  ( 0.7086614173228352742, -0.1870078740157480601, -0.3641732283464567677 ) ) ;
#45157=CARTESIAN_POINT ( 'NONE',  ( -1.587926509186350810, 0.05413385826771626580, -0.4176697321401330321 ) ) ;
#45158=CARTESIAN_POINT ( 'NONE',  ( -1.161417322834644716, 0.1660481256975885056, 0.3530559997133364547 ) ) ;
#45159=CARTESIAN_POINT ( 'NONE',  ( -0.5511811023622041894, -0.1870078740157480879, -0.4822834645669291653 ) ) ;
#45162=CARTESIAN_POINT ( 'NONE',  ( -0.06561679790026180015, -0.4281496062992127816, -0.4176697321401328100 ) ) ;
#45163=CARTESIAN_POINT ( 'NONE',  ( 1.148293963254593653, 0.1771653543307087075, -0.09757992244046823083 ) ) ;
#45164=CARTESIAN_POINT ( 'NONE',  ( -0.2099737532808391705, 0.2306618581243848609, 0.2411417322834645549 ) ) ;
#45165=CARTESIAN_POINT ( 'NONE',  ( 0.5643044619422579178, -0.4281496062992127816, -0.4176697321401328100 ) ) ;
#45169=CARTESIAN_POINT ( 'NONE',  ( -1.614173228346457378, 0.7794589730111968207, -0.1372047244094477536 ) ) ;
#45171=CARTESIAN_POINT ( 'NONE',  ( -0.9186351706036736120, 0.1283753931104748280, 0.1820866141732283561 ) ) ;
#45172=CARTESIAN_POINT ( 'NONE',  ( -1.338582677165353729, -0.1870078740157480879, -0.4822834645669291653 ) ) ;
#45174=CARTESIAN_POINT ( 'NONE',  ( 0.2755905511811031494, 0.2952755905511811885, 0.000000000000000000 ) ) ;
#45175=CARTESIAN_POINT ( 'NONE',  ( 1.364829396325459854, -0.6046776061558809534, -0.2411417322834644161 ) ) ;
#45176=CARTESIAN_POINT ( 'NONE',  ( 0.9186351706036751663, -0.6046776061558807314, 0.2411417322834647770 ) ) ;
#45178=AXIS2_PLACEMENT_3D ( 'NONE', #46897, #59533, #47729 ) ;
#45183=AXIS2_PLACEMENT_3D ( 'NONE', #62497, #4832, #31322 ) ;
#45184=CARTESIAN_POINT ( 'NONE',  ( 0.5577427821522314977, -0.3162353388693409650, -0.4822834645669289433 ) ) ;
#45185=CARTESIAN_POINT ( 'NONE',  ( 0.3346456692913390985, 0.1660481256975885056, 0.3530559997133364547 ) ) ;
#45186=CARTESIAN_POINT ( 'NONE',  ( 0.6955380577427828781, -0.004921259842519870586, -0.3153832671262229437 ) ) ;
#45187=CARTESIAN_POINT ( 'NONE',  ( 1.476377952755906442, -0.5400638737290844871, 0.3530559997133364547 ) ) ;
#45189=CARTESIAN_POINT ( 'NONE',  ( 0.3871391076115492380, -0.05778040916215560624, -0.4822834645669293319 ) ) ;
#45190=CARTESIAN_POINT ( 'NONE',  ( 1.049868766404200349, 0.2306618581243848609, 0.2411417322834645549 ) ) ;
#45191=CARTESIAN_POINT ( 'NONE',  ( 0.4527559055118117182, 0.1660481256975883668, -0.3530559997133364547 ) ) ;
#45192=CARTESIAN_POINT ( 'NONE',  ( 1.043307086614173818, 0.07958543189024085140, 0.2665933059059887866 ) ) ;
#45193=CARTESIAN_POINT ( 'NONE',  ( -0.8595800524934373854, -0.3162353388693409650, -0.4822834645669289433 ) ) ;
#45194=CARTESIAN_POINT ( 'NONE',  ( -0.8989501312335946848, 0.2952755905511810774, -0.1292274648535930714 ) ) ;
#45195=CARTESIAN_POINT ( 'NONE',  ( 1.161417322834646271, 0.1660481256975883668, -0.3530559997133364547 ) ) ;
#45198=( BOUNDED_SURFACE ( )  B_SPLINE_SURFACE ( 1, 2, ( 
 ( #54605, #10427, #36085, #3689, #29354, #55836, #75223, #30173, #74818, #81132, #15922, #80722, #41976, #42796, #61756, #17163, #4093, #36907, #79897, #68896, #62583, #22216, #67670, #67259, #29762, #60925, #36490, #47872, #23863, #73576, #48290, #68491, #9592, #55424, #10830, #55013, #10006, #62166, #3275, #81545, #80314, #22629, #16333, #35671, #61335, #49530, #23036, #48702, #70970, #76047, #50761, #69725, #5736, #31826, #76462, #25088, #6152, #24268, #83180, #63813, #18788, #31408, #69316, #12897, #24682, #63401, #57072, #12477, #50349, #75639, #17978, #45275, #57901, #18391, #82766, #64651, #57487, #44432, #11667, #70126, #43615, #25501, #37325, #44033, #38140, #77282, #19195, #51166, #6571, #76863, #44844, #5336, #70541, #19612, #62997, #37727, #38556, #64236, #32242, #267, #49941, #82363, #51580, #12070, #25922, #13315, #30994, #38968, #30593, #56259, #81955, #56662, #33083, #52418, #54402, #78127, #3488, #58750, #22015, #77708, #39815, #6989, #58324, #32657, #67466, #65075, #42190, #29154, #2666, #28741, #686, #66643, #26342, #79698, #47675, #73370, #61136, #1112, #41773, #26763, #60725, #28325, #41375, #80114, #9800, #71386, #53986, #54823, #7413, #8980, #80527, #52003, #34653, #67056, #60317, #20461, #20038, #71808, #73791, #46114, #13735, #3075, #22839, #48091, #9389, #15719, #35472, #48498, #74199, #35059, #22432, #14159, #16127, #16545, #45689, #39391, #82568, #81344, #24483, #11875, #69111, #23247, #18594, #18188, #81761, #75031, #49740, #37527, #24071, #11459, #56052, #29970, #10639, #43821, #75440, #62801, #68303, #10223, #74618, #55635, #50149, #75846, #31207, #29563, #23659, #43006, #48917, #69525, #5135, #16962, #4307, #42601, #36294, #17779, #63202, #5542, #61560, #43412, #3903, #37117, #61968, #56874, #49329, #17376, #68700, #30800, #56465, #11041, #36699, #62374, #24887, #50556, #55225, #4712, #76259, #30386, #67885, #35890, #82167, #80932, #482, #45064, #70767, #57283, #57700, #912, #71602, #45488, #82980, #78346, #77925, #58116, #51376, #26138, #13954, #51799, #71185, #32454, #6369, #70340, #20256, #77504, #39183, #44644, #69926, #50965, #32041, #26569, #52222, #7640, #5952, #62, #19413, #25299, #45905, #64867, #76662, #64029, #18995, #12695, #19839, #39612, #65301, #37938, #13527, #63615, #7206, #38354, #33310, #25716, #77080, #13117, #32877, #58546, #38769, #64446, #6782, #58972, #1328, #31621, #26977, #52642, #44237, #12282, #67373, #27816, #54304, #60218, #21502, #47160, #33717, #16034, #72442, #34552, #8056, #53476, #20677, #72023, #46330, #80016, #78766, #54727, #41680, #15200, #41277, #14379, #79186, #40037, #8876, #2568, #28227, #73694, #46749, #22334, #14791, #73271, #40859, #53886, #66963, #47995, #1737, #66543, #9707, #21090, #72852, #35378, #65723, #79600, #21916, #47577, #40448, #59379, #2149, #2980, #66127, #27393, #15620, #61042, #60629, #9296, #34966, #3393, #29056, #53054, #28645, #8464, #34133, #59795, #23560, #36198, #42093, #5039, #68204, #74934, #69010, #49231, #10942, #17279, #48818, #55126, #75335, #42907, #62277, #29468, #22742, #35791, #74517, #23975, #49643, #62700, #16448, #16865, #61868, #68602, #3806, #30286, #37019, #36599, #56371, #4614, #55952, #4209, #42502, #81665, #30708, #17682, #24383, #67789, #74102, #10126, #10541, #43312, #80836, #55535, #82070, #29873, #81244, #11361, #80432, #48402, #61458, #23149, #47848, #65986, #41546, #22192, #34830, #47434, #27670, #54579, #66399, #21772, #15478, #54160, #8737, #33990, #59652, #3667, #16308, #60075, #73127, #23012, #73554, #41134, #53337, #60489, #2008, #67235, #79046, #34407, #79874, #35649, #60900, #2839, #48265, #66825, #9157, #47018, #28502, #61311, #21364, #79453, #80291, #22605, #15898, #9566, #8324, #40714, #9981, #2430, #35236, #3252, #72711, #73962, #28914, #41952, #67646, #15058, #28087, #53744, #29330, #54991, #80699, #72303, #14649, #40306, #57922, #39835, #32677, #44863, #72247, #70990, #14177, #1541, #58768, #12918, #8269, #7855, #71406, #32261, #38575, #45710, #33102, #286, #77303, #25942, #46549, #27196, #70563, #19633, #14596 ),
 ( #64256, #40249, #52860, #45294, #58344, #57508, #7432, #26362, #6590, #20057, #51600, #52437, #13334, #38987, #65094, #20896, #46133, #13754, #33521, #705, #52022, #64670, #77728, #65932, #7009, #39411, #65524, #59184, #1131, #78147, #51186, #26781, #78570, #20479, #71827, #83199, #25521, #76885, #19215, #80239, #60846, #40661, #60020, #79398, #22555, #21717, #41082, #61259, #42309, #15421, #2787, #34777, #3198, #16253, #29279, #59599, #41900, #47796, #8684, #79822, #73500, #66771, #9104, #35596, #54943, #9925, #28862, #54524, #78989, #60436, #47381, #48217, #54106, #73913, #22138, #74323, #33934, #80649, #22962, #16670, #73072, #21309, #41497, #15004, #67594, #67182, #34354, #3613, #48628, #68007, #1954, #9512, #35185, #28447, #15848, #27616, #53279, #46962, #72654, #66346, #2375, #28032, #53690, #55762, #36419, #43954, #75564, #5257, #10759, #36012, #17086, #81469, #75972, #18312, #56995, #55351, #23786, #68825, #17904, #49864, #23373, #81883, #30100, #42723, #74738, #24194, #69650, #63325, #4024, #43541, #29688, #69240, #62092, #11994, #75152, #68419, #49041, #11588, #37248, #4433, #49457, #17497, #82692, #5663, #81057, #43127, #50684, #11171, #37648, #25011, #36832, #31330, #62923, #62505, #4843, #30518, #76382, #56180, #30921, #56587, #82288, #10352, #61683, #24606, #18716, #50274, #44357, #65429, #64572, #7331, #20796, #19534, #6076, #58243, #26265, #609, #39733, #12821, #20379, #38478, #39308, #6909, #19963, #32999, #46031, #51089, #32581, #33428, #70464, #45191, #7762, #70048, #70894, #45614, #13244, #44767, #12403, #51500, #52343, #6495, #76786, #64995, #59089, #26688, #71308, #51926, #71725, #14081, #1444, #38893, #27101, #78050, #64162, #52763, #77631, #57412, #78471, #188, #38060, #63737, #13655, #25424, #31750, #83105, #58669, #77205, #1034, #19118, #32165, #57821, #25841, #22459, #21621, #40987, #21210, #47281, #35497, #27518, #53594, #54428, #28765, #73394, #67081, #40154, #14906, #67491, #66247, #79722, #60749, #53174, #80138, #9006, #9413, #15745, #78889, #72559, #8585, #35083, #34257, #79303, #73816, #54849, #27936, #15322, #72971, #41399, #48118, #41800, #72145, #16153, #60341, #46865, #34678, #2689, #66667, #28349, #9827, #61162, #3513, #3101, #29182, #8171, #54010, #59918, #80553, #22039, #46452, #47699, #14501, #65838, #33836, #59503, #1856, #2273, #40566, #30414, #3930, #5163, #56082, #80959, #69137, #43851, #49767, #63230, #81787, #24098, #81371, #61995, #62402, #11902, #56492, #56902, #67912, #42216, #61585, #29998, #24511, #23274, #17402, #5570, #68327, #43032, #4332, #23684, #75467, #68727, #11068, #17806, #16571, #43440, #11489, #36726, #49358, #29589, #30827, #16987, #55661, #75055, #4741, #42630, #10248, #35919, #37556, #50178, #10665, #37143, #22865, #62828, #82194, #55252, #75873, #48943, #18216, #74645, #36320, #69554, #31235, #48526, #74226, #44672, #7558, #27736, #8798, #65219, #52559, #1252, #27316, #66050, #79108, #24915, #8387, #14299, #57309, #46251, #39960, #33229, #58892, #2070, #21427, #59715, #52975, #78689, #44264, #26900, #70367, #72366, #20599, #21012, #71947, #40777, #82596, #47081, #72772, #66462, #13872, #69955, #7976, #63642, #34052, #33640, #83007, #46672, #15123, #14714, #34474, #59302, #1659, #78268, #39531, #65646, #50583, #53401, #76290, #12309, #18621, #37966, #40369, #5980, #25328, #31651, #50992, #76690, #19024, #15958, #35298, #61377, #80352, #54642, #35707, #53806, #29390, #10043, #22665, #60960, #15540, #42421, #54222, #9627, #3310, #42013, #79938, #21834, #47497, #74857, #4132, #47911, #28975, #10866, #3726, #48324, #41199, #74021, #73189, #55050, #66887, #22253, #67707, #23483, #48739, #16367, #36119, #80757, #23071, #34890, #74436, #49150, #9217, #67294, #68121, #10466, #16783, #61792, #79519, #28566, #81167, #73616, #29797, #55458, #60551, #17199, #42832, #68525, #60140, #2902, #41605, #2491, #28150, #62202, #18823, #50384, #11283, #82398, #76082, #69351, #11705, #38175, #57525, #12514, #5774, #63438, #81584, #63032, #24306, #25125, #56699, #31443, #24716, #76900, #36527, #83216, #25537 ) ),
 .UNSPECIFIED., .F., .F., .F. ) 
 B_SPLINE_SURFACE_WITH_KNOTS ( ( 2, 2 ),
 ( 3, 2, 2, 2, 2, 2, 2, 2, 2, 2, 2, 2, 2, 2, 2, 2, 2, 2, 2, 2, 2, 2, 2, 2, 2, 2, 2, 2, 2, 2, 2, 2, 2, 2, 2, 2, 2, 2, 2, 2, 2, 2, 2, 2, 2, 2, 2, 2, 2, 2, 2, 2, 2, 2, 2, 2, 2, 2, 2, 2, 2, 2, 2, 2, 2, 2, 2, 2, 2, 2, 2, 2, 2, 2, 2, 2, 2, 2, 2, 2, 2, 2, 2, 2, 2, 2, 2, 2, 2, 2, 2, 2, 2, 2, 2, 2, 2, 2, 2, 2, 2, 2, 2, 2, 2, 2, 2, 2, 2, 2, 2, 2, 2, 2, 2, 2, 2, 2, 2, 2, 2, 2, 2, 2, 2, 2, 2, 2, 2, 2, 2, 2, 2, 2, 2, 2, 2, 2, 2, 2, 2, 2, 2, 2, 2, 2, 2, 2, 2, 2, 2, 2, 2, 2, 2, 2, 2, 2, 2, 2, 2, 2, 2, 2, 2, 2, 2, 2, 2, 2, 2, 2, 2, 2, 2, 2, 2, 2, 2, 2, 2, 2, 2, 2, 2, 2, 2, 2, 2, 2, 2, 2, 2, 2, 2, 2, 2, 2, 2, 2, 2, 2, 2, 2, 2, 2, 2, 2, 2, 2, 2, 2, 2, 2, 2, 2, 2, 2, 2, 2, 2, 2, 2, 2, 2, 2, 2, 2, 2, 2, 2, 2, 2, 2, 2, 2, 2, 2, 2, 2, 2, 2, 2, 2, 2, 2, 2, 2, 2, 2, 2, 2, 2, 2, 2, 3 ),
 ( 0.000000000000000000, 1.000000000000000000 ),
 ( 0.000000000000000000, 0.003787878787878787984, 0.007575757575757575968, 0.01136363636363636395, 0.01515151515151515194, 0.01893939393939393992, 0.02272727272727272790, 0.02651515151515151589, 0.03030303030303030387, 0.03409090909090908839, 0.03787878787878787984, 0.04166666666666666435, 0.04545454545454545581, 0.04924242424242424032, 0.05303030303030303177, 0.05681818181818181629, 0.06060606060606060774, 0.06439393939393939226, 0.06818181818181817677, 0.07196969696969697516, 0.07575757575757575968, 0.07954545454545454419, 0.08333333333333332871, 0.08712121212121212710, 0.09090909090909091161, 0.09469696969696969613, 0.09848484848484848064, 0.1022727272727272790, 0.1060606060606060635, 0.1098484848484848481, 0.1136363636363636326, 0.1174242424242424310, 0.1212121212121212155, 0.1250000000000000000, 0.1287878787878787845, 0.1325757575757575690, 0.1363636363636363535, 0.1401515151515151381, 0.1439393939393939503, 0.1477272727272727348, 0.1515151515151515194, 0.1553030303030303039, 0.1590909090909090884, 0.1628787878787878729, 0.1666666666666666574, 0.1704545454545454419, 0.1742424242424242542, 0.1780303030303030387, 0.1818181818181818232, 0.1856060606060606077, 0.1893939393939393923, 0.1931818181818181768, 0.1969696969696969613, 0.2007575757575757458, 0.2045454545454545581, 0.2083333333333333426, 0.2121212121212121271, 0.2159090909090909116, 0.2196969696969696961, 0.2234848484848484806, 0.2272727272727272652, 0.2310606060606060497, 0.2348484848484848619, 0.2386363636363636465, 0.2424242424242424310, 0.2462121212121212155, 0.2500000000000000000, 0.2537878787878787845, 0.2575757575757575690, 0.2613636363636363535, 0.2651515151515151381, 0.2689393939393939226, 0.2727272727272727071, 0.2765151515151514916, 0.2803030303030302761, 0.2840909090909091161, 0.2878787878787879007, 0.2916666666666666852, 0.2954545454545454697, 0.2992424242424242542, 0.3030303030303030387, 0.3068181818181818232, 0.3106060606060606077, 0.3143939393939393923, 0.3181818181818181768, 0.3219696969696969613, 0.3257575757575757458, 0.3295454545454545303, 0.3333333333333333148, 0.3371212121212120993, 0.3409090909090908839, 0.3446969696969697239, 0.3484848484848485084, 0.3522727272727272929, 0.3560606060606060774, 0.3598484848484848619, 0.3636363636363636465, 0.3674242424242424310, 0.3712121212121212155, 0.3750000000000000000, 0.3787878787878787845, 0.3825757575757575690, 0.3863636363636363535, 0.3901515151515151381, 0.3939393939393939226, 0.3977272727272727071, 0.4015151515151514916, 0.4053030303030302761, 0.4090909090909091161, 0.4128787878787879007, 0.4166666666666666852, 0.4204545454545454697, 0.4242424242424242542, 0.4280303030303030387, 0.4318181818181818232, 0.4356060606060606077, 0.4393939393939393923, 0.4431818181818181768, 0.4469696969696969613, 0.4507575757575757458, 0.4545454545454545303, 0.4583333333333333148, 0.4621212121212120993, 0.4659090909090908839, 0.4696969696969697239, 0.4734848484848485084, 0.4772727272727272929, 0.4810606060606060774, 0.4848484848484848619, 0.4886363636363636465, 0.4924242424242424310, 0.4962121212121212155, 0.5000000000000000000, 0.5037878787878787845, 0.5075757575757575690, 0.5113636363636363535, 0.5151515151515151381, 0.5189393939393939226, 0.5227272727272727071, 0.5265151515151514916, 0.5303030303030302761, 0.5340909090909090606, 0.5378787878787878451, 0.5416666666666666297, 0.5454545454545454142, 0.5492424242424241987, 0.5530303030303029832, 0.5568181818181817677, 0.5606060606060605522, 0.5643939393939394478, 0.5681818181818182323, 0.5719696969696970168, 0.5757575757575758013, 0.5795454545454545858, 0.5833333333333333703, 0.5871212121212121549, 0.5909090909090909394, 0.5946969696969697239, 0.5984848484848485084, 0.6022727272727272929, 0.6060606060606060774, 0.6098484848484848619, 0.6136363636363636465, 0.6174242424242424310, 0.6212121212121212155, 0.6250000000000000000, 0.6287878787878787845, 0.6325757575757575690, 0.6363636363636363535, 0.6401515151515151381, 0.6439393939393939226, 0.6477272727272727071, 0.6515151515151514916, 0.6553030303030302761, 0.6590909090909090606, 0.6628787878787878451, 0.6666666666666666297, 0.6704545454545454142, 0.6742424242424241987, 0.6780303030303029832, 0.6818181818181817677, 0.6856060606060605522, 0.6893939393939394478, 0.6931818181818182323, 0.6969696969696970168, 0.7007575757575758013, 0.7045454545454545858, 0.7083333333333333703, 0.7121212121212121549, 0.7159090909090909394, 0.7196969696969697239, 0.7234848484848485084, 0.7272727272727272929, 0.7310606060606060774, 0.7348484848484848619, 0.7386363636363636465, 0.7424242424242424310, 0.7462121212121212155, 0.7500000000000000000, 0.7537878787878787845, 0.7575757575757575690, 0.7613636363636363535, 0.7651515151515151381, 0.7689393939393939226, 0.7727272727272727071, 0.7765151515151514916, 0.7803030303030302761, 0.7840909090909090606, 0.7878787878787878451, 0.7916666666666666297, 0.7954545454545454142, 0.7992424242424241987, 0.8030303030303029832, 0.8068181818181817677, 0.8106060606060605522, 0.8143939393939394478, 0.8181818181818182323, 0.8219696969696970168, 0.8257575757575758013, 0.8295454545454545858, 0.8333333333333333703, 0.8371212121212121549, 0.8409090909090909394, 0.8446969696969697239, 0.8484848484848485084, 0.8522727272727272929, 0.8560606060606060774, 0.8598484848484848619, 0.8636363636363636465, 0.8674242424242424310, 0.8712121212121212155, 0.8750000000000000000, 0.8787878787878787845, 0.8825757575757575690, 0.8863636363636363535, 0.8901515151515151381, 0.8939393939393939226, 0.8977272727272727071, 0.9015151515151514916, 0.9053030303030302761, 0.9090909090909090606, 0.9128787878787878451, 0.9166666666666666297, 0.9204545454545454142, 0.9242424242424241987, 0.9280303030303029832, 0.9318181818181817677, 0.9356060606060605522, 0.9393939393939394478, 0.9431818181818182323, 0.9469696969696970168, 0.9507575757575758013, 0.9545454545454545858, 0.9583333333333333703, 0.9621212121212121549, 0.9659090909090909394 ),
 .UNSPECIFIED. ) 
 GEOMETRIC_REPRESENTATION_ITEM ( )  RATIONAL_B_SPLINE_SURFACE ( (
 ( 1.000000000000000000, 0.9659258262890683122, 1.000000000000000000, 0.9659258262890683122, 1.000000000000000000, 0.9659258262890683122, 1.000000000000000000, 0.9659258262890683122, 1.000000000000000000, 0.9659258262890683122, 1.000000000000000000, 0.9659258262890683122, 1.000000000000000000, 0.9659258262890683122, 1.000000000000000000, 0.9659258262890683122, 1.000000000000000000, 0.9659258262890683122, 1.000000000000000000, 0.9659258262890683122, 1.000000000000000000, 0.9659258262890683122, 1.000000000000000000, 0.9659258262890683122, 1.000000000000000000, 0.9659258262890683122, 1.000000000000000000, 0.9659258262890683122, 1.000000000000000000, 0.9659258262890683122, 1.000000000000000000, 0.9659258262890683122, 1.000000000000000000, 0.9659258262890683122, 1.000000000000000000, 0.9659258262890683122, 1.000000000000000000, 0.9659258262890683122, 1.000000000000000000, 0.9659258262890683122, 1.000000000000000000, 0.9659258262890683122, 1.000000000000000000, 0.9659258262890683122, 1.000000000000000000, 0.9659258262890683122, 1.000000000000000000, 0.9659258262890683122, 1.000000000000000000, 0.9659258262890683122, 1.000000000000000000, 0.9659258262890683122, 1.000000000000000000, 0.9659258262890683122, 1.000000000000000000, 0.9659258262890683122, 1.000000000000000000, 0.9659258262890683122, 1.000000000000000000, 0.9659258262890683122, 1.000000000000000000, 0.9659258262890683122, 1.000000000000000000, 0.9659258262890683122, 1.000000000000000000, 0.9659258262890683122, 1.000000000000000000, 0.9659258262890683122, 1.000000000000000000, 0.9659258262890683122, 1.000000000000000000, 0.9659258262890683122, 1.000000000000000000, 0.9659258262890683122, 1.000000000000000000, 0.9659258262890683122, 1.000000000000000000, 0.9659258262890683122, 1.000000000000000000, 0.9659258262890683122, 1.000000000000000000, 0.9659258262890683122, 1.000000000000000000, 0.9659258262890683122, 1.000000000000000000, 0.9659258262890683122, 1.000000000000000000, 0.9659258262890683122, 1.000000000000000000, 0.9659258262890683122, 1.000000000000000000, 0.9659258262890683122, 1.000000000000000000, 0.9659258262890683122, 1.000000000000000000, 0.9659258262890683122, 1.000000000000000000, 0.9659258262890683122, 1.000000000000000000, 0.9659258262890683122, 1.000000000000000000, 0.9659258262890683122, 1.000000000000000000, 0.9659258262890683122, 1.000000000000000000, 0.9659258262890683122, 1.000000000000000000, 0.9659258262890683122, 1.000000000000000000, 0.9659258262890683122, 1.000000000000000000, 0.9659258262890683122, 1.000000000000000000, 0.9659258262890683122, 1.000000000000000000, 0.9659258262890683122, 1.000000000000000000, 0.9659258262890683122, 1.000000000000000000, 0.9659258262890683122, 1.000000000000000000, 0.9659258262890683122, 1.000000000000000000, 0.9659258262890683122, 1.000000000000000000, 0.9659258262890683122, 1.000000000000000000, 0.9659258262890683122, 1.000000000000000000, 0.9659258262890683122, 1.000000000000000000, 0.9659258262890683122, 1.000000000000000000, 0.9659258262890683122, 1.000000000000000000, 0.9659258262890683122, 1.000000000000000000, 0.9659258262890683122, 1.000000000000000000, 0.9659258262890683122, 1.000000000000000000, 0.9659258262890683122, 1.000000000000000000, 0.9659258262890683122, 1.000000000000000000, 0.9659258262890683122, 1.000000000000000000, 0.9659258262890683122, 1.000000000000000000, 0.9659258262890683122, 1.000000000000000000, 0.9659258262890683122, 1.000000000000000000, 0.9659258262890683122, 1.000000000000000000, 0.9659258262890683122, 1.000000000000000000, 0.9659258262890683122, 1.000000000000000000, 0.9659258262890683122, 1.000000000000000000, 0.9659258262890683122, 1.000000000000000000, 0.9659258262890683122, 1.000000000000000000, 0.9659258262890683122, 1.000000000000000000, 0.9659258262890683122, 1.000000000000000000, 0.9659258262890683122, 1.000000000000000000, 0.9659258262890683122, 1.000000000000000000, 0.9659258262890683122, 1.000000000000000000, 0.9659258262890683122, 1.000000000000000000, 0.9659258262890683122, 1.000000000000000000, 0.9659258262890683122, 1.000000000000000000, 0.9659258262890683122, 1.000000000000000000, 0.9659258262890683122, 1.000000000000000000, 0.9659258262890683122, 1.000000000000000000, 0.9659258262890683122, 1.000000000000000000, 0.9659258262890683122, 1.000000000000000000, 0.9659258262890683122, 1.000000000000000000, 0.9659258262890683122, 1.000000000000000000, 0.9659258262890683122, 1.000000000000000000, 0.9659258262890683122, 1.000000000000000000, 0.9659258262890683122, 1.000000000000000000, 0.9659258262890683122, 1.000000000000000000, 0.9659258262890683122, 1.000000000000000000, 0.9659258262890683122, 1.000000000000000000, 0.9659258262890683122, 1.000000000000000000, 0.9659258262890683122, 1.000000000000000000, 0.9659258262890683122, 1.000000000000000000, 0.9659258262890683122, 1.000000000000000000, 0.9659258262890683122, 1.000000000000000000, 0.9659258262890683122, 1.000000000000000000, 0.9659258262890683122, 1.000000000000000000, 0.9659258262890683122, 1.000000000000000000, 0.9659258262890683122, 1.000000000000000000, 0.9659258262890683122, 1.000000000000000000, 0.9659258262890683122, 1.000000000000000000, 0.9659258262890683122, 1.000000000000000000, 0.9659258262890683122, 1.000000000000000000, 0.9659258262890683122, 1.000000000000000000, 0.9659258262890683122, 1.000000000000000000, 0.9659258262890683122, 1.000000000000000000, 0.9659258262890683122, 1.000000000000000000, 0.9659258262890683122, 1.000000000000000000, 0.9659258262890683122, 1.000000000000000000, 0.9659258262890683122, 1.000000000000000000, 0.9659258262890683122, 1.000000000000000000, 0.9659258262890683122, 1.000000000000000000, 0.9659258262890683122, 1.000000000000000000, 0.9659258262890683122, 1.000000000000000000, 0.9659258262890683122, 1.000000000000000000, 0.9659258262890683122, 1.000000000000000000, 0.9659258262890683122, 1.000000000000000000, 0.9659258262890683122, 1.000000000000000000, 0.9659258262890683122, 1.000000000000000000, 0.9659258262890683122, 1.000000000000000000, 0.9659258262890683122, 1.000000000000000000, 0.9659258262890683122, 1.000000000000000000, 0.9659258262890683122, 1.000000000000000000, 0.9659258262890683122, 1.000000000000000000, 0.9659258262890683122, 1.000000000000000000, 0.9659258262890683122, 1.000000000000000000, 0.9659258262890683122, 1.000000000000000000, 0.9659258262890683122, 1.000000000000000000, 0.9659258262890683122, 1.000000000000000000, 0.9659258262890683122, 1.000000000000000000, 0.9659258262890683122, 1.000000000000000000, 0.9659258262890683122, 1.000000000000000000, 0.9659258262890683122, 1.000000000000000000, 0.9659258262890683122, 1.000000000000000000, 0.9659258262890683122, 1.000000000000000000, 0.9659258262890683122, 1.000000000000000000, 0.9659258262890683122, 1.000000000000000000, 0.9659258262890683122, 1.000000000000000000, 0.9659258262890683122, 1.000000000000000000, 0.9659258262890683122, 1.000000000000000000, 0.9659258262890683122, 1.000000000000000000, 0.9659258262890683122, 1.000000000000000000, 0.9659258262890683122, 1.000000000000000000, 0.9659258262890683122, 1.000000000000000000, 0.9659258262890683122, 1.000000000000000000, 0.9659258262890683122, 1.000000000000000000, 0.9659258262890683122, 1.000000000000000000, 0.9659258262890683122, 1.000000000000000000, 0.9659258262890683122, 1.000000000000000000, 0.9659258262890683122, 1.000000000000000000, 0.9659258262890683122, 1.000000000000000000, 0.9659258262890683122, 1.000000000000000000, 0.9659258262890683122, 1.000000000000000000, 0.9659258262890683122, 1.000000000000000000, 0.9659258262890683122, 1.000000000000000000, 0.9659258262890683122, 1.000000000000000000, 0.9659258262890683122, 1.000000000000000000, 0.9659258262890683122, 1.000000000000000000, 0.9659258262890683122, 1.000000000000000000, 0.9659258262890683122, 1.000000000000000000, 0.9659258262890683122, 1.000000000000000000, 0.9659258262890683122, 1.000000000000000000, 0.9659258262890683122, 1.000000000000000000, 0.9659258262890683122, 1.000000000000000000, 0.9659258262890683122, 1.000000000000000000, 0.9659258262890683122, 1.000000000000000000, 0.9659258262890683122, 1.000000000000000000, 0.9659258262890683122, 1.000000000000000000, 0.9659258262890683122, 1.000000000000000000, 0.9659258262890683122, 1.000000000000000000, 0.9659258262890683122, 1.000000000000000000, 0.9659258262890683122, 1.000000000000000000, 0.9659258262890683122, 1.000000000000000000, 0.9659258262890683122, 1.000000000000000000, 0.9659258262890683122, 1.000000000000000000, 0.9659258262890683122, 1.000000000000000000, 0.9659258262890683122, 1.000000000000000000, 0.9659258262890683122, 1.000000000000000000, 0.9659258262890683122, 1.000000000000000000, 0.9659258262890683122, 1.000000000000000000, 0.9659258262890683122, 1.000000000000000000, 0.9659258262890683122, 1.000000000000000000, 0.9659258262890683122, 1.000000000000000000, 0.9659258262890683122, 1.000000000000000000, 0.9659258262890683122, 1.000000000000000000, 0.9659258262890683122, 1.000000000000000000, 0.9659258262890683122, 1.000000000000000000, 0.9659258262890683122, 1.000000000000000000, 0.9659258262890683122, 1.000000000000000000, 0.9659258262890683122, 1.000000000000000000, 0.9659258262890683122, 1.000000000000000000, 0.9659258262890683122, 1.000000000000000000, 0.9659258262890683122, 1.000000000000000000, 0.9659258262890683122, 1.000000000000000000, 0.9659258262890683122, 1.000000000000000000, 0.9659258262890683122, 1.000000000000000000, 0.9659258262890683122, 1.000000000000000000, 0.9659258262890683122, 1.000000000000000000, 0.9659258262890683122, 1.000000000000000000, 0.9659258262890683122, 1.000000000000000000, 0.9659258262890683122, 1.000000000000000000, 0.9659258262890683122, 1.000000000000000000, 0.9659258262890683122, 1.000000000000000000, 0.9659258262890683122, 1.000000000000000000, 0.9659258262890683122, 1.000000000000000000, 0.9659258262890683122, 1.000000000000000000, 0.9659258262890683122, 1.000000000000000000, 0.9659258262890683122, 1.000000000000000000, 0.9659258262890683122, 1.000000000000000000, 0.9659258262890683122, 1.000000000000000000, 0.9659258262890683122, 1.000000000000000000, 0.9659258262890683122, 1.000000000000000000, 0.9659258262890683122, 1.000000000000000000, 0.9659258262890683122, 1.000000000000000000, 0.9659258262890683122, 1.000000000000000000, 0.9659258262890683122, 1.000000000000000000, 0.9659258262890683122, 1.000000000000000000, 0.9659258262890683122, 1.000000000000000000, 0.9659258262890683122, 1.000000000000000000, 0.9659258262890683122, 1.000000000000000000, 0.9659258262890683122, 1.000000000000000000, 0.9659258262890683122, 1.000000000000000000, 0.9659258262890683122, 1.000000000000000000, 0.9659258262890683122, 1.000000000000000000, 0.9659258262890683122, 1.000000000000000000, 0.9659258262890683122, 1.000000000000000000, 0.9659258262890683122, 1.000000000000000000, 0.9659258262890683122, 1.000000000000000000, 0.9659258262890683122, 1.000000000000000000, 0.9659258262890683122, 1.000000000000000000, 0.9659258262890683122, 1.000000000000000000, 0.9659258262890683122, 1.000000000000000000, 0.9659258262890683122, 1.000000000000000000, 0.9659258262890683122, 1.000000000000000000, 0.9659258262890683122, 1.000000000000000000, 0.9659258262890683122, 1.000000000000000000, 0.9659258262890683122, 1.000000000000000000, 0.9659258262890683122, 1.000000000000000000, 0.9659258262890683122, 1.000000000000000000, 0.9659258262890683122, 1.000000000000000000, 0.9659258262890683122, 1.000000000000000000, 0.9659258262890683122, 1.000000000000000000),
 ( 1.000000000000000000, 0.9659258262890683122, 1.000000000000000000, 0.9659258262890683122, 1.000000000000000000, 0.9659258262890683122, 1.000000000000000000, 0.9659258262890683122, 1.000000000000000000, 0.9659258262890683122, 1.000000000000000000, 0.9659258262890683122, 1.000000000000000000, 0.9659258262890683122, 1.000000000000000000, 0.9659258262890683122, 1.000000000000000000, 0.9659258262890683122, 1.000000000000000000, 0.9659258262890683122, 1.000000000000000000, 0.9659258262890683122, 1.000000000000000000, 0.9659258262890683122, 1.000000000000000000, 0.9659258262890683122, 1.000000000000000000, 0.9659258262890683122, 1.000000000000000000, 0.9659258262890683122, 1.000000000000000000, 0.9659258262890683122, 1.000000000000000000, 0.9659258262890683122, 1.000000000000000000, 0.9659258262890683122, 1.000000000000000000, 0.9659258262890683122, 1.000000000000000000, 0.9659258262890683122, 1.000000000000000000, 0.9659258262890683122, 1.000000000000000000, 0.9659258262890683122, 1.000000000000000000, 0.9659258262890683122, 1.000000000000000000, 0.9659258262890683122, 1.000000000000000000, 0.9659258262890683122, 1.000000000000000000, 0.9659258262890683122, 1.000000000000000000, 0.9659258262890683122, 1.000000000000000000, 0.9659258262890683122, 1.000000000000000000, 0.9659258262890683122, 1.000000000000000000, 0.9659258262890683122, 1.000000000000000000, 0.9659258262890683122, 1.000000000000000000, 0.9659258262890683122, 1.000000000000000000, 0.9659258262890683122, 1.000000000000000000, 0.9659258262890683122, 1.000000000000000000, 0.9659258262890683122, 1.000000000000000000, 0.9659258262890683122, 1.000000000000000000, 0.9659258262890683122, 1.000000000000000000, 0.9659258262890683122, 1.000000000000000000, 0.9659258262890683122, 1.000000000000000000, 0.9659258262890683122, 1.000000000000000000, 0.9659258262890683122, 1.000000000000000000, 0.9659258262890683122, 1.000000000000000000, 0.9659258262890683122, 1.000000000000000000, 0.9659258262890683122, 1.000000000000000000, 0.9659258262890683122, 1.000000000000000000, 0.9659258262890683122, 1.000000000000000000, 0.9659258262890683122, 1.000000000000000000, 0.9659258262890683122, 1.000000000000000000, 0.9659258262890683122, 1.000000000000000000, 0.9659258262890683122, 1.000000000000000000, 0.9659258262890683122, 1.000000000000000000, 0.9659258262890683122, 1.000000000000000000, 0.9659258262890683122, 1.000000000000000000, 0.9659258262890683122, 1.000000000000000000, 0.9659258262890683122, 1.000000000000000000, 0.9659258262890683122, 1.000000000000000000, 0.9659258262890683122, 1.000000000000000000, 0.9659258262890683122, 1.000000000000000000, 0.9659258262890683122, 1.000000000000000000, 0.9659258262890683122, 1.000000000000000000, 0.9659258262890683122, 1.000000000000000000, 0.9659258262890683122, 1.000000000000000000, 0.9659258262890683122, 1.000000000000000000, 0.9659258262890683122, 1.000000000000000000, 0.9659258262890683122, 1.000000000000000000, 0.9659258262890683122, 1.000000000000000000, 0.9659258262890683122, 1.000000000000000000, 0.9659258262890683122, 1.000000000000000000, 0.9659258262890683122, 1.000000000000000000, 0.9659258262890683122, 1.000000000000000000, 0.9659258262890683122, 1.000000000000000000, 0.9659258262890683122, 1.000000000000000000, 0.9659258262890683122, 1.000000000000000000, 0.9659258262890683122, 1.000000000000000000, 0.9659258262890683122, 1.000000000000000000, 0.9659258262890683122, 1.000000000000000000, 0.9659258262890683122, 1.000000000000000000, 0.9659258262890683122, 1.000000000000000000, 0.9659258262890683122, 1.000000000000000000, 0.9659258262890683122, 1.000000000000000000, 0.9659258262890683122, 1.000000000000000000, 0.9659258262890683122, 1.000000000000000000, 0.9659258262890683122, 1.000000000000000000, 0.9659258262890683122, 1.000000000000000000, 0.9659258262890683122, 1.000000000000000000, 0.9659258262890683122, 1.000000000000000000, 0.9659258262890683122, 1.000000000000000000, 0.9659258262890683122, 1.000000000000000000, 0.9659258262890683122, 1.000000000000000000, 0.9659258262890683122, 1.000000000000000000, 0.9659258262890683122, 1.000000000000000000, 0.9659258262890683122, 1.000000000000000000, 0.9659258262890683122, 1.000000000000000000, 0.9659258262890683122, 1.000000000000000000, 0.9659258262890683122, 1.000000000000000000, 0.9659258262890683122, 1.000000000000000000, 0.9659258262890683122, 1.000000000000000000, 0.9659258262890683122, 1.000000000000000000, 0.9659258262890683122, 1.000000000000000000, 0.9659258262890683122, 1.000000000000000000, 0.9659258262890683122, 1.000000000000000000, 0.9659258262890683122, 1.000000000000000000, 0.9659258262890683122, 1.000000000000000000, 0.9659258262890683122, 1.000000000000000000, 0.9659258262890683122, 1.000000000000000000, 0.9659258262890683122, 1.000000000000000000, 0.9659258262890683122, 1.000000000000000000, 0.9659258262890683122, 1.000000000000000000, 0.9659258262890683122, 1.000000000000000000, 0.9659258262890683122, 1.000000000000000000, 0.9659258262890683122, 1.000000000000000000, 0.9659258262890683122, 1.000000000000000000, 0.9659258262890683122, 1.000000000000000000, 0.9659258262890683122, 1.000000000000000000, 0.9659258262890683122, 1.000000000000000000, 0.9659258262890683122, 1.000000000000000000, 0.9659258262890683122, 1.000000000000000000, 0.9659258262890683122, 1.000000000000000000, 0.9659258262890683122, 1.000000000000000000, 0.9659258262890683122, 1.000000000000000000, 0.9659258262890683122, 1.000000000000000000, 0.9659258262890683122, 1.000000000000000000, 0.9659258262890683122, 1.000000000000000000, 0.9659258262890683122, 1.000000000000000000, 0.9659258262890683122, 1.000000000000000000, 0.9659258262890683122, 1.000000000000000000, 0.9659258262890683122, 1.000000000000000000, 0.9659258262890683122, 1.000000000000000000, 0.9659258262890683122, 1.000000000000000000, 0.9659258262890683122, 1.000000000000000000, 0.9659258262890683122, 1.000000000000000000, 0.9659258262890683122, 1.000000000000000000, 0.9659258262890683122, 1.000000000000000000, 0.9659258262890683122, 1.000000000000000000, 0.9659258262890683122, 1.000000000000000000, 0.9659258262890683122, 1.000000000000000000, 0.9659258262890683122, 1.000000000000000000, 0.9659258262890683122, 1.000000000000000000, 0.9659258262890683122, 1.000000000000000000, 0.9659258262890683122, 1.000000000000000000, 0.9659258262890683122, 1.000000000000000000, 0.9659258262890683122, 1.000000000000000000, 0.9659258262890683122, 1.000000000000000000, 0.9659258262890683122, 1.000000000000000000, 0.9659258262890683122, 1.000000000000000000, 0.9659258262890683122, 1.000000000000000000, 0.9659258262890683122, 1.000000000000000000, 0.9659258262890683122, 1.000000000000000000, 0.9659258262890683122, 1.000000000000000000, 0.9659258262890683122, 1.000000000000000000, 0.9659258262890683122, 1.000000000000000000, 0.9659258262890683122, 1.000000000000000000, 0.9659258262890683122, 1.000000000000000000, 0.9659258262890683122, 1.000000000000000000, 0.9659258262890683122, 1.000000000000000000, 0.9659258262890683122, 1.000000000000000000, 0.9659258262890683122, 1.000000000000000000, 0.9659258262890683122, 1.000000000000000000, 0.9659258262890683122, 1.000000000000000000, 0.9659258262890683122, 1.000000000000000000, 0.9659258262890683122, 1.000000000000000000, 0.9659258262890683122, 1.000000000000000000, 0.9659258262890683122, 1.000000000000000000, 0.9659258262890683122, 1.000000000000000000, 0.9659258262890683122, 1.000000000000000000, 0.9659258262890683122, 1.000000000000000000, 0.9659258262890683122, 1.000000000000000000, 0.9659258262890683122, 1.000000000000000000, 0.9659258262890683122, 1.000000000000000000, 0.9659258262890683122, 1.000000000000000000, 0.9659258262890683122, 1.000000000000000000, 0.9659258262890683122, 1.000000000000000000, 0.9659258262890683122, 1.000000000000000000, 0.9659258262890683122, 1.000000000000000000, 0.9659258262890683122, 1.000000000000000000, 0.9659258262890683122, 1.000000000000000000, 0.9659258262890683122, 1.000000000000000000, 0.9659258262890683122, 1.000000000000000000, 0.9659258262890683122, 1.000000000000000000, 0.9659258262890683122, 1.000000000000000000, 0.9659258262890683122, 1.000000000000000000, 0.9659258262890683122, 1.000000000000000000, 0.9659258262890683122, 1.000000000000000000, 0.9659258262890683122, 1.000000000000000000, 0.9659258262890683122, 1.000000000000000000, 0.9659258262890683122, 1.000000000000000000, 0.9659258262890683122, 1.000000000000000000, 0.9659258262890683122, 1.000000000000000000, 0.9659258262890683122, 1.000000000000000000, 0.9659258262890683122, 1.000000000000000000, 0.9659258262890683122, 1.000000000000000000, 0.9659258262890683122, 1.000000000000000000, 0.9659258262890683122, 1.000000000000000000, 0.9659258262890683122, 1.000000000000000000, 0.9659258262890683122, 1.000000000000000000, 0.9659258262890683122, 1.000000000000000000, 0.9659258262890683122, 1.000000000000000000, 0.9659258262890683122, 1.000000000000000000, 0.9659258262890683122, 1.000000000000000000, 0.9659258262890683122, 1.000000000000000000, 0.9659258262890683122, 1.000000000000000000, 0.9659258262890683122, 1.000000000000000000, 0.9659258262890683122, 1.000000000000000000, 0.9659258262890683122, 1.000000000000000000, 0.9659258262890683122, 1.000000000000000000, 0.9659258262890683122, 1.000000000000000000, 0.9659258262890683122, 1.000000000000000000, 0.9659258262890683122, 1.000000000000000000, 0.9659258262890683122, 1.000000000000000000, 0.9659258262890683122, 1.000000000000000000, 0.9659258262890683122, 1.000000000000000000, 0.9659258262890683122, 1.000000000000000000, 0.9659258262890683122, 1.000000000000000000, 0.9659258262890683122, 1.000000000000000000, 0.9659258262890683122, 1.000000000000000000, 0.9659258262890683122, 1.000000000000000000, 0.9659258262890683122, 1.000000000000000000, 0.9659258262890683122, 1.000000000000000000, 0.9659258262890683122, 1.000000000000000000, 0.9659258262890683122, 1.000000000000000000, 0.9659258262890683122, 1.000000000000000000, 0.9659258262890683122, 1.000000000000000000, 0.9659258262890683122, 1.000000000000000000, 0.9659258262890683122, 1.000000000000000000, 0.9659258262890683122, 1.000000000000000000, 0.9659258262890683122, 1.000000000000000000, 0.9659258262890683122, 1.000000000000000000, 0.9659258262890683122, 1.000000000000000000, 0.9659258262890683122, 1.000000000000000000, 0.9659258262890683122, 1.000000000000000000, 0.9659258262890683122, 1.000000000000000000, 0.9659258262890683122, 1.000000000000000000, 0.9659258262890683122, 1.000000000000000000, 0.9659258262890683122, 1.000000000000000000, 0.9659258262890683122, 1.000000000000000000, 0.9659258262890683122, 1.000000000000000000, 0.9659258262890683122, 1.000000000000000000, 0.9659258262890683122, 1.000000000000000000, 0.9659258262890683122, 1.000000000000000000, 0.9659258262890683122, 1.000000000000000000, 0.9659258262890683122, 1.000000000000000000, 0.9659258262890683122, 1.000000000000000000, 0.9659258262890683122, 1.000000000000000000, 0.9659258262890683122, 1.000000000000000000, 0.9659258262890683122, 1.000000000000000000, 0.9659258262890683122, 1.000000000000000000, 0.9659258262890683122, 1.000000000000000000, 0.9659258262890683122, 1.000000000000000000, 0.9659258262890683122, 1.000000000000000000, 0.9659258262890683122, 1.000000000000000000, 0.9659258262890683122, 1.000000000000000000, 0.9659258262890683122, 1.000000000000000000, 0.9659258262890683122, 1.000000000000000000, 0.9659258262890683122, 1.000000000000000000, 0.9659258262890683122, 1.000000000000000000) ) ) 
 REPRESENTATION_ITEM ( '' )  SURFACE ( )  );
#45203=CARTESIAN_POINT ( 'NONE',  ( 1.364829396325460076, 0.2306618581243848609, 0.2411417322834645549 ) ) ;
#45205=CARTESIAN_POINT ( 'NONE',  ( 1.036745406824147508, -0.3690944881889765550, -0.3153832671262227771 ) ) ;
#45207=CARTESIAN_POINT ( 'NONE',  ( 1.502624671916010790, -0.08942795157527998196, 0.3641732283464567121 ) ) ;
#45212=CARTESIAN_POINT ( 'NONE',  ( -1.174540682414697335, -0.08942795157527998196, 0.3641732283464567121 ) ) ;
#45213=CARTESIAN_POINT ( 'NONE',  ( -1.594488188976377563, -0.4536011799217367080, 0.2665933059059888421 ) ) ;
#45214=CARTESIAN_POINT ( 'NONE',  ( -1.141732283464566011, 0.2952755905511811885, 0.000000000000000000 ) ) ;
#45215=CARTESIAN_POINT ( 'NONE',  ( 0.1902887139107617975, 0.2952755905511811885, 0.1292274648535926551 ) ) ;
#45216=CARTESIAN_POINT ( 'NONE',  ( 1.417322834645670104, -0.1870078740157479769, 0.4822834645669291653 ) ) ;
#45223=CARTESIAN_POINT ( 'NONE',  ( -0.7545931758530176614, -0.5511811023622048555, -0.09757992244046775898 ) ) ;
#45224=EDGE_CURVE ( 'NONE', #35196, #35306, #42516, .T. ) ;
#45225=CARTESIAN_POINT ( 'NONE',  ( -0.9908136482939626788, 0.2952755905511811885, 0.1292274648535926551 ) ) ;
#45226=CARTESIAN_POINT ( 'NONE',  ( 0.6955380577427828781, -0.4281496062992124485, 0.4176697321401328655 ) ) ;
#45227=EDGE_LOOP ( 'NONE', ( #71520, #42504, #59925, #70997 ) ) ;
#45230=CARTESIAN_POINT ( 'NONE',  ( 1.062992125984252745, 0.2952755905511811885, 0.000000000000000000 ) ) ;
#45231=CARTESIAN_POINT ( 'NONE',  ( 1.541994750656168645, -0.5511811023622046335, 0.09757992244046803654 ) ) ;
#45233=EDGE_CURVE ( 'NONE', #80562, #79831, #57364, .T. ) ;
#45234=CARTESIAN_POINT ( 'NONE',  ( -0.3412073490813641308, -0.5023911411419708095, 0.1820866141732285504 ) ) ;
#45235=CARTESIAN_POINT ( 'NONE',  ( -1.279527559055116948, 0.07958543189024071263, -0.2665933059059888421 ) ) ;
#45237=CARTESIAN_POINT ( 'NONE',  ( -0.4068241469816264999, -0.3690944881889763329, 0.3153832671262228327 ) ) ;
#45238=CARTESIAN_POINT ( 'NONE',  ( 0.3018372703412079971, -0.3690944881889763329, 0.3153832671262228327 ) ) ;
#45239=CARTESIAN_POINT ( 'NONE',  ( 0.006561679790026889343, -0.05778040916215522460, 0.4822834645669289988 ) ) ;
#45240=CARTESIAN_POINT ( 'NONE',  ( -1.102362204724408601, -0.1870078740157480601, -0.3641732283464567677 ) ) ;
#45242=CARTESIAN_POINT ( 'NONE',  ( 1.102362204724410155, -0.1870078740157479769, 0.4822834645669291653 ) ) ;
#45244=CARTESIAN_POINT ( 'NONE',  ( -1.568241469816272105, -0.3162353388693409650, -0.4822834645669289433 ) ) ;
#45248=CARTESIAN_POINT ( 'NONE',  ( -0.4133858267716528645, 0.1660481256975883668, -0.3530559997133364547 ) ) ;
#45249=CARTESIAN_POINT ( 'NONE',  ( -1.076115485564303809, -0.6046776061558809534, -0.2411417322834644161 ) ) ;
#45250=CARTESIAN_POINT ( 'NONE',  ( 0.9383202099737538715, -0.08942795157528024563, -0.3641732283464568787 ) ) ;
#45251=CARTESIAN_POINT ( 'NONE',  ( -0.3346456692913377662, -0.4536011799217367080, 0.2665933059059888421 ) ) ;
#45252=CARTESIAN_POINT ( 'NONE',  ( -0.7020997375328076329, -0.3162353388693409650, -0.4822834645669289433 ) ) ;
#45253=CARTESIAN_POINT ( 'NONE',  ( -1.633858267716534529, 0.1660481256975885056, 0.3530559997133364547 ) ) ;
#45255=CARTESIAN_POINT ( 'NONE',  ( 1.391076115485564868, 0.1283753931104746893, -0.1820866141732285504 ) ) ;
#45257=CARTESIAN_POINT ( 'NONE',  ( -1.541994750656167090, -0.6692913385826773087, -0.1292274648535924053 ) ) ;
#45258=CARTESIAN_POINT ( 'NONE',  ( -1.423884514435694859, -0.3162353388693405765, 0.4822834645669290543 ) ) ;
#45261=CARTESIAN_POINT ( 'NONE',  ( -1.010498687664041384, -0.004921259842519576551, 0.3153832671262227771 ) ) ;
#45262=CARTESIAN_POINT ( 'NONE',  ( 0.6824146981627303710, 0.2306618581243847221, -0.2411417322834647770 ) ) ;
#45263=CARTESIAN_POINT ( 'NONE',  ( -1.062992125984250968, 0.1771653543307087630, 0.000000000000000000 ) ) ;
#45265=CARTESIAN_POINT ( 'NONE',  ( -1.082677165354329896, 0.1660481256975885056, 0.3530559997133364547 ) ) ;
#45266=CARTESIAN_POINT ( 'NONE',  ( 0.7086614173228353852, -0.1870078740157479769, 0.4822834645669291653 ) ) ;
#45267=CARTESIAN_POINT ( 'NONE',  ( 0.4986876640419954376, -0.6046776061558809534, -0.2411417322834644161 ) ) ;
#45268=CARTESIAN_POINT ( 'NONE',  ( 1.410761154855643795, -0.3162353388693405765, 0.4822834645669290543 ) ) ;
#45269=CARTESIAN_POINT ( 'NONE',  ( -1.417322834645668772, -0.1870078740157479769, 0.3641732283464567677 ) ) ;
#45273=B_SPLINE_CURVE_WITH_KNOTS ( 'NONE', 3,
 ( #15511, #9191, #33202, #27708, #58867, #53374, #7950 ),
 .UNSPECIFIED., .F., .F.,
 ( 4, 3, 4 ),
 ( 3.643951726750583631E-17, 0.001246232571205267009, 0.002492492258783277591 ),
 .UNSPECIFIED. ) ;
#45275=CARTESIAN_POINT ( 'NONE',  ( 1.227034120734908917, 0.1771653543307087075, -0.09757992244046823083 ) ) ;
#45276=CARTESIAN_POINT ( 'NONE',  ( 0.5052493438320215802, 0.1771653543307087630, 0.09757992244046791164 ) ) ;
#45277=CARTESIAN_POINT ( 'NONE',  ( 0.2952755905511816326, -0.5400638737290844871, 0.3530559997133364547 ) ) ;
#45278=CARTESIAN_POINT ( 'NONE',  ( 1.384514435695538337, -0.6692913385826771977, 0.1292274648535927661 ) ) ;
#45280=CARTESIAN_POINT ( 'NONE',  ( 0.5708661417322842269, 0.07958543189024085140, 0.2665933059059887866 ) ) ;
#45281=CARTESIAN_POINT ( 'NONE',  ( -0.5971128608923877978, -0.6692913385826773087, -0.1292274648535924053 ) ) ;
#45282=CARTESIAN_POINT ( 'NONE',  ( -1.227034120734907141, -0.6692913385826773087, -0.1292274648535924053 ) ) ;
#45283=CARTESIAN_POINT ( 'NONE',  ( 0.9514435695538062676, -0.3162353388693409650, -0.4822834645669289433 ) ) ;
#45288=CARTESIAN_POINT ( 'NONE',  ( -1.167979002624671470, -0.4281496062992127816, -0.4176697321401328100 ) ) ;
#45289=CARTESIAN_POINT ( 'NONE',  ( -0.8136482939632537770, 0.2306618581243847221, -0.2411417322834647770 ) ) ;
#45290=CARTESIAN_POINT ( 'NONE',  ( -0.6692913385826764205, 0.1771653543307087630, 0.000000000000000000 ) ) ;
#45291=CARTESIAN_POINT ( 'NONE',  ( -0.8202099737532799750, 0.2952755905511810774, -0.1292274648535930714 ) ) ;
#45293=CARTESIAN_POINT ( 'NONE',  ( -0.4600214019799515053, 0.000000000000000000, 0.3464511005275205946 ) ) ;
#45294=CARTESIAN_POINT ( 'NONE',  ( 1.673228346456693494, 0.1660481256975885056, 0.3530559997133364547 ) ) ;
#45295=CARTESIAN_POINT ( 'NONE',  ( -1.410761154855642463, -0.05778040916215522460, 0.4822834645669289988 ) ) ;
#45296=CARTESIAN_POINT ( 'NONE',  ( 0.5183727034120741983, 0.2952755905511810774, -0.1292274648535930714 ) ) ;
#45297=CARTESIAN_POINT ( 'NONE',  ( -0.6824146981627288167, 0.2306618581243848609, 0.2411417322834645549 ) ) ;
#45298=CIRCLE ( 'NONE', #6321, 2.362204724409449064 ) ;
#45300=CARTESIAN_POINT ( 'NONE',  ( -0.9120734908136475250, -0.5511811023622048555, -0.09757992244046775898 ) ) ;
#45301=ORIENTED_EDGE ( 'NONE', *, *, #22330, .T. ) ;
#45305=CARTESIAN_POINT ( 'NONE',  ( -1.732283464566928277, -0.1870078740157479769, 0.3641732283464567677 ) ) ;
#45306=CARTESIAN_POINT ( 'NONE',  ( -1.292650918635170010, -0.6692913385826771977, 0.1292274648535927661 ) ) ;
#45307=CARTESIAN_POINT ( 'NONE',  ( -1.233595800524933894, -0.6046776061558809534, -0.2411417322834644161 ) ) ;
#45309=CARTESIAN_POINT ( 'NONE',  ( -1.076115485564303809, 0.2306618581243848609, 0.2411417322834645549 ) ) ;
#45310=CARTESIAN_POINT ( 'NONE',  ( -1.062992125984250968, 0.2952755905511811885, 0.000000000000000000 ) ) ;
#45312=CARTESIAN_POINT ( 'NONE',  ( -0.8530183727034112984, 0.05413385826771666132, 0.4176697321401328100 ) ) ;
#45313=CARTESIAN_POINT ( 'NONE',  ( -0.03280839895013062252, 0.1771653543307087075, -0.09757992244046823083 ) ) ;
#45316=CARTESIAN_POINT ( 'NONE',  ( -0.4724409448818890911, -0.1870078740157479769, 0.3641732283464567677 ) ) ;
#45317=CARTESIAN_POINT ( 'NONE',  ( -0.7480314960629914633, -0.6692913385826771977, 8.415575281601705876E-17 ) ) ;
#45318=CARTESIAN_POINT ( 'NONE',  ( 1.266404199475066328, -0.05778040916215522460, 0.4822834645669289988 ) ) ;
#45319=CARTESIAN_POINT ( 'NONE',  ( -0.6824146981627288167, 0.2306618581243848609, 0.2411417322834645549 ) ) ;
#45320=ORIENTED_EDGE ( 'NONE', *, *, #10592, .T. ) ;
#45323=CARTESIAN_POINT ( 'NONE',  ( -1.154855643044618851, 0.2306618581243848609, 0.2411417322834645549 ) ) ;
#45324=CARTESIAN_POINT ( 'NONE',  ( 1.279527559055118724, 0.1660481256975885056, 0.3530559997133364547 ) ) ;
#45325=CARTESIAN_POINT ( 'NONE',  ( -1.220472440944881054, 0.1771653543307087630, 0.000000000000000000 ) ) ;
#45326=CARTESIAN_POINT ( 'NONE',  ( -1.181102362204723644, -0.1870078740157480879, -0.4822834645669291653 ) ) ;
#45331=CARTESIAN_POINT ( 'NONE',  ( -0.05905511811023545637, 0.1660481256975885056, 0.3530559997133364547 ) ) ;
#45332=CARTESIAN_POINT ( 'NONE',  ( -1.417322834645668772, -0.1870078740157480601, -0.3641732283464567677 ) ) ;
#45333=CARTESIAN_POINT ( 'NONE',  ( -0.6496062992125976043, -0.5400638737290844871, 0.3530559997133364547 ) ) ;
#45335=CARTESIAN_POINT ( 'NONE',  ( -1.181102362204723644, -0.1870078740157480879, -0.4822834645669291653 ) ) ;
#45336=CARTESIAN_POINT ( 'NONE',  ( -1.187664041994750175, -0.05778040916215560624, -0.4822834645669293319 ) ) ;
#45337=CARTESIAN_POINT ( 'NONE',  ( -0.1771653543307080136, -0.5400638737290844871, 0.3530559997133364547 ) ) ;
#45339=CARTESIAN_POINT ( 'NONE',  ( 0.7742782152230978099, -0.3690944881889763329, 0.3153832671262228327 ) ) ;
#45340=CARTESIAN_POINT ( 'NONE',  ( -0.9251968503937002541, 0.07958543189024085140, 0.2665933059059887866 ) ) ;
#45342=CARTESIAN_POINT ( 'NONE',  ( 0.9120734908136490793, 0.1771653543307087075, -0.09757992244046823083 ) ) ;
#45343=CARTESIAN_POINT ( 'NONE',  ( 1.568241469816273437, -0.2845877964562159024, 0.3641732283464567677 ) ) ;
#45344=CARTESIAN_POINT ( 'NONE',  ( 1.181102362204724976, -0.1870078740157480879, -0.4822834645669291653 ) ) ;
#45345=CARTESIAN_POINT ( 'NONE',  ( 0.06561679790026316017, -0.3690944881889763329, 0.3153832671262228327 ) ) ;
#45347=CARTESIAN_POINT ( 'NONE',  ( -0.7217847769028863381, -0.4281496062992124485, 0.4176697321401328655 ) ) ;
#45348=CARTESIAN_POINT ( 'NONE',  ( 1.187664041994751285, -0.3162353388693409650, -0.4822834645669289433 ) ) ;
#45350=CARTESIAN_POINT ( 'NONE',  ( -0.4790026246719152336, -0.08942795157528024563, -0.3641732283464568787 ) ) ;
#45352=CARTESIAN_POINT ( 'NONE',  ( 0.4330708661417329575, 0.2952755905511811885, 0.000000000000000000 ) ) ;
#45353=DIRECTION ( 'NONE',  ( -3.096699300667737957E-16, 1.000000000000000000, -0.000000000000000000 ) ) ;
#45354=CARTESIAN_POINT ( 'NONE',  ( 0.7808398950131240079, -0.2845877964562159024, 0.3641732283464567677 ) ) ;
#45355=CARTESIAN_POINT ( 'NONE',  ( 0.3412073490813655186, 0.1283753931104748280, 0.1820866141732283561 ) ) ;
#45356=CARTESIAN_POINT ( 'NONE',  ( -0.5118110236220466680, 0.2952755905511811885, 0.000000000000000000 ) ) ;
#45357=CARTESIAN_POINT ( 'NONE',  ( -1.266404199475064773, -0.3162353388693405765, 0.4822834645669290543 ) ) ;
#45358=CARTESIAN_POINT ( 'NONE',  ( -0.7086614173228339419, -0.1870078740157479769, 0.3641732283464567677 ) ) ;
#45361=CARTESIAN_POINT ( 'NONE',  ( -0.7283464566929126471, -0.5400638737290844871, 0.3530559997133364547 ) ) ;
#45364=CARTESIAN_POINT ( 'NONE',  ( 0.01968503937007930540, 0.07958543189024085140, 0.2665933059059887866 ) ) ;
#45365=CARTESIAN_POINT ( 'NONE',  ( -0.8070866141732276899, 0.1660481256975883668, -0.3530559997133364547 ) ) ;
#45367=CARTESIAN_POINT ( 'NONE',  ( -0.9383202099737524282, -0.3162353388693409650, -0.4822834645669289433 ) ) ;
#45368=CARTESIAN_POINT ( 'NONE',  ( -1.417322834645668772, -0.1870078740157480601, -0.3641732283464567677 ) ) ;
#45369=CARTESIAN_POINT ( 'NONE',  ( 1.666666666666667185, 0.05413385826771666132, 0.4176697321401328100 ) ) ;
#45370=CARTESIAN_POINT ( 'NONE',  ( -0.8267716535433065062, 0.1771653543307087630, 0.000000000000000000 ) ) ;
#45371=LINE ( 'NONE', #71066, #69663 ) ;
#45372=CARTESIAN_POINT ( 'NONE',  ( 1.246719160104987623, -0.4281496062992124485, 0.4176697321401328655 ) ) ;
#45373=CARTESIAN_POINT ( 'NONE',  ( 0.01149616601327405584, 2.739544932778246860E-15, 0.3791475997938225095 ) ) ;
#45376=CARTESIAN_POINT ( 'NONE',  ( -0.2242874410717133060, -4.005968212718139582E-15, 0.3627989612356165572 ) ) ;
#45377=CARTESIAN_POINT ( 'NONE',  ( 1.397637795275591177, -0.4536011799217367080, 0.2665933059059888421 ) ) ;
#45378=CARTESIAN_POINT ( 'NONE',  ( -1.430446194225721390, -0.4281496062992124485, 0.4176697321401328655 ) ) ;
#45379=CARTESIAN_POINT ( 'NONE',  ( 1.240157480314961314, -0.5400638737290844871, 0.3530559997133364547 ) ) ;
#45381=CARTESIAN_POINT ( 'NONE',  ( -1.614173228346456712, 0.8346805926620878280, -0.1372047244094478091 ) ) ;
#45382=EDGE_CURVE ( 'NONE', #4617, #27226, #61939, .T. ) ;
#45383=CARTESIAN_POINT ( 'NONE',  ( 0.5905511811023629321, 0.2952755905511811885, 0.000000000000000000 ) ) ;
#45384=CARTESIAN_POINT ( 'NONE',  ( -0.1509186351706028884, -0.3162353388693409650, -0.4822834645669289433 ) ) ;
#45385=CARTESIAN_POINT ( 'NONE',  ( -0.6758530183727027296, 0.2952755905511811885, 0.1292274648535926551 ) ) ;
#45386=CARTESIAN_POINT ( 'NONE',  ( 0.6561679790026253567, 0.1283753931104748280, 0.1820866141732283561 ) ) ;
#45390=ORIENTED_EDGE ( 'NONE', *, *, #79506, .F. ) ;
#45391=CARTESIAN_POINT ( 'NONE',  ( -0.1509186351706028884, -0.05778040916215522460, 0.4822834645669289988 ) ) ;
#45392=CARTESIAN_POINT ( 'NONE',  ( -1.587926509186350810, 0.05413385826771626580, -0.4176697321401330321 ) ) ;
#45393=CARTESIAN_POINT ( 'NONE',  ( 0.7086614173228353852, -0.1870078740157479769, 0.4822834645669291653 ) ) ;
#45394=CARTESIAN_POINT ( 'NONE',  ( 1.023622047244095334, -0.1870078740157479769, 0.4822834645669291653 ) ) ;
#45395=FACE_OUTER_BOUND ( 'NONE', #33529, .T. ) ;
#45396=CARTESIAN_POINT ( 'NONE',  ( -0.5249343832020990641, 0.2306618581243848609, 0.2411417322834645549 ) ) ;
#45397=CARTESIAN_POINT ( 'NONE',  ( 0.2165354330708668673, 0.1660481256975883668, -0.3530559997133364547 ) ) ;
#45398=CARTESIAN_POINT ( 'NONE',  ( 1.489501312335958172, -0.05778040916215560624, -0.4822834645669293319 ) ) ;
#45399=CARTESIAN_POINT ( 'NONE',  ( 1.292650918635171564, 0.2952755905511811885, 0.1292274648535926551 ) ) ;
#45400=EDGE_CURVE ( 'NONE', #36200, #16126, #31130, .T. ) ;
#45401=CARTESIAN_POINT ( 'NONE',  ( 1.030183727034121421, -0.05778040916215522460, 0.4822834645669289988 ) ) ;
#45402=CARTESIAN_POINT ( 'NONE',  ( -0.1312335958005241554, 0.2306618581243848609, 0.2411417322834645549 ) ) ;
#45404=CARTESIAN_POINT ( 'NONE',  ( 0.4658792650918641698, -0.08942795157528024563, -0.3641732283464568787 ) ) ;
#45405=ORIENTED_EDGE ( 'NONE', *, *, #37854, .T. ) ;
#45408=CARTESIAN_POINT ( 'NONE',  ( -0.3871391076115479057, -0.2845877964562161244, -0.3641732283464567121 ) ) ;
#45410=CARTESIAN_POINT ( 'NONE',  ( 0.2690288713910767848, -0.6692913385826773087, -0.1292274648535924053 ) ) ;
#45411=CARTESIAN_POINT ( 'NONE',  ( -0.1902887139107604098, -0.6692913385826771977, 0.1292274648535927661 ) ) ;
#45412=CARTESIAN_POINT ( 'NONE',  ( -0.8530183727034112984, -0.4281496062992127816, -0.4176697321401328100 ) ) ;
#45414=CARTESIAN_POINT ( 'NONE',  ( -1.581364829396324945, -0.05778040916215560624, -0.4822834645669293319 ) ) ;
#45415=CARTESIAN_POINT ( 'NONE',  ( -0.1455472725388424760, -1.150887559458346504E-15, 0.3627985898453522928 ) ) ;
#45416=CARTESIAN_POINT ( 'NONE',  ( 1.062992125984252745, -0.5511811023622047445, 6.969142054262312111E-17 ) ) ;
#45417=CARTESIAN_POINT ( 'NONE',  ( 0.3149606299212606708, -0.1870078740157480879, -0.4822834645669291653 ) ) ;
#45418=CARTESIAN_POINT ( 'NONE',  ( 0.7808398950131241190, -0.05778040916215560624, -0.4822834645669293319 ) ) ;
#45423=CARTESIAN_POINT ( 'NONE',  ( -0.1509186351706028884, -0.05778040916215522460, 0.4822834645669289988 ) ) ;
#45426=CARTESIAN_POINT ( 'NONE',  ( -1.410761154855641575, -0.2845877964562161244, -0.3641732283464567121 ) ) ;
#45427=CARTESIAN_POINT ( 'NONE',  ( 1.135170603674541256, 0.2952755905511811885, 0.1292274648535926551 ) ) ;
#45428=VECTOR ( 'NONE', #38649, 39.37007874015748143 ) ;
#45429=CARTESIAN_POINT ( 'NONE',  ( 1.450131233595801428, -0.6692913385826773087, -0.1292274648535924053 ) ) ;
#45430=CARTESIAN_POINT ( 'NONE',  ( 0.2362204724409456558, -0.1870078740157479769, 0.3641732283464567677 ) ) ;
#45431=CARTESIAN_POINT ( 'NONE',  ( 0.3937007874015754361, -0.1870078740157480879, -0.4822834645669291653 ) ) ;
#45433=CARTESIAN_POINT ( 'NONE',  ( 0.3608923884514443348, -0.5511811023622046335, 0.09757992244046803654 ) ) ;
#45434=CARTESIAN_POINT ( 'NONE',  ( 0.09842519685039434474, -0.5400638737290845981, -0.3530559997133363437 ) ) ;
#45436=CARTESIAN_POINT ( 'NONE',  ( -1.397637795275589623, 0.1660481256975885056, 0.3530559997133364547 ) ) ;
#45437=CARTESIAN_POINT ( 'NONE',  ( 0.5708661417322841158, -0.4536011799217368745, -0.2665933059059886201 ) ) ;
#45439=CARTESIAN_POINT ( 'NONE',  ( -0.6627296587926503335, -0.6692913385826771977, 0.1292274648535927661 ) ) ;
#45440=CARTESIAN_POINT ( 'NONE',  ( -0.3412073490813641308, 0.1283753931104746893, -0.1820866141732285504 ) ) ;
#45441=CARTESIAN_POINT ( 'NONE',  ( -0.7345763329969765554, 1.945772889739036060, -0.5309055118110235227 ) ) ;
#45442=CARTESIAN_POINT ( 'NONE',  ( -0.9055118110236215490, 0.2952755905511811885, 0.000000000000000000 ) ) ;
#45443=CARTESIAN_POINT ( 'NONE',  ( -0.08530183727034056085, -0.3162353388693405765, 0.4822834645669290543 ) ) ;
#45444=CARTESIAN_POINT ( 'NONE',  ( 0.2559055118110243332, -0.4536011799217368745, -0.2665933059059886201 ) ) ;
#45446=CARTESIAN_POINT ( 'NONE',  ( 0.07874015748031558404, -0.1870078740157479769, 0.4822834645669291653 ) ) ;
#45448=CARTESIAN_POINT ( 'NONE',  ( 0.7020997375328090762, -0.2845877964562159024, 0.3641732283464567677 ) ) ;
#45449=CARTESIAN_POINT ( 'NONE',  ( 1.286089238845145033, 0.2306618581243848609, 0.2411417322834645549 ) ) ;
#45450=CARTESIAN_POINT ( 'NONE',  ( -0.6430446194225716283, -0.3690944881889763329, 0.3153832671262228327 ) ) ;
#45451=CARTESIAN_POINT ( 'NONE',  ( -1.325459317585300889, -0.3690944881889765550, -0.3153832671262227771 ) ) ;
#45452=CARTESIAN_POINT ( 'NONE',  ( -0.5774278215223089816, -0.6046776061558807314, 0.2411417322834647770 ) ) ;
#45453=CARTESIAN_POINT ( 'NONE',  ( 0.04593175853018440641, 0.2952755905511810774, -0.1292274648535930714 ) ) ;
#45454=CARTESIAN_POINT ( 'NONE',  ( 0.4265091863517067594, 0.1771653543307087630, 0.09757992244046791164 ) ) ;
#45456=CARTESIAN_POINT ( 'NONE',  ( 1.187664041994751285, -0.2845877964562161244, -0.3641732283464567121 ) ) ;
#45457=ADVANCED_FACE ( 'NONE', ( #35106 ), #63563, .F. ) ;
#45458=CARTESIAN_POINT ( 'NONE',  ( 0.2887139107611556010, 0.2306618581243847221, -0.2411417322834647770 ) ) ;
#45460=CARTESIAN_POINT ( 'NONE',  ( -0.2230971128608915943, -0.4281496062992127816, -0.4176697321401328100 ) ) ;
#45462=CARTESIAN_POINT ( 'NONE',  ( 1.548556430446194954, -0.5023911411419708095, 0.1820866141732285504 ) ) ;
#45463=CARTESIAN_POINT ( 'NONE',  ( 0.2690288713910767848, 0.2952755905511811885, 0.1292274648535926551 ) ) ;
#45464=CARTESIAN_POINT ( 'NONE',  ( 0.2821522309711292364, 0.2952755905511810774, -0.1292274648535930714 ) ) ;
#45465=CARTESIAN_POINT ( 'NONE',  ( 0.5774278215223104249, 0.1539470093639523085, 0.1968503937007873850 ) ) ;
#45466=CARTESIAN_POINT ( 'NONE',  ( 0.07217847769028949700, -0.2845877964562159024, 0.3641732283464567677 ) ) ;
#45467=CARTESIAN_POINT ( 'NONE',  ( 0.9776902887139113929, -0.6692913385826773087, -0.1292274648535924053 ) ) ;
#45468=CARTESIAN_POINT ( 'NONE',  ( -0.1771653543307080136, -0.4536011799217367080, 0.2665933059059888421 ) ) ;
#45469=CARTESIAN_POINT ( 'NONE',  ( -0.8136482939632537770, 0.2306618581243847221, -0.2411417322834647770 ) ) ;
#45471=CARTESIAN_POINT ( 'NONE',  ( -0.2493438320209966919, 0.05413385826771626580, -0.4176697321401330321 ) ) ;
#45472=APPLICATION_CONTEXT ( 'automotive_design' ) ;
#45473=CARTESIAN_POINT ( 'NONE',  ( -1.240157480314959759, -0.5400638737290845981, -0.3530559997133363437 ) ) ;
#45474=CARTESIAN_POINT ( 'NONE',  ( -0.7874015748031489847, -0.1870078740157479769, 0.3641732283464567677 ) ) ;
#45475=CARTESIAN_POINT ( 'NONE',  ( 0.3280839895013130669, 0.05413385826771666132, 0.4176697321401328100 ) ) ;
#45476=CARTESIAN_POINT ( 'NONE',  ( -1.246719160104986512, 0.05413385826771666132, 0.4176697321401328100 ) ) ;
#45477=CARTESIAN_POINT ( 'NONE',  ( -0.1574803149606292529, -0.1870078740157480879, -0.4822834645669291653 ) ) ;
#45480=CARTESIAN_POINT ( 'NONE',  ( 1.404199475065617264, -0.4281496062992124485, 0.4176697321401328655 ) ) ;
#45481=CARTESIAN_POINT ( 'NONE',  ( 1.305774278215223960, -0.6692913385826771977, 0.1292274648535927661 ) ) ;
#45484=CARTESIAN_POINT ( 'NONE',  ( -1.122047244094487306, -0.5400638737290844871, 0.3530559997133364547 ) ) ;
#45488=CARTESIAN_POINT ( 'NONE',  ( 0.07217847769028949700, -0.2845877964562159024, 0.3641732283464567677 ) ) ;
#45490=ORIENTED_EDGE ( 'NONE', *, *, #11466, .T. ) ;
#45491=CARTESIAN_POINT ( 'NONE',  ( 0.2952755905511816326, -0.5400638737290844871, 0.3530559997133364547 ) ) ;
#45492=CARTESIAN_POINT ( 'NONE',  ( 0.3543307086614179147, 0.2952755905511811885, 0.000000000000000000 ) ) ;
#45495=CARTESIAN_POINT ( 'NONE',  ( -0.9251968503937002541, -0.4536011799217368745, -0.2665933059059886201 ) ) ;
#45497=CARTESIAN_POINT ( 'NONE',  ( 0.9251968503937015864, 0.1660481256975883668, -0.3530559997133364547 ) ) ;
#45498=CARTESIAN_POINT ( 'NONE',  ( 1.089238845144357537, -0.3690944881889763329, 0.3153832671262228327 ) ) ;
#45499=CARTESIAN_POINT ( 'NONE',  ( -0.2690288713910754526, -0.6692913385826771977, 0.1292274648535927661 ) ) ;
#45501=CARTESIAN_POINT ( 'NONE',  ( -0.6824146981627288167, 0.2306618581243848609, 0.2411417322834645549 ) ) ;
#45502=CARTESIAN_POINT ( 'NONE',  ( -1.207349081364828880, 0.1283753931104746893, -0.1820866141732285504 ) ) ;
#45503=CARTESIAN_POINT ( 'NONE',  ( -0.8136482939632537770, -0.6046776061558807314, 0.2411417322834647770 ) ) ;
#45504=CARTESIAN_POINT ( 'NONE',  ( 1.450131233595801428, -0.6692913385826773087, -0.1292274648535924053 ) ) ;
#45505=CARTESIAN_POINT ( 'NONE',  ( 1.673228346456693494, 0.07958543189024085140, 0.2665933059059887866 ) ) ;
#45508=CARTESIAN_POINT ( 'NONE',  ( 0.1049868766404206816, 0.2306618581243848609, 0.2411417322834645549 ) ) ;
#45510=CARTESIAN_POINT ( 'NONE',  ( -0.6102362204724400829, 0.1660481256975885056, 0.3530559997133364547 ) ) ;
#45511=CARTESIAN_POINT ( 'NONE',  ( 1.423884514435696191, -0.05778040916215522460, 0.4822834645669289988 ) ) ;
#45512=CARTESIAN_POINT ( 'NONE',  ( 1.417322834645670104, -0.1870078740157479769, 0.4822834645669291653 ) ) ;
#45513=ADVANCED_FACE ( 'NONE', ( #28789 ), #38829, .F. ) ;
#45514=CARTESIAN_POINT ( 'NONE',  ( 0.1968503937007881344, 0.2952755905511811885, 0.000000000000000000 ) ) ;
#45515=CARTESIAN_POINT ( 'NONE',  ( -0.02624671916010428221, 0.2306618581243847221, -0.2411417322834647770 ) ) ;
#45517=CARTESIAN_POINT ( 'NONE',  ( -1.030183727034119867, -0.05778040916215560624, -0.4822834645669293319 ) ) ;
#45518=CARTESIAN_POINT ( 'NONE',  ( -0.1837270341207340729, 0.2306618581243847221, -0.2411417322834647770 ) ) ;
#45519=EDGE_CURVE ( 'NONE', #38656, #4617, #21170, .T. ) ;
#45520=CARTESIAN_POINT ( 'NONE',  ( -0.03280839895013062252, 0.1771653543307087075, -0.09757992244046823083 ) ) ;
#45521=CARTESIAN_POINT ( 'NONE',  ( 1.299212598425197429, -0.6692913385826771977, 8.415575281601705876E-17 ) ) ;
#45522=CARTESIAN_POINT ( 'NONE',  ( -0.4068241469816267775, 0.05413385826771626580, -0.4176697321401330321 ) ) ;
#45524=CARTESIAN_POINT ( 'NONE',  ( 0.9973753280839902091, 0.2306618581243847221, -0.2411417322834647770 ) ) ;
#45525=DIRECTION ( 'NONE',  ( -3.096699300667737957E-16, 1.000000000000000000, -0.000000000000000000 ) ) ;
#45526=ORIENTED_EDGE ( 'NONE', *, *, #69939, .F. ) ;
#45528=CARTESIAN_POINT ( 'NONE',  ( 0.3805774278215230400, -0.4281496062992124485, 0.4176697321401328655 ) ) ;
#45529=CARTESIAN_POINT ( 'NONE',  ( -0.2559055118110230564, 0.07958543189024071263, -0.2665933059059888421 ) ) ;
#45530=CARTESIAN_POINT ( 'NONE',  ( 1.384514435695538559, 0.1771653543307087075, -0.09757992244046823083 ) ) ;
#45533=CARTESIAN_POINT ( 'NONE',  ( 1.614173228346457378, 1.330640075373405118, -0.1372047244094476148 ) ) ;
#45534=CARTESIAN_POINT ( 'NONE',  ( 1.233595800524935227, -0.6046776061558807314, 0.2411417322834647770 ) ) ;
#45536=CARTESIAN_POINT ( 'NONE',  ( 0.02624671916010564918, 0.2306618581243848609, 0.2411417322834645549 ) ) ;
#45538=CARTESIAN_POINT ( 'NONE',  ( -1.653543307086613234, -0.1870078740157480879, -0.4822834645669291653 ) ) ;
#45539=CARTESIAN_POINT ( 'NONE',  ( -0.1049868766404193215, 0.2306618581243847221, -0.2411417322834647770 ) ) ;
#45541=CARTESIAN_POINT ( 'NONE',  ( 1.581364829396326277, -0.3162353388693409650, -0.4822834645669289433 ) ) ;
#45542=CARTESIAN_POINT ( 'NONE',  ( 0.3346456692913390985, 0.1660481256975885056, 0.3530559997133364547 ) ) ;
#45543=CARTESIAN_POINT ( 'NONE',  ( 1.049868766404200349, 0.1283753931104748280, 0.1820866141732283561 ) ) ;
#45545=CARTESIAN_POINT ( 'NONE',  ( 0.9580052493438327987, -0.3690944881889765550, -0.3153832671262227771 ) ) ;
#45546=CARTESIAN_POINT ( 'NONE',  ( -1.410761154855641575, -0.3162353388693409650, -0.4822834645669289433 ) ) ;
#45549=CARTESIAN_POINT ( 'NONE',  ( 1.299212598425197429, -0.6692913385826771977, 8.415575281601705876E-17 ) ) ;
#45551=CARTESIAN_POINT ( 'NONE',  ( 0.8530183727034128527, -0.4281496062992124485, 0.4176697321401328655 ) ) ;
#45554=CARTESIAN_POINT ( 'NONE',  ( 0.2427821522309716595, -0.2845877964562161244, -0.3641732283464567121 ) ) ;
#45555=EDGE_CURVE ( 'NONE', #28439, #42372, #43195, .T. ) ;
#45556=CARTESIAN_POINT ( 'NONE',  ( 0.5774278215223104249, 0.2306618581243848609, 0.2411417322834645549 ) ) ;
#45557=CARTESIAN_POINT ( 'NONE',  ( 1.614173228346457378, 0.5038684218300975015, 0.1372047244094478369 ) ) ;
#45558=CARTESIAN_POINT ( 'NONE',  ( -0.9514435695538050464, -0.2845877964562159024, 0.3641732283464567677 ) ) ;
#45559=CARTESIAN_POINT ( 'NONE',  ( -0.9055118110236215490, 0.2952755905511811885, 0.000000000000000000 ) ) ;
#45560=CARTESIAN_POINT ( 'NONE',  ( 1.010498687664042716, -0.4281496062992124485, 0.4176697321401328655 ) ) ;
#45561=CARTESIAN_POINT ( 'NONE',  ( -1.135170603674539924, -0.6692913385826771977, 0.1292274648535927661 ) ) ;
#45562=CARTESIAN_POINT ( 'NONE',  ( 1.076115485564305141, 0.2306618581243847221, -0.2411417322834647770 ) ) ;
#45563=CARTESIAN_POINT ( 'NONE',  ( -1.246719160104985846, -0.3690944881889765550, -0.3153832671262227771 ) ) ;
#45565=CARTESIAN_POINT ( 'NONE',  ( -1.646051170424378096, 0.000000000000000000, 0.3464511005275205946 ) ) ;
#45566=CARTESIAN_POINT ( 'NONE',  ( 1.115485564304462551, 0.05413385826771666132, 0.4176697321401328100 ) ) ;
#45569=CARTESIAN_POINT ( 'NONE',  ( 1.594488188976378673, -0.5400638737290845981, -0.3530559997133363437 ) ) ;
#45570=CARTESIAN_POINT ( 'NONE',  ( -1.305774278215222184, -0.5511811023622048555, -0.09757992244046775898 ) ) ;
#45571=( BOUNDED_SURFACE ( )  B_SPLINE_SURFACE ( 1, 2, ( 
 ( #23085, #48752, #74451, #16797, #43251, #42434, #80365, #48337, #36957, #4978, #68134, #10479, #74034, #16381, #42027, #10057, #37778, #57121, #76509, #77333, #70593, #76914, #82815, #7040, #12527, #83229, #31878, #57949, #38188, #25970, #69776, #25139, #317, #31459, #39016, #51629, #63863, #6200, #32709, #52053, #63454, #50808, #64700, #57538, #12947, #58375, #13785, #25550, #12120, #19662, #26395, #45324, #77758, #20091, #71437, #5789, #738, #45741, #71019, #56714, #13363, #39441, #51217, #65129, #38605, #19243, #64283, #18838, #82412, #50399, #44894, #18440, #6618, #31045, #32289, #24731, #76096, #44082, #44483, #70175, #58804, #1162, #42647, #40279, #26813, #79021, #67509, #74663, #52471, #20510, #29201, #74245, #21340, #14625, #41818, #54867, #67927, #71859, #65962, #9845, #27646, #7464, #35517, #8298, #72278, #61180, #39865, #10268, #46163, #52889, #16587, #27229, #14209, #3534, #3948, #48547, #80573, #72686, #80980, #22883, #53308, #61605, #35936, #42233, #7887, #29609, #55269, #46993, #15034, #65556, #48963, #59628, #78179, #1983, #33134, #23292, #17007, #33966, #78601, #33551, #59213, #1574, #20925, #46580, #43459, #51010, #4350, #31670, #25348, #63660, #75072, #30435, #50601, #76308, #36745, #55682, #76709, #36339, #6001, #17419, #62013, #4759, #30017, #57331, #82615, #5180, #44283, #37985, #81389, #56509, #23705, #82211, #62422, #18639, #19042, #43050, #75486, #68344, #83025, #49376, #10684, #11089, #30844, #43873, #68746, #56100, #81804, #5586, #69973, #24530, #17826, #18233, #31253, #12327, #24116, #69157, #69571, #50195, #49785, #11919, #11508, #37164, #37574, #62844, #75893, #63247, #56920, #24931, #64494, #51425, #39659, #40080, #1373, #77973, #26615, #33764, #33354, #7254, #14428, #72069, #52685, #45111, #27024, #20303, #961, #52268, #19461, #1781, #13578, #64080, #39232, #78811, #78393, #58592, #51848, #6832, #65767, #45953, #77555, #71234, #71650, #19888, #45536, #25764, #65349, #8099, #59017, #59426, #27440, #53102, #58165, #20724, #64917, #44689, #14001, #7687, #46376, #77127, #32086, #70385, #70818, #12741, #38400, #32927, #533, #6417, #57747, #109, #13166, #38816, #32502, #26187, #34602, #73743, #29513, #79232, #66590, #40908, #54352, #53935, #21964, #16496, #72486, #48042, #8925, #8513, #60267, #80064, #67008, #79647, #59844, #22789, #21547, #2617, #47208, #3025, #15249, #66175, #34179, #10174, #35423, #67418, #47624, #2196, #74149, #21140, #14835, #9341, #27864, #16079, #53524, #72898, #41724, #9751, #73320, #28273, #60676, #35839, #54773, #55174, #15666, #40495, #35012, #41328, #61088, #46795, #28691, #22382, #3439, #29102, #80477, #48449, #42140, #67835, #61507, #3853, #68253, #17325, #30752, #43357, #55999, #36245, #82518, #55582, #42954, #23608, #62748, #74980, #42550, #10588, #69879, #11826, #43769, #81710, #61914, #50503, #80883, #74566, #69057, #4256, #75793, #29919, #5899, #37479, #76207, #11407, #56820, #63151, #5083, #18544, #81293, #24020, #12232, #49277, #68648, #10986, #36647, #62322, #37063, #4659, #23196, #63565, #82114, #69473, #30333, #49688, #5492, #56415, #31153, #24428, #75381, #17729, #50097, #24834, #18135, #44188, #37889, #31571, #48867, #16912, #58064, #856, #38717, #52167, #12640, #12, #26513, #57650, #65245, #77871, #6731, #32401, #58917, #78293, #6312, #25665, #7583, #431, #31989, #20201, #19362, #64395, #38300, #45851, #52584, #71550, #20625, #46276, #14326, #70711, #33255, #26086, #26925, #32824, #7153, #39557, #63976, #44593, #1276, #77030, #71972, #58491, #51746, #13899, #39984, #65674, #76615, #18945, #8001, #57228, #82929, #51326, #45011, #25251, #50915, #13063, #70288, #77449, #19783, #45436, #71131, #13474, #39131, #64812, #80379, #47940, #53833, #9656, #3338, #27342, #21860, #53000, #47525, #2096, #41632, #16396, #40393, #40804, #42042, #29002, #14740, #74048, #59742, #79547, #66075, #67322, #22692, #54251, #59327, #22280, #54668, #66488, #35326, #73216, #34500, #41226, #27761, #1683, #78713, #15566, #21038, #8823, #33665, #60165, #2518, #28176, #73643, #66913, #67738, #46697, #72390 ),
 ( #48351, #8411, #34079, #53426, #79134, #21451, #9245, #47108, #72798, #15147, #34917, #15985, #60579, #2930, #60989, #28594, #79967, #36971, #16813, #36147, #55486, #56323, #49596, #55903, #61819, #69380, #74884, #62230, #10894, #62651, #17230, #4992, #48767, #4159, #30660, #10493, #18044, #82022, #42860, #68553, #11734, #75290, #29824, #55075, #80783, #82426, #24335, #50005, #36554, #74466, #63061, #10071, #3752, #81615, #23099, #75702, #42449, #18454, #43677, #5398, #23929, #37389, #31061, #17633, #56729, #68149, #4569, #24746, #81197, #23512, #49181, #30240, #43265, #68962, #11312, #35735, #76113, #50413, #44097, #61403, #29416, #52067, #32304, #32725, #13379, #76525, #12544, #31892, #58393, #25986, #57965, #38203, #45756, #51232, #38620, #70608, #39032, #76931, #64716, #25155, #63877, #7057, #70190, #77774, #753, #19258, #44911, #71452, #7482, #18853, #6216, #20107, #12963, #44500, #26414, #57553, #64298, #50823, #13800, #65146, #39458, #33152, #58821, #26829, #83244, #1178, #6632, #52487, #45339, #19680, #78195, #25566, #57136, #20526, #332, #69790, #12136, #51645, #77349, #71035, #37792, #63470, #5804, #31475, #82833, #34398, #59642, #15468, #54569, #20940, #8314, #65977, #79443, #79036, #47008, #41538, #14224, #73116, #33981, #33566, #1999, #21762, #8728, #21355, #1589, #47840, #46598, #27661, #72294, #60066, #40296, #71875, #28906, #47425, #34821, #52903, #14640, #28491, #2420, #9149, #41125, #78617, #53327, #72702, #60479, #28077, #53735, #15049, #22183, #40705, #66389, #66816, #2830, #54151, #79865, #27244, #73546, #15889, #67226, #9557, #35227, #60891, #3241, #80283, #46178, #39884, #65571, #7905, #59228, #80691, #17536, #68049, #29729, #3659, #43168, #17944, #11213, #69282, #11628, #62964, #36053, #30560, #55391, #75605, #81509, #55803, #4886, #29322, #9970, #56226, #48670, #75192, #49499, #81097, #61725, #62132, #37289, #81924, #56628, #67638, #41942, #10798, #4062, #68864, #30961, #23004, #10396, #42351, #23831, #23414, #49081, #43580, #73953, #36872, #74781, #35641, #17132, #62550, #68460, #42764, #61301, #24235, #74367, #36458, #16710, #4472, #30140, #54983, #49908, #5302, #22596, #48257, #16299, #37691, #51962, #82329, #76012, #44807, #69691, #77244, #63366, #7367, #38931, #77669, #12861, #58281, #13279, #6535, #19999, #57036, #57451, #71345, #5700, #82731, #25050, #50725, #31372, #64611, #45234, #83144, #76423, #45650, #24647, #18354, #70502, #12034, #19574, #18752, #33037, #6948, #13692, #38518, #646, #32619, #32205, #39347, #44396, #25463, #65032, #70088, #12442, #38101, #63776, #6116, #64201, #31788, #50314, #43997, #229, #70934, #51130, #76824, #26303, #57862, #19157, #25880, #51541, #1482, #20833, #21658, #14943, #21247, #27136, #34714, #40190, #27555, #59539, #2311, #65874, #53630, #14116, #52801, #27972, #59125, #66707, #79338, #8209, #33874, #60375, #79758, #7797, #78510, #9040, #1895, #33463, #47318, #46486, #53214, #39769, #73009, #54044, #15360, #22075, #47734, #15782, #72181, #2723, #78925, #28384, #34295, #8624, #41021, #65464, #46071, #73432, #14539, #41434, #67117, #46902, #72596, #40602, #9448, #58705, #1071, #20418, #78087, #66285, #59956, #26724, #52378, #71763, #80591, #54886, #68364, #67945, #35954, #30454, #3138, #62033, #22899, #22493, #48566, #10702, #80998, #10287, #73851, #36766, #9866, #74264, #61197, #17026, #29219, #80178, #48156, #24134, #16192, #30038, #56118, #23725, #81824, #49804, #75505, #16607, #43068, #42250, #4778, #36358, #4369, #17438, #41838, #67528, #68765, #3554, #55700, #81408, #61623, #3965, #74680, #17844, #11109, #69174, #35535, #54465, #23312, #29628, #49396, #43478, #55288, #48981, #42665, #75090, #62442, #35119, #60785, #28801, #39569, #31272, #82230, #56937, #45864, #58505, #69990, #50215, #14337, #69589, #82634, #37590, #77883, #5604, #56527, #24549, #1695, #26936, #58928, #12345, #75911, #65685, #11525, #5198, #868, #18250, #7595, #43892, #21050, #52598, #8012, #26526, #71984, #78304, #20215, #33676, #11935, #38001, #27353, #63263, #24947, #50620, #76325, #18655, #52180, #44299 ) ),
 .UNSPECIFIED., .F., .F., .F. ) 
 B_SPLINE_SURFACE_WITH_KNOTS ( ( 2, 2 ),
 ( 3, 2, 2, 2, 2, 2, 2, 2, 2, 2, 2, 2, 2, 2, 2, 2, 2, 2, 2, 2, 2, 2, 2, 2, 2, 2, 2, 2, 2, 2, 2, 2, 2, 2, 2, 2, 2, 2, 2, 2, 2, 2, 2, 2, 2, 2, 2, 2, 2, 2, 2, 2, 2, 2, 2, 2, 2, 2, 2, 2, 2, 2, 2, 2, 2, 2, 2, 2, 2, 2, 2, 2, 2, 2, 2, 2, 2, 2, 2, 2, 2, 2, 2, 2, 2, 2, 2, 2, 2, 2, 2, 2, 2, 2, 2, 2, 2, 2, 2, 2, 2, 2, 2, 2, 2, 2, 2, 2, 2, 2, 2, 2, 2, 2, 2, 2, 2, 2, 2, 2, 2, 2, 2, 2, 2, 2, 2, 2, 2, 2, 2, 2, 2, 2, 2, 2, 2, 2, 2, 2, 2, 2, 2, 2, 2, 2, 2, 2, 2, 2, 2, 2, 2, 2, 2, 2, 2, 2, 2, 2, 2, 2, 2, 2, 2, 2, 2, 2, 2, 2, 2, 2, 2, 2, 2, 2, 2, 2, 2, 2, 2, 2, 2, 2, 2, 2, 2, 2, 2, 2, 2, 2, 2, 2, 2, 2, 2, 2, 2, 2, 2, 2, 2, 2, 2, 2, 2, 2, 2, 2, 2, 2, 2, 2, 2, 2, 2, 2, 2, 2, 2, 2, 2, 2, 2, 2, 2, 2, 2, 2, 2, 2, 2, 2, 2, 2, 2, 2, 2, 2, 2, 2, 2, 2, 2, 2, 2, 2, 2, 2, 2, 2, 2, 2, 2, 3 ),
 ( 0.000000000000000000, 1.000000000000000000 ),
 ( 0.000000000000000000, 0.003787878787878787984, 0.007575757575757575968, 0.01136363636363636395, 0.01515151515151515194, 0.01893939393939393992, 0.02272727272727272790, 0.02651515151515151589, 0.03030303030303030387, 0.03409090909090908839, 0.03787878787878787984, 0.04166666666666666435, 0.04545454545454545581, 0.04924242424242424032, 0.05303030303030303177, 0.05681818181818181629, 0.06060606060606060774, 0.06439393939393939226, 0.06818181818181817677, 0.07196969696969697516, 0.07575757575757575968, 0.07954545454545454419, 0.08333333333333332871, 0.08712121212121212710, 0.09090909090909091161, 0.09469696969696969613, 0.09848484848484848064, 0.1022727272727272790, 0.1060606060606060635, 0.1098484848484848481, 0.1136363636363636326, 0.1174242424242424310, 0.1212121212121212155, 0.1250000000000000000, 0.1287878787878787845, 0.1325757575757575690, 0.1363636363636363535, 0.1401515151515151381, 0.1439393939393939503, 0.1477272727272727348, 0.1515151515151515194, 0.1553030303030303039, 0.1590909090909090884, 0.1628787878787878729, 0.1666666666666666574, 0.1704545454545454419, 0.1742424242424242542, 0.1780303030303030387, 0.1818181818181818232, 0.1856060606060606077, 0.1893939393939393923, 0.1931818181818181768, 0.1969696969696969613, 0.2007575757575757458, 0.2045454545454545581, 0.2083333333333333426, 0.2121212121212121271, 0.2159090909090909116, 0.2196969696969696961, 0.2234848484848484806, 0.2272727272727272652, 0.2310606060606060497, 0.2348484848484848619, 0.2386363636363636465, 0.2424242424242424310, 0.2462121212121212155, 0.2500000000000000000, 0.2537878787878787845, 0.2575757575757575690, 0.2613636363636363535, 0.2651515151515151381, 0.2689393939393939226, 0.2727272727272727071, 0.2765151515151514916, 0.2803030303030302761, 0.2840909090909091161, 0.2878787878787879007, 0.2916666666666666852, 0.2954545454545454697, 0.2992424242424242542, 0.3030303030303030387, 0.3068181818181818232, 0.3106060606060606077, 0.3143939393939393923, 0.3181818181818181768, 0.3219696969696969613, 0.3257575757575757458, 0.3295454545454545303, 0.3333333333333333148, 0.3371212121212120993, 0.3409090909090908839, 0.3446969696969697239, 0.3484848484848485084, 0.3522727272727272929, 0.3560606060606060774, 0.3598484848484848619, 0.3636363636363636465, 0.3674242424242424310, 0.3712121212121212155, 0.3750000000000000000, 0.3787878787878787845, 0.3825757575757575690, 0.3863636363636363535, 0.3901515151515151381, 0.3939393939393939226, 0.3977272727272727071, 0.4015151515151514916, 0.4053030303030302761, 0.4090909090909091161, 0.4128787878787879007, 0.4166666666666666852, 0.4204545454545454697, 0.4242424242424242542, 0.4280303030303030387, 0.4318181818181818232, 0.4356060606060606077, 0.4393939393939393923, 0.4431818181818181768, 0.4469696969696969613, 0.4507575757575757458, 0.4545454545454545303, 0.4583333333333333148, 0.4621212121212120993, 0.4659090909090908839, 0.4696969696969697239, 0.4734848484848485084, 0.4772727272727272929, 0.4810606060606060774, 0.4848484848484848619, 0.4886363636363636465, 0.4924242424242424310, 0.4962121212121212155, 0.5000000000000000000, 0.5037878787878787845, 0.5075757575757575690, 0.5113636363636363535, 0.5151515151515151381, 0.5189393939393939226, 0.5227272727272727071, 0.5265151515151514916, 0.5303030303030302761, 0.5340909090909090606, 0.5378787878787878451, 0.5416666666666666297, 0.5454545454545454142, 0.5492424242424241987, 0.5530303030303029832, 0.5568181818181817677, 0.5606060606060605522, 0.5643939393939394478, 0.5681818181818182323, 0.5719696969696970168, 0.5757575757575758013, 0.5795454545454545858, 0.5833333333333333703, 0.5871212121212121549, 0.5909090909090909394, 0.5946969696969697239, 0.5984848484848485084, 0.6022727272727272929, 0.6060606060606060774, 0.6098484848484848619, 0.6136363636363636465, 0.6174242424242424310, 0.6212121212121212155, 0.6250000000000000000, 0.6287878787878787845, 0.6325757575757575690, 0.6363636363636363535, 0.6401515151515151381, 0.6439393939393939226, 0.6477272727272727071, 0.6515151515151514916, 0.6553030303030302761, 0.6590909090909090606, 0.6628787878787878451, 0.6666666666666666297, 0.6704545454545454142, 0.6742424242424241987, 0.6780303030303029832, 0.6818181818181817677, 0.6856060606060605522, 0.6893939393939394478, 0.6931818181818182323, 0.6969696969696970168, 0.7007575757575758013, 0.7045454545454545858, 0.7083333333333333703, 0.7121212121212121549, 0.7159090909090909394, 0.7196969696969697239, 0.7234848484848485084, 0.7272727272727272929, 0.7310606060606060774, 0.7348484848484848619, 0.7386363636363636465, 0.7424242424242424310, 0.7462121212121212155, 0.7500000000000000000, 0.7537878787878787845, 0.7575757575757575690, 0.7613636363636363535, 0.7651515151515151381, 0.7689393939393939226, 0.7727272727272727071, 0.7765151515151514916, 0.7803030303030302761, 0.7840909090909090606, 0.7878787878787878451, 0.7916666666666666297, 0.7954545454545454142, 0.7992424242424241987, 0.8030303030303029832, 0.8068181818181817677, 0.8106060606060605522, 0.8143939393939394478, 0.8181818181818182323, 0.8219696969696970168, 0.8257575757575758013, 0.8295454545454545858, 0.8333333333333333703, 0.8371212121212121549, 0.8409090909090909394, 0.8446969696969697239, 0.8484848484848485084, 0.8522727272727272929, 0.8560606060606060774, 0.8598484848484848619, 0.8636363636363636465, 0.8674242424242424310, 0.8712121212121212155, 0.8750000000000000000, 0.8787878787878787845, 0.8825757575757575690, 0.8863636363636363535, 0.8901515151515151381, 0.8939393939393939226, 0.8977272727272727071, 0.9015151515151514916, 0.9053030303030302761, 0.9090909090909090606, 0.9128787878787878451, 0.9166666666666666297, 0.9204545454545454142, 0.9242424242424241987, 0.9280303030303029832, 0.9318181818181817677, 0.9356060606060605522, 0.9393939393939394478, 0.9431818181818182323, 0.9469696969696970168, 0.9507575757575758013, 0.9545454545454545858, 0.9583333333333333703, 0.9621212121212121549, 0.9659090909090909394 ),
 .UNSPECIFIED. ) 
 GEOMETRIC_REPRESENTATION_ITEM ( )  RATIONAL_B_SPLINE_SURFACE ( (
 ( 1.000000000000000000, 0.9659258262890683122, 1.000000000000000000, 0.9659258262890683122, 1.000000000000000000, 0.9659258262890683122, 1.000000000000000000, 0.9659258262890683122, 1.000000000000000000, 0.9659258262890683122, 1.000000000000000000, 0.9659258262890683122, 1.000000000000000000, 0.9659258262890683122, 1.000000000000000000, 0.9659258262890683122, 1.000000000000000000, 0.9659258262890683122, 1.000000000000000000, 0.9659258262890683122, 1.000000000000000000, 0.9659258262890683122, 1.000000000000000000, 0.9659258262890683122, 1.000000000000000000, 0.9659258262890683122, 1.000000000000000000, 0.9659258262890683122, 1.000000000000000000, 0.9659258262890683122, 1.000000000000000000, 0.9659258262890683122, 1.000000000000000000, 0.9659258262890683122, 1.000000000000000000, 0.9659258262890683122, 1.000000000000000000, 0.9659258262890683122, 1.000000000000000000, 0.9659258262890683122, 1.000000000000000000, 0.9659258262890683122, 1.000000000000000000, 0.9659258262890683122, 1.000000000000000000, 0.9659258262890683122, 1.000000000000000000, 0.9659258262890683122, 1.000000000000000000, 0.9659258262890683122, 1.000000000000000000, 0.9659258262890683122, 1.000000000000000000, 0.9659258262890683122, 1.000000000000000000, 0.9659258262890683122, 1.000000000000000000, 0.9659258262890683122, 1.000000000000000000, 0.9659258262890683122, 1.000000000000000000, 0.9659258262890683122, 1.000000000000000000, 0.9659258262890683122, 1.000000000000000000, 0.9659258262890683122, 1.000000000000000000, 0.9659258262890683122, 1.000000000000000000, 0.9659258262890683122, 1.000000000000000000, 0.9659258262890683122, 1.000000000000000000, 0.9659258262890683122, 1.000000000000000000, 0.9659258262890683122, 1.000000000000000000, 0.9659258262890683122, 1.000000000000000000, 0.9659258262890683122, 1.000000000000000000, 0.9659258262890683122, 1.000000000000000000, 0.9659258262890683122, 1.000000000000000000, 0.9659258262890683122, 1.000000000000000000, 0.9659258262890683122, 1.000000000000000000, 0.9659258262890683122, 1.000000000000000000, 0.9659258262890683122, 1.000000000000000000, 0.9659258262890683122, 1.000000000000000000, 0.9659258262890683122, 1.000000000000000000, 0.9659258262890683122, 1.000000000000000000, 0.9659258262890683122, 1.000000000000000000, 0.9659258262890683122, 1.000000000000000000, 0.9659258262890683122, 1.000000000000000000, 0.9659258262890683122, 1.000000000000000000, 0.9659258262890683122, 1.000000000000000000, 0.9659258262890683122, 1.000000000000000000, 0.9659258262890683122, 1.000000000000000000, 0.9659258262890683122, 1.000000000000000000, 0.9659258262890683122, 1.000000000000000000, 0.9659258262890683122, 1.000000000000000000, 0.9659258262890683122, 1.000000000000000000, 0.9659258262890683122, 1.000000000000000000, 0.9659258262890683122, 1.000000000000000000, 0.9659258262890683122, 1.000000000000000000, 0.9659258262890683122, 1.000000000000000000, 0.9659258262890683122, 1.000000000000000000, 0.9659258262890683122, 1.000000000000000000, 0.9659258262890683122, 1.000000000000000000, 0.9659258262890683122, 1.000000000000000000, 0.9659258262890683122, 1.000000000000000000, 0.9659258262890683122, 1.000000000000000000, 0.9659258262890683122, 1.000000000000000000, 0.9659258262890683122, 1.000000000000000000, 0.9659258262890683122, 1.000000000000000000, 0.9659258262890683122, 1.000000000000000000, 0.9659258262890683122, 1.000000000000000000, 0.9659258262890683122, 1.000000000000000000, 0.9659258262890683122, 1.000000000000000000, 0.9659258262890683122, 1.000000000000000000, 0.9659258262890683122, 1.000000000000000000, 0.9659258262890683122, 1.000000000000000000, 0.9659258262890683122, 1.000000000000000000, 0.9659258262890683122, 1.000000000000000000, 0.9659258262890683122, 1.000000000000000000, 0.9659258262890683122, 1.000000000000000000, 0.9659258262890683122, 1.000000000000000000, 0.9659258262890683122, 1.000000000000000000, 0.9659258262890683122, 1.000000000000000000, 0.9659258262890683122, 1.000000000000000000, 0.9659258262890683122, 1.000000000000000000, 0.9659258262890683122, 1.000000000000000000, 0.9659258262890683122, 1.000000000000000000, 0.9659258262890683122, 1.000000000000000000, 0.9659258262890683122, 1.000000000000000000, 0.9659258262890683122, 1.000000000000000000, 0.9659258262890683122, 1.000000000000000000, 0.9659258262890683122, 1.000000000000000000, 0.9659258262890683122, 1.000000000000000000, 0.9659258262890683122, 1.000000000000000000, 0.9659258262890683122, 1.000000000000000000, 0.9659258262890683122, 1.000000000000000000, 0.9659258262890683122, 1.000000000000000000, 0.9659258262890683122, 1.000000000000000000, 0.9659258262890683122, 1.000000000000000000, 0.9659258262890683122, 1.000000000000000000, 0.9659258262890683122, 1.000000000000000000, 0.9659258262890683122, 1.000000000000000000, 0.9659258262890683122, 1.000000000000000000, 0.9659258262890683122, 1.000000000000000000, 0.9659258262890683122, 1.000000000000000000, 0.9659258262890683122, 1.000000000000000000, 0.9659258262890683122, 1.000000000000000000, 0.9659258262890683122, 1.000000000000000000, 0.9659258262890683122, 1.000000000000000000, 0.9659258262890683122, 1.000000000000000000, 0.9659258262890683122, 1.000000000000000000, 0.9659258262890683122, 1.000000000000000000, 0.9659258262890683122, 1.000000000000000000, 0.9659258262890683122, 1.000000000000000000, 0.9659258262890683122, 1.000000000000000000, 0.9659258262890683122, 1.000000000000000000, 0.9659258262890683122, 1.000000000000000000, 0.9659258262890683122, 1.000000000000000000, 0.9659258262890683122, 1.000000000000000000, 0.9659258262890683122, 1.000000000000000000, 0.9659258262890683122, 1.000000000000000000, 0.9659258262890683122, 1.000000000000000000, 0.9659258262890683122, 1.000000000000000000, 0.9659258262890683122, 1.000000000000000000, 0.9659258262890683122, 1.000000000000000000, 0.9659258262890683122, 1.000000000000000000, 0.9659258262890683122, 1.000000000000000000, 0.9659258262890683122, 1.000000000000000000, 0.9659258262890683122, 1.000000000000000000, 0.9659258262890683122, 1.000000000000000000, 0.9659258262890683122, 1.000000000000000000, 0.9659258262890683122, 1.000000000000000000, 0.9659258262890683122, 1.000000000000000000, 0.9659258262890683122, 1.000000000000000000, 0.9659258262890683122, 1.000000000000000000, 0.9659258262890683122, 1.000000000000000000, 0.9659258262890683122, 1.000000000000000000, 0.9659258262890683122, 1.000000000000000000, 0.9659258262890683122, 1.000000000000000000, 0.9659258262890683122, 1.000000000000000000, 0.9659258262890683122, 1.000000000000000000, 0.9659258262890683122, 1.000000000000000000, 0.9659258262890683122, 1.000000000000000000, 0.9659258262890683122, 1.000000000000000000, 0.9659258262890683122, 1.000000000000000000, 0.9659258262890683122, 1.000000000000000000, 0.9659258262890683122, 1.000000000000000000, 0.9659258262890683122, 1.000000000000000000, 0.9659258262890683122, 1.000000000000000000, 0.9659258262890683122, 1.000000000000000000, 0.9659258262890683122, 1.000000000000000000, 0.9659258262890683122, 1.000000000000000000, 0.9659258262890683122, 1.000000000000000000, 0.9659258262890683122, 1.000000000000000000, 0.9659258262890683122, 1.000000000000000000, 0.9659258262890683122, 1.000000000000000000, 0.9659258262890683122, 1.000000000000000000, 0.9659258262890683122, 1.000000000000000000, 0.9659258262890683122, 1.000000000000000000, 0.9659258262890683122, 1.000000000000000000, 0.9659258262890683122, 1.000000000000000000, 0.9659258262890683122, 1.000000000000000000, 0.9659258262890683122, 1.000000000000000000, 0.9659258262890683122, 1.000000000000000000, 0.9659258262890683122, 1.000000000000000000, 0.9659258262890683122, 1.000000000000000000, 0.9659258262890683122, 1.000000000000000000, 0.9659258262890683122, 1.000000000000000000, 0.9659258262890683122, 1.000000000000000000, 0.9659258262890683122, 1.000000000000000000, 0.9659258262890683122, 1.000000000000000000, 0.9659258262890683122, 1.000000000000000000, 0.9659258262890683122, 1.000000000000000000, 0.9659258262890683122, 1.000000000000000000, 0.9659258262890683122, 1.000000000000000000, 0.9659258262890683122, 1.000000000000000000, 0.9659258262890683122, 1.000000000000000000, 0.9659258262890683122, 1.000000000000000000, 0.9659258262890683122, 1.000000000000000000, 0.9659258262890683122, 1.000000000000000000, 0.9659258262890683122, 1.000000000000000000, 0.9659258262890683122, 1.000000000000000000, 0.9659258262890683122, 1.000000000000000000, 0.9659258262890683122, 1.000000000000000000, 0.9659258262890683122, 1.000000000000000000, 0.9659258262890683122, 1.000000000000000000, 0.9659258262890683122, 1.000000000000000000, 0.9659258262890683122, 1.000000000000000000, 0.9659258262890683122, 1.000000000000000000, 0.9659258262890683122, 1.000000000000000000, 0.9659258262890683122, 1.000000000000000000, 0.9659258262890683122, 1.000000000000000000, 0.9659258262890683122, 1.000000000000000000, 0.9659258262890683122, 1.000000000000000000, 0.9659258262890683122, 1.000000000000000000, 0.9659258262890683122, 1.000000000000000000, 0.9659258262890683122, 1.000000000000000000, 0.9659258262890683122, 1.000000000000000000, 0.9659258262890683122, 1.000000000000000000, 0.9659258262890683122, 1.000000000000000000, 0.9659258262890683122, 1.000000000000000000, 0.9659258262890683122, 1.000000000000000000, 0.9659258262890683122, 1.000000000000000000, 0.9659258262890683122, 1.000000000000000000, 0.9659258262890683122, 1.000000000000000000, 0.9659258262890683122, 1.000000000000000000, 0.9659258262890683122, 1.000000000000000000, 0.9659258262890683122, 1.000000000000000000, 0.9659258262890683122, 1.000000000000000000, 0.9659258262890683122, 1.000000000000000000, 0.9659258262890683122, 1.000000000000000000, 0.9659258262890683122, 1.000000000000000000, 0.9659258262890683122, 1.000000000000000000, 0.9659258262890683122, 1.000000000000000000, 0.9659258262890683122, 1.000000000000000000, 0.9659258262890683122, 1.000000000000000000, 0.9659258262890683122, 1.000000000000000000, 0.9659258262890683122, 1.000000000000000000, 0.9659258262890683122, 1.000000000000000000, 0.9659258262890683122, 1.000000000000000000, 0.9659258262890683122, 1.000000000000000000, 0.9659258262890683122, 1.000000000000000000, 0.9659258262890683122, 1.000000000000000000, 0.9659258262890683122, 1.000000000000000000, 0.9659258262890683122, 1.000000000000000000, 0.9659258262890683122, 1.000000000000000000, 0.9659258262890683122, 1.000000000000000000, 0.9659258262890683122, 1.000000000000000000, 0.9659258262890683122, 1.000000000000000000, 0.9659258262890683122, 1.000000000000000000, 0.9659258262890683122, 1.000000000000000000, 0.9659258262890683122, 1.000000000000000000, 0.9659258262890683122, 1.000000000000000000, 0.9659258262890683122, 1.000000000000000000, 0.9659258262890683122, 1.000000000000000000, 0.9659258262890683122, 1.000000000000000000, 0.9659258262890683122, 1.000000000000000000, 0.9659258262890683122, 1.000000000000000000, 0.9659258262890683122, 1.000000000000000000, 0.9659258262890683122, 1.000000000000000000, 0.9659258262890683122, 1.000000000000000000, 0.9659258262890683122, 1.000000000000000000, 0.9659258262890683122, 1.000000000000000000, 0.9659258262890683122, 1.000000000000000000, 0.9659258262890683122, 1.000000000000000000, 0.9659258262890683122, 1.000000000000000000, 0.9659258262890683122, 1.000000000000000000, 0.9659258262890683122, 1.000000000000000000, 0.9659258262890683122, 1.000000000000000000, 0.9659258262890683122, 1.000000000000000000, 0.9659258262890683122, 1.000000000000000000),
 ( 1.000000000000000000, 0.9659258262890683122, 1.000000000000000000, 0.9659258262890683122, 1.000000000000000000, 0.9659258262890683122, 1.000000000000000000, 0.9659258262890683122, 1.000000000000000000, 0.9659258262890683122, 1.000000000000000000, 0.9659258262890683122, 1.000000000000000000, 0.9659258262890683122, 1.000000000000000000, 0.9659258262890683122, 1.000000000000000000, 0.9659258262890683122, 1.000000000000000000, 0.9659258262890683122, 1.000000000000000000, 0.9659258262890683122, 1.000000000000000000, 0.9659258262890683122, 1.000000000000000000, 0.9659258262890683122, 1.000000000000000000, 0.9659258262890683122, 1.000000000000000000, 0.9659258262890683122, 1.000000000000000000, 0.9659258262890683122, 1.000000000000000000, 0.9659258262890683122, 1.000000000000000000, 0.9659258262890683122, 1.000000000000000000, 0.9659258262890683122, 1.000000000000000000, 0.9659258262890683122, 1.000000000000000000, 0.9659258262890683122, 1.000000000000000000, 0.9659258262890683122, 1.000000000000000000, 0.9659258262890683122, 1.000000000000000000, 0.9659258262890683122, 1.000000000000000000, 0.9659258262890683122, 1.000000000000000000, 0.9659258262890683122, 1.000000000000000000, 0.9659258262890683122, 1.000000000000000000, 0.9659258262890683122, 1.000000000000000000, 0.9659258262890683122, 1.000000000000000000, 0.9659258262890683122, 1.000000000000000000, 0.9659258262890683122, 1.000000000000000000, 0.9659258262890683122, 1.000000000000000000, 0.9659258262890683122, 1.000000000000000000, 0.9659258262890683122, 1.000000000000000000, 0.9659258262890683122, 1.000000000000000000, 0.9659258262890683122, 1.000000000000000000, 0.9659258262890683122, 1.000000000000000000, 0.9659258262890683122, 1.000000000000000000, 0.9659258262890683122, 1.000000000000000000, 0.9659258262890683122, 1.000000000000000000, 0.9659258262890683122, 1.000000000000000000, 0.9659258262890683122, 1.000000000000000000, 0.9659258262890683122, 1.000000000000000000, 0.9659258262890683122, 1.000000000000000000, 0.9659258262890683122, 1.000000000000000000, 0.9659258262890683122, 1.000000000000000000, 0.9659258262890683122, 1.000000000000000000, 0.9659258262890683122, 1.000000000000000000, 0.9659258262890683122, 1.000000000000000000, 0.9659258262890683122, 1.000000000000000000, 0.9659258262890683122, 1.000000000000000000, 0.9659258262890683122, 1.000000000000000000, 0.9659258262890683122, 1.000000000000000000, 0.9659258262890683122, 1.000000000000000000, 0.9659258262890683122, 1.000000000000000000, 0.9659258262890683122, 1.000000000000000000, 0.9659258262890683122, 1.000000000000000000, 0.9659258262890683122, 1.000000000000000000, 0.9659258262890683122, 1.000000000000000000, 0.9659258262890683122, 1.000000000000000000, 0.9659258262890683122, 1.000000000000000000, 0.9659258262890683122, 1.000000000000000000, 0.9659258262890683122, 1.000000000000000000, 0.9659258262890683122, 1.000000000000000000, 0.9659258262890683122, 1.000000000000000000, 0.9659258262890683122, 1.000000000000000000, 0.9659258262890683122, 1.000000000000000000, 0.9659258262890683122, 1.000000000000000000, 0.9659258262890683122, 1.000000000000000000, 0.9659258262890683122, 1.000000000000000000, 0.9659258262890683122, 1.000000000000000000, 0.9659258262890683122, 1.000000000000000000, 0.9659258262890683122, 1.000000000000000000, 0.9659258262890683122, 1.000000000000000000, 0.9659258262890683122, 1.000000000000000000, 0.9659258262890683122, 1.000000000000000000, 0.9659258262890683122, 1.000000000000000000, 0.9659258262890683122, 1.000000000000000000, 0.9659258262890683122, 1.000000000000000000, 0.9659258262890683122, 1.000000000000000000, 0.9659258262890683122, 1.000000000000000000, 0.9659258262890683122, 1.000000000000000000, 0.9659258262890683122, 1.000000000000000000, 0.9659258262890683122, 1.000000000000000000, 0.9659258262890683122, 1.000000000000000000, 0.9659258262890683122, 1.000000000000000000, 0.9659258262890683122, 1.000000000000000000, 0.9659258262890683122, 1.000000000000000000, 0.9659258262890683122, 1.000000000000000000, 0.9659258262890683122, 1.000000000000000000, 0.9659258262890683122, 1.000000000000000000, 0.9659258262890683122, 1.000000000000000000, 0.9659258262890683122, 1.000000000000000000, 0.9659258262890683122, 1.000000000000000000, 0.9659258262890683122, 1.000000000000000000, 0.9659258262890683122, 1.000000000000000000, 0.9659258262890683122, 1.000000000000000000, 0.9659258262890683122, 1.000000000000000000, 0.9659258262890683122, 1.000000000000000000, 0.9659258262890683122, 1.000000000000000000, 0.9659258262890683122, 1.000000000000000000, 0.9659258262890683122, 1.000000000000000000, 0.9659258262890683122, 1.000000000000000000, 0.9659258262890683122, 1.000000000000000000, 0.9659258262890683122, 1.000000000000000000, 0.9659258262890683122, 1.000000000000000000, 0.9659258262890683122, 1.000000000000000000, 0.9659258262890683122, 1.000000000000000000, 0.9659258262890683122, 1.000000000000000000, 0.9659258262890683122, 1.000000000000000000, 0.9659258262890683122, 1.000000000000000000, 0.9659258262890683122, 1.000000000000000000, 0.9659258262890683122, 1.000000000000000000, 0.9659258262890683122, 1.000000000000000000, 0.9659258262890683122, 1.000000000000000000, 0.9659258262890683122, 1.000000000000000000, 0.9659258262890683122, 1.000000000000000000, 0.9659258262890683122, 1.000000000000000000, 0.9659258262890683122, 1.000000000000000000, 0.9659258262890683122, 1.000000000000000000, 0.9659258262890683122, 1.000000000000000000, 0.9659258262890683122, 1.000000000000000000, 0.9659258262890683122, 1.000000000000000000, 0.9659258262890683122, 1.000000000000000000, 0.9659258262890683122, 1.000000000000000000, 0.9659258262890683122, 1.000000000000000000, 0.9659258262890683122, 1.000000000000000000, 0.9659258262890683122, 1.000000000000000000, 0.9659258262890683122, 1.000000000000000000, 0.9659258262890683122, 1.000000000000000000, 0.9659258262890683122, 1.000000000000000000, 0.9659258262890683122, 1.000000000000000000, 0.9659258262890683122, 1.000000000000000000, 0.9659258262890683122, 1.000000000000000000, 0.9659258262890683122, 1.000000000000000000, 0.9659258262890683122, 1.000000000000000000, 0.9659258262890683122, 1.000000000000000000, 0.9659258262890683122, 1.000000000000000000, 0.9659258262890683122, 1.000000000000000000, 0.9659258262890683122, 1.000000000000000000, 0.9659258262890683122, 1.000000000000000000, 0.9659258262890683122, 1.000000000000000000, 0.9659258262890683122, 1.000000000000000000, 0.9659258262890683122, 1.000000000000000000, 0.9659258262890683122, 1.000000000000000000, 0.9659258262890683122, 1.000000000000000000, 0.9659258262890683122, 1.000000000000000000, 0.9659258262890683122, 1.000000000000000000, 0.9659258262890683122, 1.000000000000000000, 0.9659258262890683122, 1.000000000000000000, 0.9659258262890683122, 1.000000000000000000, 0.9659258262890683122, 1.000000000000000000, 0.9659258262890683122, 1.000000000000000000, 0.9659258262890683122, 1.000000000000000000, 0.9659258262890683122, 1.000000000000000000, 0.9659258262890683122, 1.000000000000000000, 0.9659258262890683122, 1.000000000000000000, 0.9659258262890683122, 1.000000000000000000, 0.9659258262890683122, 1.000000000000000000, 0.9659258262890683122, 1.000000000000000000, 0.9659258262890683122, 1.000000000000000000, 0.9659258262890683122, 1.000000000000000000, 0.9659258262890683122, 1.000000000000000000, 0.9659258262890683122, 1.000000000000000000, 0.9659258262890683122, 1.000000000000000000, 0.9659258262890683122, 1.000000000000000000, 0.9659258262890683122, 1.000000000000000000, 0.9659258262890683122, 1.000000000000000000, 0.9659258262890683122, 1.000000000000000000, 0.9659258262890683122, 1.000000000000000000, 0.9659258262890683122, 1.000000000000000000, 0.9659258262890683122, 1.000000000000000000, 0.9659258262890683122, 1.000000000000000000, 0.9659258262890683122, 1.000000000000000000, 0.9659258262890683122, 1.000000000000000000, 0.9659258262890683122, 1.000000000000000000, 0.9659258262890683122, 1.000000000000000000, 0.9659258262890683122, 1.000000000000000000, 0.9659258262890683122, 1.000000000000000000, 0.9659258262890683122, 1.000000000000000000, 0.9659258262890683122, 1.000000000000000000, 0.9659258262890683122, 1.000000000000000000, 0.9659258262890683122, 1.000000000000000000, 0.9659258262890683122, 1.000000000000000000, 0.9659258262890683122, 1.000000000000000000, 0.9659258262890683122, 1.000000000000000000, 0.9659258262890683122, 1.000000000000000000, 0.9659258262890683122, 1.000000000000000000, 0.9659258262890683122, 1.000000000000000000, 0.9659258262890683122, 1.000000000000000000, 0.9659258262890683122, 1.000000000000000000, 0.9659258262890683122, 1.000000000000000000, 0.9659258262890683122, 1.000000000000000000, 0.9659258262890683122, 1.000000000000000000, 0.9659258262890683122, 1.000000000000000000, 0.9659258262890683122, 1.000000000000000000, 0.9659258262890683122, 1.000000000000000000, 0.9659258262890683122, 1.000000000000000000, 0.9659258262890683122, 1.000000000000000000, 0.9659258262890683122, 1.000000000000000000, 0.9659258262890683122, 1.000000000000000000, 0.9659258262890683122, 1.000000000000000000, 0.9659258262890683122, 1.000000000000000000, 0.9659258262890683122, 1.000000000000000000, 0.9659258262890683122, 1.000000000000000000, 0.9659258262890683122, 1.000000000000000000, 0.9659258262890683122, 1.000000000000000000, 0.9659258262890683122, 1.000000000000000000, 0.9659258262890683122, 1.000000000000000000, 0.9659258262890683122, 1.000000000000000000, 0.9659258262890683122, 1.000000000000000000, 0.9659258262890683122, 1.000000000000000000, 0.9659258262890683122, 1.000000000000000000, 0.9659258262890683122, 1.000000000000000000, 0.9659258262890683122, 1.000000000000000000, 0.9659258262890683122, 1.000000000000000000, 0.9659258262890683122, 1.000000000000000000, 0.9659258262890683122, 1.000000000000000000, 0.9659258262890683122, 1.000000000000000000, 0.9659258262890683122, 1.000000000000000000, 0.9659258262890683122, 1.000000000000000000, 0.9659258262890683122, 1.000000000000000000, 0.9659258262890683122, 1.000000000000000000, 0.9659258262890683122, 1.000000000000000000, 0.9659258262890683122, 1.000000000000000000, 0.9659258262890683122, 1.000000000000000000, 0.9659258262890683122, 1.000000000000000000, 0.9659258262890683122, 1.000000000000000000, 0.9659258262890683122, 1.000000000000000000, 0.9659258262890683122, 1.000000000000000000, 0.9659258262890683122, 1.000000000000000000, 0.9659258262890683122, 1.000000000000000000, 0.9659258262890683122, 1.000000000000000000, 0.9659258262890683122, 1.000000000000000000, 0.9659258262890683122, 1.000000000000000000, 0.9659258262890683122, 1.000000000000000000, 0.9659258262890683122, 1.000000000000000000, 0.9659258262890683122, 1.000000000000000000, 0.9659258262890683122, 1.000000000000000000, 0.9659258262890683122, 1.000000000000000000, 0.9659258262890683122, 1.000000000000000000, 0.9659258262890683122, 1.000000000000000000, 0.9659258262890683122, 1.000000000000000000, 0.9659258262890683122, 1.000000000000000000, 0.9659258262890683122, 1.000000000000000000, 0.9659258262890683122, 1.000000000000000000, 0.9659258262890683122, 1.000000000000000000, 0.9659258262890683122, 1.000000000000000000, 0.9659258262890683122, 1.000000000000000000, 0.9659258262890683122, 1.000000000000000000, 0.9659258262890683122, 1.000000000000000000, 0.9659258262890683122, 1.000000000000000000, 0.9659258262890683122, 1.000000000000000000, 0.9659258262890683122, 1.000000000000000000, 0.9659258262890683122, 1.000000000000000000) ) ) 
 REPRESENTATION_ITEM ( '' )  SURFACE ( )  );
#45572=CARTESIAN_POINT ( 'NONE',  ( 1.456692913385827515, -0.5511811023622047445, 6.969142054262312111E-17 ) ) ;
#45573=CARTESIAN_POINT ( 'NONE',  ( -1.482939632545930975, -0.004921259842519576551, 0.3153832671262227771 ) ) ;
#45574=CARTESIAN_POINT ( 'NONE',  ( -0.4002624671916004129, -0.2845877964562159024, 0.3641732283464567677 ) ) ;
#45575=CARTESIAN_POINT ( 'NONE',  ( -1.528871391076114250, 0.1771653543307087075, -0.09757992244046823083 ) ) ;
#45576=CARTESIAN_POINT ( 'NONE',  ( 0.9842519685039375910, 0.1771653543307087630, 0.000000000000000000 ) ) ;
#45577=CARTESIAN_POINT ( 'NONE',  ( 0.6561679790026253567, -0.6046776061558809534, -0.2411417322834644161 ) ) ;
#45578=CARTESIAN_POINT ( 'NONE',  ( 1.299212598425197429, 0.2952755905511811885, 0.000000000000000000 ) ) ;
#45579=CARTESIAN_POINT ( 'NONE',  ( 0.05249343832021075018, -0.6046776061558807314, 0.2411417322834647770 ) ) ;
#45580=CARTESIAN_POINT ( 'NONE',  ( 0.5446194225721792126, -0.08942795157528024563, -0.3641732283464568787 ) ) ;
#45581=CARTESIAN_POINT ( 'NONE',  ( 1.509186351706037543, -0.4281496062992127816, -0.4176697321401328100 ) ) ;
#45582=CARTESIAN_POINT ( 'NONE',  ( 1.586052503253845503, 1.023622047244095556, 0.1653254495020588799 ) ) ;
#45583=CARTESIAN_POINT ( 'NONE',  ( -0.4593175853018366950, 0.05413385826771666132, 0.4176697321401328100 ) ) ;
#45585=CARTESIAN_POINT ( 'NONE',  ( -2.787279214012418738, 0.000000000000000000, 0.000000000000000000 ) ) ;
#45586=CARTESIAN_POINT ( 'NONE',  ( 0.1640419947506569498, -0.05778040916215522460, 0.4822834645669289988 ) ) ;
#45587=CARTESIAN_POINT ( 'NONE',  ( -0.4724409448818890911, -0.1870078740157480879, -0.4822834645669291653 ) ) ;
#45588=CARTESIAN_POINT ( 'NONE',  ( 0.04593175853018440641, 0.2952755905511810774, -0.1292274648535930714 ) ) ;
#45589=AXIS2_PLACEMENT_3D ( 'NONE', #67472, #47680, #54829 ) ;
#45595=CARTESIAN_POINT ( 'NONE',  ( -1.030183727034119867, -0.08942795157528024563, -0.3641732283464568787 ) ) ;
#45597=CARTESIAN_POINT ( 'NONE',  ( -1.122047244094487306, -0.5400638737290844871, 0.3530559997133364547 ) ) ;
#45599=CARTESIAN_POINT ( 'NONE',  ( 0.5511811023622055217, -0.1870078740157479769, 0.4822834645669291653 ) ) ;
#45600=CARTESIAN_POINT ( 'NONE',  ( -0.1509186351706028884, -0.08942795157527998196, 0.3641732283464567121 ) ) ;
#45601=CARTESIAN_POINT ( 'NONE',  ( 1.318897637795276356, 0.1660481256975883668, -0.3530559997133364547 ) ) ;
#45602=CARTESIAN_POINT ( 'NONE',  ( 0.2755905511811031494, -0.6692913385826771977, 8.415575281601705876E-17 ) ) ;
#45606=CARTESIAN_POINT ( 'NONE',  ( 1.122047244094488860, -0.5400638737290845981, -0.3530559997133363437 ) ) ;
#45607=CARTESIAN_POINT ( 'NONE',  ( 0.4396325459317590445, -0.6692913385826771977, 0.1292274648535927661 ) ) ;
#45609=CARTESIAN_POINT ( 'NONE',  ( 0.2493438320209980519, -0.4281496062992127816, -0.4176697321401328100 ) ) ;
#45610=CARTESIAN_POINT ( 'NONE',  ( 1.443569553805774897, -0.6046776061558809534, -0.2411417322834644161 ) ) ;
#45612=CARTESIAN_POINT ( 'NONE',  ( -0.09186351706036689768, 0.05413385826771626580, -0.4176697321401330321 ) ) ;
#45613=CARTESIAN_POINT ( 'NONE',  ( 0.9580052493438327987, -0.4281496062992127816, -0.4176697321401328100 ) ) ;
#45614=CARTESIAN_POINT ( 'NONE',  ( 0.4265091863517067594, 0.2952755905511811885, 0.1292274648535926551 ) ) ;
#45615=CARTESIAN_POINT ( 'NONE',  ( 1.010498687664042716, -0.3690944881889763329, 0.3153832671262228327 ) ) ;
#45616=CARTESIAN_POINT ( 'NONE',  ( -1.056430446194224881, 0.2952755905511810774, -0.1292274648535930714 ) ) ;
#45617=CARTESIAN_POINT ( 'NONE',  ( -1.305774278215222184, -0.6692913385826773087, -0.1292274648535924053 ) ) ;
#45618=CARTESIAN_POINT ( 'NONE',  ( 0.6889763779527563470, 0.1660481256975883668, -0.3530559997133364547 ) ) ;
#45621=CARTESIAN_POINT ( 'NONE',  ( 1.535433070866142558, 0.2952755905511811885, 0.000000000000000000 ) ) ;
#45624=ORIENTED_EDGE ( 'NONE', *, *, #20141, .F. ) ;
#45625=CARTESIAN_POINT ( 'NONE',  ( 1.358267716535433323, 0.1660481256975885056, 0.3530559997133364547 ) ) ;
#45626=CARTESIAN_POINT ( 'NONE',  ( 0.9908136482939640111, 0.1771653543307087075, -0.09757992244046823083 ) ) ;
#45629=CARTESIAN_POINT ( 'NONE',  ( -1.614173228346457378, 0.2753471884572478157, -0.1372047244094478091 ) ) ;
#45631=CARTESIAN_POINT ( 'NONE',  ( -1.286089238845143479, 0.1283753931104746893, -0.1820866141732285504 ) ) ;
#45632=CARTESIAN_POINT ( 'NONE',  ( -1.732283464566928277, -0.1870078740157479769, 0.3641732283464567677 ) ) ;
#45634=CARTESIAN_POINT ( 'NONE',  ( -0.3215223097112853146, -0.3162353388693405765, 0.4822834645669290543 ) ) ;
#45635=CARTESIAN_POINT ( 'NONE',  ( 1.463254593175853824, 0.2952755905511810774, -0.1292274648535930714 ) ) ;
#45637=CARTESIAN_POINT ( 'NONE',  ( -0.7186703366786194591, -2.567464376874931580E-15, -0.4445507791589072832 ) ) ;
#45640=CARTESIAN_POINT ( 'NONE',  ( -1.603475055217291612, 1.881749232079046097, 0.04573490813648253134 ) ) ;
#45641=CARTESIAN_POINT ( 'NONE',  ( -1.036745406824146176, -0.3690944881889763329, 0.3153832671262228327 ) ) ;
#45642=CARTESIAN_POINT ( 'NONE',  ( -1.509186351706035767, -0.4281496062992124485, 0.4176697321401328655 ) ) ;
#45643=CARTESIAN_POINT ( 'NONE',  ( 0.4527559055118117182, 0.1660481256975883668, -0.3530559997133364547 ) ) ;
#45647=CARTESIAN_POINT ( 'NONE',  ( 1.187664041994751285, -0.05778040916215522460, 0.4822834645669289988 ) ) ;
#45648=CARTESIAN_POINT ( 'NONE',  ( 1.561679790026247350, -0.3690944881889763329, 0.3153832671262228327 ) ) ;
#45650=CARTESIAN_POINT ( 'NONE',  ( -0.3608923884514428360, -0.5511811023622048555, -0.09757992244046775898 ) ) ;
#45651=CARTESIAN_POINT ( 'NONE',  ( -1.640419947506561060, -0.004921259842519576551, 0.3153832671262227771 ) ) ;
#45653=CARTESIAN_POINT ( 'NONE',  ( 0.3149606299212603933, -0.1870078740157479769, 0.4822834645669291653 ) ) ;
#45654=CARTESIAN_POINT ( 'NONE',  ( -0.4921259842519677963, 0.07958543189024071263, -0.2665933059059888421 ) ) ;
#45655=CARTESIAN_POINT ( 'NONE',  ( 0.05249343832021075018, 0.1283753931104746893, -0.1820866141732285504 ) ) ;
#45656=CARTESIAN_POINT ( 'NONE',  ( 0.2952755905511816326, -0.5400638737290844871, 0.3530559997133364547 ) ) ;
#45657=CARTESIAN_POINT ( 'NONE',  ( -1.233595800524933894, -0.5023911411419708095, -0.1820866141732282451 ) ) ;
#45659=CARTESIAN_POINT ( 'NONE',  ( 0.8464566929133865436, 0.1660481256975883668, -0.3530559997133364547 ) ) ;
#45660=CARTESIAN_POINT ( 'NONE',  ( -1.489501312335957062, -0.05778040916215522460, 0.4822834645669289988 ) ) ;
#45662=CARTESIAN_POINT ( 'NONE',  ( -0.4593175853018366950, 0.05413385826771666132, 0.4176697321401328100 ) ) ;
#45663=CARTESIAN_POINT ( 'NONE',  ( 0.2952755905511816326, -0.4536011799217367080, 0.2665933059059888421 ) ) ;
#45664=CARTESIAN_POINT ( 'NONE',  ( -1.082677165354329896, -0.5400638737290845981, -0.3530559997133363437 ) ) ;
#45665=CARTESIAN_POINT ( 'NONE',  ( 0.7874015748031503170, -0.1870078740157480601, -0.3641732283464567677 ) ) ;
#45666=CARTESIAN_POINT ( 'NONE',  ( -0.1706036745406816491, -0.3690944881889763329, 0.3153832671262228327 ) ) ;
#45667=CARTESIAN_POINT ( 'NONE',  ( -0.6627296587926503335, -0.6692913385826771977, 0.1292274648535927661 ) ) ;
#45668=CARTESIAN_POINT ( 'NONE',  ( -1.568241469816272105, -0.3162353388693409650, -0.4822834645669289433 ) ) ;
#45670=CARTESIAN_POINT ( 'NONE',  ( 1.443569553805774897, -0.5023911411419708095, -0.1820866141732282451 ) ) ;
#45671=CARTESIAN_POINT ( 'NONE',  ( 0.3740157480314966754, -0.5400638737290844871, 0.3530559997133364547 ) ) ;
#45672=CARTESIAN_POINT ( 'NONE',  ( -1.614173228346455824, 0.2952755905511811885, 0.000000000000000000 ) ) ;
#45673=CARTESIAN_POINT ( 'NONE',  ( -1.502624671916009680, -0.05778040916215560624, -0.4822834645669293319 ) ) ;
#45676=CARTESIAN_POINT ( 'NONE',  ( -0.9645669291338575535, 0.07958543189024071263, -0.2665933059059888421 ) ) ;
#45677=CARTESIAN_POINT ( 'NONE',  ( 0.8005249343832027131, 0.05413385826771666132, 0.4176697321401328100 ) ) ;
#45678=CARTESIAN_POINT ( 'NONE',  ( -0.9448818897637790704, -0.1870078740157479769, 0.3641732283464567677 ) ) ;
#45680=CARTESIAN_POINT ( 'NONE',  ( -1.049868766404198794, 0.2306618581243847221, -0.2411417322834647770 ) ) ;
#45681=CARTESIAN_POINT ( 'NONE',  ( 1.043307086614173818, 0.1660481256975885056, 0.3530559997133364547 ) ) ;
#45682=CARTESIAN_POINT ( 'NONE',  ( 0.4790026246719168435, -0.3162353388693409650, -0.4822834645669289433 ) ) ;
#45683=CARTESIAN_POINT ( 'NONE',  ( 1.476377952755906220, 0.1660481256975883668, -0.3530559997133364547 ) ) ;
#45684=CARTESIAN_POINT ( 'NONE',  ( -1.692913385826770645, 0.1771653543307087630, 0.000000000000000000 ) ) ;
#45689=CARTESIAN_POINT ( 'NONE',  ( 0.5511811023622055217, -0.1870078740157479769, 0.3641732283464567677 ) ) ;
#45690=CARTESIAN_POINT ( 'NONE',  ( 0.3280839895013130669, -0.004921259842519576551, 0.3153832671262227771 ) ) ;
#45691=CARTESIAN_POINT ( 'NONE',  ( 0.1706036745406830368, 0.05413385826771666132, 0.4176697321401328100 ) ) ;
#45692=CARTESIAN_POINT ( 'NONE',  ( 1.437007874015748810, 0.1660481256975885056, 0.3530559997133364547 ) ) ;
#45694=CARTESIAN_POINT ( 'NONE',  ( 0.4199475065616805614, 0.1283753931104748280, 0.1820866141732283561 ) ) ;
#45695=( BOUNDED_CURVE ( )  B_SPLINE_CURVE ( 2, ( #41534, #28073, #21758, #47421, #53322, #52899, #9553, #14636, #20522, #35223, #15045, #53731, #47836 ),
 .UNSPECIFIED., .F., .F. ) 
 B_SPLINE_CURVE_WITH_KNOTS ( ( 3, 2, 2, 2, 2, 2, 3 ),
 ( 0.6740332660251416863, 0.6742424242424241987, 0.6780303030303029832, 0.6818181818181817677, 0.6856060606060605522, 0.6893939393939394478, 0.6896030976112219602 ),
 .UNSPECIFIED. ) 
 CURVE ( )  GEOMETRIC_REPRESENTATION_ITEM ( )  RATIONAL_B_SPLINE_CURVE ( ( 0.9964447847208419695, 0.9981185001348091834, 1.000000000000000000, 0.9659258262890683122, 1.000000000000000000, 0.9659258262890683122, 1.000000000000000000, 0.9659258262890683122, 1.000000000000000000, 0.9659258262890683122, 1.000000000000000000, 0.9981185001348091834, 0.9964447847208420805 ) ) 
 REPRESENTATION_ITEM ( '' )  );
#45696=CARTESIAN_POINT ( 'NONE',  ( -0.7677165354330699465, -0.5400638737290845981, -0.3530559997133363437 ) ) ;
#45697=CARTESIAN_POINT ( 'NONE',  ( -1.450131233595799651, 0.2952755905511810774, -0.1292274648535930714 ) ) ;
#45698=CARTESIAN_POINT ( 'NONE',  ( 0.7874015748031503170, -0.1870078740157480879, -0.4822834645669291653 ) ) ;
#45701=ORIENTED_EDGE ( 'NONE', *, *, #24294, .F. ) ;
#45704=CARTESIAN_POINT ( 'NONE',  ( -1.417322834645668772, -0.1870078740157479769, 0.4822834645669291653 ) ) ;
#45705=CARTESIAN_POINT ( 'NONE',  ( -1.207349081364828436, -0.6046776061558807314, 0.2411417322834647770 ) ) ;
#45706=CARTESIAN_POINT ( 'NONE',  ( -0.7611548556430438595, -0.5023911411419708095, -0.1820866141732282451 ) ) ;
#45707=CARTESIAN_POINT ( 'NONE',  ( -0.6233595800524928121, -0.3162353388693409650, -0.4822834645669289433 ) ) ;
#45709=CARTESIAN_POINT ( 'NONE',  ( -0.4624320255261038515, -2.191421614605370878E-15, 0.4445507791589071167 ) ) ;
#45710=CARTESIAN_POINT ( 'NONE',  ( -1.594488188976377119, 0.07958543189024071263, -0.2665933059059888421 ) ) ;
#45711=CARTESIAN_POINT ( 'NONE',  ( -1.417322834645668772, -0.1870078740157479769, 0.4822834645669291653 ) ) ;
#45712=CARTESIAN_POINT ( 'NONE',  ( 0.2755905511811031494, -0.6692913385826771977, 8.415575281601705876E-17 ) ) ;
#45713=CARTESIAN_POINT ( 'NONE',  ( -0.9383202099737524282, -0.3162353388693409650, -0.4822834645669289433 ) ) ;
#45715=CARTESIAN_POINT ( 'NONE',  ( 0.5971128608923890191, -0.6692913385826771977, 0.1292274648535927661 ) ) ;
#45717=CARTESIAN_POINT ( 'NONE',  ( -0.7480314960629914633, -0.5511811023622047445, 6.969142054262312111E-17 ) ) ;
#45718=EDGE_LOOP ( 'NONE', ( #12488, #33901, #37957, #72275, #63945 ) ) ;
#45720=ORIENTED_EDGE ( 'NONE', *, *, #44425, .T. ) ;
#45721=CARTESIAN_POINT ( 'NONE',  ( -1.673228346456691717, 0.07958543189024071263, -0.2665933059059888421 ) ) ;
#45722=CARTESIAN_POINT ( 'NONE',  ( -0.9383202099737524282, -0.05778040916215522460, 0.4822834645669289988 ) ) ;
#45723=CARTESIAN_POINT ( 'NONE',  ( -1.391076115485563314, -0.6046776061558809534, -0.2411417322834644161 ) ) ;
#45725=CARTESIAN_POINT ( 'NONE',  ( -1.299212598425196097, -0.6692913385826771977, 8.415575281601705876E-17 ) ) ;
#45726=CARTESIAN_POINT ( 'NONE',  ( -1.463254593175852492, -0.6692913385826773087, -0.1292274648535924053 ) ) ;
#45727=CARTESIAN_POINT ( 'NONE',  ( -1.391076115485563314, -0.6046776061558809534, -0.2411417322834644161 ) ) ;
#45729=CARTESIAN_POINT ( 'NONE',  ( -1.586052503253848389, 0.7480314960629931287, -0.1653254495020559933 ) ) ;
#45730=CARTESIAN_POINT ( 'NONE',  ( 0.2821522309711292364, 0.1771653543307087075, -0.09757992244046823083 ) ) ;
#45733=CARTESIAN_POINT ( 'NONE',  ( -0.3740157480314953431, -0.4536011799217368745, -0.2665933059059886201 ) ) ;
#45734=CARTESIAN_POINT ( 'NONE',  ( -0.9645669291338575535, 0.1660481256975883668, -0.3530559997133364547 ) ) ;
#45735=CARTESIAN_POINT ( 'NONE',  ( 1.141732283464567566, 0.2952755905511811885, 0.000000000000000000 ) ) ;
#45736=CARTESIAN_POINT ( 'NONE',  ( -0.4133858267716528645, -0.5400638737290844871, 0.3530559997133364547 ) ) ;
#45740=CARTESIAN_POINT ( 'NONE',  ( -0.8070866141732276899, 0.1660481256975883668, -0.3530559997133364547 ) ) ;
#45741=CARTESIAN_POINT ( 'NONE',  ( 1.240157480314961314, -0.5400638737290844871, 0.3530559997133364547 ) ) ;
#45742=CARTESIAN_POINT ( 'NONE',  ( -1.614173228346456268, -0.5511811023622047445, 6.969142054262312111E-17 ) ) ;
#45748=CARTESIAN_POINT ( 'NONE',  ( -0.2493438320209966919, -0.4281496062992124485, 0.4176697321401328655 ) ) ;
#45749=CARTESIAN_POINT ( 'NONE',  ( -1.607611548556429737, 0.1771653543307087075, -0.09757992244046823083 ) ) ;
#45750=CARTESIAN_POINT ( 'NONE',  ( -0.6889763779527552368, -0.5400638737290845981, -0.3530559997133363437 ) ) ;
#45752=CARTESIAN_POINT ( 'NONE',  ( -1.450131233595799651, -0.6692913385826771977, 0.1292274648535927661 ) ) ;
#45753=CARTESIAN_POINT ( 'NONE',  ( -1.141732283464566011, -0.6692913385826771977, 8.415575281601705876E-17 ) ) ;
#45754=CARTESIAN_POINT ( 'NONE',  ( -0.4199475065616791736, 0.2306618581243847221, -0.2411417322834647770 ) ) ;
#45756=CARTESIAN_POINT ( 'NONE',  ( 1.010498687664042716, -0.004921259842519870586, -0.3153832671262229437 ) ) ;
#45757=CARTESIAN_POINT ( 'NONE',  ( 0.6233595800524942554, -0.08942795157528024563, -0.3641732283464568787 ) ) ;
#45758=CARTESIAN_POINT ( 'NONE',  ( 1.391076115485564868, -0.5023911411419708095, 0.1820866141732285504 ) ) ;
#45759=CARTESIAN_POINT ( 'NONE',  ( 1.227034120734908917, -0.6692913385826771977, 0.1292274648535927661 ) ) ;
#45760=CARTESIAN_POINT ( 'NONE',  ( 0.04593175853018440641, -0.5511811023622046335, 0.09757992244046803654 ) ) ;
#45762=CARTESIAN_POINT ( 'NONE',  ( -1.299212598425196097, 0.2952755905511811885, 0.000000000000000000 ) ) ;
#45763=CARTESIAN_POINT ( 'NONE',  ( 1.082677165354331228, -0.5400638737290844871, 0.3530559997133364547 ) ) ;
#45765=CARTESIAN_POINT ( 'NONE',  ( -0.6824146981627288167, 0.1283753931104748280, 0.1820866141732283561 ) ) ;
#45766=LINE ( 'NONE', #764, #42617 ) ;
#45767=CARTESIAN_POINT ( 'NONE',  ( 0.4396325459317593221, 0.2952755905511810774, -0.1292274648535930714 ) ) ;
#45769=CARTESIAN_POINT ( 'NONE',  ( 0.8267716535433077274, 0.1771653543307087630, 0.000000000000000000 ) ) ;
#45770=CARTESIAN_POINT ( 'NONE',  ( 0.05249343832021075018, 0.1283753931104746893, -0.1820866141732285504 ) ) ;
#45771=CARTESIAN_POINT ( 'NONE',  ( -0.2821522309711278487, -0.6692913385826773087, -0.1292274648535924053 ) ) ;
#45772=CARTESIAN_POINT ( 'NONE',  ( -1.338582677165353729, -0.1870078740157480879, -0.4822834645669291653 ) ) ;
#45773=CARTESIAN_POINT ( 'NONE',  ( -0.5118110236220466680, 0.1771653543307087630, 0.000000000000000000 ) ) ;
#45775=CARTESIAN_POINT ( 'NONE',  ( 0.4855643044619430415, -0.4281496062992127816, -0.4176697321401328100 ) ) ;
#45777=CARTESIAN_POINT ( 'NONE',  ( -1.056430446194224881, -0.6692913385826771977, 0.1292274648535927661 ) ) ;
#45780=CARTESIAN_POINT ( 'NONE',  ( 0.1706036745406830368, -0.004921259842519576551, 0.3153832671262227771 ) ) ;
#45781=CARTESIAN_POINT ( 'NONE',  ( -0.9186351706036736120, -0.6046776061558809534, -0.2411417322834644161 ) ) ;
#45782=CARTESIAN_POINT ( 'NONE',  ( -1.003937007874014853, 0.1660481256975885056, 0.3530559997133364547 ) ) ;
#45783=CARTESIAN_POINT ( 'NONE',  ( -1.141732283464566011, 0.1771653543307087630, 0.000000000000000000 ) ) ;
#45784=CARTESIAN_POINT ( 'NONE',  ( 1.614173228346457378, -0.6692913385826771977, 8.415575281601705876E-17 ) ) ;
#45785=CARTESIAN_POINT ( 'NONE',  ( -1.095800524934382292, -0.2845877964562161244, -0.3641732283464567121 ) ) ;
#45787=CARTESIAN_POINT ( 'NONE',  ( 1.377952755905512472, -0.6692913385826771977, 8.415575281601705876E-17 ) ) ;
#45788=CARTESIAN_POINT ( 'NONE',  ( 0.01109768429471727318, 2.739544932778246860E-15, 0.3954974714151458515 ) ) ;
#45790=ORIENTED_EDGE ( 'NONE', *, *, #68162, .T. ) ;
#45793=CARTESIAN_POINT ( 'NONE',  ( 1.384514435695538337, -0.5511811023622046335, 0.09757992244046803654 ) ) ;
#45794=CARTESIAN_POINT ( 'NONE',  ( -1.272965879265091305, -0.4281496062992124485, 0.4176697321401328655 ) ) ;
#45795=CARTESIAN_POINT ( 'NONE',  ( 1.141732283464567566, 0.2952755905511811885, 0.000000000000000000 ) ) ;
#45797=CARTESIAN_POINT ( 'NONE',  ( 1.679790026246720025, 0.1283753931104748280, 0.1820866141732283561 ) ) ;
#45799=CARTESIAN_POINT ( 'NONE',  ( 0.5118110236220480003, -0.6692913385826771977, 8.415575281601705876E-17 ) ) ;
#45800=CARTESIAN_POINT ( 'NONE',  ( 0.1115485564304470323, 0.2952755905511811885, 0.1292274648535926551 ) ) ;
#45802=CARTESIAN_POINT ( 'NONE',  ( -0.7330049731598978768, 2.188112158500873150, -0.5178675056768471396 ) ) ;
#45803=CARTESIAN_POINT ( 'NONE',  ( 0.8070866141732288002, 0.07958543189024085140, 0.2665933059059887866 ) ) ;
#45805=ORIENTED_EDGE ( 'NONE', *, *, #68362, .T. ) ;
#45808=CARTESIAN_POINT ( 'NONE',  ( 0.1771653543307093182, 0.1660481256975885056, 0.3530559997133364547 ) ) ;
#45809=CARTESIAN_POINT ( 'NONE',  ( 1.535433070866142335, -0.6692913385826771977, 8.415575281601705876E-17 ) ) ;
#45810=CARTESIAN_POINT ( 'NONE',  ( 0.7152230971128616943, -0.05778040916215522460, 0.4822834645669289988 ) ) ;
#45811=CARTESIAN_POINT ( 'NONE',  ( 1.049868766404200349, 0.2306618581243848609, 0.2411417322834645549 ) ) ;
#45812=CARTESIAN_POINT ( 'NONE',  ( -0.4265091863517051496, -0.6692913385826771977, 0.1292274648535927661 ) ) ;
#45813=CARTESIAN_POINT ( 'NONE',  ( -0.006561679790025524116, -0.3162353388693405765, 0.4822834645669290543 ) ) ;
#45814=CARTESIAN_POINT ( 'NONE',  ( 1.614173228346457378, 0.2952755905511811885, 0.000000000000000000 ) ) ;
#45815=CARTESIAN_POINT ( 'NONE',  ( 1.364829396325459854, -0.6046776061558809534, -0.2411417322834644161 ) ) ;
#45816=CARTESIAN_POINT ( 'NONE',  ( 0.9973753280839902091, -0.6046776061558807314, 0.2411417322834647770 ) ) ;
#45818=CARTESIAN_POINT ( 'NONE',  ( 0.5511811023622055217, -0.1870078740157479769, 0.3641732283464567677 ) ) ;
#45822=CARTESIAN_POINT ( 'NONE',  ( -0.3937007874015740483, -0.1870078740157480601, -0.3641732283464567677 ) ) ;
#45823=CARTESIAN_POINT ( 'NONE',  ( -0.01968503937007793844, 0.1660481256975883668, -0.3530559997133364547 ) ) ;
#45825=CARTESIAN_POINT ( 'NONE',  ( 0.3215223097112867578, -0.05778040916215522460, 0.4822834645669289988 ) ) ;
#45826=CARTESIAN_POINT ( 'NONE',  ( 0.1706036745406830368, 0.05413385826771666132, 0.4176697321401328100 ) ) ;
#45827=CARTESIAN_POINT ( 'NONE',  ( -0.9580052493438311334, -0.4281496062992124485, 0.4176697321401328655 ) ) ;
#45828=CARTESIAN_POINT ( 'NONE',  ( 1.482939632545932307, -0.3690944881889763329, 0.3153832671262228327 ) ) ;
#45829=CARTESIAN_POINT ( 'NONE',  ( -1.535433070866141225, -0.6692913385826771977, 8.415575281601705876E-17 ) ) ;
#45831=CARTESIAN_POINT ( 'NONE',  ( 1.010498687664042716, -0.004921259842519870586, -0.3153832671262229437 ) ) ;
#45832=CARTESIAN_POINT ( 'NONE',  ( 0.4658792650918641698, -0.05778040916215560624, -0.4822834645669293319 ) ) ;
#45833=CARTESIAN_POINT ( 'NONE',  ( 0.9186351706036752773, 0.2306618581243847221, -0.2411417322834647770 ) ) ;
#45836=CARTESIAN_POINT ( 'NONE',  ( -1.692913385826770645, 0.2952755905511811885, 0.000000000000000000 ) ) ;
#45839=CARTESIAN_POINT ( 'NONE',  ( -0.1771653543307080136, -0.5400638737290844871, 0.3530559997133364547 ) ) ;
#45842=CARTESIAN_POINT ( 'NONE',  ( -1.128608923884513837, 0.1283753931104746893, -0.1820866141732285504 ) ) ;
#45843=CARTESIAN_POINT ( 'NONE',  ( 1.181102362204724976, -0.1870078740157480879, -0.4822834645669291653 ) ) ;
#45844=CARTESIAN_POINT ( 'NONE',  ( 1.135170603674541256, -0.6692913385826773087, -0.1292274648535924053 ) ) ;
#45845=CARTESIAN_POINT ( 'NONE',  ( -0.1640419947506553400, -0.08942795157528024563, -0.3641732283464568787 ) ) ;
#45846=CARTESIAN_POINT ( 'NONE',  ( 0.3674540682414705883, 0.2306618581243847221, -0.2411417322834647770 ) ) ;
#45848=CARTESIAN_POINT ( 'NONE',  ( 0.2296587926509192634, -0.2845877964562159024, 0.3641732283464567677 ) ) ;
#45849=CARTESIAN_POINT ( 'NONE',  ( 0.09186351706036799403, -0.4281496062992127816, -0.4176697321401328100 ) ) ;
#45851=CARTESIAN_POINT ( 'NONE',  ( -1.161417322834644716, -0.5400638737290845981, -0.3530559997133363437 ) ) ;
#45852=CARTESIAN_POINT ( 'NONE',  ( 0.4790026246719167324, -0.08942795157527998196, 0.3641732283464567121 ) ) ;
#45854=CARTESIAN_POINT ( 'NONE',  ( 0.4687358108553562053, 1.787282772535974340, 0.5180085934481408749 ) ) ;
#45855=CARTESIAN_POINT ( 'NONE',  ( -0.5905511811023615998, 0.2952755905511811885, 0.000000000000000000 ) ) ;
#45856=CARTESIAN_POINT ( 'NONE',  ( -0.4921259842519677963, 0.07958543189024071263, -0.2665933059059888421 ) ) ;
#45857=CARTESIAN_POINT ( 'NONE',  ( -1.604771003085130543, 0.4514378173630710367, -0.1466069496707740061 ) ) ;
#45858=CARTESIAN_POINT ( 'NONE',  ( -0.6299212598425188991, -0.1870078740157479769, 0.4822834645669291653 ) ) ;
#45859=CARTESIAN_POINT ( 'NONE',  ( -0.1902887139107604098, 0.2952755905511810774, -0.1292274648535930714 ) ) ;
#45860=CARTESIAN_POINT ( 'NONE',  ( 0.3018372703412079971, -0.3690944881889763329, 0.3153832671262228327 ) ) ;
#45862=CARTESIAN_POINT ( 'NONE',  ( 0.05249343832021075018, -0.6046776061558807314, 0.2411417322834647770 ) ) ;
#45864=CARTESIAN_POINT ( 'NONE',  ( -1.463254593175852492, -0.5511811023622048555, -0.09757992244046775898 ) ) ;
#45865=CARTESIAN_POINT ( 'NONE',  ( 0.5905511811023629321, 0.1771653543307087630, 0.000000000000000000 ) ) ;
#45866=CARTESIAN_POINT ( 'NONE',  ( 1.364829396325459854, -0.6046776061558809534, -0.2411417322834644161 ) ) ;
#45867=CARTESIAN_POINT ( 'NONE',  ( -0.9251968503937002541, 0.07958543189024085140, 0.2665933059059887866 ) ) ;
#45868=CARTESIAN_POINT ( 'NONE',  ( -1.181102362204723644, -0.1870078740157480601, -0.3641732283464567677 ) ) ;
#45869=CARTESIAN_POINT ( 'NONE',  ( -0.7874015748031489847, -0.1870078740157480879, -0.4822834645669291653 ) ) ;
#45870=CARTESIAN_POINT ( 'NONE',  ( -0.09842519685039295696, 0.1660481256975883668, -0.3530559997133364547 ) ) ;
#45871=CARTESIAN_POINT ( 'NONE',  ( 0.5971128608923891301, 0.1771653543307087075, -0.09757992244046823083 ) ) ;
#45873=CARTESIAN_POINT ( 'NONE',  ( 0.8858267716535438430, -0.4536011799217368745, -0.2665933059059886201 ) ) ;
#45874=CARTESIAN_POINT ( 'NONE',  ( 0.1837270341207357105, -0.6046776061558809534, -0.2411417322834644161 ) ) ;
#45876=CARTESIAN_POINT ( 'NONE',  ( -0.5249343832020990641, -0.6046776061558809534, -0.2411417322834644161 ) ) ;
#45878=CARTESIAN_POINT ( 'NONE',  ( 1.397637795275591177, -0.4536011799217367080, 0.2665933059059888421 ) ) ;
#45879=CARTESIAN_POINT ( 'NONE',  ( 0.4199475065616805614, 0.2306618581243848609, 0.2411417322834645549 ) ) ;
#45880=CARTESIAN_POINT ( 'NONE',  ( 0.2493438320209980519, 0.05413385826771666132, 0.4176697321401328100 ) ) ;
#45881=FACE_OUTER_BOUND ( 'NONE', #31874, .T. ) ;
#45882=CARTESIAN_POINT ( 'NONE',  ( -0.006561679790025524116, -0.08942795157528024563, -0.3641732283464568787 ) ) ;
#45883=CARTESIAN_POINT ( 'NONE',  ( 0.8333333333333340365, -0.6692913385826771977, 0.1292274648535927661 ) ) ;
#45884=CARTESIAN_POINT ( 'NONE',  ( -0.2690288713910754526, 0.1771653543307087075, -0.09757992244046823083 ) ) ;
#45885=CARTESIAN_POINT ( 'NONE',  ( -0.8464566929133852113, 0.1660481256975885056, 0.3530559997133364547 ) ) ;
#45887=CARTESIAN_POINT ( 'NONE',  ( -0.06561679790026180015, -0.4281496062992127816, -0.4176697321401328100 ) ) ;
#45889=CARTESIAN_POINT ( 'NONE',  ( -1.036745406824146176, -0.4281496062992124485, 0.4176697321401328655 ) ) ;
#45890=CARTESIAN_POINT ( 'NONE',  ( -0.5380577427821514602, -0.3690944881889765550, -0.3153832671262227771 ) ) ;
#45892=CARTESIAN_POINT ( 'NONE',  ( 0.006561679790026889343, -0.05778040916215522460, 0.4822834645669289988 ) ) ;
#45893=CARTESIAN_POINT ( 'NONE',  ( -1.161417322834644716, -0.5400638737290845981, -0.3530559997133363437 ) ) ;
#45894=CARTESIAN_POINT ( 'NONE',  ( -0.9251968503937002541, -0.5400638737290845981, -0.3530559997133363437 ) ) ;
#45895=CARTESIAN_POINT ( 'NONE',  ( 1.220472440944882386, 0.000000000000000000, 0.4445507791589061175 ) ) ;
#45896=CARTESIAN_POINT ( 'NONE',  ( 0.4665770185116077107, 1.519790403714398108, -0.5309055118110237448 ) ) ;
#45897=CARTESIAN_POINT ( 'NONE',  ( 1.017060367454068581, -0.05778040916215560624, -0.4822834645669293319 ) ) ;
#45898=CARTESIAN_POINT ( 'NONE',  ( 1.089238845144357759, 0.05413385826771626580, -0.4176697321401330321 ) ) ;
#45900=CARTESIAN_POINT ( 'NONE',  ( 1.541994750656168645, -0.6692913385826771977, 0.1292274648535927661 ) ) ;
#45901=CARTESIAN_POINT ( 'NONE',  ( -1.522309711286088607, 0.2306618581243847221, -0.2411417322834647770 ) ) ;
#45905=CARTESIAN_POINT ( 'NONE',  ( -0.1049868766404193215, -0.5023911411419708095, 0.1820866141732285504 ) ) ;
#45908=CARTESIAN_POINT ( 'NONE',  ( 0.08530183727034192087, -0.3162353388693409650, -0.4822834645669289433 ) ) ;
#45909=CARTESIAN_POINT ( 'NONE',  ( 0.006561679790026889343, -0.05778040916215522460, 0.4822834645669289988 ) ) ;
#45911=DIRECTION ( 'NONE',  ( -0.000000000000000000, 1.000000000000000000, -0.000000000000000000 ) ) ;
#45912=CARTESIAN_POINT ( 'NONE',  ( -0.8989501312335946848, -0.5511811023622046335, 0.09757992244046803654 ) ) ;
#45914=CARTESIAN_POINT ( 'NONE',  ( 0.7677165354330716118, 0.1660481256975883668, -0.3530559997133364547 ) ) ;
#45915=CARTESIAN_POINT ( 'NONE',  ( 0.9120734908136489683, -0.5511811023622046335, 0.09757992244046803654 ) ) ;
#45916=CARTESIAN_POINT ( 'NONE',  ( -0.3740157480314953431, 0.1660481256975885056, 0.3530559997133364547 ) ) ;
#45918=CARTESIAN_POINT ( 'NONE',  ( -0.9251968503937002541, -0.5400638737290845981, -0.3530559997133363437 ) ) ;
#45920=CARTESIAN_POINT ( 'NONE',  ( 1.345144356955381593, -0.05778040916215522460, 0.4822834645669289988 ) ) ;
#45921=CARTESIAN_POINT ( 'NONE',  ( 1.561679790026247350, -0.004921259842519870586, -0.3153832671262229437 ) ) ;
#45922=ORIENTED_EDGE ( 'NONE', *, *, #64052, .F. ) ;
#45924=CARTESIAN_POINT ( 'NONE',  ( -0.006561679790025524116, -0.05778040916215560624, -0.4822834645669293319 ) ) ;
#45926=CARTESIAN_POINT ( 'NONE',  ( -0.7480314960629914633, 0.2952755905511811885, 0.000000000000000000 ) ) ;
#45927=CARTESIAN_POINT ( 'NONE',  ( 1.200787401574803681, -0.5400638737290845981, -0.3530559997133363437 ) ) ;
#45928=CARTESIAN_POINT ( 'NONE',  ( 1.240157480314961314, -0.5400638737290844871, 0.3530559997133364547 ) ) ;
#45929=CARTESIAN_POINT ( 'NONE',  ( 0.2099737532808405305, 0.2306618581243847221, -0.2411417322834647770 ) ) ;
#45930=CARTESIAN_POINT ( 'NONE',  ( -0.3280839895013117347, 0.05413385826771626580, -0.4176697321401330321 ) ) ;
#45932=CARTESIAN_POINT ( 'NONE',  ( -1.332020997375327642, -0.3162353388693409650, -0.4822834645669289433 ) ) ;
#45933=CARTESIAN_POINT ( 'NONE',  ( -0.1574803149606292529, -0.1870078740157480879, -0.4822834645669291653 ) ) ;
#45934=CARTESIAN_POINT ( 'NONE',  ( -0.01312335958005186876, -0.004921259842519870586, -0.3153832671262229437 ) ) ;
#45936=EDGE_CURVE ( 'NONE', #16761, #4749, #70336, .T. ) ;
#45937=CARTESIAN_POINT ( 'NONE',  ( 1.404199475065617708, 0.05413385826771626580, -0.4176697321401330321 ) ) ;
#45938=CARTESIAN_POINT ( 'NONE',  ( -0.5643044619422565855, 0.05413385826771626580, -0.4176697321401330321 ) ) ;
#45939=LINE ( 'NONE', #39645, #74908 ) ;
#45940=CARTESIAN_POINT ( 'NONE',  ( 1.141732283464567566, 0.2952755905511811885, 0.000000000000000000 ) ) ;
#45941=CARTESIAN_POINT ( 'NONE',  ( 0.5314960629921265944, 0.1012011053420775880, -0.2882089793578257453 ) ) ;
#45942=EDGE_CURVE ( 'NONE', #8792, #10560, #65155, .T. ) ;
#45944=CARTESIAN_POINT ( 'NONE',  ( 0.4658792650918641698, -0.05778040916215560624, -0.4822834645669293319 ) ) ;
#45945=CARTESIAN_POINT ( 'NONE',  ( -0.3871391076115479057, -0.2845877964562161244, -0.3641732283464567121 ) ) ;
#45946=CARTESIAN_POINT ( 'NONE',  ( 1.095800524934383846, -0.08942795157528024563, -0.3641732283464568787 ) ) ;
#45949=CARTESIAN_POINT ( 'NONE',  ( 1.633858267716535639, -0.4536011799217367080, 0.2665933059059888421 ) ) ;
#45950=CARTESIAN_POINT ( 'NONE',  ( 1.391076115485564868, -0.6046776061558807314, 0.2411417322834647770 ) ) ;
#45953=CARTESIAN_POINT ( 'NONE',  ( 0.05905511811023681640, 0.1660481256975883668, -0.3530559997133364547 ) ) ;
#45954=CARTESIAN_POINT ( 'NONE',  ( -1.620734908136482577, 0.2952755905511811885, 0.1292274648535926551 ) ) ;
#45955=CARTESIAN_POINT ( 'NONE',  ( -1.496062992125983815, -0.1870078740157480879, -0.4822834645669291653 ) ) ;
#45956=CARTESIAN_POINT ( 'NONE',  ( -0.09842519685039295696, 0.1660481256975883668, -0.3530559997133364547 ) ) ;
#45958=CARTESIAN_POINT ( 'NONE',  ( 1.633858267716535639, -0.5400638737290844871, 0.3530559997133364547 ) ) ;
#45959=CARTESIAN_POINT ( 'NONE',  ( 0.4921259842519691285, 0.1660481256975885056, 0.3530559997133364547 ) ) ;
#45961=CARTESIAN_POINT ( 'NONE',  ( 0.9842519685039378130, -0.5511811023622047445, 6.969142054262312111E-17 ) ) ;
#45962=CARTESIAN_POINT ( 'NONE',  ( -0.05249343832020911260, 0.2306618581243848609, 0.2411417322834645549 ) ) ;
#45963=CARTESIAN_POINT ( 'NONE',  ( 1.036745406824147731, -0.004921259842519576551, 0.3153832671262227771 ) ) ;
#45964=CARTESIAN_POINT ( 'NONE',  ( -1.167979002624671470, 0.05413385826771666132, 0.4176697321401328100 ) ) ;
#45966=CARTESIAN_POINT ( 'NONE',  ( 1.017060367454068803, -0.3162353388693405765, 0.4822834645669290543 ) ) ;
#45969=EDGE_CURVE ( 'NONE', #48621, #69752, #28826, .T. ) ;
#45970=CARTESIAN_POINT ( 'NONE',  ( 0.5905511811023629321, 0.2952755905511811885, 0.000000000000000000 ) ) ;
#45973=CARTESIAN_POINT ( 'NONE',  ( 0.5708661417322841158, -0.4536011799217368745, -0.2665933059059886201 ) ) ;
#45974=CARTESIAN_POINT ( 'NONE',  ( 0.6561679790026253567, -0.6046776061558809534, -0.2411417322834644161 ) ) ;
#45975=CARTESIAN_POINT ( 'NONE',  ( 0.7214341416610914326, 0.004960608223780192325, 0.3437734562760181856 ) ) ;
#45976=CARTESIAN_POINT ( 'NONE',  ( -0.9973753280839886548, -0.5023911411419708095, -0.1820866141732282451 ) ) ;
#45977=CARTESIAN_POINT ( 'NONE',  ( -1.181102362204723644, -0.1870078740157480879, -0.4822834645669291653 ) ) ;
#45978=CARTESIAN_POINT ( 'NONE',  ( -1.450131233595799651, -0.6692913385826771977, 0.1292274648535927661 ) ) ;
#45979=CARTESIAN_POINT ( 'NONE',  ( 0.7677165354330716118, 0.1660481256975883668, -0.3530559997133364547 ) ) ;
#45980=CARTESIAN_POINT ( 'NONE',  ( -1.607611548556429737, 0.1771653543307087075, -0.09757992244046823083 ) ) ;
#45982=CARTESIAN_POINT ( 'NONE',  ( 0.8136482939632553313, 0.2306618581243848609, 0.2411417322834645549 ) ) ;
#45985=CARTESIAN_POINT ( 'NONE',  ( 1.338582677165355062, -0.1870078740157479769, 0.4822834645669291653 ) ) ;
#45986=CARTESIAN_POINT ( 'NONE',  ( -1.456692913385826182, -0.5511811023622047445, 6.969142054262312111E-17 ) ) ;
#45987=CARTESIAN_POINT ( 'NONE',  ( 1.062992125984252745, 0.1771653543307087630, 0.000000000000000000 ) ) ;
#45988=CARTESIAN_POINT ( 'NONE',  ( -1.213910761154854745, -0.5511811023622046335, 0.09757992244046803654 ) ) ;
#45989=CARTESIAN_POINT ( 'NONE',  ( -0.5511811023622038563, -0.1870078740157479769, 0.3641732283464567677 ) ) ;
#45991=CARTESIAN_POINT ( 'NONE',  ( 0.8530183727034126306, -0.004921259842519870586, -0.3153832671262229437 ) ) ;
#45992=CARTESIAN_POINT ( 'NONE',  ( 0.4724409448818904789, -0.1870078740157480879, -0.4822834645669291653 ) ) ;
#45993=CARTESIAN_POINT ( 'NONE',  ( 0.9776902887139113929, 0.2952755905511811885, 0.1292274648535926551 ) ) ;
#45994=CARTESIAN_POINT ( 'NONE',  ( 0.2493438320209980519, 0.05413385826771666132, 0.4176697321401328100 ) ) ;
#45995=CARTESIAN_POINT ( 'NONE',  ( 0.5905511811023629321, -0.5511811023622047445, 6.969142054262312111E-17 ) ) ;
#45997=CARTESIAN_POINT ( 'NONE',  ( 1.200787401574803681, -0.5400638737290845981, -0.3530559997133363437 ) ) ;
#45998=CARTESIAN_POINT ( 'NONE',  ( -0.1837270341207340729, 0.1539470093639521697, -0.1968503937007875793 ) ) ;
#45999=CARTESIAN_POINT ( 'NONE',  ( -0.5118110236220466680, -0.6692913385826771977, 8.415575281601705876E-17 ) ) ;
#46002=CARTESIAN_POINT ( 'NONE',  ( 5.463695987328526437E-16, -0.1870078740157479769, 0.4822834645669291653 ) ) ;
#46003=CARTESIAN_POINT ( 'NONE',  ( -0.5511811023622038563, -0.1870078740157479769, 0.4822834645669291653 ) ) ;
#46004=CARTESIAN_POINT ( 'NONE',  ( 0.1181102362204730916, -0.6692913385826771977, 8.415575281601705876E-17 ) ) ;
#46010=CARTESIAN_POINT ( 'NONE',  ( -0.9514435695538050464, -0.2845877964562159024, 0.3641732283464567677 ) ) ;
#46012=CARTESIAN_POINT ( 'NONE',  ( -1.371391076115484831, 0.2952755905511810774, -0.1292274648535930714 ) ) ;
#46013=VECTOR ( 'NONE', #3064, 39.37007874015748143 ) ;
#46016=CARTESIAN_POINT ( 'NONE',  ( 0.6364829396325465405, -0.3162353388693409650, -0.4822834645669289433 ) ) ;
#46017=CARTESIAN_POINT ( 'NONE',  ( -0.3805774278215216522, -0.3690944881889765550, -0.3153832671262227771 ) ) ;
#46018=CARTESIAN_POINT ( 'NONE',  ( 1.095800524934383846, -0.3162353388693405765, 0.4822834645669290543 ) ) ;
#46019=CARTESIAN_POINT ( 'NONE',  ( 0.5643044619422579178, -0.4281496062992127816, -0.4176697321401328100 ) ) ;
#46023=CARTESIAN_POINT ( 'NONE',  ( 1.194225721784777594, 0.05413385826771666132, 0.4176697321401328100 ) ) ;
#46024=CARTESIAN_POINT ( 'NONE',  ( 0.5774278215223103139, -0.6046776061558809534, -0.2411417322834644161 ) ) ;
#46025=CARTESIAN_POINT ( 'NONE',  ( 0.1902887139107617975, 0.2952755905511811885, 0.1292274648535926551 ) ) ;
#46026=CARTESIAN_POINT ( 'NONE',  ( 1.548556430446194954, -0.6046776061558807314, 0.2411417322834647770 ) ) ;
#46027=CARTESIAN_POINT ( 'NONE',  ( 0.7611548556430454138, 0.2306618581243847221, -0.2411417322834647770 ) ) ;
#46029=CARTESIAN_POINT ( 'NONE',  ( -0.1181102362204717315, 0.2952755905511811885, 0.000000000000000000 ) ) ;
#46030=CARTESIAN_POINT ( 'NONE',  ( 1.082677165354331228, 0.1660481256975883668, -0.3530559997133364547 ) ) ;
#46031=CARTESIAN_POINT ( 'NONE',  ( 0.4855643044619430415, -0.4281496062992127816, -0.4176697321401328100 ) ) ;
#46032=CARTESIAN_POINT ( 'NONE',  ( 1.017060367454068803, -0.2845877964562159024, 0.3641732283464567677 ) ) ;
#46033=CARTESIAN_POINT ( 'NONE',  ( -0.8267716535433065062, -0.6692913385826771977, 8.415575281601705876E-17 ) ) ;
#46034=CARTESIAN_POINT ( 'NONE',  ( -1.430446194225721390, -0.4281496062992124485, 0.4176697321401328655 ) ) ;
#46035=CARTESIAN_POINT ( 'NONE',  ( 0.6561679790026253567, 0.2306618581243848609, 0.2411417322834645549 ) ) ;
#46038=EDGE_CURVE ( 'NONE', #24368, #21487, #35979, .T. ) ;
#46042=CARTESIAN_POINT ( 'NONE',  ( 1.515748031496063408, 0.1660481256975885056, 0.3530559997133364547 ) ) ;
#46043=CARTESIAN_POINT ( 'NONE',  ( 0.8398950131233602345, 0.1283753931104746893, -0.1820866141732285504 ) ) ;
#46049=CARTESIAN_POINT ( 'NONE',  ( -1.049868766404198794, -0.5023911411419708095, 0.1820866141732285504 ) ) ;
#46050=CARTESIAN_POINT ( 'NONE',  ( 1.541994750656168645, -0.6692913385826771977, 0.1292274648535927661 ) ) ;
#46052=CARTESIAN_POINT ( 'NONE',  ( -0.3412073490813641308, -0.6046776061558807314, 0.2411417322834647770 ) ) ;
#46053=CARTESIAN_POINT ( 'NONE',  ( 1.010498687664042716, 0.05413385826771626580, -0.4176697321401330321 ) ) ;
#46054=ORIENTED_EDGE ( 'NONE', *, *, #25485, .T. ) ;
#46055=CARTESIAN_POINT ( 'NONE',  ( -1.666666666666665853, 0.05413385826771626580, -0.4176697321401330321 ) ) ;
#46058=CARTESIAN_POINT ( 'NONE',  ( 1.614173228346457378, 1.267785121476991073, -0.1372047244094476148 ) ) ;
#46059=CARTESIAN_POINT ( 'NONE',  ( -0.8792650918635160906, -0.3690944881889763329, 0.3153832671262228327 ) ) ;
#46061=CARTESIAN_POINT ( 'NONE',  ( -1.476377952755905110, 0.1660481256975885056, 0.3530559997133364547 ) ) ;
#46062=CARTESIAN_POINT ( 'NONE',  ( 0.4921259842519691285, -0.5400638737290845981, -0.3530559997133363437 ) ) ;
#46063=ORIENTED_EDGE ( 'NONE', *, *, #27570, .F. ) ;
#46065=CARTESIAN_POINT ( 'NONE',  ( -0.4593175853018366950, 0.009842519685039463617, 0.3409548833797002576 ) ) ;
#46067=CARTESIAN_POINT ( 'NONE',  ( 0.8923884514435703741, 0.2306618581243848609, 0.2411417322834645549 ) ) ;
#46068=CARTESIAN_POINT ( 'NONE',  ( 1.509186351706037543, -0.3690944881889765550, -0.3153832671262227771 ) ) ;
#46071=CARTESIAN_POINT ( 'NONE',  ( -0.8989501312335946848, 0.1771653543307087075, -0.09757992244046823083 ) ) ;
#46072=CARTESIAN_POINT ( 'NONE',  ( -1.653543307086613234, -0.1870078740157479769, 0.3641732283464567677 ) ) ;
#46074=CARTESIAN_POINT ( 'NONE',  ( 0.5643044619422579178, -0.4281496062992127816, -0.4176697321401328100 ) ) ;
#46075=CARTESIAN_POINT ( 'NONE',  ( -0.7677165354330699465, -0.4536011799217368745, -0.2665933059059886201 ) ) ;
#46076=CARTESIAN_POINT ( 'NONE',  ( 0.1640419947506569498, -0.08942795157527998196, 0.3641732283464567121 ) ) ;
#46077=CARTESIAN_POINT ( 'NONE',  ( -0.2493438320209966919, 0.05413385826771626580, -0.4176697321401330321 ) ) ;
#46078=CARTESIAN_POINT ( 'NONE',  ( -1.128608923884513837, 0.1283753931104746893, -0.1820866141732285504 ) ) ;
#46080=CARTESIAN_POINT ( 'NONE',  ( 0.7545931758530188826, -0.6692913385826771977, 0.1292274648535927661 ) ) ;
#46081=CARTESIAN_POINT ( 'NONE',  ( -1.476377952755905110, 0.1660481256975885056, 0.3530559997133364547 ) ) ;
#46083=CARTESIAN_POINT ( 'NONE',  ( -0.8792650918635160906, 0.05413385826771626580, -0.4176697321401330321 ) ) ;
#46084=CARTESIAN_POINT ( 'NONE',  ( -0.2559055118110230564, 0.07958543189024071263, -0.2665933059059888421 ) ) ;
#46085=EDGE_CURVE ( 'NONE', #38268, #43230, #66730, .T. ) ;
#46086=CARTESIAN_POINT ( 'NONE',  ( -1.535433070866141225, -0.6692913385826771977, 8.415575281601705876E-17 ) ) ;
#46087=CARTESIAN_POINT ( 'NONE',  ( 0.7742782152230979209, -0.004921259842519870586, -0.3153832671262229437 ) ) ;
#46088=CARTESIAN_POINT ( 'NONE',  ( -0.3740157480314953431, -0.4536011799217368745, -0.2665933059059886201 ) ) ;
#46089=CARTESIAN_POINT ( 'NONE',  ( -0.8661417322834640276, -0.1870078740157480879, -0.4822834645669291653 ) ) ;
#46090=CARTESIAN_POINT ( 'NONE',  ( -1.246719160104986512, 0.05413385826771666132, 0.4176697321401328100 ) ) ;
#46091=CARTESIAN_POINT ( 'NONE',  ( -1.397637795275589623, -0.5400638737290845981, -0.3530559997133363437 ) ) ;
#46093=CARTESIAN_POINT ( 'NONE',  ( 1.417322834645670104, -0.1870078740157480601, -0.3641732283464567677 ) ) ;
#46094=CARTESIAN_POINT ( 'NONE',  ( 0.5708661417322842269, 0.1660481256975885056, 0.3530559997133364547 ) ) ;
#46096=CARTESIAN_POINT ( 'NONE',  ( -1.489501312335957062, -0.05778040916215522460, 0.4822834645669289988 ) ) ;
#46097=CARTESIAN_POINT ( 'NONE',  ( -1.732283464566928277, -0.1870078740157479769, 0.4822834645669291653 ) ) ;
#46098=ORIENTED_EDGE ( 'NONE', *, *, #47242, .F. ) ;
#46100=CARTESIAN_POINT ( 'NONE',  ( -0.9580052493438311334, -0.004921259842519870586, -0.3153832671262229437 ) ) ;
#46101=CARTESIAN_POINT ( 'NONE',  ( 0.5708661417322841158, -0.5400638737290845981, -0.3530559997133363437 ) ) ;
#46102=CARTESIAN_POINT ( 'NONE',  ( -1.220472440944881054, 0.1771653543307087630, 0.000000000000000000 ) ) ;
#46104=CARTESIAN_POINT ( 'NONE',  ( -1.509186351706035767, 0.05413385826771626580, -0.4176697321401330321 ) ) ;
#46105=CARTESIAN_POINT ( 'NONE',  ( 0.7808398950131241190, -0.05778040916215560624, -0.4822834645669293319 ) ) ;
#46106=CARTESIAN_POINT ( 'NONE',  ( 0.4724409448818904789, -0.1870078740157480879, -0.4822834645669291653 ) ) ;
#46107=CARTESIAN_POINT ( 'NONE',  ( 1.148293963254593653, 0.2952755905511810774, -0.1292274648535930714 ) ) ;
#46108=CARTESIAN_POINT ( 'NONE',  ( -1.719160104986876103, -0.004921259842519576551, 0.3153832671262227771 ) ) ;
#46114=CARTESIAN_POINT ( 'NONE',  ( 0.6496062992125991586, -0.4536011799217368745, -0.2665933059059886201 ) ) ;
#46115=CARTESIAN_POINT ( 'NONE',  ( 0.4724409448818904789, -0.1870078740157479769, 0.3641732283464567677 ) ) ;
#46116=CARTESIAN_POINT ( 'NONE',  ( -0.1049868766404193215, 0.2306618581243847221, -0.2411417322834647770 ) ) ;
#46117=CARTESIAN_POINT ( 'NONE',  ( 1.476377952755906220, 0.1660481256975883668, -0.3530559997133364547 ) ) ;
#46119=CARTESIAN_POINT ( 'NONE',  ( 0.3149606299212606708, -0.1870078740157480601, -0.3641732283464567677 ) ) ;
#46120=CARTESIAN_POINT ( 'NONE',  ( -0.8202099737532799750, 0.2952755905511810774, -0.1292274648535930714 ) ) ;
#46121=CARTESIAN_POINT ( 'NONE',  ( -1.502624671916009680, -0.3162353388693405765, 0.4822834645669290543 ) ) ;
#46122=CARTESIAN_POINT ( 'NONE',  ( 0.9973753280839902091, -0.6046776061558807314, 0.2411417322834647770 ) ) ;
#46126=ORIENTED_EDGE ( 'NONE', *, *, #45224, .F. ) ;
#46128=CARTESIAN_POINT ( 'NONE',  ( -1.272965879265091305, -0.4281496062992124485, 0.4176697321401328655 ) ) ;
#46129=CARTESIAN_POINT ( 'NONE',  ( -0.9120734908136475250, -0.5511811023622048555, -0.09757992244046775898 ) ) ;
#46130=CARTESIAN_POINT ( 'NONE',  ( -1.279527559055116948, 0.1660481256975883668, -0.3530559997133364547 ) ) ;
#46132=DIRECTION ( 'NONE',  ( 0.000000000000000000, 1.000000000000000000, 0.000000000000000000 ) ) ;
#46133=CARTESIAN_POINT ( 'NONE',  ( 1.587926509186352586, -0.4281496062992127816, -0.4176697321401328100 ) ) ;
#46134=CARTESIAN_POINT ( 'NONE',  ( -1.299212598425196097, -0.6692913385826771977, 8.415575281601705876E-17 ) ) ;
#46135=CARTESIAN_POINT ( 'NONE',  ( 0.3346456692913390985, 0.1660481256975885056, 0.3530559997133364547 ) ) ;
#46136=CARTESIAN_POINT ( 'NONE',  ( -1.069553805774277722, -0.6692913385826773087, -0.1292274648535924053 ) ) ;
#46138=CARTESIAN_POINT ( 'NONE',  ( 0.6364829396325465405, -0.05778040916215522460, 0.4822834645669289988 ) ) ;
#46140=CARTESIAN_POINT ( 'NONE',  ( -0.8792650918635160906, -0.3690944881889763329, 0.3153832671262228327 ) ) ;
#46145=CARTESIAN_POINT ( 'NONE',  ( -1.010498687664041384, -0.4281496062992127816, -0.4176697321401328100 ) ) ;
#46146=CARTESIAN_POINT ( 'NONE',  ( -1.469816272965878357, 0.2306618581243848609, 0.2411417322834645549 ) ) ;
#46148=CARTESIAN_POINT ( 'NONE',  ( -1.660104986876639543, -0.05778040916215560624, -0.4822834645669293319 ) ) ;
#46149=CARTESIAN_POINT ( 'NONE',  ( -1.286089238845143479, -0.6046776061558807314, 0.2411417322834647770 ) ) ;
#46150=CARTESIAN_POINT ( 'NONE',  ( -1.646981627296586703, -0.05778040916215522460, 0.4822834645669289988 ) ) ;
#46151=CARTESIAN_POINT ( 'NONE',  ( -1.595398199321655497, 1.839868176060737159, 0.1559797534342489411 ) ) ;
#46152=CARTESIAN_POINT ( 'NONE',  ( -0.8333333333333323711, 0.2952755905511811885, 0.1292274648535926551 ) ) ;
#46153=CARTESIAN_POINT ( 'NONE',  ( 0.01312335958005323398, -0.3690944881889765550, -0.3153832671262227771 ) ) ;
#46154=CARTESIAN_POINT ( 'NONE',  ( 1.614173228346457378, 0.5038684218300975015, 0.1372047244094478369 ) ) ;
#46156=CARTESIAN_POINT ( 'NONE',  ( -0.4986876640419942164, -0.5023911411419708095, 0.1820866141732285504 ) ) ;
#46157=CARTESIAN_POINT ( 'NONE',  ( -0.8070866141732276899, 0.1660481256975883668, -0.3530559997133364547 ) ) ;
#46158=CARTESIAN_POINT ( 'NONE',  ( 0.9776902887139113929, 0.2952755905511811885, 0.1292274648535926551 ) ) ;
#46159=CARTESIAN_POINT ( 'NONE',  ( -1.082677165354329896, -0.5400638737290845981, -0.3530559997133363437 ) ) ;
#46160=VERTEX_POINT ( 'NONE', #80201 ) ;
#46162=CARTESIAN_POINT ( 'NONE',  ( -0.8464566929133852113, 0.1660481256975885056, 0.3530559997133364547 ) ) ;
#46163=CARTESIAN_POINT ( 'NONE',  ( 0.9055118110236227702, -0.6692913385826771977, 8.415575281601705876E-17 ) ) ;
#46164=CARTESIAN_POINT ( 'NONE',  ( -1.351706036745406347, -0.004921259842519870586, -0.3153832671262229437 ) ) ;
#46169=CARTESIAN_POINT ( 'NONE',  ( -0.4330708661417315697, -0.6692913385826771977, 8.415575281601705876E-17 ) ) ;
#46170=CARTESIAN_POINT ( 'NONE',  ( -1.555118110236219930, -0.4536011799217368745, -0.2665933059059886201 ) ) ;
#46171=CARTESIAN_POINT ( 'NONE',  ( -0.5971128608923877978, 0.2952755905511811885, 0.1292274648535926551 ) ) ;
#46173=CARTESIAN_POINT ( 'NONE',  ( -1.404199475065615932, 0.05413385826771666132, 0.4176697321401328100 ) ) ;
#46175=CARTESIAN_POINT ( 'NONE',  ( -0.9383202099737524282, -0.05778040916215522460, 0.4822834645669289988 ) ) ;
#46176=CARTESIAN_POINT ( 'NONE',  ( -0.2755905511811018171, 0.2952755905511811885, 0.000000000000000000 ) ) ;
#46178=CARTESIAN_POINT ( 'NONE',  ( 0.2755905511811031494, -0.5511811023622047445, 6.969142054262312111E-17 ) ) ;
#46179=CARTESIAN_POINT ( 'NONE',  ( 1.220472440944879722, 2.401574803149606474, 0.5309055118110233007 ) ) ;
#46180=CARTESIAN_POINT ( 'NONE',  ( 0.4199475065616805614, 0.1283753931104748280, 0.1820866141732283561 ) ) ;
#46181=CARTESIAN_POINT ( 'NONE',  ( 1.377952755905512472, -0.5511811023622047445, 6.969142054262312111E-17 ) ) ;
#46182=CARTESIAN_POINT ( 'NONE',  ( 1.305774278215223960, 0.2952755905511810774, -0.1292274648535930714 ) ) ;
#46183=CARTESIAN_POINT ( 'NONE',  ( 0.1049868766404206816, 0.1283753931104748280, 0.1820866141732283561 ) ) ;
#46185=CARTESIAN_POINT ( 'NONE',  ( -1.437007874015747477, 0.1660481256975883668, -0.3530559997133364547 ) ) ;
#46186=CARTESIAN_POINT ( 'NONE',  ( 1.430446194225722500, 0.05413385826771666132, 0.4176697321401328100 ) ) ;
#46188=CARTESIAN_POINT ( 'NONE',  ( -0.4724409448818890911, -0.1870078740157480601, -0.3641732283464567677 ) ) ;
#46191=CARTESIAN_POINT ( 'NONE',  ( 0.1968503937007881344, -0.6692913385826771977, 8.415575281601705876E-17 ) ) ;
#46194=CARTESIAN_POINT ( 'NONE',  ( 0.7677165354330716118, -0.4536011799217367080, 0.2665933059059888421 ) ) ;
#46195=CARTESIAN_POINT ( 'NONE',  ( 0.2559055118110243332, -0.4536011799217368745, -0.2665933059059886201 ) ) ;
#46196=CARTESIAN_POINT ( 'NONE',  ( -0.1640419947506553400, -0.05778040916215560624, -0.4822834645669293319 ) ) ;
#46197=CARTESIAN_POINT ( 'NONE',  ( -1.712598425196849572, 0.1660481256975885056, 0.3530559997133364547 ) ) ;
#46198=CARTESIAN_POINT ( 'NONE',  ( -0.5577427821522301654, -0.2845877964562159024, 0.3641732283464567677 ) ) ;
#46200=CARTESIAN_POINT ( 'NONE',  ( 0.4002624671916016896, -0.05778040916215522460, 0.4822834645669289988 ) ) ;
#46201=CARTESIAN_POINT ( 'NONE',  ( -0.8923884514435688198, -0.6046776061558807314, 0.2411417322834647770 ) ) ;
#46205=CARTESIAN_POINT ( 'NONE',  ( 0.2034120734908142214, 0.1771653543307087075, -0.09757992244046823083 ) ) ;
#46206=CARTESIAN_POINT ( 'NONE',  ( -0.6430446194225712953, 0.05413385826771626580, -0.4176697321401330321 ) ) ;
#46207=CARTESIAN_POINT ( 'NONE',  ( -1.062992125984250968, -0.6692913385826771977, 8.415575281601705876E-17 ) ) ;
#46208=CARTESIAN_POINT ( 'NONE',  ( -1.358267716535432434, -0.4536011799217367080, 0.2665933059059888421 ) ) ;
#46209=LINE ( 'NONE', #7084, #45428 ) ;
#46210=CARTESIAN_POINT ( 'NONE',  ( -0.9973753280839886548, 0.1283753931104748280, 0.1820866141732283561 ) ) ;
#46212=CARTESIAN_POINT ( 'NONE',  ( 0.8070866141732288002, 0.1660481256975885056, 0.3530559997133364547 ) ) ;
#46217=CARTESIAN_POINT ( 'NONE',  ( 1.377952755905512472, -0.5511811023622047445, 6.969142054262312111E-17 ) ) ;
#46218=CARTESIAN_POINT ( 'NONE',  ( -1.154855643044618851, -0.6046776061558809534, -0.2411417322834644161 ) ) ;
#46219=CARTESIAN_POINT ( 'NONE',  ( 1.187664041994751285, -0.3162353388693409650, -0.4822834645669289433 ) ) ;
#46221=CARTESIAN_POINT ( 'NONE',  ( 1.548556430446194954, 0.1283753931104746893, -0.1820866141732285504 ) ) ;
#46222=CARTESIAN_POINT ( 'NONE',  ( 0.5314960629921267055, -0.5400638737290844871, 0.3530559997133364547 ) ) ;
#46223=CARTESIAN_POINT ( 'NONE',  ( -0.2559055118110227234, -0.5400638737290844871, 0.3530559997133364547 ) ) ;
#46226=CARTESIAN_POINT ( 'NONE',  ( 0.8136482939632553313, 0.1283753931104748280, 0.1820866141732283561 ) ) ;
#46231=CARTESIAN_POINT ( 'NONE',  ( -0.1574803149606292529, -0.1870078740157479769, 0.4822834645669291653 ) ) ;
#46232=CARTESIAN_POINT ( 'NONE',  ( 1.351706036745407458, -0.4281496062992127816, -0.4176697321401328100 ) ) ;
#46233=CARTESIAN_POINT ( 'NONE',  ( 0.2362204724409456558, -0.1870078740157479769, 0.4822834645669291653 ) ) ;
#46235=CARTESIAN_POINT ( 'NONE',  ( 1.227034120734908917, 0.2952755905511810774, -0.1292274648535930714 ) ) ;
#46236=CARTESIAN_POINT ( 'NONE',  ( -0.3805774278215216522, 0.05413385826771666132, 0.4176697321401328100 ) ) ;
#46237=CARTESIAN_POINT ( 'NONE',  ( -0.1509186351706028884, -0.05778040916215522460, 0.4822834645669289988 ) ) ;
#46238=CARTESIAN_POINT ( 'NONE',  ( -1.541994750656167090, -0.6692913385826773087, -0.1292274648535924053 ) ) ;
#46239=CARTESIAN_POINT ( 'NONE',  ( 1.338582677165355062, -0.1870078740157480879, -0.4822834645669291653 ) ) ;
#46240=CARTESIAN_POINT ( 'NONE',  ( 0.9842519685039378130, -0.6692913385826771977, 8.415575281601705876E-17 ) ) ;
#46242=CARTESIAN_POINT ( 'NONE',  ( 0.3805774278215230400, -0.3690944881889763329, 0.3153832671262228327 ) ) ;
#46246=CARTESIAN_POINT ( 'NONE',  ( -0.5774278215223089816, 0.1283753931104746893, -0.1820866141732285504 ) ) ;
#46247=CARTESIAN_POINT ( 'NONE',  ( -0.2165354330708654795, 0.1660481256975885056, 0.3530559997133364547 ) ) ;
#46248=CARTESIAN_POINT ( 'NONE',  ( 1.604771003085129433, 0.4934440724007136403, -0.1466069496707749775 ) ) ;
#46249=CARTESIAN_POINT ( 'NONE',  ( 0.3280839895013130669, 0.05413385826771666132, 0.4176697321401328100 ) ) ;
#46250=CARTESIAN_POINT ( 'NONE',  ( 0.006561679790026889343, -0.05778040916215522460, 0.4822834645669289988 ) ) ;
#46251=CARTESIAN_POINT ( 'NONE',  ( -0.7545931758530176614, -0.6692913385826773087, -0.1292274648535924053 ) ) ;
#46252=CARTESIAN_POINT ( 'NONE',  ( -1.181102362204723644, -0.1870078740157480879, -0.4822834645669291653 ) ) ;
#46254=CARTESIAN_POINT ( 'NONE',  ( 1.181102362204725198, -0.1870078740157479769, 0.3641732283464567677 ) ) ;
#46256=CARTESIAN_POINT ( 'NONE',  ( -1.586052503253847057, 1.574803149606300412, -0.1653254495020572423 ) ) ;
#46257=CARTESIAN_POINT ( 'NONE',  ( 0.9645669291338588858, 0.07958543189024085140, 0.2665933059059887866 ) ) ;
#46258=CARTESIAN_POINT ( 'NONE',  ( 0.2624671916010504757, 0.2306618581243848609, 0.2411417322834645549 ) ) ;
#46259=CARTESIAN_POINT ( 'NONE',  ( 0.6627296587926517768, -0.6692913385826773087, -0.1292274648535924053 ) ) ;
#46261=CARTESIAN_POINT ( 'NONE',  ( -1.574803149606298636, -0.1870078740157479769, 0.4822834645669291653 ) ) ;
#46264=CARTESIAN_POINT ( 'NONE',  ( -0.6299212598425188991, -0.1870078740157479769, 0.4822834645669291653 ) ) ;
#46267=CARTESIAN_POINT ( 'NONE',  ( -1.062992125984250968, -0.5511811023622047445, 6.969142054262312111E-17 ) ) ;
#46268=CARTESIAN_POINT ( 'NONE',  ( 1.489501312335958172, -0.05778040916215560624, -0.4822834645669293319 ) ) ;
#46269=CARTESIAN_POINT ( 'NONE',  ( 1.082677165354331228, 0.1660481256975883668, -0.3530559997133364547 ) ) ;
#46270=CARTESIAN_POINT ( 'NONE',  ( -0.3149606299212590610, -0.1870078740157480601, -0.3641732283464567677 ) ) ;
#46271=CARTESIAN_POINT ( 'NONE',  ( 0.4527559055118117182, -0.5400638737290844871, 0.3530559997133364547 ) ) ;
#46273=CARTESIAN_POINT ( 'NONE',  ( -0.2427821522309703550, -0.2845877964562159024, 0.3641732283464567677 ) ) ;
#46274=CARTESIAN_POINT ( 'NONE',  ( 0.06561679790026316017, 0.05413385826771626580, -0.4176697321401330321 ) ) ;
#46276=CARTESIAN_POINT ( 'NONE',  ( -1.187664041994750175, -0.05778040916215560624, -0.4822834645669293319 ) ) ;
#46277=CARTESIAN_POINT ( 'NONE',  ( 0.5314960629921264834, 0.07958543189024071263, -0.2665933059059888421 ) ) ;
#46278=CARTESIAN_POINT ( 'NONE',  ( 1.220472440944882386, -0.1870078740157480046, 1.254653134982923898E-17 ) ) ;
#46279=CARTESIAN_POINT ( 'NONE',  ( -0.5643044619422565855, 0.05413385826771626580, -0.4176697321401330321 ) ) ;
#46280=CARTESIAN_POINT ( 'NONE',  ( -0.1049868766404193215, -0.5023911411419708095, 0.1820866141732285504 ) ) ;
#46281=CARTESIAN_POINT ( 'NONE',  ( -1.614173228346457378, 0.2753471884572480932, 0.1372047244094471985 ) ) ;
#46282=CARTESIAN_POINT ( 'NONE',  ( -0.5314960629921254842, -0.5400638737290845981, -0.3530559997133363437 ) ) ;
#46283=CARTESIAN_POINT ( 'NONE',  ( -0.4658792650918627265, -0.3162353388693409650, -0.4822834645669289433 ) ) ;
#46284=CARTESIAN_POINT ( 'NONE',  ( -0.01968503937007793844, 0.1660481256975883668, -0.3530559997133364547 ) ) ;
#46286=EDGE_CURVE ( 'NONE', #38370, #82979, #73767, .T. ) ;
#46289=CARTESIAN_POINT ( 'NONE',  ( 0.7808398950131241190, -0.08942795157528024563, -0.3641732283464568787 ) ) ;
#46290=CARTESIAN_POINT ( 'NONE',  ( 1.299212598425197429, 0.2952755905511811885, 0.000000000000000000 ) ) ;
#46291=CARTESIAN_POINT ( 'NONE',  ( -0.8989501312335946848, 0.1771653543307087075, -0.09757992244046823083 ) ) ;
#46292=CARTESIAN_POINT ( 'NONE',  ( -1.089238845144356427, -0.004921259842519576551, 0.3153832671262227771 ) ) ;
#46294=CARTESIAN_POINT ( 'NONE',  ( -0.8136482939632537770, 0.2306618581243847221, -0.2411417322834647770 ) ) ;
#46295=CARTESIAN_POINT ( 'NONE',  ( 0.1049868766404206816, -0.6046776061558809534, -0.2411417322834644161 ) ) ;
#46296=CARTESIAN_POINT ( 'NONE',  ( 0.5774278215223104249, 0.1283753931104748280, 0.1820866141732283561 ) ) ;
#46298=CARTESIAN_POINT ( 'NONE',  ( 1.174540682414699111, -0.08942795157528024563, -0.3641732283464568787 ) ) ;
#46299=AXIS2_PLACEMENT_3D ( 'NONE', #24642, #62127, #55797 ) ;
#46300=CARTESIAN_POINT ( 'NONE',  ( 0.4658792650918641698, -0.05778040916215560624, -0.4822834645669293319 ) ) ;
#46302=CARTESIAN_POINT ( 'NONE',  ( -0.6955380577427815458, -0.4281496062992127816, -0.4176697321401328100 ) ) ;
#46304=CARTESIAN_POINT ( 'NONE',  ( 1.286089238845145033, 0.1283753931104748280, 0.1820866141732283561 ) ) ;
#46305=CARTESIAN_POINT ( 'NONE',  ( 0.5446194225721792126, -0.3162353388693405765, 0.4822834645669290543 ) ) ;
#46306=CARTESIAN_POINT ( 'NONE',  ( 0.2427821522309719648, -0.05778040916215522460, 0.4822834645669289988 ) ) ;
#46307=CARTESIAN_POINT ( 'NONE',  ( -0.09842519685039295696, -0.4536011799217367080, 0.2665933059059888421 ) ) ;
#46308=DIRECTION ( 'NONE',  ( -1.000000000000000000, 0.000000000000000000, 0.000000000000000000 ) ) ;
#46309=CARTESIAN_POINT ( 'NONE',  ( -0.1706036745406816491, -0.004921259842519870586, -0.3153832671262229437 ) ) ;
#46310=CARTESIAN_POINT ( 'NONE',  ( 0.8792650918635177559, 0.05413385826771666132, 0.4176697321401328100 ) ) ;
#46311=CARTESIAN_POINT ( 'NONE',  ( -0.7874015748031489847, -0.1870078740157479769, 0.3641732283464567677 ) ) ;
#46312=AXIS2_PLACEMENT_3D ( 'NONE', #3283, #41168, #41577 ) ;
#46313=CARTESIAN_POINT ( 'NONE',  ( -0.8202099737532799750, 0.2952755905511810774, -0.1292274648535930714 ) ) ;
#46316=CARTESIAN_POINT ( 'NONE',  ( -1.220472440944881054, -0.6692913385826771977, 8.415575281601705876E-17 ) ) ;
#46317=CARTESIAN_POINT ( 'NONE',  ( -0.9120734908136475250, 0.1771653543307087630, 0.09757992244046791164 ) ) ;
#46318=CARTESIAN_POINT ( 'NONE',  ( -0.1706036745406816491, -0.4281496062992124485, 0.4176697321401328655 ) ) ;
#46319=CARTESIAN_POINT ( 'NONE',  ( -1.640419947506561060, -0.4281496062992127816, -0.4176697321401328100 ) ) ;
#46320=CARTESIAN_POINT ( 'NONE',  ( -0.6430446194225712953, 0.05413385826771626580, -0.4176697321401330321 ) ) ;
#46322=CARTESIAN_POINT ( 'NONE',  ( 1.633858267716535639, -0.5400638737290844871, 0.3530559997133364547 ) ) ;
#46323=CARTESIAN_POINT ( 'NONE',  ( 1.108923884514436242, -0.05778040916215522460, 0.4822834645669289988 ) ) ;
#46324=CARTESIAN_POINT ( 'NONE',  ( 0.6955380577427828781, -0.4281496062992124485, 0.4176697321401328655 ) ) ;
#46327=CARTESIAN_POINT ( 'NONE',  ( -1.528871391076114250, 0.2952755905511810774, -0.1292274648535930714 ) ) ;
#46330=CARTESIAN_POINT ( 'NONE',  ( -0.3937007874015740483, -0.1870078740157479769, 0.3641732283464567677 ) ) ;
#46333=CARTESIAN_POINT ( 'NONE',  ( 0.1115485564304467270, -0.6692913385826773087, -0.1292274648535924053 ) ) ;
#46334=CARTESIAN_POINT ( 'NONE',  ( 0.2362204724409456558, -0.1870078740157480879, -0.4822834645669291653 ) ) ;
#46335=CARTESIAN_POINT ( 'NONE',  ( -0.7020997375328074108, -0.05778040916215522460, 0.4822834645669289988 ) ) ;
#46336=CARTESIAN_POINT ( 'NONE',  ( 1.279527559055118724, -0.5400638737290845981, -0.3530559997133363437 ) ) ;
#46337=CARTESIAN_POINT ( 'NONE',  ( -0.7086614173228339419, -0.1870078740157479769, 0.3641732283464567677 ) ) ;
#46338=CARTESIAN_POINT ( 'NONE',  ( 0.8267716535433078384, -0.6692913385826771977, 8.415575281601705876E-17 ) ) ;
#46339=CARTESIAN_POINT ( 'NONE',  ( 0.3937007874015754361, -0.1870078740157480601, -0.3641732283464567677 ) ) ;
#46340=CARTESIAN_POINT ( 'NONE',  ( -0.2559055118110227234, -0.5400638737290844871, 0.3530559997133364547 ) ) ;
#46342=CARTESIAN_POINT ( 'NONE',  ( -0.6496062992125976043, 0.1660481256975883668, -0.3530559997133364547 ) ) ;
#46343=CARTESIAN_POINT ( 'NONE',  ( 1.604771003085129433, 0.7270283685441705224, 0.1466069496707753106 ) ) ;
#46344=CARTESIAN_POINT ( 'NONE',  ( 1.423884514435696413, -0.3162353388693409650, -0.4822834645669289433 ) ) ;
#46345=CARTESIAN_POINT ( 'NONE',  ( 1.646981627296588035, -0.2845877964562159024, 0.3641732283464567677 ) ) ;
#46346=ORIENTED_EDGE ( 'NONE', *, *, #42674, .F. ) ;
#46348=CARTESIAN_POINT ( 'NONE',  ( -0.06561679790026180015, 0.05413385826771666132, 0.4176697321401328100 ) ) ;
#46350=CARTESIAN_POINT ( 'NONE',  ( -1.351706036745406347, 0.05413385826771626580, -0.4176697321401330321 ) ) ;
#46351=CARTESIAN_POINT ( 'NONE',  ( 1.607611548556431069, 0.2952755905511811885, 0.1292274648535926551 ) ) ;
#46352=CARTESIAN_POINT ( 'NONE',  ( 1.456692913385827515, 0.2952755905511811885, 0.000000000000000000 ) ) ;
#46354=CARTESIAN_POINT ( 'NONE',  ( 0.4133858267716541968, -0.5400638737290845981, -0.3530559997133363437 ) ) ;
#46356=CARTESIAN_POINT ( 'NONE',  ( -0.1640419947506553400, -0.05778040916215560624, -0.4822834645669293319 ) ) ;
#46358=CARTESIAN_POINT ( 'NONE',  ( -1.312335958005248715, -0.6046776061558809534, -0.2411417322834644161 ) ) ;
#46359=CARTESIAN_POINT ( 'NONE',  ( -0.6955380577427815458, 0.05413385826771666132, 0.4176697321401328100 ) ) ;
#46361=CARTESIAN_POINT ( 'NONE',  ( -0.1443569553805765515, -0.3690944881889765550, -0.3153832671262227771 ) ) ;
#46362=CARTESIAN_POINT ( 'NONE',  ( 1.528871391076116026, 0.2952755905511811885, 0.1292274648535926551 ) ) ;
#46363=CARTESIAN_POINT ( 'NONE',  ( -0.6102362204724400829, 0.1660481256975885056, 0.3530559997133364547 ) ) ;
#46364=CARTESIAN_POINT ( 'NONE',  ( -1.207349081364828880, 0.2306618581243847221, -0.2411417322834647770 ) ) ;
#46365=CARTESIAN_POINT ( 'NONE',  ( 0.8267716535433077274, 0.2952755905511811885, 0.000000000000000000 ) ) ;
#46366=CYLINDRICAL_SURFACE ( 'NONE', #63090, 3.543307086614173151 ) ;
#46367=CARTESIAN_POINT ( 'NONE',  ( -0.1902887139107604098, 0.2952755905511810774, -0.1292274648535930714 ) ) ;
#46368=CARTESIAN_POINT ( 'NONE',  ( -0.3674540682414692561, -0.5023911411419708095, -0.1820866141732282451 ) ) ;
#46369=CARTESIAN_POINT ( 'NONE',  ( 1.181102362204725198, -0.1870078740157479769, 0.3641732283464567677 ) ) ;
#46370=CARTESIAN_POINT ( 'NONE',  ( -0.9317585301837263412, 0.009842519685039463617, 0.3409548833797002576 ) ) ;
#46372=CARTESIAN_POINT ( 'NONE',  ( 1.686351706036745890, 0.1771653543307087630, 0.09757992244046791164 ) ) ;
#46373=CARTESIAN_POINT ( 'NONE',  ( 1.292650918635171564, 0.2952755905511811885, 0.1292274648535926551 ) ) ;
#46374=CONICAL_SURFACE ( 'NONE', #32925, 3.582677165354330562, 0.7853981633974415066 ) ;
#46376=CARTESIAN_POINT ( 'NONE',  ( -0.06561679790026180015, -0.4281496062992127816, -0.4176697321401328100 ) ) ;
#46377=CARTESIAN_POINT ( 'NONE',  ( -1.561679790026246017, -0.4281496062992127816, -0.4176697321401328100 ) ) ;
#46378=CARTESIAN_POINT ( 'NONE',  ( -1.686351706036744558, 0.2952755905511810774, -0.1292274648535930714 ) ) ;
#46379=CARTESIAN_POINT ( 'NONE',  ( -0.3083989501312330295, -0.05778040916215522460, 0.4822834645669289988 ) ) ;
#46381=CARTESIAN_POINT ( 'NONE',  ( 1.653543307086614789, -0.1870078740157479769, 0.4822834645669291653 ) ) ;
#46382=CARTESIAN_POINT ( 'NONE',  ( 0.6233595800524939223, -0.3162353388693405765, 0.4822834645669290543 ) ) ;
#46383=CARTESIAN_POINT ( 'NONE',  ( 1.128608923884515169, -0.5023911411419708095, -0.1820866141732282451 ) ) ;
#46385=CARTESIAN_POINT ( 'NONE',  ( 0.4002624671916016896, -0.08942795157527998196, 0.3641732283464567121 ) ) ;
#46386=CARTESIAN_POINT ( 'NONE',  ( -1.233595800524933894, -0.6046776061558809534, -0.2411417322834644161 ) ) ;
#46388=CARTESIAN_POINT ( 'NONE',  ( 1.240157480314961314, 0.1660481256975883668, -0.3530559997133364547 ) ) ;
#46390=CARTESIAN_POINT ( 'NONE',  ( 0.4002624671916016896, -0.05778040916215522460, 0.4822834645669289988 ) ) ;
#46392=CARTESIAN_POINT ( 'NONE',  ( 0.3025410870193226964, 2.784432375088962958E-17, -0.3464511005275205946 ) ) ;
#46393=CARTESIAN_POINT ( 'NONE',  ( 0.3608923884514443348, 0.1771653543307087075, -0.09757992244046823083 ) ) ;
#46394=CARTESIAN_POINT ( 'NONE',  ( 0.4986876640419954376, -0.6046776061558809534, -0.2411417322834644161 ) ) ;
#46395=CARTESIAN_POINT ( 'NONE',  ( -0.7080320533160967544, 1.900312960331933976, 0.5309055118110236338 ) ) ;
#46396=CARTESIAN_POINT ( 'NONE',  ( -0.9645669291338575535, -0.4536011799217367080, 0.2665933059059888421 ) ) ;
#46397=CARTESIAN_POINT ( 'NONE',  ( -0.8398950131233589023, -0.6046776061558809534, -0.2411417322834644161 ) ) ;
#46398=CARTESIAN_POINT ( 'NONE',  ( -1.673228346456691717, 0.1660481256975883668, -0.3530559997133364547 ) ) ;
#46399=CARTESIAN_POINT ( 'NONE',  ( 0.8595800524934390507, -0.3162353388693405765, 0.4822834645669290543 ) ) ;
#46400=CARTESIAN_POINT ( 'NONE',  ( 1.653543307086614789, -0.1870078740157479769, 0.4822834645669291653 ) ) ;
#46402=CARTESIAN_POINT ( 'NONE',  ( 0.4724409448818904789, -0.1870078740157479769, 0.4822834645669291653 ) ) ;
#46404=CARTESIAN_POINT ( 'NONE',  ( 1.607611548556431069, -0.6692913385826773087, -0.1292274648535924053 ) ) ;
#46405=CARTESIAN_POINT ( 'NONE',  ( 1.299212598425197429, -0.6692913385826771977, 8.415575281601705876E-17 ) ) ;
#46406=CARTESIAN_POINT ( 'NONE',  ( -1.640419947506561060, -0.3690944881889765550, -0.3153832671262227771 ) ) ;
#46407=CARTESIAN_POINT ( 'NONE',  ( 1.364829396325460076, 0.1283753931104748280, 0.1820866141732283561 ) ) ;
#46408=CARTESIAN_POINT ( 'NONE',  ( -1.187664041994749731, -0.2845877964562159024, 0.3641732283464567677 ) ) ;
#46409=CARTESIAN_POINT ( 'NONE',  ( -0.2362204724409440182, -0.1870078740157479769, 0.3641732283464567677 ) ) ;
#46411=CARTESIAN_POINT ( 'NONE',  ( 0.3346456692913390985, 0.07958543189024085140, 0.2665933059059887866 ) ) ;
#46412=CARTESIAN_POINT ( 'NONE',  ( 0.6824146981627303710, -0.6046776061558807314, 0.2411417322834647770 ) ) ;
#46413=CARTESIAN_POINT ( 'NONE',  ( 1.272965879265092637, 0.05413385826771666132, 0.4176697321401328100 ) ) ;
#46414=CARTESIAN_POINT ( 'NONE',  ( 0.1443569553805781891, 0.05413385826771626580, -0.4176697321401330321 ) ) ;
#46416=CARTESIAN_POINT ( 'NONE',  ( -0.02624671916010428221, -0.5023911411419708095, 0.1820866141732285504 ) ) ;
#46417=CARTESIAN_POINT ( 'NONE',  ( 1.043307086614173818, -0.5400638737290845981, -0.3530559997133363437 ) ) ;
#46420=CARTESIAN_POINT ( 'NONE',  ( -1.056430446194224881, 0.2952755905511810774, -0.1292274648535930714 ) ) ;
#46423=CARTESIAN_POINT ( 'NONE',  ( 0.1706036745406830368, 0.05413385826771666132, 0.4176697321401328100 ) ) ;
#46424=CARTESIAN_POINT ( 'NONE',  ( -0.7808398950131222316, -0.3162353388693409650, -0.4822834645669289433 ) ) ;
#46426=CARTESIAN_POINT ( 'NONE',  ( -0.2559055118110230564, 0.1660481256975883668, -0.3530559997133364547 ) ) ;
#46431=CARTESIAN_POINT ( 'NONE',  ( -1.128608923884513837, -0.5023911411419708095, 0.1820866141732285504 ) ) ;
#46433=CARTESIAN_POINT ( 'NONE',  ( -1.719160104986876103, 0.05413385826771666132, 0.4176697321401328100 ) ) ;
#46436=CARTESIAN_POINT ( 'NONE',  ( 0.4593175853018380828, 0.05413385826771626580, -0.4176697321401330321 ) ) ;
#46437=CARTESIAN_POINT ( 'NONE',  ( -0.4133858267716528645, 0.07958543189024071263, -0.2665933059059888421 ) ) ;
#46438=EDGE_CURVE ( 'NONE', #37352, #37974, #50612, .T. ) ;
#46439=CARTESIAN_POINT ( 'NONE',  ( 0.7677165354330716118, -0.5400638737290844871, 0.3530559997133364547 ) ) ;
#46440=CARTESIAN_POINT ( 'NONE',  ( 0.4002624671916016896, -0.3162353388693409650, -0.4822834645669289433 ) ) ;
#46444=CARTESIAN_POINT ( 'NONE',  ( 1.332020997375329197, -0.3162353388693405765, 0.4822834645669290543 ) ) ;
#46445=CARTESIAN_POINT ( 'NONE',  ( 0.5511811023622054106, -0.1870078740157480879, -0.4822834645669291653 ) ) ;
#46446=CARTESIAN_POINT ( 'NONE',  ( 0.1968503937007881344, 0.2952755905511811885, 0.000000000000000000 ) ) ;
#46447=CARTESIAN_POINT ( 'NONE',  ( 1.332020997375328974, -0.05778040916215560624, -0.4822834645669293319 ) ) ;
#46448=CARTESIAN_POINT ( 'NONE',  ( 1.082677165354331228, 0.1660481256975883668, -0.3530559997133364547 ) ) ;
#46450=CARTESIAN_POINT ( 'NONE',  ( 0.1049868766404206816, -0.6046776061558809534, -0.2411417322834644161 ) ) ;
#46451=CARTESIAN_POINT ( 'NONE',  ( 0.8595800524934390507, -0.3162353388693405765, 0.4822834645669290543 ) ) ;
#46452=CARTESIAN_POINT ( 'NONE',  ( -0.1837270341207340729, 0.2306618581243847221, -0.2411417322834647770 ) ) ;
#46453=CARTESIAN_POINT ( 'NONE',  ( 1.279527559055118724, -0.4536011799217368745, -0.2665933059059886201 ) ) ;
#46454=CARTESIAN_POINT ( 'NONE',  ( -1.482939632545930975, -0.4281496062992127816, -0.4176697321401328100 ) ) ;
#46455=CARTESIAN_POINT ( 'NONE',  ( -1.351706036745406347, 0.05413385826771626580, -0.4176697321401330321 ) ) ;
#46456=CARTESIAN_POINT ( 'NONE',  ( 0.7086614173228352742, -0.1870078740157480879, -0.4822834645669291653 ) ) ;
#46459=ORIENTED_EDGE ( 'NONE', *, *, #66425, .F. ) ;
#46462=CARTESIAN_POINT ( 'NONE',  ( 1.122047244094488860, -0.5400638737290845981, -0.3530559997133363437 ) ) ;
#46463=CARTESIAN_POINT ( 'NONE',  ( 1.030183727034121421, -0.2845877964562161244, -0.3641732283464567121 ) ) ;
#46464=CARTESIAN_POINT ( 'NONE',  ( -0.7770624478417540448, -4.378520898609941727E-15, 0.4281989832122463091 ) ) ;
#46468=CARTESIAN_POINT ( 'NONE',  ( 1.161417322834646271, 0.1660481256975883668, -0.3530559997133364547 ) ) ;
#46469=CARTESIAN_POINT ( 'NONE',  ( -1.528871391076114250, -0.6692913385826771977, 0.1292274648535927661 ) ) ;
#46470=CARTESIAN_POINT ( 'NONE',  ( -0.4527559055118102749, 0.1660481256975885056, 0.3530559997133364547 ) ) ;
#46471=CARTESIAN_POINT ( 'NONE',  ( 1.036745406824147508, -0.4281496062992127816, -0.4176697321401328100 ) ) ;
#46473=CARTESIAN_POINT ( 'NONE',  ( -1.404199475065615932, 0.05413385826771666132, 0.4176697321401328100 ) ) ;
#46476=CARTESIAN_POINT ( 'NONE',  ( -1.043307086614172041, -0.4536011799217367080, 0.2665933059059888421 ) ) ;
#46477=CARTESIAN_POINT ( 'NONE',  ( -1.397637795275589623, -0.5400638737290845981, -0.3530559997133363437 ) ) ;
#46478=CARTESIAN_POINT ( 'NONE',  ( 0.4986876640419954376, -0.6046776061558809534, -0.2411417322834644161 ) ) ;
#46479=AXIS2_PLACEMENT_3D ( 'NONE', #24524, #50190, #43867 ) ;
#46483=CARTESIAN_POINT ( 'NONE',  ( 0.9317585301837276734, 0.05413385826771626580, -0.4176697321401330321 ) ) ;
#46484=CARTESIAN_POINT ( 'NONE',  ( 1.587926509186352142, -0.004921259842519576551, 0.3153832671262227771 ) ) ;
#46486=CARTESIAN_POINT ( 'NONE',  ( -0.7874015748031489847, -0.1870078740157479769, 0.3641732283464567677 ) ) ;
#46487=CARTESIAN_POINT ( 'NONE',  ( 1.633858267716535639, -0.5400638737290844871, 0.3530559997133364547 ) ) ;
#46489=CARTESIAN_POINT ( 'NONE',  ( 0.6364829396325465405, -0.05778040916215522460, 0.4822834645669289988 ) ) ;
#46490=CARTESIAN_POINT ( 'NONE',  ( -0.8792650918635160906, -0.3690944881889763329, 0.3153832671262228327 ) ) ;
#46491=CARTESIAN_POINT ( 'NONE',  ( 0.09186351706036799403, -0.3690944881889765550, -0.3153832671262227771 ) ) ;
#46492=CARTESIAN_POINT ( 'NONE',  ( -0.4921259842519677963, -0.5400638737290844871, 0.3530559997133364547 ) ) ;
#46493=CARTESIAN_POINT ( 'NONE',  ( -1.161417322834644716, 0.07958543189024085140, 0.2665933059059887866 ) ) ;
#46495=CARTESIAN_POINT ( 'NONE',  ( 0.9186351706036751663, -0.6046776061558807314, 0.2411417322834647770 ) ) ;
#46497=CARTESIAN_POINT ( 'NONE',  ( 0.4047984445375535922, 7.699586553780600482E-16, 0.3954985857520059711 ) ) ;
#46499=CARTESIAN_POINT ( 'NONE',  ( -0.9514435695538050464, -0.3162353388693405765, 0.4822834645669290543 ) ) ;
#46500=CARTESIAN_POINT ( 'NONE',  ( -0.2427821522309703550, -0.08942795157528024563, -0.3641732283464568787 ) ) ;
#46501=CARTESIAN_POINT ( 'NONE',  ( -1.476377952755905110, 0.1660481256975885056, 0.3530559997133364547 ) ) ;
#46502=CARTESIAN_POINT ( 'NONE',  ( 1.017060367454068803, -0.2845877964562159024, 0.3641732283464567677 ) ) ;
#46503=CARTESIAN_POINT ( 'NONE',  ( -0.7020997375328076329, -0.2845877964562161244, -0.3641732283464567121 ) ) ;
#46504=CARTESIAN_POINT ( 'NONE',  ( -1.017060367454067249, -0.3162353388693409650, -0.4822834645669289433 ) ) ;
#46505=CARTESIAN_POINT ( 'NONE',  ( -1.194225721784776262, 0.05413385826771626580, -0.4176697321401330321 ) ) ;
#46506=CARTESIAN_POINT ( 'NONE',  ( -1.555118110236219930, -0.5400638737290845981, -0.3530559997133363437 ) ) ;
#46508=CARTESIAN_POINT ( 'NONE',  ( 1.076115485564305141, 0.1283753931104746893, -0.1820866141732285504 ) ) ;
#46509=CARTESIAN_POINT ( 'NONE',  ( 0.4724409448818904789, -0.1870078740157480879, -0.4822834645669291653 ) ) ;
#46510=CARTESIAN_POINT ( 'NONE',  ( -1.620734908136482577, 0.2952755905511811885, 0.1292274648535926551 ) ) ;
#46511=CARTESIAN_POINT ( 'NONE',  ( -1.601049868766403650, -0.6046776061558807314, 0.2411417322834647770 ) ) ;
#46514=CARTESIAN_POINT ( 'NONE',  ( -1.108923884514435132, -0.08942795157528024563, -0.3641732283464568787 ) ) ;
#46515=CARTESIAN_POINT ( 'NONE',  ( -0.6561679790026240244, 0.2306618581243847221, -0.2411417322834647770 ) ) ;
#46516=CARTESIAN_POINT ( 'NONE',  ( 0.7217847769028878924, -0.4281496062992127816, -0.4176697321401328100 ) ) ;
#46517=AXIS2_PLACEMENT_3D ( 'NONE', #1067, #1478, #14535 ) ;
#46518=CARTESIAN_POINT ( 'NONE',  ( -1.528871391076114250, 0.1771653543307087075, -0.09757992244046823083 ) ) ;
#46520=CARTESIAN_POINT ( 'NONE',  ( -1.266404199475064773, -0.3162353388693405765, 0.4822834645669290543 ) ) ;
#46523=CARTESIAN_POINT ( 'NONE',  ( 0.4790026246719168435, -0.3162353388693409650, -0.4822834645669289433 ) ) ;
#46524=CARTESIAN_POINT ( 'NONE',  ( 0.6364829396325465405, -0.3162353388693409650, -0.4822834645669289433 ) ) ;
#46525=CARTESIAN_POINT ( 'NONE',  ( 1.056430446194226436, -0.6692913385826773087, -0.1292274648535924053 ) ) ;
#46530=CARTESIAN_POINT ( 'NONE',  ( 0.2230971128608929543, -0.004921259842519870586, -0.3153832671262229437 ) ) ;
#46531=CARTESIAN_POINT ( 'NONE',  ( 0.08530183727034192087, -0.3162353388693409650, -0.4822834645669289433 ) ) ;
#46532=CARTESIAN_POINT ( 'NONE',  ( 1.272965879265092637, 0.05413385826771666132, 0.4176697321401328100 ) ) ;
#46534=CARTESIAN_POINT ( 'NONE',  ( 0.4527559055118117182, 0.07958543189024071263, -0.2665933059059888421 ) ) ;
#46535=CARTESIAN_POINT ( 'NONE',  ( -0.6627296587926501115, 0.2952755905511810774, -0.1292274648535930714 ) ) ;
#46536=CARTESIAN_POINT ( 'NONE',  ( 1.482939632545932307, 0.05413385826771626580, -0.4176697321401330321 ) ) ;
#46537=CARTESIAN_POINT ( 'NONE',  ( 0.3412073490813655186, -0.6046776061558809534, -0.2411417322834644161 ) ) ;
#46543=CARTESIAN_POINT ( 'NONE',  ( -1.541994750656167090, 0.2952755905511811885, 0.1292274648535926551 ) ) ;
#46545=CARTESIAN_POINT ( 'NONE',  ( -1.122047244094487306, 0.07958543189024071263, -0.2665933059059888421 ) ) ;
#46546=CARTESIAN_POINT ( 'NONE',  ( -1.312335958005248715, 0.2306618581243848609, 0.2411417322834645549 ) ) ;
#46549=CARTESIAN_POINT ( 'NONE',  ( -1.627296587926508442, 0.1283753931104748280, 0.1820866141732283561 ) ) ;
#46550=CARTESIAN_POINT ( 'NONE',  ( -1.318897637795274802, -0.5400638737290845981, -0.3530559997133363437 ) ) ;
#46551=CARTESIAN_POINT ( 'NONE',  ( -0.03280839895013062252, -0.6692913385826771977, 0.1292274648535927661 ) ) ;
#46552=CARTESIAN_POINT ( 'NONE',  ( -1.089238845144356427, -0.4281496062992127816, -0.4176697321401328100 ) ) ;
#46554=CARTESIAN_POINT ( 'NONE',  ( 0.7349081364829402885, -0.6046776061558809534, -0.2411417322834644161 ) ) ;
#46556=CARTESIAN_POINT ( 'NONE',  ( -1.410761154855641575, -0.2845877964562161244, -0.3641732283464567121 ) ) ;
#46557=ORIENTED_EDGE ( 'NONE', *, *, #21129, .F. ) ;
#46559=ORIENTED_EDGE ( 'NONE', *, *, #63918, .F. ) ;
#46560=CARTESIAN_POINT ( 'NONE',  ( -1.719160104986876103, -0.004921259842519576551, 0.3153832671262227771 ) ) ;
#46561=CARTESIAN_POINT ( 'NONE',  ( -1.332020997375327642, -0.3162353388693409650, -0.4822834645669289433 ) ) ;
#46562=CARTESIAN_POINT ( 'NONE',  ( -1.299212598425196097, 0.2952755905511811885, 0.000000000000000000 ) ) ;
#46564=CARTESIAN_POINT ( 'NONE',  ( -1.732283464566928277, -0.1870078740157479769, 0.4822834645669291653 ) ) ;
#46565=CARTESIAN_POINT ( 'NONE',  ( -1.509186351706035767, 0.05413385826771626580, -0.4176697321401330321 ) ) ;
#46566=CARTESIAN_POINT ( 'NONE',  ( -1.476377952755905110, 0.1660481256975885056, 0.3530559997133364547 ) ) ;
#46569=CARTESIAN_POINT ( 'NONE',  ( 1.604771003085129433, 1.278209470906375156, -0.1466069496707750330 ) ) ;
#46570=CARTESIAN_POINT ( 'NONE',  ( 0.1902887139107617975, -0.5511811023622048555, -0.09757992244046775898 ) ) ;
#46572=CARTESIAN_POINT ( 'NONE',  ( -0.9120734908136475250, 0.1771653543307087630, 0.09757992244046791164 ) ) ;
#46573=CARTESIAN_POINT ( 'NONE',  ( -0.8989501312335946848, -0.6692913385826771977, 0.1292274648535927661 ) ) ;
#46575=CARTESIAN_POINT ( 'NONE',  ( 0.8333333333333340365, 0.2952755905511810774, -0.1292274648535930714 ) ) ;
#46576=CARTESIAN_POINT ( 'NONE',  ( -0.9448818897637790704, -0.1870078740157480879, -0.4822834645669291653 ) ) ;
#46579=CARTESIAN_POINT ( 'NONE',  ( -0.8333333333333323711, 0.2952755905511811885, 0.1292274648535926551 ) ) ;
#46580=CARTESIAN_POINT ( 'NONE',  ( 0.6758530183727039509, 0.2952755905511810774, -0.1292274648535930714 ) ) ;
#46581=CARTESIAN_POINT ( 'NONE',  ( -1.620734908136482577, -0.5511811023622048555, -0.09757992244046775898 ) ) ;
#46582=CARTESIAN_POINT ( 'NONE',  ( -1.699475065616797398, 0.2952755905511811885, 0.1292274648535926551 ) ) ;
#46588=CARTESIAN_POINT ( 'NONE',  ( -0.3346456692913377662, 0.1660481256975883668, -0.3530559997133364547 ) ) ;
#46589=CARTESIAN_POINT ( 'NONE',  ( -1.332020997375327642, -0.08942795157527998196, 0.3641732283464567121 ) ) ;
#46593=CARTESIAN_POINT ( 'NONE',  ( -1.279527559055116948, -0.5400638737290844871, 0.3530559997133364547 ) ) ;
#46594=CARTESIAN_POINT ( 'NONE',  ( 0.06873123812453012238, 8.471767977567108961E-16, -0.4445507791589058955 ) ) ;
#46595=CARTESIAN_POINT ( 'NONE',  ( -1.607611548556429737, -0.6692913385826771977, 0.1292274648535927661 ) ) ;
#46596=CARTESIAN_POINT ( 'NONE',  ( -0.5643044619422565855, 0.05413385826771626580, -0.4176697321401330321 ) ) ;
#46598=CARTESIAN_POINT ( 'NONE',  ( 0.5249343832021003964, 0.1283753931104746893, -0.1820866141732285504 ) ) ;
#46599=CARTESIAN_POINT ( 'NONE',  ( 2.795275590551181466, 2.793565526369266916, 0.000000000000000000 ) ) ;
#46600=CARTESIAN_POINT ( 'NONE',  ( 0.4724409448818904789, -0.1870078740157480601, -0.3641732283464567677 ) ) ;
#46601=CARTESIAN_POINT ( 'NONE',  ( 1.213910761154856299, -0.5511811023622048555, -0.09757992244046775898 ) ) ;
#46602=CARTESIAN_POINT ( 'NONE',  ( 1.115485564304462551, 0.05413385826771666132, 0.4176697321401328100 ) ) ;
#46603=CARTESIAN_POINT ( 'NONE',  ( 0.1312335958005257930, 0.1283753931104746893, -0.1820866141732285504 ) ) ;
#46605=CARTESIAN_POINT ( 'NONE',  ( -1.476377952755905110, 0.1660481256975885056, 0.3530559997133364547 ) ) ;
#46606=CARTESIAN_POINT ( 'NONE',  ( -0.05905511811023545637, -0.4536011799217368745, -0.2665933059059886201 ) ) ;
#46609=CARTESIAN_POINT ( 'NONE',  ( -0.4330708661417315697, -0.5511811023622047445, 6.969142054262312111E-17 ) ) ;
#46610=DIRECTION ( 'NONE',  ( -1.000000000000000000, 0.000000000000000000, 0.000000000000000000 ) ) ;
#46611=CARTESIAN_POINT ( 'NONE',  ( 0.05249343832021075018, -0.6046776061558807314, 0.2411417322834647770 ) ) ;
#46614=CARTESIAN_POINT ( 'NONE',  ( 0.5118110236220478892, 0.1771653543307087630, 0.000000000000000000 ) ) ;
#46615=CARTESIAN_POINT ( 'NONE',  ( -0.3805774278215216522, -0.3690944881889765550, -0.3153832671262227771 ) ) ;
#46616=CARTESIAN_POINT ( 'NONE',  ( -0.3215223097112853146, -0.05778040916215560624, -0.4822834645669293319 ) ) ;
#46618=CARTESIAN_POINT ( 'NONE',  ( -1.325459317585300889, -0.004921259842519576551, 0.3153832671262227771 ) ) ;
#46620=CARTESIAN_POINT ( 'NONE',  ( 0.7283464566929143125, 0.1660481256975885056, 0.3530559997133364547 ) ) ;
#46621=CARTESIAN_POINT ( 'NONE',  ( -0.7742782152230962556, -0.4281496062992127816, -0.4176697321401328100 ) ) ;
#46624=CARTESIAN_POINT ( 'NONE',  ( -0.03280839895013062252, -0.5511811023622046335, 0.09757992244046803654 ) ) ;
#46625=CARTESIAN_POINT ( 'NONE',  ( -1.017060367454067249, -0.05778040916215522460, 0.4822834645669289988 ) ) ;
#46626=CARTESIAN_POINT ( 'NONE',  ( -1.056430446194224881, -0.5511811023622046335, 0.09757992244046803654 ) ) ;
#46627=DIRECTION ( 'NONE',  ( 0.7071067811865462405, -0.000000000000000000, 0.7071067811865486830 ) ) ;
#46628=CARTESIAN_POINT ( 'NONE',  ( -0.9645669291338575535, 0.07958543189024071263, -0.2665933059059888421 ) ) ;
#46630=CARTESIAN_POINT ( 'NONE',  ( 0.9645669291338588858, 0.1660481256975885056, 0.3530559997133364547 ) ) ;
#46634=CARTESIAN_POINT ( 'NONE',  ( 1.509186351706037543, -0.3690944881889765550, -0.3153832671262227771 ) ) ;
#46635=CARTESIAN_POINT ( 'NONE',  ( -1.358267716535432434, 0.1660481256975883668, -0.3530559997133364547 ) ) ;
#46637=CARTESIAN_POINT ( 'NONE',  ( 1.345144356955381593, -0.3162353388693409650, -0.4822834645669289433 ) ) ;
#46639=CARTESIAN_POINT ( 'NONE',  ( 1.633858267716535639, -0.4536011799217367080, 0.2665933059059888421 ) ) ;
#46640=CARTESIAN_POINT ( 'NONE',  ( 0.3346456692913393205, -0.5400638737290845981, -0.3530559997133363437 ) ) ;
#46641=CARTESIAN_POINT ( 'NONE',  ( -0.5643044619422565855, -0.4281496062992124485, 0.4176697321401328655 ) ) ;
#46643=AXIS2_PLACEMENT_3D ( 'NONE', #19028, #62407, #24919 ) ;
#46646=CARTESIAN_POINT ( 'NONE',  ( 0.7742782152230978099, -0.3690944881889763329, 0.3153832671262228327 ) ) ;
#46651=CARTESIAN_POINT ( 'NONE',  ( -0.4396325459317579898, 0.2952755905511811885, 0.1292274648535926551 ) ) ;
#46653=CARTESIAN_POINT ( 'NONE',  ( 1.430446194225722500, 0.05413385826771666132, 0.4176697321401328100 ) ) ;
#46654=CARTESIAN_POINT ( 'NONE',  ( 0.4002624671916016896, -0.05778040916215522460, 0.4822834645669289988 ) ) ;
#46655=CARTESIAN_POINT ( 'NONE',  ( -0.3149606299212590610, -0.1870078740157480601, -0.3641732283464567677 ) ) ;
#46656=CARTESIAN_POINT ( 'NONE',  ( 1.017060367454068803, -0.3162353388693405765, 0.4822834645669290543 ) ) ;
#46657=CARTESIAN_POINT ( 'NONE',  ( -0.5905511811023613777, -0.6692913385826771977, 8.415575281601705876E-17 ) ) ;
#46658=CARTESIAN_POINT ( 'NONE',  ( 0.1443569553805781891, -0.4281496062992124485, 0.4176697321401328655 ) ) ;
#46659=CARTESIAN_POINT ( 'NONE',  ( -1.522309711286088607, -0.6046776061558807314, 0.2411417322834647770 ) ) ;
#46660=CARTESIAN_POINT ( 'NONE',  ( 0.9711286089238851948, 0.2306618581243848609, 0.2411417322834645549 ) ) ;
#46661=CARTESIAN_POINT ( 'NONE',  ( 1.082677165354331228, 0.1660481256975883668, -0.3530559997133364547 ) ) ;
#46663=CARTESIAN_POINT ( 'NONE',  ( 0.006561679790026889343, -0.2845877964562161244, -0.3641732283464567121 ) ) ;
#46664=VERTEX_POINT ( 'NONE', #32859 ) ;
#46667=CARTESIAN_POINT ( 'NONE',  ( -0.4527559055118102749, 0.07958543189024085140, 0.2665933059059887866 ) ) ;
#46668=CARTESIAN_POINT ( 'NONE',  ( 0.1246719160104994284, 0.2952755905511810774, -0.1292274648535930714 ) ) ;
#46670=CARTESIAN_POINT ( 'NONE',  ( -0.3018372703412066094, 0.05413385826771666132, 0.4176697321401328100 ) ) ;
#46671=CARTESIAN_POINT ( 'NONE',  ( -0.4199475065616791736, 0.2306618581243847221, -0.2411417322834647770 ) ) ;
#46672=CARTESIAN_POINT ( 'NONE',  ( -0.9383202099737524282, -0.3162353388693409650, -0.4822834645669289433 ) ) ;
#46674=CARTESIAN_POINT ( 'NONE',  ( -1.200787401574802349, 0.1660481256975883668, -0.3530559997133364547 ) ) ;
#46675=CARTESIAN_POINT ( 'NONE',  ( 1.325459317585302665, -0.3690944881889763329, 0.3153832671262228327 ) ) ;
#46677=CARTESIAN_POINT ( 'NONE',  ( -0.1471411879992342853, -4.378520898609941727E-15, 0.4281989832122466977 ) ) ;
#46678=CARTESIAN_POINT ( 'NONE',  ( 0.7414698162729663755, -0.5511811023622048555, -0.09757992244046775898 ) ) ;
#46679=CARTESIAN_POINT ( 'NONE',  ( 0.6299212598425204535, -0.1870078740157480879, -0.4822834645669291653 ) ) ;
#46680=CARTESIAN_POINT ( 'NONE',  ( 0.2165354330708668673, -0.5400638737290844871, 0.3530559997133364547 ) ) ;
#46685=CARTESIAN_POINT ( 'NONE',  ( -0.4265091863517051496, 0.2952755905511810774, -0.1292274648535930714 ) ) ;
#46688=CARTESIAN_POINT ( 'NONE',  ( -1.043307086614172041, -0.4536011799217367080, 0.2665933059059888421 ) ) ;
#46689=CARTESIAN_POINT ( 'NONE',  ( 0.9055118110236227702, -0.6692913385826771977, 8.415575281601705876E-17 ) ) ;
#46690=CARTESIAN_POINT ( 'NONE',  ( 0.9776902887139113929, -0.6692913385826773087, -0.1292274648535924053 ) ) ;
#46691=CARTESIAN_POINT ( 'NONE',  ( -0.2099737532808391705, 0.1283753931104748280, 0.1820866141732283561 ) ) ;
#46692=CARTESIAN_POINT ( 'NONE',  ( 0.5118110236220478892, 0.2952755905511811885, 0.000000000000000000 ) ) ;
#46694=CARTESIAN_POINT ( 'NONE',  ( 0.1312335958005257930, 0.1283753931104746893, -0.1820866141732285504 ) ) ;
#46695=CARTESIAN_POINT ( 'NONE',  ( -0.2099737532808391705, -0.6046776061558809534, -0.2411417322834644161 ) ) ;
#46697=CARTESIAN_POINT ( 'NONE',  ( -1.725721784776902190, -0.05778040916215522460, 0.4822834645669289988 ) ) ;
#46698=CARTESIAN_POINT ( 'NONE',  ( 0.4593175853018379162, -0.3690944881889763329, 0.3153832671262228327 ) ) ;
#46699=CARTESIAN_POINT ( 'NONE',  ( 1.033630966599880630, -4.927456884911482678E-16, 0.4445507791589062840 ) ) ;
#46700=CARTESIAN_POINT ( 'NONE',  ( -0.7677165354330699465, 0.1660481256975885056, 0.3530559997133364547 ) ) ;
#46701=CARTESIAN_POINT ( 'NONE',  ( -0.7742782152230962556, -0.3690944881889765550, -0.3153832671262227771 ) ) ;
#46702=DIRECTION ( 'NONE',  ( -1.000000000000000000, 0.000000000000000000, 1.692413147294446216E-16 ) ) ;
#46703=CARTESIAN_POINT ( 'NONE',  ( -0.6627296587926503335, -0.6692913385826771977, 0.1292274648535927661 ) ) ;
#46704=CARTESIAN_POINT ( 'NONE',  ( -0.4790026246719152336, -0.05778040916215560624, -0.4822834645669293319 ) ) ;
#46705=CARTESIAN_POINT ( 'NONE',  ( -0.006561679790025524116, -0.05778040916215560624, -0.4822834645669293319 ) ) ;
#46707=( BOUNDED_CURVE ( )  B_SPLINE_CURVE ( 1, ( #31766, #44782 ),
 .UNSPECIFIED., .F., .F. ) 
 B_SPLINE_CURVE_WITH_KNOTS ( ( 2, 2 ),
 ( 0.000000000000000000, 0.002000000000000002644 ),
 .UNSPECIFIED. ) 
 CURVE ( )  GEOMETRIC_REPRESENTATION_ITEM ( )  RATIONAL_B_SPLINE_CURVE ( ( 0.9875488213027523443, 0.9875488213027523443 ) ) 
 REPRESENTATION_ITEM ( '' )  );
#46711=CARTESIAN_POINT ( 'NONE',  ( 0.7414698162729663755, 0.1771653543307087630, 0.09757992244046791164 ) ) ;
#46712=CARTESIAN_POINT ( 'NONE',  ( 1.397637795275591177, -0.5400638737290844871, 0.3530559997133364547 ) ) ;
#46713=CARTESIAN_POINT ( 'NONE',  ( -1.384514435695537005, 0.1771653543307087630, 0.09757992244046791164 ) ) ;
#46714=CARTESIAN_POINT ( 'NONE',  ( -1.036745406824146176, -0.004921259842519870586, -0.3153832671262229437 ) ) ;
#46715=CARTESIAN_POINT ( 'NONE',  ( -0.6955380577427815458, -0.4281496062992127816, -0.4176697321401328100 ) ) ;
#46716=CARTESIAN_POINT ( 'NONE',  ( 0.09186351706036827158, -0.004921259842519576551, 0.3153832671262227771 ) ) ;
#46718=CARTESIAN_POINT ( 'NONE',  ( 0.9514435695538062676, -0.08942795157527998196, 0.3641732283464567121 ) ) ;
#46719=CARTESIAN_POINT ( 'NONE',  ( 0.3477690288713918276, -0.6692913385826773087, -0.1292274648535924053 ) ) ;
#46721=CARTESIAN_POINT ( 'NONE',  ( -0.5774278215223089816, 0.2306618581243847221, -0.2411417322834647770 ) ) ;
#46723=CARTESIAN_POINT ( 'NONE',  ( 1.561679790026247350, -0.3690944881889763329, 0.3153832671262228327 ) ) ;
#46724=CARTESIAN_POINT ( 'NONE',  ( 0.4133858267716541968, 0.1660481256975885056, 0.3530559997133364547 ) ) ;
#46725=CARTESIAN_POINT ( 'NONE',  ( 0.07217847769028949700, -0.3162353388693405765, 0.4822834645669290543 ) ) ;
#46726=CARTESIAN_POINT ( 'NONE',  ( -0.01312335958005186876, -0.004921259842519870586, -0.3153832671262229437 ) ) ;
#46727=CARTESIAN_POINT ( 'NONE',  ( 0.5639538267004613470, 0.004960608223780119466, 0.3437734562760182411 ) ) ;
#46728=CARTESIAN_POINT ( 'NONE',  ( -0.2296587926509179312, -0.08942795157527998196, 0.3641732283464567121 ) ) ;
#46729=CARTESIAN_POINT ( 'NONE',  ( 0.8727034120734913358, -0.05778040916215522460, 0.4822834645669289988 ) ) ;
#46730=CARTESIAN_POINT ( 'NONE',  ( -0.8267716535433065062, -0.5511811023622047445, 6.969142054262312111E-17 ) ) ;
#46732=CARTESIAN_POINT ( 'NONE',  ( -1.135170603674539924, 0.2952755905511810774, -0.1292274648535930714 ) ) ;
#46733=CARTESIAN_POINT ( 'NONE',  ( 0.1902887139107617975, 0.2066929133858267931, 0.1054918080437490802 ) ) ;
#46735=CARTESIAN_POINT ( 'NONE',  ( -1.364829396325458521, -0.6046776061558807314, 0.2411417322834647770 ) ) ;
#46736=CARTESIAN_POINT ( 'NONE',  ( -1.240157480314959759, 0.07958543189024085140, 0.2665933059059887866 ) ) ;
#46737=CARTESIAN_POINT ( 'NONE',  ( 0.1115485564304467270, -0.6692913385826773087, -0.1292274648535924053 ) ) ;
#46738=CARTESIAN_POINT ( 'NONE',  ( -1.476377952755905110, -0.5400638737290845981, -0.3530559997133363437 ) ) ;
#46739=CARTESIAN_POINT ( 'NONE',  ( -0.6561679790026240244, 0.2306618581243847221, -0.2411417322834647770 ) ) ;
#46740=DIRECTION ( 'NONE',  ( -3.096699300667737957E-16, 1.000000000000000000, -0.000000000000000000 ) ) ;
#46741=CARTESIAN_POINT ( 'NONE',  ( 1.601049868766404982, -0.6046776061558809534, -0.2411417322834644161 ) ) ;
#46742=CARTESIAN_POINT ( 'NONE',  ( 1.141732283464567566, 0.2952755905511811885, 0.000000000000000000 ) ) ;
#46743=CARTESIAN_POINT ( 'NONE',  ( 0.9645669291338591078, -0.5400638737290845981, -0.3530559997133363437 ) ) ;
#46745=CARTESIAN_POINT ( 'NONE',  ( 1.587926509186352142, 0.05413385826771666132, 0.4176697321401328100 ) ) ;
#46746=CARTESIAN_POINT ( 'NONE',  ( -1.496062992125983815, -0.1870078740157480879, -0.4822834645669291653 ) ) ;
#46749=CARTESIAN_POINT ( 'NONE',  ( -0.4855643044619415427, -0.004921259842519870586, -0.3153832671262229437 ) ) ;
#46752=CARTESIAN_POINT ( 'NONE',  ( 0.2559055118110243332, -0.5400638737290845981, -0.3530559997133363437 ) ) ;
#46753=CARTESIAN_POINT ( 'NONE',  ( -0.07874015748031421014, -0.1870078740157480879, -0.4822834645669291653 ) ) ;
#46754=CARTESIAN_POINT ( 'NONE',  ( -0.8005249343832011588, 0.05413385826771626580, -0.4176697321401330321 ) ) ;
#46755=CARTESIAN_POINT ( 'NONE',  ( 1.364829396325460076, 0.2306618581243848609, 0.2411417322834645549 ) ) ;
#46756=CARTESIAN_POINT ( 'NONE',  ( -1.030183727034119867, -0.2845877964562159024, 0.3641732283464567677 ) ) ;
#46758=CARTESIAN_POINT ( 'NONE',  ( 0.8202099737532814183, -0.6692913385826773087, -0.1292274648535924053 ) ) ;
#46759=CARTESIAN_POINT ( 'NONE',  ( 0.4593175853018379162, -0.3690944881889763329, 0.3153832671262228327 ) ) ;
#46760=CARTESIAN_POINT ( 'NONE',  ( -0.4527559055118102749, -0.5400638737290845981, -0.3530559997133363437 ) ) ;
#46762=CARTESIAN_POINT ( 'NONE',  ( -1.128608923884513837, 0.2306618581243847221, -0.2411417322834647770 ) ) ;
#46763=CARTESIAN_POINT ( 'NONE',  ( -1.607611548556429737, -0.5511811023622046335, 0.09757992244046803654 ) ) ;
#46765=CARTESIAN_POINT ( 'NONE',  ( 1.430446194225722500, -0.4281496062992127816, -0.4176697321401328100 ) ) ;
#46766=CARTESIAN_POINT ( 'NONE',  ( 1.535433070866142558, 0.1771653543307087630, 0.000000000000000000 ) ) ;
#46767=VERTEX_POINT ( 'NONE', #14363 ) ;
#46769=CARTESIAN_POINT ( 'NONE',  ( 0.1574803149606306130, -0.1870078740157480879, -0.4822834645669291653 ) ) ;
#46770=ORIENTED_EDGE ( 'NONE', *, *, #67786, .F. ) ;
#46772=CARTESIAN_POINT ( 'NONE',  ( 0.8595800524934390507, -0.08942795157528024563, -0.3641732283464568787 ) ) ;
#46773=CARTESIAN_POINT ( 'NONE',  ( -1.286089238845143479, -0.6046776061558807314, 0.2411417322834647770 ) ) ;
#46774=CARTESIAN_POINT ( 'NONE',  ( 1.049868766404200127, -0.6046776061558809534, -0.2411417322834644161 ) ) ;
#46775=CARTESIAN_POINT ( 'NONE',  ( 1.227034120734908917, -0.6692913385826771977, 0.1292274648535927661 ) ) ;
#46776=CARTESIAN_POINT ( 'NONE',  ( 0.1902887139107617975, 0.2952755905511811885, 0.1292274648535926551 ) ) ;
#46777=CARTESIAN_POINT ( 'NONE',  ( -0.4133858267716528645, -0.5400638737290844871, 0.3530559997133364547 ) ) ;
#46779=CARTESIAN_POINT ( 'NONE',  ( -1.253280839895012377, -0.05778040916215522460, 0.4822834645669289988 ) ) ;
#46780=CARTESIAN_POINT ( 'NONE',  ( -0.7677165354330699465, -0.5400638737290845981, -0.3530559997133363437 ) ) ;
#46781=CARTESIAN_POINT ( 'NONE',  ( -0.4330708661417315697, -0.5511811023622047445, 6.969142054262312111E-17 ) ) ;
#46782=CARTESIAN_POINT ( 'NONE',  ( 1.640419947506562393, -0.4281496062992124485, 0.4176697321401328655 ) ) ;
#46783=CARTESIAN_POINT ( 'NONE',  ( -0.7152230971128602510, -0.05778040916215560624, -0.4822834645669293319 ) ) ;
#46785=CARTESIAN_POINT ( 'NONE',  ( 0.6496062992125991586, 0.1660481256975885056, 0.3530559997133364547 ) ) ;
#46787=CARTESIAN_POINT ( 'NONE',  ( 0.8785612751854029456, 3.421639014772782816E-16, 0.3464511005275203726 ) ) ;
#46788=CARTESIAN_POINT ( 'NONE',  ( -0.3215223097112853146, -0.05778040916215560624, -0.4822834645669293319 ) ) ;
#46789=CARTESIAN_POINT ( 'NONE',  ( 0.8333333333333340365, -0.5511811023622046335, 0.09757992244046803654 ) ) ;
#46790=CARTESIAN_POINT ( 'NONE',  ( -1.603475055217291612, 0.4410854135902512185, 0.04573490813648251746 ) ) ;
#46792=CARTESIAN_POINT ( 'NONE',  ( 1.095800524934383846, -0.08942795157528024563, -0.3641732283464568787 ) ) ;
#46793=CARTESIAN_POINT ( 'NONE',  ( 1.089238845144357537, -0.4281496062992124485, 0.4176697321401328655 ) ) ;
#46795=CARTESIAN_POINT ( 'NONE',  ( -0.5183727034120726440, -0.6692913385826773087, -0.1292274648535924053 ) ) ;
#46796=CARTESIAN_POINT ( 'NONE',  ( -1.515748031496062076, -0.5400638737290844871, 0.3530559997133364547 ) ) ;
#46797=CARTESIAN_POINT ( 'NONE',  ( -1.646981627296586703, -0.3162353388693409650, -0.4822834645669289433 ) ) ;
#46798=CARTESIAN_POINT ( 'NONE',  ( -0.05249343832020938322, -0.6046776061558809534, -0.2411417322834644161 ) ) ;
#46800=CARTESIAN_POINT ( 'NONE',  ( 1.167979002624672580, -0.4281496062992124485, 0.4176697321401328655 ) ) ;
#46801=CARTESIAN_POINT ( 'NONE',  ( 0.6430446194225728496, 0.05413385826771666132, 0.4176697321401328100 ) ) ;
#46802=CARTESIAN_POINT ( 'NONE',  ( 1.161417322834646493, -0.4536011799217367080, 0.2665933059059888421 ) ) ;
#46804=CARTESIAN_POINT ( 'NONE',  ( 0.4133858267716541968, 0.07958543189024085140, 0.2665933059059887866 ) ) ;
#46805=CARTESIAN_POINT ( 'NONE',  ( -1.076115485564303809, 0.1539470093639523085, 0.1968503937007873850 ) ) ;
#46807=CARTESIAN_POINT ( 'NONE',  ( 0.6233595800524942554, -0.05778040916215560624, -0.4822834645669293319 ) ) ;
#46809=CARTESIAN_POINT ( 'NONE',  ( 0.2690288713910767848, 0.2952755905511811885, 0.1292274648535926551 ) ) ;
#46810=CARTESIAN_POINT ( 'NONE',  ( 0.6423408027444581503, 0.000000000000000000, 0.3464511005275205946 ) ) ;
#46812=CARTESIAN_POINT ( 'NONE',  ( 0.2624671916010504757, -0.5023911411419708095, -0.1820866141732282451 ) ) ;
#46813=CARTESIAN_POINT ( 'NONE',  ( 0.3477690288713918276, -0.6692913385826773087, -0.1292274648535924053 ) ) ;
#46814=CARTESIAN_POINT ( 'NONE',  ( 0.7283464566929142014, 0.1012011053420777407, 0.2882089793578256898 ) ) ;
#46815=CARTESIAN_POINT ( 'NONE',  ( -0.7874015748031489847, -0.1870078740157479769, 0.3641732283464567677 ) ) ;
#46816=CARTESIAN_POINT ( 'NONE',  ( -1.023622047244094002, -0.1870078740157480879, -0.4822834645669291653 ) ) ;
#46817=CARTESIAN_POINT ( 'NONE',  ( -1.351706036745406347, 0.05413385826771626580, -0.4176697321401330321 ) ) ;
#46818=CARTESIAN_POINT ( 'NONE',  ( 0.4921259842519691285, -0.5400638737290845981, -0.3530559997133363437 ) ) ;
#46819=CARTESIAN_POINT ( 'NONE',  ( 1.437007874015748810, -0.5400638737290845981, -0.3530559997133363437 ) ) ;
#46821=CARTESIAN_POINT ( 'NONE',  ( 0.5511811023622054106, -0.1870078740157480879, -0.4822834645669291653 ) ) ;
#46824=CARTESIAN_POINT ( 'NONE',  ( 1.371391076115485941, 0.2952755905511811885, 0.1292274648535926551 ) ) ;
#46825=CARTESIAN_POINT ( 'NONE',  ( -1.292650918635170010, -0.5511811023622046335, 0.09757992244046803654 ) ) ;
#46826=CARTESIAN_POINT ( 'NONE',  ( 1.312335958005250269, -0.5023911411419708095, 0.1820866141732285504 ) ) ;
#46827=CARTESIAN_POINT ( 'NONE',  ( -1.496062992125983815, -0.1870078740157479769, 0.3641732283464567677 ) ) ;
#46828=CARTESIAN_POINT ( 'NONE',  ( -0.6430446194225712953, -0.004921259842519870586, -0.3153832671262229437 ) ) ;
#46830=CARTESIAN_POINT ( 'NONE',  ( 0.5839895013123367340, -0.5511811023622048555, -0.09757992244046775898 ) ) ;
#46831=CARTESIAN_POINT ( 'NONE',  ( 8.195543980992789655E-16, -0.1870078740157480879, -0.4822834645669291653 ) ) ;
#46832=CARTESIAN_POINT ( 'NONE',  ( 1.023622047244095112, -0.1870078740157480879, -0.4822834645669291653 ) ) ;
#46833=CARTESIAN_POINT ( 'NONE',  ( 0.2099737532808405305, -0.6046776061558807314, 0.2411417322834647770 ) ) ;
#46834=CARTESIAN_POINT ( 'NONE',  ( 0.01968503937007930540, 0.07958543189024085140, 0.2665933059059887866 ) ) ;
#46835=CARTESIAN_POINT ( 'NONE',  ( 1.266404199475066328, -0.05778040916215522460, 0.4822834645669289988 ) ) ;
#46836=PLANE ( 'NONE',  #3032 ) ;
#46837=CARTESIAN_POINT ( 'NONE',  ( -0.9120734908136475250, 0.2952755905511811885, 0.1292274648535926551 ) ) ;
#46840=CARTESIAN_POINT ( 'NONE',  ( -1.017060367454067249, -0.05778040916215522460, 0.4822834645669289988 ) ) ;
#46841=CARTESIAN_POINT ( 'NONE',  ( -0.01312335958005186876, -0.4281496062992124485, 0.4176697321401328655 ) ) ;
#46846=CARTESIAN_POINT ( 'NONE',  ( -1.450131233595799651, -0.5511811023622046335, 0.09757992244046803654 ) ) ;
#46848=CARTESIAN_POINT ( 'NONE',  ( -1.607611548556429737, -0.6692913385826771977, 0.1292274648535927661 ) ) ;
#46850=CARTESIAN_POINT ( 'NONE',  ( 0.4658792650918641698, -0.05778040916215560624, -0.4822834645669293319 ) ) ;
#46851=CARTESIAN_POINT ( 'NONE',  ( -0.5577427821522301654, -0.08942795157528024563, -0.3641732283464568787 ) ) ;
#46852=CARTESIAN_POINT ( 'NONE',  ( 1.036745406824147508, -0.4281496062992127816, -0.4176697321401328100 ) ) ;
#46854=CARTESIAN_POINT ( 'NONE',  ( 0.4855643044619428750, 0.05413385826771666132, 0.4176697321401328100 ) ) ;
#46858=CARTESIAN_POINT ( 'NONE',  ( 1.292650918635171564, -0.6692913385826773087, -0.1292274648535924053 ) ) ;
#46859=CARTESIAN_POINT ( 'NONE',  ( 0.1771653543307093182, 0.1660481256975885056, 0.3530559997133364547 ) ) ;
#46860=CARTESIAN_POINT ( 'NONE',  ( 1.489501312335958172, -0.05778040916215560624, -0.4822834645669293319 ) ) ;
#46861=CARTESIAN_POINT ( 'NONE',  ( 0.6955380577427828781, -0.4281496062992124485, 0.4176697321401328655 ) ) ;
#46863=CARTESIAN_POINT ( 'NONE',  ( 0.07217847769028949700, -0.05778040916215560624, -0.4822834645669293319 ) ) ;
#46864=CARTESIAN_POINT ( 'NONE',  ( 0.7086614173228353852, -0.1870078740157479769, 0.4822834645669291653 ) ) ;
#46865=CARTESIAN_POINT ( 'NONE',  ( -0.08530183727034056085, -0.3162353388693405765, 0.4822834645669290543 ) ) ;
#46866=CARTESIAN_POINT ( 'NONE',  ( 0.5643044619422579178, -0.004921259842519576551, 0.3153832671262227771 ) ) ;
#46867=CARTESIAN_POINT ( 'NONE',  ( -1.450131233595799651, -0.6692913385826771977, 0.1292274648535927661 ) ) ;
#46868=CARTESIAN_POINT ( 'NONE',  ( -1.548556430446193399, 0.2306618581243848609, 0.2411417322834645549 ) ) ;
#46869=CARTESIAN_POINT ( 'NONE',  ( 0.6233595800524939223, -0.3162353388693405765, 0.4822834645669290543 ) ) ;
#46875=CARTESIAN_POINT ( 'NONE',  ( 1.325459317585302665, -0.4281496062992124485, 0.4176697321401328655 ) ) ;
#46876=CARTESIAN_POINT ( 'NONE',  ( 1.056430446194226436, -0.5511811023622048555, -0.09757992244046775898 ) ) ;
#46878=DIRECTION ( 'NONE',  ( -3.096699300667737957E-16, 1.000000000000000000, -0.000000000000000000 ) ) ;
#46881=CARTESIAN_POINT ( 'NONE',  ( 1.246719160104987623, -0.4281496062992124485, 0.4176697321401328655 ) ) ;
#46883=CARTESIAN_POINT ( 'NONE',  ( -0.1771653543307080136, -0.5400638737290844871, 0.3530559997133364547 ) ) ;
#46884=CARTESIAN_POINT ( 'NONE',  ( 1.259842519685040019, -0.1870078740157479769, 0.4822834645669291653 ) ) ;
#46886=EDGE_CURVE ( 'NONE', #57436, #29775, #16107, .T. ) ;
#46887=CARTESIAN_POINT ( 'NONE',  ( -1.719160104986876103, 0.05413385826771666132, 0.4176697321401328100 ) ) ;
#46890=CARTESIAN_POINT ( 'NONE',  ( 1.482939632545932307, -0.3690944881889763329, 0.3153832671262228327 ) ) ;
#46892=CARTESIAN_POINT ( 'NONE',  ( -1.069553805774277722, -0.5511811023622048555, -0.09757992244046775898 ) ) ;
#46893=CARTESIAN_POINT ( 'NONE',  ( -1.450131233595799651, 0.2952755905511810774, -0.1292274648535930714 ) ) ;
#46894=CARTESIAN_POINT ( 'NONE',  ( 0.7152230971128616943, -0.05778040916215522460, 0.4822834645669289988 ) ) ;
#46895=ORIENTED_EDGE ( 'NONE', *, *, #1251, .F. ) ;
#46896=CARTESIAN_POINT ( 'NONE',  ( 1.476377952755906442, -0.5400638737290844871, 0.3530559997133364547 ) ) ;
#46897=CARTESIAN_POINT ( 'NONE',  ( 2.795275590551181466, 1.968503937007874960, 0.000000000000000000 ) ) ;
#46898=CARTESIAN_POINT ( 'NONE',  ( -0.6758530183727028406, -0.5511811023622048555, -0.09757992244046775898 ) ) ;
#46899=CARTESIAN_POINT ( 'NONE',  ( 0.8136482939632553313, -0.6046776061558809534, -0.2411417322834644161 ) ) ;
#46900=CARTESIAN_POINT ( 'NONE',  ( -1.482939632545930975, -0.4281496062992127816, -0.4176697321401328100 ) ) ;
#46902=CARTESIAN_POINT ( 'NONE',  ( -0.9317585301837263412, -0.004921259842519576551, 0.3153832671262227771 ) ) ;
#46903=CARTESIAN_POINT ( 'NONE',  ( -1.476377952755905110, 0.07958543189024085140, 0.2665933059059887866 ) ) ;
#46905=CARTESIAN_POINT ( 'NONE',  ( 0.4921259842519691285, 0.1660481256975885056, 0.3530559997133364547 ) ) ;
#46906=CARTESIAN_POINT ( 'NONE',  ( -0.9908136482939626788, 0.1771653543307087630, 0.09757992244046791164 ) ) ;
#46907=CARTESIAN_POINT ( 'NONE',  ( -0.1640419947506555343, -0.2845877964562159024, 0.3641732283464567677 ) ) ;
#46908=CARTESIAN_POINT ( 'NONE',  ( -0.1312335958005241554, 0.2306618581243848609, 0.2411417322834645549 ) ) ;
#46909=CARTESIAN_POINT ( 'NONE',  ( -1.587926509186350810, -0.004921259842519870586, -0.3153832671262229437 ) ) ;
#46911=CARTESIAN_POINT ( 'NONE',  ( 0.6036745406824153282, -0.6046776061558807314, 0.2411417322834647770 ) ) ;
#46912=EDGE_CURVE ( 'NONE', #74748, #78909, #9281, .T. ) ;
#46913=CARTESIAN_POINT ( 'NONE',  ( 0.4051969335537412009, 7.699586553780600482E-16, 0.3791483426435171555 ) ) ;
#46915=CARTESIAN_POINT ( 'NONE',  ( -0.5839895013123351797, 0.2952755905511810774, -0.1292274648535930714 ) ) ;
#46917=CARTESIAN_POINT ( 'NONE',  ( -0.04593175853018302557, -0.5511811023622048555, -0.09757992244046775898 ) ) ;
#46918=CARTESIAN_POINT ( 'NONE',  ( -1.456692913385826182, 0.2952755905511811885, 0.000000000000000000 ) ) ;
#46919=CARTESIAN_POINT ( 'NONE',  ( 0.4199475065616805614, 0.1283753931104748280, 0.1820866141732283561 ) ) ;
#46920=CARTESIAN_POINT ( 'NONE',  ( -0.5774278215223089816, 0.1283753931104746893, -0.1820866141732285504 ) ) ;
#46921=CARTESIAN_POINT ( 'NONE',  ( -1.095800524934382292, -0.05778040916215522460, 0.4822834645669289988 ) ) ;
#46922=CARTESIAN_POINT ( 'NONE',  ( -1.476377952755905110, -0.5400638737290845981, -0.3530559997133363437 ) ) ;
#46923=CARTESIAN_POINT ( 'NONE',  ( -1.463254593175852492, 0.2952755905511811885, 0.1292274648535926551 ) ) ;
#46925=CARTESIAN_POINT ( 'NONE',  ( 0.7020997375328090762, -0.2845877964562159024, 0.3641732283464567677 ) ) ;
#46926=CARTESIAN_POINT ( 'NONE',  ( 0.4199475065616805614, 0.2306618581243848609, 0.2411417322834645549 ) ) ;
#46927=CARTESIAN_POINT ( 'NONE',  ( -1.476377952755905110, 0.1660481256975885056, 0.3530559997133364547 ) ) ;
#46928=CARTESIAN_POINT ( 'NONE',  ( 1.509186351706037543, -0.3690944881889765550, -0.3153832671262227771 ) ) ;
#46932=CARTESIAN_POINT ( 'NONE',  ( -1.095800524934382292, -0.2845877964562161244, -0.3641732283464567121 ) ) ;
#46933=CARTESIAN_POINT ( 'NONE',  ( -0.4396325459317577122, -0.6692913385826773087, -0.1292274648535924053 ) ) ;
#46934=CARTESIAN_POINT ( 'NONE',  ( 0.4133858267716541968, -0.5400638737290845981, -0.3530559997133363437 ) ) ;
#46935=CARTESIAN_POINT ( 'NONE',  ( -1.371391076115484831, 0.1771653543307087075, -0.09757992244046823083 ) ) ;
#46937=CARTESIAN_POINT ( 'NONE',  ( -1.371391076115484831, 0.2952755905511810774, -0.1292274648535930714 ) ) ;
#46938=CARTESIAN_POINT ( 'NONE',  ( 0.5380577427821529035, -0.4281496062992124485, 0.4176697321401328655 ) ) ;
#46939=CARTESIAN_POINT ( 'NONE',  ( 0.1509186351706045259, -0.05778040916215560624, -0.4822834645669293319 ) ) ;
#46940=CARTESIAN_POINT ( 'NONE',  ( 1.345144356955381593, -0.3162353388693409650, -0.4822834645669289433 ) ) ;
#46941=DIRECTION ( 'NONE',  ( -0.7071067811865462405, -2.189697074797793155E-16, -0.7071067811865486830 ) ) ;
#46945=CARTESIAN_POINT ( 'NONE',  ( 5.463695987328526437E-16, -0.1870078740157479769, 0.3641732283464567677 ) ) ;
#46946=CARTESIAN_POINT ( 'NONE',  ( -0.1837270341207343505, -0.6046776061558807314, 0.2411417322834647770 ) ) ;
#46947=CARTESIAN_POINT ( 'NONE',  ( 1.391076115485564868, -0.6046776061558807314, 0.2411417322834647770 ) ) ;
#46949=CARTESIAN_POINT ( 'NONE',  ( 8.195543980992789655E-16, -0.1870078740157480601, -0.3641732283464567677 ) ) ;
#46950=CARTESIAN_POINT ( 'NONE',  ( -1.108923884514435132, -0.05778040916215560624, -0.4822834645669293319 ) ) ;
#46951=CARTESIAN_POINT ( 'NONE',  ( -1.496062992125983815, -0.1870078740157479769, 0.4822834645669291653 ) ) ;
#46955=VERTEX_POINT ( 'NONE', #41667 ) ;
#46956=CARTESIAN_POINT ( 'NONE',  ( 1.404199475065617264, -0.4281496062992124485, 0.4176697321401328655 ) ) ;
#46957=CARTESIAN_POINT ( 'NONE',  ( -1.673228346456691717, 0.1660481256975883668, -0.3530559997133364547 ) ) ;
#46958=CARTESIAN_POINT ( 'NONE',  ( -1.036745406824146176, -0.3690944881889763329, 0.3153832671262228327 ) ) ;
#46959=CARTESIAN_POINT ( 'NONE',  ( -1.358267716535432434, -0.5400638737290844871, 0.3530559997133364547 ) ) ;
#46961=CARTESIAN_POINT ( 'NONE',  ( -0.9580052493438311334, 0.009842519685039147898, -0.3409548833797004797 ) ) ;
#46962=CARTESIAN_POINT ( 'NONE',  ( 1.056430446194226658, 0.2952755905511811885, 0.1292274648535926551 ) ) ;
#46963=CARTESIAN_POINT ( 'NONE',  ( -1.633858267716534529, -0.5400638737290845981, -0.3530559997133363437 ) ) ;
#46964=CARTESIAN_POINT ( 'NONE',  ( -0.2165354330708654795, -0.5400638737290845981, -0.3530559997133363437 ) ) ;
#46965=CARTESIAN_POINT ( 'NONE',  ( -0.09186351706036689768, 0.05413385826771626580, -0.4176697321401330321 ) ) ;
#46966=CARTESIAN_POINT ( 'NONE',  ( -1.095800524934382292, -0.3162353388693409650, -0.4822834645669289433 ) ) ;
#46968=CARTESIAN_POINT ( 'NONE',  ( 0.7808398950131240079, -0.3162353388693405765, 0.4822834645669290543 ) ) ;
#46970=CARTESIAN_POINT ( 'NONE',  ( -1.279527559055116948, 0.07958543189024071263, -0.2665933059059888421 ) ) ;
#46973=ORIENTED_EDGE ( 'NONE', *, *, #78501, .F. ) ;
#46975=CARTESIAN_POINT ( 'NONE',  ( -1.108923884514435132, -0.3162353388693405765, 0.4822834645669290543 ) ) ;
#46976=CARTESIAN_POINT ( 'NONE',  ( -1.279527559055116948, 0.1660481256975883668, -0.3530559997133364547 ) ) ;
#46978=CARTESIAN_POINT ( 'NONE',  ( -1.345144356955379816, -0.05778040916215560624, -0.4822834645669293319 ) ) ;
#46980=CARTESIAN_POINT ( 'NONE',  ( -1.541994750656167090, -0.6692913385826773087, -0.1292274648535924053 ) ) ;
#46981=LINE ( 'NONE', #8287, #35104 ) ;
#46983=CARTESIAN_POINT ( 'NONE',  ( 0.02624671916010564918, -0.5023911411419708095, -0.1820866141732282451 ) ) ;
#46985=CARTESIAN_POINT ( 'NONE',  ( -0.9580052493438311334, -0.3690944881889763329, 0.3153832671262228327 ) ) ;
#46986=CARTESIAN_POINT ( 'NONE',  ( -1.233595800524933894, -0.6046776061558809534, -0.2411417322834644161 ) ) ;
#46987=CARTESIAN_POINT ( 'NONE',  ( 0.8792650918635177559, -0.4281496062992127816, -0.4176697321401328100 ) ) ;
#46988=CARTESIAN_POINT ( 'NONE',  ( -1.062992125984250968, -0.6692913385826771977, 8.415575281601705876E-17 ) ) ;
#46992=CARTESIAN_POINT ( 'NONE',  ( -1.259842519685038686, -0.1870078740157480879, -0.4822834645669291653 ) ) ;
#46993=CARTESIAN_POINT ( 'NONE',  ( 0.7808398950131240079, -0.3162353388693405765, 0.4822834645669290543 ) ) ;
#46994=CARTESIAN_POINT ( 'NONE',  ( -1.404199475065615932, -0.004921259842519576551, 0.3153832671262227771 ) ) ;
#47000=CARTESIAN_POINT ( 'NONE',  ( -0.1706036745406816491, 0.05413385826771626580, -0.4176697321401330321 ) ) ;
#47001=CARTESIAN_POINT ( 'NONE',  ( -1.620734908136482577, 0.1771653543307087630, 0.09757992244046791164 ) ) ;
#47003=CARTESIAN_POINT ( 'NONE',  ( -1.679790026246718693, 0.2306618581243847221, -0.2411417322834647770 ) ) ;
#47005=CARTESIAN_POINT ( 'NONE',  ( -1.246719160104986512, 0.05413385826771666132, 0.4176697321401328100 ) ) ;
#47006=CARTESIAN_POINT ( 'NONE',  ( -0.2493438320209966919, 0.05413385826771626580, -0.4176697321401330321 ) ) ;
#47008=CARTESIAN_POINT ( 'NONE',  ( 0.6036745406824153282, -0.5023911411419708095, 0.1820866141732285504 ) ) ;
#47010=CARTESIAN_POINT ( 'NONE',  ( 0.5052493438320218022, -0.5511811023622048555, -0.09757992244046775898 ) ) ;
#47011=CARTESIAN_POINT ( 'NONE',  ( 0.9120734908136489683, -0.5511811023622046335, 0.09757992244046803654 ) ) ;
#47012=CARTESIAN_POINT ( 'NONE',  ( 0.9908136482939640111, 0.2952755905511810774, -0.1292274648535930714 ) ) ;
#47013=CARTESIAN_POINT ( 'NONE',  ( 0.07217847769028949700, -0.2845877964562159024, 0.3641732283464567677 ) ) ;
#47015=CARTESIAN_POINT ( 'NONE',  ( -1.332020997375327642, -0.05778040916215522460, 0.4822834645669289988 ) ) ;
#47016=CARTESIAN_POINT ( 'NONE',  ( -0.2952755905511804668, 0.07958543189024085140, 0.2665933059059887866 ) ) ;
#47018=CARTESIAN_POINT ( 'NONE',  ( -1.305774278215222184, 0.1771653543307087630, 0.09757992244046791164 ) ) ;
#47020=CARTESIAN_POINT ( 'NONE',  ( -0.7808398950131222316, -0.2845877964562161244, -0.3641732283464567121 ) ) ;
#47022=FACE_OUTER_BOUND ( 'NONE', #82810, .T. ) ;
#47023=CARTESIAN_POINT ( 'NONE',  ( -0.1377952755905504645, -0.5400638737290845981, -0.3530559997133363437 ) ) ;
#47025=CARTESIAN_POINT ( 'NONE',  ( 0.6299212598425204535, -0.1870078740157479769, 0.3641732283464567677 ) ) ;
#47026=CARTESIAN_POINT ( 'NONE',  ( -0.4002624671916004129, -0.08942795157528024563, -0.3641732283464568787 ) ) ;
#47027=CARTESIAN_POINT ( 'NONE',  ( -0.4921259842519677963, 0.1660481256975883668, -0.3530559997133364547 ) ) ;
#47029=CARTESIAN_POINT ( 'NONE',  ( -1.167979002624671470, -0.004921259842519576551, 0.3153832671262227771 ) ) ;
#47031=CARTESIAN_POINT ( 'NONE',  ( 0.4396325459317593221, 0.2952755905511810774, -0.1292274648535930714 ) ) ;
#47033=CARTESIAN_POINT ( 'NONE',  ( 1.541994750656168645, -0.6692913385826771977, 0.1292274648535927661 ) ) ;
#47034=CARTESIAN_POINT ( 'NONE',  ( -0.01968503937007793844, -0.4536011799217367080, 0.2665933059059888421 ) ) ;
#47035=CARTESIAN_POINT ( 'NONE',  ( -1.528871391076114250, -0.6692913385826771977, 0.1292274648535927661 ) ) ;
#47036=CARTESIAN_POINT ( 'NONE',  ( -1.555118110236219930, -0.4536011799217368745, -0.2665933059059886201 ) ) ;
#47037=CARTESIAN_POINT ( 'NONE',  ( 1.417322834645670104, -0.1870078740157480879, -0.4822834645669291653 ) ) ;
#47039=CARTESIAN_POINT ( 'NONE',  ( -0.6430446194225716283, -0.3690944881889763329, 0.3153832671262228327 ) ) ;
#47041=CARTESIAN_POINT ( 'NONE',  ( 0.9842519685039375910, 0.2952755905511811885, 0.000000000000000000 ) ) ;
#47044=ADVANCED_FACE ( 'NONE', ( #1720 ), #62244, .F. ) ;
#47045=CARTESIAN_POINT ( 'NONE',  ( 0.7186703366786207914, -1.374501131054255944E-15, 0.4445507791589066726 ) ) ;
#47046=CARTESIAN_POINT ( 'NONE',  ( 1.515748031496063186, -0.4536011799217368745, -0.2665933059059886201 ) ) ;
#47047=CARTESIAN_POINT ( 'NONE',  ( -1.332020997375327642, -0.3162353388693409650, -0.4822834645669289433 ) ) ;
#47048=CARTESIAN_POINT ( 'NONE',  ( 1.384514435695538337, -0.6692913385826771977, 0.1292274648535927661 ) ) ;
#47050=CARTESIAN_POINT ( 'NONE',  ( 1.332020997375329197, -0.2845877964562159024, 0.3641732283464567677 ) ) ;
#47051=CARTESIAN_POINT ( 'NONE',  ( 0.02624671916010564918, -0.6046776061558809534, -0.2411417322834644161 ) ) ;
#47052=CARTESIAN_POINT ( 'NONE',  ( -0.4396325459317577122, -0.6692913385826773087, -0.1292274648535924053 ) ) ;
#47053=CARTESIAN_POINT ( 'NONE',  ( 1.679790026246720025, 0.2306618581243848609, 0.2411417322834645549 ) ) ;
#47055=CARTESIAN_POINT ( 'NONE',  ( 0.2362204724409456558, -0.1870078740157480601, -0.3641732283464567677 ) ) ;
#47058=VERTEX_POINT ( 'NONE', #72007 ) ;
#47059=CARTESIAN_POINT ( 'NONE',  ( -0.3871391076115479057, -0.3162353388693409650, -0.4822834645669289433 ) ) ;
#47060=CARTESIAN_POINT ( 'NONE',  ( 1.515748031496063186, -0.5400638737290845981, -0.3530559997133363437 ) ) ;
#47061=CARTESIAN_POINT ( 'NONE',  ( 0.3477690288713918276, -0.6692913385826773087, -0.1292274648535924053 ) ) ;
#47062=CARTESIAN_POINT ( 'NONE',  ( -0.4133858267716528645, -0.4536011799217367080, 0.2665933059059888421 ) ) ;
#47063=CARTESIAN_POINT ( 'NONE',  ( 1.036745406824147731, 0.05413385826771666132, 0.4176697321401328100 ) ) ;
#47064=CARTESIAN_POINT ( 'NONE',  ( -0.9842519685039360366, 0.2952755905511811885, 0.000000000000000000 ) ) ;
#47065=CARTESIAN_POINT ( 'NONE',  ( 0.1837270341207354329, 0.2306618581243848609, 0.2411417322834645549 ) ) ;
#47066=CARTESIAN_POINT ( 'NONE',  ( -0.9448818897637790704, -0.1870078740157479769, 0.4822834645669291653 ) ) ;
#47067=CARTESIAN_POINT ( 'NONE',  ( 1.200787401574803681, -0.5400638737290845981, -0.3530559997133363437 ) ) ;
#47068=CARTESIAN_POINT ( 'NONE',  ( 1.069553805774278610, -0.6692913385826771977, 0.1292274648535927661 ) ) ;
#47070=CARTESIAN_POINT ( 'NONE',  ( 1.154855643044620184, -0.6046776061558807314, 0.2411417322834647770 ) ) ;
#47072=CARTESIAN_POINT ( 'NONE',  ( 0.09842519685039434474, 0.07958543189024085140, 0.2665933059059887866 ) ) ;
#47076=CARTESIAN_POINT ( 'NONE',  ( -0.9711286089238838626, -0.5023911411419708095, 0.1820866141732285504 ) ) ;
#47077=CARTESIAN_POINT ( 'NONE',  ( -0.1509186351706028884, -0.3162353388693409650, -0.4822834645669289433 ) ) ;
#47079=CARTESIAN_POINT ( 'NONE',  ( -0.2034120734908131112, -0.6692913385826773087, -0.1292274648535924053 ) ) ;
#47080=CARTESIAN_POINT ( 'NONE',  ( -0.3937007874015740483, -0.1870078740157480879, -0.4822834645669291653 ) ) ;
#47081=CARTESIAN_POINT ( 'NONE',  ( -0.8727034120734901146, -0.3162353388693405765, 0.4822834645669290543 ) ) ;
#47082=CARTESIAN_POINT ( 'NONE',  ( -1.548556430446193399, 0.2306618581243848609, 0.2411417322834645549 ) ) ;
#47083=EDGE_CURVE ( 'NONE', #37352, #32456, #36679, .T. ) ;
#47084=CARTESIAN_POINT ( 'NONE',  ( 1.404199475065617708, -0.004921259842519870586, -0.3153832671262229437 ) ) ;
#47085=CARTESIAN_POINT ( 'NONE',  ( -1.502624671916009680, -0.3162353388693405765, 0.4822834645669290543 ) ) ;
#47087=CARTESIAN_POINT ( 'NONE',  ( 0.3477690288713918276, 0.1771653543307087630, 0.09757992244046791164 ) ) ;
#47088=CARTESIAN_POINT ( 'NONE',  ( 0.2427821522309719648, -0.05778040916215522460, 0.4822834645669289988 ) ) ;
#47089=CARTESIAN_POINT ( 'NONE',  ( 0.5314960629921267055, -0.5400638737290844871, 0.3530559997133364547 ) ) ;
#47092=CARTESIAN_POINT ( 'NONE',  ( -0.6171485355042630738, 0.004960608223778823628, 0.3437734562760190182 ) ) ;
#47095=CARTESIAN_POINT ( 'NONE',  ( -0.7020997375328076329, -0.3162353388693409650, -0.4822834645669289433 ) ) ;
#47099=CARTESIAN_POINT ( 'NONE',  ( -1.633858267716534529, 0.07958543189024085140, 0.2665933059059887866 ) ) ;
#47100=CARTESIAN_POINT ( 'NONE',  ( 0.8792650918635177559, -0.4281496062992127816, -0.4176697321401328100 ) ) ;
#47101=CARTESIAN_POINT ( 'NONE',  ( 0.7874015748031503170, -0.1870078740157480879, -0.4822834645669291653 ) ) ;
#47102=CARTESIAN_POINT ( 'NONE',  ( -0.3280839895013117347, -0.004921259842519870586, -0.3153832671262229437 ) ) ;
#47103=CARTESIAN_POINT ( 'NONE',  ( 0.1509186351706042484, -0.3162353388693405765, 0.4822834645669290543 ) ) ;
#47105=CARTESIAN_POINT ( 'NONE',  ( -0.1246719160104980823, -0.5511811023622048555, -0.09757992244046775898 ) ) ;
#47106=CARTESIAN_POINT ( 'NONE',  ( 0.1640419947506569498, -0.05778040916215522460, 0.4822834645669289988 ) ) ;
#47108=CARTESIAN_POINT ( 'NONE',  ( 1.568241469816273437, -0.2845877964562159024, 0.3641732283464567677 ) ) ;
#47109=CARTESIAN_POINT ( 'NONE',  ( 0.1574803149606306130, -0.1870078740157479769, 0.3641732283464567677 ) ) ;
#47110=CARTESIAN_POINT ( 'NONE',  ( 1.555118110236221041, 0.07958543189024071263, -0.2665933059059888421 ) ) ;
#47111=CARTESIAN_POINT ( 'NONE',  ( -0.6364829396325453192, -0.3162353388693405765, 0.4822834645669290543 ) ) ;
#47113=CARTESIAN_POINT ( 'NONE',  ( -0.7086614173228339419, -0.1870078740157479769, 0.3641732283464567677 ) ) ;
#47114=CARTESIAN_POINT ( 'NONE',  ( -1.033961166703848411, -1.283732188437465593E-15, -0.4281993546915532911 ) ) ;
#47115=CARTESIAN_POINT ( 'NONE',  ( -0.7480314960629914633, 0.2952755905511811885, 0.000000000000000000 ) ) ;
#47116=CARTESIAN_POINT ( 'NONE',  ( -0.6692913385826764205, 0.2952755905511811885, 0.000000000000000000 ) ) ;
#47117=CARTESIAN_POINT ( 'NONE',  ( -0.03937007874015669567, 0.2952755905511811885, 0.000000000000000000 ) ) ;
#47121=CARTESIAN_POINT ( 'NONE',  ( 0.9448818897637802916, -0.1870078740157480601, -0.3641732283464567677 ) ) ;
#47122=CARTESIAN_POINT ( 'NONE',  ( 1.423884514435696191, -0.05778040916215522460, 0.4822834645669289988 ) ) ;
#47123=CARTESIAN_POINT ( 'NONE',  ( -1.207349081364828880, 0.1283753931104746893, -0.1820866141732285504 ) ) ;
#47124=CARTESIAN_POINT ( 'NONE',  ( 0.9645669291338591078, -0.5400638737290845981, -0.3530559997133363437 ) ) ;
#47125=CARTESIAN_POINT ( 'NONE',  ( -1.167979002624671470, -0.3690944881889765550, -0.3153832671262227771 ) ) ;
#47126=CARTESIAN_POINT ( 'NONE',  ( -0.6430446194225716283, -0.4281496062992124485, 0.4176697321401328655 ) ) ;
#47127=CARTESIAN_POINT ( 'NONE',  ( 0.1771653543307093182, -0.4536011799217368745, -0.2665933059059886201 ) ) ;
#47129=CARTESIAN_POINT ( 'NONE',  ( 0.7020997375328090762, -0.08942795157528024563, -0.3641732283464568787 ) ) ;
#47130=CARTESIAN_POINT ( 'NONE',  ( 0.2165354330708668673, -0.5400638737290844871, 0.3530559997133364547 ) ) ;
#47132=CARTESIAN_POINT ( 'NONE',  ( -0.8005249343832013809, -0.4281496062992124485, 0.4176697321401328655 ) ) ;
#47134=CARTESIAN_POINT ( 'NONE',  ( 1.200787401574803681, -0.4536011799217368745, -0.2665933059059886201 ) ) ;
#47135=CARTESIAN_POINT ( 'NONE',  ( 0.4658792650918641698, -0.05778040916215560624, -0.4822834645669293319 ) ) ;
#47136=CARTESIAN_POINT ( 'NONE',  ( -0.3805774278215216522, 0.05413385826771666132, 0.4176697321401328100 ) ) ;
#47137=CARTESIAN_POINT ( 'NONE',  ( -0.3740157480314953431, 0.07958543189024085140, 0.2665933059059887866 ) ) ;
#47139=CARTESIAN_POINT ( 'NONE',  ( 0.02624671916010564918, -0.5023911411419708095, -0.1820866141732282451 ) ) ;
#47140=CARTESIAN_POINT ( 'NONE',  ( 0.5118110236220480003, -0.6692913385826771977, 8.415575281601705876E-17 ) ) ;
#47142=CARTESIAN_POINT ( 'NONE',  ( -0.8398950131233589023, -0.5023911411419708095, -0.1820866141732282451 ) ) ;
#47144=CARTESIAN_POINT ( 'NONE',  ( -1.023622047244093558, -0.1870078740157479769, 0.4822834645669291653 ) ) ;
#47145=CARTESIAN_POINT ( 'NONE',  ( 0.8561328129276796206, 8.471767977567108961E-16, -0.4445507791589058955 ) ) ;
#47146=VERTEX_POINT ( 'NONE', #9691 ) ;
#47147=CARTESIAN_POINT ( 'NONE',  ( -1.233595800524933894, 0.1283753931104748280, 0.1820866141732283561 ) ) ;
#47148=CARTESIAN_POINT ( 'NONE',  ( 0.04593175853018440641, 0.2952755905511810774, -0.1292274648535930714 ) ) ;
#47150=CARTESIAN_POINT ( 'NONE',  ( -0.6036745406824141069, -0.6046776061558809534, -0.2411417322834644161 ) ) ;
#47152=CARTESIAN_POINT ( 'NONE',  ( 0.4800390104732029095, 1.504150543744002810, -0.5309055118110237448 ) ) ;
#47153=CARTESIAN_POINT ( 'NONE',  ( 1.135170603674541256, 0.2952755905511811885, 0.1292274648535926551 ) ) ;
#47154=CARTESIAN_POINT ( 'NONE',  ( 0.7152230971128616943, -0.05778040916215522460, 0.4822834645669289988 ) ) ;
#47156=CARTESIAN_POINT ( 'NONE',  ( 1.489501312335958172, -0.05778040916215560624, -0.4822834645669293319 ) ) ;
#47157=CARTESIAN_POINT ( 'NONE',  ( -1.318897637795274802, -0.5400638737290845981, -0.3530559997133363437 ) ) ;
#47159=ORIENTED_EDGE ( 'NONE', *, *, #66845, .F. ) ;
#47160=CARTESIAN_POINT ( 'NONE',  ( -0.3346456692913377662, 0.07958543189024071263, -0.2665933059059888421 ) ) ;
#47162=ORIENTED_EDGE ( 'NONE', *, *, #45233, .T. ) ;
#47163=CARTESIAN_POINT ( 'NONE',  ( 0.8727034120734912248, -0.3162353388693409650, -0.4822834645669289433 ) ) ;
#47164=CARTESIAN_POINT ( 'NONE',  ( -0.1574803149606292529, -0.1870078740157479769, 0.4822834645669291653 ) ) ;
#47165=CARTESIAN_POINT ( 'NONE',  ( -0.8530183727034112984, 0.05413385826771666132, 0.4176697321401328100 ) ) ;
#47166=CARTESIAN_POINT ( 'NONE',  ( 1.568241469816273659, -0.05778040916215560624, -0.4822834645669293319 ) ) ;
#47167=CARTESIAN_POINT ( 'NONE',  ( -1.076115485564303809, -0.5023911411419708095, -0.1820866141732282451 ) ) ;
#47169=CARTESIAN_POINT ( 'NONE',  ( 0.2493438320209980519, 0.05413385826771666132, 0.4176697321401328100 ) ) ;
#47170=CARTESIAN_POINT ( 'NONE',  ( 0.5511811023622054106, -0.1870078740157480601, -0.3641732283464567677 ) ) ;
#47172=CARTESIAN_POINT ( 'NONE',  ( -1.003937007874014853, 0.1660481256975885056, 0.3530559997133364547 ) ) ;
#47174=CARTESIAN_POINT ( 'NONE',  ( -1.377952755905511140, -0.6692913385826771977, 8.415575281601705876E-17 ) ) ;
#47176=CARTESIAN_POINT ( 'NONE',  ( 1.220472440944882608, 0.2952755905511811885, 0.000000000000000000 ) ) ;
#47177=CARTESIAN_POINT ( 'NONE',  ( 1.259842519685040019, -0.1870078740157480601, -0.3641732283464567677 ) ) ;
#47180=CARTESIAN_POINT ( 'NONE',  ( -0.2493438320209966919, -0.4281496062992124485, 0.4176697321401328655 ) ) ;
#47182=CARTESIAN_POINT ( 'NONE',  ( 0.9186351706036751663, -0.5023911411419708095, 0.1820866141732285504 ) ) ;
#47183=CARTESIAN_POINT ( 'NONE',  ( -1.167979002624671470, -0.4281496062992127816, -0.4176697321401328100 ) ) ;
#47184=CARTESIAN_POINT ( 'NONE',  ( 0.8858267716535438430, -0.5400638737290845981, -0.3530559997133363437 ) ) ;
#47185=CARTESIAN_POINT ( 'NONE',  ( 0.7677165354330716118, -0.5400638737290844871, 0.3530559997133364547 ) ) ;
#47186=CARTESIAN_POINT ( 'NONE',  ( 0.4068241469816279987, -0.4281496062992127816, -0.4176697321401328100 ) ) ;
#47187=CARTESIAN_POINT ( 'NONE',  ( -0.5577427821522301654, -0.3162353388693405765, 0.4822834645669290543 ) ) ;
#47189=CARTESIAN_POINT ( 'NONE',  ( -1.568241469816272105, -0.05778040916215522460, 0.4822834645669289988 ) ) ;
#47190=CARTESIAN_POINT ( 'NONE',  ( -0.7808398950131222316, -0.3162353388693409650, -0.4822834645669289433 ) ) ;
#47191=CARTESIAN_POINT ( 'NONE',  ( -0.6036745406824141069, -0.5023911411419708095, -0.1820866141732282451 ) ) ;
#47194=CARTESIAN_POINT ( 'NONE',  ( 1.528871391076116026, 0.2952755905511811885, 0.1292274648535926551 ) ) ;
#47195=CARTESIAN_POINT ( 'NONE',  ( -0.5577427821522301654, -0.05778040916215560624, -0.4822834645669293319 ) ) ;
#47197=CARTESIAN_POINT ( 'NONE',  ( 0.5643044619422579178, -0.4281496062992127816, -0.4176697321401328100 ) ) ;
#47199=FACE_OUTER_BOUND ( 'NONE', #47392, .T. ) ;
#47200=( BOUNDED_SURFACE ( )  B_SPLINE_SURFACE ( 1, 2, ( 
 ( #20669, #33709, #1729, #40439, #52213, #51790, #7196, #71593, #78338, #46322, #65716, #59370, #14783, #27385, #46741, #66119, #8455, #2140, #67366, #10534, #55528, #17272, #61861, #61035, #3798, #2972, #22736, #66956, #48811, #60622, #60210, #16441, #67781, #9288, #29461, #55119, #41270, #80425, #22325, #23142, #9700, #28638, #74095, #73263, #21907, #35370, #81237, #68196, #41674, #3385, #79592, #2560, #29047, #74510, #54296, #15611, #61450, #4202, #16857, #42086, #48395, #28218, #10119, #54719, #47988, #35781, #42492, #80828, #36190, #29866, #8866, #23553, #47569, #34544, #49221, #73687, #74927, #53877, #16027, #66535, #34959, #80010, #50048, #57176, #69420, #25609, #44541, #43305, #57596, #69003, #6257, #62690, #75742, #49635, #5032, #25198, #50864, #31935, #4607, #30700, #18083, #23968, #76564, #63513, #75328, #56364, #11354, #83286, #51272, #81657, #76974, #82063, #62270, #18892, #24376, #42900, #76153, #38245, #63923, #43718, #11775, #5440, #31101, #36592, #68595, #70232, #10935, #37012, #37428, #5843, #12587, #56768, #12177, #37835, #30279, #63101, #55942, #17675, #31519, #82875, #82468, #24783, #50452, #18493, #44136, #69828, #14268, #33609, #32768, #6677, #19725, #51690, #59685, #77393, #8357, #38663, #65616, #40340, #32349, #26458, #34024, #52111, #58010, #20149, #53368, #52531, #71496, #375, #45383, #64759, #20571, #26030, #7098, #26871, #71079, #19304, #2040, #46222, #39927, #7947, #45799, #13422, #27705, #58435, #13008, #44956, #7526, #71918, #66021, #33196, #797, #59272, #58864, #70652, #64341, #39078, #1628, #65190, #27287, #52945, #77819, #13844, #39502, #78659, #1222, #20980, #78239, #46640, #72335, #14683, #79079, #34859, #55021, #79487, #36092, #16752, #40749, #54611, #23043, #28120, #35678, #3281, #80729, #68090, #35266, #60931, #41983, #28946, #21802, #79906, #48710, #9598, #22636, #73993, #29361, #47466, #42391, #10435, #61763, #9187, #66432, #80320, #60109, #61344, #4103, #74408, #29769, #73158, #2870, #22222, #28533, #15507, #41166, #21396, #47051, #54190, #2462, #72743, #53775, #48296, #15091, #3696, #8768, #34442, #66855, #60521, #47878, #16340, #67677, #73583, #10013, #15928, #41575, #67265, #49119, #5342, #56669, #55842, #18397, #76053, #30180, #69323, #11255, #12076, #81961, #49536, #63003, #62172, #10837, #56265, #70132, #57078, #30599, #75645, #68497, #74825, #17985, #37734, #75231, #4511, #50356, #50767, #63408, #31001, #37330, #17169, #11673, #24276, #36913, #49947, #5743, #43621, #82369, #24688, #81139, #76468, #36497, #23454, #44039, #62589, #18795, #42803, #4931, #69732, #44439, #81551, #31414, #82773, #25095, #38147, #12483, #23869, #63819, #17574, #6158, #43207, #55430, #68903, #77288, #14165, #39822, #78558, #76869, #19619, #6996, #12903, #65510, #52424, #38562, #45281, #273, #20884, #14584, #70548, #72235, #70976, #51173, #7842, #13321, #46535, #65081, #27183, #52847, #38974, #51587, #77714, #20044, #25508, #40237, #33509, #65920, #57909, #32663, #78134, #59171, #45696, #1118, #26769, #1529, #25928, #31833, #19201, #20467, #46120, #64242, #71392, #58756, #6577, #57494, #71815, #58330, #83185, #44850, #32248, #64657, #26348, #692, #39398, #52009, #13741, #7419, #33089, #9912, #66758, #28435, #21297, #1943, #54094, #73899, #28019, #14992, #3185, #3601, #48204, #41484, #73486, #27605, #47784, #9092, #47369, #60424, #16240, #79809, #15836, #2775, #33922, #29266, #46950, #59586, #67170, #73059, #54930, #53266, #15409, #34765, #80637, #78976, #41069, #22541, #22126, #74310, #35584, #8671, #22949, #34342, #48616, #53678, #9499, #40649, #79386, #41887, #67580, #16657, #72642, #21705, #35172, #66333, #61247, #28849, #60007, #60833, #2363, #42297, #8257, #54511, #80225, #55750, #4012, #75961, #23775, #31318, #17891, #63314, #5652, #81458, #4420, #30506, #56168, #61671, #50672, #18299, #56983, #10748, #43116, #5245, #43943, #81871, #37234, #62912, #69638, #62080, #11983, #29676, #56576, #82277, #74726, #24183, #11574, #23359, #82680, #24595, #68813, #37637, #24997, #18705, #76371, #62493, #30909, #30087, #49852, #68408 ),
 ( #67994, #10340, #17485, #17075, #36001, #49030, #75552, #55339, #50263, #81047, #42712, #49446, #36405, #75140, #43528, #69227, #11159, #36818, #4828, #38462, #70037, #39296, #58655, #57808, #31735, #44754, #76774, #1431, #19106, #33414, #63724, #7318, #65411, #57400, #51487, #59076, #77190, #83091, #45175, #78458, #77618, #13230, #25412, #70450, #6482, #45601, #51076, #32152, #51911, #12808, #44346, #27087, #71295, #64983, #32987, #70881, #64148, #52750, #175, #38048, #12391, #32567, #13643, #7749, #58229, #25828, #1022, #596, #6064, #19522, #38880, #26675, #6896, #52330, #78036, #64559, #26252, #19951, #20366, #46018, #71712, #14067, #39720, #21198, #2676, #20783, #59905, #80125, #46852, #61148, #41786, #65826, #79709, #48105, #53162, #60736, #28335, #22444, #9812, #60328, #53997, #67067, #22025, #72547, #21608, #73803, #34664, #47685, #15730, #54414, #14894, #67478, #35484, #3500, #34243, #8159, #73380, #1844, #3088, #29166, #16139, #54835, #40554, #27923, #47268, #53581, #66235, #9400, #41386, #46439, #72129, #33824, #28752, #66654, #35070, #14487, #27505, #8573, #2257, #40141, #79290, #59490, #78874, #72958, #15309, #40972, #8991, #36306, #57612, #80945, #38679, #19321, #42202, #56064, #25625, #29576, #37129, #4725, #83303, #70669, #36712, #62387, #43426, #30399, #23261, #81358, #51288, #11054, #24083, #75453, #31951, #48930, #44973, #13025, #64357, #10651, #67898, #81773, #61572, #62813, #6694, #76991, #32364, #74630, #4319, #23670, #29984, #16974, #42614, #80540, #22852, #55648, #3915, #48512, #55239, #49753, #74213, #6275, #16558, #10236, #68314, #35903, #61982, #17791, #69123, #49342, #75042, #17388, #43019, #68713, #11472, #72352, #71511, #45397, #58453, #7113, #15106, #32784, #47065, #77408, #20996, #79093, #71094, #65205, #46658, #13437, #14699, #8783, #53386, #52545, #78675, #77833, #14282, #812, #40355, #52125, #51706, #7962, #59287, #26475, #66034, #8372, #20163, #71933, #13858, #34038, #1236, #45813, #65631, #64774, #39093, #58878, #72757, #59700, #33214, #39517, #2055, #58026, #21412, #78254, #27719, #7542, #39946, #26885, #40762, #20585, #19743, #33624, #1644, #46237, #66447, #390, #27302, #52961, #26048, #74422, #60945, #28549, #41998, #41182, #73174, #35283, #49137, #36106, #9613, #54625, #47481, #28135, #80336, #16769, #54206, #66872, #29375, #29783, #42406, #67693, #16354, #53791, #74007, #3296, #73601, #28960, #68104, #22651, #10028, #48310, #60125, #55445, #15524, #2476, #35693, #15943, #81154, #79502, #41590, #61358, #23470, #21818, #67280, #48725, #3712, #17185, #61777, #34875, #74841, #60536, #42818, #79922, #55036, #9202, #22238, #10450, #4118, #68512, #2887, #47893, #80743, #23057, #34456, #31430, #17591, #24292, #62606, #57510, #76886, #49551, #51188, #81977, #30196, #18810, #49963, #83201, #44054, #6172, #31847, #75660, #30617, #56684, #82385, #4526, #19216, #44457, #25523, #36929, #69338, #57092, #70147, #24702, #63423, #5760, #12499, #4947, #38161, #55858, #82788, #25109, #43222, #50371, #37749, #75246, #44864, #76483, #50782, #18001, #81568, #11270, #68920, #10852, #56280, #36513, #23886, #63835, #62189, #43635, #11688, #37346, #63019, #5356, #31016, #76069, #69746, #18411, #12092, #13335, #32678, #71828, #25943, #58345, #78149, #287, #21310, #1955, #14178, #65525, #7856, #13755, #38988, #53280, #706, #64257, #78990, #58769, #39836, #8270, #1132, #52023, #59185, #26782, #70564, #27617, #51601, #52861, #33103, #33522, #1543, #77304, #64671, #26363, #27197, #7010, #78571, #20480, #52438, #70991, #46134, #12919, #77729, #46550, #20058, #38576, #33935, #32262, #20897, #14597, #19634, #72248, #40250, #65933, #59600, #6591, #57923, #45295, #45711, #71408, #39412, #65095, #7433, #73914, #41901, #80650, #73073, #10353, #36013, #4025, #60437, #34355, #54525, #28033, #29280, #61684, #16671, #81058, #41083, #54107, #47797, #79823, #15422, #66772, #68008, #29689, #22139, #53691, #55352, #79399, #60847, #46963, #3614, #15005, #72655, #34778, #22963, #21718, #80240, #22556, #48629, #60021, #42310, #9105, #40662, #67595, #61260 ) ),
 .UNSPECIFIED., .F., .F., .F. ) 
 B_SPLINE_SURFACE_WITH_KNOTS ( ( 2, 2 ),
 ( 3, 2, 2, 2, 2, 2, 2, 2, 2, 2, 2, 2, 2, 2, 2, 2, 2, 2, 2, 2, 2, 2, 2, 2, 2, 2, 2, 2, 2, 2, 2, 2, 2, 2, 2, 2, 2, 2, 2, 2, 2, 2, 2, 2, 2, 2, 2, 2, 2, 2, 2, 2, 2, 2, 2, 2, 2, 2, 2, 2, 2, 2, 2, 2, 2, 2, 2, 2, 2, 2, 2, 2, 2, 2, 2, 2, 2, 2, 2, 2, 2, 2, 2, 2, 2, 2, 2, 2, 2, 2, 2, 2, 2, 2, 2, 2, 2, 2, 2, 2, 2, 2, 2, 2, 2, 2, 2, 2, 2, 2, 2, 2, 2, 2, 2, 2, 2, 2, 2, 2, 2, 2, 2, 2, 2, 2, 2, 2, 2, 2, 2, 2, 2, 2, 2, 2, 2, 2, 2, 2, 2, 2, 2, 2, 2, 2, 2, 2, 2, 2, 2, 2, 2, 2, 2, 2, 2, 2, 2, 2, 2, 2, 2, 2, 2, 2, 2, 2, 2, 2, 2, 2, 2, 2, 2, 2, 2, 2, 2, 2, 2, 2, 2, 2, 2, 2, 2, 2, 2, 2, 2, 2, 2, 2, 2, 2, 2, 2, 2, 2, 2, 2, 2, 2, 2, 2, 2, 2, 2, 2, 2, 2, 2, 2, 2, 2, 2, 2, 2, 2, 2, 2, 2, 2, 2, 2, 2, 2, 2, 2, 2, 2, 2, 2, 2, 2, 2, 2, 2, 2, 2, 2, 2, 2, 2, 2, 2, 2, 2, 2, 2, 2, 2, 2, 2, 3 ),
 ( 0.000000000000000000, 1.000000000000000000 ),
 ( 0.000000000000000000, 0.003787878787878787984, 0.007575757575757575968, 0.01136363636363636395, 0.01515151515151515194, 0.01893939393939393992, 0.02272727272727272790, 0.02651515151515151589, 0.03030303030303030387, 0.03409090909090908839, 0.03787878787878787984, 0.04166666666666666435, 0.04545454545454545581, 0.04924242424242424032, 0.05303030303030303177, 0.05681818181818181629, 0.06060606060606060774, 0.06439393939393939226, 0.06818181818181817677, 0.07196969696969697516, 0.07575757575757575968, 0.07954545454545454419, 0.08333333333333332871, 0.08712121212121212710, 0.09090909090909091161, 0.09469696969696969613, 0.09848484848484848064, 0.1022727272727272790, 0.1060606060606060635, 0.1098484848484848481, 0.1136363636363636326, 0.1174242424242424310, 0.1212121212121212155, 0.1250000000000000000, 0.1287878787878787845, 0.1325757575757575690, 0.1363636363636363535, 0.1401515151515151381, 0.1439393939393939503, 0.1477272727272727348, 0.1515151515151515194, 0.1553030303030303039, 0.1590909090909090884, 0.1628787878787878729, 0.1666666666666666574, 0.1704545454545454419, 0.1742424242424242542, 0.1780303030303030387, 0.1818181818181818232, 0.1856060606060606077, 0.1893939393939393923, 0.1931818181818181768, 0.1969696969696969613, 0.2007575757575757458, 0.2045454545454545581, 0.2083333333333333426, 0.2121212121212121271, 0.2159090909090909116, 0.2196969696969696961, 0.2234848484848484806, 0.2272727272727272652, 0.2310606060606060497, 0.2348484848484848619, 0.2386363636363636465, 0.2424242424242424310, 0.2462121212121212155, 0.2500000000000000000, 0.2537878787878787845, 0.2575757575757575690, 0.2613636363636363535, 0.2651515151515151381, 0.2689393939393939226, 0.2727272727272727071, 0.2765151515151514916, 0.2803030303030302761, 0.2840909090909091161, 0.2878787878787879007, 0.2916666666666666852, 0.2954545454545454697, 0.2992424242424242542, 0.3030303030303030387, 0.3068181818181818232, 0.3106060606060606077, 0.3143939393939393923, 0.3181818181818181768, 0.3219696969696969613, 0.3257575757575757458, 0.3295454545454545303, 0.3333333333333333148, 0.3371212121212120993, 0.3409090909090908839, 0.3446969696969697239, 0.3484848484848485084, 0.3522727272727272929, 0.3560606060606060774, 0.3598484848484848619, 0.3636363636363636465, 0.3674242424242424310, 0.3712121212121212155, 0.3750000000000000000, 0.3787878787878787845, 0.3825757575757575690, 0.3863636363636363535, 0.3901515151515151381, 0.3939393939393939226, 0.3977272727272727071, 0.4015151515151514916, 0.4053030303030302761, 0.4090909090909091161, 0.4128787878787879007, 0.4166666666666666852, 0.4204545454545454697, 0.4242424242424242542, 0.4280303030303030387, 0.4318181818181818232, 0.4356060606060606077, 0.4393939393939393923, 0.4431818181818181768, 0.4469696969696969613, 0.4507575757575757458, 0.4545454545454545303, 0.4583333333333333148, 0.4621212121212120993, 0.4659090909090908839, 0.4696969696969697239, 0.4734848484848485084, 0.4772727272727272929, 0.4810606060606060774, 0.4848484848484848619, 0.4886363636363636465, 0.4924242424242424310, 0.4962121212121212155, 0.5000000000000000000, 0.5037878787878787845, 0.5075757575757575690, 0.5113636363636363535, 0.5151515151515151381, 0.5189393939393939226, 0.5227272727272727071, 0.5265151515151514916, 0.5303030303030302761, 0.5340909090909090606, 0.5378787878787878451, 0.5416666666666666297, 0.5454545454545454142, 0.5492424242424241987, 0.5530303030303029832, 0.5568181818181817677, 0.5606060606060605522, 0.5643939393939394478, 0.5681818181818182323, 0.5719696969696970168, 0.5757575757575758013, 0.5795454545454545858, 0.5833333333333333703, 0.5871212121212121549, 0.5909090909090909394, 0.5946969696969697239, 0.5984848484848485084, 0.6022727272727272929, 0.6060606060606060774, 0.6098484848484848619, 0.6136363636363636465, 0.6174242424242424310, 0.6212121212121212155, 0.6250000000000000000, 0.6287878787878787845, 0.6325757575757575690, 0.6363636363636363535, 0.6401515151515151381, 0.6439393939393939226, 0.6477272727272727071, 0.6515151515151514916, 0.6553030303030302761, 0.6590909090909090606, 0.6628787878787878451, 0.6666666666666666297, 0.6704545454545454142, 0.6742424242424241987, 0.6780303030303029832, 0.6818181818181817677, 0.6856060606060605522, 0.6893939393939394478, 0.6931818181818182323, 0.6969696969696970168, 0.7007575757575758013, 0.7045454545454545858, 0.7083333333333333703, 0.7121212121212121549, 0.7159090909090909394, 0.7196969696969697239, 0.7234848484848485084, 0.7272727272727272929, 0.7310606060606060774, 0.7348484848484848619, 0.7386363636363636465, 0.7424242424242424310, 0.7462121212121212155, 0.7500000000000000000, 0.7537878787878787845, 0.7575757575757575690, 0.7613636363636363535, 0.7651515151515151381, 0.7689393939393939226, 0.7727272727272727071, 0.7765151515151514916, 0.7803030303030302761, 0.7840909090909090606, 0.7878787878787878451, 0.7916666666666666297, 0.7954545454545454142, 0.7992424242424241987, 0.8030303030303029832, 0.8068181818181817677, 0.8106060606060605522, 0.8143939393939394478, 0.8181818181818182323, 0.8219696969696970168, 0.8257575757575758013, 0.8295454545454545858, 0.8333333333333333703, 0.8371212121212121549, 0.8409090909090909394, 0.8446969696969697239, 0.8484848484848485084, 0.8522727272727272929, 0.8560606060606060774, 0.8598484848484848619, 0.8636363636363636465, 0.8674242424242424310, 0.8712121212121212155, 0.8750000000000000000, 0.8787878787878787845, 0.8825757575757575690, 0.8863636363636363535, 0.8901515151515151381, 0.8939393939393939226, 0.8977272727272727071, 0.9015151515151514916, 0.9053030303030302761, 0.9090909090909090606, 0.9128787878787878451, 0.9166666666666666297, 0.9204545454545454142, 0.9242424242424241987, 0.9280303030303029832, 0.9318181818181817677, 0.9356060606060605522, 0.9393939393939394478, 0.9431818181818182323, 0.9469696969696970168, 0.9507575757575758013, 0.9545454545454545858, 0.9583333333333333703, 0.9621212121212121549, 0.9659090909090909394 ),
 .UNSPECIFIED. ) 
 GEOMETRIC_REPRESENTATION_ITEM ( )  RATIONAL_B_SPLINE_SURFACE ( (
 ( 1.000000000000000000, 0.9659258262890683122, 1.000000000000000000, 0.9659258262890683122, 1.000000000000000000, 0.9659258262890683122, 1.000000000000000000, 0.9659258262890683122, 1.000000000000000000, 0.9659258262890683122, 1.000000000000000000, 0.9659258262890683122, 1.000000000000000000, 0.9659258262890683122, 1.000000000000000000, 0.9659258262890683122, 1.000000000000000000, 0.9659258262890683122, 1.000000000000000000, 0.9659258262890683122, 1.000000000000000000, 0.9659258262890683122, 1.000000000000000000, 0.9659258262890683122, 1.000000000000000000, 0.9659258262890683122, 1.000000000000000000, 0.9659258262890683122, 1.000000000000000000, 0.9659258262890683122, 1.000000000000000000, 0.9659258262890683122, 1.000000000000000000, 0.9659258262890683122, 1.000000000000000000, 0.9659258262890683122, 1.000000000000000000, 0.9659258262890683122, 1.000000000000000000, 0.9659258262890683122, 1.000000000000000000, 0.9659258262890683122, 1.000000000000000000, 0.9659258262890683122, 1.000000000000000000, 0.9659258262890683122, 1.000000000000000000, 0.9659258262890683122, 1.000000000000000000, 0.9659258262890683122, 1.000000000000000000, 0.9659258262890683122, 1.000000000000000000, 0.9659258262890683122, 1.000000000000000000, 0.9659258262890683122, 1.000000000000000000, 0.9659258262890683122, 1.000000000000000000, 0.9659258262890683122, 1.000000000000000000, 0.9659258262890683122, 1.000000000000000000, 0.9659258262890683122, 1.000000000000000000, 0.9659258262890683122, 1.000000000000000000, 0.9659258262890683122, 1.000000000000000000, 0.9659258262890683122, 1.000000000000000000, 0.9659258262890683122, 1.000000000000000000, 0.9659258262890683122, 1.000000000000000000, 0.9659258262890683122, 1.000000000000000000, 0.9659258262890683122, 1.000000000000000000, 0.9659258262890683122, 1.000000000000000000, 0.9659258262890683122, 1.000000000000000000, 0.9659258262890683122, 1.000000000000000000, 0.9659258262890683122, 1.000000000000000000, 0.9659258262890683122, 1.000000000000000000, 0.9659258262890683122, 1.000000000000000000, 0.9659258262890683122, 1.000000000000000000, 0.9659258262890683122, 1.000000000000000000, 0.9659258262890683122, 1.000000000000000000, 0.9659258262890683122, 1.000000000000000000, 0.9659258262890683122, 1.000000000000000000, 0.9659258262890683122, 1.000000000000000000, 0.9659258262890683122, 1.000000000000000000, 0.9659258262890683122, 1.000000000000000000, 0.9659258262890683122, 1.000000000000000000, 0.9659258262890683122, 1.000000000000000000, 0.9659258262890683122, 1.000000000000000000, 0.9659258262890683122, 1.000000000000000000, 0.9659258262890683122, 1.000000000000000000, 0.9659258262890683122, 1.000000000000000000, 0.9659258262890683122, 1.000000000000000000, 0.9659258262890683122, 1.000000000000000000, 0.9659258262890683122, 1.000000000000000000, 0.9659258262890683122, 1.000000000000000000, 0.9659258262890683122, 1.000000000000000000, 0.9659258262890683122, 1.000000000000000000, 0.9659258262890683122, 1.000000000000000000, 0.9659258262890683122, 1.000000000000000000, 0.9659258262890683122, 1.000000000000000000, 0.9659258262890683122, 1.000000000000000000, 0.9659258262890683122, 1.000000000000000000, 0.9659258262890683122, 1.000000000000000000, 0.9659258262890683122, 1.000000000000000000, 0.9659258262890683122, 1.000000000000000000, 0.9659258262890683122, 1.000000000000000000, 0.9659258262890683122, 1.000000000000000000, 0.9659258262890683122, 1.000000000000000000, 0.9659258262890683122, 1.000000000000000000, 0.9659258262890683122, 1.000000000000000000, 0.9659258262890683122, 1.000000000000000000, 0.9659258262890683122, 1.000000000000000000, 0.9659258262890683122, 1.000000000000000000, 0.9659258262890683122, 1.000000000000000000, 0.9659258262890683122, 1.000000000000000000, 0.9659258262890683122, 1.000000000000000000, 0.9659258262890683122, 1.000000000000000000, 0.9659258262890683122, 1.000000000000000000, 0.9659258262890683122, 1.000000000000000000, 0.9659258262890683122, 1.000000000000000000, 0.9659258262890683122, 1.000000000000000000, 0.9659258262890683122, 1.000000000000000000, 0.9659258262890683122, 1.000000000000000000, 0.9659258262890683122, 1.000000000000000000, 0.9659258262890683122, 1.000000000000000000, 0.9659258262890683122, 1.000000000000000000, 0.9659258262890683122, 1.000000000000000000, 0.9659258262890683122, 1.000000000000000000, 0.9659258262890683122, 1.000000000000000000, 0.9659258262890683122, 1.000000000000000000, 0.9659258262890683122, 1.000000000000000000, 0.9659258262890683122, 1.000000000000000000, 0.9659258262890683122, 1.000000000000000000, 0.9659258262890683122, 1.000000000000000000, 0.9659258262890683122, 1.000000000000000000, 0.9659258262890683122, 1.000000000000000000, 0.9659258262890683122, 1.000000000000000000, 0.9659258262890683122, 1.000000000000000000, 0.9659258262890683122, 1.000000000000000000, 0.9659258262890683122, 1.000000000000000000, 0.9659258262890683122, 1.000000000000000000, 0.9659258262890683122, 1.000000000000000000, 0.9659258262890683122, 1.000000000000000000, 0.9659258262890683122, 1.000000000000000000, 0.9659258262890683122, 1.000000000000000000, 0.9659258262890683122, 1.000000000000000000, 0.9659258262890683122, 1.000000000000000000, 0.9659258262890683122, 1.000000000000000000, 0.9659258262890683122, 1.000000000000000000, 0.9659258262890683122, 1.000000000000000000, 0.9659258262890683122, 1.000000000000000000, 0.9659258262890683122, 1.000000000000000000, 0.9659258262890683122, 1.000000000000000000, 0.9659258262890683122, 1.000000000000000000, 0.9659258262890683122, 1.000000000000000000, 0.9659258262890683122, 1.000000000000000000, 0.9659258262890683122, 1.000000000000000000, 0.9659258262890683122, 1.000000000000000000, 0.9659258262890683122, 1.000000000000000000, 0.9659258262890683122, 1.000000000000000000, 0.9659258262890683122, 1.000000000000000000, 0.9659258262890683122, 1.000000000000000000, 0.9659258262890683122, 1.000000000000000000, 0.9659258262890683122, 1.000000000000000000, 0.9659258262890683122, 1.000000000000000000, 0.9659258262890683122, 1.000000000000000000, 0.9659258262890683122, 1.000000000000000000, 0.9659258262890683122, 1.000000000000000000, 0.9659258262890683122, 1.000000000000000000, 0.9659258262890683122, 1.000000000000000000, 0.9659258262890683122, 1.000000000000000000, 0.9659258262890683122, 1.000000000000000000, 0.9659258262890683122, 1.000000000000000000, 0.9659258262890683122, 1.000000000000000000, 0.9659258262890683122, 1.000000000000000000, 0.9659258262890683122, 1.000000000000000000, 0.9659258262890683122, 1.000000000000000000, 0.9659258262890683122, 1.000000000000000000, 0.9659258262890683122, 1.000000000000000000, 0.9659258262890683122, 1.000000000000000000, 0.9659258262890683122, 1.000000000000000000, 0.9659258262890683122, 1.000000000000000000, 0.9659258262890683122, 1.000000000000000000, 0.9659258262890683122, 1.000000000000000000, 0.9659258262890683122, 1.000000000000000000, 0.9659258262890683122, 1.000000000000000000, 0.9659258262890683122, 1.000000000000000000, 0.9659258262890683122, 1.000000000000000000, 0.9659258262890683122, 1.000000000000000000, 0.9659258262890683122, 1.000000000000000000, 0.9659258262890683122, 1.000000000000000000, 0.9659258262890683122, 1.000000000000000000, 0.9659258262890683122, 1.000000000000000000, 0.9659258262890683122, 1.000000000000000000, 0.9659258262890683122, 1.000000000000000000, 0.9659258262890683122, 1.000000000000000000, 0.9659258262890683122, 1.000000000000000000, 0.9659258262890683122, 1.000000000000000000, 0.9659258262890683122, 1.000000000000000000, 0.9659258262890683122, 1.000000000000000000, 0.9659258262890683122, 1.000000000000000000, 0.9659258262890683122, 1.000000000000000000, 0.9659258262890683122, 1.000000000000000000, 0.9659258262890683122, 1.000000000000000000, 0.9659258262890683122, 1.000000000000000000, 0.9659258262890683122, 1.000000000000000000, 0.9659258262890683122, 1.000000000000000000, 0.9659258262890683122, 1.000000000000000000, 0.9659258262890683122, 1.000000000000000000, 0.9659258262890683122, 1.000000000000000000, 0.9659258262890683122, 1.000000000000000000, 0.9659258262890683122, 1.000000000000000000, 0.9659258262890683122, 1.000000000000000000, 0.9659258262890683122, 1.000000000000000000, 0.9659258262890683122, 1.000000000000000000, 0.9659258262890683122, 1.000000000000000000, 0.9659258262890683122, 1.000000000000000000, 0.9659258262890683122, 1.000000000000000000, 0.9659258262890683122, 1.000000000000000000, 0.9659258262890683122, 1.000000000000000000, 0.9659258262890683122, 1.000000000000000000, 0.9659258262890683122, 1.000000000000000000, 0.9659258262890683122, 1.000000000000000000, 0.9659258262890683122, 1.000000000000000000, 0.9659258262890683122, 1.000000000000000000, 0.9659258262890683122, 1.000000000000000000, 0.9659258262890683122, 1.000000000000000000, 0.9659258262890683122, 1.000000000000000000, 0.9659258262890683122, 1.000000000000000000, 0.9659258262890683122, 1.000000000000000000, 0.9659258262890683122, 1.000000000000000000, 0.9659258262890683122, 1.000000000000000000, 0.9659258262890683122, 1.000000000000000000, 0.9659258262890683122, 1.000000000000000000, 0.9659258262890683122, 1.000000000000000000, 0.9659258262890683122, 1.000000000000000000, 0.9659258262890683122, 1.000000000000000000, 0.9659258262890683122, 1.000000000000000000, 0.9659258262890683122, 1.000000000000000000, 0.9659258262890683122, 1.000000000000000000, 0.9659258262890683122, 1.000000000000000000, 0.9659258262890683122, 1.000000000000000000, 0.9659258262890683122, 1.000000000000000000, 0.9659258262890683122, 1.000000000000000000, 0.9659258262890683122, 1.000000000000000000, 0.9659258262890683122, 1.000000000000000000, 0.9659258262890683122, 1.000000000000000000, 0.9659258262890683122, 1.000000000000000000, 0.9659258262890683122, 1.000000000000000000, 0.9659258262890683122, 1.000000000000000000, 0.9659258262890683122, 1.000000000000000000, 0.9659258262890683122, 1.000000000000000000, 0.9659258262890683122, 1.000000000000000000, 0.9659258262890683122, 1.000000000000000000, 0.9659258262890683122, 1.000000000000000000, 0.9659258262890683122, 1.000000000000000000, 0.9659258262890683122, 1.000000000000000000, 0.9659258262890683122, 1.000000000000000000, 0.9659258262890683122, 1.000000000000000000, 0.9659258262890683122, 1.000000000000000000, 0.9659258262890683122, 1.000000000000000000, 0.9659258262890683122, 1.000000000000000000, 0.9659258262890683122, 1.000000000000000000, 0.9659258262890683122, 1.000000000000000000, 0.9659258262890683122, 1.000000000000000000, 0.9659258262890683122, 1.000000000000000000, 0.9659258262890683122, 1.000000000000000000, 0.9659258262890683122, 1.000000000000000000, 0.9659258262890683122, 1.000000000000000000, 0.9659258262890683122, 1.000000000000000000, 0.9659258262890683122, 1.000000000000000000, 0.9659258262890683122, 1.000000000000000000, 0.9659258262890683122, 1.000000000000000000, 0.9659258262890683122, 1.000000000000000000, 0.9659258262890683122, 1.000000000000000000, 0.9659258262890683122, 1.000000000000000000, 0.9659258262890683122, 1.000000000000000000, 0.9659258262890683122, 1.000000000000000000, 0.9659258262890683122, 1.000000000000000000, 0.9659258262890683122, 1.000000000000000000, 0.9659258262890683122, 1.000000000000000000, 0.9659258262890683122, 1.000000000000000000, 0.9659258262890683122, 1.000000000000000000, 0.9659258262890683122, 1.000000000000000000, 0.9659258262890683122, 1.000000000000000000, 0.9659258262890683122, 1.000000000000000000, 0.9659258262890683122, 1.000000000000000000),
 ( 1.000000000000000000, 0.9659258262890683122, 1.000000000000000000, 0.9659258262890683122, 1.000000000000000000, 0.9659258262890683122, 1.000000000000000000, 0.9659258262890683122, 1.000000000000000000, 0.9659258262890683122, 1.000000000000000000, 0.9659258262890683122, 1.000000000000000000, 0.9659258262890683122, 1.000000000000000000, 0.9659258262890683122, 1.000000000000000000, 0.9659258262890683122, 1.000000000000000000, 0.9659258262890683122, 1.000000000000000000, 0.9659258262890683122, 1.000000000000000000, 0.9659258262890683122, 1.000000000000000000, 0.9659258262890683122, 1.000000000000000000, 0.9659258262890683122, 1.000000000000000000, 0.9659258262890683122, 1.000000000000000000, 0.9659258262890683122, 1.000000000000000000, 0.9659258262890683122, 1.000000000000000000, 0.9659258262890683122, 1.000000000000000000, 0.9659258262890683122, 1.000000000000000000, 0.9659258262890683122, 1.000000000000000000, 0.9659258262890683122, 1.000000000000000000, 0.9659258262890683122, 1.000000000000000000, 0.9659258262890683122, 1.000000000000000000, 0.9659258262890683122, 1.000000000000000000, 0.9659258262890683122, 1.000000000000000000, 0.9659258262890683122, 1.000000000000000000, 0.9659258262890683122, 1.000000000000000000, 0.9659258262890683122, 1.000000000000000000, 0.9659258262890683122, 1.000000000000000000, 0.9659258262890683122, 1.000000000000000000, 0.9659258262890683122, 1.000000000000000000, 0.9659258262890683122, 1.000000000000000000, 0.9659258262890683122, 1.000000000000000000, 0.9659258262890683122, 1.000000000000000000, 0.9659258262890683122, 1.000000000000000000, 0.9659258262890683122, 1.000000000000000000, 0.9659258262890683122, 1.000000000000000000, 0.9659258262890683122, 1.000000000000000000, 0.9659258262890683122, 1.000000000000000000, 0.9659258262890683122, 1.000000000000000000, 0.9659258262890683122, 1.000000000000000000, 0.9659258262890683122, 1.000000000000000000, 0.9659258262890683122, 1.000000000000000000, 0.9659258262890683122, 1.000000000000000000, 0.9659258262890683122, 1.000000000000000000, 0.9659258262890683122, 1.000000000000000000, 0.9659258262890683122, 1.000000000000000000, 0.9659258262890683122, 1.000000000000000000, 0.9659258262890683122, 1.000000000000000000, 0.9659258262890683122, 1.000000000000000000, 0.9659258262890683122, 1.000000000000000000, 0.9659258262890683122, 1.000000000000000000, 0.9659258262890683122, 1.000000000000000000, 0.9659258262890683122, 1.000000000000000000, 0.9659258262890683122, 1.000000000000000000, 0.9659258262890683122, 1.000000000000000000, 0.9659258262890683122, 1.000000000000000000, 0.9659258262890683122, 1.000000000000000000, 0.9659258262890683122, 1.000000000000000000, 0.9659258262890683122, 1.000000000000000000, 0.9659258262890683122, 1.000000000000000000, 0.9659258262890683122, 1.000000000000000000, 0.9659258262890683122, 1.000000000000000000, 0.9659258262890683122, 1.000000000000000000, 0.9659258262890683122, 1.000000000000000000, 0.9659258262890683122, 1.000000000000000000, 0.9659258262890683122, 1.000000000000000000, 0.9659258262890683122, 1.000000000000000000, 0.9659258262890683122, 1.000000000000000000, 0.9659258262890683122, 1.000000000000000000, 0.9659258262890683122, 1.000000000000000000, 0.9659258262890683122, 1.000000000000000000, 0.9659258262890683122, 1.000000000000000000, 0.9659258262890683122, 1.000000000000000000, 0.9659258262890683122, 1.000000000000000000, 0.9659258262890683122, 1.000000000000000000, 0.9659258262890683122, 1.000000000000000000, 0.9659258262890683122, 1.000000000000000000, 0.9659258262890683122, 1.000000000000000000, 0.9659258262890683122, 1.000000000000000000, 0.9659258262890683122, 1.000000000000000000, 0.9659258262890683122, 1.000000000000000000, 0.9659258262890683122, 1.000000000000000000, 0.9659258262890683122, 1.000000000000000000, 0.9659258262890683122, 1.000000000000000000, 0.9659258262890683122, 1.000000000000000000, 0.9659258262890683122, 1.000000000000000000, 0.9659258262890683122, 1.000000000000000000, 0.9659258262890683122, 1.000000000000000000, 0.9659258262890683122, 1.000000000000000000, 0.9659258262890683122, 1.000000000000000000, 0.9659258262890683122, 1.000000000000000000, 0.9659258262890683122, 1.000000000000000000, 0.9659258262890683122, 1.000000000000000000, 0.9659258262890683122, 1.000000000000000000, 0.9659258262890683122, 1.000000000000000000, 0.9659258262890683122, 1.000000000000000000, 0.9659258262890683122, 1.000000000000000000, 0.9659258262890683122, 1.000000000000000000, 0.9659258262890683122, 1.000000000000000000, 0.9659258262890683122, 1.000000000000000000, 0.9659258262890683122, 1.000000000000000000, 0.9659258262890683122, 1.000000000000000000, 0.9659258262890683122, 1.000000000000000000, 0.9659258262890683122, 1.000000000000000000, 0.9659258262890683122, 1.000000000000000000, 0.9659258262890683122, 1.000000000000000000, 0.9659258262890683122, 1.000000000000000000, 0.9659258262890683122, 1.000000000000000000, 0.9659258262890683122, 1.000000000000000000, 0.9659258262890683122, 1.000000000000000000, 0.9659258262890683122, 1.000000000000000000, 0.9659258262890683122, 1.000000000000000000, 0.9659258262890683122, 1.000000000000000000, 0.9659258262890683122, 1.000000000000000000, 0.9659258262890683122, 1.000000000000000000, 0.9659258262890683122, 1.000000000000000000, 0.9659258262890683122, 1.000000000000000000, 0.9659258262890683122, 1.000000000000000000, 0.9659258262890683122, 1.000000000000000000, 0.9659258262890683122, 1.000000000000000000, 0.9659258262890683122, 1.000000000000000000, 0.9659258262890683122, 1.000000000000000000, 0.9659258262890683122, 1.000000000000000000, 0.9659258262890683122, 1.000000000000000000, 0.9659258262890683122, 1.000000000000000000, 0.9659258262890683122, 1.000000000000000000, 0.9659258262890683122, 1.000000000000000000, 0.9659258262890683122, 1.000000000000000000, 0.9659258262890683122, 1.000000000000000000, 0.9659258262890683122, 1.000000000000000000, 0.9659258262890683122, 1.000000000000000000, 0.9659258262890683122, 1.000000000000000000, 0.9659258262890683122, 1.000000000000000000, 0.9659258262890683122, 1.000000000000000000, 0.9659258262890683122, 1.000000000000000000, 0.9659258262890683122, 1.000000000000000000, 0.9659258262890683122, 1.000000000000000000, 0.9659258262890683122, 1.000000000000000000, 0.9659258262890683122, 1.000000000000000000, 0.9659258262890683122, 1.000000000000000000, 0.9659258262890683122, 1.000000000000000000, 0.9659258262890683122, 1.000000000000000000, 0.9659258262890683122, 1.000000000000000000, 0.9659258262890683122, 1.000000000000000000, 0.9659258262890683122, 1.000000000000000000, 0.9659258262890683122, 1.000000000000000000, 0.9659258262890683122, 1.000000000000000000, 0.9659258262890683122, 1.000000000000000000, 0.9659258262890683122, 1.000000000000000000, 0.9659258262890683122, 1.000000000000000000, 0.9659258262890683122, 1.000000000000000000, 0.9659258262890683122, 1.000000000000000000, 0.9659258262890683122, 1.000000000000000000, 0.9659258262890683122, 1.000000000000000000, 0.9659258262890683122, 1.000000000000000000, 0.9659258262890683122, 1.000000000000000000, 0.9659258262890683122, 1.000000000000000000, 0.9659258262890683122, 1.000000000000000000, 0.9659258262890683122, 1.000000000000000000, 0.9659258262890683122, 1.000000000000000000, 0.9659258262890683122, 1.000000000000000000, 0.9659258262890683122, 1.000000000000000000, 0.9659258262890683122, 1.000000000000000000, 0.9659258262890683122, 1.000000000000000000, 0.9659258262890683122, 1.000000000000000000, 0.9659258262890683122, 1.000000000000000000, 0.9659258262890683122, 1.000000000000000000, 0.9659258262890683122, 1.000000000000000000, 0.9659258262890683122, 1.000000000000000000, 0.9659258262890683122, 1.000000000000000000, 0.9659258262890683122, 1.000000000000000000, 0.9659258262890683122, 1.000000000000000000, 0.9659258262890683122, 1.000000000000000000, 0.9659258262890683122, 1.000000000000000000, 0.9659258262890683122, 1.000000000000000000, 0.9659258262890683122, 1.000000000000000000, 0.9659258262890683122, 1.000000000000000000, 0.9659258262890683122, 1.000000000000000000, 0.9659258262890683122, 1.000000000000000000, 0.9659258262890683122, 1.000000000000000000, 0.9659258262890683122, 1.000000000000000000, 0.9659258262890683122, 1.000000000000000000, 0.9659258262890683122, 1.000000000000000000, 0.9659258262890683122, 1.000000000000000000, 0.9659258262890683122, 1.000000000000000000, 0.9659258262890683122, 1.000000000000000000, 0.9659258262890683122, 1.000000000000000000, 0.9659258262890683122, 1.000000000000000000, 0.9659258262890683122, 1.000000000000000000, 0.9659258262890683122, 1.000000000000000000, 0.9659258262890683122, 1.000000000000000000, 0.9659258262890683122, 1.000000000000000000, 0.9659258262890683122, 1.000000000000000000, 0.9659258262890683122, 1.000000000000000000, 0.9659258262890683122, 1.000000000000000000, 0.9659258262890683122, 1.000000000000000000, 0.9659258262890683122, 1.000000000000000000, 0.9659258262890683122, 1.000000000000000000, 0.9659258262890683122, 1.000000000000000000, 0.9659258262890683122, 1.000000000000000000, 0.9659258262890683122, 1.000000000000000000, 0.9659258262890683122, 1.000000000000000000, 0.9659258262890683122, 1.000000000000000000, 0.9659258262890683122, 1.000000000000000000, 0.9659258262890683122, 1.000000000000000000, 0.9659258262890683122, 1.000000000000000000, 0.9659258262890683122, 1.000000000000000000, 0.9659258262890683122, 1.000000000000000000, 0.9659258262890683122, 1.000000000000000000, 0.9659258262890683122, 1.000000000000000000, 0.9659258262890683122, 1.000000000000000000, 0.9659258262890683122, 1.000000000000000000, 0.9659258262890683122, 1.000000000000000000, 0.9659258262890683122, 1.000000000000000000, 0.9659258262890683122, 1.000000000000000000, 0.9659258262890683122, 1.000000000000000000, 0.9659258262890683122, 1.000000000000000000, 0.9659258262890683122, 1.000000000000000000, 0.9659258262890683122, 1.000000000000000000, 0.9659258262890683122, 1.000000000000000000, 0.9659258262890683122, 1.000000000000000000, 0.9659258262890683122, 1.000000000000000000, 0.9659258262890683122, 1.000000000000000000, 0.9659258262890683122, 1.000000000000000000, 0.9659258262890683122, 1.000000000000000000, 0.9659258262890683122, 1.000000000000000000, 0.9659258262890683122, 1.000000000000000000, 0.9659258262890683122, 1.000000000000000000, 0.9659258262890683122, 1.000000000000000000, 0.9659258262890683122, 1.000000000000000000, 0.9659258262890683122, 1.000000000000000000, 0.9659258262890683122, 1.000000000000000000, 0.9659258262890683122, 1.000000000000000000, 0.9659258262890683122, 1.000000000000000000, 0.9659258262890683122, 1.000000000000000000, 0.9659258262890683122, 1.000000000000000000, 0.9659258262890683122, 1.000000000000000000, 0.9659258262890683122, 1.000000000000000000, 0.9659258262890683122, 1.000000000000000000, 0.9659258262890683122, 1.000000000000000000, 0.9659258262890683122, 1.000000000000000000, 0.9659258262890683122, 1.000000000000000000, 0.9659258262890683122, 1.000000000000000000, 0.9659258262890683122, 1.000000000000000000, 0.9659258262890683122, 1.000000000000000000, 0.9659258262890683122, 1.000000000000000000, 0.9659258262890683122, 1.000000000000000000, 0.9659258262890683122, 1.000000000000000000, 0.9659258262890683122, 1.000000000000000000, 0.9659258262890683122, 1.000000000000000000, 0.9659258262890683122, 1.000000000000000000, 0.9659258262890683122, 1.000000000000000000, 0.9659258262890683122, 1.000000000000000000, 0.9659258262890683122, 1.000000000000000000) ) ) 
 REPRESENTATION_ITEM ( '' )  SURFACE ( )  );
#47201=CARTESIAN_POINT ( 'NONE',  ( -0.2230971128608915943, 0.05413385826771666132, 0.4176697321401328100 ) ) ;
#47202=CARTESIAN_POINT ( 'NONE',  ( 1.194225721784777594, -0.004921259842519576551, 0.3153832671262227771 ) ) ;
#47203=CARTESIAN_POINT ( 'NONE',  ( 0.4849061582275022153, 1.967896864084103914, -0.4921425059946357705 ) ) ;
#47205=CARTESIAN_POINT ( 'NONE',  ( 1.003937007874016407, -0.4536011799217367080, 0.2665933059059888421 ) ) ;
#47206=CARTESIAN_POINT ( 'NONE',  ( 1.246719160104987623, -0.4281496062992124485, 0.4176697321401328655 ) ) ;
#47208=CARTESIAN_POINT ( 'NONE',  ( -0.3149606299212590610, -0.1870078740157479769, 0.4822834645669291653 ) ) ;
#47209=CARTESIAN_POINT ( 'NONE',  ( -1.594488188976377119, 0.1660481256975883668, -0.3530559997133364547 ) ) ;
#47210=CARTESIAN_POINT ( 'NONE',  ( 1.364829396325459854, -0.5023911411419708095, -0.1820866141732282451 ) ) ;
#47211=CARTESIAN_POINT ( 'NONE',  ( 0.01312335958005323398, 0.05413385826771666132, 0.4176697321401328100 ) ) ;
#47213=CARTESIAN_POINT ( 'NONE',  ( 1.233595800524935227, 0.2306618581243847221, -0.2411417322834647770 ) ) ;
#47214=CARTESIAN_POINT ( 'NONE',  ( 0.3871391076115492380, -0.05778040916215560624, -0.4822834645669293319 ) ) ;
#47215=CARTESIAN_POINT ( 'NONE',  ( 0.4986876640419954376, -0.5023911411419708095, -0.1820866141732282451 ) ) ;
#47217=CARTESIAN_POINT ( 'NONE',  ( 0.3149606299212606708, -0.1870078740157480601, -0.3641732283464567677 ) ) ;
#47218=CARTESIAN_POINT ( 'NONE',  ( -1.036041590146031366, -2.613618158232546091E-15, -0.3464511005275220379 ) ) ;
#47219=B_SPLINE_CURVE_WITH_KNOTS ( 'NONE', 3,
 ( #59761, #53445, #60185, #66509, #10091, #29436, #2537, #67342, #41245, #9675 ),
 .UNSPECIFIED., .F., .F.,
 ( 4, 2, 2, 2, 4 ),
 ( 0.000000000000000000, 0.2500000000000000000, 0.3750000000000000000, 0.5000000000000000000, 1.000000000000000000 ),
 .UNSPECIFIED. ) ;
#47221=CARTESIAN_POINT ( 'NONE',  ( 0.6299212598425204535, -0.1870078740157480879, -0.4822834645669291653 ) ) ;
#47223=DIRECTION ( 'NONE',  ( -3.096699300667737957E-16, 1.000000000000000000, -0.000000000000000000 ) ) ;
#47225=CARTESIAN_POINT ( 'NONE',  ( 0.03280839895013198948, 0.1771653543307087630, 0.09757992244046791164 ) ) ;
#47226=CARTESIAN_POINT ( 'NONE',  ( -0.07217847769028787330, -0.05778040916215522460, 0.4822834645669289988 ) ) ;
#47227=CARTESIAN_POINT ( 'NONE',  ( 1.509186351706037543, -0.004921259842519576551, 0.3153832671262227771 ) ) ;
#47228=CARTESIAN_POINT ( 'NONE',  ( -1.384514435695537005, 0.1771653543307087630, 0.09757992244046791164 ) ) ;
#47229=CARTESIAN_POINT ( 'NONE',  ( -1.030183727034119867, -0.05778040916215560624, -0.4822834645669293319 ) ) ;
#47231=CARTESIAN_POINT ( 'NONE',  ( 0.5511811023622055217, -0.1870078740157479769, 0.4822834645669291653 ) ) ;
#47232=CARTESIAN_POINT ( 'NONE',  ( 1.391076115485564868, 0.2306618581243847221, -0.2411417322834647770 ) ) ;
#47234=CARTESIAN_POINT ( 'NONE',  ( 0.4658792650918640033, -0.3162353388693405765, 0.4822834645669290543 ) ) ;
#47237=CARTESIAN_POINT ( 'NONE',  ( 1.148293963254593875, -0.6692913385826771977, 0.1292274648535927661 ) ) ;
#47238=CARTESIAN_POINT ( 'NONE',  ( -1.345144356955379816, -0.08942795157528024563, -0.3641732283464568787 ) ) ;
#47239=CARTESIAN_POINT ( 'NONE',  ( 1.358267716535433323, 0.07958543189024085140, 0.2665933059059887866 ) ) ;
#47240=CARTESIAN_POINT ( 'NONE',  ( -1.377952755905511140, -0.5511811023622047445, 6.969142054262312111E-17 ) ) ;
#47241=CARTESIAN_POINT ( 'NONE',  ( -0.8070866141732276899, 0.07958543189024071263, -0.2665933059059888421 ) ) ;
#47242=EDGE_CURVE ( 'NONE', #1065, #22644, #14028, .T. ) ;
#47243=CARTESIAN_POINT ( 'NONE',  ( 1.528871391076116026, -0.6692913385826773087, -0.1292274648535924053 ) ) ;
#47244=CARTESIAN_POINT ( 'NONE',  ( 0.5577427821522314977, -0.2845877964562161244, -0.3641732283464567121 ) ) ;
#47245=CARTESIAN_POINT ( 'NONE',  ( 0.3149606299212606708, -0.1870078740157480879, -0.4822834645669291653 ) ) ;
#47246=CARTESIAN_POINT ( 'NONE',  ( 1.167979002624672580, 0.05413385826771626580, -0.4176697321401330321 ) ) ;
#47247=CARTESIAN_POINT ( 'NONE',  ( 0.2230971128608932319, -0.4281496062992124485, 0.4176697321401328655 ) ) ;
#47248=CARTESIAN_POINT ( 'NONE',  ( 5.463695987328526437E-16, -0.1870078740157479769, 0.3641732283464567677 ) ) ;
#47249=CARTESIAN_POINT ( 'NONE',  ( 1.049868766404200127, -0.6046776061558809534, -0.2411417322834644161 ) ) ;
#47250=CARTESIAN_POINT ( 'NONE',  ( -0.1968503937007867743, 0.2066929133858268208, 0.000000000000000000 ) ) ;
#47251=CARTESIAN_POINT ( 'NONE',  ( -1.108923884514435132, -0.3162353388693405765, 0.4822834645669290543 ) ) ;
#47254=CARTESIAN_POINT ( 'NONE',  ( -0.8005249343832011588, 0.05413385826771626580, -0.4176697321401330321 ) ) ;
#47255=CARTESIAN_POINT ( 'NONE',  ( -0.1115485564304456306, 0.2952755905511810774, -0.1292274648535930714 ) ) ;
#47260=CARTESIAN_POINT ( 'NONE',  ( 1.023622047244095112, -0.1870078740157480879, -0.4822834645669291653 ) ) ;
#47262=CARTESIAN_POINT ( 'NONE',  ( -1.502624671916009680, -0.08942795157528024563, -0.3641732283464568787 ) ) ;
#47264=CARTESIAN_POINT ( 'NONE',  ( 1.574803149606299746, -0.1870078740157479769, 0.3641732283464567677 ) ) ;
#47266=CARTESIAN_POINT ( 'NONE',  ( -0.1706036745406816491, 0.05413385826771626580, -0.4176697321401330321 ) ) ;
#47267=CARTESIAN_POINT ( 'NONE',  ( -0.4921259842519677963, -0.4536011799217367080, 0.2665933059059888421 ) ) ;
#47268=CARTESIAN_POINT ( 'NONE',  ( 0.8005249343832027131, 0.05413385826771666132, 0.4176697321401328100 ) ) ;
#47269=CARTESIAN_POINT ( 'NONE',  ( 0.4921259842519691285, 0.1660481256975885056, 0.3530559997133364547 ) ) ;
#47273=CARTESIAN_POINT ( 'NONE',  ( 1.364829396325460076, 0.2306618581243848609, 0.2411417322834645549 ) ) ;
#47274=CARTESIAN_POINT ( 'NONE',  ( 0.2296587926509192634, -0.05778040916215560624, -0.4822834645669293319 ) ) ;
#47275=CARTESIAN_POINT ( 'NONE',  ( -1.043307086614172041, -0.5400638737290844871, 0.3530559997133364547 ) ) ;
#47276=CARTESIAN_POINT ( 'NONE',  ( 1.318897637795276356, 0.1660481256975883668, -0.3530559997133364547 ) ) ;
#47277=CARTESIAN_POINT ( 'NONE',  ( 0.7808398950131241190, -0.05778040916215560624, -0.4822834645669293319 ) ) ;
#47279=CARTESIAN_POINT ( 'NONE',  ( 5.463695987328526437E-16, -0.1870078740157479769, 0.4822834645669291653 ) ) ;
#47280=CARTESIAN_POINT ( 'NONE',  ( 0.5183727034120741983, -0.6692913385826771977, 0.1292274648535927661 ) ) ;
#47281=CARTESIAN_POINT ( 'NONE',  ( 0.1509186351706045259, -0.05778040916215560624, -0.4822834645669293319 ) ) ;
#47282=CARTESIAN_POINT ( 'NONE',  ( 0.9120734908136490793, 0.1771653543307087075, -0.09757992244046823083 ) ) ;
#47283=CARTESIAN_POINT ( 'NONE',  ( -1.522309711286088607, 0.2306618581243847221, -0.2411417322834647770 ) ) ;
#47284=CARTESIAN_POINT ( 'NONE',  ( -1.496062992125983815, -0.1870078740157480879, -0.4822834645669291653 ) ) ;
#47285=CARTESIAN_POINT ( 'NONE',  ( 0.5643044619422579178, -0.4281496062992127816, -0.4176697321401328100 ) ) ;
#47292=CARTESIAN_POINT ( 'NONE',  ( 0.9514435695538062676, -0.3162353388693409650, -0.4822834645669289433 ) ) ;
#47293=CARTESIAN_POINT ( 'NONE',  ( 0.5446194225721792126, -0.08942795157528024563, -0.3641732283464568787 ) ) ;
#47299=CARTESIAN_POINT ( 'NONE',  ( -1.614173228346455824, 0.2952755905511811885, 0.000000000000000000 ) ) ;
#47300=CARTESIAN_POINT ( 'NONE',  ( -0.2362204724409442680, -0.1870078740157480879, -0.4822834645669291653 ) ) ;
#47301=CARTESIAN_POINT ( 'NONE',  ( 0.8923884514435701520, -0.6046776061558809534, -0.2411417322834644161 ) ) ;
#47303=CARTESIAN_POINT ( 'NONE',  ( -1.548556430446193399, 0.2306618581243848609, 0.2411417322834645549 ) ) ;
#47304=CARTESIAN_POINT ( 'NONE',  ( 1.620734908136483465, -0.5511811023622046335, 0.09757992244046803654 ) ) ;
#47306=CARTESIAN_POINT ( 'NONE',  ( 1.463254593175853824, -0.5511811023622046335, 0.09757992244046803654 ) ) ;
#47308=CARTESIAN_POINT ( 'NONE',  ( -1.305774278215222184, 0.1771653543307087630, 0.09757992244046791164 ) ) ;
#47310=CARTESIAN_POINT ( 'NONE',  ( 0.2493438320209980519, 0.05413385826771666132, 0.4176697321401328100 ) ) ;
#47311=ORIENTED_EDGE ( 'NONE', *, *, #38741, .F. ) ;
#47312=CARTESIAN_POINT ( 'NONE',  ( 1.574803149606299746, -0.1870078740157480879, -0.4822834645669291653 ) ) ;
#47314=CARTESIAN_POINT ( 'NONE',  ( -0.6430446194225716283, -0.3690944881889763329, 0.3153832671262228327 ) ) ;
#47315=CARTESIAN_POINT ( 'NONE',  ( 0.8070866141732289112, -0.5400638737290845981, -0.3530559997133363437 ) ) ;
#47316=CARTESIAN_POINT ( 'NONE',  ( 1.371391076115485719, -0.5511811023622048555, -0.09757992244046775898 ) ) ;
#47318=CARTESIAN_POINT ( 'NONE',  ( -0.7808398950131225646, -0.08942795157527998196, 0.3641732283464567121 ) ) ;
#47319=CARTESIAN_POINT ( 'NONE',  ( -1.384514435695537005, -0.5511811023622048555, -0.09757992244046775898 ) ) ;
#47321=CARTESIAN_POINT ( 'NONE',  ( 0.4593175853018379162, -0.4281496062992124485, 0.4176697321401328655 ) ) ;
#47322=CARTESIAN_POINT ( 'NONE',  ( -0.8202099737532799750, 0.1771653543307087075, -0.09757992244046823083 ) ) ;
#47323=CARTESIAN_POINT ( 'NONE',  ( -0.4068241469816267775, -0.004921259842519870586, -0.3153832671262229437 ) ) ;
#47324=CARTESIAN_POINT ( 'NONE',  ( -0.1968503937007867743, -0.6692913385826771977, 8.415575281601705876E-17 ) ) ;
#47325=CARTESIAN_POINT ( 'NONE',  ( -1.535433070866141225, -0.5511811023622047445, 6.969142054262312111E-17 ) ) ;
#47327=CARTESIAN_POINT ( 'NONE',  ( 0.5314960629921264834, 0.1660481256975883668, -0.3530559997133364547 ) ) ;
#47328=B_SPLINE_CURVE_WITH_KNOTS ( 'NONE', 3,
 ( #32921, #21542, #46790, #58587 ),
 .UNSPECIFIED., .F., .F.,
 ( 4, 4 ),
 ( 1.999999999897049408E-07, 0.006970199999999935128 ),
 .UNSPECIFIED. ) ;
#47332=CARTESIAN_POINT ( 'NONE',  ( -0.6561679790026240244, -0.6046776061558807314, 0.2411417322834647770 ) ) ;
#47333=CARTESIAN_POINT ( 'NONE',  ( -0.1640419947506555343, -0.2845877964562159024, 0.3641732283464567677 ) ) ;
#47334=CARTESIAN_POINT ( 'NONE',  ( -1.417322834645668772, -0.1870078740157480879, -0.4822834645669291653 ) ) ;
#47335=CARTESIAN_POINT ( 'NONE',  ( 0.3608923884514443348, -0.5511811023622046335, 0.09757992244046803654 ) ) ;
#47336=CARTESIAN_POINT ( 'NONE',  ( -0.7545931758530177724, 0.1771653543307087630, 0.09757992244046791164 ) ) ;
#47337=CARTESIAN_POINT ( 'NONE',  ( -0.9645669291338575535, -0.5400638737290844871, 0.3530559997133364547 ) ) ;
#47338=CARTESIAN_POINT ( 'NONE',  ( 1.587926509186352142, -0.004921259842519576551, 0.3153832671262227771 ) ) ;
#47339=CARTESIAN_POINT ( 'NONE',  ( 1.456692913385827515, -0.6692913385826771977, 8.415575281601705876E-17 ) ) ;
#47340=CARTESIAN_POINT ( 'NONE',  ( 1.082677165354331228, 0.1012011053420775880, -0.2882089793578256898 ) ) ;
#47341=CARTESIAN_POINT ( 'NONE',  ( 0.9776902887139113929, -0.5511811023622048555, -0.09757992244046775898 ) ) ;
#47343=CARTESIAN_POINT ( 'NONE',  ( 0.2493438320209980519, 0.05413385826771666132, 0.4176697321401328100 ) ) ;
#47345=CARTESIAN_POINT ( 'NONE',  ( 1.581364829396326277, -0.08942795157527998196, 0.3641732283464567121 ) ) ;
#47349=CARTESIAN_POINT ( 'NONE',  ( -1.135170603674539924, 0.1771653543307087075, -0.09757992244046823083 ) ) ;
#47350=CARTESIAN_POINT ( 'NONE',  ( -0.3805774278215216522, 0.05413385826771666132, 0.4176697321401328100 ) ) ;
#47351=CARTESIAN_POINT ( 'NONE',  ( 0.1115485564304467270, -0.6692913385826773087, -0.1292274648535924053 ) ) ;
#47352=CARTESIAN_POINT ( 'NONE',  ( -1.522309711286088607, 0.1283753931104746893, -0.1820866141732285504 ) ) ;
#47354=CARTESIAN_POINT ( 'NONE',  ( -1.423884514435694859, -0.3162353388693405765, 0.4822834645669290543 ) ) ;
#47355=CARTESIAN_POINT ( 'NONE',  ( 0.3018372703412079971, 0.05413385826771626580, -0.4176697321401330321 ) ) ;
#47356=CARTESIAN_POINT ( 'NONE',  ( -0.07217847769028787330, -0.05778040916215522460, 0.4822834645669289988 ) ) ;
#47357=CARTESIAN_POINT ( 'NONE',  ( 1.200787401574803681, -0.5400638737290845981, -0.3530559997133363437 ) ) ;
#47363=CARTESIAN_POINT ( 'NONE',  ( -0.07217847769028813698, -0.2845877964562161244, -0.3641732283464567121 ) ) ;
#47364=CARTESIAN_POINT ( 'NONE',  ( -0.3871391076115479057, -0.3162353388693409650, -0.4822834645669289433 ) ) ;
#47365=CARTESIAN_POINT ( 'NONE',  ( 0.9711286089238851948, 0.2306618581243848609, 0.2411417322834645549 ) ) ;
#47367=B_SPLINE_CURVE_WITH_KNOTS ( 'NONE', 3,
 ( #14534, #38926, #38513, #6111 ),
 .UNSPECIFIED., .F., .F.,
 ( 4, 4 ),
 ( 1.999999999927407068E-07, 0.006970199999999936863 ),
 .UNSPECIFIED. ) ;
#47368=CARTESIAN_POINT ( 'NONE',  ( -0.04593175853018302557, 0.1771653543307087630, 0.09757992244046791164 ) ) ;
#47369=CARTESIAN_POINT ( 'NONE',  ( -1.056430446194224881, -0.6692913385826771977, 0.1292274648535927661 ) ) ;
#47370=CARTESIAN_POINT ( 'NONE',  ( -1.463254593175852492, 0.2952755905511811885, 0.1292274648535926551 ) ) ;
#47372=CARTESIAN_POINT ( 'NONE',  ( 1.603475055217291612, 1.330568129716842130, -0.04573490813648244807 ) ) ;
#47375=CARTESIAN_POINT ( 'NONE',  ( 1.115485564304462551, 0.05413385826771666132, 0.4176697321401328100 ) ) ;
#47376=CARTESIAN_POINT ( 'NONE',  ( 1.515748031496063186, -0.4536011799217368745, -0.2665933059059886201 ) ) ;
#47377=CARTESIAN_POINT ( 'NONE',  ( -1.095800524934382292, -0.2845877964562161244, -0.3641732283464567121 ) ) ;
#47378=CARTESIAN_POINT ( 'NONE',  ( -1.108923884514435132, -0.05778040916215560624, -0.4822834645669293319 ) ) ;
#47380=LINE ( 'NONE', #54105, #23543 ) ;
#47381=CARTESIAN_POINT ( 'NONE',  ( 1.233595800524935227, 0.2306618581243847221, -0.2411417322834647770 ) ) ;
#47383=CARTESIAN_POINT ( 'NONE',  ( -0.03937007874015669567, -0.6692913385826771977, 8.415575281601705876E-17 ) ) ;
#47384=CARTESIAN_POINT ( 'NONE',  ( -0.1574803149606292529, -0.1870078740157479769, 0.4822834645669291653 ) ) ;
#47385=CARTESIAN_POINT ( 'NONE',  ( -1.312335958005248715, 0.2306618581243848609, 0.2411417322834645549 ) ) ;
#47387=CARTESIAN_POINT ( 'NONE',  ( 0.5708661417322841158, -0.5400638737290845981, -0.3530559997133363437 ) ) ;
#47389=CARTESIAN_POINT ( 'NONE',  ( -1.161417322834644716, 0.07958543189024085140, 0.2665933059059887866 ) ) ;
#47392=EDGE_LOOP ( 'NONE', ( #81478, #77506, #14381, #18499 ) ) ;
#47394=CARTESIAN_POINT ( 'NONE',  ( -1.574803149606298636, -0.1870078740157479769, 0.4822834645669291653 ) ) ;
#47395=CARTESIAN_POINT ( 'NONE',  ( 1.417322834645670104, -0.1870078740157479769, 0.4822834645669291653 ) ) ;
#47397=CARTESIAN_POINT ( 'NONE',  ( -1.640419947506561060, -0.4281496062992127816, -0.4176697321401328100 ) ) ;
#47398=CARTESIAN_POINT ( 'NONE',  ( -1.653543307086613234, -0.1870078740157480879, -0.4822834645669291653 ) ) ;
#47400=B_SPLINE_CURVE_WITH_KNOTS ( 'NONE', 3,
 ( #73843, #23303, #62025, #66698 ),
 .UNSPECIFIED., .F., .F.,
 ( 4, 4 ),
 ( 3.593986969204291827E-07, 0.001287825409103289694 ),
 .UNSPECIFIED. ) ;
#47401=CARTESIAN_POINT ( 'NONE',  ( -0.3543307086614165824, 0.2952755905511811885, 0.000000000000000000 ) ) ;
#47404=CARTESIAN_POINT ( 'NONE',  ( -0.3805774278215216522, -0.004921259842519576551, 0.3153832671262227771 ) ) ;
#47405=CARTESIAN_POINT ( 'NONE',  ( -0.7283464566929126471, 0.07958543189024071263, -0.2665933059059888421 ) ) ;
#47406=CARTESIAN_POINT ( 'NONE',  ( -1.043307086614172041, -0.5400638737290844871, 0.3530559997133364547 ) ) ;
#47407=CARTESIAN_POINT ( 'NONE',  ( 0.9186351706036751663, -0.6046776061558807314, 0.2411417322834647770 ) ) ;
#47408=CARTESIAN_POINT ( 'NONE',  ( -0.9776902887139098386, 0.2952755905511810774, -0.1292274648535930714 ) ) ;
#47411=CARTESIAN_POINT ( 'NONE',  ( -1.384514435695537005, -0.6692913385826773087, -0.1292274648535924053 ) ) ;
#47412=CARTESIAN_POINT ( 'NONE',  ( -1.555118110236219930, 0.07958543189024085140, 0.2665933059059887866 ) ) ;
#47414=DIRECTION ( 'NONE',  ( 0.000000000000000000, 0.000000000000000000, -1.000000000000000000 ) ) ;
#47417=CARTESIAN_POINT ( 'NONE',  ( -0.1837270341207340729, 0.2306618581243847221, -0.2411417322834647770 ) ) ;
#47418=CARTESIAN_POINT ( 'NONE',  ( 1.469816272965879911, -0.6046776061558807314, 0.2411417322834647770 ) ) ;
#47420=CARTESIAN_POINT ( 'NONE',  ( 0.4606732211678801203, 2.401574803149606030, -0.5309055118110237448 ) ) ;
#47421=CARTESIAN_POINT ( 'NONE',  ( -0.6496062992125976043, 0.1012011053420775880, -0.2882089793578256898 ) ) ;
#47422=CARTESIAN_POINT ( 'NONE',  ( -1.286089238845143479, -0.6046776061558807314, 0.2411417322834647770 ) ) ;
#47423=CARTESIAN_POINT ( 'NONE',  ( -0.2427821522309703550, -0.05778040916215560624, -0.4822834645669293319 ) ) ;
#47425=CARTESIAN_POINT ( 'NONE',  ( 0.4790026246719167324, -0.08942795157527998196, 0.3641732283464567121 ) ) ;
#47427=CARTESIAN_POINT ( 'NONE',  ( 0.4986876640419954376, -0.5023911411419708095, -0.1820866141732282451 ) ) ;
#47428=CARTESIAN_POINT ( 'NONE',  ( 0.7480314960629927956, -0.5511811023622047445, 6.969142054262312111E-17 ) ) ;
#47429=CARTESIAN_POINT ( 'NONE',  ( 1.043307086614173818, -0.5400638737290845981, -0.3530559997133363437 ) ) ;
#47430=CARTESIAN_POINT ( 'NONE',  ( -0.4658792650918627265, -0.2845877964562161244, -0.3641732283464567121 ) ) ;
#47432=CARTESIAN_POINT ( 'NONE',  ( -1.371391076115484609, -0.6692913385826771977, 0.1292274648535927661 ) ) ;
#47433=CARTESIAN_POINT ( 'NONE',  ( -0.1443569553805768291, -0.004921259842519576551, 0.3153832671262227771 ) ) ;
#47434=CARTESIAN_POINT ( 'NONE',  ( -1.108923884514435132, -0.08942795157528024563, -0.3641732283464568787 ) ) ;
#47436=CARTESIAN_POINT ( 'NONE',  ( -0.7152230971128602510, -0.2845877964562159024, 0.3641732283464567677 ) ) ;
#47437=CARTESIAN_POINT ( 'NONE',  ( -0.2493438320209966919, -0.4281496062992124485, 0.4176697321401328655 ) ) ;
#47439=CARTESIAN_POINT ( 'NONE',  ( 0.3477690288713918276, 0.1771653543307087630, 0.09757992244046791164 ) ) ;
#47440=CARTESIAN_POINT ( 'NONE',  ( -0.2887139107611542133, 0.1283753931104748280, 0.1820866141732283561 ) ) ;
#47441=CARTESIAN_POINT ( 'NONE',  ( -0.8792650918635160906, -0.4281496062992124485, 0.4176697321401328655 ) ) ;
#47442=CARTESIAN_POINT ( 'NONE',  ( -1.601049868766403650, -0.6046776061558807314, 0.2411417322834647770 ) ) ;
#47443=CARTESIAN_POINT ( 'NONE',  ( -0.9973753280839886548, 0.1283753931104748280, 0.1820866141732283561 ) ) ;
#47445=CARTESIAN_POINT ( 'NONE',  ( 0.3674540682414705883, -0.6046776061558807314, 0.2411417322834647770 ) ) ;
#47447=CARTESIAN_POINT ( 'NONE',  ( 2.795275590551181466, 0.4724409448818907564, -3.234977217930338483E-16 ) ) ;
#47448=CARTESIAN_POINT ( 'NONE',  ( -0.1574803149606292529, -0.1870078740157479769, 0.3641732283464567677 ) ) ;
#47449=CARTESIAN_POINT ( 'NONE',  ( -0.09186351706036689768, 0.05413385826771626580, -0.4176697321401330321 ) ) ;
#47450=CARTESIAN_POINT ( 'NONE',  ( -1.502624671916009680, -0.3162353388693405765, 0.4822834645669290543 ) ) ;
#47451=CARTESIAN_POINT ( 'NONE',  ( -1.515748031496062076, -0.4536011799217367080, 0.2665933059059888421 ) ) ;
#47452=CARTESIAN_POINT ( 'NONE',  ( 1.266404199475066328, -0.3162353388693409650, -0.4822834645669289433 ) ) ;
#47454=CARTESIAN_POINT ( 'NONE',  ( -0.8398950131233589023, -0.5023911411419708095, -0.1820866141732282451 ) ) ;
#47455=CARTESIAN_POINT ( 'NONE',  ( 0.4581548273333326815, 1.539554514603150404, 0.5309055118110234117 ) ) ;
#47460=CARTESIAN_POINT ( 'NONE',  ( 0.9448818897637802916, -0.1870078740157479769, 0.3641732283464567677 ) ) ;
#47462=CARTESIAN_POINT ( 'NONE',  ( 0.8136482939632553313, 0.2306618581243848609, 0.2411417322834645549 ) ) ;
#47464=CARTESIAN_POINT ( 'NONE',  ( 1.240157480314961314, 0.07958543189024071263, -0.2665933059059888421 ) ) ;
#47466=CARTESIAN_POINT ( 'NONE',  ( 0.1509186351706045259, -0.05778040916215560624, -0.4822834645669293319 ) ) ;
#47467=CARTESIAN_POINT ( 'NONE',  ( -0.5577427821522301654, -0.3162353388693405765, 0.4822834645669290543 ) ) ;
#47468=CARTESIAN_POINT ( 'NONE',  ( 1.522309711286089939, 0.2306618581243848609, 0.2411417322834645549 ) ) ;
#47471=CARTESIAN_POINT ( 'NONE',  ( 0.2165354330708668673, 0.07958543189024071263, -0.2665933059059888421 ) ) ;
#47472=ORIENTED_EDGE ( 'NONE', *, *, #32543, .F. ) ;
#47474=VERTEX_POINT ( 'NONE', #56355 ) ;
#47475=CARTESIAN_POINT ( 'NONE',  ( -0.3215223097112853146, -0.3162353388693405765, 0.4822834645669290543 ) ) ;
#47476=CARTESIAN_POINT ( 'NONE',  ( 1.200787401574803681, -0.5400638737290845981, -0.3530559997133363437 ) ) ;
#47477=CARTESIAN_POINT ( 'NONE',  ( 0.1902887139107617975, -0.6692913385826773087, -0.1292274648535924053 ) ) ;
#47478=CARTESIAN_POINT ( 'NONE',  ( -0.3412073490813641308, 0.1283753931104746893, -0.1820866141732285504 ) ) ;
#47479=CARTESIAN_POINT ( 'NONE',  ( 0.6430446194225729606, -0.4281496062992127816, -0.4176697321401328100 ) ) ;
#47480=CARTESIAN_POINT ( 'NONE',  ( -1.036745406824146176, -0.4281496062992124485, 0.4176697321401328655 ) ) ;
#47481=CARTESIAN_POINT ( 'NONE',  ( -0.2624671916010490880, 0.2306618581243847221, -0.2411417322834647770 ) ) ;
#47482=CARTESIAN_POINT ( 'NONE',  ( -0.9514435695538050464, -0.3162353388693405765, 0.4822834645669290543 ) ) ;
#47483=CARTESIAN_POINT ( 'NONE',  ( 1.095800524934383846, -0.3162353388693405765, 0.4822834645669290543 ) ) ;
#47484=CARTESIAN_POINT ( 'NONE',  ( 1.056430446194226436, -0.6692913385826773087, -0.1292274648535924053 ) ) ;
#47485=CARTESIAN_POINT ( 'NONE',  ( 0.8202099737532814183, -0.6692913385826773087, -0.1292274648535924053 ) ) ;
#47488=CARTESIAN_POINT ( 'NONE',  ( -0.006561679790025524116, -0.08942795157528024563, -0.3641732283464568787 ) ) ;
#47489=ORIENTED_EDGE ( 'NONE', *, *, #37822, .F. ) ;
#47491=ORIENTED_EDGE ( 'NONE', *, *, #42958, .T. ) ;
#47492=CARTESIAN_POINT ( 'NONE',  ( -0.7152230971128602510, -0.08942795157528024563, -0.3641732283464568787 ) ) ;
#47493=CARTESIAN_POINT ( 'NONE',  ( 0.05905511811023709395, -0.5400638737290844871, 0.3530559997133364547 ) ) ;
#47495=CARTESIAN_POINT ( 'NONE',  ( -0.4396325459317579898, 0.2952755905511811885, 0.1292274648535926551 ) ) ;
#47496=CARTESIAN_POINT ( 'NONE',  ( -0.5905511811023615998, 0.2952755905511811885, 0.000000000000000000 ) ) ;
#47497=CARTESIAN_POINT ( 'NONE',  ( -1.207349081364828436, -0.6046776061558807314, 0.2411417322834647770 ) ) ;
#47498=CARTESIAN_POINT ( 'NONE',  ( -1.443569553805773564, -0.6046776061558807314, 0.2411417322834647770 ) ) ;
#47499=CARTESIAN_POINT ( 'NONE',  ( 1.305774278215223960, -0.5511811023622046335, 0.09757992244046803654 ) ) ;
#47502=CARTESIAN_POINT ( 'NONE',  ( 0.4199475065616803948, -0.5023911411419708095, -0.1820866141732282451 ) ) ;
#47504=CARTESIAN_POINT ( 'NONE',  ( 0.2034120734908144990, -0.6692913385826771977, 0.1292274648535927661 ) ) ;
#47505=CARTESIAN_POINT ( 'NONE',  ( 0.2821522309711292364, 0.2952755905511810774, -0.1292274648535930714 ) ) ;
#47512=CARTESIAN_POINT ( 'NONE',  ( -0.4068241469816267775, 0.05413385826771626580, -0.4176697321401330321 ) ) ;
#47515=CARTESIAN_POINT ( 'NONE',  ( -1.522309711286088607, -0.5023911411419708095, 0.1820866141732285504 ) ) ;
#47516=CARTESIAN_POINT ( 'NONE',  ( 0.8070866141732288002, 0.1660481256975885056, 0.3530559997133364547 ) ) ;
#47517=CARTESIAN_POINT ( 'NONE',  ( 0.7349081364829403995, 0.2306618581243848609, 0.2411417322834645549 ) ) ;
#47518=CARTESIAN_POINT ( 'NONE',  ( -0.1049868766404193215, -0.5023911411419708095, 0.1820866141732285504 ) ) ;
#47519=CARTESIAN_POINT ( 'NONE',  ( -0.1246719160104980823, 0.2952755905511811885, 0.1292274648535926551 ) ) ;
#47521=CARTESIAN_POINT ( 'NONE',  ( -0.09186351706036663400, -0.3690944881889763329, 0.3153832671262228327 ) ) ;
#47522=CARTESIAN_POINT ( 'NONE',  ( -0.5446194225721777693, -0.3162353388693409650, -0.4822834645669289433 ) ) ;
#47525=CARTESIAN_POINT ( 'NONE',  ( -1.482939632545930975, -0.4281496062992127816, -0.4176697321401328100 ) ) ;
#47526=CARTESIAN_POINT ( 'NONE',  ( 0.1312335958005255154, -0.5023911411419708095, 0.1820866141732285504 ) ) ;
#47527=CARTESIAN_POINT ( 'NONE',  ( 1.548556430446194954, 0.1283753931104746893, -0.1820866141732285504 ) ) ;
#47528=CARTESIAN_POINT ( 'NONE',  ( -1.200787401574802349, 0.1660481256975883668, -0.3530559997133364547 ) ) ;
#47529=CARTESIAN_POINT ( 'NONE',  ( -0.6889763779527552368, 0.07958543189024085140, 0.2665933059059887866 ) ) ;
#47531=CARTESIAN_POINT ( 'NONE',  ( -1.345144356955379816, -0.05778040916215560624, -0.4822834645669293319 ) ) ;
#47532=CARTESIAN_POINT ( 'NONE',  ( -0.6561679790026240244, 0.2306618581243847221, -0.2411417322834647770 ) ) ;
#47533=CARTESIAN_POINT ( 'NONE',  ( 0.1115485564304470323, 0.2952755905511811885, 0.1292274648535926551 ) ) ;
#47537=CARTESIAN_POINT ( 'NONE',  ( 0.4461942257217856311, 0.1283753931104746893, -0.1820866141732285504 ) ) ;
#47539=CARTESIAN_POINT ( 'NONE',  ( 0.9055118110236227702, -0.6692913385826771977, 8.415575281601705876E-17 ) ) ;
#47540=CARTESIAN_POINT ( 'NONE',  ( -1.069553805774277722, 0.1771653543307087630, 0.09757992244046791164 ) ) ;
#47541=CARTESIAN_POINT ( 'NONE',  ( 1.227034120734908917, 0.2952755905511810774, -0.1292274648535930714 ) ) ;
#47542=CARTESIAN_POINT ( 'NONE',  ( -1.384514435695537005, 0.1771653543307087630, 0.09757992244046791164 ) ) ;
#47543=CARTESIAN_POINT ( 'NONE',  ( -0.3280839895013117347, -0.4281496062992124485, 0.4176697321401328655 ) ) ;
#47544=CARTESIAN_POINT ( 'NONE',  ( 0.1181102362204730916, 0.1771653543307087630, 0.000000000000000000 ) ) ;
#47546=CARTESIAN_POINT ( 'NONE',  ( 0.5511811023622054106, -0.1870078740157480601, -0.3641732283464567677 ) ) ;
#47547=EDGE_CURVE ( 'NONE', #18898, #69738, #7151, .T. ) ;
#47548=CARTESIAN_POINT ( 'NONE',  ( -0.2165354330708654795, 0.1660481256975885056, 0.3530559997133364547 ) ) ;
#47550=CARTESIAN_POINT ( 'NONE',  ( -0.6430446194225716283, -0.4281496062992124485, 0.4176697321401328655 ) ) ;
#47552=CARTESIAN_POINT ( 'NONE',  ( 1.003937007874016185, 0.07958543189024071263, -0.2665933059059888421 ) ) ;
#47553=CARTESIAN_POINT ( 'NONE',  ( 0.2559055118110243332, 0.1660481256975885056, 0.3530559997133364547 ) ) ;
#47554=CARTESIAN_POINT ( 'NONE',  ( -0.1968503937007867743, 0.2952755905511811885, 0.000000000000000000 ) ) ;
#47555=CARTESIAN_POINT ( 'NONE',  ( -0.1968503937007867743, 0.1771653543307087630, 0.000000000000000000 ) ) ;
#47556=CARTESIAN_POINT ( 'NONE',  ( -0.6167979002624665030, -0.3690944881889765550, -0.3153832671262227771 ) ) ;
#47557=CARTESIAN_POINT ( 'NONE',  ( 0.4133858267716541968, 0.1660481256975885056, 0.3530559997133364547 ) ) ;
#47558=CARTESIAN_POINT ( 'NONE',  ( -0.7217847769028863381, -0.004921259842519870586, -0.3153832671262229437 ) ) ;
#47560=CARTESIAN_POINT ( 'NONE',  ( -1.279527559055116948, 0.1660481256975883668, -0.3530559997133364547 ) ) ;
#47562=ORIENTED_EDGE ( 'NONE', *, *, #21129, .T. ) ;
#47564=CARTESIAN_POINT ( 'NONE',  ( -1.036745406824146176, -0.004921259842519870586, -0.3153832671262229437 ) ) ;
#47565=CARTESIAN_POINT ( 'NONE',  ( -0.3740157480314953431, -0.5400638737290845981, -0.3530559997133363437 ) ) ;
#47567=CARTESIAN_POINT ( 'NONE',  ( -0.5971128608923877978, -0.6692913385826773087, -0.1292274648535924053 ) ) ;
#47569=CARTESIAN_POINT ( 'NONE',  ( 1.220472440944882608, 0.2952755905511811885, 0.000000000000000000 ) ) ;
#47570=CARTESIAN_POINT ( 'NONE',  ( 1.023622047244095334, -0.1870078740157479769, 0.4822834645669291653 ) ) ;
#47574=CARTESIAN_POINT ( 'NONE',  ( -1.699475065616797398, 0.2952755905511811885, 0.1292274648535926551 ) ) ;
#47577=CARTESIAN_POINT ( 'NONE',  ( -0.5971128608923877978, -0.5511811023622048555, -0.09757992244046775898 ) ) ;
#47581=CARTESIAN_POINT ( 'NONE',  ( 0.7545931758530188826, -0.6692913385826771977, 0.1292274648535927661 ) ) ;
#47582=CARTESIAN_POINT ( 'NONE',  ( 0.05249343832021075018, 0.2306618581243847221, -0.2411417322834647770 ) ) ;
#47583=CARTESIAN_POINT ( 'NONE',  ( -0.6430446194225712953, 0.05413385826771626580, -0.4176697321401330321 ) ) ;
#47584=CARTESIAN_POINT ( 'NONE',  ( 1.423884514435696413, -0.3162353388693409650, -0.4822834645669289433 ) ) ;
#47585=CARTESIAN_POINT ( 'NONE',  ( -1.430446194225720724, -0.004921259842519870586, -0.3153832671262229437 ) ) ;
#47587=CARTESIAN_POINT ( 'NONE',  ( 0.4002624671916016896, -0.05778040916215522460, 0.4822834645669289988 ) ) ;
#47588=CARTESIAN_POINT ( 'NONE',  ( 0.6167979002624678353, -0.3690944881889763329, 0.3153832671262228327 ) ) ;
#47589=CARTESIAN_POINT ( 'NONE',  ( -0.6430446194225712953, 0.05413385826771626580, -0.4176697321401330321 ) ) ;
#47591=CARTESIAN_POINT ( 'NONE',  ( -1.259842519685038686, -0.1870078740157480879, -0.4822834645669291653 ) ) ;
#47593=CARTESIAN_POINT ( 'NONE',  ( 0.8792650918635177559, 0.05413385826771666132, 0.4176697321401328100 ) ) ;
#47594=CARTESIAN_POINT ( 'NONE',  ( 1.423884514435696413, -0.2845877964562161244, -0.3641732283464567121 ) ) ;
#47595=ORIENTED_EDGE ( 'NONE', *, *, #24051, .F. ) ;
#47597=CARTESIAN_POINT ( 'NONE',  ( -0.4593175853018364174, -0.4281496062992127816, -0.4176697321401328100 ) ) ;
#47599=CARTESIAN_POINT ( 'NONE',  ( 0.5183727034120741983, 0.1771653543307087075, -0.09757992244046823083 ) ) ;
#47600=CARTESIAN_POINT ( 'NONE',  ( -1.069553805774277722, 0.2952755905511811885, 0.1292274648535926551 ) ) ;
#47601=CARTESIAN_POINT ( 'NONE',  ( 0.8727034120734912248, -0.3162353388693409650, -0.4822834645669289433 ) ) ;
#47602=CARTESIAN_POINT ( 'NONE',  ( 0.9580052493438326877, 0.05413385826771666132, 0.4176697321401328100 ) ) ;
#47603=CARTESIAN_POINT ( 'NONE',  ( -0.1377952755905504645, 0.1660481256975885056, 0.3530559997133364547 ) ) ;
#47604=CARTESIAN_POINT ( 'NONE',  ( -0.5118110236220466680, 0.2952755905511811885, 0.000000000000000000 ) ) ;
#47606=CARTESIAN_POINT ( 'NONE',  ( 1.528871391076116026, -0.5511811023622048555, -0.09757992244046775898 ) ) ;
#47607=CARTESIAN_POINT ( 'NONE',  ( -0.4265091863517051496, -0.6692913385826771977, 0.1292274648535927661 ) ) ;
#47608=CARTESIAN_POINT ( 'NONE',  ( -0.3674540682414689785, 0.1283753931104748280, 0.1820866141732283561 ) ) ;
#47609=CARTESIAN_POINT ( 'NONE',  ( 1.227034120734908917, 0.2952755905511810774, -0.1292274648535930714 ) ) ;
#47610=CARTESIAN_POINT ( 'NONE',  ( -0.9973753280839886548, -0.6046776061558809534, -0.2411417322834644161 ) ) ;
#47612=CARTESIAN_POINT ( 'NONE',  ( 0.7152230971128614723, -0.3162353388693409650, -0.4822834645669289433 ) ) ;
#47616=CARTESIAN_POINT ( 'NONE',  ( -0.3149606299212590610, -0.1870078740157480879, -0.4822834645669291653 ) ) ;
#47617=CARTESIAN_POINT ( 'NONE',  ( -1.003937007874014853, 0.07958543189024085140, 0.2665933059059887866 ) ) ;
#47618=CARTESIAN_POINT ( 'NONE',  ( 1.148293963254593875, -0.5511811023622046335, 0.09757992244046803654 ) ) ;
#47620=CARTESIAN_POINT ( 'NONE',  ( 1.292650918635171564, -0.5511811023622048555, -0.09757992244046775898 ) ) ;
#47622=CARTESIAN_POINT ( 'NONE',  ( 0.7611548556430451917, -0.6046776061558807314, 0.2411417322834647770 ) ) ;
#47624=CARTESIAN_POINT ( 'NONE',  ( -0.3674540682414692561, -0.6046776061558809534, -0.2411417322834644161 ) ) ;
#47626=AXIS2_PLACEMENT_3D ( 'NONE', #65753, #77958, #33341 ) ;
#47627=CARTESIAN_POINT ( 'NONE',  ( 1.528871391076116026, -0.5511811023622048555, -0.09757992244046775898 ) ) ;
#47628=CARTESIAN_POINT ( 'NONE',  ( -0.7414698162729651543, 0.2952755905511810774, -0.1292274648535930714 ) ) ;
#47629=EDGE_CURVE ( 'NONE', #53888, #42092, #15539, .T. ) ;
#47631=CARTESIAN_POINT ( 'NONE',  ( 1.318897637795276356, -0.5400638737290844871, 0.3530559997133364547 ) ) ;
#47632=CARTESIAN_POINT ( 'NONE',  ( 0.09842519685039434474, -0.5400638737290845981, -0.3530559997133363437 ) ) ;
#47633=CARTESIAN_POINT ( 'NONE',  ( 0.4133858267716541968, 0.07958543189024085140, 0.2665933059059887866 ) ) ;
#47635=CARTESIAN_POINT ( 'NONE',  ( 0.4199475065616805614, 0.1283753931104748280, 0.1820866141732283561 ) ) ;
#47638=CARTESIAN_POINT ( 'NONE',  ( 0.5774278215223104249, 0.2306618581243848609, 0.2411417322834645549 ) ) ;
#47640=CARTESIAN_POINT ( 'NONE',  ( 1.417322834645670104, -0.1870078740157480601, -0.3641732283464567677 ) ) ;
#47642=CARTESIAN_POINT ( 'NONE',  ( -0.1509186351706028884, -0.08942795157527998196, 0.3641732283464567121 ) ) ;
#47644=CARTESIAN_POINT ( 'NONE',  ( 0.3083989501312343062, -0.05778040916215560624, -0.4822834645669293319 ) ) ;
#47645=CARTESIAN_POINT ( 'NONE',  ( 1.351706036745407680, -0.004921259842519576551, 0.3153832671262227771 ) ) ;
#47646=CARTESIAN_POINT ( 'NONE',  ( -1.528871391076114250, 0.1771653543307087075, -0.09757992244046823083 ) ) ;
#47647=CARTESIAN_POINT ( 'NONE',  ( -1.509186351706035767, 0.05413385826771626580, -0.4176697321401330321 ) ) ;
#47648=CARTESIAN_POINT ( 'NONE',  ( 0.6299212598425204535, -0.1870078740157480879, -0.4822834645669291653 ) ) ;
#47649=CARTESIAN_POINT ( 'NONE',  ( 1.673228346456693494, 0.1660481256975885056, 0.3530559997133364547 ) ) ;
#47650=CARTESIAN_POINT ( 'NONE',  ( 1.614173228346457378, 1.330640075373405118, -0.1372047244094476148 ) ) ;
#47651=CARTESIAN_POINT ( 'NONE',  ( 0.4330708661417329575, -0.6692913385826771977, 8.415575281601705876E-17 ) ) ;
#47652=CARTESIAN_POINT ( 'NONE',  ( 1.174540682414699111, -0.3162353388693405765, 0.4822834645669290543 ) ) ;
#47653=CARTESIAN_POINT ( 'NONE',  ( 1.049868766404200349, 0.2306618581243848609, 0.2411417322834645549 ) ) ;
#47655=CARTESIAN_POINT ( 'NONE',  ( 1.154855643044620184, -0.5023911411419708095, 0.1820866141732285504 ) ) ;
#47656=CARTESIAN_POINT ( 'NONE',  ( -1.653543307086613234, -0.1870078740157479769, 0.3641732283464567677 ) ) ;
#47657=CARTESIAN_POINT ( 'NONE',  ( -0.9317585301837263412, -0.3690944881889765550, -0.3153832671262227771 ) ) ;
#47659=CARTESIAN_POINT ( 'NONE',  ( 0.5971128608923890191, -0.5511811023622046335, 0.09757992244046803654 ) ) ;
#47660=CARTESIAN_POINT ( 'NONE',  ( 0.01312335958005323398, -0.4281496062992127816, -0.4176697321401328100 ) ) ;
#47661=CARTESIAN_POINT ( 'NONE',  ( 0.7939632545931766261, -0.05778040916215522460, 0.4822834645669289988 ) ) ;
#47662=CARTESIAN_POINT ( 'NONE',  ( -0.4790026246719152336, -0.05778040916215560624, -0.4822834645669293319 ) ) ;
#47663=CARTESIAN_POINT ( 'NONE',  ( 0.1443569553805781891, -0.3690944881889763329, 0.3153832671262228327 ) ) ;
#47664=CARTESIAN_POINT ( 'NONE',  ( 1.351706036745407458, -0.4281496062992127816, -0.4176697321401328100 ) ) ;
#47666=CARTESIAN_POINT ( 'NONE',  ( -1.017060367454067249, -0.3162353388693409650, -0.4822834645669289433 ) ) ;
#47670=CARTESIAN_POINT ( 'NONE',  ( -0.7217847769028863381, -0.4281496062992124485, 0.4176697321401328655 ) ) ;
#47671=CARTESIAN_POINT ( 'NONE',  ( -0.4330708661417315697, 0.2952755905511811885, 0.000000000000000000 ) ) ;
#47675=CARTESIAN_POINT ( 'NONE',  ( 0.8136482939632553313, -0.5023911411419708095, -0.1820866141732282451 ) ) ;
#47677=CARTESIAN_POINT ( 'NONE',  ( 1.292650918635171564, 0.2952755905511811885, 0.1292274648535926551 ) ) ;
#47679=CARTESIAN_POINT ( 'NONE',  ( -1.561679790026246017, -0.004921259842519576551, 0.3153832671262227771 ) ) ;
#47680=DIRECTION ( 'NONE',  ( -3.096699300667737957E-16, 1.000000000000000000, -0.000000000000000000 ) ) ;
#47681=CARTESIAN_POINT ( 'NONE',  ( -1.706036745406823485, 0.2306618581243848609, 0.2411417322834645549 ) ) ;
#47683=CARTESIAN_POINT ( 'NONE',  ( -0.09842519685039295696, -0.5400638737290844871, 0.3530559997133364547 ) ) ;
#47684=CARTESIAN_POINT ( 'NONE',  ( -0.6561679790026240244, -0.5023911411419708095, 0.1820866141732285504 ) ) ;
#47685=CARTESIAN_POINT ( 'NONE',  ( 0.9120734908136489683, -0.6692913385826771977, 0.1292274648535927661 ) ) ;
#47686=CARTESIAN_POINT ( 'NONE',  ( 0.1181102362204730916, -0.6692913385826771977, 8.415575281601705876E-17 ) ) ;
#47691=CARTESIAN_POINT ( 'NONE',  ( 0.7611548556430454138, 0.2306618581243847221, -0.2411417322834647770 ) ) ;
#47692=CARTESIAN_POINT ( 'NONE',  ( 0.2559055118110243332, -0.5400638737290845981, -0.3530559997133363437 ) ) ;
#47693=CARTESIAN_POINT ( 'NONE',  ( -0.9514435695538050464, -0.05778040916215560624, -0.4822834645669293319 ) ) ;
#47694=CARTESIAN_POINT ( 'NONE',  ( 1.266404199475066328, -0.05778040916215522460, 0.4822834645669289988 ) ) ;
#47695=CARTESIAN_POINT ( 'NONE',  ( 0.9055118110236227702, 0.2952755905511811885, 0.000000000000000000 ) ) ;
#47697=CARTESIAN_POINT ( 'NONE',  ( -0.3215223097112853146, -0.3162353388693405765, 0.4822834645669290543 ) ) ;
#47698=CARTESIAN_POINT ( 'NONE',  ( 0.6036745406824154392, 0.2306618581243847221, -0.2411417322834647770 ) ) ;
#47699=CARTESIAN_POINT ( 'NONE',  ( -0.1902887139107604098, 0.2952755905511810774, -0.1292274648535930714 ) ) ;
#47700=CARTESIAN_POINT ( 'NONE',  ( 0.8202099737532814183, -0.5511811023622048555, -0.09757992244046775898 ) ) ;
#47701=CARTESIAN_POINT ( 'NONE',  ( -1.286089238845143479, -0.6046776061558807314, 0.2411417322834647770 ) ) ;
#47702=CARTESIAN_POINT ( 'NONE',  ( -1.699475065616797398, 0.2952755905511811885, 0.1292274648535926551 ) ) ;
#47703=CARTESIAN_POINT ( 'NONE',  ( 0.3477690288713918276, 0.2952755905511811885, 0.1292274648535926551 ) ) ;
#47708=CARTESIAN_POINT ( 'NONE',  ( 1.017060367454068803, -0.3162353388693405765, 0.4822834645669290543 ) ) ;
#47709=CARTESIAN_POINT ( 'NONE',  ( 0.7217847769028878924, -0.3690944881889765550, -0.3153832671262227771 ) ) ;
#47714=B_SPLINE_CURVE_WITH_KNOTS ( 'NONE', 3,
 ( #6484, #38050, #75963, #38464, #37236, #32154, #76373 ),
 .UNSPECIFIED., .F., .F.,
 ( 4, 3, 4 ),
 ( 1.387778780781445521E-17, 0.001246230184515555910, 0.002492489877932651133 ),
 .UNSPECIFIED. ) ;
#47715=EDGE_CURVE ( 'NONE', #65845, #71339, #27595, .T. ) ;
#47717=CARTESIAN_POINT ( 'NONE',  ( -0.9776902887139098386, 0.2952755905511810774, -0.1292274648535930714 ) ) ;
#47718=CARTESIAN_POINT ( 'NONE',  ( -0.5708661417322828946, 0.1660481256975883668, -0.3530559997133364547 ) ) ;
#47719=CARTESIAN_POINT ( 'NONE',  ( 1.161417322834646271, 0.1660481256975883668, -0.3530559997133364547 ) ) ;
#47721=CARTESIAN_POINT ( 'NONE',  ( 1.253280839895013710, -0.3162353388693405765, 0.4822834645669290543 ) ) ;
#47724=CARTESIAN_POINT ( 'NONE',  ( -1.614173228346456712, 0.4405861044731111953, -0.1372047244094478091 ) ) ;
#47725=CARTESIAN_POINT ( 'NONE',  ( -1.220472440944881054, -0.5511811023622047445, 6.969142054262312111E-17 ) ) ;
#47726=DIRECTION ( 'NONE',  ( -3.096699300667737957E-16, 1.000000000000000000, -0.000000000000000000 ) ) ;
#47727=CARTESIAN_POINT ( 'NONE',  ( 0.1837270341207357105, -0.6046776061558809534, -0.2411417322834644161 ) ) ;
#47728=CARTESIAN_POINT ( 'NONE',  ( 1.548556430446194954, 0.2306618581243847221, -0.2411417322834647770 ) ) ;
#47729=DIRECTION ( 'NONE',  ( -1.000000000000000000, -3.050063254464715288E-16, 0.000000000000000000 ) ) ;
#47730=CARTESIAN_POINT ( 'NONE',  ( -1.246719160104986512, -0.004921259842519576551, 0.3153832671262227771 ) ) ;
#47731=CARTESIAN_POINT ( 'NONE',  ( 0.8595800524934390507, -0.3162353388693405765, 0.4822834645669290543 ) ) ;
#47732=CARTESIAN_POINT ( 'NONE',  ( 1.423884514435696191, -0.08942795157527998196, 0.3641732283464567121 ) ) ;
#47734=CARTESIAN_POINT ( 'NONE',  ( -0.8333333333333323711, -0.5511811023622048555, -0.09757992244046775898 ) ) ;
#47735=CARTESIAN_POINT ( 'NONE',  ( 1.555118110236221041, 0.1660481256975883668, -0.3530559997133364547 ) ) ;
#47737=CARTESIAN_POINT ( 'NONE',  ( -0.05249343832020938322, -0.6046776061558809534, -0.2411417322834644161 ) ) ;
#47738=CARTESIAN_POINT ( 'NONE',  ( -0.9448818897637790704, -0.1870078740157480601, -0.3641732283464567677 ) ) ;
#47739=CARTESIAN_POINT ( 'NONE',  ( -0.2559055118110230564, 0.07958543189024071263, -0.2665933059059888421 ) ) ;
#47740=CARTESIAN_POINT ( 'NONE',  ( -0.09186351706036689768, 0.05413385826771626580, -0.4176697321401330321 ) ) ;
#47741=CARTESIAN_POINT ( 'NONE',  ( -1.423884514435694859, -0.08942795157528024563, -0.3641732283464568787 ) ) ;
#47743=CARTESIAN_POINT ( 'NONE',  ( 0.3937007874015754361, -0.1870078740157480879, -0.4822834645669291653 ) ) ;
#47744=LINE ( 'NONE', #35132, #29635 ) ;
#47747=CARTESIAN_POINT ( 'NONE',  ( -0.6758530183727028406, -0.6692913385826773087, -0.1292274648535924053 ) ) ;
#47748=CARTESIAN_POINT ( 'NONE',  ( -0.1377952755905504645, 0.07958543189024085140, 0.2665933059059887866 ) ) ;
#47749=CARTESIAN_POINT ( 'NONE',  ( -1.377952755905511140, -0.6692913385826771977, 8.415575281601705876E-17 ) ) ;
#47750=CARTESIAN_POINT ( 'NONE',  ( 0.1902887139107617975, -0.6692913385826773087, -0.1292274648535924053 ) ) ;
#47751=CARTESIAN_POINT ( 'NONE',  ( 0.5643044619422579178, -0.004921259842519576551, 0.3153832671262227771 ) ) ;
#47753=CARTESIAN_POINT ( 'NONE',  ( -0.7939632545931754048, -0.2845877964562159024, 0.3641732283464567677 ) ) ;
#47754=CARTESIAN_POINT ( 'NONE',  ( -0.9776902887139098386, -0.6692913385826771977, 0.1292274648535927661 ) ) ;
#47755=CARTESIAN_POINT ( 'NONE',  ( -1.561679790026246017, 0.05413385826771666132, 0.4176697321401328100 ) ) ;
#47756=CARTESIAN_POINT ( 'NONE',  ( 1.522309711286089939, 0.2306618581243848609, 0.2411417322834645549 ) ) ;
#47758=CARTESIAN_POINT ( 'NONE',  ( 1.069553805774278832, 0.1771653543307087075, -0.09757992244046823083 ) ) ;
#47759=CARTESIAN_POINT ( 'NONE',  ( 0.7086614173228353852, -0.1870078740157479769, 0.4822834645669291653 ) ) ;
#47761=CARTESIAN_POINT ( 'NONE',  ( 1.259842519685040019, -0.1870078740157479769, 0.3641732283464567677 ) ) ;
#47763=CARTESIAN_POINT ( 'NONE',  ( -0.6955380577427815458, 0.05413385826771666132, 0.4176697321401328100 ) ) ;
#47765=CARTESIAN_POINT ( 'NONE',  ( -1.364829396325458521, -0.5023911411419708095, 0.1820866141732285504 ) ) ;
#47766=CARTESIAN_POINT ( 'NONE',  ( -0.5774278215223089816, -0.6046776061558807314, 0.2411417322834647770 ) ) ;
#47767=CARTESIAN_POINT ( 'NONE',  ( 0.4790026246719167324, -0.05778040916215522460, 0.4822834645669289988 ) ) ;
#47768=CARTESIAN_POINT ( 'NONE',  ( -1.686351706036744558, 0.1771653543307087075, -0.09757992244046823083 ) ) ;
#47770=CARTESIAN_POINT ( 'NONE',  ( -1.253280839895012377, -0.05778040916215522460, 0.4822834645669289988 ) ) ;
#47771=CARTESIAN_POINT ( 'NONE',  ( 0.3871391076115493490, -0.3162353388693405765, 0.4822834645669290543 ) ) ;
#47772=CARTESIAN_POINT ( 'NONE',  ( -0.1312335958005241554, -0.6046776061558809534, -0.2411417322834644161 ) ) ;
#47773=CARTESIAN_POINT ( 'NONE',  ( 1.062992125984252745, -0.6692913385826771977, 8.415575281601705876E-17 ) ) ;
#47779=CARTESIAN_POINT ( 'NONE',  ( -0.1771653543307080136, -0.4536011799217367080, 0.2665933059059888421 ) ) ;
#47780=CARTESIAN_POINT ( 'NONE',  ( -0.2362204724409442680, -0.1870078740157480879, -0.4822834645669291653 ) ) ;
#47781=CARTESIAN_POINT ( 'NONE',  ( 1.076115485564305141, -0.6046776061558807314, 0.2411417322834647770 ) ) ;
#47783=CARTESIAN_POINT ( 'NONE',  ( 0.01968503937007957949, -0.4536011799217368745, -0.2665933059059886201 ) ) ;
#47784=CARTESIAN_POINT ( 'NONE',  ( -1.043307086614172041, -0.5400638737290844871, 0.3530559997133364547 ) ) ;
#47785=CARTESIAN_POINT ( 'NONE',  ( 1.082677165354331228, -0.5400638737290844871, 0.3530559997133364547 ) ) ;
#47790=CARTESIAN_POINT ( 'NONE',  ( 1.003937007874016185, 0.1660481256975883668, -0.3530559997133364547 ) ) ;
#47791=CARTESIAN_POINT ( 'NONE',  ( 1.587926509186352142, -0.004921259842519576551, 0.3153832671262227771 ) ) ;
#47792=CARTESIAN_POINT ( 'NONE',  ( -1.141732283464566011, 0.1771653543307087630, 0.000000000000000000 ) ) ;
#47793=CARTESIAN_POINT ( 'NONE',  ( -1.213910761154854745, -0.6692913385826771977, 0.1292274648535927661 ) ) ;
#47795=CARTESIAN_POINT ( 'NONE',  ( 1.191441481664479829, -2.398893483443748302E-16, 0.4281993546915529580 ) ) ;
#47796=CARTESIAN_POINT ( 'NONE',  ( 1.318897637795276356, -0.5400638737290844871, 0.3530559997133364547 ) ) ;
#47797=CARTESIAN_POINT ( 'NONE',  ( -1.561679790026246017, 0.05413385826771666132, 0.4176697321401328100 ) ) ;
#47798=CARTESIAN_POINT ( 'NONE',  ( -0.05905511811023545637, -0.5400638737290845981, -0.3530559997133363437 ) ) ;
#47799=CARTESIAN_POINT ( 'NONE',  ( -0.4330708661417315697, 0.2952755905511811885, 0.000000000000000000 ) ) ;
#47800=CARTESIAN_POINT ( 'NONE',  ( -1.443569553805773564, 0.2306618581243847221, -0.2411417322834647770 ) ) ;
#47803=CARTESIAN_POINT ( 'NONE',  ( 0.006561679790026889343, -0.05778040916215522460, 0.4822834645669289988 ) ) ;
#47805=CARTESIAN_POINT ( 'NONE',  ( -1.292650918635170010, 0.1771653543307087075, -0.09757992244046823083 ) ) ;
#47808=VERTEX_POINT ( 'NONE', #82459 ) ;
#47811=CARTESIAN_POINT ( 'NONE',  ( -1.673228346456691717, 0.1660481256975883668, -0.3530559997133364547 ) ) ;
#47813=CARTESIAN_POINT ( 'NONE',  ( -1.515748031496062076, 0.1660481256975883668, -0.3530559997133364547 ) ) ;
#47815=CARTESIAN_POINT ( 'NONE',  ( 0.4265091863517068149, 0.2952755905511811885, 0.1292274648535926551 ) ) ;
#47816=LINE ( 'NONE', #54961, #68686 ) ;
#47819=CARTESIAN_POINT ( 'NONE',  ( -0.4396325459317577122, -0.5511811023622048555, -0.09757992244046775898 ) ) ;
#47820=CARTESIAN_POINT ( 'NONE',  ( -0.8792650918635160906, -0.004921259842519870586, -0.3153832671262229437 ) ) ;
#47821=CARTESIAN_POINT ( 'NONE',  ( -1.108923884514435132, -0.05778040916215560624, -0.4822834645669293319 ) ) ;
#47822=CARTESIAN_POINT ( 'NONE',  ( 0.5511811023622054106, -0.1870078740157480879, -0.4822834645669291653 ) ) ;
#47823=CARTESIAN_POINT ( 'NONE',  ( -0.7086614173228339419, -0.1870078740157479769, 0.4822834645669291653 ) ) ;
#47826=CARTESIAN_POINT ( 'NONE',  ( -1.581364829396324945, -0.05778040916215560624, -0.4822834645669293319 ) ) ;
#47832=CARTESIAN_POINT ( 'NONE',  ( -0.8005249343832011588, 0.05413385826771626580, -0.4176697321401330321 ) ) ;
#47833=CARTESIAN_POINT ( 'NONE',  ( 1.561679790026247350, 0.05413385826771626580, -0.4176697321401330321 ) ) ;
#47835=CARTESIAN_POINT ( 'NONE',  ( -1.594488188976377563, -0.5400638737290844871, 0.3530559997133364547 ) ) ;
#47836=CARTESIAN_POINT ( 'NONE',  ( -0.6962418744208963561, -2.294479370626195693E-15, 0.3464511005275217603 ) ) ;
#47837=CARTESIAN_POINT ( 'NONE',  ( -1.522309711286088607, 0.2306618581243847221, -0.2411417322834647770 ) ) ;
#47838=CARTESIAN_POINT ( 'NONE',  ( -0.9120734908136475250, 0.2952755905511811885, 0.1292274648535926551 ) ) ;
#47840=CARTESIAN_POINT ( 'NONE',  ( 0.5314960629921264834, 0.07958543189024071263, -0.2665933059059888421 ) ) ;
#47842=CARTESIAN_POINT ( 'NONE',  ( 0.1771653543307093182, -0.4536011799217368745, -0.2665933059059886201 ) ) ;
#47843=CARTESIAN_POINT ( 'NONE',  ( 1.010498687664042716, -0.004921259842519870586, -0.3153832671262229437 ) ) ;
#47844=CARTESIAN_POINT ( 'NONE',  ( 0.9317585301837276734, -0.4281496062992124485, 0.4176697321401328655 ) ) ;
#47845=CARTESIAN_POINT ( 'NONE',  ( -0.1246719160104980823, -0.5511811023622048555, -0.09757992244046775898 ) ) ;
#47847=CARTESIAN_POINT ( 'NONE',  ( 1.561679790026247350, -0.4281496062992124485, 0.4176697321401328655 ) ) ;
#47848=CARTESIAN_POINT ( 'NONE',  ( -1.076115485564303809, -0.5023911411419708095, -0.1820866141732282451 ) ) ;
#47849=VECTOR ( 'NONE', #12978, 39.37007874015748143 ) ;
#47852=CARTESIAN_POINT ( 'NONE',  ( -0.8923884514435688198, -0.5023911411419708095, 0.1820866141732285504 ) ) ;
#47853=CARTESIAN_POINT ( 'NONE',  ( 0.03280839895013198948, -0.6692913385826773087, -0.1292274648535924053 ) ) ;
#47854=CARTESIAN_POINT ( 'NONE',  ( 0.5314960629921264834, 0.07958543189024071263, -0.2665933059059888421 ) ) ;
#47855=CARTESIAN_POINT ( 'NONE',  ( -0.3018372703412066094, -0.004921259842519576551, 0.3153832671262227771 ) ) ;
#47856=CARTESIAN_POINT ( 'NONE',  ( -0.5577427821522301654, -0.3162353388693405765, 0.4822834645669290543 ) ) ;
#47857=DIRECTION ( 'NONE',  ( -3.096699300667737957E-16, 1.000000000000000000, -0.000000000000000000 ) ) ;
#47859=CARTESIAN_POINT ( 'NONE',  ( 0.2952755905511819101, 0.1660481256975883668, -0.3530559997133364547 ) ) ;
#47861=CARTESIAN_POINT ( 'NONE',  ( 1.384514435695538337, -0.6692913385826771977, 0.1292274648535927661 ) ) ;
#47862=CARTESIAN_POINT ( 'NONE',  ( -0.1443569553805768291, -0.004921259842519576551, 0.3153832671262227771 ) ) ;
#47863=VECTOR ( 'NONE', #217, 39.37007874015748143 ) ;
#47864=CARTESIAN_POINT ( 'NONE',  ( -0.2362204724409442680, -0.1870078740157480879, -0.4822834645669291653 ) ) ;
#47865=CARTESIAN_POINT ( 'NONE',  ( -1.476377952755905110, 0.1660481256975885056, 0.3530559997133364547 ) ) ;
#47866=CARTESIAN_POINT ( 'NONE',  ( -1.587926509186350810, -0.004921259842519870586, -0.3153832671262229437 ) ) ;
#47867=CARTESIAN_POINT ( 'NONE',  ( 1.450131233595801428, -0.6692913385826773087, -0.1292274648535924053 ) ) ;
#47868=CARTESIAN_POINT ( 'NONE',  ( -0.6364829396325453192, -0.2845877964562159024, 0.3641732283464567677 ) ) ;
#47872=CARTESIAN_POINT ( 'NONE',  ( 1.515748031496063408, 0.07958543189024085140, 0.2665933059059887866 ) ) ;
#47873=CARTESIAN_POINT ( 'NONE',  ( 1.240157480314961314, -0.4536011799217367080, 0.2665933059059888421 ) ) ;
#47875=CARTESIAN_POINT ( 'NONE',  ( 0.7939632545931766261, -0.05778040916215522460, 0.4822834645669289988 ) ) ;
#47877=CARTESIAN_POINT ( 'NONE',  ( 1.259842519685040019, -0.1870078740157480601, -0.3641732283464567677 ) ) ;
#47878=CARTESIAN_POINT ( 'NONE',  ( -0.05249343832020911260, 0.2306618581243848609, 0.2411417322834645549 ) ) ;
#47879=CARTESIAN_POINT ( 'NONE',  ( -0.4068241469816264999, -0.4281496062992124485, 0.4176697321401328655 ) ) ;
#47883=CARTESIAN_POINT ( 'NONE',  ( 0.1509186351706042484, -0.2845877964562159024, 0.3641732283464567677 ) ) ;
#47886=ORIENTED_EDGE ( 'NONE', *, *, #8937, .T. ) ;
#47887=CARTESIAN_POINT ( 'NONE',  ( -0.3149606299212590610, -0.1870078740157479769, 0.4822834645669291653 ) ) ;
#47888=CARTESIAN_POINT ( 'NONE',  ( 1.043307086614173818, -0.5400638737290845981, -0.3530559997133363437 ) ) ;
#47889=CARTESIAN_POINT ( 'NONE',  ( 0.3937007874015754361, -0.1870078740157479769, 0.4822834645669291653 ) ) ;
#47890=CARTESIAN_POINT ( 'NONE',  ( -0.4199475065616791736, -0.5023911411419708095, 0.1820866141732285504 ) ) ;
#47891=CARTESIAN_POINT ( 'NONE',  ( 0.9776902887139113929, -0.6692913385826773087, -0.1292274648535924053 ) ) ;
#47892=CARTESIAN_POINT ( 'NONE',  ( -0.7742782152230962556, -0.4281496062992127816, -0.4176697321401328100 ) ) ;
#47893=CARTESIAN_POINT ( 'NONE',  ( -0.5839895013123351797, 0.2952755905511810774, -0.1292274648535930714 ) ) ;
#47894=CARTESIAN_POINT ( 'NONE',  ( -0.7152230971128602510, -0.05778040916215560624, -0.4822834645669293319 ) ) ;
#47895=CARTESIAN_POINT ( 'NONE',  ( 1.325459317585302665, 0.05413385826771626580, -0.4176697321401330321 ) ) ;
#47896=CARTESIAN_POINT ( 'NONE',  ( 0.8136482939632553313, 0.2306618581243848609, 0.2411417322834645549 ) ) ;
#47897=CARTESIAN_POINT ( 'NONE',  ( 0.8530183727034128527, -0.4281496062992124485, 0.4176697321401328655 ) ) ;
#47899=CARTESIAN_POINT ( 'NONE',  ( 0.1509186351706045259, -0.08942795157528024563, -0.3641732283464568787 ) ) ;
#47900=ORIENTED_EDGE ( 'NONE', *, *, #29559, .T. ) ;
#47904=CARTESIAN_POINT ( 'NONE',  ( -1.043307086614172707, 0.07958543189024071263, -0.2665933059059888421 ) ) ;
#47905=CIRCLE ( 'NONE', #33143, 2.362204724409449064 ) ;
#47907=CARTESIAN_POINT ( 'NONE',  ( -0.2690288713910754526, -0.6692913385826771977, 0.1292274648535927661 ) ) ;
#47909=CARTESIAN_POINT ( 'NONE',  ( -0.3149606299212590610, -0.1870078740157479769, 0.4822834645669291653 ) ) ;
#47910=CARTESIAN_POINT ( 'NONE',  ( -0.5839895013123351797, 0.2952755905511810774, -0.1292274648535930714 ) ) ;
#47911=CARTESIAN_POINT ( 'NONE',  ( -1.227034120734907141, -0.6692913385826773087, -0.1292274648535924053 ) ) ;
#47912=CARTESIAN_POINT ( 'NONE',  ( -1.286089238845143479, -0.6046776061558807314, 0.2411417322834647770 ) ) ;
#47913=CARTESIAN_POINT ( 'NONE',  ( 0.8136482939632553313, -0.5023911411419708095, -0.1820866141732282451 ) ) ;
#47916=CARTESIAN_POINT ( 'NONE',  ( 0.5774278215223103139, -0.5023911411419708095, -0.1820866141732282451 ) ) ;
#47917=CARTESIAN_POINT ( 'NONE',  ( 0.2099737532808405305, -0.6046776061558807314, 0.2411417322834647770 ) ) ;
#47918=CARTESIAN_POINT ( 'NONE',  ( 0.1443569553805781891, 0.05413385826771626580, -0.4176697321401330321 ) ) ;
#47921=CARTESIAN_POINT ( 'NONE',  ( -1.614173228346457378, 0.9921945702958913094, 0.1372047244094476981 ) ) ;
#47925=CARTESIAN_POINT ( 'NONE',  ( -0.6167979002624665030, -0.004921259842519576551, 0.3153832671262227771 ) ) ;
#47926=CARTESIAN_POINT ( 'NONE',  ( -1.010498687664041384, -0.4281496062992127816, -0.4176697321401328100 ) ) ;
#47928=( BOUNDED_CURVE ( )  B_SPLINE_CURVE ( 2, ( #65085, #7423, #1123, #9503, #10752, #36005, #3189, #74730, #49450, #62084, #28438, #67174, #29680 ),
 .UNSPECIFIED., .F., .F. ) 
 B_SPLINE_CURVE_WITH_KNOTS ( ( 3, 2, 2, 2, 2, 2, 3 ),
 ( 0.1278765491802554000, 0.1287878787878787845, 0.1325757575757575690, 0.1363636363636363535, 0.1401515151515151381, 0.1439393939393939503, 0.1448507235470174181 ),
 .UNSPECIFIED. ) 
 CURVE ( )  GEOMETRIC_REPRESENTATION_ITEM ( )  RATIONAL_B_SPLINE_CURVE ( ( 0.9875488213027527884, 0.9918020599134683701, 1.000000000000000000, 0.9659258262890683122, 1.000000000000000000, 0.9659258262890683122, 1.000000000000000000, 0.9659258262890683122, 1.000000000000000000, 0.9659258262890683122, 1.000000000000000000, 0.9918020599134675930, 0.9875488213027519002 ) ) 
 REPRESENTATION_ITEM ( '' )  );
#47930=CARTESIAN_POINT ( 'NONE',  ( 1.548556430446194954, 0.2306618581243847221, -0.2411417322834647770 ) ) ;
#47931=CARTESIAN_POINT ( 'NONE',  ( 0.9383202099737536495, -0.3162353388693405765, 0.4822834645669290543 ) ) ;
#47933=CARTESIAN_POINT ( 'NONE',  ( 0.3477690288713918276, -0.6692913385826773087, -0.1292274648535924053 ) ) ;
#47934=CARTESIAN_POINT ( 'NONE',  ( -0.6102362204724400829, -0.4536011799217368745, -0.2665933059059886201 ) ) ;
#47935=CARTESIAN_POINT ( 'NONE',  ( 0.1377952755905518800, -0.5400638737290844871, 0.3530559997133364547 ) ) ;
#47937=CARTESIAN_POINT ( 'NONE',  ( -0.07217847769028787330, -0.08942795157527998196, 0.3641732283464567121 ) ) ;
#47938=CARTESIAN_POINT ( 'NONE',  ( -0.3740157480314953431, -0.5400638737290845981, -0.3530559997133363437 ) ) ;
#47940=CARTESIAN_POINT ( 'NONE',  ( -1.437007874015747477, -0.5400638737290844871, 0.3530559997133364547 ) ) ;
#47941=CARTESIAN_POINT ( 'NONE',  ( 0.1837270341207354329, 0.1283753931104748280, 0.1820866141732283561 ) ) ;
#47942=CARTESIAN_POINT ( 'NONE',  ( 1.496062992125985147, -0.1870078740157479769, 0.3641732283464567677 ) ) ;
#47943=CARTESIAN_POINT ( 'NONE',  ( -1.253280839895012377, -0.05778040916215522460, 0.4822834645669289988 ) ) ;
#47944=ADVANCED_FACE ( 'NONE', ( #57586 ), #64954, .F. ) ;
#47945=CARTESIAN_POINT ( 'NONE',  ( -0.7939632545931750718, -0.08942795157528024563, -0.3641732283464568787 ) ) ;
#47947=CARTESIAN_POINT ( 'NONE',  ( -1.167979002624671470, -0.4281496062992127816, -0.4176697321401328100 ) ) ;
#47948=CARTESIAN_POINT ( 'NONE',  ( -0.01312335958005186876, 0.05413385826771626580, -0.4176697321401330321 ) ) ;
#47951=CARTESIAN_POINT ( 'NONE',  ( -1.243977641345850094, 2.305458150815133500, 0.5876520854053413068 ) ) ;
#47952=CARTESIAN_POINT ( 'NONE',  ( 0.4133858267716541968, 0.07958543189024085140, 0.2665933059059887866 ) ) ;
#47953=CARTESIAN_POINT ( 'NONE',  ( 1.089238845144357537, -0.4281496062992124485, 0.4176697321401328655 ) ) ;
#47954=CARTESIAN_POINT ( 'NONE',  ( -1.332020997375327642, -0.2845877964562161244, -0.3641732283464567121 ) ) ;
#47955=CARTESIAN_POINT ( 'NONE',  ( 1.181102362204725198, -0.1870078740157479769, 0.4822834645669291653 ) ) ;
#47956=CARTESIAN_POINT ( 'NONE',  ( -1.515748031496062076, 0.07958543189024071263, -0.2665933059059888421 ) ) ;
#47957=CARTESIAN_POINT ( 'NONE',  ( -0.6627296587926503335, -0.6692913385826771977, 0.1292274648535927661 ) ) ;
#47958=CARTESIAN_POINT ( 'NONE',  ( 0.2690288713910767848, 0.1771653543307087630, 0.09757992244046791164 ) ) ;
#47960=CARTESIAN_POINT ( 'NONE',  ( 0.4724409448818904789, -0.1870078740157479769, 0.3641732283464567677 ) ) ;
#47962=CARTESIAN_POINT ( 'NONE',  ( -0.1837270341207340729, 0.2306618581243847221, -0.2411417322834647770 ) ) ;
#47965=CARTESIAN_POINT ( 'NONE',  ( -1.154855643044618851, -0.6046776061558809534, -0.2411417322834644161 ) ) ;
#47966=VECTOR ( 'NONE', #74359, 39.37007874015748143 ) ;
#47968=CARTESIAN_POINT ( 'NONE',  ( 1.115485564304462551, -0.004921259842519576551, 0.3153832671262227771 ) ) ;
#47969=CARTESIAN_POINT ( 'NONE',  ( -0.1181102362204717315, -0.6692913385826771977, 8.415575281601705876E-17 ) ) ;
#47970=COLOUR_RGB ( '', 0.09019608, 0.27058824, 0.51372549) ;
#47972=CARTESIAN_POINT ( 'NONE',  ( -0.3083989501312330295, -0.3162353388693409650, -0.4822834645669289433 ) ) ;
#47973=CARTESIAN_POINT ( 'NONE',  ( -0.5643044619422565855, -0.3690944881889763329, 0.3153832671262228327 ) ) ;
#47975=CARTESIAN_POINT ( 'NONE',  ( -0.5314960629921250401, 0.07958543189024085140, 0.2665933059059887866 ) ) ;
#47976=CARTESIAN_POINT ( 'NONE',  ( 0.2559055118110243332, 0.1660481256975885056, 0.3530559997133364547 ) ) ;
#47977=CARTESIAN_POINT ( 'NONE',  ( -0.6233595800524928121, -0.08942795157527998196, 0.3641732283464567121 ) ) ;
#47979=CARTESIAN_POINT ( 'NONE',  ( -1.010498687664041384, 0.05413385826771666132, 0.4176697321401328100 ) ) ;
#47981=ORIENTED_EDGE ( 'NONE', *, *, #54784, .F. ) ;
#47982=CARTESIAN_POINT ( 'NONE',  ( -1.272965879265091305, -0.3690944881889763329, 0.3153832671262228327 ) ) ;
#47983=CARTESIAN_POINT ( 'NONE',  ( -0.2559055118110230564, 0.1660481256975883668, -0.3530559997133364547 ) ) ;
#47985=CARTESIAN_POINT ( 'NONE',  ( -1.719160104986876103, 0.05413385826771666132, 0.4176697321401328100 ) ) ;
#47986=CARTESIAN_POINT ( 'NONE',  ( -1.194225721784776262, -0.4281496062992124485, 0.4176697321401328655 ) ) ;
#47988=CARTESIAN_POINT ( 'NONE',  ( 1.272965879265092637, -0.4281496062992127816, -0.4176697321401328100 ) ) ;
#47989=CARTESIAN_POINT ( 'NONE',  ( 0.8595800524934390507, -0.3162353388693405765, 0.4822834645669290543 ) ) ;
#47990=CARTESIAN_POINT ( 'NONE',  ( 1.013613127888309595, -4.408777212815537393E-16, -0.4445507791589063395 ) ) ;
#47991=CARTESIAN_POINT ( 'NONE',  ( 1.473278426072732961, 0.2335363939278403966, 0.2780995266831706725 ) ) ;
#47992=CARTESIAN_POINT ( 'NONE',  ( 1.555118110236221041, -0.4536011799217367080, 0.2665933059059888421 ) ) ;
#47995=CARTESIAN_POINT ( 'NONE',  ( -0.5314960629921250401, 0.07958543189024085140, 0.2665933059059887866 ) ) ;
#47998=CARTESIAN_POINT ( 'NONE',  ( 0.7414698162729663755, -0.6692913385826773087, -0.1292274648535924053 ) ) ;
#47999=CARTESIAN_POINT ( 'NONE',  ( -0.4133858267716528645, 0.1660481256975883668, -0.3530559997133364547 ) ) ;
#48000=CARTESIAN_POINT ( 'NONE',  ( -1.181102362204723644, -0.1870078740157479769, 0.4822834645669291653 ) ) ;
#48001=CARTESIAN_POINT ( 'NONE',  ( 1.318897637795276356, -0.5400638737290844871, 0.3530559997133364547 ) ) ;
#48002=CARTESIAN_POINT ( 'NONE',  ( -1.102362204724408601, -0.1870078740157480601, -0.3641732283464567677 ) ) ;
#48004=CARTESIAN_POINT ( 'NONE',  ( 0.2296587926509192634, -0.3162353388693405765, 0.4822834645669290543 ) ) ;
#48005=CARTESIAN_POINT ( 'NONE',  ( -0.8727034120734901146, -0.3162353388693405765, 0.4822834645669290543 ) ) ;
#48007=CARTESIAN_POINT ( 'NONE',  ( -1.141732283464566011, 0.2952755905511811885, 0.000000000000000000 ) ) ;
#48009=CARTESIAN_POINT ( 'NONE',  ( 0.8333333333333340365, -0.6692913385826771977, 0.1292274648535927661 ) ) ;
#48010=CARTESIAN_POINT ( 'NONE',  ( 1.417322834645670104, -0.1870078740157480601, -0.3641732283464567677 ) ) ;
#48013=CARTESIAN_POINT ( 'NONE',  ( -0.4396325459317577122, -0.6692913385826773087, -0.1292274648535924053 ) ) ;
#48015=CARTESIAN_POINT ( 'NONE',  ( 0.5118110236220478892, 0.1771653543307087630, 0.000000000000000000 ) ) ;
#48016=CARTESIAN_POINT ( 'NONE',  ( -1.115485564304461219, -0.4281496062992124485, 0.4176697321401328655 ) ) ;
#48017=CARTESIAN_POINT ( 'NONE',  ( 0.9514435695538062676, -0.05778040916215522460, 0.4822834645669289988 ) ) ;
#48018=CARTESIAN_POINT ( 'NONE',  ( 1.036745406824147508, -0.4281496062992127816, -0.4176697321401328100 ) ) ;
#48019=CARTESIAN_POINT ( 'NONE',  ( -0.2690288713910754526, 0.2952755905511810774, -0.1292274648535930714 ) ) ;
#48021=CARTESIAN_POINT ( 'NONE',  ( -0.5971128608923877978, -0.6692913385826773087, -0.1292274648535924053 ) ) ;
#48023=CARTESIAN_POINT ( 'NONE',  ( -1.423884514435694859, -0.3162353388693405765, 0.4822834645669290543 ) ) ;
#48024=CARTESIAN_POINT ( 'NONE',  ( -0.7020997375328074108, -0.05778040916215522460, 0.4822834645669289988 ) ) ;
#48025=CARTESIAN_POINT ( 'NONE',  ( -0.3280839895013117347, -0.004921259842519870586, -0.3153832671262229437 ) ) ;
#48026=CARTESIAN_POINT ( 'NONE',  ( 1.338582677165355062, -0.1870078740157479769, 0.4822834645669291653 ) ) ;
#48027=CARTESIAN_POINT ( 'NONE',  ( 1.627296587926509996, -0.6046776061558807314, 0.2411417322834647770 ) ) ;
#48028=CARTESIAN_POINT ( 'NONE',  ( -1.108923884514435132, -0.3162353388693405765, 0.4822834645669290543 ) ) ;
#48030=CARTESIAN_POINT ( 'NONE',  ( 0.7020997375328090762, -0.05778040916215560624, -0.4822834645669293319 ) ) ;
#48032=CARTESIAN_POINT ( 'NONE',  ( 1.594488188976378673, 0.1660481256975885056, 0.3530559997133364547 ) ) ;
#48034=CARTESIAN_POINT ( 'NONE',  ( 0.006561679790026889343, -0.3162353388693409650, -0.4822834645669289433 ) ) ;
#48035=CARTESIAN_POINT ( 'NONE',  ( -1.141732283464566011, 0.1771653543307087630, 0.000000000000000000 ) ) ;
#48036=CARTESIAN_POINT ( 'NONE',  ( 0.4002624671916016896, -0.08942795157527998196, 0.3641732283464567121 ) ) ;
#48038=CARTESIAN_POINT ( 'NONE',  ( 1.364829396325460076, 0.1283753931104748280, 0.1820866141732283561 ) ) ;
#48039=CARTESIAN_POINT ( 'NONE',  ( 0.7480314960629927956, -0.6692913385826771977, 8.415575281601705876E-17 ) ) ;
#48042=CARTESIAN_POINT ( 'NONE',  ( -0.2427821522309703550, -0.05778040916215560624, -0.4822834645669293319 ) ) ;
#48044=CARTESIAN_POINT ( 'NONE',  ( 1.450131233595801428, 0.1771653543307087630, 0.09757992244046791164 ) ) ;
#48045=CARTESIAN_POINT ( 'NONE',  ( -0.5380577427821514602, -0.4281496062992127816, -0.4176697321401328100 ) ) ;
#48047=CARTESIAN_POINT ( 'NONE',  ( 1.443569553805774897, -0.6046776061558809534, -0.2411417322834644161 ) ) ;
#48048=CARTESIAN_POINT ( 'NONE',  ( -0.01968503937007793844, -0.5400638737290844871, 0.3530559997133364547 ) ) ;
#48049=CARTESIAN_POINT ( 'NONE',  ( 0.4068241469816281097, -0.004921259842519576551, 0.3153832671262227771 ) ) ;
#48051=CARTESIAN_POINT ( 'NONE',  ( 0.03937007874015833325, -0.5511811023622047445, 6.969142054262312111E-17 ) ) ;
#48052=CARTESIAN_POINT ( 'NONE',  ( -1.489501312335957062, -0.05778040916215522460, 0.4822834645669289988 ) ) ;
#48054=CARTESIAN_POINT ( 'NONE',  ( 0.8595800524934390507, -0.3162353388693405765, 0.4822834645669290543 ) ) ;
#48056=CARTESIAN_POINT ( 'NONE',  ( 1.666666666666667185, -0.004921259842519576551, 0.3153832671262227771 ) ) ;
#48058=CARTESIAN_POINT ( 'NONE',  ( 0.02624671916010564918, 0.1283753931104748280, 0.1820866141732283561 ) ) ;
#48059=CARTESIAN_POINT ( 'NONE',  ( 0.07217847769028949700, -0.3162353388693405765, 0.4822834645669290543 ) ) ;
#48060=CARTESIAN_POINT ( 'NONE',  ( 1.437007874015748810, -0.4536011799217368745, -0.2665933059059886201 ) ) ;
#48061=CARTESIAN_POINT ( 'NONE',  ( -1.443569553805773564, -0.5023911411419708095, 0.1820866141732285504 ) ) ;
#48062=CARTESIAN_POINT ( 'NONE',  ( -1.548556430446193399, 0.2306618581243848609, 0.2411417322834645549 ) ) ;
#48063=CARTESIAN_POINT ( 'NONE',  ( 0.3543307086614181922, -0.6692913385826771977, 8.415575281601705876E-17 ) ) ;
#48064=CARTESIAN_POINT ( 'NONE',  ( 1.095800524934383846, -0.05778040916215560624, -0.4822834645669293319 ) ) ;
#48066=CARTESIAN_POINT ( 'NONE',  ( 0.5118110236220478892, 0.2952755905511811885, 0.000000000000000000 ) ) ;
#48067=CARTESIAN_POINT ( 'NONE',  ( 1.240157480314961314, 0.1660481256975883668, -0.3530559997133364547 ) ) ;
#48068=CARTESIAN_POINT ( 'NONE',  ( 1.017060367454068803, -0.3162353388693405765, 0.4822834645669290543 ) ) ;
#48070=CARTESIAN_POINT ( 'NONE',  ( 0.9055118110236227702, 0.1771653543307087630, 0.000000000000000000 ) ) ;
#48071=CARTESIAN_POINT ( 'NONE',  ( 1.469816272965879911, -0.6046776061558807314, 0.2411417322834647770 ) ) ;
#48072=CARTESIAN_POINT ( 'NONE',  ( -0.9908136482939626788, 0.1771653543307087630, 0.09757992244046791164 ) ) ;
#48073=CARTESIAN_POINT ( 'NONE',  ( 0.3805774278215230400, -0.004921259842519870586, -0.3153832671262229437 ) ) ;
#48074=CARTESIAN_POINT ( 'NONE',  ( 0.1181102362204730916, 0.2952755905511811885, 0.000000000000000000 ) ) ;
#48075=CARTESIAN_POINT ( 'NONE',  ( 0.6364829396325465405, -0.05778040916215522460, 0.4822834645669289988 ) ) ;
#48076=CARTESIAN_POINT ( 'NONE',  ( -0.4199475065616791736, -0.6046776061558807314, 0.2411417322834647770 ) ) ;
#48077=CARTESIAN_POINT ( 'NONE',  ( 0.1246719160104994284, -0.5511811023622046335, 0.09757992244046803654 ) ) ;
#48078=CARTESIAN_POINT ( 'NONE',  ( 0.7414698162729663755, -0.6692913385826773087, -0.1292274648535924053 ) ) ;
#48079=CARTESIAN_POINT ( 'NONE',  ( -1.220472440944878834, 0.8346805926620878280, -0.5309055118110234117 ) ) ;
#48080=CARTESIAN_POINT ( 'NONE',  ( -0.8661417322834640276, -0.1870078740157480879, -0.4822834645669291653 ) ) ;
#48081=CARTESIAN_POINT ( 'NONE',  ( 1.586688153636164111, 1.522296263979924902, 0.1275903502784767052 ) ) ;
#48084=VECTOR ( 'NONE', #66521, 39.37007874015748854 ) ;
#48085=CARTESIAN_POINT ( 'NONE',  ( -0.8661417322834640276, -0.1870078740157479769, 0.4822834645669291653 ) ) ;
#48086=CARTESIAN_POINT ( 'NONE',  ( -0.6561679790026240244, -0.6046776061558807314, 0.2411417322834647770 ) ) ;
#48091=CARTESIAN_POINT ( 'NONE',  ( 0.6233595800524942554, -0.08942795157528024563, -0.3641732283464568787 ) ) ;
#48093=CARTESIAN_POINT ( 'NONE',  ( 1.207349081364829990, -0.6046776061558809534, -0.2411417322834644161 ) ) ;
#48096=CARTESIAN_POINT ( 'NONE',  ( -1.443569553805773564, -0.5023911411419708095, 0.1820866141732285504 ) ) ;
#48097=CARTESIAN_POINT ( 'NONE',  ( 1.443569553805774897, -0.6046776061558809534, -0.2411417322834644161 ) ) ;
#48098=CARTESIAN_POINT ( 'NONE',  ( -1.614173228346456268, -0.6692913385826771977, 8.415575281601705876E-17 ) ) ;
#48099=CARTESIAN_POINT ( 'NONE',  ( 0.2821522309711292364, 0.2952755905511810774, -0.1292274648535930714 ) ) ;
#48102=CARTESIAN_POINT ( 'NONE',  ( -0.04593175853018302557, 0.2952755905511811885, 0.1292274648535926551 ) ) ;
#48103=SHAPE_REPRESENTATION ( 'Reversible Hardened Steel Jaws', ( #22098 ), #14119 ) ;
#48104=CARTESIAN_POINT ( 'NONE',  ( -0.8923884514435688198, 0.1283753931104746893, -0.1820866141732285504 ) ) ;
#48105=CARTESIAN_POINT ( 'NONE',  ( 1.003937007874016185, 0.1660481256975883668, -0.3530559997133364547 ) ) ;
#48106=CARTESIAN_POINT ( 'NONE',  ( -0.04593175853018302557, -0.6692913385826773087, -0.1292274648535924053 ) ) ;
#48110=CARTESIAN_POINT ( 'NONE',  ( 0.6496062992125991586, -0.5400638737290845981, -0.3530559997133363437 ) ) ;
#48111=CARTESIAN_POINT ( 'NONE',  ( 0.06561679790026316017, 0.05413385826771626580, -0.4176697321401330321 ) ) ;
#48112=CARTESIAN_POINT ( 'NONE',  ( -1.141732283464566011, 0.2952755905511811885, 0.000000000000000000 ) ) ;
#48113=CARTESIAN_POINT ( 'NONE',  ( 1.187664041994751285, -0.3162353388693409650, -0.4822834645669289433 ) ) ;
#48114=CARTESIAN_POINT ( 'NONE',  ( 0.6036745406824154392, 0.2306618581243847221, -0.2411417322834647770 ) ) ;
#48116=CARTESIAN_POINT ( 'NONE',  ( -0.4330708661417315697, 0.2952755905511811885, 0.000000000000000000 ) ) ;
#48117=CARTESIAN_POINT ( 'NONE',  ( 0.6692913385826778638, -0.6692913385826771977, 8.415575281601705876E-17 ) ) ;
#48118=CARTESIAN_POINT ( 'NONE',  ( -0.05249343832020911260, 0.2306618581243848609, 0.2411417322834645549 ) ) ;
#48119=CARTESIAN_POINT ( 'NONE',  ( 0.7874015748031503170, -0.1870078740157480601, -0.3641732283464567677 ) ) ;
#48120=CARTESIAN_POINT ( 'NONE',  ( -1.312335958005248715, -0.6046776061558809534, -0.2411417322834644161 ) ) ;
#48122=CARTESIAN_POINT ( 'NONE',  ( 0.3083989501312343062, -0.3162353388693405765, 0.4822834645669290543 ) ) ;
#48128=CARTESIAN_POINT ( 'NONE',  ( 1.332020997375329197, -0.3162353388693405765, 0.4822834645669290543 ) ) ;
#48129=CARTESIAN_POINT ( 'NONE',  ( 0.7283464566929140904, -0.4536011799217368745, -0.2665933059059886201 ) ) ;
#48136=CARTESIAN_POINT ( 'NONE',  ( -0.7808398950131222316, -0.3162353388693409650, -0.4822834645669289433 ) ) ;
#48137=CARTESIAN_POINT ( 'NONE',  ( -0.7480314960629914633, 0.2952755905511811885, 0.000000000000000000 ) ) ;
#48138=CARTESIAN_POINT ( 'NONE',  ( 0.7611548556430451917, -0.6046776061558807314, 0.2411417322834647770 ) ) ;
#48140=CARTESIAN_POINT ( 'NONE',  ( 1.528871391076116026, -0.6692913385826773087, -0.1292274648535924053 ) ) ;
#48141=CARTESIAN_POINT ( 'NONE',  ( 1.646981627296588035, -0.2845877964562159024, 0.3641732283464567677 ) ) ;
#48145=CARTESIAN_POINT ( 'NONE',  ( -1.279527559055116948, 0.07958543189024071263, -0.2665933059059888421 ) ) ;
#48146=ADVANCED_FACE ( 'NONE', ( #17893 ), #50674, .F. ) ;
#48148=CARTESIAN_POINT ( 'NONE',  ( 0.2296587926509192634, -0.3162353388693405765, 0.4822834645669290543 ) ) ;
#48150=CARTESIAN_POINT ( 'NONE',  ( 1.679790026246720025, 0.2306618581243848609, 0.2411417322834645549 ) ) ;
#48152=CARTESIAN_POINT ( 'NONE',  ( -1.003937007874015297, -0.4536011799217368745, -0.2665933059059886201 ) ) ;
#48153=CARTESIAN_POINT ( 'NONE',  ( 0.2755905511811031494, 0.2952755905511811885, 0.000000000000000000 ) ) ;
#48154=CARTESIAN_POINT ( 'NONE',  ( 1.148293963254593653, 0.1771653543307087075, -0.09757992244046823083 ) ) ;
#48156=CARTESIAN_POINT ( 'NONE',  ( -1.161417322834644716, -0.4536011799217368745, -0.2665933059059886201 ) ) ;
#48157=CARTESIAN_POINT ( 'NONE',  ( 1.391076115485564868, 0.2306618581243847221, -0.2411417322834647770 ) ) ;
#48159=CARTESIAN_POINT ( 'NONE',  ( -0.05905511811023545637, -0.5400638737290845981, -0.3530559997133363437 ) ) ;
#48160=CARTESIAN_POINT ( 'NONE',  ( -1.253280839895012377, -0.2845877964562161244, -0.3641732283464567121 ) ) ;
#48161=CARTESIAN_POINT ( 'NONE',  ( -0.4790026246719154557, -0.2845877964562159024, 0.3641732283464567677 ) ) ;
#48162=CARTESIAN_POINT ( 'NONE',  ( -0.8595800524934373854, -0.3162353388693409650, -0.4822834645669289433 ) ) ;
#48163=CARTESIAN_POINT ( 'NONE',  ( -1.371391076115484609, -0.5511811023622046335, 0.09757992244046803654 ) ) ;
#48165=CARTESIAN_POINT ( 'NONE',  ( 0.4133858267716541968, -0.5400638737290845981, -0.3530559997133363437 ) ) ;
#48168=CARTESIAN_POINT ( 'NONE',  ( -1.062992125984250968, 0.2952755905511811885, 0.000000000000000000 ) ) ;
#48169=CARTESIAN_POINT ( 'NONE',  ( -0.4133858267716528645, 0.07958543189024071263, -0.2665933059059888421 ) ) ;
#48170=CARTESIAN_POINT ( 'NONE',  ( 0.7981007675632553200, -1.206088964116209378E-16, 0.4118477457932991359 ) ) ;
#48171=CARTESIAN_POINT ( 'NONE',  ( -0.04593175853018302557, 0.2952755905511811885, 0.1292274648535926551 ) ) ;
#48172=CARTESIAN_POINT ( 'NONE',  ( 0.3018372703412079971, -0.004921259842519870586, -0.3153832671262229437 ) ) ;
#48173=CARTESIAN_POINT ( 'NONE',  ( -0.5577427821522301654, -0.08942795157528024563, -0.3641732283464568787 ) ) ;
#48174=CARTESIAN_POINT ( 'NONE',  ( -1.620734908136482577, -0.6692913385826773087, -0.1292274648535924053 ) ) ;
#48175=CARTESIAN_POINT ( 'NONE',  ( -1.371391076115484831, 0.2952755905511810774, -0.1292274648535930714 ) ) ;
#48176=CARTESIAN_POINT ( 'NONE',  ( 1.338582677165355062, -0.1870078740157479769, 0.4822834645669291653 ) ) ;
#48178=CARTESIAN_POINT ( 'NONE',  ( 0.9448818897637802916, -0.1870078740157480601, -0.3641732283464567677 ) ) ;
#48179=CARTESIAN_POINT ( 'NONE',  ( 0.8202099737532814183, -0.6692913385826773087, -0.1292274648535924053 ) ) ;
#48180=CARTESIAN_POINT ( 'NONE',  ( -0.01000891935578489267, 8.471767977567108961E-16, -0.4445507791589058955 ) ) ;
#48181=CARTESIAN_POINT ( 'NONE',  ( 1.574803149606299746, -0.1870078740157479769, 0.3641732283464567677 ) ) ;
#48183=CARTESIAN_POINT ( 'NONE',  ( -1.305774278215222184, 0.2952755905511811885, 0.1292274648535926551 ) ) ;
#48184=CARTESIAN_POINT ( 'NONE',  ( -0.8792650918635160906, -0.4281496062992124485, 0.4176697321401328655 ) ) ;
#48185=CARTESIAN_POINT ( 'NONE',  ( 0.2755905511811031494, -0.6692913385826771977, 8.415575281601705876E-17 ) ) ;
#48186=CARTESIAN_POINT ( 'NONE',  ( -1.358267716535432434, 0.07958543189024071263, -0.2665933059059888421 ) ) ;
#48188=CARTESIAN_POINT ( 'NONE',  ( 1.541994750656168645, -0.5511811023622046335, 0.09757992244046803654 ) ) ;
#48189=CARTESIAN_POINT ( 'NONE',  ( 0.2427821522309719648, -0.05778040916215522460, 0.4822834645669289988 ) ) ;
#48190=CARTESIAN_POINT ( 'NONE',  ( 0.7742782152230978099, -0.4281496062992124485, 0.4176697321401328655 ) ) ;
#48192=EDGE_CURVE ( 'NONE', #33111, #31856, #47714, .T. ) ;
#48199=CARTESIAN_POINT ( 'NONE',  ( 0.04593175853018440641, 0.1771653543307087075, -0.09757992244046823083 ) ) ;
#48200=CARTESIAN_POINT ( 'NONE',  ( -0.2821522309711278487, 0.2952755905511811885, 0.1292274648535926551 ) ) ;
#48201=CARTESIAN_POINT ( 'NONE',  ( 0.9251968503937015864, -0.5400638737290844871, 0.3530559997133364547 ) ) ;
#48203=CARTESIAN_POINT ( 'NONE',  ( -0.05249343832020911260, 0.1283753931104748280, 0.1820866141732283561 ) ) ;
#48204=CARTESIAN_POINT ( 'NONE',  ( -1.017060367454067249, -0.05778040916215522460, 0.4822834645669289988 ) ) ;
#48205=CARTESIAN_POINT ( 'NONE',  ( 1.141732283464567566, 0.2952755905511811885, 0.000000000000000000 ) ) ;
#48209=ORIENTED_EDGE ( 'NONE', *, *, #49907, .T. ) ;
#48211=CARTESIAN_POINT ( 'NONE',  ( 0.8727034120734912248, -0.3162353388693409650, -0.4822834645669289433 ) ) ;
#48212=CARTESIAN_POINT ( 'NONE',  ( -1.712598425196849572, 0.1660481256975885056, 0.3530559997133364547 ) ) ;
#48213=CARTESIAN_POINT ( 'NONE',  ( -1.332020997375327642, -0.08942795157527998196, 0.3641732283464567121 ) ) ;
#48214=CARTESIAN_POINT ( 'NONE',  ( -1.456692913385826182, 0.2952755905511811885, 0.000000000000000000 ) ) ;
#48216=DIRECTION ( 'NONE',  ( 0.000000000000000000, 1.000000000000000000, 0.000000000000000000 ) ) ;
#48217=CARTESIAN_POINT ( 'NONE',  ( 1.227034120734908917, 0.2952755905511810774, -0.1292274648535930714 ) ) ;
#48219=CARTESIAN_POINT ( 'NONE',  ( 5.463695987328526437E-16, -0.1870078740157479769, 0.4822834645669291653 ) ) ;
#48220=CARTESIAN_POINT ( 'NONE',  ( -0.7283464566929126471, 0.1660481256975883668, -0.3530559997133364547 ) ) ;
#48221=CARTESIAN_POINT ( 'NONE',  ( -1.594488188976377119, 0.1660481256975883668, -0.3530559997133364547 ) ) ;
#48223=CARTESIAN_POINT ( 'NONE',  ( 0.09842519685039434474, -0.5400638737290845981, -0.3530559997133363437 ) ) ;
#48225=CARTESIAN_POINT ( 'NONE',  ( -1.240157480314959759, -0.4536011799217368745, -0.2665933059059886201 ) ) ;
#48230=CARTESIAN_POINT ( 'NONE',  ( -1.377952755905511140, 0.2952755905511811885, 0.000000000000000000 ) ) ;
#48233=CARTESIAN_POINT ( 'NONE',  ( -1.574803149606298636, -0.1870078740157479769, 0.4822834645669291653 ) ) ;
#48234=FACE_OUTER_BOUND ( 'NONE', #40346, .T. ) ;
#48237=CARTESIAN_POINT ( 'NONE',  ( -0.2034120734908128059, 0.1771653543307087630, 0.09757992244046791164 ) ) ;
#48238=CARTESIAN_POINT ( 'NONE',  ( -0.6758530183727028406, -0.5511811023622048555, -0.09757992244046775898 ) ) ;
#48239=CARTESIAN_POINT ( 'NONE',  ( -1.397637795275589623, -0.5400638737290845981, -0.3530559997133363437 ) ) ;
#48240=CARTESIAN_POINT ( 'NONE',  ( 0.5839895013123367340, -0.6692913385826773087, -0.1292274648535924053 ) ) ;
#48241=CARTESIAN_POINT ( 'NONE',  ( -1.450131233595799651, 0.2952755905511810774, -0.1292274648535930714 ) ) ;
#48244=CARTESIAN_POINT ( 'NONE',  ( -1.364829396325458521, -0.6046776061558807314, 0.2411417322834647770 ) ) ;
#48245=CYLINDRICAL_SURFACE ( 'NONE', #82377, 3.543307086614173151 ) ;
#48249=CARTESIAN_POINT ( 'NONE',  ( 0.4768139191967274981, 1.559564387633094018, -0.5050868514466849701 ) ) ;
#48250=CARTESIAN_POINT ( 'NONE',  ( -0.8858267716535425107, -0.5400638737290844871, 0.3530559997133364547 ) ) ;
#48251=CARTESIAN_POINT ( 'NONE',  ( 1.450131233595801428, -0.6692913385826773087, -0.1292274648535924053 ) ) ;
#48252=DIRECTION ( 'NONE',  ( 0.000000000000000000, -1.000000000000000000, -0.000000000000000000 ) ) ;
#48254=CARTESIAN_POINT ( 'NONE',  ( -1.312335958005248715, -0.6046776061558809534, -0.2411417322834644161 ) ) ;
#48255=CARTESIAN_POINT ( 'NONE',  ( -0.7742782152230965886, 0.05413385826771666132, 0.4176697321401328100 ) ) ;
#48257=CARTESIAN_POINT ( 'NONE',  ( -0.1640419947506555343, -0.2845877964562159024, 0.3641732283464567677 ) ) ;
#48259=CARTESIAN_POINT ( 'NONE',  ( -0.2690288713910754526, -0.5511811023622046335, 0.09757992244046803654 ) ) ;
#48260=CARTESIAN_POINT ( 'NONE',  ( 1.017060367454068581, -0.08942795157528024563, -0.3641732283464568787 ) ) ;
#48261=CARTESIAN_POINT ( 'NONE',  ( 0.8398950131233602345, 0.2306618581243847221, -0.2411417322834647770 ) ) ;
#48262=CARTESIAN_POINT ( 'NONE',  ( -0.3018372703412066094, -0.3690944881889765550, -0.3153832671262227771 ) ) ;
#48264=CARTESIAN_POINT ( 'NONE',  ( -1.496062992125983815, -0.1870078740157479769, 0.4822834645669291653 ) ) ;
#48265=CARTESIAN_POINT ( 'NONE',  ( -1.286089238845143479, 0.1283753931104746893, -0.1820866141732285504 ) ) ;
#48267=CARTESIAN_POINT ( 'NONE',  ( 0.2165354330708668673, 0.1660481256975883668, -0.3530559997133364547 ) ) ;
#48268=CARTESIAN_POINT ( 'NONE',  ( -0.2887139107611542133, -0.6046776061558809534, -0.2411417322834644161 ) ) ;
#48269=CARTESIAN_POINT ( 'NONE',  ( 1.568241469816273659, -0.08942795157528024563, -0.3641732283464568787 ) ) ;
#48270=CARTESIAN_POINT ( 'NONE',  ( 0.6955380577427828781, -0.004921259842519870586, -0.3153832671262229437 ) ) ;
#48271=CARTESIAN_POINT ( 'NONE',  ( -0.1509186351706028884, -0.08942795157527998196, 0.3641732283464567121 ) ) ;
#48272=CARTESIAN_POINT ( 'NONE',  ( -0.6167979002624665030, -0.4281496062992127816, -0.4176697321401328100 ) ) ;
#48275=CARTESIAN_POINT ( 'NONE',  ( 8.195543980992789655E-16, -0.1870078740157480879, -0.4822834645669291653 ) ) ;
#48277=CARTESIAN_POINT ( 'NONE',  ( 1.502624671916010790, -0.3162353388693409650, -0.4822834645669289433 ) ) ;
#48278=CARTESIAN_POINT ( 'NONE',  ( -0.1115485564304456306, 0.1771653543307087075, -0.09757992244046823083 ) ) ;
#48279=CARTESIAN_POINT ( 'NONE',  ( -0.07874015748031421014, -0.1870078740157480879, -0.4822834645669291653 ) ) ;
#48280=CARTESIAN_POINT ( 'NONE',  ( -1.469816272965878357, 0.2306618581243848609, 0.2411417322834645549 ) ) ;
#48281=CARTESIAN_POINT ( 'NONE',  ( -1.456692913385826182, 0.1771653543307087630, 0.000000000000000000 ) ) ;
#48282=CARTESIAN_POINT ( 'NONE',  ( 1.430446194225722500, -0.4281496062992127816, -0.4176697321401328100 ) ) ;
#48284=CARTESIAN_POINT ( 'NONE',  ( -1.515748031496062076, -0.5400638737290844871, 0.3530559997133364547 ) ) ;
#48285=CARTESIAN_POINT ( 'NONE',  ( -0.6561679790026240244, -0.5023911411419708095, 0.1820866141732285504 ) ) ;
#48290=CARTESIAN_POINT ( 'NONE',  ( 1.496062992125985147, -0.1870078740157479769, 0.3641732283464567677 ) ) ;
#48291=CARTESIAN_POINT ( 'NONE',  ( 1.076115485564305141, -0.5023911411419708095, 0.1820866141732285504 ) ) ;
#48292=CARTESIAN_POINT ( 'NONE',  ( -1.587926509186350810, -0.4281496062992124485, 0.4176697321401328655 ) ) ;
#48293=CARTESIAN_POINT ( 'NONE',  ( 0.8595800524934390507, -0.05778040916215560624, -0.4822834645669293319 ) ) ;
#48295=CARTESIAN_POINT ( 'NONE',  ( 1.036745406824147731, -0.004921259842519576551, 0.3153832671262227771 ) ) ;
#48296=CARTESIAN_POINT ( 'NONE',  ( -0.006561679790025524116, -0.05778040916215560624, -0.4822834645669293319 ) ) ;
#48297=CARTESIAN_POINT ( 'NONE',  ( -1.010498687664041384, 0.05413385826771666132, 0.4176697321401328100 ) ) ;
#48301=CARTESIAN_POINT ( 'NONE',  ( 0.3280839895013130669, -0.004921259842519576551, 0.3153832671262227771 ) ) ;
#48305=CARTESIAN_POINT ( 'NONE',  ( -0.3543307086614165824, -0.6692913385826771977, 8.415575281601705876E-17 ) ) ;
#48306=CARTESIAN_POINT ( 'NONE',  ( -0.1640419947506553400, -0.05778040916215560624, -0.4822834645669293319 ) ) ;
#48307=CARTESIAN_POINT ( 'NONE',  ( -0.3280839895013117347, -0.004921259842519870586, -0.3153832671262229437 ) ) ;
#48308=CARTESIAN_POINT ( 'NONE',  ( 0.8070866141732289112, -0.5400638737290845981, -0.3530559997133363437 ) ) ;
#48309=CARTESIAN_POINT ( 'NONE',  ( -0.8530183727034112984, 0.05413385826771666132, 0.4176697321401328100 ) ) ;
#48310=CARTESIAN_POINT ( 'NONE',  ( -0.3871391076115479057, -0.3162353388693409650, -0.4822834645669289433 ) ) ;
#48311=CARTESIAN_POINT ( 'NONE',  ( 1.082677165354331228, -0.5400638737290844871, 0.3530559997133364547 ) ) ;
#48312=CARTESIAN_POINT ( 'NONE',  ( 0.9383202099737536495, -0.3162353388693405765, 0.4822834645669290543 ) ) ;
#48313=CARTESIAN_POINT ( 'NONE',  ( 0.6955380577427828781, -0.4281496062992124485, 0.4176697321401328655 ) ) ;
#48315=CARTESIAN_POINT ( 'NONE',  ( -0.1837270341207340729, 0.1283753931104746893, -0.1820866141732285504 ) ) ;
#48316=ORIENTED_EDGE ( 'NONE', *, *, #405, .T. ) ;
#48319=CARTESIAN_POINT ( 'NONE',  ( -0.7480314960629914633, 0.1771653543307087630, 0.000000000000000000 ) ) ;
#48320=CARTESIAN_POINT ( 'NONE',  ( -0.6627296587926501115, 0.2952755905511810774, -0.1292274648535930714 ) ) ;
#48322=CARTESIAN_POINT ( 'NONE',  ( -0.5380577427821514602, -0.4281496062992127816, -0.4176697321401328100 ) ) ;
#48323=CARTESIAN_POINT ( 'NONE',  ( -0.2099737532808391705, -0.6046776061558809534, -0.2411417322834644161 ) ) ;
#48324=CARTESIAN_POINT ( 'NONE',  ( -1.253280839895012377, -0.3162353388693409650, -0.4822834645669289433 ) ) ;
#48325=CARTESIAN_POINT ( 'NONE',  ( -1.397637795275589623, 0.1660481256975885056, 0.3530559997133364547 ) ) ;
#48326=CARTESIAN_POINT ( 'NONE',  ( 0.9448818897637802916, -0.1870078740157480601, -0.3641732283464567677 ) ) ;
#48327=CARTESIAN_POINT ( 'NONE',  ( -1.646051170424378096, 0.8346805926620876059, 0.5309055118110233007 ) ) ;
#48329=CARTESIAN_POINT ( 'NONE',  ( 0.5511811023622054106, -0.1870078740157480601, -0.3641732283464567677 ) ) ;
#48330=CARTESIAN_POINT ( 'NONE',  ( 0.08530183727034192087, -0.05778040916215522460, 0.4822834645669289988 ) ) ;
#48331=CARTESIAN_POINT ( 'NONE',  ( 0.2952755905511819101, 0.1660481256975883668, -0.3530559997133364547 ) ) ;
#48332=ORIENTED_EDGE ( 'NONE', *, *, #15774, .T. ) ;
#48334=CARTESIAN_POINT ( 'NONE',  ( -0.6986524979670485358, -2.191421614605370878E-15, 0.4445507791589071167 ) ) ;
#48335=EDGE_LOOP ( 'NONE', ( #37283, #70255, #20169, #15952 ) ) ;
#48337=CARTESIAN_POINT ( 'NONE',  ( 1.568241469816273437, -0.3162353388693405765, 0.4822834645669290543 ) ) ;
#48338=CARTESIAN_POINT ( 'NONE',  ( -0.5446194225721777693, -0.2845877964562161244, -0.3641732283464567121 ) ) ;
#48339=CARTESIAN_POINT ( 'NONE',  ( -1.148293963254592542, -0.6692913385826773087, -0.1292274648535924053 ) ) ;
#48342=CARTESIAN_POINT ( 'NONE',  ( -1.509186351706035767, -0.3690944881889763329, 0.3153832671262228327 ) ) ;
#48343=CARTESIAN_POINT ( 'NONE',  ( 0.3937007874015754361, -0.1870078740157480879, -0.4822834645669291653 ) ) ;
#48344=CARTESIAN_POINT ( 'NONE',  ( 0.6889763779527566800, -0.5400638737290844871, 0.3530559997133364547 ) ) ;
#48345=CARTESIAN_POINT ( 'NONE',  ( -0.6692913385826764205, 0.1771653543307087630, 0.000000000000000000 ) ) ;
#48346=CARTESIAN_POINT ( 'NONE',  ( -0.01312335958005186876, -0.4281496062992124485, 0.4176697321401328655 ) ) ;
#48348=CARTESIAN_POINT ( 'NONE',  ( -0.3018372703412066094, -0.3690944881889765550, -0.3153832671262227771 ) ) ;
#48349=CARTESIAN_POINT ( 'NONE',  ( -0.4265091863517051496, 0.2952755905511810774, -0.1292274648535930714 ) ) ;
#48351=CARTESIAN_POINT ( 'NONE',  ( 1.614173228346457378, 0.1771653543307087630, 0.000000000000000000 ) ) ;
#48352=CARTESIAN_POINT ( 'NONE',  ( -0.08530183727034056085, -0.08942795157528024563, -0.3641732283464568787 ) ) ;
#48353=CARTESIAN_POINT ( 'NONE',  ( 1.266404199475066328, -0.2845877964562161244, -0.3641732283464567121 ) ) ;
#48354=CARTESIAN_POINT ( 'NONE',  ( -1.299212598425196097, -0.6692913385826771977, 8.415575281601705876E-17 ) ) ;
#48355=CARTESIAN_POINT ( 'NONE',  ( -0.6102362204724400829, -0.4536011799217368745, -0.2665933059059886201 ) ) ;
#48357=CARTESIAN_POINT ( 'NONE',  ( -1.233595800524933894, 0.2306618581243848609, 0.2411417322834645549 ) ) ;
#48358=CARTESIAN_POINT ( 'NONE',  ( -0.4396325459317577122, -0.6692913385826773087, -0.1292274648535924053 ) ) ;
#48359=CARTESIAN_POINT ( 'NONE',  ( 0.4855643044619430415, -0.4281496062992127816, -0.4176697321401328100 ) ) ;
#48362=CARTESIAN_POINT ( 'NONE',  ( 0.2493438320209980519, -0.004921259842519576551, 0.3153832671262227771 ) ) ;
#48363=CARTESIAN_POINT ( 'NONE',  ( 0.9251968503937015864, -0.5400638737290844871, 0.3530559997133364547 ) ) ;
#48364=CARTESIAN_POINT ( 'NONE',  ( -1.227034120734907585, 0.1771653543307087630, 0.09757992244046791164 ) ) ;
#48365=CARTESIAN_POINT ( 'NONE',  ( 1.246719160104987623, 0.05413385826771626580, -0.4176697321401330321 ) ) ;
#48366=CARTESIAN_POINT ( 'NONE',  ( -1.443569553805773564, -0.5023911411419708095, 0.1820866141732285504 ) ) ;
#48367=CARTESIAN_POINT ( 'NONE',  ( -1.456692913385826182, -0.6692913385826771977, 8.415575281601705876E-17 ) ) ;
#48368=CARTESIAN_POINT ( 'NONE',  ( -0.9317585301837263412, 0.05413385826771666132, 0.4176697321401328100 ) ) ;
#48369=CARTESIAN_POINT ( 'NONE',  ( 0.1049868766404206816, 0.1283753931104748280, 0.1820866141732283561 ) ) ;
#48371=CARTESIAN_POINT ( 'NONE',  ( 0.7217847769028878924, -0.3690944881889765550, -0.3153832671262227771 ) ) ;
#48372=CARTESIAN_POINT ( 'NONE',  ( -0.1771653543307080136, 0.1660481256975883668, -0.3530559997133364547 ) ) ;
#48375=CARTESIAN_POINT ( 'NONE',  ( -0.9908136482939626788, -0.6692913385826773087, -0.1292274648535924053 ) ) ;
#48377=CARTESIAN_POINT ( 'NONE',  ( 1.240157480314961314, -0.4536011799217367080, 0.2665933059059888421 ) ) ;
#48378=CARTESIAN_POINT ( 'NONE',  ( 0.05905511811023709395, -0.5400638737290844871, 0.3530559997133364547 ) ) ;
#48379=CARTESIAN_POINT ( 'NONE',  ( -0.1771653543307080136, 0.1660481256975883668, -0.3530559997133364547 ) ) ;
#48380=CARTESIAN_POINT ( 'NONE',  ( -0.4724409448818890911, -0.1870078740157480601, -0.3641732283464567677 ) ) ;
#48381=CARTESIAN_POINT ( 'NONE',  ( 1.220472440944882386, 0.2952755905511811885, 0.000000000000000000 ) ) ;
#48382=CARTESIAN_POINT ( 'NONE',  ( -0.6692913385826764205, 0.1771653543307087630, 0.000000000000000000 ) ) ;
#48383=CARTESIAN_POINT ( 'NONE',  ( 0.5708661417322842269, 0.1660481256975885056, 0.3530559997133364547 ) ) ;
#48384=CARTESIAN_POINT ( 'NONE',  ( -1.194225721784776262, -0.004921259842519870586, -0.3153832671262229437 ) ) ;
#48386=CARTESIAN_POINT ( 'NONE',  ( -1.108923884514435132, -0.05778040916215560624, -0.4822834645669293319 ) ) ;
#48389=CARTESIAN_POINT ( 'NONE',  ( -1.528871391076114250, 0.1771653543307087075, -0.09757992244046823083 ) ) ;
#48390=CARTESIAN_POINT ( 'NONE',  ( -0.3412073490813641308, -0.6046776061558807314, 0.2411417322834647770 ) ) ;
#48392=CARTESIAN_POINT ( 'NONE',  ( -1.115485564304461219, 0.05413385826771626580, -0.4176697321401330321 ) ) ;
#48395=CARTESIAN_POINT ( 'NONE',  ( 1.299212598425197429, -0.6692913385826771977, 8.415575281601705876E-17 ) ) ;
#48396=CARTESIAN_POINT ( 'NONE',  ( 0.3805774278215230400, -0.4281496062992124485, 0.4176697321401328655 ) ) ;
#48399=CARTESIAN_POINT ( 'NONE',  ( -1.568241469816272105, -0.05778040916215522460, 0.4822834645669289988 ) ) ;
#48402=CARTESIAN_POINT ( 'NONE',  ( -1.056430446194224881, -0.5511811023622046335, 0.09757992244046803654 ) ) ;
#48405=CARTESIAN_POINT ( 'NONE',  ( 0.6233595800524939223, -0.3162353388693405765, 0.4822834645669290543 ) ) ;
#48406=CARTESIAN_POINT ( 'NONE',  ( -0.2624671916010490880, 0.2306618581243847221, -0.2411417322834647770 ) ) ;
#48407=CARTESIAN_POINT ( 'NONE',  ( -1.233595800524933894, -0.6046776061558809534, -0.2411417322834644161 ) ) ;
#48408=CARTESIAN_POINT ( 'NONE',  ( 1.213910761154856299, 0.2952755905511811885, 0.1292274648535926551 ) ) ;
#48409=CARTESIAN_POINT ( 'NONE',  ( -1.095800524934382292, -0.2845877964562161244, -0.3641732283464567121 ) ) ;
#48411=CARTESIAN_POINT ( 'NONE',  ( 0.3346456692913393205, -0.5400638737290845981, -0.3530559997133363437 ) ) ;
#48412=CARTESIAN_POINT ( 'NONE',  ( -0.7349081364829387342, -0.6046776061558807314, 0.2411417322834647770 ) ) ;
#48414=CARTESIAN_POINT ( 'NONE',  ( -1.423884514435694859, -0.05778040916215560624, -0.4822834645669293319 ) ) ;
#48417=( BOUNDED_CURVE ( )  B_SPLINE_CURVE ( 2, ( #1800, #32109, #25784, #77994, #19481, #27045, #13187, #14022, #554, #46814, #78416, #45975, #8119 ),
 .UNSPECIFIED., .F., .F. ) 
 B_SPLINE_CURVE_WITH_KNOTS ( ( 3, 2, 2, 2, 2, 2, 3 ),
 ( 0.2649423569342326812, 0.2651515151515151381, 0.2689393939393939226, 0.2727272727272727071, 0.2765151515151514916, 0.2803030303030302761, 0.2805121885203127330 ),
 .UNSPECIFIED. ) 
 CURVE ( )  GEOMETRIC_REPRESENTATION_ITEM ( )  RATIONAL_B_SPLINE_CURVE ( ( 0.9964447847208428577, 0.9981185001348096275, 1.000000000000000000, 0.9659258262890683122, 1.000000000000000000, 0.9659258262890683122, 1.000000000000000000, 0.9659258262890683122, 1.000000000000000000, 0.9659258262890683122, 1.000000000000000000, 0.9981185001348097385, 0.9964447847208430797 ) ) 
 REPRESENTATION_ITEM ( '' )  );
#48418=CARTESIAN_POINT ( 'NONE',  ( 0.7939632545931766261, -0.3162353388693409650, -0.4822834645669289433 ) ) ;
#48419=CARTESIAN_POINT ( 'NONE',  ( 1.089238845144357759, -0.004921259842519870586, -0.3153832671262229437 ) ) ;
#48420=ORIENTED_EDGE ( 'NONE', *, *, #39780, .T. ) ;
#48422=CARTESIAN_POINT ( 'NONE',  ( -0.5446194225721777693, -0.05778040916215522460, 0.4822834645669289988 ) ) ;
#48424=CARTESIAN_POINT ( 'NONE',  ( 0.4461942257217855201, -0.5023911411419708095, 0.1820866141732285504 ) ) ;
#48425=CARTESIAN_POINT ( 'NONE',  ( -1.528871391076114250, 0.2952755905511810774, -0.1292274648535930714 ) ) ;
#48426=CARTESIAN_POINT ( 'NONE',  ( 0.9580052493438326877, 0.05413385826771666132, 0.4176697321401328100 ) ) ;
#48427=CARTESIAN_POINT ( 'NONE',  ( 0.9514435695538062676, -0.05778040916215522460, 0.4822834645669289988 ) ) ;
#48428=CARTESIAN_POINT ( 'NONE',  ( -0.3674540682414692561, -0.6046776061558809534, -0.2411417322834644161 ) ) ;
#48431=CARTESIAN_POINT ( 'NONE',  ( -0.6758530183727028406, 0.2952755905511811885, 0.1292274648535926551 ) ) ;
#48433=CARTESIAN_POINT ( 'NONE',  ( -1.410761154855642463, -0.05778040916215522460, 0.4822834645669289988 ) ) ;
#48434=CARTESIAN_POINT ( 'NONE',  ( -0.9580052493438311334, 0.05413385826771626580, -0.4176697321401330321 ) ) ;
#48435=CARTESIAN_POINT ( 'NONE',  ( 1.187664041994751285, -0.05778040916215522460, 0.4822834645669289988 ) ) ;
#48436=CARTESIAN_POINT ( 'NONE',  ( 1.653543307086614789, -0.1870078740157479769, 0.4822834645669291653 ) ) ;
#48437=CARTESIAN_POINT ( 'NONE',  ( -0.7611548556430438595, 0.2306618581243848609, 0.2411417322834645549 ) ) ;
#48439=CARTESIAN_POINT ( 'NONE',  ( 0.1640419947506569498, -0.05778040916215522460, 0.4822834645669289988 ) ) ;
#48441=CARTESIAN_POINT ( 'NONE',  ( -0.3477690288713902178, 0.2952755905511810774, -0.1292274648535930714 ) ) ;
#48442=CARTESIAN_POINT ( 'NONE',  ( -1.443569553805773564, 0.1283753931104746893, -0.1820866141732285504 ) ) ;
#48443=CARTESIAN_POINT ( 'NONE',  ( 0.4199475065616805614, 0.1283753931104748280, 0.1820866141732283561 ) ) ;
#48444=CARTESIAN_POINT ( 'NONE',  ( 1.305774278215223960, 0.2952755905511810774, -0.1292274648535930714 ) ) ;
#48446=CARTESIAN_POINT ( 'NONE',  ( 1.358267716535433323, 0.07958543189024085140, 0.2665933059059887866 ) ) ;
#48447=CARTESIAN_POINT ( 'NONE',  ( 0.8005249343832027131, 0.05413385826771666132, 0.4176697321401328100 ) ) ;
#48449=CARTESIAN_POINT ( 'NONE',  ( -0.5577427821522301654, -0.05778040916215560624, -0.4822834645669293319 ) ) ;
#48451=CARTESIAN_POINT ( 'NONE',  ( 1.469816272965879911, 0.1283753931104746893, -0.1820866141732285504 ) ) ;
#48452=CARTESIAN_POINT ( 'NONE',  ( -0.6824146981627291497, -0.6046776061558809534, -0.2411417322834644161 ) ) ;
#48454=CARTESIAN_POINT ( 'NONE',  ( 1.450131233595801428, -0.6692913385826773087, -0.1292274648535924053 ) ) ;
#48455=CARTESIAN_POINT ( 'NONE',  ( 0.05905511811023681640, 0.1660481256975883668, -0.3530559997133364547 ) ) ;
#48456=CARTESIAN_POINT ( 'NONE',  ( 0.3674540682414705883, -0.5023911411419708095, 0.1820866141732285504 ) ) ;
#48458=CARTESIAN_POINT ( 'NONE',  ( -0.1246719160104980823, -0.5511811023622048555, -0.09757992244046775898 ) ) ;
#48459=CARTESIAN_POINT ( 'NONE',  ( 0.7874015748031503170, -0.1870078740157479769, 0.3641732283464567677 ) ) ;
#48460=CARTESIAN_POINT ( 'NONE',  ( -1.496062992125983815, -0.1870078740157479769, 0.4822834645669291653 ) ) ;
#48462=CARTESIAN_POINT ( 'NONE',  ( 0.8530183727034128527, -0.4281496062992124485, 0.4176697321401328655 ) ) ;
#48464=CARTESIAN_POINT ( 'NONE',  ( 1.587926509186352586, -0.3690944881889765550, -0.3153832671262227771 ) ) ;
#48466=CARTESIAN_POINT ( 'NONE',  ( -0.1771653543307080136, -0.4536011799217367080, 0.2665933059059888421 ) ) ;
#48467=CARTESIAN_POINT ( 'NONE',  ( 0.1377952755905518800, 0.1660481256975883668, -0.3530559997133364547 ) ) ;
#48468=CARTESIAN_POINT ( 'NONE',  ( 1.345144356955381593, -0.08942795157527998196, 0.3641732283464567121 ) ) ;
#48469=CARTESIAN_POINT ( 'NONE',  ( -1.259842519685038686, -0.1870078740157479769, 0.3641732283464567677 ) ) ;
#48470=CARTESIAN_POINT ( 'NONE',  ( -1.456692913385826182, -0.6692913385826771977, 8.415575281601705876E-17 ) ) ;
#48471=CARTESIAN_POINT ( 'NONE',  ( 0.4986876640419954376, -0.6046776061558809534, -0.2411417322834644161 ) ) ;
#48472=CARTESIAN_POINT ( 'NONE',  ( 1.030183727034121421, -0.05778040916215522460, 0.4822834645669289988 ) ) ;
#48474=CARTESIAN_POINT ( 'NONE',  ( 0.3215223097112867578, -0.05778040916215522460, 0.4822834645669289988 ) ) ;
#48475=CARTESIAN_POINT ( 'NONE',  ( 1.122047244094488860, -0.5400638737290845981, -0.3530559997133363437 ) ) ;
#48476=B_SPLINE_CURVE_WITH_KNOTS ( 'NONE', 3,
 ( #2387, #66783, #59610, #1965 ),
 .UNSPECIFIED., .F., .F.,
 ( 4, 4 ),
 ( 3.210432057656183116E-07, 0.001287787053612127848 ),
 .UNSPECIFIED. ) ;
#48477=CARTESIAN_POINT ( 'NONE',  ( 1.135170603674541256, -0.6692913385826773087, -0.1292274648535924053 ) ) ;
#48479=CARTESIAN_POINT ( 'NONE',  ( 0.7414698162729663755, 0.1771653543307087630, 0.09757992244046791164 ) ) ;
#48480=CARTESIAN_POINT ( 'NONE',  ( -1.581364829396324945, -0.08942795157528024563, -0.3641732283464568787 ) ) ;
#48481=CARTESIAN_POINT ( 'NONE',  ( 0.04593175853018440641, 0.1771653543307087075, -0.09757992244046823083 ) ) ;
#48482=CARTESIAN_POINT ( 'NONE',  ( 0.3083989501312343062, -0.05778040916215560624, -0.4822834645669293319 ) ) ;
#48483=CARTESIAN_POINT ( 'NONE',  ( 0.7152230971128614723, -0.3162353388693409650, -0.4822834645669289433 ) ) ;
#48484=CARTESIAN_POINT ( 'NONE',  ( -0.4068241469816264999, -0.4281496062992124485, 0.4176697321401328655 ) ) ;
#48485=CARTESIAN_POINT ( 'NONE',  ( -0.3149606299212590610, -0.1870078740157479769, 0.3641732283464567677 ) ) ;
#48487=CARTESIAN_POINT ( 'NONE',  ( 0.6692913385826777528, 0.2952755905511811885, 0.000000000000000000 ) ) ;
#48488=CARTESIAN_POINT ( 'NONE',  ( 0.7742782152230979209, -0.004921259842519870586, -0.3153832671262229437 ) ) ;
#48493=CARTESIAN_POINT ( 'NONE',  ( -1.213910761154854745, -0.6692913385826771977, 0.1292274648535927661 ) ) ;
#48494=CARTESIAN_POINT ( 'NONE',  ( -0.2821522309711278487, 0.2952755905511811885, 0.1292274648535926551 ) ) ;
#48498=CARTESIAN_POINT ( 'NONE',  ( 0.5971128608923891301, 0.1771653543307087075, -0.09757992244046823083 ) ) ;
#48500=CARTESIAN_POINT ( 'NONE',  ( 1.076115485564305141, -0.6046776061558807314, 0.2411417322834647770 ) ) ;
#48503=CARTESIAN_POINT ( 'NONE',  ( -1.338582677165353729, -0.1870078740157480601, -0.3641732283464567677 ) ) ;
#48504=CONICAL_SURFACE ( 'NONE', #41778, 2.401574803149606918, 0.6981317007977250189 ) ;
#48505=CARTESIAN_POINT ( 'NONE',  ( 1.568241469816273659, -0.05778040916215560624, -0.4822834645669293319 ) ) ;
#48507=CARTESIAN_POINT ( 'NONE',  ( 1.227034120734908917, -0.5511811023622046335, 0.09757992244046803654 ) ) ;
#48508=CARTESIAN_POINT ( 'NONE',  ( 0.5774278215223104249, 0.2306618581243848609, 0.2411417322834645549 ) ) ;
#48510=CARTESIAN_POINT ( 'NONE',  ( -0.1902887139107604098, 0.2952755905511810774, -0.1292274648535930714 ) ) ;
#48511=CARTESIAN_POINT ( 'NONE',  ( -0.9120734908136475250, 0.1771653543307087630, 0.09757992244046791164 ) ) ;
#48512=CARTESIAN_POINT ( 'NONE',  ( 0.3477690288713918276, 0.2952755905511811885, 0.1292274648535926551 ) ) ;
#48513=CARTESIAN_POINT ( 'NONE',  ( -0.1312335958005241554, 0.2306618581243848609, 0.2411417322834645549 ) ) ;
#48518=CARTESIAN_POINT ( 'NONE',  ( 0.7283464566929143125, 0.1660481256975885056, 0.3530559997133364547 ) ) ;
#48519=CARTESIAN_POINT ( 'NONE',  ( -0.006561679790025524116, -0.3162353388693405765, 0.4822834645669290543 ) ) ;
#48520=CARTESIAN_POINT ( 'NONE',  ( -1.030183727034119867, -0.3162353388693405765, 0.4822834645669290543 ) ) ;
#48521=CARTESIAN_POINT ( 'NONE',  ( 0.9448818897637802916, -0.1870078740157479769, 0.4822834645669291653 ) ) ;
#48522=CARTESIAN_POINT ( 'NONE',  ( 0.4330708661417329575, 0.2952755905511811885, 0.000000000000000000 ) ) ;
#48524=CARTESIAN_POINT ( 'NONE',  ( -0.5183727034120726440, -0.6692913385826773087, -0.1292274648535924053 ) ) ;
#48525=CARTESIAN_POINT ( 'NONE',  ( 0.1443569553805781891, 0.05413385826771626580, -0.4176697321401330321 ) ) ;
#48526=CARTESIAN_POINT ( 'NONE',  ( -0.6496062992125976043, 0.1660481256975883668, -0.3530559997133364547 ) ) ;
#48527=CARTESIAN_POINT ( 'NONE',  ( 0.5774278215223104249, 0.1283753931104748280, 0.1820866141732283561 ) ) ;
#48528=DIRECTION ( 'NONE',  ( -0.000000000000000000, 1.000000000000000000, -0.000000000000000000 ) ) ;
#48530=CARTESIAN_POINT ( 'NONE',  ( 0.3871391076115492380, -0.05778040916215560624, -0.4822834645669293319 ) ) ;
#48533=ORIENTED_EDGE ( 'NONE', *, *, #27901, .T. ) ;
#48534=EDGE_CURVE ( 'NONE', #1757, #75163, #10819, .T. ) ;
#48535=ORIENTED_EDGE ( 'NONE', *, *, #24322, .F. ) ;
#48536=CARTESIAN_POINT ( 'NONE',  ( 0.6299212598425204535, -0.1870078740157480879, -0.4822834645669291653 ) ) ;
#48537=CARTESIAN_POINT ( 'NONE',  ( 0.6955380577427828781, -0.004921259842519870586, -0.3153832671262229437 ) ) ;
#48547=CARTESIAN_POINT ( 'NONE',  ( 0.8595800524934390507, -0.05778040916215560624, -0.4822834645669293319 ) ) ;
#48548=CARTESIAN_POINT ( 'NONE',  ( -0.6758530183727028406, 0.2952755905511811885, 0.1292274648535926551 ) ) ;
#48549=CARTESIAN_POINT ( 'NONE',  ( -0.5839895013123351797, 0.2952755905511810774, -0.1292274648535930714 ) ) ;
#48550=CARTESIAN_POINT ( 'NONE',  ( 0.5314960629921264834, 0.1660481256975883668, -0.3530559997133364547 ) ) ;
#48552=CARTESIAN_POINT ( 'NONE',  ( 1.515748031496063186, -0.5400638737290845981, -0.3530559997133363437 ) ) ;
#48553=CARTESIAN_POINT ( 'NONE',  ( 1.220472440944882164, 0.2066929133858268208, 4.479895975645240118E-15 ) ) ;
#48555=CARTESIAN_POINT ( 'NONE',  ( 1.122047244094488860, -0.4536011799217368745, -0.2665933059059886201 ) ) ;
#48557=CARTESIAN_POINT ( 'NONE',  ( -1.128608923884513837, 0.1283753931104746893, -0.1820866141732285504 ) ) ;
#48559=CARTESIAN_POINT ( 'NONE',  ( -0.006561679790025524116, -0.05778040916215560624, -0.4822834645669293319 ) ) ;
#48562=CARTESIAN_POINT ( 'NONE',  ( -1.272965879265091305, -0.3690944881889763329, 0.3153832671262228327 ) ) ;
#48563=CARTESIAN_POINT ( 'NONE',  ( 0.3740157480314966754, -0.5400638737290844871, 0.3530559997133364547 ) ) ;
#48564=CARTESIAN_POINT ( 'NONE',  ( 1.135170603674541256, 0.1771653543307087630, 0.09757992244046791164 ) ) ;
#48566=CARTESIAN_POINT ( 'NONE',  ( -1.082677165354329896, 0.07958543189024085140, 0.2665933059059887866 ) ) ;
#48567=CARTESIAN_POINT ( 'NONE',  ( 1.305774278215223960, -0.6692913385826771977, 0.1292274648535927661 ) ) ;
#48569=CARTESIAN_POINT ( 'NONE',  ( -0.2559055118110230564, 0.1660481256975883668, -0.3530559997133364547 ) ) ;
#48570=CARTESIAN_POINT ( 'NONE',  ( -1.272965879265091305, -0.004921259842519870586, -0.3153832671262229437 ) ) ;
#48572=CARTESIAN_POINT ( 'NONE',  ( -0.5249343832020990641, -0.6046776061558809534, -0.2411417322834644161 ) ) ;
#48573=CARTESIAN_POINT ( 'NONE',  ( -1.456692913385826182, 0.1771653543307087630, 0.000000000000000000 ) ) ;
#48575=CARTESIAN_POINT ( 'NONE',  ( 0.3805774278215230400, 0.05413385826771626580, -0.4176697321401330321 ) ) ;
#48576=DIRECTION ( 'NONE',  ( -3.096699300667737957E-16, 1.000000000000000000, -0.000000000000000000 ) ) ;
#48577=CARTESIAN_POINT ( 'NONE',  ( 1.286089238845145033, 0.2306618581243848609, 0.2411417322834645549 ) ) ;
#48579=CARTESIAN_POINT ( 'NONE',  ( -1.135170603674539924, -0.6692913385826771977, 0.1292274648535927661 ) ) ;
#48580=CARTESIAN_POINT ( 'NONE',  ( -0.4002624671916004129, -0.08942795157528024563, -0.3641732283464568787 ) ) ;
#48581=CARTESIAN_POINT ( 'NONE',  ( -0.5052493438320202479, 0.2066929133858267098, -0.1054918080437494132 ) ) ;
#48582=CARTESIAN_POINT ( 'NONE',  ( -0.1706036745406816491, 0.05413385826771626580, -0.4176697321401330321 ) ) ;
#48583=CARTESIAN_POINT ( 'NONE',  ( 0.2493438320209980519, -0.004921259842519576551, 0.3153832671262227771 ) ) ;
#48584=CARTESIAN_POINT ( 'NONE',  ( -1.076115485564303809, 0.1283753931104748280, 0.1820866141732283561 ) ) ;
#48585=CARTESIAN_POINT ( 'NONE',  ( -1.410761154855642463, -0.05778040916215522460, 0.4822834645669289988 ) ) ;
#48586=CARTESIAN_POINT ( 'NONE',  ( -1.456692913385826182, -0.6692913385826771977, 8.415575281601705876E-17 ) ) ;
#48587=CARTESIAN_POINT ( 'NONE',  ( 1.292650918635171564, -0.6692913385826773087, -0.1292274648535924053 ) ) ;
#48589=CARTESIAN_POINT ( 'NONE',  ( 0.3412073490813655186, -0.5023911411419708095, -0.1820866141732282451 ) ) ;
#48590=CARTESIAN_POINT ( 'NONE',  ( 1.023622047244095334, -0.1870078740157479769, 0.4822834645669291653 ) ) ;
#48592=CARTESIAN_POINT ( 'NONE',  ( 1.430446194225722500, -0.004921259842519576551, 0.3153832671262227771 ) ) ;
#48594=CARTESIAN_POINT ( 'NONE',  ( -1.167979002624671470, 0.05413385826771666132, 0.4176697321401328100 ) ) ;
#48596=CARTESIAN_POINT ( 'NONE',  ( -0.7808398950131222316, -0.3162353388693409650, -0.4822834645669289433 ) ) ;
#48597=CARTESIAN_POINT ( 'NONE',  ( 0.2559055118110243332, -0.5400638737290845981, -0.3530559997133363437 ) ) ;
#48600=CARTESIAN_POINT ( 'NONE',  ( 0.8136482939632553313, 0.2306618581243848609, 0.2411417322834645549 ) ) ;
#48601=CARTESIAN_POINT ( 'NONE',  ( 1.528871391076116026, -0.5511811023622048555, -0.09757992244046775898 ) ) ;
#48602=CARTESIAN_POINT ( 'NONE',  ( 0.07217847769028949700, -0.3162353388693405765, 0.4822834645669290543 ) ) ;
#48603=CARTESIAN_POINT ( 'NONE',  ( 0.6167979002624678353, -0.4281496062992124485, 0.4176697321401328655 ) ) ;
#48610=CARTESIAN_POINT ( 'NONE',  ( -0.03937007874015669567, -0.5511811023622047445, 6.969142054262312111E-17 ) ) ;
#48612=CARTESIAN_POINT ( 'NONE',  ( -0.3477690288713905509, -0.6692913385826771977, 0.1292274648535927661 ) ) ;
#48613=CARTESIAN_POINT ( 'NONE',  ( 0.6824146981627303710, 0.2306618581243847221, -0.2411417322834647770 ) ) ;
#48615=CARTESIAN_POINT ( 'NONE',  ( 0.1246719160104994284, 0.1771653543307087075, -0.09757992244046823083 ) ) ;
#48616=CARTESIAN_POINT ( 'NONE',  ( -1.227034120734907141, -0.6692913385826773087, -0.1292274648535924053 ) ) ;
#48617=CARTESIAN_POINT ( 'NONE',  ( 1.220472440944882386, -0.6692913385826771977, 8.415575281601705876E-17 ) ) ;
#48620=CARTESIAN_POINT ( 'NONE',  ( -0.7426113562969628434, 2.209901789876557832, 0.5309055118110236338 ) ) ;
#48621=VERTEX_POINT ( 'NONE', #77620 ) ;
#48622=CARTESIAN_POINT ( 'NONE',  ( 0.8595800524934390507, -0.05778040916215560624, -0.4822834645669293319 ) ) ;
#48623=CARTESIAN_POINT ( 'NONE',  ( 1.286089238845145033, 0.1283753931104748280, 0.1820866141732283561 ) ) ;
#48624=CARTESIAN_POINT ( 'NONE',  ( 1.640419947506562393, -0.4281496062992124485, 0.4176697321401328655 ) ) ;
#48625=CARTESIAN_POINT ( 'NONE',  ( 1.482939632545932307, 0.05413385826771626580, -0.4176697321401330321 ) ) ;
#48628=CARTESIAN_POINT ( 'NONE',  ( 1.115485564304462551, -0.4281496062992127816, -0.4176697321401328100 ) ) ;
#48629=CARTESIAN_POINT ( 'NONE',  ( -1.692913385826770645, 0.2952755905511811885, 0.000000000000000000 ) ) ;
#48630=CARTESIAN_POINT ( 'NONE',  ( -0.5971128608923877978, 0.2952755905511811885, 0.1292274648535926551 ) ) ;
#48631=CARTESIAN_POINT ( 'NONE',  ( -0.6889763779527552368, -0.5400638737290845981, -0.3530559997133363437 ) ) ;
#48632=CARTESIAN_POINT ( 'NONE',  ( 1.410761154855643795, -0.3162353388693405765, 0.4822834645669290543 ) ) ;
#48634=CARTESIAN_POINT ( 'NONE',  ( 0.1771653543307093182, 0.1660481256975885056, 0.3530559997133364547 ) ) ;
#48636=EDGE_CURVE ( 'NONE', #29791, #35196, #10339, .T. ) ;
#48637=CARTESIAN_POINT ( 'NONE',  ( -1.469816272965878357, 0.1283753931104748280, 0.1820866141732283561 ) ) ;
#48642=CARTESIAN_POINT ( 'NONE',  ( -1.502624671916009680, -0.05778040916215560624, -0.4822834645669293319 ) ) ;
#48644=CARTESIAN_POINT ( 'NONE',  ( 1.673228346456693494, 0.07958543189024085140, 0.2665933059059887866 ) ) ;
#48646=CARTESIAN_POINT ( 'NONE',  ( 0.4052866537519773660, 0.02791078216816386681, 0.4328096321851896966 ) ) ;
#48649=CARTESIAN_POINT ( 'NONE',  ( -0.2755905511811015396, -0.5511811023622047445, 6.969142054262312111E-17 ) ) ;
#48650=CARTESIAN_POINT ( 'NONE',  ( -1.089238845144356427, -0.004921259842519576551, 0.3153832671262227771 ) ) ;
#48651=CARTESIAN_POINT ( 'NONE',  ( -1.049868766404198794, -0.6046776061558807314, 0.2411417322834647770 ) ) ;
#48652=CARTESIAN_POINT ( 'NONE',  ( 0.3477690288713918276, 0.2952755905511811885, 0.1292274648535926551 ) ) ;
#48653=CARTESIAN_POINT ( 'NONE',  ( -1.482939632545930975, 0.05413385826771666132, 0.4176697321401328100 ) ) ;
#48655=ORIENTED_EDGE ( 'NONE', *, *, #42359, .T. ) ;
#48656=CARTESIAN_POINT ( 'NONE',  ( -1.345144356955379816, -0.3162353388693405765, 0.4822834645669290543 ) ) ;
#48657=CARTESIAN_POINT ( 'NONE',  ( -1.595398199321655275, 2.115458727241839476, -0.1559797534342494962 ) ) ;
#48662=CARTESIAN_POINT ( 'NONE',  ( -0.6167979002624665030, -0.4281496062992127816, -0.4176697321401328100 ) ) ;
#48663=CARTESIAN_POINT ( 'NONE',  ( 1.318897637795276356, -0.5400638737290844871, 0.3530559997133364547 ) ) ;
#48667=CARTESIAN_POINT ( 'NONE',  ( 0.1674892343164159914, -2.191421614605370878E-15, 0.4445507791589071167 ) ) ;
#48668=CARTESIAN_POINT ( 'NONE',  ( -0.9055118110236215490, 0.2952755905511811885, 0.000000000000000000 ) ) ;
#48670=CARTESIAN_POINT ( 'NONE',  ( 0.1049868766404206816, -0.5023911411419708095, -0.1820866141732282451 ) ) ;
#48673=CARTESIAN_POINT ( 'NONE',  ( -0.09186351706036663400, -0.3690944881889763329, 0.3153832671262228327 ) ) ;
#48674=CARTESIAN_POINT ( 'NONE',  ( 0.7545931758530188826, -0.5511811023622046335, 0.09757992244046803654 ) ) ;
#48675=CARTESIAN_POINT ( 'NONE',  ( 0.5643044619422579178, -0.4281496062992127816, -0.4176697321401328100 ) ) ;
#48677=CARTESIAN_POINT ( 'NONE',  ( -0.2165354330708654795, 0.07958543189024085140, 0.2665933059059887866 ) ) ;
#48679=CARTESIAN_POINT ( 'NONE',  ( -1.620734908136482577, 0.2952755905511811885, 0.1292274648535926551 ) ) ;
#48680=CARTESIAN_POINT ( 'NONE',  ( -0.8464566929133852113, 0.1660481256975885056, 0.3530559997133364547 ) ) ;
#48682=CARTESIAN_POINT ( 'NONE',  ( 0.05249343832021075018, 0.2306618581243847221, -0.2411417322834647770 ) ) ;
#48683=CARTESIAN_POINT ( 'NONE',  ( -0.4921259842519677963, 0.1660481256975883668, -0.3530559997133364547 ) ) ;
#48685=CARTESIAN_POINT ( 'NONE',  ( 0.006561679790026889343, -0.08942795157527998196, 0.3641732283464567121 ) ) ;
#48686=CARTESIAN_POINT ( 'NONE',  ( -0.2296587926509179312, -0.3162353388693409650, -0.4822834645669289433 ) ) ;
#48687=CARTESIAN_POINT ( 'NONE',  ( -0.6299212598425188991, -0.1870078740157480879, -0.4822834645669291653 ) ) ;
#48688=CARTESIAN_POINT ( 'NONE',  ( 1.604771003085129433, 0.7270283685441701893, -0.1466069496707750053 ) ) ;
#48689=CARTESIAN_POINT ( 'NONE',  ( -1.012922870834580324, 5.991678263669262536E-15, 0.4118484887281945728 ) ) ;
#48690=CARTESIAN_POINT ( 'NONE',  ( 0.1049868766404206816, 0.2306618581243848609, 0.2411417322834645549 ) ) ;
#48692=CARTESIAN_POINT ( 'NONE',  ( 1.574803149606299746, -0.1870078740157479769, 0.4822834645669291653 ) ) ;
#48693=CARTESIAN_POINT ( 'NONE',  ( -0.4461942257217840213, 0.1283753931104748280, 0.1820866141732283561 ) ) ;
#48694=CARTESIAN_POINT ( 'NONE',  ( -0.5511811023622041894, -0.1870078740157480879, -0.4822834645669291653 ) ) ;
#48695=CARTESIAN_POINT ( 'NONE',  ( 1.640419947506562393, -0.4281496062992124485, 0.4176697321401328655 ) ) ;
#48696=CARTESIAN_POINT ( 'NONE',  ( 1.305774278215223960, -0.6692913385826771977, 0.1292274648535927661 ) ) ;
#48697=CARTESIAN_POINT ( 'NONE',  ( -1.482939632545930975, 0.05413385826771666132, 0.4176697321401328100 ) ) ;
#48698=CARTESIAN_POINT ( 'NONE',  ( -0.6692913385826764205, -0.5511811023622047445, 6.969142054262312111E-17 ) ) ;
#48702=CARTESIAN_POINT ( 'NONE',  ( 1.384514435695538559, 0.1771653543307087075, -0.09757992244046823083 ) ) ;
#48703=CARTESIAN_POINT ( 'NONE',  ( 1.318897637795276356, 0.07958543189024071263, -0.2665933059059888421 ) ) ;
#48704=CARTESIAN_POINT ( 'NONE',  ( 0.8858267716535438430, -0.5400638737290845981, -0.3530559997133363437 ) ) ;
#48705=CARTESIAN_POINT ( 'NONE',  ( 0.4330708661417329020, 0.2066929133858268208, 0.000000000000000000 ) ) ;
#48707=CARTESIAN_POINT ( 'NONE',  ( 0.7414698162729663755, -0.6692913385826773087, -0.1292274648535924053 ) ) ;
#48709=CARTESIAN_POINT ( 'NONE',  ( 1.141732283464567788, -0.5511811023622047445, 6.969142054262312111E-17 ) ) ;
#48710=CARTESIAN_POINT ( 'NONE',  ( 0.1837270341207357105, -0.6046776061558809534, -0.2411417322834644161 ) ) ;
#48711=CARTESIAN_POINT ( 'NONE',  ( -0.9448818897637790704, -0.1870078740157480879, -0.4822834645669291653 ) ) ;
#48712=CARTESIAN_POINT ( 'NONE',  ( 1.233595800524935227, 0.2306618581243847221, -0.2411417322834647770 ) ) ;
#48715=CARTESIAN_POINT ( 'NONE',  ( 0.2296587926509192634, -0.08942795157528024563, -0.3641732283464568787 ) ) ;
#48716=ORIENTED_EDGE ( 'NONE', *, *, #815, .F. ) ;
#48718=VERTEX_POINT ( 'NONE', #3917 ) ;
#48720=CARTESIAN_POINT ( 'NONE',  ( -0.6824146981627291497, -0.6046776061558809534, -0.2411417322834644161 ) ) ;
#48721=CARTESIAN_POINT ( 'NONE',  ( -0.4002624671916004129, -0.3162353388693405765, 0.4822834645669290543 ) ) ;
#48722=CARTESIAN_POINT ( 'NONE',  ( -0.3871391076115476282, -0.05778040916215522460, 0.4822834645669289988 ) ) ;
#48723=CARTESIAN_POINT ( 'NONE',  ( 0.7545931758530189937, 0.2952755905511810774, -0.1292274648535930714 ) ) ;
#48724=CARTESIAN_POINT ( 'NONE',  ( -0.8989501312335946848, -0.6692913385826771977, 0.1292274648535927661 ) ) ;
#48725=CARTESIAN_POINT ( 'NONE',  ( -0.4790026246719154557, -0.3162353388693405765, 0.4822834645669290543 ) ) ;
#48726=CARTESIAN_POINT ( 'NONE',  ( 1.181102362204724976, -0.1870078740157480879, -0.4822834645669291653 ) ) ;
#48727=CARTESIAN_POINT ( 'NONE',  ( 0.4199475065616803948, -0.6046776061558809534, -0.2411417322834644161 ) ) ;
#48728=CARTESIAN_POINT ( 'NONE',  ( 0.6299212598425204535, -0.1870078740157480879, -0.4822834645669291653 ) ) ;
#48730=CARTESIAN_POINT ( 'NONE',  ( -0.5839895013123351797, -0.5511811023622046335, 0.09757992244046803654 ) ) ;
#48731=ORIENTED_EDGE ( 'NONE', *, *, #58543, .F. ) ;
#48734=CARTESIAN_POINT ( 'NONE',  ( -0.7611548556430438595, 0.1283753931104748280, 0.1820866141732283561 ) ) ;
#48735=CARTESIAN_POINT ( 'NONE',  ( -0.3346456692913377662, 0.1660481256975883668, -0.3530559997133364547 ) ) ;
#48737=CARTESIAN_POINT ( 'NONE',  ( -0.6889763779527552368, -0.5400638737290845981, -0.3530559997133363437 ) ) ;
#48738=CARTESIAN_POINT ( 'NONE',  ( -1.030183727034119867, -0.05778040916215560624, -0.4822834645669293319 ) ) ;
#48739=CARTESIAN_POINT ( 'NONE',  ( -1.312335958005248715, 0.2306618581243848609, 0.2411417322834645549 ) ) ;
#48740=CARTESIAN_POINT ( 'NONE',  ( -1.338582677165353729, -0.1870078740157480879, -0.4822834645669291653 ) ) ;
#48741=CARTESIAN_POINT ( 'NONE',  ( 0.7545931758530189937, 0.1771653543307087075, -0.09757992244046823083 ) ) ;
#48744=CARTESIAN_POINT ( 'NONE',  ( 0.4921259842519691285, 0.07958543189024085140, 0.2665933059059887866 ) ) ;
#48745=CARTESIAN_POINT ( 'NONE',  ( 0.1377952755905518800, 0.1660481256975883668, -0.3530559997133364547 ) ) ;
#48746=CARTESIAN_POINT ( 'NONE',  ( 0.1181102362204730916, 0.2952755905511811885, 0.000000000000000000 ) ) ;
#48747=ORIENTED_EDGE ( 'NONE', *, *, #27995, .F. ) ;
#48752=CARTESIAN_POINT ( 'NONE',  ( 1.607611548556431069, 0.2952755905511811885, 0.1292274648535926551 ) ) ;
#48753=CARTESIAN_POINT ( 'NONE',  ( -0.5577427821522301654, -0.08942795157528024563, -0.3641732283464568787 ) ) ;
#48754=CARTESIAN_POINT ( 'NONE',  ( -1.030183727034119867, -0.05778040916215560624, -0.4822834645669293319 ) ) ;
#48758=CARTESIAN_POINT ( 'NONE',  ( -1.417322834645668772, -0.1870078740157480601, -0.3641732283464567677 ) ) ;
#48759=CARTESIAN_POINT ( 'NONE',  ( 0.6233595800524939223, -0.3162353388693405765, 0.4822834645669290543 ) ) ;
#48760=CARTESIAN_POINT ( 'NONE',  ( 0.4921259842519691285, -0.5400638737290845981, -0.3530559997133363437 ) ) ;
#48761=CARTESIAN_POINT ( 'NONE',  ( -0.5774278215223089816, -0.5023911411419708095, 0.1820866141732285504 ) ) ;
#48762=CARTESIAN_POINT ( 'NONE',  ( 0.1115485564304467270, -0.6692913385826773087, -0.1292274648535924053 ) ) ;
#48764=CARTESIAN_POINT ( 'NONE',  ( -0.2493438320209966919, 0.05413385826771626580, -0.4176697321401330321 ) ) ;
#48767=CARTESIAN_POINT ( 'NONE',  ( 1.404199475065617264, -0.3690944881889763329, 0.3153832671262228327 ) ) ;
#48768=CARTESIAN_POINT ( 'NONE',  ( 0.07874015748031558404, -0.1870078740157480601, -0.3641732283464567677 ) ) ;
#48769=CARTESIAN_POINT ( 'NONE',  ( 1.312335958005250269, -0.5023911411419708095, 0.1820866141732285504 ) ) ;
#48770=CARTESIAN_POINT ( 'NONE',  ( -1.082677165354329896, 0.1660481256975885056, 0.3530559997133364547 ) ) ;
#48771=CARTESIAN_POINT ( 'NONE',  ( -1.338582677165353729, -0.1870078740157479769, 0.3641732283464567677 ) ) ;
#48773=CARTESIAN_POINT ( 'NONE',  ( -0.9776902887139098386, -0.6692913385826771977, 0.1292274648535927661 ) ) ;
#48774=CARTESIAN_POINT ( 'NONE',  ( -0.3740157480314953431, 0.1660481256975885056, 0.3530559997133364547 ) ) ;
#48775=CARTESIAN_POINT ( 'NONE',  ( 0.1968503937007881344, -0.6692913385826771977, 8.415575281601705876E-17 ) ) ;
#48777=CARTESIAN_POINT ( 'NONE',  ( 1.090866038711136632, -3.876714527516387216E-16, -0.3791475997938230647 ) ) ;
#48778=CARTESIAN_POINT ( 'NONE',  ( 0.1574803149606306130, -0.1870078740157480601, -0.3641732283464567677 ) ) ;
#48779=CARTESIAN_POINT ( 'NONE',  ( 0.8530183727034126306, 0.05413385826771626580, -0.4176697321401330321 ) ) ;
#48780=CARTESIAN_POINT ( 'NONE',  ( -1.496062992125983815, -0.1870078740157480601, -0.3641732283464567677 ) ) ;
#48781=( BOUNDED_CURVE ( )  B_SPLINE_CURVE ( 2, ( #33287, #78324, #39159, #14358, #8441, #8853, #19816, #77481, #45465, #71163, #59356, #46727, #40015 ),
 .UNSPECIFIED., .F., .F. ) 
 B_SPLINE_CURVE_WITH_KNOTS ( ( 3, 2, 2, 2, 2, 2, 3 ),
 ( 0.3103969023887781509, 0.3106060606060606077, 0.3143939393939393923, 0.3181818181818181768, 0.3219696969696969613, 0.3257575757575757458, 0.3259667339748582027 ),
 .UNSPECIFIED. ) 
 CURVE ( )  GEOMETRIC_REPRESENTATION_ITEM ( )  RATIONAL_B_SPLINE_CURVE ( ( 0.9964447847208428577, 0.9981185001348096275, 1.000000000000000000, 0.9659258262890683122, 1.000000000000000000, 0.9659258262890683122, 1.000000000000000000, 0.9659258262890683122, 1.000000000000000000, 0.9659258262890683122, 1.000000000000000000, 0.9981185001348097385, 0.9964447847208430797 ) ) 
 REPRESENTATION_ITEM ( '' )  );
#48782=CARTESIAN_POINT ( 'NONE',  ( 0.8333333333333340365, -0.6692913385826771977, 0.1292274648535927661 ) ) ;
#48783=CARTESIAN_POINT ( 'NONE',  ( -1.410761154855642463, -0.08942795157527998196, 0.3641732283464567121 ) ) ;
#48785=CARTESIAN_POINT ( 'NONE',  ( -1.423884514435694859, -0.3162353388693405765, 0.4822834645669290543 ) ) ;
#48786=CARTESIAN_POINT ( 'NONE',  ( -1.043307086614172707, 0.1660481256975883668, -0.3530559997133364547 ) ) ;
#48787=CARTESIAN_POINT ( 'NONE',  ( -0.2821522309711278487, -0.5511811023622048555, -0.09757992244046775898 ) ) ;
#48789=CARTESIAN_POINT ( 'NONE',  ( 0.7545931758530188826, -0.5511811023622046335, 0.09757992244046803654 ) ) ;
#48790=CARTESIAN_POINT ( 'NONE',  ( -0.1574803149606292529, -0.1870078740157480879, -0.4822834645669291653 ) ) ;
#48792=CARTESIAN_POINT ( 'NONE',  ( -0.9580052493438311334, -0.4281496062992124485, 0.4176697321401328655 ) ) ;
#48794=CARTESIAN_POINT ( 'NONE',  ( 0.8530183727034126306, -0.004921259842519870586, -0.3153832671262229437 ) ) ;
#48795=CARTESIAN_POINT ( 'NONE',  ( -0.1443569553805765515, -0.4281496062992127816, -0.4176697321401328100 ) ) ;
#48796=CARTESIAN_POINT ( 'NONE',  ( -0.1312335958005241554, -0.6046776061558809534, -0.2411417322834644161 ) ) ;
#48797=CARTESIAN_POINT ( 'NONE',  ( -0.4002624671916004129, -0.2845877964562159024, 0.3641732283464567677 ) ) ;
#48799=CARTESIAN_POINT ( 'NONE',  ( -0.4593175853018364174, -0.3690944881889765550, -0.3153832671262227771 ) ) ;
#48800=CARTESIAN_POINT ( 'NONE',  ( 0.2034120734908144990, -0.6692913385826771977, 0.1292274648535927661 ) ) ;
#48801=CARTESIAN_POINT ( 'NONE',  ( -1.364829396325458521, 0.1283753931104746893, -0.1820866141732285504 ) ) ;
#48803=CARTESIAN_POINT ( 'NONE',  ( 1.607611548556431069, 0.2952755905511811885, 0.1292274648535926551 ) ) ;
#48805=ORIENTED_EDGE ( 'NONE', *, *, #51403, .T. ) ;
#48806=CARTESIAN_POINT ( 'NONE',  ( -1.614173228346456268, -0.5511811023622047445, 6.969142054262312111E-17 ) ) ;
#48807=CARTESIAN_POINT ( 'NONE',  ( -0.3608923884514428360, -0.6692913385826773087, -0.1292274648535924053 ) ) ;
#48808=CARTESIAN_POINT ( 'NONE',  ( -1.089238845144356427, -0.4281496062992127816, -0.4176697321401328100 ) ) ;
#48811=CARTESIAN_POINT ( 'NONE',  ( 1.509186351706037543, 0.05413385826771666132, 0.4176697321401328100 ) ) ;
#48812=CARTESIAN_POINT ( 'NONE',  ( 0.2559055118110243332, 0.1660481256975885056, 0.3530559997133364547 ) ) ;
#48815=CARTESIAN_POINT ( 'NONE',  ( -1.594488188976377563, -0.5400638737290844871, 0.3530559997133364547 ) ) ;
#48818=CARTESIAN_POINT ( 'NONE',  ( -0.7874015748031489847, -0.1870078740157480601, -0.3641732283464567677 ) ) ;
#48821=CARTESIAN_POINT ( 'NONE',  ( 0.6758530183727039509, 0.2952755905511810774, -0.1292274648535930714 ) ) ;
#48822=CARTESIAN_POINT ( 'NONE',  ( -0.1837270341207343505, -0.6046776061558807314, 0.2411417322834647770 ) ) ;
#48823=CARTESIAN_POINT ( 'NONE',  ( -1.108923884514435132, -0.05778040916215560624, -0.4822834645669293319 ) ) ;
#48824=CARTESIAN_POINT ( 'NONE',  ( 1.056430446194226658, 0.2952755905511811885, 0.1292274648535926551 ) ) ;
#48825=CARTESIAN_POINT ( 'NONE',  ( -1.181102362204723644, -0.1870078740157479769, 0.3641732283464567677 ) ) ;
#48827=CARTESIAN_POINT ( 'NONE',  ( 0.1640419947506569498, -0.3162353388693409650, -0.4822834645669289433 ) ) ;
#48828=CARTESIAN_POINT ( 'NONE',  ( -0.9120734908136475250, -0.6692913385826773087, -0.1292274648535924053 ) ) ;
#48830=CARTESIAN_POINT ( 'NONE',  ( 1.601049868766404982, 0.2306618581243848609, 0.2411417322834645549 ) ) ;
#48831=CARTESIAN_POINT ( 'NONE',  ( -0.7426113562972000981, 2.362204724409448620, -0.5309055118110235227 ) ) ;
#48832=CARTESIAN_POINT ( 'NONE',  ( 0.9580052493438327987, -0.4281496062992127816, -0.4176697321401328100 ) ) ;
#48834=CARTESIAN_POINT ( 'NONE',  ( 1.345144356955381593, -0.08942795157527998196, 0.3641732283464567121 ) ) ;
#48837=CARTESIAN_POINT ( 'NONE',  ( -0.6167979002624665030, -0.4281496062992127816, -0.4176697321401328100 ) ) ;
#48838=VERTEX_POINT ( 'NONE', #53999 ) ;
#48839=CARTESIAN_POINT ( 'NONE',  ( 0.2362204724409456558, -0.1870078740157480601, -0.3641732283464567677 ) ) ;
#48840=CARTESIAN_POINT ( 'NONE',  ( -1.456692913385826182, -0.6692913385826771977, 8.415575281601705876E-17 ) ) ;
#48841=CARTESIAN_POINT ( 'NONE',  ( 0.6233595800524939223, -0.3162353388693405765, 0.4822834645669290543 ) ) ;
#48842=CARTESIAN_POINT ( 'NONE',  ( 0.7414698162729663755, -0.6692913385826773087, -0.1292274648535924053 ) ) ;
#48843=CARTESIAN_POINT ( 'NONE',  ( -0.07874015748031421014, -0.1870078740157480879, -0.4822834645669291653 ) ) ;
#48846=CARTESIAN_POINT ( 'NONE',  ( -0.9514435695538050464, -0.05778040916215560624, -0.4822834645669293319 ) ) ;
#48848=CARTESIAN_POINT ( 'NONE',  ( -1.633858267716534529, -0.5400638737290845981, -0.3530559997133363437 ) ) ;
#48849=CARTESIAN_POINT ( 'NONE',  ( -1.122047244094487306, 0.1660481256975883668, -0.3530559997133364547 ) ) ;
#48850=CARTESIAN_POINT ( 'NONE',  ( 1.358267716535433323, 0.1660481256975885056, 0.3530559997133364547 ) ) ;
#48851=CARTESIAN_POINT ( 'NONE',  ( 1.076115485564305141, 0.2306618581243847221, -0.2411417322834647770 ) ) ;
#48853=CARTESIAN_POINT ( 'NONE',  ( -1.062992125984250968, 0.2952755905511811885, 0.000000000000000000 ) ) ;
#48855=CARTESIAN_POINT ( 'NONE',  ( 0.4396325459317590445, -0.6692913385826771977, 0.1292274648535927661 ) ) ;
#48858=CARTESIAN_POINT ( 'NONE',  ( -0.4527559055118102749, -0.5400638737290845981, -0.3530559997133363437 ) ) ;
#48859=CARTESIAN_POINT ( 'NONE',  ( 1.653543307086614789, -0.1870078740157479769, 0.4822834645669291653 ) ) ;
#48860=CARTESIAN_POINT ( 'NONE',  ( 0.5708661417322842269, 0.07958543189024085140, 0.2665933059059887866 ) ) ;
#48861=CARTESIAN_POINT ( 'NONE',  ( 1.338582677165355062, -0.1870078740157480879, -0.4822834645669291653 ) ) ;
#48863=CARTESIAN_POINT ( 'NONE',  ( 0.8595800524934390507, -0.2845877964562159024, 0.3641732283464567677 ) ) ;
#48864=CARTESIAN_POINT ( 'NONE',  ( 0.8136482939632553313, 0.2306618581243848609, 0.2411417322834645549 ) ) ;
#48867=CARTESIAN_POINT ( 'NONE',  ( -0.9973753280839886548, -0.6046776061558809534, -0.2411417322834644161 ) ) ;
#48868=CARTESIAN_POINT ( 'NONE',  ( -1.603475055217291612, 2.157339783260149080, 0.04573490813648253134 ) ) ;
#48869=CARTESIAN_POINT ( 'NONE',  ( 1.200787401574803681, -0.4536011799217368745, -0.2665933059059886201 ) ) ;
#48870=CARTESIAN_POINT ( 'NONE',  ( -0.7874015748031489847, -0.1870078740157479769, 0.4822834645669291653 ) ) ;
#48871=CARTESIAN_POINT ( 'NONE',  ( 0.05905511811023681640, 0.1660481256975883668, -0.3530559997133364547 ) ) ;
#48873=CARTESIAN_POINT ( 'NONE',  ( -0.08530183727034056085, -0.05778040916215560624, -0.4822834645669293319 ) ) ;
#48874=CARTESIAN_POINT ( 'NONE',  ( 0.6889763779527566800, -0.4536011799217367080, 0.2665933059059888421 ) ) ;
#48876=CARTESIAN_POINT ( 'NONE',  ( 0.1509186351706045259, -0.08942795157528024563, -0.3641732283464568787 ) ) ;
#48877=CARTESIAN_POINT ( 'NONE',  ( 0.8595800524934390507, -0.08942795157528024563, -0.3641732283464568787 ) ) ;
#48878=DIRECTION ( 'NONE',  ( 0.8050726085550603539, 2.493067783899206833E-16, -0.5931762764594944448 ) ) ;
#48880=CARTESIAN_POINT ( 'NONE',  ( 0.4855643044619430415, -0.4281496062992127816, -0.4176697321401328100 ) ) ;
#48882=CARTESIAN_POINT ( 'NONE',  ( 1.430446194225722500, -0.3690944881889765550, -0.3153832671262227771 ) ) ;
#48884=CARTESIAN_POINT ( 'NONE',  ( 0.1115485564304467270, -0.5511811023622048555, -0.09757992244046775898 ) ) ;
#48885=CARTESIAN_POINT ( 'NONE',  ( 0.006561679790026889343, -0.3162353388693409650, -0.4822834645669289433 ) ) ;
#48886=CARTESIAN_POINT ( 'NONE',  ( 1.246719160104987623, -0.004921259842519870586, -0.3153832671262229437 ) ) ;
#48887=CARTESIAN_POINT ( 'NONE',  ( -1.397637795275589623, 0.07958543189024085140, 0.2665933059059887866 ) ) ;
#48888=CARTESIAN_POINT ( 'NONE',  ( -1.443569553805773564, -0.6046776061558807314, 0.2411417322834647770 ) ) ;
#48889=CARTESIAN_POINT ( 'NONE',  ( 0.3149606299212606708, -0.1870078740157480879, -0.4822834645669291653 ) ) ;
#48890=CARTESIAN_POINT ( 'NONE',  ( 1.049868766404200349, 0.2306618581243848609, 0.2411417322834645549 ) ) ;
#48891=CARTESIAN_POINT ( 'NONE',  ( 1.604771003085129433, 1.320215725944020813, -0.1466069496707750330 ) ) ;
#48892=CARTESIAN_POINT ( 'NONE',  ( 0.3412073490813655186, 0.2306618581243848609, 0.2411417322834645549 ) ) ;
#48893=CARTESIAN_POINT ( 'NONE',  ( 1.200787401574803681, 0.1660481256975885056, 0.3530559997133364547 ) ) ;
#48894=CARTESIAN_POINT ( 'NONE',  ( 0.9251968503937015864, 0.1660481256975883668, -0.3530559997133364547 ) ) ;
#48895=CARTESIAN_POINT ( 'NONE',  ( -1.614173228346457378, 1.330640075373402897, -0.1372047244094477536 ) ) ;
#48896=CARTESIAN_POINT ( 'NONE',  ( 0.8005249343832028242, -0.3690944881889765550, -0.3153832671262227771 ) ) ;
#48897=CARTESIAN_POINT ( 'NONE',  ( -1.561679790026246017, -0.3690944881889765550, -0.3153832671262227771 ) ) ;
#48898=CARTESIAN_POINT ( 'NONE',  ( -0.05249343832020938322, -0.5023911411419708095, -0.1820866141732282451 ) ) ;
#48900=CARTESIAN_POINT ( 'NONE',  ( -0.09842519685039295696, -0.5400638737290844871, 0.3530559997133364547 ) ) ;
#48901=CARTESIAN_POINT ( 'NONE',  ( 0.8923884514435701520, -0.6046776061558809534, -0.2411417322834644161 ) ) ;
#48902=CARTESIAN_POINT ( 'NONE',  ( -0.2690288713910754526, -0.6692913385826771977, 0.1292274648535927661 ) ) ;
#48904=CARTESIAN_POINT ( 'NONE',  ( -0.1049868766404193215, 0.1283753931104746893, -0.1820866141732285504 ) ) ;
#48905=CARTESIAN_POINT ( 'NONE',  ( 0.9120734908136489683, -0.6692913385826771977, 0.1292274648535927661 ) ) ;
#48906=CARTESIAN_POINT ( 'NONE',  ( 0.9580052493438327987, -0.3690944881889765550, -0.3153832671262227771 ) ) ;
#48908=CARTESIAN_POINT ( 'NONE',  ( -0.3249695492770445782, -2.567464376874931580E-15, -0.4445507791589072832 ) ) ;
#48909=CARTESIAN_POINT ( 'NONE',  ( 1.614173228346456712, 1.496062992125984481, 0.1372047244094478646 ) ) ;
#48911=CARTESIAN_POINT ( 'NONE',  ( -1.193875086542979913, 0.004960608223780448196, -0.3437734562760181856 ) ) ;
#48912=CARTESIAN_POINT ( 'NONE',  ( -1.174540682414697335, -0.05778040916215522460, 0.4822834645669289988 ) ) ;
#48913=CARTESIAN_POINT ( 'NONE',  ( -0.3215223097112853146, -0.3162353388693405765, 0.4822834645669290543 ) ) ;
#48917=CARTESIAN_POINT ( 'NONE',  ( 0.3412073490813655186, -0.5023911411419708095, -0.1820866141732282451 ) ) ;
#48919=CARTESIAN_POINT ( 'NONE',  ( 1.154855643044620184, 0.2306618581243847221, -0.2411417322834647770 ) ) ;
#48920=EDGE_CURVE ( 'NONE', #50394, #44445, #49640, .T. ) ;
#48922=CARTESIAN_POINT ( 'NONE',  ( 0.9645669291338588858, 0.1660481256975885056, 0.3530559997133364547 ) ) ;
#48924=CARTESIAN_POINT ( 'NONE',  ( 1.509186351706037543, 0.05413385826771666132, 0.4176697321401328100 ) ) ;
#48925=CARTESIAN_POINT ( 'NONE',  ( 1.266404199475066328, -0.08942795157527998196, 0.3641732283464567121 ) ) ;
#48926=CARTESIAN_POINT ( 'NONE',  ( 0.2165354330708668673, -0.5400638737290844871, 0.3530559997133364547 ) ) ;
#48928=CARTESIAN_POINT ( 'NONE',  ( -0.01312335958005186876, 0.05413385826771626580, -0.4176697321401330321 ) ) ;
#48929=CARTESIAN_POINT ( 'NONE',  ( -0.8267716535433065062, -0.5511811023622047445, 6.969142054262312111E-17 ) ) ;
#48930=CARTESIAN_POINT ( 'NONE',  ( 0.4921259842519691285, 0.1660481256975885056, 0.3530559997133364547 ) ) ;
#48931=CARTESIAN_POINT ( 'NONE',  ( -0.2559055118110230564, 0.1660481256975883668, -0.3530559997133364547 ) ) ;
#48935=CARTESIAN_POINT ( 'NONE',  ( 0.6889763779527566800, -0.5400638737290844871, 0.3530559997133364547 ) ) ;
#48936=CARTESIAN_POINT ( 'NONE',  ( -0.2165354330708654795, -0.5400638737290845981, -0.3530559997133363437 ) ) ;
#48937=CARTESIAN_POINT ( 'NONE',  ( -1.430446194225720724, 0.05413385826771626580, -0.4176697321401330321 ) ) ;
#48938=CARTESIAN_POINT ( 'NONE',  ( 1.023622047244095112, -0.1870078740157480879, -0.4822834645669291653 ) ) ;
#48939=CARTESIAN_POINT ( 'NONE',  ( 0.5511811023622055217, -0.1870078740157479769, 0.4822834645669291653 ) ) ;
#48941=CARTESIAN_POINT ( 'NONE',  ( -0.2099737532808391705, -0.6046776061558809534, -0.2411417322834644161 ) ) ;
#48942=CARTESIAN_POINT ( 'NONE',  ( 0.2165354330708668673, -0.5400638737290844871, 0.3530559997133364547 ) ) ;
#48943=CARTESIAN_POINT ( 'NONE',  ( -0.6102362204724400829, -0.5400638737290845981, -0.3530559997133363437 ) ) ;
#48945=CARTESIAN_POINT ( 'NONE',  ( 0.1509186351706045259, -0.08942795157528024563, -0.3641732283464568787 ) ) ;
#48946=CARTESIAN_POINT ( 'NONE',  ( -1.620734908136482577, -0.6692913385826773087, -0.1292274648535924053 ) ) ;
#48948=CARTESIAN_POINT ( 'NONE',  ( 0.2690288713910767848, -0.6692913385826773087, -0.1292274648535924053 ) ) ;
#48950=CARTESIAN_POINT ( 'NONE',  ( -1.515748031496062076, -0.5400638737290844871, 0.3530559997133364547 ) ) ;
#48953=ORIENTED_EDGE ( 'NONE', *, *, #16637, .T. ) ;
#48954=CARTESIAN_POINT ( 'NONE',  ( 0.7874015748031503170, -0.1870078740157480879, -0.4822834645669291653 ) ) ;
#48955=CARTESIAN_POINT ( 'NONE',  ( 0.1115485564304467270, -0.5511811023622048555, -0.09757992244046775898 ) ) ;
#48956=CARTESIAN_POINT ( 'NONE',  ( 1.673228346456693494, 0.07958543189024085140, 0.2665933059059887866 ) ) ;
#48963=CARTESIAN_POINT ( 'NONE',  ( 0.7611548556430451917, -0.6046776061558807314, 0.2411417322834647770 ) ) ;
#48964=CARTESIAN_POINT ( 'NONE',  ( -0.7086614173228339419, -0.1870078740157479769, 0.4822834645669291653 ) ) ;
#48965=CARTESIAN_POINT ( 'NONE',  ( -0.7545931758530177724, 0.2952755905511811885, 0.1292274648535926551 ) ) ;
#48966=CARTESIAN_POINT ( 'NONE',  ( 0.8333333333333340365, 0.2952755905511810774, -0.1292274648535930714 ) ) ;
#48967=CARTESIAN_POINT ( 'NONE',  ( 1.227034120734908917, -0.6692913385826771977, 0.1292274648535927661 ) ) ;
#48968=CARTESIAN_POINT ( 'NONE',  ( -1.170763242744969235, -1.094630224652485432E-15, 0.4281993546915541238 ) ) ;
#48970=CARTESIAN_POINT ( 'NONE',  ( 1.207349081364829990, 0.1283753931104748280, 0.1820866141732283561 ) ) ;
#48972=CARTESIAN_POINT ( 'NONE',  ( -1.502624671916009680, -0.2845877964562159024, 0.3641732283464567677 ) ) ;
#48974=CARTESIAN_POINT ( 'NONE',  ( 0.1115485564304470323, 0.2952755905511811885, 0.1292274648535926551 ) ) ;
#48975=CARTESIAN_POINT ( 'NONE',  ( 1.345144356955381593, -0.05778040916215522460, 0.4822834645669289988 ) ) ;
#48977=CARTESIAN_POINT ( 'NONE',  ( -1.338582677165353729, -0.1870078740157480601, -0.3641732283464567677 ) ) ;
#48978=CARTESIAN_POINT ( 'NONE',  ( 0.3083989501312343062, -0.05778040916215560624, -0.4822834645669293319 ) ) ;
#48979=CARTESIAN_POINT ( 'NONE',  ( 1.397637795275591177, -0.4536011799217367080, 0.2665933059059888421 ) ) ;
#48981=CARTESIAN_POINT ( 'NONE',  ( -1.391076115485563758, 0.1283753931104748280, 0.1820866141732283561 ) ) ;
#48982=CARTESIAN_POINT ( 'NONE',  ( 1.535433070866142558, 0.2952755905511811885, 0.000000000000000000 ) ) ;
#48984=CARTESIAN_POINT ( 'NONE',  ( 0.03937007874015806264, 0.1771653543307087630, 0.000000000000000000 ) ) ;
#48985=CARTESIAN_POINT ( 'NONE',  ( -0.08530183727034056085, -0.05778040916215560624, -0.4822834645669293319 ) ) ;
#48986=CARTESIAN_POINT ( 'NONE',  ( -1.233595800524933894, -0.5023911411419708095, -0.1820866141732282451 ) ) ;
#48987=EDGE_CURVE ( 'NONE', #65960, #69752, #39676, .T. ) ;
#48988=CARTESIAN_POINT ( 'NONE',  ( -0.7742782152230965886, 0.05413385826771666132, 0.4176697321401328100 ) ) ;
#48989=CARTESIAN_POINT ( 'NONE',  ( 1.522309711286089939, 0.2306618581243848609, 0.2411417322834645549 ) ) ;
#48992=CARTESIAN_POINT ( 'NONE',  ( 1.213910761154856299, -0.6692913385826773087, -0.1292274648535924053 ) ) ;
#48994=CARTESIAN_POINT ( 'NONE',  ( -1.003937007874015297, -0.5400638737290845981, -0.3530559997133363437 ) ) ;
#48995=CARTESIAN_POINT ( 'NONE',  ( -1.115485564304461219, -0.004921259842519870586, -0.3153832671262229437 ) ) ;
#48996=CARTESIAN_POINT ( 'NONE',  ( -0.5774278215223089816, 0.1283753931104746893, -0.1820866141732285504 ) ) ;
#48997=CARTESIAN_POINT ( 'NONE',  ( 0.7977407017645454790, -9.595573933774993207E-16, 0.4281989832122458095 ) ) ;
#48998=CARTESIAN_POINT ( 'NONE',  ( 0.1246719160104994284, 0.2952755905511810774, -0.1292274648535930714 ) ) ;
#48999=CARTESIAN_POINT ( 'NONE',  ( -0.05905511811023545637, 0.07958543189024085140, 0.2665933059059887866 ) ) ;
#49000=CARTESIAN_POINT ( 'NONE',  ( -1.266404199475064773, -0.2845877964562159024, 0.3641732283464567677 ) ) ;
#49001=CARTESIAN_POINT ( 'NONE',  ( -1.587926509186350810, -0.4281496062992124485, 0.4176697321401328655 ) ) ;
#49002=CARTESIAN_POINT ( 'NONE',  ( 1.489501312335958172, -0.08942795157528024563, -0.3641732283464568787 ) ) ;
#49003=CARTESIAN_POINT ( 'NONE',  ( 1.259842519685040019, -0.1870078740157480879, -0.4822834645669291653 ) ) ;
#49005=CARTESIAN_POINT ( 'NONE',  ( 0.5708661417322842269, 0.07958543189024085140, 0.2665933059059887866 ) ) ;
#49006=CARTESIAN_POINT ( 'NONE',  ( 1.010498687664042716, -0.4281496062992124485, 0.4176697321401328655 ) ) ;
#49007=CARTESIAN_POINT ( 'NONE',  ( 0.8530183727034126306, -0.004921259842519870586, -0.3153832671262229437 ) ) ;
#49009=EDGE_CURVE ( 'NONE', #17299, #57855, #32740, .T. ) ;
#49010=CARTESIAN_POINT ( 'NONE',  ( -1.076115485564303809, -0.6046776061558809534, -0.2411417322834644161 ) ) ;
#49012=CARTESIAN_POINT ( 'NONE',  ( -0.7545931758530176614, -0.6692913385826773087, -0.1292274648535924053 ) ) ;
#49013=CARTESIAN_POINT ( 'NONE',  ( -0.2099737532808391705, -0.6046776061558809534, -0.2411417322834644161 ) ) ;
#49014=CARTESIAN_POINT ( 'NONE',  ( -0.6575345472713096662, 1.929133858267489954, 0.5309055118110236338 ) ) ;
#49016=CARTESIAN_POINT ( 'NONE',  ( 0.7874015748031503170, -0.1870078740157479769, 0.4822834645669291653 ) ) ;
#49017=CARTESIAN_POINT ( 'NONE',  ( 1.581364829396326277, -0.08942795157527998196, 0.3641732283464567121 ) ) ;
#49018=CARTESIAN_POINT ( 'NONE',  ( 0.2099737532808405305, -0.6046776061558807314, 0.2411417322834647770 ) ) ;
#49019=CARTESIAN_POINT ( 'NONE',  ( 0.9448818897637802916, -0.1870078740157479769, 0.4822834645669291653 ) ) ;
#49026=CARTESIAN_POINT ( 'NONE',  ( -0.3937007874015740483, -0.1870078740157480601, -0.3641732283464567677 ) ) ;
#49027=CARTESIAN_POINT ( 'NONE',  ( -0.5905511811023615998, 0.2952755905511811885, 0.000000000000000000 ) ) ;
#49028=CARTESIAN_POINT ( 'NONE',  ( 0.3018372703412079971, -0.4281496062992124485, 0.4176697321401328655 ) ) ;
#49030=CARTESIAN_POINT ( 'NONE',  ( 1.581364829396326277, -0.05778040916215522460, 0.4822834645669289988 ) ) ;
#49031=CARTESIAN_POINT ( 'NONE',  ( 0.9973753280839902091, 0.2306618581243847221, -0.2411417322834647770 ) ) ;
#49034=CARTESIAN_POINT ( 'NONE',  ( 0.4849061582275019378, 1.967896864084105024, 0.4921425059946345493 ) ) ;
#49035=CARTESIAN_POINT ( 'NONE',  ( 1.154855643044620184, 0.2306618581243847221, -0.2411417322834647770 ) ) ;
#49036=CARTESIAN_POINT ( 'NONE',  ( 1.089238845144357537, -0.3690944881889763329, 0.3153832671262228327 ) ) ;
#49037=CARTESIAN_POINT ( 'NONE',  ( -1.450131233595799651, 0.1771653543307087075, -0.09757992244046823083 ) ) ;
#49038=CARTESIAN_POINT ( 'NONE',  ( -1.509186351706035767, -0.4281496062992124485, 0.4176697321401328655 ) ) ;
#49040=CARTESIAN_POINT ( 'NONE',  ( -1.614173228346457378, 2.094556775020298023, 0.1372047244094476981 ) ) ;
#49041=CARTESIAN_POINT ( 'NONE',  ( 0.8005249343832028242, -0.4281496062992127816, -0.4176697321401328100 ) ) ;
#49042=CARTESIAN_POINT ( 'NONE',  ( 1.364829396325460076, 0.1283753931104748280, 0.1820866141732283561 ) ) ;
#49043=CARTESIAN_POINT ( 'NONE',  ( -0.5511811023622041894, -0.1870078740157480879, -0.4822834645669291653 ) ) ;
#49044=CARTESIAN_POINT ( 'NONE',  ( -0.4133858267716528645, 0.1660481256975883668, -0.3530559997133364547 ) ) ;
#49045=CARTESIAN_POINT ( 'NONE',  ( 1.502624671916010790, -0.3162353388693409650, -0.4822834645669289433 ) ) ;
#49047=CARTESIAN_POINT ( 'NONE',  ( 0.3083989501312343062, -0.3162353388693405765, 0.4822834645669290543 ) ) ;
#49049=CARTESIAN_POINT ( 'NONE',  ( 1.627296587926509996, -0.6046776061558807314, 0.2411417322834647770 ) ) ;
#49050=ORIENTED_EDGE ( 'NONE', *, *, #35952, .T. ) ;
#49053=DIRECTION ( 'NONE',  ( -0.2810846377148243924, -0.6785983445458325658, -0.6785983445458596552 ) ) ;
#49054=CARTESIAN_POINT ( 'NONE',  ( -1.482939632545930975, -0.4281496062992127816, -0.4176697321401328100 ) ) ;
#49056=CARTESIAN_POINT ( 'NONE',  ( 0.4889872687189470435, 1.535433070866141225, 0.4915354330708653907 ) ) ;
#49061=CARTESIAN_POINT ( 'NONE',  ( -0.1377952755905504645, -0.4536011799217368745, -0.2665933059059886201 ) ) ;
#49062=CARTESIAN_POINT ( 'NONE',  ( -1.017060367454067249, -0.2845877964562161244, -0.3641732283464567121 ) ) ;
#49064=CARTESIAN_POINT ( 'NONE',  ( -1.515748031496062076, -0.5400638737290844871, 0.3530559997133364547 ) ) ;
#49065=CARTESIAN_POINT ( 'NONE',  ( 0.4133858267716541968, -0.5400638737290845981, -0.3530559997133363437 ) ) ;
#49066=CARTESIAN_POINT ( 'NONE',  ( -1.541994750656167090, -0.6692913385826773087, -0.1292274648535924053 ) ) ;
#49068=VERTEX_POINT ( 'NONE', #30813 ) ;
#49069=CARTESIAN_POINT ( 'NONE',  ( 1.541994750656168645, -0.6692913385826771977, 0.1292274648535927661 ) ) ;
#49073=DIRECTION ( 'NONE',  ( 0.000000000000000000, -1.000000000000000000, 0.000000000000000000 ) ) ;
#49074=CARTESIAN_POINT ( 'NONE',  ( -0.9448818897637790704, -0.1870078740157480879, -0.4822834645669291653 ) ) ;
#49075=CARTESIAN_POINT ( 'NONE',  ( 1.371391076115485941, 0.2952755905511811885, 0.1292274648535926551 ) ) ;
#49076=CARTESIAN_POINT ( 'NONE',  ( 0.6423408027444581503, 0.000000000000000000, 0.3464511005275205946 ) ) ;
#49077=CARTESIAN_POINT ( 'NONE',  ( 1.574803149606299746, -0.1870078740157480879, -0.4822834645669291653 ) ) ;
#49078=CARTESIAN_POINT ( 'NONE',  ( -0.7349081364829390672, 0.2306618581243847221, -0.2411417322834647770 ) ) ;
#49079=AXIS2_PLACEMENT_3D ( 'NONE', #56916, #36336, #29605 ) ;
#49081=CARTESIAN_POINT ( 'NONE',  ( -0.02624671916010428221, -0.5023911411419708095, 0.1820866141732285504 ) ) ;
#49083=CARTESIAN_POINT ( 'NONE',  ( 0.08530183727034192087, -0.08942795157527998196, 0.3641732283464567121 ) ) ;
#49084=CARTESIAN_POINT ( 'NONE',  ( 0.5577427821522314977, -0.2845877964562161244, -0.3641732283464567121 ) ) ;
#49085=CARTESIAN_POINT ( 'NONE',  ( 0.4593175853018379162, -0.4281496062992124485, 0.4176697321401328655 ) ) ;
#49086=CARTESIAN_POINT ( 'NONE',  ( -0.2624671916010490880, -0.5023911411419708095, 0.1820866141732285504 ) ) ;
#49088=CARTESIAN_POINT ( 'NONE',  ( 1.482939632545932307, 0.05413385826771626580, -0.4176697321401330321 ) ) ;
#49089=CARTESIAN_POINT ( 'NONE',  ( -1.194225721784776262, -0.4281496062992124485, 0.4176697321401328655 ) ) ;
#49091=CARTESIAN_POINT ( 'NONE',  ( -0.1049868766404193215, 0.2306618581243847221, -0.2411417322834647770 ) ) ;
#49092=CARTESIAN_POINT ( 'NONE',  ( -0.5971128608923877978, -0.6692913385826773087, -0.1292274648535924053 ) ) ;
#49093=CARTESIAN_POINT ( 'NONE',  ( 1.509186351706037543, -0.004921259842519576551, 0.3153832671262227771 ) ) ;
#49094=CARTESIAN_POINT ( 'NONE',  ( 0.2690288713910767848, -0.5511811023622048555, -0.09757992244046775898 ) ) ;
#49095=CARTESIAN_POINT ( 'NONE',  ( -0.3477690288713905509, -0.6692913385826771977, 0.1292274648535927661 ) ) ;
#49096=CARTESIAN_POINT ( 'NONE',  ( -0.7545931758530176614, -0.6692913385826773087, -0.1292274648535924053 ) ) ;
#49098=CARTESIAN_POINT ( 'NONE',  ( 1.515748031496063408, 0.07958543189024085140, 0.2665933059059887866 ) ) ;
#49099=CARTESIAN_POINT ( 'NONE',  ( 0.1837270341207357105, -0.6046776061558809534, -0.2411417322834644161 ) ) ;
#49102=CARTESIAN_POINT ( 'NONE',  ( 1.318897637795276356, 0.1660481256975883668, -0.3530559997133364547 ) ) ;
#49103=CARTESIAN_POINT ( 'NONE',  ( -0.5971128608923877978, 0.1771653543307087630, 0.09757992244046791164 ) ) ;
#49104=CARTESIAN_POINT ( 'NONE',  ( -0.7742782152230965886, 0.05413385826771666132, 0.4176697321401328100 ) ) ;
#49105=CARTESIAN_POINT ( 'NONE',  ( 1.233595800524935227, 0.2306618581243847221, -0.2411417322834647770 ) ) ;
#49106=CARTESIAN_POINT ( 'NONE',  ( 0.7414698162729663755, 0.2952755905511811885, 0.1292274648535926551 ) ) ;
#49108=CARTESIAN_POINT ( 'NONE',  ( -1.148293963254592542, -0.5511811023622048555, -0.09757992244046775898 ) ) ;
#49112=EDGE_CURVE ( 'NONE', #6101, #78909, #32055, .T. ) ;
#49113=DIRECTION ( 'NONE',  ( 9.929802617766460227E-17, -0.7071067811865515695, -0.7071067811865434649 ) ) ;
#49114=CARTESIAN_POINT ( 'NONE',  ( 1.030183727034121421, -0.2845877964562161244, -0.3641732283464567121 ) ) ;
#49115=CARTESIAN_POINT ( 'NONE',  ( 0.3740157480314966754, 0.1660481256975883668, -0.3530559997133364547 ) ) ;
#49116=CARTESIAN_POINT ( 'NONE',  ( -1.548556430446193399, 0.2306618581243848609, 0.2411417322834645549 ) ) ;
#49118=CARTESIAN_POINT ( 'NONE',  ( 1.003937007874016407, -0.4536011799217367080, 0.2665933059059888421 ) ) ;
#49119=CARTESIAN_POINT ( 'NONE',  ( -0.1049868766404193215, -0.6046776061558807314, 0.2411417322834647770 ) ) ;
#49120=CARTESIAN_POINT ( 'NONE',  ( -0.7808398950131222316, -0.3162353388693409650, -0.4822834645669289433 ) ) ;
#49121=CARTESIAN_POINT ( 'NONE',  ( 1.220472440944882608, 0.2952755905511811885, 0.000000000000000000 ) ) ;
#49125=CARTESIAN_POINT ( 'NONE',  ( -0.2165354330708654795, -0.4536011799217368745, -0.2665933059059886201 ) ) ;
#49126=EDGE_CURVE ( 'NONE', #64347, #16662, #25639, .T. ) ;
#49127=ORIENTED_EDGE ( 'NONE', *, *, #65114, .F. ) ;
#49130=CARTESIAN_POINT ( 'NONE',  ( -1.017060367454067249, -0.3162353388693409650, -0.4822834645669289433 ) ) ;
#49131=CARTESIAN_POINT ( 'NONE',  ( -0.09842519685039295696, -0.5400638737290844871, 0.3530559997133364547 ) ) ;
#49132=CARTESIAN_POINT ( 'NONE',  ( -0.1246719160104980823, -0.6692913385826773087, -0.1292274648535924053 ) ) ;
#49133=CARTESIAN_POINT ( 'NONE',  ( 0.8398950131233602345, -0.6046776061558807314, 0.2411417322834647770 ) ) ;
#49135=CARTESIAN_POINT ( 'NONE',  ( -0.5708661417322825615, -0.5400638737290844871, 0.3530559997133364547 ) ) ;
#49136=CARTESIAN_POINT ( 'NONE',  ( -1.246719160104985846, -0.4281496062992127816, -0.4176697321401328100 ) ) ;
#49137=CARTESIAN_POINT ( 'NONE',  ( -0.2362204724409442680, -0.1870078740157480879, -0.4822834645669291653 ) ) ;
#49138=CARTESIAN_POINT ( 'NONE',  ( 0.9251968503937015864, -0.5400638737290844871, 0.3530559997133364547 ) ) ;
#49139=CARTESIAN_POINT ( 'NONE',  ( 0.5446194225721792126, -0.05778040916215560624, -0.4822834645669293319 ) ) ;
#49141=CARTESIAN_POINT ( 'NONE',  ( -0.2559055118110227234, -0.4536011799217367080, 0.2665933059059888421 ) ) ;
#49145=CARTESIAN_POINT ( 'NONE',  ( -1.240157480314959759, 0.07958543189024085140, 0.2665933059059887866 ) ) ;
#49146=CARTESIAN_POINT ( 'NONE',  ( -0.6299212598425188991, -0.1870078740157480879, -0.4822834645669291653 ) ) ;
#49147=CARTESIAN_POINT ( 'NONE',  ( -1.191111281560509383, -2.567464376874931580E-15, -0.4445507791589072832 ) ) ;
#49148=CARTESIAN_POINT ( 'NONE',  ( -0.8005249343832013809, -0.4281496062992124485, 0.4176697321401328655 ) ) ;
#49149=CARTESIAN_POINT ( 'NONE',  ( -0.9973753280839886548, -0.6046776061558809534, -0.2411417322834644161 ) ) ;
#49150=CARTESIAN_POINT ( 'NONE',  ( -1.358267716535432434, -0.5400638737290844871, 0.3530559997133364547 ) ) ;
#49152=B_SPLINE_CURVE_WITH_KNOTS ( 'NONE', 3,
 ( #25603, #51266, #13415, #44130 ),
 .UNSPECIFIED., .F., .F.,
 ( 4, 4 ),
 ( 1.999999999910059834E-07, 0.006970199999999934261 ),
 .UNSPECIFIED. ) ;
#49153=CARTESIAN_POINT ( 'NONE',  ( 0.7349081364829403995, 0.1283753931104748280, 0.1820866141732283561 ) ) ;
#49156=CARTESIAN_POINT ( 'NONE',  ( 0.09842519685039434474, -0.4536011799217368745, -0.2665933059059886201 ) ) ;
#49157=CARTESIAN_POINT ( 'NONE',  ( -0.4461942257217840213, -0.6046776061558809534, -0.2411417322834644161 ) ) ;
#49158=CARTESIAN_POINT ( 'NONE',  ( -0.04593175853018302557, 0.2952755905511811885, 0.1292274648535926551 ) ) ;
#49159=EDGE_LOOP ( 'NONE', ( #65722, #2151, #65449, #19221, #56910, #26156, #44678, #67500, #32668, #7939, #6505, #72025, #69026, #24709, #34551, #30955, #31760, #53497, #63534, #10768, #77811, #54449, #20389, #1947, #18800, #21727, #29872, #67372, #5562, #15811, #3109, #65126, #6267, #20088, #2079, #56622, #1739, #75334, #36428, #75274, #12462, #9195, #4033, #22247, #19329, #68000, #28574, #78681, #60838, #2485, #7548, #15199, #41047, #59592, #51526, #6686, #33943, #36601, #44080, #83279, #64906, #58018, #8675, #20023, #4552, #47491, #79527, #10345, #33858 ) ) ;
#49161=CARTESIAN_POINT ( 'NONE',  ( -0.5643044619422565855, 0.009842519685039144428, -0.3409548833797004797 ) ) ;
#49162=ORIENTED_EDGE ( 'NONE', *, *, #80402, .F. ) ;
#49165=CARTESIAN_POINT ( 'NONE',  ( -0.6430446194225716283, -0.3690944881889763329, 0.3153832671262228327 ) ) ;
#49166=CARTESIAN_POINT ( 'NONE',  ( -0.8398950131233589023, -0.6046776061558809534, -0.2411417322834644161 ) ) ;
#49168=EDGE_CURVE ( 'NONE', #3211, #21404, #66340, .T. ) ;
#49171=CARTESIAN_POINT ( 'NONE',  ( 1.292650918635171564, -0.6692913385826773087, -0.1292274648535924053 ) ) ;
#49172=CARTESIAN_POINT ( 'NONE',  ( 0.3412073490813655186, 0.2306618581243848609, 0.2411417322834645549 ) ) ;
#49173=CARTESIAN_POINT ( 'NONE',  ( 0.5971128608923891301, 0.2952755905511810774, -0.1292274648535930714 ) ) ;
#49174=CARTESIAN_POINT ( 'NONE',  ( -0.8595800524934373854, -0.08942795157527998196, 0.3641732283464567121 ) ) ;
#49175=AXIS2_PLACEMENT_3D ( 'NONE', #55593, #48878, #74578 ) ;
#49176=CARTESIAN_POINT ( 'NONE',  ( -0.2755905511811018171, 0.2952755905511811885, 0.000000000000000000 ) ) ;
#49178=CARTESIAN_POINT ( 'NONE',  ( -0.3346456692913377662, -0.5400638737290844871, 0.3530559997133364547 ) ) ;
#49181=CARTESIAN_POINT ( 'NONE',  ( 1.154855643044620184, 0.1283753931104746893, -0.1820866141732285504 ) ) ;
#49182=CARTESIAN_POINT ( 'NONE',  ( -0.2887139107611542133, 0.1283753931104748280, 0.1820866141732283561 ) ) ;
#49183=CARTESIAN_POINT ( 'NONE',  ( 1.318897637795276356, -0.4536011799217367080, 0.2665933059059888421 ) ) ;
#49184=CARTESIAN_POINT ( 'NONE',  ( -1.732283464566928277, -0.1870078740157479769, 0.4822834645669291653 ) ) ;
#49185=CARTESIAN_POINT ( 'NONE',  ( -1.200787401574802349, -0.4536011799217367080, 0.2665933059059888421 ) ) ;
#49186=FACE_OUTER_BOUND ( 'NONE', #50746, .T. ) ;
#49187=CARTESIAN_POINT ( 'NONE',  ( -1.299212598425196097, -0.6692913385826771977, 8.415575281601705876E-17 ) ) ;
#49188=CARTESIAN_POINT ( 'NONE',  ( -0.3871391076115476282, -0.05778040916215522460, 0.4822834645669289988 ) ) ;
#49192=CARTESIAN_POINT ( 'NONE',  ( 0.1312335958005257930, 0.1283753931104746893, -0.1820866141732285504 ) ) ;
#49193=CARTESIAN_POINT ( 'NONE',  ( -1.469816272965878357, -0.5023911411419708095, -0.1820866141732282451 ) ) ;
#49194=CARTESIAN_POINT ( 'NONE',  ( 0.9055118110236227702, 0.2952755905511811885, 0.000000000000000000 ) ) ;
#49195=CARTESIAN_POINT ( 'NONE',  ( -1.673228346456691717, 0.07958543189024071263, -0.2665933059059888421 ) ) ;
#49196=CARTESIAN_POINT ( 'NONE',  ( 1.404199475065617264, -0.3690944881889763329, 0.3153832671262228327 ) ) ;
#49197=CARTESIAN_POINT ( 'NONE',  ( -0.8267716535433065062, -0.6692913385826771977, 8.415575281601705876E-17 ) ) ;
#49198=CARTESIAN_POINT ( 'NONE',  ( -0.4724409448818890911, -0.1870078740157480601, -0.3641732283464567677 ) ) ;
#49200=CARTESIAN_POINT ( 'NONE',  ( 0.1837270341207354329, 0.1283753931104748280, 0.1820866141732283561 ) ) ;
#49201=CARTESIAN_POINT ( 'NONE',  ( 0.09186351706036827158, 0.05413385826771666132, 0.4176697321401328100 ) ) ;
#49204=CARTESIAN_POINT ( 'NONE',  ( 0.5577427821522314977, -0.2845877964562161244, -0.3641732283464567121 ) ) ;
#49205=CARTESIAN_POINT ( 'NONE',  ( 0.09842519685039434474, 0.1660481256975885056, 0.3530559997133364547 ) ) ;
#49206=CARTESIAN_POINT ( 'NONE',  ( -0.7677165354330699465, -0.5400638737290845981, -0.3530559997133363437 ) ) ;
#49207=CARTESIAN_POINT ( 'NONE',  ( -0.7939632545931750718, -0.08942795157528024563, -0.3641732283464568787 ) ) ;
#49208=CARTESIAN_POINT ( 'NONE',  ( 0.9973753280839902091, 0.1539470093639521697, -0.1968503937007875793 ) ) ;
#49209=CARTESIAN_POINT ( 'NONE',  ( -0.2887139107611542133, -0.5023911411419708095, -0.1820866141732282451 ) ) ;
#49210=CARTESIAN_POINT ( 'NONE',  ( -0.06561679790026180015, 0.05413385826771666132, 0.4176697321401328100 ) ) ;
#49211=CARTESIAN_POINT ( 'NONE',  ( -1.325459317585300889, -0.3690944881889765550, -0.3153832671262227771 ) ) ;
#49213=CARTESIAN_POINT ( 'NONE',  ( -1.640419947506561060, 0.05413385826771666132, 0.4176697321401328100 ) ) ;
#49215=ORIENTED_EDGE ( 'NONE', *, *, #5901, .F. ) ;
#49216=CARTESIAN_POINT ( 'NONE',  ( -1.541994750656167090, 0.1771653543307087630, 0.09757992244046791164 ) ) ;
#49217=CARTESIAN_POINT ( 'NONE',  ( -0.3215223097112853146, -0.3162353388693405765, 0.4822834645669290543 ) ) ;
#49218=CARTESIAN_POINT ( 'NONE',  ( -0.9973753280839886548, 0.2306618581243848609, 0.2411417322834645549 ) ) ;
#49221=CARTESIAN_POINT ( 'NONE',  ( 1.207349081364829990, 0.2306618581243848609, 0.2411417322834645549 ) ) ;
#49222=CARTESIAN_POINT ( 'NONE',  ( 0.4265091863517067594, 0.2952755905511811885, 0.1292274648535926551 ) ) ;
#49226=CIRCLE ( 'NONE', #76159, 2.362204724409449064 ) ;
#49227=CARTESIAN_POINT ( 'NONE',  ( -1.732283464566928277, -0.1870078740157479769, 0.4822834645669291653 ) ) ;
#49231=CARTESIAN_POINT ( 'NONE',  ( -0.7677165354330699465, -0.4536011799217368745, -0.2665933059059886201 ) ) ;
#49233=ORIENTED_EDGE ( 'NONE', *, *, #31679, .F. ) ;
#49234=CARTESIAN_POINT ( 'NONE',  ( 0.3018372703412079971, -0.4281496062992124485, 0.4176697321401328655 ) ) ;
#49235=CARTESIAN_POINT ( 'NONE',  ( -0.4396325459317579898, 0.2952755905511811885, 0.1292274648535926551 ) ) ;
#49236=CARTESIAN_POINT ( 'NONE',  ( -1.161417322834644716, 0.1660481256975885056, 0.3530559997133364547 ) ) ;
#49237=CARTESIAN_POINT ( 'NONE',  ( 0.8792650918635177559, 0.05413385826771666132, 0.4176697321401328100 ) ) ;
#49238=CARTESIAN_POINT ( 'NONE',  ( -1.417322834645668772, -0.1870078740157480601, -0.3641732283464567677 ) ) ;
#49239=CARTESIAN_POINT ( 'NONE',  ( 1.092343761084409559, 1.535433070866141447, 0.6033564923654649581 ) ) ;
#49240=CARTESIAN_POINT ( 'NONE',  ( -0.01968503937007793844, 0.1660481256975883668, -0.3530559997133364547 ) ) ;
#49241=CARTESIAN_POINT ( 'NONE',  ( -1.207349081364828436, -0.6046776061558807314, 0.2411417322834647770 ) ) ;
#49243=CARTESIAN_POINT ( 'NONE',  ( -1.587926509186350810, 0.05413385826771626580, -0.4176697321401330321 ) ) ;
#49246=CARTESIAN_POINT ( 'NONE',  ( 0.8923884514435703741, 0.1283753931104748280, 0.1820866141732283561 ) ) ;
#49247=ORIENTED_EDGE ( 'NONE', *, *, #82686, .T. ) ;
#49249=CARTESIAN_POINT ( 'NONE',  ( -0.9842519685039360366, 0.2952755905511811885, 0.000000000000000000 ) ) ;
#49250=ORIENTED_EDGE ( 'NONE', *, *, #67975, .F. ) ;
#49251=CARTESIAN_POINT ( 'NONE',  ( 0.01312335958005323398, -0.004921259842519576551, 0.3153832671262227771 ) ) ;
#49253=CARTESIAN_POINT ( 'NONE',  ( -1.469816272965878357, -0.6046776061558809534, -0.2411417322834644161 ) ) ;
#49254=CARTESIAN_POINT ( 'NONE',  ( 0.7349081364829402885, -0.6046776061558809534, -0.2411417322834644161 ) ) ;
#49255=CARTESIAN_POINT ( 'NONE',  ( 0.3543307086614179147, 0.2952755905511811885, 0.000000000000000000 ) ) ;
#49256=CARTESIAN_POINT ( 'NONE',  ( -0.2624671916010490880, 0.2306618581243847221, -0.2411417322834647770 ) ) ;
#49258=CARTESIAN_POINT ( 'NONE',  ( -0.9908136482939626788, 0.2952755905511811885, 0.1292274648535926551 ) ) ;
#49260=CARTESIAN_POINT ( 'NONE',  ( 1.496062992125984703, -0.1870078740157480601, -0.3641732283464567677 ) ) ;
#49261=CARTESIAN_POINT ( 'NONE',  ( -1.030183727034119867, -0.3162353388693405765, 0.4822834645669290543 ) ) ;
#49262=CARTESIAN_POINT ( 'NONE',  ( 0.8923884514435703741, 0.2306618581243848609, 0.2411417322834645549 ) ) ;
#49263=CARTESIAN_POINT ( 'NONE',  ( 1.332020997375329197, -0.3162353388693405765, 0.4822834645669290543 ) ) ;
#49265=CARTESIAN_POINT ( 'NONE',  ( -0.8005249343832013809, -0.4281496062992124485, 0.4176697321401328655 ) ) ;
#49267=CARTESIAN_POINT ( 'NONE',  ( 0.2296587926509192634, -0.05778040916215560624, -0.4822834645669293319 ) ) ;
#49269=CARTESIAN_POINT ( 'NONE',  ( -0.7020997375328074108, -0.05778040916215522460, 0.4822834645669289988 ) ) ;
#49270=CARTESIAN_POINT ( 'NONE',  ( -1.653543307086613234, -0.1870078740157479769, 0.3641732283464567677 ) ) ;
#49271=CARTESIAN_POINT ( 'NONE',  ( 0.6955380577427828781, -0.3690944881889763329, 0.3153832671262228327 ) ) ;
#49272=CARTESIAN_POINT ( 'NONE',  ( 1.515748031496063186, -0.5400638737290845981, -0.3530559997133363437 ) ) ;
#49274=CARTESIAN_POINT ( 'NONE',  ( 0.8333333333333340365, -0.5511811023622046335, 0.09757992244046803654 ) ) ;
#49275=CARTESIAN_POINT ( 'NONE',  ( 0.9776902887139113929, 0.2952755905511811885, 0.1292274648535926551 ) ) ;
#49277=CARTESIAN_POINT ( 'NONE',  ( -0.8333333333333323711, -0.6692913385826773087, -0.1292274648535924053 ) ) ;
#49279=CARTESIAN_POINT ( 'NONE',  ( 0.9120734908136489683, -0.5511811023622046335, 0.09757992244046803654 ) ) ;
#49280=CARTESIAN_POINT ( 'NONE',  ( -0.5052493438320203589, -0.6692913385826771977, 0.1292274648535927661 ) ) ;
#49281=CARTESIAN_POINT ( 'NONE',  ( -0.06561679790026180015, -0.4281496062992127816, -0.4176697321401328100 ) ) ;
#49282=CARTESIAN_POINT ( 'NONE',  ( 0.1447075906223747321, 0.004960608223779807216, -0.3437734562760184631 ) ) ;
#49283=CARTESIAN_POINT ( 'NONE',  ( 0.1377952755905518800, -0.5400638737290844871, 0.3530559997133364547 ) ) ;
#49284=CARTESIAN_POINT ( 'NONE',  ( 0.2952755905511819101, 0.07958543189024071263, -0.2665933059059888421 ) ) ;
#49286=CARTESIAN_POINT ( 'NONE',  ( -0.09842519685039295696, -0.4536011799217367080, 0.2665933059059888421 ) ) ;
#49287=CARTESIAN_POINT ( 'NONE',  ( 0.6036745406824153282, -0.5023911411419708095, 0.1820866141732285504 ) ) ;
#49290=CARTESIAN_POINT ( 'NONE',  ( 0.5380577427821529035, -0.4281496062992124485, 0.4176697321401328655 ) ) ;
#49291=AXIS2_PLACEMENT_3D ( 'NONE', #35530, #43063, #61192 ) ;
#49296=CARTESIAN_POINT ( 'NONE',  ( -0.2952755905511804668, 0.07958543189024085140, 0.2665933059059887866 ) ) ;
#49297=CARTESIAN_POINT ( 'NONE',  ( -0.4790026246719152336, -0.05778040916215560624, -0.4822834645669293319 ) ) ;
#49298=CARTESIAN_POINT ( 'NONE',  ( 1.128608923884515169, -0.5023911411419708095, -0.1820866141732282451 ) ) ;
#49299=CARTESIAN_POINT ( 'NONE',  ( -1.706036745406823485, 0.1283753931104748280, 0.1820866141732283561 ) ) ;
#49300=CARTESIAN_POINT ( 'NONE',  ( -1.391076115485563758, 0.2306618581243848609, 0.2411417322834645549 ) ) ;
#49301=CARTESIAN_POINT ( 'NONE',  ( -0.03280839895013062252, 0.2952755905511810774, -0.1292274648535930714 ) ) ;
#49302=CARTESIAN_POINT ( 'NONE',  ( 0.9842519685039378130, -0.6692913385826771977, 8.415575281601705876E-17 ) ) ;
#49304=CARTESIAN_POINT ( 'NONE',  ( 0.2624671916010504757, -0.6046776061558809534, -0.2411417322834644161 ) ) ;
#49305=CARTESIAN_POINT ( 'NONE',  ( 1.469816272965879911, -0.6046776061558807314, 0.2411417322834647770 ) ) ;
#49306=CARTESIAN_POINT ( 'NONE',  ( 0.3543307086614181922, -0.6692913385826771977, 8.415575281601705876E-17 ) ) ;
#49308=CARTESIAN_POINT ( 'NONE',  ( 0.9580052493438327987, -0.3690944881889765550, -0.3153832671262227771 ) ) ;
#49309=CARTESIAN_POINT ( 'NONE',  ( 1.633858267716535639, -0.5400638737290844871, 0.3530559997133364547 ) ) ;
#49310=CARTESIAN_POINT ( 'NONE',  ( 0.2034120734908142214, 0.1771653543307087075, -0.09757992244046823083 ) ) ;
#49311=CARTESIAN_POINT ( 'NONE',  ( -0.1574803149606292529, -0.1870078740157480879, -0.4822834645669291653 ) ) ;
#49312=CARTESIAN_POINT ( 'NONE',  ( 0.5708661417322841158, -0.5400638737290845981, -0.3530559997133363437 ) ) ;
#49313=B_SPLINE_CURVE_WITH_KNOTS ( 'NONE', 3,
 ( #25869, #51531, #53201, #78499, #27126, #39335, #19563 ),
 .UNSPECIFIED., .F., .F.,
 ( 4, 3, 4 ),
 ( 1.561251128379126385E-17, 0.001246230184515585400, 0.002492489877932649832 ),
 .UNSPECIFIED. ) ;
#49314=CARTESIAN_POINT ( 'NONE',  ( -0.4724409448818890911, -0.1870078740157480879, -0.4822834645669291653 ) ) ;
#49316=CARTESIAN_POINT ( 'NONE',  ( -0.3740157480314953431, -0.4536011799217368745, -0.2665933059059886201 ) ) ;
#49317=CARTESIAN_POINT ( 'NONE',  ( 0.6233595800524939223, -0.3162353388693405765, 0.4822834645669290543 ) ) ;
#49318=CARTESIAN_POINT ( 'NONE',  ( 0.8333333333333340365, -0.5511811023622046335, 0.09757992244046803654 ) ) ;
#49319=CARTESIAN_POINT ( 'NONE',  ( 0.2296587926509192634, -0.3162353388693405765, 0.4822834645669290543 ) ) ;
#49324=CARTESIAN_POINT ( 'NONE',  ( -1.246719160104985846, -0.4281496062992127816, -0.4176697321401328100 ) ) ;
#49325=CARTESIAN_POINT ( 'NONE',  ( -0.3083989501312330295, -0.05778040916215522460, 0.4822834645669289988 ) ) ;
#49328=VERTEX_POINT ( 'NONE', #50979 ) ;
#49329=CARTESIAN_POINT ( 'NONE',  ( 0.2362204724409456558, -0.1870078740157479769, 0.3641732283464567677 ) ) ;
#49331=EDGE_CURVE ( 'NONE', #65960, #19643, #5557, .T. ) ;
#49332=CARTESIAN_POINT ( 'NONE',  ( 0.5643044619422579178, -0.4281496062992127816, -0.4176697321401328100 ) ) ;
#49336=FACE_OUTER_BOUND ( 'NONE', #43505, .T. ) ;
#49337=CARTESIAN_POINT ( 'NONE',  ( 1.174540682414699111, -0.08942795157528024563, -0.3641732283464568787 ) ) ;
#49338=CARTESIAN_POINT ( 'NONE',  ( 0.5577427821522316087, -0.05778040916215522460, 0.4822834645669289988 ) ) ;
#49340=CARTESIAN_POINT ( 'NONE',  ( -0.5314960629921250401, 0.1660481256975885056, 0.3530559997133364547 ) ) ;
#49341=CARTESIAN_POINT ( 'NONE',  ( -1.030183727034119867, -0.08942795157528024563, -0.3641732283464568787 ) ) ;
#49342=CARTESIAN_POINT ( 'NONE',  ( 0.2690288713910767848, -0.6692913385826773087, -0.1292274648535924053 ) ) ;
#49343=CARTESIAN_POINT ( 'NONE',  ( -0.08530183727034056085, -0.05778040916215560624, -0.4822834645669293319 ) ) ;
#49344=CARTESIAN_POINT ( 'NONE',  ( 0.5052493438320215802, 0.2952755905511811885, 0.1292274648535926551 ) ) ;
#49348=CARTESIAN_POINT ( 'NONE',  ( 0.6299212598425204535, -0.1870078740157480879, -0.4822834645669291653 ) ) ;
#49350=AXIS2_PLACEMENT_3D ( 'NONE', #55179, #24024, #4261 ) ;
#49351=CARTESIAN_POINT ( 'NONE',  ( -0.1968503937007867743, -0.6692913385826771977, 8.415575281601705876E-17 ) ) ;
#49352=CARTESIAN_POINT ( 'NONE',  ( -1.292650918635170010, 0.2952755905511810774, -0.1292274648535930714 ) ) ;
#49353=CARTESIAN_POINT ( 'NONE',  ( 1.305774278215223960, 0.2952755905511810774, -0.1292274648535930714 ) ) ;
#49354=CARTESIAN_POINT ( 'NONE',  ( 0.3477690288713918276, -0.6692913385826773087, -0.1292274648535924053 ) ) ;
#49356=CARTESIAN_POINT ( 'NONE',  ( -0.6692913385826764205, -0.6692913385826771977, 8.415575281601705876E-17 ) ) ;
#49357=CARTESIAN_POINT ( 'NONE',  ( 0.07217847769028949700, -0.3162353388693405765, 0.4822834645669290543 ) ) ;
#49358=CARTESIAN_POINT ( 'NONE',  ( -0.4855643044619415427, 0.05413385826771626580, -0.4176697321401330321 ) ) ;
#49359=CARTESIAN_POINT ( 'NONE',  ( 0.4724409448818904789, -0.1870078740157480601, -0.3641732283464567677 ) ) ;
#49360=CARTESIAN_POINT ( 'NONE',  ( 1.587926509186352586, -0.3690944881889765550, -0.3153832671262227771 ) ) ;
#49362=CARTESIAN_POINT ( 'NONE',  ( 0.2427821522309716595, -0.3162353388693409650, -0.4822834645669289433 ) ) ;
#49364=CARTESIAN_POINT ( 'NONE',  ( -1.535433070866141225, -0.6692913385826771977, 8.415575281601705876E-17 ) ) ;
#49368=CARTESIAN_POINT ( 'NONE',  ( 0.5118110236220480003, -0.6692913385826771977, 8.415575281601705876E-17 ) ) ;
#49369=CARTESIAN_POINT ( 'NONE',  ( 0.1312335958005255154, -0.5023911411419708095, 0.1820866141732285504 ) ) ;
#49376=CARTESIAN_POINT ( 'NONE',  ( 0.4396325459317590445, -0.6692913385826771977, 0.1292274648535927661 ) ) ;
#49377=CARTESIAN_POINT ( 'NONE',  ( -0.9448818897637790704, -0.1870078740157480879, -0.4822834645669291653 ) ) ;
#49378=CARTESIAN_POINT ( 'NONE',  ( -0.9186351706036736120, 0.2306618581243848609, 0.2411417322834645549 ) ) ;
#49379=CARTESIAN_POINT ( 'NONE',  ( 0.6364829396325465405, -0.05778040916215522460, 0.4822834645669289988 ) ) ;
#49380=CARTESIAN_POINT ( 'NONE',  ( 1.548556430446194954, -0.6046776061558807314, 0.2411417322834647770 ) ) ;
#49381=CARTESIAN_POINT ( 'NONE',  ( 1.187664041994751285, -0.08942795157527998196, 0.3641732283464567121 ) ) ;
#49383=CARTESIAN_POINT ( 'NONE',  ( 1.266404199475066328, -0.2845877964562161244, -0.3641732283464567121 ) ) ;
#49384=CARTESIAN_POINT ( 'NONE',  ( -0.7939632545931750718, -0.05778040916215560624, -0.4822834645669293319 ) ) ;
#49386=CARTESIAN_POINT ( 'NONE',  ( 1.456692913385827515, -0.6692913385826771977, 8.415575281601705876E-17 ) ) ;
#49388=CARTESIAN_POINT ( 'NONE',  ( -0.1837270341207340729, 0.2306618581243847221, -0.2411417322834647770 ) ) ;
#49390=CARTESIAN_POINT ( 'NONE',  ( 1.207349081364829990, 0.2306618581243848609, 0.2411417322834645549 ) ) ;
#49392=CARTESIAN_POINT ( 'NONE',  ( -0.9973753280839886548, -0.5023911411419708095, -0.1820866141732282451 ) ) ;
#49393=CARTESIAN_POINT ( 'NONE',  ( 0.5118110236220480003, -0.6692913385826771977, 8.415575281601705876E-17 ) ) ;
#49394=CARTESIAN_POINT ( 'NONE',  ( 0.8530183727034126306, -0.004921259842519870586, -0.3153832671262229437 ) ) ;
#49396=CARTESIAN_POINT ( 'NONE',  ( -1.371391076115484831, 0.1771653543307087075, -0.09757992244046823083 ) ) ;
#49397=CARTESIAN_POINT ( 'NONE',  ( 1.502624671916010790, -0.05778040916215522460, 0.4822834645669289988 ) ) ;
#49399=CARTESIAN_POINT ( 'NONE',  ( 0.03280839895013198948, 0.1771653543307087630, 0.09757992244046791164 ) ) ;
#49400=CARTESIAN_POINT ( 'NONE',  ( -0.1968503937007867743, -0.6692913385826771977, 8.415575281601705876E-17 ) ) ;
#49401=CARTESIAN_POINT ( 'NONE',  ( -1.430446194225720724, -0.004921259842519870586, -0.3153832671262229437 ) ) ;
#49402=CARTESIAN_POINT ( 'NONE',  ( -0.5643044619422565855, 0.05413385826771626580, -0.4176697321401330321 ) ) ;
#49403=CARTESIAN_POINT ( 'NONE',  ( 1.417322834645670104, -0.1870078740157480879, -0.4822834645669291653 ) ) ;
#49405=CARTESIAN_POINT ( 'NONE',  ( -0.8136482939632537770, 0.1283753931104746893, -0.1820866141732285504 ) ) ;
#49406=( BOUNDED_SURFACE ( )  B_SPLINE_SURFACE ( 1, 2, ( 
 ( #34635, #72521, #21580, #40114, #60299, #8135, #2649, #27478, #53136, #78847, #14870, #40531, #66210, #47243, #72932, #15283, #40944, #66623, #65237, #46268, #6304, #26078, #77440, #20616, #12632, #20192, #32816, #31980, #82921, #18937, #78285, #76607, #51738, #50906, #19354, #13889, #70279, #6723, #52576, #57641, #32393, #51318, #70702, #13466, #58056, #4, #37881, #7143, #26505, #52158, #33247, #77021, #7574, #58908, #38291, #44585, #422, #71123, #63967, #25656, #45003, #1268, #26916, #25241, #13055, #58483, #45843, #19774, #64804, #38708, #39123, #64387, #57219, #45427, #848, #77863, #71542, #39548, #12224, #63556, #5890, #31562, #39976, #35317, #14317, #22684, #67313, #66480, #9236, #27332, #41624, #8815, #9648, #71963, #65665, #7992, #73208, #78705, #33656, #59319, #1675, #21852, #34908, #47931, #52992, #66067, #79539, #21029, #46689, #72789, #3330, #73635, #47100, #34491, #72382, #14732, #60157, #54242, #8403, #40384, #66905, #60980, #28586, #47516, #53825, #2088, #34070, #2509, #27753, #15558, #41217, #28168, #59734, #15139, #53417, #28994, #79126, #60571, #21443, #40795, #2922, #79959, #22272, #15977, #54660, #80371, #55478, #62641, #74877, #31053, #49998, #48759, #63053, #30232, #43258, #74458, #74040, #55068, #10486, #30652, #56316, #11726, #10063, #36140, #23505, #29409, #82014, #68955, #80776, #56722, #24328, #3745, #81188, #23092, #75695, #16387, #61396, #18036, #4152, #37382, #81606, #29817, #82419, #42441, #62223, #55894, #48343, #16805, #43670, #11305, #68141, #35726, #61812, #42034, #49172, #4561, #17221, #42853, #69373, #68546, #10887, #5391, #36547, #23922, #49588, #75283, #17626, #36964, #4985, #67728, #330, #61918, #37066, #10593, #80887, #68257, #83242, #68652, #30755, #49691, #23200, #10990, #35843, #57551, #3857, #25984, #61512, #71033, #32302, #30336, #25564, #74571, #6630, #56002, #57963, #29517, #55178, #48871, #62751, #42554, #16916, #36249, #4260, #69061, #51230, #12961, #29923, #55586, #43360, #81298, #23612, #36651, #51642, #38618, #62326, #81713, #49281, #74984, #24023, #19256, #17329, #42959, #76929, #77347, #44908, #11411, #17732, #4663, #75385, #5087, #70606, #64296, #19678, #45337, #58819, #71872, #751, #28075, #26827, #8312, #52485, #39030, #72292, #47423, #47006, #27242, #20524, #7055, #46176, #27659, #39882, #79441, #15047, #13798, #53733, #78614, #33979, #39456, #64714, #20104, #1176, #79034, #21353, #60064, #58390, #78193, #14222, #77772, #72700, #65569, #45754, #7903, #21760, #33564, #65975, #20938, #40703, #71450, #59226, #26412, #13377, #66387, #8725, #65143, #1587, #2418, #7480, #32723, #52065, #52901, #14638, #34396, #46596, #40294, #1996, #59640, #33150, #53325, #2828, #55389, #35638, #36050, #16708, #79863, #15887, #35225, #61723, #54149, #23002, #4060, #42762, #81095, #22180, #60889, #68047, #23412, #68458, #15465, #49078, #73114, #41536, #28489, #16297, #22594, #48255, #74779, #10796, #29320, #54981, #29727, #80689, #73544, #73951, #36456, #3657, #42349, #9967, #30138, #41123, #62130, #4470, #55800, #3239, #60477, #48668, #47838, #17130, #81507, #23829, #66814, #67223, #74365, #10394, #9147, #9555, #34819, #28903, #54566, #80281, #41940, #67636, #61299, #63364, #4884, #56626, #51128, #24233, #43995, #6533, #11626, #69689, #5300, #24645, #50723, #12032, #37689, #25048, #43166, #18750, #6114, #70500, #30959, #19154, #12858, #32203, #76822, #44394, #31369, #43578, #11211, #36870, #82326, #62962, #57860, #38516, #227, #82729, #12439, #50312, #70086, #5698, #62547, #76010, #49497, #38099, #17534, #64199, #75190, #68862, #44805, #57034, #63773, #30558, #56224, #76421, #81922, #49905, #75603, #17942, #31786, #69280, #37287, #25461, #18352, #57449, #83141, #14941, #6946, #19572, #8622, #14114, #27134, #46900, #39767, #7365, #14537, #65462, #59954, #40600, #38929, #8207, #71761, #72179, #52798, #32617, #51960, #71343, #40188, #58279, #59123, #65872, #78923, #33872, #644, #13690, #20831, #59536, #21245, #51539, #1893, #25877, #77666, #64609, #52376, #58703, #1069, #27553, #72594, #7795, #33461, #53212 ),
 ( #39344, #26722, #26301, #66282, #46484, #19997, #34293, #77242, #45648, #78084, #65030, #45231, #70932, #33035, #13277, #20416, #46068, #1480, #78508, #60373, #41019, #73849, #61195, #2721, #22072, #28382, #74678, #55286, #73006, #47732, #42663, #60783, #29626, #48979, #54042, #3551, #79755, #47316, #34712, #15358, #79336, #22491, #67943, #73430, #9038, #80589, #80996, #42248, #35533, #67526, #15780, #41432, #80176, #67115, #29217, #9863, #16189, #9446, #3135, #66705, #17024, #35117, #22896, #28799, #27970, #54884, #36355, #35951, #41836, #54462, #21656, #48154, #16604, #48564, #68361, #3963, #74262, #10700, #10285, #61621, #23309, #53628, #2309, #24132, #44298, #69989, #25366, #23723, #49801, #37181, #43066, #12344, #82632, #68763, #44708, #38000, #17435, #11524, #11107, #63676, #30035, #75088, #6017, #17842, #51029, #11934, #43477, #36763, #62439, #50212, #37589, #4776, #81822, #30452, #76728, #31688, #49394, #75503, #19060, #62860, #57347, #70404, #56116, #63262, #69173, #5196, #30861, #24946, #56526, #56936, #75910, #82228, #24548, #62031, #50619, #55698, #12760, #4367, #81406, #83043, #18249, #76324, #43891, #69588, #5603, #31270, #18654, #52286, #8116, #64513, #45131, #38418, #72503, #127, #71668, #59034, #14445, #19479, #32520, #45973, #70836, #77146, #39251, #53119, #40096, #13597, #58610, #32106, #21156, #26632, #39677, #59445, #77991, #19905, #27042, #20320, #64099, #78830, #51443, #20742, #978, #1389, #65369, #13184, #6850, #551, #52703, #38834, #14019, #78413, #33782, #46393, #58182, #26204, #33371, #72087, #1798, #6435, #65784, #57765, #51867, #77572, #64933, #71251, #7272, #27460, #46812, #7704, #25782, #45554, #32944, #15266, #15686, #67852, #28707, #67434, #35028, #55193, #14852, #61525, #3871, #80900, #28289, #2214, #22401, #79248, #80493, #29530, #10191, #48884, #8943, #54369, #80081, #23214, #40926, #22809, #35439, #34619, #27880, #21563, #40512, #47225, #48058, #53540, #21980, #16514, #72914, #9357, #66193, #60283, #60692, #53951, #73337, #16095, #3042, #73760, #41740, #8529, #9768, #54790, #35859, #79664, #34196, #59861, #66607, #42157, #61104, #3456, #2633, #47642, #41344, #67024, #29122, #48466, #74167, #25263, #24444, #43375, #55600, #69075, #5912, #62339, #43784, #36665, #82129, #37901, #63167, #61932, #57241, #50518, #44201, #49296, #49704, #63577, #81311, #68667, #5100, #56428, #82945, #74997, #82532, #11839, #11006, #4275, #23625, #74584, #17342, #30767, #29936, #81726, #76224, #42971, #11424, #31585, #4677, #37079, #30349, #75400, #75809, #62766, #50112, #18151, #68270, #69490, #31167, #12245, #56018, #69891, #16929, #42569, #18557, #37492, #5505, #24035, #36263, #17746, #56834, #24850, #10606, #14340, #1698, #871, #19801, #32004, #45450, #65688, #38733, #20218, #13080, #58508, #40000, #39572, #38315, #33679, #26939, #20639, #25679, #26100, #8015, #57664, #44606, #59341, #39145, #52183, #71987, #64829, #32417, #65262, #7168, #50929, #76627, #63990, #33272, #13489, #13915, #77887, #26, #77043, #64410, #7598, #51339, #26529, #58931, #46291, #1290, #19375, #6745, #45867, #52601, #18958, #70302, #78307, #12654, #45025, #6331, #77463, #445, #51761, #70726, #58079, #32839, #71565, #71148, #9259, #27776, #28190, #80394, #41239, #79980, #47540, #67751, #27356, #74063, #16409, #10085, #40819, #14754, #34931, #8425, #9670, #42055, #22706, #61416, #29017, #2532, #73230, #40408, #21053, #15581, #35340, #47123, #34093, #22293, #48364, #67337, #60593, #2943, #66503, #2111, #21874, #8838, #28607, #54264, #66927, #72812, #53848, #66090, #35749, #34514, #47954, #60179, #53015, #73657, #78729, #61003, #15999, #79561, #46713, #41646, #3351, #54682, #72405, #59756, #53440, #79148, #21465, #15162, #4172, #29430, #10505, #49193, #69391, #11744, #50422, #48780, #74894, #62241, #68161, #37400, #24346, #36158, #69799, #63072, #42462, #36564, #61832, #5409, #55088, #16826, #31070, #42870, #76122, #36981, #68564, #29836, #55499, #75300, #62662, #81208, #23523, #17242, #18463, #56739, #74479, #10906, #44107, #4579, #82436, #12146, #30250, #5002 ) ),
 .UNSPECIFIED., .F., .F., .F. ) 
 B_SPLINE_SURFACE_WITH_KNOTS ( ( 2, 2 ),
 ( 3, 2, 2, 2, 2, 2, 2, 2, 2, 2, 2, 2, 2, 2, 2, 2, 2, 2, 2, 2, 2, 2, 2, 2, 2, 2, 2, 2, 2, 2, 2, 2, 2, 2, 2, 2, 2, 2, 2, 2, 2, 2, 2, 2, 2, 2, 2, 2, 2, 2, 2, 2, 2, 2, 2, 2, 2, 2, 2, 2, 2, 2, 2, 2, 2, 2, 2, 2, 2, 2, 2, 2, 2, 2, 2, 2, 2, 2, 2, 2, 2, 2, 2, 2, 2, 2, 2, 2, 2, 2, 2, 2, 2, 2, 2, 2, 2, 2, 2, 2, 2, 2, 2, 2, 2, 2, 2, 2, 2, 2, 2, 2, 2, 2, 2, 2, 2, 2, 2, 2, 2, 2, 2, 2, 2, 2, 2, 2, 2, 2, 2, 2, 2, 2, 2, 2, 2, 2, 2, 2, 2, 2, 2, 2, 2, 2, 2, 2, 2, 2, 2, 2, 2, 2, 2, 2, 2, 2, 2, 2, 2, 2, 2, 2, 2, 2, 2, 2, 2, 2, 2, 2, 2, 2, 2, 2, 2, 2, 2, 2, 2, 2, 2, 2, 2, 2, 2, 2, 2, 2, 2, 2, 2, 2, 2, 2, 2, 2, 2, 2, 2, 2, 2, 2, 2, 2, 2, 2, 2, 2, 2, 2, 2, 2, 2, 2, 2, 2, 2, 2, 2, 2, 2, 2, 2, 2, 2, 2, 2, 2, 2, 2, 2, 2, 2, 2, 2, 2, 2, 2, 2, 2, 2, 2, 2, 2, 2, 2, 2, 2, 2, 2, 2, 2, 2, 3 ),
 ( 0.000000000000000000, 1.000000000000000000 ),
 ( 0.000000000000000000, 0.003787878787878787984, 0.007575757575757575968, 0.01136363636363636395, 0.01515151515151515194, 0.01893939393939393992, 0.02272727272727272790, 0.02651515151515151589, 0.03030303030303030387, 0.03409090909090908839, 0.03787878787878787984, 0.04166666666666666435, 0.04545454545454545581, 0.04924242424242424032, 0.05303030303030303177, 0.05681818181818181629, 0.06060606060606060774, 0.06439393939393939226, 0.06818181818181817677, 0.07196969696969697516, 0.07575757575757575968, 0.07954545454545454419, 0.08333333333333332871, 0.08712121212121212710, 0.09090909090909091161, 0.09469696969696969613, 0.09848484848484848064, 0.1022727272727272790, 0.1060606060606060635, 0.1098484848484848481, 0.1136363636363636326, 0.1174242424242424310, 0.1212121212121212155, 0.1250000000000000000, 0.1287878787878787845, 0.1325757575757575690, 0.1363636363636363535, 0.1401515151515151381, 0.1439393939393939503, 0.1477272727272727348, 0.1515151515151515194, 0.1553030303030303039, 0.1590909090909090884, 0.1628787878787878729, 0.1666666666666666574, 0.1704545454545454419, 0.1742424242424242542, 0.1780303030303030387, 0.1818181818181818232, 0.1856060606060606077, 0.1893939393939393923, 0.1931818181818181768, 0.1969696969696969613, 0.2007575757575757458, 0.2045454545454545581, 0.2083333333333333426, 0.2121212121212121271, 0.2159090909090909116, 0.2196969696969696961, 0.2234848484848484806, 0.2272727272727272652, 0.2310606060606060497, 0.2348484848484848619, 0.2386363636363636465, 0.2424242424242424310, 0.2462121212121212155, 0.2500000000000000000, 0.2537878787878787845, 0.2575757575757575690, 0.2613636363636363535, 0.2651515151515151381, 0.2689393939393939226, 0.2727272727272727071, 0.2765151515151514916, 0.2803030303030302761, 0.2840909090909091161, 0.2878787878787879007, 0.2916666666666666852, 0.2954545454545454697, 0.2992424242424242542, 0.3030303030303030387, 0.3068181818181818232, 0.3106060606060606077, 0.3143939393939393923, 0.3181818181818181768, 0.3219696969696969613, 0.3257575757575757458, 0.3295454545454545303, 0.3333333333333333148, 0.3371212121212120993, 0.3409090909090908839, 0.3446969696969697239, 0.3484848484848485084, 0.3522727272727272929, 0.3560606060606060774, 0.3598484848484848619, 0.3636363636363636465, 0.3674242424242424310, 0.3712121212121212155, 0.3750000000000000000, 0.3787878787878787845, 0.3825757575757575690, 0.3863636363636363535, 0.3901515151515151381, 0.3939393939393939226, 0.3977272727272727071, 0.4015151515151514916, 0.4053030303030302761, 0.4090909090909091161, 0.4128787878787879007, 0.4166666666666666852, 0.4204545454545454697, 0.4242424242424242542, 0.4280303030303030387, 0.4318181818181818232, 0.4356060606060606077, 0.4393939393939393923, 0.4431818181818181768, 0.4469696969696969613, 0.4507575757575757458, 0.4545454545454545303, 0.4583333333333333148, 0.4621212121212120993, 0.4659090909090908839, 0.4696969696969697239, 0.4734848484848485084, 0.4772727272727272929, 0.4810606060606060774, 0.4848484848484848619, 0.4886363636363636465, 0.4924242424242424310, 0.4962121212121212155, 0.5000000000000000000, 0.5037878787878787845, 0.5075757575757575690, 0.5113636363636363535, 0.5151515151515151381, 0.5189393939393939226, 0.5227272727272727071, 0.5265151515151514916, 0.5303030303030302761, 0.5340909090909090606, 0.5378787878787878451, 0.5416666666666666297, 0.5454545454545454142, 0.5492424242424241987, 0.5530303030303029832, 0.5568181818181817677, 0.5606060606060605522, 0.5643939393939394478, 0.5681818181818182323, 0.5719696969696970168, 0.5757575757575758013, 0.5795454545454545858, 0.5833333333333333703, 0.5871212121212121549, 0.5909090909090909394, 0.5946969696969697239, 0.5984848484848485084, 0.6022727272727272929, 0.6060606060606060774, 0.6098484848484848619, 0.6136363636363636465, 0.6174242424242424310, 0.6212121212121212155, 0.6250000000000000000, 0.6287878787878787845, 0.6325757575757575690, 0.6363636363636363535, 0.6401515151515151381, 0.6439393939393939226, 0.6477272727272727071, 0.6515151515151514916, 0.6553030303030302761, 0.6590909090909090606, 0.6628787878787878451, 0.6666666666666666297, 0.6704545454545454142, 0.6742424242424241987, 0.6780303030303029832, 0.6818181818181817677, 0.6856060606060605522, 0.6893939393939394478, 0.6931818181818182323, 0.6969696969696970168, 0.7007575757575758013, 0.7045454545454545858, 0.7083333333333333703, 0.7121212121212121549, 0.7159090909090909394, 0.7196969696969697239, 0.7234848484848485084, 0.7272727272727272929, 0.7310606060606060774, 0.7348484848484848619, 0.7386363636363636465, 0.7424242424242424310, 0.7462121212121212155, 0.7500000000000000000, 0.7537878787878787845, 0.7575757575757575690, 0.7613636363636363535, 0.7651515151515151381, 0.7689393939393939226, 0.7727272727272727071, 0.7765151515151514916, 0.7803030303030302761, 0.7840909090909090606, 0.7878787878787878451, 0.7916666666666666297, 0.7954545454545454142, 0.7992424242424241987, 0.8030303030303029832, 0.8068181818181817677, 0.8106060606060605522, 0.8143939393939394478, 0.8181818181818182323, 0.8219696969696970168, 0.8257575757575758013, 0.8295454545454545858, 0.8333333333333333703, 0.8371212121212121549, 0.8409090909090909394, 0.8446969696969697239, 0.8484848484848485084, 0.8522727272727272929, 0.8560606060606060774, 0.8598484848484848619, 0.8636363636363636465, 0.8674242424242424310, 0.8712121212121212155, 0.8750000000000000000, 0.8787878787878787845, 0.8825757575757575690, 0.8863636363636363535, 0.8901515151515151381, 0.8939393939393939226, 0.8977272727272727071, 0.9015151515151514916, 0.9053030303030302761, 0.9090909090909090606, 0.9128787878787878451, 0.9166666666666666297, 0.9204545454545454142, 0.9242424242424241987, 0.9280303030303029832, 0.9318181818181817677, 0.9356060606060605522, 0.9393939393939394478, 0.9431818181818182323, 0.9469696969696970168, 0.9507575757575758013, 0.9545454545454545858, 0.9583333333333333703, 0.9621212121212121549, 0.9659090909090909394 ),
 .UNSPECIFIED. ) 
 GEOMETRIC_REPRESENTATION_ITEM ( )  RATIONAL_B_SPLINE_SURFACE ( (
 ( 1.000000000000000000, 0.9659258262890683122, 1.000000000000000000, 0.9659258262890683122, 1.000000000000000000, 0.9659258262890683122, 1.000000000000000000, 0.9659258262890683122, 1.000000000000000000, 0.9659258262890683122, 1.000000000000000000, 0.9659258262890683122, 1.000000000000000000, 0.9659258262890683122, 1.000000000000000000, 0.9659258262890683122, 1.000000000000000000, 0.9659258262890683122, 1.000000000000000000, 0.9659258262890683122, 1.000000000000000000, 0.9659258262890683122, 1.000000000000000000, 0.9659258262890683122, 1.000000000000000000, 0.9659258262890683122, 1.000000000000000000, 0.9659258262890683122, 1.000000000000000000, 0.9659258262890683122, 1.000000000000000000, 0.9659258262890683122, 1.000000000000000000, 0.9659258262890683122, 1.000000000000000000, 0.9659258262890683122, 1.000000000000000000, 0.9659258262890683122, 1.000000000000000000, 0.9659258262890683122, 1.000000000000000000, 0.9659258262890683122, 1.000000000000000000, 0.9659258262890683122, 1.000000000000000000, 0.9659258262890683122, 1.000000000000000000, 0.9659258262890683122, 1.000000000000000000, 0.9659258262890683122, 1.000000000000000000, 0.9659258262890683122, 1.000000000000000000, 0.9659258262890683122, 1.000000000000000000, 0.9659258262890683122, 1.000000000000000000, 0.9659258262890683122, 1.000000000000000000, 0.9659258262890683122, 1.000000000000000000, 0.9659258262890683122, 1.000000000000000000, 0.9659258262890683122, 1.000000000000000000, 0.9659258262890683122, 1.000000000000000000, 0.9659258262890683122, 1.000000000000000000, 0.9659258262890683122, 1.000000000000000000, 0.9659258262890683122, 1.000000000000000000, 0.9659258262890683122, 1.000000000000000000, 0.9659258262890683122, 1.000000000000000000, 0.9659258262890683122, 1.000000000000000000, 0.9659258262890683122, 1.000000000000000000, 0.9659258262890683122, 1.000000000000000000, 0.9659258262890683122, 1.000000000000000000, 0.9659258262890683122, 1.000000000000000000, 0.9659258262890683122, 1.000000000000000000, 0.9659258262890683122, 1.000000000000000000, 0.9659258262890683122, 1.000000000000000000, 0.9659258262890683122, 1.000000000000000000, 0.9659258262890683122, 1.000000000000000000, 0.9659258262890683122, 1.000000000000000000, 0.9659258262890683122, 1.000000000000000000, 0.9659258262890683122, 1.000000000000000000, 0.9659258262890683122, 1.000000000000000000, 0.9659258262890683122, 1.000000000000000000, 0.9659258262890683122, 1.000000000000000000, 0.9659258262890683122, 1.000000000000000000, 0.9659258262890683122, 1.000000000000000000, 0.9659258262890683122, 1.000000000000000000, 0.9659258262890683122, 1.000000000000000000, 0.9659258262890683122, 1.000000000000000000, 0.9659258262890683122, 1.000000000000000000, 0.9659258262890683122, 1.000000000000000000, 0.9659258262890683122, 1.000000000000000000, 0.9659258262890683122, 1.000000000000000000, 0.9659258262890683122, 1.000000000000000000, 0.9659258262890683122, 1.000000000000000000, 0.9659258262890683122, 1.000000000000000000, 0.9659258262890683122, 1.000000000000000000, 0.9659258262890683122, 1.000000000000000000, 0.9659258262890683122, 1.000000000000000000, 0.9659258262890683122, 1.000000000000000000, 0.9659258262890683122, 1.000000000000000000, 0.9659258262890683122, 1.000000000000000000, 0.9659258262890683122, 1.000000000000000000, 0.9659258262890683122, 1.000000000000000000, 0.9659258262890683122, 1.000000000000000000, 0.9659258262890683122, 1.000000000000000000, 0.9659258262890683122, 1.000000000000000000, 0.9659258262890683122, 1.000000000000000000, 0.9659258262890683122, 1.000000000000000000, 0.9659258262890683122, 1.000000000000000000, 0.9659258262890683122, 1.000000000000000000, 0.9659258262890683122, 1.000000000000000000, 0.9659258262890683122, 1.000000000000000000, 0.9659258262890683122, 1.000000000000000000, 0.9659258262890683122, 1.000000000000000000, 0.9659258262890683122, 1.000000000000000000, 0.9659258262890683122, 1.000000000000000000, 0.9659258262890683122, 1.000000000000000000, 0.9659258262890683122, 1.000000000000000000, 0.9659258262890683122, 1.000000000000000000, 0.9659258262890683122, 1.000000000000000000, 0.9659258262890683122, 1.000000000000000000, 0.9659258262890683122, 1.000000000000000000, 0.9659258262890683122, 1.000000000000000000, 0.9659258262890683122, 1.000000000000000000, 0.9659258262890683122, 1.000000000000000000, 0.9659258262890683122, 1.000000000000000000, 0.9659258262890683122, 1.000000000000000000, 0.9659258262890683122, 1.000000000000000000, 0.9659258262890683122, 1.000000000000000000, 0.9659258262890683122, 1.000000000000000000, 0.9659258262890683122, 1.000000000000000000, 0.9659258262890683122, 1.000000000000000000, 0.9659258262890683122, 1.000000000000000000, 0.9659258262890683122, 1.000000000000000000, 0.9659258262890683122, 1.000000000000000000, 0.9659258262890683122, 1.000000000000000000, 0.9659258262890683122, 1.000000000000000000, 0.9659258262890683122, 1.000000000000000000, 0.9659258262890683122, 1.000000000000000000, 0.9659258262890683122, 1.000000000000000000, 0.9659258262890683122, 1.000000000000000000, 0.9659258262890683122, 1.000000000000000000, 0.9659258262890683122, 1.000000000000000000, 0.9659258262890683122, 1.000000000000000000, 0.9659258262890683122, 1.000000000000000000, 0.9659258262890683122, 1.000000000000000000, 0.9659258262890683122, 1.000000000000000000, 0.9659258262890683122, 1.000000000000000000, 0.9659258262890683122, 1.000000000000000000, 0.9659258262890683122, 1.000000000000000000, 0.9659258262890683122, 1.000000000000000000, 0.9659258262890683122, 1.000000000000000000, 0.9659258262890683122, 1.000000000000000000, 0.9659258262890683122, 1.000000000000000000, 0.9659258262890683122, 1.000000000000000000, 0.9659258262890683122, 1.000000000000000000, 0.9659258262890683122, 1.000000000000000000, 0.9659258262890683122, 1.000000000000000000, 0.9659258262890683122, 1.000000000000000000, 0.9659258262890683122, 1.000000000000000000, 0.9659258262890683122, 1.000000000000000000, 0.9659258262890683122, 1.000000000000000000, 0.9659258262890683122, 1.000000000000000000, 0.9659258262890683122, 1.000000000000000000, 0.9659258262890683122, 1.000000000000000000, 0.9659258262890683122, 1.000000000000000000, 0.9659258262890683122, 1.000000000000000000, 0.9659258262890683122, 1.000000000000000000, 0.9659258262890683122, 1.000000000000000000, 0.9659258262890683122, 1.000000000000000000, 0.9659258262890683122, 1.000000000000000000, 0.9659258262890683122, 1.000000000000000000, 0.9659258262890683122, 1.000000000000000000, 0.9659258262890683122, 1.000000000000000000, 0.9659258262890683122, 1.000000000000000000, 0.9659258262890683122, 1.000000000000000000, 0.9659258262890683122, 1.000000000000000000, 0.9659258262890683122, 1.000000000000000000, 0.9659258262890683122, 1.000000000000000000, 0.9659258262890683122, 1.000000000000000000, 0.9659258262890683122, 1.000000000000000000, 0.9659258262890683122, 1.000000000000000000, 0.9659258262890683122, 1.000000000000000000, 0.9659258262890683122, 1.000000000000000000, 0.9659258262890683122, 1.000000000000000000, 0.9659258262890683122, 1.000000000000000000, 0.9659258262890683122, 1.000000000000000000, 0.9659258262890683122, 1.000000000000000000, 0.9659258262890683122, 1.000000000000000000, 0.9659258262890683122, 1.000000000000000000, 0.9659258262890683122, 1.000000000000000000, 0.9659258262890683122, 1.000000000000000000, 0.9659258262890683122, 1.000000000000000000, 0.9659258262890683122, 1.000000000000000000, 0.9659258262890683122, 1.000000000000000000, 0.9659258262890683122, 1.000000000000000000, 0.9659258262890683122, 1.000000000000000000, 0.9659258262890683122, 1.000000000000000000, 0.9659258262890683122, 1.000000000000000000, 0.9659258262890683122, 1.000000000000000000, 0.9659258262890683122, 1.000000000000000000, 0.9659258262890683122, 1.000000000000000000, 0.9659258262890683122, 1.000000000000000000, 0.9659258262890683122, 1.000000000000000000, 0.9659258262890683122, 1.000000000000000000, 0.9659258262890683122, 1.000000000000000000, 0.9659258262890683122, 1.000000000000000000, 0.9659258262890683122, 1.000000000000000000, 0.9659258262890683122, 1.000000000000000000, 0.9659258262890683122, 1.000000000000000000, 0.9659258262890683122, 1.000000000000000000, 0.9659258262890683122, 1.000000000000000000, 0.9659258262890683122, 1.000000000000000000, 0.9659258262890683122, 1.000000000000000000, 0.9659258262890683122, 1.000000000000000000, 0.9659258262890683122, 1.000000000000000000, 0.9659258262890683122, 1.000000000000000000, 0.9659258262890683122, 1.000000000000000000, 0.9659258262890683122, 1.000000000000000000, 0.9659258262890683122, 1.000000000000000000, 0.9659258262890683122, 1.000000000000000000, 0.9659258262890683122, 1.000000000000000000, 0.9659258262890683122, 1.000000000000000000, 0.9659258262890683122, 1.000000000000000000, 0.9659258262890683122, 1.000000000000000000, 0.9659258262890683122, 1.000000000000000000, 0.9659258262890683122, 1.000000000000000000, 0.9659258262890683122, 1.000000000000000000, 0.9659258262890683122, 1.000000000000000000, 0.9659258262890683122, 1.000000000000000000, 0.9659258262890683122, 1.000000000000000000, 0.9659258262890683122, 1.000000000000000000, 0.9659258262890683122, 1.000000000000000000, 0.9659258262890683122, 1.000000000000000000, 0.9659258262890683122, 1.000000000000000000, 0.9659258262890683122, 1.000000000000000000, 0.9659258262890683122, 1.000000000000000000, 0.9659258262890683122, 1.000000000000000000, 0.9659258262890683122, 1.000000000000000000, 0.9659258262890683122, 1.000000000000000000, 0.9659258262890683122, 1.000000000000000000, 0.9659258262890683122, 1.000000000000000000, 0.9659258262890683122, 1.000000000000000000, 0.9659258262890683122, 1.000000000000000000, 0.9659258262890683122, 1.000000000000000000, 0.9659258262890683122, 1.000000000000000000, 0.9659258262890683122, 1.000000000000000000, 0.9659258262890683122, 1.000000000000000000, 0.9659258262890683122, 1.000000000000000000, 0.9659258262890683122, 1.000000000000000000, 0.9659258262890683122, 1.000000000000000000, 0.9659258262890683122, 1.000000000000000000, 0.9659258262890683122, 1.000000000000000000, 0.9659258262890683122, 1.000000000000000000, 0.9659258262890683122, 1.000000000000000000, 0.9659258262890683122, 1.000000000000000000, 0.9659258262890683122, 1.000000000000000000, 0.9659258262890683122, 1.000000000000000000, 0.9659258262890683122, 1.000000000000000000, 0.9659258262890683122, 1.000000000000000000, 0.9659258262890683122, 1.000000000000000000, 0.9659258262890683122, 1.000000000000000000, 0.9659258262890683122, 1.000000000000000000, 0.9659258262890683122, 1.000000000000000000, 0.9659258262890683122, 1.000000000000000000, 0.9659258262890683122, 1.000000000000000000, 0.9659258262890683122, 1.000000000000000000, 0.9659258262890683122, 1.000000000000000000, 0.9659258262890683122, 1.000000000000000000, 0.9659258262890683122, 1.000000000000000000, 0.9659258262890683122, 1.000000000000000000, 0.9659258262890683122, 1.000000000000000000, 0.9659258262890683122, 1.000000000000000000, 0.9659258262890683122, 1.000000000000000000, 0.9659258262890683122, 1.000000000000000000, 0.9659258262890683122, 1.000000000000000000, 0.9659258262890683122, 1.000000000000000000, 0.9659258262890683122, 1.000000000000000000, 0.9659258262890683122, 1.000000000000000000, 0.9659258262890683122, 1.000000000000000000, 0.9659258262890683122, 1.000000000000000000, 0.9659258262890683122, 1.000000000000000000, 0.9659258262890683122, 1.000000000000000000, 0.9659258262890683122, 1.000000000000000000),
 ( 1.000000000000000000, 0.9659258262890683122, 1.000000000000000000, 0.9659258262890683122, 1.000000000000000000, 0.9659258262890683122, 1.000000000000000000, 0.9659258262890683122, 1.000000000000000000, 0.9659258262890683122, 1.000000000000000000, 0.9659258262890683122, 1.000000000000000000, 0.9659258262890683122, 1.000000000000000000, 0.9659258262890683122, 1.000000000000000000, 0.9659258262890683122, 1.000000000000000000, 0.9659258262890683122, 1.000000000000000000, 0.9659258262890683122, 1.000000000000000000, 0.9659258262890683122, 1.000000000000000000, 0.9659258262890683122, 1.000000000000000000, 0.9659258262890683122, 1.000000000000000000, 0.9659258262890683122, 1.000000000000000000, 0.9659258262890683122, 1.000000000000000000, 0.9659258262890683122, 1.000000000000000000, 0.9659258262890683122, 1.000000000000000000, 0.9659258262890683122, 1.000000000000000000, 0.9659258262890683122, 1.000000000000000000, 0.9659258262890683122, 1.000000000000000000, 0.9659258262890683122, 1.000000000000000000, 0.9659258262890683122, 1.000000000000000000, 0.9659258262890683122, 1.000000000000000000, 0.9659258262890683122, 1.000000000000000000, 0.9659258262890683122, 1.000000000000000000, 0.9659258262890683122, 1.000000000000000000, 0.9659258262890683122, 1.000000000000000000, 0.9659258262890683122, 1.000000000000000000, 0.9659258262890683122, 1.000000000000000000, 0.9659258262890683122, 1.000000000000000000, 0.9659258262890683122, 1.000000000000000000, 0.9659258262890683122, 1.000000000000000000, 0.9659258262890683122, 1.000000000000000000, 0.9659258262890683122, 1.000000000000000000, 0.9659258262890683122, 1.000000000000000000, 0.9659258262890683122, 1.000000000000000000, 0.9659258262890683122, 1.000000000000000000, 0.9659258262890683122, 1.000000000000000000, 0.9659258262890683122, 1.000000000000000000, 0.9659258262890683122, 1.000000000000000000, 0.9659258262890683122, 1.000000000000000000, 0.9659258262890683122, 1.000000000000000000, 0.9659258262890683122, 1.000000000000000000, 0.9659258262890683122, 1.000000000000000000, 0.9659258262890683122, 1.000000000000000000, 0.9659258262890683122, 1.000000000000000000, 0.9659258262890683122, 1.000000000000000000, 0.9659258262890683122, 1.000000000000000000, 0.9659258262890683122, 1.000000000000000000, 0.9659258262890683122, 1.000000000000000000, 0.9659258262890683122, 1.000000000000000000, 0.9659258262890683122, 1.000000000000000000, 0.9659258262890683122, 1.000000000000000000, 0.9659258262890683122, 1.000000000000000000, 0.9659258262890683122, 1.000000000000000000, 0.9659258262890683122, 1.000000000000000000, 0.9659258262890683122, 1.000000000000000000, 0.9659258262890683122, 1.000000000000000000, 0.9659258262890683122, 1.000000000000000000, 0.9659258262890683122, 1.000000000000000000, 0.9659258262890683122, 1.000000000000000000, 0.9659258262890683122, 1.000000000000000000, 0.9659258262890683122, 1.000000000000000000, 0.9659258262890683122, 1.000000000000000000, 0.9659258262890683122, 1.000000000000000000, 0.9659258262890683122, 1.000000000000000000, 0.9659258262890683122, 1.000000000000000000, 0.9659258262890683122, 1.000000000000000000, 0.9659258262890683122, 1.000000000000000000, 0.9659258262890683122, 1.000000000000000000, 0.9659258262890683122, 1.000000000000000000, 0.9659258262890683122, 1.000000000000000000, 0.9659258262890683122, 1.000000000000000000, 0.9659258262890683122, 1.000000000000000000, 0.9659258262890683122, 1.000000000000000000, 0.9659258262890683122, 1.000000000000000000, 0.9659258262890683122, 1.000000000000000000, 0.9659258262890683122, 1.000000000000000000, 0.9659258262890683122, 1.000000000000000000, 0.9659258262890683122, 1.000000000000000000, 0.9659258262890683122, 1.000000000000000000, 0.9659258262890683122, 1.000000000000000000, 0.9659258262890683122, 1.000000000000000000, 0.9659258262890683122, 1.000000000000000000, 0.9659258262890683122, 1.000000000000000000, 0.9659258262890683122, 1.000000000000000000, 0.9659258262890683122, 1.000000000000000000, 0.9659258262890683122, 1.000000000000000000, 0.9659258262890683122, 1.000000000000000000, 0.9659258262890683122, 1.000000000000000000, 0.9659258262890683122, 1.000000000000000000, 0.9659258262890683122, 1.000000000000000000, 0.9659258262890683122, 1.000000000000000000, 0.9659258262890683122, 1.000000000000000000, 0.9659258262890683122, 1.000000000000000000, 0.9659258262890683122, 1.000000000000000000, 0.9659258262890683122, 1.000000000000000000, 0.9659258262890683122, 1.000000000000000000, 0.9659258262890683122, 1.000000000000000000, 0.9659258262890683122, 1.000000000000000000, 0.9659258262890683122, 1.000000000000000000, 0.9659258262890683122, 1.000000000000000000, 0.9659258262890683122, 1.000000000000000000, 0.9659258262890683122, 1.000000000000000000, 0.9659258262890683122, 1.000000000000000000, 0.9659258262890683122, 1.000000000000000000, 0.9659258262890683122, 1.000000000000000000, 0.9659258262890683122, 1.000000000000000000, 0.9659258262890683122, 1.000000000000000000, 0.9659258262890683122, 1.000000000000000000, 0.9659258262890683122, 1.000000000000000000, 0.9659258262890683122, 1.000000000000000000, 0.9659258262890683122, 1.000000000000000000, 0.9659258262890683122, 1.000000000000000000, 0.9659258262890683122, 1.000000000000000000, 0.9659258262890683122, 1.000000000000000000, 0.9659258262890683122, 1.000000000000000000, 0.9659258262890683122, 1.000000000000000000, 0.9659258262890683122, 1.000000000000000000, 0.9659258262890683122, 1.000000000000000000, 0.9659258262890683122, 1.000000000000000000, 0.9659258262890683122, 1.000000000000000000, 0.9659258262890683122, 1.000000000000000000, 0.9659258262890683122, 1.000000000000000000, 0.9659258262890683122, 1.000000000000000000, 0.9659258262890683122, 1.000000000000000000, 0.9659258262890683122, 1.000000000000000000, 0.9659258262890683122, 1.000000000000000000, 0.9659258262890683122, 1.000000000000000000, 0.9659258262890683122, 1.000000000000000000, 0.9659258262890683122, 1.000000000000000000, 0.9659258262890683122, 1.000000000000000000, 0.9659258262890683122, 1.000000000000000000, 0.9659258262890683122, 1.000000000000000000, 0.9659258262890683122, 1.000000000000000000, 0.9659258262890683122, 1.000000000000000000, 0.9659258262890683122, 1.000000000000000000, 0.9659258262890683122, 1.000000000000000000, 0.9659258262890683122, 1.000000000000000000, 0.9659258262890683122, 1.000000000000000000, 0.9659258262890683122, 1.000000000000000000, 0.9659258262890683122, 1.000000000000000000, 0.9659258262890683122, 1.000000000000000000, 0.9659258262890683122, 1.000000000000000000, 0.9659258262890683122, 1.000000000000000000, 0.9659258262890683122, 1.000000000000000000, 0.9659258262890683122, 1.000000000000000000, 0.9659258262890683122, 1.000000000000000000, 0.9659258262890683122, 1.000000000000000000, 0.9659258262890683122, 1.000000000000000000, 0.9659258262890683122, 1.000000000000000000, 0.9659258262890683122, 1.000000000000000000, 0.9659258262890683122, 1.000000000000000000, 0.9659258262890683122, 1.000000000000000000, 0.9659258262890683122, 1.000000000000000000, 0.9659258262890683122, 1.000000000000000000, 0.9659258262890683122, 1.000000000000000000, 0.9659258262890683122, 1.000000000000000000, 0.9659258262890683122, 1.000000000000000000, 0.9659258262890683122, 1.000000000000000000, 0.9659258262890683122, 1.000000000000000000, 0.9659258262890683122, 1.000000000000000000, 0.9659258262890683122, 1.000000000000000000, 0.9659258262890683122, 1.000000000000000000, 0.9659258262890683122, 1.000000000000000000, 0.9659258262890683122, 1.000000000000000000, 0.9659258262890683122, 1.000000000000000000, 0.9659258262890683122, 1.000000000000000000, 0.9659258262890683122, 1.000000000000000000, 0.9659258262890683122, 1.000000000000000000, 0.9659258262890683122, 1.000000000000000000, 0.9659258262890683122, 1.000000000000000000, 0.9659258262890683122, 1.000000000000000000, 0.9659258262890683122, 1.000000000000000000, 0.9659258262890683122, 1.000000000000000000, 0.9659258262890683122, 1.000000000000000000, 0.9659258262890683122, 1.000000000000000000, 0.9659258262890683122, 1.000000000000000000, 0.9659258262890683122, 1.000000000000000000, 0.9659258262890683122, 1.000000000000000000, 0.9659258262890683122, 1.000000000000000000, 0.9659258262890683122, 1.000000000000000000, 0.9659258262890683122, 1.000000000000000000, 0.9659258262890683122, 1.000000000000000000, 0.9659258262890683122, 1.000000000000000000, 0.9659258262890683122, 1.000000000000000000, 0.9659258262890683122, 1.000000000000000000, 0.9659258262890683122, 1.000000000000000000, 0.9659258262890683122, 1.000000000000000000, 0.9659258262890683122, 1.000000000000000000, 0.9659258262890683122, 1.000000000000000000, 0.9659258262890683122, 1.000000000000000000, 0.9659258262890683122, 1.000000000000000000, 0.9659258262890683122, 1.000000000000000000, 0.9659258262890683122, 1.000000000000000000, 0.9659258262890683122, 1.000000000000000000, 0.9659258262890683122, 1.000000000000000000, 0.9659258262890683122, 1.000000000000000000, 0.9659258262890683122, 1.000000000000000000, 0.9659258262890683122, 1.000000000000000000, 0.9659258262890683122, 1.000000000000000000, 0.9659258262890683122, 1.000000000000000000, 0.9659258262890683122, 1.000000000000000000, 0.9659258262890683122, 1.000000000000000000, 0.9659258262890683122, 1.000000000000000000, 0.9659258262890683122, 1.000000000000000000, 0.9659258262890683122, 1.000000000000000000, 0.9659258262890683122, 1.000000000000000000, 0.9659258262890683122, 1.000000000000000000, 0.9659258262890683122, 1.000000000000000000, 0.9659258262890683122, 1.000000000000000000, 0.9659258262890683122, 1.000000000000000000, 0.9659258262890683122, 1.000000000000000000, 0.9659258262890683122, 1.000000000000000000, 0.9659258262890683122, 1.000000000000000000, 0.9659258262890683122, 1.000000000000000000, 0.9659258262890683122, 1.000000000000000000, 0.9659258262890683122, 1.000000000000000000, 0.9659258262890683122, 1.000000000000000000, 0.9659258262890683122, 1.000000000000000000, 0.9659258262890683122, 1.000000000000000000, 0.9659258262890683122, 1.000000000000000000, 0.9659258262890683122, 1.000000000000000000, 0.9659258262890683122, 1.000000000000000000, 0.9659258262890683122, 1.000000000000000000, 0.9659258262890683122, 1.000000000000000000, 0.9659258262890683122, 1.000000000000000000, 0.9659258262890683122, 1.000000000000000000, 0.9659258262890683122, 1.000000000000000000, 0.9659258262890683122, 1.000000000000000000, 0.9659258262890683122, 1.000000000000000000, 0.9659258262890683122, 1.000000000000000000, 0.9659258262890683122, 1.000000000000000000, 0.9659258262890683122, 1.000000000000000000, 0.9659258262890683122, 1.000000000000000000, 0.9659258262890683122, 1.000000000000000000, 0.9659258262890683122, 1.000000000000000000, 0.9659258262890683122, 1.000000000000000000, 0.9659258262890683122, 1.000000000000000000, 0.9659258262890683122, 1.000000000000000000, 0.9659258262890683122, 1.000000000000000000, 0.9659258262890683122, 1.000000000000000000, 0.9659258262890683122, 1.000000000000000000, 0.9659258262890683122, 1.000000000000000000, 0.9659258262890683122, 1.000000000000000000, 0.9659258262890683122, 1.000000000000000000, 0.9659258262890683122, 1.000000000000000000, 0.9659258262890683122, 1.000000000000000000, 0.9659258262890683122, 1.000000000000000000, 0.9659258262890683122, 1.000000000000000000, 0.9659258262890683122, 1.000000000000000000, 0.9659258262890683122, 1.000000000000000000, 0.9659258262890683122, 1.000000000000000000, 0.9659258262890683122, 1.000000000000000000) ) ) 
 REPRESENTATION_ITEM ( '' )  SURFACE ( )  );
#49408=CARTESIAN_POINT ( 'NONE',  ( 1.561679790026247350, -0.4281496062992124485, 0.4176697321401328655 ) ) ;
#49411=CARTESIAN_POINT ( 'NONE',  ( -1.036745406824146176, 0.05413385826771626580, -0.4176697321401330321 ) ) ;
#49412=CARTESIAN_POINT ( 'NONE',  ( -0.9842519685039360366, 0.1771653543307087630, 0.000000000000000000 ) ) ;
#49413=CARTESIAN_POINT ( 'NONE',  ( -0.5643044619422565855, -0.004921259842519870586, -0.3153832671262229437 ) ) ;
#49414=CARTESIAN_POINT ( 'NONE',  ( -1.220472440944881054, 0.000000000000000000, 0.5309055118110237448 ) ) ;
#49415=CARTESIAN_POINT ( 'NONE',  ( 0.05905511811023709395, -0.5400638737290844871, 0.3530559997133364547 ) ) ;
#49416=CARTESIAN_POINT ( 'NONE',  ( 0.05249343832021075018, -0.5023911411419708095, 0.1820866141732285504 ) ) ;
#49417=CARTESIAN_POINT ( 'NONE',  ( -0.9973753280839886548, -0.5023911411419708095, -0.1820866141732282451 ) ) ;
#49418=CARTESIAN_POINT ( 'NONE',  ( -1.496062992125983815, -0.1870078740157480879, -0.4822834645669291653 ) ) ;
#49419=CARTESIAN_POINT ( 'NONE',  ( 1.154855643044620184, 0.1283753931104746893, -0.1820866141732285504 ) ) ;
#49420=CARTESIAN_POINT ( 'NONE',  ( 0.8202099737532814183, -0.6692913385826773087, -0.1292274648535924053 ) ) ;
#49421=CARTESIAN_POINT ( 'NONE',  ( 2.795275590551181910, 1.535433070866142335, 0.000000000000000000 ) ) ;
#49422=CARTESIAN_POINT ( 'NONE',  ( 0.6561679790026253567, -0.5023911411419708095, -0.1820866141732282451 ) ) ;
#49423=CARTESIAN_POINT ( 'NONE',  ( 0.7480314960629927956, 0.2952755905511811885, 0.000000000000000000 ) ) ;
#49424=CARTESIAN_POINT ( 'NONE',  ( 1.030183727034121421, -0.2845877964562161244, -0.3641732283464567121 ) ) ;
#49426=CARTESIAN_POINT ( 'NONE',  ( -1.227034120734907141, -0.6692913385826773087, -0.1292274648535924053 ) ) ;
#49428=CARTESIAN_POINT ( 'NONE',  ( -0.8989501312335946848, -0.6692913385826771977, 0.1292274648535927661 ) ) ;
#49429=CARTESIAN_POINT ( 'NONE',  ( 0.07874015748031558404, -0.1870078740157480879, -0.4822834645669291653 ) ) ;
#49432=CARTESIAN_POINT ( 'NONE',  ( 0.3280839895013130669, 0.05413385826771666132, 0.4176697321401328100 ) ) ;
#49433=CARTESIAN_POINT ( 'NONE',  ( 1.594488188976378673, 0.07958543189024085140, 0.2665933059059887866 ) ) ;
#49434=CARTESIAN_POINT ( 'NONE',  ( 0.006561679790026889343, -0.3162353388693409650, -0.4822834645669289433 ) ) ;
#49435=CARTESIAN_POINT ( 'NONE',  ( 0.6299212598425204535, -0.1870078740157479769, 0.4822834645669291653 ) ) ;
#49441=CARTESIAN_POINT ( 'NONE',  ( -0.4330708661417315697, 0.1771653543307087630, 0.000000000000000000 ) ) ;
#49442=CARTESIAN_POINT ( 'NONE',  ( -0.8595800524934373854, -0.3162353388693409650, -0.4822834645669289433 ) ) ;
#49443=CARTESIAN_POINT ( 'NONE',  ( 0.6167979002624678353, -0.4281496062992124485, 0.4176697321401328655 ) ) ;
#49445=CARTESIAN_POINT ( 'NONE',  ( 1.049868766404200349, 0.2306618581243848609, 0.2411417322834645549 ) ) ;
#49446=CARTESIAN_POINT ( 'NONE',  ( 1.541994750656168645, -0.6692913385826771977, 0.1292274648535927661 ) ) ;
#49447=CARTESIAN_POINT ( 'NONE',  ( 1.338582677165355062, -0.1870078740157480879, -0.4822834645669291653 ) ) ;
#49450=CARTESIAN_POINT ( 'NONE',  ( 1.128608923884514947, 0.2306618581243848609, 0.2411417322834645549 ) ) ;
#49451=CARTESIAN_POINT ( 'NONE',  ( 0.8727034120734912248, -0.3162353388693409650, -0.4822834645669289433 ) ) ;
#49452=CARTESIAN_POINT ( 'NONE',  ( 0.4396325459317590445, -0.6692913385826771977, 0.1292274648535927661 ) ) ;
#49453=CARTESIAN_POINT ( 'NONE',  ( 1.056430446194226436, -0.5511811023622048555, -0.09757992244046775898 ) ) ;
#49454=CARTESIAN_POINT ( 'NONE',  ( -1.594488188976377119, 0.07958543189024071263, -0.2665933059059888421 ) ) ;
#49455=CARTESIAN_POINT ( 'NONE',  ( 1.587926509186352142, 0.05413385826771666132, 0.4176697321401328100 ) ) ;
#49457=CARTESIAN_POINT ( 'NONE',  ( 0.7742782152230979209, 0.05413385826771626580, -0.4176697321401330321 ) ) ;
#49458=CARTESIAN_POINT ( 'NONE',  ( 1.587926509186352586, -0.3690944881889765550, -0.3153832671262227771 ) ) ;
#49459=CARTESIAN_POINT ( 'NONE',  ( -0.6824146981627291497, -0.6046776061558809534, -0.2411417322834644161 ) ) ;
#49460=CARTESIAN_POINT ( 'NONE',  ( -0.3937007874015740483, -0.1870078740157480879, -0.4822834645669291653 ) ) ;
#49462=CARTESIAN_POINT ( 'NONE',  ( -1.601049868766403650, 0.2306618581243847221, -0.2411417322834647770 ) ) ;
#49464=CARTESIAN_POINT ( 'NONE',  ( 0.1837270341207354329, 0.2306618581243848609, 0.2411417322834645549 ) ) ;
#49466=CARTESIAN_POINT ( 'NONE',  ( -1.541994750656167090, -0.5511811023622048555, -0.09757992244046775898 ) ) ;
#49472=CARTESIAN_POINT ( 'NONE',  ( 1.174540682414699111, -0.08942795157528024563, -0.3641732283464568787 ) ) ;
#49474=CARTESIAN_POINT ( 'NONE',  ( 1.528871391076116026, 0.1771653543307087630, 0.09757992244046791164 ) ) ;
#49475=CARTESIAN_POINT ( 'NONE',  ( -0.1115485564304456445, 0.2066929133858267098, -0.1054918080437494132 ) ) ;
#49476=CARTESIAN_POINT ( 'NONE',  ( 0.4800390104732028540, 1.504150543744003032, 0.5309055118110234117 ) ) ;
#49479=CARTESIAN_POINT ( 'NONE',  ( -0.7152230971128602510, -0.2845877964562159024, 0.3641732283464567677 ) ) ;
#49480=CARTESIAN_POINT ( 'NONE',  ( -1.030183727034119867, -0.08942795157528024563, -0.3641732283464568787 ) ) ;
#49481=CARTESIAN_POINT ( 'NONE',  ( -1.430446194225720724, 0.05413385826771626580, -0.4176697321401330321 ) ) ;
#49482=CARTESIAN_POINT ( 'NONE',  ( 0.4855643044619428750, 0.05413385826771666132, 0.4176697321401328100 ) ) ;
#49483=CARTESIAN_POINT ( 'NONE',  ( -1.128608923884513837, 0.2306618581243847221, -0.2411417322834647770 ) ) ;
#49486=CARTESIAN_POINT ( 'NONE',  ( 1.404199475065617264, -0.4281496062992124485, 0.4176697321401328655 ) ) ;
#49487=CARTESIAN_POINT ( 'NONE',  ( -0.7749820319012115100, 0.000000000000000000, 0.3464511005275205946 ) ) ;
#49490=EDGE_CURVE ( 'NONE', #46160, #54098, #56067, .T. ) ;
#49492=CARTESIAN_POINT ( 'NONE',  ( -0.7611548556430438595, -0.6046776061558809534, -0.2411417322834644161 ) ) ;
#49493=CARTESIAN_POINT ( 'NONE',  ( 0.8333333333333340365, -0.6692913385826771977, 0.1292274648535927661 ) ) ;
#49494=PLANE ( 'NONE',  #36874 ) ;
#49496=CARTESIAN_POINT ( 'NONE',  ( 1.482939632545932307, -0.4281496062992124485, 0.4176697321401328655 ) ) ;
#49497=CARTESIAN_POINT ( 'NONE',  ( -1.292650918635170010, -0.6692913385826771977, 0.1292274648535927661 ) ) ;
#49499=CARTESIAN_POINT ( 'NONE',  ( 0.09186351706036799403, -0.3690944881889765550, -0.3153832671262227771 ) ) ;
#49501=CARTESIAN_POINT ( 'NONE',  ( -0.1837270341207340729, 0.1283753931104746893, -0.1820866141732285504 ) ) ;
#49502=CARTESIAN_POINT ( 'NONE',  ( 0.4527559055118117182, -0.4536011799217367080, 0.2665933059059888421 ) ) ;
#49503=CARTESIAN_POINT ( 'NONE',  ( 0.5577427821522314977, -0.3162353388693409650, -0.4822834645669289433 ) ) ;
#49504=CARTESIAN_POINT ( 'NONE',  ( -0.7480314960629914633, -0.5511811023622047445, 6.969142054262312111E-17 ) ) ;
#49506=CARTESIAN_POINT ( 'NONE',  ( -1.509186351706035767, -0.4281496062992124485, 0.4176697321401328655 ) ) ;
#49507=CARTESIAN_POINT ( 'NONE',  ( -1.069553805774277722, -0.6692913385826773087, -0.1292274648535924053 ) ) ;
#49509=CARTESIAN_POINT ( 'NONE',  ( -0.04593175853018302557, -0.6692913385826773087, -0.1292274648535924053 ) ) ;
#49510=CARTESIAN_POINT ( 'NONE',  ( -0.6036745406824141069, -0.6046776061558809534, -0.2411417322834644161 ) ) ;
#49511=CARTESIAN_POINT ( 'NONE',  ( 1.338582677165355062, -0.1870078740157479769, 0.3641732283464567677 ) ) ;
#49512=CARTESIAN_POINT ( 'NONE',  ( 0.3215223097112867578, -0.08942795157527998196, 0.3641732283464567121 ) ) ;
#49513=CARTESIAN_POINT ( 'NONE',  ( -0.2690288713910754526, 0.2952755905511810774, -0.1292274648535930714 ) ) ;
#49514=CARTESIAN_POINT ( 'NONE',  ( -1.272965879265091305, 0.05413385826771626580, -0.4176697321401330321 ) ) ;
#49515=CARTESIAN_POINT ( 'NONE',  ( 0.7773926554473647998, 8.471767977567108961E-16, -0.4445507791589058955 ) ) ;
#49516=CARTESIAN_POINT ( 'NONE',  ( -0.5611900217179893735, -2.567464376874931580E-15, -0.4445507791589072832 ) ) ;
#49517=CARTESIAN_POINT ( 'NONE',  ( 0.08530183727034192087, -0.05778040916215522460, 0.4822834645669289988 ) ) ;
#49518=ORIENTED_EDGE ( 'NONE', *, *, #54812, .F. ) ;
#49520=CARTESIAN_POINT ( 'NONE',  ( 1.181102362204724976, -0.1870078740157480879, -0.4822834645669291653 ) ) ;
#49521=CARTESIAN_POINT ( 'NONE',  ( -0.6758530183727028406, -0.5511811023622048555, -0.09757992244046775898 ) ) ;
#49522=CARTESIAN_POINT ( 'NONE',  ( -0.5446194225721777693, -0.3162353388693409650, -0.4822834645669289433 ) ) ;
#49523=CARTESIAN_POINT ( 'NONE',  ( 1.272965879265092637, -0.4281496062992127816, -0.4176697321401328100 ) ) ;
#49524=CARTESIAN_POINT ( 'NONE',  ( 1.069553805774278832, 0.2952755905511810774, -0.1292274648535930714 ) ) ;
#49525=CARTESIAN_POINT ( 'NONE',  ( -1.640419947506561060, 0.05413385826771666132, 0.4176697321401328100 ) ) ;
#49526=CARTESIAN_POINT ( 'NONE',  ( -1.227034120734907585, 0.1771653543307087630, 0.09757992244046791164 ) ) ;
#49530=CARTESIAN_POINT ( 'NONE',  ( 1.397637795275591177, 0.07958543189024071263, -0.2665933059059888421 ) ) ;
#49531=CARTESIAN_POINT ( 'NONE',  ( 0.5446194225721792126, -0.08942795157528024563, -0.3641732283464568787 ) ) ;
#49532=CARTESIAN_POINT ( 'NONE',  ( 0.7020997375328090762, -0.05778040916215560624, -0.4822834645669293319 ) ) ;
#49535=CARTESIAN_POINT ( 'NONE',  ( 0.9251968503937015864, 0.07958543189024071263, -0.2665933059059888421 ) ) ;
#49536=CARTESIAN_POINT ( 'NONE',  ( -0.1771653543307080136, 0.1660481256975883668, -0.3530559997133364547 ) ) ;
#49537=CARTESIAN_POINT ( 'NONE',  ( -0.7283464566929126471, -0.5400638737290844871, 0.3530559997133364547 ) ) ;
#49538=CARTESIAN_POINT ( 'NONE',  ( 1.122047244094488860, -0.5400638737290845981, -0.3530559997133363437 ) ) ;
#49541=CARTESIAN_POINT ( 'NONE',  ( -0.2230971128608915943, -0.3690944881889765550, -0.3153832671262227771 ) ) ;
#49544=EDGE_LOOP ( 'NONE', ( #25449, #44446, #73081, #37827 ) ) ;
#49545=CARTESIAN_POINT ( 'NONE',  ( -0.9580052493438311334, -0.4281496062992124485, 0.4176697321401328655 ) ) ;
#49546=CARTESIAN_POINT ( 'NONE',  ( -0.2624671916010490880, -0.6046776061558807314, 0.2411417322834647770 ) ) ;
#49547=CARTESIAN_POINT ( 'NONE',  ( -0.2034120734908128059, 0.2952755905511811885, 0.1292274648535926551 ) ) ;
#49548=CARTESIAN_POINT ( 'NONE',  ( 0.5118110236220480003, -0.6692913385826771977, 8.415575281601705876E-17 ) ) ;
#49549=CARTESIAN_POINT ( 'NONE',  ( -0.6364829396325453192, -0.05778040916215560624, -0.4822834645669293319 ) ) ;
#49550=CARTESIAN_POINT ( 'NONE',  ( -1.456692913385826182, 0.2952755905511811885, 0.000000000000000000 ) ) ;
#49551=CARTESIAN_POINT ( 'NONE',  ( -0.6496062992125976043, -0.5400638737290844871, 0.3530559997133364547 ) ) ;
#49552=CARTESIAN_POINT ( 'NONE',  ( 0.7480314960629927956, -0.6692913385826771977, 8.415575281601705876E-17 ) ) ;
#49553=ADVANCED_FACE ( 'NONE', ( #19010 ), #53336, .F. ) ;
#49554=CARTESIAN_POINT ( 'NONE',  ( 0.3477690288713918276, 0.2952755905511811885, 0.1292274648535926551 ) ) ;
#49557=CARTESIAN_POINT ( 'NONE',  ( -0.2755905511811015396, -0.5511811023622047445, 6.969142054262312111E-17 ) ) ;
#49561=CARTESIAN_POINT ( 'NONE',  ( -1.102362204724408601, -0.1870078740157479769, 0.3641732283464567677 ) ) ;
#49562=CARTESIAN_POINT ( 'NONE',  ( -1.286089238845143479, 0.2306618581243847221, -0.2411417322834647770 ) ) ;
#49563=CARTESIAN_POINT ( 'NONE',  ( -0.3477690288713902178, 0.2952755905511810774, -0.1292274648535930714 ) ) ;
#49564=CARTESIAN_POINT ( 'NONE',  ( 0.3836918680457899744, 8.471767977567108961E-16, -0.4445507791589058955 ) ) ;
#49565=CARTESIAN_POINT ( 'NONE',  ( -0.7020997375328076329, -0.3162353388693409650, -0.4822834645669289433 ) ) ;
#49566=CARTESIAN_POINT ( 'NONE',  ( -0.7283464566929126471, 0.1660481256975883668, -0.3530559997133364547 ) ) ;
#49568=CARTESIAN_POINT ( 'NONE',  ( 1.017060367454068803, -0.2845877964562159024, 0.3641732283464567677 ) ) ;
#49569=LINE ( 'NONE', #37766, #59251 ) ;
#49571=CARTESIAN_POINT ( 'NONE',  ( -0.01312335958005186876, -0.3690944881889763329, 0.3153832671262228327 ) ) ;
#49572=CARTESIAN_POINT ( 'NONE',  ( -0.5643044619422565855, -0.4281496062992124485, 0.4176697321401328655 ) ) ;
#49573=CARTESIAN_POINT ( 'NONE',  ( -0.7080320533160963103, 1.900312960331933976, -0.5309055118110235227 ) ) ;
#49574=CARTESIAN_POINT ( 'NONE',  ( 0.04593175853018440641, -0.6692913385826771977, 0.1292274648535927661 ) ) ;
#49577=CARTESIAN_POINT ( 'NONE',  ( -0.8001742991414044770, 0.004960608223778509643, -0.3437734562760191848 ) ) ;
#49580=DIRECTION ( 'NONE',  ( -1.000000000000000000, 0.000000000000000000, 0.000000000000000000 ) ) ;
#49581=CARTESIAN_POINT ( 'NONE',  ( -0.8792650918635160906, -0.004921259842519870586, -0.3153832671262229437 ) ) ;
#49582=CARTESIAN_POINT ( 'NONE',  ( -0.7677165354330699465, 0.1660481256975885056, 0.3530559997133364547 ) ) ;
#49584=DIRECTION ( 'NONE',  ( 1.000000000000000000, 3.083952846180989294E-16, 0.000000000000000000 ) ) ;
#49587=CARTESIAN_POINT ( 'NONE',  ( 1.161417322834646493, -0.5400638737290844871, 0.3530559997133364547 ) ) ;
#49588=CARTESIAN_POINT ( 'NONE',  ( 0.2755905511811031494, -0.6692913385826771977, 8.415575281601705876E-17 ) ) ;
#49589=CARTESIAN_POINT ( 'NONE',  ( 0.4199475065616805614, 0.2306618581243848609, 0.2411417322834645549 ) ) ;
#49590=CARTESIAN_POINT ( 'NONE',  ( -0.6758530183727028406, 0.1771653543307087630, 0.09757992244046791164 ) ) ;
#49591=CARTESIAN_POINT ( 'NONE',  ( -0.5249343832020990641, -0.6046776061558809534, -0.2411417322834644161 ) ) ;
#49593=ADVANCED_FACE ( 'NONE', ( #18518 ), #13037, .F. ) ;
#49594=CARTESIAN_POINT ( 'NONE',  ( -0.7742782152230965886, 0.05413385826771666132, 0.4176697321401328100 ) ) ;
#49596=CARTESIAN_POINT ( 'NONE',  ( 1.469816272965879911, 0.1283753931104746893, -0.1820866141732285504 ) ) ;
#49597=CARTESIAN_POINT ( 'NONE',  ( -0.3805774278215216522, -0.3690944881889765550, -0.3153832671262227771 ) ) ;
#49598=CARTESIAN_POINT ( 'NONE',  ( 0.9908136482939640111, -0.5511811023622046335, 0.09757992244046803654 ) ) ;
#49599=CARTESIAN_POINT ( 'NONE',  ( -1.581364829396324945, -0.3162353388693405765, 0.4822834645669290543 ) ) ;
#49600=CARTESIAN_POINT ( 'NONE',  ( -1.194225721784776262, -0.3690944881889763329, 0.3153832671262228327 ) ) ;
#49602=CARTESIAN_POINT ( 'NONE',  ( 0.6102362204724416372, 0.07958543189024071263, -0.2665933059059888421 ) ) ;
#49603=CARTESIAN_POINT ( 'NONE',  ( -0.3215223097112853146, -0.05778040916215560624, -0.4822834645669293319 ) ) ;
#49604=CARTESIAN_POINT ( 'NONE',  ( 0.3049517105654749871, 8.471767977567108961E-16, -0.4445507791589058955 ) ) ;
#49605=CARTESIAN_POINT ( 'NONE',  ( -0.2755905511811015396, -0.5511811023622047445, 6.969142054262312111E-17 ) ) ;
#49606=CARTESIAN_POINT ( 'NONE',  ( 0.8923884514435703741, 0.2306618581243848609, 0.2411417322834645549 ) ) ;
#49608=CARTESIAN_POINT ( 'NONE',  ( 1.174540682414699111, -0.08942795157528024563, -0.3641732283464568787 ) ) ;
#49609=CARTESIAN_POINT ( 'NONE',  ( -0.8202099737532801971, -0.6692913385826771977, 0.1292274648535927661 ) ) ;
#49610=CARTESIAN_POINT ( 'NONE',  ( -0.3412073490813641308, 0.1283753931104746893, -0.1820866141732285504 ) ) ;
#49611=CARTESIAN_POINT ( 'NONE',  ( 1.035118193396260766, 4.339766966676338660E-16, 0.3791483426435169335 ) ) ;
#49612=CARTESIAN_POINT ( 'NONE',  ( 0.2493438320209980519, -0.3690944881889765550, -0.3153832671262227771 ) ) ;
#49614=CARTESIAN_POINT ( 'NONE',  ( -0.6233595800524928121, -0.3162353388693409650, -0.4822834645669289433 ) ) ;
#49617=CARTESIAN_POINT ( 'NONE',  ( 0.5380577427821529035, -0.004921259842519870586, -0.3153832671262229437 ) ) ;
#49618=CARTESIAN_POINT ( 'NONE',  ( -0.3674540682414689785, 0.2306618581243848609, 0.2411417322834645549 ) ) ;
#49619=CARTESIAN_POINT ( 'NONE',  ( -0.8923884514435688198, -0.6046776061558807314, 0.2411417322834647770 ) ) ;
#49620=CARTESIAN_POINT ( 'NONE',  ( -0.6167979002624665030, -0.3690944881889765550, -0.3153832671262227771 ) ) ;
#49622=CARTESIAN_POINT ( 'NONE',  ( -0.03937007874015669567, 0.2952755905511811885, 0.000000000000000000 ) ) ;
#49623=AXIS2_PLACEMENT_3D ( 'NONE', #67000, #43243, #60668 ) ;
#49624=CARTESIAN_POINT ( 'NONE',  ( -1.069553805774277722, 0.1771653543307087630, 0.09757992244046791164 ) ) ;
#49625=CARTESIAN_POINT ( 'NONE',  ( -1.384514435695537005, -0.6692913385826773087, -0.1292274648535924053 ) ) ;
#49628=CARTESIAN_POINT ( 'NONE',  ( -1.620734908136482577, -0.5511811023622048555, -0.09757992244046775898 ) ) ;
#49629=CARTESIAN_POINT ( 'NONE',  ( -1.384514435695537005, 0.2952755905511811885, 0.1292274648535926551 ) ) ;
#49630=CARTESIAN_POINT ( 'NONE',  ( -1.056430446194224881, 0.2952755905511810774, -0.1292274648535930714 ) ) ;
#49632=CARTESIAN_POINT ( 'NONE',  ( 1.587926509186352142, 0.05413385826771666132, 0.4176697321401328100 ) ) ;
#49635=CARTESIAN_POINT ( 'NONE',  ( 1.082677165354331228, 0.1660481256975883668, -0.3530559997133364547 ) ) ;
#49636=CARTESIAN_POINT ( 'NONE',  ( 0.2821522309711292364, 0.2952755905511810774, -0.1292274648535930714 ) ) ;
#49639=CARTESIAN_POINT ( 'NONE',  ( 1.174540682414699111, -0.08942795157528024563, -0.3641732283464568787 ) ) ;
#49640=B_SPLINE_CURVE_WITH_KNOTS ( 'NONE', 3,
 ( #16142, #22854, #36714, #23673, #9402, #68715, #41789 ),
 .UNSPECIFIED., .F., .F.,
 ( 4, 3, 4 ),
 ( 1.232595164407830946E-32, 0.001246232571205264407, 0.002492492258783314020 ),
 .UNSPECIFIED. ) ;
#49643=CARTESIAN_POINT ( 'NONE',  ( -0.8530183727034112984, -0.004921259842519576551, 0.3153832671262227771 ) ) ;
#49645=ORIENTED_EDGE ( 'NONE', *, *, #51403, .F. ) ;
#49646=CARTESIAN_POINT ( 'NONE',  ( 0.4527559055118117182, -0.5400638737290844871, 0.3530559997133364547 ) ) ;
#49647=CARTESIAN_POINT ( 'NONE',  ( -0.2230971128608915943, -0.4281496062992127816, -0.4176697321401328100 ) ) ;
#49648=CARTESIAN_POINT ( 'NONE',  ( -1.286089238845143479, 0.2306618581243847221, -0.2411417322834647770 ) ) ;
#49649=CARTESIAN_POINT ( 'NONE',  ( 1.108923884514436686, -0.3162353388693409650, -0.4822834645669289433 ) ) ;
#49650=CARTESIAN_POINT ( 'NONE',  ( 1.692913385826772421, 0.2952755905511811885, 0.000000000000000000 ) ) ;
#49652=CARTESIAN_POINT ( 'NONE',  ( -0.08530183727034056085, -0.3162353388693405765, 0.4822834645669290543 ) ) ;
#49653=CARTESIAN_POINT ( 'NONE',  ( -1.266404199475064773, -0.05778040916215560624, -0.4822834645669293319 ) ) ;
#49656=CARTESIAN_POINT ( 'NONE',  ( 1.450131233595801428, -0.6692913385826773087, -0.1292274648535924053 ) ) ;
#49659=CARTESIAN_POINT ( 'NONE',  ( 0.7349081364829403995, 0.1283753931104748280, 0.1820866141732283561 ) ) ;
#49660=ORIENTED_EDGE ( 'NONE', *, *, #45936, .F. ) ;
#49662=CARTESIAN_POINT ( 'NONE',  ( -0.6889763779527552368, 0.1660481256975885056, 0.3530559997133364547 ) ) ;
#49663=EDGE_LOOP ( 'NONE', ( #47311, #56690, #54196, #11263, #81264 ) ) ;
#49664=CARTESIAN_POINT ( 'NONE',  ( -0.1181102362204717315, 0.1771653543307087630, 0.000000000000000000 ) ) ;
#49665=CARTESIAN_POINT ( 'NONE',  ( -1.555118110236219930, 0.1660481256975885056, 0.3530559997133364547 ) ) ;
#49666=CARTESIAN_POINT ( 'NONE',  ( 0.3543307086614179147, 0.2952755905511811885, 0.000000000000000000 ) ) ;
#49667=CARTESIAN_POINT ( 'NONE',  ( 0.3477690288713918276, 0.2952755905511811885, 0.1292274648535926551 ) ) ;
#49668=CARTESIAN_POINT ( 'NONE',  ( -0.5183727034120726440, -0.6692913385826773087, -0.1292274648535924053 ) ) ;
#49670=CARTESIAN_POINT ( 'NONE',  ( -0.9251968503937002541, -0.5400638737290845981, -0.3530559997133363437 ) ) ;
#49672=CARTESIAN_POINT ( 'NONE',  ( 1.272965879265092637, -0.004921259842519576551, 0.3153832671262227771 ) ) ;
#49673=CARTESIAN_POINT ( 'NONE',  ( -1.161417322834644716, 0.1660481256975885056, 0.3530559997133364547 ) ) ;
#49674=CARTESIAN_POINT ( 'NONE',  ( 0.7414698162729663755, 0.2952755905511811885, 0.1292274648535926551 ) ) ;
#49675=CARTESIAN_POINT ( 'NONE',  ( 1.371391076115485941, 0.2952755905511811885, 0.1292274648535926551 ) ) ;
#49677=CARTESIAN_POINT ( 'NONE',  ( -1.194225721784776262, 0.05413385826771626580, -0.4176697321401330321 ) ) ;
#49679=CARTESIAN_POINT ( 'NONE',  ( 0.4790026246719167324, -0.05778040916215522460, 0.4822834645669289988 ) ) ;
#49681=CARTESIAN_POINT ( 'NONE',  ( -1.522309711286088607, -0.5023911411419708095, 0.1820866141732285504 ) ) ;
#49682=CARTESIAN_POINT ( 'NONE',  ( 0.6692913385826778638, -0.5511811023622047445, 6.969142054262312111E-17 ) ) ;
#49683=CARTESIAN_POINT ( 'NONE',  ( 1.102362204724410155, -0.1870078740157479769, 0.4822834645669291653 ) ) ;
#49685=CARTESIAN_POINT ( 'NONE',  ( 0.6430446194225729606, -0.3690944881889765550, -0.3153832671262227771 ) ) ;
#49686=CARTESIAN_POINT ( 'NONE',  ( 0.4724409448818904789, -0.1870078740157479769, 0.4822834645669291653 ) ) ;
#49688=CARTESIAN_POINT ( 'NONE',  ( -0.9120734908136475250, 0.2952755905511811885, 0.1292274648535926551 ) ) ;
#49689=CARTESIAN_POINT ( 'NONE',  ( -0.1674892343164145203, -2.567464376874931580E-15, -0.4445507791589072832 ) ) ;
#49690=CARTESIAN_POINT ( 'NONE',  ( 0.9448818897637802916, -0.1870078740157479769, 0.3641732283464567677 ) ) ;
#49691=CARTESIAN_POINT ( 'NONE',  ( 0.1771653543307093182, 0.1660481256975885056, 0.3530559997133364547 ) ) ;
#49693=CARTESIAN_POINT ( 'NONE',  ( -0.5118110236220466680, -0.6692913385826771977, 8.415575281601705876E-17 ) ) ;
#49694=CARTESIAN_POINT ( 'NONE',  ( 0.3149606299212606708, -0.1870078740157480601, -0.3641732283464567677 ) ) ;
#49696=CARTESIAN_POINT ( 'NONE',  ( -0.04593175853018302557, 0.1771653543307087630, 0.09757992244046791164 ) ) ;
#49697=CARTESIAN_POINT ( 'NONE',  ( 0.6364829396325465405, -0.08942795157527998196, 0.3641732283464567121 ) ) ;
#49700=CARTESIAN_POINT ( 'NONE',  ( 0.1377952755905518800, 0.1660481256975883668, -0.3530559997133364547 ) ) ;
#49702=CARTESIAN_POINT ( 'NONE',  ( 1.266404199475066328, -0.2845877964562161244, -0.3641732283464567121 ) ) ;
#49704=CARTESIAN_POINT ( 'NONE',  ( -0.3018372703412066094, -0.004921259842519576551, 0.3153832671262227771 ) ) ;
#49706=CARTESIAN_POINT ( 'NONE',  ( -0.2099737532808391705, -0.5023911411419708095, -0.1820866141732282451 ) ) ;
#49707=CARTESIAN_POINT ( 'NONE',  ( -0.3740157480314953431, 0.1660481256975885056, 0.3530559997133364547 ) ) ;
#49708=CARTESIAN_POINT ( 'NONE',  ( 0.7742782152230979209, -0.004921259842519870586, -0.3153832671262229437 ) ) ;
#49710=CARTESIAN_POINT ( 'NONE',  ( 1.587926509186352142, -0.004921259842519576551, 0.3153832671262227771 ) ) ;
#49712=CARTESIAN_POINT ( 'NONE',  ( 0.09842519685039434474, 0.1660481256975885056, 0.3530559997133364547 ) ) ;
#49713=CARTESIAN_POINT ( 'NONE',  ( 1.174540682414699111, -0.3162353388693405765, 0.4822834645669290543 ) ) ;
#49714=CARTESIAN_POINT ( 'NONE',  ( -1.595398199321655275, 1.839868176060737381, -0.1559797534342491077 ) ) ;
#49715=CARTESIAN_POINT ( 'NONE',  ( 0.2427821522309716595, -0.3162353388693409650, -0.4822834645669289433 ) ) ;
#49717=CARTESIAN_POINT ( 'NONE',  ( 0.7152230971128616943, -0.05778040916215522460, 0.4822834645669289988 ) ) ;
#49718=CARTESIAN_POINT ( 'NONE',  ( 0.6233595800524942554, -0.05778040916215560624, -0.4822834645669293319 ) ) ;
#49720=CARTESIAN_POINT ( 'NONE',  ( 0.6758530183727039509, -0.5511811023622046335, 0.09757992244046803654 ) ) ;
#49721=CARTESIAN_POINT ( 'NONE',  ( 1.049868766404200349, 0.2306618581243848609, 0.2411417322834645549 ) ) ;
#49722=CARTESIAN_POINT ( 'NONE',  ( 0.1509186351706042484, -0.2845877964562159024, 0.3641732283464567677 ) ) ;
#49723=CARTESIAN_POINT ( 'NONE',  ( -0.4199475065616791736, -0.6046776061558807314, 0.2411417322834647770 ) ) ;
#49724=CARTESIAN_POINT ( 'NONE',  ( 0.1443569553805781891, -0.4281496062992124485, 0.4176697321401328655 ) ) ;
#49725=CARTESIAN_POINT ( 'NONE',  ( -0.7152230971128602510, -0.3162353388693405765, 0.4822834645669290543 ) ) ;
#49726=CARTESIAN_POINT ( 'NONE',  ( -0.2952755905511804668, 0.07958543189024085140, 0.2665933059059887866 ) ) ;
#49727=CARTESIAN_POINT ( 'NONE',  ( 0.8333333333333340365, 0.2952755905511810774, -0.1292274648535930714 ) ) ;
#49728=CARTESIAN_POINT ( 'NONE',  ( 1.148293963254593875, -0.5511811023622046335, 0.09757992244046803654 ) ) ;
#49729=CARTESIAN_POINT ( 'NONE',  ( -0.01968503937007793844, 0.1660481256975883668, -0.3530559997133364547 ) ) ;
#49733=FACE_OUTER_BOUND ( 'NONE', #2996, .T. ) ;
#49735=CARTESIAN_POINT ( 'NONE',  ( -1.049868766404198794, -0.6046776061558807314, 0.2411417322834647770 ) ) ;
#49736=CARTESIAN_POINT ( 'NONE',  ( -1.056430446194224881, 0.2952755905511810774, -0.1292274648535930714 ) ) ;
#49739=ORIENTED_EDGE ( 'NONE', *, *, #70319, .F. ) ;
#49740=CARTESIAN_POINT ( 'NONE',  ( 0.4724409448818904789, -0.1870078740157480601, -0.3641732283464567677 ) ) ;
#49742=CARTESIAN_POINT ( 'NONE',  ( 0.5052493438320215802, 0.2952755905511811885, 0.1292274648535926551 ) ) ;
#49745=CARTESIAN_POINT ( 'NONE',  ( -0.3049517105654738214, -2.191421614605370878E-15, 0.4445507791589071167 ) ) ;
#49746=CARTESIAN_POINT ( 'NONE',  ( 0.9973753280839902091, -0.6046776061558807314, 0.2411417322834647770 ) ) ;
#49747=CARTESIAN_POINT ( 'NONE',  ( 1.351706036745407458, -0.3690944881889765550, -0.3153832671262227771 ) ) ;
#49748=CARTESIAN_POINT ( 'NONE',  ( -0.03937007874015669567, 0.2952755905511811885, 0.000000000000000000 ) ) ;
#49751=CARTESIAN_POINT ( 'NONE',  ( -0.5380577427821514602, 0.05413385826771666132, 0.4176697321401328100 ) ) ;
#49752=CARTESIAN_POINT ( 'NONE',  ( -0.7283464566929126471, 0.07958543189024071263, -0.2665933059059888421 ) ) ;
#49753=CARTESIAN_POINT ( 'NONE',  ( 0.3346456692913390985, 0.1660481256975885056, 0.3530559997133364547 ) ) ;
#49754=CARTESIAN_POINT ( 'NONE',  ( -0.4199475065616791736, 0.2306618581243847221, -0.2411417322834647770 ) ) ;
#49755=CARTESIAN_POINT ( 'NONE',  ( 1.660104986876641320, -0.05778040916215522460, 0.4822834645669289988 ) ) ;
#49756=CARTESIAN_POINT ( 'NONE',  ( 0.09115970038225353067, 3.421639014772782816E-16, 0.3464511005275203726 ) ) ;
#49757=ORIENTED_EDGE ( 'NONE', *, *, #49168, .T. ) ;
#49759=CARTESIAN_POINT ( 'NONE',  ( 0.2099737532808405305, -0.6046776061558807314, 0.2411417322834647770 ) ) ;
#49760=CARTESIAN_POINT ( 'NONE',  ( -0.3805774278215216522, -0.4281496062992127816, -0.4176697321401328100 ) ) ;
#49761=CARTESIAN_POINT ( 'NONE',  ( -1.601049868766403650, 0.2306618581243847221, -0.2411417322834647770 ) ) ;
#49762=CARTESIAN_POINT ( 'NONE',  ( 0.8333333333333340365, 0.2952755905511810774, -0.1292274648535930714 ) ) ;
#49763=CARTESIAN_POINT ( 'NONE',  ( 0.4855643044619430415, -0.4281496062992127816, -0.4176697321401328100 ) ) ;
#49765=CARTESIAN_POINT ( 'NONE',  ( -0.6167979002624665030, 0.05413385826771666132, 0.4176697321401328100 ) ) ;
#49766=CARTESIAN_POINT ( 'NONE',  ( 0.2099737532808405305, -0.6046776061558807314, 0.2411417322834647770 ) ) ;
#49767=CARTESIAN_POINT ( 'NONE',  ( -0.2887139107611542133, -0.6046776061558809534, -0.2411417322834644161 ) ) ;
#49768=CARTESIAN_POINT ( 'NONE',  ( 0.2099737532808405305, -0.5023911411419708095, 0.1820866141732285504 ) ) ;
#49769=CARTESIAN_POINT ( 'NONE',  ( -1.561679790026246017, 0.05413385826771666132, 0.4176697321401328100 ) ) ;
#49771=CARTESIAN_POINT ( 'NONE',  ( -0.2296587926509179312, -0.3162353388693409650, -0.4822834645669289433 ) ) ;
#49772=CYLINDRICAL_SURFACE ( 'NONE', #76221, 1.181102362204724310 ) ;
#49773=CARTESIAN_POINT ( 'NONE',  ( 1.614173228346457378, 0.2952755905511811885, 0.000000000000000000 ) ) ;
#49777=CARTESIAN_POINT ( 'NONE',  ( 0.7545931758530189937, 0.2952755905511810774, -0.1292274648535930714 ) ) ;
#49778=CARTESIAN_POINT ( 'NONE',  ( 0.2034120734908142214, 0.1771653543307087075, -0.09757992244046823083 ) ) ;
#49783=CARTESIAN_POINT ( 'NONE',  ( 0.3038629456265435902, -3.790565315793794774E-16, -0.3954974714151277548 ) ) ;
#49785=CARTESIAN_POINT ( 'NONE',  ( 0.3149606299212603933, -0.1870078740157479769, 0.4822834645669291653 ) ) ;
#49786=CARTESIAN_POINT ( 'NONE',  ( -1.259842519685038686, -0.1870078740157480879, -0.4822834645669291653 ) ) ;
#49787=CARTESIAN_POINT ( 'NONE',  ( -1.181102362204723644, -0.1870078740157480879, -0.4822834645669291653 ) ) ;
#49788=CARTESIAN_POINT ( 'NONE',  ( 0.7152230971128614723, -0.3162353388693409650, -0.4822834645669289433 ) ) ;
#49789=CARTESIAN_POINT ( 'NONE',  ( 0.7742782152230978099, -0.4281496062992124485, 0.4176697321401328655 ) ) ;
#49790=CARTESIAN_POINT ( 'NONE',  ( 1.430446194225722500, -0.3690944881889765550, -0.3153832671262227771 ) ) ;
#49791=CARTESIAN_POINT ( 'NONE',  ( 1.049868766404200349, 0.1283753931104748280, 0.1820866141732283561 ) ) ;
#49792=CARTESIAN_POINT ( 'NONE',  ( -0.9711286089238838626, 0.2306618581243847221, -0.2411417322834647770 ) ) ;
#49794=CARTESIAN_POINT ( 'NONE',  ( 1.620734908136483465, -0.6692913385826771977, 0.1292274648535927661 ) ) ;
#49796=CARTESIAN_POINT ( 'NONE',  ( -0.3346456692913377662, 0.1660481256975883668, -0.3530559997133364547 ) ) ;
#49797=CARTESIAN_POINT ( 'NONE',  ( 1.154855643044620184, -0.6046776061558807314, 0.2411417322834647770 ) ) ;
#49800=CARTESIAN_POINT ( 'NONE',  ( 0.3018372703412079971, 0.05413385826771626580, -0.4176697321401330321 ) ) ;
#49801=CARTESIAN_POINT ( 'NONE',  ( 1.036745406824147508, -0.3690944881889765550, -0.3153832671262227771 ) ) ;
#49804=CARTESIAN_POINT ( 'NONE',  ( -1.207349081364828880, 0.1283753931104746893, -0.1820866141732285504 ) ) ;
#49805=CARTESIAN_POINT ( 'NONE',  ( 1.017060367454068803, -0.3162353388693405765, 0.4822834645669290543 ) ) ;
#49807=CARTESIAN_POINT ( 'NONE',  ( -0.4265091863517051496, 0.1771653543307087075, -0.09757992244046823083 ) ) ;
#49808=CARTESIAN_POINT ( 'NONE',  ( -0.5380577427821514602, -0.4281496062992127816, -0.4176697321401328100 ) ) ;
#49809=CARTESIAN_POINT ( 'NONE',  ( 1.502624671916010790, -0.05778040916215522460, 0.4822834645669289988 ) ) ;
#49810=CARTESIAN_POINT ( 'NONE',  ( -0.7480314960629914633, 0.2952755905511811885, 0.000000000000000000 ) ) ;
#49812=CARTESIAN_POINT ( 'NONE',  ( 1.469816272965879911, -0.6046776061558807314, 0.2411417322834647770 ) ) ;
#49814=CARTESIAN_POINT ( 'NONE',  ( -0.8202099737532799750, 0.1771653543307087075, -0.09757992244046823083 ) ) ;
#49816=CARTESIAN_POINT ( 'NONE',  ( 1.318897637795276356, 0.1660481256975883668, -0.3530559997133364547 ) ) ;
#49818=CARTESIAN_POINT ( 'NONE',  ( -1.272965879265091305, -0.4281496062992124485, 0.4176697321401328655 ) ) ;
#49819=CARTESIAN_POINT ( 'NONE',  ( -1.646981627296586703, -0.08942795157527998196, 0.3641732283464567121 ) ) ;
#49820=CARTESIAN_POINT ( 'NONE',  ( -0.5118110236220466680, -0.5511811023622047445, 6.969142054262312111E-17 ) ) ;
#49821=CARTESIAN_POINT ( 'NONE',  ( -1.620734908136482577, 0.2952755905511811885, 0.1292274648535926551 ) ) ;
#49822=CARTESIAN_POINT ( 'NONE',  ( -0.2099737532808391705, 0.2306618581243848609, 0.2411417322834645549 ) ) ;
#49823=CARTESIAN_POINT ( 'NONE',  ( 0.09842519685039434474, 0.07958543189024085140, 0.2665933059059887866 ) ) ;
#49824=CARTESIAN_POINT ( 'NONE',  ( -1.036745406824146176, -0.004921259842519870586, -0.3153832671262229437 ) ) ;
#49825=CARTESIAN_POINT ( 'NONE',  ( 1.233595800524935227, -0.5023911411419708095, 0.1820866141732285504 ) ) ;
#49826=CARTESIAN_POINT ( 'NONE',  ( 0.9842519685039378130, -0.6692913385826771977, 8.415575281601705876E-17 ) ) ;
#49828=CARTESIAN_POINT ( 'NONE',  ( 0.4133858267716541968, 0.07958543189024085140, 0.2665933059059887866 ) ) ;
#49829=CARTESIAN_POINT ( 'NONE',  ( 0.2887139107611556010, 0.2306618581243847221, -0.2411417322834647770 ) ) ;
#49831=CARTESIAN_POINT ( 'NONE',  ( 0.8858267716535438430, -0.4536011799217368745, -0.2665933059059886201 ) ) ;
#49833=CARTESIAN_POINT ( 'NONE',  ( -1.174540682414697335, -0.05778040916215522460, 0.4822834645669289988 ) ) ;
#49834=CARTESIAN_POINT ( 'NONE',  ( -0.9711286089238838626, 0.2306618581243847221, -0.2411417322834647770 ) ) ;
#49835=CARTESIAN_POINT ( 'NONE',  ( -0.06561679790026180015, -0.4281496062992127816, -0.4176697321401328100 ) ) ;
#49838=CARTESIAN_POINT ( 'NONE',  ( 0.6430446194225728496, 0.05413385826771666132, 0.4176697321401328100 ) ) ;
#49839=CARTESIAN_POINT ( 'NONE',  ( -1.686351706036744558, 0.2952755905511810774, -0.1292274648535930714 ) ) ;
#49840=CARTESIAN_POINT ( 'NONE',  ( 0.01312335958005323398, -0.4281496062992127816, -0.4176697321401328100 ) ) ;
#49841=CARTESIAN_POINT ( 'NONE',  ( 0.8464566929133865436, 0.1660481256975883668, -0.3530559997133364547 ) ) ;
#49847=CARTESIAN_POINT ( 'NONE',  ( -0.6758530183727028406, -0.5511811023622048555, -0.09757992244046775898 ) ) ;
#49848=CARTESIAN_POINT ( 'NONE',  ( -0.9448818897637790704, -0.1870078740157479769, 0.4822834645669291653 ) ) ;
#49849=CARTESIAN_POINT ( 'NONE',  ( 0.5118110236220478892, 0.2952755905511811885, 0.000000000000000000 ) ) ;
#49851=CARTESIAN_POINT ( 'NONE',  ( 0.9514435695538062676, -0.3162353388693409650, -0.4822834645669289433 ) ) ;
#49852=CARTESIAN_POINT ( 'NONE',  ( -1.646981627296586703, -0.05778040916215522460, 0.4822834645669289988 ) ) ;
#49853=CARTESIAN_POINT ( 'NONE',  ( 0.7217847769028878924, -0.4281496062992127816, -0.4176697321401328100 ) ) ;
#49856=FACE_OUTER_BOUND ( 'NONE', #9298, .T. ) ;
#49857=CARTESIAN_POINT ( 'NONE',  ( 0.9580052493438326877, 0.05413385826771666132, 0.4176697321401328100 ) ) ;
#49858=CARTESIAN_POINT ( 'NONE',  ( 0.7874015748031503170, -0.1870078740157479769, 0.4822834645669291653 ) ) ;
#49859=CARTESIAN_POINT ( 'NONE',  ( 1.049868766404200127, -0.5023911411419708095, -0.1820866141732282451 ) ) ;
#49860=CARTESIAN_POINT ( 'NONE',  ( -1.568241469816272105, -0.2845877964562161244, -0.3641732283464567121 ) ) ;
#49861=CARTESIAN_POINT ( 'NONE',  ( -1.574803149606298192, -0.1870078740157480879, -0.4822834645669291653 ) ) ;
#49864=CARTESIAN_POINT ( 'NONE',  ( 0.9120734908136490793, 0.2952755905511810774, -0.1292274648535930714 ) ) ;
#49865=CARTESIAN_POINT ( 'NONE',  ( 1.541994750656168645, 0.1771653543307087075, -0.09757992244046823083 ) ) ;
#49866=CARTESIAN_POINT ( 'NONE',  ( -0.5643044619422565855, 0.05413385826771626580, -0.4176697321401330321 ) ) ;
#49867=CARTESIAN_POINT ( 'NONE',  ( -1.089238845144356427, 0.05413385826771666132, 0.4176697321401328100 ) ) ;
#49869=CARTESIAN_POINT ( 'NONE',  ( -1.568241469816272105, -0.3162353388693409650, -0.4822834645669289433 ) ) ;
#49873=CARTESIAN_POINT ( 'NONE',  ( -1.528871391076114250, -0.5511811023622046335, 0.09757992244046803654 ) ) ;
#49877=CARTESIAN_POINT ( 'NONE',  ( -0.04593175853018303251, 0.2066929133858267931, 0.1054918080437490802 ) ) ;
#49878=CARTESIAN_POINT ( 'NONE',  ( 1.318897637795276356, 0.07958543189024071263, -0.2665933059059888421 ) ) ;
#49880=LINE ( 'NONE', #22977, #4833 ) ;
#49882=CARTESIAN_POINT ( 'NONE',  ( 0.4935044252197980930, 1.488513638086841118, 0.5309055118110234117 ) ) ;
#49885=CARTESIAN_POINT ( 'NONE',  ( -0.8858267716535425107, -0.4536011799217367080, 0.2665933059059888421 ) ) ;
#49886=CARTESIAN_POINT ( 'NONE',  ( -1.115485564304461219, -0.3690944881889763329, 0.3153832671262228327 ) ) ;
#49887=CARTESIAN_POINT ( 'NONE',  ( -1.128608923884513837, 0.2306618581243847221, -0.2411417322834647770 ) ) ;
#49888=CARTESIAN_POINT ( 'NONE',  ( 0.2230971128608929543, 0.05413385826771626580, -0.4176697321401330321 ) ) ;
#49889=CARTESIAN_POINT ( 'NONE',  ( -1.325459317585300889, 0.05413385826771666132, 0.4176697321401328100 ) ) ;
#49892=CARTESIAN_POINT ( 'NONE',  ( 1.397637795275591177, -0.5400638737290844871, 0.3530559997133364547 ) ) ;
#49893=CARTESIAN_POINT ( 'NONE',  ( -1.092353285368623750, -2.191421614605370878E-15, 0.4445507791589071167 ) ) ;
#49896=CARTESIAN_POINT ( 'NONE',  ( -1.646051170424378096, 0.8346805926620876059, 0.3149606299212598381 ) ) ;
#49897=CARTESIAN_POINT ( 'NONE',  ( -0.3215223097112853146, -0.08942795157528024563, -0.3641732283464568787 ) ) ;
#49899=CARTESIAN_POINT ( 'NONE',  ( -1.062992125984250968, -0.6692913385826771977, 8.415575281601705876E-17 ) ) ;
#49900=CARTESIAN_POINT ( 'NONE',  ( 1.023622047244095334, -0.1870078740157479769, 0.4822834645669291653 ) ) ;
#49904=CARTESIAN_POINT ( 'NONE',  ( 1.581364829396326277, -0.3162353388693409650, -0.4822834645669289433 ) ) ;
#49905=CARTESIAN_POINT ( 'NONE',  ( -1.377952755905511140, 0.2952755905511811885, 0.000000000000000000 ) ) ;
#49907=EDGE_CURVE ( 'NONE', #62516, #47058, #53398, .T. ) ;
#49908=CARTESIAN_POINT ( 'NONE',  ( -0.1443569553805768291, -0.004921259842519576551, 0.3153832671262227771 ) ) ;
#49910=CARTESIAN_POINT ( 'NONE',  ( -0.1771653543307080136, 0.07958543189024071263, -0.2665933059059888421 ) ) ;
#49911=CARTESIAN_POINT ( 'NONE',  ( 0.3805774278215230400, -0.004921259842519870586, -0.3153832671262229437 ) ) ;
#49912=CARTESIAN_POINT ( 'NONE',  ( 0.5118110236220478892, 0.2952755905511811885, 0.000000000000000000 ) ) ;
#49913=CARTESIAN_POINT ( 'NONE',  ( -0.7217847769028863381, -0.3690944881889763329, 0.3153832671262228327 ) ) ;
#49915=CARTESIAN_POINT ( 'NONE',  ( 1.141732283464567566, 0.2952755905511811885, 0.000000000000000000 ) ) ;
#49916=CARTESIAN_POINT ( 'NONE',  ( -0.9514435695538050464, -0.05778040916215560624, -0.4822834645669293319 ) ) ;
#49918=CARTESIAN_POINT ( 'NONE',  ( 0.006561679790026889343, -0.05778040916215522460, 0.4822834645669289988 ) ) ;
#49919=CARTESIAN_POINT ( 'NONE',  ( -0.3346456692913377662, 0.1660481256975883668, -0.3530559997133364547 ) ) ;
#49920=CARTESIAN_POINT ( 'NONE',  ( 1.410761154855643795, -0.08942795157528024563, -0.3641732283464568787 ) ) ;
#49921=CARTESIAN_POINT ( 'NONE',  ( 0.2559055118110243332, -0.4536011799217368745, -0.2665933059059886201 ) ) ;
#49922=CARTESIAN_POINT ( 'NONE',  ( -0.2821522309711278487, 0.2952755905511811885, 0.1292274648535926551 ) ) ;
#49923=CARTESIAN_POINT ( 'NONE',  ( -1.082677165354329896, -0.5400638737290845981, -0.3530559997133363437 ) ) ;
#49925=CARTESIAN_POINT ( 'NONE',  ( 0.3937007874015751585, 1.771653543307086354, 0.000000000000000000 ) ) ;
#49926=CARTESIAN_POINT ( 'NONE',  ( -0.1968503937007867743, 0.2952755905511811885, 0.000000000000000000 ) ) ;
#49928=ORIENTED_EDGE ( 'NONE', *, *, #38011, .F. ) ;
#49930=CARTESIAN_POINT ( 'NONE',  ( 1.003937007874016185, 0.1660481256975883668, -0.3530559997133364547 ) ) ;
#49931=CARTESIAN_POINT ( 'NONE',  ( -0.5446194225721777693, -0.2845877964562161244, -0.3641732283464567121 ) ) ;
#49932=CARTESIAN_POINT ( 'NONE',  ( -0.4527559055118102749, 0.1660481256975885056, 0.3530559997133364547 ) ) ;
#49933=CARTESIAN_POINT ( 'NONE',  ( 1.410761154855643795, -0.05778040916215560624, -0.4822834645669293319 ) ) ;
#49934=CARTESIAN_POINT ( 'NONE',  ( 0.9055118110236227702, 0.2952755905511811885, 0.000000000000000000 ) ) ;
#49935=FACE_OUTER_BOUND ( 'NONE', #23693, .T. ) ;
#49936=CARTESIAN_POINT ( 'NONE',  ( -1.069553805774277722, 0.1771653543307087630, 0.09757992244046791164 ) ) ;
#49941=CARTESIAN_POINT ( 'NONE',  ( 1.036745406824147731, -0.004921259842519576551, 0.3153832671262227771 ) ) ;
#49942=CARTESIAN_POINT ( 'NONE',  ( 0.5249343832021003964, 0.1283753931104746893, -0.1820866141732285504 ) ) ;
#49943=CARTESIAN_POINT ( 'NONE',  ( 0.3083989501312343062, -0.3162353388693405765, 0.4822834645669290543 ) ) ;
#49944=DIRECTION ( 'NONE',  ( 0.000000000000000000, 0.000000000000000000, -1.000000000000000000 ) ) ;
#49946=CARTESIAN_POINT ( 'NONE',  ( 0.8202099737532814183, -0.5511811023622048555, -0.09757992244046775898 ) ) ;
#49947=CARTESIAN_POINT ( 'NONE',  ( -0.3346456692913377662, 0.1660481256975883668, -0.3530559997133364547 ) ) ;
#49948=CARTESIAN_POINT ( 'NONE',  ( -0.6955380577427815458, 0.05413385826771666132, 0.4176697321401328100 ) ) ;
#49949=CARTESIAN_POINT ( 'NONE',  ( 1.371391076115485941, 0.2952755905511811885, 0.1292274648535926551 ) ) ;
#49952=CARTESIAN_POINT ( 'NONE',  ( -0.1312335958005241554, 0.1283753931104748280, 0.1820866141732283561 ) ) ;
#49956=CARTESIAN_POINT ( 'NONE',  ( -0.8136482939632537770, -0.6046776061558807314, 0.2411417322834647770 ) ) ;
#49958=CARTESIAN_POINT ( 'NONE',  ( -0.3083989501312330295, -0.3162353388693409650, -0.4822834645669289433 ) ) ;
#49959=CARTESIAN_POINT ( 'NONE',  ( -0.3543307086614165824, 0.2952755905511811885, 0.000000000000000000 ) ) ;
#49960=CARTESIAN_POINT ( 'NONE',  ( 0.3280839895013130669, -0.4281496062992127816, -0.4176697321401328100 ) ) ;
#49961=CARTESIAN_POINT ( 'NONE',  ( -0.5380577427821514602, 0.05413385826771666132, 0.4176697321401328100 ) ) ;
#49962=CARTESIAN_POINT ( 'NONE',  ( -1.417322834645668772, -0.1870078740157480879, -0.4822834645669291653 ) ) ;
#49963=CARTESIAN_POINT ( 'NONE',  ( -0.6824146981627291497, -0.6046776061558809534, -0.2411417322834644161 ) ) ;
#49964=CARTESIAN_POINT ( 'NONE',  ( 0.6627296587926515548, 0.2952755905511811885, 0.1292274648535926551 ) ) ;
#49966=CARTESIAN_POINT ( 'NONE',  ( -0.2887139107611542133, -0.5023911411419708095, -0.1820866141732282451 ) ) ;
#49967=ORIENTED_EDGE ( 'NONE', *, *, #53789, .T. ) ;
#49970=CARTESIAN_POINT ( 'NONE',  ( -1.108923884514435132, -0.2845877964562159024, 0.3641732283464567677 ) ) ;
#49971=CARTESIAN_POINT ( 'NONE',  ( -0.9908136482939626788, 0.2952755905511811885, 0.1292274648535926551 ) ) ;
#49972=CARTESIAN_POINT ( 'NONE',  ( -0.7939632545931750718, -0.05778040916215560624, -0.4822834645669293319 ) ) ;
#49973=CARTESIAN_POINT ( 'NONE',  ( 0.4624320255261049062, 8.471767977567108961E-16, -0.4445507791589058955 ) ) ;
#49974=CARTESIAN_POINT ( 'NONE',  ( -0.5839895013123351797, 0.2952755905511810774, -0.1292274648535930714 ) ) ;
#49975=CARTESIAN_POINT ( 'NONE',  ( -0.6824146981627291497, -0.6046776061558809534, -0.2411417322834644161 ) ) ;
#49978=CARTESIAN_POINT ( 'NONE',  ( 0.4593175853018380828, -0.004921259842519870586, -0.3153832671262229437 ) ) ;
#49979=LINE ( 'NONE', #76499, #32326 ) ;
#49981=CARTESIAN_POINT ( 'NONE',  ( -0.08530183727034056085, -0.08942795157528024563, -0.3641732283464568787 ) ) ;
#49982=CARTESIAN_POINT ( 'NONE',  ( -0.1902887139107604098, 0.2952755905511810774, -0.1292274648535930714 ) ) ;
#49984=CARTESIAN_POINT ( 'NONE',  ( 8.195543980992789655E-16, -0.1870078740157480879, -0.4822834645669291653 ) ) ;
#49985=ORIENTED_EDGE ( 'NONE', *, *, #61823, .T. ) ;
#49992=CARTESIAN_POINT ( 'NONE',  ( -1.213910761154854745, 0.1771653543307087075, -0.09757992244046823083 ) ) ;
#49993=CARTESIAN_POINT ( 'NONE',  ( -1.338582677165353729, -0.1870078740157480879, -0.4822834645669291653 ) ) ;
#49995=CARTESIAN_POINT ( 'NONE',  ( 0.4037097067573611753, 1.223219560026271499E-15, 0.4445507791589056734 ) ) ;
#49997=CARTESIAN_POINT ( 'NONE',  ( 1.325459317585302665, -0.4281496062992124485, 0.4176697321401328655 ) ) ;
#49998=CARTESIAN_POINT ( 'NONE',  ( 0.6299212598425204535, -0.1870078740157479769, 0.4822834645669291653 ) ) ;
#49999=CARTESIAN_POINT ( 'NONE',  ( -0.09842519685039295696, -0.5400638737290844871, 0.3530559997133364547 ) ) ;
#50000=CARTESIAN_POINT ( 'NONE',  ( -0.9317585301837263412, -0.3690944881889765550, -0.3153832671262227771 ) ) ;
#50001=CARTESIAN_POINT ( 'NONE',  ( -0.3412073490813641308, -0.6046776061558807314, 0.2411417322834647770 ) ) ;
#50003=CARTESIAN_POINT ( 'NONE',  ( -0.8792650918635160906, 0.05413385826771626580, -0.4176697321401330321 ) ) ;
#50005=CARTESIAN_POINT ( 'NONE',  ( 1.305774278215223960, 0.1771653543307087075, -0.09757992244046823083 ) ) ;
#50006=CARTESIAN_POINT ( 'NONE',  ( -0.5249343832020990641, -0.5023911411419708095, -0.1820866141732282451 ) ) ;
#50007=CARTESIAN_POINT ( 'NONE',  ( 1.299212598425197429, -0.5511811023622047445, 6.969142054262312111E-17 ) ) ;
#50008=CARTESIAN_POINT ( 'NONE',  ( -1.482939632545930975, -0.4281496062992127816, -0.4176697321401328100 ) ) ;
#50009=CARTESIAN_POINT ( 'NONE',  ( -1.207349081364828436, -0.5023911411419708095, 0.1820866141732285504 ) ) ;
#50010=CARTESIAN_POINT ( 'NONE',  ( 0.1459841489473573395, 2.110655687203366066E-15, -0.3791475997938226761 ) ) ;
#50011=CARTESIAN_POINT ( 'NONE',  ( 0.3871391076115493490, -0.2845877964562159024, 0.3641732283464567677 ) ) ;
#50012=CARTESIAN_POINT ( 'NONE',  ( -0.4133858267716528645, -0.5400638737290844871, 0.3530559997133364547 ) ) ;
#50014=CARTESIAN_POINT ( 'NONE',  ( -0.006561679790025524116, -0.08942795157528024563, -0.3641732283464568787 ) ) ;
#50016=CARTESIAN_POINT ( 'NONE',  ( 0.8070866141732289112, -0.5400638737290845981, -0.3530559997133363437 ) ) ;
#50018=CARTESIAN_POINT ( 'NONE',  ( 1.240157480314961314, -0.4536011799217367080, 0.2665933059059888421 ) ) ;
#50019=CARTESIAN_POINT ( 'NONE',  ( -0.8595800524934373854, -0.3162353388693409650, -0.4822834645669289433 ) ) ;
#50020=CARTESIAN_POINT ( 'NONE',  ( -0.3083989501312330295, -0.2845877964562161244, -0.3641732283464567121 ) ) ;
#50021=CARTESIAN_POINT ( 'NONE',  ( 1.033630966599880630, -4.927456884911482678E-16, 0.4445507791589062840 ) ) ;
#50022=CARTESIAN_POINT ( 'NONE',  ( 0.3018372703412079971, -0.3690944881889763329, 0.3153832671262228327 ) ) ;
#50023=CARTESIAN_POINT ( 'NONE',  ( -1.135170603674539924, -0.6692913385826771977, 0.1292274648535927661 ) ) ;
#50024=EDGE_CURVE ( 'NONE', #22657, #65086, #50517, .T. ) ;
#50025=CARTESIAN_POINT ( 'NONE',  ( -0.5380577427821514602, 0.05413385826771666132, 0.4176697321401328100 ) ) ;
#50029=CARTESIAN_POINT ( 'NONE',  ( 0.4068241469816279987, -0.3690944881889765550, -0.3153832671262227771 ) ) ;
#50030=CARTESIAN_POINT ( 'NONE',  ( -0.2034120734908128059, 0.2952755905511811885, 0.1292274648535926551 ) ) ;
#50031=CARTESIAN_POINT ( 'NONE',  ( -0.5249343832020990641, 0.2306618581243848609, 0.2411417322834645549 ) ) ;
#50032=CARTESIAN_POINT ( 'NONE',  ( -0.7152230971128602510, -0.2845877964562159024, 0.3641732283464567677 ) ) ;
#50034=CARTESIAN_POINT ( 'NONE',  ( 0.02624671916010564918, -0.6046776061558809534, -0.2411417322834644161 ) ) ;
#50035=CARTESIAN_POINT ( 'NONE',  ( -1.154855643044618851, -0.5023911411419708095, -0.1820866141732282451 ) ) ;
#50036=CARTESIAN_POINT ( 'NONE',  ( -1.607611548556429737, 0.2952755905511810774, -0.1292274648535930714 ) ) ;
#50040=CARTESIAN_POINT ( 'NONE',  ( -1.699475065616797398, 0.1771653543307087630, 0.09757992244046791164 ) ) ;
#50041=CARTESIAN_POINT ( 'NONE',  ( -1.391076115485563758, 0.2306618581243848609, 0.2411417322834645549 ) ) ;
#50043=CARTESIAN_POINT ( 'NONE',  ( -0.7217847769028863381, 0.05413385826771626580, -0.4176697321401330321 ) ) ;
#50044=CARTESIAN_POINT ( 'NONE',  ( -1.489501312335957062, -0.05778040916215522460, 0.4822834645669289988 ) ) ;
#50048=CARTESIAN_POINT ( 'NONE',  ( 1.154855643044620184, -0.6046776061558807314, 0.2411417322834647770 ) ) ;
#50049=CARTESIAN_POINT ( 'NONE',  ( 0.5643044619422579178, 0.05413385826771666132, 0.4176697321401328100 ) ) ;
#50052=CARTESIAN_POINT ( 'NONE',  ( 1.279527559055118724, 0.07958543189024085140, 0.2665933059059887866 ) ) ;
#50057=CARTESIAN_POINT ( 'NONE',  ( 0.4396325459317590445, -0.6692913385826771977, 0.1292274648535927661 ) ) ;
#50058=CARTESIAN_POINT ( 'NONE',  ( -0.7611548556430438595, 0.2306618581243848609, 0.2411417322834645549 ) ) ;
#50059=CARTESIAN_POINT ( 'NONE',  ( 1.581364829396326277, -0.05778040916215522460, 0.4822834645669289988 ) ) ;
#50060=CARTESIAN_POINT ( 'NONE',  ( 1.266404199475066328, -0.3162353388693409650, -0.4822834645669289433 ) ) ;
#50061=CARTESIAN_POINT ( 'NONE',  ( 1.587926509186352586, -0.4281496062992127816, -0.4176697321401328100 ) ) ;
#50063=CARTESIAN_POINT ( 'NONE',  ( -0.1115485564304453947, -0.6692913385826771977, 0.1292274648535927661 ) ) ;
#50064=CARTESIAN_POINT ( 'NONE',  ( -1.410761154855641575, -0.3162353388693409650, -0.4822834645669289433 ) ) ;
#50065=CARTESIAN_POINT ( 'NONE',  ( -1.496062992125983815, -0.1870078740157479769, 0.4822834645669291653 ) ) ;
#50066=CARTESIAN_POINT ( 'NONE',  ( 1.423884514435696413, -0.3162353388693409650, -0.4822834645669289433 ) ) ;
#50068=CARTESIAN_POINT ( 'NONE',  ( 0.7020997375328090762, -0.2845877964562159024, 0.3641732283464567677 ) ) ;
#50069=ORIENTED_EDGE ( 'NONE', *, *, #4912, .T. ) ;
#50072=CARTESIAN_POINT ( 'NONE',  ( -0.05249343832020938322, -0.5023911411419708095, -0.1820866141732282451 ) ) ;
#50074=CARTESIAN_POINT ( 'NONE',  ( 0.7480314960629927956, -0.6692913385826771977, 8.415575281601705876E-17 ) ) ;
#50075=CARTESIAN_POINT ( 'NONE',  ( 0.2821522309711292364, -0.6692913385826771977, 0.1292274648535927661 ) ) ;
#50076=CARTESIAN_POINT ( 'NONE',  ( -0.6758530183727028406, -0.6692913385826773087, -0.1292274648535924053 ) ) ;
#50078=CARTESIAN_POINT ( 'NONE',  ( -1.279527559055116948, 0.1660481256975883668, -0.3530559997133364547 ) ) ;
#50080=CARTESIAN_POINT ( 'NONE',  ( 1.450131233595801428, 0.1771653543307087630, 0.09757992244046791164 ) ) ;
#50081=CARTESIAN_POINT ( 'NONE',  ( -1.108923884514435132, -0.05778040916215560624, -0.4822834645669293319 ) ) ;
#50082=CARTESIAN_POINT ( 'NONE',  ( 0.8267716535433078384, -0.6692913385826771977, 8.415575281601705876E-17 ) ) ;
#50083=CARTESIAN_POINT ( 'NONE',  ( 1.187664041994751285, -0.05778040916215522460, 0.4822834645669289988 ) ) ;
#50085=CARTESIAN_POINT ( 'NONE',  ( -1.292650918635170010, -0.6692913385826771977, 0.1292274648535927661 ) ) ;
#50087=CARTESIAN_POINT ( 'NONE',  ( 0.2427821522309716595, -0.3162353388693409650, -0.4822834645669289433 ) ) ;
#50090=CARTESIAN_POINT ( 'NONE',  ( 1.646981627296588035, -0.3162353388693405765, 0.4822834645669290543 ) ) ;
#50091=CARTESIAN_POINT ( 'NONE',  ( 0.1509186351706045259, -0.08942795157528024563, -0.3641732283464568787 ) ) ;
#50092=CARTESIAN_POINT ( 'NONE',  ( 0.8989501312335963501, -0.6692913385826773087, -0.1292274648535924053 ) ) ;
#50094=CARTESIAN_POINT ( 'NONE',  ( 0.8136482939632553313, -0.5023911411419708095, -0.1820866141732282451 ) ) ;
#50095=CARTESIAN_POINT ( 'NONE',  ( 0.3477690288713918276, 0.2952755905511811885, 0.1292274648535926551 ) ) ;
#50097=CARTESIAN_POINT ( 'NONE',  ( -0.9580052493438311334, -0.4281496062992124485, 0.4176697321401328655 ) ) ;
#50098=CARTESIAN_POINT ( 'NONE',  ( -1.646051170424378096, 0.000000000000000000, 0.3464511005275205946 ) ) ;
#50099=CARTESIAN_POINT ( 'NONE',  ( 0.8005249343832027131, -0.004921259842519576551, 0.3153832671262227771 ) ) ;
#50101=CARTESIAN_POINT ( 'NONE',  ( -0.2887139107611542133, 0.2306618581243848609, 0.2411417322834645549 ) ) ;
#50102=CARTESIAN_POINT ( 'NONE',  ( 0.2296587926509192634, -0.2845877964562159024, 0.3641732283464567677 ) ) ;
#50104=CARTESIAN_POINT ( 'NONE',  ( -0.4658792650918627265, -0.05778040916215522460, 0.4822834645669289988 ) ) ;
#50105=CARTESIAN_POINT ( 'NONE',  ( 0.7611548556430451917, -0.5023911411419708095, 0.1820866141732285504 ) ) ;
#50106=CARTESIAN_POINT ( 'NONE',  ( -1.114781747626346187, -2.609869883881465018E-15, -0.3464511005275220379 ) ) ;
#50107=EDGE_CURVE ( 'NONE', #42092, #56464, #25662, .T. ) ;
#50109=CARTESIAN_POINT ( 'NONE',  ( 0.1771653543307093182, -0.5400638737290845981, -0.3530559997133363437 ) ) ;
#50110=CARTESIAN_POINT ( 'NONE',  ( 1.292650918635171564, -0.5511811023622048555, -0.09757992244046775898 ) ) ;
#50112=CARTESIAN_POINT ( 'NONE',  ( -0.4855643044619415427, -0.3690944881889763329, 0.3153832671262228327 ) ) ;
#50113=CARTESIAN_POINT ( 'NONE',  ( -0.6430446194225716283, -0.3690944881889763329, 0.3153832671262228327 ) ) ;
#50114=CARTESIAN_POINT ( 'NONE',  ( -0.5052493438320203589, 0.2952755905511810774, -0.1292274648535930714 ) ) ;
#50115=CARTESIAN_POINT ( 'NONE',  ( 0.1640419947506569498, -0.05778040916215522460, 0.4822834645669289988 ) ) ;
#50116=CARTESIAN_POINT ( 'NONE',  ( 1.043307086614173818, 0.07958543189024085140, 0.2665933059059887866 ) ) ;
#50117=CARTESIAN_POINT ( 'NONE',  ( -1.686351706036744558, 0.1771653543307087075, -0.09757992244046823083 ) ) ;
#50118=CARTESIAN_POINT ( 'NONE',  ( -1.699475065616797398, 0.2952755905511811885, 0.1292274648535926551 ) ) ;
#50119=CARTESIAN_POINT ( 'NONE',  ( 0.9383202099737538715, -0.05778040916215560624, -0.4822834645669293319 ) ) ;
#50121=CARTESIAN_POINT ( 'NONE',  ( -0.3674540682414692561, -0.6046776061558809534, -0.2411417322834644161 ) ) ;
#50123=CARTESIAN_POINT ( 'NONE',  ( 0.9711286089238851948, -0.6046776061558809534, -0.2411417322834644161 ) ) ;
#50124=CARTESIAN_POINT ( 'NONE',  ( 0.5446194225721792126, -0.3162353388693405765, 0.4822834645669290543 ) ) ;
#50126=CARTESIAN_POINT ( 'NONE',  ( 0.4396325459317593221, 0.1771653543307087075, -0.09757992244046823083 ) ) ;
#50127=CARTESIAN_POINT ( 'NONE',  ( 1.246719160104987623, 0.05413385826771626580, -0.4176697321401330321 ) ) ;
#50128=CARTESIAN_POINT ( 'NONE',  ( 0.1902887139107617975, 0.1771653543307087630, 0.09757992244046791164 ) ) ;
#50129=CARTESIAN_POINT ( 'NONE',  ( -0.3740157480314953431, 0.1660481256975885056, 0.3530559997133364547 ) ) ;
#50130=CARTESIAN_POINT ( 'NONE',  ( -0.7137454485294948414, 2.793565526369265584, 0.4917280318828576857 ) ) ;
#50131=CARTESIAN_POINT ( 'NONE',  ( 0.2427821522309716595, -0.3162353388693409650, -0.4822834645669289433 ) ) ;
#50132=CARTESIAN_POINT ( 'NONE',  ( -0.7480314960629914633, -0.6692913385826771977, 8.415575281601705876E-17 ) ) ;
#50134=CARTESIAN_POINT ( 'NONE',  ( -0.2821522309711278487, 0.1771653543307087630, 0.09757992244046791164 ) ) ;
#50135=B_SPLINE_CURVE_WITH_KNOTS ( 'NONE', 3,
 ( #7561, #33233, #1255, #59719 ),
 .UNSPECIFIED., .F., .F.,
 ( 4, 4 ),
 ( 3.210432057730625665E-07, 0.001287787053612126763 ),
 .UNSPECIFIED. ) ;
#50136=CARTESIAN_POINT ( 'NONE',  ( 0.4002624671916016896, -0.3162353388693409650, -0.4822834645669289433 ) ) ;
#50137=CARTESIAN_POINT ( 'NONE',  ( 0.8202099737532814183, -0.5511811023622048555, -0.09757992244046775898 ) ) ;
#50138=CARTESIAN_POINT ( 'NONE',  ( -0.3018372703412066094, -0.4281496062992127816, -0.4176697321401328100 ) ) ;
#50140=CARTESIAN_POINT ( 'NONE',  ( 0.6986524979670498681, 8.471767977567108961E-16, -0.4445507791589058955 ) ) ;
#50141=CARTESIAN_POINT ( 'NONE',  ( 1.482939632545932307, 0.05413385826771626580, -0.4176697321401330321 ) ) ;
#50142=CARTESIAN_POINT ( 'NONE',  ( 1.660104986876641320, -0.05778040916215522460, 0.4822834645669289988 ) ) ;
#50144=CARTESIAN_POINT ( 'NONE',  ( -1.076115485564303809, -0.6046776061558809534, -0.2411417322834644161 ) ) ;
#50145=CARTESIAN_POINT ( 'NONE',  ( -0.9317585301837263412, 0.05413385826771666132, 0.4176697321401328100 ) ) ;
#50148=ORIENTED_EDGE ( 'NONE', *, *, #41951, .T. ) ;
#50149=CARTESIAN_POINT ( 'NONE',  ( 0.3805774278215230400, -0.3690944881889763329, 0.3153832671262228327 ) ) ;
#50152=CARTESIAN_POINT ( 'NONE',  ( 0.8792650918635177559, -0.4281496062992127816, -0.4176697321401328100 ) ) ;
#50155=CARTESIAN_POINT ( 'NONE',  ( -0.3083989501312330295, -0.2845877964562161244, -0.3641732283464567121 ) ) ;
#50156=CARTESIAN_POINT ( 'NONE',  ( -0.2690288713910753970, 0.2952755905511810219, -0.1292274648535930437 ) ) ;
#50157=CARTESIAN_POINT ( 'NONE',  ( 1.194225721784777594, 0.05413385826771666132, 0.4176697321401328100 ) ) ;
#50158=CARTESIAN_POINT ( 'NONE',  ( 1.489501312335958172, -0.08942795157528024563, -0.3641732283464568787 ) ) ;
#50159=CARTESIAN_POINT ( 'NONE',  ( -0.1049868766404193215, -0.6046776061558807314, 0.2411417322834647770 ) ) ;
#50161=CARTESIAN_POINT ( 'NONE',  ( -0.4133858267716528645, -0.5400638737290844871, 0.3530559997133364547 ) ) ;
#50162=CARTESIAN_POINT ( 'NONE',  ( -1.154855643044618851, -0.5023911411419708095, -0.1820866141732282451 ) ) ;
#50163=CARTESIAN_POINT ( 'NONE',  ( -0.6364829396325453192, -0.3162353388693405765, 0.4822834645669290543 ) ) ;
#50164=CARTESIAN_POINT ( 'NONE',  ( -1.646051170424378096, 0.000000000000000000, 0.3464511005275205946 ) ) ;
#50166=ORIENTED_EDGE ( 'NONE', *, *, #39397, .F. ) ;
#50168=CARTESIAN_POINT ( 'NONE',  ( 0.6036745406824154392, 0.2306618581243847221, -0.2411417322834647770 ) ) ;
#50170=CARTESIAN_POINT ( 'NONE',  ( -0.3674540682414692561, -0.6046776061558809534, -0.2411417322834644161 ) ) ;
#50171=CARTESIAN_POINT ( 'NONE',  ( -1.351706036745406347, -0.4281496062992124485, 0.4176697321401328655 ) ) ;
#50173=CARTESIAN_POINT ( 'NONE',  ( 0.8792650918635177559, -0.4281496062992127816, -0.4176697321401328100 ) ) ;
#50174=CARTESIAN_POINT ( 'NONE',  ( -0.03937007874015669567, 0.2952755905511811885, 0.000000000000000000 ) ) ;
#50176=CARTESIAN_POINT ( 'NONE',  ( -0.8202099737532801971, -0.6692913385826771977, 0.1292274648535927661 ) ) ;
#50177=CARTESIAN_POINT ( 'NONE',  ( 0.3083989501312343062, -0.05778040916215560624, -0.4822834645669293319 ) ) ;
#50178=CARTESIAN_POINT ( 'NONE',  ( -0.5577427821522301654, -0.3162353388693405765, 0.4822834645669290543 ) ) ;
#50180=CARTESIAN_POINT ( 'NONE',  ( 0.2034120734908144990, -0.5511811023622046335, 0.09757992244046803654 ) ) ;
#50182=CARTESIAN_POINT ( 'NONE',  ( -0.09842519685039295696, 0.1660481256975883668, -0.3530559997133364547 ) ) ;
#50183=CARTESIAN_POINT ( 'NONE',  ( 1.522309711286089939, -0.6046776061558809534, -0.2411417322834644161 ) ) ;
#50186=ORIENTED_EDGE ( 'NONE', *, *, #81979, .T. ) ;
#50187=CARTESIAN_POINT ( 'NONE',  ( 0.7414698162729663755, 0.2952755905511811885, 0.1292274648535926551 ) ) ;
#50188=CARTESIAN_POINT ( 'NONE',  ( 0.3215223097112867578, -0.08942795157527998196, 0.3641732283464567121 ) ) ;
#50189=CARTESIAN_POINT ( 'NONE',  ( 0.9568149321855670131, 1.522401787774001735E-16, 0.3627985898453514046 ) ) ;
#50190=DIRECTION ( 'NONE',  ( 0.000000000000000000, -1.000000000000000000, 0.000000000000000000 ) ) ;
#50195=CARTESIAN_POINT ( 'NONE',  ( 0.3215223097112867578, -0.05778040916215522460, 0.4822834645669289988 ) ) ;
#50196=CARTESIAN_POINT ( 'NONE',  ( -1.023622047244093558, -0.1870078740157479769, 0.4822834645669291653 ) ) ;
#50198=CARTESIAN_POINT ( 'NONE',  ( -0.9711286089238838626, -0.6046776061558807314, 0.2411417322834647770 ) ) ;
#50199=CARTESIAN_POINT ( 'NONE',  ( 0.1968503937007881344, 0.2952755905511811885, 0.000000000000000000 ) ) ;
#50200=CARTESIAN_POINT ( 'NONE',  ( 1.023622047244095112, -0.1870078740157480879, -0.4822834645669291653 ) ) ;
#50201=CARTESIAN_POINT ( 'NONE',  ( 1.358267716535433323, 0.07958543189024085140, 0.2665933059059887866 ) ) ;
#50202=CARTESIAN_POINT ( 'NONE',  ( 1.187664041994751285, -0.08942795157527998196, 0.3641732283464567121 ) ) ;
#50203=CARTESIAN_POINT ( 'NONE',  ( -0.8070866141732276899, 0.1660481256975883668, -0.3530559997133364547 ) ) ;
#50205=CARTESIAN_POINT ( 'NONE',  ( -1.594488188976377119, 0.07958543189024071263, -0.2665933059059888421 ) ) ;
#50207=CARTESIAN_POINT ( 'NONE',  ( -0.2296587926509179312, -0.05778040916215522460, 0.4822834645669289988 ) ) ;
#50208=CARTESIAN_POINT ( 'NONE',  ( 1.332020997375329197, -0.3162353388693405765, 0.4822834645669290543 ) ) ;
#50209=CARTESIAN_POINT ( 'NONE',  ( -1.220472440944881054, 2.362204724409448620, 0.5309055118110237448 ) ) ;
#50210=CARTESIAN_POINT ( 'NONE',  ( -1.450131233595799651, -0.5511811023622046335, 0.09757992244046803654 ) ) ;
#50211=CARTESIAN_POINT ( 'NONE',  ( 0.05249343832021075018, -0.6046776061558807314, 0.2411417322834647770 ) ) ;
#50212=CARTESIAN_POINT ( 'NONE',  ( 0.8989501312335963501, -0.5511811023622048555, -0.09757992244046775898 ) ) ;
#50215=CARTESIAN_POINT ( 'NONE',  ( -1.482939632545930975, -0.3690944881889765550, -0.3153832671262227771 ) ) ;
#50216=CARTESIAN_POINT ( 'NONE',  ( 0.9580052493438327987, -0.4281496062992127816, -0.4176697321401328100 ) ) ;
#50218=CARTESIAN_POINT ( 'NONE',  ( -0.3083989501312330295, -0.08942795157527998196, 0.3641732283464567121 ) ) ;
#50219=CARTESIAN_POINT ( 'NONE',  ( -0.6824146981627291497, -0.6046776061558809534, -0.2411417322834644161 ) ) ;
#50220=CARTESIAN_POINT ( 'NONE',  ( 1.614173228346457378, -0.6692913385826771977, 8.415575281601705876E-17 ) ) ;
#50221=CARTESIAN_POINT ( 'NONE',  ( -1.318897637795274802, -0.5400638737290845981, -0.3530559997133363437 ) ) ;
#50222=CARTESIAN_POINT ( 'NONE',  ( 1.482939632545932307, -0.4281496062992124485, 0.4176697321401328655 ) ) ;
#50224=CARTESIAN_POINT ( 'NONE',  ( -1.515748031496062076, -0.4536011799217367080, 0.2665933059059888421 ) ) ;
#50226=CARTESIAN_POINT ( 'NONE',  ( 1.371391076115485719, -0.6692913385826773087, -0.1292274648535924053 ) ) ;
#50228=CARTESIAN_POINT ( 'NONE',  ( -1.469816272965878357, -0.6046776061558809534, -0.2411417322834644161 ) ) ;
#50229=CARTESIAN_POINT ( 'NONE',  ( 1.627296587926509996, -0.6046776061558807314, 0.2411417322834647770 ) ) ;
#50230=CARTESIAN_POINT ( 'NONE',  ( -1.043307086614172707, 0.07958543189024071263, -0.2665933059059888421 ) ) ;
#50231=CARTESIAN_POINT ( 'NONE',  ( 1.548556430446194954, 0.1283753931104746893, -0.1820866141732285504 ) ) ;
#50232=CARTESIAN_POINT ( 'NONE',  ( -0.2821522309711278487, -0.6692913385826773087, -0.1292274648535924053 ) ) ;
#50233=CARTESIAN_POINT ( 'NONE',  ( -0.08530183727034056085, -0.2845877964562159024, 0.3641732283464567677 ) ) ;
#50234=CARTESIAN_POINT ( 'NONE',  ( -0.9711286089238838626, -0.5023911411419708095, 0.1820866141732285504 ) ) ;
#50235=CARTESIAN_POINT ( 'NONE',  ( 1.384514435695538337, -0.5511811023622046335, 0.09757992244046803654 ) ) ;
#50236=CARTESIAN_POINT ( 'NONE',  ( 0.8595800524934390507, -0.3162353388693405765, 0.4822834645669290543 ) ) ;
#50237=CARTESIAN_POINT ( 'NONE',  ( 1.463254593175853824, 0.2952755905511810774, -0.1292274648535930714 ) ) ;
#50238=CARTESIAN_POINT ( 'NONE',  ( 0.6167979002624679463, -0.004921259842519870586, -0.3153832671262229437 ) ) ;
#50240=CARTESIAN_POINT ( 'NONE',  ( 0.4133858267716541968, 0.1660481256975885056, 0.3530559997133364547 ) ) ;
#50241=CARTESIAN_POINT ( 'NONE',  ( 0.9120734908136489683, -0.5511811023622046335, 0.09757992244046803654 ) ) ;
#50243=CARTESIAN_POINT ( 'NONE',  ( -1.463254593175852492, 0.2952755905511811885, 0.1292274648535926551 ) ) ;
#50244=CARTESIAN_POINT ( 'NONE',  ( -1.417322834645668772, -0.1870078740157480879, -0.4822834645669291653 ) ) ;
#50245=CARTESIAN_POINT ( 'NONE',  ( -0.01312335958005186876, -0.4281496062992124485, 0.4176697321401328655 ) ) ;
#50248=CARTESIAN_POINT ( 'NONE',  ( 0.3412073490813655186, 0.2306618581243848609, 0.2411417322834645549 ) ) ;
#50249=CARTESIAN_POINT ( 'NONE',  ( 1.233595800524935227, -0.5023911411419708095, 0.1820866141732285504 ) ) ;
#50250=CARTESIAN_POINT ( 'NONE',  ( -0.1706036745406816491, 0.05413385826771626580, -0.4176697321401330321 ) ) ;
#50251=CARTESIAN_POINT ( 'NONE',  ( 0.2362204724409456558, -0.1870078740157480879, -0.4822834645669291653 ) ) ;
#50258=CARTESIAN_POINT ( 'NONE',  ( -0.4461942257217840213, 0.1283753931104748280, 0.1820866141732283561 ) ) ;
#50259=CARTESIAN_POINT ( 'NONE',  ( -0.6692913385826764205, -0.6692913385826771977, 8.415575281601705876E-17 ) ) ;
#50260=CARTESIAN_POINT ( 'NONE',  ( 0.6299212598425204535, -0.1870078740157479769, 0.4822834645669291653 ) ) ;
#50262=CARTESIAN_POINT ( 'NONE',  ( 0.7480314960629927956, 0.2952755905511811885, 0.000000000000000000 ) ) ;
#50263=CARTESIAN_POINT ( 'NONE',  ( 1.561679790026247350, -0.4281496062992124485, 0.4176697321401328655 ) ) ;
#50264=CARTESIAN_POINT ( 'NONE',  ( 0.9776902887139113929, 0.2952755905511811885, 0.1292274648535926551 ) ) ;
#50267=CARTESIAN_POINT ( 'NONE',  ( 1.633858267716535639, -0.5400638737290844871, 0.3530559997133364547 ) ) ;
#50268=CARTESIAN_POINT ( 'NONE',  ( 0.7611548556430451917, -0.6046776061558807314, 0.2411417322834647770 ) ) ;
#50269=EDGE_CURVE ( 'NONE', #32791, #11499, #73676, .T. ) ;
#50270=CARTESIAN_POINT ( 'NONE',  ( 0.3937007874015754361, -0.1870078740157480879, -0.4822834645669291653 ) ) ;
#50271=CARTESIAN_POINT ( 'NONE',  ( 1.443569553805774897, 0.1283753931104748280, 0.1820866141732283561 ) ) ;
#50272=CARTESIAN_POINT ( 'NONE',  ( -1.489501312335957062, -0.08942795157527998196, 0.3641732283464567121 ) ) ;
#50274=CARTESIAN_POINT ( 'NONE',  ( 0.6102362204724416372, 0.1660481256975883668, -0.3530559997133364547 ) ) ;
#50275=DIRECTION ( 'NONE',  ( -1.000000000000000000, -3.412570772413389987E-16, 0.000000000000000000 ) ) ;
#50276=CARTESIAN_POINT ( 'NONE',  ( -0.3543307086614165824, -0.6692913385826771977, 8.415575281601705876E-17 ) ) ;
#50277=CARTESIAN_POINT ( 'NONE',  ( -1.082677165354329896, 0.1660481256975885056, 0.3530559997133364547 ) ) ;
#50278=CARTESIAN_POINT ( 'NONE',  ( 1.030183727034121421, -0.3162353388693409650, -0.4822834645669289433 ) ) ;
#50282=CARTESIAN_POINT ( 'NONE',  ( 1.528871391076116026, 0.2952755905511811885, 0.1292274648535926551 ) ) ;
#50283=ORIENTED_EDGE ( 'NONE', *, *, #64378, .F. ) ;
#50286=CARTESIAN_POINT ( 'NONE',  ( 0.5027385518326215053, 1.496062992125283708, 0.5309055118110234117 ) ) ;
#50287=CARTESIAN_POINT ( 'NONE',  ( 1.482939632545932307, -0.004921259842519870586, -0.3153832671262229437 ) ) ;
#50289=CARTESIAN_POINT ( 'NONE',  ( 1.456692913385827515, -0.5511811023622047445, 6.969142054262312111E-17 ) ) ;
#50294=CARTESIAN_POINT ( 'NONE',  ( -0.8005249343832011588, -0.004921259842519870586, -0.3153832671262229437 ) ) ;
#50295=CARTESIAN_POINT ( 'NONE',  ( -1.384514435695537005, 0.1771653543307087630, 0.09757992244046791164 ) ) ;
#50296=CARTESIAN_POINT ( 'NONE',  ( -1.417322834645668772, -0.1870078740157480879, -0.4822834645669291653 ) ) ;
#50297=CARTESIAN_POINT ( 'NONE',  ( 0.1771653543307093182, 0.1660481256975885056, 0.3530559997133364547 ) ) ;
#50298=CARTESIAN_POINT ( 'NONE',  ( -1.627296587926508442, 0.2306618581243848609, 0.2411417322834645549 ) ) ;
#50300=CARTESIAN_POINT ( 'NONE',  ( 1.509186351706037543, -0.4281496062992127816, -0.4176697321401328100 ) ) ;
#50305=CARTESIAN_POINT ( 'NONE',  ( -0.3871391076115476282, -0.08942795157527998196, 0.3641732283464567121 ) ) ;
#50306=CARTESIAN_POINT ( 'NONE',  ( -1.345144356955379816, -0.3162353388693405765, 0.4822834645669290543 ) ) ;
#50307=CARTESIAN_POINT ( 'NONE',  ( 1.181102362204725198, -0.1870078740157479769, 0.4822834645669291653 ) ) ;
#50309=CARTESIAN_POINT ( 'NONE',  ( 0.7611548556430454138, 0.2306618581243847221, -0.2411417322834647770 ) ) ;
#50311=CARTESIAN_POINT ( 'NONE',  ( -1.692913385826770645, 0.2952755905511811885, 0.000000000000000000 ) ) ;
#50312=CARTESIAN_POINT ( 'NONE',  ( -1.259842519685038686, -0.1870078740157479769, 0.4822834645669291653 ) ) ;
#50314=CARTESIAN_POINT ( 'NONE',  ( -0.5249343832020990641, -0.5023911411419708095, -0.1820866141732282451 ) ) ;
#50317=CARTESIAN_POINT ( 'NONE',  ( -0.6167979002624665030, -0.3690944881889765550, -0.3153832671262227771 ) ) ;
#50318=CARTESIAN_POINT ( 'NONE',  ( 0.3477690288713918276, 0.1771653543307087630, 0.09757992244046791164 ) ) ;
#50319=CARTESIAN_POINT ( 'NONE',  ( 0.6364829396325465405, -0.05778040916215522460, 0.4822834645669289988 ) ) ;
#50320=CARTESIAN_POINT ( 'NONE',  ( -0.7742782152230962556, -0.3690944881889765550, -0.3153832671262227771 ) ) ;
#50322=CARTESIAN_POINT ( 'NONE',  ( 1.253280839895013710, -0.3162353388693405765, 0.4822834645669290543 ) ) ;
#50323=CARTESIAN_POINT ( 'NONE',  ( -1.023622047244093558, -0.1870078740157479769, 0.4822834645669291653 ) ) ;
#50325=CARTESIAN_POINT ( 'NONE',  ( -0.5183727034120726440, -0.6692913385826773087, -0.1292274648535924053 ) ) ;
#50326=CARTESIAN_POINT ( 'NONE',  ( -0.3280839895013117347, 0.05413385826771626580, -0.4176697321401330321 ) ) ;
#50327=CARTESIAN_POINT ( 'NONE',  ( 1.397637795275591177, 0.07958543189024071263, -0.2665933059059888421 ) ) ;
#50329=CARTESIAN_POINT ( 'NONE',  ( 0.1902887139107617975, 0.1771653543307087630, 0.09757992244046791164 ) ) ;
#50330=CARTESIAN_POINT ( 'NONE',  ( -0.07217847769028813698, -0.3162353388693409650, -0.4822834645669289433 ) ) ;
#50331=CARTESIAN_POINT ( 'NONE',  ( -1.010498687664041384, 0.05413385826771666132, 0.4176697321401328100 ) ) ;
#50333=CARTESIAN_POINT ( 'NONE',  ( 1.666666666666667185, -0.004921259842519576551, 0.3153832671262227771 ) ) ;
#50334=CARTESIAN_POINT ( 'NONE',  ( -0.3215223097112853146, -0.05778040916215560624, -0.4822834645669293319 ) ) ;
#50335=CARTESIAN_POINT ( 'NONE',  ( -0.9645669291338575535, -0.5400638737290844871, 0.3530559997133364547 ) ) ;
#50336=ORIENTED_EDGE ( 'NONE', *, *, #40513, .F. ) ;
#50338=CARTESIAN_POINT ( 'NONE',  ( 1.358267716535433323, -0.5400638737290845981, -0.3530559997133363437 ) ) ;
#50339=CARTESIAN_POINT ( 'NONE',  ( -0.5577427821522301654, -0.08942795157528024563, -0.3641732283464568787 ) ) ;
#50340=CARTESIAN_POINT ( 'NONE',  ( -0.4593175853018366950, 0.05413385826771666132, 0.4176697321401328100 ) ) ;
#50341=CARTESIAN_POINT ( 'NONE',  ( 1.200787401574803681, 0.1660481256975885056, 0.3530559997133364547 ) ) ;
#50342=CARTESIAN_POINT ( 'NONE',  ( 0.7611548556430454138, 0.2306618581243847221, -0.2411417322834647770 ) ) ;
#50344=CARTESIAN_POINT ( 'NONE',  ( -1.122047244094487306, -0.4536011799217367080, 0.2665933059059888421 ) ) ;
#50349=CARTESIAN_POINT ( 'NONE',  ( 1.246719160104987623, -0.004921259842519870586, -0.3153832671262229437 ) ) ;
#50350=CARTESIAN_POINT ( 'NONE',  ( 0.8923884514435701520, -0.5023911411419708095, -0.1820866141732282451 ) ) ;
#50351=CARTESIAN_POINT ( 'NONE',  ( 0.5905511811023629321, -0.6692913385826771977, 8.415575281601705876E-17 ) ) ;
#50352=CARTESIAN_POINT ( 'NONE',  ( 1.522309711286089939, -0.6046776061558809534, -0.2411417322834644161 ) ) ;
#50354=CARTESIAN_POINT ( 'NONE',  ( 0.9383202099737538715, -0.08942795157528024563, -0.3641732283464568787 ) ) ;
#50356=CARTESIAN_POINT ( 'NONE',  ( -0.2755905511811015396, -0.6692913385826771977, 8.415575281601705876E-17 ) ) ;
#50357=CARTESIAN_POINT ( 'NONE',  ( -1.161417322834644716, 0.1660481256975885056, 0.3530559997133364547 ) ) ;
#50358=CARTESIAN_POINT ( 'NONE',  ( 1.318897637795276356, -0.5400638737290844871, 0.3530559997133364547 ) ) ;
#50361=CARTESIAN_POINT ( 'NONE',  ( -0.08530183727034056085, -0.08942795157528024563, -0.3641732283464568787 ) ) ;
#50365=CARTESIAN_POINT ( 'NONE',  ( -0.8858267716535425107, 0.1660481256975883668, -0.3530559997133364547 ) ) ;
#50366=CARTESIAN_POINT ( 'NONE',  ( -0.4265091863517051496, -0.6692913385826771977, 0.1292274648535927661 ) ) ;
#50367=CARTESIAN_POINT ( 'NONE',  ( -0.1968503937007867743, 0.2952755905511811885, 0.000000000000000000 ) ) ;
#50368=CARTESIAN_POINT ( 'NONE',  ( 0.4461942257217856311, 0.2306618581243847221, -0.2411417322834647770 ) ) ;
#50369=CARTESIAN_POINT ( 'NONE',  ( -0.4461942257217840213, -0.6046776061558809534, -0.2411417322834644161 ) ) ;
#50370=CARTESIAN_POINT ( 'NONE',  ( -1.515748031496062076, -0.5400638737290844871, 0.3530559997133364547 ) ) ;
#50371=CARTESIAN_POINT ( 'NONE',  ( -0.8595800524934373854, -0.3162353388693409650, -0.4822834645669289433 ) ) ;
#50372=CARTESIAN_POINT ( 'NONE',  ( 0.6889763779527563470, 0.1660481256975883668, -0.3530559997133364547 ) ) ;
#50374=CARTESIAN_POINT ( 'NONE',  ( -0.4855643044619415427, -0.004921259842519870586, -0.3153832671262229437 ) ) ;
#50377=ORIENTED_EDGE ( 'NONE', *, *, #8937, .F. ) ;
#50378=CARTESIAN_POINT ( 'NONE',  ( -1.345144356955379816, -0.08942795157528024563, -0.3641732283464568787 ) ) ;
#50379=CARTESIAN_POINT ( 'NONE',  ( -1.043307086614172041, -0.5400638737290844871, 0.3530559997133364547 ) ) ;
#50380=CARTESIAN_POINT ( 'NONE',  ( -0.7349081364829387342, -0.6046776061558807314, 0.2411417322834647770 ) ) ;
#50382=CARTESIAN_POINT ( 'NONE',  ( -1.128608923884513837, -0.6046776061558807314, 0.2411417322834647770 ) ) ;
#50383=CARTESIAN_POINT ( 'NONE',  ( -0.6889763779527552368, -0.5400638737290845981, -0.3530559997133363437 ) ) ;
#50384=CARTESIAN_POINT ( 'NONE',  ( -1.515748031496062076, -0.5400638737290844871, 0.3530559997133364547 ) ) ;
#50387=CARTESIAN_POINT ( 'NONE',  ( 0.4002624671916016896, -0.08942795157527998196, 0.3641732283464567121 ) ) ;
#50388=CARTESIAN_POINT ( 'NONE',  ( -0.4835386291766053946, -3.153061149046662969E-15, -0.3954974714151482384 ) ) ;
#50390=CARTESIAN_POINT ( 'NONE',  ( 0.04593175853018440641, 0.1771653543307087075, -0.09757992244046823083 ) ) ;
#50391=CARTESIAN_POINT ( 'NONE',  ( -0.4068241469816264999, -0.4281496062992124485, 0.4176697321401328655 ) ) ;
#50392=CARTESIAN_POINT ( 'NONE',  ( 1.528871391076116026, -0.6692913385826773087, -0.1292274648535924053 ) ) ;
#50393=CARTESIAN_POINT ( 'NONE',  ( -0.1443569553805765515, -0.4281496062992127816, -0.4176697321401328100 ) ) ;
#50394=VERTEX_POINT ( 'NONE', #49147 ) ;
#50399=CARTESIAN_POINT ( 'NONE',  ( 1.161417322834646271, 0.1660481256975883668, -0.3530559997133364547 ) ) ;
#50400=CARTESIAN_POINT ( 'NONE',  ( -1.115485564304461219, -0.3690944881889763329, 0.3153832671262228327 ) ) ;
#50401=CARTESIAN_POINT ( 'NONE',  ( -1.358267716535432434, 0.1660481256975883668, -0.3530559997133364547 ) ) ;
#50403=CARTESIAN_POINT ( 'NONE',  ( 2.795275590551181466, 2.244094488188977277, 0.000000000000000000 ) ) ;
#50405=CARTESIAN_POINT ( 'NONE',  ( 1.351706036745407680, 0.05413385826771666132, 0.4176697321401328100 ) ) ;
#50407=CARTESIAN_POINT ( 'NONE',  ( 0.1574803149606306130, -0.1870078740157480879, -0.4822834645669291653 ) ) ;
#50408=CARTESIAN_POINT ( 'NONE',  ( -1.010498687664041384, -0.004921259842519576551, 0.3153832671262227771 ) ) ;
#50409=CARTESIAN_POINT ( 'NONE',  ( -0.5314960629921254842, -0.5400638737290845981, -0.3530559997133363437 ) ) ;
#50411=CARTESIAN_POINT ( 'NONE',  ( -1.076115485564303809, 0.2306618581243848609, 0.2411417322834645549 ) ) ;
#50413=CARTESIAN_POINT ( 'NONE',  ( 1.108923884514436242, -0.08942795157527998196, 0.3641732283464567121 ) ) ;
#50414=CARTESIAN_POINT ( 'NONE',  ( -0.1246719160104980823, 0.1771653543307087630, 0.09757992244046791164 ) ) ;
#50415=CARTESIAN_POINT ( 'NONE',  ( 0.7086614173228353852, -0.1870078740157479769, 0.3641732283464567677 ) ) ;
#50416=CARTESIAN_POINT ( 'NONE',  ( -1.673228346456691717, 0.1660481256975883668, -0.3530559997133364547 ) ) ;
#50417=CARTESIAN_POINT ( 'NONE',  ( 0.8561328129276796206, 8.471767977567108961E-16, -0.4445507791589058955 ) ) ;
#50418=CARTESIAN_POINT ( 'NONE',  ( 0.5643044619422579178, -0.004921259842519576551, 0.3153832671262227771 ) ) ;
#50419=CARTESIAN_POINT ( 'NONE',  ( -0.7545931758530176614, -0.6692913385826773087, -0.1292274648535924053 ) ) ;
#50420=CARTESIAN_POINT ( 'NONE',  ( 0.2462293917967310342, -2.191421614605370878E-15, 0.4445507791589071167 ) ) ;
#50421=CARTESIAN_POINT ( 'NONE',  ( 0.09842519685039434474, 0.07958543189024085140, 0.2665933059059887866 ) ) ;
#50422=CARTESIAN_POINT ( 'NONE',  ( -1.489501312335957062, -0.2845877964562161244, -0.3641732283464567121 ) ) ;
#50423=CARTESIAN_POINT ( 'NONE',  ( 0.5839895013123367340, 0.2952755905511811885, 0.1292274648535926551 ) ) ;
#50425=CARTESIAN_POINT ( 'NONE',  ( 1.430446194225722500, -0.004921259842519576551, 0.3153832671262227771 ) ) ;
#50426=CARTESIAN_POINT ( 'NONE',  ( -1.305774278215222184, -0.6692913385826773087, -0.1292274648535924053 ) ) ;
#50427=CARTESIAN_POINT ( 'NONE',  ( -0.4199475065616791736, -0.5023911411419708095, 0.1820866141732285504 ) ) ;
#50429=CARTESIAN_POINT ( 'NONE',  ( 0.05905511811023681640, 0.07958543189024071263, -0.2665933059059888421 ) ) ;
#50430=CARTESIAN_POINT ( 'NONE',  ( -1.351706036745406347, 0.05413385826771626580, -0.4176697321401330321 ) ) ;
#50431=CARTESIAN_POINT ( 'NONE',  ( -0.6627296587926501115, 0.2952755905511810774, -0.1292274648535930714 ) ) ;
#50434=CARTESIAN_POINT ( 'NONE',  ( 0.7217847769028878924, -0.3690944881889765550, -0.3153832671262227771 ) ) ;
#50435=CARTESIAN_POINT ( 'NONE',  ( -0.3740157480314953431, 0.1660481256975885056, 0.3530559997133364547 ) ) ;
#50437=CARTESIAN_POINT ( 'NONE',  ( -0.8858267716535425107, -0.5400638737290844871, 0.3530559997133364547 ) ) ;
#50438=CARTESIAN_POINT ( 'NONE',  ( -0.8989501312335946848, -0.5511811023622046335, 0.09757992244046803654 ) ) ;
#50440=CARTESIAN_POINT ( 'NONE',  ( -0.2493438320209966919, -0.4281496062992124485, 0.4176697321401328655 ) ) ;
#50441=FACE_OUTER_BOUND ( 'NONE', #45718, .T. ) ;
#50442=CARTESIAN_POINT ( 'NONE',  ( 1.561679790026247350, -0.4281496062992124485, 0.4176697321401328655 ) ) ;
#50445=LINE ( 'NONE', #43712, #20326 ) ;
#50446=CARTESIAN_POINT ( 'NONE',  ( -1.522309711286088607, 0.2306618581243847221, -0.2411417322834647770 ) ) ;
#50447=CARTESIAN_POINT ( 'NONE',  ( -0.8858267716535425107, 0.1660481256975883668, -0.3530559997133364547 ) ) ;
#50448=CARTESIAN_POINT ( 'NONE',  ( -1.502624671916009680, -0.3162353388693405765, 0.4822834645669290543 ) ) ;
#50451=EDGE_CURVE ( 'NONE', #57855, #62837, #21999, .T. ) ;
#50452=CARTESIAN_POINT ( 'NONE',  ( 0.7611548556430454138, 0.2306618581243847221, -0.2411417322834647770 ) ) ;
#50453=CARTESIAN_POINT ( 'NONE',  ( 0.1902887139107617975, -0.6692913385826773087, -0.1292274648535924053 ) ) ;
#50455=CARTESIAN_POINT ( 'NONE',  ( -0.6955380577427815458, 0.05413385826771666132, 0.4176697321401328100 ) ) ;
#50456=CARTESIAN_POINT ( 'NONE',  ( 1.240157480314961314, -0.4536011799217367080, 0.2665933059059888421 ) ) ;
#50461=CARTESIAN_POINT ( 'NONE',  ( 0.6036745406824153282, -0.6046776061558807314, 0.2411417322834647770 ) ) ;
#50462=CARTESIAN_POINT ( 'NONE',  ( -0.8530183727034112984, -0.4281496062992127816, -0.4176697321401328100 ) ) ;
#50463=CARTESIAN_POINT ( 'NONE',  ( -1.646981627296586703, -0.05778040916215522460, 0.4822834645669289988 ) ) ;
#50464=CARTESIAN_POINT ( 'NONE',  ( 0.6233595800524942554, -0.05778040916215560624, -0.4822834645669293319 ) ) ;
#50465=CARTESIAN_POINT ( 'NONE',  ( 1.482939632545932307, -0.4281496062992124485, 0.4176697321401328655 ) ) ;
#50466=CARTESIAN_POINT ( 'NONE',  ( 1.345144356955381593, -0.3162353388693409650, -0.4822834645669289433 ) ) ;
#50467=CARTESIAN_POINT ( 'NONE',  ( 0.1246719160104994284, 0.2952755905511810774, -0.1292274648535930714 ) ) ;
#50468=CARTESIAN_POINT ( 'NONE',  ( -1.069553805774277722, -0.6692913385826773087, -0.1292274648535924053 ) ) ;
#50469=CARTESIAN_POINT ( 'NONE',  ( -1.220472440944881054, 0.4405861044731111953, 0.5309055118110237448 ) ) ;
#50472=CARTESIAN_POINT ( 'NONE',  ( 0.7480314960629927956, 0.1771653543307087630, 0.000000000000000000 ) ) ;
#50476=CARTESIAN_POINT ( 'NONE',  ( -0.04593175853018302557, -0.5511811023622048555, -0.09757992244046775898 ) ) ;
#50478=CARTESIAN_POINT ( 'NONE',  ( 0.6496062992125991586, 0.1660481256975885056, 0.3530559997133364547 ) ) ;
#50479=CARTESIAN_POINT ( 'NONE',  ( 0.2362204724409456558, -0.1870078740157480879, -0.4822834645669291653 ) ) ;
#50480=CARTESIAN_POINT ( 'NONE',  ( -0.5314960629921254842, -0.5400638737290845981, -0.3530559997133363437 ) ) ;
#50482=CARTESIAN_POINT ( 'NONE',  ( -1.069553805774277722, -0.6692913385826773087, -0.1292274648535924053 ) ) ;
#50484=CARTESIAN_POINT ( 'NONE',  ( 1.181102362204724976, -0.1870078740157480601, -0.3641732283464567677 ) ) ;
#50485=CARTESIAN_POINT ( 'NONE',  ( -1.417322834645668772, -0.1870078740157480879, -0.4822834645669291653 ) ) ;
#50486=CARTESIAN_POINT ( 'NONE',  ( 0.7874015748031503170, -0.1870078740157480879, -0.4822834645669291653 ) ) ;
#50487=CARTESIAN_POINT ( 'NONE',  ( 1.128608923884515169, -0.6046776061558809534, -0.2411417322834644161 ) ) ;
#50490=CARTESIAN_POINT ( 'NONE',  ( -1.358267716535432434, 0.1660481256975883668, -0.3530559997133364547 ) ) ;
#50492=CARTESIAN_POINT ( 'NONE',  ( -0.1246719160104980823, 0.2952755905511811885, 0.1292274648535926551 ) ) ;
#50495=CIRCLE ( 'NONE', #19624, 3.543307086614173596 ) ;
#50496=CARTESIAN_POINT ( 'NONE',  ( 1.515748031496063408, 0.1660481256975885056, 0.3530559997133364547 ) ) ;
#50497=CARTESIAN_POINT ( 'NONE',  ( 0.1640419947506569498, -0.2845877964562161244, -0.3641732283464567121 ) ) ;
#50498=CARTESIAN_POINT ( 'NONE',  ( 0.7480314960629927956, -0.6692913385826771977, 8.415575281601705876E-17 ) ) ;
#50500=CARTESIAN_POINT ( 'NONE',  ( 0.1771653543307093182, -0.4536011799217368745, -0.2665933059059886201 ) ) ;
#50501=CARTESIAN_POINT ( 'NONE',  ( 0.4265091863517067039, -0.6692913385826773087, -0.1292274648535924053 ) ) ;
#50503=CARTESIAN_POINT ( 'NONE',  ( -0.7152230971128602510, -0.05778040916215560624, -0.4822834645669293319 ) ) ;
#50505=CARTESIAN_POINT ( 'NONE',  ( 0.7545931758530188826, -0.5511811023622046335, 0.09757992244046803654 ) ) ;
#50507=CARTESIAN_POINT ( 'NONE',  ( -0.2362204724409442680, -0.1870078740157480879, -0.4822834645669291653 ) ) ;
#50508=CARTESIAN_POINT ( 'NONE',  ( 0.1706036745406830368, -0.3690944881889765550, -0.3153832671262227771 ) ) ;
#50510=CARTESIAN_POINT ( 'NONE',  ( -0.2099737532808391705, -0.6046776061558809534, -0.2411417322834644161 ) ) ;
#50511=CARTESIAN_POINT ( 'NONE',  ( 0.3871391076115492380, -0.08942795157528024563, -0.3641732283464568787 ) ) ;
#50513=CARTESIAN_POINT ( 'NONE',  ( 0.4002624671916016896, -0.05778040916215522460, 0.4822834645669289988 ) ) ;
#50515=CARTESIAN_POINT ( 'NONE',  ( 1.017060367454068803, -0.2845877964562159024, 0.3641732283464567677 ) ) ;
#50516=CARTESIAN_POINT ( 'NONE',  ( 0.2165354330708668951, 0.1660481256975883391, -0.3530559997133364547 ) ) ;
#50517=B_SPLINE_CURVE_WITH_KNOTS ( 'NONE', 3,
 ( #58889, #27733, #46248, #15120 ),
 .UNSPECIFIED., .F., .F.,
 ( 4, 4 ),
 ( 3.210432057746194131E-07, 0.001287787053612155170 ),
 .UNSPECIFIED. ) ;
#50518=CARTESIAN_POINT ( 'NONE',  ( -0.2821522309711278487, 0.1771653543307087630, 0.09757992244046791164 ) ) ;
#50519=CARTESIAN_POINT ( 'NONE',  ( -0.7414698162729651543, 0.1771653543307087075, -0.09757992244046823083 ) ) ;
#50520=CARTESIAN_POINT ( 'NONE',  ( -0.4396325459317577122, -0.6692913385826773087, -0.1292274648535924053 ) ) ;
#50521=CARTESIAN_POINT ( 'NONE',  ( 0.4068241469816279987, -0.4281496062992127816, -0.4176697321401328100 ) ) ;
#50522=CARTESIAN_POINT ( 'NONE',  ( 0.7874015748031503170, -0.1870078740157480601, -0.3641732283464567677 ) ) ;
#50523=CARTESIAN_POINT ( 'NONE',  ( -1.594488188976377563, -0.4536011799217367080, 0.2665933059059888421 ) ) ;
#50524=CARTESIAN_POINT ( 'NONE',  ( 1.430446194225722500, -0.004921259842519576551, 0.3153832671262227771 ) ) ;
#50525=CARTESIAN_POINT ( 'NONE',  ( 0.6692913385826778638, -0.6692913385826771977, 8.415575281601705876E-17 ) ) ;
#50527=CARTESIAN_POINT ( 'NONE',  ( -0.4133858267716528645, 0.1660481256975883668, -0.3530559997133364547 ) ) ;
#50529=AXIS2_PLACEMENT_3D ( 'NONE', #7213, #45911, #52648 ) ;
#50530=CARTESIAN_POINT ( 'NONE',  ( 0.7414698162729663755, 0.2952755905511811885, 0.1292274648535926551 ) ) ;
#50532=CARTESIAN_POINT ( 'NONE',  ( 0.7152230971128616943, -0.05778040916215522460, 0.4822834645669289988 ) ) ;
#50534=CARTESIAN_POINT ( 'NONE',  ( 0.3937007874015754361, -0.1870078740157479769, 0.3641732283464567677 ) ) ;
#50535=CARTESIAN_POINT ( 'NONE',  ( 1.358267716535433323, 0.1660481256975885056, 0.3530559997133364547 ) ) ;
#50536=CARTESIAN_POINT ( 'NONE',  ( -0.3608923884514428360, -0.5511811023622048555, -0.09757992244046775898 ) ) ;
#50537=CARTESIAN_POINT ( 'NONE',  ( -0.3608923884514428360, 0.2952755905511811885, 0.1292274648535926551 ) ) ;
#50539=CARTESIAN_POINT ( 'NONE',  ( 0.2362204724409456558, -0.1870078740157480879, -0.4822834645669291653 ) ) ;
#50540=CARTESIAN_POINT ( 'NONE',  ( -0.7217847769028863381, -0.4281496062992124485, 0.4176697321401328655 ) ) ;
#50541=CARTESIAN_POINT ( 'NONE',  ( -0.6692913385826764205, -0.5511811023622047445, 6.969142054262312111E-17 ) ) ;
#50542=CARTESIAN_POINT ( 'NONE',  ( 0.2690288713910767848, -0.6692913385826773087, -0.1292274648535924053 ) ) ;
#50543=CARTESIAN_POINT ( 'NONE',  ( -1.253280839895012377, -0.05778040916215522460, 0.4822834645669289988 ) ) ;
#50544=CARTESIAN_POINT ( 'NONE',  ( -0.4330708661417315697, -0.6692913385826771977, 8.415575281601705876E-17 ) ) ;
#50546=CARTESIAN_POINT ( 'NONE',  ( -0.9345427628023836863, -4.378520898609941727E-15, 0.4281989832122466977 ) ) ;
#50547=CARTESIAN_POINT ( 'NONE',  ( 1.450131233595801428, 0.2952755905511811885, 0.1292274648535926551 ) ) ;
#50548=CARTESIAN_POINT ( 'NONE',  ( 1.581364829396326277, -0.3162353388693409650, -0.4822834645669289433 ) ) ;
#50550=CARTESIAN_POINT ( 'NONE',  ( -1.633858267716534529, 0.1660481256975885056, 0.3530559997133364547 ) ) ;
#50551=VECTOR ( 'NONE', #20298, 39.37007874015748143 ) ;
#50552=CARTESIAN_POINT ( 'NONE',  ( -1.095800524934382292, -0.05778040916215522460, 0.4822834645669289988 ) ) ;
#50556=CARTESIAN_POINT ( 'NONE',  ( 0.1771653543307093182, -0.4536011799217368745, -0.2665933059059886201 ) ) ;
#50558=CARTESIAN_POINT ( 'NONE',  ( 0.8398950131233602345, 0.2306618581243847221, -0.2411417322834647770 ) ) ;
#50561=CARTESIAN_POINT ( 'NONE',  ( -0.6233595800524928121, -0.2845877964562161244, -0.3641732283464567121 ) ) ;
#50563=CARTESIAN_POINT ( 'NONE',  ( 1.069553805774278832, 0.2952755905511810774, -0.1292274648535930714 ) ) ;
#50564=CARTESIAN_POINT ( 'NONE',  ( 0.8005249343832027131, -0.004921259842519576551, 0.3153832671262227771 ) ) ;
#50565=CARTESIAN_POINT ( 'NONE',  ( -0.01968503937007793844, 0.1660481256975883668, -0.3530559997133364547 ) ) ;
#50567=CARTESIAN_POINT ( 'NONE',  ( -0.5511811023622038563, -0.1870078740157479769, 0.4822834645669291653 ) ) ;
#50568=CARTESIAN_POINT ( 'NONE',  ( -1.325459317585300889, -0.3690944881889765550, -0.3153832671262227771 ) ) ;
#50569=CARTESIAN_POINT ( 'NONE',  ( -0.3543307086614165824, -0.6692913385826771977, 8.415575281601705876E-17 ) ) ;
#50572=ORIENTED_EDGE ( 'NONE', *, *, #38397, .T. ) ;
#50574=CARTESIAN_POINT ( 'NONE',  ( 0.5380577427821529035, -0.4281496062992124485, 0.4176697321401328655 ) ) ;
#50576=CARTESIAN_POINT ( 'NONE',  ( -0.8989501312335946848, 0.2952755905511810774, -0.1292274648535930714 ) ) ;
#50577=CARTESIAN_POINT ( 'NONE',  ( -1.299212598425196097, 0.2952755905511811885, 0.000000000000000000 ) ) ;
#50578=CARTESIAN_POINT ( 'NONE',  ( 0.5446194225721792126, -0.05778040916215560624, -0.4822834645669293319 ) ) ;
#50579=CARTESIAN_POINT ( 'NONE',  ( 0.1377952755905518800, 0.1660481256975883668, -0.3530559997133364547 ) ) ;
#50581=CARTESIAN_POINT ( 'NONE',  ( -0.7217847769028863381, 0.05413385826771626580, -0.4176697321401330321 ) ) ;
#50582=CARTESIAN_POINT ( 'NONE',  ( -0.2427821522309703550, -0.3162353388693405765, 0.4822834645669290543 ) ) ;
#50583=CARTESIAN_POINT ( 'NONE',  ( -0.9973753280839886548, 0.2306618581243848609, 0.2411417322834645549 ) ) ;
#50584=CARTESIAN_POINT ( 'NONE',  ( 0.4396325459317593221, 0.1771653543307087075, -0.09757992244046823083 ) ) ;
#50586=CARTESIAN_POINT ( 'NONE',  ( -0.03937007874015669567, -0.6692913385826771977, 8.415575281601705876E-17 ) ) ;
#50588=CARTESIAN_POINT ( 'NONE',  ( 0.9645669291338588858, 0.1660481256975885056, 0.3530559997133364547 ) ) ;
#50592=CARTESIAN_POINT ( 'NONE',  ( 0.4265091863517067594, 0.2952755905511811885, 0.1292274648535926551 ) ) ;
#50593=CARTESIAN_POINT ( 'NONE',  ( -0.07217847769028813698, -0.2845877964562161244, -0.3641732283464567121 ) ) ;
#50595=CARTESIAN_POINT ( 'NONE',  ( 1.627296587926509996, -0.5023911411419708095, 0.1820866141732285504 ) ) ;
#50601=CARTESIAN_POINT ( 'NONE',  ( 0.6167979002624678353, -0.4281496062992124485, 0.4176697321401328655 ) ) ;
#50602=CARTESIAN_POINT ( 'NONE',  ( -1.220472440944881054, -0.6692913385826771977, 8.415575281601705876E-17 ) ) ;
#50603=CARTESIAN_POINT ( 'NONE',  ( -1.167979002624671470, -0.4281496062992127816, -0.4176697321401328100 ) ) ;
#50604=CARTESIAN_POINT ( 'NONE',  ( 0.2690288713910767848, -0.6692913385826773087, -0.1292274648535924053 ) ) ;
#50605=CARTESIAN_POINT ( 'NONE',  ( 1.115485564304462551, 0.05413385826771666132, 0.4176697321401328100 ) ) ;
#50606=CARTESIAN_POINT ( 'NONE',  ( 1.522309711286089939, 0.1283753931104748280, 0.1820866141732283561 ) ) ;
#50608=CARTESIAN_POINT ( 'NONE',  ( 0.7152230971128616943, -0.08942795157527998196, 0.3641732283464567121 ) ) ;
#50609=CARTESIAN_POINT ( 'NONE',  ( -0.6758530183727028406, 0.2952755905511811885, 0.1292274648535926551 ) ) ;
#50611=CARTESIAN_POINT ( 'NONE',  ( -1.633858267716534529, 0.07958543189024085140, 0.2665933059059887866 ) ) ;
#50612=( BOUNDED_CURVE ( )  B_SPLINE_CURVE ( 2, ( #58099, #32023, #64011, #51782, #57264, #58527, #37921, #44626, #64849, #18977, #50949, #77486, #77907 ),
 .UNSPECIFIED., .F., .F. ) 
 B_SPLINE_CURVE_WITH_KNOTS ( ( 3, 2, 2, 2, 2, 2, 3 ),
 ( 0.2187856400893463393, 0.2196969696969696961, 0.2234848484848484806, 0.2272727272727272652, 0.2310606060606060497, 0.2348484848484848619, 0.2357598144561083298 ),
 .UNSPECIFIED. ) 
 CURVE ( )  GEOMETRIC_REPRESENTATION_ITEM ( )  RATIONAL_B_SPLINE_CURVE ( ( 0.9875488213027530104, 0.9918020599134685922, 1.000000000000000000, 0.9659258262890683122, 1.000000000000000000, 0.9659258262890683122, 1.000000000000000000, 0.9659258262890683122, 1.000000000000000000, 0.9659258262890683122, 1.000000000000000000, 0.9918020599134675930, 0.9875488213027519002 ) ) 
 REPRESENTATION_ITEM ( '' )  );
#50614=ADVANCED_FACE ( 'NONE', ( #6372 ), #82571, .F. ) ;
#50615=CARTESIAN_POINT ( 'NONE',  ( 1.246719160104987623, 0.05413385826771626580, -0.4176697321401330321 ) ) ;
#50617=CARTESIAN_POINT ( 'NONE',  ( -1.410761154855642463, -0.08942795157527998196, 0.3641732283464567121 ) ) ;
#50618=CARTESIAN_POINT ( 'NONE',  ( 0.01312335958005323398, -0.4281496062992127816, -0.4176697321401328100 ) ) ;
#50619=CARTESIAN_POINT ( 'NONE',  ( 0.7349081364829402885, -0.5023911411419708095, -0.1820866141732282451 ) ) ;
#50620=CARTESIAN_POINT ( 'NONE',  ( -1.706036745406823485, 0.1283753931104748280, 0.1820866141732283561 ) ) ;
#50621=CARTESIAN_POINT ( 'NONE',  ( 0.8727034120734913358, -0.05778040916215522460, 0.4822834645669289988 ) ) ;
#50623=CARTESIAN_POINT ( 'NONE',  ( -0.3740157480314953431, -0.4536011799217368745, -0.2665933059059886201 ) ) ;
#50624=CARTESIAN_POINT ( 'NONE',  ( -0.7742782152230965886, 0.05413385826771666132, 0.4176697321401328100 ) ) ;
#50625=CARTESIAN_POINT ( 'NONE',  ( 1.397637795275591177, 0.1660481256975883668, -0.3530559997133364547 ) ) ;
#50626=CARTESIAN_POINT ( 'NONE',  ( -1.187664041994750175, -0.05778040916215560624, -0.4822834645669293319 ) ) ;
#50627=CARTESIAN_POINT ( 'NONE',  ( 1.181102362204725198, -0.1870078740157479769, 0.4822834645669291653 ) ) ;
#50629=CARTESIAN_POINT ( 'NONE',  ( -1.286089238845143479, 0.1283753931104746893, -0.1820866141732285504 ) ) ;
#50631=CARTESIAN_POINT ( 'NONE',  ( 0.8464566929133865436, 0.1660481256975883668, -0.3530559997133364547 ) ) ;
#50633=CARTESIAN_POINT ( 'NONE',  ( -1.627296587926508442, -0.6046776061558809534, -0.2411417322834644161 ) ) ;
#50634=CARTESIAN_POINT ( 'NONE',  ( -1.384514435695537005, -0.5511811023622048555, -0.09757992244046775898 ) ) ;
#50635=CARTESIAN_POINT ( 'NONE',  ( -0.8202099737532801971, -0.5511811023622046335, 0.09757992244046803654 ) ) ;
#50637=CARTESIAN_POINT ( 'NONE',  ( 1.443569553805774897, -0.5023911411419708095, -0.1820866141732282451 ) ) ;
#50638=CARTESIAN_POINT ( 'NONE',  ( -0.3543307086614165824, 0.2952755905511811885, 0.000000000000000000 ) ) ;
#50639=CARTESIAN_POINT ( 'NONE',  ( 0.04593175853018440641, -0.5511811023622046335, 0.09757992244046803654 ) ) ;
#50640=CARTESIAN_POINT ( 'NONE',  ( -1.502624671916009680, -0.08942795157528024563, -0.3641732283464568787 ) ) ;
#50641=CARTESIAN_POINT ( 'NONE',  ( 1.253280839895013710, -0.2845877964562159024, 0.3641732283464567677 ) ) ;
#50642=CARTESIAN_POINT ( 'NONE',  ( 1.128608923884515169, -0.6046776061558809534, -0.2411417322834644161 ) ) ;
#50643=CARTESIAN_POINT ( 'NONE',  ( 1.391076115485564868, -0.6046776061558807314, 0.2411417322834647770 ) ) ;
#50644=CARTESIAN_POINT ( 'NONE',  ( -0.04593175853018302557, 0.1771653543307087630, 0.09757992244046791164 ) ) ;
#50645=CARTESIAN_POINT ( 'NONE',  ( 0.5839895013123367340, 0.2952755905511811885, 0.1292274648535926551 ) ) ;
#50647=CARTESIAN_POINT ( 'NONE',  ( 1.174540682414699111, -0.08942795157528024563, -0.3641732283464568787 ) ) ;
#50648=ORIENTED_EDGE ( 'NONE', *, *, #32070, .T. ) ;
#50649=CARTESIAN_POINT ( 'NONE',  ( -1.509186351706035767, -0.4281496062992124485, 0.4176697321401328655 ) ) ;
#50651=CARTESIAN_POINT ( 'NONE',  ( -1.345144356955379816, -0.3162353388693405765, 0.4822834645669290543 ) ) ;
#50652=CARTESIAN_POINT ( 'NONE',  ( -0.1049868766404193215, 0.2306618581243847221, -0.2411417322834647770 ) ) ;
#50656=CARTESIAN_POINT ( 'NONE',  ( 0.4461942257217855201, -0.6046776061558807314, 0.2411417322834647770 ) ) ;
#50657=CARTESIAN_POINT ( 'NONE',  ( 1.246719160104987623, -0.3690944881889763329, 0.3153832671262228327 ) ) ;
#50659=AXIS2_PLACEMENT_3D ( 'NONE', #28576, #9639, #67304 ) ;
#50660=CARTESIAN_POINT ( 'NONE',  ( -0.3280839895013117347, 0.05413385826771626580, -0.4176697321401330321 ) ) ;
#50661=CARTESIAN_POINT ( 'NONE',  ( 0.3018372703412079971, -0.4281496062992124485, 0.4176697321401328655 ) ) ;
#50667=CARTESIAN_POINT ( 'NONE',  ( -0.6955380577427815458, -0.3690944881889765550, -0.3153832671262227771 ) ) ;
#50668=CARTESIAN_POINT ( 'NONE',  ( -0.9645669291338575535, -0.5400638737290844871, 0.3530559997133364547 ) ) ;
#50670=EDGE_CURVE ( 'NONE', #49068, #22657, #22529, .T. ) ;
#50671=CARTESIAN_POINT ( 'NONE',  ( 0.6824146981627303710, -0.6046776061558807314, 0.2411417322834647770 ) ) ;
#50672=CARTESIAN_POINT ( 'NONE',  ( -1.450131233595799651, 0.2952755905511810774, -0.1292274648535930714 ) ) ;
#50673=CARTESIAN_POINT ( 'NONE',  ( 0.5971128608923890191, -0.6692913385826771977, 0.1292274648535927661 ) ) ;
#50674=CYLINDRICAL_SURFACE ( 'NONE', #69035, 1.181102362204724310 ) ;
#50677=CARTESIAN_POINT ( 'NONE',  ( 1.108923884514436242, -0.05778040916215522460, 0.4822834645669289988 ) ) ;
#50678=CARTESIAN_POINT ( 'NONE',  ( 0.5643044619422579178, -0.4281496062992127816, -0.4176697321401328100 ) ) ;
#50680=CARTESIAN_POINT ( 'NONE',  ( 0.8005249343832027131, -0.004921259842519576551, 0.3153832671262227771 ) ) ;
#50681=CARTESIAN_POINT ( 'NONE',  ( 1.227034120734908917, 0.2952755905511810774, -0.1292274648535930714 ) ) ;
#50684=CARTESIAN_POINT ( 'NONE',  ( 0.7349081364829403995, 0.2306618581243848609, 0.2411417322834645549 ) ) ;
#50685=CARTESIAN_POINT ( 'NONE',  ( 1.456692913385827515, -0.5511811023622047445, 6.969142054262312111E-17 ) ) ;
#50686=CARTESIAN_POINT ( 'NONE',  ( -1.122047244094487306, -0.5400638737290844871, 0.3530559997133364547 ) ) ;
#50687=CARTESIAN_POINT ( 'NONE',  ( -0.9973753280839886548, -0.6046776061558809534, -0.2411417322834644161 ) ) ;
#50688=CARTESIAN_POINT ( 'NONE',  ( 0.9645669291338588858, 0.1660481256975885056, 0.3530559997133364547 ) ) ;
#50693=ORIENTED_EDGE ( 'NONE', *, *, #81557, .F. ) ;
#50696=CARTESIAN_POINT ( 'NONE',  ( 1.640419947506562393, -0.4281496062992124485, 0.4176697321401328655 ) ) ;
#50697=CARTESIAN_POINT ( 'NONE',  ( 1.227034120734908917, -0.5511811023622046335, 0.09757992244046803654 ) ) ;
#50699=CARTESIAN_POINT ( 'NONE',  ( 1.417322834645670104, -0.1870078740157480601, -0.3641732283464567677 ) ) ;
#50702=CARTESIAN_POINT ( 'NONE',  ( 0.4330708661417329575, 1.568468489416427580, 0.000000000000000000 ) ) ;
#50704=CARTESIAN_POINT ( 'NONE',  ( -0.8595800524934373854, -0.08942795157527998196, 0.3641732283464567121 ) ) ;
#50705=CARTESIAN_POINT ( 'NONE',  ( -1.528871391076114250, 0.1771653543307087075, -0.09757992244046823083 ) ) ;
#50706=CARTESIAN_POINT ( 'NONE',  ( -1.456692913385826182, 0.2952755905511811885, 0.000000000000000000 ) ) ;
#50707=CARTESIAN_POINT ( 'NONE',  ( -0.07217847769028813698, -0.3162353388693409650, -0.4822834645669289433 ) ) ;
#50708=CARTESIAN_POINT ( 'NONE',  ( 1.384514435695538337, -0.6692913385826771977, 0.1292274648535927661 ) ) ;
#50714=CARTESIAN_POINT ( 'NONE',  ( -0.5118110236220466680, 0.1771653543307087630, 0.000000000000000000 ) ) ;
#50716=CARTESIAN_POINT ( 'NONE',  ( -1.220472440944881054, -0.6692913385826771977, 8.415575281601705876E-17 ) ) ;
#50717=CARTESIAN_POINT ( 'NONE',  ( 0.9645669291338591078, -0.5400638737290845981, -0.3530559997133363437 ) ) ;
#50720=CARTESIAN_POINT ( 'NONE',  ( 0.7773926554473647998, 8.471767977567108961E-16, -0.4445507791589058955 ) ) ;
#50721=CARTESIAN_POINT ( 'NONE',  ( -2.787279214012418738, 0.000000000000000000, 0.000000000000000000 ) ) ;
#50722=CARTESIAN_POINT ( 'NONE',  ( 1.325459317585302665, -0.4281496062992124485, 0.4176697321401328655 ) ) ;
#50723=CARTESIAN_POINT ( 'NONE',  ( -1.095800524934382292, -0.05778040916215522460, 0.4822834645669289988 ) ) ;
#50725=CARTESIAN_POINT ( 'NONE',  ( -0.3215223097112853146, -0.2845877964562159024, 0.3641732283464567677 ) ) ;
#50727=CARTESIAN_POINT ( 'NONE',  ( -0.5052493438320203589, 0.1771653543307087075, -0.09757992244046823083 ) ) ;
#50728=CARTESIAN_POINT ( 'NONE',  ( 0.6824146981627303710, 0.1283753931104746893, -0.1820866141732285504 ) ) ;
#50729=CARTESIAN_POINT ( 'NONE',  ( 0.06561679790026316017, 0.05413385826771626580, -0.4176697321401330321 ) ) ;
#50730=CARTESIAN_POINT ( 'NONE',  ( -0.6102362204724400829, -0.4536011799217368745, -0.2665933059059886201 ) ) ;
#50732=CARTESIAN_POINT ( 'NONE',  ( 1.305774278215223960, 0.2952755905511810774, -0.1292274648535930714 ) ) ;
#50733=CARTESIAN_POINT ( 'NONE',  ( -1.450131233595799651, 0.2952755905511810774, -0.1292274648535930714 ) ) ;
#50735=CARTESIAN_POINT ( 'NONE',  ( -0.4986876640419942164, -0.6046776061558807314, 0.2411417322834647770 ) ) ;
#50737=CARTESIAN_POINT ( 'NONE',  ( -0.9908136482939626788, 0.2952755905511811885, 0.1292274648535926551 ) ) ;
#50738=CARTESIAN_POINT ( 'NONE',  ( 1.450131233595801428, -0.5511811023622048555, -0.09757992244046775898 ) ) ;
#50739=CARTESIAN_POINT ( 'NONE',  ( -0.4593175853018366950, -0.004921259842519576551, 0.3153832671262227771 ) ) ;
#50740=CARTESIAN_POINT ( 'NONE',  ( -0.4593175853018366950, 0.05413385826771666132, 0.4176697321401328100 ) ) ;
#50741=CARTESIAN_POINT ( 'NONE',  ( -1.240157480314959759, -0.5400638737290845981, -0.3530559997133363437 ) ) ;
#50743=CARTESIAN_POINT ( 'NONE',  ( 1.148293963254593875, -0.5511811023622046335, 0.09757992244046803654 ) ) ;
#50744=CARTESIAN_POINT ( 'NONE',  ( -0.3412073490813641308, 0.2306618581243847221, -0.2411417322834647770 ) ) ;
#50745=CARTESIAN_POINT ( 'NONE',  ( -1.128608923884513837, -0.6046776061558807314, 0.2411417322834647770 ) ) ;
#50746=EDGE_LOOP ( 'NONE', ( #73198, #37434, #26879, #45624 ) ) ;
#50748=CARTESIAN_POINT ( 'NONE',  ( -0.7677165354330699465, -0.4536011799217368745, -0.2665933059059886201 ) ) ;
#50749=CARTESIAN_POINT ( 'NONE',  ( 1.246719160104987623, -0.4281496062992124485, 0.4176697321401328655 ) ) ;
#50750=CARTESIAN_POINT ( 'NONE',  ( -0.8661417322834640276, -0.1870078740157480601, -0.3641732283464567677 ) ) ;
#50752=CARTESIAN_POINT ( 'NONE',  ( -1.076115485564303809, 0.2306618581243848609, 0.2411417322834645549 ) ) ;
#50753=CARTESIAN_POINT ( 'NONE',  ( 1.377952755905512472, 0.2952755905511811885, 0.000000000000000000 ) ) ;
#50754=CARTESIAN_POINT ( 'NONE',  ( 0.7808398950131241190, -0.05778040916215560624, -0.4822834645669293319 ) ) ;
#50756=CARTESIAN_POINT ( 'NONE',  ( -1.292650918635170010, -0.5511811023622046335, 0.09757992244046803654 ) ) ;
#50761=CARTESIAN_POINT ( 'NONE',  ( 1.364829396325460076, 0.1283753931104748280, 0.1820866141732283561 ) ) ;
#50762=CARTESIAN_POINT ( 'NONE',  ( 0.8202099737532813073, 0.1771653543307087630, 0.09757992244046791164 ) ) ;
#50763=CARTESIAN_POINT ( 'NONE',  ( 0.4593175853018379162, -0.4281496062992124485, 0.4176697321401328655 ) ) ;
#50766=CARTESIAN_POINT ( 'NONE',  ( 0.8267716535433078384, -0.5511811023622047445, 6.969142054262312111E-17 ) ) ;
#50767=CARTESIAN_POINT ( 'NONE',  ( -0.2821522309711278487, -0.6692913385826773087, -0.1292274648535924053 ) ) ;
#50768=CARTESIAN_POINT ( 'NONE',  ( -1.102362204724408601, -0.1870078740157480879, -0.4822834645669291653 ) ) ;
#50769=CARTESIAN_POINT ( 'NONE',  ( 0.8595800524934390507, -0.3162353388693405765, 0.4822834645669290543 ) ) ;
#50773=VERTEX_POINT ( 'NONE', #69365 ) ;
#50775=CARTESIAN_POINT ( 'NONE',  ( -1.089238845144356427, 0.05413385826771666132, 0.4176697321401328100 ) ) ;
#50776=CARTESIAN_POINT ( 'NONE',  ( -0.7677165354330699465, -0.5400638737290845981, -0.3530559997133363437 ) ) ;
#50777=CARTESIAN_POINT ( 'NONE',  ( -0.5971128608923877978, -0.5511811023622048555, -0.09757992244046775898 ) ) ;
#50778=CARTESIAN_POINT ( 'NONE',  ( -0.7414698162729651543, -0.6692913385826771977, 0.1292274648535927661 ) ) ;
#50779=CARTESIAN_POINT ( 'NONE',  ( 0.3018372703412079971, 0.05413385826771626580, -0.4176697321401330321 ) ) ;
#50780=CARTESIAN_POINT ( 'NONE',  ( -0.6036745406824141069, -0.6046776061558809534, -0.2411417322834644161 ) ) ;
#50781=CARTESIAN_POINT ( 'NONE',  ( -1.194225721784776262, -0.4281496062992124485, 0.4176697321401328655 ) ) ;
#50782=CARTESIAN_POINT ( 'NONE',  ( -0.8923884514435688198, 0.2306618581243847221, -0.2411417322834647770 ) ) ;
#50783=CARTESIAN_POINT ( 'NONE',  ( 0.7677165354330716118, -0.5400638737290844871, 0.3530559997133364547 ) ) ;
#50785=CARTESIAN_POINT ( 'NONE',  ( -0.6233595800524928121, -0.2845877964562161244, -0.3641732283464567121 ) ) ;
#50789=CARTESIAN_POINT ( 'NONE',  ( -1.410761154855642463, -0.08942795157527998196, 0.3641732283464567121 ) ) ;
#50790=CARTESIAN_POINT ( 'NONE',  ( -0.9186351706036736120, -0.6046776061558809534, -0.2411417322834644161 ) ) ;
#50791=CARTESIAN_POINT ( 'NONE',  ( -0.9908136482939626788, 0.2952755905511811885, 0.1292274648535926551 ) ) ;
#50793=CARTESIAN_POINT ( 'NONE',  ( -0.9842519685039365918, -0.6692913385826771977, 8.415575281601705876E-17 ) ) ;
#50794=CARTESIAN_POINT ( 'NONE',  ( -1.056430446194224881, 0.2952755905511810774, -0.1292274648535930714 ) ) ;
#50795=FACE_OUTER_BOUND ( 'NONE', #24282, .T. ) ;
#50796=DIRECTION ( 'NONE',  ( 1.000000000000000000, -0.000000000000000000, -0.000000000000000000 ) ) ;
#50797=CARTESIAN_POINT ( 'NONE',  ( 0.3937007874015754361, -0.1870078740157479769, 0.3641732283464567677 ) ) ;
#50800=CARTESIAN_POINT ( 'NONE',  ( -0.5380577427821514602, -0.3690944881889765550, -0.3153832671262227771 ) ) ;
#50801=CARTESIAN_POINT ( 'NONE',  ( -0.3608923884514428360, 0.2952755905511811885, 0.1292274648535926551 ) ) ;
#50802=CARTESIAN_POINT ( 'NONE',  ( 1.318897637795276356, 0.1660481256975883668, -0.3530559997133364547 ) ) ;
#50803=CARTESIAN_POINT ( 'NONE',  ( -0.3805774278215216522, 0.05413385826771666132, 0.4176697321401328100 ) ) ;
#50805=ORIENTED_EDGE ( 'NONE', *, *, #2022, .T. ) ;
#50807=CARTESIAN_POINT ( 'NONE',  ( -0.4396325459317577122, -0.6692913385826773087, -0.1292274648535924053 ) ) ;
#50808=CARTESIAN_POINT ( 'NONE',  ( 1.345144356955381593, -0.3162353388693409650, -0.4822834645669289433 ) ) ;
#50809=CARTESIAN_POINT ( 'NONE',  ( -1.128608923884513837, -0.5023911411419708095, 0.1820866141732285504 ) ) ;
#50810=CARTESIAN_POINT ( 'NONE',  ( -1.482939632545930975, -0.4281496062992127816, -0.4176697321401328100 ) ) ;
#50814=CARTESIAN_POINT ( 'NONE',  ( 1.213910761154856299, 0.2952755905511811885, 0.1292274648535926551 ) ) ;
#50816=CARTESIAN_POINT ( 'NONE',  ( 0.006561679790026889343, -0.3162353388693409650, -0.4822834645669289433 ) ) ;
#50817=CARTESIAN_POINT ( 'NONE',  ( -1.062992125984250968, -0.5511811023622047445, 6.969142054262312111E-17 ) ) ;
#50818=CARTESIAN_POINT ( 'NONE',  ( -0.3608923884514428360, -0.6692913385826773087, -0.1292274648535924053 ) ) ;
#50820=CARTESIAN_POINT ( 'NONE',  ( -0.8661417322834640276, -0.1870078740157480879, -0.4822834645669291653 ) ) ;
#50821=CARTESIAN_POINT ( 'NONE',  ( -0.8398950131233589023, -0.6046776061558809534, -0.2411417322834644161 ) ) ;
#50823=CARTESIAN_POINT ( 'NONE',  ( 0.8464566929133865436, 0.07958543189024071263, -0.2665933059059888421 ) ) ;
#50824=CARTESIAN_POINT ( 'NONE',  ( -0.4068241469816267775, -0.004921259842519870586, -0.3153832671262229437 ) ) ;
#50825=CARTESIAN_POINT ( 'NONE',  ( 0.6758530183727039509, -0.5511811023622046335, 0.09757992244046803654 ) ) ;
#50826=CARTESIAN_POINT ( 'NONE',  ( -1.456692913385826182, -0.6692913385826771977, 8.415575281601705876E-17 ) ) ;
#50827=CARTESIAN_POINT ( 'NONE',  ( 1.482939632545932307, 0.05413385826771626580, -0.4176697321401330321 ) ) ;
#50828=CARTESIAN_POINT ( 'NONE',  ( 0.4461942257217856311, 0.1283753931104746893, -0.1820866141732285504 ) ) ;
#50829=CARTESIAN_POINT ( 'NONE',  ( -0.8464566929133852113, 0.1660481256975885056, 0.3530559997133364547 ) ) ;
#50830=CARTESIAN_POINT ( 'NONE',  ( 1.312335958005249825, 0.2306618581243847221, -0.2411417322834647770 ) ) ;
#50831=CONICAL_SURFACE ( 'NONE', #14415, 1.181102362204724310, 0.7853981633974621568 ) ;
#50833=CARTESIAN_POINT ( 'NONE',  ( 0.01312335958005323398, -0.3690944881889765550, -0.3153832671262227771 ) ) ;
#50834=DIRECTION ( 'NONE',  ( 9.929802617766423249E-17, -0.7071067811865507924, -0.7071067811865442421 ) ) ;
#50836=CARTESIAN_POINT ( 'NONE',  ( 0.1509186351706045259, -0.05778040916215560624, -0.4822834645669293319 ) ) ;
#50838=CARTESIAN_POINT ( 'NONE',  ( 1.502624671916010790, -0.2845877964562161244, -0.3641732283464567121 ) ) ;
#50839=CARTESIAN_POINT ( 'NONE',  ( 0.06561679790026316017, -0.004921259842519870586, -0.3153832671262229437 ) ) ;
#50840=CARTESIAN_POINT ( 'NONE',  ( -1.233595800524933894, 0.2306618581243848609, 0.2411417322834645549 ) ) ;
#50841=CARTESIAN_POINT ( 'NONE',  ( -0.4921259842519677963, 0.07958543189024071263, -0.2665933059059888421 ) ) ;
#50843=CARTESIAN_POINT ( 'NONE',  ( -1.259842519685038686, -0.1870078740157479769, 0.4822834645669291653 ) ) ;
#50844=CARTESIAN_POINT ( 'NONE',  ( -0.3149606299212590610, -0.1870078740157480879, -0.4822834645669291653 ) ) ;
#50847=CARTESIAN_POINT ( 'NONE',  ( 0.7283464566929140904, -0.4536011799217368745, -0.2665933059059886201 ) ) ;
#50848=CARTESIAN_POINT ( 'NONE',  ( -0.5708661417322825615, -0.5400638737290844871, 0.3530559997133364547 ) ) ;
#50849=CARTESIAN_POINT ( 'NONE',  ( -0.6889763779527552368, 0.1660481256975885056, 0.3530559997133364547 ) ) ;
#50850=CARTESIAN_POINT ( 'NONE',  ( -0.6036745406824141069, -0.5023911411419708095, -0.1820866141732282451 ) ) ;
#50852=CARTESIAN_POINT ( 'NONE',  ( 0.05249343832021075018, -0.6046776061558807314, 0.2411417322834647770 ) ) ;
#50853=CARTESIAN_POINT ( 'NONE',  ( -1.482939632545930975, -0.3690944881889765550, -0.3153832671262227771 ) ) ;
#50854=CARTESIAN_POINT ( 'NONE',  ( 1.423884514435696191, -0.05778040916215522460, 0.4822834645669289988 ) ) ;
#50857=ORIENTED_EDGE ( 'NONE', *, *, #46912, .F. ) ;
#50858=CARTESIAN_POINT ( 'NONE',  ( -0.7461015444985823475, 1.969952063678500842, 0.5309055118110236338 ) ) ;
#50859=CARTESIAN_POINT ( 'NONE',  ( -1.220472440944881054, 0.2952755905511811885, 0.000000000000000000 ) ) ;
#50860=CARTESIAN_POINT ( 'NONE',  ( -0.8923884514435688198, 0.2306618581243847221, -0.2411417322834647770 ) ) ;
#50861=CARTESIAN_POINT ( 'NONE',  ( -1.437007874015747477, 0.1660481256975883668, -0.3530559997133364547 ) ) ;
#50864=CARTESIAN_POINT ( 'NONE',  ( 1.062992125984252745, 0.2952755905511811885, 0.000000000000000000 ) ) ;
#50865=CARTESIAN_POINT ( 'NONE',  ( -0.08530183727034056085, -0.3162353388693405765, 0.4822834645669290543 ) ) ;
#50868=CARTESIAN_POINT ( 'NONE',  ( 1.017060367454068581, -0.08942795157528024563, -0.3641732283464568787 ) ) ;
#50870=EDGE_LOOP ( 'NONE', ( #40753, #22466, #18801, #19430 ) ) ;
#50873=CARTESIAN_POINT ( 'NONE',  ( 0.3871391076115492380, -0.05778040916215560624, -0.4822834645669293319 ) ) ;
#50874=CARTESIAN_POINT ( 'NONE',  ( -0.6824146981627291497, -0.6046776061558809534, -0.2411417322834644161 ) ) ;
#50875=CARTESIAN_POINT ( 'NONE',  ( 1.574803149606299746, -0.1870078740157479769, 0.4822834645669291653 ) ) ;
#50876=CARTESIAN_POINT ( 'NONE',  ( 0.4724409448818904789, -0.1870078740157480879, -0.4822834645669291653 ) ) ;
#50877=CARTESIAN_POINT ( 'NONE',  ( 1.502624671916010790, -0.05778040916215522460, 0.4822834645669289988 ) ) ;
#50878=CARTESIAN_POINT ( 'NONE',  ( 1.410761154855643795, -0.3162353388693405765, 0.4822834645669290543 ) ) ;
#50879=CARTESIAN_POINT ( 'NONE',  ( -0.03280839895013062252, 0.2952755905511810774, -0.1292274648535930714 ) ) ;
#50880=CARTESIAN_POINT ( 'NONE',  ( -1.351706036745406347, -0.4281496062992124485, 0.4176697321401328655 ) ) ;
#50881=CARTESIAN_POINT ( 'NONE',  ( 1.463254593175853824, 0.2952755905511810774, -0.1292274648535930714 ) ) ;
#50882=CARTESIAN_POINT ( 'NONE',  ( 1.482939632545932307, -0.4281496062992124485, 0.4176697321401328655 ) ) ;
#50884=CARTESIAN_POINT ( 'NONE',  ( 0.9514435695538062676, -0.2845877964562161244, -0.3641732283464567121 ) ) ;
#50888=CARTESIAN_POINT ( 'NONE',  ( 0.1706036745406830368, -0.004921259842519576551, 0.3153832671262227771 ) ) ;
#50890=CARTESIAN_POINT ( 'NONE',  ( 0.09842519685039434474, -0.5400638737290845981, -0.3530559997133363437 ) ) ;
#50891=CARTESIAN_POINT ( 'NONE',  ( 0.5183727034120741983, 0.2952755905511810774, -0.1292274648535930714 ) ) ;
#50892=CARTESIAN_POINT ( 'NONE',  ( -0.3871391076115479057, -0.3162353388693409650, -0.4822834645669289433 ) ) ;
#50894=CARTESIAN_POINT ( 'NONE',  ( -1.023622047244093558, -0.1870078740157479769, 0.4822834645669291653 ) ) ;
#50896=CARTESIAN_POINT ( 'NONE',  ( 1.187664041994751285, -0.2845877964562161244, -0.3641732283464567121 ) ) ;
#50897=CARTESIAN_POINT ( 'NONE',  ( 0.8333333333333340365, -0.6692913385826771977, 0.1292274648535927661 ) ) ;
#50898=CARTESIAN_POINT ( 'NONE',  ( 0.6561679790026253567, -0.6046776061558809534, -0.2411417322834644161 ) ) ;
#50900=CARTESIAN_POINT ( 'NONE',  ( -1.318897637795274802, -0.5400638737290845981, -0.3530559997133363437 ) ) ;
#50903=CARTESIAN_POINT ( 'NONE',  ( -0.05905511811023545637, -0.5400638737290845981, -0.3530559997133363437 ) ) ;
#50906=CARTESIAN_POINT ( 'NONE',  ( 1.397637795275591177, -0.5400638737290844871, 0.3530559997133364547 ) ) ;
#50907=CARTESIAN_POINT ( 'NONE',  ( 1.469816272965879911, -0.6046776061558807314, 0.2411417322834647770 ) ) ;
#50908=CARTESIAN_POINT ( 'NONE',  ( 0.05249343832021075018, -0.5023911411419708095, 0.1820866141732285504 ) ) ;
#50909=CARTESIAN_POINT ( 'NONE',  ( 0.9383202099737536495, -0.3162353388693405765, 0.4822834645669290543 ) ) ;
#50911=CARTESIAN_POINT ( 'NONE',  ( 0.2624671916010504757, 0.1283753931104748280, 0.1820866141732283561 ) ) ;
#50912=CARTESIAN_POINT ( 'NONE',  ( 0.2296587926509192634, -0.05778040916215560624, -0.4822834645669293319 ) ) ;
#50915=CARTESIAN_POINT ( 'NONE',  ( -1.364829396325458521, 0.2306618581243847221, -0.2411417322834647770 ) ) ;
#50916=CARTESIAN_POINT ( 'NONE',  ( 1.122047244094488860, 0.07958543189024085140, 0.2665933059059887866 ) ) ;
#50918=CARTESIAN_POINT ( 'NONE',  ( -0.3674540682414692561, -0.6046776061558809534, -0.2411417322834644161 ) ) ;
#50919=CARTESIAN_POINT ( 'NONE',  ( 0.1115485564304470323, 0.1771653543307087630, 0.09757992244046791164 ) ) ;
#50920=CARTESIAN_POINT ( 'NONE',  ( 0.4531182788721078158, 1.771653543307086354, 0.5309055118110234117 ) ) ;
#50921=CARTESIAN_POINT ( 'NONE',  ( -0.3608923884514428360, -0.6692913385826773087, -0.1292274648535924053 ) ) ;
#50922=CARTESIAN_POINT ( 'NONE',  ( 0.1706036745406830368, -0.004921259842519576551, 0.3153832671262227771 ) ) ;
#50924=CARTESIAN_POINT ( 'NONE',  ( -0.2165354330708654795, 0.1660481256975885056, 0.3530559997133364547 ) ) ;
#50926=CARTESIAN_POINT ( 'NONE',  ( 1.062992125984252745, 0.1771653543307087630, 0.000000000000000000 ) ) ;
#50927=CARTESIAN_POINT ( 'NONE',  ( 1.614173228346457378, 0.2952755905511811885, 0.000000000000000000 ) ) ;
#50929=CARTESIAN_POINT ( 'NONE',  ( -0.8070866141732276899, -0.4536011799217367080, 0.2665933059059888421 ) ) ;
#50930=CARTESIAN_POINT ( 'NONE',  ( -0.6036745406824141069, 0.1283753931104748280, 0.1820866141732283561 ) ) ;
#50931=CARTESIAN_POINT ( 'NONE',  ( -0.4199475065616791736, -0.6046776061558807314, 0.2411417322834647770 ) ) ;
#50932=CARTESIAN_POINT ( 'NONE',  ( -0.1771653543307080136, -0.5400638737290844871, 0.3530559997133364547 ) ) ;
#50933=CARTESIAN_POINT ( 'NONE',  ( 1.082677165354331228, 0.07958543189024071263, -0.2665933059059888421 ) ) ;
#50935=CARTESIAN_POINT ( 'NONE',  ( 1.437007874015748810, 0.07958543189024085140, 0.2665933059059887866 ) ) ;
#50937=CARTESIAN_POINT ( 'NONE',  ( 0.5446194225721792126, -0.3162353388693405765, 0.4822834645669290543 ) ) ;
#50938=CARTESIAN_POINT ( 'NONE',  ( -1.603475055217291612, 1.819038169495759361, -0.04573490813648263542 ) ) ;
#50939=CARTESIAN_POINT ( 'NONE',  ( -0.4527559055118102749, 0.1660481256975885056, 0.3530559997133364547 ) ) ;
#50941=CARTESIAN_POINT ( 'NONE',  ( -1.423884514435694859, -0.3162353388693405765, 0.4822834645669290543 ) ) ;
#50942=CARTESIAN_POINT ( 'NONE',  ( 0.8267716535433078384, -0.6692913385826771977, 8.415575281601705876E-17 ) ) ;
#50943=CARTESIAN_POINT ( 'NONE',  ( 0.5249343832021005074, -0.6046776061558807314, 0.2411417322834647770 ) ) ;
#50945=CARTESIAN_POINT ( 'NONE',  ( 0.2296587926509192634, -0.2845877964562159024, 0.3641732283464567677 ) ) ;
#50946=CARTESIAN_POINT ( 'NONE',  ( 1.391076115485564868, 0.2306618581243847221, -0.2411417322834647770 ) ) ;
#50947=CARTESIAN_POINT ( 'NONE',  ( -0.4593175853018366950, -0.004921259842519576551, 0.3153832671262227771 ) ) ;
#50948=CARTESIAN_POINT ( 'NONE',  ( -0.7349081364829387342, -0.6046776061558807314, 0.2411417322834647770 ) ) ;
#50949=CARTESIAN_POINT ( 'NONE',  ( 0.8005249343832027131, 0.05413385826771666132, 0.4176697321401328100 ) ) ;
#50950=CARTESIAN_POINT ( 'NONE',  ( 0.1509186351706042484, -0.3162353388693405765, 0.4822834645669290543 ) ) ;
#50951=CARTESIAN_POINT ( 'NONE',  ( -0.9251968503937002541, -0.5400638737290845981, -0.3530559997133363437 ) ) ;
#50952=CARTESIAN_POINT ( 'NONE',  ( -0.7217847769028863381, -0.004921259842519870586, -0.3153832671262229437 ) ) ;
#50953=CARTESIAN_POINT ( 'NONE',  ( 0.3740157480314966754, 0.1660481256975883668, -0.3530559997133364547 ) ) ;
#50954=CARTESIAN_POINT ( 'NONE',  ( -1.443569553805773564, -0.6046776061558807314, 0.2411417322834647770 ) ) ;
#50955=CARTESIAN_POINT ( 'NONE',  ( -0.1837270341207340729, 0.2306618581243847221, -0.2411417322834647770 ) ) ;
#50956=DIRECTION ( 'NONE',  ( 1.000000000000000000, -0.000000000000000000, -0.000000000000000000 ) ) ;
#50957=CARTESIAN_POINT ( 'NONE',  ( 1.253280839895013710, -0.3162353388693405765, 0.4822834645669290543 ) ) ;
#50958=CARTESIAN_POINT ( 'NONE',  ( 1.174540682414699111, -0.3162353388693405765, 0.4822834645669290543 ) ) ;
#50961=CARTESIAN_POINT ( 'NONE',  ( -0.7020997375328076329, -0.3162353388693409650, -0.4822834645669289433 ) ) ;
#50964=VERTEX_POINT ( 'NONE', #61390 ) ;
#50965=CARTESIAN_POINT ( 'NONE',  ( -0.04593175853018302557, 0.1771653543307087630, 0.09757992244046791164 ) ) ;
#50967=CARTESIAN_POINT ( 'NONE',  ( 0.8530183727034126306, 0.05413385826771626580, -0.4176697321401330321 ) ) ;
#50970=CARTESIAN_POINT ( 'NONE',  ( -0.4461942257217840213, -0.5023911411419708095, -0.1820866141732282451 ) ) ;
#50972=CARTESIAN_POINT ( 'NONE',  ( 1.286089238845145033, -0.6046776061558809534, -0.2411417322834644161 ) ) ;
#50973=CARTESIAN_POINT ( 'NONE',  ( 0.9776902887139113929, 0.1771653543307087630, 0.09757992244046791164 ) ) ;
#50974=CARTESIAN_POINT ( 'NONE',  ( -0.1574803149606292529, -0.1870078740157480879, -0.4822834645669291653 ) ) ;
#50976=CARTESIAN_POINT ( 'NONE',  ( -0.2362204724409440182, -0.1870078740157479769, 0.4822834645669291653 ) ) ;
#50977=CARTESIAN_POINT ( 'NONE',  ( -1.397637795275589623, 0.07958543189024085140, 0.2665933059059887866 ) ) ;
#50978=CARTESIAN_POINT ( 'NONE',  ( -0.5708661417322828946, 0.1660481256975883668, -0.3530559997133364547 ) ) ;
#50979=CARTESIAN_POINT ( 'NONE',  ( 0.4849061582275022153, 1.967896864084103914, -0.4921425059946357705 ) ) ;
#50980=CARTESIAN_POINT ( 'NONE',  ( 0.6423408027444581503, 0.000000000000000000, 0.3464511005275205946 ) ) ;
#50981=VERTEX_POINT ( 'NONE', #22678 ) ;
#50983=CARTESIAN_POINT ( 'NONE',  ( 0.4790026246719168435, -0.3162353388693409650, -0.4822834645669289433 ) ) ;
#50985=CARTESIAN_POINT ( 'NONE',  ( -0.6364829396325453192, -0.3162353388693405765, 0.4822834645669290543 ) ) ;
#50986=CARTESIAN_POINT ( 'NONE',  ( 1.555118110236221041, -0.5400638737290844871, 0.3530559997133364547 ) ) ;
#50987=CARTESIAN_POINT ( 'NONE',  ( 0.5380577427821529035, 0.05413385826771626580, -0.4176697321401330321 ) ) ;
#50988=CARTESIAN_POINT ( 'NONE',  ( 0.1706036745406830368, -0.4281496062992127816, -0.4176697321401328100 ) ) ;
#50990=CARTESIAN_POINT ( 'NONE',  ( -0.8464566929133852113, -0.5400638737290845981, -0.3530559997133363437 ) ) ;
#50991=CARTESIAN_POINT ( 'NONE',  ( -0.2362204724409440182, -0.1870078740157479769, 0.4822834645669291653 ) ) ;
#50992=CARTESIAN_POINT ( 'NONE',  ( -1.062992125984250968, -0.6692913385826771977, 8.415575281601705876E-17 ) ) ;
#50993=CARTESIAN_POINT ( 'NONE',  ( -0.1509186351706028884, -0.2845877964562161244, -0.3641732283464567121 ) ) ;
#50995=CARTESIAN_POINT ( 'NONE',  ( -0.09186351706036689768, 0.05413385826771626580, -0.4176697321401330321 ) ) ;
#50997=CARTESIAN_POINT ( 'NONE',  ( 1.095800524934383846, -0.3162353388693405765, 0.4822834645669290543 ) ) ;
#50999=VERTEX_POINT ( 'NONE', #36540 ) ;
#51001=CARTESIAN_POINT ( 'NONE',  ( 0.2493438320209980519, 0.05413385826771666132, 0.4176697321401328100 ) ) ;
#51002=CARTESIAN_POINT ( 'NONE',  ( -0.1181102362204717315, 0.1771653543307087630, 0.000000000000000000 ) ) ;
#51003=CARTESIAN_POINT ( 'NONE',  ( 1.541994750656168645, 0.1771653543307087075, -0.09757992244046823083 ) ) ;
#51007=CARTESIAN_POINT ( 'NONE',  ( 1.469816272965879911, -0.5023911411419708095, 0.1820866141732285504 ) ) ;
#51008=CARTESIAN_POINT ( 'NONE',  ( 1.496062992125984703, -0.1870078740157480879, -0.4822834645669291653 ) ) ;
#51010=CARTESIAN_POINT ( 'NONE',  ( 0.6627296587926515548, 0.2952755905511811885, 0.1292274648535926551 ) ) ;
#51011=CARTESIAN_POINT ( 'NONE',  ( -1.286089238845143479, 0.2306618581243847221, -0.2411417322834647770 ) ) ;
#51012=CARTESIAN_POINT ( 'NONE',  ( -1.266404199475064773, -0.3162353388693405765, 0.4822834645669290543 ) ) ;
#51013=CARTESIAN_POINT ( 'NONE',  ( 0.1049868766404206816, -0.6046776061558809534, -0.2411417322834644161 ) ) ;
#51015=CARTESIAN_POINT ( 'NONE',  ( 1.541994750656168645, 0.2952755905511810774, -0.1292274648535930714 ) ) ;
#51016=CARTESIAN_POINT ( 'NONE',  ( 0.9251968503937015864, -0.5400638737290844871, 0.3530559997133364547 ) ) ;
#51017=CARTESIAN_POINT ( 'NONE',  ( 1.496062992125985147, -0.1870078740157479769, 0.3641732283464567677 ) ) ;
#51018=LINE ( 'NONE', #80682, #58658 ) ;
#51020=CARTESIAN_POINT ( 'NONE',  ( 0.7611548556430454138, 0.1283753931104746893, -0.1820866141732285504 ) ) ;
#51021=CARTESIAN_POINT ( 'NONE',  ( -0.9776902887139098386, 0.2952755905511810774, -0.1292274648535930714 ) ) ;
#51023=CARTESIAN_POINT ( 'NONE',  ( -1.640419947506561060, -0.004921259842519576551, 0.3153832671262227771 ) ) ;
#51025=CARTESIAN_POINT ( 'NONE',  ( 0.6364829396325465405, -0.3162353388693409650, -0.4822834645669289433 ) ) ;
#51027=CARTESIAN_POINT ( 'NONE',  ( -1.548556430446193399, 0.1283753931104748280, 0.1820866141732283561 ) ) ;
#51028=CARTESIAN_POINT ( 'NONE',  ( -0.09842519685039295696, -0.5400638737290844871, 0.3530559997133364547 ) ) ;
#51029=CARTESIAN_POINT ( 'NONE',  ( 0.9317585301837276734, -0.3690944881889763329, 0.3153832671262228327 ) ) ;
#51030=CARTESIAN_POINT ( 'NONE',  ( 0.9645669291338591078, -0.5400638737290845981, -0.3530559997133363437 ) ) ;
#51032=CARTESIAN_POINT ( 'NONE',  ( -0.6692913385826764205, -0.5511811023622047445, 6.969142054262312111E-17 ) ) ;
#51033=CARTESIAN_POINT ( 'NONE',  ( -0.6233595800524928121, -0.05778040916215522460, 0.4822834645669289988 ) ) ;
#51034=CARTESIAN_POINT ( 'NONE',  ( 1.601049868766404982, -0.6046776061558809534, -0.2411417322834644161 ) ) ;
#51035=CARTESIAN_POINT ( 'NONE',  ( -1.154855643044618851, -0.6046776061558809534, -0.2411417322834644161 ) ) ;
#51036=CARTESIAN_POINT ( 'NONE',  ( 1.010498687664042716, -0.4281496062992124485, 0.4176697321401328655 ) ) ;
#51038=CARTESIAN_POINT ( 'NONE',  ( -1.266404199475064773, -0.08942795157528024563, -0.3641732283464568787 ) ) ;
#51039=DIRECTION ( 'NONE',  ( 1.000000000000000000, -0.000000000000000000, -0.000000000000000000 ) ) ;
#51040=CARTESIAN_POINT ( 'NONE',  ( 1.095800524934383846, -0.3162353388693405765, 0.4822834645669290543 ) ) ;
#51042=CARTESIAN_POINT ( 'NONE',  ( -1.732283464566928277, -0.1870078740157479769, 0.4822834645669291653 ) ) ;
#51043=CARTESIAN_POINT ( 'NONE',  ( 1.607611548556431069, -0.6692913385826773087, -0.1292274648535924053 ) ) ;
#51044=CARTESIAN_POINT ( 'NONE',  ( -1.174540682414697335, -0.2845877964562161244, -0.3641732283464567121 ) ) ;
#51046=CARTESIAN_POINT ( 'NONE',  ( -0.4593175853018364174, -0.4281496062992127816, -0.4176697321401328100 ) ) ;
#51047=CARTESIAN_POINT ( 'NONE',  ( -0.2296587926509179312, -0.08942795157527998196, 0.3641732283464567121 ) ) ;
#51048=CARTESIAN_POINT ( 'NONE',  ( -1.706036745406823485, 0.1283753931104748280, 0.1820866141732283561 ) ) ;
#51049=CARTESIAN_POINT ( 'NONE',  ( 1.076115485564305141, -0.5023911411419708095, 0.1820866141732285504 ) ) ;
#51050=CARTESIAN_POINT ( 'NONE',  ( 1.115485564304462551, -0.4281496062992127816, -0.4176697321401328100 ) ) ;
#51051=CARTESIAN_POINT ( 'NONE',  ( 1.548556430446194954, -0.6046776061558807314, 0.2411417322834647770 ) ) ;
#51052=CARTESIAN_POINT ( 'NONE',  ( -0.1049868766404193215, -0.5023911411419708095, 0.1820866141732285504 ) ) ;
#51053=CARTESIAN_POINT ( 'NONE',  ( 0.5183727034120741983, -0.6692913385826771977, 0.1292274648535927661 ) ) ;
#51054=EDGE_CURVE ( 'NONE', #14996, #25851, #11719, .T. ) ;
#51055=CARTESIAN_POINT ( 'NONE',  ( 0.4461942257217855201, -0.5023911411419708095, 0.1820866141732285504 ) ) ;
#51056=CARTESIAN_POINT ( 'NONE',  ( 1.456692913385827515, 0.2952755905511811885, 0.000000000000000000 ) ) ;
#51057=ADVANCED_FACE ( 'NONE', ( #75276 ), #45571, .F. ) ;
#51058=CARTESIAN_POINT ( 'NONE',  ( -1.292650918635170010, 0.2952755905511810774, -0.1292274648535930714 ) ) ;
#51059=CARTESIAN_POINT ( 'NONE',  ( -0.3740157480314953431, -0.5400638737290845981, -0.3530559997133363437 ) ) ;
#51062=CARTESIAN_POINT ( 'NONE',  ( 0.6364829396325465405, -0.05778040916215522460, 0.4822834645669289988 ) ) ;
#51063=CARTESIAN_POINT ( 'NONE',  ( 1.181102362204724976, -0.1870078740157480601, -0.3641732283464567677 ) ) ;
#51064=CARTESIAN_POINT ( 'NONE',  ( -0.4593175853018364174, -0.4281496062992127816, -0.4176697321401328100 ) ) ;
#51065=CARTESIAN_POINT ( 'NONE',  ( 0.5249343832021003964, 0.2306618581243847221, -0.2411417322834647770 ) ) ;
#51071=CARTESIAN_POINT ( 'NONE',  ( -0.8136482939632537770, -0.5023911411419708095, 0.1820866141732285504 ) ) ;
#51072=CARTESIAN_POINT ( 'NONE',  ( -0.9842519685039365918, -0.6692913385826771977, 8.415575281601705876E-17 ) ) ;
#51074=CARTESIAN_POINT ( 'NONE',  ( 0.9842519685039378130, -0.6692913385826771977, 8.415575281601705876E-17 ) ) ;
#51076=CARTESIAN_POINT ( 'NONE',  ( 1.312335958005249825, 0.2306618581243847221, -0.2411417322834647770 ) ) ;
#51077=CARTESIAN_POINT ( 'NONE',  ( 0.7414698162729663755, -0.6692913385826773087, -0.1292274648535924053 ) ) ;
#51082=CARTESIAN_POINT ( 'NONE',  ( 0.4199475065616803948, -0.6046776061558809534, -0.2411417322834644161 ) ) ;
#51083=CARTESIAN_POINT ( 'NONE',  ( 0.7283464566929140904, -0.5400638737290845981, -0.3530559997133363437 ) ) ;
#51084=CARTESIAN_POINT ( 'NONE',  ( 0.6430446194225728496, -0.004921259842519576551, 0.3153832671262227771 ) ) ;
#51085=CARTESIAN_POINT ( 'NONE',  ( 1.502624671916010790, -0.05778040916215522460, 0.4822834645669289988 ) ) ;
#51087=CARTESIAN_POINT ( 'NONE',  ( 0.5708661417322841158, -0.5400638737290845981, -0.3530559997133363437 ) ) ;
#51088=CARTESIAN_POINT ( 'NONE',  ( 1.056430446194226658, 0.2952755905511811885, 0.1292274648535926551 ) ) ;
#51089=CARTESIAN_POINT ( 'NONE',  ( 0.4790026246719168435, -0.3162353388693409650, -0.4822834645669289433 ) ) ;
#51090=CARTESIAN_POINT ( 'NONE',  ( 1.325459317585302665, -0.3690944881889763329, 0.3153832671262228327 ) ) ;
#51091=CARTESIAN_POINT ( 'NONE',  ( -0.9645669291338575535, -0.5400638737290844871, 0.3530559997133364547 ) ) ;
#51092=CARTESIAN_POINT ( 'NONE',  ( -0.7874015748031489847, -0.1870078740157479769, 0.4822834645669291653 ) ) ;
#51093=CARTESIAN_POINT ( 'NONE',  ( 1.181102362204724976, -0.1870078740157480879, -0.4822834645669291653 ) ) ;
#51101=CARTESIAN_POINT ( 'NONE',  ( 1.660104986876641320, -0.05778040916215522460, 0.4822834645669289988 ) ) ;
#51102=CARTESIAN_POINT ( 'NONE',  ( 1.240157480314961314, -0.4536011799217367080, 0.2665933059059888421 ) ) ;
#51104=CARTESIAN_POINT ( 'NONE',  ( 1.410761154855643795, -0.08942795157528024563, -0.3641732283464568787 ) ) ;
#51106=CARTESIAN_POINT ( 'NONE',  ( -0.09842519685039295696, 0.1660481256975883391, -0.3530559997133364547 ) ) ;
#51109=CARTESIAN_POINT ( 'NONE',  ( -0.6758530183727028406, 0.1771653543307087630, 0.09757992244046791164 ) ) ;
#51110=CARTESIAN_POINT ( 'NONE',  ( -1.706036745406823485, 0.1283753931104748280, 0.1820866141732283561 ) ) ;
#51111=CARTESIAN_POINT ( 'NONE',  ( -1.463254593175852492, 0.2952755905511811885, 0.1292274648535926551 ) ) ;
#51112=CARTESIAN_POINT ( 'NONE',  ( 0.2624671916010504757, -0.6046776061558809534, -0.2411417322834644161 ) ) ;
#51113=CARTESIAN_POINT ( 'NONE',  ( 1.489501312335958172, -0.05778040916215560624, -0.4822834645669293319 ) ) ;
#51120=CARTESIAN_POINT ( 'NONE',  ( -0.6889763779527552368, 0.07958543189024085140, 0.2665933059059887866 ) ) ;
#51121=CARTESIAN_POINT ( 'NONE',  ( -1.141732283464566011, 0.2952755905511811885, 0.000000000000000000 ) ) ;
#51122=CARTESIAN_POINT ( 'NONE',  ( 0.9186351706036752773, 0.2306618581243847221, -0.2411417322834647770 ) ) ;
#51127=CARTESIAN_POINT ( 'NONE',  ( 1.056430446194226658, 0.2952755905511811885, 0.1292274648535926551 ) ) ;
#51128=CARTESIAN_POINT ( 'NONE',  ( -1.043307086614172707, 0.1660481256975883668, -0.3530559997133364547 ) ) ;
#51130=CARTESIAN_POINT ( 'NONE',  ( -0.5511811023622041894, -0.1870078740157480601, -0.3641732283464567677 ) ) ;
#51132=CARTESIAN_POINT ( 'NONE',  ( -0.3346456692913377662, 0.07958543189024071263, -0.2665933059059888421 ) ) ;
#51133=CARTESIAN_POINT ( 'NONE',  ( -0.04593175853018302557, -0.5511811023622048555, -0.09757992244046775898 ) ) ;
#51134=CARTESIAN_POINT ( 'NONE',  ( 0.1377952755905518800, -0.5400638737290844871, 0.3530559997133364547 ) ) ;
#51135=CARTESIAN_POINT ( 'NONE',  ( -0.8333333333333323711, 0.1771653543307087630, 0.09757992244046791164 ) ) ;
#51137=CARTESIAN_POINT ( 'NONE',  ( 1.128608923884514947, 0.2306618581243848609, 0.2411417322834645549 ) ) ;
#51139=CARTESIAN_POINT ( 'NONE',  ( -1.305774278215222184, 0.2952755905511811885, 0.1292274648535926551 ) ) ;
#51141=CARTESIAN_POINT ( 'NONE',  ( -0.1771653543307080136, -0.5400638737290844871, 0.3530559997133364547 ) ) ;
#51142=CARTESIAN_POINT ( 'NONE',  ( -0.7874015748031489847, -0.1870078740157480879, -0.4822834645669291653 ) ) ;
#51143=CARTESIAN_POINT ( 'NONE',  ( 1.456692913385827515, -0.5511811023622047445, 6.969142054262312111E-17 ) ) ;
#51144=CARTESIAN_POINT ( 'NONE',  ( -0.4658792650918627265, -0.08942795157527998196, 0.3641732283464567121 ) ) ;
#51145=CARTESIAN_POINT ( 'NONE',  ( -0.6102362204724400829, 0.1660481256975885056, 0.3530559997133364547 ) ) ;
#51146=CARTESIAN_POINT ( 'NONE',  ( -1.167979002624671470, 0.05413385826771666132, 0.4176697321401328100 ) ) ;
#51148=CARTESIAN_POINT ( 'NONE',  ( 1.404199475065617708, -0.004921259842519870586, -0.3153832671262229437 ) ) ;
#51149=CARTESIAN_POINT ( 'NONE',  ( -0.05905511811023545637, 0.1660481256975885056, 0.3530559997133364547 ) ) ;
#51150=CARTESIAN_POINT ( 'NONE',  ( -1.496062992125983815, -0.1870078740157480879, -0.4822834645669291653 ) ) ;
#51153=CARTESIAN_POINT ( 'NONE',  ( -0.8136482939632537770, 0.1283753931104746893, -0.1820866141732285504 ) ) ;
#51154=CARTESIAN_POINT ( 'NONE',  ( 0.6561679790026253567, 0.2306618581243848609, 0.2411417322834645549 ) ) ;
#51155=CARTESIAN_POINT ( 'NONE',  ( -0.9383202099737524282, -0.08942795157527998196, 0.3641732283464567121 ) ) ;
#51157=CARTESIAN_POINT ( 'NONE',  ( -1.141732283464566011, -0.6692913385826771977, 8.415575281601705876E-17 ) ) ;
#51158=CARTESIAN_POINT ( 'NONE',  ( 0.9580052493438327987, -0.4281496062992127816, -0.4176697321401328100 ) ) ;
#51159=CARTESIAN_POINT ( 'NONE',  ( 0.5971128608923891301, 0.2952755905511810774, -0.1292274648535930714 ) ) ;
#51161=CARTESIAN_POINT ( 'NONE',  ( -1.581364829396324945, -0.2845877964562159024, 0.3641732283464567677 ) ) ;
#51166=CARTESIAN_POINT ( 'NONE',  ( 1.122047244094488860, -0.4536011799217368745, -0.2665933059059886201 ) ) ;
#51167=CARTESIAN_POINT ( 'NONE',  ( 0.8005249343832027131, -0.004921259842519576551, 0.3153832671262227771 ) ) ;
#51169=CARTESIAN_POINT ( 'NONE',  ( 0.1049868766404206816, -0.6046776061558809534, -0.2411417322834644161 ) ) ;
#51172=CARTESIAN_POINT ( 'NONE',  ( 0.2624671916010504757, 0.1283753931104748280, 0.1820866141732283561 ) ) ;
#51173=CARTESIAN_POINT ( 'NONE',  ( -0.6430446194225712953, 0.05413385826771626580, -0.4176697321401330321 ) ) ;
#51174=CARTESIAN_POINT ( 'NONE',  ( -1.318897637795274802, 0.1660481256975885056, 0.3530559997133364547 ) ) ;
#51175=CARTESIAN_POINT ( 'NONE',  ( 0.7152230971128616943, -0.05778040916215522460, 0.4822834645669289988 ) ) ;
#51180=CARTESIAN_POINT ( 'NONE',  ( -1.148293963254592542, -0.6692913385826773087, -0.1292274648535924053 ) ) ;
#51181=CARTESIAN_POINT ( 'NONE',  ( -0.7480314960629914633, -0.6692913385826771977, 8.415575281601705876E-17 ) ) ;
#51182=CARTESIAN_POINT ( 'NONE',  ( -0.7874015748031489847, -0.1870078740157480601, -0.3641732283464567677 ) ) ;
#51183=CARTESIAN_POINT ( 'NONE',  ( -0.6692913385826764205, 0.2952755905511811885, 0.000000000000000000 ) ) ;
#51186=CARTESIAN_POINT ( 'NONE',  ( 1.496062992125985147, -0.1870078740157479769, 0.4822834645669291653 ) ) ;
#51188=CARTESIAN_POINT ( 'NONE',  ( -0.6561679790026240244, -0.6046776061558807314, 0.2411417322834647770 ) ) ;
#51189=CARTESIAN_POINT ( 'NONE',  ( 0.3805774278215230400, 0.05413385826771626580, -0.4176697321401330321 ) ) ;
#51190=CARTESIAN_POINT ( 'NONE',  ( -0.9120734908136475250, -0.6692913385826773087, -0.1292274648535924053 ) ) ;
#51192=CARTESIAN_POINT ( 'NONE',  ( -0.9908136482939626788, 0.1771653543307087630, 0.09757992244046791164 ) ) ;
#51196=CARTESIAN_POINT ( 'NONE',  ( -1.502624671916009680, -0.08942795157528024563, -0.3641732283464568787 ) ) ;
#51197=CARTESIAN_POINT ( 'NONE',  ( -1.272965879265091305, 0.05413385826771626580, -0.4176697321401330321 ) ) ;
#51198=CARTESIAN_POINT ( 'NONE',  ( -1.082677165354329896, -0.5400638737290845981, -0.3530559997133363437 ) ) ;
#51200=CARTESIAN_POINT ( 'NONE',  ( -1.220472440944881054, 0.2952755905511811885, 0.000000000000000000 ) ) ;
#51201=CARTESIAN_POINT ( 'NONE',  ( -1.122047244094487306, -0.5400638737290844871, 0.3530559997133364547 ) ) ;
#51202=CARTESIAN_POINT ( 'NONE',  ( 0.4606732211678788991, 2.793565526369266028, 0.5309055118110233007 ) ) ;
#51203=EDGE_CURVE ( 'NONE', #73164, #12831, #72809, .T. ) ;
#51205=CARTESIAN_POINT ( 'NONE',  ( 0.3215223097112867578, -0.2845877964562161244, -0.3641732283464567121 ) ) ;
#51206=CARTESIAN_POINT ( 'NONE',  ( 2.795275590551181910, 1.488513638086842006, 0.000000000000000000 ) ) ;
#51208=CARTESIAN_POINT ( 'NONE',  ( -0.1968503937007867743, -0.5511811023622047445, 6.969142054262312111E-17 ) ) ;
#51209=CARTESIAN_POINT ( 'NONE',  ( -0.8727034120734901146, -0.3162353388693405765, 0.4822834645669290543 ) ) ;
#51211=CARTESIAN_POINT ( 'NONE',  ( 1.535433070866142335, -0.6692913385826771977, 8.415575281601705876E-17 ) ) ;
#51212=CARTESIAN_POINT ( 'NONE',  ( -0.4068241469816264999, -0.4281496062992124485, 0.4176697321401328655 ) ) ;
#51213=ORIENTED_EDGE ( 'NONE', *, *, #78524, .F. ) ;
#51214=ORIENTED_EDGE ( 'NONE', *, *, #48987, .F. ) ;
#51216=CARTESIAN_POINT ( 'NONE',  ( -0.4133858267716528645, -0.5400638737290844871, 0.3530559997133364547 ) ) ;
#51217=CARTESIAN_POINT ( 'NONE',  ( 1.207349081364829990, -0.6046776061558809534, -0.2411417322834644161 ) ) ;
#51218=CARTESIAN_POINT ( 'NONE',  ( -1.318897637795274802, -0.4536011799217368745, -0.2665933059059886201 ) ) ;
#51219=CARTESIAN_POINT ( 'NONE',  ( -1.207349081364828880, 0.2306618581243847221, -0.2411417322834647770 ) ) ;
#51224=CARTESIAN_POINT ( 'NONE',  ( 0.2624671916010504757, 0.2306618581243848609, 0.2411417322834645549 ) ) ;
#51225=CARTESIAN_POINT ( 'NONE',  ( -1.017060367454067249, -0.08942795157527998196, 0.3641732283464567121 ) ) ;
#51226=CARTESIAN_POINT ( 'NONE',  ( -0.6233595800524928121, -0.05778040916215522460, 0.4822834645669289988 ) ) ;
#51228=CARTESIAN_POINT ( 'NONE',  ( -0.6824146981627291497, -0.6046776061558809534, -0.2411417322834644161 ) ) ;
#51229=CARTESIAN_POINT ( 'NONE',  ( -1.148293963254592542, -0.6692913385826773087, -0.1292274648535924053 ) ) ;
#51230=CARTESIAN_POINT ( 'NONE',  ( 0.01312335958005323398, 0.05413385826771666132, 0.4176697321401328100 ) ) ;
#51232=CARTESIAN_POINT ( 'NONE',  ( 1.003937007874016185, 0.07958543189024071263, -0.2665933059059888421 ) ) ;
#51233=CARTESIAN_POINT ( 'NONE',  ( -0.9055118110236215490, 0.1771653543307087630, 0.000000000000000000 ) ) ;
#51234=CARTESIAN_POINT ( 'NONE',  ( 0.7283464566929143125, 0.07958543189024085140, 0.2665933059059887866 ) ) ;
#51235=CARTESIAN_POINT ( 'NONE',  ( 1.227034120734908917, -0.5511811023622046335, 0.09757992244046803654 ) ) ;
#51236=CARTESIAN_POINT ( 'NONE',  ( 1.272965879265092637, 0.05413385826771666132, 0.4176697321401328100 ) ) ;
#51237=CARTESIAN_POINT ( 'NONE',  ( 0.5249343832021005074, -0.5023911411419708095, 0.1820866141732285504 ) ) ;
#51239=CARTESIAN_POINT ( 'NONE',  ( -0.6889763779527552368, 0.1660481256975885056, 0.3530559997133364547 ) ) ;
#51240=CARTESIAN_POINT ( 'NONE',  ( 1.062992125984252745, -0.6692913385826771977, 8.415575281601705876E-17 ) ) ;
#51241=CARTESIAN_POINT ( 'NONE',  ( 0.01968503937007957949, -0.4536011799217368745, -0.2665933059059886201 ) ) ;
#51243=CARTESIAN_POINT ( 'NONE',  ( 0.3477690288713918276, -0.6692913385826773087, -0.1292274648535924053 ) ) ;
#51245=CARTESIAN_POINT ( 'NONE',  ( 0.8595800524934390507, -0.08942795157528024563, -0.3641732283464568787 ) ) ;
#51246=CARTESIAN_POINT ( 'NONE',  ( 0.2034120734908142214, 0.1771653543307087075, -0.09757992244046823083 ) ) ;
#51247=CARTESIAN_POINT ( 'NONE',  ( 0.05905511811023709395, -0.5400638737290844871, 0.3530559997133364547 ) ) ;
#51248=CARTESIAN_POINT ( 'NONE',  ( -1.253280839895012377, -0.05778040916215522460, 0.4822834645669289988 ) ) ;
#51249=CARTESIAN_POINT ( 'NONE',  ( -0.8727034120734901146, -0.2845877964562159024, 0.3641732283464567677 ) ) ;
#51250=DIRECTION ( 'NONE',  ( -3.096699300667737957E-16, 1.000000000000000000, -0.000000000000000000 ) ) ;
#51251=CARTESIAN_POINT ( 'NONE',  ( -0.5511811023622038563, -0.1870078740157479769, 0.4822834645669291653 ) ) ;
#51254=CARTESIAN_POINT ( 'NONE',  ( 0.01312335958005323398, -0.004921259842519576551, 0.3153832671262227771 ) ) ;
#51255=CARTESIAN_POINT ( 'NONE',  ( -0.4921259842519677963, 0.1660481256975883668, -0.3530559997133364547 ) ) ;
#51256=CARTESIAN_POINT ( 'NONE',  ( -1.128608923884513837, 0.2306618581243847221, -0.2411417322834647770 ) ) ;
#51257=CARTESIAN_POINT ( 'NONE',  ( -1.095800524934382292, -0.2845877964562161244, -0.3641732283464567121 ) ) ;
#51259=CARTESIAN_POINT ( 'NONE',  ( -0.3937007874015740483, -0.1870078740157479769, 0.4822834645669291653 ) ) ;
#51260=CARTESIAN_POINT ( 'NONE',  ( -0.7020997375328074108, -0.08942795157527998196, 0.3641732283464567121 ) ) ;
#51261=CARTESIAN_POINT ( 'NONE',  ( -1.496062992125983815, -0.1870078740157480601, -0.3641732283464567677 ) ) ;
#51262=CARTESIAN_POINT ( 'NONE',  ( 1.148293963254593653, 0.2952755905511810774, -0.1292274648535930714 ) ) ;
#51263=DIRECTION ( 'NONE',  ( -1.000000000000000000, -3.050063254464715781E-16, 0.000000000000000000 ) ) ;
#51265=ORIENTED_EDGE ( 'NONE', *, *, #58971, .T. ) ;
#51266=CARTESIAN_POINT ( 'NONE',  ( 1.603475055217291612, 1.054977578535739591, 0.04573490813648269093 ) ) ;
#51267=CARTESIAN_POINT ( 'NONE',  ( -1.351706036745406347, 0.05413385826771626580, -0.4176697321401330321 ) ) ;
#51268=CARTESIAN_POINT ( 'NONE',  ( -1.069553805774277722, 0.2952755905511811885, 0.1292274648535926551 ) ) ;
#51269=CARTESIAN_POINT ( 'NONE',  ( -1.443569553805773564, 0.2306618581243847221, -0.2411417322834647770 ) ) ;
#51272=CARTESIAN_POINT ( 'NONE',  ( 0.9842519685039378130, -0.6692913385826771977, 8.415575281601705876E-17 ) ) ;
#51273=CARTESIAN_POINT ( 'NONE',  ( -0.1246719160104980823, -0.6692913385826773087, -0.1292274648535924053 ) ) ;
#51274=CARTESIAN_POINT ( 'NONE',  ( -0.3260583142159755865, -3.773335473449285555E-15, -0.3954974714151476278 ) ) ;
#51276=CARTESIAN_POINT ( 'NONE',  ( 1.010498687664042716, -0.004921259842519870586, -0.3153832671262229437 ) ) ;
#51280=ORIENTED_EDGE ( 'NONE', *, *, #81557, .T. ) ;
#51281=CARTESIAN_POINT ( 'NONE',  ( -0.1902887139107604098, -0.6692913385826771977, 0.1292274648535927661 ) ) ;
#51282=CARTESIAN_POINT ( 'NONE',  ( -0.9317585301837263412, 0.05413385826771666132, 0.4176697321401328100 ) ) ;
#51283=CARTESIAN_POINT ( 'NONE',  ( -1.391076115485563314, -0.6046776061558809534, -0.2411417322834644161 ) ) ;
#51284=CARTESIAN_POINT ( 'NONE',  ( 0.5446194225721792126, -0.3162353388693405765, 0.4822834645669290543 ) ) ;
#51285=CARTESIAN_POINT ( 'NONE',  ( -1.541994750656167090, -0.5511811023622048555, -0.09757992244046775898 ) ) ;
#51286=CARTESIAN_POINT ( 'NONE',  ( 1.299212598425197429, 0.2952755905511811885, 0.000000000000000000 ) ) ;
#51287=CARTESIAN_POINT ( 'NONE',  ( -0.6167979002624665030, -0.4281496062992127816, -0.4176697321401328100 ) ) ;
#51288=CARTESIAN_POINT ( 'NONE',  ( 0.5249343832021003964, 0.2306618581243847221, -0.2411417322834647770 ) ) ;
#51289=CARTESIAN_POINT ( 'NONE',  ( 1.469816272965879911, 0.2306618581243847221, -0.2411417322834647770 ) ) ;
#51290=CARTESIAN_POINT ( 'NONE',  ( 1.318897637795276356, 0.1660481256975883668, -0.3530559997133364547 ) ) ;
#51291=CARTESIAN_POINT ( 'NONE',  ( 1.404199475065617708, 0.05413385826771626580, -0.4176697321401330321 ) ) ;
#51292=CARTESIAN_POINT ( 'NONE',  ( -0.1640419947506555343, -0.3162353388693405765, 0.4822834645669290543 ) ) ;
#51294=CARTESIAN_POINT ( 'NONE',  ( 0.4396325459317593221, 0.1771653543307087075, -0.09757992244046823083 ) ) ;
#51298=CARTESIAN_POINT ( 'NONE',  ( -0.3280839895013117347, -0.3690944881889763329, 0.3153832671262228327 ) ) ;
#51300=CARTESIAN_POINT ( 'NONE',  ( 0.1181102362204730916, -0.6692913385826771977, 8.415575281601705876E-17 ) ) ;
#51301=CARTESIAN_POINT ( 'NONE',  ( 0.08530183727034192087, -0.3162353388693409650, -0.4822834645669289433 ) ) ;
#51303=CARTESIAN_POINT ( 'NONE',  ( -0.7152230971128602510, -0.05778040916215560624, -0.4822834645669293319 ) ) ;
#51305=CARTESIAN_POINT ( 'NONE',  ( -1.181102362204723644, -0.1870078740157479769, 0.4822834645669291653 ) ) ;
#51306=CARTESIAN_POINT ( 'NONE',  ( 1.436417322834644184, 2.401574803149606474, 0.3149606299212598381 ) ) ;
#51307=CARTESIAN_POINT ( 'NONE',  ( 0.9317585301837276734, -0.3690944881889763329, 0.3153832671262228327 ) ) ;
#51308=CARTESIAN_POINT ( 'NONE',  ( 0.5446194225721792126, -0.3162353388693405765, 0.4822834645669290543 ) ) ;
#51309=CARTESIAN_POINT ( 'NONE',  ( 0.8530183727034128527, -0.4281496062992124485, 0.4176697321401328655 ) ) ;
#51311=CARTESIAN_POINT ( 'NONE',  ( -1.266404199475064773, -0.3162353388693405765, 0.4822834645669290543 ) ) ;
#51314=CARTESIAN_POINT ( 'NONE',  ( -0.07217847769028813698, -0.3162353388693409650, -0.4822834645669289433 ) ) ;
#51317=CARTESIAN_POINT ( 'NONE',  ( -1.108923884514435132, -0.08942795157528024563, -0.3641732283464568787 ) ) ;
#51318=CARTESIAN_POINT ( 'NONE',  ( 1.345144356955381593, -0.3162353388693409650, -0.4822834645669289433 ) ) ;
#51319=CARTESIAN_POINT ( 'NONE',  ( 1.266404199475066328, -0.3162353388693409650, -0.4822834645669289433 ) ) ;
#51320=CARTESIAN_POINT ( 'NONE',  ( 0.2624671916010504757, 0.1283753931104748280, 0.1820866141732283561 ) ) ;
#51321=CARTESIAN_POINT ( 'NONE',  ( 0.9645669291338588858, 0.1660481256975885056, 0.3530559997133364547 ) ) ;
#51323=CARTESIAN_POINT ( 'NONE',  ( 0.4593175853018380828, -0.004921259842519870586, -0.3153832671262229437 ) ) ;
#51324=CARTESIAN_POINT ( 'NONE',  ( 0.3805774278215230400, 0.05413385826771626580, -0.4176697321401330321 ) ) ;
#51326=CARTESIAN_POINT ( 'NONE',  ( -1.345144356955379816, -0.05778040916215560624, -0.4822834645669293319 ) ) ;
#51327=CARTESIAN_POINT ( 'NONE',  ( 0.4921259842519691285, 0.07958543189024085140, 0.2665933059059887866 ) ) ;
#51329=CARTESIAN_POINT ( 'NONE',  ( -0.3149606299212590610, -0.1870078740157479769, 0.4822834645669291653 ) ) ;
#51330=CARTESIAN_POINT ( 'NONE',  ( -0.4133858267716528645, -0.4536011799217367080, 0.2665933059059888421 ) ) ;
#51332=CARTESIAN_POINT ( 'NONE',  ( -0.4002624671916004129, -0.05778040916215560624, -0.4822834645669293319 ) ) ;
#51333=CARTESIAN_POINT ( 'NONE',  ( 0.4461942257217855201, -0.5023911411419708095, 0.1820866141732285504 ) ) ;
#51335=CARTESIAN_POINT ( 'NONE',  ( -0.05905511811023545637, 0.1660481256975885056, 0.3530559997133364547 ) ) ;
#51337=CARTESIAN_POINT ( 'NONE',  ( 1.272965879265092637, -0.3690944881889765550, -0.3153832671262227771 ) ) ;
#51338=CARTESIAN_POINT ( 'NONE',  ( 0.1968503937007881344, 0.2952755905511811885, 0.000000000000000000 ) ) ;
#51339=CARTESIAN_POINT ( 'NONE',  ( -0.8792650918635160906, -0.004921259842519870586, -0.3153832671262229437 ) ) ;
#51340=CARTESIAN_POINT ( 'NONE',  ( -0.8923884514435688198, 0.1283753931104746893, -0.1820866141732285504 ) ) ;
#51341=CARTESIAN_POINT ( 'NONE',  ( -0.6233595800524928121, -0.3162353388693409650, -0.4822834645669289433 ) ) ;
#51342=CARTESIAN_POINT ( 'NONE',  ( -0.05249343832020938322, -0.6046776061558809534, -0.2411417322834644161 ) ) ;
#51343=CARTESIAN_POINT ( 'NONE',  ( 0.7283464566929143125, 0.07958543189024085140, 0.2665933059059887866 ) ) ;
#51345=CARTESIAN_POINT ( 'NONE',  ( 1.338582677165355062, -0.1870078740157480601, -0.3641732283464567677 ) ) ;
#51347=CARTESIAN_POINT ( 'NONE',  ( 0.8989501312335964611, 0.2952755905511811885, 0.1292274648535926551 ) ) ;
#51349=CARTESIAN_POINT ( 'NONE',  ( -0.4658792650918627265, -0.05778040916215522460, 0.4822834645669289988 ) ) ;
#51351=CARTESIAN_POINT ( 'NONE',  ( 1.614173228346457378, 0.1771653543307087630, 0.000000000000000000 ) ) ;
#51352=CARTESIAN_POINT ( 'NONE',  ( 0.7939632545931766261, -0.3162353388693409650, -0.4822834645669289433 ) ) ;
#51353=CARTESIAN_POINT ( 'NONE',  ( -0.03937007874015669567, 0.2952755905511811885, 0.000000000000000000 ) ) ;
#51355=CARTESIAN_POINT ( 'NONE',  ( 0.4330708661417329575, 0.1771653543307087630, 0.000000000000000000 ) ) ;
#51356=CARTESIAN_POINT ( 'NONE',  ( 0.5774278215223104249, 0.2306618581243848609, 0.2411417322834645549 ) ) ;
#51357=CARTESIAN_POINT ( 'NONE',  ( -0.4068241469816267775, -0.004921259842519870586, -0.3153832671262229437 ) ) ;
#51358=CARTESIAN_POINT ( 'NONE',  ( -0.9186351706036736120, -0.6046776061558809534, -0.2411417322834644161 ) ) ;
#51360=CARTESIAN_POINT ( 'NONE',  ( 0.1049868766404206816, -0.6046776061558809534, -0.2411417322834644161 ) ) ;
#51361=CARTESIAN_POINT ( 'NONE',  ( -0.7939632545931750718, -0.05778040916215560624, -0.4822834645669293319 ) ) ;
#51362=CARTESIAN_POINT ( 'NONE',  ( -0.7545931758530177724, 0.1771653543307087630, 0.09757992244046791164 ) ) ;
#51363=CARTESIAN_POINT ( 'NONE',  ( 0.4593175853018379162, -0.4281496062992124485, 0.4176697321401328655 ) ) ;
#51364=CARTESIAN_POINT ( 'NONE',  ( -1.233595800524933894, 0.2306618581243848609, 0.2411417322834645549 ) ) ;
#51365=CARTESIAN_POINT ( 'NONE',  ( -0.4593175853018364174, -0.4281496062992127816, -0.4176697321401328100 ) ) ;
#51366=CARTESIAN_POINT ( 'NONE',  ( 1.154855643044620184, 0.1539470093639521697, -0.1968503937007875793 ) ) ;
#51368=CARTESIAN_POINT ( 'NONE',  ( 1.384514435695538337, -0.6692913385826771977, 0.1292274648535927661 ) ) ;
#51369=CARTESIAN_POINT ( 'NONE',  ( 1.482939632545932307, -0.4281496062992124485, 0.4176697321401328655 ) ) ;
#51371=CARTESIAN_POINT ( 'NONE',  ( -1.515748031496062076, -0.5400638737290844871, 0.3530559997133364547 ) ) ;
#51372=CARTESIAN_POINT ( 'NONE',  ( -0.8923884514435688198, 0.2306618581243847221, -0.2411417322834647770 ) ) ;
#51376=CARTESIAN_POINT ( 'NONE',  ( 0.03937007874015833325, -0.5511811023622047445, 6.969142054262312111E-17 ) ) ;
#51379=CARTESIAN_POINT ( 'NONE',  ( 0.2624671916010504757, -0.6046776061558809534, -0.2411417322834644161 ) ) ;
#51382=CARTESIAN_POINT ( 'NONE',  ( -0.3149606299212590610, -0.1870078740157480601, -0.3641732283464567677 ) ) ;
#51383=CARTESIAN_POINT ( 'NONE',  ( 0.3265464962716623232, 0.02791078216816386681, 0.4328096321851896966 ) ) ;
#51384=CARTESIAN_POINT ( 'NONE',  ( 0.5708661417322842269, 0.1660481256975885056, 0.3530559997133364547 ) ) ;
#51385=CARTESIAN_POINT ( 'NONE',  ( 0.7217847769028878924, -0.3690944881889765550, -0.3153832671262227771 ) ) ;
#51386=CARTESIAN_POINT ( 'NONE',  ( 0.1115485564304470323, 0.2952755905511811885, 0.1292274648535926551 ) ) ;
#51388=CARTESIAN_POINT ( 'NONE',  ( -0.6167979002624665030, -0.4281496062992127816, -0.4176697321401328100 ) ) ;
#51389=CARTESIAN_POINT ( 'NONE',  ( -1.200787401574802349, 0.07958543189024071263, -0.2665933059059888421 ) ) ;
#51391=CARTESIAN_POINT ( 'NONE',  ( -0.5577427821522301654, -0.05778040916215560624, -0.4822834645669293319 ) ) ;
#51396=CARTESIAN_POINT ( 'NONE',  ( 0.4199475065616805614, 0.2306618581243848609, 0.2411417322834645549 ) ) ;
#51398=CARTESIAN_POINT ( 'NONE',  ( -0.5905511811023615998, 0.2952755905511811885, 0.000000000000000000 ) ) ;
#51399=CARTESIAN_POINT ( 'NONE',  ( 1.443569553805774897, 0.2306618581243848609, 0.2411417322834645549 ) ) ;
#51400=CARTESIAN_POINT ( 'NONE',  ( 1.095800524934383846, -0.3162353388693405765, 0.4822834645669290543 ) ) ;
#51401=CARTESIAN_POINT ( 'NONE',  ( 0.7677165354330716118, -0.5400638737290844871, 0.3530559997133364547 ) ) ;
#51403=EDGE_CURVE ( 'NONE', #19450, #9917, #28380, .T. ) ;
#51404=CARTESIAN_POINT ( 'NONE',  ( 0.1640419947506569498, -0.3162353388693409650, -0.4822834645669289433 ) ) ;
#51406=CARTESIAN_POINT ( 'NONE',  ( -1.167979002624671470, -0.4281496062992127816, -0.4176697321401328100 ) ) ;
#51407=CARTESIAN_POINT ( 'NONE',  ( -0.3543307086614165824, 0.2952755905511811885, 0.000000000000000000 ) ) ;
#51408=CARTESIAN_POINT ( 'NONE',  ( -0.1771653543307080136, 0.07958543189024071263, -0.2665933059059888421 ) ) ;
#51410=CARTESIAN_POINT ( 'NONE',  ( -0.1246719160104980823, 0.2952755905511811885, 0.1292274648535926551 ) ) ;
#51412=CARTESIAN_POINT ( 'NONE',  ( 0.9383202099737536495, -0.3162353388693405765, 0.4822834645669290543 ) ) ;
#51416=CARTESIAN_POINT ( 'NONE',  ( 0.1640419947506569498, -0.3162353388693409650, -0.4822834645669289433 ) ) ;
#51417=CARTESIAN_POINT ( 'NONE',  ( -0.1902887139107604098, -0.5511811023622046335, 0.09757992244046803654 ) ) ;
#51418=CARTESIAN_POINT ( 'NONE',  ( 1.614173228346457378, -0.5511811023622047445, 6.969142054262312111E-17 ) ) ;
#51422=CARTESIAN_POINT ( 'NONE',  ( 1.476377952755906442, -0.4536011799217367080, 0.2665933059059888421 ) ) ;
#51423=CARTESIAN_POINT ( 'NONE',  ( -1.627296587926508442, 0.2306618581243848609, 0.2411417322834645549 ) ) ;
#51425=CARTESIAN_POINT ( 'NONE',  ( 0.2427821522309716595, -0.3162353388693409650, -0.4822834645669289433 ) ) ;
#51426=CARTESIAN_POINT ( 'NONE',  ( -1.089238845144356427, -0.4281496062992127816, -0.4176697321401328100 ) ) ;
#51427=CARTESIAN_POINT ( 'NONE',  ( -1.056430446194224881, 0.2952755905511810774, -0.1292274648535930714 ) ) ;
#51428=CARTESIAN_POINT ( 'NONE',  ( 0.1312335958005255154, -0.6046776061558807314, 0.2411417322834647770 ) ) ;
#51430=CARTESIAN_POINT ( 'NONE',  ( -1.509186351706035767, -0.3690944881889763329, 0.3153832671262228327 ) ) ;
#51431=CARTESIAN_POINT ( 'NONE',  ( 1.017060367454068581, -0.05778040916215560624, -0.4822834645669293319 ) ) ;
#51432=CARTESIAN_POINT ( 'NONE',  ( 0.7939632545931766261, -0.2845877964562161244, -0.3641732283464567121 ) ) ;
#51433=CARTESIAN_POINT ( 'NONE',  ( 0.8202099737532814183, 0.2066929133858267931, 0.1054918080437490802 ) ) ;
#51434=CARTESIAN_POINT ( 'NONE',  ( 0.9842519685039378130, -0.5511811023622047445, 6.969142054262312111E-17 ) ) ;
#51435=CARTESIAN_POINT ( 'NONE',  ( -1.266404199475064773, -0.05778040916215560624, -0.4822834645669293319 ) ) ;
#51437=CARTESIAN_POINT ( 'NONE',  ( 1.030183727034121421, -0.05778040916215522460, 0.4822834645669289988 ) ) ;
#51439=CARTESIAN_POINT ( 'NONE',  ( 0.8267716535433078384, -0.6692913385826771977, 8.415575281601705876E-17 ) ) ;
#51440=LINE ( 'NONE', #17839, #81575 ) ;
#51441=CARTESIAN_POINT ( 'NONE',  ( -1.603475055217291612, 1.054977578535736926, 0.04573490813648253134 ) ) ;
#51442=CARTESIAN_POINT ( 'NONE',  ( -0.03937007874015669567, 0.2952755905511811885, 0.000000000000000000 ) ) ;
#51443=CARTESIAN_POINT ( 'NONE',  ( 0.4461942257217855201, -0.5023911411419708095, 0.1820866141732285504 ) ) ;
#51444=CARTESIAN_POINT ( 'NONE',  ( 0.8136482939632553313, -0.6046776061558809534, -0.2411417322834644161 ) ) ;
#51445=CARTESIAN_POINT ( 'NONE',  ( 1.633858267716535639, -0.4536011799217367080, 0.2665933059059888421 ) ) ;
#51446=CARTESIAN_POINT ( 'NONE',  ( -0.7611548556430438595, 0.1283753931104748280, 0.1820866141732283561 ) ) ;
#51447=CARTESIAN_POINT ( 'NONE',  ( -0.8005249343832013809, -0.4281496062992124485, 0.4176697321401328655 ) ) ;
#51449=CARTESIAN_POINT ( 'NONE',  ( 1.541994750656168645, 0.2952755905511810774, -0.1292274648535930714 ) ) ;
#51450=CARTESIAN_POINT ( 'NONE',  ( -1.161417322834644716, -0.5400638737290845981, -0.3530559997133363437 ) ) ;
#51451=CARTESIAN_POINT ( 'NONE',  ( 1.128608923884515169, -0.6046776061558809534, -0.2411417322834644161 ) ) ;
#51452=CARTESIAN_POINT ( 'NONE',  ( -1.154855643044618851, 0.1283753931104748280, 0.1820866141732283561 ) ) ;
#51454=CARTESIAN_POINT ( 'NONE',  ( 1.043307086614173818, -0.5400638737290845981, -0.3530559997133363437 ) ) ;
#51456=CARTESIAN_POINT ( 'NONE',  ( -1.719160104986876103, 0.05413385826771666132, 0.4176697321401328100 ) ) ;
#51457=CARTESIAN_POINT ( 'NONE',  ( -1.423884514435694859, -0.08942795157528024563, -0.3641732283464568787 ) ) ;
#51458=CARTESIAN_POINT ( 'NONE',  ( -1.233595800524933894, 0.1283753931104748280, 0.1820866141732283561 ) ) ;
#51460=CARTESIAN_POINT ( 'NONE',  ( 1.476377952755906442, -0.4536011799217367080, 0.2665933059059888421 ) ) ;
#51461=CARTESIAN_POINT ( 'NONE',  ( -0.2427821522309703550, -0.3162353388693405765, 0.4822834645669290543 ) ) ;
#51462=CARTESIAN_POINT ( 'NONE',  ( -0.2690288713910754526, -0.5511811023622046335, 0.09757992244046803654 ) ) ;
#51463=CARTESIAN_POINT ( 'NONE',  ( -1.496062992125983815, -0.1870078740157480601, -0.3641732283464567677 ) ) ;
#51464=CARTESIAN_POINT ( 'NONE',  ( 0.8923884514435701520, -0.5023911411419708095, -0.1820866141732282451 ) ) ;
#51465=CARTESIAN_POINT ( 'NONE',  ( 0.3740157480314966754, -0.5400638737290844871, 0.3530559997133364547 ) ) ;
#51466=CARTESIAN_POINT ( 'NONE',  ( 1.351706036745407458, -0.4281496062992127816, -0.4176697321401328100 ) ) ;
#51467=CARTESIAN_POINT ( 'NONE',  ( 0.6167979002624679463, 0.05413385826771626580, -0.4176697321401330321 ) ) ;
#51468=CARTESIAN_POINT ( 'NONE',  ( 0.6758530183727039509, 0.1771653543307087075, -0.09757992244046823083 ) ) ;
#51469=CARTESIAN_POINT ( 'NONE',  ( -1.594488188976377119, 0.1660481256975883668, -0.3530559997133364547 ) ) ;
#51470=CARTESIAN_POINT ( 'NONE',  ( -1.122047244094487306, 0.1660481256975883668, -0.3530559997133364547 ) ) ;
#51471=CARTESIAN_POINT ( 'NONE',  ( -0.3805774278215216522, -0.4281496062992127816, -0.4176697321401328100 ) ) ;
#51474=CARTESIAN_POINT ( 'NONE',  ( -0.05249343832020938322, -0.6046776061558809534, -0.2411417322834644161 ) ) ;
#51475=CARTESIAN_POINT ( 'NONE',  ( 1.227034120734908917, -0.5511811023622046335, 0.09757992244046803654 ) ) ;
#51476=CARTESIAN_POINT ( 'NONE',  ( -0.5577427821522301654, -0.3162353388693405765, 0.4822834645669290543 ) ) ;
#51477=CARTESIAN_POINT ( 'NONE',  ( 0.4199475065616803948, -0.6046776061558809534, -0.2411417322834644161 ) ) ;
#51483=CARTESIAN_POINT ( 'NONE',  ( -0.8595800524934373854, -0.2845877964562161244, -0.3641732283464567121 ) ) ;
#51484=CARTESIAN_POINT ( 'NONE',  ( -1.292650918635170010, -0.6692913385826771977, 0.1292274648535927661 ) ) ;
#51486=CARTESIAN_POINT ( 'NONE',  ( 0.3149606299212606708, -0.1870078740157480879, -0.4822834645669291653 ) ) ;
#51487=CARTESIAN_POINT ( 'NONE',  ( 1.391076115485564868, -0.6046776061558807314, 0.2411417322834647770 ) ) ;
#51488=CARTESIAN_POINT ( 'NONE',  ( 0.7742782152230978099, -0.4281496062992124485, 0.4176697321401328655 ) ) ;
#51493=CARTESIAN_POINT ( 'NONE',  ( 0.3412073490813655186, 0.2306618581243848609, 0.2411417322834645549 ) ) ;
#51494=CARTESIAN_POINT ( 'NONE',  ( 0.3215223097112867578, -0.05778040916215522460, 0.4822834645669289988 ) ) ;
#51495=CARTESIAN_POINT ( 'NONE',  ( 0.9580052493438326877, -0.004921259842519576551, 0.3153832671262227771 ) ) ;
#51496=CARTESIAN_POINT ( 'NONE',  ( 1.286089238845145033, -0.6046776061558809534, -0.2411417322834644161 ) ) ;
#51498=CARTESIAN_POINT ( 'NONE',  ( 0.4396325459317590445, -0.6692913385826771977, 0.1292274648535927661 ) ) ;
#51499=CARTESIAN_POINT ( 'NONE',  ( 1.187664041994751285, -0.05778040916215522460, 0.4822834645669289988 ) ) ;
#51500=CARTESIAN_POINT ( 'NONE',  ( 0.4002624671916016896, -0.05778040916215522460, 0.4822834645669289988 ) ) ;
#51502=CARTESIAN_POINT ( 'NONE',  ( 1.049868766404200349, 0.1283753931104748280, 0.1820866141732283561 ) ) ;
#51503=CARTESIAN_POINT ( 'NONE',  ( -1.069553805774277722, 0.2952755905511811885, 0.1292274648535926551 ) ) ;
#51504=CARTESIAN_POINT ( 'NONE',  ( -0.8595800524934373854, -0.3162353388693409650, -0.4822834645669289433 ) ) ;
#51505=CARTESIAN_POINT ( 'NONE',  ( 1.207349081364829990, -0.6046776061558809534, -0.2411417322834644161 ) ) ;
#51509=VERTEX_POINT ( 'NONE', #30670 ) ;
#51512=CARTESIAN_POINT ( 'NONE',  ( 1.371391076115485941, 0.2952755905511811885, 0.1292274648535926551 ) ) ;
#51513=CARTESIAN_POINT ( 'NONE',  ( 0.8661417322834652488, -0.1870078740157480601, -0.3641732283464567677 ) ) ;
#51515=CARTESIAN_POINT ( 'NONE',  ( 1.200787401574803681, 0.07958543189024085140, 0.2665933059059887866 ) ) ;
#51521=CARTESIAN_POINT ( 'NONE',  ( -1.030183727034119867, -0.2845877964562159024, 0.3641732283464567677 ) ) ;
#51522=CARTESIAN_POINT ( 'NONE',  ( -1.548556430446193399, 0.1283753931104748280, 0.1820866141732283561 ) ) ;
#51523=CARTESIAN_POINT ( 'NONE',  ( -1.489501312335957062, -0.05778040916215522460, 0.4822834645669289988 ) ) ;
#51524=CARTESIAN_POINT ( 'NONE',  ( -0.09186351706036689768, 0.05413385826771626580, -0.4176697321401330321 ) ) ;
#51525=CARTESIAN_POINT ( 'NONE',  ( 1.555118110236221041, -0.5400638737290844871, 0.3530559997133364547 ) ) ;
#51526=ORIENTED_EDGE ( 'NONE', *, *, #69760, .T. ) ;
#51531=CARTESIAN_POINT ( 'NONE',  ( -0.3030275874994723395, -1.146068349578384814E-15, 0.3627985898453523483 ) ) ;
#51532=CARTESIAN_POINT ( 'NONE',  ( -0.7874015748031489847, -0.1870078740157480601, -0.3641732283464567677 ) ) ;
#51533=CARTESIAN_POINT ( 'NONE',  ( -1.240157480314959759, -0.5400638737290845981, -0.3530559997133363437 ) ) ;
#51534=CARTESIAN_POINT ( 'NONE',  ( 0.5839895013123367340, 0.2952755905511811885, 0.1292274648535926551 ) ) ;
#51537=CARTESIAN_POINT ( 'NONE',  ( 0.6955380577427828781, 0.009842519685039144428, -0.3409548833797004797 ) ) ;
#51538=CARTESIAN_POINT ( 'NONE',  ( 1.141732283464567788, -0.6692913385826771977, 8.415575281601705876E-17 ) ) ;
#51539=CARTESIAN_POINT ( 'NONE',  ( -1.653543307086613234, -0.1870078740157480879, -0.4822834645669291653 ) ) ;
#51541=CARTESIAN_POINT ( 'NONE',  ( -0.5905511811023615998, 0.1771653543307087630, 0.000000000000000000 ) ) ;
#51542=CARTESIAN_POINT ( 'NONE',  ( -1.141732283464566011, 0.1771653543307087630, 0.000000000000000000 ) ) ;
#51544=CARTESIAN_POINT ( 'NONE',  ( -0.7152230971128602510, -0.2845877964562159024, 0.3641732283464567677 ) ) ;
#51545=CARTESIAN_POINT ( 'NONE',  ( 0.1246719160104994284, -0.5511811023622046335, 0.09757992244046803654 ) ) ;
#51546=CARTESIAN_POINT ( 'NONE',  ( 0.1837270341207354329, 0.2306618581243848609, 0.2411417322834645549 ) ) ;
#51547=CARTESIAN_POINT ( 'NONE',  ( -1.122047244094487306, 0.07958543189024071263, -0.2665933059059888421 ) ) ;
#51549=CARTESIAN_POINT ( 'NONE',  ( 1.023622047244095112, -0.1870078740157480879, -0.4822834645669291653 ) ) ;
#51551=CARTESIAN_POINT ( 'NONE',  ( -1.391076115485563314, -0.6046776061558809534, -0.2411417322834644161 ) ) ;
#51553=CARTESIAN_POINT ( 'NONE',  ( -0.3346456692913377662, -0.5400638737290844871, 0.3530559997133364547 ) ) ;
#51554=CARTESIAN_POINT ( 'NONE',  ( -0.9645669291338575535, 0.1660481256975883668, -0.3530559997133364547 ) ) ;
#51555=CARTESIAN_POINT ( 'NONE',  ( 0.9776902887139113929, -0.5511811023622048555, -0.09757992244046775898 ) ) ;
#51556=CARTESIAN_POINT ( 'NONE',  ( -0.3477690288713905509, -0.5511811023622046335, 0.09757992244046803654 ) ) ;
#51557=CARTESIAN_POINT ( 'NONE',  ( -0.5446194225721777693, -0.3162353388693409650, -0.4822834645669289433 ) ) ;
#51558=CARTESIAN_POINT ( 'NONE',  ( -1.371391076115484609, -0.6692913385826771977, 0.1292274648535927661 ) ) ;
#51559=CARTESIAN_POINT ( 'NONE',  ( -0.4061203303035118561, -2.613618158232546091E-15, -0.3464511005275220379 ) ) ;
#51560=CARTESIAN_POINT ( 'NONE',  ( 1.082677165354331228, 0.07958543189024071263, -0.2665933059059888421 ) ) ;
#51561=VECTOR ( 'NONE', #7019, 39.37007874015748854 ) ;
#51562=CARTESIAN_POINT ( 'NONE',  ( -0.08530183727034056085, -0.3162353388693405765, 0.4822834645669290543 ) ) ;
#51563=CARTESIAN_POINT ( 'NONE',  ( -1.594488188976377563, -0.5400638737290844871, 0.3530559997133364547 ) ) ;
#51566=CARTESIAN_POINT ( 'NONE',  ( -1.017060367454067249, -0.08942795157527998196, 0.3641732283464567121 ) ) ;
#51567=CARTESIAN_POINT ( 'NONE',  ( 0.7020997375328090762, -0.05778040916215560624, -0.4822834645669293319 ) ) ;
#51568=CARTESIAN_POINT ( 'NONE',  ( -0.9842519685039365918, -0.5511811023622047445, 6.969142054262312111E-17 ) ) ;
#51570=CARTESIAN_POINT ( 'NONE',  ( -1.089238845144356427, 0.05413385826771666132, 0.4176697321401328100 ) ) ;
#51571=CARTESIAN_POINT ( 'NONE',  ( 0.6889763779527566800, -0.5400638737290844871, 0.3530559997133364547 ) ) ;
#51572=CARTESIAN_POINT ( 'NONE',  ( 0.5577427821522316087, -0.05778040916215522460, 0.4822834645669289988 ) ) ;
#51574=CARTESIAN_POINT ( 'NONE',  ( -1.469816272965878357, -0.5023911411419708095, -0.1820866141732282451 ) ) ;
#51580=CARTESIAN_POINT ( 'NONE',  ( 1.023622047244095334, -0.1870078740157479769, 0.3641732283464567677 ) ) ;
#51581=CARTESIAN_POINT ( 'NONE',  ( 0.2755905511811031494, -0.5511811023622047445, 6.969142054262312111E-17 ) ) ;
#51582=CARTESIAN_POINT ( 'NONE',  ( 0.1115485564304467270, -0.6692913385826773087, -0.1292274648535924053 ) ) ;
#51583=CARTESIAN_POINT ( 'NONE',  ( 1.404199475065617264, -0.4281496062992124485, 0.4176697321401328655 ) ) ;
#51585=CARTESIAN_POINT ( 'NONE',  ( 0.4658792650918641698, -0.08942795157528024563, -0.3641732283464568787 ) ) ;
#51587=CARTESIAN_POINT ( 'NONE',  ( -0.6955380577427815458, 0.05413385826771666132, 0.4176697321401328100 ) ) ;
#51588=CARTESIAN_POINT ( 'NONE',  ( -1.410761154855641575, -0.3162353388693409650, -0.4822834645669289433 ) ) ;
#51589=CARTESIAN_POINT ( 'NONE',  ( 0.7545931758530189937, 0.2952755905511810774, -0.1292274648535930714 ) ) ;
#51591=CARTESIAN_POINT ( 'NONE',  ( -0.7186703366786194591, -2.567464376874931580E-15, -0.4445507791589072832 ) ) ;
#51594=CARTESIAN_POINT ( 'NONE',  ( -1.266404199475064773, -0.3162353388693405765, 0.4822834645669290543 ) ) ;
#51595=CARTESIAN_POINT ( 'NONE',  ( -0.4921259842519677963, 0.1660481256975883668, -0.3530559997133364547 ) ) ;
#51596=CARTESIAN_POINT ( 'NONE',  ( -0.5839895013123351797, -0.5511811023622046335, 0.09757992244046803654 ) ) ;
#51597=CARTESIAN_POINT ( 'NONE',  ( -0.8070866141732276899, 0.1660481256975883668, -0.3530559997133364547 ) ) ;
#51600=CARTESIAN_POINT ( 'NONE',  ( 1.627296587926509996, -0.6046776061558807314, 0.2411417322834647770 ) ) ;
#51601=CARTESIAN_POINT ( 'NONE',  ( -1.207349081364828880, 0.2306618581243847221, -0.2411417322834647770 ) ) ;
#51602=CARTESIAN_POINT ( 'NONE',  ( 0.2296587926509192634, -0.05778040916215560624, -0.4822834645669293319 ) ) ;
#51603=CARTESIAN_POINT ( 'NONE',  ( -0.7742782152230962556, -0.4281496062992127816, -0.4176697321401328100 ) ) ;
#51605=CARTESIAN_POINT ( 'NONE',  ( -0.9645669291338575535, 0.07958543189024071263, -0.2665933059059888421 ) ) ;
#51608=ORIENTED_EDGE ( 'NONE', *, *, #41805, .T. ) ;
#51610=CARTESIAN_POINT ( 'NONE',  ( -1.266404199475064773, -0.3162353388693405765, 0.4822834645669290543 ) ) ;
#51611=CARTESIAN_POINT ( 'NONE',  ( -0.7808398950131222316, -0.3162353388693409650, -0.4822834645669289433 ) ) ;
#51613=CARTESIAN_POINT ( 'NONE',  ( -0.9383202099737524282, -0.05778040916215522460, 0.4822834645669289988 ) ) ;
#51614=CARTESIAN_POINT ( 'NONE',  ( -1.292650918635170010, -0.6692913385826771977, 0.1292274648535927661 ) ) ;
#51615=CARTESIAN_POINT ( 'NONE',  ( -0.3817677560323433084, -4.005968212718139582E-15, 0.3627989612356165572 ) ) ;
#51616=CARTESIAN_POINT ( 'NONE',  ( -0.8545558659330622087, 0.02791078216816064370, 0.4328096321851915285 ) ) ;
#51617=CARTESIAN_POINT ( 'NONE',  ( 0.6102362204724416372, 0.07958543189024071263, -0.2665933059059888421 ) ) ;
#51620=CARTESIAN_POINT ( 'NONE',  ( -0.3543307086614165824, -0.5511811023622047445, 6.969142054262312111E-17 ) ) ;
#51621=CARTESIAN_POINT ( 'NONE',  ( -0.6758530183727028406, 0.2952755905511811885, 0.1292274648535926551 ) ) ;
#51622=CARTESIAN_POINT ( 'NONE',  ( 1.463254593175853824, 0.2952755905511810774, -0.1292274648535930714 ) ) ;
#51623=CARTESIAN_POINT ( 'NONE',  ( -0.6758530183727028406, 0.2952755905511811885, 0.1292274648535926551 ) ) ;
#51624=EDGE_CURVE ( 'NONE', #44566, #18339, #75747, .T. ) ;
#51625=ORIENTED_EDGE ( 'NONE', *, *, #58543, .T. ) ;
#51628=CARTESIAN_POINT ( 'NONE',  ( -0.8727034120734901146, -0.3162353388693405765, 0.4822834645669290543 ) ) ;
#51629=CARTESIAN_POINT ( 'NONE',  ( 1.384514435695538337, -0.6692913385826771977, 0.1292274648535927661 ) ) ;
#51630=CARTESIAN_POINT ( 'NONE',  ( -1.233595800524933894, 0.1283753931104748280, 0.1820866141732283561 ) ) ;
#51631=CARTESIAN_POINT ( 'NONE',  ( -1.371391076115484831, 0.2952755905511810774, -0.1292274648535930714 ) ) ;
#51636=CARTESIAN_POINT ( 'NONE',  ( -0.03937007874015669567, 0.2952755905511811885, 0.000000000000000000 ) ) ;
#51637=CARTESIAN_POINT ( 'NONE',  ( -1.181102362204723644, -0.1870078740157479769, 0.3641732283464567677 ) ) ;
#51638=CARTESIAN_POINT ( 'NONE',  ( -0.8005249343832013809, -0.4281496062992124485, 0.4176697321401328655 ) ) ;
#51640=CARTESIAN_POINT ( 'NONE',  ( -1.213910761154854745, 0.2952755905511810774, -0.1292274648535930714 ) ) ;
#51641=CARTESIAN_POINT ( 'NONE',  ( -0.8005249343832013809, -0.4281496062992124485, 0.4176697321401328655 ) ) ;
#51642=CARTESIAN_POINT ( 'NONE',  ( -0.03937007874015669567, -0.6692913385826771977, 8.415575281601705876E-17 ) ) ;
#51645=CARTESIAN_POINT ( 'NONE',  ( 0.7152230971128614723, -0.2845877964562161244, -0.3641732283464567121 ) ) ;
#51646=CARTESIAN_POINT ( 'NONE',  ( -0.7874015748031489847, -0.1870078740157479769, 0.3641732283464567677 ) ) ;
#51648=CARTESIAN_POINT ( 'NONE',  ( 0.8530183727034128527, -0.3690944881889763329, 0.3153832671262228327 ) ) ;
#51649=CARTESIAN_POINT ( 'NONE',  ( 1.502624671916010790, -0.2845877964562161244, -0.3641732283464567121 ) ) ;
#51650=CARTESIAN_POINT ( 'NONE',  ( 1.187664041994751285, -0.3162353388693409650, -0.4822834645669289433 ) ) ;
#51651=CARTESIAN_POINT ( 'NONE',  ( -0.07217847769028787330, -0.08942795157527998196, 0.3641732283464567121 ) ) ;
#51653=CARTESIAN_POINT ( 'NONE',  ( -1.049868766404198794, -0.6046776061558807314, 0.2411417322834647770 ) ) ;
#51654=CARTESIAN_POINT ( 'NONE',  ( 1.036745406824147508, -0.4281496062992127816, -0.4176697321401328100 ) ) ;
#51657=CARTESIAN_POINT ( 'NONE',  ( -0.4199475065616791736, -0.5023911411419708095, 0.1820866141732285504 ) ) ;
#51658=CARTESIAN_POINT ( 'NONE',  ( -0.4037097067573596210, -2.567464376874931580E-15, -0.4445507791589072832 ) ) ;
#51659=CARTESIAN_POINT ( 'NONE',  ( 0.4790026246719168435, -0.3162353388693409650, -0.4822834645669289433 ) ) ;
#51661=CARTESIAN_POINT ( 'NONE',  ( 0.8070866141732288002, 0.07958543189024085140, 0.2665933059059887866 ) ) ;
#51662=CARTESIAN_POINT ( 'NONE',  ( 0.006561679790026889343, -0.08942795157527998196, 0.3641732283464567121 ) ) ;
#51663=CARTESIAN_POINT ( 'NONE',  ( -0.08530183727034056085, -0.3162353388693405765, 0.4822834645669290543 ) ) ;
#51664=CARTESIAN_POINT ( 'NONE',  ( -1.167979002624671470, -0.4281496062992127816, -0.4176697321401328100 ) ) ;
#51665=CARTESIAN_POINT ( 'NONE',  ( -0.7874015748031489847, -0.1870078740157480601, -0.3641732283464567677 ) ) ;
#51667=B_SPLINE_CURVE_WITH_KNOTS ( 'NONE', 1,
 ( #42605, #16966 ),
 .UNSPECIFIED., .F., .F.,
 ( 2, 2 ),
 ( 0.0007499999999999989314, 0.002999999999999998328 ),
 .UNSPECIFIED. ) ;
#51668=CARTESIAN_POINT ( 'NONE',  ( -1.010498687664041384, 0.05413385826771666132, 0.4176697321401328100 ) ) ;
#51671=CARTESIAN_POINT ( 'NONE',  ( 0.1968503937007881344, 0.1771653543307087630, 0.000000000000000000 ) ) ;
#51672=CARTESIAN_POINT ( 'NONE',  ( -0.7283464566929126471, -0.5400638737290844871, 0.3530559997133364547 ) ) ;
#51673=CARTESIAN_POINT ( 'NONE',  ( -1.148293963254592542, 0.2952755905511811885, 0.1292274648535926551 ) ) ;
#51674=CARTESIAN_POINT ( 'NONE',  ( -1.102362204724408601, -0.1870078740157480601, -0.3641732283464567677 ) ) ;
#51675=CARTESIAN_POINT ( 'NONE',  ( 1.653543307086614789, -0.1870078740157479769, 0.4822834645669291653 ) ) ;
#51676=EDGE_CURVE ( 'NONE', #29291, #31839, #38137, .T. ) ;
#51677=CARTESIAN_POINT ( 'NONE',  ( -0.8989501312335946848, -0.5511811023622046335, 0.09757992244046803654 ) ) ;
#51678=CARTESIAN_POINT ( 'NONE',  ( -1.443569553805773564, -0.5023911411419708095, 0.1820866141732285504 ) ) ;
#51679=CARTESIAN_POINT ( 'NONE',  ( 1.443569553805774897, 0.2306618581243848609, 0.2411417322834645549 ) ) ;
#51684=CARTESIAN_POINT ( 'NONE',  ( -0.2258813529811895260, -1.094630224652485432E-15, 0.4281993546915541238 ) ) ;
#51685=CARTESIAN_POINT ( 'NONE',  ( -1.646981627296586703, -0.3162353388693409650, -0.4822834645669289433 ) ) ;
#51686=CARTESIAN_POINT ( 'NONE',  ( -1.384514435695537005, 0.2952755905511811885, 0.1292274648535926551 ) ) ;
#51687=CARTESIAN_POINT ( 'NONE',  ( 1.102362204724410155, -0.1870078740157479769, 0.4822834645669291653 ) ) ;
#51689=CARTESIAN_POINT ( 'NONE',  ( 1.660104986876641320, -0.08942795157527998196, 0.3641732283464567121 ) ) ;
#51690=CARTESIAN_POINT ( 'NONE',  ( 0.7020997375328090762, -0.3162353388693405765, 0.4822834645669290543 ) ) ;
#51691=CARTESIAN_POINT ( 'NONE',  ( -0.07217847769028787330, -0.05778040916215522460, 0.4822834645669289988 ) ) ;
#51692=CARTESIAN_POINT ( 'NONE',  ( 2.795275590551181466, 2.204724409448820310, 0.000000000000000000 ) ) ;
#51694=CARTESIAN_POINT ( 'NONE',  ( 0.7611548556430451917, -0.5023911411419708095, 0.1820866141732285504 ) ) ;
#51700=CARTESIAN_POINT ( 'NONE',  ( -0.09186351706036689768, 0.05413385826771626580, -0.4176697321401330321 ) ) ;
#51701=CARTESIAN_POINT ( 'NONE',  ( -1.502624671916009680, -0.3162353388693405765, 0.4822834645669290543 ) ) ;
#51702=CARTESIAN_POINT ( 'NONE',  ( 0.7480314960629927956, 0.2952755905511811885, 0.000000000000000000 ) ) ;
#51703=CARTESIAN_POINT ( 'NONE',  ( 1.332020997375329197, -0.3162353388693405765, 0.4822834645669290543 ) ) ;
#51704=CARTESIAN_POINT ( 'NONE',  ( 1.305774278215223960, 0.2952755905511810774, -0.1292274648535930714 ) ) ;
#51705=CARTESIAN_POINT ( 'NONE',  ( -0.6036745406824141069, -0.6046776061558809534, -0.2411417322834644161 ) ) ;
#51706=CARTESIAN_POINT ( 'NONE',  ( 0.06561679790026316017, 0.05413385826771626580, -0.4176697321401330321 ) ) ;
#51707=CARTESIAN_POINT ( 'NONE',  ( 1.423884514435696191, -0.05778040916215522460, 0.4822834645669289988 ) ) ;
#51708=CARTESIAN_POINT ( 'NONE',  ( 1.496062992125984703, -0.1870078740157480879, -0.4822834645669291653 ) ) ;
#51710=CARTESIAN_POINT ( 'NONE',  ( 1.194225721784777594, 0.05413385826771666132, 0.4176697321401328100 ) ) ;
#51711=CARTESIAN_POINT ( 'NONE',  ( -0.1706036745406816491, -0.4281496062992124485, 0.4176697321401328655 ) ) ;
#51713=CARTESIAN_POINT ( 'NONE',  ( 0.5708661417322842269, 0.07958543189024085140, 0.2665933059059887866 ) ) ;
#51717=CARTESIAN_POINT ( 'NONE',  ( -0.6036745406824141069, 0.1283753931104748280, 0.1820866141732283561 ) ) ;
#51719=CARTESIAN_POINT ( 'NONE',  ( 0.1246719160104994284, -0.6692913385826771977, 0.1292274648535927661 ) ) ;
#51720=CARTESIAN_POINT ( 'NONE',  ( -0.04593175853018302557, -0.6692913385826773087, -0.1292274648535924053 ) ) ;
#51721=CARTESIAN_POINT ( 'NONE',  ( -1.023622047244094002, -0.1870078740157480879, -0.4822834645669291653 ) ) ;
#51724=CARTESIAN_POINT ( 'NONE',  ( -1.286089238845143479, 0.2306618581243847221, -0.2411417322834647770 ) ) ;
#51726=CARTESIAN_POINT ( 'NONE',  ( 0.8530183727034126306, -0.004921259842519870586, -0.3153832671262229437 ) ) ;
#51727=CARTESIAN_POINT ( 'NONE',  ( 0.3215223097112867578, -0.3162353388693409650, -0.4822834645669289433 ) ) ;
#51728=CARTESIAN_POINT ( 'NONE',  ( 0.5577427821522316087, -0.05778040916215522460, 0.4822834645669289988 ) ) ;
#51730=LINE ( 'NONE', #1668, #11699 ) ;
#51733=CARTESIAN_POINT ( 'NONE',  ( -0.006561679790025524116, -0.3162353388693405765, 0.4822834645669290543 ) ) ;
#51735=ADVANCED_FACE ( 'NONE', ( #26234 ), #56990, .F. ) ;
#51737=CARTESIAN_POINT ( 'NONE',  ( -1.391076115485563314, -0.5023911411419708095, -0.1820866141732282451 ) ) ;
#51738=CARTESIAN_POINT ( 'NONE',  ( 1.404199475065617264, -0.4281496062992124485, 0.4176697321401328655 ) ) ;
#51739=CARTESIAN_POINT ( 'NONE',  ( 1.522309711286089939, 0.2306618581243848609, 0.2411417322834645549 ) ) ;
#51740=CARTESIAN_POINT ( 'NONE',  ( 0.3871391076115493490, -0.2845877964562159024, 0.3641732283464567677 ) ) ;
#51741=CARTESIAN_POINT ( 'NONE',  ( 0.6036745406824153282, -0.6046776061558807314, 0.2411417322834647770 ) ) ;
#51743=CARTESIAN_POINT ( 'NONE',  ( 0.5118110236220480003, -0.5511811023622047445, 6.969142054262312111E-17 ) ) ;
#51744=CARTESIAN_POINT ( 'NONE',  ( 0.07874015748031558404, -0.1870078740157480879, -0.4822834645669291653 ) ) ;
#51746=CARTESIAN_POINT ( 'NONE',  ( -1.286089238845143479, -0.6046776061558807314, 0.2411417322834647770 ) ) ;
#51747=CARTESIAN_POINT ( 'NONE',  ( 0.4527559055118117182, -0.4536011799217367080, 0.2665933059059888421 ) ) ;
#51748=CARTESIAN_POINT ( 'NONE',  ( 0.3277333542595164406, 0.004960608223778823628, 0.3437734562760190182 ) ) ;
#51749=CARTESIAN_POINT ( 'NONE',  ( -0.6233595800524928121, -0.05778040916215522460, 0.4822834645669289988 ) ) ;
#51750=CARTESIAN_POINT ( 'NONE',  ( -0.3215223097112853146, -0.08942795157528024563, -0.3641732283464568787 ) ) ;
#51752=CARTESIAN_POINT ( 'NONE',  ( -0.7349081364829390672, 0.2306618581243847221, -0.2411417322834647770 ) ) ;
#51753=CARTESIAN_POINT ( 'NONE',  ( -0.06561679790026180015, 0.05413385826771666132, 0.4176697321401328100 ) ) ;
#51754=CARTESIAN_POINT ( 'NONE',  ( 0.2821522309711292364, -0.5511811023622046335, 0.09757992244046803654 ) ) ;
#51756=CARTESIAN_POINT ( 'NONE',  ( 0.03937007874015833325, -0.6692913385826771977, 8.415575281601705876E-17 ) ) ;
#51759=CARTESIAN_POINT ( 'NONE',  ( 0.7217847769028878924, -0.004921259842519576551, 0.3153832671262227771 ) ) ;
#51760=CARTESIAN_POINT ( 'NONE',  ( 1.535433070866142335, -0.6692913385826771977, 8.415575281601705876E-17 ) ) ;
#51761=CARTESIAN_POINT ( 'NONE',  ( -0.9908136482939626788, -0.5511811023622048555, -0.09757992244046775898 ) ) ;
#51762=VECTOR ( 'NONE', #83198, 39.37007874015748143 ) ;
#51763=CARTESIAN_POINT ( 'NONE',  ( -1.305774278215222184, -0.5511811023622048555, -0.09757992244046775898 ) ) ;
#51764=CARTESIAN_POINT ( 'NONE',  ( -0.6102362204724400829, -0.5400638737290845981, -0.3530559997133363437 ) ) ;
#51765=CARTESIAN_POINT ( 'NONE',  ( -0.2427821522309703550, -0.05778040916215560624, -0.4822834645669293319 ) ) ;
#51766=CARTESIAN_POINT ( 'NONE',  ( 0.5643044619422579178, -0.004921259842519576551, 0.3153832671262227771 ) ) ;
#51768=CARTESIAN_POINT ( 'NONE',  ( 1.108923884514436242, -0.08942795157527998196, 0.3641732283464567121 ) ) ;
#51769=CARTESIAN_POINT ( 'NONE',  ( 0.6561679790026253567, -0.6046776061558809534, -0.2411417322834644161 ) ) ;
#51771=CARTESIAN_POINT ( 'NONE',  ( -0.2821522309711278487, 0.2952755905511811885, 0.1292274648535926551 ) ) ;
#51773=CARTESIAN_POINT ( 'NONE',  ( 1.312335958005249825, 0.1283753931104746893, -0.1820866141732285504 ) ) ;
#51774=CARTESIAN_POINT ( 'NONE',  ( 0.4855643044619430415, -0.4281496062992127816, -0.4176697321401328100 ) ) ;
#51775=CARTESIAN_POINT ( 'NONE',  ( -0.04593175853018302557, 0.2952755905511811885, 0.1292274648535926551 ) ) ;
#51777=CARTESIAN_POINT ( 'NONE',  ( 0.4593175853018380828, -0.004921259842519870586, -0.3153832671262229437 ) ) ;
#51778=CARTESIAN_POINT ( 'NONE',  ( 0.6758530183727039509, -0.6692913385826771977, 0.1292274648535927661 ) ) ;
#51779=EDGE_CURVE ( 'NONE', #65845, #14996, #5749, .T. ) ;
#51780=CARTESIAN_POINT ( 'NONE',  ( -0.3083989501312330295, -0.08942795157527998196, 0.3641732283464567121 ) ) ;
#51781=CARTESIAN_POINT ( 'NONE',  ( -0.8005249343832011588, 0.05413385826771626580, -0.4176697321401330321 ) ) ;
#51782=CARTESIAN_POINT ( 'NONE',  ( 0.8464566929133864326, 0.1660481256975883391, -0.3530559997133364547 ) ) ;
#51783=CARTESIAN_POINT ( 'NONE',  ( -0.3018372703412066094, 0.05413385826771666132, 0.4176697321401328100 ) ) ;
#51784=CARTESIAN_POINT ( 'NONE',  ( -1.213910761154854745, -0.6692913385826771977, 0.1292274648535927661 ) ) ;
#51785=CARTESIAN_POINT ( 'NONE',  ( -0.8792650918635160906, -0.004921259842519870586, -0.3153832671262229437 ) ) ;
#51786=CARTESIAN_POINT ( 'NONE',  ( 0.5446194225721792126, -0.05778040916215560624, -0.4822834645669293319 ) ) ;
#51787=CARTESIAN_POINT ( 'NONE',  ( -1.181102362204723644, -0.1870078740157480879, -0.4822834645669291653 ) ) ;
#51788=CARTESIAN_POINT ( 'NONE',  ( -0.2755905511811015396, -0.6692913385826771977, 8.415575281601705876E-17 ) ) ;
#51790=CARTESIAN_POINT ( 'NONE',  ( 1.660104986876641320, -0.05778040916215522460, 0.4822834645669289988 ) ) ;
#51791=CARTESIAN_POINT ( 'NONE',  ( 1.371391076115485719, -0.6692913385826773087, -0.1292274648535924053 ) ) ;
#51792=CARTESIAN_POINT ( 'NONE',  ( 1.233595800524935227, 0.2306618581243847221, -0.2411417322834647770 ) ) ;
#51795=CARTESIAN_POINT ( 'NONE',  ( -1.456692913385826182, -0.6692913385826771977, 8.415575281601705876E-17 ) ) ;
#51799=CARTESIAN_POINT ( 'NONE',  ( 0.01968503937007957949, -0.4536011799217368745, -0.2665933059059886201 ) ) ;
#51802=CARTESIAN_POINT ( 'NONE',  ( 0.3149606299212603933, -0.1870078740157479769, 0.4822834645669291653 ) ) ;
#51803=CARTESIAN_POINT ( 'NONE',  ( 0.4593175853018379162, -0.4281496062992124485, 0.4176697321401328655 ) ) ;
#51806=CARTESIAN_POINT ( 'NONE',  ( -0.3477690288713902178, 0.1771653543307087075, -0.09757992244046823083 ) ) ;
#51808=CARTESIAN_POINT ( 'NONE',  ( 0.7611548556430454138, 0.2306618581243847221, -0.2411417322834647770 ) ) ;
#51809=CARTESIAN_POINT ( 'NONE',  ( 1.043307086614173818, -0.4536011799217368745, -0.2665933059059886201 ) ) ;
#51810=CARTESIAN_POINT ( 'NONE',  ( -0.2296587926509179312, -0.05778040916215522460, 0.4822834645669289988 ) ) ;
#51812=CARTESIAN_POINT ( 'NONE',  ( -0.8595800524934373854, -0.05778040916215522460, 0.4822834645669289988 ) ) ;
#51813=CARTESIAN_POINT ( 'NONE',  ( -1.128608923884513837, -0.5023911411419708095, 0.1820866141732285504 ) ) ;
#51814=CARTESIAN_POINT ( 'NONE',  ( -1.036745406824146176, 0.05413385826771626580, -0.4176697321401330321 ) ) ;
#51815=CARTESIAN_POINT ( 'NONE',  ( 1.364829396325460076, 0.2306618581243848609, 0.2411417322834645549 ) ) ;
#51816=CARTESIAN_POINT ( 'NONE',  ( 0.4847769261806181285, 1.968503937007873850, -0.4915354330708656128 ) ) ;
#51817=EDGE_LOOP ( 'NONE', ( #25134, #2877, #48655, #37564, #75030 ) ) ;
#51819=CARTESIAN_POINT ( 'NONE',  ( 0.05905511811023709395, -0.5400638737290844871, 0.3530559997133364547 ) ) ;
#51821=CIRCLE ( 'NONE', #18263, 3.543307086614173151 ) ;
#51822=CARTESIAN_POINT ( 'NONE',  ( -0.9645669291338575535, -0.5400638737290844871, 0.3530559997133364547 ) ) ;
#51823=CARTESIAN_POINT ( 'NONE',  ( 1.528871391076116026, -0.6692913385826773087, -0.1292274648535924053 ) ) ;
#51824=CARTESIAN_POINT ( 'NONE',  ( 1.391076115485564868, -0.6046776061558807314, 0.2411417322834647770 ) ) ;
#51825=CARTESIAN_POINT ( 'NONE',  ( 0.3543307086614179147, 0.2952755905511811885, 0.000000000000000000 ) ) ;
#51826=CARTESIAN_POINT ( 'NONE',  ( 0.02624671916010564918, -0.6046776061558809534, -0.2411417322834644161 ) ) ;
#51828=CARTESIAN_POINT ( 'NONE',  ( -1.279527559055116948, -0.5400638737290844871, 0.3530559997133364547 ) ) ;
#51829=CARTESIAN_POINT ( 'NONE',  ( -0.1246719160104980823, -0.6692913385826773087, -0.1292274648535924053 ) ) ;
#51830=CARTESIAN_POINT ( 'NONE',  ( -0.2952755905511803003, -0.4536011799217368745, -0.2665933059059886201 ) ) ;
#51831=CARTESIAN_POINT ( 'NONE',  ( -1.614173228346457378, 0.7166040191147894367, 0.1372047244094476981 ) ) ;
#51832=CARTESIAN_POINT ( 'NONE',  ( 1.364829396325460076, 0.2306618581243848609, 0.2411417322834645549 ) ) ;
#51833=CARTESIAN_POINT ( 'NONE',  ( -0.6692913385826764205, -0.6692913385826771977, 8.415575281601705876E-17 ) ) ;
#51835=B_SPLINE_CURVE_WITH_KNOTS ( 'NONE', 3,
 ( #10202, #35871, #55204, #80912 ),
 .UNSPECIFIED., .F., .F.,
 ( 4, 4 ),
 ( 3.593986969189856268E-07, 0.001287825409103294464 ),
 .UNSPECIFIED. ) ;
#51836=CARTESIAN_POINT ( 'NONE',  ( 1.207349081364829990, -0.6046776061558809534, -0.2411417322834644161 ) ) ;
#51840=CARTESIAN_POINT ( 'NONE',  ( 0.3871391076115493490, -0.3162353388693405765, 0.4822834645669290543 ) ) ;
#51841=CARTESIAN_POINT ( 'NONE',  ( -0.4855643044619415427, -0.3690944881889763329, 0.3153832671262228327 ) ) ;
#51842=CARTESIAN_POINT ( 'NONE',  ( 1.535433070866142558, 0.1771653543307087630, 0.000000000000000000 ) ) ;
#51845=CARTESIAN_POINT ( 'NONE',  ( 1.627296587926509996, -0.5023911411419708095, 0.1820866141732285504 ) ) ;
#51846=CARTESIAN_POINT ( 'NONE',  ( 1.332020997375328974, -0.05778040916215560624, -0.4822834645669293319 ) ) ;
#51848=CARTESIAN_POINT ( 'NONE',  ( 0.07874015748031558404, -0.1870078740157480879, -0.4822834645669291653 ) ) ;
#51849=CARTESIAN_POINT ( 'NONE',  ( 0.1474713956048451791, 8.471767977567108961E-16, -0.4445507791589058955 ) ) ;
#51850=CARTESIAN_POINT ( 'NONE',  ( -1.443569553805773564, -0.6046776061558807314, 0.2411417322834647770 ) ) ;
#51851=CARTESIAN_POINT ( 'NONE',  ( 0.06561679790026316017, 0.05413385826771626580, -0.4176697321401330321 ) ) ;
#51853=CARTESIAN_POINT ( 'NONE',  ( 1.561679790026247350, 0.05413385826771626580, -0.4176697321401330321 ) ) ;
#51854=CARTESIAN_POINT ( 'NONE',  ( 0.3477690288713918276, 0.2952755905511811885, 0.1292274648535926551 ) ) ;
#51855=CARTESIAN_POINT ( 'NONE',  ( 0.9120734908136490793, 0.1771653543307087075, -0.09757992244046823083 ) ) ;
#51857=CARTESIAN_POINT ( 'NONE',  ( 0.6496062992125991586, -0.4536011799217368745, -0.2665933059059886201 ) ) ;
#51858=CARTESIAN_POINT ( 'NONE',  ( -1.227034120734907141, -0.6692913385826773087, -0.1292274648535924053 ) ) ;
#51860=CARTESIAN_POINT ( 'NONE',  ( 1.266404199475066328, -0.3162353388693409650, -0.4822834645669289433 ) ) ;
#51864=CARTESIAN_POINT ( 'NONE',  ( 0.7611548556430454138, 0.2306618581243847221, -0.2411417322834647770 ) ) ;
#51867=CARTESIAN_POINT ( 'NONE',  ( 0.3018372703412079971, -0.3690944881889763329, 0.3153832671262228327 ) ) ;
#51868=CARTESIAN_POINT ( 'NONE',  ( 0.4527559055118117182, 0.1660481256975883668, -0.3530559997133364547 ) ) ;
#51870=CARTESIAN_POINT ( 'NONE',  ( -1.102362204724408601, -0.1870078740157479769, 0.3641732283464567677 ) ) ;
#51871=CARTESIAN_POINT ( 'NONE',  ( -1.082677165354329896, 0.1660481256975885056, 0.3530559997133364547 ) ) ;
#51872=CARTESIAN_POINT ( 'NONE',  ( 1.023622047244095334, -0.1870078740157479769, 0.4822834645669291653 ) ) ;
#51873=CARTESIAN_POINT ( 'NONE',  ( -0.9317585301837263412, 0.05413385826771666132, 0.4176697321401328100 ) ) ;
#51874=CARTESIAN_POINT ( 'NONE',  ( 0.9514435695538062676, -0.3162353388693409650, -0.4822834645669289433 ) ) ;
#51875=CARTESIAN_POINT ( 'NONE',  ( -1.476377952755905110, 0.07958543189024085140, 0.2665933059059887866 ) ) ;
#51877=CARTESIAN_POINT ( 'NONE',  ( 0.8989501312335963501, -0.6692913385826773087, -0.1292274648535924053 ) ) ;
#51880=CARTESIAN_POINT ( 'NONE',  ( -0.08907927694006900765, -1.283732188437465593E-15, -0.4281993546915538462 ) ) ;
#51881=CARTESIAN_POINT ( 'NONE',  ( 1.548556430446194954, 0.2306618581243847221, -0.2411417322834647770 ) ) ;
#51882=CARTESIAN_POINT ( 'NONE',  ( -0.9645669291338575535, -0.4536011799217367080, 0.2665933059059888421 ) ) ;
#51883=CARTESIAN_POINT ( 'NONE',  ( 1.469816272965879911, -0.5023911411419708095, 0.1820866141732285504 ) ) ;
#51884=CARTESIAN_POINT ( 'NONE',  ( -1.437007874015747477, 0.07958543189024071263, -0.2665933059059888421 ) ) ;
#51885=CARTESIAN_POINT ( 'NONE',  ( -0.2624671916010490880, -0.5023911411419708095, 0.1820866141732285504 ) ) ;
#51886=ADVANCED_FACE ( 'NONE', ( #78859 ), #71697, .F. ) ;
#51888=CARTESIAN_POINT ( 'NONE',  ( 1.030183727034121421, -0.2845877964562161244, -0.3641732283464567121 ) ) ;
#51889=CARTESIAN_POINT ( 'NONE',  ( 0.6889763779527566800, -0.5400638737290844871, 0.3530559997133364547 ) ) ;
#51890=CARTESIAN_POINT ( 'NONE',  ( 1.115485564304462551, 0.05413385826771666132, 0.4176697321401328100 ) ) ;
#51891=CARTESIAN_POINT ( 'NONE',  ( 0.01968503937007957949, -0.5400638737290845981, -0.3530559997133363437 ) ) ;
#51892=CARTESIAN_POINT ( 'NONE',  ( 0.5708661417322841158, -0.4536011799217368745, -0.2665933059059886201 ) ) ;
#51893=CARTESIAN_POINT ( 'NONE',  ( -1.430446194225720724, 0.05413385826771626580, -0.4176697321401330321 ) ) ;
#51894=CARTESIAN_POINT ( 'NONE',  ( -1.509186351706035767, -0.4281496062992124485, 0.4176697321401328655 ) ) ;
#51895=CARTESIAN_POINT ( 'NONE',  ( -0.7217847769028863381, 0.05413385826771626580, -0.4176697321401330321 ) ) ;
#51897=CARTESIAN_POINT ( 'NONE',  ( -0.09842519685039295696, 0.1660481256975883668, -0.3530559997133364547 ) ) ;
#51898=CARTESIAN_POINT ( 'NONE',  ( -0.4396325459317577122, -0.6692913385826773087, -0.1292274648535924053 ) ) ;
#51899=CARTESIAN_POINT ( 'NONE',  ( 0.4330708661417329575, -0.6692913385826771977, 8.415575281601705876E-17 ) ) ;
#51905=CARTESIAN_POINT ( 'NONE',  ( -1.036745406824146176, -0.004921259842519870586, -0.3153832671262229437 ) ) ;
#51907=CARTESIAN_POINT ( 'NONE',  ( -1.069553805774277722, 0.2952755905511811885, 0.1292274648535926551 ) ) ;
#51909=CARTESIAN_POINT ( 'NONE',  ( 0.3937007874015754361, -0.1870078740157479769, 0.4822834645669291653 ) ) ;
#51910=CARTESIAN_POINT ( 'NONE',  ( -0.01312335958005186876, -0.3690944881889763329, 0.3153832671262228327 ) ) ;
#51911=CARTESIAN_POINT ( 'NONE',  ( 1.299212598425197429, 0.2952755905511811885, 0.000000000000000000 ) ) ;
#51912=CARTESIAN_POINT ( 'NONE',  ( 0.2952755905511816326, -0.5400638737290844871, 0.3530559997133364547 ) ) ;
#51916=CARTESIAN_POINT ( 'NONE',  ( 1.456692913385827515, -0.6692913385826771977, 8.415575281601705876E-17 ) ) ;
#51919=CARTESIAN_POINT ( 'NONE',  ( 0.5905511811023629321, -0.6692913385826771977, 8.415575281601705876E-17 ) ) ;
#51920=CARTESIAN_POINT ( 'NONE',  ( 0.2559055118110243332, -0.5400638737290845981, -0.3530559997133363437 ) ) ;
#51921=CARTESIAN_POINT ( 'NONE',  ( 0.8202099737532813073, 0.1771653543307087630, 0.09757992244046791164 ) ) ;
#51922=CARTESIAN_POINT ( 'NONE',  ( 1.482939632545932307, -0.4281496062992124485, 0.4176697321401328655 ) ) ;
#51924=CARTESIAN_POINT ( 'NONE',  ( 0.1968503937007881344, 0.2952755905511811885, 0.000000000000000000 ) ) ;
#51925=CARTESIAN_POINT ( 'NONE',  ( 0.8727034120734913358, -0.05778040916215522460, 0.4822834645669289988 ) ) ;
#51926=CARTESIAN_POINT ( 'NONE',  ( 0.3477690288713918276, -0.6692913385826773087, -0.1292274648535924053 ) ) ;
#51927=CARTESIAN_POINT ( 'NONE',  ( 1.253280839895013710, -0.08942795157528024563, -0.3641732283464568787 ) ) ;
#51928=CARTESIAN_POINT ( 'NONE',  ( -0.7677165354330699465, 0.1660481256975885056, 0.3530559997133364547 ) ) ;
#51929=CARTESIAN_POINT ( 'NONE',  ( -1.220472440944881054, 0.2952755905511811885, 0.000000000000000000 ) ) ;
#51930=CARTESIAN_POINT ( 'NONE',  ( 1.056430446194226436, -0.6692913385826773087, -0.1292274648535924053 ) ) ;
#51933=CARTESIAN_POINT ( 'NONE',  ( 1.607611548556431069, -0.6692913385826773087, -0.1292274648535924053 ) ) ;
#51937=CARTESIAN_POINT ( 'NONE',  ( 1.561679790026247350, 0.05413385826771626580, -0.4176697321401330321 ) ) ;
#51939=CARTESIAN_POINT ( 'NONE',  ( 0.7611548556430451917, -0.5023911411419708095, 0.1820866141732285504 ) ) ;
#51943=CARTESIAN_POINT ( 'NONE',  ( -0.9842519685039360366, 0.1771653543307087630, 0.000000000000000000 ) ) ;
#51944=CARTESIAN_POINT ( 'NONE',  ( -1.574803149606298636, -0.1870078740157479769, 0.3641732283464567677 ) ) ;
#51946=CARTESIAN_POINT ( 'NONE',  ( -0.1902887139107604098, -0.6692913385826771977, 0.1292274648535927661 ) ) ;
#51947=CARTESIAN_POINT ( 'NONE',  ( 1.482939632545932307, 0.05413385826771626580, -0.4176697321401330321 ) ) ;
#51953=CARTESIAN_POINT ( 'NONE',  ( -1.108923884514435132, -0.08942795157528024563, -0.3641732283464568787 ) ) ;
#51954=CARTESIAN_POINT ( 'NONE',  ( -1.437007874015747477, 0.1660481256975883668, -0.3530559997133364547 ) ) ;
#51955=CARTESIAN_POINT ( 'NONE',  ( 0.6496062992125991586, -0.5400638737290845981, -0.3530559997133363437 ) ) ;
#51958=( BOUNDED_SURFACE ( )  B_SPLINE_SURFACE ( 1, 2, ( 
 ( #69257, #16270, #23388, #48644, #74338, #16685, #42324, #41915, #67609, #4039, #30533, #56197, #11604, #60861, #17512, #29704, #81072, #74755, #68434, #3215, #10774, #4450, #30115, #81485, #23801, #49474, #5272, #30936, #18329, #45207, #25438, #13258, #56603, #24622, #43969, #82303, #50289, #75987, #83120, #44781, #57835, #69666, #50699, #51104, #12417, #37263, #12009, #37663, #63341, #62939, #70478, #5676, #31344, #70063, #57010, #76801, #82706, #25026, #31765, #64587, #57426, #76397, #19132, #18729, #12835, #38493, #44371, #38075, #64176, #6510, #32180, #63751, #6090, #203, #25855, #51515, #77219, #19548, #70907, #38907, #4296, #23647, #42993, #49728, #37515, #69099, #82155, #68688, #80514, #11030, #42592, #75426, #3892, #29959, #18176, #10212, #29552, #55215, #80922, #61549, #35880, #23237, #43400, #36687, #17768, #17365, #22829, #75019, #11447, #62362, #37103, #56040, #48906, #4700, #62788, #5122, #30373, #81748, #74607, #30789, #10628, #81333, #55624, #24059, #36284, #56453, #67874, #16950, #11862, #54810, #24470, #49318, #61957, #50137, #75835, #43809, #68292, #69513, #63190, #29144, #48488, #74189, #16535, #42180, #56735, #12141, #69795, #37798, #63067, #36977, #12550, #18858, #55909, #38208, #31066, #76118, #82432, #69386, #44506, #23934, #81621, #5810, #24750, #18050, #19264, #49602, #75296, #17640, #18459, #56329, #63883, #44102, #50418, #11740, #43272, #5404, #31480, #76936, #51237, #44917, #75709, #70614, #68969, #63475, #11318, #57141, #6221, #31897, #25160, #82838, #50828, #62657, #76530, #57558, #38626, #4998, #30666, #82028, #24342, #50011, #83249, #70195, #25572, #12969, #43683, #37395, #4575, #30246, #58826, #65982, #27666, #71041, #39889, #13386, #65576, #64723, #20946, #7062, #39038, #33571, #15054, #58398, #32731, #758, #33986, #53332, #59233, #14229, #79041, #7910, #21360, #72707, #71459, #39465, #1183, #78201, #1594, #64304, #46603, #59648, #20531, #32310, #46183, #77779, #27249, #26419, #65151, #47013, #45345, #52072, #20113, #45760, #13806, #7488, #33157, #78622, #71880, #52908, #52492, #57973, #26834, #72299, #14645, #40302, #8320, #2004, #6638, #338, #25994, #51651, #77356, #19687, #16716, #22188, #9562, #41543, #67643, #47845, #35646, #79448, #66821, #23420, #66395, #23009, #60896, #73551, #15895, #42356, #61730, #73123, #41130, #48677, #67232, #22602, #61307, #68054, #4067, #80288, #49086, #3248, #35233, #28911, #74786, #54575, #48262, #10401, #36058, #21768, #73959, #16305, #60071, #2426, #41948, #81103, #40710, #9977, #3664, #29327, #54988, #80696, #8733, #74372, #29734, #55397, #34403, #28082, #54156, #53740, #15473, #47430, #9154, #34827, #60485, #2835, #28498, #79871, #23836, #75197, #31377, #82334, #37696, #5307, #10803, #62969, #82736, #30966, #63371, #44003, #68870, #76017, #5706, #50730, #56633, #24652, #43173, #76429, #81929, #69287, #17949, #69696, #24240, #12040, #55808, #11218, #83149, #42769, #25055, #37294, #49913, #75611, #18757, #38106, #49504, #17541, #44401, #43586, #50320, #57042, #70093, #63782, #18359, #25469, #12447, #11634, #6121, #51135, #31793, #57456, #17137, #68465, #81515, #36463, #62138, #4477, #30147, #36878, #62556, #4891, #30566, #56231, #51968, #13699, #57869, #33044, #27143, #27563, #38523, #12866, #6540, #13285, #19580, #20841, #59132, #77676, #59547, #77251, #64618, #71353, #38937, #39355, #78517, #40198, #235, #52385, #25887, #78094, #45240, #33470, #70940, #51547, #46078, #76830, #6955, #32625, #58288, #46493, #65881, #71771, #26731, #8217, #653, #72189, #1490, #20006, #1902, #26310, #45657, #65039, #7376, #58713, #14546, #33881, #1078, #20425, #14124, #39777, #65471, #52807, #7805, #19162, #44812, #70508, #64206, #32210, #53638, #22905, #42256, #48163, #3145, #16614, #28808, #10294, #61630, #60382, #28392, #47741, #67125, #73858, #3972, #9873, #48573, #9455, #21255, #35128, #66714, #16199, #27979, #54051, #67951, #34302, #79345, #21666, #47325, #2319, #59963, #73016, #67536, #60792, #41846, #41441, #46909, #15789, #35542, #54472, #61203, #80185, #15367, #22500, #3560, #29225, #54892 ),
 ( #73439, #2731, #79765, #80597, #74270, #41028, #9047, #35961, #22082, #53222, #78932, #72604, #14951, #40609, #66292, #8631, #34722, #75512, #38008, #43485, #69181, #31279, #82641, #10709, #24141, #11532, #48989, #74687, #17033, #56125, #5611, #37597, #50222, #4785, #49812, #36366, #37189, #63271, #63686, #42672, #68371, #62040, #49403, #17851, #81831, #11116, #69596, #4377, #81005, #30869, #62869, #43075, #44307, #23319, #30045, #55707, #5205, #81416, #56944, #56535, #82237, #36773, #23732, #30462, #24556, #18662, #76332, #69997, #17445, #12352, #75097, #75918, #68772, #62449, #18257, #43899, #11943, #24954, #50627, #29636, #55296, #39683, #78421, #20327, #25790, #19486, #51451, #6858, #59041, #33377, #7280, #26212, #6024, #32950, #45562, #83050, #57354, #12768, #20749, #64940, #72092, #25373, #19067, #64107, #51036, #76737, #38425, #39258, #26639, #65375, #70412, #38841, #58616, #51874, #31695, #6442, #44715, #32114, #40102, #64520, #57772, #7710, #135, #71675, #77154, #45139, #983, #46399, #70843, #1395, #13604, #14451, #77998, #77580, #27050, #52709, #14026, #13192, #32527, #52293, #71258, #45979, #58191, #559, #19912, #33789, #79254, #16519, #16100, #79669, #72920, #2220, #61110, #41349, #15272, #34624, #15691, #60288, #54795, #65790, #2638, #73343, #47648, #67030, #40932, #14858, #73765, #80086, #59452, #41745, #8948, #67440, #21987, #28295, #47231, #21162, #66612, #9362, #80498, #29127, #22814, #53546, #48471, #46818, #53957, #27886, #8537, #66199, #21569, #1805, #72509, #27467, #9773, #35445, #3462, #74173, #22406, #35033, #60698, #3047, #28713, #8123, #53125, #54376, #48063, #78836, #40520, #34204, #59867, #10196, #48889, #57984, #17752, #26006, #35865, #55198, #16934, #61530, #3876, #74590, #75406, #63894, #19276, #23219, #75002, #43381, #62346, #42164, #42574, #80906, #29535, #77367, #17349, #67858, #44928, #68276, #25583, #61937, #10611, #38219, #349, #36268, #38637, #49712, #32322, #31908, #4684, #12981, #70625, #51247, #4280, #76949, #69082, #81732, #24041, #29941, #68672, #30355, #55606, #81317, #23630, #64315, #56024, #49301, #42976, #6649, #12561, #11011, #36670, #6232, #57569, #51663, #83261, #71891, #27260, #1604, #52920, #78212, #52082, #27680, #33998, #71053, #53345, #46196, #7921, #14242, #1195, #59660, #39050, #13397, #20958, #39900, #33169, #34416, #64735, #7073, #32743, #33582, #71470, #13818, #20124, #45771, #72719, #8745, #14658, #78634, #66408, #46616, #60084, #28096, #26844, #20544, #65588, #59245, #40315, #53752, #2016, #15066, #72311, #58410, #65994, #58837, #8332, #77791, #79055, #2438, #769, #39477, #65164, #7500, #52503, #26431, #21372, #47027, #40722, #19699, #45356, #73135, #41960, #61740, #67653, #42368, #23020, #47856, #54998, #68067, #29744, #35656, #9990, #22200, #55408, #60907, #48272, #80298, #48687, #3259, #74384, #34837, #73561, #62148, #21779, #4077, #16315, #28920, #54588, #81114, #17147, #28510, #79882, #23432, #22612, #61319, #16727, #49096, #42779, #3674, #4489, #29337, #73970, #80706, #30157, #10411, #36068, #74800, #68475, #60497, #10813, #36473, #15485, #41142, #66832, #79462, #47441, #9165, #2846, #54167, #15905, #41554, #67242, #9573, #35243, #17551, #75207, #68880, #75621, #81939, #83160, #38118, #56643, #38535, #56242, #43596, #50331, #17959, #76028, #57466, #19174, #62566, #31387, #4905, #57053, #24250, #12457, #49923, #30576, #25067, #6550, #82344, #18373, #23847, #69298, #55819, #6131, #69707, #62979, #11647, #51146, #82746, #5318, #24662, #5717, #44013, #44822, #81527, #12051, #63381, #37708, #50741, #30976, #37305, #63793, #70105, #49514, #31806, #76439, #18768, #44411, #25479, #76840, #43183, #11229, #70520, #12876, #64216, #36890, #25898, #246, #51558, #20437, #666, #40211, #46091, #78106, #13713, #70950, #7390, #59146, #21268, #78950, #72616, #20017, #46923, #13295, #71783, #77687, #58300, #32637, #71364, #77262, #38947, #19591, #65894, #8229, #33893, #14964, #46506, #51982, #45668, #39367, #33058, #1914, #59559, #33483, #52397, #32221, #1503, #14138, #45253, #64630, #6966, #40621 ) ),
 .UNSPECIFIED., .F., .F., .F. ) 
 B_SPLINE_SURFACE_WITH_KNOTS ( ( 2, 2 ),
 ( 3, 2, 2, 2, 2, 2, 2, 2, 2, 2, 2, 2, 2, 2, 2, 2, 2, 2, 2, 2, 2, 2, 2, 2, 2, 2, 2, 2, 2, 2, 2, 2, 2, 2, 2, 2, 2, 2, 2, 2, 2, 2, 2, 2, 2, 2, 2, 2, 2, 2, 2, 2, 2, 2, 2, 2, 2, 2, 2, 2, 2, 2, 2, 2, 2, 2, 2, 2, 2, 2, 2, 2, 2, 2, 2, 2, 2, 2, 2, 2, 2, 2, 2, 2, 2, 2, 2, 2, 2, 2, 2, 2, 2, 2, 2, 2, 2, 2, 2, 2, 2, 2, 2, 2, 2, 2, 2, 2, 2, 2, 2, 2, 2, 2, 2, 2, 2, 2, 2, 2, 2, 2, 2, 2, 2, 2, 2, 2, 2, 2, 2, 2, 2, 2, 2, 2, 2, 2, 2, 2, 2, 2, 2, 2, 2, 2, 2, 2, 2, 2, 2, 2, 2, 2, 2, 2, 2, 2, 2, 2, 2, 2, 2, 2, 2, 2, 2, 2, 2, 2, 2, 2, 2, 2, 2, 2, 2, 2, 2, 2, 2, 2, 2, 2, 2, 2, 2, 2, 2, 2, 2, 2, 2, 2, 2, 2, 2, 2, 2, 2, 2, 2, 2, 2, 2, 2, 2, 2, 2, 2, 2, 2, 2, 2, 2, 2, 2, 2, 2, 2, 2, 2, 2, 2, 2, 2, 2, 2, 2, 2, 2, 2, 2, 2, 2, 2, 2, 2, 2, 2, 2, 2, 2, 2, 2, 2, 2, 2, 2, 2, 2, 2, 2, 2, 2, 3 ),
 ( 0.000000000000000000, 1.000000000000000000 ),
 ( 0.000000000000000000, 0.003787878787878787984, 0.007575757575757575968, 0.01136363636363636395, 0.01515151515151515194, 0.01893939393939393992, 0.02272727272727272790, 0.02651515151515151589, 0.03030303030303030387, 0.03409090909090908839, 0.03787878787878787984, 0.04166666666666666435, 0.04545454545454545581, 0.04924242424242424032, 0.05303030303030303177, 0.05681818181818181629, 0.06060606060606060774, 0.06439393939393939226, 0.06818181818181817677, 0.07196969696969697516, 0.07575757575757575968, 0.07954545454545454419, 0.08333333333333332871, 0.08712121212121212710, 0.09090909090909091161, 0.09469696969696969613, 0.09848484848484848064, 0.1022727272727272790, 0.1060606060606060635, 0.1098484848484848481, 0.1136363636363636326, 0.1174242424242424310, 0.1212121212121212155, 0.1250000000000000000, 0.1287878787878787845, 0.1325757575757575690, 0.1363636363636363535, 0.1401515151515151381, 0.1439393939393939503, 0.1477272727272727348, 0.1515151515151515194, 0.1553030303030303039, 0.1590909090909090884, 0.1628787878787878729, 0.1666666666666666574, 0.1704545454545454419, 0.1742424242424242542, 0.1780303030303030387, 0.1818181818181818232, 0.1856060606060606077, 0.1893939393939393923, 0.1931818181818181768, 0.1969696969696969613, 0.2007575757575757458, 0.2045454545454545581, 0.2083333333333333426, 0.2121212121212121271, 0.2159090909090909116, 0.2196969696969696961, 0.2234848484848484806, 0.2272727272727272652, 0.2310606060606060497, 0.2348484848484848619, 0.2386363636363636465, 0.2424242424242424310, 0.2462121212121212155, 0.2500000000000000000, 0.2537878787878787845, 0.2575757575757575690, 0.2613636363636363535, 0.2651515151515151381, 0.2689393939393939226, 0.2727272727272727071, 0.2765151515151514916, 0.2803030303030302761, 0.2840909090909091161, 0.2878787878787879007, 0.2916666666666666852, 0.2954545454545454697, 0.2992424242424242542, 0.3030303030303030387, 0.3068181818181818232, 0.3106060606060606077, 0.3143939393939393923, 0.3181818181818181768, 0.3219696969696969613, 0.3257575757575757458, 0.3295454545454545303, 0.3333333333333333148, 0.3371212121212120993, 0.3409090909090908839, 0.3446969696969697239, 0.3484848484848485084, 0.3522727272727272929, 0.3560606060606060774, 0.3598484848484848619, 0.3636363636363636465, 0.3674242424242424310, 0.3712121212121212155, 0.3750000000000000000, 0.3787878787878787845, 0.3825757575757575690, 0.3863636363636363535, 0.3901515151515151381, 0.3939393939393939226, 0.3977272727272727071, 0.4015151515151514916, 0.4053030303030302761, 0.4090909090909091161, 0.4128787878787879007, 0.4166666666666666852, 0.4204545454545454697, 0.4242424242424242542, 0.4280303030303030387, 0.4318181818181818232, 0.4356060606060606077, 0.4393939393939393923, 0.4431818181818181768, 0.4469696969696969613, 0.4507575757575757458, 0.4545454545454545303, 0.4583333333333333148, 0.4621212121212120993, 0.4659090909090908839, 0.4696969696969697239, 0.4734848484848485084, 0.4772727272727272929, 0.4810606060606060774, 0.4848484848484848619, 0.4886363636363636465, 0.4924242424242424310, 0.4962121212121212155, 0.5000000000000000000, 0.5037878787878787845, 0.5075757575757575690, 0.5113636363636363535, 0.5151515151515151381, 0.5189393939393939226, 0.5227272727272727071, 0.5265151515151514916, 0.5303030303030302761, 0.5340909090909090606, 0.5378787878787878451, 0.5416666666666666297, 0.5454545454545454142, 0.5492424242424241987, 0.5530303030303029832, 0.5568181818181817677, 0.5606060606060605522, 0.5643939393939394478, 0.5681818181818182323, 0.5719696969696970168, 0.5757575757575758013, 0.5795454545454545858, 0.5833333333333333703, 0.5871212121212121549, 0.5909090909090909394, 0.5946969696969697239, 0.5984848484848485084, 0.6022727272727272929, 0.6060606060606060774, 0.6098484848484848619, 0.6136363636363636465, 0.6174242424242424310, 0.6212121212121212155, 0.6250000000000000000, 0.6287878787878787845, 0.6325757575757575690, 0.6363636363636363535, 0.6401515151515151381, 0.6439393939393939226, 0.6477272727272727071, 0.6515151515151514916, 0.6553030303030302761, 0.6590909090909090606, 0.6628787878787878451, 0.6666666666666666297, 0.6704545454545454142, 0.6742424242424241987, 0.6780303030303029832, 0.6818181818181817677, 0.6856060606060605522, 0.6893939393939394478, 0.6931818181818182323, 0.6969696969696970168, 0.7007575757575758013, 0.7045454545454545858, 0.7083333333333333703, 0.7121212121212121549, 0.7159090909090909394, 0.7196969696969697239, 0.7234848484848485084, 0.7272727272727272929, 0.7310606060606060774, 0.7348484848484848619, 0.7386363636363636465, 0.7424242424242424310, 0.7462121212121212155, 0.7500000000000000000, 0.7537878787878787845, 0.7575757575757575690, 0.7613636363636363535, 0.7651515151515151381, 0.7689393939393939226, 0.7727272727272727071, 0.7765151515151514916, 0.7803030303030302761, 0.7840909090909090606, 0.7878787878787878451, 0.7916666666666666297, 0.7954545454545454142, 0.7992424242424241987, 0.8030303030303029832, 0.8068181818181817677, 0.8106060606060605522, 0.8143939393939394478, 0.8181818181818182323, 0.8219696969696970168, 0.8257575757575758013, 0.8295454545454545858, 0.8333333333333333703, 0.8371212121212121549, 0.8409090909090909394, 0.8446969696969697239, 0.8484848484848485084, 0.8522727272727272929, 0.8560606060606060774, 0.8598484848484848619, 0.8636363636363636465, 0.8674242424242424310, 0.8712121212121212155, 0.8750000000000000000, 0.8787878787878787845, 0.8825757575757575690, 0.8863636363636363535, 0.8901515151515151381, 0.8939393939393939226, 0.8977272727272727071, 0.9015151515151514916, 0.9053030303030302761, 0.9090909090909090606, 0.9128787878787878451, 0.9166666666666666297, 0.9204545454545454142, 0.9242424242424241987, 0.9280303030303029832, 0.9318181818181817677, 0.9356060606060605522, 0.9393939393939394478, 0.9431818181818182323, 0.9469696969696970168, 0.9507575757575758013, 0.9545454545454545858, 0.9583333333333333703, 0.9621212121212121549, 0.9659090909090909394 ),
 .UNSPECIFIED. ) 
 GEOMETRIC_REPRESENTATION_ITEM ( )  RATIONAL_B_SPLINE_SURFACE ( (
 ( 1.000000000000000000, 0.9659258262890683122, 1.000000000000000000, 0.9659258262890683122, 1.000000000000000000, 0.9659258262890683122, 1.000000000000000000, 0.9659258262890683122, 1.000000000000000000, 0.9659258262890683122, 1.000000000000000000, 0.9659258262890683122, 1.000000000000000000, 0.9659258262890683122, 1.000000000000000000, 0.9659258262890683122, 1.000000000000000000, 0.9659258262890683122, 1.000000000000000000, 0.9659258262890683122, 1.000000000000000000, 0.9659258262890683122, 1.000000000000000000, 0.9659258262890683122, 1.000000000000000000, 0.9659258262890683122, 1.000000000000000000, 0.9659258262890683122, 1.000000000000000000, 0.9659258262890683122, 1.000000000000000000, 0.9659258262890683122, 1.000000000000000000, 0.9659258262890683122, 1.000000000000000000, 0.9659258262890683122, 1.000000000000000000, 0.9659258262890683122, 1.000000000000000000, 0.9659258262890683122, 1.000000000000000000, 0.9659258262890683122, 1.000000000000000000, 0.9659258262890683122, 1.000000000000000000, 0.9659258262890683122, 1.000000000000000000, 0.9659258262890683122, 1.000000000000000000, 0.9659258262890683122, 1.000000000000000000, 0.9659258262890683122, 1.000000000000000000, 0.9659258262890683122, 1.000000000000000000, 0.9659258262890683122, 1.000000000000000000, 0.9659258262890683122, 1.000000000000000000, 0.9659258262890683122, 1.000000000000000000, 0.9659258262890683122, 1.000000000000000000, 0.9659258262890683122, 1.000000000000000000, 0.9659258262890683122, 1.000000000000000000, 0.9659258262890683122, 1.000000000000000000, 0.9659258262890683122, 1.000000000000000000, 0.9659258262890683122, 1.000000000000000000, 0.9659258262890683122, 1.000000000000000000, 0.9659258262890683122, 1.000000000000000000, 0.9659258262890683122, 1.000000000000000000, 0.9659258262890683122, 1.000000000000000000, 0.9659258262890683122, 1.000000000000000000, 0.9659258262890683122, 1.000000000000000000, 0.9659258262890683122, 1.000000000000000000, 0.9659258262890683122, 1.000000000000000000, 0.9659258262890683122, 1.000000000000000000, 0.9659258262890683122, 1.000000000000000000, 0.9659258262890683122, 1.000000000000000000, 0.9659258262890683122, 1.000000000000000000, 0.9659258262890683122, 1.000000000000000000, 0.9659258262890683122, 1.000000000000000000, 0.9659258262890683122, 1.000000000000000000, 0.9659258262890683122, 1.000000000000000000, 0.9659258262890683122, 1.000000000000000000, 0.9659258262890683122, 1.000000000000000000, 0.9659258262890683122, 1.000000000000000000, 0.9659258262890683122, 1.000000000000000000, 0.9659258262890683122, 1.000000000000000000, 0.9659258262890683122, 1.000000000000000000, 0.9659258262890683122, 1.000000000000000000, 0.9659258262890683122, 1.000000000000000000, 0.9659258262890683122, 1.000000000000000000, 0.9659258262890683122, 1.000000000000000000, 0.9659258262890683122, 1.000000000000000000, 0.9659258262890683122, 1.000000000000000000, 0.9659258262890683122, 1.000000000000000000, 0.9659258262890683122, 1.000000000000000000, 0.9659258262890683122, 1.000000000000000000, 0.9659258262890683122, 1.000000000000000000, 0.9659258262890683122, 1.000000000000000000, 0.9659258262890683122, 1.000000000000000000, 0.9659258262890683122, 1.000000000000000000, 0.9659258262890683122, 1.000000000000000000, 0.9659258262890683122, 1.000000000000000000, 0.9659258262890683122, 1.000000000000000000, 0.9659258262890683122, 1.000000000000000000, 0.9659258262890683122, 1.000000000000000000, 0.9659258262890683122, 1.000000000000000000, 0.9659258262890683122, 1.000000000000000000, 0.9659258262890683122, 1.000000000000000000, 0.9659258262890683122, 1.000000000000000000, 0.9659258262890683122, 1.000000000000000000, 0.9659258262890683122, 1.000000000000000000, 0.9659258262890683122, 1.000000000000000000, 0.9659258262890683122, 1.000000000000000000, 0.9659258262890683122, 1.000000000000000000, 0.9659258262890683122, 1.000000000000000000, 0.9659258262890683122, 1.000000000000000000, 0.9659258262890683122, 1.000000000000000000, 0.9659258262890683122, 1.000000000000000000, 0.9659258262890683122, 1.000000000000000000, 0.9659258262890683122, 1.000000000000000000, 0.9659258262890683122, 1.000000000000000000, 0.9659258262890683122, 1.000000000000000000, 0.9659258262890683122, 1.000000000000000000, 0.9659258262890683122, 1.000000000000000000, 0.9659258262890683122, 1.000000000000000000, 0.9659258262890683122, 1.000000000000000000, 0.9659258262890683122, 1.000000000000000000, 0.9659258262890683122, 1.000000000000000000, 0.9659258262890683122, 1.000000000000000000, 0.9659258262890683122, 1.000000000000000000, 0.9659258262890683122, 1.000000000000000000, 0.9659258262890683122, 1.000000000000000000, 0.9659258262890683122, 1.000000000000000000, 0.9659258262890683122, 1.000000000000000000, 0.9659258262890683122, 1.000000000000000000, 0.9659258262890683122, 1.000000000000000000, 0.9659258262890683122, 1.000000000000000000, 0.9659258262890683122, 1.000000000000000000, 0.9659258262890683122, 1.000000000000000000, 0.9659258262890683122, 1.000000000000000000, 0.9659258262890683122, 1.000000000000000000, 0.9659258262890683122, 1.000000000000000000, 0.9659258262890683122, 1.000000000000000000, 0.9659258262890683122, 1.000000000000000000, 0.9659258262890683122, 1.000000000000000000, 0.9659258262890683122, 1.000000000000000000, 0.9659258262890683122, 1.000000000000000000, 0.9659258262890683122, 1.000000000000000000, 0.9659258262890683122, 1.000000000000000000, 0.9659258262890683122, 1.000000000000000000, 0.9659258262890683122, 1.000000000000000000, 0.9659258262890683122, 1.000000000000000000, 0.9659258262890683122, 1.000000000000000000, 0.9659258262890683122, 1.000000000000000000, 0.9659258262890683122, 1.000000000000000000, 0.9659258262890683122, 1.000000000000000000, 0.9659258262890683122, 1.000000000000000000, 0.9659258262890683122, 1.000000000000000000, 0.9659258262890683122, 1.000000000000000000, 0.9659258262890683122, 1.000000000000000000, 0.9659258262890683122, 1.000000000000000000, 0.9659258262890683122, 1.000000000000000000, 0.9659258262890683122, 1.000000000000000000, 0.9659258262890683122, 1.000000000000000000, 0.9659258262890683122, 1.000000000000000000, 0.9659258262890683122, 1.000000000000000000, 0.9659258262890683122, 1.000000000000000000, 0.9659258262890683122, 1.000000000000000000, 0.9659258262890683122, 1.000000000000000000, 0.9659258262890683122, 1.000000000000000000, 0.9659258262890683122, 1.000000000000000000, 0.9659258262890683122, 1.000000000000000000, 0.9659258262890683122, 1.000000000000000000, 0.9659258262890683122, 1.000000000000000000, 0.9659258262890683122, 1.000000000000000000, 0.9659258262890683122, 1.000000000000000000, 0.9659258262890683122, 1.000000000000000000, 0.9659258262890683122, 1.000000000000000000, 0.9659258262890683122, 1.000000000000000000, 0.9659258262890683122, 1.000000000000000000, 0.9659258262890683122, 1.000000000000000000, 0.9659258262890683122, 1.000000000000000000, 0.9659258262890683122, 1.000000000000000000, 0.9659258262890683122, 1.000000000000000000, 0.9659258262890683122, 1.000000000000000000, 0.9659258262890683122, 1.000000000000000000, 0.9659258262890683122, 1.000000000000000000, 0.9659258262890683122, 1.000000000000000000, 0.9659258262890683122, 1.000000000000000000, 0.9659258262890683122, 1.000000000000000000, 0.9659258262890683122, 1.000000000000000000, 0.9659258262890683122, 1.000000000000000000, 0.9659258262890683122, 1.000000000000000000, 0.9659258262890683122, 1.000000000000000000, 0.9659258262890683122, 1.000000000000000000, 0.9659258262890683122, 1.000000000000000000, 0.9659258262890683122, 1.000000000000000000, 0.9659258262890683122, 1.000000000000000000, 0.9659258262890683122, 1.000000000000000000, 0.9659258262890683122, 1.000000000000000000, 0.9659258262890683122, 1.000000000000000000, 0.9659258262890683122, 1.000000000000000000, 0.9659258262890683122, 1.000000000000000000, 0.9659258262890683122, 1.000000000000000000, 0.9659258262890683122, 1.000000000000000000, 0.9659258262890683122, 1.000000000000000000, 0.9659258262890683122, 1.000000000000000000, 0.9659258262890683122, 1.000000000000000000, 0.9659258262890683122, 1.000000000000000000, 0.9659258262890683122, 1.000000000000000000, 0.9659258262890683122, 1.000000000000000000, 0.9659258262890683122, 1.000000000000000000, 0.9659258262890683122, 1.000000000000000000, 0.9659258262890683122, 1.000000000000000000, 0.9659258262890683122, 1.000000000000000000, 0.9659258262890683122, 1.000000000000000000, 0.9659258262890683122, 1.000000000000000000, 0.9659258262890683122, 1.000000000000000000, 0.9659258262890683122, 1.000000000000000000, 0.9659258262890683122, 1.000000000000000000, 0.9659258262890683122, 1.000000000000000000, 0.9659258262890683122, 1.000000000000000000, 0.9659258262890683122, 1.000000000000000000, 0.9659258262890683122, 1.000000000000000000, 0.9659258262890683122, 1.000000000000000000, 0.9659258262890683122, 1.000000000000000000, 0.9659258262890683122, 1.000000000000000000, 0.9659258262890683122, 1.000000000000000000, 0.9659258262890683122, 1.000000000000000000, 0.9659258262890683122, 1.000000000000000000, 0.9659258262890683122, 1.000000000000000000, 0.9659258262890683122, 1.000000000000000000, 0.9659258262890683122, 1.000000000000000000, 0.9659258262890683122, 1.000000000000000000, 0.9659258262890683122, 1.000000000000000000, 0.9659258262890683122, 1.000000000000000000, 0.9659258262890683122, 1.000000000000000000, 0.9659258262890683122, 1.000000000000000000, 0.9659258262890683122, 1.000000000000000000, 0.9659258262890683122, 1.000000000000000000, 0.9659258262890683122, 1.000000000000000000, 0.9659258262890683122, 1.000000000000000000, 0.9659258262890683122, 1.000000000000000000, 0.9659258262890683122, 1.000000000000000000, 0.9659258262890683122, 1.000000000000000000, 0.9659258262890683122, 1.000000000000000000, 0.9659258262890683122, 1.000000000000000000, 0.9659258262890683122, 1.000000000000000000, 0.9659258262890683122, 1.000000000000000000, 0.9659258262890683122, 1.000000000000000000, 0.9659258262890683122, 1.000000000000000000, 0.9659258262890683122, 1.000000000000000000, 0.9659258262890683122, 1.000000000000000000, 0.9659258262890683122, 1.000000000000000000, 0.9659258262890683122, 1.000000000000000000, 0.9659258262890683122, 1.000000000000000000, 0.9659258262890683122, 1.000000000000000000, 0.9659258262890683122, 1.000000000000000000, 0.9659258262890683122, 1.000000000000000000, 0.9659258262890683122, 1.000000000000000000, 0.9659258262890683122, 1.000000000000000000, 0.9659258262890683122, 1.000000000000000000, 0.9659258262890683122, 1.000000000000000000, 0.9659258262890683122, 1.000000000000000000, 0.9659258262890683122, 1.000000000000000000, 0.9659258262890683122, 1.000000000000000000, 0.9659258262890683122, 1.000000000000000000, 0.9659258262890683122, 1.000000000000000000, 0.9659258262890683122, 1.000000000000000000, 0.9659258262890683122, 1.000000000000000000, 0.9659258262890683122, 1.000000000000000000, 0.9659258262890683122, 1.000000000000000000, 0.9659258262890683122, 1.000000000000000000, 0.9659258262890683122, 1.000000000000000000, 0.9659258262890683122, 1.000000000000000000, 0.9659258262890683122, 1.000000000000000000, 0.9659258262890683122, 1.000000000000000000, 0.9659258262890683122, 1.000000000000000000, 0.9659258262890683122, 1.000000000000000000, 0.9659258262890683122, 1.000000000000000000, 0.9659258262890683122, 1.000000000000000000, 0.9659258262890683122, 1.000000000000000000, 0.9659258262890683122, 1.000000000000000000, 0.9659258262890683122, 1.000000000000000000),
 ( 1.000000000000000000, 0.9659258262890683122, 1.000000000000000000, 0.9659258262890683122, 1.000000000000000000, 0.9659258262890683122, 1.000000000000000000, 0.9659258262890683122, 1.000000000000000000, 0.9659258262890683122, 1.000000000000000000, 0.9659258262890683122, 1.000000000000000000, 0.9659258262890683122, 1.000000000000000000, 0.9659258262890683122, 1.000000000000000000, 0.9659258262890683122, 1.000000000000000000, 0.9659258262890683122, 1.000000000000000000, 0.9659258262890683122, 1.000000000000000000, 0.9659258262890683122, 1.000000000000000000, 0.9659258262890683122, 1.000000000000000000, 0.9659258262890683122, 1.000000000000000000, 0.9659258262890683122, 1.000000000000000000, 0.9659258262890683122, 1.000000000000000000, 0.9659258262890683122, 1.000000000000000000, 0.9659258262890683122, 1.000000000000000000, 0.9659258262890683122, 1.000000000000000000, 0.9659258262890683122, 1.000000000000000000, 0.9659258262890683122, 1.000000000000000000, 0.9659258262890683122, 1.000000000000000000, 0.9659258262890683122, 1.000000000000000000, 0.9659258262890683122, 1.000000000000000000, 0.9659258262890683122, 1.000000000000000000, 0.9659258262890683122, 1.000000000000000000, 0.9659258262890683122, 1.000000000000000000, 0.9659258262890683122, 1.000000000000000000, 0.9659258262890683122, 1.000000000000000000, 0.9659258262890683122, 1.000000000000000000, 0.9659258262890683122, 1.000000000000000000, 0.9659258262890683122, 1.000000000000000000, 0.9659258262890683122, 1.000000000000000000, 0.9659258262890683122, 1.000000000000000000, 0.9659258262890683122, 1.000000000000000000, 0.9659258262890683122, 1.000000000000000000, 0.9659258262890683122, 1.000000000000000000, 0.9659258262890683122, 1.000000000000000000, 0.9659258262890683122, 1.000000000000000000, 0.9659258262890683122, 1.000000000000000000, 0.9659258262890683122, 1.000000000000000000, 0.9659258262890683122, 1.000000000000000000, 0.9659258262890683122, 1.000000000000000000, 0.9659258262890683122, 1.000000000000000000, 0.9659258262890683122, 1.000000000000000000, 0.9659258262890683122, 1.000000000000000000, 0.9659258262890683122, 1.000000000000000000, 0.9659258262890683122, 1.000000000000000000, 0.9659258262890683122, 1.000000000000000000, 0.9659258262890683122, 1.000000000000000000, 0.9659258262890683122, 1.000000000000000000, 0.9659258262890683122, 1.000000000000000000, 0.9659258262890683122, 1.000000000000000000, 0.9659258262890683122, 1.000000000000000000, 0.9659258262890683122, 1.000000000000000000, 0.9659258262890683122, 1.000000000000000000, 0.9659258262890683122, 1.000000000000000000, 0.9659258262890683122, 1.000000000000000000, 0.9659258262890683122, 1.000000000000000000, 0.9659258262890683122, 1.000000000000000000, 0.9659258262890683122, 1.000000000000000000, 0.9659258262890683122, 1.000000000000000000, 0.9659258262890683122, 1.000000000000000000, 0.9659258262890683122, 1.000000000000000000, 0.9659258262890683122, 1.000000000000000000, 0.9659258262890683122, 1.000000000000000000, 0.9659258262890683122, 1.000000000000000000, 0.9659258262890683122, 1.000000000000000000, 0.9659258262890683122, 1.000000000000000000, 0.9659258262890683122, 1.000000000000000000, 0.9659258262890683122, 1.000000000000000000, 0.9659258262890683122, 1.000000000000000000, 0.9659258262890683122, 1.000000000000000000, 0.9659258262890683122, 1.000000000000000000, 0.9659258262890683122, 1.000000000000000000, 0.9659258262890683122, 1.000000000000000000, 0.9659258262890683122, 1.000000000000000000, 0.9659258262890683122, 1.000000000000000000, 0.9659258262890683122, 1.000000000000000000, 0.9659258262890683122, 1.000000000000000000, 0.9659258262890683122, 1.000000000000000000, 0.9659258262890683122, 1.000000000000000000, 0.9659258262890683122, 1.000000000000000000, 0.9659258262890683122, 1.000000000000000000, 0.9659258262890683122, 1.000000000000000000, 0.9659258262890683122, 1.000000000000000000, 0.9659258262890683122, 1.000000000000000000, 0.9659258262890683122, 1.000000000000000000, 0.9659258262890683122, 1.000000000000000000, 0.9659258262890683122, 1.000000000000000000, 0.9659258262890683122, 1.000000000000000000, 0.9659258262890683122, 1.000000000000000000, 0.9659258262890683122, 1.000000000000000000, 0.9659258262890683122, 1.000000000000000000, 0.9659258262890683122, 1.000000000000000000, 0.9659258262890683122, 1.000000000000000000, 0.9659258262890683122, 1.000000000000000000, 0.9659258262890683122, 1.000000000000000000, 0.9659258262890683122, 1.000000000000000000, 0.9659258262890683122, 1.000000000000000000, 0.9659258262890683122, 1.000000000000000000, 0.9659258262890683122, 1.000000000000000000, 0.9659258262890683122, 1.000000000000000000, 0.9659258262890683122, 1.000000000000000000, 0.9659258262890683122, 1.000000000000000000, 0.9659258262890683122, 1.000000000000000000, 0.9659258262890683122, 1.000000000000000000, 0.9659258262890683122, 1.000000000000000000, 0.9659258262890683122, 1.000000000000000000, 0.9659258262890683122, 1.000000000000000000, 0.9659258262890683122, 1.000000000000000000, 0.9659258262890683122, 1.000000000000000000, 0.9659258262890683122, 1.000000000000000000, 0.9659258262890683122, 1.000000000000000000, 0.9659258262890683122, 1.000000000000000000, 0.9659258262890683122, 1.000000000000000000, 0.9659258262890683122, 1.000000000000000000, 0.9659258262890683122, 1.000000000000000000, 0.9659258262890683122, 1.000000000000000000, 0.9659258262890683122, 1.000000000000000000, 0.9659258262890683122, 1.000000000000000000, 0.9659258262890683122, 1.000000000000000000, 0.9659258262890683122, 1.000000000000000000, 0.9659258262890683122, 1.000000000000000000, 0.9659258262890683122, 1.000000000000000000, 0.9659258262890683122, 1.000000000000000000, 0.9659258262890683122, 1.000000000000000000, 0.9659258262890683122, 1.000000000000000000, 0.9659258262890683122, 1.000000000000000000, 0.9659258262890683122, 1.000000000000000000, 0.9659258262890683122, 1.000000000000000000, 0.9659258262890683122, 1.000000000000000000, 0.9659258262890683122, 1.000000000000000000, 0.9659258262890683122, 1.000000000000000000, 0.9659258262890683122, 1.000000000000000000, 0.9659258262890683122, 1.000000000000000000, 0.9659258262890683122, 1.000000000000000000, 0.9659258262890683122, 1.000000000000000000, 0.9659258262890683122, 1.000000000000000000, 0.9659258262890683122, 1.000000000000000000, 0.9659258262890683122, 1.000000000000000000, 0.9659258262890683122, 1.000000000000000000, 0.9659258262890683122, 1.000000000000000000, 0.9659258262890683122, 1.000000000000000000, 0.9659258262890683122, 1.000000000000000000, 0.9659258262890683122, 1.000000000000000000, 0.9659258262890683122, 1.000000000000000000, 0.9659258262890683122, 1.000000000000000000, 0.9659258262890683122, 1.000000000000000000, 0.9659258262890683122, 1.000000000000000000, 0.9659258262890683122, 1.000000000000000000, 0.9659258262890683122, 1.000000000000000000, 0.9659258262890683122, 1.000000000000000000, 0.9659258262890683122, 1.000000000000000000, 0.9659258262890683122, 1.000000000000000000, 0.9659258262890683122, 1.000000000000000000, 0.9659258262890683122, 1.000000000000000000, 0.9659258262890683122, 1.000000000000000000, 0.9659258262890683122, 1.000000000000000000, 0.9659258262890683122, 1.000000000000000000, 0.9659258262890683122, 1.000000000000000000, 0.9659258262890683122, 1.000000000000000000, 0.9659258262890683122, 1.000000000000000000, 0.9659258262890683122, 1.000000000000000000, 0.9659258262890683122, 1.000000000000000000, 0.9659258262890683122, 1.000000000000000000, 0.9659258262890683122, 1.000000000000000000, 0.9659258262890683122, 1.000000000000000000, 0.9659258262890683122, 1.000000000000000000, 0.9659258262890683122, 1.000000000000000000, 0.9659258262890683122, 1.000000000000000000, 0.9659258262890683122, 1.000000000000000000, 0.9659258262890683122, 1.000000000000000000, 0.9659258262890683122, 1.000000000000000000, 0.9659258262890683122, 1.000000000000000000, 0.9659258262890683122, 1.000000000000000000, 0.9659258262890683122, 1.000000000000000000, 0.9659258262890683122, 1.000000000000000000, 0.9659258262890683122, 1.000000000000000000, 0.9659258262890683122, 1.000000000000000000, 0.9659258262890683122, 1.000000000000000000, 0.9659258262890683122, 1.000000000000000000, 0.9659258262890683122, 1.000000000000000000, 0.9659258262890683122, 1.000000000000000000, 0.9659258262890683122, 1.000000000000000000, 0.9659258262890683122, 1.000000000000000000, 0.9659258262890683122, 1.000000000000000000, 0.9659258262890683122, 1.000000000000000000, 0.9659258262890683122, 1.000000000000000000, 0.9659258262890683122, 1.000000000000000000, 0.9659258262890683122, 1.000000000000000000, 0.9659258262890683122, 1.000000000000000000, 0.9659258262890683122, 1.000000000000000000, 0.9659258262890683122, 1.000000000000000000, 0.9659258262890683122, 1.000000000000000000, 0.9659258262890683122, 1.000000000000000000, 0.9659258262890683122, 1.000000000000000000, 0.9659258262890683122, 1.000000000000000000, 0.9659258262890683122, 1.000000000000000000, 0.9659258262890683122, 1.000000000000000000, 0.9659258262890683122, 1.000000000000000000, 0.9659258262890683122, 1.000000000000000000, 0.9659258262890683122, 1.000000000000000000, 0.9659258262890683122, 1.000000000000000000, 0.9659258262890683122, 1.000000000000000000, 0.9659258262890683122, 1.000000000000000000, 0.9659258262890683122, 1.000000000000000000, 0.9659258262890683122, 1.000000000000000000, 0.9659258262890683122, 1.000000000000000000, 0.9659258262890683122, 1.000000000000000000, 0.9659258262890683122, 1.000000000000000000, 0.9659258262890683122, 1.000000000000000000, 0.9659258262890683122, 1.000000000000000000, 0.9659258262890683122, 1.000000000000000000, 0.9659258262890683122, 1.000000000000000000, 0.9659258262890683122, 1.000000000000000000, 0.9659258262890683122, 1.000000000000000000, 0.9659258262890683122, 1.000000000000000000, 0.9659258262890683122, 1.000000000000000000, 0.9659258262890683122, 1.000000000000000000, 0.9659258262890683122, 1.000000000000000000, 0.9659258262890683122, 1.000000000000000000, 0.9659258262890683122, 1.000000000000000000, 0.9659258262890683122, 1.000000000000000000, 0.9659258262890683122, 1.000000000000000000, 0.9659258262890683122, 1.000000000000000000, 0.9659258262890683122, 1.000000000000000000, 0.9659258262890683122, 1.000000000000000000, 0.9659258262890683122, 1.000000000000000000, 0.9659258262890683122, 1.000000000000000000, 0.9659258262890683122, 1.000000000000000000, 0.9659258262890683122, 1.000000000000000000, 0.9659258262890683122, 1.000000000000000000, 0.9659258262890683122, 1.000000000000000000, 0.9659258262890683122, 1.000000000000000000, 0.9659258262890683122, 1.000000000000000000, 0.9659258262890683122, 1.000000000000000000, 0.9659258262890683122, 1.000000000000000000, 0.9659258262890683122, 1.000000000000000000, 0.9659258262890683122, 1.000000000000000000, 0.9659258262890683122, 1.000000000000000000, 0.9659258262890683122, 1.000000000000000000, 0.9659258262890683122, 1.000000000000000000, 0.9659258262890683122, 1.000000000000000000, 0.9659258262890683122, 1.000000000000000000, 0.9659258262890683122, 1.000000000000000000, 0.9659258262890683122, 1.000000000000000000, 0.9659258262890683122, 1.000000000000000000, 0.9659258262890683122, 1.000000000000000000, 0.9659258262890683122, 1.000000000000000000, 0.9659258262890683122, 1.000000000000000000, 0.9659258262890683122, 1.000000000000000000, 0.9659258262890683122, 1.000000000000000000, 0.9659258262890683122, 1.000000000000000000, 0.9659258262890683122, 1.000000000000000000) ) ) 
 REPRESENTATION_ITEM ( '' )  SURFACE ( )  );
#51959=CARTESIAN_POINT ( 'NONE',  ( 1.318897637795276356, -0.5400638737290844871, 0.3530559997133364547 ) ) ;
#51960=CARTESIAN_POINT ( 'NONE',  ( -1.568241469816272105, -0.05778040916215522460, 0.4822834645669289988 ) ) ;
#51962=CARTESIAN_POINT ( 'NONE',  ( -0.1837270341207343505, -0.5023911411419708095, 0.1820866141732285504 ) ) ;
#51963=CARTESIAN_POINT ( 'NONE',  ( -1.515748031496062076, -0.4536011799217367080, 0.2665933059059888421 ) ) ;
#51964=CARTESIAN_POINT ( 'NONE',  ( 0.4531182788721080934, 1.535433070866141447, -0.5309055118110237448 ) ) ;
#51965=CARTESIAN_POINT ( 'NONE',  ( -0.5314960629921250401, 0.07958543189024085140, 0.2665933059059887866 ) ) ;
#51966=CARTESIAN_POINT ( 'NONE',  ( 0.08530183727034192087, -0.2845877964562161244, -0.3641732283464567121 ) ) ;
#51967=CARTESIAN_POINT ( 'NONE',  ( 0.02624671916010564918, 0.2306618581243848609, 0.2411417322834645549 ) ) ;
#51968=CARTESIAN_POINT ( 'NONE',  ( -0.9317585301837263412, -0.3690944881889765550, -0.3153832671262227771 ) ) ;
#51970=CARTESIAN_POINT ( 'NONE',  ( 0.8858267716535438430, -0.5400638737290845981, -0.3530559997133363437 ) ) ;
#51972=CARTESIAN_POINT ( 'NONE',  ( -1.528871391076114250, -0.6692913385826771977, 0.1292274648535927661 ) ) ;
#51976=CARTESIAN_POINT ( 'NONE',  ( -0.3740157480314953431, -0.5400638737290845981, -0.3530559997133363437 ) ) ;
#51977=CARTESIAN_POINT ( 'NONE',  ( 0.3346456692913390985, 0.07958543189024085140, 0.2665933059059887866 ) ) ;
#51978=CARTESIAN_POINT ( 'NONE',  ( -0.9186351706036736120, -0.6046776061558809534, -0.2411417322834644161 ) ) ;
#51979=CARTESIAN_POINT ( 'NONE',  ( 0.9711286089238851948, -0.5023911411419708095, -0.1820866141732282451 ) ) ;
#51980=CARTESIAN_POINT ( 'NONE',  ( -0.4527559055118102749, 0.07958543189024085140, 0.2665933059059887866 ) ) ;
#51981=CARTESIAN_POINT ( 'NONE',  ( -0.5314960629921254842, -0.5400638737290845981, -0.3530559997133363437 ) ) ;
#51982=CARTESIAN_POINT ( 'NONE',  ( -1.561679790026246017, -0.4281496062992127816, -0.4176697321401328100 ) ) ;
#51984=CARTESIAN_POINT ( 'NONE',  ( 1.371391076115485941, 0.1771653543307087630, 0.09757992244046791164 ) ) ;
#51985=CARTESIAN_POINT ( 'NONE',  ( 0.5118110236220480003, -0.6692913385826771977, 8.415575281601705876E-17 ) ) ;
#51986=CARTESIAN_POINT ( 'NONE',  ( -1.371391076115484609, -0.6692913385826771977, 0.1292274648535927661 ) ) ;
#51987=CARTESIAN_POINT ( 'NONE',  ( -1.489501312335957062, -0.3162353388693409650, -0.4822834645669289433 ) ) ;
#51990=CARTESIAN_POINT ( 'NONE',  ( -1.036745406824146176, -0.3690944881889763329, 0.3153832671262228327 ) ) ;
#51991=CARTESIAN_POINT ( 'NONE',  ( 0.5971128608923890191, -0.6692913385826771977, 0.1292274648535927661 ) ) ;
#51992=CARTESIAN_POINT ( 'NONE',  ( -1.161417322834644716, -0.4536011799217368745, -0.2665933059059886201 ) ) ;
#51994=CARTESIAN_POINT ( 'NONE',  ( -1.187664041994750175, -0.05778040916215560624, -0.4822834645669293319 ) ) ;
#51995=CARTESIAN_POINT ( 'NONE',  ( 0.9251968503937015864, 0.1660481256975883668, -0.3530559997133364547 ) ) ;
#51996=CARTESIAN_POINT ( 'NONE',  ( 0.4002624671916016896, -0.05778040916215522460, 0.4822834645669289988 ) ) ;
#51997=CARTESIAN_POINT ( 'NONE',  ( -1.220472440944881054, 0.000000000000000000, 0.5309055118110237448 ) ) ;
#51998=CARTESIAN_POINT ( 'NONE',  ( -1.666666666666665853, -0.004921259842519870586, -0.3153832671262229437 ) ) ;
#52003=CARTESIAN_POINT ( 'NONE',  ( 0.7020997375328090762, -0.2845877964562159024, 0.3641732283464567677 ) ) ;
#52004=CARTESIAN_POINT ( 'NONE',  ( 0.4527559055118117182, -0.4536011799217367080, 0.2665933059059888421 ) ) ;
#52005=CARTESIAN_POINT ( 'NONE',  ( 0.2230971128608929543, 0.05413385826771626580, -0.4176697321401330321 ) ) ;
#52006=CARTESIAN_POINT ( 'NONE',  ( 1.207349081364829990, -0.6046776061558809534, -0.2411417322834644161 ) ) ;
#52008=CARTESIAN_POINT ( 'NONE',  ( 0.5314960629921267055, -0.4536011799217367080, 0.2665933059059888421 ) ) ;
#52009=CARTESIAN_POINT ( 'NONE',  ( -0.9186351706036736120, -0.6046776061558809534, -0.2411417322834644161 ) ) ;
#52010=CARTESIAN_POINT ( 'NONE',  ( -1.240157480314959759, -0.5400638737290845981, -0.3530559997133363437 ) ) ;
#52011=CARTESIAN_POINT ( 'NONE',  ( 1.030183727034121421, -0.05778040916215522460, 0.4822834645669289988 ) ) ;
#52015=ORIENTED_EDGE ( 'NONE', *, *, #62252, .F. ) ;
#52016=CARTESIAN_POINT ( 'NONE',  ( -1.253280839895012377, -0.05778040916215522460, 0.4822834645669289988 ) ) ;
#52017=CARTESIAN_POINT ( 'NONE',  ( -0.5052493438320203589, 0.2952755905511810774, -0.1292274648535930714 ) ) ;
#52018=CARTESIAN_POINT ( 'NONE',  ( -0.9580052493438311334, -0.004921259842519870586, -0.3153832671262229437 ) ) ;
#52019=CARTESIAN_POINT ( 'NONE',  ( -0.9514435695538050464, -0.05778040916215560624, -0.4822834645669293319 ) ) ;
#52022=CARTESIAN_POINT ( 'NONE',  ( 1.561679790026247350, 0.05413385826771626580, -0.4176697321401330321 ) ) ;
#52023=CARTESIAN_POINT ( 'NONE',  ( -1.174540682414697335, -0.3162353388693409650, -0.4822834645669289433 ) ) ;
#52024=CARTESIAN_POINT ( 'NONE',  ( 0.4658792650918640033, -0.3162353388693405765, 0.4822834645669290543 ) ) ;
#52025=CARTESIAN_POINT ( 'NONE',  ( -0.8858267716535425107, -0.5400638737290844871, 0.3530559997133364547 ) ) ;
#52026=CARTESIAN_POINT ( 'NONE',  ( 0.6233595800524939223, -0.3162353388693405765, 0.4822834645669290543 ) ) ;
#52028=CARTESIAN_POINT ( 'NONE',  ( -0.7086614173228339419, -0.1870078740157479769, 0.3641732283464567677 ) ) ;
#52032=ORIENTED_EDGE ( 'NONE', *, *, #79015, .F. ) ;
#52033=CARTESIAN_POINT ( 'NONE',  ( -1.633858267716534529, -0.4536011799217368745, -0.2665933059059886201 ) ) ;
#52035=CARTESIAN_POINT ( 'NONE',  ( -1.279527559055116948, -0.5400638737290844871, 0.3530559997133364547 ) ) ;
#52036=CARTESIAN_POINT ( 'NONE',  ( -1.377952755905511140, -0.6692913385826771977, 8.415575281601705876E-17 ) ) ;
#52038=CARTESIAN_POINT ( 'NONE',  ( -1.292650918635170010, -0.6692913385826771977, 0.1292274648535927661 ) ) ;
#52039=CARTESIAN_POINT ( 'NONE',  ( -1.318897637795274802, -0.5400638737290845981, -0.3530559997133363437 ) ) ;
#52040=CARTESIAN_POINT ( 'NONE',  ( -1.614173228346455824, 0.2952755905511811885, 0.000000000000000000 ) ) ;
#52042=CARTESIAN_POINT ( 'NONE',  ( 0.2690288713910767848, 0.1771653543307087630, 0.09757992244046791164 ) ) ;
#52045=CARTESIAN_POINT ( 'NONE',  ( -0.4133858267716528645, 0.07958543189024071263, -0.2665933059059888421 ) ) ;
#52046=CARTESIAN_POINT ( 'NONE',  ( -0.6167979002624665030, -0.4281496062992127816, -0.4176697321401328100 ) ) ;
#52047=CARTESIAN_POINT ( 'NONE',  ( 1.502624671916010790, -0.3162353388693409650, -0.4822834645669289433 ) ) ;
#52048=CARTESIAN_POINT ( 'NONE',  ( -0.3674540682414689785, 0.2306618581243848609, 0.2411417322834645549 ) ) ;
#52050=ORIENTED_EDGE ( 'NONE', *, *, #60654, .T. ) ;
#52052=CARTESIAN_POINT ( 'NONE',  ( -0.8792650918635160906, -0.4281496062992124485, 0.4176697321401328655 ) ) ;
#52053=CARTESIAN_POINT ( 'NONE',  ( 1.358267716535433323, -0.5400638737290845981, -0.3530559997133363437 ) ) ;
#52054=CARTESIAN_POINT ( 'NONE',  ( -1.476377952755905110, -0.4536011799217368745, -0.2665933059059886201 ) ) ;
#52059=CARTESIAN_POINT ( 'NONE',  ( -0.4068241469816264999, -0.4281496062992124485, 0.4176697321401328655 ) ) ;
#52060=CARTESIAN_POINT ( 'NONE',  ( -1.489501312335957062, -0.08942795157527998196, 0.3641732283464567121 ) ) ;
#52061=CARTESIAN_POINT ( 'NONE',  ( -0.5774278215223089816, 0.2306618581243847221, -0.2411417322834647770 ) ) ;
#52063=CARTESIAN_POINT ( 'NONE',  ( -1.391076115485563758, 0.2306618581243848609, 0.2411417322834645549 ) ) ;
#52064=CARTESIAN_POINT ( 'NONE',  ( -0.9908136482939626788, -0.6692913385826773087, -0.1292274648535924053 ) ) ;
#52065=CARTESIAN_POINT ( 'NONE',  ( -0.5380577427821514602, -0.4281496062992127816, -0.4176697321401328100 ) ) ;
#52067=CARTESIAN_POINT ( 'NONE',  ( 1.082677165354331228, -0.4536011799217367080, 0.2665933059059888421 ) ) ;
#52068=DIRECTION ( 'NONE',  ( -3.096699300667737957E-16, 1.000000000000000000, -0.000000000000000000 ) ) ;
#52069=CARTESIAN_POINT ( 'NONE',  ( 0.5774278215223104249, 0.1283753931104748280, 0.1820866141732283561 ) ) ;
#52070=CARTESIAN_POINT ( 'NONE',  ( 1.272965879265092637, -0.004921259842519576551, 0.3153832671262227771 ) ) ;
#52071=CARTESIAN_POINT ( 'NONE',  ( 1.364829396325459854, -0.6046776061558809534, -0.2411417322834644161 ) ) ;
#52072=CARTESIAN_POINT ( 'NONE',  ( 0.05905511811023709395, -0.4536011799217367080, 0.2665933059059888421 ) ) ;
#52074=CARTESIAN_POINT ( 'NONE',  ( -0.9842519685039360366, 0.2952755905511811885, 0.000000000000000000 ) ) ;
#52075=CARTESIAN_POINT ( 'NONE',  ( 1.102362204724410155, -0.1870078740157479769, 0.4822834645669291653 ) ) ;
#52077=CARTESIAN_POINT ( 'NONE',  ( -0.5643044619422565855, -0.3690944881889763329, 0.3153832671262228327 ) ) ;
#52078=CARTESIAN_POINT ( 'NONE',  ( -0.4396325459317579343, 0.2952755905511811885, 0.1292274648535926551 ) ) ;
#52079=CARTESIAN_POINT ( 'NONE',  ( 0.2559055118110243332, 0.1660481256975885056, 0.3530559997133364547 ) ) ;
#52080=CARTESIAN_POINT ( 'NONE',  ( 1.030183727034121421, -0.2845877964562161244, -0.3641732283464567121 ) ) ;
#52081=CARTESIAN_POINT ( 'NONE',  ( 0.05905511811023681640, 0.07958543189024071263, -0.2665933059059888421 ) ) ;
#52082=CARTESIAN_POINT ( 'NONE',  ( -0.1312335958005241554, -0.6046776061558809534, -0.2411417322834644161 ) ) ;
#52083=CARTESIAN_POINT ( 'NONE',  ( -1.509186351706035767, 0.05413385826771626580, -0.4176697321401330321 ) ) ;
#52084=CARTESIAN_POINT ( 'NONE',  ( -0.8070866141732276899, 0.07958543189024071263, -0.2665933059059888421 ) ) ;
#52085=CARTESIAN_POINT ( 'NONE',  ( -1.586052503253846169, 1.850393700787402729, 0.1653254495020583248 ) ) ;
#52086=CARTESIAN_POINT ( 'NONE',  ( 0.7349081364829403995, 0.2306618581243848609, 0.2411417322834645549 ) ) ;
#52087=CARTESIAN_POINT ( 'NONE',  ( -1.036745406824146176, -0.4281496062992124485, 0.4176697321401328655 ) ) ;
#52091=CARTESIAN_POINT ( 'NONE',  ( 0.2230971128608929543, -0.004921259842519870586, -0.3153832671262229437 ) ) ;
#52092=CARTESIAN_POINT ( 'NONE',  ( -0.8923884514435688198, -0.6046776061558807314, 0.2411417322834647770 ) ) ;
#52094=CARTESIAN_POINT ( 'NONE',  ( -1.154855643044618851, 0.2306618581243848609, 0.2411417322834645549 ) ) ;
#52095=CARTESIAN_POINT ( 'NONE',  ( -1.266404199475064773, -0.08942795157528024563, -0.3641732283464568787 ) ) ;
#52097=CARTESIAN_POINT ( 'NONE',  ( -0.9908136482939626788, 0.1771653543307087630, 0.09757992244046791164 ) ) ;
#52098=CARTESIAN_POINT ( 'NONE',  ( -1.430446194225721390, -0.3690944881889763329, 0.3153832671262228327 ) ) ;
#52099=CARTESIAN_POINT ( 'NONE',  ( 1.279527559055118724, 0.1660481256975885056, 0.3530559997133364547 ) ) ;
#52102=ORIENTED_EDGE ( 'NONE', *, *, #76299, .T. ) ;
#52103=CARTESIAN_POINT ( 'NONE',  ( -0.2262115530851587786, -2.191421614605370878E-15, 0.4445507791589071167 ) ) ;
#52105=CARTESIAN_POINT ( 'NONE',  ( 1.601049868766404982, 0.1283753931104748280, 0.1820866141732283561 ) ) ;
#52106=CARTESIAN_POINT ( 'NONE',  ( -1.240157480314959759, 0.1660481256975885056, 0.3530559997133364547 ) ) ;
#52107=CARTESIAN_POINT ( 'NONE',  ( 1.437007874015748810, 0.1660481256975885056, 0.3530559997133364547 ) ) ;
#52109=FACE_OUTER_BOUND ( 'NONE', #13679, .T. ) ;
#52110=EDGE_CURVE ( 'NONE', #70238, #44445, #14405, .T. ) ;
#52111=CARTESIAN_POINT ( 'NONE',  ( 0.6364829396325465405, -0.3162353388693409650, -0.4822834645669289433 ) ) ;
#52112=CARTESIAN_POINT ( 'NONE',  ( -0.1574803149606292529, -0.1870078740157480879, -0.4822834645669291653 ) ) ;
#52114=CARTESIAN_POINT ( 'NONE',  ( -0.7233831536534669482, 2.176714048050446326, -0.5048085489442492024 ) ) ;
#52115=CARTESIAN_POINT ( 'NONE',  ( 0.9055118110236227702, -0.5511811023622047445, 6.969142054262312111E-17 ) ) ;
#52119=ORIENTED_EDGE ( 'NONE', *, *, #23584, .T. ) ;
#52120=CARTESIAN_POINT ( 'NONE',  ( 0.1181102362204730916, -0.6692913385826771977, 8.415575281601705876E-17 ) ) ;
#52121=CARTESIAN_POINT ( 'NONE',  ( 1.141732283464567566, 0.2952755905511811885, 0.000000000000000000 ) ) ;
#52122=CARTESIAN_POINT ( 'NONE',  ( 0.8464566929133866546, -0.5400638737290844871, 0.3530559997133364547 ) ) ;
#52123=CARTESIAN_POINT ( 'NONE',  ( 1.397637795275591177, 0.1660481256975883668, -0.3530559997133364547 ) ) ;
#52124=CARTESIAN_POINT ( 'NONE',  ( -0.6889763779527552368, 0.1660481256975885056, 0.3530559997133364547 ) ) ;
#52125=CARTESIAN_POINT ( 'NONE',  ( 0.07217847769028949700, -0.05778040916215560624, -0.4822834645669293319 ) ) ;
#52126=CARTESIAN_POINT ( 'NONE',  ( 1.391076115485564868, -0.6046776061558807314, 0.2411417322834647770 ) ) ;
#52127=CARTESIAN_POINT ( 'NONE',  ( 1.200787401574803681, -0.5400638737290845981, -0.3530559997133363437 ) ) ;
#52128=CARTESIAN_POINT ( 'NONE',  ( 1.305774278215223960, -0.6692913385826771977, 0.1292274648535927661 ) ) ;
#52129=CARTESIAN_POINT ( 'NONE',  ( 5.463695987328526437E-16, -0.1870078740157479769, 0.4822834645669291653 ) ) ;
#52132=CARTESIAN_POINT ( 'NONE',  ( 0.3477690288713918276, -0.5511811023622048555, -0.09757992244046775898 ) ) ;
#52136=CARTESIAN_POINT ( 'NONE',  ( -0.5708661417322828946, 0.07958543189024071263, -0.2665933059059888421 ) ) ;
#52137=CARTESIAN_POINT ( 'NONE',  ( -0.006561679790025524116, -0.05778040916215560624, -0.4822834645669293319 ) ) ;
#52139=CARTESIAN_POINT ( 'NONE',  ( 0.1509186351706042484, -0.3162353388693405765, 0.4822834645669290543 ) ) ;
#52140=CARTESIAN_POINT ( 'NONE',  ( 0.1312335958005255154, -0.6046776061558807314, 0.2411417322834647770 ) ) ;
#52141=EDGE_CURVE ( 'NONE', #50999, #4208, #37572, .T. ) ;
#52142=CARTESIAN_POINT ( 'NONE',  ( -1.115485564304461219, -0.4281496062992124485, 0.4176697321401328655 ) ) ;
#52143=CARTESIAN_POINT ( 'NONE',  ( 1.292650918635171564, -0.5511811023622048555, -0.09757992244046775898 ) ) ;
#52144=CARTESIAN_POINT ( 'NONE',  ( -1.601049868766403650, 0.2306618581243847221, -0.2411417322834647770 ) ) ;
#52146=CARTESIAN_POINT ( 'NONE',  ( 1.069553805774278610, -0.5511811023622046335, 0.09757992244046803654 ) ) ;
#52147=CARTESIAN_POINT ( 'NONE',  ( 0.3477690288713918276, -0.6692913385826773087, -0.1292274648535924053 ) ) ;
#52148=CARTESIAN_POINT ( 'NONE',  ( 0.7283464566929143125, 0.1660481256975885056, 0.3530559997133364547 ) ) ;
#52150=DIRECTION ( 'NONE',  ( -0.4043106043482678214, -0.6467352376403849856, 0.6467352376403909808 ) ) ;
#52153=CARTESIAN_POINT ( 'NONE',  ( -0.08530183727034056085, -0.05778040916215560624, -0.4822834645669293319 ) ) ;
#52157=CARTESIAN_POINT ( 'NONE',  ( -1.036745406824146176, -0.3690944881889763329, 0.3153832671262228327 ) ) ;
#52158=CARTESIAN_POINT ( 'NONE',  ( 1.292650918635171564, 0.2952755905511811885, 0.1292274648535926551 ) ) ;
#52160=CARTESIAN_POINT ( 'NONE',  ( 1.397637795275591177, 0.1660481256975883668, -0.3530559997133364547 ) ) ;
#52161=CARTESIAN_POINT ( 'NONE',  ( -0.4330708661417315697, -0.5511811023622047445, 6.969142054262312111E-17 ) ) ;
#52162=CARTESIAN_POINT ( 'NONE',  ( 0.6299212598425204535, -0.1870078740157479769, 0.4822834645669291653 ) ) ;
#52164=CARTESIAN_POINT ( 'NONE',  ( 0.4265091863517067594, 0.1771653543307087630, 0.09757992244046791164 ) ) ;
#52165=CARTESIAN_POINT ( 'NONE',  ( -0.1574803149606292529, -0.1870078740157479769, 0.4822834645669291653 ) ) ;
#52167=CARTESIAN_POINT ( 'NONE',  ( -1.030183727034119867, -0.05778040916215560624, -0.4822834645669293319 ) ) ;
#52168=CARTESIAN_POINT ( 'NONE',  ( 0.3149606299212603933, -0.1870078740157479769, 0.3641732283464567677 ) ) ;
#52170=CARTESIAN_POINT ( 'NONE',  ( -1.171093442848938793, -2.191421614605370878E-15, 0.4445507791589071167 ) ) ;
#52171=CARTESIAN_POINT ( 'NONE',  ( -0.8267716535433065062, -0.6692913385826771977, 8.415575281601705876E-17 ) ) ;
#52172=CARTESIAN_POINT ( 'NONE',  ( -0.4330708661417315697, -0.5511811023622047445, 6.969142054262312111E-17 ) ) ;
#52174=CARTESIAN_POINT ( 'NONE',  ( -0.5905511811023615998, 0.2952755905511811885, 0.000000000000000000 ) ) ;
#52175=CARTESIAN_POINT ( 'NONE',  ( -0.3215223097112853146, -0.05778040916215560624, -0.4822834645669293319 ) ) ;
#52176=CARTESIAN_POINT ( 'NONE',  ( 0.2099737532808405305, 0.1283753931104746893, -0.1820866141732285504 ) ) ;
#52178=CARTESIAN_POINT ( 'NONE',  ( -0.04593175853018302557, 0.2952755905511811885, 0.1292274648535926551 ) ) ;
#52180=CARTESIAN_POINT ( 'NONE',  ( -1.725721784776902190, -0.08942795157527998196, 0.3641732283464567121 ) ) ;
#52181=CARTESIAN_POINT ( 'NONE',  ( 0.7152230971128616943, -0.08942795157527998196, 0.3641732283464567121 ) ) ;
#52182=CARTESIAN_POINT ( 'NONE',  ( 1.522309711286089939, -0.6046776061558809534, -0.2411417322834644161 ) ) ;
#52183=CARTESIAN_POINT ( 'NONE',  ( -0.7677165354330699465, 0.07958543189024085140, 0.2665933059059887866 ) ) ;
#52184=CARTESIAN_POINT ( 'NONE',  ( -1.115485564304461219, -0.3690944881889763329, 0.3153832671262228327 ) ) ;
#52185=CARTESIAN_POINT ( 'NONE',  ( -0.6167979002624665030, -0.4281496062992127816, -0.4176697321401328100 ) ) ;
#52186=CARTESIAN_POINT ( 'NONE',  ( -0.01968503937007793844, -0.5400638737290844871, 0.3530559997133364547 ) ) ;
#52187=CARTESIAN_POINT ( 'NONE',  ( 0.5052493438320218022, -0.5511811023622048555, -0.09757992244046775898 ) ) ;
#52189=CARTESIAN_POINT ( 'NONE',  ( 0.9448818897637802916, -0.1870078740157479769, 0.3641732283464567677 ) ) ;
#52191=CARTESIAN_POINT ( 'NONE',  ( 0.4199475065616805614, 0.2306618581243848609, 0.2411417322834645549 ) ) ;
#52193=CARTESIAN_POINT ( 'NONE',  ( -0.8792650918635160906, 0.05413385826771626580, -0.4176697321401330321 ) ) ;
#52195=CARTESIAN_POINT ( 'NONE',  ( 1.535433070866142335, -0.5511811023622047445, 6.969142054262312111E-17 ) ) ;
#52196=CARTESIAN_POINT ( 'NONE',  ( 0.4461942257217856311, 0.2306618581243847221, -0.2411417322834647770 ) ) ;
#52197=CARTESIAN_POINT ( 'NONE',  ( 0.1706036745406830368, -0.4281496062992127816, -0.4176697321401328100 ) ) ;
#52199=CARTESIAN_POINT ( 'NONE',  ( -0.02624671916010428221, 0.1283753931104746893, -0.1820866141732285504 ) ) ;
#52200=CARTESIAN_POINT ( 'NONE',  ( 0.9514435695538062676, -0.3162353388693409650, -0.4822834645669289433 ) ) ;
#52201=CARTESIAN_POINT ( 'NONE',  ( -0.1377952755905504645, 0.07958543189024085140, 0.2665933059059887866 ) ) ;
#52202=CARTESIAN_POINT ( 'NONE',  ( -0.6102362204724400829, -0.5400638737290845981, -0.3530559997133363437 ) ) ;
#52204=CARTESIAN_POINT ( 'NONE',  ( -0.2821522309711278487, 0.2952755905511811885, 0.1292274648535926551 ) ) ;
#52206=CARTESIAN_POINT ( 'NONE',  ( -1.095800524934382292, -0.3162353388693409650, -0.4822834645669289433 ) ) ;
#52207=CARTESIAN_POINT ( 'NONE',  ( -0.5249343832020990641, -0.5023911411419708095, -0.1820866141732282451 ) ) ;
#52208=CARTESIAN_POINT ( 'NONE',  ( 0.03937007874015806264, 0.2952755905511811885, 0.000000000000000000 ) ) ;
#52209=CARTESIAN_POINT ( 'NONE',  ( -1.154855643044618851, -0.6046776061558809534, -0.2411417322834644161 ) ) ;
#52210=CARTESIAN_POINT ( 'NONE',  ( -0.8595800524934373854, -0.05778040916215522460, 0.4822834645669289988 ) ) ;
#52213=CARTESIAN_POINT ( 'NONE',  ( 1.666666666666667185, 0.05413385826771666132, 0.4176697321401328100 ) ) ;
#52214=CARTESIAN_POINT ( 'NONE',  ( 0.8202099737532813073, 0.2952755905511811885, 0.1292274648535926551 ) ) ;
#52215=CARTESIAN_POINT ( 'NONE',  ( 1.246719160104987623, 0.05413385826771626580, -0.4176697321401330321 ) ) ;
#52217=CARTESIAN_POINT ( 'NONE',  ( -1.548556430446193399, -0.6046776061558809534, -0.2411417322834644161 ) ) ;
#52218=CARTESIAN_POINT ( 'NONE',  ( -1.417322834645668772, -0.1870078740157479769, 0.4822834645669291653 ) ) ;
#52222=CARTESIAN_POINT ( 'NONE',  ( -0.06561679790026180015, -0.004921259842519576551, 0.3153832671262227771 ) ) ;
#52224=ORIENTED_EDGE ( 'NONE', *, *, #64962, .T. ) ;
#52225=CARTESIAN_POINT ( 'NONE',  ( 0.1181102362204730916, -0.6692913385826771977, 8.415575281601705876E-17 ) ) ;
#52226=CARTESIAN_POINT ( 'NONE',  ( 0.2099737532808405305, 0.2306618581243847221, -0.2411417322834647770 ) ) ;
#52229=CARTESIAN_POINT ( 'NONE',  ( -0.7545931758530176614, -0.5511811023622048555, -0.09757992244046775898 ) ) ;
#52231=CARTESIAN_POINT ( 'NONE',  ( 0.7808398950131241190, -0.05778040916215560624, -0.4822834645669293319 ) ) ;
#52232=CARTESIAN_POINT ( 'NONE',  ( 1.135170603674541256, 0.1771653543307087630, 0.09757992244046791164 ) ) ;
#52233=CARTESIAN_POINT ( 'NONE',  ( -0.3871391076115476282, -0.05778040916215522460, 0.4822834645669289988 ) ) ;
#52235=CARTESIAN_POINT ( 'NONE',  ( -0.6233595800524928121, -0.3162353388693409650, -0.4822834645669289433 ) ) ;
#52236=CARTESIAN_POINT ( 'NONE',  ( 2.795275590551181910, 1.726086921369709426, 0.000000000000000000 ) ) ;
#52237=CARTESIAN_POINT ( 'NONE',  ( 1.174540682414699111, -0.3162353388693405765, 0.4822834645669290543 ) ) ;
#52241=CARTESIAN_POINT ( 'NONE',  ( 0.1706036745406830368, -0.4281496062992127816, -0.4176697321401328100 ) ) ;
#52242=ORIENTED_EDGE ( 'NONE', *, *, #77894, .T. ) ;
#52243=CARTESIAN_POINT ( 'NONE',  ( -0.6692913385826764205, -0.6692913385826771977, 8.415575281601705876E-17 ) ) ;
#52244=CARTESIAN_POINT ( 'NONE',  ( 1.227034120734908917, -0.6692913385826771977, 0.1292274648535927661 ) ) ;
#52245=CARTESIAN_POINT ( 'NONE',  ( 1.253280839895013710, -0.3162353388693405765, 0.4822834645669290543 ) ) ;
#52246=CARTESIAN_POINT ( 'NONE',  ( 0.4461942257217855201, -0.6046776061558807314, 0.2411417322834647770 ) ) ;
#52247=CARTESIAN_POINT ( 'NONE',  ( -0.2296587926509179312, -0.05778040916215522460, 0.4822834645669289988 ) ) ;
#52249=CARTESIAN_POINT ( 'NONE',  ( -1.148293963254592542, -0.6692913385826773087, -0.1292274648535924053 ) ) ;
#52250=CARTESIAN_POINT ( 'NONE',  ( 0.01312335958005323398, -0.4281496062992127816, -0.4176697321401328100 ) ) ;
#52251=CARTESIAN_POINT ( 'NONE',  ( 0.01312335958005323398, -0.3690944881889765550, -0.3153832671262227771 ) ) ;
#52252=CARTESIAN_POINT ( 'NONE',  ( 1.581364829396326277, -0.3162353388693409650, -0.4822834645669289433 ) ) ;
#52253=CARTESIAN_POINT ( 'NONE',  ( 1.318897637795276356, -0.5400638737290844871, 0.3530559997133364547 ) ) ;
#52254=CARTESIAN_POINT ( 'NONE',  ( -0.4199475065616791736, 0.2306618581243847221, -0.2411417322834647770 ) ) ;
#52256=CARTESIAN_POINT ( 'NONE',  ( 1.043307086614173818, -0.5400638737290845981, -0.3530559997133363437 ) ) ;
#52258=ORIENTED_EDGE ( 'NONE', *, *, #2422, .T. ) ;
#52259=CARTESIAN_POINT ( 'NONE',  ( 0.3018372703412079971, 0.05413385826771626580, -0.4176697321401330321 ) ) ;
#52260=CARTESIAN_POINT ( 'NONE',  ( -0.09842519685039295696, 0.07958543189024071263, -0.2665933059059888421 ) ) ;
#52261=CARTESIAN_POINT ( 'NONE',  ( 1.391076115485564868, 0.1283753931104746893, -0.1820866141732285504 ) ) ;
#52262=CARTESIAN_POINT ( 'NONE',  ( -0.9055118110236215490, 0.2066929133858268208, 0.000000000000000000 ) ) ;
#52264=CARTESIAN_POINT ( 'NONE',  ( 1.535433070866142558, 0.1771653543307087630, 0.000000000000000000 ) ) ;
#52266=CARTESIAN_POINT ( 'NONE',  ( 1.076115485564305141, -0.6046776061558807314, 0.2411417322834647770 ) ) ;
#52268=CARTESIAN_POINT ( 'NONE',  ( 0.1377952755905518800, -0.5400638737290844871, 0.3530559997133364547 ) ) ;
#52270=CARTESIAN_POINT ( 'NONE',  ( -1.620734908136482577, -0.6692913385826773087, -0.1292274648535924053 ) ) ;
#52271=CARTESIAN_POINT ( 'NONE',  ( -0.1837270341207343505, -0.6046776061558807314, 0.2411417322834647770 ) ) ;
#52274=CARTESIAN_POINT ( 'NONE',  ( 1.509186351706037543, 0.05413385826771666132, 0.4176697321401328100 ) ) ;
#52275=CARTESIAN_POINT ( 'NONE',  ( 0.6824146981627303710, 0.2306618581243847221, -0.2411417322834647770 ) ) ;
#52276=CARTESIAN_POINT ( 'NONE',  ( 1.069553805774278832, 0.1771653543307087075, -0.09757992244046823083 ) ) ;
#52277=CARTESIAN_POINT ( 'NONE',  ( -0.05905511811023545637, 0.1660481256975885056, 0.3530559997133364547 ) ) ;
#52278=CARTESIAN_POINT ( 'NONE',  ( 0.8595800524934390507, -0.2845877964562159024, 0.3641732283464567677 ) ) ;
#52279=CARTESIAN_POINT ( 'NONE',  ( -1.253280839895012377, -0.3162353388693409650, -0.4822834645669289433 ) ) ;
#52281=CARTESIAN_POINT ( 'NONE',  ( 1.056430446194226658, 0.2952755905511811885, 0.1292274648535926551 ) ) ;
#52283=CARTESIAN_POINT ( 'NONE',  ( 0.5511811023622055217, -0.1870078740157479769, 0.4822834645669291653 ) ) ;
#52286=CARTESIAN_POINT ( 'NONE',  ( 0.6496062992125991586, 0.07958543189024085140, 0.2665933059059887866 ) ) ;
#52287=B_SPLINE_CURVE_WITH_KNOTS ( 'NONE', 3,
 ( #54504, #74303, #67162, #55743 ),
 .UNSPECIFIED., .F., .F.,
 ( 4, 4 ),
 ( 3.210432057682506253E-07, 0.001287787053612018777 ),
 .UNSPECIFIED. ) ;
#52288=CARTESIAN_POINT ( 'NONE',  ( 0.6692913385826778638, -0.6692913385826771977, 8.415575281601705876E-17 ) ) ;
#52289=CARTESIAN_POINT ( 'NONE',  ( 1.653543307086614789, -0.1870078740157479769, 0.3641732283464567677 ) ) ;
#52290=CARTESIAN_POINT ( 'NONE',  ( -0.8989501312335946848, 0.1771653543307087075, -0.09757992244046823083 ) ) ;
#52291=CARTESIAN_POINT ( 'NONE',  ( -0.8267716535433065062, -0.6692913385826771977, 8.415575281601705876E-17 ) ) ;
#52292=CARTESIAN_POINT ( 'NONE',  ( -1.437007874015747477, -0.5400638737290844871, 0.3530559997133364547 ) ) ;
#52293=CARTESIAN_POINT ( 'NONE',  ( 0.7808398950131241190, -0.05778040916215560624, -0.4822834645669293319 ) ) ;
#52294=CARTESIAN_POINT ( 'NONE',  ( -1.555118110236219930, -0.4536011799217368745, -0.2665933059059886201 ) ) ;
#52296=CARTESIAN_POINT ( 'NONE',  ( 1.023622047244095112, -0.1870078740157480879, -0.4822834645669291653 ) ) ;
#52299=CARTESIAN_POINT ( 'NONE',  ( 1.489501312335958172, -0.3162353388693405765, 0.4822834645669290543 ) ) ;
#52300=CARTESIAN_POINT ( 'NONE',  ( -1.377952755905511140, 0.1771653543307087630, 0.000000000000000000 ) ) ;
#52301=CARTESIAN_POINT ( 'NONE',  ( 1.043307086614173818, 0.07958543189024085140, 0.2665933059059887866 ) ) ;
#52302=CARTESIAN_POINT ( 'NONE',  ( -1.102362204724408601, -0.1870078740157480601, -0.3641732283464567677 ) ) ;
#52303=CARTESIAN_POINT ( 'NONE',  ( -0.6036745406824141069, -0.5023911411419708095, -0.1820866141732282451 ) ) ;
#52305=CARTESIAN_POINT ( 'NONE',  ( 0.7414698162729663755, -0.5511811023622048555, -0.09757992244046775898 ) ) ;
#52306=CARTESIAN_POINT ( 'NONE',  ( 0.4921259842519691285, -0.5400638737290845981, -0.3530559997133363437 ) ) ;
#52307=CARTESIAN_POINT ( 'NONE',  ( 1.194225721784777594, -0.4281496062992127816, -0.4176697321401328100 ) ) ;
#52308=CARTESIAN_POINT ( 'NONE',  ( -0.09842519685039295696, -0.5400638737290844871, 0.3530559997133364547 ) ) ;
#52309=CARTESIAN_POINT ( 'NONE',  ( 0.7217847769028878924, -0.3690944881889765550, -0.3153832671262227771 ) ) ;
#52310=CARTESIAN_POINT ( 'NONE',  ( 1.233595800524935227, -0.6046776061558807314, 0.2411417322834647770 ) ) ;
#52312=CARTESIAN_POINT ( 'NONE',  ( -0.3608923884514428360, -0.6692913385826773087, -0.1292274648535924053 ) ) ;
#52315=CARTESIAN_POINT ( 'NONE',  ( 0.07217847769028949700, -0.05778040916215560624, -0.4822834645669293319 ) ) ;
#52316=CARTESIAN_POINT ( 'NONE',  ( -0.2952755905511803003, -0.5400638737290845981, -0.3530559997133363437 ) ) ;
#52317=CARTESIAN_POINT ( 'NONE',  ( -0.1443569553805768291, 0.05413385826771666132, 0.4176697321401328100 ) ) ;
#52324=CARTESIAN_POINT ( 'NONE',  ( -1.089238845144356427, -0.004921259842519576551, 0.3153832671262227771 ) ) ;
#52326=CARTESIAN_POINT ( 'NONE',  ( -1.036745406824146176, 0.05413385826771626580, -0.4176697321401330321 ) ) ;
#52328=CARTESIAN_POINT ( 'NONE',  ( 0.2296587926509192634, -0.3162353388693405765, 0.4822834645669290543 ) ) ;
#52329=CARTESIAN_POINT ( 'NONE',  ( -0.5380577427821514602, -0.3690944881889765550, -0.3153832671262227771 ) ) ;
#52330=CARTESIAN_POINT ( 'NONE',  ( 1.135170603674541256, 0.2952755905511811885, 0.1292274648535926551 ) ) ;
#52331=CARTESIAN_POINT ( 'NONE',  ( 0.4133858267716541968, -0.5400638737290845981, -0.3530559997133363437 ) ) ;
#52335=CARTESIAN_POINT ( 'NONE',  ( 1.299212598425197429, -0.6692913385826771977, 8.415575281601705876E-17 ) ) ;
#52336=CARTESIAN_POINT ( 'NONE',  ( 0.6364829396325465405, -0.05778040916215522460, 0.4822834645669289988 ) ) ;
#52337=CARTESIAN_POINT ( 'NONE',  ( 0.2427821522309716595, -0.3162353388693409650, -0.4822834645669289433 ) ) ;
#52338=CARTESIAN_POINT ( 'NONE',  ( 1.312335958005249825, 0.2306618581243847221, -0.2411417322834647770 ) ) ;
#52339=CARTESIAN_POINT ( 'NONE',  ( 0.9448818897637802916, -0.1870078740157480879, -0.4822834645669291653 ) ) ;
#52341=CARTESIAN_POINT ( 'NONE',  ( -0.1049868766404193215, 0.2306618581243847221, -0.2411417322834647770 ) ) ;
#52342=CARTESIAN_POINT ( 'NONE',  ( 0.9120734908136490793, 0.2952755905511810774, -0.1292274648535930714 ) ) ;
#52343=CARTESIAN_POINT ( 'NONE',  ( 0.3937007874015754361, -0.1870078740157479769, 0.4822834645669291653 ) ) ;
#52344=CARTESIAN_POINT ( 'NONE',  ( 0.9580052493438327987, -0.3690944881889765550, -0.3153832671262227771 ) ) ;
#52345=CARTESIAN_POINT ( 'NONE',  ( -0.8398950131233589023, -0.6046776061558809534, -0.2411417322834644161 ) ) ;
#52346=CARTESIAN_POINT ( 'NONE',  ( -1.332020997375327642, -0.3162353388693409650, -0.4822834645669289433 ) ) ;
#52347=CARTESIAN_POINT ( 'NONE',  ( 0.6692913385826777528, 0.2952755905511811885, 0.000000000000000000 ) ) ;
#52350=ORIENTED_EDGE ( 'NONE', *, *, #45382, .F. ) ;
#52353=CARTESIAN_POINT ( 'NONE',  ( 1.581364829396326277, -0.3162353388693409650, -0.4822834645669289433 ) ) ;
#52354=CARTESIAN_POINT ( 'NONE',  ( 0.9776902887139113929, 0.1771653543307087630, 0.09757992244046791164 ) ) ;
#52355=CARTESIAN_POINT ( 'NONE',  ( -0.6575345472709128725, 1.929133858267715773, -0.5309055118110235227 ) ) ;
#52360=CARTESIAN_POINT ( 'NONE',  ( -1.010498687664041384, -0.004921259842519576551, 0.3153832671262227771 ) ) ;
#52361=CARTESIAN_POINT ( 'NONE',  ( -1.620734908136482577, -0.5511811023622048555, -0.09757992244046775898 ) ) ;
#52363=CARTESIAN_POINT ( 'NONE',  ( -0.4461942257217840213, 0.2306618581243848609, 0.2411417322834645549 ) ) ;
#52364=CARTESIAN_POINT ( 'NONE',  ( 1.207349081364829990, -0.6046776061558809534, -0.2411417322834644161 ) ) ;
#52365=ORIENTED_EDGE ( 'NONE', *, *, #3407, .F. ) ;
#52366=CARTESIAN_POINT ( 'NONE',  ( -1.574803149606298636, -0.1870078740157479769, 0.4822834645669291653 ) ) ;
#52368=CARTESIAN_POINT ( 'NONE',  ( 1.614173228346456712, 1.267785121476991517, 0.1372047244094478646 ) ) ;
#52369=CARTESIAN_POINT ( 'NONE',  ( -0.8661417322834640276, -0.1870078740157479769, 0.3641732283464567677 ) ) ;
#52370=CARTESIAN_POINT ( 'NONE',  ( 1.614173228346456712, 0.9921945702958890889, 0.1372047244094478646 ) ) ;
#52371=CARTESIAN_POINT ( 'NONE',  ( 0.5380577427821529035, -0.4281496062992124485, 0.4176697321401328655 ) ) ;
#52372=ORIENTED_EDGE ( 'NONE', *, *, #52141, .F. ) ;
#52375=CARTESIAN_POINT ( 'NONE',  ( 1.351706036745407680, 0.05413385826771666132, 0.4176697321401328100 ) ) ;
#52376=CARTESIAN_POINT ( 'NONE',  ( -1.686351706036744558, 0.2952755905511810774, -0.1292274648535930714 ) ) ;
#52378=CARTESIAN_POINT ( 'NONE',  ( -1.003937007874015297, -0.4536011799217368745, -0.2665933059059886201 ) ) ;
#52379=CARTESIAN_POINT ( 'NONE',  ( -1.404199475065615932, -0.3690944881889765550, -0.3153832671262227771 ) ) ;
#52381=CARTESIAN_POINT ( 'NONE',  ( 0.2887139107611556010, -0.6046776061558807314, 0.2411417322834647770 ) ) ;
#52382=CARTESIAN_POINT ( 'NONE',  ( -1.115485564304461219, -0.004921259842519870586, -0.3153832671262229437 ) ) ;
#52383=CARTESIAN_POINT ( 'NONE',  ( -0.02624671916010428221, -0.5023911411419708095, 0.1820866141732285504 ) ) ;
#52384=CARTESIAN_POINT ( 'NONE',  ( -0.4855643044619415427, -0.4281496062992124485, 0.4176697321401328655 ) ) ;
#52385=CARTESIAN_POINT ( 'NONE',  ( -1.082677165354329896, -0.4536011799217368745, -0.2665933059059886201 ) ) ;
#52387=CARTESIAN_POINT ( 'NONE',  ( 0.7742782152230978099, -0.4281496062992124485, 0.4176697321401328655 ) ) ;
#52388=CARTESIAN_POINT ( 'NONE',  ( -1.351706036745406347, -0.4281496062992124485, 0.4176697321401328655 ) ) ;
#52390=CARTESIAN_POINT ( 'NONE',  ( -0.6036745406824141069, 0.2306618581243848609, 0.2411417322834645549 ) ) ;
#52391=CARTESIAN_POINT ( 'NONE',  ( -0.1115485564304456306, 0.1771653543307087075, -0.09757992244046823083 ) ) ;
#52392=CARTESIAN_POINT ( 'NONE',  ( -1.240157480314959759, -0.5400638737290845981, -0.3530559997133363437 ) ) ;
#52393=CARTESIAN_POINT ( 'NONE',  ( 0.8398950131233602345, -0.5023911411419708095, 0.1820866141732285504 ) ) ;
#52394=CARTESIAN_POINT ( 'NONE',  ( -0.2821522309711278487, 0.1771653543307087630, 0.09757992244046791164 ) ) ;
#52395=CARTESIAN_POINT ( 'NONE',  ( -0.6955380577427815458, -0.4281496062992127816, -0.4176697321401328100 ) ) ;
#52396=CARTESIAN_POINT ( 'NONE',  ( -1.056430446194224881, 0.2952755905511810774, -0.1292274648535930714 ) ) ;
#52397=CARTESIAN_POINT ( 'NONE',  ( -1.607611548556429737, 0.2952755905511810774, -0.1292274648535930714 ) ) ;
#52399=CARTESIAN_POINT ( 'NONE',  ( 1.358267716535433323, 0.07958543189024085140, 0.2665933059059887866 ) ) ;
#52400=CARTESIAN_POINT ( 'NONE',  ( 0.2362204724409456558, -0.1870078740157479769, 0.4822834645669291653 ) ) ;
#52401=CARTESIAN_POINT ( 'NONE',  ( -1.377952755905511140, -0.6692913385826771977, 8.415575281601705876E-17 ) ) ;
#52402=CARTESIAN_POINT ( 'NONE',  ( -1.686351706036744558, 0.2952755905511810774, -0.1292274648535930714 ) ) ;
#52403=EDGE_LOOP ( 'NONE', ( #27729, #45390, #41091, #44947 ) ) ;
#52405=CARTESIAN_POINT ( 'NONE',  ( -1.076115485564303809, -0.5023911411419708095, -0.1820866141732282451 ) ) ;
#52406=CARTESIAN_POINT ( 'NONE',  ( 0.7939632545931766261, -0.05778040916215522460, 0.4822834645669289988 ) ) ;
#52407=CARTESIAN_POINT ( 'NONE',  ( -1.233595800524933894, 0.1283753931104748280, 0.1820866141732283561 ) ) ;
#52409=CARTESIAN_POINT ( 'NONE',  ( -1.220472440944881054, 0.2952755905511811885, 0.000000000000000000 ) ) ;
#52410=CARTESIAN_POINT ( 'NONE',  ( 0.8464566929133866546, -0.5400638737290844871, 0.3530559997133364547 ) ) ;
#52411=CARTESIAN_POINT ( 'NONE',  ( 0.4658792650918641698, -0.05778040916215560624, -0.4822834645669293319 ) ) ;
#52412=CARTESIAN_POINT ( 'NONE',  ( 1.187664041994751285, -0.3162353388693409650, -0.4822834645669289433 ) ) ;
#52413=CARTESIAN_POINT ( 'NONE',  ( -1.607611548556429737, -0.5511811023622046335, 0.09757992244046803654 ) ) ;
#52418=CARTESIAN_POINT ( 'NONE',  ( 0.9514435695538062676, -0.2845877964562161244, -0.3641732283464567121 ) ) ;
#52419=CARTESIAN_POINT ( 'NONE',  ( 0.1509186351706042484, -0.2845877964562159024, 0.3641732283464567677 ) ) ;
#52420=CARTESIAN_POINT ( 'NONE',  ( 0.1181102362204730916, -0.6692913385826771977, 8.415575281601705876E-17 ) ) ;
#52421=CARTESIAN_POINT ( 'NONE',  ( 1.128608923884514947, 0.2306618581243848609, 0.2411417322834645549 ) ) ;
#52423=CARTESIAN_POINT ( 'NONE',  ( 0.2099737532808405305, -0.5023911411419708095, 0.1820866141732285504 ) ) ;
#52424=CARTESIAN_POINT ( 'NONE',  ( -0.5839895013123351797, -0.6692913385826771977, 0.1292274648535927661 ) ) ;
#52425=CARTESIAN_POINT ( 'NONE',  ( -1.476377952755905110, 0.1660481256975885056, 0.3530559997133364547 ) ) ;
#52426=CARTESIAN_POINT ( 'NONE',  ( 0.7808398950131241190, -0.05778040916215560624, -0.4822834645669293319 ) ) ;
#52431=CARTESIAN_POINT ( 'NONE',  ( -1.240157480314959759, 0.1660481256975885056, 0.3530559997133364547 ) ) ;
#52433=CARTESIAN_POINT ( 'NONE',  ( -0.8858267716535425107, -0.4536011799217367080, 0.2665933059059888421 ) ) ;
#52434=CARTESIAN_POINT ( 'NONE',  ( -1.240157480314959759, -0.5400638737290845981, -0.3530559997133363437 ) ) ;
#52437=CARTESIAN_POINT ( 'NONE',  ( 1.620734908136483465, -0.6692913385826771977, 0.1292274648535927661 ) ) ;
#52438=CARTESIAN_POINT ( 'NONE',  ( -1.286089238845143479, -0.6046776061558807314, 0.2411417322834647770 ) ) ;
#52439=CARTESIAN_POINT ( 'NONE',  ( 0.2887139107611556010, -0.6046776061558807314, 0.2411417322834647770 ) ) ;
#52440=CARTESIAN_POINT ( 'NONE',  ( -1.122047244094487306, 0.1660481256975883668, -0.3530559997133364547 ) ) ;
#52443=CARTESIAN_POINT ( 'NONE',  ( 0.4790026246719167324, -0.05778040916215522460, 0.4822834645669289988 ) ) ;
#52445=CARTESIAN_POINT ( 'NONE',  ( -0.7414698162729651543, -0.5511811023622046335, 0.09757992244046803654 ) ) ;
#52448=VERTEX_POINT ( 'NONE', #9383 ) ;
#52449=CARTESIAN_POINT ( 'NONE',  ( -0.6418543022643059537, 1.311896022878452671E-15, -0.3627985898453513491 ) ) ;
#52450=CARTESIAN_POINT ( 'NONE',  ( -1.312335958005248715, -0.6046776061558809534, -0.2411417322834644161 ) ) ;
#52451=CARTESIAN_POINT ( 'NONE',  ( -1.161417322834644716, 0.1660481256975885056, 0.3530559997133364547 ) ) ;
#52453=CARTESIAN_POINT ( 'NONE',  ( -1.574803149606298636, -0.1870078740157479769, 0.4822834645669291653 ) ) ;
#52454=CARTESIAN_POINT ( 'NONE',  ( -1.266404199475064773, -0.3162353388693405765, 0.4822834645669290543 ) ) ;
#52455=CARTESIAN_POINT ( 'NONE',  ( -1.253280839895012377, -0.3162353388693409650, -0.4822834645669289433 ) ) ;
#52460=CARTESIAN_POINT ( 'NONE',  ( 0.01968503937007957949, -0.4536011799217368745, -0.2665933059059886201 ) ) ;
#52461=CARTESIAN_POINT ( 'NONE',  ( 0.5419760673063064305, 1.535433070866141447, -0.4915354330708657793 ) ) ;
#52463=CARTESIAN_POINT ( 'NONE',  ( -0.3346456692913377662, -0.4536011799217367080, 0.2665933059059888421 ) ) ;
#52464=CARTESIAN_POINT ( 'NONE',  ( -0.9908136482939626788, 0.2952755905511811885, 0.1292274648535926551 ) ) ;
#52465=CARTESIAN_POINT ( 'NONE',  ( 0.8136482939632553313, 0.2306618581243848609, 0.2411417322834645549 ) ) ;
#52466=CARTESIAN_POINT ( 'NONE',  ( -0.6627296587926501115, 0.2952755905511810774, -0.1292274648535930714 ) ) ;
#52467=VERTEX_POINT ( 'NONE', #64022 ) ;
#52468=ORIENTED_EDGE ( 'NONE', *, *, #37540, .T. ) ;
#52470=CARTESIAN_POINT ( 'NONE',  ( -0.9448818897637790704, -0.1870078740157480879, -0.4822834645669291653 ) ) ;
#52471=CARTESIAN_POINT ( 'NONE',  ( 1.036745406824147508, -0.4281496062992127816, -0.4176697321401328100 ) ) ;
#52473=CARTESIAN_POINT ( 'NONE',  ( -1.725721784776902190, -0.05778040916215522460, 0.4822834645669289988 ) ) ;
#52478=CARTESIAN_POINT ( 'NONE',  ( -0.4658792650918627265, -0.3162353388693409650, -0.4822834645669289433 ) ) ;
#52479=CARTESIAN_POINT ( 'NONE',  ( -1.364829396325458521, -0.5023911411419708095, 0.1820866141732285504 ) ) ;
#52480=CARTESIAN_POINT ( 'NONE',  ( -0.8792650918635160906, 0.05413385826771626580, -0.4176697321401330321 ) ) ;
#52482=CARTESIAN_POINT ( 'NONE',  ( -1.351706036745406347, 0.05413385826771626580, -0.4176697321401330321 ) ) ;
#52484=CARTESIAN_POINT ( 'NONE',  ( -0.8070866141732276899, -0.5400638737290844871, 0.3530559997133364547 ) ) ;
#52485=CARTESIAN_POINT ( 'NONE',  ( -0.2230971128608915943, -0.4281496062992127816, -0.4176697321401328100 ) ) ;
#52487=CARTESIAN_POINT ( 'NONE',  ( 0.7808398950131240079, -0.2845877964562159024, 0.3641732283464567677 ) ) ;
#52488=DIRECTION ( 'NONE',  ( 0.000000000000000000, 0.000000000000000000, 1.000000000000000000 ) ) ;
#52489=CARTESIAN_POINT ( 'NONE',  ( 0.2952755905511819101, 0.07958543189024071263, -0.2665933059059888421 ) ) ;
#52490=CARTESIAN_POINT ( 'NONE',  ( 1.423884514435696191, -0.08942795157527998196, 0.3641732283464567121 ) ) ;
#52491=CARTESIAN_POINT ( 'NONE',  ( 1.528871391076116026, -0.6692913385826773087, -0.1292274648535924053 ) ) ;
#52492=CARTESIAN_POINT ( 'NONE',  ( 8.195543980992789655E-16, -0.1870078740157480601, -0.3641732283464567677 ) ) ;
#52494=CARTESIAN_POINT ( 'NONE',  ( -1.417322834645668772, -0.1870078740157480879, -0.4822834645669291653 ) ) ;
#52495=CARTESIAN_POINT ( 'NONE',  ( 1.233595800524935227, -0.6046776061558807314, 0.2411417322834647770 ) ) ;
#52497=CARTESIAN_POINT ( 'NONE',  ( -0.4002624671916004129, -0.2845877964562159024, 0.3641732283464567677 ) ) ;
#52498=PLANE ( 'NONE',  #17121 ) ;
#52499=CARTESIAN_POINT ( 'NONE',  ( 0.2624671916010504757, 0.2306618581243848609, 0.2411417322834645549 ) ) ;
#52501=CARTESIAN_POINT ( 'NONE',  ( 0.9186351706036751663, -0.5023911411419708095, 0.1820866141732285504 ) ) ;
#52502=CARTESIAN_POINT ( 'NONE',  ( 0.1968503937007881344, 0.1771653543307087630, 0.000000000000000000 ) ) ;
#52503=CARTESIAN_POINT ( 'NONE',  ( -0.4724409448818890911, -0.1870078740157480879, -0.4822834645669291653 ) ) ;
#52504=CARTESIAN_POINT ( 'NONE',  ( -1.620734908136482577, -0.6692913385826773087, -0.1292274648535924053 ) ) ;
#52505=CARTESIAN_POINT ( 'NONE',  ( -0.7742782152230962556, -0.3690944881889765550, -0.3153832671262227771 ) ) ;
#52507=CARTESIAN_POINT ( 'NONE',  ( 0.4986876640419954376, -0.6046776061558809534, -0.2411417322834644161 ) ) ;
#52509=CARTESIAN_POINT ( 'NONE',  ( -0.9317585301837263412, -0.4281496062992127816, -0.4176697321401328100 ) ) ;
#52512=CARTESIAN_POINT ( 'NONE',  ( 0.3083989501312343062, -0.2845877964562159024, 0.3641732283464567677 ) ) ;
#52513=CARTESIAN_POINT ( 'NONE',  ( -0.7611548556430438595, -0.6046776061558809534, -0.2411417322834644161 ) ) ;
#52514=CARTESIAN_POINT ( 'NONE',  ( -0.9973753280839886548, 0.2306618581243848609, 0.2411417322834645549 ) ) ;
#52515=CARTESIAN_POINT ( 'NONE',  ( -1.338582677165353729, -0.1870078740157479769, 0.3641732283464567677 ) ) ;
#52516=CARTESIAN_POINT ( 'NONE',  ( 1.220472440944881942, 0.000000000000000000, -0.5309055118110238558 ) ) ;
#52517=CARTESIAN_POINT ( 'NONE',  ( -0.9383202099737524282, -0.2845877964562161244, -0.3641732283464567121 ) ) ;
#52518=CARTESIAN_POINT ( 'NONE',  ( -1.604771003085129655, 1.871396828306225002, 0.1466069496707748665 ) ) ;
#52519=CARTESIAN_POINT ( 'NONE',  ( 1.482939632545932307, 0.05413385826771626580, -0.4176697321401330321 ) ) ;
#52524=VECTOR ( 'NONE', #14267, 39.37007874015748143 ) ;
#52526=CARTESIAN_POINT ( 'NONE',  ( 1.469816272965879911, 0.1283753931104746893, -0.1820866141732285504 ) ) ;
#52527=CARTESIAN_POINT ( 'NONE',  ( -1.299212598425196097, -0.6692913385826771977, 8.415575281601705876E-17 ) ) ;
#52528=CARTESIAN_POINT ( 'NONE',  ( 1.194225721784777594, -0.4281496062992127816, -0.4176697321401328100 ) ) ;
#52530=CARTESIAN_POINT ( 'NONE',  ( 1.666666666666667185, -0.004921259842519576551, 0.3153832671262227771 ) ) ;
#52531=CARTESIAN_POINT ( 'NONE',  ( 0.6102362204724416372, 0.1660481256975883668, -0.3530559997133364547 ) ) ;
#52532=CARTESIAN_POINT ( 'NONE',  ( -0.2296587926509179312, -0.05778040916215522460, 0.4822834645669289988 ) ) ;
#52533=CARTESIAN_POINT ( 'NONE',  ( -0.6975637601868556192, 5.991678263669262536E-15, 0.3954985857520036951 ) ) ;
#52535=CARTESIAN_POINT ( 'NONE',  ( 0.7086614173228352742, -0.1870078740157480601, -0.3641732283464567677 ) ) ;
#52539=ORIENTED_EDGE ( 'NONE', *, *, #73492, .F. ) ;
#52540=CARTESIAN_POINT ( 'NONE',  ( -0.03280839895013062252, -0.6692913385826771977, 0.1292274648535927661 ) ) ;
#52541=CARTESIAN_POINT ( 'NONE',  ( 1.443569553805774897, 0.2306618581243848609, 0.2411417322834645549 ) ) ;
#52542=CARTESIAN_POINT ( 'NONE',  ( 0.4265091863517067594, 0.2952755905511811885, 0.1292274648535926551 ) ) ;
#52543=CARTESIAN_POINT ( 'NONE',  ( 1.253280839895013710, -0.05778040916215560624, -0.4822834645669293319 ) ) ;
#52544=CARTESIAN_POINT ( 'NONE',  ( -0.5577427821522301654, -0.3162353388693405765, 0.4822834645669290543 ) ) ;
#52545=CARTESIAN_POINT ( 'NONE',  ( 0.1115485564304467270, -0.6692913385826773087, -0.1292274648535924053 ) ) ;
#52546=CARTESIAN_POINT ( 'NONE',  ( 1.476377952755906220, 0.1660481256975883668, -0.3530559997133364547 ) ) ;
#52547=CARTESIAN_POINT ( 'NONE',  ( 1.194225721784777594, -0.4281496062992127816, -0.4176697321401328100 ) ) ;
#52548=CARTESIAN_POINT ( 'NONE',  ( 1.253280839895013710, -0.05778040916215560624, -0.4822834645669293319 ) ) ;
#52550=CARTESIAN_POINT ( 'NONE',  ( 0.4593175853018380828, -0.004921259842519870586, -0.3153832671262229437 ) ) ;
#52553=ORIENTED_EDGE ( 'NONE', *, *, #69619, .F. ) ;
#52554=CARTESIAN_POINT ( 'NONE',  ( -0.5577427821522301654, -0.08942795157528024563, -0.3641732283464568787 ) ) ;
#52555=CARTESIAN_POINT ( 'NONE',  ( -0.1968503937007867743, 0.2952755905511811885, 0.000000000000000000 ) ) ;
#52557=CARTESIAN_POINT ( 'NONE',  ( 0.2362204724409456558, -0.1870078740157480879, -0.4822834645669291653 ) ) ;
#52558=CARTESIAN_POINT ( 'NONE',  ( 0.1640419947506569498, -0.05778040916215522460, 0.4822834645669289988 ) ) ;
#52559=CARTESIAN_POINT ( 'NONE',  ( -0.6955380577427815458, 0.05413385826771666132, 0.4176697321401328100 ) ) ;
#52560=CARTESIAN_POINT ( 'NONE',  ( -0.7939632545931754048, -0.3162353388693405765, 0.4822834645669290543 ) ) ;
#52561=CARTESIAN_POINT ( 'NONE',  ( 1.443569553805774897, -0.5023911411419708095, -0.1820866141732282451 ) ) ;
#52562=CARTESIAN_POINT ( 'NONE',  ( -1.437007874015747477, 0.1660481256975883668, -0.3530559997133364547 ) ) ;
#52564=CARTESIAN_POINT ( 'NONE',  ( 1.017060367454068581, -0.08942795157528024563, -0.3641732283464568787 ) ) ;
#52565=CARTESIAN_POINT ( 'NONE',  ( 0.6364829396325465405, -0.3162353388693409650, -0.4822834645669289433 ) ) ;
#52566=CARTESIAN_POINT ( 'NONE',  ( 0.7414698162729663755, 0.2952755905511811885, 0.1292274648535926551 ) ) ;
#52569=CARTESIAN_POINT ( 'NONE',  ( 0.3264567959345339720, 2.726622551019859153E-15, 0.3791475997938225095 ) ) ;
#52572=CARTESIAN_POINT ( 'NONE',  ( -0.4396325459317579898, 0.2952755905511811885, 0.1292274648535926551 ) ) ;
#52575=CARTESIAN_POINT ( 'NONE',  ( -1.286089238845143479, 0.1283753931104746893, -0.1820866141732285504 ) ) ;
#52576=CARTESIAN_POINT ( 'NONE',  ( 1.364829396325459854, -0.6046776061558809534, -0.2411417322834644161 ) ) ;
#52577=CARTESIAN_POINT ( 'NONE',  ( 1.056430446194226658, 0.2952755905511811885, 0.1292274648535926551 ) ) ;
#52578=CARTESIAN_POINT ( 'NONE',  ( -0.08530183727034056085, -0.2845877964562159024, 0.3641732283464567677 ) ) ;
#52579=CARTESIAN_POINT ( 'NONE',  ( 0.6364829396325465405, -0.05778040916215522460, 0.4822834645669289988 ) ) ;
#52581=CARTESIAN_POINT ( 'NONE',  ( -0.01312335958005186876, -0.004921259842519870586, -0.3153832671262229437 ) ) ;
#52582=CARTESIAN_POINT ( 'NONE',  ( 0.01968503937007930540, 0.1660481256975885056, 0.3530559997133364547 ) ) ;
#52584=CARTESIAN_POINT ( 'NONE',  ( -1.167979002624671470, -0.4281496062992127816, -0.4176697321401328100 ) ) ;
#52585=CARTESIAN_POINT ( 'NONE',  ( 0.5380577427821529035, -0.004921259842519870586, -0.3153832671262229437 ) ) ;
#52587=CARTESIAN_POINT ( 'NONE',  ( 0.3477690288713918276, 0.2066929133858267931, 0.1054918080437490802 ) ) ;
#52588=CARTESIAN_POINT ( 'NONE',  ( -0.7808398950131225646, -0.05778040916215522460, 0.4822834645669289988 ) ) ;
#52590=CARTESIAN_POINT ( 'NONE',  ( -0.09842519685039295696, -0.4536011799217367080, 0.2665933059059888421 ) ) ;
#52592=CARTESIAN_POINT ( 'NONE',  ( -0.7939632545931754048, -0.3162353388693405765, 0.4822834645669290543 ) ) ;
#52593=CARTESIAN_POINT ( 'NONE',  ( -0.7939632545931750718, -0.05778040916215560624, -0.4822834645669293319 ) ) ;
#52594=CARTESIAN_POINT ( 'NONE',  ( 0.06561679790026316017, -0.4281496062992124485, 0.4176697321401328655 ) ) ;
#52598=CARTESIAN_POINT ( 'NONE',  ( -1.627296587926508442, -0.5023911411419708095, -0.1820866141732282451 ) ) ;
#52599=CARTESIAN_POINT ( 'NONE',  ( 0.5839895013123367340, 0.1771653543307087630, 0.09757992244046791164 ) ) ;
#52600=CARTESIAN_POINT ( 'NONE',  ( 1.325459317585302665, 0.05413385826771626580, -0.4176697321401330321 ) ) ;
#52601=CARTESIAN_POINT ( 'NONE',  ( -0.9317585301837263412, -0.004921259842519576551, 0.3153832671262227771 ) ) ;
#52602=CARTESIAN_POINT ( 'NONE',  ( -1.017060367454067249, -0.2845877964562161244, -0.3641732283464567121 ) ) ;
#52603=CARTESIAN_POINT ( 'NONE',  ( -0.7677165354330699465, -0.5400638737290845981, -0.3530559997133363437 ) ) ;
#52604=CARTESIAN_POINT ( 'NONE',  ( -0.2690288713910754526, 0.2952755905511810774, -0.1292274648535930714 ) ) ;
#52605=CARTESIAN_POINT ( 'NONE',  ( 0.6561679790026253567, -0.5023911411419708095, -0.1820866141732282451 ) ) ;
#52607=CARTESIAN_POINT ( 'NONE',  ( 0.9383202099737536495, -0.2845877964562159024, 0.3641732283464567677 ) ) ;
#52609=CARTESIAN_POINT ( 'NONE',  ( 0.2559055118110243332, 0.1660481256975885056, 0.3530559997133364547 ) ) ;
#52610=EDGE_CURVE ( 'NONE', #18339, #50999, #62797, .T. ) ;
#52612=CARTESIAN_POINT ( 'NONE',  ( -0.8661417322834640276, -0.1870078740157480879, -0.4822834645669291653 ) ) ;
#52614=CARTESIAN_POINT ( 'NONE',  ( 1.325459317585302665, -0.004921259842519870586, -0.3153832671262229437 ) ) ;
#52615=CARTESIAN_POINT ( 'NONE',  ( 0.2952755905511819101, 0.1660481256975883668, -0.3530559997133364547 ) ) ;
#52616=CARTESIAN_POINT ( 'NONE',  ( 0.2362204724409456558, -0.1870078740157479769, 0.4822834645669291653 ) ) ;
#52617=CARTESIAN_POINT ( 'NONE',  ( 0.03280839895013198948, -0.5511811023622048555, -0.09757992244046775898 ) ) ;
#52619=CARTESIAN_POINT ( 'NONE',  ( 0.09186351706036827158, -0.004921259842519576551, 0.3153832671262227771 ) ) ;
#52620=CARTESIAN_POINT ( 'NONE',  ( 0.7611548556430454138, 0.2306618581243847221, -0.2411417322834647770 ) ) ;
#52622=CARTESIAN_POINT ( 'NONE',  ( -0.9383202099737524282, -0.08942795157527998196, 0.3641732283464567121 ) ) ;
#52623=CARTESIAN_POINT ( 'NONE',  ( -0.6299212598425188991, -0.1870078740157480879, -0.4822834645669291653 ) ) ;
#52624=DIRECTION ( 'NONE',  ( 0.000000000000000000, 0.000000000000000000, -1.000000000000000000 ) ) ;
#52625=ORIENTED_EDGE ( 'NONE', *, *, #32904, .T. ) ;
#52626=CARTESIAN_POINT ( 'NONE',  ( -1.023622047244093558, -0.1870078740157479769, 0.4822834645669291653 ) ) ;
#52627=CARTESIAN_POINT ( 'NONE',  ( -0.9251968503937002541, 0.07958543189024085140, 0.2665933059059887866 ) ) ;
#52629=CARTESIAN_POINT ( 'NONE',  ( -0.06561679790026180015, -0.4281496062992127816, -0.4176697321401328100 ) ) ;
#52630=CARTESIAN_POINT ( 'NONE',  ( -1.541994750656167090, 0.2952755905511811885, 0.1292274648535926551 ) ) ;
#52631=CARTESIAN_POINT ( 'NONE',  ( -0.9448818897637790704, -0.1870078740157480879, -0.4822834645669291653 ) ) ;
#52634=CARTESIAN_POINT ( 'NONE',  ( 1.095800524934383846, -0.3162353388693405765, 0.4822834645669290543 ) ) ;
#52635=CARTESIAN_POINT ( 'NONE',  ( 1.200787401574803681, 0.1660481256975885056, 0.3530559997133364547 ) ) ;
#52637=CARTESIAN_POINT ( 'NONE',  ( -1.604771003085130321, 1.320215725944019258, 0.1466069496707743391 ) ) ;
#52638=CARTESIAN_POINT ( 'NONE',  ( -1.345144356955379816, -0.05778040916215560624, -0.4822834645669293319 ) ) ;
#52642=CARTESIAN_POINT ( 'NONE',  ( -0.2821522309711278487, -0.5511811023622048555, -0.09757992244046775898 ) ) ;
#52645=CARTESIAN_POINT ( 'NONE',  ( 0.3346456692913390985, 0.1660481256975885056, 0.3530559997133364547 ) ) ;
#52646=CARTESIAN_POINT ( 'NONE',  ( 0.09842519685039434474, -0.5400638737290845981, -0.3530559997133363437 ) ) ;
#52647=CARTESIAN_POINT ( 'NONE',  ( -0.7283464566929126471, -0.5400638737290844871, 0.3530559997133364547 ) ) ;
#52648=DIRECTION ( 'NONE',  ( 0.000000000000000000, 0.000000000000000000, 1.000000000000000000 ) ) ;
#52649=CARTESIAN_POINT ( 'NONE',  ( -0.7020997375328074108, -0.08942795157527998196, 0.3641732283464567121 ) ) ;
#52650=CARTESIAN_POINT ( 'NONE',  ( 0.5905511811023629321, 0.2952755905511811885, 0.000000000000000000 ) ) ;
#52651=CARTESIAN_POINT ( 'NONE',  ( 0.4265091863517067039, -0.5511811023622048555, -0.09757992244046775898 ) ) ;
#52652=CARTESIAN_POINT ( 'NONE',  ( -0.4921259842519677963, 0.1660481256975883668, -0.3530559997133364547 ) ) ;
#52654=CARTESIAN_POINT ( 'NONE',  ( -0.7152230971128602510, -0.3162353388693405765, 0.4822834645669290543 ) ) ;
#52656=CARTESIAN_POINT ( 'NONE',  ( 1.469816272965879911, -0.6046776061558807314, 0.2411417322834647770 ) ) ;
#52657=CARTESIAN_POINT ( 'NONE',  ( 1.581364829396326277, -0.2845877964562161244, -0.3641732283464567121 ) ) ;
#52660=CARTESIAN_POINT ( 'NONE',  ( -0.1902887139107604098, 0.2952755905511810774, -0.1292274648535930714 ) ) ;
#52661=ORIENTED_EDGE ( 'NONE', *, *, #23107, .T. ) ;
#52662=CARTESIAN_POINT ( 'NONE',  ( -1.332020997375327642, -0.3162353388693409650, -0.4822834645669289433 ) ) ;
#52663=CARTESIAN_POINT ( 'NONE',  ( 1.286089238845145033, 0.2306618581243848609, 0.2411417322834645549 ) ) ;
#52664=CARTESIAN_POINT ( 'NONE',  ( 1.272965879265092637, 0.05413385826771666132, 0.4176697321401328100 ) ) ;
#52665=CARTESIAN_POINT ( 'NONE',  ( 0.1443569553805781891, -0.4281496062992124485, 0.4176697321401328655 ) ) ;
#52666=CARTESIAN_POINT ( 'NONE',  ( -0.3149606299212590610, -0.1870078740157480879, -0.4822834645669291653 ) ) ;
#52668=CARTESIAN_POINT ( 'NONE',  ( -1.023622047244094002, -0.1870078740157480879, -0.4822834645669291653 ) ) ;
#52669=CARTESIAN_POINT ( 'NONE',  ( -0.4921259842519677963, 0.1660481256975883668, -0.3530559997133364547 ) ) ;
#52670=CARTESIAN_POINT ( 'NONE',  ( 0.01968503937007957949, -0.4536011799217368745, -0.2665933059059886201 ) ) ;
#52672=CARTESIAN_POINT ( 'NONE',  ( -0.3215223097112853146, -0.3162353388693405765, 0.4822834645669290543 ) ) ;
#52674=EDGE_CURVE ( 'NONE', #20402, #60445, #66504, .T. ) ;
#52675=CARTESIAN_POINT ( 'NONE',  ( 0.6824146981627303710, 0.2306618581243847221, -0.2411417322834647770 ) ) ;
#52677=CARTESIAN_POINT ( 'NONE',  ( -0.1377952755905504645, -0.5400638737290845981, -0.3530559997133363437 ) ) ;
#52678=CARTESIAN_POINT ( 'NONE',  ( -0.3477690288713905509, -0.5511811023622046335, 0.09757992244046803654 ) ) ;
#52679=CARTESIAN_POINT ( 'NONE',  ( 1.122047244094488860, -0.4536011799217368745, -0.2665933059059886201 ) ) ;
#52682=CARTESIAN_POINT ( 'NONE',  ( 1.496062992125985147, -0.1870078740157479769, 0.3641732283464567677 ) ) ;
#52683=CARTESIAN_POINT ( 'NONE',  ( 1.135170603674541256, 0.2952755905511811885, 0.1292274648535926551 ) ) ;
#52685=CARTESIAN_POINT ( 'NONE',  ( 0.1706036745406830368, 0.05413385826771666132, 0.4176697321401328100 ) ) ;
#52686=CARTESIAN_POINT ( 'NONE',  ( -1.450131233595799651, 0.2952755905511810774, -0.1292274648535930714 ) ) ;
#52687=CARTESIAN_POINT ( 'NONE',  ( -1.528871391076114250, 0.2952755905511810774, -0.1292274648535930714 ) ) ;
#52688=CARTESIAN_POINT ( 'NONE',  ( -0.2099737532808391705, -0.6046776061558809534, -0.2411417322834644161 ) ) ;
#52690=CARTESIAN_POINT ( 'NONE',  ( -1.476377952755905110, 0.07958543189024085140, 0.2665933059059887866 ) ) ;
#52691=CARTESIAN_POINT ( 'NONE',  ( 0.5314960629921264834, 0.1660481256975883668, -0.3530559997133364547 ) ) ;
#52693=CARTESIAN_POINT ( 'NONE',  ( 1.148293963254593875, -0.5511811023622046335, 0.09757992244046803654 ) ) ;
#52695=CARTESIAN_POINT ( 'NONE',  ( 0.4855643044619430415, -0.3690944881889765550, -0.3153832671262227771 ) ) ;
#52696=CARTESIAN_POINT ( 'NONE',  ( -1.194225721784776262, -0.4281496062992124485, 0.4176697321401328655 ) ) ;
#52698=CARTESIAN_POINT ( 'NONE',  ( 1.312335958005250269, -0.6046776061558807314, 0.2411417322834647770 ) ) ;
#52700=CARTESIAN_POINT ( 'NONE',  ( 0.9120734908136490793, 0.2952755905511810774, -0.1292274648535930714 ) ) ;
#52702=CARTESIAN_POINT ( 'NONE',  ( -0.7998211177050861265, -2.609869883881465018E-15, -0.3464511005275220379 ) ) ;
#52703=CARTESIAN_POINT ( 'NONE',  ( 0.3937007874015754361, -0.1870078740157480601, -0.3641732283464567677 ) ) ;
#52704=CARTESIAN_POINT ( 'NONE',  ( 0.7283464566929143125, 0.1660481256975885056, 0.3530559997133364547 ) ) ;
#52705=CARTESIAN_POINT ( 'NONE',  ( 1.620734908136483465, -0.5511811023622046335, 0.09757992244046803654 ) ) ;
#52706=CARTESIAN_POINT ( 'NONE',  ( -0.7414698162729651543, 0.1771653543307087075, -0.09757992244046823083 ) ) ;
#52707=CARTESIAN_POINT ( 'NONE',  ( -0.8464566929133852113, -0.5400638737290845981, -0.3530559997133363437 ) ) ;
#52708=CARTESIAN_POINT ( 'NONE',  ( -1.633858267716534529, -0.5400638737290845981, -0.3530559997133363437 ) ) ;
#52709=CARTESIAN_POINT ( 'NONE',  ( 0.8070866141732289112, -0.5400638737290845981, -0.3530559997133363437 ) ) ;
#52710=CARTESIAN_POINT ( 'NONE',  ( 1.692913385826772421, 0.2952755905511811885, 0.000000000000000000 ) ) ;
#52712=CARTESIAN_POINT ( 'NONE',  ( 0.7086614173228352742, -0.1870078740157480879, -0.4822834645669291653 ) ) ;
#52713=B_SPLINE_CURVE_WITH_KNOTS ( 'NONE', 3,
 ( #75085, #62028, #4364, #55695 ),
 .UNSPECIFIED., .F., .F.,
 ( 4, 4 ),
 ( 0.05917802304550456166, 0.06118368893514435081 ),
 .UNSPECIFIED. ) ;
#52716=CARTESIAN_POINT ( 'NONE',  ( 1.364829396325460076, 0.2306618581243848609, 0.2411417322834645549 ) ) ;
#52717=CARTESIAN_POINT ( 'NONE',  ( -1.541994750656167090, 0.1771653543307087630, 0.09757992244046791164 ) ) ;
#52718=CARTESIAN_POINT ( 'NONE',  ( 1.391076115485564868, 0.1283753931104746893, -0.1820866141732285504 ) ) ;
#52719=CARTESIAN_POINT ( 'NONE',  ( -1.338582677165353729, -0.1870078740157479769, 0.3641732283464567677 ) ) ;
#52720=CARTESIAN_POINT ( 'NONE',  ( -0.6364829396325453192, -0.08942795157528024563, -0.3641732283464568787 ) ) ;
#52722=CARTESIAN_POINT ( 'NONE',  ( 0.4921259842519691285, 0.07958543189024085140, 0.2665933059059887866 ) ) ;
#52723=CARTESIAN_POINT ( 'NONE',  ( 0.6036745406824154392, 0.2306618581243847221, -0.2411417322834647770 ) ) ;
#52724=CARTESIAN_POINT ( 'NONE',  ( 1.017060367454068581, -0.05778040916215560624, -0.4822834645669293319 ) ) ;
#52725=CARTESIAN_POINT ( 'NONE',  ( -0.01968503937007793844, 0.1660481256975883668, -0.3530559997133364547 ) ) ;
#52726=CARTESIAN_POINT ( 'NONE',  ( -0.01968503937007793844, -0.4536011799217367080, 0.2665933059059888421 ) ) ;
#52728=CARTESIAN_POINT ( 'NONE',  ( 1.108923884514436242, -0.05778040916215522460, 0.4822834645669289988 ) ) ;
#52729=CARTESIAN_POINT ( 'NONE',  ( -1.646981627296586703, -0.05778040916215522460, 0.4822834645669289988 ) ) ;
#52730=CARTESIAN_POINT ( 'NONE',  ( -0.3871391076115479057, -0.3162353388693409650, -0.4822834645669289433 ) ) ;
#52732=CARTESIAN_POINT ( 'NONE',  ( 0.03280839895013198948, 0.2066929133858267931, 0.1054918080437490802 ) ) ;
#52733=CARTESIAN_POINT ( 'NONE',  ( 0.2362204724409456558, -0.1870078740157480879, -0.4822834645669291653 ) ) ;
#52734=CARTESIAN_POINT ( 'NONE',  ( -0.7283464566929126471, -0.5400638737290844871, 0.3530559997133364547 ) ) ;
#52735=CARTESIAN_POINT ( 'NONE',  ( -0.03937007874015669567, -0.6692913385826771977, 8.415575281601705876E-17 ) ) ;
#52736=ADVANCED_FACE ( 'NONE', ( #41272 ), #55121, .F. ) ;
#52741=FACE_OUTER_BOUND ( 'NONE', #82256, .T. ) ;
#52743=CARTESIAN_POINT ( 'NONE',  ( -0.7808398950131225646, -0.08942795157527998196, 0.3641732283464567121 ) ) ;
#52745=CARTESIAN_POINT ( 'NONE',  ( -1.660104986876639543, -0.05778040916215560624, -0.4822834645669293319 ) ) ;
#52748=CARTESIAN_POINT ( 'NONE',  ( 0.4986876640419954376, -0.6046776061558809534, -0.2411417322834644161 ) ) ;
#52749=CARTESIAN_POINT ( 'NONE',  ( -0.6824146981627291497, -0.5023911411419708095, -0.1820866141732282451 ) ) ;
#52750=CARTESIAN_POINT ( 'NONE',  ( 1.240157480314961314, -0.5400638737290844871, 0.3530559997133364547 ) ) ;
#52751=CARTESIAN_POINT ( 'NONE',  ( 0.3215223097112867578, -0.05778040916215522460, 0.4822834645669289988 ) ) ;
#52755=CARTESIAN_POINT ( 'NONE',  ( 1.384514435695538559, 0.2952755905511810774, -0.1292274648535930714 ) ) ;
#52756=CARTESIAN_POINT ( 'NONE',  ( 0.6824146981627303710, 0.2306618581243847221, -0.2411417322834647770 ) ) ;
#52757=CARTESIAN_POINT ( 'NONE',  ( 0.2034120734908142214, 0.2952755905511810774, -0.1292274648535930714 ) ) ;
#52758=CARTESIAN_POINT ( 'NONE',  ( -1.653543307086613234, -0.1870078740157479769, 0.4822834645669291653 ) ) ;
#52759=CARTESIAN_POINT ( 'NONE',  ( 0.7480314960629927956, 0.2952755905511811885, 0.000000000000000000 ) ) ;
#52761=CARTESIAN_POINT ( 'NONE',  ( 0.04593175853018440641, 0.2952755905511810774, -0.1292274648535930714 ) ) ;
#52762=CARTESIAN_POINT ( 'NONE',  ( 1.220472440944882608, 0.2952755905511811885, 0.000000000000000000 ) ) ;
#52763=CARTESIAN_POINT ( 'NONE',  ( 0.2952755905511819101, 0.1660481256975883668, -0.3530559997133364547 ) ) ;
#52764=CARTESIAN_POINT ( 'NONE',  ( 0.9383202099737538715, -0.08942795157528024563, -0.3641732283464568787 ) ) ;
#52765=CARTESIAN_POINT ( 'NONE',  ( -1.496062992125983815, -0.1870078740157480879, -0.4822834645669291653 ) ) ;
#52766=CARTESIAN_POINT ( 'NONE',  ( -1.561679790026246017, 0.05413385826771666132, 0.4176697321401328100 ) ) ;
#52767=CARTESIAN_POINT ( 'NONE',  ( 0.8595800524934390507, -0.05778040916215560624, -0.4822834645669293319 ) ) ;
#52774=CARTESIAN_POINT ( 'NONE',  ( 1.253280839895013710, -0.05778040916215560624, -0.4822834645669293319 ) ) ;
#52775=CARTESIAN_POINT ( 'NONE',  ( 0.8923884514435701520, -0.5023911411419708095, -0.1820866141732282451 ) ) ;
#52776=CARTESIAN_POINT ( 'NONE',  ( -1.614173228346457378, 1.330640075373402897, 0.1372047244094476981 ) ) ;
#52781=CARTESIAN_POINT ( 'NONE',  ( 1.358267716535433323, -0.5400638737290845981, -0.3530559997133363437 ) ) ;
#52783=CARTESIAN_POINT ( 'NONE',  ( -0.4921259842519677963, -0.5400638737290844871, 0.3530559997133364547 ) ) ;
#52784=CARTESIAN_POINT ( 'NONE',  ( 0.9580052493438326877, 0.05413385826771666132, 0.4176697321401328100 ) ) ;
#52785=ORIENTED_EDGE ( 'NONE', *, *, #42363, .T. ) ;
#52786=CARTESIAN_POINT ( 'NONE',  ( -1.463254593175852492, -0.6692913385826773087, -0.1292274648535924053 ) ) ;
#52787=CARTESIAN_POINT ( 'NONE',  ( -0.7205944486920646819, -4.754953748228849300E-15, -0.3627989612356167237 ) ) ;
#52789=CARTESIAN_POINT ( 'NONE',  ( 1.522309711286089939, 0.1283753931104748280, 0.1820866141732283561 ) ) ;
#52791=CARTESIAN_POINT ( 'NONE',  ( -1.010498687664041384, -0.004921259842519576551, 0.3153832671262227771 ) ) ;
#52792=CARTESIAN_POINT ( 'NONE',  ( 0.8789144566217211851, 0.004960608223779470680, 0.3437734562760185741 ) ) ;
#52793=CARTESIAN_POINT ( 'NONE',  ( 0.7742782152230979209, 0.05413385826771626580, -0.4176697321401330321 ) ) ;
#52796=CARTESIAN_POINT ( 'NONE',  ( -0.4199475065616791736, 0.1539470093639521697, -0.1968503937007875793 ) ) ;
#52797=CARTESIAN_POINT ( 'NONE',  ( 0.6955380577427828781, -0.4281496062992124485, 0.4176697321401328655 ) ) ;
#52798=CARTESIAN_POINT ( 'NONE',  ( -1.555118110236219930, 0.1660481256975885056, 0.3530559997133364547 ) ) ;
#52800=VECTOR ( 'NONE', #80614, 39.37007874015748143 ) ;
#52801=CARTESIAN_POINT ( 'NONE',  ( -0.6889763779527552368, -0.4536011799217368745, -0.2665933059059886201 ) ) ;
#52802=CARTESIAN_POINT ( 'NONE',  ( 1.653543307086614789, -0.1870078740157479769, 0.4822834645669291653 ) ) ;
#52803=CARTESIAN_POINT ( 'NONE',  ( 0.4330708661417329575, -0.6692913385826771977, 8.415575281601705876E-17 ) ) ;
#52804=CARTESIAN_POINT ( 'NONE',  ( -1.135170603674539924, 0.1771653543307087075, -0.09757992244046823083 ) ) ;
#52805=CARTESIAN_POINT ( 'NONE',  ( 0.06561679790026316017, -0.004921259842519870586, -0.3153832671262229437 ) ) ;
#52806=CARTESIAN_POINT ( 'NONE',  ( -0.2887139107611542133, 0.2306618581243848609, 0.2411417322834645549 ) ) ;
#52807=CARTESIAN_POINT ( 'NONE',  ( -1.305774278215222184, 0.1771653543307087630, 0.09757992244046791164 ) ) ;
#52809=CARTESIAN_POINT ( 'NONE',  ( 0.6102362204724416372, -0.5400638737290844871, 0.3530559997133364547 ) ) ;
#52812=CARTESIAN_POINT ( 'NONE',  ( -0.9251968503937002541, 0.1660481256975885056, 0.3530559997133364547 ) ) ;
#52813=CARTESIAN_POINT ( 'NONE',  ( -0.05905511811023545637, -0.4536011799217368745, -0.2665933059059886201 ) ) ;
#52814=CARTESIAN_POINT ( 'NONE',  ( -1.404199475065615932, -0.4281496062992127816, -0.4176697321401328100 ) ) ;
#52815=CARTESIAN_POINT ( 'NONE',  ( 0.8267716535433078384, -0.5511811023622047445, 6.969142054262312111E-17 ) ) ;
#52816=CARTESIAN_POINT ( 'NONE',  ( -0.6496062992125976043, -0.4536011799217367080, 0.2665933059059888421 ) ) ;
#52817=CARTESIAN_POINT ( 'NONE',  ( -0.9055118110236215490, 0.2952755905511811885, 0.000000000000000000 ) ) ;
#52818=CARTESIAN_POINT ( 'NONE',  ( -1.095800524934382292, -0.05778040916215522460, 0.4822834645669289988 ) ) ;
#52819=CARTESIAN_POINT ( 'NONE',  ( 1.646981627296588035, -0.3162353388693405765, 0.4822834645669290543 ) ) ;
#52821=CARTESIAN_POINT ( 'NONE',  ( 0.8070866141732289112, -0.4536011799217368745, -0.2665933059059886201 ) ) ;
#52822=CARTESIAN_POINT ( 'NONE',  ( 0.2034120734908144990, -0.6692913385826771977, 0.1292274648535927661 ) ) ;
#52823=CARTESIAN_POINT ( 'NONE',  ( -1.496062992125983815, -0.1870078740157479769, 0.4822834645669291653 ) ) ;
#52824=CARTESIAN_POINT ( 'NONE',  ( -1.338582677165353729, -0.1870078740157480879, -0.4822834645669291653 ) ) ;
#52827=CARTESIAN_POINT ( 'NONE',  ( -1.154855643044618851, 0.1283753931104748280, 0.1820866141732283561 ) ) ;
#52828=CARTESIAN_POINT ( 'NONE',  ( -0.5380577427821514602, 0.05413385826771666132, 0.4176697321401328100 ) ) ;
#52829=CARTESIAN_POINT ( 'NONE',  ( 0.5380577427821529035, 0.05413385826771626580, -0.4176697321401330321 ) ) ;
#52830=CARTESIAN_POINT ( 'NONE',  ( -1.305774278215222184, -0.5511811023622048555, -0.09757992244046775898 ) ) ;
#52832=CARTESIAN_POINT ( 'NONE',  ( -1.587926509186350810, -0.4281496062992124485, 0.4176697321401328655 ) ) ;
#52833=CARTESIAN_POINT ( 'NONE',  ( 0.8333333333333340365, -0.6692913385826771977, 0.1292274648535927661 ) ) ;
#52834=CARTESIAN_POINT ( 'NONE',  ( 0.4133858267716541968, 0.1660481256975885056, 0.3530559997133364547 ) ) ;
#52835=CARTESIAN_POINT ( 'NONE',  ( 1.043307086614173818, -0.5400638737290845981, -0.3530559997133363437 ) ) ;
#52840=AXIS2_PLACEMENT_3D ( 'NONE', #6872, #75527, #32541 ) ;
#52841=DIRECTION ( 'NONE',  ( -3.096699300667737957E-16, 1.000000000000000000, -0.000000000000000000 ) ) ;
#52842=CARTESIAN_POINT ( 'NONE',  ( 0.1181102362204730916, -0.5511811023622047445, 6.969142054262312111E-17 ) ) ;
#52843=CARTESIAN_POINT ( 'NONE',  ( 0.2559055118110243332, -0.5400638737290845981, -0.3530559997133363437 ) ) ;
#52844=CARTESIAN_POINT ( 'NONE',  ( 1.187664041994751285, -0.3162353388693409650, -0.4822834645669289433 ) ) ;
#52846=CARTESIAN_POINT ( 'NONE',  ( 0.4593175853018380828, -0.004921259842519870586, -0.3153832671262229437 ) ) ;
#52847=CARTESIAN_POINT ( 'NONE',  ( -0.6824146981627288167, 0.2306618581243848609, 0.2411417322834645549 ) ) ;
#52848=CARTESIAN_POINT ( 'NONE',  ( -1.614173228346455824, 0.2952755905511811885, 0.000000000000000000 ) ) ;
#52849=CARTESIAN_POINT ( 'NONE',  ( 0.4593175853018380828, 0.05413385826771626580, -0.4176697321401330321 ) ) ;
#52855=CARTESIAN_POINT ( 'NONE',  ( -1.706036745406823485, 0.2306618581243848609, 0.2411417322834645549 ) ) ;
#52856=CARTESIAN_POINT ( 'NONE',  ( -1.371391076115484609, -0.5511811023622046335, 0.09757992244046803654 ) ) ;
#52857=CARTESIAN_POINT ( 'NONE',  ( -1.194225721784776262, -0.4281496062992124485, 0.4176697321401328655 ) ) ;
#52860=CARTESIAN_POINT ( 'NONE',  ( 1.679790026246720025, 0.2306618581243848609, 0.2411417322834645549 ) ) ;
#52861=CARTESIAN_POINT ( 'NONE',  ( -1.213910761154854745, 0.2952755905511810774, -0.1292274648535930714 ) ) ;
#52862=CARTESIAN_POINT ( 'NONE',  ( 0.4986876640419954376, 0.2306618581243848609, 0.2411417322834645549 ) ) ;
#52863=CARTESIAN_POINT ( 'NONE',  ( -1.141732283464566011, 0.2952755905511811885, 0.000000000000000000 ) ) ;
#52865=CARTESIAN_POINT ( 'NONE',  ( 0.6889763779527563470, 0.1660481256975883668, -0.3530559997133364547 ) ) ;
#52867=CARTESIAN_POINT ( 'NONE',  ( -1.384514435695537005, -0.5511811023622048555, -0.09757992244046775898 ) ) ;
#52871=CARTESIAN_POINT ( 'NONE',  ( -1.699475065616797398, 0.1771653543307087630, 0.09757992244046791164 ) ) ;
#52872=CARTESIAN_POINT ( 'NONE',  ( -1.181102362204723644, -0.1870078740157480879, -0.4822834645669291653 ) ) ;
#52873=CARTESIAN_POINT ( 'NONE',  ( -1.272965879265091305, 0.05413385826771626580, -0.4176697321401330321 ) ) ;
#52875=CARTESIAN_POINT ( 'NONE',  ( -1.410761154855642463, -0.05778040916215522460, 0.4822834645669289988 ) ) ;
#52876=CARTESIAN_POINT ( 'NONE',  ( -1.620734908136482577, -0.6692913385826773087, -0.1292274648535924053 ) ) ;
#52877=CARTESIAN_POINT ( 'NONE',  ( -1.437007874015747477, 0.1660481256975883668, -0.3530559997133364547 ) ) ;
#52878=CARTESIAN_POINT ( 'NONE',  ( -0.8398950131233585692, 0.2306618581243848609, 0.2411417322834645549 ) ) ;
#52879=CARTESIAN_POINT ( 'NONE',  ( 0.03937007874015833325, -0.5511811023622047445, 6.969142054262312111E-17 ) ) ;
#52882=CARTESIAN_POINT ( 'NONE',  ( -0.8464566929133852113, -0.4536011799217368745, -0.2665933059059886201 ) ) ;
#52883=CARTESIAN_POINT ( 'NONE',  ( -0.8464566929133852113, 0.1660481256975885056, 0.3530559997133364547 ) ) ;
#52884=CARTESIAN_POINT ( 'NONE',  ( 0.7939632545931766261, -0.05778040916215522460, 0.4822834645669289988 ) ) ;
#52885=CARTESIAN_POINT ( 'NONE',  ( -0.8661417322834640276, -0.1870078740157479769, 0.4822834645669291653 ) ) ;
#52888=CARTESIAN_POINT ( 'NONE',  ( -1.128608923884513837, 0.2306618581243847221, -0.2411417322834647770 ) ) ;
#52889=CARTESIAN_POINT ( 'NONE',  ( 0.8989501312335963501, -0.6692913385826773087, -0.1292274648535924053 ) ) ;
#52890=CARTESIAN_POINT ( 'NONE',  ( -1.496062992125983815, -0.1870078740157480601, -0.3641732283464567677 ) ) ;
#52895=CARTESIAN_POINT ( 'NONE',  ( -0.4396325459317577122, -0.6692913385826773087, -0.1292274648535924053 ) ) ;
#52896=CARTESIAN_POINT ( 'NONE',  ( -1.482939632545930975, -0.004921259842519576551, 0.3153832671262227771 ) ) ;
#52898=CARTESIAN_POINT ( 'NONE',  ( -1.417322834645668772, -0.1870078740157479769, 0.4822834645669291653 ) ) ;
#52899=CARTESIAN_POINT ( 'NONE',  ( -0.6627296587926501115, 0.2066929133858267098, -0.1054918080437494132 ) ) ;
#52900=CARTESIAN_POINT ( 'NONE',  ( -1.587926509186350810, -0.4281496062992124485, 0.4176697321401328655 ) ) ;
#52901=CARTESIAN_POINT ( 'NONE',  ( -0.5446194225721777693, -0.3162353388693409650, -0.4822834645669289433 ) ) ;
#52903=CARTESIAN_POINT ( 'NONE',  ( 0.4658792650918640033, -0.2845877964562159024, 0.3641732283464567677 ) ) ;
#52905=CARTESIAN_POINT ( 'NONE',  ( 0.4461942257217856311, 0.1283753931104746893, -0.1820866141732285504 ) ) ;
#52906=CARTESIAN_POINT ( 'NONE',  ( 1.266404199475066328, -0.08942795157527998196, 0.3641732283464567121 ) ) ;
#52907=CARTESIAN_POINT ( 'NONE',  ( 1.148293963254593653, 0.2952755905511810774, -0.1292274648535930714 ) ) ;
#52908=CARTESIAN_POINT ( 'NONE',  ( 0.006561679790026889343, -0.2845877964562161244, -0.3641732283464567121 ) ) ;
#52910=CARTESIAN_POINT ( 'NONE',  ( -1.089238845144356427, -0.4281496062992127816, -0.4176697321401328100 ) ) ;
#52911=CARTESIAN_POINT ( 'NONE',  ( -0.2493438320209966919, -0.004921259842519870586, -0.3153832671262229437 ) ) ;
#52913=CARTESIAN_POINT ( 'NONE',  ( -0.3805774278215216522, -0.004921259842519576551, 0.3153832671262227771 ) ) ;
#52915=CARTESIAN_POINT ( 'NONE',  ( -0.09186351706036663400, -0.4281496062992124485, 0.4176697321401328655 ) ) ;
#52918=CARTESIAN_POINT ( 'NONE',  ( 1.102362204724410155, -0.1870078740157479769, 0.3641732283464567677 ) ) ;
#52919=CARTESIAN_POINT ( 'NONE',  ( -0.3674540682414692561, -0.5023911411419708095, -0.1820866141732282451 ) ) ;
#52920=CARTESIAN_POINT ( 'NONE',  ( -0.1181102362204717315, -0.6692913385826771977, 8.415575281601705876E-17 ) ) ;
#52921=DIRECTION ( 'NONE',  ( -1.000000000000000000, 0.000000000000000000, 0.000000000000000000 ) ) ;
#52922=CARTESIAN_POINT ( 'NONE',  ( -1.312335958005248715, 0.1283753931104748280, 0.1820866141732283561 ) ) ;
#52924=CARTESIAN_POINT ( 'NONE',  ( 0.5839895013123367340, 0.2952755905511811885, 0.1292274648535926551 ) ) ;
#52925=CARTESIAN_POINT ( 'NONE',  ( -0.9383202099737524282, -0.3162353388693409650, -0.4822834645669289433 ) ) ;
#52929=CARTESIAN_POINT ( 'NONE',  ( 0.4002624671916016896, -0.2845877964562161244, -0.3641732283464567121 ) ) ;
#52930=CARTESIAN_POINT ( 'NONE',  ( -0.6036745406824141069, -0.6046776061558809534, -0.2411417322834644161 ) ) ;
#52931=CARTESIAN_POINT ( 'NONE',  ( -1.299212598425196097, 0.2952755905511811885, 0.000000000000000000 ) ) ;
#52932=CARTESIAN_POINT ( 'NONE',  ( -1.167979002624671470, -0.004921259842519576551, 0.3153832671262227771 ) ) ;
#52934=CARTESIAN_POINT ( 'NONE',  ( -0.7808398950131222316, -0.2845877964562161244, -0.3641732283464567121 ) ) ;
#52936=CARTESIAN_POINT ( 'NONE',  ( 0.9383202099737536495, -0.3162353388693405765, 0.4822834645669290543 ) ) ;
#52940=CARTESIAN_POINT ( 'NONE',  ( -1.607611548556429737, -0.6692913385826771977, 0.1292274648535927661 ) ) ;
#52941=CARTESIAN_POINT ( 'NONE',  ( -1.450131233595799651, -0.6692913385826771977, 0.1292274648535927661 ) ) ;
#52942=CARTESIAN_POINT ( 'NONE',  ( 1.200787401574803681, -0.5400638737290845981, -0.3530559997133363437 ) ) ;
#52944=CARTESIAN_POINT ( 'NONE',  ( 1.594488188976378673, -0.4536011799217368745, -0.2665933059059886201 ) ) ;
#52945=CARTESIAN_POINT ( 'NONE',  ( 0.3871391076115493490, -0.3162353388693405765, 0.4822834645669290543 ) ) ;
#52946=CARTESIAN_POINT ( 'NONE',  ( -0.2755905511811015396, -0.6692913385826771977, 8.415575281601705876E-17 ) ) ;
#52947=CARTESIAN_POINT ( 'NONE',  ( -0.6979622409133203753, 5.991678263669262536E-15, 0.4118484887281945728 ) ) ;
#52949=CARTESIAN_POINT ( 'NONE',  ( 0.5905511811023629321, -0.5511811023622047445, 6.969142054262312111E-17 ) ) ;
#52954=CARTESIAN_POINT ( 'NONE',  ( 0.006561679790026889343, -0.05778040916215522460, 0.4822834645669289988 ) ) ;
#52955=CARTESIAN_POINT ( 'NONE',  ( 1.292650918635171564, 0.2952755905511811885, 0.1292274648535926551 ) ) ;
#52956=CARTESIAN_POINT ( 'NONE',  ( 0.1837270341207357105, -0.6046776061558809534, -0.2411417322834644161 ) ) ;
#52957=CARTESIAN_POINT ( 'NONE',  ( -0.5643044619422565855, -0.3690944881889763329, 0.3153832671262228327 ) ) ;
#52959=CARTESIAN_POINT ( 'NONE',  ( 1.299212598425197429, -0.6692913385826771977, 8.415575281601705876E-17 ) ) ;
#52960=CARTESIAN_POINT ( 'NONE',  ( -0.2952755905511803003, -0.5400638737290845981, -0.3530559997133363437 ) ) ;
#52961=CARTESIAN_POINT ( 'NONE',  ( -0.1771653543307080136, -0.5400638737290844871, 0.3530559997133364547 ) ) ;
#52962=CARTESIAN_POINT ( 'NONE',  ( -1.548556430446193399, -0.6046776061558809534, -0.2411417322834644161 ) ) ;
#52963=CARTESIAN_POINT ( 'NONE',  ( 0.7020997375328090762, -0.05778040916215560624, -0.4822834645669293319 ) ) ;
#52964=CARTESIAN_POINT ( 'NONE',  ( 1.167979002624672580, -0.4281496062992124485, 0.4176697321401328655 ) ) ;
#52966=CARTESIAN_POINT ( 'NONE',  ( 0.3740157480314966754, -0.4536011799217367080, 0.2665933059059888421 ) ) ;
#52969=ORIENTED_EDGE ( 'NONE', *, *, #56716, .T. ) ;
#52970=CARTESIAN_POINT ( 'NONE',  ( -0.6430446194225716283, -0.3690944881889763329, 0.3153832671262228327 ) ) ;
#52971=CARTESIAN_POINT ( 'NONE',  ( -0.09186351706036663400, -0.4281496062992124485, 0.4176697321401328655 ) ) ;
#52973=CARTESIAN_POINT ( 'NONE',  ( -0.2493438320209966919, 0.05413385826771626580, -0.4176697321401330321 ) ) ;
#52974=CARTESIAN_POINT ( 'NONE',  ( 0.1574803149606306130, -0.1870078740157479769, 0.4822834645669291653 ) ) ;
#52975=CARTESIAN_POINT ( 'NONE',  ( -0.8005249343832011588, 0.05413385826771626580, -0.4176697321401330321 ) ) ;
#52976=CARTESIAN_POINT ( 'NONE',  ( -1.154855643044618851, -0.6046776061558809534, -0.2411417322834644161 ) ) ;
#52978=CARTESIAN_POINT ( 'NONE',  ( 1.371391076115485941, 0.1771653543307087630, 0.09757992244046791164 ) ) ;
#52981=CARTESIAN_POINT ( 'NONE',  ( 0.8202099737532813073, 0.1771653543307087630, 0.09757992244046791164 ) ) ;
#52982=CARTESIAN_POINT ( 'NONE',  ( 0.5643044619422579178, 0.05413385826771666132, 0.4176697321401328100 ) ) ;
#52983=CARTESIAN_POINT ( 'NONE',  ( 0.4855643044619430415, -0.4281496062992127816, -0.4176697321401328100 ) ) ;
#52988=CARTESIAN_POINT ( 'NONE',  ( -0.3412073490813641308, -0.6046776061558807314, 0.2411417322834647770 ) ) ;
#52991=CARTESIAN_POINT ( 'NONE',  ( -1.003937007874014853, 0.07958543189024085140, 0.2665933059059887866 ) ) ;
#52992=CARTESIAN_POINT ( 'NONE',  ( 0.9317585301837276734, -0.4281496062992124485, 0.4176697321401328655 ) ) ;
#52993=CARTESIAN_POINT ( 'NONE',  ( 0.9055118110236227702, 0.2952755905511811885, 0.000000000000000000 ) ) ;
#52994=CARTESIAN_POINT ( 'NONE',  ( -0.2427821522309703550, -0.2845877964562159024, 0.3641732283464567677 ) ) ;
#52995=CARTESIAN_POINT ( 'NONE',  ( 0.6758530183727039509, 0.2952755905511810774, -0.1292274648535930714 ) ) ;
#52997=CARTESIAN_POINT ( 'NONE',  ( 0.07217847769028949700, -0.2845877964562159024, 0.3641732283464567677 ) ) ;
#52998=CARTESIAN_POINT ( 'NONE',  ( -0.1837270341207343505, -0.6046776061558807314, 0.2411417322834647770 ) ) ;
#53000=CARTESIAN_POINT ( 'NONE',  ( -1.476377952755905110, -0.5400638737290845981, -0.3530559997133363437 ) ) ;
#53001=CARTESIAN_POINT ( 'NONE',  ( 0.3674540682414705883, 0.1283753931104746893, -0.1820866141732285504 ) ) ;
#53002=CARTESIAN_POINT ( 'NONE',  ( 1.410761154855643795, -0.08942795157528024563, -0.3641732283464568787 ) ) ;
#53003=CARTESIAN_POINT ( 'NONE',  ( -0.9186351706036736120, 0.2306618581243848609, 0.2411417322834645549 ) ) ;
#53004=CARTESIAN_POINT ( 'NONE',  ( -0.6955380577427815458, -0.004921259842519576551, 0.3153832671262227771 ) ) ;
#53006=CARTESIAN_POINT ( 'NONE',  ( -0.5839895013123351797, 0.2952755905511810774, -0.1292274648535930714 ) ) ;
#53007=CARTESIAN_POINT ( 'NONE',  ( -0.5511811023622038563, -0.1870078740157479769, 0.4822834645669291653 ) ) ;
#53008=CARTESIAN_POINT ( 'NONE',  ( -0.1574803149606292529, -0.1870078740157480879, -0.4822834645669291653 ) ) ;
#53013=CARTESIAN_POINT ( 'NONE',  ( 0.5511811023622055217, -0.1870078740157479769, 0.3641732283464567677 ) ) ;
#53014=CARTESIAN_POINT ( 'NONE',  ( 1.200787401574803681, -0.5400638737290845981, -0.3530559997133363437 ) ) ;
#53015=CARTESIAN_POINT ( 'NONE',  ( -1.345144356955379816, -0.08942795157528024563, -0.3641732283464568787 ) ) ;
#53016=CARTESIAN_POINT ( 'NONE',  ( -1.259842519685038686, -0.1870078740157479769, 0.3641732283464567677 ) ) ;
#53017=CARTESIAN_POINT ( 'NONE',  ( -0.6889763779527552368, -0.5400638737290845981, -0.3530559997133363437 ) ) ;
#53018=CARTESIAN_POINT ( 'NONE',  ( 0.4133858267716541968, 0.07958543189024085140, 0.2665933059059887866 ) ) ;
#53020=CARTESIAN_POINT ( 'NONE',  ( 1.194225721784777594, -0.3690944881889765550, -0.3153832671262227771 ) ) ;
#53022=CARTESIAN_POINT ( 'NONE',  ( 0.3937007874015754361, -0.1870078740157479769, 0.4822834645669291653 ) ) ;
#53025=CARTESIAN_POINT ( 'NONE',  ( -0.6758530183727028406, -0.6692913385826773087, -0.1292274648535924053 ) ) ;
#53027=CARTESIAN_POINT ( 'NONE',  ( 1.430446194225722500, -0.004921259842519576551, 0.3153832671262227771 ) ) ;
#53028=CARTESIAN_POINT ( 'NONE',  ( 0.5380577427821529035, -0.4281496062992124485, 0.4176697321401328655 ) ) ;
#53029=CARTESIAN_POINT ( 'NONE',  ( 0.08530183727034192087, -0.05778040916215522460, 0.4822834645669289988 ) ) ;
#53030=CARTESIAN_POINT ( 'NONE',  ( 8.195543980992789655E-16, -0.1870078740157480601, -0.3641732283464567677 ) ) ;
#53032=CARTESIAN_POINT ( 'NONE',  ( -0.2099737532808391705, 0.1283753931104748280, 0.1820866141732283561 ) ) ;
#53033=CARTESIAN_POINT ( 'NONE',  ( 0.9383202099737538715, -0.05778040916215560624, -0.4822834645669293319 ) ) ;
#53034=CARTESIAN_POINT ( 'NONE',  ( -0.8070866141732276899, -0.4536011799217367080, 0.2665933059059888421 ) ) ;
#53037=CARTESIAN_POINT ( 'NONE',  ( -0.9645669291338575535, 0.1660481256975883668, -0.3530559997133364547 ) ) ;
#53038=CARTESIAN_POINT ( 'NONE',  ( -0.8542087009142328435, -4.039970415760091124E-15, 0.3627989612356165572 ) ) ;
#53040=CARTESIAN_POINT ( 'NONE',  ( -1.358267716535432434, -0.5400638737290844871, 0.3530559997133364547 ) ) ;
#53041=CARTESIAN_POINT ( 'NONE',  ( -1.141732283464566011, -0.5511811023622047445, 6.969142054262312111E-17 ) ) ;
#53042=CARTESIAN_POINT ( 'NONE',  ( -0.1574803149606292529, -0.1870078740157479769, 0.4822834645669291653 ) ) ;
#53044=CARTESIAN_POINT ( 'NONE',  ( -0.8398950131233585692, 0.2306618581243848609, 0.2411417322834645549 ) ) ;
#53046=CARTESIAN_POINT ( 'NONE',  ( -0.8761506516392493227, -2.567464376874931580E-15, -0.4445507791589072832 ) ) ;
#53047=CARTESIAN_POINT ( 'NONE',  ( 0.7808398950131240079, -0.3162353388693405765, 0.4822834645669290543 ) ) ;
#53048=CARTESIAN_POINT ( 'NONE',  ( 0.9383202099737538715, -0.05778040916215560624, -0.4822834645669293319 ) ) ;
#53050=CARTESIAN_POINT ( 'NONE',  ( 1.509186351706037543, -0.4281496062992127816, -0.4176697321401328100 ) ) ;
#53051=CARTESIAN_POINT ( 'NONE',  ( -1.161417322834644716, -0.5400638737290845981, -0.3530559997133363437 ) ) ;
#53053=ORIENTED_EDGE ( 'NONE', *, *, #63775, .F. ) ;
#53054=CARTESIAN_POINT ( 'NONE',  ( -0.6889763779527552368, 0.07958543189024085140, 0.2665933059059887866 ) ) ;
#53057=CARTESIAN_POINT ( 'NONE',  ( 0.3543307086614179147, 0.2952755905511811885, 0.000000000000000000 ) ) ;
#53058=CARTESIAN_POINT ( 'NONE',  ( -0.06561679790026180015, -0.4281496062992127816, -0.4176697321401328100 ) ) ;
#53059=CARTESIAN_POINT ( 'NONE',  ( -0.7939632545931750718, -0.05778040916215560624, -0.4822834645669293319 ) ) ;
#53060=CARTESIAN_POINT ( 'NONE',  ( 1.601049868766404982, -0.6046776061558809534, -0.2411417322834644161 ) ) ;
#53061=CARTESIAN_POINT ( 'NONE',  ( -0.8267716535433065062, 0.1771653543307087630, 0.000000000000000000 ) ) ;
#53063=CARTESIAN_POINT ( 'NONE',  ( 0.6496062992125991586, -0.5400638737290845981, -0.3530559997133363437 ) ) ;
#53065=CARTESIAN_POINT ( 'NONE',  ( 0.4921259842519691285, 0.07958543189024085140, 0.2665933059059887866 ) ) ;
#53066=CARTESIAN_POINT ( 'NONE',  ( -0.4265091863517051496, -0.6692913385826771977, 0.1292274648535927661 ) ) ;
#53068=CARTESIAN_POINT ( 'NONE',  ( -0.9645669291338575535, 0.1660481256975883668, -0.3530559997133364547 ) ) ;
#53069=CARTESIAN_POINT ( 'NONE',  ( -1.679790026246718693, 0.1283753931104746893, -0.1820866141732285504 ) ) ;
#53070=CARTESIAN_POINT ( 'NONE',  ( 1.541994750656168645, 0.2952755905511810774, -0.1292274648535930714 ) ) ;
#53074=CARTESIAN_POINT ( 'NONE',  ( 0.07874015748031558404, -0.1870078740157479769, 0.4822834645669291653 ) ) ;
#53075=ORIENTED_EDGE ( 'NONE', *, *, #46886, .F. ) ;
#53076=CARTESIAN_POINT ( 'NONE',  ( -1.003937007874015297, -0.5400638737290845981, -0.3530559997133363437 ) ) ;
#53077=CARTESIAN_POINT ( 'NONE',  ( 1.154855643044620184, 0.2306618581243847221, -0.2411417322834647770 ) ) ;
#53078=CARTESIAN_POINT ( 'NONE',  ( 1.305774278215223960, 0.2952755905511810774, -0.1292274648535930714 ) ) ;
#53079=CARTESIAN_POINT ( 'NONE',  ( 0.4396325459317590445, -0.6692913385826771977, 0.1292274648535927661 ) ) ;
#53080=CARTESIAN_POINT ( 'NONE',  ( -0.1837270341207340729, 0.2306618581243847221, -0.2411417322834647770 ) ) ;
#53082=CARTESIAN_POINT ( 'NONE',  ( -1.345144356955379816, -0.05778040916215560624, -0.4822834645669293319 ) ) ;
#53083=CARTESIAN_POINT ( 'NONE',  ( -0.6889763779527552368, 0.1660481256975885056, 0.3530559997133364547 ) ) ;
#53085=CARTESIAN_POINT ( 'NONE',  ( -0.6364829396325453192, -0.08942795157528024563, -0.3641732283464568787 ) ) ;
#53086=CARTESIAN_POINT ( 'NONE',  ( -1.614173228346456712, 0.7166040191147899918, -0.1372047244094478091 ) ) ;
#53087=CARTESIAN_POINT ( 'NONE',  ( -0.6364829396325453192, -0.3162353388693405765, 0.4822834645669290543 ) ) ;
#53088=CARTESIAN_POINT ( 'NONE',  ( -1.192688228555125685, 0.02791078216816347476, -0.4328096321851898631 ) ) ;
#53089=CARTESIAN_POINT ( 'NONE',  ( 0.6955380577427828781, 0.05413385826771626580, -0.4176697321401330321 ) ) ;
#53093=( BOUNDED_SURFACE ( )  B_SPLINE_SURFACE ( 1, 2, ( 
 ( #68295, #10632, #36287, #75023, #17771, #29963, #17369, #68692, #474, #13519, #64020, #6361, #70757, #32033, #24879, #25291, #58108, #11866, #19831, #18585, #50141, #19405, #38761, #37930, #37519, #50547, #56865, #64859, #82560, #39175, #43812, #13108, #45480, #63194, #31613, #51368, #63607, #51791, #24475, #45056, #26129, #44634, #58537, #76251, #69918, #25708, #5534, #12272, #57692, #31199, #75838, #7197, #77071, #64438, #6774, #50957, #44228, #32869, #5944, #18180, #69517, #12687, #32446, #57274, #82972, #76654, #18987, #38346, #70331, #54, #77495, #71177, #46742, #47153, #27809, #7631, #26969, #46323, #72844, #52634, #53469, #34126, #40440, #1320, #66120, #903, #40029, #61338, #78339, #42386, #23038, #45897, #59787, #29356, #33302, #41978, #8456, #3691, #74403, #2141, #79179, #16335, #21494, #20670, #1730, #55015, #14784, #67672, #10008, #35673, #72016, #48704, #16747, #68085, #14372, #71594, #80724, #65292, #10430, #36087, #26560, #52214, #65717, #8048, #27386, #33710, #59371, #53047, #77917, #20248, #78758, #58963, #13946, #21083, #39603, #72434, #18393, #29764, #82768, #49532, #12072, #68493, #69318, #11669, #4507, #75641, #12479, #76464, #74820, #44035, #24272, #24684, #5338, #10833, #30175, #23865, #50351, #55838, #30997, #37327, #17980, #62168, #43617, #61758, #17570, #37730, #81547, #18790, #25090, #23450, #62999, #5739, #36492, #69727, #56665, #63403, #50763, #82365, #76049, #31410, #57074, #75226, #62585, #44435, #70128, #4096, #55426, #81134, #43203, #49115, #17165, #42799, #68898, #11251, #36909, #4927, #30595, #56261, #81957, #49943, #32244, #45277, #38970, #70972, #64238, #57904, #59167, #52843, #13317, #44846, #20879, #19197, #52005, #78554, #78130, #6154, #1525, #25924, #71810, #70544, #45691, #71388, #14161, #25503, #33505, #269, #63815, #33085, #52420, #51582, #51169, #38558, #12899, #46531, #6573, #27179, #57489, #1114, #72231, #76865, #64653, #65077, #77284, #65506, #38143, #58752, #39817, #58326, #31828, #19615, #6991, #39393, #32659, #688, #13737, #26344, #83182, #77710, #7415, #26765, #20463, #20040, #46116, #7838, #60003, #8253, #80633, #2771, #15832, #28014, #3597, #40645, #73482, #41883, #46946, #54507, #22121, #73895, #29262, #54090, #79805, #60829, #47780, #14987, #15405, #67576, #28431, #41480, #9495, #48200, #66329, #61243, #54926, #22944, #53674, #1939, #67165, #78972, #80221, #48612, #9908, #14580, #8667, #21701, #41065, #47364, #34338, #2358, #35580, #40233, #73055, #21293, #65916, #72638, #35168, #33917, #22537, #59582, #27601, #79382, #16235, #66754, #3181, #28845, #53261, #9088, #34760, #60420, #16653, #69222, #5241, #4415, #61667, #74723, #23356, #31315, #49027, #63310, #10335, #37229, #11979, #4008, #81454, #17887, #30084, #18295, #74306, #11570, #50259, #11155, #24994, #17072, #36402, #75547, #29672, #62077, #81867, #55334, #42293, #5648, #43524, #62906, #30905, #17481, #42709, #56980, #55746, #67990, #82677, #62489, #56572, #23771, #35997, #68405, #10745, #4823, #81043, #49442, #75136, #82273, #36813, #24591, #75957, #43112, #68808, #30501, #43940, #56164, #69634, #24179, #49848, #37634, #32562, #50668, #6479, #26671, #51072, #7745, #71708, #12387, #32148, #78032, #76368, #71291, #52326, #70878, #1427, #76771, #12804, #51907, #6061, #38459, #58225, #63721, #18701, #65407, #77614, #45597, #13638, #77187, #19102, #33410, #64145, #44343, #59072, #38877, #19947, #57805, #39716, #44751, #70447, #64555, #70034, #38045, #31732, #32983, #13227, #39291, #64977, #57397, #171, #25824, #7314, #51484, #58651, #592, #6893, #19519, #26248, #83087, #45172, #20362, #1018, #25409, #14062, #46012, #2672, #54409, #59486, #67063, #34660, #3083, #16134, #66650, #8986, #73376, #60323, #27500, #27918, #80120, #40968, #53993, #22021, #60731, #53156, #73797, #41780, #67473, #40550, #14483, #28331, #8155, #9395, #9807, #22438, #61143, #21194, #34239, #53577, #59900, #78868, #46848, #48098, #35479, #2253, #33820, #27083, #1840, #79705, #52745, #35066, #78453, #20779, #14890, #28747, #72543, #47681, #15726, #46433, #40137, #72125 ),
 ( #65822, #41381, #66231, #8569, #79286, #21604, #47264, #72954, #15305, #24491, #18196, #36301, #10230, #69533, #67893, #17383, #43830, #43421, #54830, #50158, #74625, #37124, #35897, #11049, #36707, #62808, #74206, #82175, #80940, #29160, #81768, #17786, #16969, #16553, #3910, #61567, #11883, #29571, #75854, #22846, #49747, #37535, #42197, #10646, #30393, #42608, #30807, #3495, #24078, #5142, #23665, #80535, #55233, #48925, #4719, #23255, #68309, #62382, #61977, #48507, #4314, #56058, #75448, #69118, #29979, #55642, #81353, #49337, #75037, #43013, #68708, #11467, #56472, #52232, #5960, #31630, #77090, #13965, #77935, #76268, #45498, #25725, #26148, #6792, #69934, #57290, #25309, #51809, #82988, #32464, #13128, #19422, #63623, #45074, #63211, #19003, #39194, #50973, #20265, #922, #24895, #38779, #7216, #12290, #19849, #70777, #64877, #45915, #64456, #58126, #77514, #493, #76670, #64038, #32887, #71195, #13537, #58556, #26579, #44652, #71613, #5551, #31215, #70348, #50564, #56883, #44245, #82576, #18602, #37946, #12703, #38362, #6377, #32049, #57709, #71, #51385, #1337, #41287, #21927, #27826, #79196, #21512, #21100, #72033, #73282, #65733, #7650, #15630, #40458, #53486, #33727, #47588, #14389, #40047, #66137, #39621, #65311, #20688, #60228, #8475, #40871, #47170, #8066, #59389, #1747, #66553, #27404, #72862, #15211, #2160, #53065, #8886, #33320, #78776, #53896, #46759, #58982, #26987, #72452, #34563, #52651, #14801, #79610, #2578, #78356, #46339, #34144, #59805, #28237, #13396, #31907, #32321, #1194, #45355, #58409, #26430, #65163, #57568, #78211, #20543, #71890, #44927, #18867, #39049, #12560, #13817, #46195, #26843, #65587, #25582, #38636, #57983, #64314, #83260, #51246, #52502, #14241, #6648, #38218, #39899, #63893, #71052, #31489, #71469, #82849, #57150, #19275, #7499, #6231, #64734, #7072, #33168, #44516, #25170, #76948, #50839, #52081, #45770, #70624, #70203, #12980, #348, #76539, #26005, #51662, #77366, #77790, #19698, #32742, #768, #20123, #39476, #58836, #7920, #28509, #67241, #28095, #41959, #8331, #8744, #60906, #21778, #34836, #2845, #41553, #33997, #54587, #80297, #48271, #21371, #78633, #15484, #72310, #73560, #22611, #3258, #33581, #2015, #15065, #34415, #40721, #59659, #27679, #28919, #73969, #66407, #14657, #16314, #40314, #47440, #59244, #47855, #1603, #27259, #79054, #9572, #65993, #41141, #66831, #35242, #20957, #52919, #53344, #46615, #54166, #22198, #47026, #72718, #60083, #2437, #53751, #79461, #73134, #9164, #79881, #60496, #15904, #54601, #41155, #67665, #29350, #66843, #8345, #40736, #53358, #60098, #79893, #66420, #22625, #34432, #34011, #73572, #41565, #8756, #3271, #60920, #15078, #54180, #79475, #80310, #9177, #2452, #47868, #47039, #79068, #48285, #34848, #48698, #59673, #60511, #21384, #2028, #2859, #73982, #28110, #72732, #35256, #35667, #16328, #15917, #22211, #27694, #67254, #28523, #21791, #9587, #41972, #28932, #10002, #61331, #66007, #3685, #53764, #47454, #55009, #73148, #80717, #15497, #23032, #74396, #40328, #10423, #23859, #30989, #43197, #44027, #36081, #5331, #56657, #23444, #30588, #43609, #55420, #5731, #82358, #17564, #69720, #31402, #68892, #68079, #17159, #29757, #36486, #56254, #42792, #24676, #10826, #61752, #49936, #17972, #68487, #62992, #37320, #74814, #81950, #55832, #50344, #11242, #62161, #24263, #49108, #81127, #76041, #36902, #25082, #4089, #62578, #4502, #30169, #4920, #18386, #81540, #49526, #11661, #12064, #37722, #75634, #69311, #75219, #63396, #57067, #82761, #50756, #16740, #42380, #58318, #70965, #18783, #71801, #31821, #44427, #681, #32237, #14154, #70121, #262, #19607, #40953, #12472, #25915, #7408, #45269, #60309, #78122, #76857, #8970, #19189, #66633, #12892, #51574, #83175, #38551, #58745, #1107, #34644, #38134, #64231, #77277, #57481, #26758, #13730, #25495, #6565, #44838, #2658, #28317, #51161, #76456, #57895, #63808, #52413, #13310, #6147, #26337, #70536, #38962, #64646, #6983, #32652, #51998, #77703, #20033, #20455, #45684, #71380, #39384, #65069, #46108, #33078, #23239 ) ),
 .UNSPECIFIED., .F., .F., .F. ) 
 B_SPLINE_SURFACE_WITH_KNOTS ( ( 2, 2 ),
 ( 3, 2, 2, 2, 2, 2, 2, 2, 2, 2, 2, 2, 2, 2, 2, 2, 2, 2, 2, 2, 2, 2, 2, 2, 2, 2, 2, 2, 2, 2, 2, 2, 2, 2, 2, 2, 2, 2, 2, 2, 2, 2, 2, 2, 2, 2, 2, 2, 2, 2, 2, 2, 2, 2, 2, 2, 2, 2, 2, 2, 2, 2, 2, 2, 2, 2, 2, 2, 2, 2, 2, 2, 2, 2, 2, 2, 2, 2, 2, 2, 2, 2, 2, 2, 2, 2, 2, 2, 2, 2, 2, 2, 2, 2, 2, 2, 2, 2, 2, 2, 2, 2, 2, 2, 2, 2, 2, 2, 2, 2, 2, 2, 2, 2, 2, 2, 2, 2, 2, 2, 2, 2, 2, 2, 2, 2, 2, 2, 2, 2, 2, 2, 2, 2, 2, 2, 2, 2, 2, 2, 2, 2, 2, 2, 2, 2, 2, 2, 2, 2, 2, 2, 2, 2, 2, 2, 2, 2, 2, 2, 2, 2, 2, 2, 2, 2, 2, 2, 2, 2, 2, 2, 2, 2, 2, 2, 2, 2, 2, 2, 2, 2, 2, 2, 2, 2, 2, 2, 2, 2, 2, 2, 2, 2, 2, 2, 2, 2, 2, 2, 2, 2, 2, 2, 2, 2, 2, 2, 2, 2, 2, 2, 2, 2, 2, 2, 2, 2, 2, 2, 2, 2, 2, 2, 2, 2, 2, 2, 2, 2, 2, 2, 2, 2, 2, 2, 2, 2, 2, 2, 2, 2, 2, 2, 2, 2, 2, 2, 2, 2, 2, 2, 2, 2, 2, 3 ),
 ( 0.000000000000000000, 1.000000000000000000 ),
 ( 0.000000000000000000, 0.003787878787878787984, 0.007575757575757575968, 0.01136363636363636395, 0.01515151515151515194, 0.01893939393939393992, 0.02272727272727272790, 0.02651515151515151589, 0.03030303030303030387, 0.03409090909090908839, 0.03787878787878787984, 0.04166666666666666435, 0.04545454545454545581, 0.04924242424242424032, 0.05303030303030303177, 0.05681818181818181629, 0.06060606060606060774, 0.06439393939393939226, 0.06818181818181817677, 0.07196969696969697516, 0.07575757575757575968, 0.07954545454545454419, 0.08333333333333332871, 0.08712121212121212710, 0.09090909090909091161, 0.09469696969696969613, 0.09848484848484848064, 0.1022727272727272790, 0.1060606060606060635, 0.1098484848484848481, 0.1136363636363636326, 0.1174242424242424310, 0.1212121212121212155, 0.1250000000000000000, 0.1287878787878787845, 0.1325757575757575690, 0.1363636363636363535, 0.1401515151515151381, 0.1439393939393939503, 0.1477272727272727348, 0.1515151515151515194, 0.1553030303030303039, 0.1590909090909090884, 0.1628787878787878729, 0.1666666666666666574, 0.1704545454545454419, 0.1742424242424242542, 0.1780303030303030387, 0.1818181818181818232, 0.1856060606060606077, 0.1893939393939393923, 0.1931818181818181768, 0.1969696969696969613, 0.2007575757575757458, 0.2045454545454545581, 0.2083333333333333426, 0.2121212121212121271, 0.2159090909090909116, 0.2196969696969696961, 0.2234848484848484806, 0.2272727272727272652, 0.2310606060606060497, 0.2348484848484848619, 0.2386363636363636465, 0.2424242424242424310, 0.2462121212121212155, 0.2500000000000000000, 0.2537878787878787845, 0.2575757575757575690, 0.2613636363636363535, 0.2651515151515151381, 0.2689393939393939226, 0.2727272727272727071, 0.2765151515151514916, 0.2803030303030302761, 0.2840909090909091161, 0.2878787878787879007, 0.2916666666666666852, 0.2954545454545454697, 0.2992424242424242542, 0.3030303030303030387, 0.3068181818181818232, 0.3106060606060606077, 0.3143939393939393923, 0.3181818181818181768, 0.3219696969696969613, 0.3257575757575757458, 0.3295454545454545303, 0.3333333333333333148, 0.3371212121212120993, 0.3409090909090908839, 0.3446969696969697239, 0.3484848484848485084, 0.3522727272727272929, 0.3560606060606060774, 0.3598484848484848619, 0.3636363636363636465, 0.3674242424242424310, 0.3712121212121212155, 0.3750000000000000000, 0.3787878787878787845, 0.3825757575757575690, 0.3863636363636363535, 0.3901515151515151381, 0.3939393939393939226, 0.3977272727272727071, 0.4015151515151514916, 0.4053030303030302761, 0.4090909090909091161, 0.4128787878787879007, 0.4166666666666666852, 0.4204545454545454697, 0.4242424242424242542, 0.4280303030303030387, 0.4318181818181818232, 0.4356060606060606077, 0.4393939393939393923, 0.4431818181818181768, 0.4469696969696969613, 0.4507575757575757458, 0.4545454545454545303, 0.4583333333333333148, 0.4621212121212120993, 0.4659090909090908839, 0.4696969696969697239, 0.4734848484848485084, 0.4772727272727272929, 0.4810606060606060774, 0.4848484848484848619, 0.4886363636363636465, 0.4924242424242424310, 0.4962121212121212155, 0.5000000000000000000, 0.5037878787878787845, 0.5075757575757575690, 0.5113636363636363535, 0.5151515151515151381, 0.5189393939393939226, 0.5227272727272727071, 0.5265151515151514916, 0.5303030303030302761, 0.5340909090909090606, 0.5378787878787878451, 0.5416666666666666297, 0.5454545454545454142, 0.5492424242424241987, 0.5530303030303029832, 0.5568181818181817677, 0.5606060606060605522, 0.5643939393939394478, 0.5681818181818182323, 0.5719696969696970168, 0.5757575757575758013, 0.5795454545454545858, 0.5833333333333333703, 0.5871212121212121549, 0.5909090909090909394, 0.5946969696969697239, 0.5984848484848485084, 0.6022727272727272929, 0.6060606060606060774, 0.6098484848484848619, 0.6136363636363636465, 0.6174242424242424310, 0.6212121212121212155, 0.6250000000000000000, 0.6287878787878787845, 0.6325757575757575690, 0.6363636363636363535, 0.6401515151515151381, 0.6439393939393939226, 0.6477272727272727071, 0.6515151515151514916, 0.6553030303030302761, 0.6590909090909090606, 0.6628787878787878451, 0.6666666666666666297, 0.6704545454545454142, 0.6742424242424241987, 0.6780303030303029832, 0.6818181818181817677, 0.6856060606060605522, 0.6893939393939394478, 0.6931818181818182323, 0.6969696969696970168, 0.7007575757575758013, 0.7045454545454545858, 0.7083333333333333703, 0.7121212121212121549, 0.7159090909090909394, 0.7196969696969697239, 0.7234848484848485084, 0.7272727272727272929, 0.7310606060606060774, 0.7348484848484848619, 0.7386363636363636465, 0.7424242424242424310, 0.7462121212121212155, 0.7500000000000000000, 0.7537878787878787845, 0.7575757575757575690, 0.7613636363636363535, 0.7651515151515151381, 0.7689393939393939226, 0.7727272727272727071, 0.7765151515151514916, 0.7803030303030302761, 0.7840909090909090606, 0.7878787878787878451, 0.7916666666666666297, 0.7954545454545454142, 0.7992424242424241987, 0.8030303030303029832, 0.8068181818181817677, 0.8106060606060605522, 0.8143939393939394478, 0.8181818181818182323, 0.8219696969696970168, 0.8257575757575758013, 0.8295454545454545858, 0.8333333333333333703, 0.8371212121212121549, 0.8409090909090909394, 0.8446969696969697239, 0.8484848484848485084, 0.8522727272727272929, 0.8560606060606060774, 0.8598484848484848619, 0.8636363636363636465, 0.8674242424242424310, 0.8712121212121212155, 0.8750000000000000000, 0.8787878787878787845, 0.8825757575757575690, 0.8863636363636363535, 0.8901515151515151381, 0.8939393939393939226, 0.8977272727272727071, 0.9015151515151514916, 0.9053030303030302761, 0.9090909090909090606, 0.9128787878787878451, 0.9166666666666666297, 0.9204545454545454142, 0.9242424242424241987, 0.9280303030303029832, 0.9318181818181817677, 0.9356060606060605522, 0.9393939393939394478, 0.9431818181818182323, 0.9469696969696970168, 0.9507575757575758013, 0.9545454545454545858, 0.9583333333333333703, 0.9621212121212121549, 0.9659090909090909394 ),
 .UNSPECIFIED. ) 
 GEOMETRIC_REPRESENTATION_ITEM ( )  RATIONAL_B_SPLINE_SURFACE ( (
 ( 1.000000000000000000, 0.9659258262890683122, 1.000000000000000000, 0.9659258262890683122, 1.000000000000000000, 0.9659258262890683122, 1.000000000000000000, 0.9659258262890683122, 1.000000000000000000, 0.9659258262890683122, 1.000000000000000000, 0.9659258262890683122, 1.000000000000000000, 0.9659258262890683122, 1.000000000000000000, 0.9659258262890683122, 1.000000000000000000, 0.9659258262890683122, 1.000000000000000000, 0.9659258262890683122, 1.000000000000000000, 0.9659258262890683122, 1.000000000000000000, 0.9659258262890683122, 1.000000000000000000, 0.9659258262890683122, 1.000000000000000000, 0.9659258262890683122, 1.000000000000000000, 0.9659258262890683122, 1.000000000000000000, 0.9659258262890683122, 1.000000000000000000, 0.9659258262890683122, 1.000000000000000000, 0.9659258262890683122, 1.000000000000000000, 0.9659258262890683122, 1.000000000000000000, 0.9659258262890683122, 1.000000000000000000, 0.9659258262890683122, 1.000000000000000000, 0.9659258262890683122, 1.000000000000000000, 0.9659258262890683122, 1.000000000000000000, 0.9659258262890683122, 1.000000000000000000, 0.9659258262890683122, 1.000000000000000000, 0.9659258262890683122, 1.000000000000000000, 0.9659258262890683122, 1.000000000000000000, 0.9659258262890683122, 1.000000000000000000, 0.9659258262890683122, 1.000000000000000000, 0.9659258262890683122, 1.000000000000000000, 0.9659258262890683122, 1.000000000000000000, 0.9659258262890683122, 1.000000000000000000, 0.9659258262890683122, 1.000000000000000000, 0.9659258262890683122, 1.000000000000000000, 0.9659258262890683122, 1.000000000000000000, 0.9659258262890683122, 1.000000000000000000, 0.9659258262890683122, 1.000000000000000000, 0.9659258262890683122, 1.000000000000000000, 0.9659258262890683122, 1.000000000000000000, 0.9659258262890683122, 1.000000000000000000, 0.9659258262890683122, 1.000000000000000000, 0.9659258262890683122, 1.000000000000000000, 0.9659258262890683122, 1.000000000000000000, 0.9659258262890683122, 1.000000000000000000, 0.9659258262890683122, 1.000000000000000000, 0.9659258262890683122, 1.000000000000000000, 0.9659258262890683122, 1.000000000000000000, 0.9659258262890683122, 1.000000000000000000, 0.9659258262890683122, 1.000000000000000000, 0.9659258262890683122, 1.000000000000000000, 0.9659258262890683122, 1.000000000000000000, 0.9659258262890683122, 1.000000000000000000, 0.9659258262890683122, 1.000000000000000000, 0.9659258262890683122, 1.000000000000000000, 0.9659258262890683122, 1.000000000000000000, 0.9659258262890683122, 1.000000000000000000, 0.9659258262890683122, 1.000000000000000000, 0.9659258262890683122, 1.000000000000000000, 0.9659258262890683122, 1.000000000000000000, 0.9659258262890683122, 1.000000000000000000, 0.9659258262890683122, 1.000000000000000000, 0.9659258262890683122, 1.000000000000000000, 0.9659258262890683122, 1.000000000000000000, 0.9659258262890683122, 1.000000000000000000, 0.9659258262890683122, 1.000000000000000000, 0.9659258262890683122, 1.000000000000000000, 0.9659258262890683122, 1.000000000000000000, 0.9659258262890683122, 1.000000000000000000, 0.9659258262890683122, 1.000000000000000000, 0.9659258262890683122, 1.000000000000000000, 0.9659258262890683122, 1.000000000000000000, 0.9659258262890683122, 1.000000000000000000, 0.9659258262890683122, 1.000000000000000000, 0.9659258262890683122, 1.000000000000000000, 0.9659258262890683122, 1.000000000000000000, 0.9659258262890683122, 1.000000000000000000, 0.9659258262890683122, 1.000000000000000000, 0.9659258262890683122, 1.000000000000000000, 0.9659258262890683122, 1.000000000000000000, 0.9659258262890683122, 1.000000000000000000, 0.9659258262890683122, 1.000000000000000000, 0.9659258262890683122, 1.000000000000000000, 0.9659258262890683122, 1.000000000000000000, 0.9659258262890683122, 1.000000000000000000, 0.9659258262890683122, 1.000000000000000000, 0.9659258262890683122, 1.000000000000000000, 0.9659258262890683122, 1.000000000000000000, 0.9659258262890683122, 1.000000000000000000, 0.9659258262890683122, 1.000000000000000000, 0.9659258262890683122, 1.000000000000000000, 0.9659258262890683122, 1.000000000000000000, 0.9659258262890683122, 1.000000000000000000, 0.9659258262890683122, 1.000000000000000000, 0.9659258262890683122, 1.000000000000000000, 0.9659258262890683122, 1.000000000000000000, 0.9659258262890683122, 1.000000000000000000, 0.9659258262890683122, 1.000000000000000000, 0.9659258262890683122, 1.000000000000000000, 0.9659258262890683122, 1.000000000000000000, 0.9659258262890683122, 1.000000000000000000, 0.9659258262890683122, 1.000000000000000000, 0.9659258262890683122, 1.000000000000000000, 0.9659258262890683122, 1.000000000000000000, 0.9659258262890683122, 1.000000000000000000, 0.9659258262890683122, 1.000000000000000000, 0.9659258262890683122, 1.000000000000000000, 0.9659258262890683122, 1.000000000000000000, 0.9659258262890683122, 1.000000000000000000, 0.9659258262890683122, 1.000000000000000000, 0.9659258262890683122, 1.000000000000000000, 0.9659258262890683122, 1.000000000000000000, 0.9659258262890683122, 1.000000000000000000, 0.9659258262890683122, 1.000000000000000000, 0.9659258262890683122, 1.000000000000000000, 0.9659258262890683122, 1.000000000000000000, 0.9659258262890683122, 1.000000000000000000, 0.9659258262890683122, 1.000000000000000000, 0.9659258262890683122, 1.000000000000000000, 0.9659258262890683122, 1.000000000000000000, 0.9659258262890683122, 1.000000000000000000, 0.9659258262890683122, 1.000000000000000000, 0.9659258262890683122, 1.000000000000000000, 0.9659258262890683122, 1.000000000000000000, 0.9659258262890683122, 1.000000000000000000, 0.9659258262890683122, 1.000000000000000000, 0.9659258262890683122, 1.000000000000000000, 0.9659258262890683122, 1.000000000000000000, 0.9659258262890683122, 1.000000000000000000, 0.9659258262890683122, 1.000000000000000000, 0.9659258262890683122, 1.000000000000000000, 0.9659258262890683122, 1.000000000000000000, 0.9659258262890683122, 1.000000000000000000, 0.9659258262890683122, 1.000000000000000000, 0.9659258262890683122, 1.000000000000000000, 0.9659258262890683122, 1.000000000000000000, 0.9659258262890683122, 1.000000000000000000, 0.9659258262890683122, 1.000000000000000000, 0.9659258262890683122, 1.000000000000000000, 0.9659258262890683122, 1.000000000000000000, 0.9659258262890683122, 1.000000000000000000, 0.9659258262890683122, 1.000000000000000000, 0.9659258262890683122, 1.000000000000000000, 0.9659258262890683122, 1.000000000000000000, 0.9659258262890683122, 1.000000000000000000, 0.9659258262890683122, 1.000000000000000000, 0.9659258262890683122, 1.000000000000000000, 0.9659258262890683122, 1.000000000000000000, 0.9659258262890683122, 1.000000000000000000, 0.9659258262890683122, 1.000000000000000000, 0.9659258262890683122, 1.000000000000000000, 0.9659258262890683122, 1.000000000000000000, 0.9659258262890683122, 1.000000000000000000, 0.9659258262890683122, 1.000000000000000000, 0.9659258262890683122, 1.000000000000000000, 0.9659258262890683122, 1.000000000000000000, 0.9659258262890683122, 1.000000000000000000, 0.9659258262890683122, 1.000000000000000000, 0.9659258262890683122, 1.000000000000000000, 0.9659258262890683122, 1.000000000000000000, 0.9659258262890683122, 1.000000000000000000, 0.9659258262890683122, 1.000000000000000000, 0.9659258262890683122, 1.000000000000000000, 0.9659258262890683122, 1.000000000000000000, 0.9659258262890683122, 1.000000000000000000, 0.9659258262890683122, 1.000000000000000000, 0.9659258262890683122, 1.000000000000000000, 0.9659258262890683122, 1.000000000000000000, 0.9659258262890683122, 1.000000000000000000, 0.9659258262890683122, 1.000000000000000000, 0.9659258262890683122, 1.000000000000000000, 0.9659258262890683122, 1.000000000000000000, 0.9659258262890683122, 1.000000000000000000, 0.9659258262890683122, 1.000000000000000000, 0.9659258262890683122, 1.000000000000000000, 0.9659258262890683122, 1.000000000000000000, 0.9659258262890683122, 1.000000000000000000, 0.9659258262890683122, 1.000000000000000000, 0.9659258262890683122, 1.000000000000000000, 0.9659258262890683122, 1.000000000000000000, 0.9659258262890683122, 1.000000000000000000, 0.9659258262890683122, 1.000000000000000000, 0.9659258262890683122, 1.000000000000000000, 0.9659258262890683122, 1.000000000000000000, 0.9659258262890683122, 1.000000000000000000, 0.9659258262890683122, 1.000000000000000000, 0.9659258262890683122, 1.000000000000000000, 0.9659258262890683122, 1.000000000000000000, 0.9659258262890683122, 1.000000000000000000, 0.9659258262890683122, 1.000000000000000000, 0.9659258262890683122, 1.000000000000000000, 0.9659258262890683122, 1.000000000000000000, 0.9659258262890683122, 1.000000000000000000, 0.9659258262890683122, 1.000000000000000000, 0.9659258262890683122, 1.000000000000000000, 0.9659258262890683122, 1.000000000000000000, 0.9659258262890683122, 1.000000000000000000, 0.9659258262890683122, 1.000000000000000000, 0.9659258262890683122, 1.000000000000000000, 0.9659258262890683122, 1.000000000000000000, 0.9659258262890683122, 1.000000000000000000, 0.9659258262890683122, 1.000000000000000000, 0.9659258262890683122, 1.000000000000000000, 0.9659258262890683122, 1.000000000000000000, 0.9659258262890683122, 1.000000000000000000, 0.9659258262890683122, 1.000000000000000000, 0.9659258262890683122, 1.000000000000000000, 0.9659258262890683122, 1.000000000000000000, 0.9659258262890683122, 1.000000000000000000, 0.9659258262890683122, 1.000000000000000000, 0.9659258262890683122, 1.000000000000000000, 0.9659258262890683122, 1.000000000000000000, 0.9659258262890683122, 1.000000000000000000, 0.9659258262890683122, 1.000000000000000000, 0.9659258262890683122, 1.000000000000000000, 0.9659258262890683122, 1.000000000000000000, 0.9659258262890683122, 1.000000000000000000, 0.9659258262890683122, 1.000000000000000000, 0.9659258262890683122, 1.000000000000000000, 0.9659258262890683122, 1.000000000000000000, 0.9659258262890683122, 1.000000000000000000, 0.9659258262890683122, 1.000000000000000000, 0.9659258262890683122, 1.000000000000000000, 0.9659258262890683122, 1.000000000000000000, 0.9659258262890683122, 1.000000000000000000, 0.9659258262890683122, 1.000000000000000000, 0.9659258262890683122, 1.000000000000000000, 0.9659258262890683122, 1.000000000000000000, 0.9659258262890683122, 1.000000000000000000, 0.9659258262890683122, 1.000000000000000000, 0.9659258262890683122, 1.000000000000000000, 0.9659258262890683122, 1.000000000000000000, 0.9659258262890683122, 1.000000000000000000, 0.9659258262890683122, 1.000000000000000000, 0.9659258262890683122, 1.000000000000000000, 0.9659258262890683122, 1.000000000000000000, 0.9659258262890683122, 1.000000000000000000, 0.9659258262890683122, 1.000000000000000000, 0.9659258262890683122, 1.000000000000000000, 0.9659258262890683122, 1.000000000000000000, 0.9659258262890683122, 1.000000000000000000, 0.9659258262890683122, 1.000000000000000000, 0.9659258262890683122, 1.000000000000000000, 0.9659258262890683122, 1.000000000000000000, 0.9659258262890683122, 1.000000000000000000, 0.9659258262890683122, 1.000000000000000000, 0.9659258262890683122, 1.000000000000000000, 0.9659258262890683122, 1.000000000000000000, 0.9659258262890683122, 1.000000000000000000, 0.9659258262890683122, 1.000000000000000000, 0.9659258262890683122, 1.000000000000000000, 0.9659258262890683122, 1.000000000000000000, 0.9659258262890683122, 1.000000000000000000, 0.9659258262890683122, 1.000000000000000000, 0.9659258262890683122, 1.000000000000000000, 0.9659258262890683122, 1.000000000000000000),
 ( 1.000000000000000000, 0.9659258262890683122, 1.000000000000000000, 0.9659258262890683122, 1.000000000000000000, 0.9659258262890683122, 1.000000000000000000, 0.9659258262890683122, 1.000000000000000000, 0.9659258262890683122, 1.000000000000000000, 0.9659258262890683122, 1.000000000000000000, 0.9659258262890683122, 1.000000000000000000, 0.9659258262890683122, 1.000000000000000000, 0.9659258262890683122, 1.000000000000000000, 0.9659258262890683122, 1.000000000000000000, 0.9659258262890683122, 1.000000000000000000, 0.9659258262890683122, 1.000000000000000000, 0.9659258262890683122, 1.000000000000000000, 0.9659258262890683122, 1.000000000000000000, 0.9659258262890683122, 1.000000000000000000, 0.9659258262890683122, 1.000000000000000000, 0.9659258262890683122, 1.000000000000000000, 0.9659258262890683122, 1.000000000000000000, 0.9659258262890683122, 1.000000000000000000, 0.9659258262890683122, 1.000000000000000000, 0.9659258262890683122, 1.000000000000000000, 0.9659258262890683122, 1.000000000000000000, 0.9659258262890683122, 1.000000000000000000, 0.9659258262890683122, 1.000000000000000000, 0.9659258262890683122, 1.000000000000000000, 0.9659258262890683122, 1.000000000000000000, 0.9659258262890683122, 1.000000000000000000, 0.9659258262890683122, 1.000000000000000000, 0.9659258262890683122, 1.000000000000000000, 0.9659258262890683122, 1.000000000000000000, 0.9659258262890683122, 1.000000000000000000, 0.9659258262890683122, 1.000000000000000000, 0.9659258262890683122, 1.000000000000000000, 0.9659258262890683122, 1.000000000000000000, 0.9659258262890683122, 1.000000000000000000, 0.9659258262890683122, 1.000000000000000000, 0.9659258262890683122, 1.000000000000000000, 0.9659258262890683122, 1.000000000000000000, 0.9659258262890683122, 1.000000000000000000, 0.9659258262890683122, 1.000000000000000000, 0.9659258262890683122, 1.000000000000000000, 0.9659258262890683122, 1.000000000000000000, 0.9659258262890683122, 1.000000000000000000, 0.9659258262890683122, 1.000000000000000000, 0.9659258262890683122, 1.000000000000000000, 0.9659258262890683122, 1.000000000000000000, 0.9659258262890683122, 1.000000000000000000, 0.9659258262890683122, 1.000000000000000000, 0.9659258262890683122, 1.000000000000000000, 0.9659258262890683122, 1.000000000000000000, 0.9659258262890683122, 1.000000000000000000, 0.9659258262890683122, 1.000000000000000000, 0.9659258262890683122, 1.000000000000000000, 0.9659258262890683122, 1.000000000000000000, 0.9659258262890683122, 1.000000000000000000, 0.9659258262890683122, 1.000000000000000000, 0.9659258262890683122, 1.000000000000000000, 0.9659258262890683122, 1.000000000000000000, 0.9659258262890683122, 1.000000000000000000, 0.9659258262890683122, 1.000000000000000000, 0.9659258262890683122, 1.000000000000000000, 0.9659258262890683122, 1.000000000000000000, 0.9659258262890683122, 1.000000000000000000, 0.9659258262890683122, 1.000000000000000000, 0.9659258262890683122, 1.000000000000000000, 0.9659258262890683122, 1.000000000000000000, 0.9659258262890683122, 1.000000000000000000, 0.9659258262890683122, 1.000000000000000000, 0.9659258262890683122, 1.000000000000000000, 0.9659258262890683122, 1.000000000000000000, 0.9659258262890683122, 1.000000000000000000, 0.9659258262890683122, 1.000000000000000000, 0.9659258262890683122, 1.000000000000000000, 0.9659258262890683122, 1.000000000000000000, 0.9659258262890683122, 1.000000000000000000, 0.9659258262890683122, 1.000000000000000000, 0.9659258262890683122, 1.000000000000000000, 0.9659258262890683122, 1.000000000000000000, 0.9659258262890683122, 1.000000000000000000, 0.9659258262890683122, 1.000000000000000000, 0.9659258262890683122, 1.000000000000000000, 0.9659258262890683122, 1.000000000000000000, 0.9659258262890683122, 1.000000000000000000, 0.9659258262890683122, 1.000000000000000000, 0.9659258262890683122, 1.000000000000000000, 0.9659258262890683122, 1.000000000000000000, 0.9659258262890683122, 1.000000000000000000, 0.9659258262890683122, 1.000000000000000000, 0.9659258262890683122, 1.000000000000000000, 0.9659258262890683122, 1.000000000000000000, 0.9659258262890683122, 1.000000000000000000, 0.9659258262890683122, 1.000000000000000000, 0.9659258262890683122, 1.000000000000000000, 0.9659258262890683122, 1.000000000000000000, 0.9659258262890683122, 1.000000000000000000, 0.9659258262890683122, 1.000000000000000000, 0.9659258262890683122, 1.000000000000000000, 0.9659258262890683122, 1.000000000000000000, 0.9659258262890683122, 1.000000000000000000, 0.9659258262890683122, 1.000000000000000000, 0.9659258262890683122, 1.000000000000000000, 0.9659258262890683122, 1.000000000000000000, 0.9659258262890683122, 1.000000000000000000, 0.9659258262890683122, 1.000000000000000000, 0.9659258262890683122, 1.000000000000000000, 0.9659258262890683122, 1.000000000000000000, 0.9659258262890683122, 1.000000000000000000, 0.9659258262890683122, 1.000000000000000000, 0.9659258262890683122, 1.000000000000000000, 0.9659258262890683122, 1.000000000000000000, 0.9659258262890683122, 1.000000000000000000, 0.9659258262890683122, 1.000000000000000000, 0.9659258262890683122, 1.000000000000000000, 0.9659258262890683122, 1.000000000000000000, 0.9659258262890683122, 1.000000000000000000, 0.9659258262890683122, 1.000000000000000000, 0.9659258262890683122, 1.000000000000000000, 0.9659258262890683122, 1.000000000000000000, 0.9659258262890683122, 1.000000000000000000, 0.9659258262890683122, 1.000000000000000000, 0.9659258262890683122, 1.000000000000000000, 0.9659258262890683122, 1.000000000000000000, 0.9659258262890683122, 1.000000000000000000, 0.9659258262890683122, 1.000000000000000000, 0.9659258262890683122, 1.000000000000000000, 0.9659258262890683122, 1.000000000000000000, 0.9659258262890683122, 1.000000000000000000, 0.9659258262890683122, 1.000000000000000000, 0.9659258262890683122, 1.000000000000000000, 0.9659258262890683122, 1.000000000000000000, 0.9659258262890683122, 1.000000000000000000, 0.9659258262890683122, 1.000000000000000000, 0.9659258262890683122, 1.000000000000000000, 0.9659258262890683122, 1.000000000000000000, 0.9659258262890683122, 1.000000000000000000, 0.9659258262890683122, 1.000000000000000000, 0.9659258262890683122, 1.000000000000000000, 0.9659258262890683122, 1.000000000000000000, 0.9659258262890683122, 1.000000000000000000, 0.9659258262890683122, 1.000000000000000000, 0.9659258262890683122, 1.000000000000000000, 0.9659258262890683122, 1.000000000000000000, 0.9659258262890683122, 1.000000000000000000, 0.9659258262890683122, 1.000000000000000000, 0.9659258262890683122, 1.000000000000000000, 0.9659258262890683122, 1.000000000000000000, 0.9659258262890683122, 1.000000000000000000, 0.9659258262890683122, 1.000000000000000000, 0.9659258262890683122, 1.000000000000000000, 0.9659258262890683122, 1.000000000000000000, 0.9659258262890683122, 1.000000000000000000, 0.9659258262890683122, 1.000000000000000000, 0.9659258262890683122, 1.000000000000000000, 0.9659258262890683122, 1.000000000000000000, 0.9659258262890683122, 1.000000000000000000, 0.9659258262890683122, 1.000000000000000000, 0.9659258262890683122, 1.000000000000000000, 0.9659258262890683122, 1.000000000000000000, 0.9659258262890683122, 1.000000000000000000, 0.9659258262890683122, 1.000000000000000000, 0.9659258262890683122, 1.000000000000000000, 0.9659258262890683122, 1.000000000000000000, 0.9659258262890683122, 1.000000000000000000, 0.9659258262890683122, 1.000000000000000000, 0.9659258262890683122, 1.000000000000000000, 0.9659258262890683122, 1.000000000000000000, 0.9659258262890683122, 1.000000000000000000, 0.9659258262890683122, 1.000000000000000000, 0.9659258262890683122, 1.000000000000000000, 0.9659258262890683122, 1.000000000000000000, 0.9659258262890683122, 1.000000000000000000, 0.9659258262890683122, 1.000000000000000000, 0.9659258262890683122, 1.000000000000000000, 0.9659258262890683122, 1.000000000000000000, 0.9659258262890683122, 1.000000000000000000, 0.9659258262890683122, 1.000000000000000000, 0.9659258262890683122, 1.000000000000000000, 0.9659258262890683122, 1.000000000000000000, 0.9659258262890683122, 1.000000000000000000, 0.9659258262890683122, 1.000000000000000000, 0.9659258262890683122, 1.000000000000000000, 0.9659258262890683122, 1.000000000000000000, 0.9659258262890683122, 1.000000000000000000, 0.9659258262890683122, 1.000000000000000000, 0.9659258262890683122, 1.000000000000000000, 0.9659258262890683122, 1.000000000000000000, 0.9659258262890683122, 1.000000000000000000, 0.9659258262890683122, 1.000000000000000000, 0.9659258262890683122, 1.000000000000000000, 0.9659258262890683122, 1.000000000000000000, 0.9659258262890683122, 1.000000000000000000, 0.9659258262890683122, 1.000000000000000000, 0.9659258262890683122, 1.000000000000000000, 0.9659258262890683122, 1.000000000000000000, 0.9659258262890683122, 1.000000000000000000, 0.9659258262890683122, 1.000000000000000000, 0.9659258262890683122, 1.000000000000000000, 0.9659258262890683122, 1.000000000000000000, 0.9659258262890683122, 1.000000000000000000, 0.9659258262890683122, 1.000000000000000000, 0.9659258262890683122, 1.000000000000000000, 0.9659258262890683122, 1.000000000000000000, 0.9659258262890683122, 1.000000000000000000, 0.9659258262890683122, 1.000000000000000000, 0.9659258262890683122, 1.000000000000000000, 0.9659258262890683122, 1.000000000000000000, 0.9659258262890683122, 1.000000000000000000, 0.9659258262890683122, 1.000000000000000000, 0.9659258262890683122, 1.000000000000000000, 0.9659258262890683122, 1.000000000000000000, 0.9659258262890683122, 1.000000000000000000, 0.9659258262890683122, 1.000000000000000000, 0.9659258262890683122, 1.000000000000000000, 0.9659258262890683122, 1.000000000000000000, 0.9659258262890683122, 1.000000000000000000, 0.9659258262890683122, 1.000000000000000000, 0.9659258262890683122, 1.000000000000000000, 0.9659258262890683122, 1.000000000000000000, 0.9659258262890683122, 1.000000000000000000, 0.9659258262890683122, 1.000000000000000000, 0.9659258262890683122, 1.000000000000000000, 0.9659258262890683122, 1.000000000000000000, 0.9659258262890683122, 1.000000000000000000, 0.9659258262890683122, 1.000000000000000000, 0.9659258262890683122, 1.000000000000000000, 0.9659258262890683122, 1.000000000000000000, 0.9659258262890683122, 1.000000000000000000, 0.9659258262890683122, 1.000000000000000000, 0.9659258262890683122, 1.000000000000000000, 0.9659258262890683122, 1.000000000000000000, 0.9659258262890683122, 1.000000000000000000, 0.9659258262890683122, 1.000000000000000000, 0.9659258262890683122, 1.000000000000000000, 0.9659258262890683122, 1.000000000000000000, 0.9659258262890683122, 1.000000000000000000, 0.9659258262890683122, 1.000000000000000000, 0.9659258262890683122, 1.000000000000000000, 0.9659258262890683122, 1.000000000000000000, 0.9659258262890683122, 1.000000000000000000, 0.9659258262890683122, 1.000000000000000000, 0.9659258262890683122, 1.000000000000000000, 0.9659258262890683122, 1.000000000000000000, 0.9659258262890683122, 1.000000000000000000, 0.9659258262890683122, 1.000000000000000000, 0.9659258262890683122, 1.000000000000000000, 0.9659258262890683122, 1.000000000000000000, 0.9659258262890683122, 1.000000000000000000, 0.9659258262890683122, 1.000000000000000000, 0.9659258262890683122, 1.000000000000000000, 0.9659258262890683122, 1.000000000000000000, 0.9659258262890683122, 1.000000000000000000, 0.9659258262890683122, 1.000000000000000000, 0.9659258262890683122, 1.000000000000000000, 0.9659258262890683122, 1.000000000000000000, 0.9659258262890683122, 1.000000000000000000) ) ) 
 REPRESENTATION_ITEM ( '' )  SURFACE ( )  );
#53094=CARTESIAN_POINT ( 'NONE',  ( -0.2887139107611542133, -0.6046776061558809534, -0.2411417322834644161 ) ) ;
#53095=CARTESIAN_POINT ( 'NONE',  ( 1.056430446194226658, 0.1771653543307087630, 0.09757992244046791164 ) ) ;
#53096=CARTESIAN_POINT ( 'NONE',  ( 0.6975637601868572846, -4.135162568743707313E-16, -0.3954985857520056380 ) ) ;
#53098=CARTESIAN_POINT ( 'NONE',  ( 1.213910761154856299, 0.1771653543307087630, 0.09757992244046791164 ) ) ;
#53099=CARTESIAN_POINT ( 'NONE',  ( 1.102362204724410155, -0.1870078740157479769, 0.4822834645669291653 ) ) ;
#53102=CARTESIAN_POINT ( 'NONE',  ( -0.01968503937007793844, -0.5400638737290844871, 0.3530559997133364547 ) ) ;
#53104=CARTESIAN_POINT ( 'NONE',  ( -1.463254593175852492, -0.6692913385826773087, -0.1292274648535924053 ) ) ;
#53105=CARTESIAN_POINT ( 'NONE',  ( -0.2493438320209966919, 0.05413385826771626580, -0.4176697321401330321 ) ) ;
#53107=CARTESIAN_POINT ( 'NONE',  ( 1.174540682414699111, -0.3162353388693405765, 0.4822834645669290543 ) ) ;
#53108=CARTESIAN_POINT ( 'NONE',  ( 0.5183727034120741983, 0.2952755905511810774, -0.1292274648535930714 ) ) ;
#53109=CARTESIAN_POINT ( 'NONE',  ( 0.8595800524934390507, -0.2845877964562159024, 0.3641732283464567677 ) ) ;
#53110=CARTESIAN_POINT ( 'NONE',  ( 1.192633591291867967, 1.535433070866141447, -0.5030666621580099918 ) ) ;
#53111=CARTESIAN_POINT ( 'NONE',  ( 0.2559055118110243332, 0.07958543189024085140, 0.2665933059059887866 ) ) ;
#53114=CARTESIAN_POINT ( 'NONE',  ( 0.9251968503937015864, 0.1660481256975883668, -0.3530559997133364547 ) ) ;
#53116=CARTESIAN_POINT ( 'NONE',  ( 0.2362204724409456558, -0.1870078740157479769, 0.4822834645669291653 ) ) ;
#53117=CARTESIAN_POINT ( 'NONE',  ( 0.8989501312335965721, 0.2952755905511811885, 0.1292274648535926551 ) ) ;
#53119=CARTESIAN_POINT ( 'NONE',  ( 0.5446194225721792126, -0.08942795157528024563, -0.3641732283464568787 ) ) ;
#53120=CARTESIAN_POINT ( 'NONE',  ( 0.3740157480314966754, -0.5400638737290844871, 0.3530559997133364547 ) ) ;
#53122=CARTESIAN_POINT ( 'NONE',  ( -1.030183727034119867, -0.08942795157528024563, -0.3641732283464568787 ) ) ;
#53123=CARTESIAN_POINT ( 'NONE',  ( -0.8333333333333323711, -0.6692913385826773087, -0.1292274648535924053 ) ) ;
#53124=CARTESIAN_POINT ( 'NONE',  ( -1.666666666666665853, 0.05413385826771626580, -0.4176697321401330321 ) ) ;
#53125=CARTESIAN_POINT ( 'NONE',  ( 0.3674540682414705883, -0.6046776061558807314, 0.2411417322834647770 ) ) ;
#53126=CARTESIAN_POINT ( 'NONE',  ( 1.482939632545932307, -0.4281496062992124485, 0.4176697321401328655 ) ) ;
#53128=CARTESIAN_POINT ( 'NONE',  ( 0.5183727034120741983, 0.2952755905511810774, -0.1292274648535930714 ) ) ;
#53131=CARTESIAN_POINT ( 'NONE',  ( 1.541994750656168645, 0.2952755905511810774, -0.1292274648535930714 ) ) ;
#53132=CARTESIAN_POINT ( 'NONE',  ( -1.482939632545930975, -0.3690944881889765550, -0.3153832671262227771 ) ) ;
#53133=CARTESIAN_POINT ( 'NONE',  ( 1.174540682414699111, -0.2845877964562159024, 0.3641732283464567677 ) ) ;
#53134=CARTESIAN_POINT ( 'NONE',  ( -1.246719160104985846, -0.3690944881889765550, -0.3153832671262227771 ) ) ;
#53135=CARTESIAN_POINT ( 'NONE',  ( -0.6758530183727028406, 0.1771653543307087630, 0.09757992244046791164 ) ) ;
#53136=CARTESIAN_POINT ( 'NONE',  ( 1.561679790026247350, -0.4281496062992124485, 0.4176697321401328655 ) ) ;
#53137=CARTESIAN_POINT ( 'NONE',  ( 0.7152230971128614723, -0.2845877964562161244, -0.3641732283464567121 ) ) ;
#53138=CARTESIAN_POINT ( 'NONE',  ( 0.5052493438320218022, -0.6692913385826773087, -0.1292274648535924053 ) ) ;
#53139=CARTESIAN_POINT ( 'NONE',  ( 1.259842519685040019, -0.1870078740157479769, 0.4822834645669291653 ) ) ;
#53140=CARTESIAN_POINT ( 'NONE',  ( -0.006561679790025524116, -0.05778040916215560624, -0.4822834645669293319 ) ) ;
#53141=CARTESIAN_POINT ( 'NONE',  ( 0.3280839895013130669, -0.004921259842519576551, 0.3153832671262227771 ) ) ;
#53142=CARTESIAN_POINT ( 'NONE',  ( 1.358267716535433323, -0.5400638737290845981, -0.3530559997133363437 ) ) ;
#53143=CARTESIAN_POINT ( 'NONE',  ( -0.1771653543307080136, 0.1012011053420775880, -0.2882089793578256898 ) ) ;
#53144=CARTESIAN_POINT ( 'NONE',  ( -0.7611548556430438595, 0.2306618581243848609, 0.2411417322834645549 ) ) ;
#53146=CARTESIAN_POINT ( 'NONE',  ( 0.06632061457837788720, 2.409604939980833412E-17, -0.3464511005275205946 ) ) ;
#53147=CARTESIAN_POINT ( 'NONE',  ( -0.9973753280839886548, 0.2306618581243848609, 0.2411417322834645549 ) ) ;
#53149=CARTESIAN_POINT ( 'NONE',  ( -0.1640419947506555343, -0.3162353388693405765, 0.4822834645669290543 ) ) ;
#53154=CARTESIAN_POINT ( 'NONE',  ( -1.246719160104986512, -0.004921259842519576551, 0.3153832671262227771 ) ) ;
#53156=CARTESIAN_POINT ( 'NONE',  ( -1.496062992125983815, -0.1870078740157480879, -0.4822834645669291653 ) ) ;
#53157=B_SPLINE_CURVE_WITH_KNOTS ( 'NONE', 3,
 ( #36152, #69385, #11739, #5403 ),
 .UNSPECIFIED., .F., .F.,
 ( 4, 4 ),
 ( 2.453269466693398698E-18, 0.001494448006632143403 ),
 .UNSPECIFIED. ) ;
#53160=CARTESIAN_POINT ( 'NONE',  ( 0.4921259842519691285, -0.5400638737290845981, -0.3530559997133363437 ) ) ;
#53161=CARTESIAN_POINT ( 'NONE',  ( -0.3280839895013117347, -0.3690944881889763329, 0.3153832671262228327 ) ) ;
#53162=CARTESIAN_POINT ( 'NONE',  ( 0.9973753280839902091, 0.2306618581243847221, -0.2411417322834647770 ) ) ;
#53163=CARTESIAN_POINT ( 'NONE',  ( 0.5249343832021003964, 0.2306618581243847221, -0.2411417322834647770 ) ) ;
#53167=CARTESIAN_POINT ( 'NONE',  ( 1.187664041994751285, -0.05778040916215522460, 0.4822834645669289988 ) ) ;
#53168=CARTESIAN_POINT ( 'NONE',  ( -0.1312335958005241554, 0.2306618581243848609, 0.2411417322834645549 ) ) ;
#53169=CARTESIAN_POINT ( 'NONE',  ( 1.391076115485564868, -0.6046776061558807314, 0.2411417322834647770 ) ) ;
#53170=CARTESIAN_POINT ( 'NONE',  ( 1.043307086614173818, 0.1660481256975885056, 0.3530559997133364547 ) ) ;
#53172=CARTESIAN_POINT ( 'NONE',  ( 0.1246719160104994284, -0.6692913385826771977, 0.1292274648535927661 ) ) ;
#53173=CARTESIAN_POINT ( 'NONE',  ( 0.7874015748031503170, -0.1870078740157480879, -0.4822834645669291653 ) ) ;
#53174=CARTESIAN_POINT ( 'NONE',  ( 0.05905511811023709395, -0.5400638737290844871, 0.3530559997133364547 ) ) ;
#53175=CARTESIAN_POINT ( 'NONE',  ( 0.8333333333333340365, -0.5511811023622046335, 0.09757992244046803654 ) ) ;
#53176=CARTESIAN_POINT ( 'NONE',  ( -1.332020997375327642, -0.3162353388693409650, -0.4822834645669289433 ) ) ;
#53177=CARTESIAN_POINT ( 'NONE',  ( -1.568241469816272105, -0.05778040916215522460, 0.4822834645669289988 ) ) ;
#53178=CARTESIAN_POINT ( 'NONE',  ( 0.8661417322834652488, -0.1870078740157480879, -0.4822834645669291653 ) ) ;
#53184=CARTESIAN_POINT ( 'NONE',  ( 1.023622047244095334, -0.1870078740157479769, 0.4822834645669291653 ) ) ;
#53185=CARTESIAN_POINT ( 'NONE',  ( 1.154855643044620184, 0.1283753931104746893, -0.1820866141732285504 ) ) ;
#53192=CARTESIAN_POINT ( 'NONE',  ( 1.528871391076116026, -0.6692913385826773087, -0.1292274648535924053 ) ) ;
#53193=CARTESIAN_POINT ( 'NONE',  ( -1.587926509186350810, 0.05413385826771626580, -0.4176697321401330321 ) ) ;
#53194=CARTESIAN_POINT ( 'NONE',  ( -0.5249343832020990641, -0.6046776061558809534, -0.2411417322834644161 ) ) ;
#53195=CARTESIAN_POINT ( 'NONE',  ( 1.266404199475066328, -0.05778040916215522460, 0.4822834645669289988 ) ) ;
#53197=CARTESIAN_POINT ( 'NONE',  ( -1.397637795275589623, 0.1660481256975885056, 0.3530559997133364547 ) ) ;
#53200=CARTESIAN_POINT ( 'NONE',  ( 1.496062992125985147, -0.1870078740157479769, 0.3641732283464567677 ) ) ;
#53201=CARTESIAN_POINT ( 'NONE',  ( -0.3034644639079859818, -2.551093532135090261E-15, 0.3791475997938242304 ) ) ;
#53202=CARTESIAN_POINT ( 'NONE',  ( -0.8398950131233585692, 0.1283753931104748280, 0.1820866141732283561 ) ) ;
#53203=CARTESIAN_POINT ( 'NONE',  ( -1.384514435695537005, -0.6692913385826773087, -0.1292274648535924053 ) ) ;
#53204=CARTESIAN_POINT ( 'NONE',  ( 0.4330708661417329575, 0.2952755905511811885, 0.000000000000000000 ) ) ;
#53207=CARTESIAN_POINT ( 'NONE',  ( 1.456692913385827515, -0.6692913385826771977, 8.415575281601705876E-17 ) ) ;
#53210=CARTESIAN_POINT ( 'NONE',  ( -0.6233595800524928121, -0.08942795157527998196, 0.3641732283464567121 ) ) ;
#53211=CARTESIAN_POINT ( 'NONE',  ( 0.8661417322834653598, -0.1870078740157479769, 0.4822834645669291653 ) ) ;
#53212=CARTESIAN_POINT ( 'NONE',  ( -1.732283464566928277, -0.1870078740157479769, 0.4822834645669291653 ) ) ;
#53214=CARTESIAN_POINT ( 'NONE',  ( -0.7939632545931754048, -0.2845877964562159024, 0.3641732283464567677 ) ) ;
#53215=CARTESIAN_POINT ( 'NONE',  ( 1.692913385826772421, 0.2952755905511811885, 0.000000000000000000 ) ) ;
#53216=LINE ( 'NONE', #71765, #31683 ) ;
#53217=CARTESIAN_POINT ( 'NONE',  ( 0.5577427821522314977, -0.3162353388693409650, -0.4822834645669289433 ) ) ;
#53219=CARTESIAN_POINT ( 'NONE',  ( -0.7217847769028863381, -0.3690944881889763329, 0.3153832671262228327 ) ) ;
#53220=CARTESIAN_POINT ( 'NONE',  ( -0.5052493438320203589, -0.5511811023622046335, 0.09757992244046803654 ) ) ;
#53221=CARTESIAN_POINT ( 'NONE',  ( -0.2559055118110230564, 0.1660481256975883668, -0.3530559997133364547 ) ) ;
#53222=CARTESIAN_POINT ( 'NONE',  ( 1.633858267716535639, -0.5400638737290844871, 0.3530559997133364547 ) ) ;
#53224=CARTESIAN_POINT ( 'NONE',  ( 0.5774278215223103139, -0.6046776061558809534, -0.2411417322834644161 ) ) ;
#53227=CARTESIAN_POINT ( 'NONE',  ( -0.9711286089238838626, -0.6046776061558807314, 0.2411417322834647770 ) ) ;
#53228=CARTESIAN_POINT ( 'NONE',  ( -0.1968503937007867743, -0.5511811023622047445, 6.969142054262312111E-17 ) ) ;
#53229=CARTESIAN_POINT ( 'NONE',  ( -1.371391076115484609, -0.6692913385826771977, 0.1292274648535927661 ) ) ;
#53230=CARTESIAN_POINT ( 'NONE',  ( 0.4396325459317593221, 0.1771653543307087075, -0.09757992244046823083 ) ) ;
#53231=CARTESIAN_POINT ( 'NONE',  ( -0.5643044619422565855, -0.004921259842519870586, -0.3153832671262229437 ) ) ;
#53232=CARTESIAN_POINT ( 'NONE',  ( -1.148293963254592542, -0.6692913385826773087, -0.1292274648535924053 ) ) ;
#53233=CARTESIAN_POINT ( 'NONE',  ( -1.581364829396324945, -0.3162353388693405765, 0.4822834645669290543 ) ) ;
#53234=CARTESIAN_POINT ( 'NONE',  ( 1.607611548556431069, -0.6692913385826773087, -0.1292274648535924053 ) ) ;
#53236=CARTESIAN_POINT ( 'NONE',  ( 1.017060367454068803, -0.2845877964562159024, 0.3641732283464567677 ) ) ;
#53237=CARTESIAN_POINT ( 'NONE',  ( 0.3215223097112867578, -0.3162353388693409650, -0.4822834645669289433 ) ) ;
#53238=CARTESIAN_POINT ( 'NONE',  ( -1.358267716535432434, -0.5400638737290844871, 0.3530559997133364547 ) ) ;
#53239=CARTESIAN_POINT ( 'NONE',  ( 1.233595800524935227, -0.5023911411419708095, 0.1820866141732285504 ) ) ;
#53240=ORIENTED_EDGE ( 'NONE', *, *, #26035, .T. ) ;
#53243=CARTESIAN_POINT ( 'NONE',  ( -1.272965879265091305, -0.004921259842519870586, -0.3153832671262229437 ) ) ;
#53244=CARTESIAN_POINT ( 'NONE',  ( -0.6824146981627288167, 0.2306618581243848609, 0.2411417322834645549 ) ) ;
#53245=CARTESIAN_POINT ( 'NONE',  ( 0.2034120734908142214, 0.2952755905511810774, -0.1292274648535930714 ) ) ;
#53247=CARTESIAN_POINT ( 'NONE',  ( -1.660104986876639543, -0.08942795157528024563, -0.3641732283464568787 ) ) ;
#53249=CARTESIAN_POINT ( 'NONE',  ( -1.213910761154854745, 0.2952755905511810774, -0.1292274648535930714 ) ) ;
#53250=AXIS2_PLACEMENT_3D ( 'NONE', #53342, #45353, #64732 ) ;
#53252=CARTESIAN_POINT ( 'NONE',  ( 0.3937007874015754361, -0.1870078740157479769, 0.4822834645669291653 ) ) ;
#53253=CARTESIAN_POINT ( 'NONE',  ( 0.06561679790026316017, -0.4281496062992124485, 0.4176697321401328655 ) ) ;
#53254=CARTESIAN_POINT ( 'NONE',  ( 1.108923884514436242, -0.05778040916215522460, 0.4822834645669289988 ) ) ;
#53260=CARTESIAN_POINT ( 'NONE',  ( 0.3608923884514443348, 0.1771653543307087075, -0.09757992244046823083 ) ) ;
#53261=CARTESIAN_POINT ( 'NONE',  ( -0.5118110236220466680, -0.6692913385826771977, 8.415575281601705876E-17 ) ) ;
#53262=CARTESIAN_POINT ( 'NONE',  ( 1.332020997375328974, -0.05778040916215560624, -0.4822834645669293319 ) ) ;
#53264=CARTESIAN_POINT ( 'NONE',  ( -0.1377952755905504645, -0.4536011799217368745, -0.2665933059059886201 ) ) ;
#53266=CARTESIAN_POINT ( 'NONE',  ( -1.141732283464566011, 0.2952755905511811885, 0.000000000000000000 ) ) ;
#53267=CARTESIAN_POINT ( 'NONE',  ( 1.587926509186352142, 0.05413385826771666132, 0.4176697321401328100 ) ) ;
#53273=CARTESIAN_POINT ( 'NONE',  ( 1.423884514435696191, -0.05778040916215522460, 0.4822834645669289988 ) ) ;
#53274=CARTESIAN_POINT ( 'NONE',  ( -1.653543307086613234, -0.1870078740157480879, -0.4822834645669291653 ) ) ;
#53275=CARTESIAN_POINT ( 'NONE',  ( -1.312335958005248715, 0.1283753931104748280, 0.1820866141732283561 ) ) ;
#53276=CARTESIAN_POINT ( 'NONE',  ( -1.338582677165353729, -0.1870078740157479769, 0.4822834645669291653 ) ) ;
#53279=CARTESIAN_POINT ( 'NONE',  ( 1.062992125984252745, 0.2952755905511811885, 0.000000000000000000 ) ) ;
#53280=CARTESIAN_POINT ( 'NONE',  ( -1.122047244094487306, -0.5400638737290844871, 0.3530559997133364547 ) ) ;
#53281=CARTESIAN_POINT ( 'NONE',  ( -0.1377952755905504645, 0.1660481256975885056, 0.3530559997133364547 ) ) ;
#53282=CARTESIAN_POINT ( 'NONE',  ( -1.246719160104985846, -0.4281496062992127816, -0.4176697321401328100 ) ) ;
#53284=CARTESIAN_POINT ( 'NONE',  ( 0.4265091863517067039, -0.6692913385826773087, -0.1292274648535924053 ) ) ;
#53286=CARTESIAN_POINT ( 'NONE',  ( -1.259842519685038686, -0.1870078740157480601, -0.3641732283464567677 ) ) ;
#53291=CARTESIAN_POINT ( 'NONE',  ( -1.017060367454067249, -0.3162353388693409650, -0.4822834645669289433 ) ) ;
#53292=CARTESIAN_POINT ( 'NONE',  ( -1.095800524934382292, -0.3162353388693409650, -0.4822834645669289433 ) ) ;
#53294=CARTESIAN_POINT ( 'NONE',  ( -1.371391076115484831, 0.2952755905511810774, -0.1292274648535930714 ) ) ;
#53295=CARTESIAN_POINT ( 'NONE',  ( -1.568241469816272105, -0.05778040916215522460, 0.4822834645669289988 ) ) ;
#53296=CARTESIAN_POINT ( 'NONE',  ( -1.496062992125983815, -0.1870078740157479769, 0.4822834645669291653 ) ) ;
#53299=CARTESIAN_POINT ( 'NONE',  ( -0.05905511811023545637, 0.07958543189024085140, 0.2665933059059887866 ) ) ;
#53301=CARTESIAN_POINT ( 'NONE',  ( -0.9055118110236215490, 0.1771653543307087630, 0.000000000000000000 ) ) ;
#53302=CARTESIAN_POINT ( 'NONE',  ( -1.253280839895012377, -0.3162353388693409650, -0.4822834645669289433 ) ) ;
#53303=CARTESIAN_POINT ( 'NONE',  ( 0.8858267716535438430, -0.5400638737290845981, -0.3530559997133363437 ) ) ;
#53304=CARTESIAN_POINT ( 'NONE',  ( -0.8595800524934373854, -0.05778040916215522460, 0.4822834645669289988 ) ) ;
#53305=CARTESIAN_POINT ( 'NONE',  ( 0.4606732211678798428, 1.541615089183433485, -0.5309055118110237448 ) ) ;
#53307=CARTESIAN_POINT ( 'NONE',  ( -1.391076115485563314, -0.6046776061558809534, -0.2411417322834644161 ) ) ;
#53308=CARTESIAN_POINT ( 'NONE',  ( 0.8267716535433077274, 0.2952755905511811885, 0.000000000000000000 ) ) ;
#53309=CARTESIAN_POINT ( 'NONE',  ( -1.660104986876639543, -0.08942795157528024563, -0.3641732283464568787 ) ) ;
#53310=CARTESIAN_POINT ( 'NONE',  ( -1.653543307086613234, -0.1870078740157480879, -0.4822834645669291653 ) ) ;
#53312=FACE_OUTER_BOUND ( 'NONE', #7461, .T. ) ;
#53314=AXIS2_PLACEMENT_3D ( 'NONE', #35431, #40917, #34610 ) ;
#53316=CARTESIAN_POINT ( 'NONE',  ( -0.1312335958005241554, -0.6046776061558809534, -0.2411417322834644161 ) ) ;
#53317=CARTESIAN_POINT ( 'NONE',  ( 1.653543307086614789, -0.1870078740157479769, 0.4822834645669291653 ) ) ;
#53321=CARTESIAN_POINT ( 'NONE',  ( -1.601049868766403650, -0.6046776061558807314, 0.2411417322834647770 ) ) ;
#53322=CARTESIAN_POINT ( 'NONE',  ( -0.6561679790026240244, 0.1539470093639521697, -0.1968503937007875793 ) ) ;
#53324=CARTESIAN_POINT ( 'NONE',  ( -1.620734908136482577, -0.6692913385826773087, -0.1292274648535924053 ) ) ;
#53325=CARTESIAN_POINT ( 'NONE',  ( -0.5971128608923877978, 0.2952755905511811885, 0.1292274648535926551 ) ) ;
#53327=CARTESIAN_POINT ( 'NONE',  ( 0.4199475065616803948, -0.5023911411419708095, -0.1820866141732282451 ) ) ;
#53329=CARTESIAN_POINT ( 'NONE',  ( 0.4265091863517067594, 0.1771653543307087630, 0.09757992244046791164 ) ) ;
#53330=CARTESIAN_POINT ( 'NONE',  ( 1.108923884514436242, -0.08942795157527998196, 0.3641732283464567121 ) ) ;
#53331=CARTESIAN_POINT ( 'NONE',  ( 1.076115485564305141, -0.6046776061558807314, 0.2411417322834647770 ) ) ;
#53332=CARTESIAN_POINT ( 'NONE',  ( 0.2165354330708668673, -0.4536011799217367080, 0.2665933059059888421 ) ) ;
#53334=CARTESIAN_POINT ( 'NONE',  ( -1.312335958005248715, 0.2306618581243848609, 0.2411417322834645549 ) ) ;
#53335=CARTESIAN_POINT ( 'NONE',  ( -0.2296587926509179312, -0.2845877964562161244, -0.3641732283464567121 ) ) ;
#53336=( BOUNDED_SURFACE ( )  B_SPLINE_SURFACE ( 1, 2, ( 
 ( #24901, #70783, #13134, #24085, #44251, #49755, #12296, #75860, #38785, #30401, #11475, #37542, #69125, #37131, #5149, #37952, #63629, #5966, #31636, #57296, #44658, #1752, #6799, #53070, #34149, #71618, #14806, #20693, #65317, #72039, #58132, #15216, #13970, #501, #52656, #7222, #59810, #45504, #78362, #27409, #46765, #46344, #39627, #14395, #78781, #40465, #71201, #19855, #13544, #40052, #51815, #65738, #7655, #45920, #8071, #39200, #66143, #77520, #26584, #72457, #927, #64883, #59394, #2165, #21106, #33734, #8480, #53492, #27831, #26993, #79201, #21517, #47176, #32894, #72868, #64462, #32470, #26154, #58561, #52237, #33325, #77941, #58987, #20270, #1343, #9721, #28660, #9310, #35392, #34980, #35806, #67387, #60644, #15635, #61472, #60235, #23163, #16879, #55140, #79616, #2994, #67804, #10141, #41292, #2583, #42517, #66558, #80851, #21933, #8891, #66977, #34568, #48832, #42107, #16048, #3820, #74533, #28242, #61057, #53902, #3408, #54321, #29481, #68220, #47593, #80030, #40876, #73287, #29070, #22349, #80446, #48009, #54741, #73708, #41694, #22756, #74116, #48418, #16462, #39904, #66412, #72315, #33586, #40319, #58841, #773, #52086, #46620, #20128, #65592, #32747, #59250, #1608, #7925, #72723, #20961, #15489, #26435, #14662, #1199, #40728, #41146, #39481, #27264, #66835, #2442, #13822, #73140, #26849, #52924, #65168, #8749, #21783, #53349, #58414, #21376, #28100, #78638, #34420, #65998, #8337, #34003, #52507, #77796, #45775, #59664, #71474, #2020, #7504, #27684, #79059, #47031, #15070, #60088, #33173, #78216, #20548, #46200, #53756, #71895, #79466, #14246, #47445, #73564, #23023, #29747, #74803, #80709, #16318, #42371, #55411, #68478, #15908, #47859, #41557, #16730, #79885, #68070, #41963, #73973, #10414, #67245, #10816, #22203, #54591, #17150, #28923, #9576, #4080, #4493, #49099, #36071, #74387, #81530, #81118, #55001, #62151, #36476, #42783, #35246, #30160, #61743, #48690, #23434, #60910, #49517, #61322, #28513, #3677, #43186, #55822, #23850, #67657, #80301, #75210, #22615, #17554, #9168, #48275, #3262, #34840, #54171, #60500, #2849, #9993, #35659, #29340, #51149, #76843, #37308, #56245, #51562, #36893, #64219, #17963, #62569, #5321, #4908, #32225, #83163, #5720, #44826, #38539, #30579, #57056, #81941, #6134, #70523, #49926, #43599, #11650, #62982, #69301, #31391, #30979, #11233, #77265, #70108, #57469, #75625, #56646, #19177, #82748, #31809, #12460, #82347, #24666, #50334, #25482, #25070, #50744, #76031, #12879, #18376, #37711, #69710, #38122, #44016, #63796, #24253, #12054, #6553, #63384, #57882, #249, #76442, #18771, #25901, #19594, #44414, #68883, #21095, #59800, #33722, #14384, #21921, #7645, #34971, #28650, #66968, #78351, #59384, #53891, #79605, #40042, #58977, #54310, #39617, #9301, #20683, #65306, #8061, #33315, #60634, #2573, #8469, #47583, #41282, #1333, #2154, #26982, #27821, #65728, #73277, #80021, #46335, #78771, #22340, #2985, #52647, #71607, #1742, #34139, #72028, #15625, #13960, #8881, #27399, #60223, #53059, #46754, #72447, #53481, #14796, #79191, #40453, #66132, #21507, #47165, #72857, #15205, #40866, #66548, #34557, #28232, #4620, #36204, #30713, #16039, #41685, #82075, #80841, #67378, #61873, #74107, #43317, #29061, #4214, #68607, #30291, #29878, #55131, #81250, #23154, #56376, #17687, #54732, #5044, #16453, #68209, #80437, #55957, #37024, #10947, #73699, #36604, #69015, #48823, #81670, #55540, #74524, #23565, #42098, #9712, #35383, #49236, #61048, #16870, #48000, #42507, #10546, #74939, #23981, #17284, #3398, #22747, #48407, #67795, #42912, #10132, #62282, #35796, #11367, #61463, #49648, #75340, #62706, #3811, #29473, #57607, #44968, #385, #5451, #57187, #83298, #44553, #24388, #25620, #82889, #5854, #51283, #56780, #26041, #37439, #69839, #6689, #44147, #31112, #19315, #19738, #64352, #76986, #6270, #13432, #13020, #70243, #77403, #51701, #32359, #24795, #58021, #70664, #63934, #31946, #82479, #64769, #76575, #43729, #18903, #58447, #45392, #38257, #31531, #12189, #71089, #38674, #25209, #12598, #37846, #50463, #39088 ),
 ( #76167, #11786, #7108, #18504, #32778, #50059, #50875, #63524, #75754, #18096, #69433, #63113, #45809, #20159, #72346, #47060, #60120, #15101, #8367, #21812, #58874, #59282, #73168, #65201, #1232, #26881, #52541, #33210, #46653, #78250, #26470, #66867, #2050, #72752, #7537, #20581, #66441, #14694, #40757, #27714, #46232, #71929, #14278, #8778, #40350, #66029, #39940, #2471, #65626, #52955, #1639, #53381, #7957, #79088, #39512, #33619, #21406, #27297, #34451, #28130, #78670, #20991, #53785, #47476, #34033, #59694, #79497, #15519, #41177, #9197, #34870, #807, #52121, #77829, #71507, #13854, #25005, #50677, #18710, #75145, #69644, #68818, #31324, #37240, #11581, #43948, #41585, #47888, #11988, #4426, #30914, #5250, #36823, #17490, #17896, #76376, #37642, #12396, #22233, #79916, #49857, #43121, #56581, #70042, #36411, #23780, #81462, #62917, #11164, #62498, #56988, #28544, #82282, #49451, #73596, #4836, #24600, #24188, #30511, #15938, #63319, #62085, #56173, #30092, #43533, #55756, #67275, #9608, #44351, #75966, #50268, #81876, #75557, #82685, #60531, #54200, #69232, #18306, #5657, #2881, #19957, #6488, #52756, #33420, #70456, #6069, #57814, #31742, #1437, #52336, #58235, #14073, #7755, #57405, #26258, #83096, #51919, #32158, #46024, #20789, #44760, #45184, #46445, #59082, #19111, #78464, #64154, #602, #12814, #71718, #27093, #58663, #63729, #26681, #72138, #70887, #39726, #77624, #38886, #45607, #181, #25417, #51082, #71301, #76779, #13236, #38053, #64565, #6902, #32573, #78042, #13649, #38471, #25834, #51493, #77196, #39302, #19527, #64989, #7324, #32993, #1028, #20372, #65421, #80131, #2682, #21614, #47692, #35076, #73809, #78883, #47274, #73386, #34671, #14494, #15738, #72964, #79296, #41392, #46859, #16146, #27511, #59911, #22451, #34249, #21204, #9406, #9819, #54420, #67074, #79715, #3506, #3094, #60334, #67484, #41793, #48111, #14900, #35490, #60742, #54003, #22031, #72553, #54841, #66660, #33830, #8999, #48519, #61154, #28342, #15315, #2266, #29175, #28758, #40978, #80546, #27929, #40560, #22858, #59496, #40147, #65832, #8165, #66241, #53587, #1850, #53168, #8578, #61578, #56895, #42209, #10657, #3921, #36312, #24090, #36719, #49351, #29582, #75866, #48936, #61988, #16980, #56074, #68320, #35912, #55245, #63223, #5155, #37136, #75048, #80952, #43844, #74219, #67904, #62395, #23267, #69130, #74637, #81780, #42623, #5563, #62821, #50170, #30819, #49760, #11895, #4325, #17394, #31227, #29991, #55654, #81364, #23677, #43025, #4733, #68719, #16564, #82588, #75460, #56484, #11061, #30406, #82187, #17798, #24504, #43433, #11481, #18209, #69547, #37548, #24908, #10241, #76683, #26591, #32061, #19434, #51398, #77526, #57721, #45510, #5973, #19016, #19862, #50985, #58568, #71207, #84, #25737, #52243, #71624, #83000, #44664, #933, #77102, #45085, #38375, #39206, #70789, #31643, #13550, #45926, #64889, #13976, #39633, #7661, #64050, #77947, #13140, #20276, #26160, #507, #32900, #57302, #37958, #65324, #70360, #7228, #33332, #38791, #6390, #6805, #58993, #1349, #50576, #12302, #69947, #64468, #32476, #76283, #18614, #25321, #12715, #58138, #51822, #44257, #63635, #22357, #78368, #53909, #53076, #3001, #8487, #79208, #27838, #79623, #34156, #21940, #65744, #78788, #47600, #27415, #34987, #73294, #59817, #2172, #28667, #48016, #59400, #21113, #60651, #53500, #21524, #14813, #15643, #47183, #8077, #41299, #73716, #66985, #16055, #41701, #67394, #40472, #54328, #72875, #80037, #2590, #60243, #9317, #33740, #14401, #9728, #46773, #35399, #61064, #15223, #66150, #66565, #26999, #52662, #20700, #72046, #46350, #40883, #8899, #40057, #1758, #72464, #34575, #28249, #36621, #36220, #4230, #82089, #54748, #30307, #23171, #74124, #48840, #62299, #49253, #61889, #42115, #5058, #61480, #74541, #29489, #68623, #80859, #48425, #16470, #75768, #17703, #49665, #29894, #67812, #56390, #3415, #80454, #74955, #10149, #81686, #35815, #10963, #55148, #18110, #75355, #62721, #43331, #4636, #24403, #3829, #55557, #43743, #16887, #42526, #68228, #10562, #81266, #17301, #23581 ) ),
 .UNSPECIFIED., .F., .F., .F. ) 
 B_SPLINE_SURFACE_WITH_KNOTS ( ( 2, 2 ),
 ( 3, 2, 2, 2, 2, 2, 2, 2, 2, 2, 2, 2, 2, 2, 2, 2, 2, 2, 2, 2, 2, 2, 2, 2, 2, 2, 2, 2, 2, 2, 2, 2, 2, 2, 2, 2, 2, 2, 2, 2, 2, 2, 2, 2, 2, 2, 2, 2, 2, 2, 2, 2, 2, 2, 2, 2, 2, 2, 2, 2, 2, 2, 2, 2, 2, 2, 2, 2, 2, 2, 2, 2, 2, 2, 2, 2, 2, 2, 2, 2, 2, 2, 2, 2, 2, 2, 2, 2, 2, 2, 2, 2, 2, 2, 2, 2, 2, 2, 2, 2, 2, 2, 2, 2, 2, 2, 2, 2, 2, 2, 2, 2, 2, 2, 2, 2, 2, 2, 2, 2, 2, 2, 2, 2, 2, 2, 2, 2, 2, 2, 2, 2, 2, 2, 2, 2, 2, 2, 2, 2, 2, 2, 2, 2, 2, 2, 2, 2, 2, 2, 2, 2, 2, 2, 2, 2, 2, 2, 2, 2, 2, 2, 2, 2, 2, 2, 2, 2, 2, 2, 2, 2, 2, 2, 2, 2, 2, 2, 2, 2, 2, 2, 2, 2, 2, 2, 2, 2, 2, 2, 2, 2, 2, 2, 2, 2, 2, 2, 2, 2, 2, 2, 2, 2, 2, 2, 2, 2, 2, 2, 2, 2, 2, 2, 2, 2, 2, 2, 2, 2, 2, 2, 2, 2, 2, 2, 2, 2, 2, 2, 2, 2, 2, 2, 2, 2, 2, 2, 2, 2, 2, 2, 2, 2, 2, 2, 2, 2, 2, 2, 2, 2, 2, 2, 2, 3 ),
 ( 0.000000000000000000, 1.000000000000000000 ),
 ( 0.000000000000000000, 0.003787878787878787984, 0.007575757575757575968, 0.01136363636363636395, 0.01515151515151515194, 0.01893939393939393992, 0.02272727272727272790, 0.02651515151515151589, 0.03030303030303030387, 0.03409090909090908839, 0.03787878787878787984, 0.04166666666666666435, 0.04545454545454545581, 0.04924242424242424032, 0.05303030303030303177, 0.05681818181818181629, 0.06060606060606060774, 0.06439393939393939226, 0.06818181818181817677, 0.07196969696969697516, 0.07575757575757575968, 0.07954545454545454419, 0.08333333333333332871, 0.08712121212121212710, 0.09090909090909091161, 0.09469696969696969613, 0.09848484848484848064, 0.1022727272727272790, 0.1060606060606060635, 0.1098484848484848481, 0.1136363636363636326, 0.1174242424242424310, 0.1212121212121212155, 0.1250000000000000000, 0.1287878787878787845, 0.1325757575757575690, 0.1363636363636363535, 0.1401515151515151381, 0.1439393939393939503, 0.1477272727272727348, 0.1515151515151515194, 0.1553030303030303039, 0.1590909090909090884, 0.1628787878787878729, 0.1666666666666666574, 0.1704545454545454419, 0.1742424242424242542, 0.1780303030303030387, 0.1818181818181818232, 0.1856060606060606077, 0.1893939393939393923, 0.1931818181818181768, 0.1969696969696969613, 0.2007575757575757458, 0.2045454545454545581, 0.2083333333333333426, 0.2121212121212121271, 0.2159090909090909116, 0.2196969696969696961, 0.2234848484848484806, 0.2272727272727272652, 0.2310606060606060497, 0.2348484848484848619, 0.2386363636363636465, 0.2424242424242424310, 0.2462121212121212155, 0.2500000000000000000, 0.2537878787878787845, 0.2575757575757575690, 0.2613636363636363535, 0.2651515151515151381, 0.2689393939393939226, 0.2727272727272727071, 0.2765151515151514916, 0.2803030303030302761, 0.2840909090909091161, 0.2878787878787879007, 0.2916666666666666852, 0.2954545454545454697, 0.2992424242424242542, 0.3030303030303030387, 0.3068181818181818232, 0.3106060606060606077, 0.3143939393939393923, 0.3181818181818181768, 0.3219696969696969613, 0.3257575757575757458, 0.3295454545454545303, 0.3333333333333333148, 0.3371212121212120993, 0.3409090909090908839, 0.3446969696969697239, 0.3484848484848485084, 0.3522727272727272929, 0.3560606060606060774, 0.3598484848484848619, 0.3636363636363636465, 0.3674242424242424310, 0.3712121212121212155, 0.3750000000000000000, 0.3787878787878787845, 0.3825757575757575690, 0.3863636363636363535, 0.3901515151515151381, 0.3939393939393939226, 0.3977272727272727071, 0.4015151515151514916, 0.4053030303030302761, 0.4090909090909091161, 0.4128787878787879007, 0.4166666666666666852, 0.4204545454545454697, 0.4242424242424242542, 0.4280303030303030387, 0.4318181818181818232, 0.4356060606060606077, 0.4393939393939393923, 0.4431818181818181768, 0.4469696969696969613, 0.4507575757575757458, 0.4545454545454545303, 0.4583333333333333148, 0.4621212121212120993, 0.4659090909090908839, 0.4696969696969697239, 0.4734848484848485084, 0.4772727272727272929, 0.4810606060606060774, 0.4848484848484848619, 0.4886363636363636465, 0.4924242424242424310, 0.4962121212121212155, 0.5000000000000000000, 0.5037878787878787845, 0.5075757575757575690, 0.5113636363636363535, 0.5151515151515151381, 0.5189393939393939226, 0.5227272727272727071, 0.5265151515151514916, 0.5303030303030302761, 0.5340909090909090606, 0.5378787878787878451, 0.5416666666666666297, 0.5454545454545454142, 0.5492424242424241987, 0.5530303030303029832, 0.5568181818181817677, 0.5606060606060605522, 0.5643939393939394478, 0.5681818181818182323, 0.5719696969696970168, 0.5757575757575758013, 0.5795454545454545858, 0.5833333333333333703, 0.5871212121212121549, 0.5909090909090909394, 0.5946969696969697239, 0.5984848484848485084, 0.6022727272727272929, 0.6060606060606060774, 0.6098484848484848619, 0.6136363636363636465, 0.6174242424242424310, 0.6212121212121212155, 0.6250000000000000000, 0.6287878787878787845, 0.6325757575757575690, 0.6363636363636363535, 0.6401515151515151381, 0.6439393939393939226, 0.6477272727272727071, 0.6515151515151514916, 0.6553030303030302761, 0.6590909090909090606, 0.6628787878787878451, 0.6666666666666666297, 0.6704545454545454142, 0.6742424242424241987, 0.6780303030303029832, 0.6818181818181817677, 0.6856060606060605522, 0.6893939393939394478, 0.6931818181818182323, 0.6969696969696970168, 0.7007575757575758013, 0.7045454545454545858, 0.7083333333333333703, 0.7121212121212121549, 0.7159090909090909394, 0.7196969696969697239, 0.7234848484848485084, 0.7272727272727272929, 0.7310606060606060774, 0.7348484848484848619, 0.7386363636363636465, 0.7424242424242424310, 0.7462121212121212155, 0.7500000000000000000, 0.7537878787878787845, 0.7575757575757575690, 0.7613636363636363535, 0.7651515151515151381, 0.7689393939393939226, 0.7727272727272727071, 0.7765151515151514916, 0.7803030303030302761, 0.7840909090909090606, 0.7878787878787878451, 0.7916666666666666297, 0.7954545454545454142, 0.7992424242424241987, 0.8030303030303029832, 0.8068181818181817677, 0.8106060606060605522, 0.8143939393939394478, 0.8181818181818182323, 0.8219696969696970168, 0.8257575757575758013, 0.8295454545454545858, 0.8333333333333333703, 0.8371212121212121549, 0.8409090909090909394, 0.8446969696969697239, 0.8484848484848485084, 0.8522727272727272929, 0.8560606060606060774, 0.8598484848484848619, 0.8636363636363636465, 0.8674242424242424310, 0.8712121212121212155, 0.8750000000000000000, 0.8787878787878787845, 0.8825757575757575690, 0.8863636363636363535, 0.8901515151515151381, 0.8939393939393939226, 0.8977272727272727071, 0.9015151515151514916, 0.9053030303030302761, 0.9090909090909090606, 0.9128787878787878451, 0.9166666666666666297, 0.9204545454545454142, 0.9242424242424241987, 0.9280303030303029832, 0.9318181818181817677, 0.9356060606060605522, 0.9393939393939394478, 0.9431818181818182323, 0.9469696969696970168, 0.9507575757575758013, 0.9545454545454545858, 0.9583333333333333703, 0.9621212121212121549, 0.9659090909090909394 ),
 .UNSPECIFIED. ) 
 GEOMETRIC_REPRESENTATION_ITEM ( )  RATIONAL_B_SPLINE_SURFACE ( (
 ( 1.000000000000000000, 0.9659258262890683122, 1.000000000000000000, 0.9659258262890683122, 1.000000000000000000, 0.9659258262890683122, 1.000000000000000000, 0.9659258262890683122, 1.000000000000000000, 0.9659258262890683122, 1.000000000000000000, 0.9659258262890683122, 1.000000000000000000, 0.9659258262890683122, 1.000000000000000000, 0.9659258262890683122, 1.000000000000000000, 0.9659258262890683122, 1.000000000000000000, 0.9659258262890683122, 1.000000000000000000, 0.9659258262890683122, 1.000000000000000000, 0.9659258262890683122, 1.000000000000000000, 0.9659258262890683122, 1.000000000000000000, 0.9659258262890683122, 1.000000000000000000, 0.9659258262890683122, 1.000000000000000000, 0.9659258262890683122, 1.000000000000000000, 0.9659258262890683122, 1.000000000000000000, 0.9659258262890683122, 1.000000000000000000, 0.9659258262890683122, 1.000000000000000000, 0.9659258262890683122, 1.000000000000000000, 0.9659258262890683122, 1.000000000000000000, 0.9659258262890683122, 1.000000000000000000, 0.9659258262890683122, 1.000000000000000000, 0.9659258262890683122, 1.000000000000000000, 0.9659258262890683122, 1.000000000000000000, 0.9659258262890683122, 1.000000000000000000, 0.9659258262890683122, 1.000000000000000000, 0.9659258262890683122, 1.000000000000000000, 0.9659258262890683122, 1.000000000000000000, 0.9659258262890683122, 1.000000000000000000, 0.9659258262890683122, 1.000000000000000000, 0.9659258262890683122, 1.000000000000000000, 0.9659258262890683122, 1.000000000000000000, 0.9659258262890683122, 1.000000000000000000, 0.9659258262890683122, 1.000000000000000000, 0.9659258262890683122, 1.000000000000000000, 0.9659258262890683122, 1.000000000000000000, 0.9659258262890683122, 1.000000000000000000, 0.9659258262890683122, 1.000000000000000000, 0.9659258262890683122, 1.000000000000000000, 0.9659258262890683122, 1.000000000000000000, 0.9659258262890683122, 1.000000000000000000, 0.9659258262890683122, 1.000000000000000000, 0.9659258262890683122, 1.000000000000000000, 0.9659258262890683122, 1.000000000000000000, 0.9659258262890683122, 1.000000000000000000, 0.9659258262890683122, 1.000000000000000000, 0.9659258262890683122, 1.000000000000000000, 0.9659258262890683122, 1.000000000000000000, 0.9659258262890683122, 1.000000000000000000, 0.9659258262890683122, 1.000000000000000000, 0.9659258262890683122, 1.000000000000000000, 0.9659258262890683122, 1.000000000000000000, 0.9659258262890683122, 1.000000000000000000, 0.9659258262890683122, 1.000000000000000000, 0.9659258262890683122, 1.000000000000000000, 0.9659258262890683122, 1.000000000000000000, 0.9659258262890683122, 1.000000000000000000, 0.9659258262890683122, 1.000000000000000000, 0.9659258262890683122, 1.000000000000000000, 0.9659258262890683122, 1.000000000000000000, 0.9659258262890683122, 1.000000000000000000, 0.9659258262890683122, 1.000000000000000000, 0.9659258262890683122, 1.000000000000000000, 0.9659258262890683122, 1.000000000000000000, 0.9659258262890683122, 1.000000000000000000, 0.9659258262890683122, 1.000000000000000000, 0.9659258262890683122, 1.000000000000000000, 0.9659258262890683122, 1.000000000000000000, 0.9659258262890683122, 1.000000000000000000, 0.9659258262890683122, 1.000000000000000000, 0.9659258262890683122, 1.000000000000000000, 0.9659258262890683122, 1.000000000000000000, 0.9659258262890683122, 1.000000000000000000, 0.9659258262890683122, 1.000000000000000000, 0.9659258262890683122, 1.000000000000000000, 0.9659258262890683122, 1.000000000000000000, 0.9659258262890683122, 1.000000000000000000, 0.9659258262890683122, 1.000000000000000000, 0.9659258262890683122, 1.000000000000000000, 0.9659258262890683122, 1.000000000000000000, 0.9659258262890683122, 1.000000000000000000, 0.9659258262890683122, 1.000000000000000000, 0.9659258262890683122, 1.000000000000000000, 0.9659258262890683122, 1.000000000000000000, 0.9659258262890683122, 1.000000000000000000, 0.9659258262890683122, 1.000000000000000000, 0.9659258262890683122, 1.000000000000000000, 0.9659258262890683122, 1.000000000000000000, 0.9659258262890683122, 1.000000000000000000, 0.9659258262890683122, 1.000000000000000000, 0.9659258262890683122, 1.000000000000000000, 0.9659258262890683122, 1.000000000000000000, 0.9659258262890683122, 1.000000000000000000, 0.9659258262890683122, 1.000000000000000000, 0.9659258262890683122, 1.000000000000000000, 0.9659258262890683122, 1.000000000000000000, 0.9659258262890683122, 1.000000000000000000, 0.9659258262890683122, 1.000000000000000000, 0.9659258262890683122, 1.000000000000000000, 0.9659258262890683122, 1.000000000000000000, 0.9659258262890683122, 1.000000000000000000, 0.9659258262890683122, 1.000000000000000000, 0.9659258262890683122, 1.000000000000000000, 0.9659258262890683122, 1.000000000000000000, 0.9659258262890683122, 1.000000000000000000, 0.9659258262890683122, 1.000000000000000000, 0.9659258262890683122, 1.000000000000000000, 0.9659258262890683122, 1.000000000000000000, 0.9659258262890683122, 1.000000000000000000, 0.9659258262890683122, 1.000000000000000000, 0.9659258262890683122, 1.000000000000000000, 0.9659258262890683122, 1.000000000000000000, 0.9659258262890683122, 1.000000000000000000, 0.9659258262890683122, 1.000000000000000000, 0.9659258262890683122, 1.000000000000000000, 0.9659258262890683122, 1.000000000000000000, 0.9659258262890683122, 1.000000000000000000, 0.9659258262890683122, 1.000000000000000000, 0.9659258262890683122, 1.000000000000000000, 0.9659258262890683122, 1.000000000000000000, 0.9659258262890683122, 1.000000000000000000, 0.9659258262890683122, 1.000000000000000000, 0.9659258262890683122, 1.000000000000000000, 0.9659258262890683122, 1.000000000000000000, 0.9659258262890683122, 1.000000000000000000, 0.9659258262890683122, 1.000000000000000000, 0.9659258262890683122, 1.000000000000000000, 0.9659258262890683122, 1.000000000000000000, 0.9659258262890683122, 1.000000000000000000, 0.9659258262890683122, 1.000000000000000000, 0.9659258262890683122, 1.000000000000000000, 0.9659258262890683122, 1.000000000000000000, 0.9659258262890683122, 1.000000000000000000, 0.9659258262890683122, 1.000000000000000000, 0.9659258262890683122, 1.000000000000000000, 0.9659258262890683122, 1.000000000000000000, 0.9659258262890683122, 1.000000000000000000, 0.9659258262890683122, 1.000000000000000000, 0.9659258262890683122, 1.000000000000000000, 0.9659258262890683122, 1.000000000000000000, 0.9659258262890683122, 1.000000000000000000, 0.9659258262890683122, 1.000000000000000000, 0.9659258262890683122, 1.000000000000000000, 0.9659258262890683122, 1.000000000000000000, 0.9659258262890683122, 1.000000000000000000, 0.9659258262890683122, 1.000000000000000000, 0.9659258262890683122, 1.000000000000000000, 0.9659258262890683122, 1.000000000000000000, 0.9659258262890683122, 1.000000000000000000, 0.9659258262890683122, 1.000000000000000000, 0.9659258262890683122, 1.000000000000000000, 0.9659258262890683122, 1.000000000000000000, 0.9659258262890683122, 1.000000000000000000, 0.9659258262890683122, 1.000000000000000000, 0.9659258262890683122, 1.000000000000000000, 0.9659258262890683122, 1.000000000000000000, 0.9659258262890683122, 1.000000000000000000, 0.9659258262890683122, 1.000000000000000000, 0.9659258262890683122, 1.000000000000000000, 0.9659258262890683122, 1.000000000000000000, 0.9659258262890683122, 1.000000000000000000, 0.9659258262890683122, 1.000000000000000000, 0.9659258262890683122, 1.000000000000000000, 0.9659258262890683122, 1.000000000000000000, 0.9659258262890683122, 1.000000000000000000, 0.9659258262890683122, 1.000000000000000000, 0.9659258262890683122, 1.000000000000000000, 0.9659258262890683122, 1.000000000000000000, 0.9659258262890683122, 1.000000000000000000, 0.9659258262890683122, 1.000000000000000000, 0.9659258262890683122, 1.000000000000000000, 0.9659258262890683122, 1.000000000000000000, 0.9659258262890683122, 1.000000000000000000, 0.9659258262890683122, 1.000000000000000000, 0.9659258262890683122, 1.000000000000000000, 0.9659258262890683122, 1.000000000000000000, 0.9659258262890683122, 1.000000000000000000, 0.9659258262890683122, 1.000000000000000000, 0.9659258262890683122, 1.000000000000000000, 0.9659258262890683122, 1.000000000000000000, 0.9659258262890683122, 1.000000000000000000, 0.9659258262890683122, 1.000000000000000000, 0.9659258262890683122, 1.000000000000000000, 0.9659258262890683122, 1.000000000000000000, 0.9659258262890683122, 1.000000000000000000, 0.9659258262890683122, 1.000000000000000000, 0.9659258262890683122, 1.000000000000000000, 0.9659258262890683122, 1.000000000000000000, 0.9659258262890683122, 1.000000000000000000, 0.9659258262890683122, 1.000000000000000000, 0.9659258262890683122, 1.000000000000000000, 0.9659258262890683122, 1.000000000000000000, 0.9659258262890683122, 1.000000000000000000, 0.9659258262890683122, 1.000000000000000000, 0.9659258262890683122, 1.000000000000000000, 0.9659258262890683122, 1.000000000000000000, 0.9659258262890683122, 1.000000000000000000, 0.9659258262890683122, 1.000000000000000000, 0.9659258262890683122, 1.000000000000000000, 0.9659258262890683122, 1.000000000000000000, 0.9659258262890683122, 1.000000000000000000, 0.9659258262890683122, 1.000000000000000000, 0.9659258262890683122, 1.000000000000000000, 0.9659258262890683122, 1.000000000000000000, 0.9659258262890683122, 1.000000000000000000, 0.9659258262890683122, 1.000000000000000000, 0.9659258262890683122, 1.000000000000000000, 0.9659258262890683122, 1.000000000000000000, 0.9659258262890683122, 1.000000000000000000, 0.9659258262890683122, 1.000000000000000000, 0.9659258262890683122, 1.000000000000000000, 0.9659258262890683122, 1.000000000000000000, 0.9659258262890683122, 1.000000000000000000, 0.9659258262890683122, 1.000000000000000000, 0.9659258262890683122, 1.000000000000000000, 0.9659258262890683122, 1.000000000000000000, 0.9659258262890683122, 1.000000000000000000, 0.9659258262890683122, 1.000000000000000000, 0.9659258262890683122, 1.000000000000000000, 0.9659258262890683122, 1.000000000000000000, 0.9659258262890683122, 1.000000000000000000, 0.9659258262890683122, 1.000000000000000000, 0.9659258262890683122, 1.000000000000000000, 0.9659258262890683122, 1.000000000000000000, 0.9659258262890683122, 1.000000000000000000, 0.9659258262890683122, 1.000000000000000000, 0.9659258262890683122, 1.000000000000000000, 0.9659258262890683122, 1.000000000000000000, 0.9659258262890683122, 1.000000000000000000, 0.9659258262890683122, 1.000000000000000000, 0.9659258262890683122, 1.000000000000000000, 0.9659258262890683122, 1.000000000000000000, 0.9659258262890683122, 1.000000000000000000, 0.9659258262890683122, 1.000000000000000000, 0.9659258262890683122, 1.000000000000000000, 0.9659258262890683122, 1.000000000000000000, 0.9659258262890683122, 1.000000000000000000, 0.9659258262890683122, 1.000000000000000000, 0.9659258262890683122, 1.000000000000000000, 0.9659258262890683122, 1.000000000000000000, 0.9659258262890683122, 1.000000000000000000, 0.9659258262890683122, 1.000000000000000000, 0.9659258262890683122, 1.000000000000000000, 0.9659258262890683122, 1.000000000000000000, 0.9659258262890683122, 1.000000000000000000, 0.9659258262890683122, 1.000000000000000000, 0.9659258262890683122, 1.000000000000000000, 0.9659258262890683122, 1.000000000000000000, 0.9659258262890683122, 1.000000000000000000, 0.9659258262890683122, 1.000000000000000000, 0.9659258262890683122, 1.000000000000000000, 0.9659258262890683122, 1.000000000000000000, 0.9659258262890683122, 1.000000000000000000, 0.9659258262890683122, 1.000000000000000000),
 ( 1.000000000000000000, 0.9659258262890683122, 1.000000000000000000, 0.9659258262890683122, 1.000000000000000000, 0.9659258262890683122, 1.000000000000000000, 0.9659258262890683122, 1.000000000000000000, 0.9659258262890683122, 1.000000000000000000, 0.9659258262890683122, 1.000000000000000000, 0.9659258262890683122, 1.000000000000000000, 0.9659258262890683122, 1.000000000000000000, 0.9659258262890683122, 1.000000000000000000, 0.9659258262890683122, 1.000000000000000000, 0.9659258262890683122, 1.000000000000000000, 0.9659258262890683122, 1.000000000000000000, 0.9659258262890683122, 1.000000000000000000, 0.9659258262890683122, 1.000000000000000000, 0.9659258262890683122, 1.000000000000000000, 0.9659258262890683122, 1.000000000000000000, 0.9659258262890683122, 1.000000000000000000, 0.9659258262890683122, 1.000000000000000000, 0.9659258262890683122, 1.000000000000000000, 0.9659258262890683122, 1.000000000000000000, 0.9659258262890683122, 1.000000000000000000, 0.9659258262890683122, 1.000000000000000000, 0.9659258262890683122, 1.000000000000000000, 0.9659258262890683122, 1.000000000000000000, 0.9659258262890683122, 1.000000000000000000, 0.9659258262890683122, 1.000000000000000000, 0.9659258262890683122, 1.000000000000000000, 0.9659258262890683122, 1.000000000000000000, 0.9659258262890683122, 1.000000000000000000, 0.9659258262890683122, 1.000000000000000000, 0.9659258262890683122, 1.000000000000000000, 0.9659258262890683122, 1.000000000000000000, 0.9659258262890683122, 1.000000000000000000, 0.9659258262890683122, 1.000000000000000000, 0.9659258262890683122, 1.000000000000000000, 0.9659258262890683122, 1.000000000000000000, 0.9659258262890683122, 1.000000000000000000, 0.9659258262890683122, 1.000000000000000000, 0.9659258262890683122, 1.000000000000000000, 0.9659258262890683122, 1.000000000000000000, 0.9659258262890683122, 1.000000000000000000, 0.9659258262890683122, 1.000000000000000000, 0.9659258262890683122, 1.000000000000000000, 0.9659258262890683122, 1.000000000000000000, 0.9659258262890683122, 1.000000000000000000, 0.9659258262890683122, 1.000000000000000000, 0.9659258262890683122, 1.000000000000000000, 0.9659258262890683122, 1.000000000000000000, 0.9659258262890683122, 1.000000000000000000, 0.9659258262890683122, 1.000000000000000000, 0.9659258262890683122, 1.000000000000000000, 0.9659258262890683122, 1.000000000000000000, 0.9659258262890683122, 1.000000000000000000, 0.9659258262890683122, 1.000000000000000000, 0.9659258262890683122, 1.000000000000000000, 0.9659258262890683122, 1.000000000000000000, 0.9659258262890683122, 1.000000000000000000, 0.9659258262890683122, 1.000000000000000000, 0.9659258262890683122, 1.000000000000000000, 0.9659258262890683122, 1.000000000000000000, 0.9659258262890683122, 1.000000000000000000, 0.9659258262890683122, 1.000000000000000000, 0.9659258262890683122, 1.000000000000000000, 0.9659258262890683122, 1.000000000000000000, 0.9659258262890683122, 1.000000000000000000, 0.9659258262890683122, 1.000000000000000000, 0.9659258262890683122, 1.000000000000000000, 0.9659258262890683122, 1.000000000000000000, 0.9659258262890683122, 1.000000000000000000, 0.9659258262890683122, 1.000000000000000000, 0.9659258262890683122, 1.000000000000000000, 0.9659258262890683122, 1.000000000000000000, 0.9659258262890683122, 1.000000000000000000, 0.9659258262890683122, 1.000000000000000000, 0.9659258262890683122, 1.000000000000000000, 0.9659258262890683122, 1.000000000000000000, 0.9659258262890683122, 1.000000000000000000, 0.9659258262890683122, 1.000000000000000000, 0.9659258262890683122, 1.000000000000000000, 0.9659258262890683122, 1.000000000000000000, 0.9659258262890683122, 1.000000000000000000, 0.9659258262890683122, 1.000000000000000000, 0.9659258262890683122, 1.000000000000000000, 0.9659258262890683122, 1.000000000000000000, 0.9659258262890683122, 1.000000000000000000, 0.9659258262890683122, 1.000000000000000000, 0.9659258262890683122, 1.000000000000000000, 0.9659258262890683122, 1.000000000000000000, 0.9659258262890683122, 1.000000000000000000, 0.9659258262890683122, 1.000000000000000000, 0.9659258262890683122, 1.000000000000000000, 0.9659258262890683122, 1.000000000000000000, 0.9659258262890683122, 1.000000000000000000, 0.9659258262890683122, 1.000000000000000000, 0.9659258262890683122, 1.000000000000000000, 0.9659258262890683122, 1.000000000000000000, 0.9659258262890683122, 1.000000000000000000, 0.9659258262890683122, 1.000000000000000000, 0.9659258262890683122, 1.000000000000000000, 0.9659258262890683122, 1.000000000000000000, 0.9659258262890683122, 1.000000000000000000, 0.9659258262890683122, 1.000000000000000000, 0.9659258262890683122, 1.000000000000000000, 0.9659258262890683122, 1.000000000000000000, 0.9659258262890683122, 1.000000000000000000, 0.9659258262890683122, 1.000000000000000000, 0.9659258262890683122, 1.000000000000000000, 0.9659258262890683122, 1.000000000000000000, 0.9659258262890683122, 1.000000000000000000, 0.9659258262890683122, 1.000000000000000000, 0.9659258262890683122, 1.000000000000000000, 0.9659258262890683122, 1.000000000000000000, 0.9659258262890683122, 1.000000000000000000, 0.9659258262890683122, 1.000000000000000000, 0.9659258262890683122, 1.000000000000000000, 0.9659258262890683122, 1.000000000000000000, 0.9659258262890683122, 1.000000000000000000, 0.9659258262890683122, 1.000000000000000000, 0.9659258262890683122, 1.000000000000000000, 0.9659258262890683122, 1.000000000000000000, 0.9659258262890683122, 1.000000000000000000, 0.9659258262890683122, 1.000000000000000000, 0.9659258262890683122, 1.000000000000000000, 0.9659258262890683122, 1.000000000000000000, 0.9659258262890683122, 1.000000000000000000, 0.9659258262890683122, 1.000000000000000000, 0.9659258262890683122, 1.000000000000000000, 0.9659258262890683122, 1.000000000000000000, 0.9659258262890683122, 1.000000000000000000, 0.9659258262890683122, 1.000000000000000000, 0.9659258262890683122, 1.000000000000000000, 0.9659258262890683122, 1.000000000000000000, 0.9659258262890683122, 1.000000000000000000, 0.9659258262890683122, 1.000000000000000000, 0.9659258262890683122, 1.000000000000000000, 0.9659258262890683122, 1.000000000000000000, 0.9659258262890683122, 1.000000000000000000, 0.9659258262890683122, 1.000000000000000000, 0.9659258262890683122, 1.000000000000000000, 0.9659258262890683122, 1.000000000000000000, 0.9659258262890683122, 1.000000000000000000, 0.9659258262890683122, 1.000000000000000000, 0.9659258262890683122, 1.000000000000000000, 0.9659258262890683122, 1.000000000000000000, 0.9659258262890683122, 1.000000000000000000, 0.9659258262890683122, 1.000000000000000000, 0.9659258262890683122, 1.000000000000000000, 0.9659258262890683122, 1.000000000000000000, 0.9659258262890683122, 1.000000000000000000, 0.9659258262890683122, 1.000000000000000000, 0.9659258262890683122, 1.000000000000000000, 0.9659258262890683122, 1.000000000000000000, 0.9659258262890683122, 1.000000000000000000, 0.9659258262890683122, 1.000000000000000000, 0.9659258262890683122, 1.000000000000000000, 0.9659258262890683122, 1.000000000000000000, 0.9659258262890683122, 1.000000000000000000, 0.9659258262890683122, 1.000000000000000000, 0.9659258262890683122, 1.000000000000000000, 0.9659258262890683122, 1.000000000000000000, 0.9659258262890683122, 1.000000000000000000, 0.9659258262890683122, 1.000000000000000000, 0.9659258262890683122, 1.000000000000000000, 0.9659258262890683122, 1.000000000000000000, 0.9659258262890683122, 1.000000000000000000, 0.9659258262890683122, 1.000000000000000000, 0.9659258262890683122, 1.000000000000000000, 0.9659258262890683122, 1.000000000000000000, 0.9659258262890683122, 1.000000000000000000, 0.9659258262890683122, 1.000000000000000000, 0.9659258262890683122, 1.000000000000000000, 0.9659258262890683122, 1.000000000000000000, 0.9659258262890683122, 1.000000000000000000, 0.9659258262890683122, 1.000000000000000000, 0.9659258262890683122, 1.000000000000000000, 0.9659258262890683122, 1.000000000000000000, 0.9659258262890683122, 1.000000000000000000, 0.9659258262890683122, 1.000000000000000000, 0.9659258262890683122, 1.000000000000000000, 0.9659258262890683122, 1.000000000000000000, 0.9659258262890683122, 1.000000000000000000, 0.9659258262890683122, 1.000000000000000000, 0.9659258262890683122, 1.000000000000000000, 0.9659258262890683122, 1.000000000000000000, 0.9659258262890683122, 1.000000000000000000, 0.9659258262890683122, 1.000000000000000000, 0.9659258262890683122, 1.000000000000000000, 0.9659258262890683122, 1.000000000000000000, 0.9659258262890683122, 1.000000000000000000, 0.9659258262890683122, 1.000000000000000000, 0.9659258262890683122, 1.000000000000000000, 0.9659258262890683122, 1.000000000000000000, 0.9659258262890683122, 1.000000000000000000, 0.9659258262890683122, 1.000000000000000000, 0.9659258262890683122, 1.000000000000000000, 0.9659258262890683122, 1.000000000000000000, 0.9659258262890683122, 1.000000000000000000, 0.9659258262890683122, 1.000000000000000000, 0.9659258262890683122, 1.000000000000000000, 0.9659258262890683122, 1.000000000000000000, 0.9659258262890683122, 1.000000000000000000, 0.9659258262890683122, 1.000000000000000000, 0.9659258262890683122, 1.000000000000000000, 0.9659258262890683122, 1.000000000000000000, 0.9659258262890683122, 1.000000000000000000, 0.9659258262890683122, 1.000000000000000000, 0.9659258262890683122, 1.000000000000000000, 0.9659258262890683122, 1.000000000000000000, 0.9659258262890683122, 1.000000000000000000, 0.9659258262890683122, 1.000000000000000000, 0.9659258262890683122, 1.000000000000000000, 0.9659258262890683122, 1.000000000000000000, 0.9659258262890683122, 1.000000000000000000, 0.9659258262890683122, 1.000000000000000000, 0.9659258262890683122, 1.000000000000000000, 0.9659258262890683122, 1.000000000000000000, 0.9659258262890683122, 1.000000000000000000, 0.9659258262890683122, 1.000000000000000000, 0.9659258262890683122, 1.000000000000000000, 0.9659258262890683122, 1.000000000000000000, 0.9659258262890683122, 1.000000000000000000, 0.9659258262890683122, 1.000000000000000000, 0.9659258262890683122, 1.000000000000000000, 0.9659258262890683122, 1.000000000000000000, 0.9659258262890683122, 1.000000000000000000, 0.9659258262890683122, 1.000000000000000000, 0.9659258262890683122, 1.000000000000000000, 0.9659258262890683122, 1.000000000000000000, 0.9659258262890683122, 1.000000000000000000, 0.9659258262890683122, 1.000000000000000000, 0.9659258262890683122, 1.000000000000000000, 0.9659258262890683122, 1.000000000000000000, 0.9659258262890683122, 1.000000000000000000, 0.9659258262890683122, 1.000000000000000000, 0.9659258262890683122, 1.000000000000000000, 0.9659258262890683122, 1.000000000000000000, 0.9659258262890683122, 1.000000000000000000, 0.9659258262890683122, 1.000000000000000000, 0.9659258262890683122, 1.000000000000000000, 0.9659258262890683122, 1.000000000000000000, 0.9659258262890683122, 1.000000000000000000, 0.9659258262890683122, 1.000000000000000000, 0.9659258262890683122, 1.000000000000000000, 0.9659258262890683122, 1.000000000000000000, 0.9659258262890683122, 1.000000000000000000, 0.9659258262890683122, 1.000000000000000000, 0.9659258262890683122, 1.000000000000000000, 0.9659258262890683122, 1.000000000000000000, 0.9659258262890683122, 1.000000000000000000, 0.9659258262890683122, 1.000000000000000000, 0.9659258262890683122, 1.000000000000000000, 0.9659258262890683122, 1.000000000000000000, 0.9659258262890683122, 1.000000000000000000, 0.9659258262890683122, 1.000000000000000000, 0.9659258262890683122, 1.000000000000000000) ) ) 
 REPRESENTATION_ITEM ( '' )  SURFACE ( )  );
#53337=CARTESIAN_POINT ( 'NONE',  ( -1.220472440944881054, -0.5511811023622047445, 6.969142054262312111E-17 ) ) ;
#53339=CARTESIAN_POINT ( 'NONE',  ( -1.115485564304461219, -0.004921259842519870586, -0.3153832671262229437 ) ) ;
#53341=CARTESIAN_POINT ( 'NONE',  ( 0.01312335958005323398, -0.4281496062992127816, -0.4176697321401328100 ) ) ;
#53342=CARTESIAN_POINT ( 'NONE',  ( 2.795275590551181466, 2.793565526369266916, 0.000000000000000000 ) ) ;
#53343=CARTESIAN_POINT ( 'NONE',  ( 0.4658792650918640033, -0.2845877964562159024, 0.3641732283464567677 ) ) ;
#53344=CARTESIAN_POINT ( 'NONE',  ( -0.3740157480314953431, -0.4536011799217368745, -0.2665933059059886201 ) ) ;
#53345=CARTESIAN_POINT ( 'NONE',  ( -0.1574803149606292529, -0.1870078740157480879, -0.4822834645669291653 ) ) ;
#53346=CARTESIAN_POINT ( 'NONE',  ( -1.725721784776902190, -0.05778040916215522460, 0.4822834645669289988 ) ) ;
#53347=CARTESIAN_POINT ( 'NONE',  ( -1.095800524934382292, -0.2845877964562161244, -0.3641732283464567121 ) ) ;
#53349=CARTESIAN_POINT ( 'NONE',  ( 0.5577427821522316087, -0.05778040916215522460, 0.4822834645669289988 ) ) ;
#53350=ORIENTED_EDGE ( 'NONE', *, *, #58379, .T. ) ;
#53353=CARTESIAN_POINT ( 'NONE',  ( -0.3346456692913377662, -0.4536011799217367080, 0.2665933059059888421 ) ) ;
#53354=CARTESIAN_POINT ( 'NONE',  ( -1.437007874015747477, 0.1660481256975883668, -0.3530559997133364547 ) ) ;
#53355=CARTESIAN_POINT ( 'NONE',  ( 1.666666666666667185, 0.05413385826771666132, 0.4176697321401328100 ) ) ;
#53357=B_SPLINE_CURVE_WITH_KNOTS ( 'NONE', 3,
 ( #45637, #1057, #27123, #26711, #33023, #52787, #71333 ),
 .UNSPECIFIED., .F., .F.,
 ( 4, 3, 4 ),
 ( 6.162975822039154730E-33, 0.001246232571205225159, 0.002492492258783241162 ),
 .UNSPECIFIED. ) ;
#53358=CARTESIAN_POINT ( 'NONE',  ( -0.5183727034120726440, -0.5511811023622048555, -0.09757992244046775898 ) ) ;
#53360=CARTESIAN_POINT ( 'NONE',  ( 1.076115485564305141, -0.6046776061558807314, 0.2411417322834647770 ) ) ;
#53364=CARTESIAN_POINT ( 'NONE',  ( -1.719160104986876103, 0.05413385826771666132, 0.4176697321401328100 ) ) ;
#53365=CARTESIAN_POINT ( 'NONE',  ( -1.161417322834644716, -0.5400638737290845981, -0.3530559997133363437 ) ) ;
#53366=CARTESIAN_POINT ( 'NONE',  ( 1.391076115485564868, -0.6046776061558807314, 0.2411417322834647770 ) ) ;
#53368=CARTESIAN_POINT ( 'NONE',  ( 0.6167979002624679463, 0.05413385826771626580, -0.4176697321401330321 ) ) ;
#53369=CARTESIAN_POINT ( 'NONE',  ( -0.2034120734908128059, 0.2952755905511811885, 0.1292274648535926551 ) ) ;
#53373=CIRCLE ( 'NONE', #28610, 0.3937007874015748254 ) ;
#53374=CARTESIAN_POINT ( 'NONE',  ( 0.06680712611108469146, -6.211426067506147994E-17, -0.3627989612356148363 ) ) ;
#53375=CARTESIAN_POINT ( 'NONE',  ( 0.9186351706036751663, -0.5023911411419708095, 0.1820866141732285504 ) ) ;
#53378=ORIENTED_EDGE ( 'NONE', *, *, #81012, .T. ) ;
#53379=CARTESIAN_POINT ( 'NONE',  ( -0.3346456692913377662, -0.5400638737290844871, 0.3530559997133364547 ) ) ;
#53381=CARTESIAN_POINT ( 'NONE',  ( 1.279527559055118724, 0.1660481256975885056, 0.3530559997133364547 ) ) ;
#53382=CARTESIAN_POINT ( 'NONE',  ( 0.1377952755905518800, 0.1660481256975883668, -0.3530559997133364547 ) ) ;
#53383=CARTESIAN_POINT ( 'NONE',  ( -0.4658792650918627265, -0.2845877964562161244, -0.3641732283464567121 ) ) ;
#53384=CARTESIAN_POINT ( 'NONE',  ( 1.292650918635171564, -0.6692913385826773087, -0.1292274648535924053 ) ) ;
#53385=CARTESIAN_POINT ( 'NONE',  ( -1.030183727034119867, -0.3162353388693405765, 0.4822834645669290543 ) ) ;
#53386=CARTESIAN_POINT ( 'NONE',  ( 0.1181102362204730916, -0.6692913385826771977, 8.415575281601705876E-17 ) ) ;
#53387=CARTESIAN_POINT ( 'NONE',  ( -0.9120734908136475250, 0.2952755905511811885, 0.1292274648535926551 ) ) ;
#53388=CARTESIAN_POINT ( 'NONE',  ( 1.351706036745407458, -0.4281496062992127816, -0.4176697321401328100 ) ) ;
#53389=CARTESIAN_POINT ( 'NONE',  ( 0.8005249343832027131, 0.05413385826771666132, 0.4176697321401328100 ) ) ;
#53390=CARTESIAN_POINT ( 'NONE',  ( 1.076115485564305141, 0.2306618581243847221, -0.2411417322834647770 ) ) ;
#53392=CARTESIAN_POINT ( 'NONE',  ( 0.09186351706036827158, -0.004921259842519576551, 0.3153832671262227771 ) ) ;
#53395=VERTEX_POINT ( 'NONE', #23970 ) ;
#53396=CARTESIAN_POINT ( 'NONE',  ( -0.6627296587926503335, -0.5511811023622046335, 0.09757992244046803654 ) ) ;
#53397=CARTESIAN_POINT ( 'NONE',  ( -0.05905511811023545637, 0.1660481256975885056, 0.3530559997133364547 ) ) ;
#53398=LINE ( 'NONE', #79516, #9919 ) ;
#53399=CARTESIAN_POINT ( 'NONE',  ( -0.08530183727034056085, -0.05778040916215560624, -0.4822834645669293319 ) ) ;
#53400=CARTESIAN_POINT ( 'NONE',  ( -0.3280839895013117347, -0.4281496062992124485, 0.4176697321401328655 ) ) ;
#53401=CARTESIAN_POINT ( 'NONE',  ( -1.003937007874014853, 0.1660481256975885056, 0.3530559997133364547 ) ) ;
#53402=CARTESIAN_POINT ( 'NONE',  ( -1.128608923884513837, -0.6046776061558807314, 0.2411417322834647770 ) ) ;
#53403=CARTESIAN_POINT ( 'NONE',  ( 1.332020997375329197, -0.2845877964562159024, 0.3641732283464567677 ) ) ;
#53404=CARTESIAN_POINT ( 'NONE',  ( -1.496062992125983815, -0.1870078740157479769, 0.4822834645669291653 ) ) ;
#53406=CARTESIAN_POINT ( 'NONE',  ( 0.5380577427821529035, -0.004921259842519870586, -0.3153832671262229437 ) ) ;
#53407=CARTESIAN_POINT ( 'NONE',  ( 0.03280839895013198948, -0.6692913385826773087, -0.1292274648535924053 ) ) ;
#53408=CARTESIAN_POINT ( 'NONE',  ( 0.2690288713910767848, 0.2952755905511811885, 0.1292274648535926551 ) ) ;
#53409=ORIENTED_EDGE ( 'NONE', *, *, #61921, .F. ) ;
#53413=CARTESIAN_POINT ( 'NONE',  ( -0.4461942257217840213, 0.2306618581243848609, 0.2411417322834645549 ) ) ;
#53416=CARTESIAN_POINT ( 'NONE',  ( -1.463254593175852492, 0.1771653543307087630, 0.09757992244046791164 ) ) ;
#53417=CARTESIAN_POINT ( 'NONE',  ( 0.7349081364829402885, -0.6046776061558809534, -0.2411417322834644161 ) ) ;
#53418=CARTESIAN_POINT ( 'NONE',  ( 0.8005249343832028242, -0.4281496062992127816, -0.4176697321401328100 ) ) ;
#53419=CARTESIAN_POINT ( 'NONE',  ( -0.2887139107611542133, -0.5023911411419708095, -0.1820866141732282451 ) ) ;
#53420=CARTESIAN_POINT ( 'NONE',  ( 0.2034120734908142214, 0.2952755905511810774, -0.1292274648535930714 ) ) ;
#53422=CARTESIAN_POINT ( 'NONE',  ( -0.1049868766404193215, -0.5023911411419708095, 0.1820866141732285504 ) ) ;
#53423=CARTESIAN_POINT ( 'NONE',  ( -0.2296587926509179312, -0.3162353388693409650, -0.4822834645669289433 ) ) ;
#53426=CARTESIAN_POINT ( 'NONE',  ( 1.594488188976378673, 0.07958543189024085140, 0.2665933059059887866 ) ) ;
#53427=CARTESIAN_POINT ( 'NONE',  ( -0.07217847769028813698, -0.2845877964562161244, -0.3641732283464567121 ) ) ;
#53428=CARTESIAN_POINT ( 'NONE',  ( 1.522309711286089939, 0.1283753931104748280, 0.1820866141732283561 ) ) ;
#53429=CARTESIAN_POINT ( 'NONE',  ( -0.6955380577427815458, -0.4281496062992127816, -0.4176697321401328100 ) ) ;
#53430=CARTESIAN_POINT ( 'NONE',  ( -0.6758530183727028406, 0.1771653543307087630, 0.09757992244046791164 ) ) ;
#53432=CARTESIAN_POINT ( 'NONE',  ( -0.5511811023622041894, -0.1870078740157480879, -0.4822834645669291653 ) ) ;
#53433=CARTESIAN_POINT ( 'NONE',  ( -0.6364829396325453192, -0.05778040916215560624, -0.4822834645669293319 ) ) ;
#53434=CARTESIAN_POINT ( 'NONE',  ( -0.1968503937007867743, 0.2952755905511811885, 0.000000000000000000 ) ) ;
#53438=CARTESIAN_POINT ( 'NONE',  ( 0.6233595800524942554, -0.08942795157528024563, -0.3641732283464568787 ) ) ;
#53439=CARTESIAN_POINT ( 'NONE',  ( 1.528871391076116026, -0.6692913385826773087, -0.1292274648535924053 ) ) ;
#53440=CARTESIAN_POINT ( 'NONE',  ( -1.423884514435694859, -0.2845877964562159024, 0.3641732283464567677 ) ) ;
#53441=CARTESIAN_POINT ( 'NONE',  ( 1.299212598425197429, -0.6692913385826771977, 8.415575281601705876E-17 ) ) ;
#53442=CARTESIAN_POINT ( 'NONE',  ( -0.9908136482939626788, -0.5511811023622048555, -0.09757992244046775898 ) ) ;
#53443=CARTESIAN_POINT ( 'NONE',  ( -0.5971128608923877978, 0.2952755905511811885, 0.1292274648535926551 ) ) ;
#53444=CARTESIAN_POINT ( 'NONE',  ( 0.1837270341207357105, -0.5023911411419708095, -0.1820866141732282451 ) ) ;
#53445=CARTESIAN_POINT ( 'NONE',  ( 1.611560603071419129, 0.2819760470925486984, 0.1148666718267763592 ) ) ;
#53446=CARTESIAN_POINT ( 'NONE',  ( 1.135170603674541256, 0.1771653543307087630, 0.09757992244046791164 ) ) ;
#53447=CARTESIAN_POINT ( 'NONE',  ( 0.2690288713910767848, 0.2952755905511811885, 0.1292274648535926551 ) ) ;
#53449=CARTESIAN_POINT ( 'NONE',  ( -0.7677165354330699465, 0.1660481256975885056, 0.3530559997133364547 ) ) ;
#53451=CARTESIAN_POINT ( 'NONE',  ( 1.043307086614173818, -0.4536011799217368745, -0.2665933059059886201 ) ) ;
#53452=CARTESIAN_POINT ( 'NONE',  ( 0.2887139107611556010, 0.2306618581243847221, -0.2411417322834647770 ) ) ;
#53453=CARTESIAN_POINT ( 'NONE',  ( -0.2559055118110227234, -0.5400638737290844871, 0.3530559997133364547 ) ) ;
#53454=CARTESIAN_POINT ( 'NONE',  ( 0.1771653543307093182, -0.4536011799217368745, -0.2665933059059886201 ) ) ;
#53456=CARTESIAN_POINT ( 'NONE',  ( 0.03280839895013198948, -0.5511811023622048555, -0.09757992244046775898 ) ) ;
#53457=CARTESIAN_POINT ( 'NONE',  ( 0.1640419947506569498, -0.3162353388693409650, -0.4822834645669289433 ) ) ;
#53458=CARTESIAN_POINT ( 'NONE',  ( -0.9317585301837263412, -0.004921259842519576551, 0.3153832671262227771 ) ) ;
#53460=CARTESIAN_POINT ( 'NONE',  ( -1.017060367454067249, -0.05778040916215522460, 0.4822834645669289988 ) ) ;
#53461=CARTESIAN_POINT ( 'NONE',  ( 2.795275590551181466, 0.7874015748031495399, -2.695814348275282069E-16 ) ) ;
#53463=CARTESIAN_POINT ( 'NONE',  ( -1.108923884514435132, -0.2845877964562159024, 0.3641732283464567677 ) ) ;
#53464=CARTESIAN_POINT ( 'NONE',  ( -0.04593175853018302557, -0.6692913385826773087, -0.1292274648535924053 ) ) ;
#53465=CARTESIAN_POINT ( 'NONE',  ( -1.548556430446193399, 0.2306618581243848609, 0.2411417322834645549 ) ) ;
#53466=CARTESIAN_POINT ( 'NONE',  ( -0.7742782152230962556, -0.4281496062992127816, -0.4176697321401328100 ) ) ;
#53467=CARTESIAN_POINT ( 'NONE',  ( -1.614173228346457378, 2.157411728916712068, -0.1372047244094477536 ) ) ;
#53468=CARTESIAN_POINT ( 'NONE',  ( 1.049868766404200349, 0.2306618581243848609, 0.2411417322834645549 ) ) ;
#53469=CARTESIAN_POINT ( 'NONE',  ( 1.089238845144357537, -0.4281496062992124485, 0.4176697321401328655 ) ) ;
#53470=CARTESIAN_POINT ( 'NONE',  ( 0.7611548556430454138, 0.2306618581243847221, -0.2411417322834647770 ) ) ;
#53472=CARTESIAN_POINT ( 'NONE',  ( 1.469816272965879911, 0.2306618581243847221, -0.2411417322834647770 ) ) ;
#53473=CARTESIAN_POINT ( 'NONE',  ( -1.338582677165353729, -0.1870078740157480879, -0.4822834645669291653 ) ) ;
#53475=VERTEX_POINT ( 'NONE', #82065 ) ;
#53476=CARTESIAN_POINT ( 'NONE',  ( -0.3740157480314953431, 0.07958543189024085140, 0.2665933059059887866 ) ) ;
#53478=EDGE_LOOP ( 'NONE', ( #43627, #74920, #29341, #40843, #37338, #33548, #58134, #59780 ) ) ;
#53479=CARTESIAN_POINT ( 'NONE',  ( 0.8792650918635177559, -0.4281496062992127816, -0.4176697321401328100 ) ) ;
#53480=CARTESIAN_POINT ( 'NONE',  ( -0.1115485564304456306, 0.2952755905511810774, -0.1292274648535930714 ) ) ;
#53481=CARTESIAN_POINT ( 'NONE',  ( -0.8136482939632537770, 0.2306618581243847221, -0.2411417322834647770 ) ) ;
#53482=CARTESIAN_POINT ( 'NONE',  ( 1.673228346456693494, 0.1660481256975885056, 0.3530559997133364547 ) ) ;
#53483=CARTESIAN_POINT ( 'NONE',  ( -1.069553805774277722, -0.5511811023622048555, -0.09757992244046775898 ) ) ;
#53485=CARTESIAN_POINT ( 'NONE',  ( 0.5249343832021005074, -0.6046776061558807314, 0.2411417322834647770 ) ) ;
#53486=CARTESIAN_POINT ( 'NONE',  ( 0.6299212598425204535, -0.1870078740157479769, 0.3641732283464567677 ) ) ;
#53487=CARTESIAN_POINT ( 'NONE',  ( -0.5577427821522301654, -0.3162353388693405765, 0.4822834645669290543 ) ) ;
#53489=CARTESIAN_POINT ( 'NONE',  ( -1.325459317585300889, 0.05413385826771666132, 0.4176697321401328100 ) ) ;
#53491=DIRECTION ( 'NONE',  ( -1.000000000000000000, -3.469446951953613696E-16, 0.000000000000000000 ) ) ;
#53492=CARTESIAN_POINT ( 'NONE',  ( 1.253280839895013710, -0.05778040916215560624, -0.4822834645669293319 ) ) ;
#53493=CARTESIAN_POINT ( 'NONE',  ( 1.391076115485564868, 0.1283753931104746893, -0.1820866141732285504 ) ) ;
#53496=CARTESIAN_POINT ( 'NONE',  ( -0.3018372703412066094, -0.4281496062992127816, -0.4176697321401328100 ) ) ;
#53497=ORIENTED_EDGE ( 'NONE', *, *, #30564, .T. ) ;
#53499=CARTESIAN_POINT ( 'NONE',  ( 0.6758530183727039509, 0.1771653543307087075, -0.09757992244046823083 ) ) ;
#53500=CARTESIAN_POINT ( 'NONE',  ( -1.141732283464566011, -0.6692913385826771977, 8.415575281601705876E-17 ) ) ;
#53501=CARTESIAN_POINT ( 'NONE',  ( 0.9776902887139113929, 0.2952755905511811885, 0.1292274648535926551 ) ) ;
#53502=CARTESIAN_POINT ( 'NONE',  ( 0.9711286089238851948, 0.2306618581243848609, 0.2411417322834645549 ) ) ;
#53503=CARTESIAN_POINT ( 'NONE',  ( 0.1377952755905518800, -0.5400638737290844871, 0.3530559997133364547 ) ) ;
#53504=CARTESIAN_POINT ( 'NONE',  ( -0.5314960629921250401, 0.1660481256975885056, 0.3530559997133364547 ) ) ;
#53506=CARTESIAN_POINT ( 'NONE',  ( 1.555118110236221041, -0.4536011799217367080, 0.2665933059059888421 ) ) ;
#53507=CARTESIAN_POINT ( 'NONE',  ( -0.5905511811023613777, -0.6692913385826771977, 8.415575281601705876E-17 ) ) ;
#53508=CARTESIAN_POINT ( 'NONE',  ( -0.5577427821522301654, -0.2845877964562159024, 0.3641732283464567677 ) ) ;
#53509=CARTESIAN_POINT ( 'NONE',  ( 1.679790026246720025, 0.2306618581243848609, 0.2411417322834645549 ) ) ;
#53511=CARTESIAN_POINT ( 'NONE',  ( -0.5380577427821514602, -0.4281496062992127816, -0.4176697321401328100 ) ) ;
#53513=CARTESIAN_POINT ( 'NONE',  ( 0.8792650918635177559, -0.4281496062992127816, -0.4176697321401328100 ) ) ;
#53517=CARTESIAN_POINT ( 'NONE',  ( -0.2099737532808391705, 0.2306618581243848609, 0.2411417322834645549 ) ) ;
#53518=CARTESIAN_POINT ( 'NONE',  ( 1.233595800524935227, 0.1283753931104746893, -0.1820866141732285504 ) ) ;
#53519=CARTESIAN_POINT ( 'NONE',  ( -1.646051170424378096, 0.000000000000000000, -0.3464511005275205946 ) ) ;
#53521=CARTESIAN_POINT ( 'NONE',  ( 1.384514435695538559, 0.1771653543307087075, -0.09757992244046823083 ) ) ;
#53522=CARTESIAN_POINT ( 'NONE',  ( 1.141732283464567566, 0.2952755905511811885, 0.000000000000000000 ) ) ;
#53524=CARTESIAN_POINT ( 'NONE',  ( -0.4199475065616791736, 0.2306618581243847221, -0.2411417322834647770 ) ) ;
#53525=CARTESIAN_POINT ( 'NONE',  ( -1.541994750656167090, -0.6692913385826773087, -0.1292274648535924053 ) ) ;
#53526=CARTESIAN_POINT ( 'NONE',  ( -1.391076115485563758, 0.2306618581243848609, 0.2411417322834645549 ) ) ;
#53527=CARTESIAN_POINT ( 'NONE',  ( -0.01312335958005186876, -0.4281496062992124485, 0.4176697321401328655 ) ) ;
#53529=CARTESIAN_POINT ( 'NONE',  ( 1.095800524934383846, -0.05778040916215560624, -0.4822834645669293319 ) ) ;
#53530=CARTESIAN_POINT ( 'NONE',  ( 0.4002624671916016896, -0.3162353388693409650, -0.4822834645669289433 ) ) ;
#53531=CARTESIAN_POINT ( 'NONE',  ( 0.5380577427821529035, -0.3690944881889763329, 0.3153832671262228327 ) ) ;
#53533=CARTESIAN_POINT ( 'NONE',  ( 0.5577427821522316087, -0.08942795157527998196, 0.3641732283464567121 ) ) ;
#53534=CARTESIAN_POINT ( 'NONE',  ( -1.561679790026246017, -0.4281496062992127816, -0.4176697321401328100 ) ) ;
#53536=CARTESIAN_POINT ( 'NONE',  ( 0.9448818897637802916, -0.1870078740157480879, -0.4822834645669291653 ) ) ;
#53540=CARTESIAN_POINT ( 'NONE',  ( 0.01968503937007930540, 0.07958543189024085140, 0.2665933059059887866 ) ) ;
#53541=CARTESIAN_POINT ( 'NONE',  ( 0.6036745406824154392, 0.2306618581243847221, -0.2411417322834647770 ) ) ;
#53542=CARTESIAN_POINT ( 'NONE',  ( 1.286089238845145033, -0.5023911411419708095, -0.1820866141732282451 ) ) ;
#53543=CARTESIAN_POINT ( 'NONE',  ( -1.299212598425196097, -0.5511811023622047445, 6.969142054262312111E-17 ) ) ;
#53544=CARTESIAN_POINT ( 'NONE',  ( -0.9842519685039365918, -0.6692913385826771977, 8.415575281601705876E-17 ) ) ;
#53545=CARTESIAN_POINT ( 'NONE',  ( -1.686351706036744558, 0.2952755905511810774, -0.1292274648535930714 ) ) ;
#53546=CARTESIAN_POINT ( 'NONE',  ( 0.5052493438320218022, -0.6692913385826773087, -0.1292274648535924053 ) ) ;
#53547=CARTESIAN_POINT ( 'NONE',  ( 1.463254593175853824, -0.6692913385826771977, 0.1292274648535927661 ) ) ;
#53549=CARTESIAN_POINT ( 'NONE',  ( 0.7414698162729663755, -0.6692913385826773087, -0.1292274648535924053 ) ) ;
#53551=CARTESIAN_POINT ( 'NONE',  ( 1.568241469816273659, -0.05778040916215560624, -0.4822834645669293319 ) ) ;
#53552=CARTESIAN_POINT ( 'NONE',  ( 1.246719160104987623, 0.05413385826771626580, -0.4176697321401330321 ) ) ;
#53553=CARTESIAN_POINT ( 'NONE',  ( -1.253280839895012377, -0.08942795157527998196, 0.3641732283464567121 ) ) ;
#53554=CARTESIAN_POINT ( 'NONE',  ( 1.299212598425197429, -0.5511811023622047445, 6.969142054262312111E-17 ) ) ;
#53555=CARTESIAN_POINT ( 'NONE',  ( -1.279527559055116948, 0.07958543189024071263, -0.2665933059059888421 ) ) ;
#53556=CARTESIAN_POINT ( 'NONE',  ( -0.8661417322834640276, -0.1870078740157479769, 0.3641732283464567677 ) ) ;
#53558=CARTESIAN_POINT ( 'NONE',  ( 0.6167979002624678353, -0.3690944881889763329, 0.3153832671262228327 ) ) ;
#53559=CARTESIAN_POINT ( 'NONE',  ( 0.2230971128608932319, -0.4281496062992124485, 0.4176697321401328655 ) ) ;
#53560=CARTESIAN_POINT ( 'NONE',  ( 1.076115485564305141, -0.6046776061558807314, 0.2411417322834647770 ) ) ;
#53561=CARTESIAN_POINT ( 'NONE',  ( 0.05905511811023709395, -0.5400638737290844871, 0.3530559997133364547 ) ) ;
#53562=CARTESIAN_POINT ( 'NONE',  ( 0.04593175853018440641, 0.1771653543307087075, -0.09757992244046823083 ) ) ;
#53563=CARTESIAN_POINT ( 'NONE',  ( 1.089238845144357537, -0.4281496062992124485, 0.4176697321401328655 ) ) ;
#53564=CARTESIAN_POINT ( 'NONE',  ( -0.2230971128608915666, 0.009842519685039467087, 0.3409548833797002021 ) ) ;
#53565=CARTESIAN_POINT ( 'NONE',  ( -0.9908136482939626788, -0.6692913385826773087, -0.1292274648535924053 ) ) ;
#53567=CARTESIAN_POINT ( 'NONE',  ( 1.011689015874864372, 1.456472319277303872E-16, -0.3627989612356145588 ) ) ;
#53568=CARTESIAN_POINT ( 'NONE',  ( -0.8202099737532799750, 0.2952755905511810774, -0.1292274648535930714 ) ) ;
#53569=CARTESIAN_POINT ( 'NONE',  ( -0.2427821522309703550, -0.05778040916215560624, -0.4822834645669293319 ) ) ;
#53575=CARTESIAN_POINT ( 'NONE',  ( -1.253280839895012377, -0.08942795157527998196, 0.3641732283464567121 ) ) ;
#53577=CARTESIAN_POINT ( 'NONE',  ( -1.587926509186350810, -0.4281496062992124485, 0.4176697321401328655 ) ) ;
#53579=CARTESIAN_POINT ( 'NONE',  ( -0.1115485564304453947, -0.6692913385826771977, 0.1292274648535927661 ) ) ;
#53580=CARTESIAN_POINT ( 'NONE',  ( -0.5249343832020990641, -0.5023911411419708095, -0.1820866141732282451 ) ) ;
#53581=CARTESIAN_POINT ( 'NONE',  ( 0.7939632545931766261, -0.05778040916215522460, 0.4822834645669289988 ) ) ;
#53582=CARTESIAN_POINT ( 'NONE',  ( 0.5052493438320215802, 0.2952755905511811885, 0.1292274648535926551 ) ) ;
#53586=CARTESIAN_POINT ( 'NONE',  ( 1.227034120734908917, 0.2952755905511810774, -0.1292274648535930714 ) ) ;
#53587=CARTESIAN_POINT ( 'NONE',  ( -0.1181102362204717315, 0.2952755905511811885, 0.000000000000000000 ) ) ;
#53588=CARTESIAN_POINT ( 'NONE',  ( -0.8333333333333323711, 0.2952755905511811885, 0.1292274648535926551 ) ) ;
#53589=CARTESIAN_POINT ( 'NONE',  ( 1.568241469816273437, -0.3162353388693405765, 0.4822834645669290543 ) ) ;
#53590=CARTESIAN_POINT ( 'NONE',  ( 0.7874015748031503170, -0.1870078740157480879, -0.4822834645669291653 ) ) ;
#53592=CARTESIAN_POINT ( 'NONE',  ( -0.006561679790025524116, -0.3162353388693405765, 0.4822834645669290543 ) ) ;
#53593=CARTESIAN_POINT ( 'NONE',  ( 0.6233595800524942554, -0.05778040916215560624, -0.4822834645669293319 ) ) ;
#53594=CARTESIAN_POINT ( 'NONE',  ( 0.1312335958005257930, 0.2306618581243847221, -0.2411417322834647770 ) ) ;
#53595=CARTESIAN_POINT ( 'NONE',  ( 0.7020997375328090762, -0.2845877964562159024, 0.3641732283464567677 ) ) ;
#53596=CARTESIAN_POINT ( 'NONE',  ( -1.456692913385826182, -0.6692913385826771977, 8.415575281601705876E-17 ) ) ;
#53597=CARTESIAN_POINT ( 'NONE',  ( -1.207349081364828880, 0.2306618581243847221, -0.2411417322834647770 ) ) ;
#53598=CARTESIAN_POINT ( 'NONE',  ( 0.9383202099737536495, -0.3162353388693405765, 0.4822834645669290543 ) ) ;
#53603=ORIENTED_EDGE ( 'NONE', *, *, #37540, .F. ) ;
#53605=CARTESIAN_POINT ( 'NONE',  ( 0.9317585301837276734, 0.05413385826771626580, -0.4176697321401330321 ) ) ;
#53606=CARTESIAN_POINT ( 'NONE',  ( 0.4986876640419954376, 0.1283753931104748280, 0.1820866141732283561 ) ) ;
#53612=CARTESIAN_POINT ( 'NONE',  ( -0.1574803149606292529, -0.1870078740157479769, 0.4822834645669291653 ) ) ;
#53613=CARTESIAN_POINT ( 'NONE',  ( 0.9186351706036751663, -0.6046776061558807314, 0.2411417322834647770 ) ) ;
#53615=CARTESIAN_POINT ( 'NONE',  ( -1.692913385826770645, 0.2952755905511811885, 0.000000000000000000 ) ) ;
#53618=CARTESIAN_POINT ( 'NONE',  ( 1.489501312335958172, -0.2845877964562159024, 0.3641732283464567677 ) ) ;
#53620=CARTESIAN_POINT ( 'NONE',  ( -1.371391076115484609, -0.5511811023622046335, 0.09757992244046803654 ) ) ;
#53621=CARTESIAN_POINT ( 'NONE',  ( -1.574803149606298192, -0.1870078740157480879, -0.4822834645669291653 ) ) ;
#53622=CARTESIAN_POINT ( 'NONE',  ( 0.1377952755905518800, 0.1660481256975883668, -0.3530559997133364547 ) ) ;
#53623=ORIENTED_EDGE ( 'NONE', *, *, #8579, .T. ) ;
#53624=CARTESIAN_POINT ( 'NONE',  ( 1.568241469816273659, -0.05778040916215560624, -0.4822834645669293319 ) ) ;
#53626=CARTESIAN_POINT ( 'NONE',  ( -0.5380577427821514602, -0.3690944881889765550, -0.3153832671262227771 ) ) ;
#53627=CARTESIAN_POINT ( 'NONE',  ( 0.9973753280839902091, -0.6046776061558807314, 0.2411417322834647770 ) ) ;
#53628=CARTESIAN_POINT ( 'NONE',  ( 1.082677165354331228, -0.4536011799217367080, 0.2665933059059888421 ) ) ;
#53630=CARTESIAN_POINT ( 'NONE',  ( -0.6758530183727028406, -0.5511811023622048555, -0.09757992244046775898 ) ) ;
#53631=CARTESIAN_POINT ( 'NONE',  ( -1.377952755905511140, -0.5511811023622047445, 6.969142054262312111E-17 ) ) ;
#53633=CARTESIAN_POINT ( 'NONE',  ( 0.6496062992125991586, 0.1660481256975885056, 0.3530559997133364547 ) ) ;
#53634=CARTESIAN_POINT ( 'NONE',  ( -0.9120734908136475250, -0.5511811023622048555, -0.09757992244046775898 ) ) ;
#53635=CARTESIAN_POINT ( 'NONE',  ( -0.3740157480314953431, -0.4536011799217368745, -0.2665933059059886201 ) ) ;
#53637=CARTESIAN_POINT ( 'NONE',  ( -0.2165354330708654795, -0.5400638737290845981, -0.3530559997133363437 ) ) ;
#53638=CARTESIAN_POINT ( 'NONE',  ( -1.351706036745406347, -0.3690944881889763329, 0.3153832671262228327 ) ) ;
#53640=CARTESIAN_POINT ( 'NONE',  ( 0.5446194225721792126, -0.05778040916215560624, -0.4822834645669293319 ) ) ;
#53641=EDGE_CURVE ( 'NONE', #50964, #78564, #34197, .T. ) ;
#53644=CARTESIAN_POINT ( 'NONE',  ( -0.8267716535433065062, -0.6692913385826771977, 8.415575281601705876E-17 ) ) ;
#53645=CARTESIAN_POINT ( 'NONE',  ( -0.3543307086614165824, -0.5511811023622047445, 6.969142054262312111E-17 ) ) ;
#53646=CARTESIAN_POINT ( 'NONE',  ( -1.154855643044618851, 0.2306618581243848609, 0.2411417322834645549 ) ) ;
#53647=CARTESIAN_POINT ( 'NONE',  ( 0.3674540682414705883, -0.5023911411419708095, 0.1820866141732285504 ) ) ;
#53648=CARTESIAN_POINT ( 'NONE',  ( -0.5971128608923877978, 0.1771653543307087630, 0.09757992244046791164 ) ) ;
#53649=CARTESIAN_POINT ( 'NONE',  ( -1.259842519685038686, -0.1870078740157479769, 0.4822834645669291653 ) ) ;
#53650=CARTESIAN_POINT ( 'NONE',  ( -1.725721784776902190, -0.05778040916215522460, 0.4822834645669289988 ) ) ;
#53651=CARTESIAN_POINT ( 'NONE',  ( 1.246719160104987623, 0.05413385826771626580, -0.4176697321401330321 ) ) ;
#53652=CARTESIAN_POINT ( 'NONE',  ( 1.043307086614173818, 0.1012011053420777407, 0.2882089793578256898 ) ) ;
#53653=CARTESIAN_POINT ( 'NONE',  ( 1.010498687664042716, -0.3690944881889763329, 0.3153832671262228327 ) ) ;
#53654=CARTESIAN_POINT ( 'NONE',  ( 0.2690288713910767848, 0.2952755905511811885, 0.1292274648535926551 ) ) ;
#53655=CARTESIAN_POINT ( 'NONE',  ( -1.384514435695537005, -0.6692913385826773087, -0.1292274648535924053 ) ) ;
#53656=CARTESIAN_POINT ( 'NONE',  ( 1.286089238845145033, 0.1283753931104748280, 0.1820866141732283561 ) ) ;
#53660=CARTESIAN_POINT ( 'NONE',  ( -1.174540682414697335, -0.08942795157527998196, 0.3641732283464567121 ) ) ;
#53661=CARTESIAN_POINT ( 'NONE',  ( -0.3280839895013117347, 0.05413385826771626580, -0.4176697321401330321 ) ) ;
#53662=CARTESIAN_POINT ( 'NONE',  ( 0.4921259842519691285, 0.1660481256975885056, 0.3530559997133364547 ) ) ;
#53663=CARTESIAN_POINT ( 'NONE',  ( -1.384514435695537005, 0.1771653543307087630, 0.09757992244046791164 ) ) ;
#53665=CARTESIAN_POINT ( 'NONE',  ( -1.279527559055116948, -0.5400638737290844871, 0.3530559997133364547 ) ) ;
#53666=CARTESIAN_POINT ( 'NONE',  ( 0.3608923884514443348, -0.6692913385826771977, 0.1292274648535927661 ) ) ;
#53667=CARTESIAN_POINT ( 'NONE',  ( -0.03937007874015669567, 0.2952755905511811885, 0.000000000000000000 ) ) ;
#53668=CARTESIAN_POINT ( 'NONE',  ( 1.299212598425197429, 0.2952755905511811885, 0.000000000000000000 ) ) ;
#53673=CARTESIAN_POINT ( 'NONE',  ( -0.04593175853018302557, -0.5511811023622048555, -0.09757992244046775898 ) ) ;
#53674=CARTESIAN_POINT ( 'NONE',  ( -0.3149606299212590610, -0.1870078740157479769, 0.4822834645669291653 ) ) ;
#53675=CARTESIAN_POINT ( 'NONE',  ( 1.062992125984252745, -0.6692913385826771977, 8.415575281601705876E-17 ) ) ;
#53677=CARTESIAN_POINT ( 'NONE',  ( 0.07874015748031558404, -0.1870078740157479769, 0.3641732283464567677 ) ) ;
#53678=CARTESIAN_POINT ( 'NONE',  ( -1.233595800524933894, -0.6046776061558809534, -0.2411417322834644161 ) ) ;
#53679=CARTESIAN_POINT ( 'NONE',  ( 1.561679790026247350, -0.4281496062992124485, 0.4176697321401328655 ) ) ;
#53684=CARTESIAN_POINT ( 'NONE',  ( 1.207349081364829990, -0.6046776061558809534, -0.2411417322834644161 ) ) ;
#53685=CARTESIAN_POINT ( 'NONE',  ( 1.476377952755906220, 0.07958543189024071263, -0.2665933059059888421 ) ) ;
#53686=CARTESIAN_POINT ( 'NONE',  ( -1.030183727034119867, -0.2845877964562159024, 0.3641732283464567677 ) ) ;
#53687=CARTESIAN_POINT ( 'NONE',  ( -1.102362204724408601, -0.1870078740157480879, -0.4822834645669291653 ) ) ;
#53689=DIRECTION ( 'NONE',  ( 0.000000000000000000, 0.000000000000000000, -1.000000000000000000 ) ) ;
#53690=CARTESIAN_POINT ( 'NONE',  ( 1.023622047244095334, -0.1870078740157479769, 0.4822834645669291653 ) ) ;
#53691=CARTESIAN_POINT ( 'NONE',  ( -1.607611548556429737, -0.6692913385826771977, 0.1292274648535927661 ) ) ;
#53692=CARTESIAN_POINT ( 'NONE',  ( -0.1640419947506555343, -0.3162353388693405765, 0.4822834645669290543 ) ) ;
#53693=CARTESIAN_POINT ( 'NONE',  ( -0.3477690288713905509, -0.6692913385826771977, 0.1292274648535927661 ) ) ;
#53694=CARTESIAN_POINT ( 'NONE',  ( -1.305774278215222184, 0.2952755905511811885, 0.1292274648535926551 ) ) ;
#53696=CARTESIAN_POINT ( 'NONE',  ( 0.6036745406824153282, -0.6046776061558807314, 0.2411417322834647770 ) ) ;
#53698=CARTESIAN_POINT ( 'NONE',  ( -1.391076115485563314, -0.5023911411419708095, -0.1820866141732282451 ) ) ;
#53703=CARTESIAN_POINT ( 'NONE',  ( -1.371391076115484831, 0.2952755905511810774, -0.1292274648535930714 ) ) ;
#53704=CARTESIAN_POINT ( 'NONE',  ( -1.240157480314959759, -0.5400638737290845981, -0.3530559997133363437 ) ) ;
#53706=CARTESIAN_POINT ( 'NONE',  ( -1.633858267716534529, -0.5400638737290845981, -0.3530559997133363437 ) ) ;
#53707=CARTESIAN_POINT ( 'NONE',  ( -1.627296587926508442, -0.6046776061558809534, -0.2411417322834644161 ) ) ;
#53708=EDGE_CURVE ( 'NONE', #40053, #1230, #44392, .T. ) ;
#53709=CARTESIAN_POINT ( 'NONE',  ( 0.4608550785314886045, 0.02791078216816508459, -0.4328096321851889194 ) ) ;
#53712=CARTESIAN_POINT ( 'NONE',  ( 0.05249343832021075018, -0.5023911411419708095, 0.1820866141732285504 ) ) ;
#53713=CARTESIAN_POINT ( 'NONE',  ( -0.7086614173228339419, -0.1870078740157480601, -0.3641732283464567677 ) ) ;
#53714=CARTESIAN_POINT ( 'NONE',  ( -1.227034120734907141, -0.6692913385826773087, -0.1292274648535924053 ) ) ;
#53715=CARTESIAN_POINT ( 'NONE',  ( 1.062992125984252745, -0.6692913385826771977, 8.415575281601705876E-17 ) ) ;
#53716=CARTESIAN_POINT ( 'NONE',  ( -0.8333333333333323711, 0.2952755905511811885, 0.1292274648535926551 ) ) ;
#53719=CARTESIAN_POINT ( 'NONE',  ( -1.561679790026246017, -0.4281496062992127816, -0.4176697321401328100 ) ) ;
#53720=CARTESIAN_POINT ( 'NONE',  ( -1.725721784776902190, -0.08942795157527998196, 0.3641732283464567121 ) ) ;
#53727=CARTESIAN_POINT ( 'NONE',  ( -0.1640419947506553400, -0.05778040916215560624, -0.4822834645669293319 ) ) ;
#53728=CARTESIAN_POINT ( 'NONE',  ( -1.502624671916009680, -0.2845877964562159024, 0.3641732283464567677 ) ) ;
#53730=LINE ( 'NONE', #47420, #74568 ) ;
#53731=CARTESIAN_POINT ( 'NONE',  ( -0.6958886929845781166, 0.004960608223778821026, 0.3437734562760189072 ) ) ;
#53732=CARTESIAN_POINT ( 'NONE',  ( -1.410761154855642463, -0.05778040916215522460, 0.4822834645669289988 ) ) ;
#53733=CARTESIAN_POINT ( 'NONE',  ( -0.3149606299212590610, -0.1870078740157479769, 0.4822834645669291653 ) ) ;
#53735=CARTESIAN_POINT ( 'NONE',  ( 0.3937007874015754361, -0.1870078740157480601, -0.3641732283464567677 ) ) ;
#53736=CARTESIAN_POINT ( 'NONE',  ( -2.795275590551185907, 0.4724409448818907564, -3.981376139758521912E-16 ) ) ;
#53737=CARTESIAN_POINT ( 'NONE',  ( 0.3149606299212606708, -0.1870078740157480601, -0.3641732283464567677 ) ) ;
#53738=CARTESIAN_POINT ( 'NONE',  ( 0.8464566929133865436, 0.07958543189024071263, -0.2665933059059888421 ) ) ;
#53739=CARTESIAN_POINT ( 'NONE',  ( 1.036745406824147508, -0.4281496062992127816, -0.4176697321401328100 ) ) ;
#53740=CARTESIAN_POINT ( 'NONE',  ( -0.4527559055118102749, -0.4536011799217368745, -0.2665933059059886201 ) ) ;
#53742=CARTESIAN_POINT ( 'NONE',  ( -1.358267716535432434, -0.5400638737290844871, 0.3530559997133364547 ) ) ;
#53743=CARTESIAN_POINT ( 'NONE',  ( 0.04593175853018440641, 0.1771653543307087075, -0.09757992244046823083 ) ) ;
#53744=CARTESIAN_POINT ( 'NONE',  ( -1.450131233595799651, 0.1771653543307087075, -0.09757992244046823083 ) ) ;
#53746=CARTESIAN_POINT ( 'NONE',  ( -0.8858267716535425107, -0.4536011799217367080, 0.2665933059059888421 ) ) ;
#53748=CARTESIAN_POINT ( 'NONE',  ( -0.2230971128608915943, 0.05413385826771666132, 0.4176697321401328100 ) ) ;
#53749=CARTESIAN_POINT ( 'NONE',  ( 1.463254593175853824, -0.5511811023622046335, 0.09757992244046803654 ) ) ;
#53750=CARTESIAN_POINT ( 'NONE',  ( 0.6036745406824153282, -0.5023911411419708095, 0.1820866141732285504 ) ) ;
#53751=CARTESIAN_POINT ( 'NONE',  ( -0.4265091863517051496, 0.1771653543307087075, -0.09757992244046823083 ) ) ;
#53752=CARTESIAN_POINT ( 'NONE',  ( -0.3740157480314953431, 0.1660481256975885056, 0.3530559997133364547 ) ) ;
#53754=CARTESIAN_POINT ( 'NONE',  ( -1.253280839895012377, -0.2845877964562161244, -0.3641732283464567121 ) ) ;
#53755=CARTESIAN_POINT ( 'NONE',  ( -1.013613127888308485, -2.191421614605370878E-15, 0.4445507791589071167 ) ) ;
#53756=CARTESIAN_POINT ( 'NONE',  ( 0.3937007874015754361, -0.1870078740157479769, 0.4822834645669291653 ) ) ;
#53758=CARTESIAN_POINT ( 'NONE',  ( 1.535433070866142335, -0.6692913385826771977, 8.415575281601705876E-17 ) ) ;
#53759=CARTESIAN_POINT ( 'NONE',  ( -0.2821522309711278487, 0.1771653543307087630, 0.09757992244046791164 ) ) ;
#53760=CARTESIAN_POINT ( 'NONE',  ( -0.1312335958005241554, 0.2306618581243848609, 0.2411417322834645549 ) ) ;
#53761=CARTESIAN_POINT ( 'NONE',  ( -1.496062992125983815, -0.1870078740157479769, 0.4822834645669291653 ) ) ;
#53762=CARTESIAN_POINT ( 'NONE',  ( 1.535433070866142558, 0.2952755905511811885, 0.000000000000000000 ) ) ;
#53763=CARTESIAN_POINT ( 'NONE',  ( 1.384514435695538559, 0.2952755905511810774, -0.1292274648535930714 ) ) ;
#53764=CARTESIAN_POINT ( 'NONE',  ( -0.8333333333333323711, -0.5511811023622048555, -0.09757992244046775898 ) ) ;
#53769=CARTESIAN_POINT ( 'NONE',  ( 0.9645669291338588858, 0.07958543189024085140, 0.2665933059059887866 ) ) ;
#53770=CARTESIAN_POINT ( 'NONE',  ( -1.633858267716534529, -0.5400638737290845981, -0.3530559997133363437 ) ) ;
#53772=CARTESIAN_POINT ( 'NONE',  ( 0.8792650918635177559, -0.4281496062992127816, -0.4176697321401328100 ) ) ;
#53774=CARTESIAN_POINT ( 'NONE',  ( 1.095800524934383846, -0.08942795157528024563, -0.3641732283464568787 ) ) ;
#53775=CARTESIAN_POINT ( 'NONE',  ( 8.195543980992789655E-16, -0.1870078740157480879, -0.4822834645669291653 ) ) ;
#53776=CARTESIAN_POINT ( 'NONE',  ( -0.5971128608923877978, -0.6692913385826773087, -0.1292274648535924053 ) ) ;
#53777=CARTESIAN_POINT ( 'NONE',  ( 1.640419947506562393, -0.4281496062992124485, 0.4176697321401328655 ) ) ;
#53779=CARTESIAN_POINT ( 'NONE',  ( 0.2230971128608929543, -0.004921259842519870586, -0.3153832671262229437 ) ) ;
#53784=CARTESIAN_POINT ( 'NONE',  ( -0.5774278215223089816, 0.2306618581243847221, -0.2411417322834647770 ) ) ;
#53785=CARTESIAN_POINT ( 'NONE',  ( 1.207349081364829990, -0.6046776061558809534, -0.2411417322834644161 ) ) ;
#53786=CARTESIAN_POINT ( 'NONE',  ( 0.2887139107611556010, 0.2306618581243847221, -0.2411417322834647770 ) ) ;
#53787=CARTESIAN_POINT ( 'NONE',  ( -0.3608923884514428360, 0.1771653543307087630, 0.09757992244046791164 ) ) ;
#53788=CARTESIAN_POINT ( 'NONE',  ( 0.9317585301837276734, 0.05413385826771626580, -0.4176697321401330321 ) ) ;
#53789=EDGE_CURVE ( 'NONE', #26484, #6163, #56486, .T. ) ;
#53790=CARTESIAN_POINT ( 'NONE',  ( -0.7152230971128602510, -0.3162353388693405765, 0.4822834645669290543 ) ) ;
#53791=CARTESIAN_POINT ( 'NONE',  ( -0.3346456692913377662, -0.5400638737290844871, 0.3530559997133364547 ) ) ;
#53792=CARTESIAN_POINT ( 'NONE',  ( -0.8923884514435688198, 0.2306618581243847221, -0.2411417322834647770 ) ) ;
#53793=CARTESIAN_POINT ( 'NONE',  ( 1.312335958005249825, 0.2306618581243847221, -0.2411417322834647770 ) ) ;
#53794=CARTESIAN_POINT ( 'NONE',  ( 0.7414698162729663755, -0.6692913385826773087, -0.1292274648535924053 ) ) ;
#53795=CARTESIAN_POINT ( 'NONE',  ( 0.9448818897637802916, -0.1870078740157480879, -0.4822834645669291653 ) ) ;
#53797=CARTESIAN_POINT ( 'NONE',  ( 0.1771653543307093182, -0.4536011799217368745, -0.2665933059059886201 ) ) ;
#53800=ORIENTED_EDGE ( 'NONE', *, *, #35952, .F. ) ;
#53801=CARTESIAN_POINT ( 'NONE',  ( -0.8202099737532801971, -0.5511811023622046335, 0.09757992244046803654 ) ) ;
#53802=CARTESIAN_POINT ( 'NONE',  ( 0.01968503937007957949, -0.5400638737290845981, -0.3530559997133363437 ) ) ;
#53804=CARTESIAN_POINT ( 'NONE',  ( -0.2559055118110230564, 0.1660481256975883668, -0.3530559997133364547 ) ) ;
#53805=CARTESIAN_POINT ( 'NONE',  ( -0.2559055118110230564, 0.1660481256975883668, -0.3530559997133364547 ) ) ;
#53806=CARTESIAN_POINT ( 'NONE',  ( -1.122047244094487306, 0.1660481256975883668, -0.3530559997133364547 ) ) ;
#53807=CARTESIAN_POINT ( 'NONE',  ( -1.292650918635170010, -0.6692913385826771977, 0.1292274648535927661 ) ) ;
#53808=CARTESIAN_POINT ( 'NONE',  ( 1.246719160104987623, -0.004921259842519870586, -0.3153832671262229437 ) ) ;
#53811=CARTESIAN_POINT ( 'NONE',  ( 0.5183727034120741983, 0.1771653543307087075, -0.09757992244046823083 ) ) ;
#53812=CARTESIAN_POINT ( 'NONE',  ( 0.1968503937007881344, -0.6692913385826771977, 8.415575281601705876E-17 ) ) ;
#53813=CARTESIAN_POINT ( 'NONE',  ( 0.5511811023622055217, -0.1870078740157479769, 0.4822834645669291653 ) ) ;
#53817=ORIENTED_EDGE ( 'NONE', *, *, #1563, .F. ) ;
#53820=CARTESIAN_POINT ( 'NONE',  ( -0.6824146981627291497, -0.6046776061558809534, -0.2411417322834644161 ) ) ;
#53824=CARTESIAN_POINT ( 'NONE',  ( -1.515748031496062076, -0.4536011799217367080, 0.2665933059059888421 ) ) ;
#53825=CARTESIAN_POINT ( 'NONE',  ( 0.8005249343832027131, 0.05413385826771666132, 0.4176697321401328100 ) ) ;
#53826=CARTESIAN_POINT ( 'NONE',  ( 0.7480314960629927956, 0.2952755905511811885, 0.000000000000000000 ) ) ;
#53827=CARTESIAN_POINT ( 'NONE',  ( -0.03280839895013062252, 0.1771653543307087075, -0.09757992244046823083 ) ) ;
#53828=CARTESIAN_POINT ( 'NONE',  ( 0.2493438320209980519, -0.4281496062992127816, -0.4176697321401328100 ) ) ;
#53830=CARTESIAN_POINT ( 'NONE',  ( 0.08530183727034192087, -0.08942795157527998196, 0.3641732283464567121 ) ) ;
#53831=CARTESIAN_POINT ( 'NONE',  ( -0.4986876640419942164, -0.6046776061558807314, 0.2411417322834647770 ) ) ;
#53833=CARTESIAN_POINT ( 'NONE',  ( -1.443569553805773564, -0.6046776061558807314, 0.2411417322834647770 ) ) ;
#53834=CARTESIAN_POINT ( 'NONE',  ( 0.2493438320209980519, -0.3690944881889765550, -0.3153832671262227771 ) ) ;
#53835=CARTESIAN_POINT ( 'NONE',  ( -0.7137454485294953965, 2.001539355558159983, -0.4917280318828584074 ) ) ;
#53836=CARTESIAN_POINT ( 'NONE',  ( -1.135170603674539924, -0.6692913385826771977, 0.1292274648535927661 ) ) ;
#53837=CONICAL_SURFACE ( 'NONE', #12216, 1.181102362204724310, 0.7853981633974621568 ) ;
#53838=CARTESIAN_POINT ( 'NONE',  ( -0.6036745406824141069, -0.5023911411419708095, -0.1820866141732282451 ) ) ;
#53840=CARTESIAN_POINT ( 'NONE',  ( -1.279527559055116948, -0.5400638737290844871, 0.3530559997133364547 ) ) ;
#53841=CARTESIAN_POINT ( 'NONE',  ( -0.5183727034120726440, 0.2952755905511811885, 0.1292274648535926551 ) ) ;
#53842=CARTESIAN_POINT ( 'NONE',  ( 0.08530183727034192087, -0.05778040916215522460, 0.4822834645669289988 ) ) ;
#53846=CARTESIAN_POINT ( 'NONE',  ( 0.4265091863517067594, 0.1771653543307087630, 0.09757992244046791164 ) ) ;
#53847=CARTESIAN_POINT ( 'NONE',  ( 1.128608923884514947, 0.2306618581243848609, 0.2411417322834645549 ) ) ;
#53848=CARTESIAN_POINT ( 'NONE',  ( -1.305774278215222184, -0.5511811023622048555, -0.09757992244046775898 ) ) ;
#53849=CARTESIAN_POINT ( 'NONE',  ( 1.259842519685040019, -0.1870078740157480879, -0.4822834645669291653 ) ) ;
#53850=CARTESIAN_POINT ( 'NONE',  ( -1.489501312335957062, -0.2845877964562161244, -0.3641732283464567121 ) ) ;
#53851=CARTESIAN_POINT ( 'NONE',  ( -0.3871391076115479057, -0.3162353388693409650, -0.4822834645669289433 ) ) ;
#53852=CARTESIAN_POINT ( 'NONE',  ( 0.1312335958005257930, 0.1283753931104746893, -0.1820866141732285504 ) ) ;
#53853=CARTESIAN_POINT ( 'NONE',  ( 1.473278426072734293, 0.2335363939278407575, -0.2780995266831703394 ) ) ;
#53854=CARTESIAN_POINT ( 'NONE',  ( 0.5774278215223103139, -0.5023911411419708095, -0.1820866141732282451 ) ) ;
#53856=CARTESIAN_POINT ( 'NONE',  ( 0.2755905511811031494, 0.2952755905511811885, 0.000000000000000000 ) ) ;
#53858=CARTESIAN_POINT ( 'NONE',  ( -0.7217847769028863381, 0.05413385826771626580, -0.4176697321401330321 ) ) ;
#53860=CARTESIAN_POINT ( 'NONE',  ( 1.194225721784777594, -0.3690944881889765550, -0.3153832671262227771 ) ) ;
#53861=CARTESIAN_POINT ( 'NONE',  ( 0.04593175853018440641, -0.6692913385826771977, 0.1292274648535927661 ) ) ;
#53862=CARTESIAN_POINT ( 'NONE',  ( -0.4790026246719152336, -0.05778040916215560624, -0.4822834645669293319 ) ) ;
#53863=CARTESIAN_POINT ( 'NONE',  ( -0.4921259842519677963, 0.07958543189024071263, -0.2665933059059888421 ) ) ;
#53865=CARTESIAN_POINT ( 'NONE',  ( -0.4265091863517051496, -0.5511811023622046335, 0.09757992244046803654 ) ) ;
#53866=CARTESIAN_POINT ( 'NONE',  ( 0.3608923884514443348, -0.6692913385826771977, 0.1292274648535927661 ) ) ;
#53867=CARTESIAN_POINT ( 'NONE',  ( -0.8464566929133852113, -0.4536011799217368745, -0.2665933059059886201 ) ) ;
#53869=CARTESIAN_POINT ( 'NONE',  ( -1.062992125984250968, -0.6692913385826771977, 8.415575281601705876E-17 ) ) ;
#53872=CARTESIAN_POINT ( 'NONE',  ( -0.9645669291338575535, -0.4536011799217367080, 0.2665933059059888421 ) ) ;
#53873=CARTESIAN_POINT ( 'NONE',  ( 0.1049868766404206816, -0.6046776061558809534, -0.2411417322834644161 ) ) ;
#53875=CARTESIAN_POINT ( 'NONE',  ( -0.6889763779527552368, 0.1660481256975885056, 0.3530559997133364547 ) ) ;
#53877=CARTESIAN_POINT ( 'NONE',  ( 1.187664041994751285, -0.05778040916215522460, 0.4822834645669289988 ) ) ;
#53878=CARTESIAN_POINT ( 'NONE',  ( 0.7545931758530189937, 0.2952755905511810774, -0.1292274648535930714 ) ) ;
#53882=CARTESIAN_POINT ( 'NONE',  ( -1.640419947506561060, -0.4281496062992127816, -0.4176697321401328100 ) ) ;
#53886=CARTESIAN_POINT ( 'NONE',  ( -0.5183727034120726440, 0.1771653543307087630, 0.09757992244046791164 ) ) ;
#53888=VERTEX_POINT ( 'NONE', #12589 ) ;
#53889=CARTESIAN_POINT ( 'NONE',  ( 0.8661417322834652488, -0.1870078740157480879, -0.4822834645669291653 ) ) ;
#53890=CARTESIAN_POINT ( 'NONE',  ( 0.1640419947506569498, -0.05778040916215522460, 0.4822834645669289988 ) ) ;
#53891=CARTESIAN_POINT ( 'NONE',  ( -0.5511811023622038563, -0.1870078740157479769, 0.4822834645669291653 ) ) ;
#53892=CARTESIAN_POINT ( 'NONE',  ( 1.660104986876641320, -0.05778040916215522460, 0.4822834645669289988 ) ) ;
#53893=CARTESIAN_POINT ( 'NONE',  ( -0.9120734908136475250, -0.5511811023622048555, -0.09757992244046775898 ) ) ;
#53895=CARTESIAN_POINT ( 'NONE',  ( 0.3871391076115493490, -0.3162353388693405765, 0.4822834645669290543 ) ) ;
#53896=CARTESIAN_POINT ( 'NONE',  ( 0.4658792650918640033, -0.2845877964562159024, 0.3641732283464567677 ) ) ;
#53898=CARTESIAN_POINT ( 'NONE',  ( -0.6561679790026240244, 0.2306618581243847221, -0.2411417322834647770 ) ) ;
#53900=CARTESIAN_POINT ( 'NONE',  ( -1.076115485564303809, -0.6046776061558809534, -0.2411417322834644161 ) ) ;
#53902=CARTESIAN_POINT ( 'NONE',  ( 0.9120734908136490793, 0.2952755905511810774, -0.1292274648535930714 ) ) ;
#53903=CARTESIAN_POINT ( 'NONE',  ( 1.108923884514436686, -0.2845877964562161244, -0.3641732283464567121 ) ) ;
#53906=CARTESIAN_POINT ( 'NONE',  ( -0.5249343832020990641, 0.2306618581243848609, 0.2411417322834645549 ) ) ;
#53907=ORIENTED_EDGE ( 'NONE', *, *, #17436, .F. ) ;
#53908=CARTESIAN_POINT ( 'NONE',  ( 0.4986876640419954376, 0.1283753931104748280, 0.1820866141732283561 ) ) ;
#53909=CARTESIAN_POINT ( 'NONE',  ( -0.9973753280839886548, -0.6046776061558809534, -0.2411417322834644161 ) ) ;
#53910=CARTESIAN_POINT ( 'NONE',  ( 0.8136482939632553313, 0.2306618581243848609, 0.2411417322834645549 ) ) ;
#53911=CARTESIAN_POINT ( 'NONE',  ( 0.8136482939632553313, 0.2306618581243848609, 0.2411417322834645549 ) ) ;
#53912=CARTESIAN_POINT ( 'NONE',  ( 5.463695987328526437E-16, -0.1870078740157479769, 0.4822834645669291653 ) ) ;
#53913=B_SPLINE_CURVE_WITH_KNOTS ( 'NONE', 3,
 ( #4268, #5094, #81305, #23619 ),
 .UNSPECIFIED., .F., .F.,
 ( 4, 4 ),
 ( 3.593986969189856268E-07, 0.001287825409103295115 ),
 .UNSPECIFIED. ) ;
#53914=CARTESIAN_POINT ( 'NONE',  ( -0.2165354330708654795, 0.1660481256975885056, 0.3530559997133364547 ) ) ;
#53916=CARTESIAN_POINT ( 'NONE',  ( -1.489501312335957062, -0.3162353388693409650, -0.4822834645669289433 ) ) ;
#53917=CARTESIAN_POINT ( 'NONE',  ( -0.4724409448818890911, -0.1870078740157480879, -0.4822834645669291653 ) ) ;
#53918=CARTESIAN_POINT ( 'NONE',  ( -0.4527559055118102749, -0.4536011799217368745, -0.2665933059059886201 ) ) ;
#53919=CARTESIAN_POINT ( 'NONE',  ( 1.325459317585302665, -0.4281496062992124485, 0.4176697321401328655 ) ) ;
#53920=VECTOR ( 'NONE', #21141, 39.37007874015748143 ) ;
#53921=CARTESIAN_POINT ( 'NONE',  ( 1.496062992125985147, -0.1870078740157479769, 0.4822834645669291653 ) ) ;
#53922=CARTESIAN_POINT ( 'NONE',  ( -0.7349081364829390672, 0.2306618581243847221, -0.2411417322834647770 ) ) ;
#53924=CARTESIAN_POINT ( 'NONE',  ( 0.6102362204724416372, -0.5400638737290844871, 0.3530559997133364547 ) ) ;
#53927=CARTESIAN_POINT ( 'NONE',  ( -0.1771653543307080136, 0.1660481256975883668, -0.3530559997133364547 ) ) ;
#53928=CARTESIAN_POINT ( 'NONE',  ( -1.148293963254592542, 0.1771653543307087630, 0.09757992244046791164 ) ) ;
#53929=CARTESIAN_POINT ( 'NONE',  ( 1.089238845144357759, -0.004921259842519870586, -0.3153832671262229437 ) ) ;
#53932=CARTESIAN_POINT ( 'NONE',  ( 1.377952755905512472, 0.1771653543307087630, 0.000000000000000000 ) ) ;
#53933=CARTESIAN_POINT ( 'NONE',  ( 0.6889763779527563470, 0.1660481256975883668, -0.3530559997133364547 ) ) ;
#53935=CARTESIAN_POINT ( 'NONE',  ( -0.2165354330708654795, -0.5400638737290845981, -0.3530559997133363437 ) ) ;
#53936=CARTESIAN_POINT ( 'NONE',  ( 0.01000891935578606708, -2.191421614605370878E-15, 0.4445507791589071167 ) ) ;
#53937=CARTESIAN_POINT ( 'NONE',  ( 1.194225721784777594, -0.3690944881889765550, -0.3153832671262227771 ) ) ;
#53938=CARTESIAN_POINT ( 'NONE',  ( -0.006561679790025524116, -0.3162353388693405765, 0.4822834645669290543 ) ) ;
#53940=CARTESIAN_POINT ( 'NONE',  ( 1.312335958005250269, -0.6046776061558807314, 0.2411417322834647770 ) ) ;
#53941=CARTESIAN_POINT ( 'NONE',  ( -0.07217847769028813698, -0.3162353388693409650, -0.4822834645669289433 ) ) ;
#53942=CARTESIAN_POINT ( 'NONE',  ( 0.7020997375328090762, -0.2845877964562159024, 0.3641732283464567677 ) ) ;
#53944=CARTESIAN_POINT ( 'NONE',  ( 0.5839895013123367340, 0.1771653543307087630, 0.09757992244046791164 ) ) ;
#53947=CARTESIAN_POINT ( 'NONE',  ( 0.9055118110236227702, 0.2952755905511811885, 0.000000000000000000 ) ) ;
#53949=CARTESIAN_POINT ( 'NONE',  ( 1.692913385826772421, 0.1771653543307087630, 0.000000000000000000 ) ) ;
#53951=CARTESIAN_POINT ( 'NONE',  ( -0.03280839895013062252, -0.5511811023622046335, 0.09757992244046803654 ) ) ;
#53952=CARTESIAN_POINT ( 'NONE',  ( 0.2624671916010504757, 0.2306618581243848609, 0.2411417322834645549 ) ) ;
#53953=CARTESIAN_POINT ( 'NONE',  ( 1.594488188976378673, -0.4536011799217368745, -0.2665933059059886201 ) ) ;
#53954=CARTESIAN_POINT ( 'NONE',  ( -1.522309711286088607, 0.1283753931104746893, -0.1820866141732285504 ) ) ;
#53955=CARTESIAN_POINT ( 'NONE',  ( -1.476377952755905110, -0.5400638737290845981, -0.3530559997133363437 ) ) ;
#53957=CARTESIAN_POINT ( 'NONE',  ( 0.4855643044619430415, -0.4281496062992127816, -0.4176697321401328100 ) ) ;
#53958=CARTESIAN_POINT ( 'NONE',  ( 1.502624671916010790, -0.05778040916215522460, 0.4822834645669289988 ) ) ;
#53959=CARTESIAN_POINT ( 'NONE',  ( 1.614173228346457378, 0.7794589730111999293, 0.1372047244094478369 ) ) ;
#53960=CARTESIAN_POINT ( 'NONE',  ( 0.3740157480314966754, 0.1660481256975883668, -0.3530559997133364547 ) ) ;
#53963=CARTESIAN_POINT ( 'NONE',  ( 0.8989501312335964611, 0.2952755905511811885, 0.1292274648535926551 ) ) ;
#53964=CARTESIAN_POINT ( 'NONE',  ( -1.614173228346456268, -0.5511811023622047445, 6.969142054262312111E-17 ) ) ;
#53965=CARTESIAN_POINT ( 'NONE',  ( 1.305774278215223960, -0.5511811023622046335, 0.09757992244046803654 ) ) ;
#53966=CARTESIAN_POINT ( 'NONE',  ( 1.660104986876641320, -0.05778040916215522460, 0.4822834645669289988 ) ) ;
#53967=CARTESIAN_POINT ( 'NONE',  ( -0.6561679790026240244, 0.1283753931104746893, -0.1820866141732285504 ) ) ;
#53969=CARTESIAN_POINT ( 'NONE',  ( 0.4986876640419954376, 0.1283753931104748280, 0.1820866141732283561 ) ) ;
#53970=CARTESIAN_POINT ( 'NONE',  ( 0.02624671916010564918, -0.6046776061558809534, -0.2411417322834644161 ) ) ;
#53971=CARTESIAN_POINT ( 'NONE',  ( 0.8858267716535438430, -0.5400638737290845981, -0.3530559997133363437 ) ) ;
#53972=CARTESIAN_POINT ( 'NONE',  ( -0.3805774278215216522, 0.05413385826771666132, 0.4176697321401328100 ) ) ;
#53973=CARTESIAN_POINT ( 'NONE',  ( 0.2099737532808405305, 0.1283753931104746893, -0.1820866141732285504 ) ) ;
#53974=CARTESIAN_POINT ( 'NONE',  ( 1.391076115485564868, -0.6046776061558807314, 0.2411417322834647770 ) ) ;
#53977=CARTESIAN_POINT ( 'NONE',  ( -0.8267716535433065062, -0.6692913385826771977, 8.415575281601705876E-17 ) ) ;
#53981=CARTESIAN_POINT ( 'NONE',  ( -0.9711286089238838626, 0.2306618581243847221, -0.2411417322834647770 ) ) ;
#53982=CARTESIAN_POINT ( 'NONE',  ( 0.07874015748031558404, -0.1870078740157480879, -0.4822834645669291653 ) ) ;
#53986=CARTESIAN_POINT ( 'NONE',  ( 0.7349081364829403995, 0.1283753931104748280, 0.1820866141732283561 ) ) ;
#53989=CARTESIAN_POINT ( 'NONE',  ( 1.056430446194226436, -0.6692913385826773087, -0.1292274648535924053 ) ) ;
#53991=CARTESIAN_POINT ( 'NONE',  ( -1.397637795275589623, 0.07958543189024085140, 0.2665933059059887866 ) ) ;
#53992=CARTESIAN_POINT ( 'NONE',  ( 1.482939632545932307, -0.4281496062992124485, 0.4176697321401328655 ) ) ;
#53993=CARTESIAN_POINT ( 'NONE',  ( -1.476377952755905110, -0.5400638737290845981, -0.3530559997133363437 ) ) ;
#53995=CARTESIAN_POINT ( 'NONE',  ( 0.1181102362204730916, 0.2952755905511811885, 0.000000000000000000 ) ) ;
#53996=CARTESIAN_POINT ( 'NONE',  ( -0.5118110236220466680, -0.5511811023622047445, 6.969142054262312111E-17 ) ) ;
#53997=CARTESIAN_POINT ( 'NONE',  ( 0.9580052493438326877, 0.05413385826771666132, 0.4176697321401328100 ) ) ;
#53998=CARTESIAN_POINT ( 'NONE',  ( 0.1246719160104994284, -0.6692913385826771977, 0.1292274648535927661 ) ) ;
#53999=CARTESIAN_POINT ( 'NONE',  ( -1.586052503253847501, 1.299212598425198095, 0.1653254495020568260 ) ) ;
#54002=CARTESIAN_POINT ( 'NONE',  ( 0.8136482939632553313, -0.6046776061558809534, -0.2411417322834644161 ) ) ;
#54003=CARTESIAN_POINT ( 'NONE',  ( 0.03937007874015806264, 0.2952755905511811885, 0.000000000000000000 ) ) ;
#54004=CARTESIAN_POINT ( 'NONE',  ( -0.9645669291338575535, 0.1660481256975883668, -0.3530559997133364547 ) ) ;
#54005=CARTESIAN_POINT ( 'NONE',  ( 0.8989501312335963501, -0.6692913385826773087, -0.1292274648535924053 ) ) ;
#54006=CARTESIAN_POINT ( 'NONE',  ( 0.8464566929133866546, -0.5400638737290844871, 0.3530559997133364547 ) ) ;
#54008=CARTESIAN_POINT ( 'NONE',  ( -0.2952755905511804668, 0.1660481256975885056, 0.3530559997133364547 ) ) ;
#54009=CARTESIAN_POINT ( 'NONE',  ( 0.6824146981627303710, -0.6046776061558807314, 0.2411417322834647770 ) ) ;
#54010=CARTESIAN_POINT ( 'NONE',  ( -0.1574803149606292529, -0.1870078740157480879, -0.4822834645669291653 ) ) ;
#54011=CARTESIAN_POINT ( 'NONE',  ( 0.5249343832021005074, -0.5023911411419708095, 0.1820866141732285504 ) ) ;
#54012=CARTESIAN_POINT ( 'NONE',  ( -1.154855643044618851, -0.6046776061558809534, -0.2411417322834644161 ) ) ;
#54013=CARTESIAN_POINT ( 'NONE',  ( -0.4061203303035118561, -2.613618158232546091E-15, -0.3464511005275220379 ) ) ;
#54014=CARTESIAN_POINT ( 'NONE',  ( 0.9317585301837276734, -0.4281496062992124485, 0.4176697321401328655 ) ) ;
#54015=VECTOR ( 'NONE', #30376, 39.37007874015748143 ) ;
#54018=ORIENTED_EDGE ( 'NONE', *, *, #66351, .F. ) ;
#54020=CARTESIAN_POINT ( 'NONE',  ( 1.305774278215223960, -0.6692913385826771977, 0.1292274648535927661 ) ) ;
#54021=CARTESIAN_POINT ( 'NONE',  ( 0.7152230971128614723, -0.2845877964562161244, -0.3641732283464567121 ) ) ;
#54023=PLANE ( 'NONE',  #31586 ) ;
#54027=CARTESIAN_POINT ( 'NONE',  ( -0.6627296587926501115, 0.2952755905511810774, -0.1292274648535930714 ) ) ;
#54028=CARTESIAN_POINT ( 'NONE',  ( -0.6167979002624665030, 0.05413385826771666132, 0.4176697321401328100 ) ) ;
#54029=CARTESIAN_POINT ( 'NONE',  ( 1.200787401574803681, -0.5400638737290845981, -0.3530559997133363437 ) ) ;
#54031=CARTESIAN_POINT ( 'NONE',  ( -1.620734908136482577, -0.6692913385826773087, -0.1292274648535924053 ) ) ;
#54033=CARTESIAN_POINT ( 'NONE',  ( 1.646981627296588035, -0.2845877964562159024, 0.3641732283464567677 ) ) ;
#54034=DIRECTION ( 'NONE',  ( 0.000000000000000000, 0.000000000000000000, -1.000000000000000000 ) ) ;
#54035=CARTESIAN_POINT ( 'NONE',  ( -1.167979002624671470, -0.004921259842519576551, 0.3153832671262227771 ) ) ;
#54037=CARTESIAN_POINT ( 'NONE',  ( 0.3477690288713918276, -0.6692913385826773087, -0.1292274648535924053 ) ) ;
#54038=CARTESIAN_POINT ( 'NONE',  ( 1.377952755905512472, 0.2952755905511811885, 0.000000000000000000 ) ) ;
#54039=CARTESIAN_POINT ( 'NONE',  ( 0.6399301791983058596, -1.374501131054255944E-15, 0.4445507791589066726 ) ) ;
#54040=CARTESIAN_POINT ( 'NONE',  ( -0.8136482939632537770, -0.5023911411419708095, 0.1820866141732285504 ) ) ;
#54041=CARTESIAN_POINT ( 'NONE',  ( 0.6102362204724416372, 0.1660481256975883668, -0.3530559997133364547 ) ) ;
#54042=CARTESIAN_POINT ( 'NONE',  ( 1.391076115485564868, -0.5023911411419708095, 0.1820866141732285504 ) ) ;
#54044=CARTESIAN_POINT ( 'NONE',  ( -0.8136482939632537770, -0.5023911411419708095, 0.1820866141732285504 ) ) ;
#54045=CARTESIAN_POINT ( 'NONE',  ( 1.174540682414699111, -0.3162353388693405765, 0.4822834645669290543 ) ) ;
#54047=CARTESIAN_POINT ( 'NONE',  ( -0.02624671916010428221, -0.6046776061558807314, 0.2411417322834647770 ) ) ;
#54048=CARTESIAN_POINT ( 'NONE',  ( -0.7480314960629914633, -0.5511811023622047445, 6.969142054262312111E-17 ) ) ;
#54049=CARTESIAN_POINT ( 'NONE',  ( -0.3412073490813641308, -0.5023911411419708095, 0.1820866141732285504 ) ) ;
#54050=CARTESIAN_POINT ( 'NONE',  ( -0.2821522309711278487, 0.2952755905511811885, 0.1292274648535926551 ) ) ;
#54051=CARTESIAN_POINT ( 'NONE',  ( -1.502624671916009680, -0.2845877964562159024, 0.3641732283464567677 ) ) ;
#54053=CARTESIAN_POINT ( 'NONE',  ( 0.4396325459317590445, -0.6692913385826771977, 0.1292274648535927661 ) ) ;
#54056=CARTESIAN_POINT ( 'NONE',  ( -0.7020997375328076329, -0.3162353388693409650, -0.4822834645669289433 ) ) ;
#54057=CARTESIAN_POINT ( 'NONE',  ( -0.1312335958005241554, 0.1283753931104748280, 0.1820866141732283561 ) ) ;
#54058=CARTESIAN_POINT ( 'NONE',  ( -1.522309711286088607, -0.6046776061558807314, 0.2411417322834647770 ) ) ;
#54059=CARTESIAN_POINT ( 'NONE',  ( -0.09842519685039295696, -0.5400638737290844871, 0.3530559997133364547 ) ) ;
#54060=CARTESIAN_POINT ( 'NONE',  ( 0.2821522309711292364, 0.1771653543307087075, -0.09757992244046823083 ) ) ;
#54061=CARTESIAN_POINT ( 'NONE',  ( -0.7808398950131225646, -0.08942795157527998196, 0.3641732283464567121 ) ) ;
#54062=CARTESIAN_POINT ( 'NONE',  ( -1.213910761154854745, 0.2952755905511810774, -0.1292274648535930714 ) ) ;
#54063=CARTESIAN_POINT ( 'NONE',  ( 1.601049868766404982, 0.1283753931104748280, 0.1820866141732283561 ) ) ;
#54064=CARTESIAN_POINT ( 'NONE',  ( 1.187664041994751285, -0.05778040916215522460, 0.4822834645669289988 ) ) ;
#54066=CARTESIAN_POINT ( 'NONE',  ( 0.7283464566929143125, 0.07958543189024085140, 0.2665933059059887866 ) ) ;
#54068=CARTESIAN_POINT ( 'NONE',  ( 0.7152230971128616943, -0.05778040916215522460, 0.4822834645669289988 ) ) ;
#54070=CARTESIAN_POINT ( 'NONE',  ( 1.371391076115485719, -0.5511811023622048555, -0.09757992244046775898 ) ) ;
#54071=AXIS2_PLACEMENT_3D ( 'NONE', #30101, #68826, #5664 ) ;
#54074=CARTESIAN_POINT ( 'NONE',  ( -1.266404199475064773, -0.08942795157528024563, -0.3641732283464568787 ) ) ;
#54075=CARTESIAN_POINT ( 'NONE',  ( -0.3740157480314953431, 0.1660481256975885056, 0.3530559997133364547 ) ) ;
#54076=CARTESIAN_POINT ( 'NONE',  ( 0.5249343832021003964, 0.2306618581243847221, -0.2411417322834647770 ) ) ;
#54077=CARTESIAN_POINT ( 'NONE',  ( -1.594488188976377563, -0.4536011799217367080, 0.2665933059059888421 ) ) ;
#54079=CARTESIAN_POINT ( 'NONE',  ( -1.522309711286088607, 0.2306618581243847221, -0.2411417322834647770 ) ) ;
#54080=CARTESIAN_POINT ( 'NONE',  ( 0.4396325459317593221, 0.2952755905511810774, -0.1292274648535930714 ) ) ;
#54081=CARTESIAN_POINT ( 'NONE',  ( 0.1771653543307093182, -0.5400638737290845981, -0.3530559997133363437 ) ) ;
#54082=CARTESIAN_POINT ( 'NONE',  ( 1.404199475065617264, -0.4281496062992124485, 0.4176697321401328655 ) ) ;
#54083=CARTESIAN_POINT ( 'NONE',  ( 1.502624671916010790, -0.05778040916215522460, 0.4822834645669289988 ) ) ;
#54087=PLANE ( 'NONE',  #19729 ) ;
#54089=CARTESIAN_POINT ( 'NONE',  ( -0.1640419947506555343, -0.2845877964562159024, 0.3641732283464567677 ) ) ;
#54090=CARTESIAN_POINT ( 'NONE',  ( -0.2165354330708654795, -0.5400638737290845981, -0.3530559997133363437 ) ) ;
#54091=CARTESIAN_POINT ( 'NONE',  ( 0.7152230971128614723, -0.3162353388693409650, -0.4822834645669289433 ) ) ;
#54093=CARTESIAN_POINT ( 'NONE',  ( -0.01312335958005186876, -0.004921259842519870586, -0.3153832671262229437 ) ) ;
#54094=CARTESIAN_POINT ( 'NONE',  ( -0.9776902887139098386, 0.2952755905511810774, -0.1292274648535930714 ) ) ;
#54095=CARTESIAN_POINT ( 'NONE',  ( -1.607611548556429737, 0.2952755905511810774, -0.1292274648535930714 ) ) ;
#54098=VERTEX_POINT ( 'NONE', #67679 ) ;
#54100=CARTESIAN_POINT ( 'NONE',  ( 1.095800524934383846, -0.3162353388693405765, 0.4822834645669290543 ) ) ;
#54101=CARTESIAN_POINT ( 'NONE',  ( -1.633858267716534529, -0.5400638737290845981, -0.3530559997133363437 ) ) ;
#54102=CARTESIAN_POINT ( 'NONE',  ( -1.404199475065615932, -0.3690944881889765550, -0.3153832671262227771 ) ) ;
#54103=CARTESIAN_POINT ( 'NONE',  ( -1.141732283464566011, 0.2952755905511811885, 0.000000000000000000 ) ) ;
#54105=CARTESIAN_POINT ( 'NONE',  ( -1.646051170424378096, 0.000000000000000000, -0.3464511005275205946 ) ) ;
#54106=CARTESIAN_POINT ( 'NONE',  ( 1.220472440944882608, 0.2952755905511811885, 0.000000000000000000 ) ) ;
#54107=CARTESIAN_POINT ( 'NONE',  ( -1.555118110236219930, 0.1660481256975885056, 0.3530559997133364547 ) ) ;
#54108=CARTESIAN_POINT ( 'NONE',  ( 0.09842519685039434474, -0.5400638737290845981, -0.3530559997133363437 ) ) ;
#54109=CARTESIAN_POINT ( 'NONE',  ( -0.09842519685039295696, 0.1660481256975883668, -0.3530559997133364547 ) ) ;
#54111=CARTESIAN_POINT ( 'NONE',  ( -1.404199475065615932, -0.4281496062992127816, -0.4176697321401328100 ) ) ;
#54113=CARTESIAN_POINT ( 'NONE',  ( 0.1312335958005255154, -0.6046776061558807314, 0.2411417322834647770 ) ) ;
#54115=CARTESIAN_POINT ( 'NONE',  ( -1.167979002624671470, -0.004921259842519576551, 0.3153832671262227771 ) ) ;
#54116=ORIENTED_EDGE ( 'NONE', *, *, #44186, .T. ) ;
#54120=DIRECTION ( 'NONE',  ( 0.000000000000000000, 0.000000000000000000, -1.000000000000000000 ) ) ;
#54121=CARTESIAN_POINT ( 'NONE',  ( -1.345144356955379816, -0.05778040916215560624, -0.4822834645669293319 ) ) ;
#54123=CARTESIAN_POINT ( 'NONE',  ( -1.561679790026246017, 0.05413385826771666132, 0.4176697321401328100 ) ) ;
#54124=CARTESIAN_POINT ( 'NONE',  ( -1.725721784776902190, -0.05778040916215522460, 0.4822834645669289988 ) ) ;
#54125=CARTESIAN_POINT ( 'NONE',  ( -0.9776902887139098386, 0.2952755905511810219, -0.1292274648535930437 ) ) ;
#54126=CARTESIAN_POINT ( 'NONE',  ( 1.220472440944882386, -0.1870078740157480046, 1.254653134982923898E-17 ) ) ;
#54128=CARTESIAN_POINT ( 'NONE',  ( -0.1902887139107604098, 0.1771653543307087075, -0.09757992244046823083 ) ) ;
#54129=CARTESIAN_POINT ( 'NONE',  ( -0.8136482939632537770, -0.5023911411419708095, 0.1820866141732285504 ) ) ;
#54130=CARTESIAN_POINT ( 'NONE',  ( -1.023622047244093558, -0.1870078740157479769, 0.4822834645669291653 ) ) ;
#54131=CARTESIAN_POINT ( 'NONE',  ( 0.8661417322834652488, -0.1870078740157480879, -0.4822834645669291653 ) ) ;
#54132=CARTESIAN_POINT ( 'NONE',  ( -0.7939632545931750718, -0.05778040916215560624, -0.4822834645669293319 ) ) ;
#54135=CARTESIAN_POINT ( 'NONE',  ( -1.548556430446193399, -0.6046776061558809534, -0.2411417322834644161 ) ) ;
#54139=FACE_OUTER_BOUND ( 'NONE', #36329, .T. ) ;
#54140=EDGE_CURVE ( 'NONE', #52448, #23493, #66464, .T. ) ;
#54143=CARTESIAN_POINT ( 'NONE',  ( -0.6496062992125976043, 0.1660481256975883668, -0.3530559997133364547 ) ) ;
#54144=CARTESIAN_POINT ( 'NONE',  ( 1.233595800524935227, 0.2306618581243847221, -0.2411417322834647770 ) ) ;
#54146=DIRECTION ( 'NONE',  ( 1.000000000000000000, -0.000000000000000000, -0.000000000000000000 ) ) ;
#54147=CARTESIAN_POINT ( 'NONE',  ( 1.112371124080195450, -4.927456884911482678E-16, 0.4445507791589062840 ) ) ;
#54148=CARTESIAN_POINT ( 'NONE',  ( -1.397637795275589623, 0.1660481256975885056, 0.3530559997133364547 ) ) ;
#54149=CARTESIAN_POINT ( 'NONE',  ( -0.6627296587926503335, -0.6692913385826771977, 0.1292274648535927661 ) ) ;
#54151=CARTESIAN_POINT ( 'NONE',  ( 0.3477690288713918276, 0.1771653543307087630, 0.09757992244046791164 ) ) ;
#54153=CARTESIAN_POINT ( 'NONE',  ( 0.3412073490813655186, -0.5023911411419708095, -0.1820866141732282451 ) ) ;
#54154=CARTESIAN_POINT ( 'NONE',  ( 1.043307086614173818, -0.4536011799217368745, -0.2665933059059886201 ) ) ;
#54155=CARTESIAN_POINT ( 'NONE',  ( 0.9383202099737536495, -0.3162353388693405765, 0.4822834645669290543 ) ) ;
#54156=CARTESIAN_POINT ( 'NONE',  ( -0.4461942257217840213, -0.5023911411419708095, -0.1820866141732282451 ) ) ;
#54158=CARTESIAN_POINT ( 'NONE',  ( -1.082677165354329896, -0.5400638737290845981, -0.3530559997133363437 ) ) ;
#54160=CARTESIAN_POINT ( 'NONE',  ( -1.148293963254592542, 0.1771653543307087630, 0.09757992244046791164 ) ) ;
#54162=CARTESIAN_POINT ( 'NONE',  ( -0.7414698162729651543, -0.5511811023622046335, 0.09757992244046803654 ) ) ;
#54163=CARTESIAN_POINT ( 'NONE',  ( -0.2427821522309703550, -0.3162353388693405765, 0.4822834645669290543 ) ) ;
#54165=CARTESIAN_POINT ( 'NONE',  ( 0.4724409448818904789, -0.1870078740157479769, 0.3641732283464567677 ) ) ;
#54166=CARTESIAN_POINT ( 'NONE',  ( -0.3871391076115479057, -0.2845877964562161244, -0.3641732283464567121 ) ) ;
#54167=CARTESIAN_POINT ( 'NONE',  ( -0.8989501312335946848, -0.6692913385826771977, 0.1292274648535927661 ) ) ;
#54168=CARTESIAN_POINT ( 'NONE',  ( -1.633858267716534529, -0.5400638737290845981, -0.3530559997133363437 ) ) ;
#54169=DIRECTION ( 'NONE',  ( 1.000000000000000000, -0.000000000000000000, -0.000000000000000000 ) ) ;
#54171=CARTESIAN_POINT ( 'NONE',  ( -0.01968503937007793844, 0.1660481256975883668, -0.3530559997133364547 ) ) ;
#54173=DIRECTION ( 'NONE',  ( 1.000000000000000000, 0.000000000000000000, 0.000000000000000000 ) ) ;
#54174=CARTESIAN_POINT ( 'NONE',  ( -0.1049868766404193215, 0.1283753931104746893, -0.1820866141732285504 ) ) ;
#54175=CARTESIAN_POINT ( 'NONE',  ( -0.01312335958005186876, -0.4281496062992124485, 0.4176697321401328655 ) ) ;
#54176=CARTESIAN_POINT ( 'NONE',  ( -1.555118110236219930, -0.5400638737290845981, -0.3530559997133363437 ) ) ;
#54177=CARTESIAN_POINT ( 'NONE',  ( 1.614173228346457378, -0.6692913385826771977, 8.415575281601705876E-17 ) ) ;
#54178=CARTESIAN_POINT ( 'NONE',  ( 1.509186351706037543, 0.05413385826771666132, 0.4176697321401328100 ) ) ;
#54179=( BOUNDED_SURFACE ( )  B_SPLINE_SURFACE ( 1, 2, ( 
 ( #67267, #79081, #47053, #9600, #72745, #80322, #22224, #28122, #53777, #73995, #16342, #66434, #8770, #41985, #79489, #34444, #10015, #60111, #2464, #21804, #35680, #78661, #20982, #72337, #14685, #40342, #47468, #73160, #15509, #66023, #34861, #54192, #8359, #2872, #42393, #5344, #81141, #24278, #81963, #30182, #10839, #11257, #44041, #31003, #5745, #16754, #74410, #43209, #68499, #49949, #63410, #37736, #12078, #56671, #10437, #4513, #55844, #50358, #23045, #75647, #74827, #68092, #17171, #81553, #55023, #42805, #80731, #23456, #4105, #17987, #48712, #36915, #49121, #36094, #61765, #69734, #43623, #4933, #18399, #29771, #24690, #55432, #36499, #17576, #62174, #23871, #68905, #49538, #63005, #75233, #62591, #30601, #56267, #69325, #11675, #76055, #37332, #82371, #63821, #39400, #20469, #52011, #57080, #20046, #1120, #76470, #46122, #694, #18797, #65083, #7421, #33091, #71817, #45283, #44441, #64244, #31416, #32250, #26771, #58758, #32665, #19621, #14167, #82775, #25097, #65512, #6579, #50769, #70978, #6998, #39824, #70134, #12485, #77716, #13743, #13323, #38564, #64659, #45698, #52426, #38149, #57911, #58332, #51589, #6160, #31835, #57496, #83187, #25510, #51175, #78136, #76871, #19203, #44852, #70550, #12905, #26350, #275, #71394, #25930, #38976, #77290, #80941, #54831, #61978, #36302, #16970, #8259, #74626, #67894, #48508, #74207, #65922, #49338, #61144, #27185, #3496, #43014, #42609, #22847, #16135, #28748, #4315, #10231, #41781, #61568, #29980, #68310, #52849, #78560, #55643, #75038, #81354, #14586, #54410, #10647, #23666, #35898, #20886, #17384, #33511, #7844, #40239, #59173, #80121, #1531, #46537, #23256, #29161, #72237, #33924, #60732, #80536, #3084, #22439, #48099, #73798, #67474, #9808, #35480, #16554, #42198, #3911, #29572, #55234, #48926, #11468, #37947, #12291, #43831, #24492, #24896, #57710, #19004, #19423, #30394, #4720, #56884, #82176, #63624, #77091, #51386, #25726, #44653, #24079, #18197, #69534, #64039, #36708, #5961, #5143, #56059, #30808, #11884, #68709, #56473, #11050, #37125, #17787, #31631, #62383, #50565, #62809, #81769, #49748, #73, #57291, #18603, #32050, #75449, #38363, #43422, #69119, #31216, #50159, #82989, #75855, #37536, #25310, #6378, #82577, #70349, #50974, #76269, #63212, #5552, #44246, #69935, #76672, #12704, #71196, #13539, #77515, #51810, #19850, #59390, #26989, #46340, #33729, #45499, #39195, #27405, #7651, #8067, #72034, #64878, #7217, #32888, #1748, #1338, #33321, #58557, #21101, #26580, #13966, #45916, #14390, #52233, #40048, #494, #923, #65734, #77936, #53066, #78777, #20266, #71614, #46760, #66138, #39622, #65312, #72453, #58983, #52652, #14802, #78357, #20689, #26149, #40460, #8476, #34145, #59806, #2161, #53487, #27827, #79197, #45075, #70778, #13129, #38780, #64457, #6794, #32465, #58127, #2579, #79611, #47589, #73283, #53898, #28238, #21928, #35801, #3403, #22752, #10137, #15631, #41288, #3816, #67383, #67800, #48412, #66973, #9306, #34976, #61468, #61053, #9717, #60640, #80847, #2990, #73704, #22345, #74112, #28656, #16458, #60229, #54315, #42103, #80026, #29477, #55136, #48005, #16044, #23159, #42512, #41690, #35388, #48828, #29066, #54737, #74529, #80442, #16875, #68214, #10551, #36209, #61878, #4219, #29883, #55546, #21513, #47172, #72863, #15212, #40872, #66554, #8887, #34564, #68612, #31536, #23986, #50468, #24800, #56381, #37029, #37444, #70248, #57192, #31952, #42917, #17289, #69438, #11372, #76172, #6276, #63939, #38261, #82894, #36609, #30718, #82080, #76580, #49241, #18509, #17693, #10952, #43321, #24394, #81255, #69021, #23570, #49653, #30296, #44152, #74944, #63118, #75345, #62288, #4625, #12604, #69844, #31118, #44559, #55962, #50880, #81675, #62711, #43734, #5049, #12194, #18101, #25214, #18908, #50064, #11791, #75759, #5456, #56785, #5860, #82485, #37852, #63529, #40356, #77409, #7114, #27303, #65206, #77834, #6695, #65632, #46659, #78255, #83304, #46238, #52962, #19322, #72353, #26886, #44974, #7963, #33625, #59288, #14700, #71512, #70670, #32785, #57613, #58454, #78676, #1645, #58879 ),
 ( #45814, #64775, #7543, #20586, #20997, #38680, #813, #33215, #20164, #25626, #32365, #13026, #76992, #8373, #58027, #66035, #64358, #19744, #39947, #45398, #391, #52546, #51289, #14283, #1237, #39518, #26049, #71934, #13859, #51707, #71095, #13438, #39094, #26476, #52126, #73603, #15945, #8785, #74423, #2889, #53388, #28551, #68105, #67694, #47895, #41184, #53793, #29376, #9614, #66874, #3297, #3713, #16355, #79095, #21414, #80744, #16770, #55037, #40764, #79504, #41999, #10029, #35284, #47067, #23058, #59702, #48726, #66449, #2057, #21820, #27721, #42407, #9204, #34039, #15108, #34458, #60127, #2478, #28137, #47483, #73176, #48311, #41591, #60946, #22652, #15526, #34877, #35694, #79924, #80337, #28961, #60538, #54208, #22240, #74008, #67281, #54626, #61359, #72759, #75247, #62607, #11271, #37347, #17592, #5357, #49138, #36514, #63020, #10853, #18412, #31017, #43223, #68921, #12093, #31431, #42819, #62190, #44055, #36930, #68513, #56685, #55859, #4948, #74842, #82386, #5761, #24703, #57093, #82789, #50783, #23887, #4527, #49552, #61778, #30197, #43636, #76070, #17186, #81155, #69747, #81569, #50372, #37750, #30618, #56281, #49964, #25110, #63424, #44458, #55446, #29784, #81978, #24293, #76484, #18811, #10451, #36107, #4119, #75661, #18002, #69339, #23471, #11689, #13756, #6592, #57511, #32263, #45296, #78572, #57924, #52862, #12920, #19217, #39413, #20898, #52024, #64258, #31848, #83202, #59186, #65096, #20059, #33523, #25524, #39837, #70148, #63836, #32679, #51189, #7434, #76887, #12500, #26783, #65526, #707, #46135, #1133, #77730, #7857, #44865, #70565, #288, #52439, #78150, #45712, #38577, #1544, #38162, #27198, #25944, #6173, #51602, #77305, #19635, #20481, #7011, #71829, #70992, #13336, #58346, #38989, #26364, #64672, #14179, #71409, #33104, #58770, #29281, #66347, #79400, #16255, #54108, #66773, #78991, #54526, #35598, #67184, #72249, #35187, #41902, #8271, #61261, #15850, #33936, #80241, #22557, #48219, #3615, #60438, #59601, #21719, #46551, #47383, #67596, #73915, #47798, #34779, #54945, #14598, #40251, #80651, #73074, #65934, #2789, #22140, #1956, #27618, #53281, #9514, #28864, #28449, #53692, #79824, #60848, #9927, #21311, #15423, #73502, #9106, #46964, #72656, #15006, #40663, #8686, #34356, #60022, #2377, #28034, #41084, #41499, #3200, #17907, #18314, #62925, #56182, #4845, #11996, #11590, #68827, #75974, #50276, #30923, #23375, #5259, #81885, #62507, #30520, #81059, #63327, #75154, #42311, #17499, #56997, #56589, #36834, #30102, #42725, #43956, #24196, #55764, #75566, #69652, #82290, #68009, #10354, #37650, #5665, #31332, #36014, #24609, #49043, #43543, #49866, #81471, #62094, #69242, #22964, #48630, #74325, #61685, #4026, #11174, #36421, #37250, #16672, #29690, #55353, #74740, #17088, #23788, #49459, #68421, #10761, #4436, #43129, #70050, #19120, #57823, #7764, #70466, #65431, #25426, #31752, #51928, #33430, #64574, #76788, #44359, #12405, #71728, #77633, #32583, #46033, #38063, #52345, #82694, #76384, #45193, #63739, #19965, #6078, #25013, #39310, #78052, #13246, #58671, #13657, #6911, #20381, #57414, #190, #14083, #83107, #51091, #44769, #12823, #38480, #64164, #6497, #64998, #58246, #611, #71310, #32167, #25843, #7333, #70896, #45616, #26267, #51503, #77207, #19536, #33001, #38895, #1036, #26690, #39735, #50686, #18717, #59920, #2691, #40568, #54012, #14503, #1858, #28351, #59505, #67083, #79724, #8588, #34259, #60751, #80140, #8173, #27520, #9415, #2275, #33838, #22041, #21212, #66249, #40156, #47701, #54430, #73397, #22462, #48120, #16155, #72561, #53176, #14908, #27103, #78891, #9008, #41401, #65840, #73818, #34680, #27938, #15747, #28768, #35085, #78474, #20798, #41802, #67493, #9829, #46867, #53596, #3103, #59091, #60343, #46454, #1446, #52765, #72147, #79305, #21623, #47283, #72973, #15325, #40990, #66669, #56084, #49769, #29184, #61997, #54852, #4334, #35921, #4743, #11491, #74228, #48946, #37145, #61587, #74647, #24100, #81373, #10667, #16573, #30416, #43442, #43034, #61164, #68730, #75469, #80555, #69140, #75057, #22867 ) ),
 .UNSPECIFIED., .F., .F., .F. ) 
 B_SPLINE_SURFACE_WITH_KNOTS ( ( 2, 2 ),
 ( 3, 2, 2, 2, 2, 2, 2, 2, 2, 2, 2, 2, 2, 2, 2, 2, 2, 2, 2, 2, 2, 2, 2, 2, 2, 2, 2, 2, 2, 2, 2, 2, 2, 2, 2, 2, 2, 2, 2, 2, 2, 2, 2, 2, 2, 2, 2, 2, 2, 2, 2, 2, 2, 2, 2, 2, 2, 2, 2, 2, 2, 2, 2, 2, 2, 2, 2, 2, 2, 2, 2, 2, 2, 2, 2, 2, 2, 2, 2, 2, 2, 2, 2, 2, 2, 2, 2, 2, 2, 2, 2, 2, 2, 2, 2, 2, 2, 2, 2, 2, 2, 2, 2, 2, 2, 2, 2, 2, 2, 2, 2, 2, 2, 2, 2, 2, 2, 2, 2, 2, 2, 2, 2, 2, 2, 2, 2, 2, 2, 2, 2, 2, 2, 2, 2, 2, 2, 2, 2, 2, 2, 2, 2, 2, 2, 2, 2, 2, 2, 2, 2, 2, 2, 2, 2, 2, 2, 2, 2, 2, 2, 2, 2, 2, 2, 2, 2, 2, 2, 2, 2, 2, 2, 2, 2, 2, 2, 2, 2, 2, 2, 2, 2, 2, 2, 2, 2, 2, 2, 2, 2, 2, 2, 2, 2, 2, 2, 2, 2, 2, 2, 2, 2, 2, 2, 2, 2, 2, 2, 2, 2, 2, 2, 2, 2, 2, 2, 2, 2, 2, 2, 2, 2, 2, 2, 2, 2, 2, 2, 2, 2, 2, 2, 2, 2, 2, 2, 2, 2, 2, 2, 2, 2, 2, 2, 2, 2, 2, 2, 2, 2, 2, 2, 2, 2, 3 ),
 ( 0.000000000000000000, 1.000000000000000000 ),
 ( 0.000000000000000000, 0.003787878787878787984, 0.007575757575757575968, 0.01136363636363636395, 0.01515151515151515194, 0.01893939393939393992, 0.02272727272727272790, 0.02651515151515151589, 0.03030303030303030387, 0.03409090909090908839, 0.03787878787878787984, 0.04166666666666666435, 0.04545454545454545581, 0.04924242424242424032, 0.05303030303030303177, 0.05681818181818181629, 0.06060606060606060774, 0.06439393939393939226, 0.06818181818181817677, 0.07196969696969697516, 0.07575757575757575968, 0.07954545454545454419, 0.08333333333333332871, 0.08712121212121212710, 0.09090909090909091161, 0.09469696969696969613, 0.09848484848484848064, 0.1022727272727272790, 0.1060606060606060635, 0.1098484848484848481, 0.1136363636363636326, 0.1174242424242424310, 0.1212121212121212155, 0.1250000000000000000, 0.1287878787878787845, 0.1325757575757575690, 0.1363636363636363535, 0.1401515151515151381, 0.1439393939393939503, 0.1477272727272727348, 0.1515151515151515194, 0.1553030303030303039, 0.1590909090909090884, 0.1628787878787878729, 0.1666666666666666574, 0.1704545454545454419, 0.1742424242424242542, 0.1780303030303030387, 0.1818181818181818232, 0.1856060606060606077, 0.1893939393939393923, 0.1931818181818181768, 0.1969696969696969613, 0.2007575757575757458, 0.2045454545454545581, 0.2083333333333333426, 0.2121212121212121271, 0.2159090909090909116, 0.2196969696969696961, 0.2234848484848484806, 0.2272727272727272652, 0.2310606060606060497, 0.2348484848484848619, 0.2386363636363636465, 0.2424242424242424310, 0.2462121212121212155, 0.2500000000000000000, 0.2537878787878787845, 0.2575757575757575690, 0.2613636363636363535, 0.2651515151515151381, 0.2689393939393939226, 0.2727272727272727071, 0.2765151515151514916, 0.2803030303030302761, 0.2840909090909091161, 0.2878787878787879007, 0.2916666666666666852, 0.2954545454545454697, 0.2992424242424242542, 0.3030303030303030387, 0.3068181818181818232, 0.3106060606060606077, 0.3143939393939393923, 0.3181818181818181768, 0.3219696969696969613, 0.3257575757575757458, 0.3295454545454545303, 0.3333333333333333148, 0.3371212121212120993, 0.3409090909090908839, 0.3446969696969697239, 0.3484848484848485084, 0.3522727272727272929, 0.3560606060606060774, 0.3598484848484848619, 0.3636363636363636465, 0.3674242424242424310, 0.3712121212121212155, 0.3750000000000000000, 0.3787878787878787845, 0.3825757575757575690, 0.3863636363636363535, 0.3901515151515151381, 0.3939393939393939226, 0.3977272727272727071, 0.4015151515151514916, 0.4053030303030302761, 0.4090909090909091161, 0.4128787878787879007, 0.4166666666666666852, 0.4204545454545454697, 0.4242424242424242542, 0.4280303030303030387, 0.4318181818181818232, 0.4356060606060606077, 0.4393939393939393923, 0.4431818181818181768, 0.4469696969696969613, 0.4507575757575757458, 0.4545454545454545303, 0.4583333333333333148, 0.4621212121212120993, 0.4659090909090908839, 0.4696969696969697239, 0.4734848484848485084, 0.4772727272727272929, 0.4810606060606060774, 0.4848484848484848619, 0.4886363636363636465, 0.4924242424242424310, 0.4962121212121212155, 0.5000000000000000000, 0.5037878787878787845, 0.5075757575757575690, 0.5113636363636363535, 0.5151515151515151381, 0.5189393939393939226, 0.5227272727272727071, 0.5265151515151514916, 0.5303030303030302761, 0.5340909090909090606, 0.5378787878787878451, 0.5416666666666666297, 0.5454545454545454142, 0.5492424242424241987, 0.5530303030303029832, 0.5568181818181817677, 0.5606060606060605522, 0.5643939393939394478, 0.5681818181818182323, 0.5719696969696970168, 0.5757575757575758013, 0.5795454545454545858, 0.5833333333333333703, 0.5871212121212121549, 0.5909090909090909394, 0.5946969696969697239, 0.5984848484848485084, 0.6022727272727272929, 0.6060606060606060774, 0.6098484848484848619, 0.6136363636363636465, 0.6174242424242424310, 0.6212121212121212155, 0.6250000000000000000, 0.6287878787878787845, 0.6325757575757575690, 0.6363636363636363535, 0.6401515151515151381, 0.6439393939393939226, 0.6477272727272727071, 0.6515151515151514916, 0.6553030303030302761, 0.6590909090909090606, 0.6628787878787878451, 0.6666666666666666297, 0.6704545454545454142, 0.6742424242424241987, 0.6780303030303029832, 0.6818181818181817677, 0.6856060606060605522, 0.6893939393939394478, 0.6931818181818182323, 0.6969696969696970168, 0.7007575757575758013, 0.7045454545454545858, 0.7083333333333333703, 0.7121212121212121549, 0.7159090909090909394, 0.7196969696969697239, 0.7234848484848485084, 0.7272727272727272929, 0.7310606060606060774, 0.7348484848484848619, 0.7386363636363636465, 0.7424242424242424310, 0.7462121212121212155, 0.7500000000000000000, 0.7537878787878787845, 0.7575757575757575690, 0.7613636363636363535, 0.7651515151515151381, 0.7689393939393939226, 0.7727272727272727071, 0.7765151515151514916, 0.7803030303030302761, 0.7840909090909090606, 0.7878787878787878451, 0.7916666666666666297, 0.7954545454545454142, 0.7992424242424241987, 0.8030303030303029832, 0.8068181818181817677, 0.8106060606060605522, 0.8143939393939394478, 0.8181818181818182323, 0.8219696969696970168, 0.8257575757575758013, 0.8295454545454545858, 0.8333333333333333703, 0.8371212121212121549, 0.8409090909090909394, 0.8446969696969697239, 0.8484848484848485084, 0.8522727272727272929, 0.8560606060606060774, 0.8598484848484848619, 0.8636363636363636465, 0.8674242424242424310, 0.8712121212121212155, 0.8750000000000000000, 0.8787878787878787845, 0.8825757575757575690, 0.8863636363636363535, 0.8901515151515151381, 0.8939393939393939226, 0.8977272727272727071, 0.9015151515151514916, 0.9053030303030302761, 0.9090909090909090606, 0.9128787878787878451, 0.9166666666666666297, 0.9204545454545454142, 0.9242424242424241987, 0.9280303030303029832, 0.9318181818181817677, 0.9356060606060605522, 0.9393939393939394478, 0.9431818181818182323, 0.9469696969696970168, 0.9507575757575758013, 0.9545454545454545858, 0.9583333333333333703, 0.9621212121212121549, 0.9659090909090909394 ),
 .UNSPECIFIED. ) 
 GEOMETRIC_REPRESENTATION_ITEM ( )  RATIONAL_B_SPLINE_SURFACE ( (
 ( 1.000000000000000000, 0.9659258262890683122, 1.000000000000000000, 0.9659258262890683122, 1.000000000000000000, 0.9659258262890683122, 1.000000000000000000, 0.9659258262890683122, 1.000000000000000000, 0.9659258262890683122, 1.000000000000000000, 0.9659258262890683122, 1.000000000000000000, 0.9659258262890683122, 1.000000000000000000, 0.9659258262890683122, 1.000000000000000000, 0.9659258262890683122, 1.000000000000000000, 0.9659258262890683122, 1.000000000000000000, 0.9659258262890683122, 1.000000000000000000, 0.9659258262890683122, 1.000000000000000000, 0.9659258262890683122, 1.000000000000000000, 0.9659258262890683122, 1.000000000000000000, 0.9659258262890683122, 1.000000000000000000, 0.9659258262890683122, 1.000000000000000000, 0.9659258262890683122, 1.000000000000000000, 0.9659258262890683122, 1.000000000000000000, 0.9659258262890683122, 1.000000000000000000, 0.9659258262890683122, 1.000000000000000000, 0.9659258262890683122, 1.000000000000000000, 0.9659258262890683122, 1.000000000000000000, 0.9659258262890683122, 1.000000000000000000, 0.9659258262890683122, 1.000000000000000000, 0.9659258262890683122, 1.000000000000000000, 0.9659258262890683122, 1.000000000000000000, 0.9659258262890683122, 1.000000000000000000, 0.9659258262890683122, 1.000000000000000000, 0.9659258262890683122, 1.000000000000000000, 0.9659258262890683122, 1.000000000000000000, 0.9659258262890683122, 1.000000000000000000, 0.9659258262890683122, 1.000000000000000000, 0.9659258262890683122, 1.000000000000000000, 0.9659258262890683122, 1.000000000000000000, 0.9659258262890683122, 1.000000000000000000, 0.9659258262890683122, 1.000000000000000000, 0.9659258262890683122, 1.000000000000000000, 0.9659258262890683122, 1.000000000000000000, 0.9659258262890683122, 1.000000000000000000, 0.9659258262890683122, 1.000000000000000000, 0.9659258262890683122, 1.000000000000000000, 0.9659258262890683122, 1.000000000000000000, 0.9659258262890683122, 1.000000000000000000, 0.9659258262890683122, 1.000000000000000000, 0.9659258262890683122, 1.000000000000000000, 0.9659258262890683122, 1.000000000000000000, 0.9659258262890683122, 1.000000000000000000, 0.9659258262890683122, 1.000000000000000000, 0.9659258262890683122, 1.000000000000000000, 0.9659258262890683122, 1.000000000000000000, 0.9659258262890683122, 1.000000000000000000, 0.9659258262890683122, 1.000000000000000000, 0.9659258262890683122, 1.000000000000000000, 0.9659258262890683122, 1.000000000000000000, 0.9659258262890683122, 1.000000000000000000, 0.9659258262890683122, 1.000000000000000000, 0.9659258262890683122, 1.000000000000000000, 0.9659258262890683122, 1.000000000000000000, 0.9659258262890683122, 1.000000000000000000, 0.9659258262890683122, 1.000000000000000000, 0.9659258262890683122, 1.000000000000000000, 0.9659258262890683122, 1.000000000000000000, 0.9659258262890683122, 1.000000000000000000, 0.9659258262890683122, 1.000000000000000000, 0.9659258262890683122, 1.000000000000000000, 0.9659258262890683122, 1.000000000000000000, 0.9659258262890683122, 1.000000000000000000, 0.9659258262890683122, 1.000000000000000000, 0.9659258262890683122, 1.000000000000000000, 0.9659258262890683122, 1.000000000000000000, 0.9659258262890683122, 1.000000000000000000, 0.9659258262890683122, 1.000000000000000000, 0.9659258262890683122, 1.000000000000000000, 0.9659258262890683122, 1.000000000000000000, 0.9659258262890683122, 1.000000000000000000, 0.9659258262890683122, 1.000000000000000000, 0.9659258262890683122, 1.000000000000000000, 0.9659258262890683122, 1.000000000000000000, 0.9659258262890683122, 1.000000000000000000, 0.9659258262890683122, 1.000000000000000000, 0.9659258262890683122, 1.000000000000000000, 0.9659258262890683122, 1.000000000000000000, 0.9659258262890683122, 1.000000000000000000, 0.9659258262890683122, 1.000000000000000000, 0.9659258262890683122, 1.000000000000000000, 0.9659258262890683122, 1.000000000000000000, 0.9659258262890683122, 1.000000000000000000, 0.9659258262890683122, 1.000000000000000000, 0.9659258262890683122, 1.000000000000000000, 0.9659258262890683122, 1.000000000000000000, 0.9659258262890683122, 1.000000000000000000, 0.9659258262890683122, 1.000000000000000000, 0.9659258262890683122, 1.000000000000000000, 0.9659258262890683122, 1.000000000000000000, 0.9659258262890683122, 1.000000000000000000, 0.9659258262890683122, 1.000000000000000000, 0.9659258262890683122, 1.000000000000000000, 0.9659258262890683122, 1.000000000000000000, 0.9659258262890683122, 1.000000000000000000, 0.9659258262890683122, 1.000000000000000000, 0.9659258262890683122, 1.000000000000000000, 0.9659258262890683122, 1.000000000000000000, 0.9659258262890683122, 1.000000000000000000, 0.9659258262890683122, 1.000000000000000000, 0.9659258262890683122, 1.000000000000000000, 0.9659258262890683122, 1.000000000000000000, 0.9659258262890683122, 1.000000000000000000, 0.9659258262890683122, 1.000000000000000000, 0.9659258262890683122, 1.000000000000000000, 0.9659258262890683122, 1.000000000000000000, 0.9659258262890683122, 1.000000000000000000, 0.9659258262890683122, 1.000000000000000000, 0.9659258262890683122, 1.000000000000000000, 0.9659258262890683122, 1.000000000000000000, 0.9659258262890683122, 1.000000000000000000, 0.9659258262890683122, 1.000000000000000000, 0.9659258262890683122, 1.000000000000000000, 0.9659258262890683122, 1.000000000000000000, 0.9659258262890683122, 1.000000000000000000, 0.9659258262890683122, 1.000000000000000000, 0.9659258262890683122, 1.000000000000000000, 0.9659258262890683122, 1.000000000000000000, 0.9659258262890683122, 1.000000000000000000, 0.9659258262890683122, 1.000000000000000000, 0.9659258262890683122, 1.000000000000000000, 0.9659258262890683122, 1.000000000000000000, 0.9659258262890683122, 1.000000000000000000, 0.9659258262890683122, 1.000000000000000000, 0.9659258262890683122, 1.000000000000000000, 0.9659258262890683122, 1.000000000000000000, 0.9659258262890683122, 1.000000000000000000, 0.9659258262890683122, 1.000000000000000000, 0.9659258262890683122, 1.000000000000000000, 0.9659258262890683122, 1.000000000000000000, 0.9659258262890683122, 1.000000000000000000, 0.9659258262890683122, 1.000000000000000000, 0.9659258262890683122, 1.000000000000000000, 0.9659258262890683122, 1.000000000000000000, 0.9659258262890683122, 1.000000000000000000, 0.9659258262890683122, 1.000000000000000000, 0.9659258262890683122, 1.000000000000000000, 0.9659258262890683122, 1.000000000000000000, 0.9659258262890683122, 1.000000000000000000, 0.9659258262890683122, 1.000000000000000000, 0.9659258262890683122, 1.000000000000000000, 0.9659258262890683122, 1.000000000000000000, 0.9659258262890683122, 1.000000000000000000, 0.9659258262890683122, 1.000000000000000000, 0.9659258262890683122, 1.000000000000000000, 0.9659258262890683122, 1.000000000000000000, 0.9659258262890683122, 1.000000000000000000, 0.9659258262890683122, 1.000000000000000000, 0.9659258262890683122, 1.000000000000000000, 0.9659258262890683122, 1.000000000000000000, 0.9659258262890683122, 1.000000000000000000, 0.9659258262890683122, 1.000000000000000000, 0.9659258262890683122, 1.000000000000000000, 0.9659258262890683122, 1.000000000000000000, 0.9659258262890683122, 1.000000000000000000, 0.9659258262890683122, 1.000000000000000000, 0.9659258262890683122, 1.000000000000000000, 0.9659258262890683122, 1.000000000000000000, 0.9659258262890683122, 1.000000000000000000, 0.9659258262890683122, 1.000000000000000000, 0.9659258262890683122, 1.000000000000000000, 0.9659258262890683122, 1.000000000000000000, 0.9659258262890683122, 1.000000000000000000, 0.9659258262890683122, 1.000000000000000000, 0.9659258262890683122, 1.000000000000000000, 0.9659258262890683122, 1.000000000000000000, 0.9659258262890683122, 1.000000000000000000, 0.9659258262890683122, 1.000000000000000000, 0.9659258262890683122, 1.000000000000000000, 0.9659258262890683122, 1.000000000000000000, 0.9659258262890683122, 1.000000000000000000, 0.9659258262890683122, 1.000000000000000000, 0.9659258262890683122, 1.000000000000000000, 0.9659258262890683122, 1.000000000000000000, 0.9659258262890683122, 1.000000000000000000, 0.9659258262890683122, 1.000000000000000000, 0.9659258262890683122, 1.000000000000000000, 0.9659258262890683122, 1.000000000000000000, 0.9659258262890683122, 1.000000000000000000, 0.9659258262890683122, 1.000000000000000000, 0.9659258262890683122, 1.000000000000000000, 0.9659258262890683122, 1.000000000000000000, 0.9659258262890683122, 1.000000000000000000, 0.9659258262890683122, 1.000000000000000000, 0.9659258262890683122, 1.000000000000000000, 0.9659258262890683122, 1.000000000000000000, 0.9659258262890683122, 1.000000000000000000, 0.9659258262890683122, 1.000000000000000000, 0.9659258262890683122, 1.000000000000000000, 0.9659258262890683122, 1.000000000000000000, 0.9659258262890683122, 1.000000000000000000, 0.9659258262890683122, 1.000000000000000000, 0.9659258262890683122, 1.000000000000000000, 0.9659258262890683122, 1.000000000000000000, 0.9659258262890683122, 1.000000000000000000, 0.9659258262890683122, 1.000000000000000000, 0.9659258262890683122, 1.000000000000000000, 0.9659258262890683122, 1.000000000000000000, 0.9659258262890683122, 1.000000000000000000, 0.9659258262890683122, 1.000000000000000000, 0.9659258262890683122, 1.000000000000000000, 0.9659258262890683122, 1.000000000000000000, 0.9659258262890683122, 1.000000000000000000, 0.9659258262890683122, 1.000000000000000000, 0.9659258262890683122, 1.000000000000000000, 0.9659258262890683122, 1.000000000000000000, 0.9659258262890683122, 1.000000000000000000, 0.9659258262890683122, 1.000000000000000000, 0.9659258262890683122, 1.000000000000000000, 0.9659258262890683122, 1.000000000000000000, 0.9659258262890683122, 1.000000000000000000, 0.9659258262890683122, 1.000000000000000000, 0.9659258262890683122, 1.000000000000000000, 0.9659258262890683122, 1.000000000000000000, 0.9659258262890683122, 1.000000000000000000, 0.9659258262890683122, 1.000000000000000000, 0.9659258262890683122, 1.000000000000000000, 0.9659258262890683122, 1.000000000000000000, 0.9659258262890683122, 1.000000000000000000, 0.9659258262890683122, 1.000000000000000000, 0.9659258262890683122, 1.000000000000000000, 0.9659258262890683122, 1.000000000000000000, 0.9659258262890683122, 1.000000000000000000, 0.9659258262890683122, 1.000000000000000000, 0.9659258262890683122, 1.000000000000000000, 0.9659258262890683122, 1.000000000000000000, 0.9659258262890683122, 1.000000000000000000, 0.9659258262890683122, 1.000000000000000000, 0.9659258262890683122, 1.000000000000000000, 0.9659258262890683122, 1.000000000000000000, 0.9659258262890683122, 1.000000000000000000, 0.9659258262890683122, 1.000000000000000000, 0.9659258262890683122, 1.000000000000000000, 0.9659258262890683122, 1.000000000000000000, 0.9659258262890683122, 1.000000000000000000, 0.9659258262890683122, 1.000000000000000000, 0.9659258262890683122, 1.000000000000000000, 0.9659258262890683122, 1.000000000000000000, 0.9659258262890683122, 1.000000000000000000, 0.9659258262890683122, 1.000000000000000000, 0.9659258262890683122, 1.000000000000000000, 0.9659258262890683122, 1.000000000000000000, 0.9659258262890683122, 1.000000000000000000, 0.9659258262890683122, 1.000000000000000000, 0.9659258262890683122, 1.000000000000000000, 0.9659258262890683122, 1.000000000000000000, 0.9659258262890683122, 1.000000000000000000, 0.9659258262890683122, 1.000000000000000000, 0.9659258262890683122, 1.000000000000000000, 0.9659258262890683122, 1.000000000000000000, 0.9659258262890683122, 1.000000000000000000),
 ( 1.000000000000000000, 0.9659258262890683122, 1.000000000000000000, 0.9659258262890683122, 1.000000000000000000, 0.9659258262890683122, 1.000000000000000000, 0.9659258262890683122, 1.000000000000000000, 0.9659258262890683122, 1.000000000000000000, 0.9659258262890683122, 1.000000000000000000, 0.9659258262890683122, 1.000000000000000000, 0.9659258262890683122, 1.000000000000000000, 0.9659258262890683122, 1.000000000000000000, 0.9659258262890683122, 1.000000000000000000, 0.9659258262890683122, 1.000000000000000000, 0.9659258262890683122, 1.000000000000000000, 0.9659258262890683122, 1.000000000000000000, 0.9659258262890683122, 1.000000000000000000, 0.9659258262890683122, 1.000000000000000000, 0.9659258262890683122, 1.000000000000000000, 0.9659258262890683122, 1.000000000000000000, 0.9659258262890683122, 1.000000000000000000, 0.9659258262890683122, 1.000000000000000000, 0.9659258262890683122, 1.000000000000000000, 0.9659258262890683122, 1.000000000000000000, 0.9659258262890683122, 1.000000000000000000, 0.9659258262890683122, 1.000000000000000000, 0.9659258262890683122, 1.000000000000000000, 0.9659258262890683122, 1.000000000000000000, 0.9659258262890683122, 1.000000000000000000, 0.9659258262890683122, 1.000000000000000000, 0.9659258262890683122, 1.000000000000000000, 0.9659258262890683122, 1.000000000000000000, 0.9659258262890683122, 1.000000000000000000, 0.9659258262890683122, 1.000000000000000000, 0.9659258262890683122, 1.000000000000000000, 0.9659258262890683122, 1.000000000000000000, 0.9659258262890683122, 1.000000000000000000, 0.9659258262890683122, 1.000000000000000000, 0.9659258262890683122, 1.000000000000000000, 0.9659258262890683122, 1.000000000000000000, 0.9659258262890683122, 1.000000000000000000, 0.9659258262890683122, 1.000000000000000000, 0.9659258262890683122, 1.000000000000000000, 0.9659258262890683122, 1.000000000000000000, 0.9659258262890683122, 1.000000000000000000, 0.9659258262890683122, 1.000000000000000000, 0.9659258262890683122, 1.000000000000000000, 0.9659258262890683122, 1.000000000000000000, 0.9659258262890683122, 1.000000000000000000, 0.9659258262890683122, 1.000000000000000000, 0.9659258262890683122, 1.000000000000000000, 0.9659258262890683122, 1.000000000000000000, 0.9659258262890683122, 1.000000000000000000, 0.9659258262890683122, 1.000000000000000000, 0.9659258262890683122, 1.000000000000000000, 0.9659258262890683122, 1.000000000000000000, 0.9659258262890683122, 1.000000000000000000, 0.9659258262890683122, 1.000000000000000000, 0.9659258262890683122, 1.000000000000000000, 0.9659258262890683122, 1.000000000000000000, 0.9659258262890683122, 1.000000000000000000, 0.9659258262890683122, 1.000000000000000000, 0.9659258262890683122, 1.000000000000000000, 0.9659258262890683122, 1.000000000000000000, 0.9659258262890683122, 1.000000000000000000, 0.9659258262890683122, 1.000000000000000000, 0.9659258262890683122, 1.000000000000000000, 0.9659258262890683122, 1.000000000000000000, 0.9659258262890683122, 1.000000000000000000, 0.9659258262890683122, 1.000000000000000000, 0.9659258262890683122, 1.000000000000000000, 0.9659258262890683122, 1.000000000000000000, 0.9659258262890683122, 1.000000000000000000, 0.9659258262890683122, 1.000000000000000000, 0.9659258262890683122, 1.000000000000000000, 0.9659258262890683122, 1.000000000000000000, 0.9659258262890683122, 1.000000000000000000, 0.9659258262890683122, 1.000000000000000000, 0.9659258262890683122, 1.000000000000000000, 0.9659258262890683122, 1.000000000000000000, 0.9659258262890683122, 1.000000000000000000, 0.9659258262890683122, 1.000000000000000000, 0.9659258262890683122, 1.000000000000000000, 0.9659258262890683122, 1.000000000000000000, 0.9659258262890683122, 1.000000000000000000, 0.9659258262890683122, 1.000000000000000000, 0.9659258262890683122, 1.000000000000000000, 0.9659258262890683122, 1.000000000000000000, 0.9659258262890683122, 1.000000000000000000, 0.9659258262890683122, 1.000000000000000000, 0.9659258262890683122, 1.000000000000000000, 0.9659258262890683122, 1.000000000000000000, 0.9659258262890683122, 1.000000000000000000, 0.9659258262890683122, 1.000000000000000000, 0.9659258262890683122, 1.000000000000000000, 0.9659258262890683122, 1.000000000000000000, 0.9659258262890683122, 1.000000000000000000, 0.9659258262890683122, 1.000000000000000000, 0.9659258262890683122, 1.000000000000000000, 0.9659258262890683122, 1.000000000000000000, 0.9659258262890683122, 1.000000000000000000, 0.9659258262890683122, 1.000000000000000000, 0.9659258262890683122, 1.000000000000000000, 0.9659258262890683122, 1.000000000000000000, 0.9659258262890683122, 1.000000000000000000, 0.9659258262890683122, 1.000000000000000000, 0.9659258262890683122, 1.000000000000000000, 0.9659258262890683122, 1.000000000000000000, 0.9659258262890683122, 1.000000000000000000, 0.9659258262890683122, 1.000000000000000000, 0.9659258262890683122, 1.000000000000000000, 0.9659258262890683122, 1.000000000000000000, 0.9659258262890683122, 1.000000000000000000, 0.9659258262890683122, 1.000000000000000000, 0.9659258262890683122, 1.000000000000000000, 0.9659258262890683122, 1.000000000000000000, 0.9659258262890683122, 1.000000000000000000, 0.9659258262890683122, 1.000000000000000000, 0.9659258262890683122, 1.000000000000000000, 0.9659258262890683122, 1.000000000000000000, 0.9659258262890683122, 1.000000000000000000, 0.9659258262890683122, 1.000000000000000000, 0.9659258262890683122, 1.000000000000000000, 0.9659258262890683122, 1.000000000000000000, 0.9659258262890683122, 1.000000000000000000, 0.9659258262890683122, 1.000000000000000000, 0.9659258262890683122, 1.000000000000000000, 0.9659258262890683122, 1.000000000000000000, 0.9659258262890683122, 1.000000000000000000, 0.9659258262890683122, 1.000000000000000000, 0.9659258262890683122, 1.000000000000000000, 0.9659258262890683122, 1.000000000000000000, 0.9659258262890683122, 1.000000000000000000, 0.9659258262890683122, 1.000000000000000000, 0.9659258262890683122, 1.000000000000000000, 0.9659258262890683122, 1.000000000000000000, 0.9659258262890683122, 1.000000000000000000, 0.9659258262890683122, 1.000000000000000000, 0.9659258262890683122, 1.000000000000000000, 0.9659258262890683122, 1.000000000000000000, 0.9659258262890683122, 1.000000000000000000, 0.9659258262890683122, 1.000000000000000000, 0.9659258262890683122, 1.000000000000000000, 0.9659258262890683122, 1.000000000000000000, 0.9659258262890683122, 1.000000000000000000, 0.9659258262890683122, 1.000000000000000000, 0.9659258262890683122, 1.000000000000000000, 0.9659258262890683122, 1.000000000000000000, 0.9659258262890683122, 1.000000000000000000, 0.9659258262890683122, 1.000000000000000000, 0.9659258262890683122, 1.000000000000000000, 0.9659258262890683122, 1.000000000000000000, 0.9659258262890683122, 1.000000000000000000, 0.9659258262890683122, 1.000000000000000000, 0.9659258262890683122, 1.000000000000000000, 0.9659258262890683122, 1.000000000000000000, 0.9659258262890683122, 1.000000000000000000, 0.9659258262890683122, 1.000000000000000000, 0.9659258262890683122, 1.000000000000000000, 0.9659258262890683122, 1.000000000000000000, 0.9659258262890683122, 1.000000000000000000, 0.9659258262890683122, 1.000000000000000000, 0.9659258262890683122, 1.000000000000000000, 0.9659258262890683122, 1.000000000000000000, 0.9659258262890683122, 1.000000000000000000, 0.9659258262890683122, 1.000000000000000000, 0.9659258262890683122, 1.000000000000000000, 0.9659258262890683122, 1.000000000000000000, 0.9659258262890683122, 1.000000000000000000, 0.9659258262890683122, 1.000000000000000000, 0.9659258262890683122, 1.000000000000000000, 0.9659258262890683122, 1.000000000000000000, 0.9659258262890683122, 1.000000000000000000, 0.9659258262890683122, 1.000000000000000000, 0.9659258262890683122, 1.000000000000000000, 0.9659258262890683122, 1.000000000000000000, 0.9659258262890683122, 1.000000000000000000, 0.9659258262890683122, 1.000000000000000000, 0.9659258262890683122, 1.000000000000000000, 0.9659258262890683122, 1.000000000000000000, 0.9659258262890683122, 1.000000000000000000, 0.9659258262890683122, 1.000000000000000000, 0.9659258262890683122, 1.000000000000000000, 0.9659258262890683122, 1.000000000000000000, 0.9659258262890683122, 1.000000000000000000, 0.9659258262890683122, 1.000000000000000000, 0.9659258262890683122, 1.000000000000000000, 0.9659258262890683122, 1.000000000000000000, 0.9659258262890683122, 1.000000000000000000, 0.9659258262890683122, 1.000000000000000000, 0.9659258262890683122, 1.000000000000000000, 0.9659258262890683122, 1.000000000000000000, 0.9659258262890683122, 1.000000000000000000, 0.9659258262890683122, 1.000000000000000000, 0.9659258262890683122, 1.000000000000000000, 0.9659258262890683122, 1.000000000000000000, 0.9659258262890683122, 1.000000000000000000, 0.9659258262890683122, 1.000000000000000000, 0.9659258262890683122, 1.000000000000000000, 0.9659258262890683122, 1.000000000000000000, 0.9659258262890683122, 1.000000000000000000, 0.9659258262890683122, 1.000000000000000000, 0.9659258262890683122, 1.000000000000000000, 0.9659258262890683122, 1.000000000000000000, 0.9659258262890683122, 1.000000000000000000, 0.9659258262890683122, 1.000000000000000000, 0.9659258262890683122, 1.000000000000000000, 0.9659258262890683122, 1.000000000000000000, 0.9659258262890683122, 1.000000000000000000, 0.9659258262890683122, 1.000000000000000000, 0.9659258262890683122, 1.000000000000000000, 0.9659258262890683122, 1.000000000000000000, 0.9659258262890683122, 1.000000000000000000, 0.9659258262890683122, 1.000000000000000000, 0.9659258262890683122, 1.000000000000000000, 0.9659258262890683122, 1.000000000000000000, 0.9659258262890683122, 1.000000000000000000, 0.9659258262890683122, 1.000000000000000000, 0.9659258262890683122, 1.000000000000000000, 0.9659258262890683122, 1.000000000000000000, 0.9659258262890683122, 1.000000000000000000, 0.9659258262890683122, 1.000000000000000000, 0.9659258262890683122, 1.000000000000000000, 0.9659258262890683122, 1.000000000000000000, 0.9659258262890683122, 1.000000000000000000, 0.9659258262890683122, 1.000000000000000000, 0.9659258262890683122, 1.000000000000000000, 0.9659258262890683122, 1.000000000000000000, 0.9659258262890683122, 1.000000000000000000, 0.9659258262890683122, 1.000000000000000000, 0.9659258262890683122, 1.000000000000000000, 0.9659258262890683122, 1.000000000000000000, 0.9659258262890683122, 1.000000000000000000, 0.9659258262890683122, 1.000000000000000000, 0.9659258262890683122, 1.000000000000000000, 0.9659258262890683122, 1.000000000000000000, 0.9659258262890683122, 1.000000000000000000, 0.9659258262890683122, 1.000000000000000000, 0.9659258262890683122, 1.000000000000000000, 0.9659258262890683122, 1.000000000000000000, 0.9659258262890683122, 1.000000000000000000, 0.9659258262890683122, 1.000000000000000000, 0.9659258262890683122, 1.000000000000000000, 0.9659258262890683122, 1.000000000000000000, 0.9659258262890683122, 1.000000000000000000, 0.9659258262890683122, 1.000000000000000000, 0.9659258262890683122, 1.000000000000000000, 0.9659258262890683122, 1.000000000000000000, 0.9659258262890683122, 1.000000000000000000, 0.9659258262890683122, 1.000000000000000000, 0.9659258262890683122, 1.000000000000000000, 0.9659258262890683122, 1.000000000000000000, 0.9659258262890683122, 1.000000000000000000, 0.9659258262890683122, 1.000000000000000000, 0.9659258262890683122, 1.000000000000000000, 0.9659258262890683122, 1.000000000000000000, 0.9659258262890683122, 1.000000000000000000, 0.9659258262890683122, 1.000000000000000000) ) ) 
 REPRESENTATION_ITEM ( '' )  SURFACE ( )  );
#54180=CARTESIAN_POINT ( 'NONE',  ( -0.6036745406824141069, 0.1283753931104748280, 0.1820866141732283561 ) ) ;
#54185=CARTESIAN_POINT ( 'NONE',  ( 1.286089238845145033, 0.1283753931104748280, 0.1820866141732283561 ) ) ;
#54187=CARTESIAN_POINT ( 'NONE',  ( 0.8267716535433077274, 0.2952755905511811885, 0.000000000000000000 ) ) ;
#54189=CARTESIAN_POINT ( 'NONE',  ( 1.286089238845145033, -0.5023911411419708095, -0.1820866141732282451 ) ) ;
#54190=CARTESIAN_POINT ( 'NONE',  ( 0.01968503937007957949, -0.5400638737290845981, -0.3530559997133363437 ) ) ;
#54191=CARTESIAN_POINT ( 'NONE',  ( -0.4593175853018364174, -0.4281496062992127816, -0.4176697321401328100 ) ) ;
#54192=CARTESIAN_POINT ( 'NONE',  ( 1.489501312335958172, -0.3162353388693405765, 0.4822834645669290543 ) ) ;
#54195=CARTESIAN_POINT ( 'NONE',  ( 0.1968503937007881344, 0.1771653543307087630, 0.000000000000000000 ) ) ;
#54196=ORIENTED_EDGE ( 'NONE', *, *, #60977, .T. ) ;
#54199=CARTESIAN_POINT ( 'NONE',  ( -0.5511811023622041894, -0.1870078740157480879, -0.4822834645669291653 ) ) ;
#54200=CARTESIAN_POINT ( 'NONE',  ( 0.7283464566929140904, -0.5400638737290845981, -0.3530559997133363437 ) ) ;
#54201=CARTESIAN_POINT ( 'NONE',  ( 0.02624671916010564918, -0.6046776061558809534, -0.2411417322834644161 ) ) ;
#54202=CARTESIAN_POINT ( 'NONE',  ( -0.3083989501312330295, -0.2845877964562161244, -0.3641732283464567121 ) ) ;
#54203=CARTESIAN_POINT ( 'NONE',  ( 0.8792650918635177559, 0.05413385826771666132, 0.4176697321401328100 ) ) ;
#54204=CARTESIAN_POINT ( 'NONE',  ( -0.8267716535433065062, 0.2952755905511811885, 0.000000000000000000 ) ) ;
#54206=CARTESIAN_POINT ( 'NONE',  ( -0.2887139107611542133, 0.2306618581243848609, 0.2411417322834645549 ) ) ;
#54207=CARTESIAN_POINT ( 'NONE',  ( -0.7020997375328076329, -0.3162353388693409650, -0.4822834645669289433 ) ) ;
#54208=CARTESIAN_POINT ( 'NONE',  ( 1.010498687664042716, 0.05413385826771626580, -0.4176697321401330321 ) ) ;
#54209=CARTESIAN_POINT ( 'NONE',  ( 0.8070866141732288002, 0.1660481256975885056, 0.3530559997133364547 ) ) ;
#54210=B_SPLINE_CURVE_WITH_KNOTS ( 'NONE', 3,
 ( #81433, #16213, #43091, #61220 ),
 .UNSPECIFIED., .F., .F.,
 ( 4, 4 ),
 ( 3.593986969197074047E-07, 0.001287825409103121209 ),
 .UNSPECIFIED. ) ;
#54211=CARTESIAN_POINT ( 'NONE',  ( 0.9186351706036752773, 0.2306618581243847221, -0.2411417322834647770 ) ) ;
#54213=CARTESIAN_POINT ( 'NONE',  ( 0.03280839895013198948, -0.5511811023622048555, -0.09757992244046775898 ) ) ;
#54217=CARTESIAN_POINT ( 'NONE',  ( -1.017060367454067249, -0.2845877964562161244, -0.3641732283464567121 ) ) ;
#54218=CARTESIAN_POINT ( 'NONE',  ( -0.5052493438320203589, 0.2952755905511810774, -0.1292274648535930714 ) ) ;
#54220=CARTESIAN_POINT ( 'NONE',  ( -0.4658792650918627265, -0.05778040916215522460, 0.4822834645669289988 ) ) ;
#54221=CARTESIAN_POINT ( 'NONE',  ( -0.5052493438320203589, -0.6692913385826771977, 0.1292274648535927661 ) ) ;
#54222=CARTESIAN_POINT ( 'NONE',  ( -1.167979002624671470, 0.05413385826771666132, 0.4176697321401328100 ) ) ;
#54223=CARTESIAN_POINT ( 'NONE',  ( -1.437007874015747477, -0.5400638737290844871, 0.3530559997133364547 ) ) ;
#54224=CARTESIAN_POINT ( 'NONE',  ( 1.141732283464567788, -0.5511811023622047445, 6.969142054262312111E-17 ) ) ;
#54227=CARTESIAN_POINT ( 'NONE',  ( 0.5118110236220478892, 0.1771653543307087630, 0.000000000000000000 ) ) ;
#54229=CARTESIAN_POINT ( 'NONE',  ( -0.1246719160104980823, -0.6692913385826773087, -0.1292274648535924053 ) ) ;
#54230=CARTESIAN_POINT ( 'NONE',  ( 0.3215223097112867578, -0.3162353388693409650, -0.4822834645669289433 ) ) ;
#54231=EDGE_LOOP ( 'NONE', ( #16634, #63536, #47900, #42600 ) ) ;
#54234=ORIENTED_EDGE ( 'NONE', *, *, #14670, .F. ) ;
#54237=CARTESIAN_POINT ( 'NONE',  ( -0.5183727034120726440, -0.5511811023622048555, -0.09757992244046775898 ) ) ;
#54238=CARTESIAN_POINT ( 'NONE',  ( -0.6430446194225716283, -0.4281496062992124485, 0.4176697321401328655 ) ) ;
#54241=CARTESIAN_POINT ( 'NONE',  ( -1.535433070866141225, -0.5511811023622047445, 6.969142054262312111E-17 ) ) ;
#54242=CARTESIAN_POINT ( 'NONE',  ( 0.8464566929133865436, 0.1660481256975883668, -0.3530559997133364547 ) ) ;
#54243=CARTESIAN_POINT ( 'NONE',  ( 1.017060367454068803, -0.3162353388693405765, 0.4822834645669290543 ) ) ;
#54244=CARTESIAN_POINT ( 'NONE',  ( -0.4724409448818890911, -0.1870078740157480601, -0.3641732283464567677 ) ) ;
#54245=CARTESIAN_POINT ( 'NONE',  ( 0.2559055118110243332, -0.5400638737290845981, -0.3530559997133363437 ) ) ;
#54247=CARTESIAN_POINT ( 'NONE',  ( 0.03937007874015833325, -0.5511811023622047445, 6.969142054262312111E-17 ) ) ;
#54248=CARTESIAN_POINT ( 'NONE',  ( -0.6561679790026240244, -0.6046776061558807314, 0.2411417322834647770 ) ) ;
#54251=CARTESIAN_POINT ( 'NONE',  ( -1.581364829396324945, -0.3162353388693405765, 0.4822834645669290543 ) ) ;
#54252=CARTESIAN_POINT ( 'NONE',  ( -0.07874015748031421014, -0.1870078740157480601, -0.3641732283464567677 ) ) ;
#54253=CARTESIAN_POINT ( 'NONE',  ( 1.587926509186352586, -0.3690944881889765550, -0.3153832671262227771 ) ) ;
#54254=CARTESIAN_POINT ( 'NONE',  ( -0.9973753280839886548, -0.6046776061558809534, -0.2411417322834644161 ) ) ;
#54255=CARTESIAN_POINT ( 'NONE',  ( -0.8464566929133852113, 0.07958543189024085140, 0.2665933059059887866 ) ) ;
#54257=CARTESIAN_POINT ( 'NONE',  ( -1.069553805774277722, 0.2952755905511811885, 0.1292274648535926551 ) ) ;
#54258=CARTESIAN_POINT ( 'NONE',  ( -0.2165354330708654795, 0.1660481256975885056, 0.3530559997133364547 ) ) ;
#54262=CARTESIAN_POINT ( 'NONE',  ( 0.2362204724409456558, -0.1870078740157479769, 0.3641732283464567677 ) ) ;
#54263=CARTESIAN_POINT ( 'NONE',  ( 0.9973753280839902091, 0.2306618581243847221, -0.2411417322834647770 ) ) ;
#54264=CARTESIAN_POINT ( 'NONE',  ( -1.286089238845143479, -0.5023911411419708095, 0.1820866141732285504 ) ) ;
#54266=CARTESIAN_POINT ( 'NONE',  ( 1.325459317585302665, -0.4281496062992124485, 0.4176697321401328655 ) ) ;
#54267=CARTESIAN_POINT ( 'NONE',  ( -1.522309711286088607, 0.1283753931104746893, -0.1820866141732285504 ) ) ;
#54268=CARTESIAN_POINT ( 'NONE',  ( -0.5380577427821514602, -0.4281496062992127816, -0.4176697321401328100 ) ) ;
#54269=CARTESIAN_POINT ( 'NONE',  ( 0.2296587926509192634, -0.2845877964562159024, 0.3641732283464567677 ) ) ;
#54271=CARTESIAN_POINT ( 'NONE',  ( 0.4921259842519691285, 0.07958543189024085140, 0.2665933059059887866 ) ) ;
#54272=ADVANCED_FACE ( 'NONE', ( #34026 ), #54179, .F. ) ;
#54273=CARTESIAN_POINT ( 'NONE',  ( -0.006561679790025524116, -0.05778040916215560624, -0.4822834645669293319 ) ) ;
#54275=CARTESIAN_POINT ( 'NONE',  ( -1.227034120734907585, 0.2952755905511811885, 0.1292274648535926551 ) ) ;
#54277=CARTESIAN_POINT ( 'NONE',  ( 1.036745406824147508, -0.3690944881889765550, -0.3153832671262227771 ) ) ;
#54278=CARTESIAN_POINT ( 'NONE',  ( -0.05905511811023545637, 0.1660481256975885056, 0.3530559997133364547 ) ) ;
#54279=CARTESIAN_POINT ( 'NONE',  ( -0.2427821522309703550, -0.3162353388693405765, 0.4822834645669290543 ) ) ;
#54280=CARTESIAN_POINT ( 'NONE',  ( -0.5118110236220466680, 0.1771653543307087630, 0.000000000000000000 ) ) ;
#54281=CARTESIAN_POINT ( 'NONE',  ( 0.9711286089238851948, 0.1539470093639523085, 0.1968503937007873850 ) ) ;
#54282=CARTESIAN_POINT ( 'NONE',  ( -0.3740157480314953431, 0.07958543189024085140, 0.2665933059059887866 ) ) ;
#54283=CARTESIAN_POINT ( 'NONE',  ( 0.3149606299212606708, -0.1870078740157480879, -0.4822834645669291653 ) ) ;
#54284=CARTESIAN_POINT ( 'NONE',  ( -0.6364829396325453192, -0.2845877964562159024, 0.3641732283464567677 ) ) ;
#54286=CARTESIAN_POINT ( 'NONE',  ( -1.174540682414697335, -0.05778040916215522460, 0.4822834645669289988 ) ) ;
#54290=CARTESIAN_POINT ( 'NONE',  ( -1.010498687664041384, -0.3690944881889765550, -0.3153832671262227771 ) ) ;
#54291=CARTESIAN_POINT ( 'NONE',  ( -0.4068241469816267775, 0.05413385826771626580, -0.4176697321401330321 ) ) ;
#54292=ADVANCED_FACE ( 'NONE', ( #80961 ), #62830, .F. ) ;
#54293=CARTESIAN_POINT ( 'NONE',  ( -1.607611548556429737, -0.6692913385826771977, 0.1292274648535927661 ) ) ;
#54294=CARTESIAN_POINT ( 'NONE',  ( -1.213910761154854745, -0.6692913385826771977, 0.1292274648535927661 ) ) ;
#54295=CARTESIAN_POINT ( 'NONE',  ( -1.092353285368623750, -2.191421614605370878E-15, 0.4445507791589071167 ) ) ;
#54296=CARTESIAN_POINT ( 'NONE',  ( 1.338582677165355062, -0.1870078740157479769, 0.4822834645669291653 ) ) ;
#54297=CARTESIAN_POINT ( 'NONE',  ( 0.9251968503937015864, 0.1660481256975883668, -0.3530559997133364547 ) ) ;
#54300=CARTESIAN_POINT ( 'NONE',  ( 1.423884514435696191, -0.08942795157527998196, 0.3641732283464567121 ) ) ;
#54302=ORIENTED_EDGE ( 'NONE', *, *, #2422, .F. ) ;
#54303=ADVANCED_FACE ( 'NONE', ( #35500 ), #54683, .F. ) ;
#54304=CARTESIAN_POINT ( 'NONE',  ( -0.3149606299212590610, -0.1870078740157480601, -0.3641732283464567677 ) ) ;
#54308=CARTESIAN_POINT ( 'NONE',  ( 0.9186351706036751663, -0.6046776061558807314, 0.2411417322834647770 ) ) ;
#54309=CARTESIAN_POINT ( 'NONE',  ( -0.5183727034120726440, -0.6692913385826773087, -0.1292274648535924053 ) ) ;
#54310=CARTESIAN_POINT ( 'NONE',  ( -0.5774278215223089816, -0.6046776061558807314, 0.2411417322834647770 ) ) ;
#54311=CARTESIAN_POINT ( 'NONE',  ( 1.574803149606299746, -0.1870078740157480879, -0.4822834645669291653 ) ) ;
#54312=CARTESIAN_POINT ( 'NONE',  ( -1.332020997375327642, -0.08942795157527998196, 0.3641732283464567121 ) ) ;
#54314=CARTESIAN_POINT ( 'NONE',  ( 0.4265091863517067594, 0.2952755905511811885, 0.1292274648535926551 ) ) ;
#54315=CARTESIAN_POINT ( 'NONE',  ( -0.8398950131233585692, 0.2306618581243848609, 0.2411417322834645549 ) ) ;
#54317=CARTESIAN_POINT ( 'NONE',  ( -1.437007874015747477, 0.1660481256975883668, -0.3530559997133364547 ) ) ;
#54318=FACE_OUTER_BOUND ( 'NONE', #40431, .T. ) ;
#54321=CARTESIAN_POINT ( 'NONE',  ( 0.8989501312335964611, 0.2952755905511811885, 0.1292274648535926551 ) ) ;
#54322=CARTESIAN_POINT ( 'NONE',  ( 1.115485564304462551, -0.3690944881889765550, -0.3153832671262227771 ) ) ;
#54323=ORIENTED_EDGE ( 'NONE', *, *, #20226, .F. ) ;
#54325=CARTESIAN_POINT ( 'NONE',  ( -0.4986876640419939388, 0.2306618581243847221, -0.2411417322834647770 ) ) ;
#54327=CARTESIAN_POINT ( 'NONE',  ( 0.2099737532808405305, 0.1283753931104746893, -0.1820866141732285504 ) ) ;
#54328=CARTESIAN_POINT ( 'NONE',  ( -1.227034120734907585, 0.2952755905511811885, 0.1292274648535926551 ) ) ;
#54329=CARTESIAN_POINT ( 'NONE',  ( 0.9908136482939640111, 0.2952755905511810774, -0.1292274648535930714 ) ) ;
#54330=CARTESIAN_POINT ( 'NONE',  ( 0.6955380577427828781, 0.05413385826771626580, -0.4176697321401330321 ) ) ;
#54331=CARTESIAN_POINT ( 'NONE',  ( 0.03937007874015806264, 0.2952755905511811885, 0.000000000000000000 ) ) ;
#54333=CARTESIAN_POINT ( 'NONE',  ( -0.7742782152230962556, -0.4281496062992127816, -0.4176697321401328100 ) ) ;
#54335=CARTESIAN_POINT ( 'NONE',  ( -1.450131233595799651, -0.6692913385826771977, 0.1292274648535927661 ) ) ;
#54336=CARTESIAN_POINT ( 'NONE',  ( -0.6102362204724400829, -0.5400638737290845981, -0.3530559997133363437 ) ) ;
#54337=CARTESIAN_POINT ( 'NONE',  ( -0.4790026246719152336, -0.08942795157528024563, -0.3641732283464568787 ) ) ;
#54338=CARTESIAN_POINT ( 'NONE',  ( 1.423884514435696413, -0.3162353388693409650, -0.4822834645669289433 ) ) ;
#54339=CARTESIAN_POINT ( 'NONE',  ( 1.640419947506562393, -0.4281496062992124485, 0.4176697321401328655 ) ) ;
#54340=CARTESIAN_POINT ( 'NONE',  ( -0.7414698162729651543, 0.2952755905511810774, -0.1292274648535930714 ) ) ;
#54342=CARTESIAN_POINT ( 'NONE',  ( 0.7414698162729663755, -0.6692913385826773087, -0.1292274648535924053 ) ) ;
#54344=CARTESIAN_POINT ( 'NONE',  ( 1.607611548556431069, 0.2952755905511811885, 0.1292274648535926551 ) ) ;
#54345=CARTESIAN_POINT ( 'NONE',  ( -0.2034120734908128059, 0.2952755905511811885, 0.1292274648535926551 ) ) ;
#54346=CARTESIAN_POINT ( 'NONE',  ( -1.108923884514435132, -0.08942795157528024563, -0.3641732283464568787 ) ) ;
#54347=CARTESIAN_POINT ( 'NONE',  ( 0.9383202099737538715, -0.08942795157528024563, -0.3641732283464568787 ) ) ;
#54349=CARTESIAN_POINT ( 'NONE',  ( 1.200787401574803681, 0.07958543189024085140, 0.2665933059059887866 ) ) ;
#54350=CARTESIAN_POINT ( 'NONE',  ( 0.9580052493438326877, 0.05413385826771666132, 0.4176697321401328100 ) ) ;
#54352=CARTESIAN_POINT ( 'NONE',  ( -0.2099737532808391705, -0.6046776061558809534, -0.2411417322834644161 ) ) ;
#54353=LINE ( 'NONE', #29920, #32403 ) ;
#54355=CARTESIAN_POINT ( 'NONE',  ( 1.292650918635171564, 0.1771653543307087630, 0.09757992244046791164 ) ) ;
#54356=CARTESIAN_POINT ( 'NONE',  ( -0.5577427821522301654, -0.05778040916215560624, -0.4822834645669293319 ) ) ;
#54358=CARTESIAN_POINT ( 'NONE',  ( 1.482939632545932307, -0.4281496062992124485, 0.4176697321401328655 ) ) ;
#54359=CARTESIAN_POINT ( 'NONE',  ( 0.01312335958005323398, 0.05413385826771666132, 0.4176697321401328100 ) ) ;
#54360=CARTESIAN_POINT ( 'NONE',  ( 0.4724409448818904789, -0.1870078740157480601, -0.3641732283464567677 ) ) ;
#54362=CARTESIAN_POINT ( 'NONE',  ( 0.2493438320209980519, -0.004921259842519576551, 0.3153832671262227771 ) ) ;
#54363=CARTESIAN_POINT ( 'NONE',  ( -1.614173228346455824, 0.2952755905511811885, 0.000000000000000000 ) ) ;
#54365=CARTESIAN_POINT ( 'NONE',  ( 0.7349081364829403995, 0.2306618581243848609, 0.2411417322834645549 ) ) ;
#54369=CARTESIAN_POINT ( 'NONE',  ( 0.09842519685039434474, -0.4536011799217368745, -0.2665933059059886201 ) ) ;
#54370=EDGE_CURVE ( 'NONE', #14171, #9936, #13271, .T. ) ;
#54371=AXIS2_PLACEMENT_3D ( 'NONE', #35945, #81400, #4361 ) ;
#54372=CARTESIAN_POINT ( 'NONE',  ( 0.2559055118110243332, 0.1660481256975885056, 0.3530559997133364547 ) ) ;
#54373=CARTESIAN_POINT ( 'NONE',  ( 1.561679790026247350, -0.004921259842519870586, -0.3153832671262229437 ) ) ;
#54374=CARTESIAN_POINT ( 'NONE',  ( -1.286089238845143479, -0.5023911411419708095, 0.1820866141732285504 ) ) ;
#54375=CARTESIAN_POINT ( 'NONE',  ( -1.528871391076114250, 0.2952755905511810774, -0.1292274648535930714 ) ) ;
#54376=CARTESIAN_POINT ( 'NONE',  ( 0.3608923884514443348, -0.6692913385826771977, 0.1292274648535927661 ) ) ;
#54377=CARTESIAN_POINT ( 'NONE',  ( 1.305774278215223960, -0.6692913385826771977, 0.1292274648535927661 ) ) ;
#54378=CARTESIAN_POINT ( 'NONE',  ( 1.603475055217291612, 0.7793870273546369409, -0.04573490813648244807 ) ) ;
#54379=CARTESIAN_POINT ( 'NONE',  ( 0.6430446194225728496, 0.05413385826771666132, 0.4176697321401328100 ) ) ;
#54380=CARTESIAN_POINT ( 'NONE',  ( 1.292650918635171564, -0.6692913385826773087, -0.1292274648535924053 ) ) ;
#54381=CARTESIAN_POINT ( 'NONE',  ( 0.7677165354330716118, 0.1660481256975883668, -0.3530559997133364547 ) ) ;
#54383=CARTESIAN_POINT ( 'NONE',  ( 0.6233595800524942554, -0.08942795157528024563, -0.3641732283464568787 ) ) ;
#54384=CARTESIAN_POINT ( 'NONE',  ( 1.653543307086614789, -0.1870078740157479769, 0.4822834645669291653 ) ) ;
#54385=CARTESIAN_POINT ( 'NONE',  ( -0.9776902887139098386, 0.1771653543307087075, -0.09757992244046823083 ) ) ;
#54386=CARTESIAN_POINT ( 'NONE',  ( 0.5380577427821529035, -0.004921259842519870586, -0.3153832671262229437 ) ) ;
#54387=CARTESIAN_POINT ( 'NONE',  ( 0.1312335958005257930, 0.2306618581243847221, -0.2411417322834647770 ) ) ;
#54388=CARTESIAN_POINT ( 'NONE',  ( 0.7349081364829402885, -0.6046776061558809534, -0.2411417322834644161 ) ) ;
#54389=CARTESIAN_POINT ( 'NONE',  ( -0.3543307086614165824, 0.2952755905511811885, 0.000000000000000000 ) ) ;
#54390=CARTESIAN_POINT ( 'NONE',  ( 0.1902887139107617975, 0.1771653543307087630, 0.09757992244046791164 ) ) ;
#54391=CARTESIAN_POINT ( 'NONE',  ( 0.8530183727034126306, 0.05413385826771626580, -0.4176697321401330321 ) ) ;
#54393=CARTESIAN_POINT ( 'NONE',  ( -0.8858267716535425107, 0.1660481256975883668, -0.3530559997133364547 ) ) ;
#54396=CARTESIAN_POINT ( 'NONE',  ( -0.8267716535433065062, 0.2952755905511811885, 0.000000000000000000 ) ) ;
#54397=CARTESIAN_POINT ( 'NONE',  ( -0.3477690288713905509, -0.6692913385826771977, 0.1292274648535927661 ) ) ;
#54402=CARTESIAN_POINT ( 'NONE',  ( 0.9448818897637802916, -0.1870078740157480601, -0.3641732283464567677 ) ) ;
#54404=CARTESIAN_POINT ( 'NONE',  ( 1.010498687664042716, 0.05413385826771626580, -0.4176697321401330321 ) ) ;
#54407=CARTESIAN_POINT ( 'NONE',  ( -1.299212598425196097, -0.5511811023622047445, 6.969142054262312111E-17 ) ) ;
#54408=CARTESIAN_POINT ( 'NONE',  ( 1.496062992125985147, -0.1870078740157479769, 0.4822834645669291653 ) ) ;
#54409=CARTESIAN_POINT ( 'NONE',  ( -1.384514435695537005, 0.2952755905511811885, 0.1292274648535926551 ) ) ;
#54410=CARTESIAN_POINT ( 'NONE',  ( 0.4199475065616805614, 0.2306618581243848609, 0.2411417322834645549 ) ) ;
#54412=CARTESIAN_POINT ( 'NONE',  ( 0.2034120734908144990, -0.6692913385826771977, 0.1292274648535927661 ) ) ;
#54413=CARTESIAN_POINT ( 'NONE',  ( -0.8661417322834640276, -0.1870078740157480601, -0.3641732283464567677 ) ) ;
#54414=CARTESIAN_POINT ( 'NONE',  ( 0.8989501312335963501, -0.6692913385826773087, -0.1292274648535924053 ) ) ;
#54415=CARTESIAN_POINT ( 'NONE',  ( 0.1115485564304467270, -0.6692913385826773087, -0.1292274648535924053 ) ) ;
#54417=CARTESIAN_POINT ( 'NONE',  ( -0.01193304242178637453, 5.354677644401852583E-19, -0.3627985898453510716 ) ) ;
#54419=CARTESIAN_POINT ( 'NONE',  ( 0.6758530183727039509, -0.6692913385826771977, 0.1292274648535927661 ) ) ;
#54420=CARTESIAN_POINT ( 'NONE',  ( 0.1181102362204730916, -0.6692913385826771977, 8.415575281601705876E-17 ) ) ;
#54421=CARTESIAN_POINT ( 'NONE',  ( -1.122047244094487306, 0.1660481256975883668, -0.3530559997133364547 ) ) ;
#54422=VECTOR ( 'NONE', #62941, 39.37007874015748143 ) ;
#54423=CARTESIAN_POINT ( 'NONE',  ( 1.082677165354331228, -0.5400638737290844871, 0.3530559997133364547 ) ) ;
#54424=CARTESIAN_POINT ( 'NONE',  ( 0.3412073490813655186, -0.6046776061558809534, -0.2411417322834644161 ) ) ;
#54426=CARTESIAN_POINT ( 'NONE',  ( -0.1837270341207343505, -0.6046776061558807314, 0.2411417322834647770 ) ) ;
#54427=CARTESIAN_POINT ( 'NONE',  ( 0.7152230971128616943, -0.05778040916215522460, 0.4822834645669289988 ) ) ;
#54428=CARTESIAN_POINT ( 'NONE',  ( 0.1246719160104994284, 0.2952755905511810774, -0.1292274648535930714 ) ) ;
#54429=CARTESIAN_POINT ( 'NONE',  ( 0.8727034120734913358, -0.08942795157527998196, 0.3641732283464567121 ) ) ;
#54430=CARTESIAN_POINT ( 'NONE',  ( -1.292650918635170010, -0.6692913385826771977, 0.1292274648535927661 ) ) ;
#54432=CARTESIAN_POINT ( 'NONE',  ( 0.2362204724409456558, -0.1870078740157480879, -0.4822834645669291653 ) ) ;
#54433=LENGTH_MEASURE_WITH_UNIT ( LENGTH_MEASURE( 0.02539999999999999897 ), #3106 );
#54436=VERTEX_POINT ( 'NONE', #52370 ) ;
#54437=CARTESIAN_POINT ( 'NONE',  ( 0.9186351706036752773, 0.2306618581243847221, -0.2411417322834647770 ) ) ;
#54438=CARTESIAN_POINT ( 'NONE',  ( 0.6299212598425204535, -0.1870078740157479769, 0.3641732283464567677 ) ) ;
#54439=B_SPLINE_CURVE_WITH_KNOTS ( 'NONE', 3,
 ( #79595, #2144, #52637, #20673 ),
 .UNSPECIFIED., .F., .F.,
 ( 4, 4 ),
 ( 3.210432057756949332E-07, 0.001287787053612054989 ),
 .UNSPECIFIED. ) ;
#54441=CARTESIAN_POINT ( 'NONE',  ( 0.6199123404867349363, 8.471767977567108961E-16, -0.4445507791589058955 ) ) ;
#54446=CARTESIAN_POINT ( 'NONE',  ( -0.8530183727034112984, 0.05413385826771666132, 0.4176697321401328100 ) ) ;
#54447=CARTESIAN_POINT ( 'NONE',  ( -0.6627296587926503335, -0.6692913385826771977, 0.1292274648535927661 ) ) ;
#54448=CARTESIAN_POINT ( 'NONE',  ( 0.8136482939632553313, 0.2306618581243848609, 0.2411417322834645549 ) ) ;
#54449=ORIENTED_EDGE ( 'NONE', *, *, #31652, .T. ) ;
#54450=CARTESIAN_POINT ( 'NONE',  ( 1.338582677165355062, -0.1870078740157480879, -0.4822834645669291653 ) ) ;
#54451=CARTESIAN_POINT ( 'NONE',  ( 1.673228346456693494, 0.07958543189024085140, 0.2665933059059887866 ) ) ;
#54453=DIRECTION ( 'NONE',  ( 0.000000000000000000, 0.000000000000000000, -1.000000000000000000 ) ) ;
#54455=CARTESIAN_POINT ( 'NONE',  ( -1.213910761154854745, -0.5511811023622046335, 0.09757992244046803654 ) ) ;
#54457=CARTESIAN_POINT ( 'NONE',  ( 0.07874015748031558404, -0.1870078740157479769, 0.4822834645669291653 ) ) ;
#54458=CARTESIAN_POINT ( 'NONE',  ( 1.384514435695538559, 0.2952755905511810774, -0.1292274648535930714 ) ) ;
#54460=CARTESIAN_POINT ( 'NONE',  ( -1.043307086614172707, 0.07958543189024071263, -0.2665933059059888421 ) ) ;
#54461=CARTESIAN_POINT ( 'NONE',  ( 0.9383202099737538715, -0.05778040916215560624, -0.4822834645669293319 ) ) ;
#54462=CARTESIAN_POINT ( 'NONE',  ( 1.161417322834646271, 0.07958543189024071263, -0.2665933059059888421 ) ) ;
#54463=EDGE_CURVE ( 'NONE', #2914, #1754, #63281, .T. ) ;
#54465=CARTESIAN_POINT ( 'NONE',  ( -1.351706036745406347, -0.004921259842519870586, -0.3153832671262229437 ) ) ;
#54466=CARTESIAN_POINT ( 'NONE',  ( 1.338582677165355062, -0.1870078740157479769, 0.4822834645669291653 ) ) ;
#54468=CARTESIAN_POINT ( 'NONE',  ( -0.07874015748031421014, -0.1870078740157480879, -0.4822834645669291653 ) ) ;
#54469=CARTESIAN_POINT ( 'NONE',  ( -1.450131233595799651, 0.1771653543307087075, -0.09757992244046823083 ) ) ;
#54470=CARTESIAN_POINT ( 'NONE',  ( -0.1837270341207343505, -0.5023911411419708095, 0.1820866141732285504 ) ) ;
#54471=CARTESIAN_POINT ( 'NONE',  ( -0.6889763779527552368, -0.5400638737290845981, -0.3530559997133363437 ) ) ;
#54472=CARTESIAN_POINT ( 'NONE',  ( -1.607611548556429737, 0.1771653543307087075, -0.09757992244046823083 ) ) ;
#54474=CARTESIAN_POINT ( 'NONE',  ( 0.2493438320209980519, -0.4281496062992127816, -0.4176697321401328100 ) ) ;
#54478=CARTESIAN_POINT ( 'NONE',  ( -1.108923884514435132, -0.3162353388693405765, 0.4822834645669290543 ) ) ;
#54479=CARTESIAN_POINT ( 'NONE',  ( -0.6036745406824141069, 0.1283753931104748280, 0.1820866141732283561 ) ) ;
#54480=CARTESIAN_POINT ( 'NONE',  ( 1.220472440944882386, 1.277248692536265747E-15, -0.4445507791589058955 ) ) ;
#54481=CARTESIAN_POINT ( 'NONE',  ( 0.06561679790026316017, -0.4281496062992124485, 0.4176697321401328655 ) ) ;
#54482=CARTESIAN_POINT ( 'NONE',  ( 0.3412073490813655186, -0.5023911411419708095, -0.1820866141732282451 ) ) ;
#54483=CARTESIAN_POINT ( 'NONE',  ( -0.8989501312335946848, 0.1771653543307087075, -0.09757992244046823083 ) ) ;
#54484=CARTESIAN_POINT ( 'NONE',  ( -1.010498687664041384, -0.4281496062992127816, -0.4176697321401328100 ) ) ;
#54485=CARTESIAN_POINT ( 'NONE',  ( -1.535433070866141225, 0.2952755905511811885, 0.000000000000000000 ) ) ;
#54486=CARTESIAN_POINT ( 'NONE',  ( 1.581364829396326277, -0.3162353388693409650, -0.4822834645669289433 ) ) ;
#54488=CARTESIAN_POINT ( 'NONE',  ( 0.8792650918635177559, -0.004921259842519576551, 0.3153832671262227771 ) ) ;
#54489=CARTESIAN_POINT ( 'NONE',  ( 0.9186351706036752773, 0.2306618581243847221, -0.2411417322834647770 ) ) ;
#54491=CARTESIAN_POINT ( 'NONE',  ( 1.515748031496063186, -0.4536011799217368745, -0.2665933059059886201 ) ) ;
#54492=ORIENTED_EDGE ( 'NONE', *, *, #15723, .T. ) ;
#54493=CARTESIAN_POINT ( 'NONE',  ( -0.9317585301837263412, -0.4281496062992127816, -0.4176697321401328100 ) ) ;
#54494=CARTESIAN_POINT ( 'NONE',  ( -1.023622047244093558, -0.1870078740157479769, 0.4822834645669291653 ) ) ;
#54495=CARTESIAN_POINT ( 'NONE',  ( 0.5183727034120741983, 0.2952755905511810774, -0.1292274648535930714 ) ) ;
#54496=CARTESIAN_POINT ( 'NONE',  ( -1.489501312335957062, -0.2845877964562161244, -0.3641732283464567121 ) ) ;
#54498=CARTESIAN_POINT ( 'NONE',  ( 1.430446194225722500, -0.004921259842519576551, 0.3153832671262227771 ) ) ;
#54499=CARTESIAN_POINT ( 'NONE',  ( 0.2493438320209980519, 0.05413385826771666132, 0.4176697321401328100 ) ) ;
#54500=CARTESIAN_POINT ( 'NONE',  ( 0.8202099737532813073, 0.2952755905511811885, 0.1292274648535926551 ) ) ;
#54504=CARTESIAN_POINT ( 'NONE',  ( -1.586052503253848167, 1.023622047244095556, -0.1653254495020564929 ) ) ;
#54506=CARTESIAN_POINT ( 'NONE',  ( -0.2690288713910754526, 0.1771653543307087075, -0.09757992244046823083 ) ) ;
#54507=CARTESIAN_POINT ( 'NONE',  ( -0.1902887139107604098, -0.6692913385826771977, 0.1292274648535927661 ) ) ;
#54508=CARTESIAN_POINT ( 'NONE',  ( 0.7414698162729663755, -0.6692913385826773087, -0.1292274648535924053 ) ) ;
#54510=CARTESIAN_POINT ( 'NONE',  ( -0.01968503937007793844, 0.07958543189024071263, -0.2665933059059888421 ) ) ;
#54511=CARTESIAN_POINT ( 'NONE',  ( -1.351706036745406347, -0.4281496062992124485, 0.4176697321401328655 ) ) ;
#54512=CARTESIAN_POINT ( 'NONE',  ( 1.377952755905512472, -0.6692913385826771977, 8.415575281601705876E-17 ) ) ;
#54518=CARTESIAN_POINT ( 'NONE',  ( 1.181102362204724976, -0.1870078740157480879, -0.4822834645669291653 ) ) ;
#54519=CARTESIAN_POINT ( 'NONE',  ( -1.614173228346456268, -0.6692913385826771977, 8.415575281601705876E-17 ) ) ;
#54520=CARTESIAN_POINT ( 'NONE',  ( -1.233595800524933894, -0.5023911411419708095, -0.1820866141732282451 ) ) ;
#54521=CARTESIAN_POINT ( 'NONE',  ( 1.496062992125984703, -0.1870078740157480879, -0.4822834645669291653 ) ) ;
#54523=CARTESIAN_POINT ( 'NONE',  ( 1.191801538614238209, 4.598214627222820490E-16, 0.4118484887281966822 ) ) ;
#54524=CARTESIAN_POINT ( 'NONE',  ( 1.253280839895013710, -0.05778040916215560624, -0.4822834645669293319 ) ) ;
#54525=CARTESIAN_POINT ( 'NONE',  ( -1.509186351706035767, 0.05413385826771626580, -0.4176697321401330321 ) ) ;
#54526=CARTESIAN_POINT ( 'NONE',  ( 0.07874015748031558404, -0.1870078740157480879, -0.4822834645669291653 ) ) ;
#54527=CARTESIAN_POINT ( 'NONE',  ( -0.6758530183727028406, -0.6692913385826773087, -0.1292274648535924053 ) ) ;
#54528=CARTESIAN_POINT ( 'NONE',  ( -1.581364829396324945, -0.05778040916215560624, -0.4822834645669293319 ) ) ;
#54530=CARTESIAN_POINT ( 'NONE',  ( 0.3477690288713918276, 0.2952755905511811885, 0.1292274648535926551 ) ) ;
#54532=CARTESIAN_POINT ( 'NONE',  ( -1.450131233595799651, 0.1771653543307087075, -0.09757992244046823083 ) ) ;
#54538=CARTESIAN_POINT ( 'NONE',  ( -1.607611548556429737, -0.6692913385826771977, 0.1292274648535927661 ) ) ;
#54541=CARTESIAN_POINT ( 'NONE',  ( -1.594488188976377563, -0.5400638737290844871, 0.3530559997133364547 ) ) ;
#54543=CARTESIAN_POINT ( 'NONE',  ( 0.9348729704079946634, -8.644661201599092366E-16, -0.4445507791589066171 ) ) ;
#54545=CARTESIAN_POINT ( 'NONE',  ( -0.4855643044619415427, -0.004921259842519870586, -0.3153832671262229437 ) ) ;
#54546=CARTESIAN_POINT ( 'NONE',  ( -0.8398950131233589023, -0.5023911411419708095, -0.1820866141732282451 ) ) ;
#54547=CARTESIAN_POINT ( 'NONE',  ( -1.174540682414697335, -0.05778040916215522460, 0.4822834645669289988 ) ) ;
#54548=CARTESIAN_POINT ( 'NONE',  ( 0.4396325459317590445, -0.6692913385826771977, 0.1292274648535927661 ) ) ;
#54549=CARTESIAN_POINT ( 'NONE',  ( -1.437007874015747477, 0.1660481256975883668, -0.3530559997133364547 ) ) ;
#54551=EDGE_LOOP ( 'NONE', ( #35505, #52625, #11693, #75882, #3395, #79203, #66898, #20487, #68621, #25634, #37116, #70555, #35178, #61460, #65103, #61388, #14088, #4109, #10019, #99, #13340, #55537, #4306, #81760, #26177, #42520, #14808, #4870, #279, #42223 ) ) ;
#54552=CARTESIAN_POINT ( 'NONE',  ( -1.220472440944881054, -0.6692913385826771977, 8.415575281601705876E-17 ) ) ;
#54553=CARTESIAN_POINT ( 'NONE',  ( -1.614173228346457378, 1.606230626554505658, 0.1372047244094476981 ) ) ;
#54556=CARTESIAN_POINT ( 'NONE',  ( -1.614173228346457378, 0.2753471884572478157, -0.1372047244094478091 ) ) ;
#54559=DIRECTION ( 'NONE',  ( 1.692413147294446216E-16, -0.000000000000000000, 1.000000000000000000 ) ) ;
#54560=CARTESIAN_POINT ( 'NONE',  ( -0.7152230971128602510, -0.3162353388693405765, 0.4822834645669290543 ) ) ;
#54561=CARTESIAN_POINT ( 'NONE',  ( 1.601049868766404982, -0.6046776061558809534, -0.2411417322834644161 ) ) ;
#54562=CARTESIAN_POINT ( 'NONE',  ( -1.509186351706035767, 0.05413385826771626580, -0.4176697321401330321 ) ) ;
#54565=CARTESIAN_POINT ( 'NONE',  ( -1.404199475065615932, 0.05413385826771666132, 0.4176697321401328100 ) ) ;
#54566=CARTESIAN_POINT ( 'NONE',  ( -0.9908136482939626788, -0.6692913385826773087, -0.1292274648535924053 ) ) ;
#54569=CARTESIAN_POINT ( 'NONE',  ( 0.6430446194225728496, -0.004921259842519576551, 0.3153832671262227771 ) ) ;
#54571=CARTESIAN_POINT ( 'NONE',  ( 0.06561679790026316017, -0.3690944881889763329, 0.3153832671262228327 ) ) ;
#54572=CARTESIAN_POINT ( 'NONE',  ( 0.9317585301837276734, -0.3690944881889763329, 0.3153832671262228327 ) ) ;
#54573=CARTESIAN_POINT ( 'NONE',  ( 1.010498687664042716, 0.05413385826771626580, -0.4176697321401330321 ) ) ;
#54575=CARTESIAN_POINT ( 'NONE',  ( -0.2952755905511803003, -0.4536011799217368745, -0.2665933059059886201 ) ) ;
#54577=CARTESIAN_POINT ( 'NONE',  ( -1.489501312335957062, -0.05778040916215522460, 0.4822834645669289988 ) ) ;
#54578=CIRCLE ( 'NONE', #15680, 1.220472440944881942 ) ;
#54579=CARTESIAN_POINT ( 'NONE',  ( -1.122047244094487306, 0.07958543189024071263, -0.2665933059059888421 ) ) ;
#54582=CONICAL_SURFACE ( 'NONE', #23635, 1.220472440944881942, 0.7853981633974621568 ) ;
#54583=CARTESIAN_POINT ( 'NONE',  ( -0.03937007874015669567, -0.6692913385826771977, 8.415575281601705876E-17 ) ) ;
#54584=CARTESIAN_POINT ( 'NONE',  ( -0.07217847769028787330, -0.05778040916215522460, 0.4822834645669289988 ) ) ;
#54585=CARTESIAN_POINT ( 'NONE',  ( 1.482939632545932307, -0.3690944881889763329, 0.3153832671262228327 ) ) ;
#54586=CARTESIAN_POINT ( 'NONE',  ( 0.4593175853018379162, -0.3690944881889763329, 0.3153832671262228327 ) ) ;
#54587=CARTESIAN_POINT ( 'NONE',  ( -0.1377952755905504645, 0.07958543189024085140, 0.2665933059059887866 ) ) ;
#54588=CARTESIAN_POINT ( 'NONE',  ( -0.6955380577427815458, 0.05413385826771666132, 0.4176697321401328100 ) ) ;
#54591=CARTESIAN_POINT ( 'NONE',  ( 0.2230971128608932319, -0.4281496062992124485, 0.4176697321401328655 ) ) ;
#54593=DIRECTION ( 'NONE',  ( 0.000000000000000000, 0.000000000000000000, 1.000000000000000000 ) ) ;
#54594=CARTESIAN_POINT ( 'NONE',  ( -0.3674540682414692561, -0.5023911411419708095, -0.1820866141732282451 ) ) ;
#54595=AXIS2_PLACEMENT_3D ( 'NONE', #50403, #31463, #49584 ) ;
#54596=CARTESIAN_POINT ( 'NONE',  ( -0.1049868766404193215, 0.2306618581243847221, -0.2411417322834647770 ) ) ;
#54597=CARTESIAN_POINT ( 'NONE',  ( -1.653543307086613234, -0.1870078740157479769, 0.4822834645669291653 ) ) ;
#54598=CARTESIAN_POINT ( 'NONE',  ( -1.463254593175852492, 0.1771653543307087630, 0.09757992244046791164 ) ) ;
#54599=CARTESIAN_POINT ( 'NONE',  ( 1.167979002624672580, -0.4281496062992124485, 0.4176697321401328655 ) ) ;
#54601=CARTESIAN_POINT ( 'NONE',  ( -0.4724409448818890911, -0.1870078740157479769, 0.3641732283464567677 ) ) ;
#54605=CARTESIAN_POINT ( 'NONE',  ( 1.692913385826772421, 0.1771653543307087630, 0.000000000000000000 ) ) ;
#54606=CARTESIAN_POINT ( 'NONE',  ( 1.089238845144357537, -0.3690944881889763329, 0.3153832671262228327 ) ) ;
#54608=CARTESIAN_POINT ( 'NONE',  ( 0.7283464566929140904, -0.5400638737290845981, -0.3530559997133363437 ) ) ;
#54610=CARTESIAN_POINT ( 'NONE',  ( 1.056430446194226658, 0.1771653543307087630, 0.09757992244046791164 ) ) ;
#54611=CARTESIAN_POINT ( 'NONE',  ( 0.2690288713910767848, 0.2952755905511811885, 0.1292274648535926551 ) ) ;
#54612=CARTESIAN_POINT ( 'NONE',  ( -0.9645669291338575535, 0.1660481256975883668, -0.3530559997133364547 ) ) ;
#54616=CARTESIAN_POINT ( 'NONE',  ( 0.3543307086614179147, 0.1771653543307087630, 0.000000000000000000 ) ) ;
#54619=ORIENTED_EDGE ( 'NONE', *, *, #9980, .F. ) ;
#54620=CARTESIAN_POINT ( 'NONE',  ( -0.6364829396325453192, -0.3162353388693405765, 0.4822834645669290543 ) ) ;
#54621=CARTESIAN_POINT ( 'NONE',  ( -0.3543307086614165824, 0.2952755905511811885, 0.000000000000000000 ) ) ;
#54622=CARTESIAN_POINT ( 'NONE',  ( -0.2559055118110227234, -0.4536011799217367080, 0.2665933059059888421 ) ) ;
#54623=CARTESIAN_POINT ( 'NONE',  ( 0.6496062992125991586, -0.5400638737290845981, -0.3530559997133363437 ) ) ;
#54624=CARTESIAN_POINT ( 'NONE',  ( -0.7349081364829387342, -0.6046776061558807314, 0.2411417322834647770 ) ) ;
#54625=CARTESIAN_POINT ( 'NONE',  ( -0.2559055118110230564, 0.1660481256975883668, -0.3530559997133364547 ) ) ;
#54626=CARTESIAN_POINT ( 'NONE',  ( 0.9842519685039375910, 0.2952755905511811885, 0.000000000000000000 ) ) ;
#54627=CARTESIAN_POINT ( 'NONE',  ( 1.010498687664042716, 0.05413385826771626580, -0.4176697321401330321 ) ) ;
#54628=CARTESIAN_POINT ( 'NONE',  ( 0.7874015748031503170, -0.1870078740157480879, -0.4822834645669291653 ) ) ;
#54630=CARTESIAN_POINT ( 'NONE',  ( -0.1640419947506553400, -0.08942795157528024563, -0.3641732283464568787 ) ) ;
#54631=ORIENTED_EDGE ( 'NONE', *, *, #27901, .F. ) ;
#54635=CARTESIAN_POINT ( 'NONE',  ( -0.8267716535433065062, -0.5511811023622047445, 6.969142054262312111E-17 ) ) ;
#54636=AXIS2_PLACEMENT_3D ( 'NONE', #4906, #42369, #62567 ) ;
#54637=VECTOR ( 'NONE', #66695, 39.37007874015748143 ) ;
#54638=CARTESIAN_POINT ( 'NONE',  ( -0.6430446194225712953, 0.05413385826771626580, -0.4176697321401330321 ) ) ;
#54639=CARTESIAN_POINT ( 'NONE',  ( 0.7754685323813633735, -1.606403293320555582E-18, -0.3627985898453514046 ) ) ;
#54640=CARTESIAN_POINT ( 'NONE',  ( -0.3280839895013117347, -0.4281496062992124485, 0.4176697321401328655 ) ) ;
#54641=CARTESIAN_POINT ( 'NONE',  ( -0.5708661417322828946, 0.1660481256975883668, -0.3530559997133364547 ) ) ;
#54642=CARTESIAN_POINT ( 'NONE',  ( -1.108923884514435132, -0.05778040916215560624, -0.4822834645669293319 ) ) ;
#54643=CARTESIAN_POINT ( 'NONE',  ( -1.253280839895012377, -0.05778040916215522460, 0.4822834645669289988 ) ) ;
#54644=CARTESIAN_POINT ( 'NONE',  ( 0.8595800524934390507, -0.2845877964562159024, 0.3641732283464567677 ) ) ;
#54647=CARTESIAN_POINT ( 'NONE',  ( 0.3346456692913390985, 0.07958543189024085140, 0.2665933059059887866 ) ) ;
#54648=CARTESIAN_POINT ( 'NONE',  ( -0.07874015748031421014, -0.1870078740157479769, 0.4822834645669291653 ) ) ;
#54649=CARTESIAN_POINT ( 'NONE',  ( 0.4986876640419954376, -0.6046776061558809534, -0.2411417322834644161 ) ) ;
#54655=CARTESIAN_POINT ( 'NONE',  ( -0.7152230971128602510, -0.08942795157528024563, -0.3641732283464568787 ) ) ;
#54656=CARTESIAN_POINT ( 'NONE',  ( -1.135170603674539924, -0.6692913385826771977, 0.1292274648535927661 ) ) ;
#54659=CARTESIAN_POINT ( 'NONE',  ( 1.541994750656168645, 0.2952755905511810774, -0.1292274648535930714 ) ) ;
#54660=CARTESIAN_POINT ( 'NONE',  ( 0.6692913385826777528, 0.2952755905511811885, 0.000000000000000000 ) ) ;
#54661=CARTESIAN_POINT ( 'NONE',  ( 0.6758530183727039509, -0.6692913385826771977, 0.1292274648535927661 ) ) ;
#54662=CARTESIAN_POINT ( 'NONE',  ( -0.4461942257217840213, -0.5023911411419708095, -0.1820866141732282451 ) ) ;
#54663=CARTESIAN_POINT ( 'NONE',  ( 0.01312335958005323398, 0.05413385826771666132, 0.4176697321401328100 ) ) ;
#54665=CARTESIAN_POINT ( 'NONE',  ( -0.6233595800524928121, -0.2845877964562161244, -0.3641732283464567121 ) ) ;
#54666=CARTESIAN_POINT ( 'NONE',  ( -0.2755905511811018171, 0.2952755905511811885, 0.000000000000000000 ) ) ;
#54668=CARTESIAN_POINT ( 'NONE',  ( -1.601049868766403650, -0.6046776061558807314, 0.2411417322834647770 ) ) ;
#54669=CARTESIAN_POINT ( 'NONE',  ( -0.1115485564304456306, 0.1771653543307087075, -0.09757992244046823083 ) ) ;
#54670=CARTESIAN_POINT ( 'NONE',  ( 1.660104986876641320, -0.08942795157527998196, 0.3641732283464567121 ) ) ;
#54671=CARTESIAN_POINT ( 'NONE',  ( -1.122047244094487306, -0.5400638737290844871, 0.3530559997133364547 ) ) ;
#54672=CARTESIAN_POINT ( 'NONE',  ( -0.8989501312335946848, -0.5511811023622046335, 0.09757992244046803654 ) ) ;
#54674=CARTESIAN_POINT ( 'NONE',  ( -1.220472440944881054, 0.2952755905511811885, 0.000000000000000000 ) ) ;
#54675=CARTESIAN_POINT ( 'NONE',  ( -0.5577427821522301654, -0.3162353388693405765, 0.4822834645669290543 ) ) ;
#54677=CARTESIAN_POINT ( 'NONE',  ( 0.4133858267716541968, 0.1660481256975885056, 0.3530559997133364547 ) ) ;
#54680=CARTESIAN_POINT ( 'NONE',  ( 0.5052493438320218022, -0.5511811023622048555, -0.09757992244046775898 ) ) ;
#54681=CARTESIAN_POINT ( 'NONE',  ( 1.043307086614173818, -0.5400638737290845981, -0.3530559997133363437 ) ) ;
#54682=CARTESIAN_POINT ( 'NONE',  ( -1.404199475065615932, -0.004921259842519576551, 0.3153832671262227771 ) ) ;
#54683=( BOUNDED_SURFACE ( )  B_SPLINE_SURFACE ( 1, 2, ( 
 ( #62404, #68329, #3933, #29591, #67914, #17809, #81789, #10250, #36323, #55254, #23276, #30000, #16989, #55664, #42632, #23686, #49360, #17404, #36728, #33232, #34054, #41201, #8389, #40371, #27738, #66465, #71527, #39962, #66052, #27318, #7128, #65222, #45828, #26491, #32802, #39534, #8800, #20178, #52561, #72774, #26902, #13874, #2073, #2493, #47084, #59718, #72368, #79521, #79111, #52978, #60142, #34476, #15125, #7560, #40779, #53403, #46675, #14717, #58894, #47499, #59304, #52143, #1661, #58469, #28153, #21014, #14302, #78270, #53808, #21429, #65649, #21836, #73192, #15542, #77849, #1254, #833, #20601, #46254, #71949, #7978, #33642, #78691, #42423, #54224, #55874, #9219, #62204, #15960, #34892, #3313, #60554, #30212, #81169, #3728, #42834, #36529, #2904, #55052, #28568, #80759, #35300, #74859, #49568, #73618, #74023, #75264, #28977, #16369, #4541, #74439, #29392, #41607, #10468, #48326, #61794, #22255, #9630, #36121, #67296, #17201, #4134, #42016, #67709, #68527, #81586, #60962, #54644, #10868, #10046, #80354, #29799, #22667, #35709, #47913, #55460, #23903, #23487, #17607, #66889, #79941, #61379, #23073, #48741, #16786, #68123, #49153, #25539, #24308, #30632, #76902, #69353, #12516, #70163, #18428, #82400, #82803, #32278, #19232, #77322, #4965, #62622, #31445, #56701, #38177, #51617, #25959, #304, #44882, #81994, #76084, #44070, #38594, #11285, #63852, #63034, #56297, #5372, #69762, #43239, #31033, #68936, #11707, #75676, #6189, #36945, #25127, #37362, #49978, #18016, #57938, #31867, #76498, #6607, #43651, #12936, #24718, #50387, #50797, #12107, #18826, #37765, #63440, #83218, #64272, #57109, #5776, #44472, #57527, #51205, #70582, #78168, #8705, #726, #77747, #45730, #71426, #52042, #26384, #20080, #33957, #1564, #20915, #8289, #13773, #39430, #1973, #65546, #65953, #46570, #65116, #7453, #33123, #59619, #59203, #7877, #58793, #79011, #1151, #71848, #20499, #21331, #40682, #39005, #78590, #2397, #13352, #32697, #26802, #72268, #53712, #14616, #52879, #40270, #46983, #52460, #46153, #27637, #39855, #19651, #14198, #58363, #64689, #45313, #33541, #72677, #27218, #53299, #15026, #66368, #34376, #60041, #28054, #71008, #7028, #61280, #68439, #68028, #41921, #49061, #23394, #4044, #79842, #61704, #54963, #35617, #3633, #54128, #36439, #48237, #15444, #73933, #30120, #29709, #9945, #3220, #15869, #74760, #80670, #28883, #48649, #17109, #55372, #41104, #66792, #42743, #62112, #10779, #2808, #41517, #81078, #4455, #22983, #9127, #79419, #21739, #47404, #28467, #73093, #67202, #34798, #60457, #10372, #16276, #22159, #47819, #73520, #67615, #9534, #29301, #35205, #60867, #54545, #80260, #22576, #74345, #16690, #42329, #36030, #63346, #75992, #4864, #63755, #44787, #76402, #81490, #44376, #25443, #17517, #70483, #25031, #43149, #6096, #31770, #57431, #12840, #69671, #68846, #5279, #55782, #56608, #51109, #83124, #57016, #43974, #38499, #23806, #49479, #82308, #76806, #19137, #56202, #38081, #31350, #12014, #37668, #30538, #64181, #24628, #75172, #50294, #6515, #11194, #5681, #62944, #75586, #36853, #82712, #30941, #50704, #62526, #81903, #24214, #49885, #17925, #43561, #69262, #11609, #37268, #18334, #18734, #70068, #12423, #22375, #57840, #28685, #64592, #208, #51943, #25861, #80057, #47617, #52360, #9334, #3018, #51521, #20397, #77224, #46049, #626, #41321, #16072, #38912, #39326, #41718, #77648, #65012, #54346, #40901, #78066, #6928, #67002, #48035, #53928, #19553, #21958, #73737, #45212, #67411, #2609, #70913, #35005, #60670, #32185, #13262, #71743, #32599, #7347, #58262, #33015, #26282, #19981, #34595, #15241, #45631, #71326, #13674, #58685, #1050, #26704, #66582, #8918, #60260, #28266, #79640, #73313, #15660, #43761, #10979, #42946, #30325, #69050, #74142, #42543, #68640, #29911, #9745, #67828, #48442, #29094, #35416, #42133, #11399, #22782, #55167, #75373, #29506, #16487, #4652, #5076, #49681, #36639, #74973, #82107, #81703, #55575, #62740, #17318, #62315, #24013, #10167, #35832, #17722, #81285, #55991, #43348, #61499, #3846, #80876, #37056, #49270 ),
 ( #30745, #68246, #10580, #56408, #24420, #23188, #48859, #50090, #36237, #74559, #75786, #16905, #61907, #4249, #18128, #61081, #3432, #54766, #80470, #23601, #82922, #18537, #25243, #37471, #44180, #19355, #51739, #50496, #56812, #19775, #12225, #38710, #13056, #44586, #50907, #25657, #58484, #45429, #20193, #31146, #5485, #57642, #76608, #64388, #77864, #52160, #26506, #71124, #24827, #18938, #70280, #64805, #63144, #6724, #5891, #82511, #31563, #12633, #69466, #57221, #11819, #37882, #69872, #32394, #76199, #51319, #63557, #38292, #63969, #849, #58057, #45004, #32817, #6305, #39124, #31982, #5, #77022, #70704, #423, #26079, #77442, #13467, #7144, #59735, #45844, #71964, #34071, #1269, #20617, #21030, #34909, #26917, #46269, #14319, #39977, #78286, #52577, #65667, #60158, #2089, #59320, #15140, #54243, #28587, #2923, #21853, #7993, #78706, #46690, #41219, #13890, #72790, #33657, #33248, #1676, #72383, #79960, #27333, #71543, #52993, #14733, #40796, #39549, #27754, #40385, #7576, #58910, #60572, #66481, #79127, #9237, #66068, #15559, #65238, #8404, #53418, #21444, #47101, #8816, #34493, #2510, #66906, #28169, #53826, #79540, #47517, #73209, #80372, #80777, #11306, #3331, #22685, #48344, #74041, #54661, #28995, #16388, #36548, #4153, #23506, #10888, #42035, #67729, #4562, #68142, #68547, #49173, #10064, #35727, #61397, #62224, #61813, #10487, #3746, #81607, #29410, #74459, #23093, #74878, #55069, #17222, #60981, #48760, #42854, #16806, #30233, #55895, #42442, #36141, #23923, #43259, #29818, #55479, #49589, #81189, #75284, #17627, #68956, #36965, #62642, #4986, #30653, #56317, #22273, #47933, #73636, #15978, #41625, #67314, #9649, #35318, #31885, #64290, #63054, #69374, #32296, #24739, #51224, #25557, #57129, #37786, #38195, #71026, #57956, #32716, #43671, #18037, #37383, #56723, #82824, #13370, #5392, #82420, #50407, #76105, #31054, #18448, #44090, #12954, #63870, #83236, #70600, #69784, #12129, #6624, #44492, #44902, #76922, #63463, #5797, #31467, #38612, #6208, #70183, #25148, #324, #50816, #76517, #18846, #19250, #12536, #25978, #57545, #51636, #77341, #19670, #45331, #39023, #64707, #7047, #82015, #24329, #49999, #75696, #11727, #59220, #33141, #53316, #20517, #65562, #39448, #79028, #53727, #47000, #21754, #47417, #15459, #71865, #7472, #14215, #26403, #58812, #8306, #40697, #65136, #45748, #8719, #1169, #27653, #1990, #33557, #39873, #14632, #73108, #34390, #9141, #20097, #77765, #46588, #7896, #21347, #66807, #41117, #58383, #60056, #13791, #1581, #27236, #79435, #52059, #72694, #78186, #71443, #46169, #52895, #744, #78608, #26820, #52478, #20931, #15041, #72286, #40288, #65969, #33973, #59634, #66382, #2411, #28069, #81502, #73537, #4467, #34812, #28483, #42344, #15882, #74360, #73946, #43161, #74774, #30132, #48662, #60471, #60883, #22997, #55795, #54143, #16703, #79857, #68042, #3234, #42757, #17530, #41530, #41935, #68857, #54560, #67631, #23823, #10388, #54976, #67216, #68452, #49492, #55384, #2822, #23407, #75184, #22174, #47832, #4055, #9549, #10791, #36451, #62125, #35219, #36045, #28898, #9962, #80275, #35633, #22589, #48250, #61717, #29722, #16291, #61294, #3650, #29315, #80683, #81090, #49074, #17123, #77236, #4878, #24227, #37281, #38093, #45225, #12433, #44387, #31780, #70494, #75597, #43987, #70080, #31363, #11206, #69273, #49899, #30552, #36865, #43572, #12852, #17936, #56620, #76816, #30953, #11619, #6107, #6527, #51121, #63767, #76414, #220, #83135, #57028, #64192, #38510, #19148, #62956, #44799, #57442, #50716, #18744, #5293, #51533, #63358, #56218, #5692, #62540, #32197, #25042, #18346, #82320, #57853, #25454, #69683, #25871, #19565, #81916, #24639, #50306, #76004, #12026, #37683, #82722, #33028, #53203, #78916, #46477, #58273, #59946, #27962, #20824, #21237, #51954, #638, #46893, #13684, #40181, #14530, #46061, #19991, #71337, #72587, #71754, #45642, #65865, #58697, #78078, #77660, #8200, #66275, #59529, #34285, #2302, #53621, #1062, #33865, #1886, #27546, #79329, #72173, #14934, #39337, #26294, #40593, #65024, #8615 ) ),
 .UNSPECIFIED., .F., .F., .F. ) 
 B_SPLINE_SURFACE_WITH_KNOTS ( ( 2, 2 ),
 ( 3, 2, 2, 2, 2, 2, 2, 2, 2, 2, 2, 2, 2, 2, 2, 2, 2, 2, 2, 2, 2, 2, 2, 2, 2, 2, 2, 2, 2, 2, 2, 2, 2, 2, 2, 2, 2, 2, 2, 2, 2, 2, 2, 2, 2, 2, 2, 2, 2, 2, 2, 2, 2, 2, 2, 2, 2, 2, 2, 2, 2, 2, 2, 2, 2, 2, 2, 2, 2, 2, 2, 2, 2, 2, 2, 2, 2, 2, 2, 2, 2, 2, 2, 2, 2, 2, 2, 2, 2, 2, 2, 2, 2, 2, 2, 2, 2, 2, 2, 2, 2, 2, 2, 2, 2, 2, 2, 2, 2, 2, 2, 2, 2, 2, 2, 2, 2, 2, 2, 2, 2, 2, 2, 2, 2, 2, 2, 2, 2, 2, 2, 2, 2, 2, 2, 2, 2, 2, 2, 2, 2, 2, 2, 2, 2, 2, 2, 2, 2, 2, 2, 2, 2, 2, 2, 2, 2, 2, 2, 2, 2, 2, 2, 2, 2, 2, 2, 2, 2, 2, 2, 2, 2, 2, 2, 2, 2, 2, 2, 2, 2, 2, 2, 2, 2, 2, 2, 2, 2, 2, 2, 2, 2, 2, 2, 2, 2, 2, 2, 2, 2, 2, 2, 2, 2, 2, 2, 2, 2, 2, 2, 2, 2, 2, 2, 2, 2, 2, 2, 2, 2, 2, 2, 2, 2, 2, 2, 2, 2, 2, 2, 2, 2, 2, 2, 2, 2, 2, 2, 2, 2, 2, 2, 2, 2, 2, 2, 2, 2, 2, 2, 2, 2, 2, 2, 3 ),
 ( 0.000000000000000000, 1.000000000000000000 ),
 ( 0.000000000000000000, 0.003787878787878787984, 0.007575757575757575968, 0.01136363636363636395, 0.01515151515151515194, 0.01893939393939393992, 0.02272727272727272790, 0.02651515151515151589, 0.03030303030303030387, 0.03409090909090908839, 0.03787878787878787984, 0.04166666666666666435, 0.04545454545454545581, 0.04924242424242424032, 0.05303030303030303177, 0.05681818181818181629, 0.06060606060606060774, 0.06439393939393939226, 0.06818181818181817677, 0.07196969696969697516, 0.07575757575757575968, 0.07954545454545454419, 0.08333333333333332871, 0.08712121212121212710, 0.09090909090909091161, 0.09469696969696969613, 0.09848484848484848064, 0.1022727272727272790, 0.1060606060606060635, 0.1098484848484848481, 0.1136363636363636326, 0.1174242424242424310, 0.1212121212121212155, 0.1250000000000000000, 0.1287878787878787845, 0.1325757575757575690, 0.1363636363636363535, 0.1401515151515151381, 0.1439393939393939503, 0.1477272727272727348, 0.1515151515151515194, 0.1553030303030303039, 0.1590909090909090884, 0.1628787878787878729, 0.1666666666666666574, 0.1704545454545454419, 0.1742424242424242542, 0.1780303030303030387, 0.1818181818181818232, 0.1856060606060606077, 0.1893939393939393923, 0.1931818181818181768, 0.1969696969696969613, 0.2007575757575757458, 0.2045454545454545581, 0.2083333333333333426, 0.2121212121212121271, 0.2159090909090909116, 0.2196969696969696961, 0.2234848484848484806, 0.2272727272727272652, 0.2310606060606060497, 0.2348484848484848619, 0.2386363636363636465, 0.2424242424242424310, 0.2462121212121212155, 0.2500000000000000000, 0.2537878787878787845, 0.2575757575757575690, 0.2613636363636363535, 0.2651515151515151381, 0.2689393939393939226, 0.2727272727272727071, 0.2765151515151514916, 0.2803030303030302761, 0.2840909090909091161, 0.2878787878787879007, 0.2916666666666666852, 0.2954545454545454697, 0.2992424242424242542, 0.3030303030303030387, 0.3068181818181818232, 0.3106060606060606077, 0.3143939393939393923, 0.3181818181818181768, 0.3219696969696969613, 0.3257575757575757458, 0.3295454545454545303, 0.3333333333333333148, 0.3371212121212120993, 0.3409090909090908839, 0.3446969696969697239, 0.3484848484848485084, 0.3522727272727272929, 0.3560606060606060774, 0.3598484848484848619, 0.3636363636363636465, 0.3674242424242424310, 0.3712121212121212155, 0.3750000000000000000, 0.3787878787878787845, 0.3825757575757575690, 0.3863636363636363535, 0.3901515151515151381, 0.3939393939393939226, 0.3977272727272727071, 0.4015151515151514916, 0.4053030303030302761, 0.4090909090909091161, 0.4128787878787879007, 0.4166666666666666852, 0.4204545454545454697, 0.4242424242424242542, 0.4280303030303030387, 0.4318181818181818232, 0.4356060606060606077, 0.4393939393939393923, 0.4431818181818181768, 0.4469696969696969613, 0.4507575757575757458, 0.4545454545454545303, 0.4583333333333333148, 0.4621212121212120993, 0.4659090909090908839, 0.4696969696969697239, 0.4734848484848485084, 0.4772727272727272929, 0.4810606060606060774, 0.4848484848484848619, 0.4886363636363636465, 0.4924242424242424310, 0.4962121212121212155, 0.5000000000000000000, 0.5037878787878787845, 0.5075757575757575690, 0.5113636363636363535, 0.5151515151515151381, 0.5189393939393939226, 0.5227272727272727071, 0.5265151515151514916, 0.5303030303030302761, 0.5340909090909090606, 0.5378787878787878451, 0.5416666666666666297, 0.5454545454545454142, 0.5492424242424241987, 0.5530303030303029832, 0.5568181818181817677, 0.5606060606060605522, 0.5643939393939394478, 0.5681818181818182323, 0.5719696969696970168, 0.5757575757575758013, 0.5795454545454545858, 0.5833333333333333703, 0.5871212121212121549, 0.5909090909090909394, 0.5946969696969697239, 0.5984848484848485084, 0.6022727272727272929, 0.6060606060606060774, 0.6098484848484848619, 0.6136363636363636465, 0.6174242424242424310, 0.6212121212121212155, 0.6250000000000000000, 0.6287878787878787845, 0.6325757575757575690, 0.6363636363636363535, 0.6401515151515151381, 0.6439393939393939226, 0.6477272727272727071, 0.6515151515151514916, 0.6553030303030302761, 0.6590909090909090606, 0.6628787878787878451, 0.6666666666666666297, 0.6704545454545454142, 0.6742424242424241987, 0.6780303030303029832, 0.6818181818181817677, 0.6856060606060605522, 0.6893939393939394478, 0.6931818181818182323, 0.6969696969696970168, 0.7007575757575758013, 0.7045454545454545858, 0.7083333333333333703, 0.7121212121212121549, 0.7159090909090909394, 0.7196969696969697239, 0.7234848484848485084, 0.7272727272727272929, 0.7310606060606060774, 0.7348484848484848619, 0.7386363636363636465, 0.7424242424242424310, 0.7462121212121212155, 0.7500000000000000000, 0.7537878787878787845, 0.7575757575757575690, 0.7613636363636363535, 0.7651515151515151381, 0.7689393939393939226, 0.7727272727272727071, 0.7765151515151514916, 0.7803030303030302761, 0.7840909090909090606, 0.7878787878787878451, 0.7916666666666666297, 0.7954545454545454142, 0.7992424242424241987, 0.8030303030303029832, 0.8068181818181817677, 0.8106060606060605522, 0.8143939393939394478, 0.8181818181818182323, 0.8219696969696970168, 0.8257575757575758013, 0.8295454545454545858, 0.8333333333333333703, 0.8371212121212121549, 0.8409090909090909394, 0.8446969696969697239, 0.8484848484848485084, 0.8522727272727272929, 0.8560606060606060774, 0.8598484848484848619, 0.8636363636363636465, 0.8674242424242424310, 0.8712121212121212155, 0.8750000000000000000, 0.8787878787878787845, 0.8825757575757575690, 0.8863636363636363535, 0.8901515151515151381, 0.8939393939393939226, 0.8977272727272727071, 0.9015151515151514916, 0.9053030303030302761, 0.9090909090909090606, 0.9128787878787878451, 0.9166666666666666297, 0.9204545454545454142, 0.9242424242424241987, 0.9280303030303029832, 0.9318181818181817677, 0.9356060606060605522, 0.9393939393939394478, 0.9431818181818182323, 0.9469696969696970168, 0.9507575757575758013, 0.9545454545454545858, 0.9583333333333333703, 0.9621212121212121549, 0.9659090909090909394 ),
 .UNSPECIFIED. ) 
 GEOMETRIC_REPRESENTATION_ITEM ( )  RATIONAL_B_SPLINE_SURFACE ( (
 ( 1.000000000000000000, 0.9659258262890683122, 1.000000000000000000, 0.9659258262890683122, 1.000000000000000000, 0.9659258262890683122, 1.000000000000000000, 0.9659258262890683122, 1.000000000000000000, 0.9659258262890683122, 1.000000000000000000, 0.9659258262890683122, 1.000000000000000000, 0.9659258262890683122, 1.000000000000000000, 0.9659258262890683122, 1.000000000000000000, 0.9659258262890683122, 1.000000000000000000, 0.9659258262890683122, 1.000000000000000000, 0.9659258262890683122, 1.000000000000000000, 0.9659258262890683122, 1.000000000000000000, 0.9659258262890683122, 1.000000000000000000, 0.9659258262890683122, 1.000000000000000000, 0.9659258262890683122, 1.000000000000000000, 0.9659258262890683122, 1.000000000000000000, 0.9659258262890683122, 1.000000000000000000, 0.9659258262890683122, 1.000000000000000000, 0.9659258262890683122, 1.000000000000000000, 0.9659258262890683122, 1.000000000000000000, 0.9659258262890683122, 1.000000000000000000, 0.9659258262890683122, 1.000000000000000000, 0.9659258262890683122, 1.000000000000000000, 0.9659258262890683122, 1.000000000000000000, 0.9659258262890683122, 1.000000000000000000, 0.9659258262890683122, 1.000000000000000000, 0.9659258262890683122, 1.000000000000000000, 0.9659258262890683122, 1.000000000000000000, 0.9659258262890683122, 1.000000000000000000, 0.9659258262890683122, 1.000000000000000000, 0.9659258262890683122, 1.000000000000000000, 0.9659258262890683122, 1.000000000000000000, 0.9659258262890683122, 1.000000000000000000, 0.9659258262890683122, 1.000000000000000000, 0.9659258262890683122, 1.000000000000000000, 0.9659258262890683122, 1.000000000000000000, 0.9659258262890683122, 1.000000000000000000, 0.9659258262890683122, 1.000000000000000000, 0.9659258262890683122, 1.000000000000000000, 0.9659258262890683122, 1.000000000000000000, 0.9659258262890683122, 1.000000000000000000, 0.9659258262890683122, 1.000000000000000000, 0.9659258262890683122, 1.000000000000000000, 0.9659258262890683122, 1.000000000000000000, 0.9659258262890683122, 1.000000000000000000, 0.9659258262890683122, 1.000000000000000000, 0.9659258262890683122, 1.000000000000000000, 0.9659258262890683122, 1.000000000000000000, 0.9659258262890683122, 1.000000000000000000, 0.9659258262890683122, 1.000000000000000000, 0.9659258262890683122, 1.000000000000000000, 0.9659258262890683122, 1.000000000000000000, 0.9659258262890683122, 1.000000000000000000, 0.9659258262890683122, 1.000000000000000000, 0.9659258262890683122, 1.000000000000000000, 0.9659258262890683122, 1.000000000000000000, 0.9659258262890683122, 1.000000000000000000, 0.9659258262890683122, 1.000000000000000000, 0.9659258262890683122, 1.000000000000000000, 0.9659258262890683122, 1.000000000000000000, 0.9659258262890683122, 1.000000000000000000, 0.9659258262890683122, 1.000000000000000000, 0.9659258262890683122, 1.000000000000000000, 0.9659258262890683122, 1.000000000000000000, 0.9659258262890683122, 1.000000000000000000, 0.9659258262890683122, 1.000000000000000000, 0.9659258262890683122, 1.000000000000000000, 0.9659258262890683122, 1.000000000000000000, 0.9659258262890683122, 1.000000000000000000, 0.9659258262890683122, 1.000000000000000000, 0.9659258262890683122, 1.000000000000000000, 0.9659258262890683122, 1.000000000000000000, 0.9659258262890683122, 1.000000000000000000, 0.9659258262890683122, 1.000000000000000000, 0.9659258262890683122, 1.000000000000000000, 0.9659258262890683122, 1.000000000000000000, 0.9659258262890683122, 1.000000000000000000, 0.9659258262890683122, 1.000000000000000000, 0.9659258262890683122, 1.000000000000000000, 0.9659258262890683122, 1.000000000000000000, 0.9659258262890683122, 1.000000000000000000, 0.9659258262890683122, 1.000000000000000000, 0.9659258262890683122, 1.000000000000000000, 0.9659258262890683122, 1.000000000000000000, 0.9659258262890683122, 1.000000000000000000, 0.9659258262890683122, 1.000000000000000000, 0.9659258262890683122, 1.000000000000000000, 0.9659258262890683122, 1.000000000000000000, 0.9659258262890683122, 1.000000000000000000, 0.9659258262890683122, 1.000000000000000000, 0.9659258262890683122, 1.000000000000000000, 0.9659258262890683122, 1.000000000000000000, 0.9659258262890683122, 1.000000000000000000, 0.9659258262890683122, 1.000000000000000000, 0.9659258262890683122, 1.000000000000000000, 0.9659258262890683122, 1.000000000000000000, 0.9659258262890683122, 1.000000000000000000, 0.9659258262890683122, 1.000000000000000000, 0.9659258262890683122, 1.000000000000000000, 0.9659258262890683122, 1.000000000000000000, 0.9659258262890683122, 1.000000000000000000, 0.9659258262890683122, 1.000000000000000000, 0.9659258262890683122, 1.000000000000000000, 0.9659258262890683122, 1.000000000000000000, 0.9659258262890683122, 1.000000000000000000, 0.9659258262890683122, 1.000000000000000000, 0.9659258262890683122, 1.000000000000000000, 0.9659258262890683122, 1.000000000000000000, 0.9659258262890683122, 1.000000000000000000, 0.9659258262890683122, 1.000000000000000000, 0.9659258262890683122, 1.000000000000000000, 0.9659258262890683122, 1.000000000000000000, 0.9659258262890683122, 1.000000000000000000, 0.9659258262890683122, 1.000000000000000000, 0.9659258262890683122, 1.000000000000000000, 0.9659258262890683122, 1.000000000000000000, 0.9659258262890683122, 1.000000000000000000, 0.9659258262890683122, 1.000000000000000000, 0.9659258262890683122, 1.000000000000000000, 0.9659258262890683122, 1.000000000000000000, 0.9659258262890683122, 1.000000000000000000, 0.9659258262890683122, 1.000000000000000000, 0.9659258262890683122, 1.000000000000000000, 0.9659258262890683122, 1.000000000000000000, 0.9659258262890683122, 1.000000000000000000, 0.9659258262890683122, 1.000000000000000000, 0.9659258262890683122, 1.000000000000000000, 0.9659258262890683122, 1.000000000000000000, 0.9659258262890683122, 1.000000000000000000, 0.9659258262890683122, 1.000000000000000000, 0.9659258262890683122, 1.000000000000000000, 0.9659258262890683122, 1.000000000000000000, 0.9659258262890683122, 1.000000000000000000, 0.9659258262890683122, 1.000000000000000000, 0.9659258262890683122, 1.000000000000000000, 0.9659258262890683122, 1.000000000000000000, 0.9659258262890683122, 1.000000000000000000, 0.9659258262890683122, 1.000000000000000000, 0.9659258262890683122, 1.000000000000000000, 0.9659258262890683122, 1.000000000000000000, 0.9659258262890683122, 1.000000000000000000, 0.9659258262890683122, 1.000000000000000000, 0.9659258262890683122, 1.000000000000000000, 0.9659258262890683122, 1.000000000000000000, 0.9659258262890683122, 1.000000000000000000, 0.9659258262890683122, 1.000000000000000000, 0.9659258262890683122, 1.000000000000000000, 0.9659258262890683122, 1.000000000000000000, 0.9659258262890683122, 1.000000000000000000, 0.9659258262890683122, 1.000000000000000000, 0.9659258262890683122, 1.000000000000000000, 0.9659258262890683122, 1.000000000000000000, 0.9659258262890683122, 1.000000000000000000, 0.9659258262890683122, 1.000000000000000000, 0.9659258262890683122, 1.000000000000000000, 0.9659258262890683122, 1.000000000000000000, 0.9659258262890683122, 1.000000000000000000, 0.9659258262890683122, 1.000000000000000000, 0.9659258262890683122, 1.000000000000000000, 0.9659258262890683122, 1.000000000000000000, 0.9659258262890683122, 1.000000000000000000, 0.9659258262890683122, 1.000000000000000000, 0.9659258262890683122, 1.000000000000000000, 0.9659258262890683122, 1.000000000000000000, 0.9659258262890683122, 1.000000000000000000, 0.9659258262890683122, 1.000000000000000000, 0.9659258262890683122, 1.000000000000000000, 0.9659258262890683122, 1.000000000000000000, 0.9659258262890683122, 1.000000000000000000, 0.9659258262890683122, 1.000000000000000000, 0.9659258262890683122, 1.000000000000000000, 0.9659258262890683122, 1.000000000000000000, 0.9659258262890683122, 1.000000000000000000, 0.9659258262890683122, 1.000000000000000000, 0.9659258262890683122, 1.000000000000000000, 0.9659258262890683122, 1.000000000000000000, 0.9659258262890683122, 1.000000000000000000, 0.9659258262890683122, 1.000000000000000000, 0.9659258262890683122, 1.000000000000000000, 0.9659258262890683122, 1.000000000000000000, 0.9659258262890683122, 1.000000000000000000, 0.9659258262890683122, 1.000000000000000000, 0.9659258262890683122, 1.000000000000000000, 0.9659258262890683122, 1.000000000000000000, 0.9659258262890683122, 1.000000000000000000, 0.9659258262890683122, 1.000000000000000000, 0.9659258262890683122, 1.000000000000000000, 0.9659258262890683122, 1.000000000000000000, 0.9659258262890683122, 1.000000000000000000, 0.9659258262890683122, 1.000000000000000000, 0.9659258262890683122, 1.000000000000000000, 0.9659258262890683122, 1.000000000000000000, 0.9659258262890683122, 1.000000000000000000, 0.9659258262890683122, 1.000000000000000000, 0.9659258262890683122, 1.000000000000000000, 0.9659258262890683122, 1.000000000000000000, 0.9659258262890683122, 1.000000000000000000, 0.9659258262890683122, 1.000000000000000000, 0.9659258262890683122, 1.000000000000000000, 0.9659258262890683122, 1.000000000000000000, 0.9659258262890683122, 1.000000000000000000, 0.9659258262890683122, 1.000000000000000000, 0.9659258262890683122, 1.000000000000000000, 0.9659258262890683122, 1.000000000000000000, 0.9659258262890683122, 1.000000000000000000, 0.9659258262890683122, 1.000000000000000000, 0.9659258262890683122, 1.000000000000000000, 0.9659258262890683122, 1.000000000000000000, 0.9659258262890683122, 1.000000000000000000, 0.9659258262890683122, 1.000000000000000000, 0.9659258262890683122, 1.000000000000000000, 0.9659258262890683122, 1.000000000000000000, 0.9659258262890683122, 1.000000000000000000, 0.9659258262890683122, 1.000000000000000000, 0.9659258262890683122, 1.000000000000000000, 0.9659258262890683122, 1.000000000000000000, 0.9659258262890683122, 1.000000000000000000, 0.9659258262890683122, 1.000000000000000000, 0.9659258262890683122, 1.000000000000000000, 0.9659258262890683122, 1.000000000000000000, 0.9659258262890683122, 1.000000000000000000, 0.9659258262890683122, 1.000000000000000000, 0.9659258262890683122, 1.000000000000000000, 0.9659258262890683122, 1.000000000000000000, 0.9659258262890683122, 1.000000000000000000, 0.9659258262890683122, 1.000000000000000000, 0.9659258262890683122, 1.000000000000000000, 0.9659258262890683122, 1.000000000000000000, 0.9659258262890683122, 1.000000000000000000, 0.9659258262890683122, 1.000000000000000000, 0.9659258262890683122, 1.000000000000000000, 0.9659258262890683122, 1.000000000000000000, 0.9659258262890683122, 1.000000000000000000, 0.9659258262890683122, 1.000000000000000000, 0.9659258262890683122, 1.000000000000000000, 0.9659258262890683122, 1.000000000000000000, 0.9659258262890683122, 1.000000000000000000, 0.9659258262890683122, 1.000000000000000000, 0.9659258262890683122, 1.000000000000000000, 0.9659258262890683122, 1.000000000000000000, 0.9659258262890683122, 1.000000000000000000, 0.9659258262890683122, 1.000000000000000000, 0.9659258262890683122, 1.000000000000000000, 0.9659258262890683122, 1.000000000000000000, 0.9659258262890683122, 1.000000000000000000, 0.9659258262890683122, 1.000000000000000000, 0.9659258262890683122, 1.000000000000000000, 0.9659258262890683122, 1.000000000000000000, 0.9659258262890683122, 1.000000000000000000, 0.9659258262890683122, 1.000000000000000000, 0.9659258262890683122, 1.000000000000000000, 0.9659258262890683122, 1.000000000000000000, 0.9659258262890683122, 1.000000000000000000, 0.9659258262890683122, 1.000000000000000000, 0.9659258262890683122, 1.000000000000000000),
 ( 1.000000000000000000, 0.9659258262890683122, 1.000000000000000000, 0.9659258262890683122, 1.000000000000000000, 0.9659258262890683122, 1.000000000000000000, 0.9659258262890683122, 1.000000000000000000, 0.9659258262890683122, 1.000000000000000000, 0.9659258262890683122, 1.000000000000000000, 0.9659258262890683122, 1.000000000000000000, 0.9659258262890683122, 1.000000000000000000, 0.9659258262890683122, 1.000000000000000000, 0.9659258262890683122, 1.000000000000000000, 0.9659258262890683122, 1.000000000000000000, 0.9659258262890683122, 1.000000000000000000, 0.9659258262890683122, 1.000000000000000000, 0.9659258262890683122, 1.000000000000000000, 0.9659258262890683122, 1.000000000000000000, 0.9659258262890683122, 1.000000000000000000, 0.9659258262890683122, 1.000000000000000000, 0.9659258262890683122, 1.000000000000000000, 0.9659258262890683122, 1.000000000000000000, 0.9659258262890683122, 1.000000000000000000, 0.9659258262890683122, 1.000000000000000000, 0.9659258262890683122, 1.000000000000000000, 0.9659258262890683122, 1.000000000000000000, 0.9659258262890683122, 1.000000000000000000, 0.9659258262890683122, 1.000000000000000000, 0.9659258262890683122, 1.000000000000000000, 0.9659258262890683122, 1.000000000000000000, 0.9659258262890683122, 1.000000000000000000, 0.9659258262890683122, 1.000000000000000000, 0.9659258262890683122, 1.000000000000000000, 0.9659258262890683122, 1.000000000000000000, 0.9659258262890683122, 1.000000000000000000, 0.9659258262890683122, 1.000000000000000000, 0.9659258262890683122, 1.000000000000000000, 0.9659258262890683122, 1.000000000000000000, 0.9659258262890683122, 1.000000000000000000, 0.9659258262890683122, 1.000000000000000000, 0.9659258262890683122, 1.000000000000000000, 0.9659258262890683122, 1.000000000000000000, 0.9659258262890683122, 1.000000000000000000, 0.9659258262890683122, 1.000000000000000000, 0.9659258262890683122, 1.000000000000000000, 0.9659258262890683122, 1.000000000000000000, 0.9659258262890683122, 1.000000000000000000, 0.9659258262890683122, 1.000000000000000000, 0.9659258262890683122, 1.000000000000000000, 0.9659258262890683122, 1.000000000000000000, 0.9659258262890683122, 1.000000000000000000, 0.9659258262890683122, 1.000000000000000000, 0.9659258262890683122, 1.000000000000000000, 0.9659258262890683122, 1.000000000000000000, 0.9659258262890683122, 1.000000000000000000, 0.9659258262890683122, 1.000000000000000000, 0.9659258262890683122, 1.000000000000000000, 0.9659258262890683122, 1.000000000000000000, 0.9659258262890683122, 1.000000000000000000, 0.9659258262890683122, 1.000000000000000000, 0.9659258262890683122, 1.000000000000000000, 0.9659258262890683122, 1.000000000000000000, 0.9659258262890683122, 1.000000000000000000, 0.9659258262890683122, 1.000000000000000000, 0.9659258262890683122, 1.000000000000000000, 0.9659258262890683122, 1.000000000000000000, 0.9659258262890683122, 1.000000000000000000, 0.9659258262890683122, 1.000000000000000000, 0.9659258262890683122, 1.000000000000000000, 0.9659258262890683122, 1.000000000000000000, 0.9659258262890683122, 1.000000000000000000, 0.9659258262890683122, 1.000000000000000000, 0.9659258262890683122, 1.000000000000000000, 0.9659258262890683122, 1.000000000000000000, 0.9659258262890683122, 1.000000000000000000, 0.9659258262890683122, 1.000000000000000000, 0.9659258262890683122, 1.000000000000000000, 0.9659258262890683122, 1.000000000000000000, 0.9659258262890683122, 1.000000000000000000, 0.9659258262890683122, 1.000000000000000000, 0.9659258262890683122, 1.000000000000000000, 0.9659258262890683122, 1.000000000000000000, 0.9659258262890683122, 1.000000000000000000, 0.9659258262890683122, 1.000000000000000000, 0.9659258262890683122, 1.000000000000000000, 0.9659258262890683122, 1.000000000000000000, 0.9659258262890683122, 1.000000000000000000, 0.9659258262890683122, 1.000000000000000000, 0.9659258262890683122, 1.000000000000000000, 0.9659258262890683122, 1.000000000000000000, 0.9659258262890683122, 1.000000000000000000, 0.9659258262890683122, 1.000000000000000000, 0.9659258262890683122, 1.000000000000000000, 0.9659258262890683122, 1.000000000000000000, 0.9659258262890683122, 1.000000000000000000, 0.9659258262890683122, 1.000000000000000000, 0.9659258262890683122, 1.000000000000000000, 0.9659258262890683122, 1.000000000000000000, 0.9659258262890683122, 1.000000000000000000, 0.9659258262890683122, 1.000000000000000000, 0.9659258262890683122, 1.000000000000000000, 0.9659258262890683122, 1.000000000000000000, 0.9659258262890683122, 1.000000000000000000, 0.9659258262890683122, 1.000000000000000000, 0.9659258262890683122, 1.000000000000000000, 0.9659258262890683122, 1.000000000000000000, 0.9659258262890683122, 1.000000000000000000, 0.9659258262890683122, 1.000000000000000000, 0.9659258262890683122, 1.000000000000000000, 0.9659258262890683122, 1.000000000000000000, 0.9659258262890683122, 1.000000000000000000, 0.9659258262890683122, 1.000000000000000000, 0.9659258262890683122, 1.000000000000000000, 0.9659258262890683122, 1.000000000000000000, 0.9659258262890683122, 1.000000000000000000, 0.9659258262890683122, 1.000000000000000000, 0.9659258262890683122, 1.000000000000000000, 0.9659258262890683122, 1.000000000000000000, 0.9659258262890683122, 1.000000000000000000, 0.9659258262890683122, 1.000000000000000000, 0.9659258262890683122, 1.000000000000000000, 0.9659258262890683122, 1.000000000000000000, 0.9659258262890683122, 1.000000000000000000, 0.9659258262890683122, 1.000000000000000000, 0.9659258262890683122, 1.000000000000000000, 0.9659258262890683122, 1.000000000000000000, 0.9659258262890683122, 1.000000000000000000, 0.9659258262890683122, 1.000000000000000000, 0.9659258262890683122, 1.000000000000000000, 0.9659258262890683122, 1.000000000000000000, 0.9659258262890683122, 1.000000000000000000, 0.9659258262890683122, 1.000000000000000000, 0.9659258262890683122, 1.000000000000000000, 0.9659258262890683122, 1.000000000000000000, 0.9659258262890683122, 1.000000000000000000, 0.9659258262890683122, 1.000000000000000000, 0.9659258262890683122, 1.000000000000000000, 0.9659258262890683122, 1.000000000000000000, 0.9659258262890683122, 1.000000000000000000, 0.9659258262890683122, 1.000000000000000000, 0.9659258262890683122, 1.000000000000000000, 0.9659258262890683122, 1.000000000000000000, 0.9659258262890683122, 1.000000000000000000, 0.9659258262890683122, 1.000000000000000000, 0.9659258262890683122, 1.000000000000000000, 0.9659258262890683122, 1.000000000000000000, 0.9659258262890683122, 1.000000000000000000, 0.9659258262890683122, 1.000000000000000000, 0.9659258262890683122, 1.000000000000000000, 0.9659258262890683122, 1.000000000000000000, 0.9659258262890683122, 1.000000000000000000, 0.9659258262890683122, 1.000000000000000000, 0.9659258262890683122, 1.000000000000000000, 0.9659258262890683122, 1.000000000000000000, 0.9659258262890683122, 1.000000000000000000, 0.9659258262890683122, 1.000000000000000000, 0.9659258262890683122, 1.000000000000000000, 0.9659258262890683122, 1.000000000000000000, 0.9659258262890683122, 1.000000000000000000, 0.9659258262890683122, 1.000000000000000000, 0.9659258262890683122, 1.000000000000000000, 0.9659258262890683122, 1.000000000000000000, 0.9659258262890683122, 1.000000000000000000, 0.9659258262890683122, 1.000000000000000000, 0.9659258262890683122, 1.000000000000000000, 0.9659258262890683122, 1.000000000000000000, 0.9659258262890683122, 1.000000000000000000, 0.9659258262890683122, 1.000000000000000000, 0.9659258262890683122, 1.000000000000000000, 0.9659258262890683122, 1.000000000000000000, 0.9659258262890683122, 1.000000000000000000, 0.9659258262890683122, 1.000000000000000000, 0.9659258262890683122, 1.000000000000000000, 0.9659258262890683122, 1.000000000000000000, 0.9659258262890683122, 1.000000000000000000, 0.9659258262890683122, 1.000000000000000000, 0.9659258262890683122, 1.000000000000000000, 0.9659258262890683122, 1.000000000000000000, 0.9659258262890683122, 1.000000000000000000, 0.9659258262890683122, 1.000000000000000000, 0.9659258262890683122, 1.000000000000000000, 0.9659258262890683122, 1.000000000000000000, 0.9659258262890683122, 1.000000000000000000, 0.9659258262890683122, 1.000000000000000000, 0.9659258262890683122, 1.000000000000000000, 0.9659258262890683122, 1.000000000000000000, 0.9659258262890683122, 1.000000000000000000, 0.9659258262890683122, 1.000000000000000000, 0.9659258262890683122, 1.000000000000000000, 0.9659258262890683122, 1.000000000000000000, 0.9659258262890683122, 1.000000000000000000, 0.9659258262890683122, 1.000000000000000000, 0.9659258262890683122, 1.000000000000000000, 0.9659258262890683122, 1.000000000000000000, 0.9659258262890683122, 1.000000000000000000, 0.9659258262890683122, 1.000000000000000000, 0.9659258262890683122, 1.000000000000000000, 0.9659258262890683122, 1.000000000000000000, 0.9659258262890683122, 1.000000000000000000, 0.9659258262890683122, 1.000000000000000000, 0.9659258262890683122, 1.000000000000000000, 0.9659258262890683122, 1.000000000000000000, 0.9659258262890683122, 1.000000000000000000, 0.9659258262890683122, 1.000000000000000000, 0.9659258262890683122, 1.000000000000000000, 0.9659258262890683122, 1.000000000000000000, 0.9659258262890683122, 1.000000000000000000, 0.9659258262890683122, 1.000000000000000000, 0.9659258262890683122, 1.000000000000000000, 0.9659258262890683122, 1.000000000000000000, 0.9659258262890683122, 1.000000000000000000, 0.9659258262890683122, 1.000000000000000000, 0.9659258262890683122, 1.000000000000000000, 0.9659258262890683122, 1.000000000000000000, 0.9659258262890683122, 1.000000000000000000, 0.9659258262890683122, 1.000000000000000000, 0.9659258262890683122, 1.000000000000000000, 0.9659258262890683122, 1.000000000000000000, 0.9659258262890683122, 1.000000000000000000, 0.9659258262890683122, 1.000000000000000000, 0.9659258262890683122, 1.000000000000000000, 0.9659258262890683122, 1.000000000000000000, 0.9659258262890683122, 1.000000000000000000, 0.9659258262890683122, 1.000000000000000000, 0.9659258262890683122, 1.000000000000000000, 0.9659258262890683122, 1.000000000000000000, 0.9659258262890683122, 1.000000000000000000, 0.9659258262890683122, 1.000000000000000000, 0.9659258262890683122, 1.000000000000000000, 0.9659258262890683122, 1.000000000000000000, 0.9659258262890683122, 1.000000000000000000, 0.9659258262890683122, 1.000000000000000000, 0.9659258262890683122, 1.000000000000000000, 0.9659258262890683122, 1.000000000000000000, 0.9659258262890683122, 1.000000000000000000, 0.9659258262890683122, 1.000000000000000000, 0.9659258262890683122, 1.000000000000000000, 0.9659258262890683122, 1.000000000000000000, 0.9659258262890683122, 1.000000000000000000, 0.9659258262890683122, 1.000000000000000000, 0.9659258262890683122, 1.000000000000000000, 0.9659258262890683122, 1.000000000000000000, 0.9659258262890683122, 1.000000000000000000, 0.9659258262890683122, 1.000000000000000000, 0.9659258262890683122, 1.000000000000000000, 0.9659258262890683122, 1.000000000000000000, 0.9659258262890683122, 1.000000000000000000, 0.9659258262890683122, 1.000000000000000000, 0.9659258262890683122, 1.000000000000000000, 0.9659258262890683122, 1.000000000000000000, 0.9659258262890683122, 1.000000000000000000, 0.9659258262890683122, 1.000000000000000000, 0.9659258262890683122, 1.000000000000000000, 0.9659258262890683122, 1.000000000000000000, 0.9659258262890683122, 1.000000000000000000, 0.9659258262890683122, 1.000000000000000000, 0.9659258262890683122, 1.000000000000000000, 0.9659258262890683122, 1.000000000000000000) ) ) 
 REPRESENTATION_ITEM ( '' )  SURFACE ( )  );
#54684=CARTESIAN_POINT ( 'NONE',  ( 0.9908136482939640111, -0.6692913385826771977, 0.1292274648535927661 ) ) ;
#54685=CARTESIAN_POINT ( 'NONE',  ( -1.640419947506561060, -0.3690944881889765550, -0.3153832671262227771 ) ) ;
#54686=CARTESIAN_POINT ( 'NONE',  ( -0.4986876640419942164, -0.6046776061558807314, 0.2411417322834647770 ) ) ;
#54687=CARTESIAN_POINT ( 'NONE',  ( 0.2099737532808405305, -0.5023911411419708095, 0.1820866141732285504 ) ) ;
#54689=CARTESIAN_POINT ( 'NONE',  ( 0.6824146981627303710, 0.1283753931104746893, -0.1820866141732285504 ) ) ;
#54690=EDGE_CURVE ( 'NONE', #57945, #79833, #55280, .T. ) ;
#54692=CARTESIAN_POINT ( 'NONE',  ( 0.01968503937007957949, -0.5400638737290845981, -0.3530559997133363437 ) ) ;
#54694=EDGE_CURVE ( 'NONE', #73064, #24616, #10694, .T. ) ;
#54695=CARTESIAN_POINT ( 'NONE',  ( -0.9120734908136475250, 0.2952755905511811885, 0.1292274648535926551 ) ) ;
#54698=CARTESIAN_POINT ( 'NONE',  ( 1.128608923884514947, 0.1283753931104748280, 0.1820866141732283561 ) ) ;
#54699=CARTESIAN_POINT ( 'NONE',  ( -0.07874015748031421014, -0.1870078740157479769, 0.4822834645669291653 ) ) ;
#54702=CARTESIAN_POINT ( 'NONE',  ( -0.3674540682414689785, 0.2306618581243848609, 0.2411417322834645549 ) ) ;
#54703=CARTESIAN_POINT ( 'NONE',  ( -0.4396325459317577122, -0.5511811023622048555, -0.09757992244046775898 ) ) ;
#54705=CARTESIAN_POINT ( 'NONE',  ( -0.4133858267716528645, -0.4536011799217367080, 0.2665933059059888421 ) ) ;
#54706=CARTESIAN_POINT ( 'NONE',  ( 0.1902887139107617975, -0.6692913385826773087, -0.1292274648535924053 ) ) ;
#54707=CARTESIAN_POINT ( 'NONE',  ( -1.266404199475064773, -0.2845877964562159024, 0.3641732283464567677 ) ) ;
#54709=CARTESIAN_POINT ( 'NONE',  ( -1.312335958005248715, 0.2306618581243848609, 0.2411417322834645549 ) ) ;
#54712=CARTESIAN_POINT ( 'NONE',  ( -1.515748031496062076, 0.07958543189024071263, -0.2665933059059888421 ) ) ;
#54713=CARTESIAN_POINT ( 'NONE',  ( -0.5905511811023615998, 0.2952755905511811885, 0.000000000000000000 ) ) ;
#54715=CARTESIAN_POINT ( 'NONE',  ( -1.377952755905511140, -0.6692913385826771977, 8.415575281601705876E-17 ) ) ;
#54719=CARTESIAN_POINT ( 'NONE',  ( 1.279527559055118724, -0.5400638737290845981, -0.3530559997133363437 ) ) ;
#54720=CARTESIAN_POINT ( 'NONE',  ( 0.6692913385826778638, -0.6692913385826771977, 8.415575281601705876E-17 ) ) ;
#54724=CARTESIAN_POINT ( 'NONE',  ( -1.686351706036744558, 0.2952755905511810774, -0.1292274648535930714 ) ) ;
#54727=CARTESIAN_POINT ( 'NONE',  ( -0.4133858267716528645, -0.4536011799217367080, 0.2665933059059888421 ) ) ;
#54730=CARTESIAN_POINT ( 'NONE',  ( 0.9317585301837276734, -0.4281496062992124485, 0.4176697321401328655 ) ) ;
#54731=CARTESIAN_POINT ( 'NONE',  ( -0.4527559055118102749, 0.1660481256975885056, 0.3530559997133364547 ) ) ;
#54732=CARTESIAN_POINT ( 'NONE',  ( -1.036745406824146176, -0.4281496062992124485, 0.4176697321401328655 ) ) ;
#54733=CARTESIAN_POINT ( 'NONE',  ( 1.404199475065617708, 0.05413385826771626580, -0.4176697321401330321 ) ) ;
#54734=CARTESIAN_POINT ( 'NONE',  ( -1.476377952755905110, 0.07958543189024085140, 0.2665933059059887866 ) ) ;
#54736=CARTESIAN_POINT ( 'NONE',  ( 0.2887139107611556010, 0.2306618581243847221, -0.2411417322834647770 ) ) ;
#54737=CARTESIAN_POINT ( 'NONE',  ( -0.9251968503937002541, -0.5400638737290845981, -0.3530559997133363437 ) ) ;
#54739=CARTESIAN_POINT ( 'NONE',  ( -1.069553805774277722, -0.6692913385826773087, -0.1292274648535924053 ) ) ;
#54740=DIRECTION ( 'NONE',  ( -0.1923134147744552658, 0.6939076129059796871, 0.6939076129060073317 ) ) ;
#54741=CARTESIAN_POINT ( 'NONE',  ( 0.8267716535433078384, -0.6692913385826771977, 8.415575281601705876E-17 ) ) ;
#54742=CARTESIAN_POINT ( 'NONE',  ( 1.266404199475066328, -0.2845877964562161244, -0.3641732283464567121 ) ) ;
#54745=CARTESIAN_POINT ( 'NONE',  ( -0.4068241469816264999, -0.4281496062992124485, 0.4176697321401328655 ) ) ;
#54747=CARTESIAN_POINT ( 'NONE',  ( 0.5577427821522314977, -0.2845877964562161244, -0.3641732283464567121 ) ) ;
#54748=CARTESIAN_POINT ( 'NONE',  ( -1.430446194225721390, -0.4281496062992124485, 0.4176697321401328655 ) ) ;
#54749=CARTESIAN_POINT ( 'NONE',  ( 0.9711286089238851948, 0.2306618581243848609, 0.2411417322834645549 ) ) ;
#54750=CARTESIAN_POINT ( 'NONE',  ( 0.7545931758530188826, -0.6692913385826771977, 0.1292274648535927661 ) ) ;
#54751=CARTESIAN_POINT ( 'NONE',  ( -0.2887139107611542133, 0.2306618581243848609, 0.2411417322834645549 ) ) ;
#54753=CARTESIAN_POINT ( 'NONE',  ( -0.7086614173228339419, -0.1870078740157479769, 0.4822834645669291653 ) ) ;
#54755=CARTESIAN_POINT ( 'NONE',  ( -1.732283464566928277, -0.1870078740157479769, 0.4822834645669291653 ) ) ;
#54756=CARTESIAN_POINT ( 'NONE',  ( -1.069553805774277722, -0.6692913385826773087, -0.1292274648535924053 ) ) ;
#54757=CARTESIAN_POINT ( 'NONE',  ( 1.318897637795276356, -0.5400638737290844871, 0.3530559997133364547 ) ) ;
#54758=CARTESIAN_POINT ( 'NONE',  ( 1.692913385826772421, 0.2952755905511811885, 0.000000000000000000 ) ) ;
#54759=CARTESIAN_POINT ( 'NONE',  ( -1.049868766404198794, 0.2306618581243847221, -0.2411417322834647770 ) ) ;
#54761=CARTESIAN_POINT ( 'NONE',  ( 0.4002624671916016896, -0.3162353388693409650, -0.4822834645669289433 ) ) ;
#54763=AXIS2_PLACEMENT_3D ( 'NONE', #79049, #36369, #55710 ) ;
#54764=CARTESIAN_POINT ( 'NONE',  ( -0.7545931758530176614, -0.6692913385826773087, -0.1292274648535924053 ) ) ;
#54766=CARTESIAN_POINT ( 'NONE',  ( 1.581364829396326277, -0.3162353388693409650, -0.4822834645669289433 ) ) ;
#54767=CARTESIAN_POINT ( 'NONE',  ( 0.7742782152230979209, -0.004921259842519870586, -0.3153832671262229437 ) ) ;
#54768=CARTESIAN_POINT ( 'NONE',  ( 1.253280839895013710, -0.3162353388693405765, 0.4822834645669290543 ) ) ;
#54770=CARTESIAN_POINT ( 'NONE',  ( 1.010498687664042716, -0.3690944881889763329, 0.3153832671262228327 ) ) ;
#54771=CARTESIAN_POINT ( 'NONE',  ( 0.8333333333333340365, 0.2952755905511810774, -0.1292274648535930714 ) ) ;
#54773=CARTESIAN_POINT ( 'NONE',  ( -0.4724409448818890911, -0.1870078740157479769, 0.4822834645669291653 ) ) ;
#54775=CARTESIAN_POINT ( 'NONE',  ( 1.279527559055118724, 0.07958543189024085140, 0.2665933059059887866 ) ) ;
#54776=CARTESIAN_POINT ( 'NONE',  ( -0.4396325459317579898, 0.2952755905511811885, 0.1292274648535926551 ) ) ;
#54778=CARTESIAN_POINT ( 'NONE',  ( 1.476377952755906442, -0.5400638737290844871, 0.3530559997133364547 ) ) ;
#54779=CARTESIAN_POINT ( 'NONE',  ( 0.1246719160104994284, -0.6692913385826771977, 0.1292274648535927661 ) ) ;
#54780=CARTESIAN_POINT ( 'NONE',  ( 0.5183727034120741983, -0.5511811023622046335, 0.09757992244046803654 ) ) ;
#54782=CARTESIAN_POINT ( 'NONE',  ( 0.1574803149606306130, -0.1870078740157480601, -0.3641732283464567677 ) ) ;
#54783=CARTESIAN_POINT ( 'NONE',  ( -1.601049868766403650, 0.2306618581243847221, -0.2411417322834647770 ) ) ;
#54784=EDGE_CURVE ( 'NONE', #17596, #24792, #47400, .T. ) ;
#54786=CARTESIAN_POINT ( 'NONE',  ( 0.7808398950131241190, -0.05778040916215560624, -0.4822834645669293319 ) ) ;
#54788=CARTESIAN_POINT ( 'NONE',  ( 1.594488188976378673, -0.4536011799217368745, -0.2665933059059886201 ) ) ;
#54789=DIRECTION ( 'NONE',  ( -0.000000000000000000, 1.000000000000000000, -0.000000000000000000 ) ) ;
#54790=CARTESIAN_POINT ( 'NONE',  ( -0.08530183727034056085, -0.08942795157528024563, -0.3641732283464568787 ) ) ;
#54791=CARTESIAN_POINT ( 'NONE',  ( 0.01312335958005323398, -0.4281496062992127816, -0.4176697321401328100 ) ) ;
#54792=CARTESIAN_POINT ( 'NONE',  ( 1.555118110236221041, 0.07958543189024071263, -0.2665933059059888421 ) ) ;
#54793=CARTESIAN_POINT ( 'NONE',  ( -1.358267716535432434, 0.07958543189024071263, -0.2665933059059888421 ) ) ;
#54794=CARTESIAN_POINT ( 'NONE',  ( -1.601049868766403650, -0.6046776061558807314, 0.2411417322834647770 ) ) ;
#54795=CARTESIAN_POINT ( 'NONE',  ( 0.6561679790026253567, -0.6046776061558809534, -0.2411417322834644161 ) ) ;
#54796=CARTESIAN_POINT ( 'NONE',  ( 1.207349081364829990, 0.2306618581243848609, 0.2411417322834645549 ) ) ;
#54798=CARTESIAN_POINT ( 'NONE',  ( 0.07874015748031558404, -0.1870078740157480879, -0.4822834645669291653 ) ) ;
#54799=CARTESIAN_POINT ( 'NONE',  ( 1.397637795275591177, 0.1660481256975883668, -0.3530559997133364547 ) ) ;
#54800=CARTESIAN_POINT ( 'NONE',  ( 1.181102362204725198, -0.1870078740157479769, 0.4822834645669291653 ) ) ;
#54802=CARTESIAN_POINT ( 'NONE',  ( 0.6955380577427828781, -0.3690944881889763329, 0.3153832671262228327 ) ) ;
#54803=CARTESIAN_POINT ( 'NONE',  ( 1.541994750656168645, 0.2952755905511810774, -0.1292274648535930714 ) ) ;
#54804=CARTESIAN_POINT ( 'NONE',  ( -0.07217847769028813698, -0.2845877964562161244, -0.3641732283464567121 ) ) ;
#54805=CARTESIAN_POINT ( 'NONE',  ( -0.03280839895013062252, 0.2952755905511810774, -0.1292274648535930714 ) ) ;
#54806=CARTESIAN_POINT ( 'NONE',  ( 0.7808398950131240079, -0.3162353388693405765, 0.4822834645669290543 ) ) ;
#54807=CARTESIAN_POINT ( 'NONE',  ( -0.3018372703412066094, -0.4281496062992127816, -0.4176697321401328100 ) ) ;
#54808=CARTESIAN_POINT ( 'NONE',  ( -0.2559055118110230564, 0.07958543189024071263, -0.2665933059059888421 ) ) ;
#54809=CARTESIAN_POINT ( 'NONE',  ( 0.7874015748031503170, -0.1870078740157479769, 0.4822834645669291653 ) ) ;
#54810=CARTESIAN_POINT ( 'NONE',  ( 0.8464566929133866546, -0.4536011799217367080, 0.2665933059059888421 ) ) ;
#54812=EDGE_CURVE ( 'NONE', #19838, #74748, #4615, .T. ) ;
#54817=CIRCLE ( 'NONE', #60241, 1.220472440944881942 ) ;
#54818=CARTESIAN_POINT ( 'NONE',  ( -1.345144356955379816, -0.3162353388693405765, 0.4822834645669290543 ) ) ;
#54819=CARTESIAN_POINT ( 'NONE',  ( -0.3543307086614165824, -0.6692913385826771977, 8.415575281601705876E-17 ) ) ;
#54822=EDGE_LOOP ( 'NONE', ( #68927, #63360, #5851, #3289 ) ) ;
#54823=CARTESIAN_POINT ( 'NONE',  ( 0.7283464566929143125, 0.07958543189024085140, 0.2665933059059887866 ) ) ;
#54825=CARTESIAN_POINT ( 'NONE',  ( 0.9711286089238851948, 0.2306618581243848609, 0.2411417322834645549 ) ) ;
#54828=CARTESIAN_POINT ( 'NONE',  ( -1.568241469816272105, -0.08942795157527998196, 0.3641732283464567121 ) ) ;
#54829=DIRECTION ( 'NONE',  ( -1.000000000000000000, -3.412570772413390973E-16, 0.000000000000000000 ) ) ;
#54830=CARTESIAN_POINT ( 'NONE',  ( 1.496062992125984703, -0.1870078740157480601, -0.3641732283464567677 ) ) ;
#54831=CARTESIAN_POINT ( 'NONE',  ( 0.6233595800524942554, -0.05778040916215560624, -0.4822834645669293319 ) ) ;
#54833=CARTESIAN_POINT ( 'NONE',  ( 0.2230971128608932319, -0.4281496062992124485, 0.4176697321401328655 ) ) ;
#54834=CARTESIAN_POINT ( 'NONE',  ( -0.8727034120734901146, -0.08942795157528024563, -0.3641732283464568787 ) ) ;
#54835=CARTESIAN_POINT ( 'NONE',  ( 0.8202099737532813073, 0.2952755905511811885, 0.1292274648535926551 ) ) ;
#54836=CARTESIAN_POINT ( 'NONE',  ( -0.2230971128608915943, -0.4281496062992127816, -0.4176697321401328100 ) ) ;
#54837=CARTESIAN_POINT ( 'NONE',  ( 0.4824498642376759960, 1.223219560026271499E-15, 0.4445507791589056734 ) ) ;
#54838=CARTESIAN_POINT ( 'NONE',  ( -0.01069919276010446348, 1.490381362800744269E-15, -0.4118477457932981367 ) ) ;
#54840=CARTESIAN_POINT ( 'NONE',  ( 0.7545931758530189937, 0.2952755905511810774, -0.1292274648535930714 ) ) ;
#54841=CARTESIAN_POINT ( 'NONE',  ( 0.01968503937007930540, 0.1660481256975885056, 0.3530559997133364547 ) ) ;
#54842=CARTESIAN_POINT ( 'NONE',  ( -1.003937007874014853, 0.1660481256975885056, 0.3530559997133364547 ) ) ;
#54844=CARTESIAN_POINT ( 'NONE',  ( 0.9645669291338588858, 0.1660481256975885056, 0.3530559997133364547 ) ) ;
#54845=CARTESIAN_POINT ( 'NONE',  ( 0.2821522309711292364, 0.2952755905511810774, -0.1292274648535930714 ) ) ;
#54847=CARTESIAN_POINT ( 'NONE',  ( -0.4199475065616791736, 0.2306618581243847221, -0.2411417322834647770 ) ) ;
#54848=CARTESIAN_POINT ( 'NONE',  ( 0.5511811023622055217, -0.1870078740157479769, 0.4822834645669291653 ) ) ;
#54849=CARTESIAN_POINT ( 'NONE',  ( -0.01968503937007793844, 0.1660481256975883668, -0.3530559997133364547 ) ) ;
#54850=EDGE_CURVE ( 'NONE', #25851, #38370, #63498, .T. ) ;
#54851=CARTESIAN_POINT ( 'NONE',  ( 0.5839895013123367340, 0.1771653543307087630, 0.09757992244046791164 ) ) ;
#54852=CARTESIAN_POINT ( 'NONE',  ( -1.581364829396324945, -0.3162353388693405765, 0.4822834645669290543 ) ) ;
#54854=CARTESIAN_POINT ( 'NONE',  ( 0.3740157480314966754, 0.1660481256975883668, -0.3530559997133364547 ) ) ;
#54856=EDGE_LOOP ( 'NONE', ( #7035, #70983, #67208, #9209 ) ) ;
#54857=VERTEX_POINT ( 'NONE', #8995 ) ;
#54858=CARTESIAN_POINT ( 'NONE',  ( 0.8398950131233602345, -0.6046776061558807314, 0.2411417322834647770 ) ) ;
#54859=CARTESIAN_POINT ( 'NONE',  ( 0.6758530183727039509, 0.1771653543307087075, -0.09757992244046823083 ) ) ;
#54867=CARTESIAN_POINT ( 'NONE',  ( 0.9908136482939640111, 0.2952755905511810774, -0.1292274648535930714 ) ) ;
#54868=CARTESIAN_POINT ( 'NONE',  ( -1.017060367454067249, -0.05778040916215522460, 0.4822834645669289988 ) ) ;
#54869=CARTESIAN_POINT ( 'NONE',  ( -0.8398950131233589023, -0.6046776061558809534, -0.2411417322834644161 ) ) ;
#54870=CARTESIAN_POINT ( 'NONE',  ( 0.7414698162729663755, -0.6692913385826773087, -0.1292274648535924053 ) ) ;
#54871=CARTESIAN_POINT ( 'NONE',  ( 1.207349081364829990, -0.6046776061558809534, -0.2411417322834644161 ) ) ;
#54874=CARTESIAN_POINT ( 'NONE',  ( 1.272965879265092637, -0.3690944881889765550, -0.3153832671262227771 ) ) ;
#54876=CARTESIAN_POINT ( 'NONE',  ( -1.463254593175852492, 0.1771653543307087630, 0.09757992244046791164 ) ) ;
#54878=CARTESIAN_POINT ( 'NONE',  ( 0.1574803149606306130, -0.1870078740157480879, -0.4822834645669291653 ) ) ;
#54880=CARTESIAN_POINT ( 'NONE',  ( 1.522309711286089939, 0.2306618581243848609, 0.2411417322834645549 ) ) ;
#54882=CARTESIAN_POINT ( 'NONE',  ( -0.9711286089238838626, -0.5023911411419708095, 0.1820866141732285504 ) ) ;
#54883=CARTESIAN_POINT ( 'NONE',  ( 0.1968503937007881344, -0.6692913385826771977, 8.415575281601705876E-17 ) ) ;
#54884=CARTESIAN_POINT ( 'NONE',  ( 1.187664041994751285, -0.2845877964562161244, -0.3641732283464567121 ) ) ;
#54886=CARTESIAN_POINT ( 'NONE',  ( -1.023622047244094002, -0.1870078740157480601, -0.3641732283464567677 ) ) ;
#54887=CARTESIAN_POINT ( 'NONE',  ( 1.463254593175853824, -0.6692913385826771977, 0.1292274648535927661 ) ) ;
#54889=CARTESIAN_POINT ( 'NONE',  ( -0.1509186351706028884, -0.05778040916215522460, 0.4822834645669289988 ) ) ;
#54890=CARTESIAN_POINT ( 'NONE',  ( -1.423884514435694859, -0.08942795157528024563, -0.3641732283464568787 ) ) ;
#54891=CARTESIAN_POINT ( 'NONE',  ( -0.5905511811023615998, 0.2952755905511811885, 0.000000000000000000 ) ) ;
#54892=CARTESIAN_POINT ( 'NONE',  ( -1.653543307086613234, -0.1870078740157479769, 0.3641732283464567677 ) ) ;
#54894=CARTESIAN_POINT ( 'NONE',  ( 0.1509186351706042484, -0.3162353388693405765, 0.4822834645669290543 ) ) ;
#54896=CARTESIAN_POINT ( 'NONE',  ( -1.384514435695537005, 0.2952755905511811885, 0.1292274648535926551 ) ) ;
#54897=CARTESIAN_POINT ( 'NONE',  ( -0.7020997375328076329, -0.2845877964562161244, -0.3641732283464567121 ) ) ;
#54898=CARTESIAN_POINT ( 'NONE',  ( -0.4855643044619415427, 0.009842519685039147898, -0.3409548833797004797 ) ) ;
#54899=CARTESIAN_POINT ( 'NONE',  ( -0.03280839895013062252, 0.2952755905511810774, -0.1292274648535930714 ) ) ;
#54900=CARTESIAN_POINT ( 'NONE',  ( 0.5839895013123367340, 0.1771653543307087630, 0.09757992244046791164 ) ) ;
#54901=CARTESIAN_POINT ( 'NONE',  ( -1.246719160104986512, -0.004921259842519576551, 0.3153832671262227771 ) ) ;
#54902=CARTESIAN_POINT ( 'NONE',  ( -1.607611548556429737, -0.6692913385826771977, 0.1292274648535927661 ) ) ;
#54903=CARTESIAN_POINT ( 'NONE',  ( -1.437007874015747477, -0.5400638737290844871, 0.3530559997133364547 ) ) ;
#54904=CARTESIAN_POINT ( 'NONE',  ( 1.561679790026247350, 0.05413385826771626580, -0.4176697321401330321 ) ) ;
#54906=CARTESIAN_POINT ( 'NONE',  ( 0.3937007874015754361, -0.1870078740157479769, 0.3641732283464567677 ) ) ;
#54907=CARTESIAN_POINT ( 'NONE',  ( 0.7677165354330716118, 0.1660481256975883668, -0.3530559997133364547 ) ) ;
#54909=CARTESIAN_POINT ( 'NONE',  ( 1.404199475065617264, -0.3690944881889763329, 0.3153832671262228327 ) ) ;
#54910=ORIENTED_EDGE ( 'NONE', *, *, #76274, .T. ) ;
#54911=CARTESIAN_POINT ( 'NONE',  ( -1.154855643044618851, 0.2306618581243848609, 0.2411417322834645549 ) ) ;
#54912=CARTESIAN_POINT ( 'NONE',  ( -0.6889763779527552368, 0.1660481256975885056, 0.3530559997133364547 ) ) ;
#54913=CARTESIAN_POINT ( 'NONE',  ( 0.3018372703412079971, -0.4281496062992124485, 0.4176697321401328655 ) ) ;
#54916=CARTESIAN_POINT ( 'NONE',  ( 0.9186351706036751663, -0.6046776061558807314, 0.2411417322834647770 ) ) ;
#54917=CARTESIAN_POINT ( 'NONE',  ( -1.706036745406823485, 0.2306618581243848609, 0.2411417322834645549 ) ) ;
#54918=CARTESIAN_POINT ( 'NONE',  ( 0.5839895013123367340, 0.2952755905511811885, 0.1292274648535926551 ) ) ;
#54919=CARTESIAN_POINT ( 'NONE',  ( 0.6102362204724416372, -0.5400638737290844871, 0.3530559997133364547 ) ) ;
#54925=CARTESIAN_POINT ( 'NONE',  ( 0.05249343832021075018, 0.1283753931104746893, -0.1820866141732285504 ) ) ;
#54926=CARTESIAN_POINT ( 'NONE',  ( -0.3018372703412066094, 0.05413385826771666132, 0.4176697321401328100 ) ) ;
#54927=CARTESIAN_POINT ( 'NONE',  ( 0.9973753280839902091, 0.2306618581243847221, -0.2411417322834647770 ) ) ;
#54929=CARTESIAN_POINT ( 'NONE',  ( -0.1312335958005241554, -0.5023911411419708095, -0.1820866141732282451 ) ) ;
#54930=CARTESIAN_POINT ( 'NONE',  ( -1.135170603674539924, 0.2952755905511810774, -0.1292274648535930714 ) ) ;
#54931=CARTESIAN_POINT ( 'NONE',  ( 1.404199475065617264, -0.4281496062992124485, 0.4176697321401328655 ) ) ;
#54935=ADVANCED_FACE ( 'NONE', ( #22855 ), #18090, .F. ) ;
#54937=CARTESIAN_POINT ( 'NONE',  ( 0.9186351706036751663, -0.6046776061558807314, 0.2411417322834647770 ) ) ;
#54938=CARTESIAN_POINT ( 'NONE',  ( 1.404199475065617264, -0.3690944881889763329, 0.3153832671262228327 ) ) ;
#54939=CARTESIAN_POINT ( 'NONE',  ( 1.535433070866142558, 0.2952755905511811885, 0.000000000000000000 ) ) ;
#54940=CARTESIAN_POINT ( 'NONE',  ( 1.555118110236221041, -0.5400638737290844871, 0.3530559997133364547 ) ) ;
#54943=CARTESIAN_POINT ( 'NONE',  ( 1.272965879265092637, -0.4281496062992127816, -0.4176697321401328100 ) ) ;
#54945=CARTESIAN_POINT ( 'NONE',  ( -0.07217847769028813698, -0.3162353388693409650, -0.4822834645669289433 ) ) ;
#54946=CARTESIAN_POINT ( 'NONE',  ( -0.6102362204724400829, 0.1660481256975885056, 0.3530559997133364547 ) ) ;
#54947=CARTESIAN_POINT ( 'NONE',  ( -1.509186351706035767, -0.4281496062992124485, 0.4176697321401328655 ) ) ;
#54949=CARTESIAN_POINT ( 'NONE',  ( 0.2690288713910767848, -0.6692913385826773087, -0.1292274648535924053 ) ) ;
#54951=CARTESIAN_POINT ( 'NONE',  ( 1.535433070866142558, 0.2952755905511811885, 0.000000000000000000 ) ) ;
#54952=ORIENTED_EDGE ( 'NONE', *, *, #39809, .T. ) ;
#54956=CARTESIAN_POINT ( 'NONE',  ( 1.607611548556431069, 0.1771653543307087630, 0.09757992244046791164 ) ) ;
#54960=CARTESIAN_POINT ( 'NONE',  ( 0.4624320255261049062, 8.471767977567108961E-16, -0.4445507791589058955 ) ) ;
#54961=CARTESIAN_POINT ( 'NONE',  ( 1.614173228346456712, 2.401574803149606474, -0.1372047244094476703 ) ) ;
#54963=CARTESIAN_POINT ( 'NONE',  ( -0.1706036745406816491, -0.004921259842519870586, -0.3153832671262229437 ) ) ;
#54964=CARTESIAN_POINT ( 'NONE',  ( -1.299212598425196097, -0.5511811023622047445, 6.969142054262312111E-17 ) ) ;
#54965=CARTESIAN_POINT ( 'NONE',  ( -1.030183727034119867, -0.3162353388693405765, 0.4822834645669290543 ) ) ;
#54966=CARTESIAN_POINT ( 'NONE',  ( 0.6627296587926515548, 0.2952755905511811885, 0.1292274648535926551 ) ) ;
#54967=CARTESIAN_POINT ( 'NONE',  ( -1.135170603674539924, 0.2952755905511810774, -0.1292274648535930714 ) ) ;
#54970=CARTESIAN_POINT ( 'NONE',  ( -1.358267716535432434, -0.5400638737290844871, 0.3530559997133364547 ) ) ;
#54976=CARTESIAN_POINT ( 'NONE',  ( -0.7414698162729651543, -0.6692913385826771977, 0.1292274648535927661 ) ) ;
#54977=CARTESIAN_POINT ( 'NONE',  ( 1.528871391076116026, 0.2952755905511811885, 0.1292274648535926551 ) ) ;
#54978=CARTESIAN_POINT ( 'NONE',  ( -1.574803149606298636, -0.1870078740157479769, 0.4822834645669291653 ) ) ;
#54980=CARTESIAN_POINT ( 'NONE',  ( 1.502624671916010790, -0.05778040916215522460, 0.4822834645669289988 ) ) ;
#54981=CARTESIAN_POINT ( 'NONE',  ( -0.8005249343832013809, -0.4281496062992124485, 0.4176697321401328655 ) ) ;
#54983=CARTESIAN_POINT ( 'NONE',  ( -0.1377952755905504645, 0.07958543189024085140, 0.2665933059059887866 ) ) ;
#54985=CARTESIAN_POINT ( 'NONE',  ( -0.2165354330708654795, 0.07958543189024085140, 0.2665933059059887866 ) ) ;
#54986=CARTESIAN_POINT ( 'NONE',  ( 0.8267716535433077274, 0.1771653543307087630, 0.000000000000000000 ) ) ;
#54987=CARTESIAN_POINT ( 'NONE',  ( 0.4724409448818904789, -0.1870078740157479769, 0.4822834645669291653 ) ) ;
#54988=CARTESIAN_POINT ( 'NONE',  ( -0.3937007874015740483, -0.1870078740157479769, 0.3641732283464567677 ) ) ;
#54990=CARTESIAN_POINT ( 'NONE',  ( 1.614173228346457378, 0.2952755905511811885, 0.000000000000000000 ) ) ;
#54991=CARTESIAN_POINT ( 'NONE',  ( -1.463254593175852492, 0.1771653543307087630, 0.09757992244046791164 ) ) ;
#54993=CARTESIAN_POINT ( 'NONE',  ( 0.07874015748031558404, -0.1870078740157480879, -0.4822834645669291653 ) ) ;
#54994=CARTESIAN_POINT ( 'NONE',  ( -0.3149606299212590610, -0.1870078740157480879, -0.4822834645669291653 ) ) ;
#54996=CARTESIAN_POINT ( 'NONE',  ( 0.07217847769028949700, -0.08942795157528024563, -0.3641732283464568787 ) ) ;
#54997=CARTESIAN_POINT ( 'NONE',  ( -0.4199475065616791736, 0.2306618581243847221, -0.2411417322834647770 ) ) ;
#54998=CARTESIAN_POINT ( 'NONE',  ( -0.5643044619422565855, -0.4281496062992124485, 0.4176697321401328655 ) ) ;
#54999=CARTESIAN_POINT ( 'NONE',  ( 1.572991167713778227, 1.535433070866141447, 0.1227090857360984416 ) ) ;
#55000=CARTESIAN_POINT ( 'NONE',  ( -0.7478466213799872531, 2.204724409448818978, 0.5309055118110236338 ) ) ;
#55001=CARTESIAN_POINT ( 'NONE',  ( 0.1509186351706045259, -0.05778040916215560624, -0.4822834645669293319 ) ) ;
#55004=CARTESIAN_POINT ( 'NONE',  ( -0.3149606299212590610, -0.1870078740157479769, 0.3641732283464567677 ) ) ;
#55005=CARTESIAN_POINT ( 'NONE',  ( -0.4724409448818890911, -0.1870078740157479769, 0.4822834645669291653 ) ) ;
#55006=CARTESIAN_POINT ( 'NONE',  ( 1.660104986876641320, -0.05778040916215522460, 0.4822834645669289988 ) ) ;
#55007=CARTESIAN_POINT ( 'NONE',  ( 1.325459317585302665, -0.4281496062992124485, 0.4176697321401328655 ) ) ;
#55008=CARTESIAN_POINT ( 'NONE',  ( -1.450131233595799651, 0.2952755905511810774, -0.1292274648535930714 ) ) ;
#55009=CARTESIAN_POINT ( 'NONE',  ( -0.8464566929133852113, -0.4536011799217368745, -0.2665933059059886201 ) ) ;
#55013=CARTESIAN_POINT ( 'NONE',  ( 1.463254593175853824, -0.5511811023622046335, 0.09757992244046803654 ) ) ;
#55014=CARTESIAN_POINT ( 'NONE',  ( 1.141732283464567566, 0.1771653543307087630, 0.000000000000000000 ) ) ;
#55015=CARTESIAN_POINT ( 'NONE',  ( 0.9251968503937015864, -0.5400638737290844871, 0.3530559997133364547 ) ) ;
#55016=CARTESIAN_POINT ( 'NONE',  ( 0.4527559055118117182, 0.1012011053420775880, -0.2882089793578256898 ) ) ;
#55017=CARTESIAN_POINT ( 'NONE',  ( 0.7480314960629927956, -0.6692913385826771977, 8.415575281601705876E-17 ) ) ;
#55019=CARTESIAN_POINT ( 'NONE',  ( 1.299212598425197429, -0.5511811023622047445, 6.969142054262312111E-17 ) ) ;
#55021=CARTESIAN_POINT ( 'NONE',  ( 0.3018372703412079971, 0.05413385826771626580, -0.4176697321401330321 ) ) ;
#55022=CARTESIAN_POINT ( 'NONE',  ( -0.7939632545931750718, -0.05778040916215560624, -0.4822834645669293319 ) ) ;
#55023=CARTESIAN_POINT ( 'NONE',  ( 1.272965879265092637, -0.4281496062992127816, -0.4176697321401328100 ) ) ;
#55026=CARTESIAN_POINT ( 'NONE',  ( 0.5052493438320215802, 0.1771653543307087630, 0.09757992244046791164 ) ) ;
#55029=ORIENTED_EDGE ( 'NONE', *, *, #81012, .F. ) ;
#55031=CARTESIAN_POINT ( 'NONE',  ( -0.4593175853018366950, 0.05413385826771666132, 0.4176697321401328100 ) ) ;
#55032=CARTESIAN_POINT ( 'NONE',  ( -0.3805774278215216522, 0.05413385826771666132, 0.4176697321401328100 ) ) ;
#55033=CARTESIAN_POINT ( 'NONE',  ( -0.4790026246719152336, -0.05778040916215560624, -0.4822834645669293319 ) ) ;
#55034=CARTESIAN_POINT ( 'NONE',  ( 0.9908136482939640111, -0.6692913385826771977, 0.1292274648535927661 ) ) ;
#55035=CARTESIAN_POINT ( 'NONE',  ( -0.7545931758530176614, -0.6692913385826773087, -0.1292274648535924053 ) ) ;
#55036=CARTESIAN_POINT ( 'NONE',  ( -0.5380577427821514602, -0.4281496062992127816, -0.4176697321401328100 ) ) ;
#55037=CARTESIAN_POINT ( 'NONE',  ( 1.240157480314961314, -0.5400638737290844871, 0.3530559997133364547 ) ) ;
#55038=CARTESIAN_POINT ( 'NONE',  ( 0.4133858267716541968, -0.5400638737290845981, -0.3530559997133363437 ) ) ;
#55039=CARTESIAN_POINT ( 'NONE',  ( 0.6496062992125991586, -0.5400638737290845981, -0.3530559997133363437 ) ) ;
#55041=CARTESIAN_POINT ( 'NONE',  ( 0.1181102362204730916, 0.1771653543307087630, 0.000000000000000000 ) ) ;
#55045=CARTESIAN_POINT ( 'NONE',  ( -0.6889763779527552368, -0.4536011799217368745, -0.2665933059059886201 ) ) ;
#55046=CARTESIAN_POINT ( 'NONE',  ( -0.5708661417322825615, -0.5400638737290844871, 0.3530559997133364547 ) ) ;
#55048=CARTESIAN_POINT ( 'NONE',  ( -0.5905511811023615998, 0.2952755905511811885, 0.000000000000000000 ) ) ;
#55049=CARTESIAN_POINT ( 'NONE',  ( -0.6496062992125976043, -0.5400638737290844871, 0.3530559997133364547 ) ) ;
#55050=CARTESIAN_POINT ( 'NONE',  ( -1.279527559055116948, 0.1660481256975883668, -0.3530559997133364547 ) ) ;
#55051=CARTESIAN_POINT ( 'NONE',  ( -1.220472440944881054, 0.2952755905511811885, 0.000000000000000000 ) ) ;
#55052=CARTESIAN_POINT ( 'NONE',  ( 1.049868766404200349, 0.1283753931104748280, 0.1820866141732283561 ) ) ;
#55054=CARTESIAN_POINT ( 'NONE',  ( 0.6167979002624678353, -0.3690944881889763329, 0.3153832671262228327 ) ) ;
#55055=CARTESIAN_POINT ( 'NONE',  ( 0.09842519685039434474, 0.1660481256975885056, 0.3530559997133364547 ) ) ;
#55056=CARTESIAN_POINT ( 'NONE',  ( -0.08530183727034056085, -0.3162353388693405765, 0.4822834645669290543 ) ) ;
#55057=ORIENTED_EDGE ( 'NONE', *, *, #27581, .F. ) ;
#55063=CARTESIAN_POINT ( 'NONE',  ( -0.9055118110236215490, 0.1771653543307087630, 0.000000000000000000 ) ) ;
#55064=CARTESIAN_POINT ( 'NONE',  ( -0.9711286089238838626, -0.6046776061558807314, 0.2411417322834647770 ) ) ;
#55067=CARTESIAN_POINT ( 'NONE',  ( 1.587926509186352586, -0.4281496062992127816, -0.4176697321401328100 ) ) ;
#55068=CARTESIAN_POINT ( 'NONE',  ( 0.5839895013123367340, -0.6692913385826773087, -0.1292274648535924053 ) ) ;
#55069=CARTESIAN_POINT ( 'NONE',  ( 0.5118110236220480003, -0.6692913385826771977, 8.415575281601705876E-17 ) ) ;
#55070=CARTESIAN_POINT ( 'NONE',  ( -0.7677165354330699465, -0.4536011799217368745, -0.2665933059059886201 ) ) ;
#55071=CARTESIAN_POINT ( 'NONE',  ( 0.2362204724409456558, -0.1870078740157480879, -0.4822834645669291653 ) ) ;
#55073=CARTESIAN_POINT ( 'NONE',  ( -0.6233595800524928121, -0.05778040916215522460, 0.4822834645669289988 ) ) ;
#55075=CARTESIAN_POINT ( 'NONE',  ( 1.332020997375328974, -0.08942795157528024563, -0.3641732283464568787 ) ) ;
#55076=CARTESIAN_POINT ( 'NONE',  ( 0.2887139107611556010, -0.5023911411419708095, 0.1820866141732285504 ) ) ;
#55077=CARTESIAN_POINT ( 'NONE',  ( 1.062992125984252745, 0.1771653543307087630, 0.000000000000000000 ) ) ;
#55078=CARTESIAN_POINT ( 'NONE',  ( -1.246719160104986512, 0.05413385826771666132, 0.4176697321401328100 ) ) ;
#55079=CARTESIAN_POINT ( 'NONE',  ( -1.318897637795274802, 0.07958543189024085140, 0.2665933059059887866 ) ) ;
#55081=CARTESIAN_POINT ( 'NONE',  ( -1.161417322834644716, -0.5400638737290845981, -0.3530559997133363437 ) ) ;
#55082=CARTESIAN_POINT ( 'NONE',  ( -0.5249343832020990641, 0.2306618581243848609, 0.2411417322834645549 ) ) ;
#55083=CARTESIAN_POINT ( 'NONE',  ( 0.4199475065616805614, 0.2306618581243848609, 0.2411417322834645549 ) ) ;
#55086=CARTESIAN_POINT ( 'NONE',  ( 0.4527559055118117182, 0.07958543189024071263, -0.2665933059059888421 ) ) ;
#55087=CARTESIAN_POINT ( 'NONE',  ( 0.9120734908136489683, -0.6692913385826771977, 0.1292274648535927661 ) ) ;
#55088=CARTESIAN_POINT ( 'NONE',  ( -1.581364829396324945, -0.2845877964562159024, 0.3641732283464567677 ) ) ;
#55089=CARTESIAN_POINT ( 'NONE',  ( 0.9317585301837276734, 0.05413385826771626580, -0.4176697321401330321 ) ) ;
#55090=CARTESIAN_POINT ( 'NONE',  ( -1.614173228346456268, -0.5511811023622047445, 6.969142054262312111E-17 ) ) ;
#55091=CARTESIAN_POINT ( 'NONE',  ( -1.417322834645668772, -0.1870078740157479769, 0.4822834645669291653 ) ) ;
#55092=EDGE_CURVE ( 'NONE', #74087, #66780, #78615, .T. ) ;
#55093=CARTESIAN_POINT ( 'NONE',  ( -0.8727034120734901146, -0.05778040916215560624, -0.4822834645669293319 ) ) ;
#55094=CARTESIAN_POINT ( 'NONE',  ( 0.01968503937007957949, -0.4536011799217368745, -0.2665933059059886201 ) ) ;
#55095=CARTESIAN_POINT ( 'NONE',  ( 1.614173228346457378, 0.2753471884572480932, -0.1372047244094471152 ) ) ;
#55096=CARTESIAN_POINT ( 'NONE',  ( 0.8070866141732288002, 0.07958543189024085140, 0.2665933059059887866 ) ) ;
#55098=CARTESIAN_POINT ( 'NONE',  ( -0.1181102362204717315, -0.6692913385826771977, 8.415575281601705876E-17 ) ) ;
#55100=CARTESIAN_POINT ( 'NONE',  ( -1.299212598425196097, -0.6692913385826771977, 8.415575281601705876E-17 ) ) ;
#55102=CARTESIAN_POINT ( 'NONE',  ( 0.8595800524934390507, -0.08942795157528024563, -0.3641732283464568787 ) ) ;
#55103=CARTESIAN_POINT ( 'NONE',  ( 0.1049868766404206816, 0.2306618581243848609, 0.2411417322834645549 ) ) ;
#55104=CARTESIAN_POINT ( 'NONE',  ( -0.2296587926509179312, -0.05778040916215522460, 0.4822834645669289988 ) ) ;
#55105=CARTESIAN_POINT ( 'NONE',  ( -0.5380577427821514602, -0.004921259842519576551, 0.3153832671262227771 ) ) ;
#55106=CARTESIAN_POINT ( 'NONE',  ( 1.003937007874016185, 0.1012011053420775880, -0.2882089793578257453 ) ) ;
#55107=CARTESIAN_POINT ( 'NONE',  ( -0.4790026246719152336, -0.08942795157528024563, -0.3641732283464568787 ) ) ;
#55108=CARTESIAN_POINT ( 'NONE',  ( 0.2690288713910767848, 0.2952755905511811885, 0.1292274648535926551 ) ) ;
#55109=CARTESIAN_POINT ( 'NONE',  ( -1.351706036745406347, -0.004921259842519870586, -0.3153832671262229437 ) ) ;
#55111=CARTESIAN_POINT ( 'NONE',  ( -1.620734908136482577, 0.2952755905511811885, 0.1292274648535926551 ) ) ;
#55114=CARTESIAN_POINT ( 'NONE',  ( -1.666666666666665853, -0.004921259842519870586, -0.3153832671262229437 ) ) ;
#55115=CARTESIAN_POINT ( 'NONE',  ( -0.6233595800524928121, -0.05778040916215522460, 0.4822834645669289988 ) ) ;
#55116=CARTESIAN_POINT ( 'NONE',  ( -1.266404199475064773, -0.05778040916215560624, -0.4822834645669293319 ) ) ;
#55119=CARTESIAN_POINT ( 'NONE',  ( 1.463254593175853824, -0.6692913385826771977, 0.1292274648535927661 ) ) ;
#55120=CARTESIAN_POINT ( 'NONE',  ( 0.5118110236220480003, -0.6692913385826771977, 8.415575281601705876E-17 ) ) ;
#55121=PLANE ( 'NONE',  #44841 ) ;
#55123=CARTESIAN_POINT ( 'NONE',  ( 1.528871391076116026, -0.5511811023622048555, -0.09757992244046775898 ) ) ;
#55126=CARTESIAN_POINT ( 'NONE',  ( -0.7939632545931750718, -0.08942795157528024563, -0.3641732283464568787 ) ) ;
#55129=CARTESIAN_POINT ( 'NONE',  ( 0.9645669291338588858, 0.1660481256975885056, 0.3530559997133364547 ) ) ;
#55130=CARTESIAN_POINT ( 'NONE',  ( -0.5380577427821514602, -0.4281496062992127816, -0.4176697321401328100 ) ) ;
#55131=CARTESIAN_POINT ( 'NONE',  ( -1.003937007874014853, 0.1660481256975885056, 0.3530559997133364547 ) ) ;
#55132=CARTESIAN_POINT ( 'NONE',  ( 1.167979002624672580, -0.4281496062992124485, 0.4176697321401328655 ) ) ;
#55133=CARTESIAN_POINT ( 'NONE',  ( -1.358267716535432434, -0.4536011799217367080, 0.2665933059059888421 ) ) ;
#55135=CARTESIAN_POINT ( 'NONE',  ( 0.1771653543307093182, -0.5400638737290845981, -0.3530559997133363437 ) ) ;
#55136=CARTESIAN_POINT ( 'NONE',  ( -0.8661417322834640276, -0.1870078740157479769, 0.4822834645669291653 ) ) ;
#55138=CARTESIAN_POINT ( 'NONE',  ( -1.220472440944881054, -0.6692913385826771977, 8.415575281601705876E-17 ) ) ;
#55140=CARTESIAN_POINT ( 'NONE',  ( 1.049868766404200349, 0.2306618581243848609, 0.2411417322834645549 ) ) ;
#55142=CARTESIAN_POINT ( 'NONE',  ( 1.194225721784777594, -0.004921259842519576551, 0.3153832671262227771 ) ) ;
#55143=VERTEX_POINT ( 'NONE', #79712 ) ;
#55145=CARTESIAN_POINT ( 'NONE',  ( -0.2165354330708654795, 0.1660481256975885056, 0.3530559997133364547 ) ) ;
#55146=ORIENTED_EDGE ( 'NONE', *, *, #3457, .F. ) ;
#55147=CARTESIAN_POINT ( 'NONE',  ( 0.3018372703412079971, -0.3690944881889763329, 0.3153832671262228327 ) ) ;
#55148=CARTESIAN_POINT ( 'NONE',  ( -1.627296587926508442, -0.6046776061558809534, -0.2411417322834644161 ) ) ;
#55149=CARTESIAN_POINT ( 'NONE',  ( 0.6299212598425204535, -0.1870078740157479769, 0.4822834645669291653 ) ) ;
#55150=CARTESIAN_POINT ( 'NONE',  ( 0.7349081364829402885, -0.6046776061558809534, -0.2411417322834644161 ) ) ;
#55151=CARTESIAN_POINT ( 'NONE',  ( -0.2034120734908131112, -0.6692913385826773087, -0.1292274648535924053 ) ) ;
#55153=CARTESIAN_POINT ( 'NONE',  ( -0.7283464566929126471, -0.5400638737290844871, 0.3530559997133364547 ) ) ;
#55155=CARTESIAN_POINT ( 'NONE',  ( -1.673228346456691717, 0.1660481256975883668, -0.3530559997133364547 ) ) ;
#55156=CARTESIAN_POINT ( 'NONE',  ( -0.8661417322834640276, -0.1870078740157479769, 0.4822834645669291653 ) ) ;
#55157=CARTESIAN_POINT ( 'NONE',  ( 1.220472440944882608, 0.2952755905511811885, 0.000000000000000000 ) ) ;
#55158=CARTESIAN_POINT ( 'NONE',  ( 1.167979002624672580, -0.4281496062992124485, 0.4176697321401328655 ) ) ;
#55161=CARTESIAN_POINT ( 'NONE',  ( -1.115485564304461219, -0.4281496062992124485, 0.4176697321401328655 ) ) ;
#55163=CARTESIAN_POINT ( 'NONE',  ( 0.3280839895013130669, 0.05413385826771666132, 0.4176697321401328100 ) ) ;
#55166=CARTESIAN_POINT ( 'NONE',  ( -0.3740157480314953431, 0.1660481256975885056, 0.3530559997133364547 ) ) ;
#55167=CARTESIAN_POINT ( 'NONE',  ( -1.482939632545930975, -0.004921259842519576551, 0.3153832671262227771 ) ) ;
#55168=CARTESIAN_POINT ( 'NONE',  ( 0.7349081364829403995, 0.1283753931104748280, 0.1820866141732283561 ) ) ;
#55169=CARTESIAN_POINT ( 'NONE',  ( 1.135170603674541256, 0.2952755905511811885, 0.1292274648535926551 ) ) ;
#55171=CARTESIAN_POINT ( 'NONE',  ( 0.6955380577427828781, -0.3690944881889763329, 0.3153832671262228327 ) ) ;
#55172=CARTESIAN_POINT ( 'NONE',  ( 0.7020997375328090762, -0.05778040916215560624, -0.4822834645669293319 ) ) ;
#55174=CARTESIAN_POINT ( 'NONE',  ( -0.4790026246719154557, -0.3162353388693405765, 0.4822834645669290543 ) ) ;
#55176=CARTESIAN_POINT ( 'NONE',  ( 1.167979002624672580, -0.004921259842519870586, -0.3153832671262229437 ) ) ;
#55177=CARTESIAN_POINT ( 'NONE',  ( -0.5774278215223089816, 0.2306618581243847221, -0.2411417322834647770 ) ) ;
#55178=CARTESIAN_POINT ( 'NONE',  ( 0.06561679790026316017, 0.05413385826771626580, -0.4176697321401330321 ) ) ;
#55179=CARTESIAN_POINT ( 'NONE',  ( -2.795275590551184575, 0.7480314960629931287, -3.317813449798768424E-16 ) ) ;
#55180=CARTESIAN_POINT ( 'NONE',  ( 0.1837270341207354329, 0.2306618581243848609, 0.2411417322834645549 ) ) ;
#55181=CARTESIAN_POINT ( 'NONE',  ( 0.5249343832021005074, -0.5023911411419708095, 0.1820866141732285504 ) ) ;
#55184=CARTESIAN_POINT ( 'NONE',  ( -0.1509186351706028884, -0.2845877964562161244, -0.3641732283464567121 ) ) ;
#55185=CARTESIAN_POINT ( 'NONE',  ( 0.6561679790026253567, 0.1283753931104748280, 0.1820866141732283561 ) ) ;
#55186=FACE_OUTER_BOUND ( 'NONE', #81983, .T. ) ;
#55188=CARTESIAN_POINT ( 'NONE',  ( 0.1312335958005257930, 0.2306618581243847221, -0.2411417322834647770 ) ) ;
#55191=CARTESIAN_POINT ( 'NONE',  ( 1.482939632545932307, -0.3690944881889763329, 0.3153832671262228327 ) ) ;
#55192=CARTESIAN_POINT ( 'NONE',  ( 0.1443569553805781891, 0.05413385826771626580, -0.4176697321401330321 ) ) ;
#55193=CARTESIAN_POINT ( 'NONE',  ( 0.1902887139107617975, 0.1771653543307087630, 0.09757992244046791164 ) ) ;
#55194=CARTESIAN_POINT ( 'NONE',  ( 0.2887139107611556010, 0.2306618581243847221, -0.2411417322834647770 ) ) ;
#55195=CARTESIAN_POINT ( 'NONE',  ( 1.384514435695538559, 0.1771653543307087075, -0.09757992244046823083 ) ) ;
#55196=CARTESIAN_POINT ( 'NONE',  ( -1.187664041994750175, -0.08942795157528024563, -0.3641732283464568787 ) ) ;
#55197=CARTESIAN_POINT ( 'NONE',  ( -1.568241469816272105, -0.05778040916215522460, 0.4822834645669289988 ) ) ;
#55198=CARTESIAN_POINT ( 'NONE',  ( 0.2821522309711292364, 0.2952755905511810774, -0.1292274648535930714 ) ) ;
#55199=CARTESIAN_POINT ( 'NONE',  ( 1.036745406824147731, 0.05413385826771666132, 0.4176697321401328100 ) ) ;
#55201=CARTESIAN_POINT ( 'NONE',  ( 0.3083989501312343062, -0.3162353388693405765, 0.4822834645669290543 ) ) ;
#55202=CARTESIAN_POINT ( 'NONE',  ( 1.246719160104987623, 0.05413385826771626580, -0.4176697321401330321 ) ) ;
#55203=CARTESIAN_POINT ( 'NONE',  ( 0.8136482939632553313, -0.6046776061558809534, -0.2411417322834644161 ) ) ;
#55204=CARTESIAN_POINT ( 'NONE',  ( -1.595398199321655275, 2.136509776695170615, -0.1559797534342494130 ) ) ;
#55205=CARTESIAN_POINT ( 'NONE',  ( 0.7480314960629927956, 0.1771653543307087630, 0.000000000000000000 ) ) ;
#55206=CARTESIAN_POINT ( 'NONE',  ( -1.535433070866141225, -0.5511811023622047445, 6.969142054262312111E-17 ) ) ;
#55207=CARTESIAN_POINT ( 'NONE',  ( 0.3018372703412079971, -0.3690944881889763329, 0.3153832671262228327 ) ) ;
#55208=CARTESIAN_POINT ( 'NONE',  ( 0.1771653543307093182, -0.5400638737290845981, -0.3530559997133363437 ) ) ;
#55209=CARTESIAN_POINT ( 'NONE',  ( 0.5511811023622054106, -0.1870078740157480879, -0.4822834645669291653 ) ) ;
#55210=CARTESIAN_POINT ( 'NONE',  ( -0.2755905511811015396, -0.6692913385826771977, 8.415575281601705876E-17 ) ) ;
#55212=CARTESIAN_POINT ( 'NONE',  ( -0.1115485564304456306, 0.1771653543307087075, -0.09757992244046823083 ) ) ;
#55214=CARTESIAN_POINT ( 'NONE',  ( 0.6167979002624678353, -0.4281496062992124485, 0.4176697321401328655 ) ) ;
#55215=CARTESIAN_POINT ( 'NONE',  ( 1.056430446194226658, 0.1771653543307087630, 0.09757992244046791164 ) ) ;
#55217=CARTESIAN_POINT ( 'NONE',  ( -1.082677165354329896, 0.1660481256975885056, 0.3530559997133364547 ) ) ;
#55220=CARTESIAN_POINT ( 'NONE',  ( -1.089238845144356427, -0.4281496062992127816, -0.4176697321401328100 ) ) ;
#55221=CARTESIAN_POINT ( 'NONE',  ( -0.4199475065616791736, 0.2306618581243847221, -0.2411417322834647770 ) ) ;
#55225=CARTESIAN_POINT ( 'NONE',  ( 0.1706036745406830368, -0.3690944881889765550, -0.3153832671262227771 ) ) ;
#55227=CARTESIAN_POINT ( 'NONE',  ( 1.246719160104987623, -0.4281496062992124485, 0.4176697321401328655 ) ) ;
#55230=CARTESIAN_POINT ( 'NONE',  ( -0.2462293917967295909, -2.567464376874931580E-15, -0.4445507791589072832 ) ) ;
#55233=CARTESIAN_POINT ( 'NONE',  ( 1.272965879265092637, -0.004921259842519576551, 0.3153832671262227771 ) ) ;
#55234=CARTESIAN_POINT ( 'NONE',  ( 0.2230971128608932319, -0.4281496062992124485, 0.4176697321401328655 ) ) ;
#55237=CARTESIAN_POINT ( 'NONE',  ( -0.006561679790025524116, -0.05778040916215560624, -0.4822834645669293319 ) ) ;
#55238=CARTESIAN_POINT ( 'NONE',  ( -1.076115485564303809, 0.1283753931104748280, 0.1820866141732283561 ) ) ;
#55239=CARTESIAN_POINT ( 'NONE',  ( 0.3412073490813655186, 0.2306618581243848609, 0.2411417322834645549 ) ) ;
#55240=CARTESIAN_POINT ( 'NONE',  ( -0.09186351706036689768, 0.05413385826771626580, -0.4176697321401330321 ) ) ;
#55244=CARTESIAN_POINT ( 'NONE',  ( 0.8530183727034128527, -0.4281496062992124485, 0.4176697321401328655 ) ) ;
#55245=CARTESIAN_POINT ( 'NONE',  ( -0.2559055118110230564, 0.1660481256975883668, -0.3530559997133364547 ) ) ;
#55246=CARTESIAN_POINT ( 'NONE',  ( -1.128608923884513837, 0.2306618581243847221, -0.2411417322834647770 ) ) ;
#55247=CARTESIAN_POINT ( 'NONE',  ( 1.167979002624672580, 0.05413385826771626580, -0.4176697321401330321 ) ) ;
#55248=CARTESIAN_POINT ( 'NONE',  ( 0.4527559055118117182, 0.1660481256975883668, -0.3530559997133364547 ) ) ;
#55250=CARTESIAN_POINT ( 'NONE',  ( -0.5577427821522301654, -0.05778040916215560624, -0.4822834645669293319 ) ) ;
#55251=CARTESIAN_POINT ( 'NONE',  ( 0.2296587926509192634, -0.3162353388693405765, 0.4822834645669290543 ) ) ;
#55252=CARTESIAN_POINT ( 'NONE',  ( -0.5971128608923877978, -0.6692913385826773087, -0.1292274648535924053 ) ) ;
#55253=CARTESIAN_POINT ( 'NONE',  ( 0.1640419947506569498, -0.2845877964562161244, -0.3641732283464567121 ) ) ;
#55254=CARTESIAN_POINT ( 'NONE',  ( 1.633858267716535639, -0.4536011799217367080, 0.2665933059059888421 ) ) ;
#55256=CARTESIAN_POINT ( 'NONE',  ( 0.2559055118110243332, -0.5400638737290845981, -0.3530559997133363437 ) ) ;
#55257=CARTESIAN_POINT ( 'NONE',  ( 1.509186351706037543, -0.4281496062992127816, -0.4176697321401328100 ) ) ;
#55261=CARTESIAN_POINT ( 'NONE',  ( 0.6824146981627303710, -0.6046776061558807314, 0.2411417322834647770 ) ) ;
#55262=CARTESIAN_POINT ( 'NONE',  ( 0.4133858267716541968, -0.4536011799217368745, -0.2665933059059886201 ) ) ;
#55263=FACE_OUTER_BOUND ( 'NONE', #31660, .T. ) ;
#55269=CARTESIAN_POINT ( 'NONE',  ( 0.7874015748031503170, -0.1870078740157479769, 0.4822834645669291653 ) ) ;
#55270=CARTESIAN_POINT ( 'NONE',  ( -0.6233595800524928121, -0.3162353388693409650, -0.4822834645669289433 ) ) ;
#55271=CARTESIAN_POINT ( 'NONE',  ( -0.7217847769028863381, 0.05413385826771626580, -0.4176697321401330321 ) ) ;
#55272=CARTESIAN_POINT ( 'NONE',  ( 0.4855643044619428750, 0.05413385826771666132, 0.4176697321401328100 ) ) ;
#55273=VECTOR ( 'NONE', #6187, 39.37007874015748143 ) ;
#55274=CARTESIAN_POINT ( 'NONE',  ( 1.404199475065617264, -0.4281496062992124485, 0.4176697321401328655 ) ) ;
#55277=CARTESIAN_POINT ( 'NONE',  ( 1.213910761154856299, 0.1771653543307087630, 0.09757992244046791164 ) ) ;
#55278=DIRECTION ( 'NONE',  ( -0.7071067811865495711, -0.000000000000000000, 0.7071067811865454633 ) ) ;
#55279=CARTESIAN_POINT ( 'NONE',  ( -1.161417322834644716, 0.07958543189024085140, 0.2665933059059887866 ) ) ;
#55280=LINE ( 'NONE', #80169, #3312 ) ;
#55281=CARTESIAN_POINT ( 'NONE',  ( 0.1706036745406830368, -0.4281496062992127816, -0.4176697321401328100 ) ) ;
#55282=CARTESIAN_POINT ( 'NONE',  ( 1.115485564304462551, -0.4281496062992127816, -0.4176697321401328100 ) ) ;
#55284=CARTESIAN_POINT ( 'NONE',  ( -1.174540682414697335, -0.2845877964562161244, -0.3641732283464567121 ) ) ;
#55285=CARTESIAN_POINT ( 'NONE',  ( 0.4593175853018380828, 0.05413385826771626580, -0.4176697321401330321 ) ) ;
#55286=CARTESIAN_POINT ( 'NONE',  ( 1.437007874015748810, 0.07958543189024085140, 0.2665933059059887866 ) ) ;
#55288=CARTESIAN_POINT ( 'NONE',  ( -1.384514435695537005, 0.1771653543307087630, 0.09757992244046791164 ) ) ;
#55289=CARTESIAN_POINT ( 'NONE',  ( 1.489501312335958172, -0.3162353388693405765, 0.4822834645669290543 ) ) ;
#55292=CARTESIAN_POINT ( 'NONE',  ( -0.2559055118110230564, 0.07958543189024071263, -0.2665933059059888421 ) ) ;
#55293=CARTESIAN_POINT ( 'NONE',  ( 0.02624671916010564918, 0.2306618581243848609, 0.2411417322834645549 ) ) ;
#55294=CARTESIAN_POINT ( 'NONE',  ( -1.174540682414697335, -0.08942795157527998196, 0.3641732283464567121 ) ) ;
#55295=CARTESIAN_POINT ( 'NONE',  ( -0.9055118110236215490, 0.2952755905511811885, 0.000000000000000000 ) ) ;
#55296=CARTESIAN_POINT ( 'NONE',  ( 1.167979002624672580, -0.4281496062992124485, 0.4176697321401328655 ) ) ;
#55298=( BOUNDED_SURFACE ( )  B_SPLINE_SURFACE ( 1, 2, ( 
 ( #35964, #11947, #56540, #55711, #81835, #61207, #10713, #80600, #49408, #17449, #75102, #30873, #3975, #11536, #29639, #30466, #81420, #11120, #24146, #37193, #42260, #23736, #24560, #61634, #36370, #82241, #3563, #62044, #36777, #4381, #55300, #29229, #42676, #43490, #81008, #67955, #56129, #50226, #17855, #62453, #43079, #62873, #5209, #75922, #30049, #49816, #23322, #68374, #68776, #4789, #48577, #18261, #74690, #69186, #43903, #75516, #16618, #22909, #69600, #74274, #10298, #48992, #17036, #77157, #38844, #25794, #83054, #63690, #71261, #19489, #32530, #38014, #63276, #44311, #25377, #19916, #45566, #987, #82645, #51040, #12772, #18666, #13607, #6446, #58194, #57359, #44719, #51454, #38429, #24959, #52296, #76741, #77583, #64943, #64524, #76336, #71678, #39261, #45142, #70417, #70846, #7283, #13196, #6861, #562, #19071, #6029, #32953, #26215, #51877, #31700, #5616, #70001, #64112, #58619, #26642, #78002, #50631, #32117, #57775, #12356, #20330, #45982, #138, #37602, #31283, #56948, #27889, #73347, #67033, #7713, #2224, #33380, #53549, #65793, #21990, #78839, #72095, #52712, #79257, #72923, #14454, #33792, #40105, #3050, #9365, #1398, #59457, #54379, #72512, #41352, #60701, #8127, #15275, #1808, #59044, #40523, #27054, #35036, #27470, #21572, #78424, #46821, #14030, #65378, #39686, #15694, #53128, #48066, #28716, #8541, #34627, #20752, #14861, #46402, #47234, #40936, #66615, #80089, #21165, #47651, #66202, #8952, #34207, #60291, #2641, #22410, #59870, #28298, #53960, #79673, #23222, #43385, #73769, #48892, #23632, #74593, #48474, #16103, #55201, #56027, #10199, #80501, #68675, #69086, #30358, #49304, #55609, #24044, #49715, #11434, #68279, #75005, #67443, #42980, #81735, #37089, #29538, #62775, #75411, #67862, #16937, #42577, #81320, #35868, #35448, #61113, #5109, #17755, #61534, #10614, #24455, #17352, #36271, #54798, #61942, #3465, #11016, #22817, #3879, #36673, #30776, #62349, #4283, #56437, #29945, #4687, #74176, #82140, #41748, #16522, #80909, #9776, #29131, #42167, #70736, #43793, #18567, #71158, #69900, #35, #64419, #31179, #32426, #12666, #13090, #77052, #56844, #76233, #12254, #38743, #37911, #57251, #77474, #58517, #6754, #38326, #82542, #39154, #58089, #45460, #75820, #454, #63999, #24860, #6341, #32013, #82954, #25272, #51771, #13498, #26110, #19385, #45037, #11848, #76636, #63588, #19811, #70311, #64839, #57673, #7177, #50121, #32848, #880, #18162, #5923, #37501, #25688, #50527, #69499, #63176, #5514, #44210, #31595, #50939, #18967, #51349, #44616, #1709, #65696, #66099, #15591, #60190, #60603, #71574, #45876, #65271, #33689, #28199, #1300, #21060, #66937, #71996, #46721, #8026, #27364, #27786, #72413, #14762, #2121, #20228, #79157, #66515, #47550, #59350, #79570, #8847, #20649, #53025, #78738, #8435, #46302, #13925, #39582, #41249, #53858, #14349, #40418, #26540, #59766, #34105, #7607, #53449, #33281, #21474, #58942, #40009, #47132, #73242, #15173, #72823, #2541, #40830, #34524, #26949, #21886, #9269, #52612, #34940, #52193, #77897, #78318, #24667, #79991, #54695, #25071, #22716, #37309, #18377, #67346, #69711, #48792, #50335, #30980, #9679, #29027, #48375, #76032, #74074, #10097, #31392, #12461, #44017, #74490, #35350, #76443, #12055, #82749, #28617, #37712, #16837, #61012, #43600, #69302, #35761, #61428, #5721, #50745, #63386, #56648, #82348, #47965, #29441, #16420, #57057, #23124, #18772, #11651, #44415, #2952, #70110, #38123, #54275, #42066, #73667, #62983, #3363, #22305, #16009, #41655, #80404, #67761, #3778, #55100, #5322, #80809, #38951, #19595, #20022, #52824, #14143, #14564, #25483, #83164, #19178, #70954, #65490, #38540, #58305, #20859, #25902, #670, #45258, #64635, #65058, #26325, #70524, #44827, #77692, #39795, #33489, #57470, #51987, #51150, #45673, #32226, #71789, #13299, #64220, #12880, #71369, #39372, #6554, #250, #57883, #78536, #59151, #76844, #51563, #46511, #6970, #7822, #27161, #77266, #7395, #32641, #13719, #33063, #58734, #1508, #1096, #26747, #52402, #78111, #63797, #31810, #6135, #72212, #20443, #46097 ),
 ( #34740, #14969, #15384, #29245, #21273, #47345, #48181, #22519, #67144, #60810, #33899, #8649, #61224, #59982, #73459, #54491, #46928, #73878, #2751, #3163, #9474, #72621, #66309, #2340, #28827, #27997, #73034, #67556, #48592, #80202, #28411, #40627, #54909, #16217, #35561, #65898, #41864, #54070, #34320, #79785, #22101, #41046, #66731, #9891, #3578, #80615, #35147, #22927, #1920, #9069, #53656, #74289, #60401, #40216, #47761, #8234, #59564, #27583, #53239, #78955, #79364, #21683, #15810, #41460, #82255, #63292, #69616, #50647, #10728, #36385, #74706, #5631, #11961, #3991, #62059, #56962, #75119, #43918, #31298, #42692, #17870, #17051, #61650, #43095, #29655, #37617, #68389, #30481, #55317, #49424, #16633, #67972, #42275, #75937, #4398, #10315, #82660, #11136, #37208, #35980, #17464, #81025, #4805, #56147, #81850, #24974, #30065, #50241, #55728, #69204, #36795, #49831, #62888, #18278, #23338, #62470, #49007, #81436, #68791, #23751, #24162, #75530, #43504, #11552, #5224, #30887, #56555, #24574, #12787, #83071, #71273, #71692, #32966, #26228, #58208, #26655, #52309, #14044, #45156, #13622, #38443, #154, #64538, #51468, #63704, #7726, #6461, #58633, #20344, #77596, #31716, #27068, #78016, #6875, #25807, #575, #45995, #32544, #19930, #51892, #64125, #19086, #39700, #45580, #39274, #76755, #18681, #25391, #32131, #1001, #65391, #33395, #38029, #57788, #77170, #57375, #59057, #64959, #51055, #19502, #44734, #70430, #7296, #1412, #76350, #70017, #44325, #12370, #6044, #70859, #13210, #38857, #27483, #8140, #40949, #28312, #53141, #9377, #2654, #34640, #3061, #28729, #73779, #21585, #73358, #72526, #59883, #66628, #27902, #40119, #67454, #66215, #35047, #80101, #53973, #33805, #3475, #54390, #8966, #2237, #60305, #22420, #79686, #22003, #47663, #14875, #78853, #48077, #15706, #41363, #21179, #78438, #59470, #40536, #60712, #16115, #41760, #14467, #8554, #53562, #1823, #9788, #67044, #46834, #34221, #79271, #47248, #35459, #61124, #52726, #46416, #20765, #72109, #65807, #72937, #15289, #10626, #3890, #67872, #17363, #4698, #29550, #48904, #55212, #18174, #82152, #16533, #74605, #69511, #4294, #56450, #75833, #80920, #30371, #23235, #74187, #55622, #42178, #24468, #16948, #42991, #10210, #61954, #29142, #80512, #54808, #5120, #42590, #63188, #50134, #23645, #49726, #22827, #29957, #48485, #68685, #11028, #36685, #43807, #68290, #62786, #36282, #81746, #49316, #62360, #75423, #30787, #35878, #75017, #11860, #81331, #56038, #37513, #61546, #24056, #17766, #43398, #69097, #11445, #37101, #71171, #25284, #12266, #468, #897, #5527, #52207, #77911, #45890, #18980, #76245, #13102, #69912, #13512, #20242, #58531, #39597, #82966, #32439, #71588, #38756, #6768, #64014, #44629, #45050, #13940, #39168, #31192, #50541, #24873, #44222, #12681, #7191, #63601, #48, #56858, #50952, #25701, #70325, #6355, #58102, #51362, #77066, #64433, #82555, #26124, #45474, #26554, #38339, #18579, #64853, #76649, #32026, #57686, #70751, #19399, #37924, #5937, #31607, #32863, #51785, #77489, #57268, #19824, #34120, #46317, #27803, #52627, #60205, #72010, #27380, #72837, #28633, #53872, #79171, #41265, #40433, #59781, #40023, #66114, #54290, #14366, #72428, #73257, #47564, #8861, #2555, #58956, #33704, #2966, #1723, #15187, #79586, #65711, #15605, #53463, #28213, #34539, #8041, #59364, #53041, #21900, #78753, #14778, #9283, #73682, #66951, #21488, #21078, #80006, #34954, #60617, #7624, #22319, #47147, #46736, #40844, #66530, #8449, #2135, #47982, #16022, #65286, #33296, #1314, #26963, #78333, #20664, #30273, #61856, #10930, #4197, #82056, #17266, #35364, #36586, #81651, #62684, #80823, #11348, #23962, #35775, #74505, #68190, #23548, #61445, #3378, #29041, #56358, #68996, #29456, #42487, #75736, #74922, #10529, #22730, #29860, #54712, #62265, #48389, #3792, #49216, #5026, #55936, #55523, #17668, #16852, #36184, #16434, #81232, #30694, #74088, #48806, #49628, #75322, #68589, #4602, #61029, #10114, #24370, #55114, #42895, #43299, #42080, #37006, #50040, #41669, #67360, #67775, #23137, #9693 ) ),
 .UNSPECIFIED., .F., .F., .F. ) 
 B_SPLINE_SURFACE_WITH_KNOTS ( ( 2, 2 ),
 ( 3, 2, 2, 2, 2, 2, 2, 2, 2, 2, 2, 2, 2, 2, 2, 2, 2, 2, 2, 2, 2, 2, 2, 2, 2, 2, 2, 2, 2, 2, 2, 2, 2, 2, 2, 2, 2, 2, 2, 2, 2, 2, 2, 2, 2, 2, 2, 2, 2, 2, 2, 2, 2, 2, 2, 2, 2, 2, 2, 2, 2, 2, 2, 2, 2, 2, 2, 2, 2, 2, 2, 2, 2, 2, 2, 2, 2, 2, 2, 2, 2, 2, 2, 2, 2, 2, 2, 2, 2, 2, 2, 2, 2, 2, 2, 2, 2, 2, 2, 2, 2, 2, 2, 2, 2, 2, 2, 2, 2, 2, 2, 2, 2, 2, 2, 2, 2, 2, 2, 2, 2, 2, 2, 2, 2, 2, 2, 2, 2, 2, 2, 2, 2, 2, 2, 2, 2, 2, 2, 2, 2, 2, 2, 2, 2, 2, 2, 2, 2, 2, 2, 2, 2, 2, 2, 2, 2, 2, 2, 2, 2, 2, 2, 2, 2, 2, 2, 2, 2, 2, 2, 2, 2, 2, 2, 2, 2, 2, 2, 2, 2, 2, 2, 2, 2, 2, 2, 2, 2, 2, 2, 2, 2, 2, 2, 2, 2, 2, 2, 2, 2, 2, 2, 2, 2, 2, 2, 2, 2, 2, 2, 2, 2, 2, 2, 2, 2, 2, 2, 2, 2, 2, 2, 2, 2, 2, 2, 2, 2, 2, 2, 2, 2, 2, 2, 2, 2, 2, 2, 2, 2, 2, 2, 2, 2, 2, 2, 2, 2, 2, 2, 2, 2, 2, 2, 3 ),
 ( 0.000000000000000000, 1.000000000000000000 ),
 ( 0.000000000000000000, 0.003787878787878787984, 0.007575757575757575968, 0.01136363636363636395, 0.01515151515151515194, 0.01893939393939393992, 0.02272727272727272790, 0.02651515151515151589, 0.03030303030303030387, 0.03409090909090908839, 0.03787878787878787984, 0.04166666666666666435, 0.04545454545454545581, 0.04924242424242424032, 0.05303030303030303177, 0.05681818181818181629, 0.06060606060606060774, 0.06439393939393939226, 0.06818181818181817677, 0.07196969696969697516, 0.07575757575757575968, 0.07954545454545454419, 0.08333333333333332871, 0.08712121212121212710, 0.09090909090909091161, 0.09469696969696969613, 0.09848484848484848064, 0.1022727272727272790, 0.1060606060606060635, 0.1098484848484848481, 0.1136363636363636326, 0.1174242424242424310, 0.1212121212121212155, 0.1250000000000000000, 0.1287878787878787845, 0.1325757575757575690, 0.1363636363636363535, 0.1401515151515151381, 0.1439393939393939503, 0.1477272727272727348, 0.1515151515151515194, 0.1553030303030303039, 0.1590909090909090884, 0.1628787878787878729, 0.1666666666666666574, 0.1704545454545454419, 0.1742424242424242542, 0.1780303030303030387, 0.1818181818181818232, 0.1856060606060606077, 0.1893939393939393923, 0.1931818181818181768, 0.1969696969696969613, 0.2007575757575757458, 0.2045454545454545581, 0.2083333333333333426, 0.2121212121212121271, 0.2159090909090909116, 0.2196969696969696961, 0.2234848484848484806, 0.2272727272727272652, 0.2310606060606060497, 0.2348484848484848619, 0.2386363636363636465, 0.2424242424242424310, 0.2462121212121212155, 0.2500000000000000000, 0.2537878787878787845, 0.2575757575757575690, 0.2613636363636363535, 0.2651515151515151381, 0.2689393939393939226, 0.2727272727272727071, 0.2765151515151514916, 0.2803030303030302761, 0.2840909090909091161, 0.2878787878787879007, 0.2916666666666666852, 0.2954545454545454697, 0.2992424242424242542, 0.3030303030303030387, 0.3068181818181818232, 0.3106060606060606077, 0.3143939393939393923, 0.3181818181818181768, 0.3219696969696969613, 0.3257575757575757458, 0.3295454545454545303, 0.3333333333333333148, 0.3371212121212120993, 0.3409090909090908839, 0.3446969696969697239, 0.3484848484848485084, 0.3522727272727272929, 0.3560606060606060774, 0.3598484848484848619, 0.3636363636363636465, 0.3674242424242424310, 0.3712121212121212155, 0.3750000000000000000, 0.3787878787878787845, 0.3825757575757575690, 0.3863636363636363535, 0.3901515151515151381, 0.3939393939393939226, 0.3977272727272727071, 0.4015151515151514916, 0.4053030303030302761, 0.4090909090909091161, 0.4128787878787879007, 0.4166666666666666852, 0.4204545454545454697, 0.4242424242424242542, 0.4280303030303030387, 0.4318181818181818232, 0.4356060606060606077, 0.4393939393939393923, 0.4431818181818181768, 0.4469696969696969613, 0.4507575757575757458, 0.4545454545454545303, 0.4583333333333333148, 0.4621212121212120993, 0.4659090909090908839, 0.4696969696969697239, 0.4734848484848485084, 0.4772727272727272929, 0.4810606060606060774, 0.4848484848484848619, 0.4886363636363636465, 0.4924242424242424310, 0.4962121212121212155, 0.5000000000000000000, 0.5037878787878787845, 0.5075757575757575690, 0.5113636363636363535, 0.5151515151515151381, 0.5189393939393939226, 0.5227272727272727071, 0.5265151515151514916, 0.5303030303030302761, 0.5340909090909090606, 0.5378787878787878451, 0.5416666666666666297, 0.5454545454545454142, 0.5492424242424241987, 0.5530303030303029832, 0.5568181818181817677, 0.5606060606060605522, 0.5643939393939394478, 0.5681818181818182323, 0.5719696969696970168, 0.5757575757575758013, 0.5795454545454545858, 0.5833333333333333703, 0.5871212121212121549, 0.5909090909090909394, 0.5946969696969697239, 0.5984848484848485084, 0.6022727272727272929, 0.6060606060606060774, 0.6098484848484848619, 0.6136363636363636465, 0.6174242424242424310, 0.6212121212121212155, 0.6250000000000000000, 0.6287878787878787845, 0.6325757575757575690, 0.6363636363636363535, 0.6401515151515151381, 0.6439393939393939226, 0.6477272727272727071, 0.6515151515151514916, 0.6553030303030302761, 0.6590909090909090606, 0.6628787878787878451, 0.6666666666666666297, 0.6704545454545454142, 0.6742424242424241987, 0.6780303030303029832, 0.6818181818181817677, 0.6856060606060605522, 0.6893939393939394478, 0.6931818181818182323, 0.6969696969696970168, 0.7007575757575758013, 0.7045454545454545858, 0.7083333333333333703, 0.7121212121212121549, 0.7159090909090909394, 0.7196969696969697239, 0.7234848484848485084, 0.7272727272727272929, 0.7310606060606060774, 0.7348484848484848619, 0.7386363636363636465, 0.7424242424242424310, 0.7462121212121212155, 0.7500000000000000000, 0.7537878787878787845, 0.7575757575757575690, 0.7613636363636363535, 0.7651515151515151381, 0.7689393939393939226, 0.7727272727272727071, 0.7765151515151514916, 0.7803030303030302761, 0.7840909090909090606, 0.7878787878787878451, 0.7916666666666666297, 0.7954545454545454142, 0.7992424242424241987, 0.8030303030303029832, 0.8068181818181817677, 0.8106060606060605522, 0.8143939393939394478, 0.8181818181818182323, 0.8219696969696970168, 0.8257575757575758013, 0.8295454545454545858, 0.8333333333333333703, 0.8371212121212121549, 0.8409090909090909394, 0.8446969696969697239, 0.8484848484848485084, 0.8522727272727272929, 0.8560606060606060774, 0.8598484848484848619, 0.8636363636363636465, 0.8674242424242424310, 0.8712121212121212155, 0.8750000000000000000, 0.8787878787878787845, 0.8825757575757575690, 0.8863636363636363535, 0.8901515151515151381, 0.8939393939393939226, 0.8977272727272727071, 0.9015151515151514916, 0.9053030303030302761, 0.9090909090909090606, 0.9128787878787878451, 0.9166666666666666297, 0.9204545454545454142, 0.9242424242424241987, 0.9280303030303029832, 0.9318181818181817677, 0.9356060606060605522, 0.9393939393939394478, 0.9431818181818182323, 0.9469696969696970168, 0.9507575757575758013, 0.9545454545454545858, 0.9583333333333333703, 0.9621212121212121549, 0.9659090909090909394 ),
 .UNSPECIFIED. ) 
 GEOMETRIC_REPRESENTATION_ITEM ( )  RATIONAL_B_SPLINE_SURFACE ( (
 ( 1.000000000000000000, 0.9659258262890683122, 1.000000000000000000, 0.9659258262890683122, 1.000000000000000000, 0.9659258262890683122, 1.000000000000000000, 0.9659258262890683122, 1.000000000000000000, 0.9659258262890683122, 1.000000000000000000, 0.9659258262890683122, 1.000000000000000000, 0.9659258262890683122, 1.000000000000000000, 0.9659258262890683122, 1.000000000000000000, 0.9659258262890683122, 1.000000000000000000, 0.9659258262890683122, 1.000000000000000000, 0.9659258262890683122, 1.000000000000000000, 0.9659258262890683122, 1.000000000000000000, 0.9659258262890683122, 1.000000000000000000, 0.9659258262890683122, 1.000000000000000000, 0.9659258262890683122, 1.000000000000000000, 0.9659258262890683122, 1.000000000000000000, 0.9659258262890683122, 1.000000000000000000, 0.9659258262890683122, 1.000000000000000000, 0.9659258262890683122, 1.000000000000000000, 0.9659258262890683122, 1.000000000000000000, 0.9659258262890683122, 1.000000000000000000, 0.9659258262890683122, 1.000000000000000000, 0.9659258262890683122, 1.000000000000000000, 0.9659258262890683122, 1.000000000000000000, 0.9659258262890683122, 1.000000000000000000, 0.9659258262890683122, 1.000000000000000000, 0.9659258262890683122, 1.000000000000000000, 0.9659258262890683122, 1.000000000000000000, 0.9659258262890683122, 1.000000000000000000, 0.9659258262890683122, 1.000000000000000000, 0.9659258262890683122, 1.000000000000000000, 0.9659258262890683122, 1.000000000000000000, 0.9659258262890683122, 1.000000000000000000, 0.9659258262890683122, 1.000000000000000000, 0.9659258262890683122, 1.000000000000000000, 0.9659258262890683122, 1.000000000000000000, 0.9659258262890683122, 1.000000000000000000, 0.9659258262890683122, 1.000000000000000000, 0.9659258262890683122, 1.000000000000000000, 0.9659258262890683122, 1.000000000000000000, 0.9659258262890683122, 1.000000000000000000, 0.9659258262890683122, 1.000000000000000000, 0.9659258262890683122, 1.000000000000000000, 0.9659258262890683122, 1.000000000000000000, 0.9659258262890683122, 1.000000000000000000, 0.9659258262890683122, 1.000000000000000000, 0.9659258262890683122, 1.000000000000000000, 0.9659258262890683122, 1.000000000000000000, 0.9659258262890683122, 1.000000000000000000, 0.9659258262890683122, 1.000000000000000000, 0.9659258262890683122, 1.000000000000000000, 0.9659258262890683122, 1.000000000000000000, 0.9659258262890683122, 1.000000000000000000, 0.9659258262890683122, 1.000000000000000000, 0.9659258262890683122, 1.000000000000000000, 0.9659258262890683122, 1.000000000000000000, 0.9659258262890683122, 1.000000000000000000, 0.9659258262890683122, 1.000000000000000000, 0.9659258262890683122, 1.000000000000000000, 0.9659258262890683122, 1.000000000000000000, 0.9659258262890683122, 1.000000000000000000, 0.9659258262890683122, 1.000000000000000000, 0.9659258262890683122, 1.000000000000000000, 0.9659258262890683122, 1.000000000000000000, 0.9659258262890683122, 1.000000000000000000, 0.9659258262890683122, 1.000000000000000000, 0.9659258262890683122, 1.000000000000000000, 0.9659258262890683122, 1.000000000000000000, 0.9659258262890683122, 1.000000000000000000, 0.9659258262890683122, 1.000000000000000000, 0.9659258262890683122, 1.000000000000000000, 0.9659258262890683122, 1.000000000000000000, 0.9659258262890683122, 1.000000000000000000, 0.9659258262890683122, 1.000000000000000000, 0.9659258262890683122, 1.000000000000000000, 0.9659258262890683122, 1.000000000000000000, 0.9659258262890683122, 1.000000000000000000, 0.9659258262890683122, 1.000000000000000000, 0.9659258262890683122, 1.000000000000000000, 0.9659258262890683122, 1.000000000000000000, 0.9659258262890683122, 1.000000000000000000, 0.9659258262890683122, 1.000000000000000000, 0.9659258262890683122, 1.000000000000000000, 0.9659258262890683122, 1.000000000000000000, 0.9659258262890683122, 1.000000000000000000, 0.9659258262890683122, 1.000000000000000000, 0.9659258262890683122, 1.000000000000000000, 0.9659258262890683122, 1.000000000000000000, 0.9659258262890683122, 1.000000000000000000, 0.9659258262890683122, 1.000000000000000000, 0.9659258262890683122, 1.000000000000000000, 0.9659258262890683122, 1.000000000000000000, 0.9659258262890683122, 1.000000000000000000, 0.9659258262890683122, 1.000000000000000000, 0.9659258262890683122, 1.000000000000000000, 0.9659258262890683122, 1.000000000000000000, 0.9659258262890683122, 1.000000000000000000, 0.9659258262890683122, 1.000000000000000000, 0.9659258262890683122, 1.000000000000000000, 0.9659258262890683122, 1.000000000000000000, 0.9659258262890683122, 1.000000000000000000, 0.9659258262890683122, 1.000000000000000000, 0.9659258262890683122, 1.000000000000000000, 0.9659258262890683122, 1.000000000000000000, 0.9659258262890683122, 1.000000000000000000, 0.9659258262890683122, 1.000000000000000000, 0.9659258262890683122, 1.000000000000000000, 0.9659258262890683122, 1.000000000000000000, 0.9659258262890683122, 1.000000000000000000, 0.9659258262890683122, 1.000000000000000000, 0.9659258262890683122, 1.000000000000000000, 0.9659258262890683122, 1.000000000000000000, 0.9659258262890683122, 1.000000000000000000, 0.9659258262890683122, 1.000000000000000000, 0.9659258262890683122, 1.000000000000000000, 0.9659258262890683122, 1.000000000000000000, 0.9659258262890683122, 1.000000000000000000, 0.9659258262890683122, 1.000000000000000000, 0.9659258262890683122, 1.000000000000000000, 0.9659258262890683122, 1.000000000000000000, 0.9659258262890683122, 1.000000000000000000, 0.9659258262890683122, 1.000000000000000000, 0.9659258262890683122, 1.000000000000000000, 0.9659258262890683122, 1.000000000000000000, 0.9659258262890683122, 1.000000000000000000, 0.9659258262890683122, 1.000000000000000000, 0.9659258262890683122, 1.000000000000000000, 0.9659258262890683122, 1.000000000000000000, 0.9659258262890683122, 1.000000000000000000, 0.9659258262890683122, 1.000000000000000000, 0.9659258262890683122, 1.000000000000000000, 0.9659258262890683122, 1.000000000000000000, 0.9659258262890683122, 1.000000000000000000, 0.9659258262890683122, 1.000000000000000000, 0.9659258262890683122, 1.000000000000000000, 0.9659258262890683122, 1.000000000000000000, 0.9659258262890683122, 1.000000000000000000, 0.9659258262890683122, 1.000000000000000000, 0.9659258262890683122, 1.000000000000000000, 0.9659258262890683122, 1.000000000000000000, 0.9659258262890683122, 1.000000000000000000, 0.9659258262890683122, 1.000000000000000000, 0.9659258262890683122, 1.000000000000000000, 0.9659258262890683122, 1.000000000000000000, 0.9659258262890683122, 1.000000000000000000, 0.9659258262890683122, 1.000000000000000000, 0.9659258262890683122, 1.000000000000000000, 0.9659258262890683122, 1.000000000000000000, 0.9659258262890683122, 1.000000000000000000, 0.9659258262890683122, 1.000000000000000000, 0.9659258262890683122, 1.000000000000000000, 0.9659258262890683122, 1.000000000000000000, 0.9659258262890683122, 1.000000000000000000, 0.9659258262890683122, 1.000000000000000000, 0.9659258262890683122, 1.000000000000000000, 0.9659258262890683122, 1.000000000000000000, 0.9659258262890683122, 1.000000000000000000, 0.9659258262890683122, 1.000000000000000000, 0.9659258262890683122, 1.000000000000000000, 0.9659258262890683122, 1.000000000000000000, 0.9659258262890683122, 1.000000000000000000, 0.9659258262890683122, 1.000000000000000000, 0.9659258262890683122, 1.000000000000000000, 0.9659258262890683122, 1.000000000000000000, 0.9659258262890683122, 1.000000000000000000, 0.9659258262890683122, 1.000000000000000000, 0.9659258262890683122, 1.000000000000000000, 0.9659258262890683122, 1.000000000000000000, 0.9659258262890683122, 1.000000000000000000, 0.9659258262890683122, 1.000000000000000000, 0.9659258262890683122, 1.000000000000000000, 0.9659258262890683122, 1.000000000000000000, 0.9659258262890683122, 1.000000000000000000, 0.9659258262890683122, 1.000000000000000000, 0.9659258262890683122, 1.000000000000000000, 0.9659258262890683122, 1.000000000000000000, 0.9659258262890683122, 1.000000000000000000, 0.9659258262890683122, 1.000000000000000000, 0.9659258262890683122, 1.000000000000000000, 0.9659258262890683122, 1.000000000000000000, 0.9659258262890683122, 1.000000000000000000, 0.9659258262890683122, 1.000000000000000000, 0.9659258262890683122, 1.000000000000000000, 0.9659258262890683122, 1.000000000000000000, 0.9659258262890683122, 1.000000000000000000, 0.9659258262890683122, 1.000000000000000000, 0.9659258262890683122, 1.000000000000000000, 0.9659258262890683122, 1.000000000000000000, 0.9659258262890683122, 1.000000000000000000, 0.9659258262890683122, 1.000000000000000000, 0.9659258262890683122, 1.000000000000000000, 0.9659258262890683122, 1.000000000000000000, 0.9659258262890683122, 1.000000000000000000, 0.9659258262890683122, 1.000000000000000000, 0.9659258262890683122, 1.000000000000000000, 0.9659258262890683122, 1.000000000000000000, 0.9659258262890683122, 1.000000000000000000, 0.9659258262890683122, 1.000000000000000000, 0.9659258262890683122, 1.000000000000000000, 0.9659258262890683122, 1.000000000000000000, 0.9659258262890683122, 1.000000000000000000, 0.9659258262890683122, 1.000000000000000000, 0.9659258262890683122, 1.000000000000000000, 0.9659258262890683122, 1.000000000000000000, 0.9659258262890683122, 1.000000000000000000, 0.9659258262890683122, 1.000000000000000000, 0.9659258262890683122, 1.000000000000000000, 0.9659258262890683122, 1.000000000000000000, 0.9659258262890683122, 1.000000000000000000, 0.9659258262890683122, 1.000000000000000000, 0.9659258262890683122, 1.000000000000000000, 0.9659258262890683122, 1.000000000000000000, 0.9659258262890683122, 1.000000000000000000, 0.9659258262890683122, 1.000000000000000000, 0.9659258262890683122, 1.000000000000000000, 0.9659258262890683122, 1.000000000000000000, 0.9659258262890683122, 1.000000000000000000, 0.9659258262890683122, 1.000000000000000000, 0.9659258262890683122, 1.000000000000000000, 0.9659258262890683122, 1.000000000000000000, 0.9659258262890683122, 1.000000000000000000, 0.9659258262890683122, 1.000000000000000000, 0.9659258262890683122, 1.000000000000000000, 0.9659258262890683122, 1.000000000000000000, 0.9659258262890683122, 1.000000000000000000, 0.9659258262890683122, 1.000000000000000000, 0.9659258262890683122, 1.000000000000000000, 0.9659258262890683122, 1.000000000000000000, 0.9659258262890683122, 1.000000000000000000, 0.9659258262890683122, 1.000000000000000000, 0.9659258262890683122, 1.000000000000000000, 0.9659258262890683122, 1.000000000000000000, 0.9659258262890683122, 1.000000000000000000, 0.9659258262890683122, 1.000000000000000000, 0.9659258262890683122, 1.000000000000000000, 0.9659258262890683122, 1.000000000000000000, 0.9659258262890683122, 1.000000000000000000, 0.9659258262890683122, 1.000000000000000000, 0.9659258262890683122, 1.000000000000000000, 0.9659258262890683122, 1.000000000000000000, 0.9659258262890683122, 1.000000000000000000, 0.9659258262890683122, 1.000000000000000000, 0.9659258262890683122, 1.000000000000000000, 0.9659258262890683122, 1.000000000000000000, 0.9659258262890683122, 1.000000000000000000, 0.9659258262890683122, 1.000000000000000000, 0.9659258262890683122, 1.000000000000000000, 0.9659258262890683122, 1.000000000000000000, 0.9659258262890683122, 1.000000000000000000, 0.9659258262890683122, 1.000000000000000000, 0.9659258262890683122, 1.000000000000000000, 0.9659258262890683122, 1.000000000000000000, 0.9659258262890683122, 1.000000000000000000, 0.9659258262890683122, 1.000000000000000000, 0.9659258262890683122, 1.000000000000000000),
 ( 1.000000000000000000, 0.9659258262890683122, 1.000000000000000000, 0.9659258262890683122, 1.000000000000000000, 0.9659258262890683122, 1.000000000000000000, 0.9659258262890683122, 1.000000000000000000, 0.9659258262890683122, 1.000000000000000000, 0.9659258262890683122, 1.000000000000000000, 0.9659258262890683122, 1.000000000000000000, 0.9659258262890683122, 1.000000000000000000, 0.9659258262890683122, 1.000000000000000000, 0.9659258262890683122, 1.000000000000000000, 0.9659258262890683122, 1.000000000000000000, 0.9659258262890683122, 1.000000000000000000, 0.9659258262890683122, 1.000000000000000000, 0.9659258262890683122, 1.000000000000000000, 0.9659258262890683122, 1.000000000000000000, 0.9659258262890683122, 1.000000000000000000, 0.9659258262890683122, 1.000000000000000000, 0.9659258262890683122, 1.000000000000000000, 0.9659258262890683122, 1.000000000000000000, 0.9659258262890683122, 1.000000000000000000, 0.9659258262890683122, 1.000000000000000000, 0.9659258262890683122, 1.000000000000000000, 0.9659258262890683122, 1.000000000000000000, 0.9659258262890683122, 1.000000000000000000, 0.9659258262890683122, 1.000000000000000000, 0.9659258262890683122, 1.000000000000000000, 0.9659258262890683122, 1.000000000000000000, 0.9659258262890683122, 1.000000000000000000, 0.9659258262890683122, 1.000000000000000000, 0.9659258262890683122, 1.000000000000000000, 0.9659258262890683122, 1.000000000000000000, 0.9659258262890683122, 1.000000000000000000, 0.9659258262890683122, 1.000000000000000000, 0.9659258262890683122, 1.000000000000000000, 0.9659258262890683122, 1.000000000000000000, 0.9659258262890683122, 1.000000000000000000, 0.9659258262890683122, 1.000000000000000000, 0.9659258262890683122, 1.000000000000000000, 0.9659258262890683122, 1.000000000000000000, 0.9659258262890683122, 1.000000000000000000, 0.9659258262890683122, 1.000000000000000000, 0.9659258262890683122, 1.000000000000000000, 0.9659258262890683122, 1.000000000000000000, 0.9659258262890683122, 1.000000000000000000, 0.9659258262890683122, 1.000000000000000000, 0.9659258262890683122, 1.000000000000000000, 0.9659258262890683122, 1.000000000000000000, 0.9659258262890683122, 1.000000000000000000, 0.9659258262890683122, 1.000000000000000000, 0.9659258262890683122, 1.000000000000000000, 0.9659258262890683122, 1.000000000000000000, 0.9659258262890683122, 1.000000000000000000, 0.9659258262890683122, 1.000000000000000000, 0.9659258262890683122, 1.000000000000000000, 0.9659258262890683122, 1.000000000000000000, 0.9659258262890683122, 1.000000000000000000, 0.9659258262890683122, 1.000000000000000000, 0.9659258262890683122, 1.000000000000000000, 0.9659258262890683122, 1.000000000000000000, 0.9659258262890683122, 1.000000000000000000, 0.9659258262890683122, 1.000000000000000000, 0.9659258262890683122, 1.000000000000000000, 0.9659258262890683122, 1.000000000000000000, 0.9659258262890683122, 1.000000000000000000, 0.9659258262890683122, 1.000000000000000000, 0.9659258262890683122, 1.000000000000000000, 0.9659258262890683122, 1.000000000000000000, 0.9659258262890683122, 1.000000000000000000, 0.9659258262890683122, 1.000000000000000000, 0.9659258262890683122, 1.000000000000000000, 0.9659258262890683122, 1.000000000000000000, 0.9659258262890683122, 1.000000000000000000, 0.9659258262890683122, 1.000000000000000000, 0.9659258262890683122, 1.000000000000000000, 0.9659258262890683122, 1.000000000000000000, 0.9659258262890683122, 1.000000000000000000, 0.9659258262890683122, 1.000000000000000000, 0.9659258262890683122, 1.000000000000000000, 0.9659258262890683122, 1.000000000000000000, 0.9659258262890683122, 1.000000000000000000, 0.9659258262890683122, 1.000000000000000000, 0.9659258262890683122, 1.000000000000000000, 0.9659258262890683122, 1.000000000000000000, 0.9659258262890683122, 1.000000000000000000, 0.9659258262890683122, 1.000000000000000000, 0.9659258262890683122, 1.000000000000000000, 0.9659258262890683122, 1.000000000000000000, 0.9659258262890683122, 1.000000000000000000, 0.9659258262890683122, 1.000000000000000000, 0.9659258262890683122, 1.000000000000000000, 0.9659258262890683122, 1.000000000000000000, 0.9659258262890683122, 1.000000000000000000, 0.9659258262890683122, 1.000000000000000000, 0.9659258262890683122, 1.000000000000000000, 0.9659258262890683122, 1.000000000000000000, 0.9659258262890683122, 1.000000000000000000, 0.9659258262890683122, 1.000000000000000000, 0.9659258262890683122, 1.000000000000000000, 0.9659258262890683122, 1.000000000000000000, 0.9659258262890683122, 1.000000000000000000, 0.9659258262890683122, 1.000000000000000000, 0.9659258262890683122, 1.000000000000000000, 0.9659258262890683122, 1.000000000000000000, 0.9659258262890683122, 1.000000000000000000, 0.9659258262890683122, 1.000000000000000000, 0.9659258262890683122, 1.000000000000000000, 0.9659258262890683122, 1.000000000000000000, 0.9659258262890683122, 1.000000000000000000, 0.9659258262890683122, 1.000000000000000000, 0.9659258262890683122, 1.000000000000000000, 0.9659258262890683122, 1.000000000000000000, 0.9659258262890683122, 1.000000000000000000, 0.9659258262890683122, 1.000000000000000000, 0.9659258262890683122, 1.000000000000000000, 0.9659258262890683122, 1.000000000000000000, 0.9659258262890683122, 1.000000000000000000, 0.9659258262890683122, 1.000000000000000000, 0.9659258262890683122, 1.000000000000000000, 0.9659258262890683122, 1.000000000000000000, 0.9659258262890683122, 1.000000000000000000, 0.9659258262890683122, 1.000000000000000000, 0.9659258262890683122, 1.000000000000000000, 0.9659258262890683122, 1.000000000000000000, 0.9659258262890683122, 1.000000000000000000, 0.9659258262890683122, 1.000000000000000000, 0.9659258262890683122, 1.000000000000000000, 0.9659258262890683122, 1.000000000000000000, 0.9659258262890683122, 1.000000000000000000, 0.9659258262890683122, 1.000000000000000000, 0.9659258262890683122, 1.000000000000000000, 0.9659258262890683122, 1.000000000000000000, 0.9659258262890683122, 1.000000000000000000, 0.9659258262890683122, 1.000000000000000000, 0.9659258262890683122, 1.000000000000000000, 0.9659258262890683122, 1.000000000000000000, 0.9659258262890683122, 1.000000000000000000, 0.9659258262890683122, 1.000000000000000000, 0.9659258262890683122, 1.000000000000000000, 0.9659258262890683122, 1.000000000000000000, 0.9659258262890683122, 1.000000000000000000, 0.9659258262890683122, 1.000000000000000000, 0.9659258262890683122, 1.000000000000000000, 0.9659258262890683122, 1.000000000000000000, 0.9659258262890683122, 1.000000000000000000, 0.9659258262890683122, 1.000000000000000000, 0.9659258262890683122, 1.000000000000000000, 0.9659258262890683122, 1.000000000000000000, 0.9659258262890683122, 1.000000000000000000, 0.9659258262890683122, 1.000000000000000000, 0.9659258262890683122, 1.000000000000000000, 0.9659258262890683122, 1.000000000000000000, 0.9659258262890683122, 1.000000000000000000, 0.9659258262890683122, 1.000000000000000000, 0.9659258262890683122, 1.000000000000000000, 0.9659258262890683122, 1.000000000000000000, 0.9659258262890683122, 1.000000000000000000, 0.9659258262890683122, 1.000000000000000000, 0.9659258262890683122, 1.000000000000000000, 0.9659258262890683122, 1.000000000000000000, 0.9659258262890683122, 1.000000000000000000, 0.9659258262890683122, 1.000000000000000000, 0.9659258262890683122, 1.000000000000000000, 0.9659258262890683122, 1.000000000000000000, 0.9659258262890683122, 1.000000000000000000, 0.9659258262890683122, 1.000000000000000000, 0.9659258262890683122, 1.000000000000000000, 0.9659258262890683122, 1.000000000000000000, 0.9659258262890683122, 1.000000000000000000, 0.9659258262890683122, 1.000000000000000000, 0.9659258262890683122, 1.000000000000000000, 0.9659258262890683122, 1.000000000000000000, 0.9659258262890683122, 1.000000000000000000, 0.9659258262890683122, 1.000000000000000000, 0.9659258262890683122, 1.000000000000000000, 0.9659258262890683122, 1.000000000000000000, 0.9659258262890683122, 1.000000000000000000, 0.9659258262890683122, 1.000000000000000000, 0.9659258262890683122, 1.000000000000000000, 0.9659258262890683122, 1.000000000000000000, 0.9659258262890683122, 1.000000000000000000, 0.9659258262890683122, 1.000000000000000000, 0.9659258262890683122, 1.000000000000000000, 0.9659258262890683122, 1.000000000000000000, 0.9659258262890683122, 1.000000000000000000, 0.9659258262890683122, 1.000000000000000000, 0.9659258262890683122, 1.000000000000000000, 0.9659258262890683122, 1.000000000000000000, 0.9659258262890683122, 1.000000000000000000, 0.9659258262890683122, 1.000000000000000000, 0.9659258262890683122, 1.000000000000000000, 0.9659258262890683122, 1.000000000000000000, 0.9659258262890683122, 1.000000000000000000, 0.9659258262890683122, 1.000000000000000000, 0.9659258262890683122, 1.000000000000000000, 0.9659258262890683122, 1.000000000000000000, 0.9659258262890683122, 1.000000000000000000, 0.9659258262890683122, 1.000000000000000000, 0.9659258262890683122, 1.000000000000000000, 0.9659258262890683122, 1.000000000000000000, 0.9659258262890683122, 1.000000000000000000, 0.9659258262890683122, 1.000000000000000000, 0.9659258262890683122, 1.000000000000000000, 0.9659258262890683122, 1.000000000000000000, 0.9659258262890683122, 1.000000000000000000, 0.9659258262890683122, 1.000000000000000000, 0.9659258262890683122, 1.000000000000000000, 0.9659258262890683122, 1.000000000000000000, 0.9659258262890683122, 1.000000000000000000, 0.9659258262890683122, 1.000000000000000000, 0.9659258262890683122, 1.000000000000000000, 0.9659258262890683122, 1.000000000000000000, 0.9659258262890683122, 1.000000000000000000, 0.9659258262890683122, 1.000000000000000000, 0.9659258262890683122, 1.000000000000000000, 0.9659258262890683122, 1.000000000000000000, 0.9659258262890683122, 1.000000000000000000, 0.9659258262890683122, 1.000000000000000000, 0.9659258262890683122, 1.000000000000000000, 0.9659258262890683122, 1.000000000000000000, 0.9659258262890683122, 1.000000000000000000, 0.9659258262890683122, 1.000000000000000000, 0.9659258262890683122, 1.000000000000000000, 0.9659258262890683122, 1.000000000000000000, 0.9659258262890683122, 1.000000000000000000, 0.9659258262890683122, 1.000000000000000000, 0.9659258262890683122, 1.000000000000000000, 0.9659258262890683122, 1.000000000000000000, 0.9659258262890683122, 1.000000000000000000, 0.9659258262890683122, 1.000000000000000000, 0.9659258262890683122, 1.000000000000000000, 0.9659258262890683122, 1.000000000000000000, 0.9659258262890683122, 1.000000000000000000, 0.9659258262890683122, 1.000000000000000000, 0.9659258262890683122, 1.000000000000000000, 0.9659258262890683122, 1.000000000000000000, 0.9659258262890683122, 1.000000000000000000, 0.9659258262890683122, 1.000000000000000000, 0.9659258262890683122, 1.000000000000000000, 0.9659258262890683122, 1.000000000000000000, 0.9659258262890683122, 1.000000000000000000, 0.9659258262890683122, 1.000000000000000000, 0.9659258262890683122, 1.000000000000000000, 0.9659258262890683122, 1.000000000000000000, 0.9659258262890683122, 1.000000000000000000, 0.9659258262890683122, 1.000000000000000000, 0.9659258262890683122, 1.000000000000000000, 0.9659258262890683122, 1.000000000000000000, 0.9659258262890683122, 1.000000000000000000, 0.9659258262890683122, 1.000000000000000000, 0.9659258262890683122, 1.000000000000000000, 0.9659258262890683122, 1.000000000000000000, 0.9659258262890683122, 1.000000000000000000, 0.9659258262890683122, 1.000000000000000000, 0.9659258262890683122, 1.000000000000000000, 0.9659258262890683122, 1.000000000000000000) ) ) 
 REPRESENTATION_ITEM ( '' )  SURFACE ( )  );
#55300=CARTESIAN_POINT ( 'NONE',  ( 1.417322834645670104, -0.1870078740157479769, 0.4822834645669291653 ) ) ;
#55302=CARTESIAN_POINT ( 'NONE',  ( -1.417322834645668772, -0.1870078740157479769, 0.4822834645669291653 ) ) ;
#55303=CARTESIAN_POINT ( 'NONE',  ( -1.259842519685038686, -0.1870078740157480601, -0.3641732283464567677 ) ) ;
#55304=CARTESIAN_POINT ( 'NONE',  ( -0.7217847769028863381, -0.004921259842519870586, -0.3153832671262229437 ) ) ;
#55305=EDGE_CURVE ( 'NONE', #13510, #11614, #27437, .T. ) ;
#55307=CARTESIAN_POINT ( 'NONE',  ( 0.08530183727034192087, -0.05778040916215522460, 0.4822834645669289988 ) ) ;
#55308=CARTESIAN_POINT ( 'NONE',  ( -0.1902887139107604098, 0.1771653543307087075, -0.09757992244046823083 ) ) ;
#55309=CARTESIAN_POINT ( 'NONE',  ( -1.062992125984250968, 0.1771653543307087630, 0.000000000000000000 ) ) ;
#55310=CARTESIAN_POINT ( 'NONE',  ( -1.568241469816272105, -0.05778040916215522460, 0.4822834645669289988 ) ) ;
#55311=CARTESIAN_POINT ( 'NONE',  ( 1.161417322834646271, 0.07958543189024071263, -0.2665933059059888421 ) ) ;
#55312=CARTESIAN_POINT ( 'NONE',  ( 1.345144356955381593, -0.05778040916215522460, 0.4822834645669289988 ) ) ;
#55314=CARTESIAN_POINT ( 'NONE',  ( 0.2559055118110243332, 0.07958543189024085140, 0.2665933059059887866 ) ) ;
#55315=CARTESIAN_POINT ( 'NONE',  ( 0.8398950131233602345, -0.6046776061558807314, 0.2411417322834647770 ) ) ;
#55317=CARTESIAN_POINT ( 'NONE',  ( 1.036745406824147508, -0.3690944881889765550, -0.3153832671262227771 ) ) ;
#55319=CARTESIAN_POINT ( 'NONE',  ( -1.312335958005248715, 0.2306618581243848609, 0.2411417322834645549 ) ) ;
#55320=CARTESIAN_POINT ( 'NONE',  ( -1.017060367454067249, -0.05778040916215522460, 0.4822834645669289988 ) ) ;
#55321=CARTESIAN_POINT ( 'NONE',  ( -0.1837270341207343505, -0.6046776061558807314, 0.2411417322834647770 ) ) ;
#55324=CARTESIAN_POINT ( 'NONE',  ( 0.8727034120734912248, -0.3162353388693409650, -0.4822834645669289433 ) ) ;
#55325=CARTESIAN_POINT ( 'NONE',  ( 1.614173228346457378, 0.1771653543307087630, 0.000000000000000000 ) ) ;
#55326=CARTESIAN_POINT ( 'NONE',  ( 0.06561679790026316017, -0.4281496062992124485, 0.4176697321401328655 ) ) ;
#55327=CARTESIAN_POINT ( 'NONE',  ( 0.9580052493438326877, 0.05413385826771666132, 0.4176697321401328100 ) ) ;
#55333=CARTESIAN_POINT ( 'NONE',  ( -0.2952755905511804668, 0.07958543189024085140, 0.2665933059059887866 ) ) ;
#55334=CARTESIAN_POINT ( 'NONE',  ( -0.7283464566929126471, 0.1660481256975883668, -0.3530559997133364547 ) ) ;
#55335=CARTESIAN_POINT ( 'NONE',  ( 0.9842519685039375910, 0.2952755905511811885, 0.000000000000000000 ) ) ;
#55338=CARTESIAN_POINT ( 'NONE',  ( -0.2952755905511803003, -0.4536011799217368745, -0.2665933059059886201 ) ) ;
#55339=CARTESIAN_POINT ( 'NONE',  ( 1.568241469816273437, -0.3162353388693405765, 0.4822834645669290543 ) ) ;
#55340=CARTESIAN_POINT ( 'NONE',  ( 1.023622047244095112, -0.1870078740157480879, -0.4822834645669291653 ) ) ;
#55343=CARTESIAN_POINT ( 'NONE',  ( 1.614173228346457378, 1.055049524192302357, 0.1372047244094478369 ) ) ;
#55344=CARTESIAN_POINT ( 'NONE',  ( 0.9120734908136489683, -0.6692913385826771977, 0.1292274648535927661 ) ) ;
#55346=CARTESIAN_POINT ( 'NONE',  ( 1.167979002624672580, -0.004921259842519870586, -0.3153832671262229437 ) ) ;
#55347=CARTESIAN_POINT ( 'NONE',  ( 1.627296587926509996, -0.6046776061558807314, 0.2411417322834647770 ) ) ;
#55348=CARTESIAN_POINT ( 'NONE',  ( -1.594488188976377119, 0.1660481256975883668, -0.3530559997133364547 ) ) ;
#55351=CARTESIAN_POINT ( 'NONE',  ( 0.9383202099737538715, -0.05778040916215560624, -0.4822834645669293319 ) ) ;
#55352=CARTESIAN_POINT ( 'NONE',  ( -1.614173228346456268, -0.6692913385826771977, 8.415575281601705876E-17 ) ) ;
#55353=CARTESIAN_POINT ( 'NONE',  ( -0.6561679790026240244, -0.6046776061558807314, 0.2411417322834647770 ) ) ;
#55354=CARTESIAN_POINT ( 'NONE',  ( -0.5839895013123351797, 0.2952755905511810774, -0.1292274648535930714 ) ) ;
#55355=CARTESIAN_POINT ( 'NONE',  ( -1.535433070866141225, -0.6692913385826771977, 8.415575281601705876E-17 ) ) ;
#55357=CARTESIAN_POINT ( 'NONE',  ( 0.1706036745406830368, 0.05413385826771666132, 0.4176697321401328100 ) ) ;
#55359=EDGE_CURVE ( 'NONE', #79849, #66112, #57524, .T. ) ;
#55360=CARTESIAN_POINT ( 'NONE',  ( -1.633858267716534529, 0.07958543189024085140, 0.2665933059059887866 ) ) ;
#55365=CARTESIAN_POINT ( 'NONE',  ( -1.437007874015747477, -0.5400638737290844871, 0.3530559997133364547 ) ) ;
#55367=LINE ( 'NONE', #49056, #80150 ) ;
#55372=CARTESIAN_POINT ( 'NONE',  ( -0.2887139107611542133, -0.5023911411419708095, -0.1820866141732282451 ) ) ;
#55373=CARTESIAN_POINT ( 'NONE',  ( -1.187664041994750175, -0.08942795157528024563, -0.3641732283464568787 ) ) ;
#55374=CARTESIAN_POINT ( 'NONE',  ( -1.653543307086613234, -0.1870078740157479769, 0.4822834645669291653 ) ) ;
#55375=CARTESIAN_POINT ( 'NONE',  ( 0.5118110236220478892, 0.2952755905511811885, 0.000000000000000000 ) ) ;
#55376=CARTESIAN_POINT ( 'NONE',  ( -1.522309711286088607, -0.6046776061558807314, 0.2411417322834647770 ) ) ;
#55379=CARTESIAN_POINT ( 'NONE',  ( -1.640419947506561060, 0.05413385826771666132, 0.4176697321401328100 ) ) ;
#55384=CARTESIAN_POINT ( 'NONE',  ( -0.7677165354330699465, -0.5400638737290845981, -0.3530559997133363437 ) ) ;
#55385=CARTESIAN_POINT ( 'NONE',  ( 1.555118110236221041, 0.1660481256975883668, -0.3530559997133364547 ) ) ;
#55387=CARTESIAN_POINT ( 'NONE',  ( 1.614173228346456712, 0.9921945702958890889, 0.1372047244094478646 ) ) ;
#55388=CARTESIAN_POINT ( 'NONE',  ( -1.686351706036744558, 0.2952755905511810774, -0.1292274648535930714 ) ) ;
#55389=CARTESIAN_POINT ( 'NONE',  ( -0.6102362204724400829, 0.1660481256975885056, 0.3530559997133364547 ) ) ;
#55391=CARTESIAN_POINT ( 'NONE',  ( 0.1574803149606306130, -0.1870078740157479769, 0.3641732283464567677 ) ) ;
#55393=CARTESIAN_POINT ( 'NONE',  ( -0.09842519685039295696, -0.4536011799217367080, 0.2665933059059888421 ) ) ;
#55394=CARTESIAN_POINT ( 'NONE',  ( 0.7086614173228352742, -0.1870078740157480601, -0.3641732283464567677 ) ) ;
#55395=CARTESIAN_POINT ( 'NONE',  ( 0.3477690288713918276, 0.2952755905511811885, 0.1292274648535926551 ) ) ;
#55397=CARTESIAN_POINT ( 'NONE',  ( -0.4265091863517051496, -0.5511811023622046335, 0.09757992244046803654 ) ) ;
#55399=CARTESIAN_POINT ( 'NONE',  ( 1.522309711286089939, -0.6046776061558809534, -0.2411417322834644161 ) ) ;
#55400=CARTESIAN_POINT ( 'NONE',  ( -1.181102362204723644, -0.1870078740157479769, 0.4822834645669291653 ) ) ;
#55402=CARTESIAN_POINT ( 'NONE',  ( -0.006561679790025524116, -0.3162353388693405765, 0.4822834645669290543 ) ) ;
#55403=ADVANCED_FACE ( 'NONE', ( #37543 ), #75045, .T. ) ;
#55404=CARTESIAN_POINT ( 'NONE',  ( -0.6364829396325453192, -0.05778040916215560624, -0.4822834645669293319 ) ) ;
#55405=CARTESIAN_POINT ( 'NONE',  ( 1.515748031496063408, 0.07958543189024085140, 0.2665933059059887866 ) ) ;
#55406=CARTESIAN_POINT ( 'NONE',  ( 5.463695987328526437E-16, -0.1870078740157479769, 0.3641732283464567677 ) ) ;
#55407=CARTESIAN_POINT ( 'NONE',  ( -0.2887139107611542133, 0.2306618581243848609, 0.2411417322834645549 ) ) ;
#55408=CARTESIAN_POINT ( 'NONE',  ( -0.6036745406824141069, -0.6046776061558809534, -0.2411417322834644161 ) ) ;
#55410=CARTESIAN_POINT ( 'NONE',  ( 1.660104986876641320, -0.08942795157527998196, 0.3641732283464567121 ) ) ;
#55411=CARTESIAN_POINT ( 'NONE',  ( 0.3149606299212606708, -0.1870078740157480879, -0.4822834645669291653 ) ) ;
#55414=CARTESIAN_POINT ( 'NONE',  ( 1.030183727034121421, -0.3162353388693409650, -0.4822834645669289433 ) ) ;
#55415=CARTESIAN_POINT ( 'NONE',  ( -0.4855643044619415427, -0.3690944881889763329, 0.3153832671262228327 ) ) ;
#55416=CARTESIAN_POINT ( 'NONE',  ( -0.7480314960629914633, 0.2952755905511811885, 0.000000000000000000 ) ) ;
#55417=CARTESIAN_POINT ( 'NONE',  ( 1.207349081364829990, 0.2306618581243848609, 0.2411417322834645549 ) ) ;
#55418=CARTESIAN_POINT ( 'NONE',  ( 1.161417322834646493, -0.5400638737290844871, 0.3530559997133364547 ) ) ;
#55419=CARTESIAN_POINT ( 'NONE',  ( -1.620734908136482577, 0.2952755905511811885, 0.1292274648535926551 ) ) ;
#55420=CARTESIAN_POINT ( 'NONE',  ( -0.9645669291338575535, -0.4536011799217367080, 0.2665933059059888421 ) ) ;
#55424=CARTESIAN_POINT ( 'NONE',  ( 1.476377952755906442, -0.4536011799217367080, 0.2665933059059888421 ) ) ;
#55425=CARTESIAN_POINT ( 'NONE',  ( 1.102362204724410155, -0.1870078740157479769, 0.3641732283464567677 ) ) ;
#55426=CARTESIAN_POINT ( 'NONE',  ( 0.3937007874015754361, -0.1870078740157480879, -0.4822834645669291653 ) ) ;
#55427=CARTESIAN_POINT ( 'NONE',  ( -1.706036745406823485, 0.2306618581243848609, 0.2411417322834645549 ) ) ;
#55429=CARTESIAN_POINT ( 'NONE',  ( 0.6233595800524942554, -0.08942795157528024563, -0.3641732283464568787 ) ) ;
#55430=CARTESIAN_POINT ( 'NONE',  ( -0.5118110236220466680, 0.2952755905511811885, 0.000000000000000000 ) ) ;
#55431=CARTESIAN_POINT ( 'NONE',  ( -0.7349081364829387342, -0.6046776061558807314, 0.2411417322834647770 ) ) ;
#55432=CARTESIAN_POINT ( 'NONE',  ( 1.161417322834646493, -0.5400638737290844871, 0.3530559997133364547 ) ) ;
#55435=CARTESIAN_POINT ( 'NONE',  ( 0.3149606299212603933, -0.1870078740157479769, 0.3641732283464567677 ) ) ;
#55436=ORIENTED_EDGE ( 'NONE', *, *, #61689, .F. ) ;
#55440=CARTESIAN_POINT ( 'NONE',  ( -0.7611548556430438595, 0.2306618581243848609, 0.2411417322834645549 ) ) ;
#55441=CARTESIAN_POINT ( 'NONE',  ( -0.03937007874015669567, 0.2952755905511811885, 0.000000000000000000 ) ) ;
#55442=CARTESIAN_POINT ( 'NONE',  ( -0.3937007874015740483, -0.1870078740157479769, 0.4822834645669291653 ) ) ;
#55443=CARTESIAN_POINT ( 'NONE',  ( 0.8923884514435703741, 0.2306618581243848609, 0.2411417322834645549 ) ) ;
#55444=CARTESIAN_POINT ( 'NONE',  ( -1.161417322834644716, 0.1660481256975885056, 0.3530559997133364547 ) ) ;
#55445=CARTESIAN_POINT ( 'NONE',  ( -0.4002624671916004129, -0.05778040916215560624, -0.4822834645669293319 ) ) ;
#55446=CARTESIAN_POINT ( 'NONE',  ( 0.6364829396325465405, -0.05778040916215522460, 0.4822834645669289988 ) ) ;
#55447=CARTESIAN_POINT ( 'NONE',  ( 0.3674540682414705883, 0.2306618581243847221, -0.2411417322834647770 ) ) ;
#55449=CARTESIAN_POINT ( 'NONE',  ( -0.4002624671916004129, -0.2845877964562159024, 0.3641732283464567677 ) ) ;
#55453=CARTESIAN_POINT ( 'NONE',  ( -1.227034120734907585, 0.1771653543307087630, 0.09757992244046791164 ) ) ;
#55454=CARTESIAN_POINT ( 'NONE',  ( -0.3937007874015740483, -0.1870078740157479769, 0.4822834645669291653 ) ) ;
#55455=DIRECTION ( 'NONE',  ( 0.000000000000000000, 1.000000000000000000, 0.000000000000000000 ) ) ;
#55456=CARTESIAN_POINT ( 'NONE',  ( -0.7742782152230965886, 0.05413385826771666132, 0.4176697321401328100 ) ) ;
#55457=CARTESIAN_POINT ( 'NONE',  ( -0.7217847769028863381, 0.05413385826771626580, -0.4176697321401330321 ) ) ;
#55458=CARTESIAN_POINT ( 'NONE',  ( -1.437007874015747477, 0.1660481256975883668, -0.3530559997133364547 ) ) ;
#55460=CARTESIAN_POINT ( 'NONE',  ( 0.8070866141732289112, -0.4536011799217368745, -0.2665933059059886201 ) ) ;
#55463=CARTESIAN_POINT ( 'NONE',  ( 0.2165354330708668673, 0.07958543189024071263, -0.2665933059059888421 ) ) ;
#55464=CARTESIAN_POINT ( 'NONE',  ( -0.3937007874015740483, -0.1870078740157479769, 0.4822834645669291653 ) ) ;
#55465=CARTESIAN_POINT ( 'NONE',  ( 0.07874015748031558404, -0.1870078740157479769, 0.4822834645669291653 ) ) ;
#55472=CARTESIAN_POINT ( 'NONE',  ( -0.8070866141732276899, -0.4536011799217367080, 0.2665933059059888421 ) ) ;
#55473=CARTESIAN_POINT ( 'NONE',  ( -1.122047244094487306, -0.5400638737290844871, 0.3530559997133364547 ) ) ;
#55475=FACE_OUTER_BOUND ( 'NONE', #14508, .T. ) ;
#55477=CARTESIAN_POINT ( 'NONE',  ( 1.338582677165355062, -0.1870078740157479769, 0.4822834645669291653 ) ) ;
#55478=CARTESIAN_POINT ( 'NONE',  ( 0.6561679790026253567, 0.2306618581243848609, 0.2411417322834645549 ) ) ;
#55479=CARTESIAN_POINT ( 'NONE',  ( 0.4265091863517067594, 0.2952755905511811885, 0.1292274648535926551 ) ) ;
#55480=CARTESIAN_POINT ( 'NONE',  ( -0.8267716535433065062, 0.1771653543307087630, 0.000000000000000000 ) ) ;
#55481=B_SPLINE_CURVE_WITH_KNOTS ( 'NONE', 3,
 ( #43966, #63338, #82703, #36431 ),
 .UNSPECIFIED., .F., .F.,
 ( 4, 4 ),
 ( 3.593986969192262371E-07, 0.001287825409103120775 ),
 .UNSPECIFIED. ) ;
#55482=CARTESIAN_POINT ( 'NONE',  ( -0.4527559055118102749, 0.1660481256975885056, 0.3530559997133364547 ) ) ;
#55484=CARTESIAN_POINT ( 'NONE',  ( -0.3412073490813641308, -0.6046776061558807314, 0.2411417322834647770 ) ) ;
#55486=CARTESIAN_POINT ( 'NONE',  ( 1.482939632545932307, -0.004921259842519870586, -0.3153832671262229437 ) ) ;
#55487=CARTESIAN_POINT ( 'NONE',  ( -0.4658792650918627265, -0.08942795157527998196, 0.3641732283464567121 ) ) ;
#55489=CARTESIAN_POINT ( 'NONE',  ( 1.338582677165355062, -0.1870078740157479769, 0.3641732283464567677 ) ) ;
#55490=CARTESIAN_POINT ( 'NONE',  ( -1.154855643044618851, -0.6046776061558809534, -0.2411417322834644161 ) ) ;
#55491=CARTESIAN_POINT ( 'NONE',  ( -0.9973753280839886548, 0.1283753931104748280, 0.1820866141732283561 ) ) ;
#55493=CARTESIAN_POINT ( 'NONE',  ( -1.286089238845143479, -0.6046776061558807314, 0.2411417322834647770 ) ) ;
#55494=CARTESIAN_POINT ( 'NONE',  ( -0.4265091863517051496, -0.6692913385826771977, 0.1292274648535927661 ) ) ;
#55495=CARTESIAN_POINT ( 'NONE',  ( 0.4658792650918641698, -0.05778040916215560624, -0.4822834645669293319 ) ) ;
#55498=CARTESIAN_POINT ( 'NONE',  ( 0.2230971128608932319, -0.3690944881889763329, 0.3153832671262228327 ) ) ;
#55499=CARTESIAN_POINT ( 'NONE',  ( -1.633858267716534529, -0.4536011799217368745, -0.2665933059059886201 ) ) ;
#55500=CARTESIAN_POINT ( 'NONE',  ( 0.7349081364829403995, 0.2306618581243848609, 0.2411417322834645549 ) ) ;
#55501=CARTESIAN_POINT ( 'NONE',  ( -1.587926509186350810, -0.3690944881889763329, 0.3153832671262228327 ) ) ;
#55503=CARTESIAN_POINT ( 'NONE',  ( 1.437007874015748810, 0.07958543189024085140, 0.2665933059059887866 ) ) ;
#55504=CARTESIAN_POINT ( 'NONE',  ( -1.036745406824146176, 0.05413385826771626580, -0.4176697321401330321 ) ) ;
#55505=CARTESIAN_POINT ( 'NONE',  ( -0.1115485564304453947, -0.5511811023622046335, 0.09757992244046803654 ) ) ;
#55506=DIRECTION ( 'NONE',  ( 1.000000000000000000, -0.000000000000000000, -0.000000000000000000 ) ) ;
#55507=CARTESIAN_POINT ( 'NONE',  ( 0.08530183727034192087, -0.2845877964562161244, -0.3641732283464567121 ) ) ;
#55508=CARTESIAN_POINT ( 'NONE',  ( -0.2559055118110227234, -0.5400638737290844871, 0.3530559997133364547 ) ) ;
#55511=CARTESIAN_POINT ( 'NONE',  ( 0.4461942257217855201, -0.5023911411419708095, 0.1820866141732285504 ) ) ;
#55512=CARTESIAN_POINT ( 'NONE',  ( 0.1443569553805781891, 0.05413385826771626580, -0.4176697321401330321 ) ) ;
#55513=CARTESIAN_POINT ( 'NONE',  ( -0.5183727034120726440, 0.2952755905511811885, 0.1292274648535926551 ) ) ;
#55514=CARTESIAN_POINT ( 'NONE',  ( -0.7217847769028863381, -0.3690944881889763329, 0.3153832671262228327 ) ) ;
#55516=CARTESIAN_POINT ( 'NONE',  ( -0.5249343832020990641, 0.1283753931104748280, 0.1820866141732283561 ) ) ;
#55517=CARTESIAN_POINT ( 'NONE',  ( 0.09842519685039434474, 0.1660481256975885056, 0.3530559997133364547 ) ) ;
#55518=CARTESIAN_POINT ( 'NONE',  ( -1.200787401574802349, 0.07958543189024071263, -0.2665933059059888421 ) ) ;
#55520=CARTESIAN_POINT ( 'NONE',  ( 1.515748031496063186, -0.5400638737290845981, -0.3530559997133363437 ) ) ;
#55521=CARTESIAN_POINT ( 'NONE',  ( 0.4609447788686172331, 1.990046790791744833E-15, -0.3791475997938225651 ) ) ;
#55522=ORIENTED_EDGE ( 'NONE', *, *, #79988, .T. ) ;
#55523=CARTESIAN_POINT ( 'NONE',  ( -1.561679790026246017, -0.004921259842519576551, 0.3153832671262227771 ) ) ;
#55524=CARTESIAN_POINT ( 'NONE',  ( -0.2887139107611542133, 0.2306618581243848609, 0.2411417322834645549 ) ) ;
#55525=CARTESIAN_POINT ( 'NONE',  ( -1.299212598425196097, 0.2952755905511811885, 0.000000000000000000 ) ) ;
#55528=CARTESIAN_POINT ( 'NONE',  ( 1.561679790026247350, 0.05413385826771626580, -0.4176697321401330321 ) ) ;
#55529=CARTESIAN_POINT ( 'NONE',  ( 0.3543307086614181922, -0.6692913385826771977, 8.415575281601705876E-17 ) ) ;
#55532=CARTESIAN_POINT ( 'NONE',  ( 1.463254593175853824, 0.1771653543307087075, -0.09757992244046823083 ) ) ;
#55534=VERTEX_POINT ( 'NONE', #49756 ) ;
#55535=CARTESIAN_POINT ( 'NONE',  ( -1.017060367454067249, -0.08942795157527998196, 0.3641732283464567121 ) ) ;
#55537=ORIENTED_EDGE ( 'NONE', *, *, #43837, .F. ) ;
#55538=CARTESIAN_POINT ( 'NONE',  ( 0.3280839895013130669, 0.05413385826771666132, 0.4176697321401328100 ) ) ;
#55539=CARTESIAN_POINT ( 'NONE',  ( -0.4002624671916004129, -0.05778040916215560624, -0.4822834645669293319 ) ) ;
#55540=CARTESIAN_POINT ( 'NONE',  ( -1.122047244094487306, 0.1660481256975883668, -0.3530559997133364547 ) ) ;
#55541=CARTESIAN_POINT ( 'NONE',  ( 1.062992125984252745, 0.2952755905511811885, 0.000000000000000000 ) ) ;
#55543=CARTESIAN_POINT ( 'NONE',  ( -1.404199475065615932, -0.3690944881889765550, -0.3153832671262227771 ) ) ;
#55545=CARTESIAN_POINT ( 'NONE',  ( 0.08530183727034192087, -0.05778040916215522460, 0.4822834645669289988 ) ) ;
#55546=CARTESIAN_POINT ( 'NONE',  ( -0.9908136482939626788, 0.2952755905511811885, 0.1292274648535926551 ) ) ;
#55548=CARTESIAN_POINT ( 'NONE',  ( -1.581364829396324945, -0.05778040916215560624, -0.4822834645669293319 ) ) ;
#55551=CARTESIAN_POINT ( 'NONE',  ( 1.043307086614173818, 0.07958543189024085140, 0.2665933059059887866 ) ) ;
#55554=CARTESIAN_POINT ( 'NONE',  ( -0.8333333333333323711, 0.2952755905511811885, 0.1292274648535926551 ) ) ;
#55556=CARTESIAN_POINT ( 'NONE',  ( 0.3674540682414705883, 0.1283753931104746893, -0.1820866141732285504 ) ) ;
#55557=CARTESIAN_POINT ( 'NONE',  ( -1.679790026246718693, 0.2306618581243847221, -0.2411417322834647770 ) ) ;
#55558=CARTESIAN_POINT ( 'NONE',  ( 0.7414698162729663755, -0.6692913385826773087, -0.1292274648535924053 ) ) ;
#55559=CARTESIAN_POINT ( 'NONE',  ( 0.4986876640419954376, 0.2306618581243848609, 0.2411417322834645549 ) ) ;
#55560=CARTESIAN_POINT ( 'NONE',  ( -0.2362204724409442680, -0.1870078740157480879, -0.4822834645669291653 ) ) ;
#55561=VECTOR ( 'NONE', #18608, 39.37007874015748143 ) ;
#55563=CARTESIAN_POINT ( 'NONE',  ( -0.9776902887139098386, 0.2952755905511810774, -0.1292274648535930714 ) ) ;
#55565=CARTESIAN_POINT ( 'NONE',  ( 1.430446194225722500, -0.004921259842519576551, 0.3153832671262227771 ) ) ;
#55566=CARTESIAN_POINT ( 'NONE',  ( -1.154855643044618851, 0.2306618581243848609, 0.2411417322834645549 ) ) ;
#55567=CARTESIAN_POINT ( 'NONE',  ( 1.200787401574803681, 0.1660481256975885056, 0.3530559997133364547 ) ) ;
#55568=CARTESIAN_POINT ( 'NONE',  ( 1.325459317585302665, -0.4281496062992124485, 0.4176697321401328655 ) ) ;
#55570=CARTESIAN_POINT ( 'NONE',  ( -0.7283464566929126471, 0.1660481256975883668, -0.3530559997133364547 ) ) ;
#55572=CARTESIAN_POINT ( 'NONE',  ( 0.1115485564304467270, -0.6692913385826773087, -0.1292274648535924053 ) ) ;
#55574=CARTESIAN_POINT ( 'NONE',  ( -0.4461942257217840213, -0.6046776061558809534, -0.2411417322834644161 ) ) ;
#55575=CARTESIAN_POINT ( 'NONE',  ( -1.555118110236219930, -0.4536011799217368745, -0.2665933059059886201 ) ) ;
#55576=CARTESIAN_POINT ( 'NONE',  ( 0.7086614173228353852, -0.1870078740157479769, 0.3641732283464567677 ) ) ;
#55577=CARTESIAN_POINT ( 'NONE',  ( 1.148293963254593653, 0.2952755905511810774, -0.1292274648535930714 ) ) ;
#55579=CARTESIAN_POINT ( 'NONE',  ( 0.9186351706036752773, 0.1283753931104746893, -0.1820866141732285504 ) ) ;
#55580=CARTESIAN_POINT ( 'NONE',  ( 1.003937007874016185, 0.1660481256975883668, -0.3530559997133364547 ) ) ;
#55582=CARTESIAN_POINT ( 'NONE',  ( -0.6364829396325453192, -0.3162353388693405765, 0.4822834645669290543 ) ) ;
#55584=CARTESIAN_POINT ( 'NONE',  ( 1.535433070866142335, -0.5511811023622047445, 6.969142054262312111E-17 ) ) ;
#55585=CARTESIAN_POINT ( 'NONE',  ( -0.4790026246719154557, -0.3162353388693405765, 0.4822834645669290543 ) ) ;
#55586=CARTESIAN_POINT ( 'NONE',  ( -0.006561679790025524116, -0.3162353388693405765, 0.4822834645669290543 ) ) ;
#55588=CARTESIAN_POINT ( 'NONE',  ( 0.1443569553805781891, -0.4281496062992124485, 0.4176697321401328655 ) ) ;
#55589=CARTESIAN_POINT ( 'NONE',  ( 0.1181102362204730916, 0.1771653543307087630, 0.000000000000000000 ) ) ;
#55591=CARTESIAN_POINT ( 'NONE',  ( 0.05905511811023709395, -0.4536011799217367080, 0.2665933059059888421 ) ) ;
#55592=CARTESIAN_POINT ( 'NONE',  ( 0.6496062992125991586, 0.07958543189024085140, 0.2665933059059887866 ) ) ;
#55593=CARTESIAN_POINT ( 'NONE',  ( -0.7426113562971995430, 2.793565526369265584, -0.5309055118110234117 ) ) ;
#55595=CARTESIAN_POINT ( 'NONE',  ( 0.4133858267716541968, 0.1660481256975885056, 0.3530559997133364547 ) ) ;
#55598=CARTESIAN_POINT ( 'NONE',  ( 1.391076115485564868, 0.1283753931104746893, -0.1820866141732285504 ) ) ;
#55600=CARTESIAN_POINT ( 'NONE',  ( -0.2099737532808391705, -0.5023911411419708095, -0.1820866141732282451 ) ) ;
#55601=CARTESIAN_POINT ( 'NONE',  ( -0.3871391076115476282, -0.05778040916215522460, 0.4822834645669289988 ) ) ;
#55602=CARTESIAN_POINT ( 'NONE',  ( 0.9973753280839902091, -0.5023911411419708095, 0.1820866141732285504 ) ) ;
#55603=CARTESIAN_POINT ( 'NONE',  ( -1.614173228346456268, -0.5511811023622047445, 6.969142054262312111E-17 ) ) ;
#55604=CARTESIAN_POINT ( 'NONE',  ( -1.358267716535432434, 0.1660481256975883668, -0.3530559997133364547 ) ) ;
#55606=CARTESIAN_POINT ( 'NONE',  ( 8.195543980992789655E-16, -0.1870078740157480879, -0.4822834645669291653 ) ) ;
#55607=CARTESIAN_POINT ( 'NONE',  ( 1.233595800524935227, 0.2306618581243847221, -0.2411417322834647770 ) ) ;
#55609=CARTESIAN_POINT ( 'NONE',  ( 0.2559055118110243332, -0.5400638737290845981, -0.3530559997133363437 ) ) ;
#55610=CARTESIAN_POINT ( 'NONE',  ( 1.417322834645670104, -0.1870078740157480879, -0.4822834645669291653 ) ) ;
#55611=CARTESIAN_POINT ( 'NONE',  ( 0.7742782152230979209, 0.05413385826771626580, -0.4176697321401330321 ) ) ;
#55612=CARTESIAN_POINT ( 'NONE',  ( -1.666666666666665853, -0.004921259842519870586, -0.3153832671262229437 ) ) ;
#55613=CARTESIAN_POINT ( 'NONE',  ( 0.5905511811023629321, 0.1771653543307087630, 0.000000000000000000 ) ) ;
#55614=CARTESIAN_POINT ( 'NONE',  ( 1.627296587926509996, -0.6046776061558807314, 0.2411417322834647770 ) ) ;
#55615=CARTESIAN_POINT ( 'NONE',  ( 0.2362204724409456558, -0.1870078740157480601, -0.3641732283464567677 ) ) ;
#55617=CARTESIAN_POINT ( 'NONE',  ( -0.4068241469816264999, -0.4281496062992124485, 0.4176697321401328655 ) ) ;
#55618=CARTESIAN_POINT ( 'NONE',  ( 0.5314960629921264834, 0.1660481256975883668, -0.3530559997133364547 ) ) ;
#55619=CARTESIAN_POINT ( 'NONE',  ( -0.3608923884514428360, 0.2952755905511811885, 0.1292274648535926551 ) ) ;
#55622=CARTESIAN_POINT ( 'NONE',  ( -0.1968503937007867743, -0.5511811023622047445, 6.969142054262312111E-17 ) ) ;
#55623=CARTESIAN_POINT ( 'NONE',  ( 0.9055118110236227702, -0.6692913385826771977, 8.415575281601705876E-17 ) ) ;
#55624=CARTESIAN_POINT ( 'NONE',  ( 0.8923884514435703741, 0.1283753931104748280, 0.1820866141732283561 ) ) ;
#55625=CARTESIAN_POINT ( 'NONE',  ( 0.2427821522309719648, -0.05778040916215522460, 0.4822834645669289988 ) ) ;
#55627=CARTESIAN_POINT ( 'NONE',  ( 1.600415083108465142, 1.509172534626478823, 0.1324231768467332149 ) ) ;
#55630=CARTESIAN_POINT ( 'NONE',  ( -1.417322834645668772, -0.1870078740157480879, -0.4822834645669291653 ) ) ;
#55631=CARTESIAN_POINT ( 'NONE',  ( -0.5446194225721777693, -0.3162353388693409650, -0.4822834645669289433 ) ) ;
#55635=CARTESIAN_POINT ( 'NONE',  ( 0.3871391076115493490, -0.2845877964562159024, 0.3641732283464567677 ) ) ;
#55637=CARTESIAN_POINT ( 'NONE',  ( 1.272965879265092637, 0.05413385826771666132, 0.4176697321401328100 ) ) ;
#55639=CARTESIAN_POINT ( 'NONE',  ( 1.003937007874016185, 0.1660481256975883391, -0.3530559997133364547 ) ) ;
#55641=CARTESIAN_POINT ( 'NONE',  ( 1.692913385826772421, 0.2952755905511811885, 0.000000000000000000 ) ) ;
#55642=CARTESIAN_POINT ( 'NONE',  ( 1.187664041994751285, -0.2845877964562161244, -0.3641732283464567121 ) ) ;
#55643=CARTESIAN_POINT ( 'NONE',  ( 0.4461942257217856311, 0.2306618581243847221, -0.2411417322834647770 ) ) ;
#55645=CARTESIAN_POINT ( 'NONE',  ( -0.5118110236220466680, 0.2952755905511811885, 0.000000000000000000 ) ) ;
#55646=CARTESIAN_POINT ( 'NONE',  ( -0.7677165354330699465, 0.07958543189024085140, 0.2665933059059887866 ) ) ;
#55648=CARTESIAN_POINT ( 'NONE',  ( 0.3608923884514443348, 0.2952755905511810774, -0.1292274648535930714 ) ) ;
#55649=CARTESIAN_POINT ( 'NONE',  ( -0.2690288713910754526, 0.2952755905511810774, -0.1292274648535930714 ) ) ;
#55650=DIRECTION ( 'NONE',  ( 0.000000000000000000, 0.000000000000000000, 1.000000000000000000 ) ) ;
#55653=CARTESIAN_POINT ( 'NONE',  ( 0.8070866141732289112, -0.5400638737290845981, -0.3530559997133363437 ) ) ;
#55654=CARTESIAN_POINT ( 'NONE',  ( -0.4199475065616791736, 0.2306618581243847221, -0.2411417322834647770 ) ) ;
#55655=CARTESIAN_POINT ( 'NONE',  ( -1.384514435695537005, -0.6692913385826773087, -0.1292274648535924053 ) ) ;
#55656=CARTESIAN_POINT ( 'NONE',  ( 1.194225721784777594, -0.4281496062992127816, -0.4176697321401328100 ) ) ;
#55657=CARTESIAN_POINT ( 'NONE',  ( 0.3805774278215230400, -0.4281496062992124485, 0.4176697321401328655 ) ) ;
#55659=CARTESIAN_POINT ( 'NONE',  ( -0.2624671916010490880, 0.2306618581243847221, -0.2411417322834647770 ) ) ;
#55660=CARTESIAN_POINT ( 'NONE',  ( 0.3346456692913393205, -0.5400638737290845981, -0.3530559997133363437 ) ) ;
#55661=CARTESIAN_POINT ( 'NONE',  ( -0.5118110236220466680, 0.2952755905511811885, 0.000000000000000000 ) ) ;
#55663=CARTESIAN_POINT ( 'NONE',  ( 0.3871391076115493490, -0.2845877964562159024, 0.3641732283464567677 ) ) ;
#55664=CARTESIAN_POINT ( 'NONE',  ( 1.607611548556431069, -0.5511811023622048555, -0.09757992244046775898 ) ) ;
#55666=CARTESIAN_POINT ( 'NONE',  ( 0.2821522309711292364, -0.6692913385826771977, 0.1292274648535927661 ) ) ;
#55667=SURFACE_STYLE_USAGE ( .BOTH. , #10253 ) ;
#55668=CARTESIAN_POINT ( 'NONE',  ( 1.437007874015748810, 0.1660481256975885056, 0.3530559997133364547 ) ) ;
#55671=VERTEX_POINT ( 'NONE', #51816 ) ;
#55672=CARTESIAN_POINT ( 'NONE',  ( 0.8858267716535438430, 0.1660481256975885056, 0.3530559997133364547 ) ) ;
#55673=CARTESIAN_POINT ( 'NONE',  ( 0.08530183727034192087, -0.2845877964562161244, -0.3641732283464567121 ) ) ;
#55674=CARTESIAN_POINT ( 'NONE',  ( 0.9573014326657177664, 0.000000000000000000, 0.3464511005275205946 ) ) ;
#55675=CARTESIAN_POINT ( 'NONE',  ( -1.220472440944882386, -0.1870078740157480046, 1.254653134982923898E-17 ) ) ;
#55677=CARTESIAN_POINT ( 'NONE',  ( -0.9555810825238836292, -3.764720552277026557E-15, -0.4118477457933000796 ) ) ;
#55682=CARTESIAN_POINT ( 'NONE',  ( 0.5971128608923890191, -0.6692913385826771977, 0.1292274648535927661 ) ) ;
#55683=CARTESIAN_POINT ( 'NONE',  ( -0.9383202099737524282, -0.3162353388693409650, -0.4822834645669289433 ) ) ;
#55684=CARTESIAN_POINT ( 'NONE',  ( -0.8923884514435688198, 0.2306618581243847221, -0.2411417322834647770 ) ) ;
#55685=CARTESIAN_POINT ( 'NONE',  ( 0.7086614173228352742, -0.1870078740157480879, -0.4822834645669291653 ) ) ;
#55686=CARTESIAN_POINT ( 'NONE',  ( 1.522309711286089939, -0.6046776061558809534, -0.2411417322834644161 ) ) ;
#55687=CARTESIAN_POINT ( 'NONE',  ( 1.220472440944882608, 0.1771653543307087630, 0.000000000000000000 ) ) ;
#55688=CARTESIAN_POINT ( 'NONE',  ( 1.450131233595801428, -0.5511811023622048555, -0.09757992244046775898 ) ) ;
#55689=CARTESIAN_POINT ( 'NONE',  ( -0.9317585301837263412, -0.4281496062992127816, -0.4176697321401328100 ) ) ;
#55691=CARTESIAN_POINT ( 'NONE',  ( 1.430446194225722500, -0.4281496062992127816, -0.4176697321401328100 ) ) ;
#55693=CARTESIAN_POINT ( 'NONE',  ( -0.3280839895013117347, 0.05413385826771626580, -0.4176697321401330321 ) ) ;
#55694=CARTESIAN_POINT ( 'NONE',  ( 1.128608923884515169, -0.6046776061558809534, -0.2411417322834644161 ) ) ;
#55695=CARTESIAN_POINT ( 'NONE',  ( -0.7478466213799878082, 1.968503937007873850, 0.5309055118110236338 ) ) ;
#55696=CARTESIAN_POINT ( 'NONE',  ( -1.062992125984250968, 0.1771653543307087630, 0.000000000000000000 ) ) ;
#55697=CARTESIAN_POINT ( 'NONE',  ( 0.4724409448818904789, -0.1870078740157480879, -0.4822834645669291653 ) ) ;
#55698=CARTESIAN_POINT ( 'NONE',  ( 0.7283464566929140904, -0.4536011799217368745, -0.2665933059059886201 ) ) ;
#55700=CARTESIAN_POINT ( 'NONE',  ( -1.292650918635170010, -0.5511811023622046335, 0.09757992244046803654 ) ) ;
#55701=CARTESIAN_POINT ( 'NONE',  ( 1.561679790026247350, 0.05413385826771626580, -0.4176697321401330321 ) ) ;
#55703=CARTESIAN_POINT ( 'NONE',  ( -0.1640419947506555343, -0.2845877964562159024, 0.3641732283464567677 ) ) ;
#55704=CARTESIAN_POINT ( 'NONE',  ( -0.09186351706036689768, 0.05413385826771626580, -0.4176697321401330321 ) ) ;
#55705=CARTESIAN_POINT ( 'NONE',  ( -1.227034120734907141, -0.5511811023622048555, -0.09757992244046775898 ) ) ;
#55706=CARTESIAN_POINT ( 'NONE',  ( -0.7414698162729651543, 0.2952755905511810774, -0.1292274648535930714 ) ) ;
#55707=CARTESIAN_POINT ( 'NONE',  ( 1.332020997375329197, -0.3162353388693405765, 0.4822834645669290543 ) ) ;
#55709=CARTESIAN_POINT ( 'NONE',  ( -0.9120734908136475250, -0.5511811023622048555, -0.09757992244046775898 ) ) ;
#55710=DIRECTION ( 'NONE',  ( 1.000000000000000000, 0.000000000000000000, -1.692413147294446216E-16 ) ) ;
#55711=CARTESIAN_POINT ( 'NONE',  ( 1.594488188976378673, 0.1660481256975885056, 0.3530559997133364547 ) ) ;
#55713=CARTESIAN_POINT ( 'NONE',  ( -1.017060367454067249, -0.3162353388693409650, -0.4822834645669289433 ) ) ;
#55714=CARTESIAN_POINT ( 'NONE',  ( -1.272965879265091305, -0.004921259842519870586, -0.3153832671262229437 ) ) ;
#55715=CARTESIAN_POINT ( 'NONE',  ( -0.7283464566929126471, 0.07958543189024071263, -0.2665933059059888421 ) ) ;
#55717=CARTESIAN_POINT ( 'NONE',  ( 0.09842519685039434474, 0.1660481256975885056, 0.3530559997133364547 ) ) ;
#55718=CARTESIAN_POINT ( 'NONE',  ( -0.1968503937007867743, 0.1771653543307087630, 0.000000000000000000 ) ) ;
#55719=CARTESIAN_POINT ( 'NONE',  ( -1.325459317585300889, -0.3690944881889765550, -0.3153832671262227771 ) ) ;
#55720=CARTESIAN_POINT ( 'NONE',  ( -1.338582677165353729, -0.1870078740157480879, -0.4822834645669291653 ) ) ;
#55721=CARTESIAN_POINT ( 'NONE',  ( 1.312335958005249825, 0.1283753931104746893, -0.1820866141732285504 ) ) ;
#55722=CARTESIAN_POINT ( 'NONE',  ( 0.7611548556430454138, 0.2306618581243847221, -0.2411417322834647770 ) ) ;
#55724=CARTESIAN_POINT ( 'NONE',  ( 0.2427821522309719648, -0.08942795157527998196, 0.3641732283464567121 ) ) ;
#55725=VECTOR ( 'NONE', #22868, 39.37007874015748854 ) ;
#55726=CARTESIAN_POINT ( 'NONE',  ( 0.7611548556430454138, 0.2306618581243847221, -0.2411417322834647770 ) ) ;
#55728=CARTESIAN_POINT ( 'NONE',  ( 0.9055118110236227702, -0.5511811023622047445, 6.969142054262312111E-17 ) ) ;
#55730=CARTESIAN_POINT ( 'NONE',  ( -1.351706036745406347, -0.4281496062992124485, 0.4176697321401328655 ) ) ;
#55731=ADVANCED_FACE ( 'NONE', ( #57716 ), #3071, .F. ) ;
#55732=CARTESIAN_POINT ( 'NONE',  ( -0.8136482939632537770, 0.2306618581243847221, -0.2411417322834647770 ) ) ;
#55733=CARTESIAN_POINT ( 'NONE',  ( -0.2427821522309703550, -0.05778040916215560624, -0.4822834645669293319 ) ) ;
#55734=CARTESIAN_POINT ( 'NONE',  ( -1.699475065616797398, 0.1771653543307087630, 0.09757992244046791164 ) ) ;
#55736=CARTESIAN_POINT ( 'NONE',  ( 1.082677165354331228, -0.5400638737290844871, 0.3530559997133364547 ) ) ;
#55737=CARTESIAN_POINT ( 'NONE',  ( 1.496062992125984703, -0.1870078740157480601, -0.3641732283464567677 ) ) ;
#55738=CARTESIAN_POINT ( 'NONE',  ( -0.06561679790026180015, 0.05413385826771666132, 0.4176697321401328100 ) ) ;
#55739=CARTESIAN_POINT ( 'NONE',  ( 0.7283464566929140904, -0.5400638737290845981, -0.3530559997133363437 ) ) ;
#55743=CARTESIAN_POINT ( 'NONE',  ( -1.614173228346456712, 0.9921945702958917535, -0.1372047244094478091 ) ) ;
#55745=CARTESIAN_POINT ( 'NONE',  ( -0.5905511811023615998, 0.1771653543307087630, 0.000000000000000000 ) ) ;
#55746=CARTESIAN_POINT ( 'NONE',  ( -0.7874015748031489847, -0.1870078740157479769, 0.4822834645669291653 ) ) ;
#55747=CARTESIAN_POINT ( 'NONE',  ( 0.6561679790026253567, 0.2306618581243848609, 0.2411417322834645549 ) ) ;
#55750=CARTESIAN_POINT ( 'NONE',  ( -1.364829396325458521, -0.6046776061558807314, 0.2411417322834647770 ) ) ;
#55751=CARTESIAN_POINT ( 'NONE',  ( 1.207349081364829990, -0.6046776061558809534, -0.2411417322834644161 ) ) ;
#55755=EDGE_CURVE ( 'NONE', #38486, #41807, #75891, .T. ) ;
#55756=CARTESIAN_POINT ( 'NONE',  ( 0.7939632545931766261, -0.05778040916215522460, 0.4822834645669289988 ) ) ;
#55757=CARTESIAN_POINT ( 'NONE',  ( 0.6430446194225728496, 0.05413385826771666132, 0.4176697321401328100 ) ) ;
#55758=CARTESIAN_POINT ( 'NONE',  ( 1.358267716535433323, -0.4536011799217368745, -0.2665933059059886201 ) ) ;
#55759=CARTESIAN_POINT ( 'NONE',  ( -1.541994750656167090, -0.5511811023622048555, -0.09757992244046775898 ) ) ;
#55760=CARTESIAN_POINT ( 'NONE',  ( 1.607611548556431069, 0.2952755905511811885, 0.1292274648535926551 ) ) ;
#55762=CARTESIAN_POINT ( 'NONE',  ( 1.017060367454068803, -0.3162353388693405765, 0.4822834645669290543 ) ) ;
#55763=CARTESIAN_POINT ( 'NONE',  ( 2.795275590551181910, 1.535433070866142335, 0.000000000000000000 ) ) ;
#55764=CARTESIAN_POINT ( 'NONE',  ( -0.4790026246719154557, -0.3162353388693405765, 0.4822834645669290543 ) ) ;
#55765=CARTESIAN_POINT ( 'NONE',  ( -0.7414698162729651543, 0.2952755905511810774, -0.1292274648535930714 ) ) ;
#55766=CARTESIAN_POINT ( 'NONE',  ( -1.515748031496062076, -0.5400638737290844871, 0.3530559997133364547 ) ) ;
#55768=CARTESIAN_POINT ( 'NONE',  ( 0.2296587926509192634, -0.05778040916215560624, -0.4822834645669293319 ) ) ;
#55770=CARTESIAN_POINT ( 'NONE',  ( 1.489501312335958172, -0.3162353388693405765, 0.4822834645669290543 ) ) ;
#55775=CARTESIAN_POINT ( 'NONE',  ( 1.279527559055118724, 0.07958543189024085140, 0.2665933059059887866 ) ) ;
#55778=CARTESIAN_POINT ( 'NONE',  ( -0.1312335958005241554, 0.1539470093639523085, 0.1968503937007873850 ) ) ;
#55782=CARTESIAN_POINT ( 'NONE',  ( -0.6627296587926501115, 0.1771653543307087075, -0.09757992244046823083 ) ) ;
#55783=CARTESIAN_POINT ( 'NONE',  ( -1.377952755905511140, 0.1771653543307087630, 0.000000000000000000 ) ) ;
#55785=CARTESIAN_POINT ( 'NONE',  ( -1.646981627296586703, -0.05778040916215522460, 0.4822834645669289988 ) ) ;
#55786=EDGE_CURVE ( 'NONE', #42092, #24707, #82711, .T. ) ;
#55787=CARTESIAN_POINT ( 'NONE',  ( 0.6167979002624678353, -0.4281496062992124485, 0.4176697321401328655 ) ) ;
#55788=CARTESIAN_POINT ( 'NONE',  ( -1.174540682414697335, -0.05778040916215522460, 0.4822834645669289988 ) ) ;
#55790=ORIENTED_EDGE ( 'NONE', *, *, #68271, .F. ) ;
#55791=CARTESIAN_POINT ( 'NONE',  ( 1.410761154855643795, -0.3162353388693405765, 0.4822834645669290543 ) ) ;
#55794=CYLINDRICAL_SURFACE ( 'NONE', #42525, 2.362204724409449508 ) ;
#55795=CARTESIAN_POINT ( 'NONE',  ( -0.6430446194225712953, 0.05413385826771626580, -0.4176697321401330321 ) ) ;
#55796=CARTESIAN_POINT ( 'NONE',  ( 1.633858267716535639, -0.5400638737290844871, 0.3530559997133364547 ) ) ;
#55797=DIRECTION ( 'NONE',  ( 0.000000000000000000, 0.000000000000000000, -1.000000000000000000 ) ) ;
#55798=CARTESIAN_POINT ( 'NONE',  ( 0.6561679790026253567, 0.1539470093639523085, 0.1968503937007873850 ) ) ;
#55799=CARTESIAN_POINT ( 'NONE',  ( 1.620734908136483465, -0.6692913385826771977, 0.1292274648535927661 ) ) ;
#55800=CARTESIAN_POINT ( 'NONE',  ( -0.8858267716535425107, 0.1660481256975883668, -0.3530559997133364547 ) ) ;
#55803=CARTESIAN_POINT ( 'NONE',  ( 0.1377952755905518800, -0.4536011799217367080, 0.2665933059059888421 ) ) ;
#55805=CARTESIAN_POINT ( 'NONE',  ( -0.1443569553805765515, -0.3690944881889765550, -0.3153832671262227771 ) ) ;
#55806=CARTESIAN_POINT ( 'NONE',  ( 0.4593175853018379162, -0.3690944881889763329, 0.3153832671262228327 ) ) ;
#55807=CARTESIAN_POINT ( 'NONE',  ( 0.6430446194225728496, 0.05413385826771666132, 0.4176697321401328100 ) ) ;
#55808=CARTESIAN_POINT ( 'NONE',  ( -0.6824146981627288167, 0.1283753931104748280, 0.1820866141732283561 ) ) ;
#55810=CARTESIAN_POINT ( 'NONE',  ( -1.581364829396324945, -0.05778040916215560624, -0.4822834645669293319 ) ) ;
#55812=CARTESIAN_POINT ( 'NONE',  ( -1.017060367454067249, -0.05778040916215522460, 0.4822834645669289988 ) ) ;
#55814=CARTESIAN_POINT ( 'NONE',  ( 0.2427821522309716595, -0.3162353388693409650, -0.4822834645669289433 ) ) ;
#55815=CARTESIAN_POINT ( 'NONE',  ( -0.3805774278215216522, 0.05413385826771666132, 0.4176697321401328100 ) ) ;
#55816=CARTESIAN_POINT ( 'NONE',  ( 1.049868766404200349, 0.1283753931104748280, 0.1820866141732283561 ) ) ;
#55817=CARTESIAN_POINT ( 'NONE',  ( -0.006561679790025524116, -0.2845877964562159024, 0.3641732283464567677 ) ) ;
#55818=CARTESIAN_POINT ( 'NONE',  ( -0.05905511811023545637, -0.5400638737290845981, -0.3530559997133363437 ) ) ;
#55819=CARTESIAN_POINT ( 'NONE',  ( -1.135170603674539924, 0.2952755905511810774, -0.1292274648535930714 ) ) ;
#55821=CARTESIAN_POINT ( 'NONE',  ( -1.011689015874862818, -4.014535696949182149E-15, 0.3627989612356152249 ) ) ;
#55822=CARTESIAN_POINT ( 'NONE',  ( 0.05249343832021075018, -0.6046776061558807314, 0.2411417322834647770 ) ) ;
#55826=CARTESIAN_POINT ( 'NONE',  ( 1.279527559055118724, 0.1660481256975885056, 0.3530559997133364547 ) ) ;
#55827=CARTESIAN_POINT ( 'NONE',  ( -0.7283464566929126471, 0.07958543189024071263, -0.2665933059059888421 ) ) ;
#55828=CARTESIAN_POINT ( 'NONE',  ( -0.3674540682414692561, -0.6046776061558809534, -0.2411417322834644161 ) ) ;
#55829=CARTESIAN_POINT ( 'NONE',  ( 1.450131233595801428, -0.6692913385826773087, -0.1292274648535924053 ) ) ;
#55830=CARTESIAN_POINT ( 'NONE',  ( 0.7283464566929143125, 0.1660481256975885056, 0.3530559997133364547 ) ) ;
#55832=CARTESIAN_POINT ( 'NONE',  ( -1.115485564304461219, -0.3690944881889763329, 0.3153832671262228327 ) ) ;
#55836=CARTESIAN_POINT ( 'NONE',  ( 1.660104986876641320, -0.08942795157527998196, 0.3641732283464567121 ) ) ;
#55837=CARTESIAN_POINT ( 'NONE',  ( 0.8727034120734912248, -0.2845877964562161244, -0.3641732283464567121 ) ) ;
#55838=CARTESIAN_POINT ( 'NONE',  ( 0.5839895013123367340, -0.6692913385826773087, -0.1292274648535924053 ) ) ;
#55841=CARTESIAN_POINT ( 'NONE',  ( 0.7545931758530189937, 0.1771653543307087075, -0.09757992244046823083 ) ) ;
#55842=CARTESIAN_POINT ( 'NONE',  ( -0.1246719160104980823, -0.6692913385826773087, -0.1292274648535924053 ) ) ;
#55843=CARTESIAN_POINT ( 'NONE',  ( -0.9383202099737524282, -0.3162353388693409650, -0.4822834645669289433 ) ) ;
#55844=CARTESIAN_POINT ( 'NONE',  ( 1.325459317585302665, -0.4281496062992124485, 0.4176697321401328655 ) ) ;
#55848=CARTESIAN_POINT ( 'NONE',  ( -0.1574803149606292529, -0.1870078740157479769, 0.3641732283464567677 ) ) ;
#55852=CARTESIAN_POINT ( 'NONE',  ( -0.7939632545931754048, -0.3162353388693405765, 0.4822834645669290543 ) ) ;
#55853=CARTESIAN_POINT ( 'NONE',  ( -0.05905511811023545637, 0.1660481256975885056, 0.3530559997133364547 ) ) ;
#55854=CARTESIAN_POINT ( 'NONE',  ( -0.4527559055118102749, -0.5400638737290845981, -0.3530559997133363437 ) ) ;
#55855=CARTESIAN_POINT ( 'NONE',  ( 0.4658792650918641698, -0.05778040916215560624, -0.4822834645669293319 ) ) ;
#55856=CARTESIAN_POINT ( 'NONE',  ( -0.3018372703412066094, -0.4281496062992127816, -0.4176697321401328100 ) ) ;
#55857=CARTESIAN_POINT ( 'NONE',  ( -1.233595800524933894, -0.6046776061558809534, -0.2411417322834644161 ) ) ;
#55858=CARTESIAN_POINT ( 'NONE',  ( -0.8333333333333323711, -0.6692913385826773087, -0.1292274648535924053 ) ) ;
#55859=CARTESIAN_POINT ( 'NONE',  ( 0.8202099737532813073, 0.2952755905511811885, 0.1292274648535926551 ) ) ;
#55860=CARTESIAN_POINT ( 'NONE',  ( 0.5971128608923890191, -0.6692913385826771977, 0.1292274648535927661 ) ) ;
#55862=CARTESIAN_POINT ( 'NONE',  ( -0.3543307086614165824, 0.1771653543307087630, 0.000000000000000000 ) ) ;
#55866=CARTESIAN_POINT ( 'NONE',  ( -1.338582677165353729, -0.1870078740157480601, -0.3641732283464567677 ) ) ;
#55867=CARTESIAN_POINT ( 'NONE',  ( -0.2887139107611542133, -0.6046776061558809534, -0.2411417322834644161 ) ) ;
#55869=CARTESIAN_POINT ( 'NONE',  ( -0.6430446194225716283, -0.4281496062992124485, 0.4176697321401328655 ) ) ;
#55870=CARTESIAN_POINT ( 'NONE',  ( -0.8398950131233589023, -0.6046776061558809534, -0.2411417322834644161 ) ) ;
#55873=CARTESIAN_POINT ( 'NONE',  ( -1.653543307086613234, -0.1870078740157480879, -0.4822834645669291653 ) ) ;
#55874=CARTESIAN_POINT ( 'NONE',  ( 1.135170603674541256, -0.5511811023622048555, -0.09757992244046775898 ) ) ;
#55875=CARTESIAN_POINT ( 'NONE',  ( -0.4827800718432839200, -5.134928753749862370E-15, -0.4281989832122469752 ) ) ;
#55877=CARTESIAN_POINT ( 'NONE',  ( -0.1049868766404193215, 0.1283753931104746893, -0.1820866141732285504 ) ) ;
#55878=CARTESIAN_POINT ( 'NONE',  ( -0.2362204724409440182, -0.1870078740157479769, 0.4822834645669291653 ) ) ;
#55879=ADVANCED_FACE ( 'NONE', ( #48234 ), #19459, .F. ) ;
#55881=CARTESIAN_POINT ( 'NONE',  ( 0.03937007874015833325, -0.6692913385826771977, 8.415575281601705876E-17 ) ) ;
#55884=CARTESIAN_POINT ( 'NONE',  ( -0.7998211177050861265, -2.609869883881465018E-15, -0.3464511005275220379 ) ) ;
#55885=ORIENTED_EDGE ( 'NONE', *, *, #9262, .F. ) ;
#55888=CARTESIAN_POINT ( 'NONE',  ( -0.6627296587926503335, -0.5511811023622046335, 0.09757992244046803654 ) ) ;
#55889=CARTESIAN_POINT ( 'NONE',  ( -0.9120734908136475250, 0.2952755905511811885, 0.1292274648535926551 ) ) ;
#55893=CARTESIAN_POINT ( 'NONE',  ( 1.181102362204725198, -0.1870078740157479769, 0.4822834645669291653 ) ) ;
#55894=CARTESIAN_POINT ( 'NONE',  ( 0.4002624671916016896, -0.3162353388693409650, -0.4822834645669289433 ) ) ;
#55895=CARTESIAN_POINT ( 'NONE',  ( 0.4658792650918641698, -0.05778040916215560624, -0.4822834645669293319 ) ) ;
#55896=CARTESIAN_POINT ( 'NONE',  ( -0.4658792650918627265, -0.2845877964562161244, -0.3641732283464567121 ) ) ;
#55897=VECTOR ( 'NONE', #71467, 39.37007874015748143 ) ;
#55899=CARTESIAN_POINT ( 'NONE',  ( -0.2624671916010490880, 0.2306618581243847221, -0.2411417322834647770 ) ) ;
#55901=CARTESIAN_POINT ( 'NONE',  ( -1.043307086614172707, 0.1660481256975883668, -0.3530559997133364547 ) ) ;
#55903=CARTESIAN_POINT ( 'NONE',  ( 1.463254593175853824, 0.1771653543307087075, -0.09757992244046823083 ) ) ;
#55904=CARTESIAN_POINT ( 'NONE',  ( -0.3608923884514428360, -0.5511811023622048555, -0.09757992244046775898 ) ) ;
#55905=CARTESIAN_POINT ( 'NONE',  ( 1.200787401574803681, 0.07958543189024085140, 0.2665933059059887866 ) ) ;
#55906=CARTESIAN_POINT ( 'NONE',  ( 1.594488188976378673, 0.07958543189024085140, 0.2665933059059887866 ) ) ;
#55907=CARTESIAN_POINT ( 'NONE',  ( -1.174540682414697335, -0.08942795157527998196, 0.3641732283464567121 ) ) ;
#55909=CARTESIAN_POINT ( 'NONE',  ( 0.6955380577427828781, -0.3690944881889763329, 0.3153832671262228327 ) ) ;
#55910=CARTESIAN_POINT ( 'NONE',  ( -0.4330708661417315697, -0.6692913385826771977, 8.415575281601705876E-17 ) ) ;
#55911=VECTOR ( 'NONE', #32595, 39.37007874015748143 ) ;
#55912=CARTESIAN_POINT ( 'NONE',  ( 1.092353285368624860, -4.408777212815537393E-16, -0.4445507791589063395 ) ) ;
#55913=CARTESIAN_POINT ( 'NONE',  ( -0.2624671916010490880, -0.5023911411419708095, 0.1820866141732285504 ) ) ;
#55915=CARTESIAN_POINT ( 'NONE',  ( 0.6824146981627303710, -0.6046776061558807314, 0.2411417322834647770 ) ) ;
#55916=CARTESIAN_POINT ( 'NONE',  ( 0.6758530183727039509, 0.2952755905511810219, -0.1292274648535930437 ) ) ;
#55917=CARTESIAN_POINT ( 'NONE',  ( 1.187664041994751285, -0.2845877964562161244, -0.3641732283464567121 ) ) ;
#55918=CARTESIAN_POINT ( 'NONE',  ( -0.9251968503937002541, 0.1660481256975885056, 0.3530559997133364547 ) ) ;
#55919=CARTESIAN_POINT ( 'NONE',  ( -0.1574803149606292529, -0.1870078740157480601, -0.3641732283464567677 ) ) ;
#55920=CARTESIAN_POINT ( 'NONE',  ( 1.033961166703849965, -2.398893483443748302E-16, 0.4281993546915529580 ) ) ;
#55921=CARTESIAN_POINT ( 'NONE',  ( 0.4330708661417329575, -0.5511811023622047445, 6.969142054262312111E-17 ) ) ;
#55922=CARTESIAN_POINT ( 'NONE',  ( -0.7020997375328074108, -0.05778040916215522460, 0.4822834645669289988 ) ) ;
#55925=CARTESIAN_POINT ( 'NONE',  ( 0.4855643044619428750, -0.004921259842519576551, 0.3153832671262227771 ) ) ;
#55926=CARTESIAN_POINT ( 'NONE',  ( -0.2624671916010490880, -0.6046776061558807314, 0.2411417322834647770 ) ) ;
#55927=CARTESIAN_POINT ( 'NONE',  ( -0.8398950131233585692, 0.2306618581243848609, 0.2411417322834645549 ) ) ;
#55928=CARTESIAN_POINT ( 'NONE',  ( -0.9186351706036736120, -0.5023911411419708095, -0.1820866141732282451 ) ) ;
#55929=DIRECTION ( 'NONE',  ( -3.096699300667737957E-16, 1.000000000000000000, -0.000000000000000000 ) ) ;
#55930=CARTESIAN_POINT ( 'NONE',  ( -0.9251968503937002541, -0.4536011799217368745, -0.2665933059059886201 ) ) ;
#55931=CARTESIAN_POINT ( 'NONE',  ( -0.1181102362204717315, -0.6692913385826771977, 8.415575281601705876E-17 ) ) ;
#55932=CARTESIAN_POINT ( 'NONE',  ( -1.141732283464566011, -0.5511811023622047445, 6.969142054262312111E-17 ) ) ;
#55933=CARTESIAN_POINT ( 'NONE',  ( -1.515748031496062076, -0.5400638737290844871, 0.3530559997133364547 ) ) ;
#55934=CARTESIAN_POINT ( 'NONE',  ( 0.01241954290193841674, 0.000000000000000000, 0.3464511005275205946 ) ) ;
#55936=CARTESIAN_POINT ( 'NONE',  ( -1.555118110236219930, 0.07958543189024085140, 0.2665933059059887866 ) ) ;
#55937=CARTESIAN_POINT ( 'NONE',  ( -0.7545931758530177724, 0.2952755905511811885, 0.1292274648535926551 ) ) ;
#55938=CARTESIAN_POINT ( 'NONE',  ( -0.5577427821522301654, -0.05778040916215560624, -0.4822834645669293319 ) ) ;
#55939=CARTESIAN_POINT ( 'NONE',  ( -1.095800524934382292, -0.3162353388693409650, -0.4822834645669289433 ) ) ;
#55942=CARTESIAN_POINT ( 'NONE',  ( 0.8005249343832028242, -0.4281496062992127816, -0.4176697321401328100 ) ) ;
#55943=CARTESIAN_POINT ( 'NONE',  ( 0.5314960629921267055, -0.5400638737290844871, 0.3530559997133364547 ) ) ;
#55946=CONICAL_SURFACE ( 'NONE', #43864, 1.181102362204724310, 0.7853981633974621568 ) ;
#55949=CARTESIAN_POINT ( 'NONE',  ( 1.384514435695538337, -0.5511811023622046335, 0.09757992244046803654 ) ) ;
#55952=CARTESIAN_POINT ( 'NONE',  ( -0.9317585301837263412, -0.3690944881889765550, -0.3153832671262227771 ) ) ;
#55955=CARTESIAN_POINT ( 'NONE',  ( 0.2296587926509192634, -0.05778040916215560624, -0.4822834645669293319 ) ) ;
#55956=CARTESIAN_POINT ( 'NONE',  ( -0.3674540682414692561, -0.6046776061558809534, -0.2411417322834644161 ) ) ;
#55957=CARTESIAN_POINT ( 'NONE',  ( -1.069553805774277722, -0.6692913385826773087, -0.1292274648535924053 ) ) ;
#55958=CARTESIAN_POINT ( 'NONE',  ( 1.194225721784777594, 0.05413385826771666132, 0.4176697321401328100 ) ) ;
#55959=CARTESIAN_POINT ( 'NONE',  ( -1.463254593175852492, 0.1771653543307087630, 0.09757992244046791164 ) ) ;
#55961=CARTESIAN_POINT ( 'NONE',  ( -0.1049868766404193215, -0.6046776061558807314, 0.2411417322834647770 ) ) ;
#55962=CARTESIAN_POINT ( 'NONE',  ( -1.345144356955379816, -0.3162353388693405765, 0.4822834645669290543 ) ) ;
#55967=CARTESIAN_POINT ( 'NONE',  ( 0.7611548556430454138, 0.1283753931104746893, -0.1820866141732285504 ) ) ;
#55970=CARTESIAN_POINT ( 'NONE',  ( -0.7480314960629914633, -0.6692913385826771977, 8.415575281601705876E-17 ) ) ;
#55972=CARTESIAN_POINT ( 'NONE',  ( -0.06561679790026180015, -0.3690944881889765550, -0.3153832671262227771 ) ) ;
#55975=CARTESIAN_POINT ( 'NONE',  ( 0.6955380577427828781, 0.05413385826771626580, -0.4176697321401330321 ) ) ;
#55976=CARTESIAN_POINT ( 'NONE',  ( 0.3412073490813655186, 0.2306618581243848609, 0.2411417322834645549 ) ) ;
#55978=CARTESIAN_POINT ( 'NONE',  ( -0.5643044619422565855, 0.05413385826771626580, -0.4176697321401330321 ) ) ;
#55980=CARTESIAN_POINT ( 'NONE',  ( -0.7020997375328074108, -0.05778040916215522460, 0.4822834645669289988 ) ) ;
#55982=CARTESIAN_POINT ( 'NONE',  ( 1.148293963254593653, 0.1771653543307087075, -0.09757992244046823083 ) ) ;
#55983=CARTESIAN_POINT ( 'NONE',  ( -0.9711286089238838626, 0.2306618581243847221, -0.2411417322834647770 ) ) ;
#55984=CARTESIAN_POINT ( 'NONE',  ( 0.8858267716535438430, 0.1660481256975885056, 0.3530559997133364547 ) ) ;
#55985=CARTESIAN_POINT ( 'NONE',  ( 1.200787401574803681, 0.1660481256975885056, 0.3530559997133364547 ) ) ;
#55987=CARTESIAN_POINT ( 'NONE',  ( -1.502624671916009680, -0.05778040916215560624, -0.4822834645669293319 ) ) ;
#55989=CARTESIAN_POINT ( 'NONE',  ( 0.1902887139107617975, 0.2952755905511811885, 0.1292274648535926551 ) ) ;
#55991=CARTESIAN_POINT ( 'NONE',  ( -1.614173228346455824, 0.1771653543307087630, 0.000000000000000000 ) ) ;
#55992=CARTESIAN_POINT ( 'NONE',  ( 0.4986876640419954376, -0.5023911411419708095, -0.1820866141732282451 ) ) ;
#55993=CARTESIAN_POINT ( 'NONE',  ( 0.7808398950131240079, -0.3162353388693405765, 0.4822834645669290543 ) ) ;
#55995=CARTESIAN_POINT ( 'NONE',  ( 0.6233595800524942554, -0.08942795157528024563, -0.3641732283464568787 ) ) ;
#55996=CARTESIAN_POINT ( 'NONE',  ( 0.5577427821522314977, -0.3162353388693409650, -0.4822834645669289433 ) ) ;
#55997=B_SPLINE_CURVE_WITH_KNOTS ( 'NONE', 3,
 ( #38078, #31768, #4862, #36437 ),
 .UNSPECIFIED., .F., .F.,
 ( 4, 4 ),
 ( 0.02951359255738795345, 0.02980295909189879799 ),
 .UNSPECIFIED. ) ;
#55999=CARTESIAN_POINT ( 'NONE',  ( -0.6167979002624665030, 0.05413385826771666132, 0.4176697321401328100 ) ) ;
#56001=CARTESIAN_POINT ( 'NONE',  ( 0.8136482939632553313, 0.1283753931104748280, 0.1820866141732283561 ) ) ;
#56002=CARTESIAN_POINT ( 'NONE',  ( 0.08530183727034192087, -0.3162353388693409650, -0.4822834645669289433 ) ) ;
#56004=CARTESIAN_POINT ( 'NONE',  ( -0.4921259842519677963, -0.5400638737290844871, 0.3530559997133364547 ) ) ;
#56005=CARTESIAN_POINT ( 'NONE',  ( 0.05249343832021075018, -0.5023911411419708095, 0.1820866141732285504 ) ) ;
#56007=CARTESIAN_POINT ( 'NONE',  ( 0.02624671916010564918, -0.5023911411419708095, -0.1820866141732282451 ) ) ;
#56008=CARTESIAN_POINT ( 'NONE',  ( 0.6889763779527563470, 0.07958543189024071263, -0.2665933059059888421 ) ) ;
#56011=CARTESIAN_POINT ( 'NONE',  ( 0.3083989501312343062, -0.05778040916215560624, -0.4822834645669293319 ) ) ;
#56015=VECTOR ( 'NONE', #81595, 39.37007874015748143 ) ;
#56016=CARTESIAN_POINT ( 'NONE',  ( 1.181102362204725198, -0.1870078740157479769, 0.3641732283464567677 ) ) ;
#56017=CARTESIAN_POINT ( 'NONE',  ( -0.1674892343164145203, -2.567464376874931580E-15, -0.4445507791589072832 ) ) ;
#56018=CARTESIAN_POINT ( 'NONE',  ( -0.5249343832020990641, -0.5023911411419708095, -0.1820866141732282451 ) ) ;
#56019=CARTESIAN_POINT ( 'NONE',  ( -0.2755905511811018171, 0.1771653543307087630, 0.000000000000000000 ) ) ;
#56020=CARTESIAN_POINT ( 'NONE',  ( -0.3149606299212590610, -0.1870078740157480879, -0.4822834645669291653 ) ) ;
#56021=CARTESIAN_POINT ( 'NONE',  ( 0.8070866141732289112, -0.4536011799217368745, -0.2665933059059886201 ) ) ;
#56023=CARTESIAN_POINT ( 'NONE',  ( 1.286089238845145033, 0.1283753931104748280, 0.1820866141732283561 ) ) ;
#56024=CARTESIAN_POINT ( 'NONE',  ( -0.02624671916010428221, 0.2306618581243847221, -0.2411417322834647770 ) ) ;
#56025=CARTESIAN_POINT ( 'NONE',  ( 1.318897637795276356, -0.5400638737290844871, 0.3530559997133364547 ) ) ;
#56027=CARTESIAN_POINT ( 'NONE',  ( 0.3018372703412079971, -0.4281496062992124485, 0.4176697321401328655 ) ) ;
#56029=CARTESIAN_POINT ( 'NONE',  ( 1.049868766404200349, 0.2306618581243848609, 0.2411417322834645549 ) ) ;
#56030=CARTESIAN_POINT ( 'NONE',  ( 0.6299212598425204535, -0.1870078740157480879, -0.4822834645669291653 ) ) ;
#56031=CARTESIAN_POINT ( 'NONE',  ( -0.7137454485294952855, 2.362204724409448620, 0.4917280318828573527 ) ) ;
#56032=CARTESIAN_POINT ( 'NONE',  ( 0.7545931758530189937, 0.1771653543307087075, -0.09757992244046823083 ) ) ;
#56033=CARTESIAN_POINT ( 'NONE',  ( 1.062992125984252745, 0.2952755905511811885, 0.000000000000000000 ) ) ;
#56034=CARTESIAN_POINT ( 'NONE',  ( 0.2690288713910767848, -0.5511811023622048555, -0.09757992244046775898 ) ) ;
#56035=CARTESIAN_POINT ( 'NONE',  ( -0.1968503937007867743, 0.2952755905511811885, 0.000000000000000000 ) ) ;
#56036=CARTESIAN_POINT ( 'NONE',  ( 0.4461942257217855201, -0.6046776061558807314, 0.2411417322834647770 ) ) ;
#56037=CARTESIAN_POINT ( 'NONE',  ( -0.6036745406824141069, -0.6046776061558809534, -0.2411417322834644161 ) ) ;
#56038=CARTESIAN_POINT ( 'NONE',  ( -0.4265091863517051496, 0.1771653543307087075, -0.09757992244046823083 ) ) ;
#56039=CARTESIAN_POINT ( 'NONE',  ( 0.7217847769028878924, -0.4281496062992127816, -0.4176697321401328100 ) ) ;
#56040=CARTESIAN_POINT ( 'NONE',  ( 0.9645669291338591078, -0.4536011799217368745, -0.2665933059059886201 ) ) ;
#56041=CARTESIAN_POINT ( 'NONE',  ( 0.2362204724409456558, -0.1870078740157479769, 0.4822834645669291653 ) ) ;
#56047=CARTESIAN_POINT ( 'NONE',  ( -1.122047244094487306, 0.1660481256975883668, -0.3530559997133364547 ) ) ;
#56048=CARTESIAN_POINT ( 'NONE',  ( -0.9580052493438311334, -0.4281496062992124485, 0.4176697321401328655 ) ) ;
#56052=CARTESIAN_POINT ( 'NONE',  ( 0.4461942257217856311, 0.1283753931104746893, -0.1820866141732285504 ) ) ;
#56054=CARTESIAN_POINT ( 'NONE',  ( 0.8136482939632553313, 0.2306618581243848609, 0.2411417322834645549 ) ) ;
#56056=CARTESIAN_POINT ( 'NONE',  ( 1.603475055217291612, 0.7166759647713492054, -0.04573490813648244807 ) ) ;
#56057=CARTESIAN_POINT ( 'NONE',  ( 1.095800524934383846, -0.05778040916215560624, -0.4822834645669293319 ) ) ;
#56058=CARTESIAN_POINT ( 'NONE',  ( 1.213910761154856299, -0.5511811023622048555, -0.09757992244046775898 ) ) ;
#56059=CARTESIAN_POINT ( 'NONE',  ( 0.04593175853018440641, -0.6692913385826771977, 0.1292274648535927661 ) ) ;
#56062=CARTESIAN_POINT ( 'NONE',  ( -0.4461942257217840213, -0.6046776061558809534, -0.2411417322834644161 ) ) ;
#56063=CARTESIAN_POINT ( 'NONE',  ( -0.9776902887139098386, -0.5511811023622046335, 0.09757992244046803654 ) ) ;
#56064=CARTESIAN_POINT ( 'NONE',  ( 0.6102362204724416372, -0.5400638737290844871, 0.3530559997133364547 ) ) ;
#56065=EDGE_CURVE ( 'NONE', #37713, #56774, #71397, .T. ) ;
#56066=CARTESIAN_POINT ( 'NONE',  ( -0.2887139107611542133, 0.2306618581243848609, 0.2411417322834645549 ) ) ;
#56067=LINE ( 'NONE', #50164, #55561 ) ;
#56068=AXIS2_PLACEMENT_3D ( 'NONE', #78298, #16401, #46702 ) ;
#56069=CARTESIAN_POINT ( 'NONE',  ( 0.4556364815871513096, 1.768811104126938094, -0.5309055118110237448 ) ) ;
#56072=CARTESIAN_POINT ( 'NONE',  ( 0.4265091863517067594, 0.2952755905511811885, 0.1292274648535926551 ) ) ;
#56073=VECTOR ( 'NONE', #60637, 39.37007874015748143 ) ;
#56074=CARTESIAN_POINT ( 'NONE',  ( -0.2362204724409442680, -0.1870078740157480879, -0.4822834645669291653 ) ) ;
#56075=CARTESIAN_POINT ( 'NONE',  ( -1.594488188976377119, 0.1660481256975883668, -0.3530559997133364547 ) ) ;
#56076=CARTESIAN_POINT ( 'NONE',  ( 0.7742782152230978099, -0.4281496062992124485, 0.4176697321401328655 ) ) ;
#56078=CARTESIAN_POINT ( 'NONE',  ( 0.4068241469816281097, 0.05413385826771666132, 0.4176697321401328100 ) ) ;
#56080=CARTESIAN_POINT ( 'NONE',  ( -0.6955380577427815458, -0.4281496062992127816, -0.4176697321401328100 ) ) ;
#56081=CARTESIAN_POINT ( 'NONE',  ( 0.1902887139107617975, -0.6692913385826773087, -0.1292274648535924053 ) ) ;
#56082=CARTESIAN_POINT ( 'NONE',  ( -0.2624671916010490880, -0.6046776061558807314, 0.2411417322834647770 ) ) ;
#56083=CARTESIAN_POINT ( 'NONE',  ( 0.1115485564304470323, 0.1771653543307087630, 0.09757992244046791164 ) ) ;
#56084=CARTESIAN_POINT ( 'NONE',  ( -1.555118110236219930, 0.1660481256975885056, 0.3530559997133364547 ) ) ;
#56086=CARTESIAN_POINT ( 'NONE',  ( -0.2624671916010490880, 0.2306618581243847221, -0.2411417322834647770 ) ) ;
#56088=CARTESIAN_POINT ( 'NONE',  ( -1.541994750656167090, -0.6692913385826773087, -0.1292274648535924053 ) ) ;
#56092=CARTESIAN_POINT ( 'NONE',  ( 0.6758530183727039509, -0.6692913385826771977, 0.1292274648535927661 ) ) ;
#56093=CARTESIAN_POINT ( 'NONE',  ( -0.006561679790025524116, -0.2845877964562159024, 0.3641732283464567677 ) ) ;
#56098=CARTESIAN_POINT ( 'NONE',  ( 0.7197590744588134859, 1.521610601467410833E-15, 0.3954985857520055270 ) ) ;
#56100=CARTESIAN_POINT ( 'NONE',  ( 0.4002624671916016896, -0.3162353388693409650, -0.4822834645669289433 ) ) ;
#56101=CARTESIAN_POINT ( 'NONE',  ( -1.371391076115484609, -0.6692913385826771977, 0.1292274648535927661 ) ) ;
#56102=CARTESIAN_POINT ( 'NONE',  ( -1.358267716535432434, 0.1660481256975883668, -0.3530559997133364547 ) ) ;
#56103=CARTESIAN_POINT ( 'NONE',  ( 0.7874015748031503170, -0.1870078740157479769, 0.4822834645669291653 ) ) ;
#56104=CARTESIAN_POINT ( 'NONE',  ( 1.450131233595801428, 0.2952755905511811885, 0.1292274648535926551 ) ) ;
#56105=CARTESIAN_POINT ( 'NONE',  ( 1.332020997375329197, -0.2845877964562159024, 0.3641732283464567677 ) ) ;
#56106=CARTESIAN_POINT ( 'NONE',  ( 1.338582677165355062, -0.1870078740157479769, 0.3641732283464567677 ) ) ;
#56107=CARTESIAN_POINT ( 'NONE',  ( -0.9383202099737524282, -0.3162353388693409650, -0.4822834645669289433 ) ) ;
#56109=CARTESIAN_POINT ( 'NONE',  ( -1.614173228346455824, 0.1771653543307087630, 0.000000000000000000 ) ) ;
#56111=CARTESIAN_POINT ( 'NONE',  ( -0.1181102362204717315, -0.6692913385826771977, 8.415575281601705876E-17 ) ) ;
#56112=CARTESIAN_POINT ( 'NONE',  ( 1.305774278215223960, -0.6692913385826771977, 0.1292274648535927661 ) ) ;
#56114=CARTESIAN_POINT ( 'NONE',  ( -1.154855643044618851, -0.5023911411419708095, -0.1820866141732282451 ) ) ;
#56115=CARTESIAN_POINT ( 'NONE',  ( 0.5052493438320218022, -0.6692913385826773087, -0.1292274648535924053 ) ) ;
#56116=CARTESIAN_POINT ( 'NONE',  ( 0.8136482939632553313, 0.1283753931104748280, 0.1820866141732283561 ) ) ;
#56118=CARTESIAN_POINT ( 'NONE',  ( -1.187664041994750175, -0.08942795157528024563, -0.3641732283464568787 ) ) ;
#56119=CARTESIAN_POINT ( 'NONE',  ( 0.8464566929133866546, -0.5400638737290844871, 0.3530559997133364547 ) ) ;
#56121=CARTESIAN_POINT ( 'NONE',  ( -0.3215223097112853146, -0.2845877964562159024, 0.3641732283464567677 ) ) ;
#56122=CARTESIAN_POINT ( 'NONE',  ( -0.6299212598425188991, -0.1870078740157479769, 0.4822834645669291653 ) ) ;
#56123=CARTESIAN_POINT ( 'NONE',  ( -1.515748031496062076, -0.4536011799217367080, 0.2665933059059888421 ) ) ;
#56124=CARTESIAN_POINT ( 'NONE',  ( -0.9251968503937002541, 0.1660481256975885056, 0.3530559997133364547 ) ) ;
#56125=CARTESIAN_POINT ( 'NONE',  ( 1.502624671916010790, -0.05778040916215522460, 0.4822834645669289988 ) ) ;
#56127=CARTESIAN_POINT ( 'NONE',  ( -0.7545931758530176614, -0.5511811023622048555, -0.09757992244046775898 ) ) ;
#56129=CARTESIAN_POINT ( 'NONE',  ( 1.377952755905512472, -0.6692913385826771977, 8.415575281601705876E-17 ) ) ;
#56132=CARTESIAN_POINT ( 'NONE',  ( -1.286089238845143479, -0.6046776061558807314, 0.2411417322834647770 ) ) ;
#56133=CARTESIAN_POINT ( 'NONE',  ( -1.358267716535432434, -0.4536011799217367080, 0.2665933059059888421 ) ) ;
#56134=CARTESIAN_POINT ( 'NONE',  ( -0.4986876640419942164, -0.5023911411419708095, 0.1820866141732285504 ) ) ;
#56136=CARTESIAN_POINT ( 'NONE',  ( -0.3608923884514428360, 0.2952755905511811885, 0.1292274648535926551 ) ) ;
#56137=CARTESIAN_POINT ( 'NONE',  ( 0.1049868766404206816, 0.1283753931104748280, 0.1820866141732283561 ) ) ;
#56138=CARTESIAN_POINT ( 'NONE',  ( -1.318897637795274802, -0.4536011799217368745, -0.2665933059059886201 ) ) ;
#56139=CARTESIAN_POINT ( 'NONE',  ( -1.305774278215222184, -0.6692913385826773087, -0.1292274648535924053 ) ) ;
#56140=CARTESIAN_POINT ( 'NONE',  ( 1.377952755905512472, -0.5511811023622047445, 6.969142054262312111E-17 ) ) ;
#56141=CARTESIAN_POINT ( 'NONE',  ( 1.102362204724410155, -0.1870078740157480879, -0.4822834645669291653 ) ) ;
#56143=CARTESIAN_POINT ( 'NONE',  ( 0.3740157480314966754, -0.4536011799217367080, 0.2665933059059888421 ) ) ;
#56146=CARTESIAN_POINT ( 'NONE',  ( 0.4855643044619430415, -0.4281496062992127816, -0.4176697321401328100 ) ) ;
#56147=CARTESIAN_POINT ( 'NONE',  ( 0.9383202099737536495, -0.2845877964562159024, 0.3641732283464567677 ) ) ;
#56149=CARTESIAN_POINT ( 'NONE',  ( -1.128608923884513837, 0.2306618581243847221, -0.2411417322834647770 ) ) ;
#56150=CARTESIAN_POINT ( 'NONE',  ( -0.8464566929133852113, 0.1660481256975885056, 0.3530559997133364547 ) ) ;
#56151=CARTESIAN_POINT ( 'NONE',  ( -0.2624671916010490880, 0.2306618581243847221, -0.2411417322834647770 ) ) ;
#56154=CARTESIAN_POINT ( 'NONE',  ( 0.5511811023622054106, -0.1870078740157480879, -0.4822834645669291653 ) ) ;
#56155=CARTESIAN_POINT ( 'NONE',  ( -1.660104986876639543, -0.05778040916215560624, -0.4822834645669293319 ) ) ;
#56156=CARTESIAN_POINT ( 'NONE',  ( -0.1115485564304453947, -0.6692913385826771977, 0.1292274648535927661 ) ) ;
#56157=CARTESIAN_POINT ( 'NONE',  ( 0.5774278215223103139, -0.6046776061558809534, -0.2411417322834644161 ) ) ;
#56163=CARTESIAN_POINT ( 'NONE',  ( -0.6627296587926503335, -0.5511811023622046335, 0.09757992244046803654 ) ) ;
#56164=CARTESIAN_POINT ( 'NONE',  ( -0.9251968503937002541, 0.1660481256975885056, 0.3530559997133364547 ) ) ;
#56165=CARTESIAN_POINT ( 'NONE',  ( 0.4986876640419954376, 0.2306618581243848609, 0.2411417322834645549 ) ) ;
#56167=CARTESIAN_POINT ( 'NONE',  ( 0.8792650918635177559, 0.05413385826771666132, 0.4176697321401328100 ) ) ;
#56168=CARTESIAN_POINT ( 'NONE',  ( -1.437007874015747477, 0.1660481256975883668, -0.3530559997133364547 ) ) ;
#56169=CARTESIAN_POINT ( 'NONE',  ( 1.161417322834646271, 0.1660481256975883668, -0.3530559997133364547 ) ) ;
#56172=CARTESIAN_POINT ( 'NONE',  ( 1.581364829396326277, -0.3162353388693409650, -0.4822834645669289433 ) ) ;
#56173=CARTESIAN_POINT ( 'NONE',  ( 0.8136482939632553313, 0.2306618581243848609, 0.2411417322834645549 ) ) ;
#56174=CARTESIAN_POINT ( 'NONE',  ( 0.4330708661417329575, -0.6692913385826771977, 8.415575281601705876E-17 ) ) ;
#56175=CARTESIAN_POINT ( 'NONE',  ( 1.246719160104987623, -0.3690944881889763329, 0.3153832671262228327 ) ) ;
#56176=CARTESIAN_POINT ( 'NONE',  ( 1.620734908136483465, -0.6692913385826771977, 0.1292274648535927661 ) ) ;
#56177=CARTESIAN_POINT ( 'NONE',  ( 1.614173228346457378, 0.2952755905511811885, 0.000000000000000000 ) ) ;
#56179=CARTESIAN_POINT ( 'NONE',  ( -0.4037097067573596210, -2.567464376874931580E-15, -0.4445507791589072832 ) ) ;
#56180=CARTESIAN_POINT ( 'NONE',  ( 0.6627296587926517768, -0.6692913385826773087, -0.1292274648535924053 ) ) ;
#56181=CARTESIAN_POINT ( 'NONE',  ( 1.384514435695538559, 0.1771653543307087075, -0.09757992244046823083 ) ) ;
#56182=CARTESIAN_POINT ( 'NONE',  ( -0.3149606299212590610, -0.1870078740157479769, 0.4822834645669291653 ) ) ;
#56183=CARTESIAN_POINT ( 'NONE',  ( -0.3805774278215216522, -0.4281496062992127816, -0.4176697321401328100 ) ) ;
#56184=CARTESIAN_POINT ( 'NONE',  ( -1.555118110236219930, -0.5400638737290845981, -0.3530559997133363437 ) ) ;
#56186=B_SPLINE_CURVE_WITH_KNOTS ( 'NONE', 3,
 ( #35933, #34271, #61176, #14919 ),
 .UNSPECIFIED., .F., .F.,
 ( 4, 4 ),
 ( 0.03408779003946453556, 0.03433871283135704611 ),
 .UNSPECIFIED. ) ;
#56189=CARTESIAN_POINT ( 'NONE',  ( 1.561679790026247350, 0.05413385826771626580, -0.4176697321401330321 ) ) ;
#56193=CARTESIAN_POINT ( 'NONE',  ( -0.7137454485294953965, 2.244094488188976388, -0.4917280318828581298 ) ) ;
#56195=CARTESIAN_POINT ( 'NONE',  ( 1.391076115485564868, -0.5023911411419708095, 0.1820866141732285504 ) ) ;
#56197=CARTESIAN_POINT ( 'NONE',  ( 1.620734908136483465, -0.5511811023622046335, 0.09757992244046803654 ) ) ;
#56198=CARTESIAN_POINT ( 'NONE',  ( -0.09115970038225217065, 2.409604939980833412E-17, -0.3464511005275205946 ) ) ;
#56202=CARTESIAN_POINT ( 'NONE',  ( -0.7414698162729651543, -0.5511811023622046335, 0.09757992244046803654 ) ) ;
#56203=CARTESIAN_POINT ( 'NONE',  ( -1.279527559055116948, -0.4536011799217367080, 0.2665933059059888421 ) ) ;
#56204=CARTESIAN_POINT ( 'NONE',  ( 0.1640419947506569498, -0.05778040916215522460, 0.4822834645669289988 ) ) ;
#56205=CARTESIAN_POINT ( 'NONE',  ( -1.312335958005248715, 0.2306618581243848609, 0.2411417322834645549 ) ) ;
#56209=CARTESIAN_POINT ( 'NONE',  ( 1.476377952755906220, 0.1660481256975883668, -0.3530559997133364547 ) ) ;
#56210=CARTESIAN_POINT ( 'NONE',  ( -1.607029103917716251, 0.2931852734392842996, 0.04634085041582033243 ) ) ;
#56212=EDGE_CURVE ( 'NONE', #43140, #66780, #8949, .T. ) ;
#56213=DIRECTION ( 'NONE',  ( 0.000000000000000000, -0.000000000000000000, -1.000000000000000000 ) ) ;
#56215=CARTESIAN_POINT ( 'NONE',  ( -0.5839895013123351797, -0.5511811023622046335, 0.09757992244046803654 ) ) ;
#56218=CARTESIAN_POINT ( 'NONE',  ( -1.253280839895012377, -0.3162353388693409650, -0.4822834645669289433 ) ) ;
#56219=CARTESIAN_POINT ( 'NONE',  ( 1.089238845144357759, 0.05413385826771626580, -0.4176697321401330321 ) ) ;
#56221=CARTESIAN_POINT ( 'NONE',  ( 0.7758157084527484981, 0.02791078216816508459, -0.4328096321851889194 ) ) ;
#56222=CARTESIAN_POINT ( 'NONE',  ( 0.6889763779527563470, 0.1012011053420775880, -0.2882089793578257453 ) ) ;
#56223=CARTESIAN_POINT ( 'NONE',  ( 1.614173228346457378, -0.6692913385826771977, 8.415575281601705876E-17 ) ) ;
#56224=CARTESIAN_POINT ( 'NONE',  ( -1.358267716535432434, 0.1660481256975883668, -0.3530559997133364547 ) ) ;
#56226=CARTESIAN_POINT ( 'NONE',  ( 0.1115485564304467270, -0.5511811023622048555, -0.09757992244046775898 ) ) ;
#56228=CARTESIAN_POINT ( 'NONE',  ( 0.02624671916010564918, -0.5023911411419708095, -0.1820866141732282451 ) ) ;
#56229=CARTESIAN_POINT ( 'NONE',  ( 0.4068241469816279987, -0.3690944881889765550, -0.3153832671262227771 ) ) ;
#56230=CARTESIAN_POINT ( 'NONE',  ( 0.5511811023622054106, -0.1870078740157480879, -0.4822834645669291653 ) ) ;
#56231=CARTESIAN_POINT ( 'NONE',  ( -0.9251968503937002541, -0.4536011799217368745, -0.2665933059059886201 ) ) ;
#56233=CARTESIAN_POINT ( 'NONE',  ( 1.515748031496063186, -0.5400638737290845981, -0.3530559997133363437 ) ) ;
#56235=CARTESIAN_POINT ( 'NONE',  ( -0.8858267716535425107, -0.5400638737290844871, 0.3530559997133364547 ) ) ;
#56237=CARTESIAN_POINT ( 'NONE',  ( 0.03937007874015806264, 0.2952755905511811885, 0.000000000000000000 ) ) ;
#56238=CARTESIAN_POINT ( 'NONE',  ( -0.7217847769028863381, -0.4281496062992124485, 0.4176697321401328655 ) ) ;
#56239=CARTESIAN_POINT ( 'NONE',  ( 1.227034120734908917, 0.1771653543307087075, -0.09757992244046823083 ) ) ;
#56240=CARTESIAN_POINT ( 'NONE',  ( 0.2821522309711292364, -0.5511811023622046335, 0.09757992244046803654 ) ) ;
#56241=CARTESIAN_POINT ( 'NONE',  ( -0.1706036745406816491, -0.4281496062992124485, 0.4176697321401328655 ) ) ;
#56242=CARTESIAN_POINT ( 'NONE',  ( -0.9973753280839886548, 0.2306618581243848609, 0.2411417322834645549 ) ) ;
#56244=FACE_OUTER_BOUND ( 'NONE', #43566, .T. ) ;
#56245=CARTESIAN_POINT ( 'NONE',  ( -0.07874015748031421014, -0.1870078740157479769, 0.4822834645669291653 ) ) ;
#56248=CARTESIAN_POINT ( 'NONE',  ( 1.266404199475066328, -0.05778040916215522460, 0.4822834645669289988 ) ) ;
#56249=CARTESIAN_POINT ( 'NONE',  ( -0.8333333333333323711, -0.5511811023622048555, -0.09757992244046775898 ) ) ;
#56250=CARTESIAN_POINT ( 'NONE',  ( -0.7086614173228339419, -0.1870078740157480879, -0.4822834645669291653 ) ) ;
#56251=CARTESIAN_POINT ( 'NONE',  ( 1.443569553805774897, -0.6046776061558809534, -0.2411417322834644161 ) ) ;
#56252=CARTESIAN_POINT ( 'NONE',  ( 1.010498687664042716, -0.4281496062992124485, 0.4176697321401328655 ) ) ;
#56253=CARTESIAN_POINT ( 'NONE',  ( -1.594488188976377119, 0.1660481256975883668, -0.3530559997133364547 ) ) ;
#56254=CARTESIAN_POINT ( 'NONE',  ( -1.036745406824146176, -0.004921259842519870586, -0.3153832671262229437 ) ) ;
#56259=CARTESIAN_POINT ( 'NONE',  ( 0.9776902887139113929, -0.5511811023622048555, -0.09757992244046775898 ) ) ;
#56260=CARTESIAN_POINT ( 'NONE',  ( 0.5971128608923890191, -0.5511811023622046335, 0.09757992244046803654 ) ) ;
#56261=CARTESIAN_POINT ( 'NONE',  ( 0.3215223097112867578, -0.05778040916215522460, 0.4822834645669289988 ) ) ;
#56264=CARTESIAN_POINT ( 'NONE',  ( 0.6758530183727039509, -0.5511811023622046335, 0.09757992244046803654 ) ) ;
#56265=CARTESIAN_POINT ( 'NONE',  ( -0.2034120734908128059, 0.2952755905511811885, 0.1292274648535926551 ) ) ;
#56266=CARTESIAN_POINT ( 'NONE',  ( -0.9120734908136475250, -0.6692913385826773087, -0.1292274648535924053 ) ) ;
#56267=CARTESIAN_POINT ( 'NONE',  ( 1.089238845144357759, 0.05413385826771626580, -0.4176697321401330321 ) ) ;
#56270=CARTESIAN_POINT ( 'NONE',  ( 0.06561679790026316017, -0.004921259842519870586, -0.3153832671262229437 ) ) ;
#56271=EDGE_LOOP ( 'NONE', ( #11894, #789, #44367, #47159 ) ) ;
#56274=CARTESIAN_POINT ( 'NONE',  ( -0.8464566929133852113, -0.5400638737290845981, -0.3530559997133363437 ) ) ;
#56275=CARTESIAN_POINT ( 'NONE',  ( -0.2755905511811015396, -0.6692913385826771977, 8.415575281601705876E-17 ) ) ;
#56276=CARTESIAN_POINT ( 'NONE',  ( -0.5380577427821514602, 0.05413385826771666132, 0.4176697321401328100 ) ) ;
#56277=CARTESIAN_POINT ( 'NONE',  ( 0.4790026246719168435, -0.3162353388693409650, -0.4822834645669289433 ) ) ;
#56278=CARTESIAN_POINT ( 'NONE',  ( -0.3477690288713902178, 0.2952755905511810774, -0.1292274648535930714 ) ) ;
#56279=CARTESIAN_POINT ( 'NONE',  ( -1.220472440944881054, -0.6692913385826771977, 8.415575281601705876E-17 ) ) ;
#56280=CARTESIAN_POINT ( 'NONE',  ( -0.9317585301837263412, 0.05413385826771666132, 0.4176697321401328100 ) ) ;
#56281=CARTESIAN_POINT ( 'NONE',  ( 0.6692913385826777528, 0.2952755905511811885, 0.000000000000000000 ) ) ;
#56283=( BOUNDED_SURFACE ( )  B_SPLINE_SURFACE ( 1, 2, ( 
 ( #55641, #23254, #67892, #35478, #74624, #67061, #81352, #36300, #60322, #74205, #42607, #73375, #15304, #35065, #61142, #9394, #80534, #22845, #3909, #48505, #60730, #16132, #4313, #29159, #3082, #2671, #28746, #28330, #48924, #22437, #54408, #10229, #53992, #35896, #79704, #16968, #80119, #73796, #48097, #29977, #3494, #40967, #22020, #66649, #8985, #41779, #64037, #63622, #70347, #43420, #75447, #30806, #6376, #31629, #43012, #12702, #62807, #25307, #81767, #82575, #63210, #24894, #50972, #32048, #37945, #38361, #57707, #5141, #11465, #37534, #5550, #68707, #70, #82987, #25724, #17785, #50157, #11882, #69117, #75036, #17382, #44244, #76669, #37123, #19002, #31214, #76266, #30392, #56471, #56882, #18601, #56057, #11048, #24077, #36706, #50563, #69933, #18195, #62380, #82174, #4718, #24490, #12289, #75853, #57289, #43828, #49746, #5959, #44651, #69532, #14388, #72032, #26147, #65310, #7215, #8065, #77934, #45497, #58981, #58125, #6790, #33726, #20264, #59804, #45073, #2158, #32463, #64455, #71194, #59388, #13536, #492, #46338, #46758, #1746, #1336, #33319, #70776, #7649, #52231, #32886, #45914, #51808, #40046, #77513, #71611, #77089, #72451, #19848, #19421, #26986, #58555, #14800, #39192, #13127, #65732, #27403, #38778, #921, #53063, #13964, #34143, #78775, #64876, #66136, #26578, #8474, #40457, #52650, #39620, #78355, #51384, #20686, #21099, #72861, #73281, #2989, #40870, #53485, #73703, #41286, #15210, #22751, #42102, #79609, #74111, #42511, #9305, #16874, #66552, #8885, #35387, #61052, #54314, #79195, #28236, #34561, #47587, #67381, #53895, #10136, #21926, #21511, #3402, #29065, #15629, #16457, #48411, #2577, #41689, #66972, #67799, #80025, #34975, #54736, #60227, #60638, #35800, #22344, #36208, #47169, #61877, #28655, #48004, #16043, #61467, #9716, #80441, #3815, #23158, #29476, #55135, #80845, #48827, #74528, #68213, #10550, #27825, #10951, #50467, #30295, #82079, #29882, #82893, #42916, #55545, #69437, #43320, #25213, #68611, #81254, #18508, #76171, #23569, #11371, #44151, #30717, #70247, #5859, #4624, #18907, #49240, #44557, #50879, #43733, #74943, #17288, #12603, #23985, #76579, #36608, #49652, #62710, #62287, #55961, #50063, #17691, #81674, #82484, #69843, #75344, #12193, #38260, #69020, #75758, #11790, #37850, #4218, #63528, #37028, #5048, #56380, #24392, #18100, #37443, #63117, #5455, #31535, #31116, #56784, #24799, #57191, #32363, #52960, #78674, #33213, #65630, #58025, #7961, #77832, #65204, #19320, #389, #20162, #7541, #44972, #46236, #26047, #70668, #58877, #59286, #20584, #13857, #45812, #83302, #71510, #64773, #19742, #32783, #13024, #26884, #6693, #58452, #6274, #1643, #38678, #31950, #39516, #45396, #27301, #64356, #57611, #78253, #52544, #25624, #71093, #71932, #7112, #46657, #33623, #51705, #20995, #51287, #72351, #14698, #1235, #76990, #77407, #63938, #13436, #39092, #811, #26474, #52124, #14281, #39945, #2886, #53790, #27718, #35282, #54624, #8782, #3295, #55035, #21816, #28548, #47892, #74006, #80742, #28959, #35692, #61357, #79501, #60124, #54204, #79921, #34037, #23056, #48309, #3711, #66446, #15523, #60535, #34455, #29374, #48724, #9612, #41997, #2475, #67692, #22237, #41589, #79092, #28134, #73600, #67279, #21411, #74421, #47064, #2054, #15942, #60944, #66871, #8371, #40761, #53385, #47480, #80335, #73173, #22650, #41181, #59699, #16353, #10027, #9201, #40354, #66033, #15105, #72756, #34874, #56683, #43221, #10851, #24290, #23469, #55444, #82384, #68919, #25108, #10449, #50781, #81153, #29782, #36512, #56279, #17589, #55857, #11269, #49136, #63018, #42817, #36928, #42405, #12091, #74840, #68103, #81976, #81567, #37747, #17184, #36105, #31014, #5355, #61776, #23885, #24701, #62605, #82787, #18410, #68511, #31429, #4117, #57091, #63422, #49962, #62188, #4525, #16768, #30195, #5759, #49550, #75245, #4946, #30616, #75659, #18000, #43634, #69337, #11687, #50370, #37345, #76068, #44053, #69745, #65833, #1851, #27931, #34673, #40561, #72966, #15317, #7757, #14076, #40149, #8166, #70146, #60336, #2268, #40982, #20374, #52758 ),
 ( #63834, #1439, #59913, #21205, #12498, #6171, #14901, #53589, #14496, #28344, #46026, #39728, #78884, #31846, #65423, #27513, #57509, #76482, #9001, #46860, #72554, #66242, #20791, #71720, #2684, #33423, #38160, #18809, #33831, #8580, #59084, #66662, #27096, #78466, #53169, #44455, #83200, #78045, #79298, #59498, #34252, #21616, #25522, #46447, #72140, #47276, #52338, #49353, #75050, #67486, #73811, #16566, #42211, #47694, #36721, #61990, #17397, #80133, #29177, #74221, #22454, #43027, #68722, #23269, #55656, #48113, #81366, #67907, #55247, #9408, #16148, #10243, #80954, #35078, #11063, #60744, #15740, #61580, #3925, #80548, #22033, #54423, #67076, #41795, #35914, #9821, #36315, #35492, #73389, #29584, #48938, #61157, #16982, #74640, #28760, #42625, #3508, #10660, #22860, #54844, #68322, #3096, #48521, #4327, #29993, #62397, #41394, #4736, #23679, #54005, #79717, #12717, #50173, #37138, #25323, #25740, #70362, #63637, #12304, #49762, #69949, #31229, #69549, #82591, #62823, #76685, #56487, #24910, #56076, #51401, #69132, #81782, #37960, #11897, #77105, #11484, #24093, #44666, #19018, #75462, #37550, #38377, #56897, #13144, #32063, #30822, #45088, #17801, #70792, #19437, #5975, #43435, #5157, #38795, #75868, #64471, #82189, #18211, #5565, #24506, #43846, #76285, #63225, #50578, #50987, #64053, #18616, #6393, #30409, #44259, #31646, #57304, #57724, #83002, #87, #33743, #13553, #32903, #52246, #53079, #58571, #59404, #40060, #46354, #47186, #14816, #1761, #27003, #66153, #7231, #72878, #27841, #51825, #65747, #34159, #39209, #15226, #26594, #58996, #64892, #72049, #14406, #78791, #8080, #936, #7664, #59820, #20703, #77951, #77530, #20280, #19865, #21116, #13979, #45929, #27418, #45514, #46776, #71210, #72467, #71627, #65327, #39636, #79211, #52665, #53503, #33335, #40475, #8492, #2175, #21527, #40886, #6808, #1352, #78371, #32479, #58141, #510, #26164, #4233, #54331, #16890, #73297, #74128, #16473, #42529, #53912, #61892, #23174, #67815, #61067, #36223, #80041, #79626, #66988, #15646, #68231, #42119, #48843, #35818, #29492, #29897, #21943, #73719, #74545, #10152, #2594, #47603, #3832, #10565, #3418, #17304, #9320, #28670, #61483, #41302, #22360, #55151, #34990, #66568, #81269, #80862, #55560, #23585, #9732, #60655, #49256, #48019, #60246, #74958, #54751, #8902, #16058, #34578, #3004, #41704, #28252, #67397, #35402, #29081, #80457, #22766, #48428, #36625, #25640, #50892, #6290, #69034, #18113, #63130, #11385, #31965, #57626, #12207, #44571, #37042, #70262, #56797, #44164, #81689, #62724, #82497, #69857, #24000, #59825, #49668, #4639, #50480, #76184, #69452, #10966, #43334, #55978, #5062, #24813, #30731, #25227, #56393, #62302, #18521, #37865, #82092, #5873, #63541, #17706, #31548, #24406, #82906, #11802, #50076, #57205, #75358, #75771, #76592, #37457, #51303, #30310, #77005, #43746, #5468, #31131, #18922, #12617, #38276, #63953, #42931, #68626, #52560, #1253, #38693, #58893, #20177, #58468, #71526, #26062, #65647, #45412, #13873, #44988, #14715, #58041, #70687, #26901, #831, #40370, #406, #13040, #33641, #7977, #64371, #26490, #59303, #45827, #2071, #21013, #19759, #34053, #6708, #59716, #66051, #78269, #32377, #51721, #27737, #39107, #8388, #77424, #64789, #77848, #71108, #13451, #65221, #32800, #7127, #14301, #1660, #52142, #27317, #53402, #39532, #7559, #20600, #52976, #19336, #78690, #33230, #46252, #71948, #39961, #46674, #72367, #15959, #55051, #79520, #36120, #16784, #40778, #54643, #23072, #28152, #4133, #15541, #47912, #53807, #35299, #60961, #42015, #3311, #21835, #79939, #48740, #9629, #66888, #66463, #73190, #8799, #67708, #2903, #9218, #48325, #34475, #28976, #60141, #61378, #34891, #54223, #47498, #68122, #41606, #42422, #2492, #35708, #80758, #74438, #10467, #10044, #61793, #41200, #60553, #28567, #29798, #3727, #47082, #79110, #22254, #29391, #73617, #80353, #22666, #21428, #67295, #72773, #15124, #74022, #16368, #25126, #68935, #42833, #55873, #4540, #57107, #31032, #37764, #24717, #18427, #76497, #68526, #62621, #63439, #82399, #74858 ) ),
 .UNSPECIFIED., .F., .F., .F. ) 
 B_SPLINE_SURFACE_WITH_KNOTS ( ( 2, 2 ),
 ( 3, 2, 2, 2, 2, 2, 2, 2, 2, 2, 2, 2, 2, 2, 2, 2, 2, 2, 2, 2, 2, 2, 2, 2, 2, 2, 2, 2, 2, 2, 2, 2, 2, 2, 2, 2, 2, 2, 2, 2, 2, 2, 2, 2, 2, 2, 2, 2, 2, 2, 2, 2, 2, 2, 2, 2, 2, 2, 2, 2, 2, 2, 2, 2, 2, 2, 2, 2, 2, 2, 2, 2, 2, 2, 2, 2, 2, 2, 2, 2, 2, 2, 2, 2, 2, 2, 2, 2, 2, 2, 2, 2, 2, 2, 2, 2, 2, 2, 2, 2, 2, 2, 2, 2, 2, 2, 2, 2, 2, 2, 2, 2, 2, 2, 2, 2, 2, 2, 2, 2, 2, 2, 2, 2, 2, 2, 2, 2, 2, 2, 2, 2, 2, 2, 2, 2, 2, 2, 2, 2, 2, 2, 2, 2, 2, 2, 2, 2, 2, 2, 2, 2, 2, 2, 2, 2, 2, 2, 2, 2, 2, 2, 2, 2, 2, 2, 2, 2, 2, 2, 2, 2, 2, 2, 2, 2, 2, 2, 2, 2, 2, 2, 2, 2, 2, 2, 2, 2, 2, 2, 2, 2, 2, 2, 2, 2, 2, 2, 2, 2, 2, 2, 2, 2, 2, 2, 2, 2, 2, 2, 2, 2, 2, 2, 2, 2, 2, 2, 2, 2, 2, 2, 2, 2, 2, 2, 2, 2, 2, 2, 2, 2, 2, 2, 2, 2, 2, 2, 2, 2, 2, 2, 2, 2, 2, 2, 2, 2, 2, 2, 2, 2, 2, 2, 2, 3 ),
 ( 0.000000000000000000, 1.000000000000000000 ),
 ( 0.000000000000000000, 0.003787878787878787984, 0.007575757575757575968, 0.01136363636363636395, 0.01515151515151515194, 0.01893939393939393992, 0.02272727272727272790, 0.02651515151515151589, 0.03030303030303030387, 0.03409090909090908839, 0.03787878787878787984, 0.04166666666666666435, 0.04545454545454545581, 0.04924242424242424032, 0.05303030303030303177, 0.05681818181818181629, 0.06060606060606060774, 0.06439393939393939226, 0.06818181818181817677, 0.07196969696969697516, 0.07575757575757575968, 0.07954545454545454419, 0.08333333333333332871, 0.08712121212121212710, 0.09090909090909091161, 0.09469696969696969613, 0.09848484848484848064, 0.1022727272727272790, 0.1060606060606060635, 0.1098484848484848481, 0.1136363636363636326, 0.1174242424242424310, 0.1212121212121212155, 0.1250000000000000000, 0.1287878787878787845, 0.1325757575757575690, 0.1363636363636363535, 0.1401515151515151381, 0.1439393939393939503, 0.1477272727272727348, 0.1515151515151515194, 0.1553030303030303039, 0.1590909090909090884, 0.1628787878787878729, 0.1666666666666666574, 0.1704545454545454419, 0.1742424242424242542, 0.1780303030303030387, 0.1818181818181818232, 0.1856060606060606077, 0.1893939393939393923, 0.1931818181818181768, 0.1969696969696969613, 0.2007575757575757458, 0.2045454545454545581, 0.2083333333333333426, 0.2121212121212121271, 0.2159090909090909116, 0.2196969696969696961, 0.2234848484848484806, 0.2272727272727272652, 0.2310606060606060497, 0.2348484848484848619, 0.2386363636363636465, 0.2424242424242424310, 0.2462121212121212155, 0.2500000000000000000, 0.2537878787878787845, 0.2575757575757575690, 0.2613636363636363535, 0.2651515151515151381, 0.2689393939393939226, 0.2727272727272727071, 0.2765151515151514916, 0.2803030303030302761, 0.2840909090909091161, 0.2878787878787879007, 0.2916666666666666852, 0.2954545454545454697, 0.2992424242424242542, 0.3030303030303030387, 0.3068181818181818232, 0.3106060606060606077, 0.3143939393939393923, 0.3181818181818181768, 0.3219696969696969613, 0.3257575757575757458, 0.3295454545454545303, 0.3333333333333333148, 0.3371212121212120993, 0.3409090909090908839, 0.3446969696969697239, 0.3484848484848485084, 0.3522727272727272929, 0.3560606060606060774, 0.3598484848484848619, 0.3636363636363636465, 0.3674242424242424310, 0.3712121212121212155, 0.3750000000000000000, 0.3787878787878787845, 0.3825757575757575690, 0.3863636363636363535, 0.3901515151515151381, 0.3939393939393939226, 0.3977272727272727071, 0.4015151515151514916, 0.4053030303030302761, 0.4090909090909091161, 0.4128787878787879007, 0.4166666666666666852, 0.4204545454545454697, 0.4242424242424242542, 0.4280303030303030387, 0.4318181818181818232, 0.4356060606060606077, 0.4393939393939393923, 0.4431818181818181768, 0.4469696969696969613, 0.4507575757575757458, 0.4545454545454545303, 0.4583333333333333148, 0.4621212121212120993, 0.4659090909090908839, 0.4696969696969697239, 0.4734848484848485084, 0.4772727272727272929, 0.4810606060606060774, 0.4848484848484848619, 0.4886363636363636465, 0.4924242424242424310, 0.4962121212121212155, 0.5000000000000000000, 0.5037878787878787845, 0.5075757575757575690, 0.5113636363636363535, 0.5151515151515151381, 0.5189393939393939226, 0.5227272727272727071, 0.5265151515151514916, 0.5303030303030302761, 0.5340909090909090606, 0.5378787878787878451, 0.5416666666666666297, 0.5454545454545454142, 0.5492424242424241987, 0.5530303030303029832, 0.5568181818181817677, 0.5606060606060605522, 0.5643939393939394478, 0.5681818181818182323, 0.5719696969696970168, 0.5757575757575758013, 0.5795454545454545858, 0.5833333333333333703, 0.5871212121212121549, 0.5909090909090909394, 0.5946969696969697239, 0.5984848484848485084, 0.6022727272727272929, 0.6060606060606060774, 0.6098484848484848619, 0.6136363636363636465, 0.6174242424242424310, 0.6212121212121212155, 0.6250000000000000000, 0.6287878787878787845, 0.6325757575757575690, 0.6363636363636363535, 0.6401515151515151381, 0.6439393939393939226, 0.6477272727272727071, 0.6515151515151514916, 0.6553030303030302761, 0.6590909090909090606, 0.6628787878787878451, 0.6666666666666666297, 0.6704545454545454142, 0.6742424242424241987, 0.6780303030303029832, 0.6818181818181817677, 0.6856060606060605522, 0.6893939393939394478, 0.6931818181818182323, 0.6969696969696970168, 0.7007575757575758013, 0.7045454545454545858, 0.7083333333333333703, 0.7121212121212121549, 0.7159090909090909394, 0.7196969696969697239, 0.7234848484848485084, 0.7272727272727272929, 0.7310606060606060774, 0.7348484848484848619, 0.7386363636363636465, 0.7424242424242424310, 0.7462121212121212155, 0.7500000000000000000, 0.7537878787878787845, 0.7575757575757575690, 0.7613636363636363535, 0.7651515151515151381, 0.7689393939393939226, 0.7727272727272727071, 0.7765151515151514916, 0.7803030303030302761, 0.7840909090909090606, 0.7878787878787878451, 0.7916666666666666297, 0.7954545454545454142, 0.7992424242424241987, 0.8030303030303029832, 0.8068181818181817677, 0.8106060606060605522, 0.8143939393939394478, 0.8181818181818182323, 0.8219696969696970168, 0.8257575757575758013, 0.8295454545454545858, 0.8333333333333333703, 0.8371212121212121549, 0.8409090909090909394, 0.8446969696969697239, 0.8484848484848485084, 0.8522727272727272929, 0.8560606060606060774, 0.8598484848484848619, 0.8636363636363636465, 0.8674242424242424310, 0.8712121212121212155, 0.8750000000000000000, 0.8787878787878787845, 0.8825757575757575690, 0.8863636363636363535, 0.8901515151515151381, 0.8939393939393939226, 0.8977272727272727071, 0.9015151515151514916, 0.9053030303030302761, 0.9090909090909090606, 0.9128787878787878451, 0.9166666666666666297, 0.9204545454545454142, 0.9242424242424241987, 0.9280303030303029832, 0.9318181818181817677, 0.9356060606060605522, 0.9393939393939394478, 0.9431818181818182323, 0.9469696969696970168, 0.9507575757575758013, 0.9545454545454545858, 0.9583333333333333703, 0.9621212121212121549, 0.9659090909090909394 ),
 .UNSPECIFIED. ) 
 GEOMETRIC_REPRESENTATION_ITEM ( )  RATIONAL_B_SPLINE_SURFACE ( (
 ( 1.000000000000000000, 0.9659258262890683122, 1.000000000000000000, 0.9659258262890683122, 1.000000000000000000, 0.9659258262890683122, 1.000000000000000000, 0.9659258262890683122, 1.000000000000000000, 0.9659258262890683122, 1.000000000000000000, 0.9659258262890683122, 1.000000000000000000, 0.9659258262890683122, 1.000000000000000000, 0.9659258262890683122, 1.000000000000000000, 0.9659258262890683122, 1.000000000000000000, 0.9659258262890683122, 1.000000000000000000, 0.9659258262890683122, 1.000000000000000000, 0.9659258262890683122, 1.000000000000000000, 0.9659258262890683122, 1.000000000000000000, 0.9659258262890683122, 1.000000000000000000, 0.9659258262890683122, 1.000000000000000000, 0.9659258262890683122, 1.000000000000000000, 0.9659258262890683122, 1.000000000000000000, 0.9659258262890683122, 1.000000000000000000, 0.9659258262890683122, 1.000000000000000000, 0.9659258262890683122, 1.000000000000000000, 0.9659258262890683122, 1.000000000000000000, 0.9659258262890683122, 1.000000000000000000, 0.9659258262890683122, 1.000000000000000000, 0.9659258262890683122, 1.000000000000000000, 0.9659258262890683122, 1.000000000000000000, 0.9659258262890683122, 1.000000000000000000, 0.9659258262890683122, 1.000000000000000000, 0.9659258262890683122, 1.000000000000000000, 0.9659258262890683122, 1.000000000000000000, 0.9659258262890683122, 1.000000000000000000, 0.9659258262890683122, 1.000000000000000000, 0.9659258262890683122, 1.000000000000000000, 0.9659258262890683122, 1.000000000000000000, 0.9659258262890683122, 1.000000000000000000, 0.9659258262890683122, 1.000000000000000000, 0.9659258262890683122, 1.000000000000000000, 0.9659258262890683122, 1.000000000000000000, 0.9659258262890683122, 1.000000000000000000, 0.9659258262890683122, 1.000000000000000000, 0.9659258262890683122, 1.000000000000000000, 0.9659258262890683122, 1.000000000000000000, 0.9659258262890683122, 1.000000000000000000, 0.9659258262890683122, 1.000000000000000000, 0.9659258262890683122, 1.000000000000000000, 0.9659258262890683122, 1.000000000000000000, 0.9659258262890683122, 1.000000000000000000, 0.9659258262890683122, 1.000000000000000000, 0.9659258262890683122, 1.000000000000000000, 0.9659258262890683122, 1.000000000000000000, 0.9659258262890683122, 1.000000000000000000, 0.9659258262890683122, 1.000000000000000000, 0.9659258262890683122, 1.000000000000000000, 0.9659258262890683122, 1.000000000000000000, 0.9659258262890683122, 1.000000000000000000, 0.9659258262890683122, 1.000000000000000000, 0.9659258262890683122, 1.000000000000000000, 0.9659258262890683122, 1.000000000000000000, 0.9659258262890683122, 1.000000000000000000, 0.9659258262890683122, 1.000000000000000000, 0.9659258262890683122, 1.000000000000000000, 0.9659258262890683122, 1.000000000000000000, 0.9659258262890683122, 1.000000000000000000, 0.9659258262890683122, 1.000000000000000000, 0.9659258262890683122, 1.000000000000000000, 0.9659258262890683122, 1.000000000000000000, 0.9659258262890683122, 1.000000000000000000, 0.9659258262890683122, 1.000000000000000000, 0.9659258262890683122, 1.000000000000000000, 0.9659258262890683122, 1.000000000000000000, 0.9659258262890683122, 1.000000000000000000, 0.9659258262890683122, 1.000000000000000000, 0.9659258262890683122, 1.000000000000000000, 0.9659258262890683122, 1.000000000000000000, 0.9659258262890683122, 1.000000000000000000, 0.9659258262890683122, 1.000000000000000000, 0.9659258262890683122, 1.000000000000000000, 0.9659258262890683122, 1.000000000000000000, 0.9659258262890683122, 1.000000000000000000, 0.9659258262890683122, 1.000000000000000000, 0.9659258262890683122, 1.000000000000000000, 0.9659258262890683122, 1.000000000000000000, 0.9659258262890683122, 1.000000000000000000, 0.9659258262890683122, 1.000000000000000000, 0.9659258262890683122, 1.000000000000000000, 0.9659258262890683122, 1.000000000000000000, 0.9659258262890683122, 1.000000000000000000, 0.9659258262890683122, 1.000000000000000000, 0.9659258262890683122, 1.000000000000000000, 0.9659258262890683122, 1.000000000000000000, 0.9659258262890683122, 1.000000000000000000, 0.9659258262890683122, 1.000000000000000000, 0.9659258262890683122, 1.000000000000000000, 0.9659258262890683122, 1.000000000000000000, 0.9659258262890683122, 1.000000000000000000, 0.9659258262890683122, 1.000000000000000000, 0.9659258262890683122, 1.000000000000000000, 0.9659258262890683122, 1.000000000000000000, 0.9659258262890683122, 1.000000000000000000, 0.9659258262890683122, 1.000000000000000000, 0.9659258262890683122, 1.000000000000000000, 0.9659258262890683122, 1.000000000000000000, 0.9659258262890683122, 1.000000000000000000, 0.9659258262890683122, 1.000000000000000000, 0.9659258262890683122, 1.000000000000000000, 0.9659258262890683122, 1.000000000000000000, 0.9659258262890683122, 1.000000000000000000, 0.9659258262890683122, 1.000000000000000000, 0.9659258262890683122, 1.000000000000000000, 0.9659258262890683122, 1.000000000000000000, 0.9659258262890683122, 1.000000000000000000, 0.9659258262890683122, 1.000000000000000000, 0.9659258262890683122, 1.000000000000000000, 0.9659258262890683122, 1.000000000000000000, 0.9659258262890683122, 1.000000000000000000, 0.9659258262890683122, 1.000000000000000000, 0.9659258262890683122, 1.000000000000000000, 0.9659258262890683122, 1.000000000000000000, 0.9659258262890683122, 1.000000000000000000, 0.9659258262890683122, 1.000000000000000000, 0.9659258262890683122, 1.000000000000000000, 0.9659258262890683122, 1.000000000000000000, 0.9659258262890683122, 1.000000000000000000, 0.9659258262890683122, 1.000000000000000000, 0.9659258262890683122, 1.000000000000000000, 0.9659258262890683122, 1.000000000000000000, 0.9659258262890683122, 1.000000000000000000, 0.9659258262890683122, 1.000000000000000000, 0.9659258262890683122, 1.000000000000000000, 0.9659258262890683122, 1.000000000000000000, 0.9659258262890683122, 1.000000000000000000, 0.9659258262890683122, 1.000000000000000000, 0.9659258262890683122, 1.000000000000000000, 0.9659258262890683122, 1.000000000000000000, 0.9659258262890683122, 1.000000000000000000, 0.9659258262890683122, 1.000000000000000000, 0.9659258262890683122, 1.000000000000000000, 0.9659258262890683122, 1.000000000000000000, 0.9659258262890683122, 1.000000000000000000, 0.9659258262890683122, 1.000000000000000000, 0.9659258262890683122, 1.000000000000000000, 0.9659258262890683122, 1.000000000000000000, 0.9659258262890683122, 1.000000000000000000, 0.9659258262890683122, 1.000000000000000000, 0.9659258262890683122, 1.000000000000000000, 0.9659258262890683122, 1.000000000000000000, 0.9659258262890683122, 1.000000000000000000, 0.9659258262890683122, 1.000000000000000000, 0.9659258262890683122, 1.000000000000000000, 0.9659258262890683122, 1.000000000000000000, 0.9659258262890683122, 1.000000000000000000, 0.9659258262890683122, 1.000000000000000000, 0.9659258262890683122, 1.000000000000000000, 0.9659258262890683122, 1.000000000000000000, 0.9659258262890683122, 1.000000000000000000, 0.9659258262890683122, 1.000000000000000000, 0.9659258262890683122, 1.000000000000000000, 0.9659258262890683122, 1.000000000000000000, 0.9659258262890683122, 1.000000000000000000, 0.9659258262890683122, 1.000000000000000000, 0.9659258262890683122, 1.000000000000000000, 0.9659258262890683122, 1.000000000000000000, 0.9659258262890683122, 1.000000000000000000, 0.9659258262890683122, 1.000000000000000000, 0.9659258262890683122, 1.000000000000000000, 0.9659258262890683122, 1.000000000000000000, 0.9659258262890683122, 1.000000000000000000, 0.9659258262890683122, 1.000000000000000000, 0.9659258262890683122, 1.000000000000000000, 0.9659258262890683122, 1.000000000000000000, 0.9659258262890683122, 1.000000000000000000, 0.9659258262890683122, 1.000000000000000000, 0.9659258262890683122, 1.000000000000000000, 0.9659258262890683122, 1.000000000000000000, 0.9659258262890683122, 1.000000000000000000, 0.9659258262890683122, 1.000000000000000000, 0.9659258262890683122, 1.000000000000000000, 0.9659258262890683122, 1.000000000000000000, 0.9659258262890683122, 1.000000000000000000, 0.9659258262890683122, 1.000000000000000000, 0.9659258262890683122, 1.000000000000000000, 0.9659258262890683122, 1.000000000000000000, 0.9659258262890683122, 1.000000000000000000, 0.9659258262890683122, 1.000000000000000000, 0.9659258262890683122, 1.000000000000000000, 0.9659258262890683122, 1.000000000000000000, 0.9659258262890683122, 1.000000000000000000, 0.9659258262890683122, 1.000000000000000000, 0.9659258262890683122, 1.000000000000000000, 0.9659258262890683122, 1.000000000000000000, 0.9659258262890683122, 1.000000000000000000, 0.9659258262890683122, 1.000000000000000000, 0.9659258262890683122, 1.000000000000000000, 0.9659258262890683122, 1.000000000000000000, 0.9659258262890683122, 1.000000000000000000, 0.9659258262890683122, 1.000000000000000000, 0.9659258262890683122, 1.000000000000000000, 0.9659258262890683122, 1.000000000000000000, 0.9659258262890683122, 1.000000000000000000, 0.9659258262890683122, 1.000000000000000000, 0.9659258262890683122, 1.000000000000000000, 0.9659258262890683122, 1.000000000000000000, 0.9659258262890683122, 1.000000000000000000, 0.9659258262890683122, 1.000000000000000000, 0.9659258262890683122, 1.000000000000000000, 0.9659258262890683122, 1.000000000000000000, 0.9659258262890683122, 1.000000000000000000, 0.9659258262890683122, 1.000000000000000000, 0.9659258262890683122, 1.000000000000000000, 0.9659258262890683122, 1.000000000000000000, 0.9659258262890683122, 1.000000000000000000, 0.9659258262890683122, 1.000000000000000000, 0.9659258262890683122, 1.000000000000000000, 0.9659258262890683122, 1.000000000000000000, 0.9659258262890683122, 1.000000000000000000, 0.9659258262890683122, 1.000000000000000000, 0.9659258262890683122, 1.000000000000000000, 0.9659258262890683122, 1.000000000000000000, 0.9659258262890683122, 1.000000000000000000, 0.9659258262890683122, 1.000000000000000000, 0.9659258262890683122, 1.000000000000000000, 0.9659258262890683122, 1.000000000000000000, 0.9659258262890683122, 1.000000000000000000, 0.9659258262890683122, 1.000000000000000000, 0.9659258262890683122, 1.000000000000000000, 0.9659258262890683122, 1.000000000000000000, 0.9659258262890683122, 1.000000000000000000, 0.9659258262890683122, 1.000000000000000000, 0.9659258262890683122, 1.000000000000000000, 0.9659258262890683122, 1.000000000000000000, 0.9659258262890683122, 1.000000000000000000, 0.9659258262890683122, 1.000000000000000000, 0.9659258262890683122, 1.000000000000000000, 0.9659258262890683122, 1.000000000000000000, 0.9659258262890683122, 1.000000000000000000, 0.9659258262890683122, 1.000000000000000000, 0.9659258262890683122, 1.000000000000000000, 0.9659258262890683122, 1.000000000000000000, 0.9659258262890683122, 1.000000000000000000, 0.9659258262890683122, 1.000000000000000000, 0.9659258262890683122, 1.000000000000000000, 0.9659258262890683122, 1.000000000000000000, 0.9659258262890683122, 1.000000000000000000, 0.9659258262890683122, 1.000000000000000000, 0.9659258262890683122, 1.000000000000000000, 0.9659258262890683122, 1.000000000000000000, 0.9659258262890683122, 1.000000000000000000, 0.9659258262890683122, 1.000000000000000000, 0.9659258262890683122, 1.000000000000000000, 0.9659258262890683122, 1.000000000000000000, 0.9659258262890683122, 1.000000000000000000, 0.9659258262890683122, 1.000000000000000000, 0.9659258262890683122, 1.000000000000000000, 0.9659258262890683122, 1.000000000000000000, 0.9659258262890683122, 1.000000000000000000, 0.9659258262890683122, 1.000000000000000000),
 ( 1.000000000000000000, 0.9659258262890683122, 1.000000000000000000, 0.9659258262890683122, 1.000000000000000000, 0.9659258262890683122, 1.000000000000000000, 0.9659258262890683122, 1.000000000000000000, 0.9659258262890683122, 1.000000000000000000, 0.9659258262890683122, 1.000000000000000000, 0.9659258262890683122, 1.000000000000000000, 0.9659258262890683122, 1.000000000000000000, 0.9659258262890683122, 1.000000000000000000, 0.9659258262890683122, 1.000000000000000000, 0.9659258262890683122, 1.000000000000000000, 0.9659258262890683122, 1.000000000000000000, 0.9659258262890683122, 1.000000000000000000, 0.9659258262890683122, 1.000000000000000000, 0.9659258262890683122, 1.000000000000000000, 0.9659258262890683122, 1.000000000000000000, 0.9659258262890683122, 1.000000000000000000, 0.9659258262890683122, 1.000000000000000000, 0.9659258262890683122, 1.000000000000000000, 0.9659258262890683122, 1.000000000000000000, 0.9659258262890683122, 1.000000000000000000, 0.9659258262890683122, 1.000000000000000000, 0.9659258262890683122, 1.000000000000000000, 0.9659258262890683122, 1.000000000000000000, 0.9659258262890683122, 1.000000000000000000, 0.9659258262890683122, 1.000000000000000000, 0.9659258262890683122, 1.000000000000000000, 0.9659258262890683122, 1.000000000000000000, 0.9659258262890683122, 1.000000000000000000, 0.9659258262890683122, 1.000000000000000000, 0.9659258262890683122, 1.000000000000000000, 0.9659258262890683122, 1.000000000000000000, 0.9659258262890683122, 1.000000000000000000, 0.9659258262890683122, 1.000000000000000000, 0.9659258262890683122, 1.000000000000000000, 0.9659258262890683122, 1.000000000000000000, 0.9659258262890683122, 1.000000000000000000, 0.9659258262890683122, 1.000000000000000000, 0.9659258262890683122, 1.000000000000000000, 0.9659258262890683122, 1.000000000000000000, 0.9659258262890683122, 1.000000000000000000, 0.9659258262890683122, 1.000000000000000000, 0.9659258262890683122, 1.000000000000000000, 0.9659258262890683122, 1.000000000000000000, 0.9659258262890683122, 1.000000000000000000, 0.9659258262890683122, 1.000000000000000000, 0.9659258262890683122, 1.000000000000000000, 0.9659258262890683122, 1.000000000000000000, 0.9659258262890683122, 1.000000000000000000, 0.9659258262890683122, 1.000000000000000000, 0.9659258262890683122, 1.000000000000000000, 0.9659258262890683122, 1.000000000000000000, 0.9659258262890683122, 1.000000000000000000, 0.9659258262890683122, 1.000000000000000000, 0.9659258262890683122, 1.000000000000000000, 0.9659258262890683122, 1.000000000000000000, 0.9659258262890683122, 1.000000000000000000, 0.9659258262890683122, 1.000000000000000000, 0.9659258262890683122, 1.000000000000000000, 0.9659258262890683122, 1.000000000000000000, 0.9659258262890683122, 1.000000000000000000, 0.9659258262890683122, 1.000000000000000000, 0.9659258262890683122, 1.000000000000000000, 0.9659258262890683122, 1.000000000000000000, 0.9659258262890683122, 1.000000000000000000, 0.9659258262890683122, 1.000000000000000000, 0.9659258262890683122, 1.000000000000000000, 0.9659258262890683122, 1.000000000000000000, 0.9659258262890683122, 1.000000000000000000, 0.9659258262890683122, 1.000000000000000000, 0.9659258262890683122, 1.000000000000000000, 0.9659258262890683122, 1.000000000000000000, 0.9659258262890683122, 1.000000000000000000, 0.9659258262890683122, 1.000000000000000000, 0.9659258262890683122, 1.000000000000000000, 0.9659258262890683122, 1.000000000000000000, 0.9659258262890683122, 1.000000000000000000, 0.9659258262890683122, 1.000000000000000000, 0.9659258262890683122, 1.000000000000000000, 0.9659258262890683122, 1.000000000000000000, 0.9659258262890683122, 1.000000000000000000, 0.9659258262890683122, 1.000000000000000000, 0.9659258262890683122, 1.000000000000000000, 0.9659258262890683122, 1.000000000000000000, 0.9659258262890683122, 1.000000000000000000, 0.9659258262890683122, 1.000000000000000000, 0.9659258262890683122, 1.000000000000000000, 0.9659258262890683122, 1.000000000000000000, 0.9659258262890683122, 1.000000000000000000, 0.9659258262890683122, 1.000000000000000000, 0.9659258262890683122, 1.000000000000000000, 0.9659258262890683122, 1.000000000000000000, 0.9659258262890683122, 1.000000000000000000, 0.9659258262890683122, 1.000000000000000000, 0.9659258262890683122, 1.000000000000000000, 0.9659258262890683122, 1.000000000000000000, 0.9659258262890683122, 1.000000000000000000, 0.9659258262890683122, 1.000000000000000000, 0.9659258262890683122, 1.000000000000000000, 0.9659258262890683122, 1.000000000000000000, 0.9659258262890683122, 1.000000000000000000, 0.9659258262890683122, 1.000000000000000000, 0.9659258262890683122, 1.000000000000000000, 0.9659258262890683122, 1.000000000000000000, 0.9659258262890683122, 1.000000000000000000, 0.9659258262890683122, 1.000000000000000000, 0.9659258262890683122, 1.000000000000000000, 0.9659258262890683122, 1.000000000000000000, 0.9659258262890683122, 1.000000000000000000, 0.9659258262890683122, 1.000000000000000000, 0.9659258262890683122, 1.000000000000000000, 0.9659258262890683122, 1.000000000000000000, 0.9659258262890683122, 1.000000000000000000, 0.9659258262890683122, 1.000000000000000000, 0.9659258262890683122, 1.000000000000000000, 0.9659258262890683122, 1.000000000000000000, 0.9659258262890683122, 1.000000000000000000, 0.9659258262890683122, 1.000000000000000000, 0.9659258262890683122, 1.000000000000000000, 0.9659258262890683122, 1.000000000000000000, 0.9659258262890683122, 1.000000000000000000, 0.9659258262890683122, 1.000000000000000000, 0.9659258262890683122, 1.000000000000000000, 0.9659258262890683122, 1.000000000000000000, 0.9659258262890683122, 1.000000000000000000, 0.9659258262890683122, 1.000000000000000000, 0.9659258262890683122, 1.000000000000000000, 0.9659258262890683122, 1.000000000000000000, 0.9659258262890683122, 1.000000000000000000, 0.9659258262890683122, 1.000000000000000000, 0.9659258262890683122, 1.000000000000000000, 0.9659258262890683122, 1.000000000000000000, 0.9659258262890683122, 1.000000000000000000, 0.9659258262890683122, 1.000000000000000000, 0.9659258262890683122, 1.000000000000000000, 0.9659258262890683122, 1.000000000000000000, 0.9659258262890683122, 1.000000000000000000, 0.9659258262890683122, 1.000000000000000000, 0.9659258262890683122, 1.000000000000000000, 0.9659258262890683122, 1.000000000000000000, 0.9659258262890683122, 1.000000000000000000, 0.9659258262890683122, 1.000000000000000000, 0.9659258262890683122, 1.000000000000000000, 0.9659258262890683122, 1.000000000000000000, 0.9659258262890683122, 1.000000000000000000, 0.9659258262890683122, 1.000000000000000000, 0.9659258262890683122, 1.000000000000000000, 0.9659258262890683122, 1.000000000000000000, 0.9659258262890683122, 1.000000000000000000, 0.9659258262890683122, 1.000000000000000000, 0.9659258262890683122, 1.000000000000000000, 0.9659258262890683122, 1.000000000000000000, 0.9659258262890683122, 1.000000000000000000, 0.9659258262890683122, 1.000000000000000000, 0.9659258262890683122, 1.000000000000000000, 0.9659258262890683122, 1.000000000000000000, 0.9659258262890683122, 1.000000000000000000, 0.9659258262890683122, 1.000000000000000000, 0.9659258262890683122, 1.000000000000000000, 0.9659258262890683122, 1.000000000000000000, 0.9659258262890683122, 1.000000000000000000, 0.9659258262890683122, 1.000000000000000000, 0.9659258262890683122, 1.000000000000000000, 0.9659258262890683122, 1.000000000000000000, 0.9659258262890683122, 1.000000000000000000, 0.9659258262890683122, 1.000000000000000000, 0.9659258262890683122, 1.000000000000000000, 0.9659258262890683122, 1.000000000000000000, 0.9659258262890683122, 1.000000000000000000, 0.9659258262890683122, 1.000000000000000000, 0.9659258262890683122, 1.000000000000000000, 0.9659258262890683122, 1.000000000000000000, 0.9659258262890683122, 1.000000000000000000, 0.9659258262890683122, 1.000000000000000000, 0.9659258262890683122, 1.000000000000000000, 0.9659258262890683122, 1.000000000000000000, 0.9659258262890683122, 1.000000000000000000, 0.9659258262890683122, 1.000000000000000000, 0.9659258262890683122, 1.000000000000000000, 0.9659258262890683122, 1.000000000000000000, 0.9659258262890683122, 1.000000000000000000, 0.9659258262890683122, 1.000000000000000000, 0.9659258262890683122, 1.000000000000000000, 0.9659258262890683122, 1.000000000000000000, 0.9659258262890683122, 1.000000000000000000, 0.9659258262890683122, 1.000000000000000000, 0.9659258262890683122, 1.000000000000000000, 0.9659258262890683122, 1.000000000000000000, 0.9659258262890683122, 1.000000000000000000, 0.9659258262890683122, 1.000000000000000000, 0.9659258262890683122, 1.000000000000000000, 0.9659258262890683122, 1.000000000000000000, 0.9659258262890683122, 1.000000000000000000, 0.9659258262890683122, 1.000000000000000000, 0.9659258262890683122, 1.000000000000000000, 0.9659258262890683122, 1.000000000000000000, 0.9659258262890683122, 1.000000000000000000, 0.9659258262890683122, 1.000000000000000000, 0.9659258262890683122, 1.000000000000000000, 0.9659258262890683122, 1.000000000000000000, 0.9659258262890683122, 1.000000000000000000, 0.9659258262890683122, 1.000000000000000000, 0.9659258262890683122, 1.000000000000000000, 0.9659258262890683122, 1.000000000000000000, 0.9659258262890683122, 1.000000000000000000, 0.9659258262890683122, 1.000000000000000000, 0.9659258262890683122, 1.000000000000000000, 0.9659258262890683122, 1.000000000000000000, 0.9659258262890683122, 1.000000000000000000, 0.9659258262890683122, 1.000000000000000000, 0.9659258262890683122, 1.000000000000000000, 0.9659258262890683122, 1.000000000000000000, 0.9659258262890683122, 1.000000000000000000, 0.9659258262890683122, 1.000000000000000000, 0.9659258262890683122, 1.000000000000000000, 0.9659258262890683122, 1.000000000000000000, 0.9659258262890683122, 1.000000000000000000, 0.9659258262890683122, 1.000000000000000000, 0.9659258262890683122, 1.000000000000000000, 0.9659258262890683122, 1.000000000000000000, 0.9659258262890683122, 1.000000000000000000, 0.9659258262890683122, 1.000000000000000000, 0.9659258262890683122, 1.000000000000000000, 0.9659258262890683122, 1.000000000000000000, 0.9659258262890683122, 1.000000000000000000, 0.9659258262890683122, 1.000000000000000000, 0.9659258262890683122, 1.000000000000000000, 0.9659258262890683122, 1.000000000000000000, 0.9659258262890683122, 1.000000000000000000, 0.9659258262890683122, 1.000000000000000000, 0.9659258262890683122, 1.000000000000000000, 0.9659258262890683122, 1.000000000000000000, 0.9659258262890683122, 1.000000000000000000, 0.9659258262890683122, 1.000000000000000000, 0.9659258262890683122, 1.000000000000000000, 0.9659258262890683122, 1.000000000000000000, 0.9659258262890683122, 1.000000000000000000, 0.9659258262890683122, 1.000000000000000000, 0.9659258262890683122, 1.000000000000000000, 0.9659258262890683122, 1.000000000000000000, 0.9659258262890683122, 1.000000000000000000, 0.9659258262890683122, 1.000000000000000000, 0.9659258262890683122, 1.000000000000000000, 0.9659258262890683122, 1.000000000000000000, 0.9659258262890683122, 1.000000000000000000, 0.9659258262890683122, 1.000000000000000000, 0.9659258262890683122, 1.000000000000000000, 0.9659258262890683122, 1.000000000000000000, 0.9659258262890683122, 1.000000000000000000, 0.9659258262890683122, 1.000000000000000000, 0.9659258262890683122, 1.000000000000000000, 0.9659258262890683122, 1.000000000000000000, 0.9659258262890683122, 1.000000000000000000, 0.9659258262890683122, 1.000000000000000000, 0.9659258262890683122, 1.000000000000000000) ) ) 
 REPRESENTATION_ITEM ( '' )  SURFACE ( )  );
#56285=CARTESIAN_POINT ( 'NONE',  ( -0.5774278215223089816, -0.5023911411419708095, 0.1820866141732285504 ) ) ;
#56286=ORIENTED_EDGE ( 'NONE', *, *, #27922, .F. ) ;
#56289=CARTESIAN_POINT ( 'NONE',  ( -1.489501312335957062, -0.2845877964562161244, -0.3641732283464567121 ) ) ;
#56290=CARTESIAN_POINT ( 'NONE',  ( -1.095800524934382292, -0.3162353388693409650, -0.4822834645669289433 ) ) ;
#56291=CARTESIAN_POINT ( 'NONE',  ( -0.8202099737532799750, 0.2952755905511810774, -0.1292274648535930714 ) ) ;
#56293=CARTESIAN_POINT ( 'NONE',  ( -0.6824146981627291497, -0.6046776061558809534, -0.2411417322834644161 ) ) ;
#56294=CARTESIAN_POINT ( 'NONE',  ( -0.8070866141732276899, -0.5400638737290844871, 0.3530559997133364547 ) ) ;
#56297=CARTESIAN_POINT ( 'NONE',  ( 0.5380577427821529035, -0.3690944881889763329, 0.3153832671262228327 ) ) ;
#56300=CARTESIAN_POINT ( 'NONE',  ( 0.2099737532808405305, 0.1283753931104746893, -0.1820866141732285504 ) ) ;
#56301=CARTESIAN_POINT ( 'NONE',  ( -0.3346456692913377662, 0.1660481256975883668, -0.3530559997133364547 ) ) ;
#56302=CARTESIAN_POINT ( 'NONE',  ( 1.574803149606299746, -0.1870078740157479769, 0.4822834645669291653 ) ) ;
#56303=CARTESIAN_POINT ( 'NONE',  ( -0.1640419947506553400, -0.05778040916215560624, -0.4822834645669293319 ) ) ;
#56306=CARTESIAN_POINT ( 'NONE',  ( 0.2481535038101765900, 6.903518153045088239E-16, 0.3627989612356144478 ) ) ;
#56307=ORIENTED_EDGE ( 'NONE', *, *, #51203, .T. ) ;
#56310=CARTESIAN_POINT ( 'NONE',  ( -1.246719160104986512, -0.004921259842519576551, 0.3153832671262227771 ) ) ;
#56311=CARTESIAN_POINT ( 'NONE',  ( -1.062992125984250968, 0.2952755905511811885, 0.000000000000000000 ) ) ;
#56313=CARTESIAN_POINT ( 'NONE',  ( -1.614173228346456712, 2.401574803149606474, 0.1372047244094477536 ) ) ;
#56315=CARTESIAN_POINT ( 'NONE',  ( 1.364829396325460076, 0.2306618581243848609, 0.2411417322834645549 ) ) ;
#56316=CARTESIAN_POINT ( 'NONE',  ( 0.5643044619422579178, -0.4281496062992127816, -0.4176697321401328100 ) ) ;
#56317=CARTESIAN_POINT ( 'NONE',  ( 0.3608923884514443348, -0.6692913385826771977, 0.1292274648535927661 ) ) ;
#56318=CARTESIAN_POINT ( 'NONE',  ( -1.128608923884513837, 0.1283753931104746893, -0.1820866141732285504 ) ) ;
#56319=CARTESIAN_POINT ( 'NONE',  ( -0.5380577427821514602, -0.4281496062992127816, -0.4176697321401328100 ) ) ;
#56321=CARTESIAN_POINT ( 'NONE',  ( -0.8005249343832013809, -0.4281496062992124485, 0.4176697321401328655 ) ) ;
#56323=CARTESIAN_POINT ( 'NONE',  ( 1.476377952755906220, 0.07958543189024071263, -0.2665933059059888421 ) ) ;
#56324=CARTESIAN_POINT ( 'NONE',  ( -0.5183727034120726440, -0.5511811023622048555, -0.09757992244046775898 ) ) ;
#56325=CARTESIAN_POINT ( 'NONE',  ( 1.377952755905512472, 0.1771653543307087630, 0.000000000000000000 ) ) ;
#56326=CARTESIAN_POINT ( 'NONE',  ( -1.450131233595799651, -0.6692913385826771977, 0.1292274648535927661 ) ) ;
#56327=CARTESIAN_POINT ( 'NONE',  ( -0.9842519685039360366, 0.1771653543307087630, 0.000000000000000000 ) ) ;
#56329=CARTESIAN_POINT ( 'NONE',  ( 0.5839895013123367340, 0.1771653543307087630, 0.09757992244046791164 ) ) ;
#56330=CARTESIAN_POINT ( 'NONE',  ( -0.3477690288713902178, 0.2952755905511810774, -0.1292274648535930714 ) ) ;
#56332=CARTESIAN_POINT ( 'NONE',  ( 0.1049868766404206816, 0.1283753931104748280, 0.1820866141732283561 ) ) ;
#56334=CARTESIAN_POINT ( 'NONE',  ( 0.6430446194225729606, -0.4281496062992127816, -0.4176697321401328100 ) ) ;
#56336=CARTESIAN_POINT ( 'NONE',  ( 1.476377952755906220, 0.07958543189024071263, -0.2665933059059888421 ) ) ;
#56337=CARTESIAN_POINT ( 'NONE',  ( -1.141732283464566011, -0.6692913385826771977, 8.415575281601705876E-17 ) ) ;
#56338=CARTESIAN_POINT ( 'NONE',  ( -0.2559055118110227234, -0.4536011799217367080, 0.2665933059059888421 ) ) ;
#56339=DIRECTION ( 'NONE',  ( 3.096699300667737957E-16, -1.000000000000000000, 0.000000000000000000 ) ) ;
#56340=CARTESIAN_POINT ( 'NONE',  ( 0.1968503937007881344, 0.1771653543307087630, 0.000000000000000000 ) ) ;
#56341=CARTESIAN_POINT ( 'NONE',  ( -1.345144356955379816, -0.05778040916215560624, -0.4822834645669293319 ) ) ;
#56342=CARTESIAN_POINT ( 'NONE',  ( -0.3215223097112853146, -0.05778040916215560624, -0.4822834645669293319 ) ) ;
#56345=CARTESIAN_POINT ( 'NONE',  ( 0.4396325459317590445, -0.5511811023622046335, 0.09757992244046803654 ) ) ;
#56346=CARTESIAN_POINT ( 'NONE',  ( -0.5314960629921250401, 0.1660481256975885056, 0.3530559997133364547 ) ) ;
#56347=CARTESIAN_POINT ( 'NONE',  ( -0.5971128608923877978, -0.6692913385826773087, -0.1292274648535924053 ) ) ;
#56348=CARTESIAN_POINT ( 'NONE',  ( -0.6627296587926501115, 0.1771653543307087075, -0.09757992244046823083 ) ) ;
#56350=CARTESIAN_POINT ( 'NONE',  ( 0.1509186351706045259, -0.05778040916215560624, -0.4822834645669293319 ) ) ;
#56353=CARTESIAN_POINT ( 'NONE',  ( -1.135170603674539924, -0.5511811023622046335, 0.09757992244046803654 ) ) ;
#56354=CARTESIAN_POINT ( 'NONE',  ( -1.627296587926508442, 0.2306618581243848609, 0.2411417322834645549 ) ) ;
#56355=CARTESIAN_POINT ( 'NONE',  ( 0.4606732211678801203, 1.929133858267716439, -0.5309055118110237448 ) ) ;
#56358=CARTESIAN_POINT ( 'NONE',  ( -1.456692913385826182, -0.5511811023622047445, 6.969142054262312111E-17 ) ) ;
#56359=CARTESIAN_POINT ( 'NONE',  ( -1.213910761154854745, 0.2952755905511810774, -0.1292274648535930714 ) ) ;
#56360=CARTESIAN_POINT ( 'NONE',  ( -1.003937007874015297, -0.5400638737290845981, -0.3530559997133363437 ) ) ;
#56361=CARTESIAN_POINT ( 'NONE',  ( -1.601049868766403650, 0.2306618581243847221, -0.2411417322834647770 ) ) ;
#56364=CARTESIAN_POINT ( 'NONE',  ( 1.003937007874016407, -0.5400638737290844871, 0.3530559997133364547 ) ) ;
#56365=CARTESIAN_POINT ( 'NONE',  ( 0.4724409448818904789, -0.1870078740157480879, -0.4822834645669291653 ) ) ;
#56368=CARTESIAN_POINT ( 'NONE',  ( 1.266404199475066328, -0.08942795157527998196, 0.3641732283464567121 ) ) ;
#56371=CARTESIAN_POINT ( 'NONE',  ( -0.9186351706036736120, -0.5023911411419708095, -0.1820866141732282451 ) ) ;
#56374=CARTESIAN_POINT ( 'NONE',  ( 0.5314960629921264834, 0.1660481256975883668, -0.3530559997133364547 ) ) ;
#56375=CARTESIAN_POINT ( 'NONE',  ( -0.6167979002624665030, 0.05413385826771666132, 0.4176697321401328100 ) ) ;
#56376=CARTESIAN_POINT ( 'NONE',  ( -1.023622047244093558, -0.1870078740157479769, 0.4822834645669291653 ) ) ;
#56377=CARTESIAN_POINT ( 'NONE',  ( 1.128608923884515169, -0.6046776061558809534, -0.2411417322834644161 ) ) ;
#56378=CARTESIAN_POINT ( 'NONE',  ( 1.568241469816273659, -0.05778040916215560624, -0.4822834645669293319 ) ) ;
#56379=CARTESIAN_POINT ( 'NONE',  ( 0.09067318884954675418, 5.832582624164717122E-16, 0.3627989612356145588 ) ) ;
#56380=CARTESIAN_POINT ( 'NONE',  ( -0.2165354330708654795, 0.1660481256975885056, 0.3530559997133364547 ) ) ;
#56381=CARTESIAN_POINT ( 'NONE',  ( -1.082677165354329896, -0.5400638737290845981, -0.3530559997133363437 ) ) ;
#56382=CARTESIAN_POINT ( 'NONE',  ( -1.535433070866141225, -0.6692913385826771977, 8.415575281601705876E-17 ) ) ;
#56383=CARTESIAN_POINT ( 'NONE',  ( 1.437007874015748810, -0.5400638737290845981, -0.3530559997133363437 ) ) ;
#56385=CARTESIAN_POINT ( 'NONE',  ( 0.9580052493438327987, -0.3690944881889765550, -0.3153832671262227771 ) ) ;
#56388=ORIENTED_EDGE ( 'NONE', *, *, #63677, .T. ) ;
#56389=CARTESIAN_POINT ( 'NONE',  ( 0.09842519685039434474, -0.4536011799217368745, -0.2665933059059886201 ) ) ;
#56390=CARTESIAN_POINT ( 'NONE',  ( -1.574803149606298636, -0.1870078740157479769, 0.4822834645669291653 ) ) ;
#56391=CARTESIAN_POINT ( 'NONE',  ( 0.5839895013123367340, -0.6692913385826773087, -0.1292274648535924053 ) ) ;
#56392=CARTESIAN_POINT ( 'NONE',  ( 0.5052493438320215802, 0.2952755905511811885, 0.1292274648535926551 ) ) ;
#56393=CARTESIAN_POINT ( 'NONE',  ( -0.5971128608923877978, 0.2952755905511811885, 0.1292274648535926551 ) ) ;
#56396=CARTESIAN_POINT ( 'NONE',  ( -1.082677165354329896, -0.5400638737290845981, -0.3530559997133363437 ) ) ;
#56398=CARTESIAN_POINT ( 'NONE',  ( 1.299212598425197429, 0.1771653543307087630, 0.000000000000000000 ) ) ;
#56399=CARTESIAN_POINT ( 'NONE',  ( -1.233595800524933894, -0.6046776061558809534, -0.2411417322834644161 ) ) ;
#56400=CARTESIAN_POINT ( 'NONE',  ( 1.056430446194226658, 0.2952755905511811885, 0.1292274648535926551 ) ) ;
#56401=CARTESIAN_POINT ( 'NONE',  ( 1.259842519685040019, -0.1870078740157480879, -0.4822834645669291653 ) ) ;
#56403=CARTESIAN_POINT ( 'NONE',  ( -1.430446194225721390, -0.4281496062992124485, 0.4176697321401328655 ) ) ;
#56405=CARTESIAN_POINT ( 'NONE',  ( 0.4921259842519691285, 0.1660481256975885056, 0.3530559997133364547 ) ) ;
#56408=CARTESIAN_POINT ( 'NONE',  ( 1.673228346456693494, 0.1660481256975885056, 0.3530559997133364547 ) ) ;
#56409=CARTESIAN_POINT ( 'NONE',  ( 0.2427821522309719648, -0.08942795157527998196, 0.3641732283464567121 ) ) ;
#56410=CARTESIAN_POINT ( 'NONE',  ( 0.7545931758530188826, -0.6692913385826771977, 0.1292274648535927661 ) ) ;
#56412=CARTESIAN_POINT ( 'NONE',  ( 0.8923884514435703741, 0.1283753931104748280, 0.1820866141732283561 ) ) ;
#56413=CARTESIAN_POINT ( 'NONE',  ( 0.4461942257217855201, -0.6046776061558807314, 0.2411417322834647770 ) ) ;
#56415=CARTESIAN_POINT ( 'NONE',  ( -0.9251968503937002541, 0.1660481256975885056, 0.3530559997133364547 ) ) ;
#56416=LINE ( 'NONE', #68649, #41844 ) ;
#56417=CARTESIAN_POINT ( 'NONE',  ( 1.023622047244095112, -0.1870078740157480601, -0.3641732283464567677 ) ) ;
#56418=CARTESIAN_POINT ( 'NONE',  ( -1.122047244094487306, 0.1660481256975883391, -0.3530559997133364547 ) ) ;
#56419=CARTESIAN_POINT ( 'NONE',  ( -0.1574803149606292529, -0.1870078740157479769, 0.4822834645669291653 ) ) ;
#56420=CARTESIAN_POINT ( 'NONE',  ( 0.1574803149606306130, -0.1870078740157480601, -0.3641732283464567677 ) ) ;
#56422=CARTESIAN_POINT ( 'NONE',  ( -0.3543307086614165824, -0.6692913385826771977, 8.415575281601705876E-17 ) ) ;
#56423=CARTESIAN_POINT ( 'NONE',  ( 0.6233595800524939223, -0.2845877964562159024, 0.3641732283464567677 ) ) ;
#56426=CARTESIAN_POINT ( 'NONE',  ( 0.2230971128608932319, -0.4281496062992124485, 0.4176697321401328655 ) ) ;
#56427=CARTESIAN_POINT ( 'NONE',  ( 1.128608923884515169, -0.5023911411419708095, -0.1820866141732282451 ) ) ;
#56428=CARTESIAN_POINT ( 'NONE',  ( -0.3346456692913377662, -0.4536011799217367080, 0.2665933059059888421 ) ) ;
#56429=CARTESIAN_POINT ( 'NONE',  ( -0.8398950131233589023, -0.5023911411419708095, -0.1820866141732282451 ) ) ;
#56430=CARTESIAN_POINT ( 'NONE',  ( -0.3215223097112853146, -0.05778040916215560624, -0.4822834645669293319 ) ) ;
#56431=CARTESIAN_POINT ( 'NONE',  ( 0.5052493438320215802, 0.2952755905511811885, 0.1292274648535926551 ) ) ;
#56432=CARTESIAN_POINT ( 'NONE',  ( 1.181102362204725198, -0.1870078740157479769, 0.3641732283464567677 ) ) ;
#56434=CARTESIAN_POINT ( 'NONE',  ( 1.509186351706037543, -0.3690944881889765550, -0.3153832671262227771 ) ) ;
#56435=CARTESIAN_POINT ( 'NONE',  ( 0.8858267716535438430, 0.1660481256975885056, 0.3530559997133364547 ) ) ;
#56437=CARTESIAN_POINT ( 'NONE',  ( 0.01312335958005323398, 0.05413385826771666132, 0.4176697321401328100 ) ) ;
#56439=CARTESIAN_POINT ( 'NONE',  ( 1.003937007874016407, -0.5400638737290844871, 0.3530559997133364547 ) ) ;
#56440=CARTESIAN_POINT ( 'NONE',  ( 0.4199475065616805614, 0.2306618581243848609, 0.2411417322834645549 ) ) ;
#56442=CARTESIAN_POINT ( 'NONE',  ( 0.2690288713910767848, 0.1771653543307087630, 0.09757992244046791164 ) ) ;
#56443=CARTESIAN_POINT ( 'NONE',  ( 1.036745406824147731, 0.05413385826771666132, 0.4176697321401328100 ) ) ;
#56444=EDGE_CURVE ( 'NONE', #47058, #59607, #62109, .T. ) ;
#56445=CARTESIAN_POINT ( 'NONE',  ( 0.1443569553805781891, -0.3690944881889763329, 0.3153832671262228327 ) ) ;
#56446=CARTESIAN_POINT ( 'NONE',  ( -0.4330708661417315697, -0.6692913385826771977, 8.415575281601705876E-17 ) ) ;
#56447=CARTESIAN_POINT ( 'NONE',  ( 0.5027385518334777093, 1.496062992125983815, -0.5309055118110237448 ) ) ;
#56448=CARTESIAN_POINT ( 'NONE',  ( 0.1574803149606306130, -0.1870078740157479769, 0.4822834645669291653 ) ) ;
#56449=CARTESIAN_POINT ( 'NONE',  ( -0.8398950131233585692, 0.2306618581243848609, 0.2411417322834645549 ) ) ;
#56450=CARTESIAN_POINT ( 'NONE',  ( -0.1574803149606292529, -0.1870078740157479769, 0.3641732283464567677 ) ) ;
#56451=CARTESIAN_POINT ( 'NONE',  ( 0.4527559055118117182, -0.5400638737290844871, 0.3530559997133364547 ) ) ;
#56453=CARTESIAN_POINT ( 'NONE',  ( 0.8727034120734913358, -0.08942795157527998196, 0.3641732283464567121 ) ) ;
#56454=CARTESIAN_POINT ( 'NONE',  ( -0.2952755905511803003, -0.5400638737290845981, -0.3530559997133363437 ) ) ;
#56460=CARTESIAN_POINT ( 'NONE',  ( -1.135170603674539924, 0.2952755905511810774, -0.1292274648535930714 ) ) ;
#56461=CARTESIAN_POINT ( 'NONE',  ( -0.9383202099737524282, -0.05778040916215522460, 0.4822834645669289988 ) ) ;
#56464=VERTEX_POINT ( 'NONE', #24624 ) ;
#56465=CARTESIAN_POINT ( 'NONE',  ( 0.2099737532808405305, -0.5023911411419708095, 0.1820866141732285504 ) ) ;
#56468=CARTESIAN_POINT ( 'NONE',  ( 0.8070866141732288002, 0.1660481256975885056, 0.3530559997133364547 ) ) ;
#56471=CARTESIAN_POINT ( 'NONE',  ( 1.115485564304462551, -0.4281496062992127816, -0.4176697321401328100 ) ) ;
#56472=CARTESIAN_POINT ( 'NONE',  ( 1.141732283464567566, 0.1771653543307087630, 0.000000000000000000 ) ) ;
#56473=CARTESIAN_POINT ( 'NONE',  ( 0.01968503937007957949, -0.5400638737290845981, -0.3530559997133363437 ) ) ;
#56475=CARTESIAN_POINT ( 'NONE',  ( -0.5643044619422565855, -0.4281496062992124485, 0.4176697321401328655 ) ) ;
#56476=CARTESIAN_POINT ( 'NONE',  ( -1.417322834645668772, -0.1870078740157479769, 0.3641732283464567677 ) ) ;
#56477=CARTESIAN_POINT ( 'NONE',  ( -0.6036745406824141069, 0.2306618581243848609, 0.2411417322834645549 ) ) ;
#56478=CARTESIAN_POINT ( 'NONE',  ( 2.795275590551181466, 1.968503937007874738, 0.000000000000000000 ) ) ;
#56482=CARTESIAN_POINT ( 'NONE',  ( 0.3412073490813655186, -0.6046776061558809534, -0.2411417322834644161 ) ) ;
#56484=CARTESIAN_POINT ( 'NONE',  ( -0.4790026246719154557, -0.3162353388693405765, 0.4822834645669290543 ) ) ;
#56485=CARTESIAN_POINT ( 'NONE',  ( -1.476377952755905110, 0.1660481256975885056, 0.3530559997133364547 ) ) ;
#56486=B_SPLINE_CURVE_WITH_KNOTS ( 'NONE', 3,
 ( #39080, #44543, #19306, #51274, #44958, #70234, #70654 ),
 .UNSPECIFIED., .F., .F.,
 ( 4, 3, 4 ),
 ( 5.727215236512864700E-17, 0.001246230184515613373, 0.002492489877932691465 ),
 .UNSPECIFIED. ) ;
#56487=CARTESIAN_POINT ( 'NONE',  ( 0.7874015748031503170, -0.1870078740157479769, 0.4822834645669291653 ) ) ;
#56488=CARTESIAN_POINT ( 'NONE',  ( -0.07217847769028787330, -0.05778040916215522460, 0.4822834645669289988 ) ) ;
#56490=CARTESIAN_POINT ( 'NONE',  ( -0.5708661417322828946, 0.1660481256975883668, -0.3530559997133364547 ) ) ;
#56491=CARTESIAN_POINT ( 'NONE',  ( 0.3608923884514443348, -0.6692913385826771977, 0.1292274648535927661 ) ) ;
#56492=CARTESIAN_POINT ( 'NONE',  ( -0.3412073490813641308, 0.2306618581243847221, -0.2411417322834647770 ) ) ;
#56493=CARTESIAN_POINT ( 'NONE',  ( 0.2493438320209980519, -0.004921259842519576551, 0.3153832671262227771 ) ) ;
#56495=CARTESIAN_POINT ( 'NONE',  ( 0.05905511811023681640, 0.1660481256975883668, -0.3530559997133364547 ) ) ;
#56497=CARTESIAN_POINT ( 'NONE',  ( 1.541994750656168645, -0.6692913385826771977, 0.1292274648535927661 ) ) ;
#56500=EDGE_LOOP ( 'NONE', ( #43298, #58254, #18324, #23382 ) ) ;
#56501=CARTESIAN_POINT ( 'NONE',  ( 0.8136482939632553313, -0.6046776061558809534, -0.2411417322834644161 ) ) ;
#56502=CARTESIAN_POINT ( 'NONE',  ( 5.463695987328526437E-16, -0.1870078740157479769, 0.3641732283464567677 ) ) ;
#56506=CARTESIAN_POINT ( 'NONE',  ( -0.7480314960629916854, 2.362204724409448620, 0.000000000000000000 ) ) ;
#56507=CARTESIAN_POINT ( 'NONE',  ( 0.3937007874015751585, 1.771653543307086354, 0.000000000000000000 ) ) ;
#56509=CARTESIAN_POINT ( 'NONE',  ( 0.5052493438320215802, 0.2952755905511811885, 0.1292274648535926551 ) ) ;
#56510=CARTESIAN_POINT ( 'NONE',  ( -1.377952755905511140, -0.6692913385826771977, 8.415575281601705876E-17 ) ) ;
#56511=CARTESIAN_POINT ( 'NONE',  ( -1.161417322834644716, -0.5400638737290845981, -0.3530559997133363437 ) ) ;
#56512=CARTESIAN_POINT ( 'NONE',  ( 0.05905511811023681640, 0.1660481256975883668, -0.3530559997133364547 ) ) ;
#56513=CARTESIAN_POINT ( 'NONE',  ( 1.036745406824147508, -0.4281496062992127816, -0.4176697321401328100 ) ) ;
#56514=CARTESIAN_POINT ( 'NONE',  ( 1.207349081364829990, 0.1283753931104748280, 0.1820866141732283561 ) ) ;
#56515=CARTESIAN_POINT ( 'NONE',  ( 1.253280839895013710, -0.08942795157528024563, -0.3641732283464568787 ) ) ;
#56516=CARTESIAN_POINT ( 'NONE',  ( -0.7677165354330699465, -0.5400638737290845981, -0.3530559997133363437 ) ) ;
#56518=CARTESIAN_POINT ( 'NONE',  ( -1.620734908136482577, 0.1771653543307087630, 0.09757992244046791164 ) ) ;
#56519=( BOUNDED_CURVE ( )  B_SPLINE_CURVE ( 2, ( #57848, #81910, #18341, #214, #64187, #24222, #32191, #43568, #37677, #69269, #25450, #6521, #12429 ),
 .UNSPECIFIED., .F., .F. ) 
 B_SPLINE_CURVE_WITH_KNOTS ( ( 3, 2, 2, 2, 2, 2, 3 ),
 ( 0.8103969023887780398, 0.8106060606060605522, 0.8143939393939394478, 0.8181818181818182323, 0.8219696969696970168, 0.8257575757575758013, 0.8259667339748583137 ),
 .UNSPECIFIED. ) 
 CURVE ( )  GEOMETRIC_REPRESENTATION_ITEM ( )  RATIONAL_B_SPLINE_CURVE ( ( 0.9964447847208419695, 0.9981185001348091834, 1.000000000000000000, 0.9659258262890683122, 1.000000000000000000, 0.9659258262890683122, 1.000000000000000000, 0.9659258262890683122, 1.000000000000000000, 0.9659258262890683122, 1.000000000000000000, 0.9981185001348091834, 0.9964447847208420805 ) ) 
 REPRESENTATION_ITEM ( '' )  );
#56521=CARTESIAN_POINT ( 'NONE',  ( -0.4461942257217840213, -0.6046776061558809534, -0.2411417322834644161 ) ) ;
#56522=CARTESIAN_POINT ( 'NONE',  ( 1.010498687664042716, -0.4281496062992124485, 0.4176697321401328655 ) ) ;
#56524=CARTESIAN_POINT ( 'NONE',  ( -1.601049868766403650, -0.5023911411419708095, 0.1820866141732285504 ) ) ;
#56525=CARTESIAN_POINT ( 'NONE',  ( 0.4986876640419954376, -0.6046776061558809534, -0.2411417322834644161 ) ) ;
#56526=CARTESIAN_POINT ( 'NONE',  ( 0.7742782152230978099, -0.3690944881889763329, 0.3153832671262228327 ) ) ;
#56527=CARTESIAN_POINT ( 'NONE',  ( -1.528871391076114250, 0.1771653543307087075, -0.09757992244046823083 ) ) ;
#56528=CARTESIAN_POINT ( 'NONE',  ( 0.9711286089238851948, -0.6046776061558809534, -0.2411417322834644161 ) ) ;
#56529=CARTESIAN_POINT ( 'NONE',  ( -1.171093442848938793, -2.191421614605370878E-15, 0.4445507791589071167 ) ) ;
#56530=CARTESIAN_POINT ( 'NONE',  ( -0.5577427821522301654, -0.08942795157528024563, -0.3641732283464568787 ) ) ;
#56531=CARTESIAN_POINT ( 'NONE',  ( -0.4986876640419942164, -0.6046776061558807314, 0.2411417322834647770 ) ) ;
#56532=CARTESIAN_POINT ( 'NONE',  ( 1.692913385826772421, 0.2952755905511811885, 0.000000000000000000 ) ) ;
#56533=CARTESIAN_POINT ( 'NONE',  ( -1.266404199475064773, -0.3162353388693405765, 0.4822834645669290543 ) ) ;
#56535=CARTESIAN_POINT ( 'NONE',  ( 1.305774278215223960, -0.6692913385826771977, 0.1292274648535927661 ) ) ;
#56537=CARTESIAN_POINT ( 'NONE',  ( -1.509186351706035767, -0.3690944881889763329, 0.3153832671262228327 ) ) ;
#56540=CARTESIAN_POINT ( 'NONE',  ( 1.601049868766404982, 0.2306618581243848609, 0.2411417322834645549 ) ) ;
#56543=CARTESIAN_POINT ( 'NONE',  ( -1.332020997375327642, -0.08942795157527998196, 0.3641732283464567121 ) ) ;
#56544=CARTESIAN_POINT ( 'NONE',  ( -0.9448818897637790704, -0.1870078740157479769, 0.3641732283464567677 ) ) ;
#56545=CARTESIAN_POINT ( 'NONE',  ( 1.692913385826772421, 0.1771653543307087630, 0.000000000000000000 ) ) ;
#56546=CARTESIAN_POINT ( 'NONE',  ( -0.4396325459317577122, -0.6692913385826773087, -0.1292274648535924053 ) ) ;
#56547=CARTESIAN_POINT ( 'NONE',  ( 0.03937007874015833325, -0.5511811023622047445, 6.969142054262312111E-17 ) ) ;
#56548=CARTESIAN_POINT ( 'NONE',  ( -1.167979002624671470, -0.3690944881889765550, -0.3153832671262227771 ) ) ;
#56549=CARTESIAN_POINT ( 'NONE',  ( 1.391076115485564868, -0.5023911411419708095, 0.1820866141732285504 ) ) ;
#56550=CARTESIAN_POINT ( 'NONE',  ( 0.8136482939632553313, -0.6046776061558809534, -0.2411417322834644161 ) ) ;
#56551=CARTESIAN_POINT ( 'NONE',  ( 1.515748031496063186, -0.5400638737290845981, -0.3530559997133363437 ) ) ;
#56552=CARTESIAN_POINT ( 'NONE',  ( 0.5643044619422579178, -0.004921259842519576551, 0.3153832671262227771 ) ) ;
#56553=CARTESIAN_POINT ( 'NONE',  ( 0.4330708661417329575, 0.2952755905511811885, 0.000000000000000000 ) ) ;
#56555=CARTESIAN_POINT ( 'NONE',  ( 0.7874015748031503170, -0.1870078740157479769, 0.3641732283464567677 ) ) ;
#56557=CARTESIAN_POINT ( 'NONE',  ( -1.135170603674539924, 0.2952755905511810774, -0.1292274648535930714 ) ) ;
#56558=CARTESIAN_POINT ( 'NONE',  ( -1.279527559055116948, 0.1660481256975883668, -0.3530559997133364547 ) ) ;
#56559=CARTESIAN_POINT ( 'NONE',  ( -0.1640419947506555343, -0.3162353388693405765, 0.4822834645669290543 ) ) ;
#56560=LINE ( 'NONE', #81442, #5649 ) ;
#56562=CARTESIAN_POINT ( 'NONE',  ( 0.3543307086614179147, 0.2952755905511811885, 0.000000000000000000 ) ) ;
#56563=CARTESIAN_POINT ( 'NONE',  ( 1.174540682414699111, -0.08942795157528024563, -0.3641732283464568787 ) ) ;
#56564=CARTESIAN_POINT ( 'NONE',  ( -0.04593175853018302557, 0.2952755905511811885, 0.1292274648535926551 ) ) ;
#56565=CARTESIAN_POINT ( 'NONE',  ( 0.2493438320209980519, -0.4281496062992127816, -0.4176697321401328100 ) ) ;
#56571=CARTESIAN_POINT ( 'NONE',  ( -0.6824146981627291497, -0.5023911411419708095, -0.1820866141732282451 ) ) ;
#56572=CARTESIAN_POINT ( 'NONE',  ( -0.8136482939632537770, -0.6046776061558807314, 0.2411417322834647770 ) ) ;
#56573=CARTESIAN_POINT ( 'NONE',  ( 0.2559055118110243332, -0.5400638737290845981, -0.3530559997133363437 ) ) ;
#56575=CARTESIAN_POINT ( 'NONE',  ( 0.7677165354330716118, 0.1660481256975883668, -0.3530559997133364547 ) ) ;
#56576=CARTESIAN_POINT ( 'NONE',  ( -1.541994750656167090, -0.6692913385826773087, -0.1292274648535924053 ) ) ;
#56577=CARTESIAN_POINT ( 'NONE',  ( 0.7152230971128614723, -0.3162353388693409650, -0.4822834645669289433 ) ) ;
#56580=CARTESIAN_POINT ( 'NONE',  ( 1.692913385826772421, 0.2952755905511811885, 0.000000000000000000 ) ) ;
#56581=CARTESIAN_POINT ( 'NONE',  ( 0.9448818897637802916, -0.1870078740157479769, 0.4822834645669291653 ) ) ;
#56582=CARTESIAN_POINT ( 'NONE',  ( 0.4002624671916016896, -0.3162353388693409650, -0.4822834645669289433 ) ) ;
#56583=CARTESIAN_POINT ( 'NONE',  ( 1.174540682414699111, -0.08942795157528024563, -0.3641732283464568787 ) ) ;
#56584=CARTESIAN_POINT ( 'NONE',  ( 1.561679790026247350, 0.05413385826771626580, -0.4176697321401330321 ) ) ;
#56587=CARTESIAN_POINT ( 'NONE',  ( 0.6496062992125991586, -0.5400638737290845981, -0.3530559997133363437 ) ) ;
#56588=CARTESIAN_POINT ( 'NONE',  ( 1.601049868766404982, -0.5023911411419708095, -0.1820866141732282451 ) ) ;
#56589=CARTESIAN_POINT ( 'NONE',  ( -0.4396325459317579898, 0.2952755905511811885, 0.1292274648535926551 ) ) ;
#56590=CARTESIAN_POINT ( 'NONE',  ( -1.036745406824146176, 0.05413385826771626580, -0.4176697321401330321 ) ) ;
#56592=CARTESIAN_POINT ( 'NONE',  ( 0.9973753280839902091, 0.2306618581243847221, -0.2411417322834647770 ) ) ;
#56596=CARTESIAN_POINT ( 'NONE',  ( -1.463254593175852492, 0.1771653543307087630, 0.09757992244046791164 ) ) ;
#56600=CARTESIAN_POINT ( 'NONE',  ( -0.7233831536535468842, 2.232734770847097039, -0.5048085489443572271 ) ) ;
#56601=CARTESIAN_POINT ( 'NONE',  ( 1.246719160104987623, -0.3690944881889763329, 0.3153832671262228327 ) ) ;
#56603=CARTESIAN_POINT ( 'NONE',  ( 1.482939632545932307, -0.3690944881889763329, 0.3153832671262228327 ) ) ;
#56605=CARTESIAN_POINT ( 'NONE',  ( -1.013613127888308485, -2.191421614605370878E-15, 0.4445507791589071167 ) ) ;
#56608=CARTESIAN_POINT ( 'NONE',  ( -0.6692913385826764205, 0.1771653543307087630, 0.000000000000000000 ) ) ;
#56609=CARTESIAN_POINT ( 'NONE',  ( -1.135170603674539924, -0.5511811023622046335, 0.09757992244046803654 ) ) ;
#56610=CARTESIAN_POINT ( 'NONE',  ( -1.259842519685038686, -0.1870078740157480879, -0.4822834645669291653 ) ) ;
#56611=CARTESIAN_POINT ( 'NONE',  ( 0.06561679790026316017, 0.05413385826771626580, -0.4176697321401330321 ) ) ;
#56612=CARTESIAN_POINT ( 'NONE',  ( 1.535433070866142335, -0.6692913385826771977, 8.415575281601705876E-17 ) ) ;
#56614=CARTESIAN_POINT ( 'NONE',  ( 1.332020997375328974, -0.05778040916215560624, -0.4822834645669293319 ) ) ;
#56619=CARTESIAN_POINT ( 'NONE',  ( -0.5183727034120726440, 0.1771653543307087630, 0.09757992244046791164 ) ) ;
#56620=CARTESIAN_POINT ( 'NONE',  ( -1.102362204724408601, -0.1870078740157480879, -0.4822834645669291653 ) ) ;
#56621=CARTESIAN_POINT ( 'NONE',  ( 1.102362204724410155, -0.1870078740157480879, -0.4822834645669291653 ) ) ;
#56622=ORIENTED_EDGE ( 'NONE', *, *, #7244, .T. ) ;
#56624=CARTESIAN_POINT ( 'NONE',  ( -0.7478466213799878082, 1.968503937007873850, 0.5309055118110236338 ) ) ;
#56625=CARTESIAN_POINT ( 'NONE',  ( -1.712598425196849572, 0.1660481256975885056, 0.3530559997133364547 ) ) ;
#56626=CARTESIAN_POINT ( 'NONE',  ( -1.036745406824146176, 0.05413385826771626580, -0.4176697321401330321 ) ) ;
#56628=CARTESIAN_POINT ( 'NONE',  ( 0.05249343832021075018, 0.1283753931104746893, -0.1820866141732285504 ) ) ;
#56630=CARTESIAN_POINT ( 'NONE',  ( -0.3608923884514428360, 0.1771653543307087630, 0.09757992244046791164 ) ) ;
#56631=CARTESIAN_POINT ( 'NONE',  ( 0.3543307086614179147, 0.1771653543307087630, 0.000000000000000000 ) ) ;
#56632=CARTESIAN_POINT ( 'NONE',  ( 0.4396325459317590445, -0.6692913385826771977, 0.1292274648535927661 ) ) ;
#56633=CARTESIAN_POINT ( 'NONE',  ( -0.6167979002624665030, -0.3690944881889765550, -0.3153832671262227771 ) ) ;
#56635=CARTESIAN_POINT ( 'NONE',  ( 1.003937007874016185, 0.1660481256975883668, -0.3530559997133364547 ) ) ;
#56636=CARTESIAN_POINT ( 'NONE',  ( -1.141732283464566011, 0.2952755905511811885, 0.000000000000000000 ) ) ;
#56638=CARTESIAN_POINT ( 'NONE',  ( -0.4921259842519677963, -0.5400638737290844871, 0.3530559997133364547 ) ) ;
#56639=CARTESIAN_POINT ( 'NONE',  ( -0.4199475065616791736, -0.6046776061558807314, 0.2411417322834647770 ) ) ;
#56640=CARTESIAN_POINT ( 'NONE',  ( 1.325459317585302665, -0.3690944881889763329, 0.3153832671262228327 ) ) ;
#56641=CARTESIAN_POINT ( 'NONE',  ( 0.1706036745406830368, -0.004921259842519576551, 0.3153832671262227771 ) ) ;
#56642=CARTESIAN_POINT ( 'NONE',  ( -0.08530183727034056085, -0.05778040916215560624, -0.4822834645669293319 ) ) ;
#56643=CARTESIAN_POINT ( 'NONE',  ( -0.9842519685039360366, 0.2952755905511811885, 0.000000000000000000 ) ) ;
#56644=CARTESIAN_POINT ( 'NONE',  ( -1.646051170424378096, 0.000000000000000000, -0.3464511005275205946 ) ) ;
#56645=CARTESIAN_POINT ( 'NONE',  ( 1.528871391076116026, 0.1771653543307087630, 0.09757992244046791164 ) ) ;
#56646=CARTESIAN_POINT ( 'NONE',  ( -0.2755905511811015396, -0.6692913385826771977, 8.415575281601705876E-17 ) ) ;
#56648=CARTESIAN_POINT ( 'NONE',  ( -1.141732283464566011, -0.6692913385826771977, 8.415575281601705876E-17 ) ) ;
#56651=CARTESIAN_POINT ( 'NONE',  ( 1.332020997375328974, -0.05778040916215560624, -0.4822834645669293319 ) ) ;
#56652=CARTESIAN_POINT ( 'NONE',  ( -0.8136482939632537770, -0.5023911411419708095, 0.1820866141732285504 ) ) ;
#56653=CARTESIAN_POINT ( 'NONE',  ( -0.7283464566929126471, 0.1660481256975883668, -0.3530559997133364547 ) ) ;
#56654=CARTESIAN_POINT ( 'NONE',  ( 1.194225721784777594, 0.05413385826771666132, 0.4176697321401328100 ) ) ;
#56655=CARTESIAN_POINT ( 'NONE',  ( 0.9973753280839902091, -0.6046776061558807314, 0.2411417322834647770 ) ) ;
#56656=CARTESIAN_POINT ( 'NONE',  ( 1.528871391076116026, -0.6692913385826773087, -0.1292274648535924053 ) ) ;
#56657=CARTESIAN_POINT ( 'NONE',  ( -0.9383202099737524282, -0.08942795157527998196, 0.3641732283464567121 ) ) ;
#56662=CARTESIAN_POINT ( 'NONE',  ( 0.9645669291338591078, -0.4536011799217368745, -0.2665933059059886201 ) ) ;
#56664=CARTESIAN_POINT ( 'NONE',  ( 0.7808398950131240079, -0.2845877964562159024, 0.3641732283464567677 ) ) ;
#56665=CARTESIAN_POINT ( 'NONE',  ( 0.4724409448818904789, -0.1870078740157479769, 0.4822834645669291653 ) ) ;
#56666=CARTESIAN_POINT ( 'NONE',  ( 1.601049868766404982, 0.2306618581243848609, 0.2411417322834645549 ) ) ;
#56668=CARTESIAN_POINT ( 'NONE',  ( 0.7611548556430454138, 0.1283753931104746893, -0.1820866141732285504 ) ) ;
#56669=CARTESIAN_POINT ( 'NONE',  ( -0.1181102362204717315, -0.6692913385826771977, 8.415575281601705876E-17 ) ) ;
#56670=CARTESIAN_POINT ( 'NONE',  ( -1.213910761154854745, -0.6692913385826771977, 0.1292274648535927661 ) ) ;
#56671=CARTESIAN_POINT ( 'NONE',  ( 1.345144356955381593, -0.05778040916215522460, 0.4822834645669289988 ) ) ;
#56674=CARTESIAN_POINT ( 'NONE',  ( -0.05249343832020938322, -0.5023911411419708095, -0.1820866141732282451 ) ) ;
#56676=ORIENTED_EDGE ( 'NONE', *, *, #33628, .T. ) ;
#56677=CARTESIAN_POINT ( 'NONE',  ( -0.7808398950131225646, -0.05778040916215522460, 0.4822834645669289988 ) ) ;
#56678=CARTESIAN_POINT ( 'NONE',  ( -0.7545931758530176614, -0.6692913385826773087, -0.1292274648535924053 ) ) ;
#56679=CARTESIAN_POINT ( 'NONE',  ( -0.3149606299212590610, -0.1870078740157480879, -0.4822834645669291653 ) ) ;
#56681=CARTESIAN_POINT ( 'NONE',  ( 0.4724409448818904789, -0.1870078740157480879, -0.4822834645669291653 ) ) ;
#56682=CARTESIAN_POINT ( 'NONE',  ( -0.3346456692913377662, 0.1660481256975883668, -0.3530559997133364547 ) ) ;
#56683=CARTESIAN_POINT ( 'NONE',  ( -1.128608923884513837, 0.2306618581243847221, -0.2411417322834647770 ) ) ;
#56684=CARTESIAN_POINT ( 'NONE',  ( -0.7283464566929126471, 0.1660481256975883668, -0.3530559997133364547 ) ) ;
#56685=CARTESIAN_POINT ( 'NONE',  ( 0.8267716535433077274, 0.2952755905511811885, 0.000000000000000000 ) ) ;
#56686=( BOUNDED_CURVE ( )  B_SPLINE_CURVE ( 1, ( #49515, #60908 ),
 .UNSPECIFIED., .F., .F. ) 
 B_SPLINE_CURVE_WITH_KNOTS ( ( 2, 2 ),
 ( 0.000000000000000000, 0.002000000000000001776 ),
 .UNSPECIFIED. ) 
 CURVE ( )  GEOMETRIC_REPRESENTATION_ITEM ( )  RATIONAL_B_SPLINE_CURVE ( ( 0.9875488213027530104, 0.9875488213027530104 ) ) 
 REPRESENTATION_ITEM ( '' )  );
#56689=CARTESIAN_POINT ( 'NONE',  ( -0.2624671916010490880, -0.5023911411419708095, 0.1820866141732285504 ) ) ;
#56690=ORIENTED_EDGE ( 'NONE', *, *, #43363, .F. ) ;
#56693=CARTESIAN_POINT ( 'NONE',  ( -1.286089238845143479, -0.5023911411419708095, 0.1820866141732285504 ) ) ;
#56694=CARTESIAN_POINT ( 'NONE',  ( -0.8923884514435688198, -0.6046776061558807314, 0.2411417322834647770 ) ) ;
#56695=CARTESIAN_POINT ( 'NONE',  ( -0.9973753280839886548, 0.2306618581243848609, 0.2411417322834645549 ) ) ;
#56697=CARTESIAN_POINT ( 'NONE',  ( -0.8858267716535425107, 0.1660481256975883668, -0.3530559997133364547 ) ) ;
#56698=CARTESIAN_POINT ( 'NONE',  ( -0.9383202099737524282, -0.05778040916215522460, 0.4822834645669289988 ) ) ;
#56699=CARTESIAN_POINT ( 'NONE',  ( -1.614173228346455824, 0.2952755905511811885, 0.000000000000000000 ) ) ;
#56701=CARTESIAN_POINT ( 'NONE',  ( 0.6233595800524942554, -0.08942795157528024563, -0.3641732283464568787 ) ) ;
#56702=CARTESIAN_POINT ( 'NONE',  ( 0.4849061582275022153, 1.568468489416427580, 0.4921425059946342717 ) ) ;
#56704=CARTESIAN_POINT ( 'NONE',  ( -0.1377952755905504645, 0.07958543189024085140, 0.2665933059059887866 ) ) ;
#56705=CARTESIAN_POINT ( 'NONE',  ( -0.4658792650918627265, -0.3162353388693409650, -0.4822834645669289433 ) ) ;
#56706=CARTESIAN_POINT ( 'NONE',  ( 1.482939632545932307, 0.05413385826771626580, -0.4176697321401330321 ) ) ;
#56707=CARTESIAN_POINT ( 'NONE',  ( 0.01312335958005323398, -0.4281496062992127816, -0.4176697321401328100 ) ) ;
#56708=ORIENTED_EDGE ( 'NONE', *, *, #3202, .T. ) ;
#56714=CARTESIAN_POINT ( 'NONE',  ( 1.227034120734908917, -0.6692913385826771977, 0.1292274648535927661 ) ) ;
#56715=CARTESIAN_POINT ( 'NONE',  ( -1.141732283464566011, -0.5511811023622047445, 6.969142054262312111E-17 ) ) ;
#56716=EDGE_CURVE ( 'NONE', #74449, #78494, #68436, .T. ) ;
#56717=CARTESIAN_POINT ( 'NONE',  ( -1.351706036745406347, 0.05413385826771626580, -0.4176697321401330321 ) ) ;
#56721=CARTESIAN_POINT ( 'NONE',  ( 1.437007874015748810, -0.5400638737290845981, -0.3530559997133363437 ) ) ;
#56722=CARTESIAN_POINT ( 'NONE',  ( 0.5052493438320215802, 0.2952755905511811885, 0.1292274648535926551 ) ) ;
#56723=CARTESIAN_POINT ( 'NONE',  ( 0.1902887139107617975, -0.6692913385826773087, -0.1292274648535924053 ) ) ;
#56724=CARTESIAN_POINT ( 'NONE',  ( -1.266404199475064773, -0.08942795157528024563, -0.3641732283464568787 ) ) ;
#56725=CARTESIAN_POINT ( 'NONE',  ( -0.4724409448818890911, -0.1870078740157479769, 0.4822834645669291653 ) ) ;
#56727=CARTESIAN_POINT ( 'NONE',  ( -0.8727034120734901146, -0.05778040916215560624, -0.4822834645669293319 ) ) ;
#56729=CARTESIAN_POINT ( 'NONE',  ( 1.194225721784777594, -0.3690944881889765550, -0.3153832671262227771 ) ) ;
#56730=CARTESIAN_POINT ( 'NONE',  ( -0.2755905511811018171, 0.1771653543307087630, 0.000000000000000000 ) ) ;
#56731=CARTESIAN_POINT ( 'NONE',  ( 1.017060367454068803, -0.2845877964562159024, 0.3641732283464567677 ) ) ;
#56732=CARTESIAN_POINT ( 'NONE',  ( -1.653543307086613234, -0.1870078740157480879, -0.4822834645669291653 ) ) ;
#56733=CARTESIAN_POINT ( 'NONE',  ( -1.246719160104985846, -0.3690944881889765550, -0.3153832671262227771 ) ) ;
#56735=CARTESIAN_POINT ( 'NONE',  ( 0.7480314960629927956, 0.1771653543307087630, 0.000000000000000000 ) ) ;
#56736=CARTESIAN_POINT ( 'NONE',  ( -0.7086614173228339419, -0.1870078740157479769, 0.4822834645669291653 ) ) ;
#56738=CARTESIAN_POINT ( 'NONE',  ( -0.04593175853018302557, 0.1771653543307087630, 0.09757992244046791164 ) ) ;
#56739=CARTESIAN_POINT ( 'NONE',  ( -1.679790026246718693, 0.1283753931104746893, -0.1820866141732285504 ) ) ;
#56740=CARTESIAN_POINT ( 'NONE',  ( 0.7874015748031503170, -0.1870078740157480879, -0.4822834645669291653 ) ) ;
#56741=CARTESIAN_POINT ( 'NONE',  ( 0.6496062992125991586, 0.1660481256975885056, 0.3530559997133364547 ) ) ;
#56742=CARTESIAN_POINT ( 'NONE',  ( 1.384514435695538337, -0.5511811023622046335, 0.09757992244046803654 ) ) ;
#56743=CARTESIAN_POINT ( 'NONE',  ( -0.9973753280839886548, -0.6046776061558809534, -0.2411417322834644161 ) ) ;
#56744=CARTESIAN_POINT ( 'NONE',  ( -0.1837270341207340729, 0.1283753931104746893, -0.1820866141732285504 ) ) ;
#56745=CARTESIAN_POINT ( 'NONE',  ( -1.646051170424378096, -0.1870078740157480046, 1.254653134982923898E-17 ) ) ;
#56746=CARTESIAN_POINT ( 'NONE',  ( 0.3280839895013130669, -0.004921259842519576551, 0.3153832671262227771 ) ) ;
#56747=CARTESIAN_POINT ( 'NONE',  ( -1.292650918635170010, -0.6692913385826771977, 0.1292274648535927661 ) ) ;
#56748=CARTESIAN_POINT ( 'NONE',  ( -0.6167979002624665030, -0.4281496062992127816, -0.4176697321401328100 ) ) ;
#56751=CARTESIAN_POINT ( 'NONE',  ( 0.5708661417322841158, -0.4536011799217368745, -0.2665933059059886201 ) ) ;
#56752=CARTESIAN_POINT ( 'NONE',  ( -0.1902887139107604098, 0.2952755905511810774, -0.1292274648535930714 ) ) ;
#56753=CARTESIAN_POINT ( 'NONE',  ( -0.8530183727034112984, 0.05413385826771666132, 0.4176697321401328100 ) ) ;
#56754=CARTESIAN_POINT ( 'NONE',  ( -0.6299212598425188991, -0.1870078740157480601, -0.3641732283464567677 ) ) ;
#56756=CARTESIAN_POINT ( 'NONE',  ( -0.2296587926509179312, -0.05778040916215522460, 0.4822834645669289988 ) ) ;
#56757=CARTESIAN_POINT ( 'NONE',  ( -1.673228346456691717, 0.07958543189024071263, -0.2665933059059888421 ) ) ;
#56758=CARTESIAN_POINT ( 'NONE',  ( 1.574803149606299746, -0.1870078740157479769, 0.4822834645669291653 ) ) ;
#56759=CARTESIAN_POINT ( 'NONE',  ( 0.01069919276010583738, 2.739544932778246860E-15, 0.4118477457932983032 ) ) ;
#56762=CARTESIAN_POINT ( 'NONE',  ( -1.312335958005248715, -0.6046776061558809534, -0.2411417322834644161 ) ) ;
#56764=CARTESIAN_POINT ( 'NONE',  ( -0.7808398950131225646, -0.05778040916215522460, 0.4822834645669289988 ) ) ;
#56765=CARTESIAN_POINT ( 'NONE',  ( 1.614173228346457378, 0.2952755905511811885, 0.000000000000000000 ) ) ;
#56768=CARTESIAN_POINT ( 'NONE',  ( 0.8333333333333340365, -0.6692913385826771977, 0.1292274648535927661 ) ) ;
#56769=CARTESIAN_POINT ( 'NONE',  ( -0.06561679790026180015, 0.05413385826771666132, 0.4176697321401328100 ) ) ;
#56772=CARTESIAN_POINT ( 'NONE',  ( 1.069553805774278610, -0.5511811023622046335, 0.09757992244046803654 ) ) ;
#56774=VERTEX_POINT ( 'NONE', #56605 ) ;
#56777=CARTESIAN_POINT ( 'NONE',  ( 0.2821522309711292364, -0.6692913385826771977, 0.1292274648535927661 ) ) ;
#56778=CARTESIAN_POINT ( 'NONE',  ( -0.6692913385826764205, -0.6692913385826771977, 8.415575281601705876E-17 ) ) ;
#56780=CARTESIAN_POINT ( 'NONE',  ( -1.397637795275589623, -0.5400638737290845981, -0.3530559997133363437 ) ) ;
#56781=CARTESIAN_POINT ( 'NONE',  ( 0.8267716535433078384, -0.6692913385826771977, 8.415575281601705876E-17 ) ) ;
#56782=CARTESIAN_POINT ( 'NONE',  ( 1.509186351706037543, 0.05413385826771666132, 0.4176697321401328100 ) ) ;
#56784=CARTESIAN_POINT ( 'NONE',  ( -0.2690288713910754526, -0.6692913385826771977, 0.1292274648535927661 ) ) ;
#56785=CARTESIAN_POINT ( 'NONE',  ( -1.437007874015747477, 0.1660481256975883668, -0.3530559997133364547 ) ) ;
#56786=CARTESIAN_POINT ( 'NONE',  ( -1.555118110236219930, -0.5400638737290845981, -0.3530559997133363437 ) ) ;
#56787=CARTESIAN_POINT ( 'NONE',  ( 1.509186351706037543, 0.05413385826771666132, 0.4176697321401328100 ) ) ;
#56789=CARTESIAN_POINT ( 'NONE',  ( 0.7283464566929143125, 0.07958543189024085140, 0.2665933059059887866 ) ) ;
#56793=CARTESIAN_POINT ( 'NONE',  ( -0.1509186351706028884, -0.08942795157527998196, 0.3641732283464567121 ) ) ;
#56795=CARTESIAN_POINT ( 'NONE',  ( 0.4461942257217855201, -0.6046776061558807314, 0.2411417322834647770 ) ) ;
#56796=CARTESIAN_POINT ( 'NONE',  ( 0.2493438320209980519, -0.4281496062992127816, -0.4176697321401328100 ) ) ;
#56797=CARTESIAN_POINT ( 'NONE',  ( -0.4658792650918627265, -0.05778040916215522460, 0.4822834645669289988 ) ) ;
#56799=CARTESIAN_POINT ( 'NONE',  ( -1.397637795275589623, -0.5400638737290845981, -0.3530559997133363437 ) ) ;
#56802=CARTESIAN_POINT ( 'NONE',  ( 1.220472440944882386, -0.5511811023622047445, 6.969142054262312111E-17 ) ) ;
#56803=CARTESIAN_POINT ( 'NONE',  ( -1.450131233595799651, 0.2952755905511810774, -0.1292274648535930714 ) ) ;
#56804=CARTESIAN_POINT ( 'NONE',  ( 0.7939632545931766261, -0.3162353388693409650, -0.4822834645669289433 ) ) ;
#56805=CARTESIAN_POINT ( 'NONE',  ( 1.279527559055118724, -0.5400638737290845981, -0.3530559997133363437 ) ) ;
#56807=CARTESIAN_POINT ( 'NONE',  ( -1.240157480314959759, 0.1660481256975885056, 0.3530559997133364547 ) ) ;
#56809=CARTESIAN_POINT ( 'NONE',  ( -0.2362204724409442680, -0.1870078740157480879, -0.4822834645669291653 ) ) ;
#56812=CARTESIAN_POINT ( 'NONE',  ( 1.509186351706037543, 0.05413385826771666132, 0.4176697321401328100 ) ) ;
#56813=CARTESIAN_POINT ( 'NONE',  ( 0.07874015748031558404, -0.1870078740157479769, 0.3641732283464567677 ) ) ;
#56814=CARTESIAN_POINT ( 'NONE',  ( 0.8858267716535438430, -0.5400638737290845981, -0.3530559997133363437 ) ) ;
#56816=CARTESIAN_POINT ( 'NONE',  ( 0.7217847769028878924, -0.004921259842519576551, 0.3153832671262227771 ) ) ;
#56818=CARTESIAN_POINT ( 'NONE',  ( 0.3083989501312343062, -0.3162353388693405765, 0.4822834645669290543 ) ) ;
#56820=CARTESIAN_POINT ( 'NONE',  ( -0.7874015748031489847, -0.1870078740157479769, 0.4822834645669291653 ) ) ;
#56822=CARTESIAN_POINT ( 'NONE',  ( 0.8727034120734912248, -0.2845877964562161244, -0.3641732283464567121 ) ) ;
#56823=EDGE_CURVE ( 'NONE', #60349, #30126, #18152, .T. ) ;
#56824=CARTESIAN_POINT ( 'NONE',  ( 0.09842519685039433086, 0.1012011053420777407, 0.2882089793578256898 ) ) ;
#56825=CARTESIAN_POINT ( 'NONE',  ( -0.4658792650918627265, -0.05778040916215522460, 0.4822834645669289988 ) ) ;
#56826=CARTESIAN_POINT ( 'NONE',  ( 0.2362204724409456558, -0.1870078740157479769, 0.3641732283464567677 ) ) ;
#56828=CARTESIAN_POINT ( 'NONE',  ( -0.1312335958005241554, 0.2306618581243848609, 0.2411417322834645549 ) ) ;
#56829=CARTESIAN_POINT ( 'NONE',  ( 0.4396325459317590445, -0.5511811023622046335, 0.09757992244046803654 ) ) ;
#56831=CARTESIAN_POINT ( 'NONE',  ( 0.3674540682414705883, -0.6046776061558807314, 0.2411417322834647770 ) ) ;
#56832=CARTESIAN_POINT ( 'NONE',  ( 1.036745406824147731, -0.004921259842519576551, 0.3153832671262227771 ) ) ;
#56833=CARTESIAN_POINT ( 'NONE',  ( 2.795275590551181910, 1.805669738366189048, 0.000000000000000000 ) ) ;
#56834=CARTESIAN_POINT ( 'NONE',  ( -0.5905511811023615998, 0.1771653543307087630, 0.000000000000000000 ) ) ;
#56835=CARTESIAN_POINT ( 'NONE',  ( -0.8202099737532801971, -0.5511811023622046335, 0.09757992244046803654 ) ) ;
#56836=CARTESIAN_POINT ( 'NONE',  ( -0.3937007874015740483, -0.1870078740157479769, 0.4822834645669291653 ) ) ;
#56837=CARTESIAN_POINT ( 'NONE',  ( 0.2099737532808405305, 0.2306618581243847221, -0.2411417322834647770 ) ) ;
#56838=CARTESIAN_POINT ( 'NONE',  ( 0.8202099737532814183, -0.5511811023622048555, -0.09757992244046775898 ) ) ;
#56840=CARTESIAN_POINT ( 'NONE',  ( 1.476377952755906220, 0.07958543189024071263, -0.2665933059059888421 ) ) ;
#56842=CARTESIAN_POINT ( 'NONE',  ( 0.7020997375328090762, -0.3162353388693405765, 0.4822834645669290543 ) ) ;
#56844=CARTESIAN_POINT ( 'NONE',  ( -0.1377952755905504645, 0.1660481256975885056, 0.3530559997133364547 ) ) ;
#56846=CARTESIAN_POINT ( 'NONE',  ( 0.8333333333333340365, -0.6692913385826771977, 0.1292274648535927661 ) ) ;
#56847=CARTESIAN_POINT ( 'NONE',  ( 0.6758530183727039509, -0.6692913385826771977, 0.1292274648535927661 ) ) ;
#56849=CARTESIAN_POINT ( 'NONE',  ( 0.1837270341207357105, -0.5023911411419708095, -0.1820866141732282451 ) ) ;
#56850=CARTESIAN_POINT ( 'NONE',  ( 1.410761154855643795, -0.05778040916215560624, -0.4822834645669293319 ) ) ;
#56852=CARTESIAN_POINT ( 'NONE',  ( -0.3149606299212590610, -0.1870078740157479769, 0.3641732283464567677 ) ) ;
#56853=CARTESIAN_POINT ( 'NONE',  ( -0.3083989501312330295, -0.3162353388693409650, -0.4822834645669289433 ) ) ;
#56854=CARTESIAN_POINT ( 'NONE',  ( 0.5157744752572718250, 1.509207849855008998, -0.5177606540819982284 ) ) ;
#56855=CARTESIAN_POINT ( 'NONE',  ( 0.3149606299212603933, -0.1870078740157479769, 0.4822834645669291653 ) ) ;
#56856=CARTESIAN_POINT ( 'NONE',  ( -0.6364829396325453192, -0.05778040916215560624, -0.4822834645669293319 ) ) ;
#56858=CARTESIAN_POINT ( 'NONE',  ( -0.7152230971128602510, -0.08942795157528024563, -0.3641732283464568787 ) ) ;
#56859=CARTESIAN_POINT ( 'NONE',  ( 0.2887139107611556010, -0.6046776061558807314, 0.2411417322834647770 ) ) ;
#56860=CARTESIAN_POINT ( 'NONE',  ( -1.056430446194224881, 0.2952755905511810774, -0.1292274648535930714 ) ) ;
#56861=CARTESIAN_POINT ( 'NONE',  ( -0.4461942257217840213, -0.6046776061558809534, -0.2411417322834644161 ) ) ;
#56862=EDGE_CURVE ( 'NONE', #73164, #52448, #13671, .T. ) ;
#56864=CARTESIAN_POINT ( 'NONE',  ( -0.5944687039322197331, 1.968503937007873850, 0.4915354330708656128 ) ) ;
#56865=CARTESIAN_POINT ( 'NONE',  ( 1.443569553805774897, 0.2306618581243848609, 0.2411417322834645549 ) ) ;
#56866=CARTESIAN_POINT ( 'NONE',  ( -0.06873123812452887338, -2.191421614605370878E-15, 0.4445507791589071167 ) ) ;
#56868=FACE_OUTER_BOUND ( 'NONE', #64279, .T. ) ;
#56869=CARTESIAN_POINT ( 'NONE',  ( -0.8202099737532801971, -0.6692913385826771977, 0.1292274648535927661 ) ) ;
#56873=EDGE_LOOP ( 'NONE', ( #12301, #70769, #43963, #63825, #5783, #43860, #40161, #15353 ) ) ;
#56874=CARTESIAN_POINT ( 'NONE',  ( 0.2427821522309719648, -0.08942795157527998196, 0.3641732283464567121 ) ) ;
#56877=CARTESIAN_POINT ( 'NONE',  ( 0.7414698162729663755, -0.6692913385826773087, -0.1292274648535924053 ) ) ;
#56879=CARTESIAN_POINT ( 'NONE',  ( -0.5631141337314348183, -4.643576453225290411E-15, -0.3627989612356168347 ) ) ;
#56880=CARTESIAN_POINT ( 'NONE',  ( -0.6167979002624665030, -0.3690944881889765550, -0.3153832671262227771 ) ) ;
#56882=CARTESIAN_POINT ( 'NONE',  ( 1.108923884514436686, -0.3162353388693409650, -0.4822834645669289433 ) ) ;
#56883=CARTESIAN_POINT ( 'NONE',  ( 0.7939632545931766261, -0.08942795157527998196, 0.3641732283464567121 ) ) ;
#56884=CARTESIAN_POINT ( 'NONE',  ( 0.1377952755905518800, 0.1660481256975883668, -0.3530559997133364547 ) ) ;
#56886=CARTESIAN_POINT ( 'NONE',  ( -0.5577427821522301654, -0.3162353388693405765, 0.4822834645669290543 ) ) ;
#56887=CARTESIAN_POINT ( 'NONE',  ( -1.240157480314959759, 0.07958543189024085140, 0.2665933059059887866 ) ) ;
#56888=CARTESIAN_POINT ( 'NONE',  ( -0.3083989501312330295, -0.05778040916215522460, 0.4822834645669289988 ) ) ;
#56889=CARTESIAN_POINT ( 'NONE',  ( -1.604771003085130321, 1.044625174762916719, 0.1466069496707742559 ) ) ;
#56891=ORIENTED_EDGE ( 'NONE', *, *, #47083, .T. ) ;
#56893=CARTESIAN_POINT ( 'NONE',  ( 0.2624671916010504757, 0.2306618581243848609, 0.2411417322834645549 ) ) ;
#56895=CARTESIAN_POINT ( 'NONE',  ( -0.1509186351706028884, -0.05778040916215522460, 0.4822834645669289988 ) ) ;
#56896=CARTESIAN_POINT ( 'NONE',  ( -1.253280839895012377, -0.3162353388693409650, -0.4822834645669289433 ) ) ;
#56897=CARTESIAN_POINT ( 'NONE',  ( 0.6824146981627303710, 0.2306618581243847221, -0.2411417322834647770 ) ) ;
#56898=CARTESIAN_POINT ( 'NONE',  ( 0.006561679790026889343, -0.3162353388693409650, -0.4822834645669289433 ) ) ;
#56900=CARTESIAN_POINT ( 'NONE',  ( -0.9842519685039365918, -0.6692913385826771977, 8.415575281601705876E-17 ) ) ;
#56901=CARTESIAN_POINT ( 'NONE',  ( 0.2034120734908144990, -0.6692913385826771977, 0.1292274648535927661 ) ) ;
#56902=CARTESIAN_POINT ( 'NONE',  ( -0.3477690288713902178, 0.2952755905511810774, -0.1292274648535930714 ) ) ;
#56903=CARTESIAN_POINT ( 'NONE',  ( 0.3149606299212606708, -0.1870078740157480601, -0.3641732283464567677 ) ) ;
#56905=CARTESIAN_POINT ( 'NONE',  ( -0.1574803149606292529, -0.1870078740157479769, 0.4822834645669291653 ) ) ;
#56907=CARTESIAN_POINT ( 'NONE',  ( 1.601049868766404982, 0.2306618581243848609, 0.2411417322834645549 ) ) ;
#56910=ORIENTED_EDGE ( 'NONE', *, *, #34100, .T. ) ;
#56911=CARTESIAN_POINT ( 'NONE',  ( 0.3937007874015754361, -0.1870078740157479769, 0.4822834645669291653 ) ) ;
#56912=CARTESIAN_POINT ( 'NONE',  ( -0.05905511811023545637, -0.4536011799217368745, -0.2665933059059886201 ) ) ;
#56913=CARTESIAN_POINT ( 'NONE',  ( 1.253280839895013710, -0.08942795157528024563, -0.3641732283464568787 ) ) ;
#56916=CARTESIAN_POINT ( 'NONE',  ( 0.4889872687189469880, 1.535433070866141225, 0.000000000000000000 ) ) ;
#56920=CARTESIAN_POINT ( 'NONE',  ( 0.2624671916010504757, -0.6046776061558809534, -0.2411417322834644161 ) ) ;
#56921=CARTESIAN_POINT ( 'NONE',  ( -1.128608923884513837, 0.2306618581243847221, -0.2411417322834647770 ) ) ;
#56923=CARTESIAN_POINT ( 'NONE',  ( -0.9776902887139098386, -0.6692913385826771977, 0.1292274648535927661 ) ) ;
#56924=CARTESIAN_POINT ( 'NONE',  ( 0.09842519685039434474, -0.5400638737290845981, -0.3530559997133363437 ) ) ;
#56925=CARTESIAN_POINT ( 'NONE',  ( 0.8661417322834652488, -0.1870078740157480879, -0.4822834645669291653 ) ) ;
#56926=CARTESIAN_POINT ( 'NONE',  ( 1.318897637795276356, -0.4536011799217367080, 0.2665933059059888421 ) ) ;
#56927=CARTESIAN_POINT ( 'NONE',  ( 1.003937007874016407, -0.4536011799217367080, 0.2665933059059888421 ) ) ;
#56928=CARTESIAN_POINT ( 'NONE',  ( -1.062992125984250968, -0.6692913385826771977, 8.415575281601705876E-17 ) ) ;
#56930=CARTESIAN_POINT ( 'NONE',  ( 1.587926509186352586, -0.4281496062992127816, -0.4176697321401328100 ) ) ;
#56932=CARTESIAN_POINT ( 'NONE',  ( 1.240157480314961314, 0.1660481256975883668, -0.3530559997133364547 ) ) ;
#56934=CARTESIAN_POINT ( 'NONE',  ( -1.686351706036744558, 0.1771653543307087075, -0.09757992244046823083 ) ) ;
#56935=CARTESIAN_POINT ( 'NONE',  ( 0.1640419947506569498, -0.3162353388693409650, -0.4822834645669289433 ) ) ;
#56936=CARTESIAN_POINT ( 'NONE',  ( 0.7677165354330716118, -0.4536011799217367080, 0.2665933059059888421 ) ) ;
#56937=CARTESIAN_POINT ( 'NONE',  ( -1.456692913385826182, -0.5511811023622047445, 6.969142054262312111E-17 ) ) ;
#56938=CARTESIAN_POINT ( 'NONE',  ( 1.122047244094488860, -0.5400638737290845981, -0.3530559997133363437 ) ) ;
#56940=CARTESIAN_POINT ( 'NONE',  ( -0.5446194225721777693, -0.2845877964562161244, -0.3641732283464567121 ) ) ;
#56941=CARTESIAN_POINT ( 'NONE',  ( -0.7349081364829390672, 0.2306618581243847221, -0.2411417322834647770 ) ) ;
#56942=CARTESIAN_POINT ( 'NONE',  ( 1.528871391076116026, 0.2952755905511811885, 0.1292274648535926551 ) ) ;
#56943=CARTESIAN_POINT ( 'NONE',  ( -1.200787401574802349, 0.1660481256975883668, -0.3530559997133364547 ) ) ;
#56944=CARTESIAN_POINT ( 'NONE',  ( 1.312335958005250269, -0.6046776061558807314, 0.2411417322834647770 ) ) ;
#56946=CARTESIAN_POINT ( 'NONE',  ( -1.259842519685038686, -0.1870078740157480601, -0.3641732283464567677 ) ) ;
#56948=CARTESIAN_POINT ( 'NONE',  ( 0.7874015748031503170, -0.1870078740157479769, 0.4822834645669291653 ) ) ;
#56950=CARTESIAN_POINT ( 'NONE',  ( -1.646981627296586703, -0.3162353388693409650, -0.4822834645669289433 ) ) ;
#56951=CARTESIAN_POINT ( 'NONE',  ( 1.660104986876641320, -0.05778040916215522460, 0.4822834645669289988 ) ) ;
#56952=CARTESIAN_POINT ( 'NONE',  ( -1.187664041994750175, -0.08942795157528024563, -0.3641732283464568787 ) ) ;
#56953=CARTESIAN_POINT ( 'NONE',  ( 1.515748031496063408, 0.07958543189024085140, 0.2665933059059887866 ) ) ;
#56954=CARTESIAN_POINT ( 'NONE',  ( -0.5446194225721777693, -0.05778040916215522460, 0.4822834645669289988 ) ) ;
#56955=CARTESIAN_POINT ( 'NONE',  ( 0.1574803149606306130, -0.1870078740157480601, -0.3641732283464567677 ) ) ;
#56956=CARTESIAN_POINT ( 'NONE',  ( -1.548556430446193399, 0.1283753931104748280, 0.1820866141732283561 ) ) ;
#56957=CARTESIAN_POINT ( 'NONE',  ( 1.272965879265092637, -0.004921259842519576551, 0.3153832671262227771 ) ) ;
#56958=CARTESIAN_POINT ( 'NONE',  ( 0.8005249343832028242, -0.4281496062992127816, -0.4176697321401328100 ) ) ;
#56959=CARTESIAN_POINT ( 'NONE',  ( 1.469816272965879911, 0.2306618581243847221, -0.2411417322834647770 ) ) ;
#56960=CARTESIAN_POINT ( 'NONE',  ( 0.1837270341207357105, -0.5023911411419708095, -0.1820866141732282451 ) ) ;
#56961=CARTESIAN_POINT ( 'NONE',  ( 0.2952755905511819101, 0.1660481256975883668, -0.3530559997133364547 ) ) ;
#56962=CARTESIAN_POINT ( 'NONE',  ( 1.122047244094488860, 0.07958543189024085140, 0.2665933059059887866 ) ) ;
#56963=ORIENTED_EDGE ( 'NONE', *, *, #28027, .T. ) ;
#56964=CARTESIAN_POINT ( 'NONE',  ( -1.469816272965878357, 0.2306618581243848609, 0.2411417322834645549 ) ) ;
#56965=CARTESIAN_POINT ( 'NONE',  ( -1.227034120734907141, -0.6692913385826773087, -0.1292274648535924053 ) ) ;
#56966=CARTESIAN_POINT ( 'NONE',  ( -0.07217847769028813698, -0.3162353388693409650, -0.4822834645669289433 ) ) ;
#56969=CARTESIAN_POINT ( 'NONE',  ( 0.4593175853018379162, -0.4281496062992124485, 0.4176697321401328655 ) ) ;
#56970=CARTESIAN_POINT ( 'NONE',  ( 1.030183727034121421, -0.2845877964562161244, -0.3641732283464567121 ) ) ;
#56971=CARTESIAN_POINT ( 'NONE',  ( -0.2690288713910754526, -0.6692913385826771977, 0.1292274648535927661 ) ) ;
#56972=CARTESIAN_POINT ( 'NONE',  ( 0.2624671916010504757, -0.6046776061558809534, -0.2411417322834644161 ) ) ;
#56979=CARTESIAN_POINT ( 'NONE',  ( -0.4265091863517051496, 0.1771653543307087075, -0.09757992244046823083 ) ) ;
#56980=CARTESIAN_POINT ( 'NONE',  ( -0.7808398950131225646, -0.05778040916215522460, 0.4822834645669289988 ) ) ;
#56982=CARTESIAN_POINT ( 'NONE',  ( 0.6955380577427828781, -0.4281496062992124485, 0.4176697321401328655 ) ) ;
#56983=CARTESIAN_POINT ( 'NONE',  ( -1.463254593175852492, 0.2952755905511811885, 0.1292274648535926551 ) ) ;
#56984=CARTESIAN_POINT ( 'NONE',  ( 0.9383202099737536495, -0.3162353388693405765, 0.4822834645669290543 ) ) ;
#56987=CARTESIAN_POINT ( 'NONE',  ( 1.614173228346457378, -0.6692913385826771977, 8.415575281601705876E-17 ) ) ;
#56988=CARTESIAN_POINT ( 'NONE',  ( 0.8923884514435701520, -0.6046776061558809534, -0.2411417322834644161 ) ) ;
#56989=CARTESIAN_POINT ( 'NONE',  ( 0.6167979002624678353, -0.4281496062992124485, 0.4176697321401328655 ) ) ;
#56990=CONICAL_SURFACE ( 'NONE', #15340, 3.582677165354331450, 0.5235987755982945968 ) ;
#56991=CARTESIAN_POINT ( 'NONE',  ( 0.8530183727034126306, -0.004921259842519870586, -0.3153832671262229437 ) ) ;
#56992=CARTESIAN_POINT ( 'NONE',  ( 1.364829396325460076, 0.2306618581243848609, 0.2411417322834645549 ) ) ;
#56995=CARTESIAN_POINT ( 'NONE',  ( 0.9448818897637802916, -0.1870078740157480879, -0.4822834645669291653 ) ) ;
#56996=CARTESIAN_POINT ( 'NONE',  ( 1.620734908136483465, -0.5511811023622046335, 0.09757992244046803654 ) ) ;
#56997=CARTESIAN_POINT ( 'NONE',  ( -0.4330708661417315697, 0.2952755905511811885, 0.000000000000000000 ) ) ;
#56998=CARTESIAN_POINT ( 'NONE',  ( -1.181102362204723644, -0.1870078740157480879, -0.4822834645669291653 ) ) ;
#56999=CARTESIAN_POINT ( 'NONE',  ( 1.049868766404200127, -0.6046776061558809534, -0.2411417322834644161 ) ) ;
#57007=CARTESIAN_POINT ( 'NONE',  ( -0.05249343832020910566, 0.1539470093639523085, 0.1968503937007873850 ) ) ;
#57008=CARTESIAN_POINT ( 'NONE',  ( 1.325459317585302665, -0.004921259842519870586, -0.3153832671262229437 ) ) ;
#57010=CARTESIAN_POINT ( 'NONE',  ( 1.338582677165355062, -0.1870078740157479769, 0.3641732283464567677 ) ) ;
#57016=CARTESIAN_POINT ( 'NONE',  ( -0.6889763779527552368, 0.07958543189024085140, 0.2665933059059887866 ) ) ;
#57017=CARTESIAN_POINT ( 'NONE',  ( -1.666666666666665853, -0.004921259842519870586, -0.3153832671262229437 ) ) ;
#57018=CARTESIAN_POINT ( 'NONE',  ( -1.312335958005248715, 0.2306618581243848609, 0.2411417322834645549 ) ) ;
#57019=CARTESIAN_POINT ( 'NONE',  ( -0.06561679790026180015, -0.4281496062992127816, -0.4176697321401328100 ) ) ;
#57020=CARTESIAN_POINT ( 'NONE',  ( 1.456692913385827515, 0.2952755905511811885, 0.000000000000000000 ) ) ;
#57021=ORIENTED_EDGE ( 'NONE', *, *, #66513, .F. ) ;
#57022=CARTESIAN_POINT ( 'NONE',  ( 1.581364829396326277, -0.05778040916215522460, 0.4822834645669289988 ) ) ;
#57023=CARTESIAN_POINT ( 'NONE',  ( 1.089942661822472569, 9.906153642143428645E-17, -0.3464511005275205946 ) ) ;
#57027=CARTESIAN_POINT ( 'NONE',  ( -0.4133858267716528645, -0.4536011799217367080, 0.2665933059059888421 ) ) ;
#57028=CARTESIAN_POINT ( 'NONE',  ( -1.174540682414697335, -0.05778040916215522460, 0.4822834645669289988 ) ) ;
#57029=CARTESIAN_POINT ( 'NONE',  ( 1.003937007874016407, -0.5400638737290844871, 0.3530559997133364547 ) ) ;
#57030=ORIENTED_EDGE ( 'NONE', *, *, #29559, .F. ) ;
#57031=CARTESIAN_POINT ( 'NONE',  ( 1.220472440944881942, 0.000000000000000000, -0.5309055118110238558 ) ) ;
#57033=CARTESIAN_POINT ( 'NONE',  ( 1.410761154855643795, -0.05778040916215560624, -0.4822834645669293319 ) ) ;
#57034=CARTESIAN_POINT ( 'NONE',  ( -1.338582677165353729, -0.1870078740157480879, -0.4822834645669291653 ) ) ;
#57036=CARTESIAN_POINT ( 'NONE',  ( -0.2821522309711278487, 0.1771653543307087630, 0.09757992244046791164 ) ) ;
#57039=CARTESIAN_POINT ( 'NONE',  ( -0.6824146981627288167, 0.1283753931104748280, 0.1820866141732283561 ) ) ;
#57040=CARTESIAN_POINT ( 'NONE',  ( 0.3412073490813655186, 0.1283753931104748280, 0.1820866141732283561 ) ) ;
#57041=CARTESIAN_POINT ( 'NONE',  ( 0.3149606299212603933, -0.1870078740157479769, 0.4822834645669291653 ) ) ;
#57042=CARTESIAN_POINT ( 'NONE',  ( -0.7808398950131222316, -0.2845877964562161244, -0.3641732283464567121 ) ) ;
#57044=CARTESIAN_POINT ( 'NONE',  ( 1.351706036745407458, -0.4281496062992127816, -0.4176697321401328100 ) ) ;
#57045=CARTESIAN_POINT ( 'NONE',  ( -0.9383202099737524282, -0.3162353388693409650, -0.4822834645669289433 ) ) ;
#57047=CARTESIAN_POINT ( 'NONE',  ( -0.2624671916010490880, 0.2306618581243847221, -0.2411417322834647770 ) ) ;
#57048=CARTESIAN_POINT ( 'NONE',  ( -0.8661417322834640276, -0.1870078740157479769, 0.4822834645669291653 ) ) ;
#57049=CARTESIAN_POINT ( 'NONE',  ( 1.167979002624672580, -0.3690944881889763329, 0.3153832671262228327 ) ) ;
#57051=CARTESIAN_POINT ( 'NONE',  ( -0.2230971128608915943, -0.3690944881889765550, -0.3153832671262227771 ) ) ;
#57052=CARTESIAN_POINT ( 'NONE',  ( -0.6824146981627291497, -0.6046776061558809534, -0.2411417322834644161 ) ) ;
#57053=CARTESIAN_POINT ( 'NONE',  ( -1.062992125984250968, -0.6692913385826771977, 8.415575281601705876E-17 ) ) ;
#57054=CARTESIAN_POINT ( 'NONE',  ( -0.7137454485294952855, 2.362204724409448620, 0.4917280318828573527 ) ) ;
#57055=CARTESIAN_POINT ( 'NONE',  ( 1.456692913385827515, -0.5511811023622047445, 6.969142054262312111E-17 ) ) ;
#57056=CARTESIAN_POINT ( 'NONE',  ( -0.1706036745406816491, 0.05413385826771626580, -0.4176697321401330321 ) ) ;
#57057=CARTESIAN_POINT ( 'NONE',  ( -1.174540682414697335, -0.3162353388693409650, -0.4822834645669289433 ) ) ;
#57058=ORIENTED_EDGE ( 'NONE', *, *, #50024, .T. ) ;
#57060=CARTESIAN_POINT ( 'NONE',  ( 1.325459317585302665, 0.05413385826771626580, -0.4176697321401330321 ) ) ;
#57061=CARTESIAN_POINT ( 'NONE',  ( -0.5905511811023615998, 0.1771653543307087630, 0.000000000000000000 ) ) ;
#57063=CARTESIAN_POINT ( 'NONE',  ( -0.9711286089238838626, -0.6046776061558807314, 0.2411417322834647770 ) ) ;
#57064=CARTESIAN_POINT ( 'NONE',  ( 1.312335958005250269, -0.6046776061558807314, 0.2411417322834647770 ) ) ;
#57065=CARTESIAN_POINT ( 'NONE',  ( 1.049868766404200349, 0.2306618581243848609, 0.2411417322834645549 ) ) ;
#57067=CARTESIAN_POINT ( 'NONE',  ( -1.279527559055116948, -0.4536011799217367080, 0.2665933059059888421 ) ) ;
#57072=CARTESIAN_POINT ( 'NONE',  ( 1.259842519685040019, -0.1870078740157480601, -0.3641732283464567677 ) ) ;
#57073=CARTESIAN_POINT ( 'NONE',  ( 0.7611548556430451917, -0.5023911411419708095, 0.1820866141732285504 ) ) ;
#57074=CARTESIAN_POINT ( 'NONE',  ( 0.4330708661417329575, -0.6692913385826771977, 8.415575281601705876E-17 ) ) ;
#57077=CARTESIAN_POINT ( 'NONE',  ( 0.9317585301837276734, -0.004921259842519870586, -0.3153832671262229437 ) ) ;
#57078=CARTESIAN_POINT ( 'NONE',  ( -0.2165354330708654795, 0.1660481256975885056, 0.3530559997133364547 ) ) ;
#57079=CARTESIAN_POINT ( 'NONE',  ( -1.266404199475064773, -0.05778040916215560624, -0.4822834645669293319 ) ) ;
#57080=CARTESIAN_POINT ( 'NONE',  ( 1.023622047244095334, -0.1870078740157479769, 0.4822834645669291653 ) ) ;
#57082=CARTESIAN_POINT ( 'NONE',  ( -0.7758157084527474989, 0.02791078216816064370, 0.4328096321851915285 ) ) ;
#57085=CARTESIAN_POINT ( 'NONE',  ( -0.7874015748031489847, -0.1870078740157479769, 0.4822834645669291653 ) ) ;
#57086=CARTESIAN_POINT ( 'NONE',  ( -0.6233595800524928121, -0.3162353388693409650, -0.4822834645669289433 ) ) ;
#57087=CARTESIAN_POINT ( 'NONE',  ( -0.9776902887139098386, 0.1771653543307087075, -0.09757992244046823083 ) ) ;
#57088=CARTESIAN_POINT ( 'NONE',  ( -0.6036745406824141069, -0.6046776061558809534, -0.2411417322834644161 ) ) ;
#57089=CARTESIAN_POINT ( 'NONE',  ( 0.2493438320209980519, 0.05413385826771666132, 0.4176697321401328100 ) ) ;
#57090=CARTESIAN_POINT ( 'NONE',  ( -0.5577427821522301654, -0.3162353388693405765, 0.4822834645669290543 ) ) ;
#57091=CARTESIAN_POINT ( 'NONE',  ( -1.404199475065615932, -0.4281496062992127816, -0.4176697321401328100 ) ) ;
#57092=CARTESIAN_POINT ( 'NONE',  ( -0.7808398950131225646, -0.05778040916215522460, 0.4822834645669289988 ) ) ;
#57093=CARTESIAN_POINT ( 'NONE',  ( 0.7808398950131240079, -0.3162353388693405765, 0.4822834645669290543 ) ) ;
#57096=CARTESIAN_POINT ( 'NONE',  ( -0.8923884514435688198, -0.5023911411419708095, 0.1820866141732285504 ) ) ;
#57100=CARTESIAN_POINT ( 'NONE',  ( -1.312335958005248715, -0.5023911411419708095, -0.1820866141732282451 ) ) ;
#57101=CARTESIAN_POINT ( 'NONE',  ( -0.8858267716535425107, -0.5400638737290844871, 0.3530559997133364547 ) ) ;
#57102=CARTESIAN_POINT ( 'NONE',  ( -0.6758530183727028406, 0.2952755905511811885, 0.1292274648535926551 ) ) ;
#57104=CARTESIAN_POINT ( 'NONE',  ( -0.9711286089238838626, -0.6046776061558807314, 0.2411417322834647770 ) ) ;
#57105=CARTESIAN_POINT ( 'NONE',  ( -1.332020997375327642, -0.3162353388693409650, -0.4822834645669289433 ) ) ;
#57107=CARTESIAN_POINT ( 'NONE',  ( -1.666666666666665853, 0.05413385826771626580, -0.4176697321401330321 ) ) ;
#57109=CARTESIAN_POINT ( 'NONE',  ( 0.3477690288713918276, -0.5511811023622048555, -0.09757992244046775898 ) ) ;
#57112=CARTESIAN_POINT ( 'NONE',  ( 0.1574803149606306130, -0.1870078740157479769, 0.3641732283464567677 ) ) ;
#57113=CARTESIAN_POINT ( 'NONE',  ( -0.3805774278215216522, 0.05413385826771666132, 0.4176697321401328100 ) ) ;
#57114=CARTESIAN_POINT ( 'NONE',  ( 1.181102362204724976, -0.1870078740157480879, -0.4822834645669291653 ) ) ;
#57115=CARTESIAN_POINT ( 'NONE',  ( -0.2887139107611542133, -0.6046776061558809534, -0.2411417322834644161 ) ) ;
#57116=ORIENTED_EDGE ( 'NONE', *, *, #81979, .F. ) ;
#57117=CARTESIAN_POINT ( 'NONE',  ( -0.8070866141732276899, 0.1012011053420775880, -0.2882089793578256898 ) ) ;
#57120=CARTESIAN_POINT ( 'NONE',  ( -0.7611548556430438595, -0.6046776061558809534, -0.2411417322834644161 ) ) ;
#57121=CARTESIAN_POINT ( 'NONE',  ( 1.502624671916010790, -0.3162353388693409650, -0.4822834645669289433 ) ) ;
#57122=CARTESIAN_POINT ( 'NONE',  ( -1.095800524934382292, -0.08942795157527998196, 0.3641732283464567121 ) ) ;
#57123=CARTESIAN_POINT ( 'NONE',  ( -1.437007874015747477, -0.5400638737290844871, 0.3530559997133364547 ) ) ;
#57125=LINE ( 'NONE', #56313, #7575 ) ;
#57127=CARTESIAN_POINT ( 'NONE',  ( 1.108923884514436686, -0.3162353388693409650, -0.4822834645669289433 ) ) ;
#57129=CARTESIAN_POINT ( 'NONE',  ( 0.2493438320209980519, 0.05413385826771666132, 0.4176697321401328100 ) ) ;
#57130=CARTESIAN_POINT ( 'NONE',  ( -1.115485564304461219, -0.004921259842519870586, -0.3153832671262229437 ) ) ;
#57131=CARTESIAN_POINT ( 'NONE',  ( -0.1771653543307080136, -0.5400638737290844871, 0.3530559997133364547 ) ) ;
#57133=CARTESIAN_POINT ( 'NONE',  ( -0.6758530183727028406, -0.6692913385826773087, -0.1292274648535924053 ) ) ;
#57134=CARTESIAN_POINT ( 'NONE',  ( -0.9580052493438311334, -0.4281496062992124485, 0.4176697321401328655 ) ) ;
#57136=CARTESIAN_POINT ( 'NONE',  ( 0.7480314960629927956, -0.5511811023622047445, 6.969142054262312111E-17 ) ) ;
#57137=CARTESIAN_POINT ( 'NONE',  ( -0.2821522309711278487, 0.1771653543307087630, 0.09757992244046791164 ) ) ;
#57138=CARTESIAN_POINT ( 'NONE',  ( 0.6889763779527566800, -0.4536011799217367080, 0.2665933059059888421 ) ) ;
#57139=CARTESIAN_POINT ( 'NONE',  ( -1.535433070866141225, 0.2952755905511811885, 0.000000000000000000 ) ) ;
#57140=CARTESIAN_POINT ( 'NONE',  ( 1.535433070866142335, -0.6692913385826771977, 8.415575281601705876E-17 ) ) ;
#57141=CARTESIAN_POINT ( 'NONE',  ( 0.4790026246719168435, -0.2845877964562161244, -0.3641732283464567121 ) ) ;
#57142=CARTESIAN_POINT ( 'NONE',  ( -0.6627296587926501115, 0.2952755905511810774, -0.1292274648535930714 ) ) ;
#57143=CARTESIAN_POINT ( 'NONE',  ( 1.450131233595801428, 0.2952755905511811885, 0.1292274648535926551 ) ) ;
#57145=CARTESIAN_POINT ( 'NONE',  ( -0.1509186351706028884, -0.2845877964562161244, -0.3641732283464567121 ) ) ;
#57146=CARTESIAN_POINT ( 'NONE',  ( 0.03280839895013198948, 0.2952755905511811885, 0.1292274648535926551 ) ) ;
#57147=CARTESIAN_POINT ( 'NONE',  ( 0.5052493438320218022, -0.6692913385826773087, -0.1292274648535924053 ) ) ;
#57149=CARTESIAN_POINT ( 'NONE',  ( 1.443569553805774897, 0.1283753931104748280, 0.1820866141732283561 ) ) ;
#57150=CARTESIAN_POINT ( 'NONE',  ( 0.1312335958005255154, -0.5023911411419708095, 0.1820866141732285504 ) ) ;
#57151=CARTESIAN_POINT ( 'NONE',  ( -1.384514435695537005, 0.2952755905511811885, 0.1292274648535926551 ) ) ;
#57152=CARTESIAN_POINT ( 'NONE',  ( -0.5446194225721777693, -0.08942795157527998196, 0.3641732283464567121 ) ) ;
#57153=CARTESIAN_POINT ( 'NONE',  ( 1.035555078613326518, 5.982513598207969926E-16, 0.3627989612356145033 ) ) ;
#57154=CARTESIAN_POINT ( 'NONE',  ( -0.9514435695538050464, -0.3162353388693405765, 0.4822834645669290543 ) ) ;
#57155=CARTESIAN_POINT ( 'NONE',  ( -0.6036745406824141069, -0.6046776061558809534, -0.2411417322834644161 ) ) ;
#57158=CARTESIAN_POINT ( 'NONE',  ( 0.7086614173228352742, -0.1870078740157480601, -0.3641732283464567677 ) ) ;
#57159=CARTESIAN_POINT ( 'NONE',  ( -0.5577427821522301654, -0.3162353388693405765, 0.4822834645669290543 ) ) ;
#57161=CARTESIAN_POINT ( 'NONE',  ( -0.6824146981627288167, 0.2306618581243848609, 0.2411417322834645549 ) ) ;
#57162=CARTESIAN_POINT ( 'NONE',  ( -0.6955380577427815458, -0.004921259842519576551, 0.3153832671262227771 ) ) ;
#57164=CARTESIAN_POINT ( 'NONE',  ( -0.2624671916010490880, -0.6046776061558807314, 0.2411417322834647770 ) ) ;
#57165=DIRECTION ( 'NONE',  ( 1.000000000000000000, 3.096699300667737957E-16, -1.692413147294446216E-16 ) ) ;
#57166=CARTESIAN_POINT ( 'NONE',  ( 1.391076115485564868, -0.6046776061558807314, 0.2411417322834647770 ) ) ;
#57169=ORIENTED_EDGE ( 'NONE', *, *, #34817, .F. ) ;
#57171=CARTESIAN_POINT ( 'NONE',  ( -1.286089238845143479, -0.6046776061558807314, 0.2411417322834647770 ) ) ;
#57172=CARTESIAN_POINT ( 'NONE',  ( -0.7939632545931754048, -0.3162353388693405765, 0.4822834645669290543 ) ) ;
#57173=CARTESIAN_POINT ( 'NONE',  ( 1.463254593175853824, 0.2952755905511810774, -0.1292274648535930714 ) ) ;
#57176=CARTESIAN_POINT ( 'NONE',  ( 1.148293963254593875, -0.6692913385826771977, 0.1292274648535927661 ) ) ;
#57177=CARTESIAN_POINT ( 'NONE',  ( 0.05249343832021075018, -0.6046776061558807314, 0.2411417322834647770 ) ) ;
#57180=CARTESIAN_POINT ( 'NONE',  ( 1.194225721784777594, -0.3690944881889765550, -0.3153832671262227771 ) ) ;
#57182=ORIENTED_EDGE ( 'NONE', *, *, #10455, .F. ) ;
#57185=CARTESIAN_POINT ( 'NONE',  ( 0.4790026246719167324, -0.05778040916215522460, 0.4822834645669289988 ) ) ;
#57186=CARTESIAN_POINT ( 'NONE',  ( -0.8792650918635160906, 0.05413385826771626580, -0.4176697321401330321 ) ) ;
#57187=CARTESIAN_POINT ( 'NONE',  ( -1.345144356955379816, -0.3162353388693405765, 0.4822834645669290543 ) ) ;
#57188=CARTESIAN_POINT ( 'NONE',  ( 0.6758530183727039509, -0.6692913385826771977, 0.1292274648535927661 ) ) ;
#57189=CARTESIAN_POINT ( 'NONE',  ( 1.660104986876641320, -0.05778040916215522460, 0.4822834645669289988 ) ) ;
#57190=CARTESIAN_POINT ( 'NONE',  ( 1.528871391076116026, -0.6692913385826773087, -0.1292274648535924053 ) ) ;
#57191=CARTESIAN_POINT ( 'NONE',  ( -0.2821522309711278487, -0.6692913385826773087, -0.1292274648535924053 ) ) ;
#57192=CARTESIAN_POINT ( 'NONE',  ( -1.108923884514435132, -0.05778040916215560624, -0.4822834645669293319 ) ) ;
#57193=CARTESIAN_POINT ( 'NONE',  ( 1.561679790026247350, -0.4281496062992124485, 0.4176697321401328655 ) ) ;
#57194=CARTESIAN_POINT ( 'NONE',  ( 1.496062992125985147, -0.1870078740157479769, 0.4822834645669291653 ) ) ;
#57196=CARTESIAN_POINT ( 'NONE',  ( 1.017060367454068803, -0.2845877964562159024, 0.3641732283464567677 ) ) ;
#57199=ORIENTED_EDGE ( 'NONE', *, *, #23584, .F. ) ;
#57200=CARTESIAN_POINT ( 'NONE',  ( 0.05905511811023681640, 0.07958543189024071263, -0.2665933059059888421 ) ) ;
#57203=CARTESIAN_POINT ( 'NONE',  ( 0.1443569553805781891, -0.4281496062992124485, 0.4176697321401328655 ) ) ;
#57204=CARTESIAN_POINT ( 'NONE',  ( 0.3280839895013130669, 0.05413385826771666132, 0.4176697321401328100 ) ) ;
#57205=CARTESIAN_POINT ( 'NONE',  ( -0.6824146981627291497, -0.6046776061558809534, -0.2411417322834644161 ) ) ;
#57207=CARTESIAN_POINT ( 'NONE',  ( -1.325459317585300889, 0.05413385826771666132, 0.4176697321401328100 ) ) ;
#57209=CARTESIAN_POINT ( 'NONE',  ( 1.391076115485564868, -0.5023911411419708095, 0.1820866141732285504 ) ) ;
#57210=CARTESIAN_POINT ( 'NONE',  ( 0.8202099737532814183, -0.6692913385826773087, -0.1292274648535924053 ) ) ;
#57211=CARTESIAN_POINT ( 'NONE',  ( 0.6036745406824154392, 0.2306618581243847221, -0.2411417322834647770 ) ) ;
#57213=CARTESIAN_POINT ( 'NONE',  ( -1.437007874015747477, -0.5400638737290844871, 0.3530559997133364547 ) ) ;
#57216=CARTESIAN_POINT ( 'NONE',  ( -0.2099737532808391705, -0.6046776061558809534, -0.2411417322834644161 ) ) ;
#57219=CARTESIAN_POINT ( 'NONE',  ( 1.141732283464567566, 0.2952755905511811885, 0.000000000000000000 ) ) ;
#57221=CARTESIAN_POINT ( 'NONE',  ( 1.305774278215223960, -0.6692913385826771977, 0.1292274648535927661 ) ) ;
#57222=CARTESIAN_POINT ( 'NONE',  ( 0.1312335958005257930, 0.1283753931104746893, -0.1820866141732285504 ) ) ;
#57223=CARTESIAN_POINT ( 'NONE',  ( 0.8005249343832027131, 0.05413385826771666132, 0.4176697321401328100 ) ) ;
#57225=CARTESIAN_POINT ( 'NONE',  ( 0.3215223097112867578, -0.2845877964562161244, -0.3641732283464567121 ) ) ;
#57226=CARTESIAN_POINT ( 'NONE',  ( 0.2165354330708668673, 0.1660481256975883668, -0.3530559997133364547 ) ) ;
#57228=CARTESIAN_POINT ( 'NONE',  ( -1.332020997375327642, -0.3162353388693409650, -0.4822834645669289433 ) ) ;
#57229=CARTESIAN_POINT ( 'NONE',  ( 0.9776902887139113929, 0.1771653543307087630, 0.09757992244046791164 ) ) ;
#57230=CARTESIAN_POINT ( 'NONE',  ( -0.2427821522309703550, -0.05778040916215560624, -0.4822834645669293319 ) ) ;
#57231=EDGE_CURVE ( 'NONE', #82979, #50773, #36982, .T. ) ;
#57232=CARTESIAN_POINT ( 'NONE',  ( 0.03937007874015833325, -0.5511811023622047445, 6.969142054262312111E-17 ) ) ;
#57234=CARTESIAN_POINT ( 'NONE',  ( -0.2624671916010490880, 0.2306618581243847221, -0.2411417322834647770 ) ) ;
#57235=CARTESIAN_POINT ( 'NONE',  ( 0.2362204724409456558, -0.1870078740157480601, -0.3641732283464567677 ) ) ;
#57237=CARTESIAN_POINT ( 'NONE',  ( 0.06561679790026316017, -0.4281496062992124485, 0.4176697321401328655 ) ) ;
#57239=CARTESIAN_POINT ( 'NONE',  ( 1.043307086614173818, 0.07958543189024085140, 0.2665933059059887866 ) ) ;
#57240=CARTESIAN_POINT ( 'NONE',  ( -0.1694133573824160299, -1.310289619585134409E-15, -0.3627985898453504054 ) ) ;
#57241=CARTESIAN_POINT ( 'NONE',  ( -0.2755905511811018171, 0.1771653543307087630, 0.000000000000000000 ) ) ;
#57242=CARTESIAN_POINT ( 'NONE',  ( -0.8005249343832013809, -0.3690944881889763329, 0.3153832671262228327 ) ) ;
#57243=CARTESIAN_POINT ( 'NONE',  ( -0.3477690288713902178, 0.2952755905511810774, -0.1292274648535930714 ) ) ;
#57244=CARTESIAN_POINT ( 'NONE',  ( 0.06561679790026316017, 0.05413385826771626580, -0.4176697321401330321 ) ) ;
#57245=CARTESIAN_POINT ( 'NONE',  ( 1.089238845144357759, -0.004921259842519870586, -0.3153832671262229437 ) ) ;
#57247=CARTESIAN_POINT ( 'NONE',  ( 1.574803149606299746, -0.1870078740157479769, 0.3641732283464567677 ) ) ;
#57248=CARTESIAN_POINT ( 'NONE',  ( 0.7611548556430454138, 0.2306618581243847221, -0.2411417322834647770 ) ) ;
#57251=CARTESIAN_POINT ( 'NONE',  ( -0.1706036745406816491, -0.4281496062992124485, 0.4176697321401328655 ) ) ;
#57255=CARTESIAN_POINT ( 'NONE',  ( 1.056430446194226658, 0.2952755905511811885, 0.1292274648535926551 ) ) ;
#57256=AXIS2_PLACEMENT_3D ( 'NONE', #42301, #15839, #61251 ) ;
#57257=CARTESIAN_POINT ( 'NONE',  ( 0.6561679790026253567, -0.6046776061558809534, -0.2411417322834644161 ) ) ;
#57259=CARTESIAN_POINT ( 'NONE',  ( -1.614173228346456712, 2.362204724409448620, -0.1372047244094478091 ) ) ;
#57260=CARTESIAN_POINT ( 'NONE',  ( 0.3805774278215230400, -0.3690944881889763329, 0.3153832671262228327 ) ) ;
#57261=CARTESIAN_POINT ( 'NONE',  ( 1.135170603674541256, -0.6692913385826773087, -0.1292274648535924053 ) ) ;
#57262=CARTESIAN_POINT ( 'NONE',  ( -0.2165354330708654795, -0.4536011799217368745, -0.2665933059059886201 ) ) ;
#57263=CARTESIAN_POINT ( 'NONE',  ( -0.5314960629921250401, 0.1660481256975885056, 0.3530559997133364547 ) ) ;
#57264=CARTESIAN_POINT ( 'NONE',  ( 0.8398950131233602345, 0.2306618581243847221, -0.2411417322834647770 ) ) ;
#57265=CARTESIAN_POINT ( 'NONE',  ( 0.2624671916010504757, -0.6046776061558809534, -0.2411417322834644161 ) ) ;
#57267=CARTESIAN_POINT ( 'NONE',  ( -0.9776902887139098386, 0.2952755905511810774, -0.1292274648535930714 ) ) ;
#57268=CARTESIAN_POINT ( 'NONE',  ( -0.8923884514435688198, 0.1283753931104746893, -0.1820866141732285504 ) ) ;
#57269=CARTESIAN_POINT ( 'NONE',  ( 0.4330708661417329575, -0.6692913385826771977, 8.415575281601705876E-17 ) ) ;
#57270=CARTESIAN_POINT ( 'NONE',  ( -1.318897637795274802, -0.5400638737290845981, -0.3530559997133363437 ) ) ;
#57271=CARTESIAN_POINT ( 'NONE',  ( -0.2296587926509179312, -0.05778040916215522460, 0.4822834645669289988 ) ) ;
#57274=CARTESIAN_POINT ( 'NONE',  ( 1.200787401574803681, -0.5400638737290845981, -0.3530559997133363437 ) ) ;
#57275=CARTESIAN_POINT ( 'NONE',  ( 1.272965879265092637, -0.4281496062992127816, -0.4176697321401328100 ) ) ;
#57277=CARTESIAN_POINT ( 'NONE',  ( -1.476377952755905110, 0.1660481256975885056, 0.3530559997133364547 ) ) ;
#57279=CARTESIAN_POINT ( 'NONE',  ( -1.036745406824146176, 0.05413385826771626580, -0.4176697321401330321 ) ) ;
#57283=CARTESIAN_POINT ( 'NONE',  ( 0.09842519685039434474, 0.07958543189024085140, 0.2665933059059887866 ) ) ;
#57285=CARTESIAN_POINT ( 'NONE',  ( 0.5380577427821529035, 0.05413385826771626580, -0.4176697321401330321 ) ) ;
#57288=CARTESIAN_POINT ( 'NONE',  ( -0.6627296587926501115, 0.1771653543307087075, -0.09757992244046823083 ) ) ;
#57289=CARTESIAN_POINT ( 'NONE',  ( 1.010498687664042716, -0.4281496062992124485, 0.4176697321401328655 ) ) ;
#57290=CARTESIAN_POINT ( 'NONE',  ( 1.056430446194226436, -0.5511811023622048555, -0.09757992244046775898 ) ) ;
#57291=CARTESIAN_POINT ( 'NONE',  ( -0.05249343832020911260, 0.2306618581243848609, 0.2411417322834645549 ) ) ;
#57293=CARTESIAN_POINT ( 'NONE',  ( -0.5774278215223089816, -0.6046776061558807314, 0.2411417322834647770 ) ) ;
#57294=CARTESIAN_POINT ( 'NONE',  ( -1.535433070866141225, 0.1771653543307087630, 0.000000000000000000 ) ) ;
#57295=CARTESIAN_POINT ( 'NONE',  ( -0.3149606299212590610, -0.1870078740157479769, 0.4822834645669291653 ) ) ;
#57296=CARTESIAN_POINT ( 'NONE',  ( 1.568241469816273659, -0.05778040916215560624, -0.4822834645669293319 ) ) ;
#57297=CARTESIAN_POINT ( 'NONE',  ( 0.6399301791983058596, -1.374501131054255944E-15, 0.4445507791589066726 ) ) ;
#57300=CARTESIAN_POINT ( 'NONE',  ( 0.5446194225721792126, -0.3162353388693405765, 0.4822834645669290543 ) ) ;
#57301=ORIENTED_EDGE ( 'NONE', *, *, #25913, .F. ) ;
#57302=CARTESIAN_POINT ( 'NONE',  ( -0.8267716535433065062, -0.6692913385826771977, 8.415575281601705876E-17 ) ) ;
#57303=CARTESIAN_POINT ( 'NONE',  ( -1.259842519685038686, -0.1870078740157480879, -0.4822834645669291653 ) ) ;
#57304=CARTESIAN_POINT ( 'NONE',  ( 0.4921259842519691285, 0.1660481256975885056, 0.3530559997133364547 ) ) ;
#57305=CARTESIAN_POINT ( 'NONE',  ( -0.1509186351706028884, -0.3162353388693409650, -0.4822834645669289433 ) ) ;
#57307=CARTESIAN_POINT ( 'NONE',  ( -0.6430446194225716283, -0.4281496062992124485, 0.4176697321401328655 ) ) ;
#57308=CARTESIAN_POINT ( 'NONE',  ( -0.03937007874015669567, 0.2952755905511811885, 0.000000000000000000 ) ) ;
#57309=CARTESIAN_POINT ( 'NONE',  ( -0.7480314960629914633, -0.6692913385826771977, 8.415575281601705876E-17 ) ) ;
#57310=CARTESIAN_POINT ( 'NONE',  ( -0.2690288713910754526, -0.5511811023622046335, 0.09757992244046803654 ) ) ;
#57312=CARTESIAN_POINT ( 'NONE',  ( 0.006561679790026889343, -0.05778040916215522460, 0.4822834645669289988 ) ) ;
#57315=CARTESIAN_POINT ( 'NONE',  ( 1.154855643044620184, 0.2306618581243847221, -0.2411417322834647770 ) ) ;
#57320=CARTESIAN_POINT ( 'NONE',  ( 0.2952755905511819101, 0.1660481256975883668, -0.3530559997133364547 ) ) ;
#57321=CARTESIAN_POINT ( 'NONE',  ( 0.2427821522309716595, -0.2845877964562161244, -0.3641732283464567121 ) ) ;
#57322=VECTOR ( 'NONE', #52921, 39.37007874015748143 ) ;
#57324=CARTESIAN_POINT ( 'NONE',  ( 1.410761154855643795, -0.08942795157528024563, -0.3641732283464568787 ) ) ;
#57328=CARTESIAN_POINT ( 'NONE',  ( 1.463254593175853824, -0.5511811023622046335, 0.09757992244046803654 ) ) ;
#57329=CARTESIAN_POINT ( 'NONE',  ( 1.601049868766404982, 0.2306618581243848609, 0.2411417322834645549 ) ) ;
#57331=CARTESIAN_POINT ( 'NONE',  ( 0.5446194225721792126, -0.05778040916215560624, -0.4822834645669293319 ) ) ;
#57332=CARTESIAN_POINT ( 'NONE',  ( -1.154855643044618851, 0.2306618581243848609, 0.2411417322834645549 ) ) ;
#57333=CARTESIAN_POINT ( 'NONE',  ( -1.003937007874015297, -0.5400638737290845981, -0.3530559997133363437 ) ) ;
#57334=CARTESIAN_POINT ( 'NONE',  ( 0.4133858267716541968, -0.5400638737290845981, -0.3530559997133363437 ) ) ;
#57335=CARTESIAN_POINT ( 'NONE',  ( 0.8398950131233602345, 0.2306618581243847221, -0.2411417322834647770 ) ) ;
#57336=CARTESIAN_POINT ( 'NONE',  ( 1.351706036745407680, -0.004921259842519576551, 0.3153832671262227771 ) ) ;
#57337=CARTESIAN_POINT ( 'NONE',  ( 0.7742782152230979209, -0.004921259842519870586, -0.3153832671262229437 ) ) ;
#57338=CARTESIAN_POINT ( 'NONE',  ( -0.9055118110236215490, -0.6692913385826771977, 8.415575281601705876E-17 ) ) ;
#57339=B_SPLINE_CURVE_WITH_KNOTS ( 'NONE', 3,
 ( #10367, #61699, #62520, #81898, #9940, #61275, #68841 ),
 .UNSPECIFIED., .F., .F.,
 ( 4, 3, 4 ),
 ( 3.469446951953614189E-17, 0.001246232571205268744, 0.002492492258783276290 ),
 .UNSPECIFIED. ) ;
#57341=CARTESIAN_POINT ( 'NONE',  ( -1.587926509186350810, -0.004921259842519870586, -0.3153832671262229437 ) ) ;
#57343=CARTESIAN_POINT ( 'NONE',  ( 0.7283464566929143125, 0.1660481256975885056, 0.3530559997133364547 ) ) ;
#57345=CARTESIAN_POINT ( 'NONE',  ( -1.404199475065615932, -0.004921259842519576551, 0.3153832671262227771 ) ) ;
#57346=CARTESIAN_POINT ( 'NONE',  ( -0.07217847769028787330, -0.05778040916215522460, 0.4822834645669289988 ) ) ;
#57347=CARTESIAN_POINT ( 'NONE',  ( 0.8267716535433077274, 0.1771653543307087630, 0.000000000000000000 ) ) ;
#57348=CARTESIAN_POINT ( 'NONE',  ( 0.9973753280839902091, -0.6046776061558807314, 0.2411417322834647770 ) ) ;
#57350=CARTESIAN_POINT ( 'NONE',  ( -0.6102362204724400829, 0.07958543189024085140, 0.2665933059059887866 ) ) ;
#57351=CARTESIAN_POINT ( 'NONE',  ( -0.4396325459317579898, 0.2952755905511811885, 0.1292274648535926551 ) ) ;
#57352=CARTESIAN_POINT ( 'NONE',  ( -1.627296587926508442, 0.1283753931104748280, 0.1820866141732283561 ) ) ;
#57353=CARTESIAN_POINT ( 'NONE',  ( -0.9514435695538050464, -0.3162353388693405765, 0.4822834645669290543 ) ) ;
#57354=CARTESIAN_POINT ( 'NONE',  ( 1.062992125984252745, 0.2952755905511811885, 0.000000000000000000 ) ) ;
#57356=CARTESIAN_POINT ( 'NONE',  ( -1.482939632545930975, -0.004921259842519576551, 0.3153832671262227771 ) ) ;
#57357=EDGE_CURVE ( 'NONE', #46955, #79849, #56186, .T. ) ;
#57359=CARTESIAN_POINT ( 'NONE',  ( 1.056430446194226436, -0.6692913385826773087, -0.1292274648535924053 ) ) ;
#57362=CARTESIAN_POINT ( 'NONE',  ( 1.679790026246720025, 0.2306618581243848609, 0.2411417322834645549 ) ) ;
#57363=CARTESIAN_POINT ( 'NONE',  ( -0.8398950131233589023, -0.5023911411419708095, -0.1820866141732282451 ) ) ;
#57364=B_SPLINE_CURVE_WITH_KNOTS ( 'NONE', 3,
 ( #1881, #71750, #58692, #14524 ),
 .UNSPECIFIED., .F., .F.,
 ( 4, 4 ),
 ( 1.027584591209733963E-14, 0.001730108991789992097 ),
 .UNSPECIFIED. ) ;
#57365=( BOUNDED_SURFACE ( )  B_SPLINE_SURFACE ( 1, 2, ( 
 ( #20332, #14863, #71680, #8543, #14032, #59872, #7715, #33383, #34209, #13609, #20754, #59046, #64945, #46404, #72098, #72925, #40938, #14456, #33794, #53551, #27472, #66617, #8955, #34629, #60293, #2643, #7285, #75006, #68280, #11017, #42579, #36674, #4688, #81321, #49305, #60702, #74177, #35869, #15696, #41353, #67034, #22818, #55610, #4284, #16938, #54799, #16523, #3051, #61535, #29946, #30361, #9366, #35037, #28717, #16104, #22411, #23634, #3880, #61114, #36272, #3466, #54380, #62350, #79674, #23223, #17353, #42981, #80090, #55202, #48067, #80910, #73770, #61943, #41749, #67444, #48893, #21991, #29132, #9777, #47652, #73348, #68676, #74594, #29539, #35449, #10615, #80502, #48475, #42168, #67863, #10200, #69902, #76639, #64422, #12669, #25691, #12256, #57255, #56029, #38746, #24046, #30778, #31181, #45040, #37091, #56439, #82142, #24457, #5111, #62777, #50123, #70314, #37913, #82956, #44619, #75822, #18164, #38329, #18569, #18970, #25274, #43796, #31597, #64003, #6344, #63590, #44212, #69501, #32016, #37503, #24862, #56846, #50942, #63178, #57676, #11436, #11850, #51352, #38, #77055, #19388, #5925, #5516, #70740, #82544, #50530, #13093, #81737, #6757, #49717, #75413, #76235, #17757, #43387, #69088, #32851, #72416, #58520, #64842, #1712, #66518, #39585, #885, #15176, #32429, #21477, #27367, #65699, #79160, #8029, #72826, #40833, #65274, #7612, #26952, #46305, #53028, #58092, #14765, #2124, #71999, #33692, #457, #26113, #51774, #7180, #33284, #47135, #13501, #26543, #52196, #77900, #20231, #39157, #45879, #46724, #14354, #59353, #21065, #71577, #13928, #40421, #78321, #78741, #66102, #58945, #8438, #34108, #59769, #40012, #20652, #1303, #27791, #52615, #53452, #77478, #19814, #45463, #71161, #47553, #34943, #61845, #10100, #10518, #2544, #41658, #67349, #36172, #29849, #41253, #9272, #16840, #9682, #74077, #29444, #4186, #55512, #73245, #3781, #81220, #80812, #23536, #55103, #49205, #17255, #74907, #42883, #15594, #3366, #48378, #28202, #53861, #79573, #35353, #68177, #42474, #23127, #61015, #29030, #66940, #16423, #8850, #34529, #21889, #60606, #2955, #28620, #54278, #60193, #67764, #54699, #80407, #42069, #22719, #79994, #22308, #47969, #73670, #16012, #35764, #48795, #61432, #74493, #82859, #36576, #18876, #11758, #56752, #37413, #50030, #25180, #4591, #62255, #69812, #63085, #82047, #83269, #30262, #55926, #81641, #82452, #36995, #76548, #24767, #31085, #75727, #23950, #5016, #18067, #12161, #43701, #57578, #5827, #75312, #49618, #50435, #30685, #11336, #68987, #24360, #17659, #43290, #62675, #44525, #70213, #12569, #25592, #31916, #38227, #63904, #5423, #69405, #6240, #51255, #37817, #76137, #68578, #63493, #18478, #56346, #44120, #31500, #76957, #57159, #19285, #50848, #10919, #7081, #32752, #78221, #52930, #20554, #65597, #22103, #26014, #77801, #46206, #65173, #44936, #19707, #357, #64323, #80204, #77375, #47763, #57993, #58419, #27269, #64743, #51672, #39910, #3165, #70633, #41462, #52513, #35149, #33591, #7509, #15812, #73461, #79787, #45365, #67146, #71900, #1204, #26854, #71061, #26440, #13405, #39060, #778, #12990, #9476, #58846, #52092, #20133, #60813, #28829, #45781, #71480, #54493, #13827, #14251, #7930, #38645, #6659, #39486, #59256, #32331, #1613, #33178, #68793, #62890, #30889, #24164, #75532, #3580, #17053, #62061, #41866, #67560, #9893, #49010, #81852, #30483, #43097, #81027, #42694, #29247, #4400, #56149, #56557, #35563, #61227, #54911, #42277, #48594, #49833, #30067, #3993, #62472, #29657, #80617, #5226, #22521, #49426, #17872, #69206, #22929, #81438, #74291, #23753, #16636, #4807, #67974, #10317, #75121, #48183, #55319, #35982, #73880, #16219, #11554, #17466, #55730, #37211, #11138, #61652, #23340, #74708, #68391, #10730, #36387, #36797, #43506, #38858, #51893, #12788, #155, #82257, #64960, #50243, #56964, #57377, #71274, #63294, #82662, #24976, #50649, #31300, #5633, #76352, #13212, #64127, #25808, #70861, #18683, #44327, #64539, #44735, #45157, #51469, #70019, #57789, #6876, #32545, #38444, #70431, #12371, #58209, #63705 ),
 ( #32967, #38030, #576, #11963, #6045, #26229, #31717, #83072, #77171, #39275, #24576, #77598, #6462, #13623, #19932, #32132, #45581, #7297, #75939, #25392, #18280, #19503, #43921, #69618, #51056, #76756, #19087, #37619, #59058, #9378, #8967, #72527, #65808, #78439, #53974, #34223, #8141, #27484, #8555, #53142, #47664, #78017, #22004, #15707, #79687, #73359, #21586, #33396, #33806, #72938, #26657, #34641, #1824, #46835, #78854, #40120, #15290, #20345, #52310, #59884, #21180, #72110, #41364, #45997, #71693, #14045, #14877, #27069, #66629, #40537, #66216, #59471, #39701, #20766, #2238, #27903, #1413, #52728, #67045, #58634, #53563, #60306, #1002, #65393, #79272, #7727, #47249, #46417, #40950, #14468, #2655, #28314, #69098, #42179, #3476, #17767, #35048, #24058, #29958, #68291, #81747, #10627, #75425, #43399, #67873, #10211, #29551, #48905, #55623, #60713, #75018, #4699, #74606, #36283, #3062, #28730, #54391, #9789, #35879, #49727, #16116, #35460, #61125, #29143, #67455, #41762, #54809, #80513, #81332, #80102, #22421, #30372, #42591, #48078, #23646, #80921, #56039, #62361, #42992, #22828, #17364, #61956, #16949, #4295, #48487, #16534, #74188, #61547, #3891, #73780, #68687, #49317, #55214, #23236, #11029, #36686, #44223, #63602, #44630, #5938, #469, #30788, #58103, #51786, #6769, #26125, #57687, #69512, #18580, #25703, #62787, #45051, #37925, #82967, #31608, #76246, #51363, #56451, #5121, #12682, #57269, #24874, #77490, #82154, #24469, #50136, #25285, #63189, #19400, #50953, #76650, #69913, #75834, #12267, #38340, #19825, #45475, #11446, #32027, #18175, #43808, #18982, #56859, #37514, #11861, #50542, #5529, #31193, #82556, #70752, #13103, #38757, #37102, #70326, #64434, #32441, #64015, #6356, #49, #77067, #72429, #8042, #71172, #14779, #27381, #64854, #39170, #77912, #2556, #46737, #53873, #7192, #898, #33297, #58957, #21079, #79172, #40434, #8450, #47148, #52208, #20665, #66115, #33705, #13513, #45892, #26555, #32864, #21901, #20243, #72838, #71589, #1315, #53464, #59366, #14367, #52629, #27804, #58532, #13941, #34121, #40024, #26964, #28214, #39598, #65287, #7625, #1724, #78334, #21489, #53042, #78754, #46318, #72011, #65712, #59782, #60206, #34540, #79588, #2136, #15188, #40845, #66531, #8862, #73683, #47983, #3379, #66952, #2968, #41266, #55524, #23549, #81233, #36588, #10931, #49217, #74923, #67776, #48390, #17267, #42896, #48807, #10115, #47565, #74506, #3793, #9284, #15606, #54291, #62266, #23138, #30275, #34955, #60618, #9695, #35365, #80824, #68590, #16853, #68191, #4603, #28634, #80419, #42488, #35776, #73258, #22320, #80007, #16023, #81653, #41670, #55938, #67361, #61030, #29862, #29042, #54713, #10530, #22731, #74089, #16436, #55115, #42081, #36185, #61446, #29457, #61857, #4198, #24372, #6253, #82870, #63508, #5839, #82058, #5436, #5028, #50043, #75738, #58006, #57592, #37831, #31096, #43714, #19300, #25194, #56764, #76149, #57172, #18489, #13003, #43301, #70648, #64336, #44951, #38659, #70228, #18079, #82463, #38241, #75324, #83282, #50447, #50860, #31513, #17670, #68998, #30696, #6673, #76560, #32345, #11350, #37008, #69416, #11770, #18888, #31930, #44537, #12582, #25605, #56360, #24779, #63917, #44132, #23964, #37424, #62686, #63097, #49630, #69824, #51268, #12173, #76970, #66016, #20145, #7094, #78655, #40744, #26026, #79075, #7942, #72739, #72331, #46218, #53365, #27701, #8352, #793, #34020, #59267, #39922, #65612, #58431, #65186, #64755, #26452, #52106, #34438, #59680, #14264, #7522, #45794, #21391, #1624, #33191, #52527, #33604, #78233, #15086, #19720, #47047, #66428, #8763, #371, #46635, #77814, #58859, #14679, #51686, #2036, #26866, #71914, #20567, #1217, #40335, #45378, #77388, #27281, #52941, #13840, #71075, #13417, #39074, #32764, #20976, #71492, #39498, #73989, #22631, #41571, #15503, #35262, #3692, #49116, #23451, #74821, #80725, #66850, #41161, #48292, #22218, #2866, #60517, #15924, #79483, #9183, #53770, #68086, #36088, #10431, #17166, #42800, #61759, #4097, #80316, #60927, #29765, #55427, #61339, #16336, #60104, #81135 ) ),
 .UNSPECIFIED., .F., .F., .F. ) 
 B_SPLINE_SURFACE_WITH_KNOTS ( ( 2, 2 ),
 ( 3, 2, 2, 2, 2, 2, 2, 2, 2, 2, 2, 2, 2, 2, 2, 2, 2, 2, 2, 2, 2, 2, 2, 2, 2, 2, 2, 2, 2, 2, 2, 2, 2, 2, 2, 2, 2, 2, 2, 2, 2, 2, 2, 2, 2, 2, 2, 2, 2, 2, 2, 2, 2, 2, 2, 2, 2, 2, 2, 2, 2, 2, 2, 2, 2, 2, 2, 2, 2, 2, 2, 2, 2, 2, 2, 2, 2, 2, 2, 2, 2, 2, 2, 2, 2, 2, 2, 2, 2, 2, 2, 2, 2, 2, 2, 2, 2, 2, 2, 2, 2, 2, 2, 2, 2, 2, 2, 2, 2, 2, 2, 2, 2, 2, 2, 2, 2, 2, 2, 2, 2, 2, 2, 2, 2, 2, 2, 2, 2, 2, 2, 2, 2, 2, 2, 2, 2, 2, 2, 2, 2, 2, 2, 2, 2, 2, 2, 2, 2, 2, 2, 2, 2, 2, 2, 2, 2, 2, 2, 2, 2, 2, 2, 2, 2, 2, 2, 2, 2, 2, 2, 2, 2, 2, 2, 2, 2, 2, 2, 2, 2, 2, 2, 2, 2, 2, 2, 2, 2, 2, 2, 2, 2, 2, 2, 2, 2, 2, 2, 2, 2, 2, 2, 2, 2, 2, 2, 2, 2, 2, 2, 2, 2, 2, 2, 2, 2, 2, 2, 2, 2, 2, 2, 2, 2, 2, 2, 2, 2, 2, 2, 2, 2, 2, 2, 2, 2, 2, 2, 2, 2, 2, 2, 2, 2, 2, 2, 2, 2, 2, 2, 2, 2, 2, 2, 3 ),
 ( 0.000000000000000000, 1.000000000000000000 ),
 ( 0.000000000000000000, 0.003787878787878787984, 0.007575757575757575968, 0.01136363636363636395, 0.01515151515151515194, 0.01893939393939393992, 0.02272727272727272790, 0.02651515151515151589, 0.03030303030303030387, 0.03409090909090908839, 0.03787878787878787984, 0.04166666666666666435, 0.04545454545454545581, 0.04924242424242424032, 0.05303030303030303177, 0.05681818181818181629, 0.06060606060606060774, 0.06439393939393939226, 0.06818181818181817677, 0.07196969696969697516, 0.07575757575757575968, 0.07954545454545454419, 0.08333333333333332871, 0.08712121212121212710, 0.09090909090909091161, 0.09469696969696969613, 0.09848484848484848064, 0.1022727272727272790, 0.1060606060606060635, 0.1098484848484848481, 0.1136363636363636326, 0.1174242424242424310, 0.1212121212121212155, 0.1250000000000000000, 0.1287878787878787845, 0.1325757575757575690, 0.1363636363636363535, 0.1401515151515151381, 0.1439393939393939503, 0.1477272727272727348, 0.1515151515151515194, 0.1553030303030303039, 0.1590909090909090884, 0.1628787878787878729, 0.1666666666666666574, 0.1704545454545454419, 0.1742424242424242542, 0.1780303030303030387, 0.1818181818181818232, 0.1856060606060606077, 0.1893939393939393923, 0.1931818181818181768, 0.1969696969696969613, 0.2007575757575757458, 0.2045454545454545581, 0.2083333333333333426, 0.2121212121212121271, 0.2159090909090909116, 0.2196969696969696961, 0.2234848484848484806, 0.2272727272727272652, 0.2310606060606060497, 0.2348484848484848619, 0.2386363636363636465, 0.2424242424242424310, 0.2462121212121212155, 0.2500000000000000000, 0.2537878787878787845, 0.2575757575757575690, 0.2613636363636363535, 0.2651515151515151381, 0.2689393939393939226, 0.2727272727272727071, 0.2765151515151514916, 0.2803030303030302761, 0.2840909090909091161, 0.2878787878787879007, 0.2916666666666666852, 0.2954545454545454697, 0.2992424242424242542, 0.3030303030303030387, 0.3068181818181818232, 0.3106060606060606077, 0.3143939393939393923, 0.3181818181818181768, 0.3219696969696969613, 0.3257575757575757458, 0.3295454545454545303, 0.3333333333333333148, 0.3371212121212120993, 0.3409090909090908839, 0.3446969696969697239, 0.3484848484848485084, 0.3522727272727272929, 0.3560606060606060774, 0.3598484848484848619, 0.3636363636363636465, 0.3674242424242424310, 0.3712121212121212155, 0.3750000000000000000, 0.3787878787878787845, 0.3825757575757575690, 0.3863636363636363535, 0.3901515151515151381, 0.3939393939393939226, 0.3977272727272727071, 0.4015151515151514916, 0.4053030303030302761, 0.4090909090909091161, 0.4128787878787879007, 0.4166666666666666852, 0.4204545454545454697, 0.4242424242424242542, 0.4280303030303030387, 0.4318181818181818232, 0.4356060606060606077, 0.4393939393939393923, 0.4431818181818181768, 0.4469696969696969613, 0.4507575757575757458, 0.4545454545454545303, 0.4583333333333333148, 0.4621212121212120993, 0.4659090909090908839, 0.4696969696969697239, 0.4734848484848485084, 0.4772727272727272929, 0.4810606060606060774, 0.4848484848484848619, 0.4886363636363636465, 0.4924242424242424310, 0.4962121212121212155, 0.5000000000000000000, 0.5037878787878787845, 0.5075757575757575690, 0.5113636363636363535, 0.5151515151515151381, 0.5189393939393939226, 0.5227272727272727071, 0.5265151515151514916, 0.5303030303030302761, 0.5340909090909090606, 0.5378787878787878451, 0.5416666666666666297, 0.5454545454545454142, 0.5492424242424241987, 0.5530303030303029832, 0.5568181818181817677, 0.5606060606060605522, 0.5643939393939394478, 0.5681818181818182323, 0.5719696969696970168, 0.5757575757575758013, 0.5795454545454545858, 0.5833333333333333703, 0.5871212121212121549, 0.5909090909090909394, 0.5946969696969697239, 0.5984848484848485084, 0.6022727272727272929, 0.6060606060606060774, 0.6098484848484848619, 0.6136363636363636465, 0.6174242424242424310, 0.6212121212121212155, 0.6250000000000000000, 0.6287878787878787845, 0.6325757575757575690, 0.6363636363636363535, 0.6401515151515151381, 0.6439393939393939226, 0.6477272727272727071, 0.6515151515151514916, 0.6553030303030302761, 0.6590909090909090606, 0.6628787878787878451, 0.6666666666666666297, 0.6704545454545454142, 0.6742424242424241987, 0.6780303030303029832, 0.6818181818181817677, 0.6856060606060605522, 0.6893939393939394478, 0.6931818181818182323, 0.6969696969696970168, 0.7007575757575758013, 0.7045454545454545858, 0.7083333333333333703, 0.7121212121212121549, 0.7159090909090909394, 0.7196969696969697239, 0.7234848484848485084, 0.7272727272727272929, 0.7310606060606060774, 0.7348484848484848619, 0.7386363636363636465, 0.7424242424242424310, 0.7462121212121212155, 0.7500000000000000000, 0.7537878787878787845, 0.7575757575757575690, 0.7613636363636363535, 0.7651515151515151381, 0.7689393939393939226, 0.7727272727272727071, 0.7765151515151514916, 0.7803030303030302761, 0.7840909090909090606, 0.7878787878787878451, 0.7916666666666666297, 0.7954545454545454142, 0.7992424242424241987, 0.8030303030303029832, 0.8068181818181817677, 0.8106060606060605522, 0.8143939393939394478, 0.8181818181818182323, 0.8219696969696970168, 0.8257575757575758013, 0.8295454545454545858, 0.8333333333333333703, 0.8371212121212121549, 0.8409090909090909394, 0.8446969696969697239, 0.8484848484848485084, 0.8522727272727272929, 0.8560606060606060774, 0.8598484848484848619, 0.8636363636363636465, 0.8674242424242424310, 0.8712121212121212155, 0.8750000000000000000, 0.8787878787878787845, 0.8825757575757575690, 0.8863636363636363535, 0.8901515151515151381, 0.8939393939393939226, 0.8977272727272727071, 0.9015151515151514916, 0.9053030303030302761, 0.9090909090909090606, 0.9128787878787878451, 0.9166666666666666297, 0.9204545454545454142, 0.9242424242424241987, 0.9280303030303029832, 0.9318181818181817677, 0.9356060606060605522, 0.9393939393939394478, 0.9431818181818182323, 0.9469696969696970168, 0.9507575757575758013, 0.9545454545454545858, 0.9583333333333333703, 0.9621212121212121549, 0.9659090909090909394 ),
 .UNSPECIFIED. ) 
 GEOMETRIC_REPRESENTATION_ITEM ( )  RATIONAL_B_SPLINE_SURFACE ( (
 ( 1.000000000000000000, 0.9659258262890683122, 1.000000000000000000, 0.9659258262890683122, 1.000000000000000000, 0.9659258262890683122, 1.000000000000000000, 0.9659258262890683122, 1.000000000000000000, 0.9659258262890683122, 1.000000000000000000, 0.9659258262890683122, 1.000000000000000000, 0.9659258262890683122, 1.000000000000000000, 0.9659258262890683122, 1.000000000000000000, 0.9659258262890683122, 1.000000000000000000, 0.9659258262890683122, 1.000000000000000000, 0.9659258262890683122, 1.000000000000000000, 0.9659258262890683122, 1.000000000000000000, 0.9659258262890683122, 1.000000000000000000, 0.9659258262890683122, 1.000000000000000000, 0.9659258262890683122, 1.000000000000000000, 0.9659258262890683122, 1.000000000000000000, 0.9659258262890683122, 1.000000000000000000, 0.9659258262890683122, 1.000000000000000000, 0.9659258262890683122, 1.000000000000000000, 0.9659258262890683122, 1.000000000000000000, 0.9659258262890683122, 1.000000000000000000, 0.9659258262890683122, 1.000000000000000000, 0.9659258262890683122, 1.000000000000000000, 0.9659258262890683122, 1.000000000000000000, 0.9659258262890683122, 1.000000000000000000, 0.9659258262890683122, 1.000000000000000000, 0.9659258262890683122, 1.000000000000000000, 0.9659258262890683122, 1.000000000000000000, 0.9659258262890683122, 1.000000000000000000, 0.9659258262890683122, 1.000000000000000000, 0.9659258262890683122, 1.000000000000000000, 0.9659258262890683122, 1.000000000000000000, 0.9659258262890683122, 1.000000000000000000, 0.9659258262890683122, 1.000000000000000000, 0.9659258262890683122, 1.000000000000000000, 0.9659258262890683122, 1.000000000000000000, 0.9659258262890683122, 1.000000000000000000, 0.9659258262890683122, 1.000000000000000000, 0.9659258262890683122, 1.000000000000000000, 0.9659258262890683122, 1.000000000000000000, 0.9659258262890683122, 1.000000000000000000, 0.9659258262890683122, 1.000000000000000000, 0.9659258262890683122, 1.000000000000000000, 0.9659258262890683122, 1.000000000000000000, 0.9659258262890683122, 1.000000000000000000, 0.9659258262890683122, 1.000000000000000000, 0.9659258262890683122, 1.000000000000000000, 0.9659258262890683122, 1.000000000000000000, 0.9659258262890683122, 1.000000000000000000, 0.9659258262890683122, 1.000000000000000000, 0.9659258262890683122, 1.000000000000000000, 0.9659258262890683122, 1.000000000000000000, 0.9659258262890683122, 1.000000000000000000, 0.9659258262890683122, 1.000000000000000000, 0.9659258262890683122, 1.000000000000000000, 0.9659258262890683122, 1.000000000000000000, 0.9659258262890683122, 1.000000000000000000, 0.9659258262890683122, 1.000000000000000000, 0.9659258262890683122, 1.000000000000000000, 0.9659258262890683122, 1.000000000000000000, 0.9659258262890683122, 1.000000000000000000, 0.9659258262890683122, 1.000000000000000000, 0.9659258262890683122, 1.000000000000000000, 0.9659258262890683122, 1.000000000000000000, 0.9659258262890683122, 1.000000000000000000, 0.9659258262890683122, 1.000000000000000000, 0.9659258262890683122, 1.000000000000000000, 0.9659258262890683122, 1.000000000000000000, 0.9659258262890683122, 1.000000000000000000, 0.9659258262890683122, 1.000000000000000000, 0.9659258262890683122, 1.000000000000000000, 0.9659258262890683122, 1.000000000000000000, 0.9659258262890683122, 1.000000000000000000, 0.9659258262890683122, 1.000000000000000000, 0.9659258262890683122, 1.000000000000000000, 0.9659258262890683122, 1.000000000000000000, 0.9659258262890683122, 1.000000000000000000, 0.9659258262890683122, 1.000000000000000000, 0.9659258262890683122, 1.000000000000000000, 0.9659258262890683122, 1.000000000000000000, 0.9659258262890683122, 1.000000000000000000, 0.9659258262890683122, 1.000000000000000000, 0.9659258262890683122, 1.000000000000000000, 0.9659258262890683122, 1.000000000000000000, 0.9659258262890683122, 1.000000000000000000, 0.9659258262890683122, 1.000000000000000000, 0.9659258262890683122, 1.000000000000000000, 0.9659258262890683122, 1.000000000000000000, 0.9659258262890683122, 1.000000000000000000, 0.9659258262890683122, 1.000000000000000000, 0.9659258262890683122, 1.000000000000000000, 0.9659258262890683122, 1.000000000000000000, 0.9659258262890683122, 1.000000000000000000, 0.9659258262890683122, 1.000000000000000000, 0.9659258262890683122, 1.000000000000000000, 0.9659258262890683122, 1.000000000000000000, 0.9659258262890683122, 1.000000000000000000, 0.9659258262890683122, 1.000000000000000000, 0.9659258262890683122, 1.000000000000000000, 0.9659258262890683122, 1.000000000000000000, 0.9659258262890683122, 1.000000000000000000, 0.9659258262890683122, 1.000000000000000000, 0.9659258262890683122, 1.000000000000000000, 0.9659258262890683122, 1.000000000000000000, 0.9659258262890683122, 1.000000000000000000, 0.9659258262890683122, 1.000000000000000000, 0.9659258262890683122, 1.000000000000000000, 0.9659258262890683122, 1.000000000000000000, 0.9659258262890683122, 1.000000000000000000, 0.9659258262890683122, 1.000000000000000000, 0.9659258262890683122, 1.000000000000000000, 0.9659258262890683122, 1.000000000000000000, 0.9659258262890683122, 1.000000000000000000, 0.9659258262890683122, 1.000000000000000000, 0.9659258262890683122, 1.000000000000000000, 0.9659258262890683122, 1.000000000000000000, 0.9659258262890683122, 1.000000000000000000, 0.9659258262890683122, 1.000000000000000000, 0.9659258262890683122, 1.000000000000000000, 0.9659258262890683122, 1.000000000000000000, 0.9659258262890683122, 1.000000000000000000, 0.9659258262890683122, 1.000000000000000000, 0.9659258262890683122, 1.000000000000000000, 0.9659258262890683122, 1.000000000000000000, 0.9659258262890683122, 1.000000000000000000, 0.9659258262890683122, 1.000000000000000000, 0.9659258262890683122, 1.000000000000000000, 0.9659258262890683122, 1.000000000000000000, 0.9659258262890683122, 1.000000000000000000, 0.9659258262890683122, 1.000000000000000000, 0.9659258262890683122, 1.000000000000000000, 0.9659258262890683122, 1.000000000000000000, 0.9659258262890683122, 1.000000000000000000, 0.9659258262890683122, 1.000000000000000000, 0.9659258262890683122, 1.000000000000000000, 0.9659258262890683122, 1.000000000000000000, 0.9659258262890683122, 1.000000000000000000, 0.9659258262890683122, 1.000000000000000000, 0.9659258262890683122, 1.000000000000000000, 0.9659258262890683122, 1.000000000000000000, 0.9659258262890683122, 1.000000000000000000, 0.9659258262890683122, 1.000000000000000000, 0.9659258262890683122, 1.000000000000000000, 0.9659258262890683122, 1.000000000000000000, 0.9659258262890683122, 1.000000000000000000, 0.9659258262890683122, 1.000000000000000000, 0.9659258262890683122, 1.000000000000000000, 0.9659258262890683122, 1.000000000000000000, 0.9659258262890683122, 1.000000000000000000, 0.9659258262890683122, 1.000000000000000000, 0.9659258262890683122, 1.000000000000000000, 0.9659258262890683122, 1.000000000000000000, 0.9659258262890683122, 1.000000000000000000, 0.9659258262890683122, 1.000000000000000000, 0.9659258262890683122, 1.000000000000000000, 0.9659258262890683122, 1.000000000000000000, 0.9659258262890683122, 1.000000000000000000, 0.9659258262890683122, 1.000000000000000000, 0.9659258262890683122, 1.000000000000000000, 0.9659258262890683122, 1.000000000000000000, 0.9659258262890683122, 1.000000000000000000, 0.9659258262890683122, 1.000000000000000000, 0.9659258262890683122, 1.000000000000000000, 0.9659258262890683122, 1.000000000000000000, 0.9659258262890683122, 1.000000000000000000, 0.9659258262890683122, 1.000000000000000000, 0.9659258262890683122, 1.000000000000000000, 0.9659258262890683122, 1.000000000000000000, 0.9659258262890683122, 1.000000000000000000, 0.9659258262890683122, 1.000000000000000000, 0.9659258262890683122, 1.000000000000000000, 0.9659258262890683122, 1.000000000000000000, 0.9659258262890683122, 1.000000000000000000, 0.9659258262890683122, 1.000000000000000000, 0.9659258262890683122, 1.000000000000000000, 0.9659258262890683122, 1.000000000000000000, 0.9659258262890683122, 1.000000000000000000, 0.9659258262890683122, 1.000000000000000000, 0.9659258262890683122, 1.000000000000000000, 0.9659258262890683122, 1.000000000000000000, 0.9659258262890683122, 1.000000000000000000, 0.9659258262890683122, 1.000000000000000000, 0.9659258262890683122, 1.000000000000000000, 0.9659258262890683122, 1.000000000000000000, 0.9659258262890683122, 1.000000000000000000, 0.9659258262890683122, 1.000000000000000000, 0.9659258262890683122, 1.000000000000000000, 0.9659258262890683122, 1.000000000000000000, 0.9659258262890683122, 1.000000000000000000, 0.9659258262890683122, 1.000000000000000000, 0.9659258262890683122, 1.000000000000000000, 0.9659258262890683122, 1.000000000000000000, 0.9659258262890683122, 1.000000000000000000, 0.9659258262890683122, 1.000000000000000000, 0.9659258262890683122, 1.000000000000000000, 0.9659258262890683122, 1.000000000000000000, 0.9659258262890683122, 1.000000000000000000, 0.9659258262890683122, 1.000000000000000000, 0.9659258262890683122, 1.000000000000000000, 0.9659258262890683122, 1.000000000000000000, 0.9659258262890683122, 1.000000000000000000, 0.9659258262890683122, 1.000000000000000000, 0.9659258262890683122, 1.000000000000000000, 0.9659258262890683122, 1.000000000000000000, 0.9659258262890683122, 1.000000000000000000, 0.9659258262890683122, 1.000000000000000000, 0.9659258262890683122, 1.000000000000000000, 0.9659258262890683122, 1.000000000000000000, 0.9659258262890683122, 1.000000000000000000, 0.9659258262890683122, 1.000000000000000000, 0.9659258262890683122, 1.000000000000000000, 0.9659258262890683122, 1.000000000000000000, 0.9659258262890683122, 1.000000000000000000, 0.9659258262890683122, 1.000000000000000000, 0.9659258262890683122, 1.000000000000000000, 0.9659258262890683122, 1.000000000000000000, 0.9659258262890683122, 1.000000000000000000, 0.9659258262890683122, 1.000000000000000000, 0.9659258262890683122, 1.000000000000000000, 0.9659258262890683122, 1.000000000000000000, 0.9659258262890683122, 1.000000000000000000, 0.9659258262890683122, 1.000000000000000000, 0.9659258262890683122, 1.000000000000000000, 0.9659258262890683122, 1.000000000000000000, 0.9659258262890683122, 1.000000000000000000, 0.9659258262890683122, 1.000000000000000000, 0.9659258262890683122, 1.000000000000000000, 0.9659258262890683122, 1.000000000000000000, 0.9659258262890683122, 1.000000000000000000, 0.9659258262890683122, 1.000000000000000000, 0.9659258262890683122, 1.000000000000000000, 0.9659258262890683122, 1.000000000000000000, 0.9659258262890683122, 1.000000000000000000, 0.9659258262890683122, 1.000000000000000000, 0.9659258262890683122, 1.000000000000000000, 0.9659258262890683122, 1.000000000000000000, 0.9659258262890683122, 1.000000000000000000, 0.9659258262890683122, 1.000000000000000000, 0.9659258262890683122, 1.000000000000000000, 0.9659258262890683122, 1.000000000000000000, 0.9659258262890683122, 1.000000000000000000, 0.9659258262890683122, 1.000000000000000000, 0.9659258262890683122, 1.000000000000000000, 0.9659258262890683122, 1.000000000000000000, 0.9659258262890683122, 1.000000000000000000, 0.9659258262890683122, 1.000000000000000000, 0.9659258262890683122, 1.000000000000000000, 0.9659258262890683122, 1.000000000000000000, 0.9659258262890683122, 1.000000000000000000, 0.9659258262890683122, 1.000000000000000000, 0.9659258262890683122, 1.000000000000000000, 0.9659258262890683122, 1.000000000000000000, 0.9659258262890683122, 1.000000000000000000, 0.9659258262890683122, 1.000000000000000000, 0.9659258262890683122, 1.000000000000000000),
 ( 1.000000000000000000, 0.9659258262890683122, 1.000000000000000000, 0.9659258262890683122, 1.000000000000000000, 0.9659258262890683122, 1.000000000000000000, 0.9659258262890683122, 1.000000000000000000, 0.9659258262890683122, 1.000000000000000000, 0.9659258262890683122, 1.000000000000000000, 0.9659258262890683122, 1.000000000000000000, 0.9659258262890683122, 1.000000000000000000, 0.9659258262890683122, 1.000000000000000000, 0.9659258262890683122, 1.000000000000000000, 0.9659258262890683122, 1.000000000000000000, 0.9659258262890683122, 1.000000000000000000, 0.9659258262890683122, 1.000000000000000000, 0.9659258262890683122, 1.000000000000000000, 0.9659258262890683122, 1.000000000000000000, 0.9659258262890683122, 1.000000000000000000, 0.9659258262890683122, 1.000000000000000000, 0.9659258262890683122, 1.000000000000000000, 0.9659258262890683122, 1.000000000000000000, 0.9659258262890683122, 1.000000000000000000, 0.9659258262890683122, 1.000000000000000000, 0.9659258262890683122, 1.000000000000000000, 0.9659258262890683122, 1.000000000000000000, 0.9659258262890683122, 1.000000000000000000, 0.9659258262890683122, 1.000000000000000000, 0.9659258262890683122, 1.000000000000000000, 0.9659258262890683122, 1.000000000000000000, 0.9659258262890683122, 1.000000000000000000, 0.9659258262890683122, 1.000000000000000000, 0.9659258262890683122, 1.000000000000000000, 0.9659258262890683122, 1.000000000000000000, 0.9659258262890683122, 1.000000000000000000, 0.9659258262890683122, 1.000000000000000000, 0.9659258262890683122, 1.000000000000000000, 0.9659258262890683122, 1.000000000000000000, 0.9659258262890683122, 1.000000000000000000, 0.9659258262890683122, 1.000000000000000000, 0.9659258262890683122, 1.000000000000000000, 0.9659258262890683122, 1.000000000000000000, 0.9659258262890683122, 1.000000000000000000, 0.9659258262890683122, 1.000000000000000000, 0.9659258262890683122, 1.000000000000000000, 0.9659258262890683122, 1.000000000000000000, 0.9659258262890683122, 1.000000000000000000, 0.9659258262890683122, 1.000000000000000000, 0.9659258262890683122, 1.000000000000000000, 0.9659258262890683122, 1.000000000000000000, 0.9659258262890683122, 1.000000000000000000, 0.9659258262890683122, 1.000000000000000000, 0.9659258262890683122, 1.000000000000000000, 0.9659258262890683122, 1.000000000000000000, 0.9659258262890683122, 1.000000000000000000, 0.9659258262890683122, 1.000000000000000000, 0.9659258262890683122, 1.000000000000000000, 0.9659258262890683122, 1.000000000000000000, 0.9659258262890683122, 1.000000000000000000, 0.9659258262890683122, 1.000000000000000000, 0.9659258262890683122, 1.000000000000000000, 0.9659258262890683122, 1.000000000000000000, 0.9659258262890683122, 1.000000000000000000, 0.9659258262890683122, 1.000000000000000000, 0.9659258262890683122, 1.000000000000000000, 0.9659258262890683122, 1.000000000000000000, 0.9659258262890683122, 1.000000000000000000, 0.9659258262890683122, 1.000000000000000000, 0.9659258262890683122, 1.000000000000000000, 0.9659258262890683122, 1.000000000000000000, 0.9659258262890683122, 1.000000000000000000, 0.9659258262890683122, 1.000000000000000000, 0.9659258262890683122, 1.000000000000000000, 0.9659258262890683122, 1.000000000000000000, 0.9659258262890683122, 1.000000000000000000, 0.9659258262890683122, 1.000000000000000000, 0.9659258262890683122, 1.000000000000000000, 0.9659258262890683122, 1.000000000000000000, 0.9659258262890683122, 1.000000000000000000, 0.9659258262890683122, 1.000000000000000000, 0.9659258262890683122, 1.000000000000000000, 0.9659258262890683122, 1.000000000000000000, 0.9659258262890683122, 1.000000000000000000, 0.9659258262890683122, 1.000000000000000000, 0.9659258262890683122, 1.000000000000000000, 0.9659258262890683122, 1.000000000000000000, 0.9659258262890683122, 1.000000000000000000, 0.9659258262890683122, 1.000000000000000000, 0.9659258262890683122, 1.000000000000000000, 0.9659258262890683122, 1.000000000000000000, 0.9659258262890683122, 1.000000000000000000, 0.9659258262890683122, 1.000000000000000000, 0.9659258262890683122, 1.000000000000000000, 0.9659258262890683122, 1.000000000000000000, 0.9659258262890683122, 1.000000000000000000, 0.9659258262890683122, 1.000000000000000000, 0.9659258262890683122, 1.000000000000000000, 0.9659258262890683122, 1.000000000000000000, 0.9659258262890683122, 1.000000000000000000, 0.9659258262890683122, 1.000000000000000000, 0.9659258262890683122, 1.000000000000000000, 0.9659258262890683122, 1.000000000000000000, 0.9659258262890683122, 1.000000000000000000, 0.9659258262890683122, 1.000000000000000000, 0.9659258262890683122, 1.000000000000000000, 0.9659258262890683122, 1.000000000000000000, 0.9659258262890683122, 1.000000000000000000, 0.9659258262890683122, 1.000000000000000000, 0.9659258262890683122, 1.000000000000000000, 0.9659258262890683122, 1.000000000000000000, 0.9659258262890683122, 1.000000000000000000, 0.9659258262890683122, 1.000000000000000000, 0.9659258262890683122, 1.000000000000000000, 0.9659258262890683122, 1.000000000000000000, 0.9659258262890683122, 1.000000000000000000, 0.9659258262890683122, 1.000000000000000000, 0.9659258262890683122, 1.000000000000000000, 0.9659258262890683122, 1.000000000000000000, 0.9659258262890683122, 1.000000000000000000, 0.9659258262890683122, 1.000000000000000000, 0.9659258262890683122, 1.000000000000000000, 0.9659258262890683122, 1.000000000000000000, 0.9659258262890683122, 1.000000000000000000, 0.9659258262890683122, 1.000000000000000000, 0.9659258262890683122, 1.000000000000000000, 0.9659258262890683122, 1.000000000000000000, 0.9659258262890683122, 1.000000000000000000, 0.9659258262890683122, 1.000000000000000000, 0.9659258262890683122, 1.000000000000000000, 0.9659258262890683122, 1.000000000000000000, 0.9659258262890683122, 1.000000000000000000, 0.9659258262890683122, 1.000000000000000000, 0.9659258262890683122, 1.000000000000000000, 0.9659258262890683122, 1.000000000000000000, 0.9659258262890683122, 1.000000000000000000, 0.9659258262890683122, 1.000000000000000000, 0.9659258262890683122, 1.000000000000000000, 0.9659258262890683122, 1.000000000000000000, 0.9659258262890683122, 1.000000000000000000, 0.9659258262890683122, 1.000000000000000000, 0.9659258262890683122, 1.000000000000000000, 0.9659258262890683122, 1.000000000000000000, 0.9659258262890683122, 1.000000000000000000, 0.9659258262890683122, 1.000000000000000000, 0.9659258262890683122, 1.000000000000000000, 0.9659258262890683122, 1.000000000000000000, 0.9659258262890683122, 1.000000000000000000, 0.9659258262890683122, 1.000000000000000000, 0.9659258262890683122, 1.000000000000000000, 0.9659258262890683122, 1.000000000000000000, 0.9659258262890683122, 1.000000000000000000, 0.9659258262890683122, 1.000000000000000000, 0.9659258262890683122, 1.000000000000000000, 0.9659258262890683122, 1.000000000000000000, 0.9659258262890683122, 1.000000000000000000, 0.9659258262890683122, 1.000000000000000000, 0.9659258262890683122, 1.000000000000000000, 0.9659258262890683122, 1.000000000000000000, 0.9659258262890683122, 1.000000000000000000, 0.9659258262890683122, 1.000000000000000000, 0.9659258262890683122, 1.000000000000000000, 0.9659258262890683122, 1.000000000000000000, 0.9659258262890683122, 1.000000000000000000, 0.9659258262890683122, 1.000000000000000000, 0.9659258262890683122, 1.000000000000000000, 0.9659258262890683122, 1.000000000000000000, 0.9659258262890683122, 1.000000000000000000, 0.9659258262890683122, 1.000000000000000000, 0.9659258262890683122, 1.000000000000000000, 0.9659258262890683122, 1.000000000000000000, 0.9659258262890683122, 1.000000000000000000, 0.9659258262890683122, 1.000000000000000000, 0.9659258262890683122, 1.000000000000000000, 0.9659258262890683122, 1.000000000000000000, 0.9659258262890683122, 1.000000000000000000, 0.9659258262890683122, 1.000000000000000000, 0.9659258262890683122, 1.000000000000000000, 0.9659258262890683122, 1.000000000000000000, 0.9659258262890683122, 1.000000000000000000, 0.9659258262890683122, 1.000000000000000000, 0.9659258262890683122, 1.000000000000000000, 0.9659258262890683122, 1.000000000000000000, 0.9659258262890683122, 1.000000000000000000, 0.9659258262890683122, 1.000000000000000000, 0.9659258262890683122, 1.000000000000000000, 0.9659258262890683122, 1.000000000000000000, 0.9659258262890683122, 1.000000000000000000, 0.9659258262890683122, 1.000000000000000000, 0.9659258262890683122, 1.000000000000000000, 0.9659258262890683122, 1.000000000000000000, 0.9659258262890683122, 1.000000000000000000, 0.9659258262890683122, 1.000000000000000000, 0.9659258262890683122, 1.000000000000000000, 0.9659258262890683122, 1.000000000000000000, 0.9659258262890683122, 1.000000000000000000, 0.9659258262890683122, 1.000000000000000000, 0.9659258262890683122, 1.000000000000000000, 0.9659258262890683122, 1.000000000000000000, 0.9659258262890683122, 1.000000000000000000, 0.9659258262890683122, 1.000000000000000000, 0.9659258262890683122, 1.000000000000000000, 0.9659258262890683122, 1.000000000000000000, 0.9659258262890683122, 1.000000000000000000, 0.9659258262890683122, 1.000000000000000000, 0.9659258262890683122, 1.000000000000000000, 0.9659258262890683122, 1.000000000000000000, 0.9659258262890683122, 1.000000000000000000, 0.9659258262890683122, 1.000000000000000000, 0.9659258262890683122, 1.000000000000000000, 0.9659258262890683122, 1.000000000000000000, 0.9659258262890683122, 1.000000000000000000, 0.9659258262890683122, 1.000000000000000000, 0.9659258262890683122, 1.000000000000000000, 0.9659258262890683122, 1.000000000000000000, 0.9659258262890683122, 1.000000000000000000, 0.9659258262890683122, 1.000000000000000000, 0.9659258262890683122, 1.000000000000000000, 0.9659258262890683122, 1.000000000000000000, 0.9659258262890683122, 1.000000000000000000, 0.9659258262890683122, 1.000000000000000000, 0.9659258262890683122, 1.000000000000000000, 0.9659258262890683122, 1.000000000000000000, 0.9659258262890683122, 1.000000000000000000, 0.9659258262890683122, 1.000000000000000000, 0.9659258262890683122, 1.000000000000000000, 0.9659258262890683122, 1.000000000000000000, 0.9659258262890683122, 1.000000000000000000, 0.9659258262890683122, 1.000000000000000000, 0.9659258262890683122, 1.000000000000000000, 0.9659258262890683122, 1.000000000000000000, 0.9659258262890683122, 1.000000000000000000, 0.9659258262890683122, 1.000000000000000000, 0.9659258262890683122, 1.000000000000000000, 0.9659258262890683122, 1.000000000000000000, 0.9659258262890683122, 1.000000000000000000, 0.9659258262890683122, 1.000000000000000000, 0.9659258262890683122, 1.000000000000000000, 0.9659258262890683122, 1.000000000000000000, 0.9659258262890683122, 1.000000000000000000, 0.9659258262890683122, 1.000000000000000000, 0.9659258262890683122, 1.000000000000000000, 0.9659258262890683122, 1.000000000000000000, 0.9659258262890683122, 1.000000000000000000, 0.9659258262890683122, 1.000000000000000000, 0.9659258262890683122, 1.000000000000000000, 0.9659258262890683122, 1.000000000000000000, 0.9659258262890683122, 1.000000000000000000, 0.9659258262890683122, 1.000000000000000000, 0.9659258262890683122, 1.000000000000000000, 0.9659258262890683122, 1.000000000000000000, 0.9659258262890683122, 1.000000000000000000, 0.9659258262890683122, 1.000000000000000000, 0.9659258262890683122, 1.000000000000000000, 0.9659258262890683122, 1.000000000000000000, 0.9659258262890683122, 1.000000000000000000, 0.9659258262890683122, 1.000000000000000000, 0.9659258262890683122, 1.000000000000000000, 0.9659258262890683122, 1.000000000000000000) ) ) 
 REPRESENTATION_ITEM ( '' )  SURFACE ( )  );
#57366=CARTESIAN_POINT ( 'NONE',  ( 1.594488188976378673, -0.4536011799217368745, -0.2665933059059886201 ) ) ;
#57367=CARTESIAN_POINT ( 'NONE',  ( -0.1902887139107604098, 0.2952755905511810774, -0.1292274648535930714 ) ) ;
#57368=CARTESIAN_POINT ( 'NONE',  ( -0.3608923884514428360, 0.1771653543307087630, 0.09757992244046791164 ) ) ;
#57369=CARTESIAN_POINT ( 'NONE',  ( -1.620734908136482577, -0.5511811023622048555, -0.09757992244046775898 ) ) ;
#57370=CARTESIAN_POINT ( 'NONE',  ( 0.8267716535433077274, 0.1771653543307087630, 0.000000000000000000 ) ) ;
#57371=CARTESIAN_POINT ( 'NONE',  ( 0.9711286089238851948, -0.6046776061558809534, -0.2411417322834644161 ) ) ;
#57372=CARTESIAN_POINT ( 'NONE',  ( 1.482939632545932307, 0.05413385826771626580, -0.4176697321401330321 ) ) ;
#57373=CARTESIAN_POINT ( 'NONE',  ( -0.09186351706036663400, -0.3690944881889763329, 0.3153832671262228327 ) ) ;
#57374=CARTESIAN_POINT ( 'NONE',  ( 0.3477690288713918276, -0.6692913385826773087, -0.1292274648535924053 ) ) ;
#57375=CARTESIAN_POINT ( 'NONE',  ( 0.4658792650918640033, -0.2845877964562159024, 0.3641732283464567677 ) ) ;
#57377=CARTESIAN_POINT ( 'NONE',  ( -1.476377952755905110, 0.1660481256975885056, 0.3530559997133364547 ) ) ;
#57378=CARTESIAN_POINT ( 'NONE',  ( -1.194225721784776262, -0.4281496062992124485, 0.4176697321401328655 ) ) ;
#57379=CARTESIAN_POINT ( 'NONE',  ( -0.4790026246719154557, -0.3162353388693405765, 0.4822834645669290543 ) ) ;
#57383=CARTESIAN_POINT ( 'NONE',  ( 0.2887139107611556010, -0.6046776061558807314, 0.2411417322834647770 ) ) ;
#57384=CARTESIAN_POINT ( 'NONE',  ( 1.043307086614173818, -0.4536011799217368745, -0.2665933059059886201 ) ) ;
#57387=CARTESIAN_POINT ( 'NONE',  ( -0.5183727034120726440, 0.2952755905511811885, 0.1292274648535926551 ) ) ;
#57388=CARTESIAN_POINT ( 'NONE',  ( 0.2296587926509192634, -0.05778040916215560624, -0.4822834645669293319 ) ) ;
#57396=CARTESIAN_POINT ( 'NONE',  ( -0.4855643044619415427, -0.3690944881889763329, 0.3153832671262228327 ) ) ;
#57397=CARTESIAN_POINT ( 'NONE',  ( -1.266404199475064773, -0.3162353388693405765, 0.4822834645669290543 ) ) ;
#57399=CARTESIAN_POINT ( 'NONE',  ( 0.9908136482939640111, -0.6692913385826771977, 0.1292274648535927661 ) ) ;
#57400=CARTESIAN_POINT ( 'NONE',  ( 1.397637795275591177, -0.5400638737290844871, 0.3530559997133364547 ) ) ;
#57401=CARTESIAN_POINT ( 'NONE',  ( 0.7020997375328090762, -0.05778040916215560624, -0.4822834645669293319 ) ) ;
#57404=CARTESIAN_POINT ( 'NONE',  ( 1.686351706036745890, 0.2952755905511811885, 0.1292274648535926551 ) ) ;
#57405=CARTESIAN_POINT ( 'NONE',  ( 0.6102362204724416372, -0.5400638737290844871, 0.3530559997133364547 ) ) ;
#57406=CARTESIAN_POINT ( 'NONE',  ( 0.6889763779527563470, 0.1660481256975883668, -0.3530559997133364547 ) ) ;
#57407=CARTESIAN_POINT ( 'NONE',  ( 0.6561679790026253567, 0.1283753931104748280, 0.1820866141732283561 ) ) ;
#57408=CARTESIAN_POINT ( 'NONE',  ( 1.194225721784777594, 0.05413385826771666132, 0.4176697321401328100 ) ) ;
#57410=CARTESIAN_POINT ( 'NONE',  ( 0.3280839895013130669, 0.05413385826771666132, 0.4176697321401328100 ) ) ;
#57411=CARTESIAN_POINT ( 'NONE',  ( 1.259842519685040019, -0.1870078740157480879, -0.4822834645669291653 ) ) ;
#57412=CARTESIAN_POINT ( 'NONE',  ( 0.2821522309711292364, 0.2952755905511810774, -0.1292274648535930714 ) ) ;
#57413=CARTESIAN_POINT ( 'NONE',  ( 1.666666666666667185, -0.004921259842519576551, 0.3153832671262227771 ) ) ;
#57414=CARTESIAN_POINT ( 'NONE',  ( -0.9383202099737524282, -0.05778040916215522460, 0.4822834645669289988 ) ) ;
#57415=CARTESIAN_POINT ( 'NONE',  ( -1.115485564304461219, -0.4281496062992124485, 0.4176697321401328655 ) ) ;
#57416=CARTESIAN_POINT ( 'NONE',  ( 1.377952755905512472, -0.6692913385826771977, 8.415575281601705876E-17 ) ) ;
#57423=CARTESIAN_POINT ( 'NONE',  ( 1.541994750656168645, 0.2952755905511810774, -0.1292274648535930714 ) ) ;
#57424=CARTESIAN_POINT ( 'NONE',  ( 1.286089238845145033, 0.1283753931104748280, 0.1820866141732283561 ) ) ;
#57426=CARTESIAN_POINT ( 'NONE',  ( 1.299212598425197429, -0.5511811023622047445, 6.969142054262312111E-17 ) ) ;
#57431=CARTESIAN_POINT ( 'NONE',  ( -0.6299212598425188991, -0.1870078740157480601, -0.3641732283464567677 ) ) ;
#57432=CARTESIAN_POINT ( 'NONE',  ( -1.601049868766403650, -0.5023911411419708095, 0.1820866141732285504 ) ) ;
#57433=CARTESIAN_POINT ( 'NONE',  ( -1.338582677165353729, -0.1870078740157479769, 0.4822834645669291653 ) ) ;
#57434=CARTESIAN_POINT ( 'NONE',  ( 0.2690288713910767848, -0.6692913385826773087, -0.1292274648535924053 ) ) ;
#57435=CARTESIAN_POINT ( 'NONE',  ( 1.437007874015748810, 0.1660481256975885056, 0.3530559997133364547 ) ) ;
#57436=VERTEX_POINT ( 'NONE', #79316 ) ;
#57441=CARTESIAN_POINT ( 'NONE',  ( -0.6496062992125976043, 0.07958543189024071263, -0.2665933059059888421 ) ) ;
#57442=CARTESIAN_POINT ( 'NONE',  ( -1.213910761154854745, -0.6692913385826771977, 0.1292274648535927661 ) ) ;
#57443=CARTESIAN_POINT ( 'NONE',  ( 1.108923884514436686, -0.3162353388693409650, -0.4822834645669289433 ) ) ;
#57448=CARTESIAN_POINT ( 'NONE',  ( 1.200787401574803681, 0.1660481256975885056, 0.3530559997133364547 ) ) ;
#57449=CARTESIAN_POINT ( 'NONE',  ( -1.430446194225721390, -0.4281496062992124485, 0.4176697321401328655 ) ) ;
#57451=CARTESIAN_POINT ( 'NONE',  ( -0.2887139107611542133, 0.1283753931104748280, 0.1820866141732283561 ) ) ;
#57453=CARTESIAN_POINT ( 'NONE',  ( -0.4790026246719152336, -0.08942795157528024563, -0.3641732283464568787 ) ) ;
#57454=CARTESIAN_POINT ( 'NONE',  ( 0.03937007874015806264, 0.1771653543307087630, 0.000000000000000000 ) ) ;
#57455=CARTESIAN_POINT ( 'NONE',  ( -0.006561679790025524116, -0.3162353388693405765, 0.4822834645669290543 ) ) ;
#57456=CARTESIAN_POINT ( 'NONE',  ( -0.8464566929133852113, 0.07958543189024085140, 0.2665933059059887866 ) ) ;
#57458=CARTESIAN_POINT ( 'NONE',  ( 1.279527559055118724, 0.1660481256975885056, 0.3530559997133364547 ) ) ;
#57459=CARTESIAN_POINT ( 'NONE',  ( -1.594488188976377119, 0.1660481256975883668, -0.3530559997133364547 ) ) ;
#57461=CARTESIAN_POINT ( 'NONE',  ( -0.3608923884514428360, -0.6692913385826773087, -0.1292274648535924053 ) ) ;
#57462=CARTESIAN_POINT ( 'NONE',  ( -1.003937007874014853, 0.1660481256975885056, 0.3530559997133364547 ) ) ;
#57463=CARTESIAN_POINT ( 'NONE',  ( 1.082677165354331228, 0.07958543189024071263, -0.2665933059059888421 ) ) ;
#57464=CARTESIAN_POINT ( 'NONE',  ( -0.1377952755905504645, 0.07958543189024085140, 0.2665933059059887866 ) ) ;
#57465=CARTESIAN_POINT ( 'NONE',  ( -0.7808398950131225646, -0.05778040916215522460, 0.4822834645669289988 ) ) ;
#57466=CARTESIAN_POINT ( 'NONE',  ( -1.030183727034119867, -0.3162353388693405765, 0.4822834645669290543 ) ) ;
#57467=FACE_OUTER_BOUND ( 'NONE', #4081, .T. ) ;
#57468=CARTESIAN_POINT ( 'NONE',  ( 1.299212598425197429, -0.5511811023622047445, 6.969142054262312111E-17 ) ) ;
#57469=CARTESIAN_POINT ( 'NONE',  ( -0.2624671916010490880, -0.6046776061558807314, 0.2411417322834647770 ) ) ;
#57470=CARTESIAN_POINT ( 'NONE',  ( -1.482939632545930975, -0.4281496062992127816, -0.4176697321401328100 ) ) ;
#57471=VERTEX_POINT ( 'NONE', #3114 ) ;
#57473=CARTESIAN_POINT ( 'NONE',  ( -0.9514435695538050464, -0.08942795157528024563, -0.3641732283464568787 ) ) ;
#57474=CARTESIAN_POINT ( 'NONE',  ( 0.7545931758530188826, -0.6692913385826771977, 0.1292274648535927661 ) ) ;
#57475=CARTESIAN_POINT ( 'NONE',  ( -0.9580052493438311334, -0.3690944881889763329, 0.3153832671262228327 ) ) ;
#57477=CARTESIAN_POINT ( 'NONE',  ( -0.8727034120734901146, -0.05778040916215560624, -0.4822834645669293319 ) ) ;
#57478=CARTESIAN_POINT ( 'NONE',  ( 0.8923884514435703741, 0.2306618581243848609, 0.2411417322834645549 ) ) ;
#57479=CARTESIAN_POINT ( 'NONE',  ( 1.056430446194226658, 0.2952755905511811885, 0.1292274648535926551 ) ) ;
#57480=CARTESIAN_POINT ( 'NONE',  ( 0.4531182788721078158, 1.771653543307086354, 0.5309055118110234117 ) ) ;
#57481=CARTESIAN_POINT ( 'NONE',  ( -1.528871391076114250, 0.1771653543307087075, -0.09757992244046823083 ) ) ;
#57487=CARTESIAN_POINT ( 'NONE',  ( 1.194225721784777594, -0.004921259842519576551, 0.3153832671262227771 ) ) ;
#57488=CARTESIAN_POINT ( 'NONE',  ( 0.6102362204724416372, -0.4536011799217367080, 0.2665933059059888421 ) ) ;
#57489=CARTESIAN_POINT ( 'NONE',  ( 0.06561679790026316017, 0.05413385826771626580, -0.4176697321401330321 ) ) ;
#57490=CARTESIAN_POINT ( 'NONE',  ( 1.587926509186352142, 0.05413385826771666132, 0.4176697321401328100 ) ) ;
#57492=CARTESIAN_POINT ( 'NONE',  ( 0.5118110236220480003, -0.5511811023622047445, 6.969142054262312111E-17 ) ) ;
#57493=( BOUNDED_SURFACE ( )  B_SPLINE_SURFACE ( 1, 2, ( 
 ( #54758, #74136, #80464, #22368, #80049, #13663, #48436, #66160, #54339, #67822, #48027, #73305, #10159, #51933, #35825, #61491, #3839, #66575, #39316, #60663, #21534, #35410, #77638, #19970, #45621, #47194, #66995, #34997, #71315, #72885, #53921, #79633, #3011, #8500, #3425, #15234, #40894, #21951, #41309, #28678, #73727, #16066, #41712, #67405, #9739, #61074, #68633, #4646, #30738, #49675, #4240, #68238, #17713, #5069, #29904, #49263, #55568, #18528, #82504, #16897, #74965, #69864, #30317, #56805, #76191, #81276, #56401, #23592, #74552, #61899, #75779, #62309, #24413, #43341, #42536, #55985, #29499, #50083, #80869, #44171, #55158, #63547, #24820, #24007, #18120, #10573, #50487, #75365, #12215, #69042, #11392, #37873, #17311, #23181, #48851, #36632, #31138, #62731, #43753, #5476, #36230, #37049, #42939, #10973, #81696, #82099, #69459, #11809, #37464, #63137, #63959, #5881, #70693, #71532, #25646, #12624, #838, #1259, #45833, #39113, #71114, #19344, #6296, #413, #44994, #64795, #13457, #19765, #51309, #64377, #76598, #20607, #13046, #13880, #33237, #7134, #44577, #39967, #39539, #45418, #38699, #32807, #58899, #58474, #26496, #52566, #78275, #52148, #70270, #77854, #20183, #31971, #31554, #38283, #77012, #65227, #7565, #46259, #50898, #6714, #32383, #57632, #26907, #71954, #28936, #14307, #57211, #58047, #26069, #82912, #25233, #18928, #77430, #51728, #53813, #34060, #73623, #47089, #41206, #66057, #2078, #40375, #54649, #35305, #52983, #27743, #22672, #40785, #9635, #28982, #8394, #66894, #59723, #27323, #14722, #28573, #15129, #60559, #79526, #78696, #66470, #65654, #2909, #33647, #80359, #7983, #16374, #60967, #60147, #54230, #21019, #3318, #2499, #48331, #21841, #47505, #74028, #53408, #59309, #1666, #72779, #67301, #15547, #79947, #41612, #46680, #28158, #72373, #79116, #8805, #9224, #21434, #22260, #34481, #73197, #34897, #47918, #15965, #24314, #61799, #48746, #36951, #37369, #82000, #75270, #23909, #55465, #16791, #36534, #81175, #17613, #49574, #55881, #4139, #17207, #29397, #56707, #23492, #49984, #69359, #43244, #80764, #76090, #75682, #81592, #49158, #68942, #11713, #11292, #62628, #5378, #55056, #63040, #4972, #30638, #62210, #82406, #42021, #31039, #24725, #50393, #74864, #23078, #56303, #74445, #18023, #67715, #10051, #35714, #36126, #43657, #61384, #3733, #42428, #42840, #68533, #68128, #10473, #29804, #10873, #4548, #30218, #57115, #25545, #20086, #25133, #63858, #732, #26390, #65124, #63446, #6195, #76908, #82809, #52048, #39011, #50803, #1157, #77753, #76504, #51212, #45736, #71432, #12113, #6613, #37771, #32284, #70169, #13779, #83224, #18833, #44478, #57944, #77328, #12522, #38183, #31873, #7459, #39436, #5782, #57533, #58799, #19238, #33129, #26808, #44889, #19657, #70588, #31452, #12942, #64695, #38600, #13358, #311, #64278, #25965, #18434, #7034, #69769, #52466, #44076, #51623, #45319, #71014, #32704, #58370, #47823, #72682, #73524, #34380, #8709, #15873, #20921, #71855, #22164, #1979, #79847, #28059, #15449, #54132, #59209, #15030, #41521, #78597, #27642, #53716, #33547, #9131, #67206, #53304, #52885, #78174, #59624, #60462, #14621, #1570, #73097, #9539, #34802, #79423, #60045, #8294, #46576, #40686, #33962, #21743, #2401, #47408, #40275, #79017, #65552, #35209, #21336, #2812, #60871, #41108, #27224, #28889, #28471, #66796, #46988, #3224, #20505, #46159, #14205, #39861, #66372, #72273, #7883, #65958, #49483, #54967, #80264, #36856, #81494, #4868, #5283, #55788, #23810, #74350, #4459, #68849, #35622, #62530, #17113, #17520, #75176, #61285, #80674, #16694, #43152, #3637, #30124, #11197, #24218, #30541, #29305, #42334, #56205, #81906, #49889, #22580, #75590, #68443, #22987, #42748, #10783, #4048, #29713, #17929, #43565, #69266, #11613, #37273, #16280, #62948, #41926, #54549, #36443, #48241, #74764, #73937, #67619, #9949, #48653, #68032, #10377, #36034, #62116, #61708, #55376, #81082, #23399, #49066, #25035, #44791, #12844, #39330, #31354, #6100, #70072, #70487, #19985, #64596, #65016, #75996, #50298, #69675, #38085, #32603, #5685 ),
 ( #18338, #63350, #77228, #63759, #25865, #38503, #43978, #31774, #30945, #51525, #82312, #77652, #56612, #24632, #26286, #25448, #19557, #12018, #630, #51113, #51947, #64185, #6519, #45635, #57020, #37673, #58266, #57435, #71330, #32189, #45216, #6932, #82715, #76810, #13678, #50708, #76407, #18738, #70917, #44380, #57845, #13266, #12427, #38916, #83128, #19141, #212, #72991, #2707, #33019, #15344, #21229, #65448, #53195, #46884, #40173, #65857, #9024, #28367, #66689, #59938, #34277, #52364, #54029, #78070, #60360, #72578, #2294, #27538, #47719, #7351, #79741, #22057, #73417, #20816, #20401, #14925, #71747, #41006, #15766, #41418, #58689, #1464, #40585, #66267, #1054, #7780, #8190, #46471, #8606, #26708, #34697, #46053, #14100, #39752, #33448, #14520, #59108, #27120, #1878, #52784, #78493, #78908, #72165, #33857, #27954, #53613, #79321, #21641, #59521, #47301, #23708, #4762, #22886, #36749, #30438, #24119, #68749, #62016, #48966, #61183, #28786, #54448, #74248, #80576, #75489, #56103, #17829, #17010, #35939, #48138, #61608, #81807, #54870, #36342, #29204, #74666, #49788, #55685, #42650, #67102, #80160, #43053, #41821, #42236, #9433, #73835, #16591, #75075, #49379, #10687, #17422, #35102, #68347, #4353, #3537, #30021, #81392, #16175, #11092, #29612, #62425, #60769, #67512, #9849, #48550, #35520, #3120, #22477, #67930, #10271, #3951, #55272, #80983, #23296, #69574, #44692, #18236, #5183, #75896, #6420, #76311, #38403, #57334, #30847, #18642, #43463, #64083, #11511, #6835, #69160, #77558, #38819, #37988, #32089, #82214, #13169, #63664, #64497, #83028, #25351, #32505, #11922, #37167, #70821, #50604, #45114, #76712, #57750, #19464, #24533, #6004, #58168, #43876, #44286, #19045, #50199, #112, #537, #69976, #37577, #62847, #24934, #25767, #63250, #5589, #51428, #26190, #77131, #70389, #51013, #56924, #31256, #31673, #82618, #12744, #51851, #56512, #12330, #78396, #7258, #34605, #33357, #59847, #47211, #21143, #58595, #53938, #53527, #33767, #27027, #1784, #72901, #59429, #46798, #15252, #40083, #20306, #79235, #27444, #14838, #45956, #45539, #26618, #65352, #2199, #27867, #66593, #64920, #7690, #20728, #964, #21550, #40498, #52271, #2620, #40912, #77976, #52688, #8928, #60270, #13581, #8102, #39235, #53105, #71653, #28276, #1375, #14005, #39662, #78814, #72489, #66178, #46379, #8516, #19891, #34183, #71237, #32930, #65770, #59020, #72072, #14431, #74570, #80067, #21967, #3028, #41727, #61917, #4259, #42957, #41331, #67421, #54776, #60679, #29922, #16915, #28694, #62325, #55585, #35015, #29105, #81297, #49280, #73323, #67838, #15669, #10177, #48045, #23611, #61091, #54356, #22385, #35842, #55177, #73746, #16082, #9754, #68651, #74983, #67011, #35426, #36650, #80479, #17328, #10989, #3442, #80886, #22792, #9344, #48452, #42553, #74152, #68256, #61510, #16499, #42143, #79650, #10591, #47628, #5802, #3856, #31472, #29516, #23199, #36248, #48870, #26826, #51641, #52484, #13376, #71032, #78192, #83241, #50821, #1175, #64295, #58818, #7054, #77771, #33149, #38200, #77346, #20523, #57550, #6629, #32722, #12542, #71449, #46175, #32301, #31890, #57134, #38617, #39455, #76927, #63875, #52064, #71871, #13797, #58389, #39029, #70605, #25563, #19677, #12960, #750, #64713, #26411, #19255, #57962, #44497, #14221, #329, #65142, #39881, #20103, #6214, #7902, #7479, #45753, #51229, #65568, #82831, #25983, #44907, #25153, #45336, #76523, #18851, #70188, #28488, #28902, #73543, #66813, #15464, #47005, #8311, #28074, #72699, #9146, #41122, #47422, #79033, #8724, #20937, #48254, #15046, #15886, #60888, #34818, #72291, #67635, #67222, #73113, #40702, #60476, #3238, #2827, #54148, #54565, #53732, #33978, #9554, #79862, #22179, #59639, #59225, #40293, #21352, #41535, #35224, #80280, #78613, #66386, #34395, #14637, #22593, #47837, #65974, #16296, #73950, #1995, #60063, #41939, #33563, #27241, #21759, #52900, #1586, #27658, #46595, #2417, #53324, #79440, #81506, #68861, #10393, #29726, #68046, #82325, #62961, #80688, #55388, #50311, #68457, #37286, #56625, #36049, #11210, #61722 ) ),
 .UNSPECIFIED., .F., .F., .F. ) 
 B_SPLINE_SURFACE_WITH_KNOTS ( ( 2, 2 ),
 ( 3, 2, 2, 2, 2, 2, 2, 2, 2, 2, 2, 2, 2, 2, 2, 2, 2, 2, 2, 2, 2, 2, 2, 2, 2, 2, 2, 2, 2, 2, 2, 2, 2, 2, 2, 2, 2, 2, 2, 2, 2, 2, 2, 2, 2, 2, 2, 2, 2, 2, 2, 2, 2, 2, 2, 2, 2, 2, 2, 2, 2, 2, 2, 2, 2, 2, 2, 2, 2, 2, 2, 2, 2, 2, 2, 2, 2, 2, 2, 2, 2, 2, 2, 2, 2, 2, 2, 2, 2, 2, 2, 2, 2, 2, 2, 2, 2, 2, 2, 2, 2, 2, 2, 2, 2, 2, 2, 2, 2, 2, 2, 2, 2, 2, 2, 2, 2, 2, 2, 2, 2, 2, 2, 2, 2, 2, 2, 2, 2, 2, 2, 2, 2, 2, 2, 2, 2, 2, 2, 2, 2, 2, 2, 2, 2, 2, 2, 2, 2, 2, 2, 2, 2, 2, 2, 2, 2, 2, 2, 2, 2, 2, 2, 2, 2, 2, 2, 2, 2, 2, 2, 2, 2, 2, 2, 2, 2, 2, 2, 2, 2, 2, 2, 2, 2, 2, 2, 2, 2, 2, 2, 2, 2, 2, 2, 2, 2, 2, 2, 2, 2, 2, 2, 2, 2, 2, 2, 2, 2, 2, 2, 2, 2, 2, 2, 2, 2, 2, 2, 2, 2, 2, 2, 2, 2, 2, 2, 2, 2, 2, 2, 2, 2, 2, 2, 2, 2, 2, 2, 2, 2, 2, 2, 2, 2, 2, 2, 2, 2, 2, 2, 2, 2, 2, 2, 3 ),
 ( 0.000000000000000000, 1.000000000000000000 ),
 ( 0.000000000000000000, 0.003787878787878787984, 0.007575757575757575968, 0.01136363636363636395, 0.01515151515151515194, 0.01893939393939393992, 0.02272727272727272790, 0.02651515151515151589, 0.03030303030303030387, 0.03409090909090908839, 0.03787878787878787984, 0.04166666666666666435, 0.04545454545454545581, 0.04924242424242424032, 0.05303030303030303177, 0.05681818181818181629, 0.06060606060606060774, 0.06439393939393939226, 0.06818181818181817677, 0.07196969696969697516, 0.07575757575757575968, 0.07954545454545454419, 0.08333333333333332871, 0.08712121212121212710, 0.09090909090909091161, 0.09469696969696969613, 0.09848484848484848064, 0.1022727272727272790, 0.1060606060606060635, 0.1098484848484848481, 0.1136363636363636326, 0.1174242424242424310, 0.1212121212121212155, 0.1250000000000000000, 0.1287878787878787845, 0.1325757575757575690, 0.1363636363636363535, 0.1401515151515151381, 0.1439393939393939503, 0.1477272727272727348, 0.1515151515151515194, 0.1553030303030303039, 0.1590909090909090884, 0.1628787878787878729, 0.1666666666666666574, 0.1704545454545454419, 0.1742424242424242542, 0.1780303030303030387, 0.1818181818181818232, 0.1856060606060606077, 0.1893939393939393923, 0.1931818181818181768, 0.1969696969696969613, 0.2007575757575757458, 0.2045454545454545581, 0.2083333333333333426, 0.2121212121212121271, 0.2159090909090909116, 0.2196969696969696961, 0.2234848484848484806, 0.2272727272727272652, 0.2310606060606060497, 0.2348484848484848619, 0.2386363636363636465, 0.2424242424242424310, 0.2462121212121212155, 0.2500000000000000000, 0.2537878787878787845, 0.2575757575757575690, 0.2613636363636363535, 0.2651515151515151381, 0.2689393939393939226, 0.2727272727272727071, 0.2765151515151514916, 0.2803030303030302761, 0.2840909090909091161, 0.2878787878787879007, 0.2916666666666666852, 0.2954545454545454697, 0.2992424242424242542, 0.3030303030303030387, 0.3068181818181818232, 0.3106060606060606077, 0.3143939393939393923, 0.3181818181818181768, 0.3219696969696969613, 0.3257575757575757458, 0.3295454545454545303, 0.3333333333333333148, 0.3371212121212120993, 0.3409090909090908839, 0.3446969696969697239, 0.3484848484848485084, 0.3522727272727272929, 0.3560606060606060774, 0.3598484848484848619, 0.3636363636363636465, 0.3674242424242424310, 0.3712121212121212155, 0.3750000000000000000, 0.3787878787878787845, 0.3825757575757575690, 0.3863636363636363535, 0.3901515151515151381, 0.3939393939393939226, 0.3977272727272727071, 0.4015151515151514916, 0.4053030303030302761, 0.4090909090909091161, 0.4128787878787879007, 0.4166666666666666852, 0.4204545454545454697, 0.4242424242424242542, 0.4280303030303030387, 0.4318181818181818232, 0.4356060606060606077, 0.4393939393939393923, 0.4431818181818181768, 0.4469696969696969613, 0.4507575757575757458, 0.4545454545454545303, 0.4583333333333333148, 0.4621212121212120993, 0.4659090909090908839, 0.4696969696969697239, 0.4734848484848485084, 0.4772727272727272929, 0.4810606060606060774, 0.4848484848484848619, 0.4886363636363636465, 0.4924242424242424310, 0.4962121212121212155, 0.5000000000000000000, 0.5037878787878787845, 0.5075757575757575690, 0.5113636363636363535, 0.5151515151515151381, 0.5189393939393939226, 0.5227272727272727071, 0.5265151515151514916, 0.5303030303030302761, 0.5340909090909090606, 0.5378787878787878451, 0.5416666666666666297, 0.5454545454545454142, 0.5492424242424241987, 0.5530303030303029832, 0.5568181818181817677, 0.5606060606060605522, 0.5643939393939394478, 0.5681818181818182323, 0.5719696969696970168, 0.5757575757575758013, 0.5795454545454545858, 0.5833333333333333703, 0.5871212121212121549, 0.5909090909090909394, 0.5946969696969697239, 0.5984848484848485084, 0.6022727272727272929, 0.6060606060606060774, 0.6098484848484848619, 0.6136363636363636465, 0.6174242424242424310, 0.6212121212121212155, 0.6250000000000000000, 0.6287878787878787845, 0.6325757575757575690, 0.6363636363636363535, 0.6401515151515151381, 0.6439393939393939226, 0.6477272727272727071, 0.6515151515151514916, 0.6553030303030302761, 0.6590909090909090606, 0.6628787878787878451, 0.6666666666666666297, 0.6704545454545454142, 0.6742424242424241987, 0.6780303030303029832, 0.6818181818181817677, 0.6856060606060605522, 0.6893939393939394478, 0.6931818181818182323, 0.6969696969696970168, 0.7007575757575758013, 0.7045454545454545858, 0.7083333333333333703, 0.7121212121212121549, 0.7159090909090909394, 0.7196969696969697239, 0.7234848484848485084, 0.7272727272727272929, 0.7310606060606060774, 0.7348484848484848619, 0.7386363636363636465, 0.7424242424242424310, 0.7462121212121212155, 0.7500000000000000000, 0.7537878787878787845, 0.7575757575757575690, 0.7613636363636363535, 0.7651515151515151381, 0.7689393939393939226, 0.7727272727272727071, 0.7765151515151514916, 0.7803030303030302761, 0.7840909090909090606, 0.7878787878787878451, 0.7916666666666666297, 0.7954545454545454142, 0.7992424242424241987, 0.8030303030303029832, 0.8068181818181817677, 0.8106060606060605522, 0.8143939393939394478, 0.8181818181818182323, 0.8219696969696970168, 0.8257575757575758013, 0.8295454545454545858, 0.8333333333333333703, 0.8371212121212121549, 0.8409090909090909394, 0.8446969696969697239, 0.8484848484848485084, 0.8522727272727272929, 0.8560606060606060774, 0.8598484848484848619, 0.8636363636363636465, 0.8674242424242424310, 0.8712121212121212155, 0.8750000000000000000, 0.8787878787878787845, 0.8825757575757575690, 0.8863636363636363535, 0.8901515151515151381, 0.8939393939393939226, 0.8977272727272727071, 0.9015151515151514916, 0.9053030303030302761, 0.9090909090909090606, 0.9128787878787878451, 0.9166666666666666297, 0.9204545454545454142, 0.9242424242424241987, 0.9280303030303029832, 0.9318181818181817677, 0.9356060606060605522, 0.9393939393939394478, 0.9431818181818182323, 0.9469696969696970168, 0.9507575757575758013, 0.9545454545454545858, 0.9583333333333333703, 0.9621212121212121549, 0.9659090909090909394 ),
 .UNSPECIFIED. ) 
 GEOMETRIC_REPRESENTATION_ITEM ( )  RATIONAL_B_SPLINE_SURFACE ( (
 ( 1.000000000000000000, 0.9659258262890683122, 1.000000000000000000, 0.9659258262890683122, 1.000000000000000000, 0.9659258262890683122, 1.000000000000000000, 0.9659258262890683122, 1.000000000000000000, 0.9659258262890683122, 1.000000000000000000, 0.9659258262890683122, 1.000000000000000000, 0.9659258262890683122, 1.000000000000000000, 0.9659258262890683122, 1.000000000000000000, 0.9659258262890683122, 1.000000000000000000, 0.9659258262890683122, 1.000000000000000000, 0.9659258262890683122, 1.000000000000000000, 0.9659258262890683122, 1.000000000000000000, 0.9659258262890683122, 1.000000000000000000, 0.9659258262890683122, 1.000000000000000000, 0.9659258262890683122, 1.000000000000000000, 0.9659258262890683122, 1.000000000000000000, 0.9659258262890683122, 1.000000000000000000, 0.9659258262890683122, 1.000000000000000000, 0.9659258262890683122, 1.000000000000000000, 0.9659258262890683122, 1.000000000000000000, 0.9659258262890683122, 1.000000000000000000, 0.9659258262890683122, 1.000000000000000000, 0.9659258262890683122, 1.000000000000000000, 0.9659258262890683122, 1.000000000000000000, 0.9659258262890683122, 1.000000000000000000, 0.9659258262890683122, 1.000000000000000000, 0.9659258262890683122, 1.000000000000000000, 0.9659258262890683122, 1.000000000000000000, 0.9659258262890683122, 1.000000000000000000, 0.9659258262890683122, 1.000000000000000000, 0.9659258262890683122, 1.000000000000000000, 0.9659258262890683122, 1.000000000000000000, 0.9659258262890683122, 1.000000000000000000, 0.9659258262890683122, 1.000000000000000000, 0.9659258262890683122, 1.000000000000000000, 0.9659258262890683122, 1.000000000000000000, 0.9659258262890683122, 1.000000000000000000, 0.9659258262890683122, 1.000000000000000000, 0.9659258262890683122, 1.000000000000000000, 0.9659258262890683122, 1.000000000000000000, 0.9659258262890683122, 1.000000000000000000, 0.9659258262890683122, 1.000000000000000000, 0.9659258262890683122, 1.000000000000000000, 0.9659258262890683122, 1.000000000000000000, 0.9659258262890683122, 1.000000000000000000, 0.9659258262890683122, 1.000000000000000000, 0.9659258262890683122, 1.000000000000000000, 0.9659258262890683122, 1.000000000000000000, 0.9659258262890683122, 1.000000000000000000, 0.9659258262890683122, 1.000000000000000000, 0.9659258262890683122, 1.000000000000000000, 0.9659258262890683122, 1.000000000000000000, 0.9659258262890683122, 1.000000000000000000, 0.9659258262890683122, 1.000000000000000000, 0.9659258262890683122, 1.000000000000000000, 0.9659258262890683122, 1.000000000000000000, 0.9659258262890683122, 1.000000000000000000, 0.9659258262890683122, 1.000000000000000000, 0.9659258262890683122, 1.000000000000000000, 0.9659258262890683122, 1.000000000000000000, 0.9659258262890683122, 1.000000000000000000, 0.9659258262890683122, 1.000000000000000000, 0.9659258262890683122, 1.000000000000000000, 0.9659258262890683122, 1.000000000000000000, 0.9659258262890683122, 1.000000000000000000, 0.9659258262890683122, 1.000000000000000000, 0.9659258262890683122, 1.000000000000000000, 0.9659258262890683122, 1.000000000000000000, 0.9659258262890683122, 1.000000000000000000, 0.9659258262890683122, 1.000000000000000000, 0.9659258262890683122, 1.000000000000000000, 0.9659258262890683122, 1.000000000000000000, 0.9659258262890683122, 1.000000000000000000, 0.9659258262890683122, 1.000000000000000000, 0.9659258262890683122, 1.000000000000000000, 0.9659258262890683122, 1.000000000000000000, 0.9659258262890683122, 1.000000000000000000, 0.9659258262890683122, 1.000000000000000000, 0.9659258262890683122, 1.000000000000000000, 0.9659258262890683122, 1.000000000000000000, 0.9659258262890683122, 1.000000000000000000, 0.9659258262890683122, 1.000000000000000000, 0.9659258262890683122, 1.000000000000000000, 0.9659258262890683122, 1.000000000000000000, 0.9659258262890683122, 1.000000000000000000, 0.9659258262890683122, 1.000000000000000000, 0.9659258262890683122, 1.000000000000000000, 0.9659258262890683122, 1.000000000000000000, 0.9659258262890683122, 1.000000000000000000, 0.9659258262890683122, 1.000000000000000000, 0.9659258262890683122, 1.000000000000000000, 0.9659258262890683122, 1.000000000000000000, 0.9659258262890683122, 1.000000000000000000, 0.9659258262890683122, 1.000000000000000000, 0.9659258262890683122, 1.000000000000000000, 0.9659258262890683122, 1.000000000000000000, 0.9659258262890683122, 1.000000000000000000, 0.9659258262890683122, 1.000000000000000000, 0.9659258262890683122, 1.000000000000000000, 0.9659258262890683122, 1.000000000000000000, 0.9659258262890683122, 1.000000000000000000, 0.9659258262890683122, 1.000000000000000000, 0.9659258262890683122, 1.000000000000000000, 0.9659258262890683122, 1.000000000000000000, 0.9659258262890683122, 1.000000000000000000, 0.9659258262890683122, 1.000000000000000000, 0.9659258262890683122, 1.000000000000000000, 0.9659258262890683122, 1.000000000000000000, 0.9659258262890683122, 1.000000000000000000, 0.9659258262890683122, 1.000000000000000000, 0.9659258262890683122, 1.000000000000000000, 0.9659258262890683122, 1.000000000000000000, 0.9659258262890683122, 1.000000000000000000, 0.9659258262890683122, 1.000000000000000000, 0.9659258262890683122, 1.000000000000000000, 0.9659258262890683122, 1.000000000000000000, 0.9659258262890683122, 1.000000000000000000, 0.9659258262890683122, 1.000000000000000000, 0.9659258262890683122, 1.000000000000000000, 0.9659258262890683122, 1.000000000000000000, 0.9659258262890683122, 1.000000000000000000, 0.9659258262890683122, 1.000000000000000000, 0.9659258262890683122, 1.000000000000000000, 0.9659258262890683122, 1.000000000000000000, 0.9659258262890683122, 1.000000000000000000, 0.9659258262890683122, 1.000000000000000000, 0.9659258262890683122, 1.000000000000000000, 0.9659258262890683122, 1.000000000000000000, 0.9659258262890683122, 1.000000000000000000, 0.9659258262890683122, 1.000000000000000000, 0.9659258262890683122, 1.000000000000000000, 0.9659258262890683122, 1.000000000000000000, 0.9659258262890683122, 1.000000000000000000, 0.9659258262890683122, 1.000000000000000000, 0.9659258262890683122, 1.000000000000000000, 0.9659258262890683122, 1.000000000000000000, 0.9659258262890683122, 1.000000000000000000, 0.9659258262890683122, 1.000000000000000000, 0.9659258262890683122, 1.000000000000000000, 0.9659258262890683122, 1.000000000000000000, 0.9659258262890683122, 1.000000000000000000, 0.9659258262890683122, 1.000000000000000000, 0.9659258262890683122, 1.000000000000000000, 0.9659258262890683122, 1.000000000000000000, 0.9659258262890683122, 1.000000000000000000, 0.9659258262890683122, 1.000000000000000000, 0.9659258262890683122, 1.000000000000000000, 0.9659258262890683122, 1.000000000000000000, 0.9659258262890683122, 1.000000000000000000, 0.9659258262890683122, 1.000000000000000000, 0.9659258262890683122, 1.000000000000000000, 0.9659258262890683122, 1.000000000000000000, 0.9659258262890683122, 1.000000000000000000, 0.9659258262890683122, 1.000000000000000000, 0.9659258262890683122, 1.000000000000000000, 0.9659258262890683122, 1.000000000000000000, 0.9659258262890683122, 1.000000000000000000, 0.9659258262890683122, 1.000000000000000000, 0.9659258262890683122, 1.000000000000000000, 0.9659258262890683122, 1.000000000000000000, 0.9659258262890683122, 1.000000000000000000, 0.9659258262890683122, 1.000000000000000000, 0.9659258262890683122, 1.000000000000000000, 0.9659258262890683122, 1.000000000000000000, 0.9659258262890683122, 1.000000000000000000, 0.9659258262890683122, 1.000000000000000000, 0.9659258262890683122, 1.000000000000000000, 0.9659258262890683122, 1.000000000000000000, 0.9659258262890683122, 1.000000000000000000, 0.9659258262890683122, 1.000000000000000000, 0.9659258262890683122, 1.000000000000000000, 0.9659258262890683122, 1.000000000000000000, 0.9659258262890683122, 1.000000000000000000, 0.9659258262890683122, 1.000000000000000000, 0.9659258262890683122, 1.000000000000000000, 0.9659258262890683122, 1.000000000000000000, 0.9659258262890683122, 1.000000000000000000, 0.9659258262890683122, 1.000000000000000000, 0.9659258262890683122, 1.000000000000000000, 0.9659258262890683122, 1.000000000000000000, 0.9659258262890683122, 1.000000000000000000, 0.9659258262890683122, 1.000000000000000000, 0.9659258262890683122, 1.000000000000000000, 0.9659258262890683122, 1.000000000000000000, 0.9659258262890683122, 1.000000000000000000, 0.9659258262890683122, 1.000000000000000000, 0.9659258262890683122, 1.000000000000000000, 0.9659258262890683122, 1.000000000000000000, 0.9659258262890683122, 1.000000000000000000, 0.9659258262890683122, 1.000000000000000000, 0.9659258262890683122, 1.000000000000000000, 0.9659258262890683122, 1.000000000000000000, 0.9659258262890683122, 1.000000000000000000, 0.9659258262890683122, 1.000000000000000000, 0.9659258262890683122, 1.000000000000000000, 0.9659258262890683122, 1.000000000000000000, 0.9659258262890683122, 1.000000000000000000, 0.9659258262890683122, 1.000000000000000000, 0.9659258262890683122, 1.000000000000000000, 0.9659258262890683122, 1.000000000000000000, 0.9659258262890683122, 1.000000000000000000, 0.9659258262890683122, 1.000000000000000000, 0.9659258262890683122, 1.000000000000000000, 0.9659258262890683122, 1.000000000000000000, 0.9659258262890683122, 1.000000000000000000, 0.9659258262890683122, 1.000000000000000000, 0.9659258262890683122, 1.000000000000000000, 0.9659258262890683122, 1.000000000000000000, 0.9659258262890683122, 1.000000000000000000, 0.9659258262890683122, 1.000000000000000000, 0.9659258262890683122, 1.000000000000000000, 0.9659258262890683122, 1.000000000000000000, 0.9659258262890683122, 1.000000000000000000, 0.9659258262890683122, 1.000000000000000000, 0.9659258262890683122, 1.000000000000000000, 0.9659258262890683122, 1.000000000000000000, 0.9659258262890683122, 1.000000000000000000, 0.9659258262890683122, 1.000000000000000000, 0.9659258262890683122, 1.000000000000000000, 0.9659258262890683122, 1.000000000000000000, 0.9659258262890683122, 1.000000000000000000, 0.9659258262890683122, 1.000000000000000000, 0.9659258262890683122, 1.000000000000000000, 0.9659258262890683122, 1.000000000000000000, 0.9659258262890683122, 1.000000000000000000, 0.9659258262890683122, 1.000000000000000000, 0.9659258262890683122, 1.000000000000000000, 0.9659258262890683122, 1.000000000000000000, 0.9659258262890683122, 1.000000000000000000, 0.9659258262890683122, 1.000000000000000000, 0.9659258262890683122, 1.000000000000000000, 0.9659258262890683122, 1.000000000000000000, 0.9659258262890683122, 1.000000000000000000, 0.9659258262890683122, 1.000000000000000000, 0.9659258262890683122, 1.000000000000000000, 0.9659258262890683122, 1.000000000000000000, 0.9659258262890683122, 1.000000000000000000, 0.9659258262890683122, 1.000000000000000000, 0.9659258262890683122, 1.000000000000000000, 0.9659258262890683122, 1.000000000000000000, 0.9659258262890683122, 1.000000000000000000, 0.9659258262890683122, 1.000000000000000000, 0.9659258262890683122, 1.000000000000000000, 0.9659258262890683122, 1.000000000000000000, 0.9659258262890683122, 1.000000000000000000, 0.9659258262890683122, 1.000000000000000000, 0.9659258262890683122, 1.000000000000000000, 0.9659258262890683122, 1.000000000000000000, 0.9659258262890683122, 1.000000000000000000, 0.9659258262890683122, 1.000000000000000000, 0.9659258262890683122, 1.000000000000000000, 0.9659258262890683122, 1.000000000000000000, 0.9659258262890683122, 1.000000000000000000, 0.9659258262890683122, 1.000000000000000000, 0.9659258262890683122, 1.000000000000000000),
 ( 1.000000000000000000, 0.9659258262890683122, 1.000000000000000000, 0.9659258262890683122, 1.000000000000000000, 0.9659258262890683122, 1.000000000000000000, 0.9659258262890683122, 1.000000000000000000, 0.9659258262890683122, 1.000000000000000000, 0.9659258262890683122, 1.000000000000000000, 0.9659258262890683122, 1.000000000000000000, 0.9659258262890683122, 1.000000000000000000, 0.9659258262890683122, 1.000000000000000000, 0.9659258262890683122, 1.000000000000000000, 0.9659258262890683122, 1.000000000000000000, 0.9659258262890683122, 1.000000000000000000, 0.9659258262890683122, 1.000000000000000000, 0.9659258262890683122, 1.000000000000000000, 0.9659258262890683122, 1.000000000000000000, 0.9659258262890683122, 1.000000000000000000, 0.9659258262890683122, 1.000000000000000000, 0.9659258262890683122, 1.000000000000000000, 0.9659258262890683122, 1.000000000000000000, 0.9659258262890683122, 1.000000000000000000, 0.9659258262890683122, 1.000000000000000000, 0.9659258262890683122, 1.000000000000000000, 0.9659258262890683122, 1.000000000000000000, 0.9659258262890683122, 1.000000000000000000, 0.9659258262890683122, 1.000000000000000000, 0.9659258262890683122, 1.000000000000000000, 0.9659258262890683122, 1.000000000000000000, 0.9659258262890683122, 1.000000000000000000, 0.9659258262890683122, 1.000000000000000000, 0.9659258262890683122, 1.000000000000000000, 0.9659258262890683122, 1.000000000000000000, 0.9659258262890683122, 1.000000000000000000, 0.9659258262890683122, 1.000000000000000000, 0.9659258262890683122, 1.000000000000000000, 0.9659258262890683122, 1.000000000000000000, 0.9659258262890683122, 1.000000000000000000, 0.9659258262890683122, 1.000000000000000000, 0.9659258262890683122, 1.000000000000000000, 0.9659258262890683122, 1.000000000000000000, 0.9659258262890683122, 1.000000000000000000, 0.9659258262890683122, 1.000000000000000000, 0.9659258262890683122, 1.000000000000000000, 0.9659258262890683122, 1.000000000000000000, 0.9659258262890683122, 1.000000000000000000, 0.9659258262890683122, 1.000000000000000000, 0.9659258262890683122, 1.000000000000000000, 0.9659258262890683122, 1.000000000000000000, 0.9659258262890683122, 1.000000000000000000, 0.9659258262890683122, 1.000000000000000000, 0.9659258262890683122, 1.000000000000000000, 0.9659258262890683122, 1.000000000000000000, 0.9659258262890683122, 1.000000000000000000, 0.9659258262890683122, 1.000000000000000000, 0.9659258262890683122, 1.000000000000000000, 0.9659258262890683122, 1.000000000000000000, 0.9659258262890683122, 1.000000000000000000, 0.9659258262890683122, 1.000000000000000000, 0.9659258262890683122, 1.000000000000000000, 0.9659258262890683122, 1.000000000000000000, 0.9659258262890683122, 1.000000000000000000, 0.9659258262890683122, 1.000000000000000000, 0.9659258262890683122, 1.000000000000000000, 0.9659258262890683122, 1.000000000000000000, 0.9659258262890683122, 1.000000000000000000, 0.9659258262890683122, 1.000000000000000000, 0.9659258262890683122, 1.000000000000000000, 0.9659258262890683122, 1.000000000000000000, 0.9659258262890683122, 1.000000000000000000, 0.9659258262890683122, 1.000000000000000000, 0.9659258262890683122, 1.000000000000000000, 0.9659258262890683122, 1.000000000000000000, 0.9659258262890683122, 1.000000000000000000, 0.9659258262890683122, 1.000000000000000000, 0.9659258262890683122, 1.000000000000000000, 0.9659258262890683122, 1.000000000000000000, 0.9659258262890683122, 1.000000000000000000, 0.9659258262890683122, 1.000000000000000000, 0.9659258262890683122, 1.000000000000000000, 0.9659258262890683122, 1.000000000000000000, 0.9659258262890683122, 1.000000000000000000, 0.9659258262890683122, 1.000000000000000000, 0.9659258262890683122, 1.000000000000000000, 0.9659258262890683122, 1.000000000000000000, 0.9659258262890683122, 1.000000000000000000, 0.9659258262890683122, 1.000000000000000000, 0.9659258262890683122, 1.000000000000000000, 0.9659258262890683122, 1.000000000000000000, 0.9659258262890683122, 1.000000000000000000, 0.9659258262890683122, 1.000000000000000000, 0.9659258262890683122, 1.000000000000000000, 0.9659258262890683122, 1.000000000000000000, 0.9659258262890683122, 1.000000000000000000, 0.9659258262890683122, 1.000000000000000000, 0.9659258262890683122, 1.000000000000000000, 0.9659258262890683122, 1.000000000000000000, 0.9659258262890683122, 1.000000000000000000, 0.9659258262890683122, 1.000000000000000000, 0.9659258262890683122, 1.000000000000000000, 0.9659258262890683122, 1.000000000000000000, 0.9659258262890683122, 1.000000000000000000, 0.9659258262890683122, 1.000000000000000000, 0.9659258262890683122, 1.000000000000000000, 0.9659258262890683122, 1.000000000000000000, 0.9659258262890683122, 1.000000000000000000, 0.9659258262890683122, 1.000000000000000000, 0.9659258262890683122, 1.000000000000000000, 0.9659258262890683122, 1.000000000000000000, 0.9659258262890683122, 1.000000000000000000, 0.9659258262890683122, 1.000000000000000000, 0.9659258262890683122, 1.000000000000000000, 0.9659258262890683122, 1.000000000000000000, 0.9659258262890683122, 1.000000000000000000, 0.9659258262890683122, 1.000000000000000000, 0.9659258262890683122, 1.000000000000000000, 0.9659258262890683122, 1.000000000000000000, 0.9659258262890683122, 1.000000000000000000, 0.9659258262890683122, 1.000000000000000000, 0.9659258262890683122, 1.000000000000000000, 0.9659258262890683122, 1.000000000000000000, 0.9659258262890683122, 1.000000000000000000, 0.9659258262890683122, 1.000000000000000000, 0.9659258262890683122, 1.000000000000000000, 0.9659258262890683122, 1.000000000000000000, 0.9659258262890683122, 1.000000000000000000, 0.9659258262890683122, 1.000000000000000000, 0.9659258262890683122, 1.000000000000000000, 0.9659258262890683122, 1.000000000000000000, 0.9659258262890683122, 1.000000000000000000, 0.9659258262890683122, 1.000000000000000000, 0.9659258262890683122, 1.000000000000000000, 0.9659258262890683122, 1.000000000000000000, 0.9659258262890683122, 1.000000000000000000, 0.9659258262890683122, 1.000000000000000000, 0.9659258262890683122, 1.000000000000000000, 0.9659258262890683122, 1.000000000000000000, 0.9659258262890683122, 1.000000000000000000, 0.9659258262890683122, 1.000000000000000000, 0.9659258262890683122, 1.000000000000000000, 0.9659258262890683122, 1.000000000000000000, 0.9659258262890683122, 1.000000000000000000, 0.9659258262890683122, 1.000000000000000000, 0.9659258262890683122, 1.000000000000000000, 0.9659258262890683122, 1.000000000000000000, 0.9659258262890683122, 1.000000000000000000, 0.9659258262890683122, 1.000000000000000000, 0.9659258262890683122, 1.000000000000000000, 0.9659258262890683122, 1.000000000000000000, 0.9659258262890683122, 1.000000000000000000, 0.9659258262890683122, 1.000000000000000000, 0.9659258262890683122, 1.000000000000000000, 0.9659258262890683122, 1.000000000000000000, 0.9659258262890683122, 1.000000000000000000, 0.9659258262890683122, 1.000000000000000000, 0.9659258262890683122, 1.000000000000000000, 0.9659258262890683122, 1.000000000000000000, 0.9659258262890683122, 1.000000000000000000, 0.9659258262890683122, 1.000000000000000000, 0.9659258262890683122, 1.000000000000000000, 0.9659258262890683122, 1.000000000000000000, 0.9659258262890683122, 1.000000000000000000, 0.9659258262890683122, 1.000000000000000000, 0.9659258262890683122, 1.000000000000000000, 0.9659258262890683122, 1.000000000000000000, 0.9659258262890683122, 1.000000000000000000, 0.9659258262890683122, 1.000000000000000000, 0.9659258262890683122, 1.000000000000000000, 0.9659258262890683122, 1.000000000000000000, 0.9659258262890683122, 1.000000000000000000, 0.9659258262890683122, 1.000000000000000000, 0.9659258262890683122, 1.000000000000000000, 0.9659258262890683122, 1.000000000000000000, 0.9659258262890683122, 1.000000000000000000, 0.9659258262890683122, 1.000000000000000000, 0.9659258262890683122, 1.000000000000000000, 0.9659258262890683122, 1.000000000000000000, 0.9659258262890683122, 1.000000000000000000, 0.9659258262890683122, 1.000000000000000000, 0.9659258262890683122, 1.000000000000000000, 0.9659258262890683122, 1.000000000000000000, 0.9659258262890683122, 1.000000000000000000, 0.9659258262890683122, 1.000000000000000000, 0.9659258262890683122, 1.000000000000000000, 0.9659258262890683122, 1.000000000000000000, 0.9659258262890683122, 1.000000000000000000, 0.9659258262890683122, 1.000000000000000000, 0.9659258262890683122, 1.000000000000000000, 0.9659258262890683122, 1.000000000000000000, 0.9659258262890683122, 1.000000000000000000, 0.9659258262890683122, 1.000000000000000000, 0.9659258262890683122, 1.000000000000000000, 0.9659258262890683122, 1.000000000000000000, 0.9659258262890683122, 1.000000000000000000, 0.9659258262890683122, 1.000000000000000000, 0.9659258262890683122, 1.000000000000000000, 0.9659258262890683122, 1.000000000000000000, 0.9659258262890683122, 1.000000000000000000, 0.9659258262890683122, 1.000000000000000000, 0.9659258262890683122, 1.000000000000000000, 0.9659258262890683122, 1.000000000000000000, 0.9659258262890683122, 1.000000000000000000, 0.9659258262890683122, 1.000000000000000000, 0.9659258262890683122, 1.000000000000000000, 0.9659258262890683122, 1.000000000000000000, 0.9659258262890683122, 1.000000000000000000, 0.9659258262890683122, 1.000000000000000000, 0.9659258262890683122, 1.000000000000000000, 0.9659258262890683122, 1.000000000000000000, 0.9659258262890683122, 1.000000000000000000, 0.9659258262890683122, 1.000000000000000000, 0.9659258262890683122, 1.000000000000000000, 0.9659258262890683122, 1.000000000000000000, 0.9659258262890683122, 1.000000000000000000, 0.9659258262890683122, 1.000000000000000000, 0.9659258262890683122, 1.000000000000000000, 0.9659258262890683122, 1.000000000000000000, 0.9659258262890683122, 1.000000000000000000, 0.9659258262890683122, 1.000000000000000000, 0.9659258262890683122, 1.000000000000000000, 0.9659258262890683122, 1.000000000000000000, 0.9659258262890683122, 1.000000000000000000, 0.9659258262890683122, 1.000000000000000000, 0.9659258262890683122, 1.000000000000000000, 0.9659258262890683122, 1.000000000000000000, 0.9659258262890683122, 1.000000000000000000, 0.9659258262890683122, 1.000000000000000000, 0.9659258262890683122, 1.000000000000000000, 0.9659258262890683122, 1.000000000000000000, 0.9659258262890683122, 1.000000000000000000, 0.9659258262890683122, 1.000000000000000000, 0.9659258262890683122, 1.000000000000000000, 0.9659258262890683122, 1.000000000000000000, 0.9659258262890683122, 1.000000000000000000, 0.9659258262890683122, 1.000000000000000000, 0.9659258262890683122, 1.000000000000000000, 0.9659258262890683122, 1.000000000000000000, 0.9659258262890683122, 1.000000000000000000, 0.9659258262890683122, 1.000000000000000000, 0.9659258262890683122, 1.000000000000000000, 0.9659258262890683122, 1.000000000000000000, 0.9659258262890683122, 1.000000000000000000, 0.9659258262890683122, 1.000000000000000000, 0.9659258262890683122, 1.000000000000000000, 0.9659258262890683122, 1.000000000000000000, 0.9659258262890683122, 1.000000000000000000, 0.9659258262890683122, 1.000000000000000000, 0.9659258262890683122, 1.000000000000000000, 0.9659258262890683122, 1.000000000000000000, 0.9659258262890683122, 1.000000000000000000, 0.9659258262890683122, 1.000000000000000000, 0.9659258262890683122, 1.000000000000000000, 0.9659258262890683122, 1.000000000000000000, 0.9659258262890683122, 1.000000000000000000, 0.9659258262890683122, 1.000000000000000000, 0.9659258262890683122, 1.000000000000000000, 0.9659258262890683122, 1.000000000000000000) ) ) 
 REPRESENTATION_ITEM ( '' )  SURFACE ( )  );
#57494=CARTESIAN_POINT ( 'NONE',  ( -0.8530183727034112984, 0.05413385826771666132, 0.4176697321401328100 ) ) ;
#57495=CARTESIAN_POINT ( 'NONE',  ( -1.069553805774277722, -0.6692913385826773087, -0.1292274648535924053 ) ) ;
#57496=CARTESIAN_POINT ( 'NONE',  ( 0.7349081364829403995, 0.2306618581243848609, 0.2411417322834645549 ) ) ;
#57502=CARTESIAN_POINT ( 'NONE',  ( -1.279527559055116948, -0.5400638737290844871, 0.3530559997133364547 ) ) ;
#57503=CARTESIAN_POINT ( 'NONE',  ( -0.8070866141732276899, 0.1660481256975883668, -0.3530559997133364547 ) ) ;
#57504=CARTESIAN_POINT ( 'NONE',  ( -0.9908136482939626788, 0.1771653543307087630, 0.09757992244046791164 ) ) ;
#57505=CARTESIAN_POINT ( 'NONE',  ( -0.7742782152230962556, -0.4281496062992127816, -0.4176697321401328100 ) ) ;
#57508=CARTESIAN_POINT ( 'NONE',  ( 1.660104986876641320, -0.05778040916215522460, 0.4822834645669289988 ) ) ;
#57509=CARTESIAN_POINT ( 'NONE',  ( 1.509186351706037543, -0.4281496062992127816, -0.4176697321401328100 ) ) ;
#57510=CARTESIAN_POINT ( 'NONE',  ( -0.6364829396325453192, -0.3162353388693405765, 0.4822834645669290543 ) ) ;
#57511=CARTESIAN_POINT ( 'NONE',  ( 0.5314960629921264834, 0.1660481256975883668, -0.3530559997133364547 ) ) ;
#57512=CARTESIAN_POINT ( 'NONE',  ( -0.6758530183727028406, 0.2952755905511811885, 0.1292274648535926551 ) ) ;
#57514=CARTESIAN_POINT ( 'NONE',  ( -0.6824146981627288167, 0.1283753931104748280, 0.1820866141732283561 ) ) ;
#57515=VERTEX_POINT ( 'NONE', #2288 ) ;
#57518=CARTESIAN_POINT ( 'NONE',  ( -1.496062992125983815, -0.1870078740157480601, -0.3641732283464567677 ) ) ;
#57519=CARTESIAN_POINT ( 'NONE',  ( -1.266404199475064773, -0.05778040916215560624, -0.4822834645669293319 ) ) ;
#57520=CARTESIAN_POINT ( 'NONE',  ( -0.9317585301837263412, -0.4281496062992127816, -0.4176697321401328100 ) ) ;
#57522=CARTESIAN_POINT ( 'NONE',  ( -1.213910761154854745, 0.2952755905511810774, -0.1292274648535930714 ) ) ;
#57523=CARTESIAN_POINT ( 'NONE',  ( -1.128608923884513837, -0.6046776061558807314, 0.2411417322834647770 ) ) ;
#57524=B_SPLINE_CURVE_WITH_KNOTS ( 'NONE', 3,
 ( #12710, #56069, #76678, #23674 ),
 .UNSPECIFIED., .F., .F.,
 ( 4, 4 ),
 ( 0.02802642476679309200, 0.02831579184770149915 ),
 .UNSPECIFIED. ) ;
#57525=CARTESIAN_POINT ( 'NONE',  ( -1.561679790026246017, -0.4281496062992127816, -0.4176697321401328100 ) ) ;
#57526=CARTESIAN_POINT ( 'NONE',  ( -0.7989874411535504706, 0.02791078216816347476, -0.4328096321851898631 ) ) ;
#57527=CARTESIAN_POINT ( 'NONE',  ( 0.3280839895013130669, -0.3690944881889765550, -0.3153832671262227771 ) ) ;
#57530=CARTESIAN_POINT ( 'NONE',  ( -0.2559055118110230564, 0.07958543189024071263, -0.2665933059059888421 ) ) ;
#57531=CARTESIAN_POINT ( 'NONE',  ( -0.8661417322834640276, -0.1870078740157479769, 0.4822834645669291653 ) ) ;
#57532=CARTESIAN_POINT ( 'NONE',  ( 1.568241469816273437, -0.3162353388693405765, 0.4822834645669290543 ) ) ;
#57533=CARTESIAN_POINT ( 'NONE',  ( -0.5380577427821514602, 0.05413385826771666132, 0.4176697321401328100 ) ) ;
#57537=CARTESIAN_POINT ( 'NONE',  ( -0.6430446194225712953, 0.05413385826771626580, -0.4176697321401330321 ) ) ;
#57538=CARTESIAN_POINT ( 'NONE',  ( 1.332020997375328974, -0.05778040916215560624, -0.4822834645669293319 ) ) ;
#57539=CARTESIAN_POINT ( 'NONE',  ( -0.9776902887139098386, -0.5511811023622046335, 0.09757992244046803654 ) ) ;
#57540=CARTESIAN_POINT ( 'NONE',  ( -1.450131233595799651, -0.6692913385826771977, 0.1292274648535927661 ) ) ;
#57545=CARTESIAN_POINT ( 'NONE',  ( -0.03280839895013062252, 0.2952755905511810774, -0.1292274648535930714 ) ) ;
#57546=CARTESIAN_POINT ( 'NONE',  ( -1.213910761154854745, -0.5511811023622046335, 0.09757992244046803654 ) ) ;
#57547=CARTESIAN_POINT ( 'NONE',  ( -0.7545931758530177724, 0.2952755905511811885, 0.1292274648535926551 ) ) ;
#57549=CARTESIAN_POINT ( 'NONE',  ( -0.7020997375328076329, -0.3162353388693409650, -0.4822834645669289433 ) ) ;
#57550=CARTESIAN_POINT ( 'NONE',  ( -0.9055118110236215490, 0.2952755905511811885, 0.000000000000000000 ) ) ;
#57551=CARTESIAN_POINT ( 'NONE',  ( 0.1509186351706042484, -0.3162353388693405765, 0.4822834645669290543 ) ) ;
#57553=CARTESIAN_POINT ( 'NONE',  ( 0.8595800524934390507, -0.08942795157528024563, -0.3641732283464568787 ) ) ;
#57554=CARTESIAN_POINT ( 'NONE',  ( -0.7808398950131225646, -0.08942795157527998196, 0.3641732283464567121 ) ) ;
#57555=CARTESIAN_POINT ( 'NONE',  ( 0.8792650918635177559, -0.004921259842519576551, 0.3153832671262227771 ) ) ;
#57556=CARTESIAN_POINT ( 'NONE',  ( -1.660104986876639543, -0.05778040916215560624, -0.4822834645669293319 ) ) ;
#57557=CARTESIAN_POINT ( 'NONE',  ( 1.279527559055118724, 0.1660481256975885056, 0.3530559997133364547 ) ) ;
#57558=CARTESIAN_POINT ( 'NONE',  ( 0.4265091863517067594, 0.1771653543307087630, 0.09757992244046791164 ) ) ;
#57560=CARTESIAN_POINT ( 'NONE',  ( -0.9186351706036736120, -0.6046776061558809534, -0.2411417322834644161 ) ) ;
#57561=CARTESIAN_POINT ( 'NONE',  ( 1.122047244094488860, 0.1660481256975885056, 0.3530559997133364547 ) ) ;
#57563=CARTESIAN_POINT ( 'NONE',  ( -0.07217847769028787330, -0.08942795157527998196, 0.3641732283464567121 ) ) ;
#57564=CARTESIAN_POINT ( 'NONE',  ( -0.4052866537519759782, 0.02791078216816347476, -0.4328096321851898631 ) ) ;
#57565=CARTESIAN_POINT ( 'NONE',  ( 0.3674540682414705883, -0.6046776061558807314, 0.2411417322834647770 ) ) ;
#57567=CARTESIAN_POINT ( 'NONE',  ( 0.8989501312335963501, -0.5511811023622048555, -0.09757992244046775898 ) ) ;
#57568=CARTESIAN_POINT ( 'NONE',  ( 0.3149606299212603933, -0.1870078740157479769, 0.3641732283464567677 ) ) ;
#57569=CARTESIAN_POINT ( 'NONE',  ( -0.07874015748031421014, -0.1870078740157479769, 0.4822834645669291653 ) ) ;
#57570=CARTESIAN_POINT ( 'NONE',  ( -1.194225721784776262, 0.05413385826771626580, -0.4176697321401330321 ) ) ;
#57571=CARTESIAN_POINT ( 'NONE',  ( -0.7349081364829387342, -0.5023911411419708095, 0.1820866141732285504 ) ) ;
#57572=CARTESIAN_POINT ( 'NONE',  ( 2.795275590551181466, 1.062992125984252079, -2.156651478620225655E-16 ) ) ;
#57573=CARTESIAN_POINT ( 'NONE',  ( -0.4461942257217840213, -0.6046776061558809534, -0.2411417322834644161 ) ) ;
#57577=CARTESIAN_POINT ( 'NONE',  ( 0.03937007874015806264, 0.1771653543307087630, 0.000000000000000000 ) ) ;
#57578=CARTESIAN_POINT ( 'NONE',  ( -0.3477690288713902178, 0.2952755905511810774, -0.1292274648535930714 ) ) ;
#57579=CARTESIAN_POINT ( 'NONE',  ( -1.181102362204723644, -0.1870078740157479769, 0.4822834645669291653 ) ) ;
#57580=CARTESIAN_POINT ( 'NONE',  ( -1.043307086614172041, -0.4536011799217367080, 0.2665933059059888421 ) ) ;
#57582=CARTESIAN_POINT ( 'NONE',  ( -0.3215223097112853146, -0.05778040916215560624, -0.4822834645669293319 ) ) ;
#57583=CARTESIAN_POINT ( 'NONE',  ( -0.9776902887139098386, 0.1771653543307087075, -0.09757992244046823083 ) ) ;
#57584=CARTESIAN_POINT ( 'NONE',  ( -1.391076115485563758, 0.1283753931104748280, 0.1820866141732283561 ) ) ;
#57585=CARTESIAN_POINT ( 'NONE',  ( 1.253280839895013710, -0.3162353388693405765, 0.4822834645669290543 ) ) ;
#57586=FACE_OUTER_BOUND ( 'NONE', #78504, .T. ) ;
#57589=ORIENTED_EDGE ( 'NONE', *, *, #66351, .T. ) ;
#57590=CARTESIAN_POINT ( 'NONE',  ( -0.2238009295390064879, -2.294479370626195693E-15, 0.3464511005275217603 ) ) ;
#57591=CARTESIAN_POINT ( 'NONE',  ( -1.509186351706035767, 0.05413385826771626580, -0.4176697321401330321 ) ) ;
#57592=CARTESIAN_POINT ( 'NONE',  ( -0.7414698162729651543, 0.2952755905511810774, -0.1292274648535930714 ) ) ;
#57593=CARTESIAN_POINT ( 'NONE',  ( -1.496062992125983815, -0.1870078740157479769, 0.4822834645669291653 ) ) ;
#57596=CARTESIAN_POINT ( 'NONE',  ( 1.115485564304462551, -0.4281496062992127816, -0.4176697321401328100 ) ) ;
#57597=CARTESIAN_POINT ( 'NONE',  ( -0.03280839895013062252, 0.2952755905511810774, -0.1292274648535930714 ) ) ;
#57599=CARTESIAN_POINT ( 'NONE',  ( -0.7426113562967729953, 2.199547029020892275, -0.5309055118110235227 ) ) ;
#57600=CARTESIAN_POINT ( 'NONE',  ( 1.108923884514436242, -0.08942795157527998196, 0.3641732283464567121 ) ) ;
#57605=CARTESIAN_POINT ( 'NONE',  ( -0.01312335958005186876, -0.4281496062992124485, 0.4176697321401328655 ) ) ;
#57606=CARTESIAN_POINT ( 'NONE',  ( -0.6889763779527552368, -0.5400638737290845981, -0.3530559997133363437 ) ) ;
#57607=CARTESIAN_POINT ( 'NONE',  ( -1.318897637795274802, 0.1660481256975885056, 0.3530559997133364547 ) ) ;
#57608=CARTESIAN_POINT ( 'NONE',  ( 0.4986876640419954376, -0.6046776061558809534, -0.2411417322834644161 ) ) ;
#57609=CARTESIAN_POINT ( 'NONE',  ( 1.673228346456693494, 0.1660481256975885056, 0.3530559997133364547 ) ) ;
#57610=CARTESIAN_POINT ( 'NONE',  ( 1.581364829396326277, -0.05778040916215522460, 0.4822834645669289988 ) ) ;
#57611=CARTESIAN_POINT ( 'NONE',  ( -0.5446194225721777693, -0.05778040916215522460, 0.4822834645669289988 ) ) ;
#57612=CARTESIAN_POINT ( 'NONE',  ( 0.6430446194225728496, 0.05413385826771666132, 0.4176697321401328100 ) ) ;
#57613=CARTESIAN_POINT ( 'NONE',  ( -1.627296587926508442, 0.2306618581243848609, 0.2411417322834645549 ) ) ;
#57614=CARTESIAN_POINT ( 'NONE',  ( 1.286089238845145033, 0.2306618581243848609, 0.2411417322834645549 ) ) ;
#57616=CARTESIAN_POINT ( 'NONE',  ( -0.1246719160104980823, 0.2952755905511811885, 0.1292274648535926551 ) ) ;
#57618=CARTESIAN_POINT ( 'NONE',  ( 0.3543307086614181922, -0.5511811023622047445, 6.969142054262312111E-17 ) ) ;
#57621=ORIENTED_EDGE ( 'NONE', *, *, #45382, .T. ) ;
#57622=CARTESIAN_POINT ( 'NONE',  ( -0.1968503937007867743, -0.5511811023622047445, 6.969142054262312111E-17 ) ) ;
#57624=CARTESIAN_POINT ( 'NONE',  ( -0.05905511811023545637, -0.5400638737290845981, -0.3530559997133363437 ) ) ;
#57625=CARTESIAN_POINT ( 'NONE',  ( -0.1509186351706028884, -0.05778040916215522460, 0.4822834645669289988 ) ) ;
#57626=CARTESIAN_POINT ( 'NONE',  ( -0.4330708661417315697, 0.2952755905511811885, 0.000000000000000000 ) ) ;
#57628=CARTESIAN_POINT ( 'NONE',  ( -1.161417322834644716, 0.1660481256975885056, 0.3530559997133364547 ) ) ;
#57630=CARTESIAN_POINT ( 'NONE',  ( 0.7020997375328090762, -0.08942795157528024563, -0.3641732283464568787 ) ) ;
#57631=CARTESIAN_POINT ( 'NONE',  ( 1.062992125984252745, 0.2952755905511811885, 0.000000000000000000 ) ) ;
#57632=CARTESIAN_POINT ( 'NONE',  ( 0.6364829396325465405, -0.3162353388693409650, -0.4822834645669289433 ) ) ;
#57634=CARTESIAN_POINT ( 'NONE',  ( -1.397637795275589623, 0.1660481256975885056, 0.3530559997133364547 ) ) ;
#57637=CARTESIAN_POINT ( 'NONE',  ( -0.3346456692913377662, -0.5400638737290844871, 0.3530559997133364547 ) ) ;
#57640=CARTESIAN_POINT ( 'NONE',  ( -1.384514435695537005, -0.5511811023622048555, -0.09757992244046775898 ) ) ;
#57641=CARTESIAN_POINT ( 'NONE',  ( 1.358267716535433323, -0.5400638737290845981, -0.3530559997133363437 ) ) ;
#57642=CARTESIAN_POINT ( 'NONE',  ( 1.423884514435696413, -0.3162353388693409650, -0.4822834645669289433 ) ) ;
#57643=CARTESIAN_POINT ( 'NONE',  ( 0.1377952755905518800, 0.07958543189024071263, -0.2665933059059888421 ) ) ;
#57644=CARTESIAN_POINT ( 'NONE',  ( 1.062992125984252745, -0.6692913385826771977, 8.415575281601705876E-17 ) ) ;
#57646=CARTESIAN_POINT ( 'NONE',  ( 0.1837270341207357105, -0.5023911411419708095, -0.1820866141732282451 ) ) ;
#57647=CARTESIAN_POINT ( 'NONE',  ( 0.5708661417322841158, -0.5400638737290845981, -0.3530559997133363437 ) ) ;
#57649=ADVANCED_FACE ( 'NONE', ( #9841 ), #46374, .F. ) ;
#57650=CARTESIAN_POINT ( 'NONE',  ( -1.056430446194224881, 0.2952755905511810774, -0.1292274648535930714 ) ) ;
#57651=CARTESIAN_POINT ( 'NONE',  ( 0.5511811023622054106, -0.1870078740157480601, -0.3641732283464567677 ) ) ;
#57652=FACE_OUTER_BOUND ( 'NONE', #37274, .T. ) ;
#57653=CARTESIAN_POINT ( 'NONE',  ( -0.4724409448818890911, -0.1870078740157479769, 0.4822834645669291653 ) ) ;
#57654=CARTESIAN_POINT ( 'NONE',  ( -0.1837270341207340729, 0.1283753931104746893, -0.1820866141732285504 ) ) ;
#57656=CARTESIAN_POINT ( 'NONE',  ( -0.1968503937007867743, -0.6692913385826771977, 8.415575281601705876E-17 ) ) ;
#57657=CARTESIAN_POINT ( 'NONE',  ( 0.4986876640419954376, 0.1283753931104748280, 0.1820866141732283561 ) ) ;
#57659=CARTESIAN_POINT ( 'NONE',  ( -0.01968503937007793844, 0.1660481256975883668, -0.3530559997133364547 ) ) ;
#57661=CARTESIAN_POINT ( 'NONE',  ( 1.167979002624672580, -0.3690944881889763329, 0.3153832671262228327 ) ) ;
#57662=CARTESIAN_POINT ( 'NONE',  ( -0.1689764809739026374, 5.625543525484885637E-15, -0.3791475997938201781 ) ) ;
#57664=CARTESIAN_POINT ( 'NONE',  ( -0.7414698162729651543, 0.1771653543307087075, -0.09757992244046823083 ) ) ;
#57665=CARTESIAN_POINT ( 'NONE',  ( -0.7742782152230965886, -0.004921259842519576551, 0.3153832671262227771 ) ) ;
#57666=CARTESIAN_POINT ( 'NONE',  ( -0.8464566929133852113, 0.1660481256975885056, 0.3530559997133364547 ) ) ;
#57667=CARTESIAN_POINT ( 'NONE',  ( -0.2952755905511804668, 0.1660481256975885056, 0.3530559997133364547 ) ) ;
#57668=CARTESIAN_POINT ( 'NONE',  ( 0.4527559055118117182, 0.07958543189024071263, -0.2665933059059888421 ) ) ;
#57670=CARTESIAN_POINT ( 'NONE',  ( 1.358267716535433323, -0.4536011799217368745, -0.2665933059059886201 ) ) ;
#57671=CARTESIAN_POINT ( 'NONE',  ( 0.7086614173228353852, -0.1870078740157479769, 0.4822834645669291653 ) ) ;
#57673=CARTESIAN_POINT ( 'NONE',  ( -0.3543307086614165824, -0.6692913385826771977, 8.415575281601705876E-17 ) ) ;
#57675=CARTESIAN_POINT ( 'NONE',  ( -1.692913385826770645, 0.2952755905511811885, 0.000000000000000000 ) ) ;
#57676=CARTESIAN_POINT ( 'NONE',  ( 0.8136482939632553313, -0.6046776061558809534, -0.2411417322834644161 ) ) ;
#57677=CARTESIAN_POINT ( 'NONE',  ( 0.3608923884514443348, -0.6692913385826771977, 0.1292274648535927661 ) ) ;
#57679=CARTESIAN_POINT ( 'NONE',  ( 0.2952755905511819101, 0.07958543189024071263, -0.2665933059059888421 ) ) ;
#57680=CARTESIAN_POINT ( 'NONE',  ( 1.272965879265092637, -0.4281496062992127816, -0.4176697321401328100 ) ) ;
#57681=CARTESIAN_POINT ( 'NONE',  ( -0.4855643044619415427, -0.3690944881889763329, 0.3153832671262228327 ) ) ;
#57682=CARTESIAN_POINT ( 'NONE',  ( -0.6824146981627288167, 0.2306618581243848609, 0.2411417322834645549 ) ) ;
#57684=CARTESIAN_POINT ( 'NONE',  ( 0.05905511811023681640, 0.1660481256975883668, -0.3530559997133364547 ) ) ;
#57685=CARTESIAN_POINT ( 'NONE',  ( -0.8530183727034112984, 0.05413385826771666132, 0.4176697321401328100 ) ) ;
#57686=CARTESIAN_POINT ( 'NONE',  ( -0.8333333333333323711, -0.5511811023622048555, -0.09757992244046775898 ) ) ;
#57687=CARTESIAN_POINT ( 'NONE',  ( 0.5249343832021003964, 0.2306618581243847221, -0.2411417322834647770 ) ) ;
#57688=CARTESIAN_POINT ( 'NONE',  ( -1.122047244094487306, -0.5400638737290844871, 0.3530559997133364547 ) ) ;
#57689=CARTESIAN_POINT ( 'NONE',  ( -0.1902887139107604098, 0.2952755905511810774, -0.1292274648535930714 ) ) ;
#57692=CARTESIAN_POINT ( 'NONE',  ( 1.299212598425197429, 0.2952755905511811885, 0.000000000000000000 ) ) ;
#57693=CARTESIAN_POINT ( 'NONE',  ( 1.292650918635171564, -0.6692913385826773087, -0.1292274648535924053 ) ) ;
#57695=CARTESIAN_POINT ( 'NONE',  ( -1.482939632545930975, 0.05413385826771666132, 0.4176697321401328100 ) ) ;
#57696=CARTESIAN_POINT ( 'NONE',  ( -0.6955380577427815458, -0.4281496062992127816, -0.4176697321401328100 ) ) ;
#57699=ORIENTED_EDGE ( 'NONE', *, *, #67786, .T. ) ;
#57700=CARTESIAN_POINT ( 'NONE',  ( 0.09186351706036827158, -0.004921259842519576551, 0.3153832671262227771 ) ) ;
#57702=CARTESIAN_POINT ( 'NONE',  ( 0.3083989501312343062, -0.3162353388693405765, 0.4822834645669290543 ) ) ;
#57704=FACE_OUTER_BOUND ( 'NONE', #61594, .T. ) ;
#57705=CARTESIAN_POINT ( 'NONE',  ( -0.4068241469816264999, -0.3690944881889763329, 0.3153832671262228327 ) ) ;
#57706=CARTESIAN_POINT ( 'NONE',  ( 0.3740157480314966754, 0.1660481256975883391, -0.3530559997133364547 ) ) ;
#57707=CARTESIAN_POINT ( 'NONE',  ( 1.259842519685040019, -0.1870078740157480879, -0.4822834645669291653 ) ) ;
#57709=CARTESIAN_POINT ( 'NONE',  ( 0.7349081364829402885, -0.5023911411419708095, -0.1820866141732282451 ) ) ;
#57710=CARTESIAN_POINT ( 'NONE',  ( 0.1706036745406830368, -0.4281496062992127816, -0.4176697321401328100 ) ) ;
#57712=CARTESIAN_POINT ( 'NONE',  ( -1.030183727034119867, -0.3162353388693405765, 0.4822834645669290543 ) ) ;
#57713=CARTESIAN_POINT ( 'NONE',  ( -1.272965879265091305, -0.3690944881889763329, 0.3153832671262228327 ) ) ;
#57714=CARTESIAN_POINT ( 'NONE',  ( -0.5314960629921254842, -0.5400638737290845981, -0.3530559997133363437 ) ) ;
#57716=FACE_OUTER_BOUND ( 'NONE', #28126, .T. ) ;
#57717=ORIENTED_EDGE ( 'NONE', *, *, #35281, .T. ) ;
#57719=CARTESIAN_POINT ( 'NONE',  ( 0.3083989501312343062, -0.05778040916215560624, -0.4822834645669293319 ) ) ;
#57721=CARTESIAN_POINT ( 'NONE',  ( -0.6036745406824141069, 0.2306618581243848609, 0.2411417322834645549 ) ) ;
#57722=CARTESIAN_POINT ( 'NONE',  ( 1.318897637795276356, 0.1660481256975883668, -0.3530559997133364547 ) ) ;
#57723=CARTESIAN_POINT ( 'NONE',  ( 1.312335958005249825, 0.2306618581243847221, -0.2411417322834647770 ) ) ;
#57724=CARTESIAN_POINT ( 'NONE',  ( 0.4855643044619428750, 0.05413385826771666132, 0.4176697321401328100 ) ) ;
#57725=CARTESIAN_POINT ( 'NONE',  ( 0.2099737532808405305, -0.6046776061558807314, 0.2411417322834647770 ) ) ;
#57727=CARTESIAN_POINT ( 'NONE',  ( -0.8858267716535425107, 0.1660481256975883668, -0.3530559997133364547 ) ) ;
#57728=CARTESIAN_POINT ( 'NONE',  ( -0.1181102362204717315, -0.6692913385826771977, 8.415575281601705876E-17 ) ) ;
#57729=CARTESIAN_POINT ( 'NONE',  ( -0.2099737532808391705, 0.1283753931104748280, 0.1820866141732283561 ) ) ;
#57731=CARTESIAN_POINT ( 'NONE',  ( -0.07874015748031421014, -0.1870078740157480879, -0.4822834645669291653 ) ) ;
#57733=CARTESIAN_POINT ( 'NONE',  ( 1.082677165354331228, -0.5400638737290844871, 0.3530559997133364547 ) ) ;
#57734=CARTESIAN_POINT ( 'NONE',  ( 0.5052493438320215802, 0.2066929133858267931, 0.1054918080437490802 ) ) ;
#57738=CARTESIAN_POINT ( 'NONE',  ( 0.4790026246719168435, -0.3162353388693409650, -0.4822834645669289433 ) ) ;
#57739=CARTESIAN_POINT ( 'NONE',  ( -0.1837270341207343505, -0.5023911411419708095, 0.1820866141732285504 ) ) ;
#57740=CARTESIAN_POINT ( 'NONE',  ( 1.594488188976378673, -0.4536011799217368745, -0.2665933059059886201 ) ) ;
#57744=CARTESIAN_POINT ( 'NONE',  ( 1.417322834645670104, -0.1870078740157480601, -0.3641732283464567677 ) ) ;
#57745=CARTESIAN_POINT ( 'NONE',  ( 1.528871391076116026, -0.6692913385826773087, -0.1292274648535924053 ) ) ;
#57747=CARTESIAN_POINT ( 'NONE',  ( -0.1312335958005241554, 0.2306618581243848609, 0.2411417322834645549 ) ) ;
#57748=CARTESIAN_POINT ( 'NONE',  ( -1.213910761154854745, -0.6692913385826771977, 0.1292274648535927661 ) ) ;
#57749=CARTESIAN_POINT ( 'NONE',  ( -1.102362204724408601, -0.1870078740157479769, 0.4822834645669291653 ) ) ;
#57750=CARTESIAN_POINT ( 'NONE',  ( 0.2493438320209980519, -0.4281496062992127816, -0.4176697321401328100 ) ) ;
#57752=CARTESIAN_POINT ( 'NONE',  ( 1.646981627296588035, -0.3162353388693405765, 0.4822834645669290543 ) ) ;
#57753=CARTESIAN_POINT ( 'NONE',  ( 1.062992125984252745, -0.6692913385826771977, 8.415575281601705876E-17 ) ) ;
#57754=CARTESIAN_POINT ( 'NONE',  ( 0.7611548556430454138, 0.1283753931104746893, -0.1820866141732285504 ) ) ;
#57756=CARTESIAN_POINT ( 'NONE',  ( 0.9908136482939640111, -0.5511811023622046335, 0.09757992244046803654 ) ) ;
#57757=CARTESIAN_POINT ( 'NONE',  ( -1.141732283464566011, 0.2952755905511811885, 0.000000000000000000 ) ) ;
#57759=CARTESIAN_POINT ( 'NONE',  ( 1.167979002624672580, -0.4281496062992124485, 0.4176697321401328655 ) ) ;
#57761=CARTESIAN_POINT ( 'NONE',  ( 0.6430446194225729606, -0.4281496062992127816, -0.4176697321401328100 ) ) ;
#57763=CARTESIAN_POINT ( 'NONE',  ( -1.620734908136482577, -0.5511811023622048555, -0.09757992244046775898 ) ) ;
#57764=CARTESIAN_POINT ( 'NONE',  ( 0.05905511811023709395, -0.5400638737290844871, 0.3530559997133364547 ) ) ;
#57765=CARTESIAN_POINT ( 'NONE',  ( 0.3083989501312343062, -0.2845877964562159024, 0.3641732283464567677 ) ) ;
#57766=CARTESIAN_POINT ( 'NONE',  ( 0.8661417322834653598, -0.1870078740157479769, 0.4822834645669291653 ) ) ;
#57768=CARTESIAN_POINT ( 'NONE',  ( -0.7217847769028863381, -0.004921259842519870586, -0.3153832671262229437 ) ) ;
#57769=CARTESIAN_POINT ( 'NONE',  ( -0.7874015748031489847, -0.1870078740157479769, 0.4822834645669291653 ) ) ;
#57770=CARTESIAN_POINT ( 'NONE',  ( 1.620734908136483465, -0.6692913385826771977, 0.1292274648535927661 ) ) ;
#57771=CARTESIAN_POINT ( 'NONE',  ( -0.9842519685039365918, -0.6692913385826771977, 8.415575281601705876E-17 ) ) ;
#57772=CARTESIAN_POINT ( 'NONE',  ( 0.9055118110236227702, 0.2952755905511811885, 0.000000000000000000 ) ) ;
#57773=CARTESIAN_POINT ( 'NONE',  ( -1.404199475065615932, -0.3690944881889765550, -0.3153832671262227771 ) ) ;
#57775=CARTESIAN_POINT ( 'NONE',  ( 0.8333333333333340365, 0.2952755905511810774, -0.1292274648535930714 ) ) ;
#57777=CARTESIAN_POINT ( 'NONE',  ( -1.482939632545930975, -0.4281496062992127816, -0.4176697321401328100 ) ) ;
#57778=CARTESIAN_POINT ( 'NONE',  ( -1.351706036745406347, -0.3690944881889763329, 0.3153832671262228327 ) ) ;
#57779=CARTESIAN_POINT ( 'NONE',  ( -1.227034120734907585, 0.1771653543307087630, 0.09757992244046791164 ) ) ;
#57780=CARTESIAN_POINT ( 'NONE',  ( 1.522309711286089939, 0.1283753931104748280, 0.1820866141732283561 ) ) ;
#57781=CARTESIAN_POINT ( 'NONE',  ( -0.3215223097112853146, -0.05778040916215560624, -0.4822834645669293319 ) ) ;
#57782=CARTESIAN_POINT ( 'NONE',  ( -0.3805774278215216522, -0.004921259842519576551, 0.3153832671262227771 ) ) ;
#57783=CARTESIAN_POINT ( 'NONE',  ( -1.633858267716534529, -0.4536011799217368745, -0.2665933059059886201 ) ) ;
#57784=CARTESIAN_POINT ( 'NONE',  ( 0.8005249343832027131, -0.004921259842519576551, 0.3153832671262227771 ) ) ;
#57785=CARTESIAN_POINT ( 'NONE',  ( 0.3805774278215230400, -0.4281496062992124485, 0.4176697321401328655 ) ) ;
#57786=CARTESIAN_POINT ( 'NONE',  ( 1.614173228346457378, 0.2952755905511811885, 0.000000000000000000 ) ) ;
#57787=CARTESIAN_POINT ( 'NONE',  ( 0.6036745406824154392, 0.2306618581243847221, -0.2411417322834647770 ) ) ;
#57788=CARTESIAN_POINT ( 'NONE',  ( 0.4790026246719167324, -0.08942795157527998196, 0.3641732283464567121 ) ) ;
#57789=CARTESIAN_POINT ( 'NONE',  ( -1.607611548556429737, 0.2952755905511810774, -0.1292274648535930714 ) ) ;
#57790=CARTESIAN_POINT ( 'NONE',  ( -1.240157480314959759, -0.5400638737290845981, -0.3530559997133363437 ) ) ;
#57791=CARTESIAN_POINT ( 'NONE',  ( -0.3149606299212590610, -0.1870078740157479769, 0.4822834645669291653 ) ) ;
#57794=CARTESIAN_POINT ( 'NONE',  ( 0.5052493438320215802, 0.2952755905511811885, 0.1292274648535926551 ) ) ;
#57795=CARTESIAN_POINT ( 'NONE',  ( 1.194225721784777594, -0.3690944881889765550, -0.3153832671262227771 ) ) ;
#57796=CARTESIAN_POINT ( 'NONE',  ( -0.5052493438320203589, 0.2952755905511810774, -0.1292274648535930714 ) ) ;
#57797=CARTESIAN_POINT ( 'NONE',  ( 0.2755905511811031494, -0.6692913385826771977, 8.415575281601705876E-17 ) ) ;
#57804=CARTESIAN_POINT ( 'NONE',  ( -0.8202099737532801971, -0.5511811023622046335, 0.09757992244046803654 ) ) ;
#57805=CARTESIAN_POINT ( 'NONE',  ( -1.187664041994750175, -0.05778040916215560624, -0.4822834645669293319 ) ) ;
#57807=CARTESIAN_POINT ( 'NONE',  ( 0.5314960629921267055, -0.5400638737290844871, 0.3530559997133364547 ) ) ;
#57808=CARTESIAN_POINT ( 'NONE',  ( 1.463254593175853824, 0.2952755905511810774, -0.1292274648535930714 ) ) ;
#57809=CARTESIAN_POINT ( 'NONE',  ( 0.8267716535433077274, 0.2952755905511811885, 0.000000000000000000 ) ) ;
#57813=CARTESIAN_POINT ( 'NONE',  ( 1.568241469816273659, -0.05778040916215560624, -0.4822834645669293319 ) ) ;
#57814=CARTESIAN_POINT ( 'NONE',  ( 0.6561679790026253567, 0.2306618581243848609, 0.2411417322834645549 ) ) ;
#57815=CARTESIAN_POINT ( 'NONE',  ( 0.04593175853018440641, 0.2952755905511810774, -0.1292274648535930714 ) ) ;
#57816=CARTESIAN_POINT ( 'NONE',  ( 0.7217847769028878924, -0.3690944881889765550, -0.3153832671262227771 ) ) ;
#57817=CARTESIAN_POINT ( 'NONE',  ( 1.437007874015748810, -0.5400638737290845981, -0.3530559997133363437 ) ) ;
#57819=CARTESIAN_POINT ( 'NONE',  ( 0.6496062992125991586, 0.1660481256975885056, 0.3530559997133364547 ) ) ;
#57820=CARTESIAN_POINT ( 'NONE',  ( 1.194225721784777594, 0.05413385826771666132, 0.4176697321401328100 ) ) ;
#57821=CARTESIAN_POINT ( 'NONE',  ( 0.1902887139107617975, -0.6692913385826773087, -0.1292274648535924053 ) ) ;
#57822=CARTESIAN_POINT ( 'NONE',  ( 1.062992125984252745, 0.1771653543307087630, 0.000000000000000000 ) ) ;
#57823=CARTESIAN_POINT ( 'NONE',  ( -0.7283464566929126471, 0.1660481256975883668, -0.3530559997133364547 ) ) ;
#57824=CARTESIAN_POINT ( 'NONE',  ( -0.9251968503937002541, 0.1660481256975885056, 0.3530559997133364547 ) ) ;
#57825=CARTESIAN_POINT ( 'NONE',  ( 1.095800524934383846, -0.3162353388693405765, 0.4822834645669290543 ) ) ;
#57831=ORIENTED_EDGE ( 'NONE', *, *, #27922, .T. ) ;
#57833=CARTESIAN_POINT ( 'NONE',  ( 0.8727034120734912248, -0.2845877964562161244, -0.3641732283464567121 ) ) ;
#57835=CARTESIAN_POINT ( 'NONE',  ( 1.430446194225722500, -0.3690944881889765550, -0.3153832671262227771 ) ) ;
#57840=CARTESIAN_POINT ( 'NONE',  ( -0.9580052493438311334, -0.004921259842519870586, -0.3153832671262229437 ) ) ;
#57841=CARTESIAN_POINT ( 'NONE',  ( -1.581364829396324945, -0.2845877964562159024, 0.3641732283464567677 ) ) ;
#57842=ADVANCED_FACE ( 'NONE', ( #66683 ), #54023, .T. ) ;
#57843=CARTESIAN_POINT ( 'NONE',  ( -1.437007874015747477, 0.1660481256975883668, -0.3530559997133364547 ) ) ;
#57844=CARTESIAN_POINT ( 'NONE',  ( -0.05905511811023545637, -0.5400638737290845981, -0.3530559997133363437 ) ) ;
#57845=CARTESIAN_POINT ( 'NONE',  ( 1.351706036745407458, -0.4281496062992127816, -0.4176697321401328100 ) ) ;
#57848=CARTESIAN_POINT ( 'NONE',  ( -1.114781747626346187, -2.609869883881465018E-15, -0.3464511005275220379 ) ) ;
#57852=CARTESIAN_POINT ( 'NONE',  ( -1.030183727034119867, -0.2845877964562159024, 0.3641732283464567677 ) ) ;
#57853=CARTESIAN_POINT ( 'NONE',  ( -1.299212598425196097, 0.2952755905511811885, 0.000000000000000000 ) ) ;
#57854=CARTESIAN_POINT ( 'NONE',  ( 0.7545931758530189937, 0.2952755905511810774, -0.1292274648535930714 ) ) ;
#57855=VERTEX_POINT ( 'NONE', #56506 ) ;
#57858=ADVANCED_FACE ( 'NONE', ( #17004 ), #10680, .F. ) ;
#57859=CARTESIAN_POINT ( 'NONE',  ( 1.148293963254593875, -0.6692913385826771977, 0.1292274648535927661 ) ) ;
#57860=CARTESIAN_POINT ( 'NONE',  ( -1.227034120734907585, 0.2952755905511811885, 0.1292274648535926551 ) ) ;
#57862=CARTESIAN_POINT ( 'NONE',  ( -0.5708661417322828946, 0.07958543189024071263, -0.2665933059059888421 ) ) ;
#57864=EDGE_CURVE ( 'NONE', #78494, #37713, #78281, .T. ) ;
#57865=CARTESIAN_POINT ( 'NONE',  ( -0.3215223097112853146, -0.08942795157528024563, -0.3641732283464568787 ) ) ;
#57866=CARTESIAN_POINT ( 'NONE',  ( -0.06561679790026180015, -0.3690944881889765550, -0.3153832671262227771 ) ) ;
#57867=VECTOR ( 'NONE', #70231, 39.37007874015748143 ) ;
#57868=CARTESIAN_POINT ( 'NONE',  ( 0.2690288713910767848, -0.6692913385826773087, -0.1292274648535924053 ) ) ;
#57869=CARTESIAN_POINT ( 'NONE',  ( -0.9448818897637790704, -0.1870078740157480601, -0.3641732283464567677 ) ) ;
#57871=CARTESIAN_POINT ( 'NONE',  ( 1.325459317585302665, 0.05413385826771626580, -0.4176697321401330321 ) ) ;
#57872=CARTESIAN_POINT ( 'NONE',  ( -1.430446194225720724, 0.05413385826771626580, -0.4176697321401330321 ) ) ;
#57874=CARTESIAN_POINT ( 'NONE',  ( -0.2165354330708654795, -0.5400638737290845981, -0.3530559997133363437 ) ) ;
#57875=CARTESIAN_POINT ( 'NONE',  ( -0.8727034120734901146, -0.3162353388693405765, 0.4822834645669290543 ) ) ;
#57876=CARTESIAN_POINT ( 'NONE',  ( 0.9580052493438327987, -0.3690944881889765550, -0.3153832671262227771 ) ) ;
#57877=CARTESIAN_POINT ( 'NONE',  ( -0.2559055118110230564, 0.07958543189024071263, -0.2665933059059888421 ) ) ;
#57878=CARTESIAN_POINT ( 'NONE',  ( -0.7611548556430438595, 0.2306618581243848609, 0.2411417322834645549 ) ) ;
#57879=CARTESIAN_POINT ( 'NONE',  ( 1.594488188976378673, -0.5400638737290845981, -0.3530559997133363437 ) ) ;
#57881=CARTESIAN_POINT ( 'NONE',  ( 1.220472440944882608, 0.1771653543307087630, 0.000000000000000000 ) ) ;
#57882=CARTESIAN_POINT ( 'NONE',  ( -0.4265091863517051496, -0.6692913385826771977, 0.1292274648535927661 ) ) ;
#57883=CARTESIAN_POINT ( 'NONE',  ( -1.568241469816272105, -0.05778040916215522460, 0.4822834645669289988 ) ) ;
#57887=CARTESIAN_POINT ( 'NONE',  ( -0.8923884514435688198, -0.5023911411419708095, 0.1820866141732285504 ) ) ;
#57888=CARTESIAN_POINT ( 'NONE',  ( 0.9186351706036751663, -0.6046776061558807314, 0.2411417322834647770 ) ) ;
#57889=CARTESIAN_POINT ( 'NONE',  ( -1.227034120734907585, 0.1771653543307087630, 0.09757992244046791164 ) ) ;
#57891=CARTESIAN_POINT ( 'NONE',  ( -0.8923884514435688198, 0.2306618581243847221, -0.2411417322834647770 ) ) ;
#57892=CARTESIAN_POINT ( 'NONE',  ( 0.7152230971128616943, -0.05778040916215522460, 0.4822834645669289988 ) ) ;
#57893=CARTESIAN_POINT ( 'NONE',  ( 0.5905511811023629321, 0.2952755905511811885, 0.000000000000000000 ) ) ;
#57894=CARTESIAN_POINT ( 'NONE',  ( 1.535433070866142335, -0.6692913385826771977, 8.415575281601705876E-17 ) ) ;
#57895=CARTESIAN_POINT ( 'NONE',  ( -1.594488188976377563, -0.4536011799217367080, 0.2665933059059888421 ) ) ;
#57901=CARTESIAN_POINT ( 'NONE',  ( 1.220472440944882608, 0.1771653543307087630, 0.000000000000000000 ) ) ;
#57902=CARTESIAN_POINT ( 'NONE',  ( 0.3937007874015754361, -0.1870078740157480601, -0.3641732283464567677 ) ) ;
#57903=AXIS2_PLACEMENT_3D ( 'NONE', #41515, #16688, #80668 ) ;
#57904=CARTESIAN_POINT ( 'NONE',  ( 0.2690288713910767848, -0.6692913385826773087, -0.1292274648535924053 ) ) ;
#57905=CARTESIAN_POINT ( 'NONE',  ( 1.167979002624672580, 0.05413385826771626580, -0.4176697321401330321 ) ) ;
#57907=CARTESIAN_POINT ( 'NONE',  ( 0.4724409448818904789, -0.1870078740157480601, -0.3641732283464567677 ) ) ;
#57909=CARTESIAN_POINT ( 'NONE',  ( -0.7414698162729651543, -0.6692913385826771977, 0.1292274648535927661 ) ) ;
#57910=CARTESIAN_POINT ( 'NONE',  ( -1.437007874015747477, 0.1660481256975883668, -0.3530559997133364547 ) ) ;
#57911=CARTESIAN_POINT ( 'NONE',  ( 0.7677165354330716118, 0.1660481256975883668, -0.3530559997133364547 ) ) ;
#57916=CARTESIAN_POINT ( 'NONE',  ( -1.286089238845143479, -0.6046776061558807314, 0.2411417322834647770 ) ) ;
#57917=CARTESIAN_POINT ( 'NONE',  ( -0.7217847769028863381, -0.4281496062992124485, 0.4176697321401328655 ) ) ;
#57918=CARTESIAN_POINT ( 'NONE',  ( -0.9514435695538050464, -0.08942795157528024563, -0.3641732283464568787 ) ) ;
#57919=CARTESIAN_POINT ( 'NONE',  ( -0.6496062992125976043, 0.1660481256975883668, -0.3530559997133364547 ) ) ;
#57922=CARTESIAN_POINT ( 'NONE',  ( -1.496062992125983815, -0.1870078740157479769, 0.3641732283464567677 ) ) ;
#57923=CARTESIAN_POINT ( 'NONE',  ( -1.404199475065615932, 0.05413385826771666132, 0.4176697321401328100 ) ) ;
#57924=CARTESIAN_POINT ( 'NONE',  ( 0.5052493438320215802, 0.2952755905511811885, 0.1292274648535926551 ) ) ;
#57925=CARTESIAN_POINT ( 'NONE',  ( -0.6561679790026240244, 0.2306618581243847221, -0.2411417322834647770 ) ) ;
#57927=CARTESIAN_POINT ( 'NONE',  ( -0.6955380577427815458, -0.004921259842519576551, 0.3153832671262227771 ) ) ;
#57928=VERTEX_POINT ( 'NONE', #39834 ) ;
#57931=CARTESIAN_POINT ( 'NONE',  ( -1.509186351706035767, -0.004921259842519870586, -0.3153832671262229437 ) ) ;
#57932=CARTESIAN_POINT ( 'NONE',  ( -1.279527559055116948, 0.1660481256975883668, -0.3530559997133364547 ) ) ;
#57933=CARTESIAN_POINT ( 'NONE',  ( -0.9448818897637790704, -0.1870078740157480879, -0.4822834645669291653 ) ) ;
#57935=CARTESIAN_POINT ( 'NONE',  ( -1.062992125984250968, 0.2952755905511811885, 0.000000000000000000 ) ) ;
#57936=CARTESIAN_POINT ( 'NONE',  ( -1.384514435695537005, 0.2952755905511811885, 0.1292274648535926551 ) ) ;
#57938=CARTESIAN_POINT ( 'NONE',  ( 0.4461942257217856311, 0.1283753931104746893, -0.1820866141732285504 ) ) ;
#57941=CARTESIAN_POINT ( 'NONE',  ( -0.3674540682414692561, -0.5023911411419708095, -0.1820866141732282451 ) ) ;
#57942=CARTESIAN_POINT ( 'NONE',  ( -0.8792650918635160906, -0.4281496062992124485, 0.4176697321401328655 ) ) ;
#57943=CARTESIAN_POINT ( 'NONE',  ( 1.292650918635171564, 0.2952755905511811885, 0.1292274648535926551 ) ) ;
#57944=CARTESIAN_POINT ( 'NONE',  ( -0.4855643044619415427, 0.05413385826771626580, -0.4176697321401330321 ) ) ;
#57945=VERTEX_POINT ( 'NONE', #77302 ) ;
#57948=CARTESIAN_POINT ( 'NONE',  ( -0.8923884514435688198, -0.6046776061558807314, 0.2411417322834647770 ) ) ;
#57949=CARTESIAN_POINT ( 'NONE',  ( 1.437007874015748810, 0.1660481256975885056, 0.3530559997133364547 ) ) ;
#57950=CARTESIAN_POINT ( 'NONE',  ( -1.174540682414697335, -0.2845877964562161244, -0.3641732283464567121 ) ) ;
#57951=CARTESIAN_POINT ( 'NONE',  ( -1.259842519685038686, -0.1870078740157479769, 0.4822834645669291653 ) ) ;
#57956=CARTESIAN_POINT ( 'NONE',  ( 0.2230971128608932319, -0.4281496062992124485, 0.4176697321401328655 ) ) ;
#57957=CARTESIAN_POINT ( 'NONE',  ( -1.082677165354329896, -0.4536011799217368745, -0.2665933059059886201 ) ) ;
#57958=CARTESIAN_POINT ( 'NONE',  ( -0.6167979002624665030, 0.05413385826771666132, 0.4176697321401328100 ) ) ;
#57960=CARTESIAN_POINT ( 'NONE',  ( -1.371391076115484831, 0.2952755905511810774, -0.1292274648535930714 ) ) ;
#57962=CARTESIAN_POINT ( 'NONE',  ( -1.076115485564303809, 0.2306618581243848609, 0.2411417322834645549 ) ) ;
#57963=CARTESIAN_POINT ( 'NONE',  ( 0.07874015748031558404, -0.1870078740157480879, -0.4822834645669291653 ) ) ;
#57965=CARTESIAN_POINT ( 'NONE',  ( 1.023622047244095112, -0.1870078740157480601, -0.3641732283464567677 ) ) ;
#57966=CARTESIAN_POINT ( 'NONE',  ( -0.7480314960629914633, 0.1771653543307087630, 0.000000000000000000 ) ) ;
#57968=CARTESIAN_POINT ( 'NONE',  ( 0.8858267716535438430, 0.07958543189024085140, 0.2665933059059887866 ) ) ;
#57969=CARTESIAN_POINT ( 'NONE',  ( 1.528871391076116026, -0.5511811023622048555, -0.09757992244046775898 ) ) ;
#57971=CARTESIAN_POINT ( 'NONE',  ( 1.325459317585302665, 0.05413385826771626580, -0.4176697321401330321 ) ) ;
#57973=CARTESIAN_POINT ( 'NONE',  ( -0.006561679790025524116, -0.08942795157528024563, -0.3641732283464568787 ) ) ;
#57975=CARTESIAN_POINT ( 'NONE',  ( -1.017060367454067249, -0.05778040916215522460, 0.4822834645669289988 ) ) ;
#57976=CARTESIAN_POINT ( 'NONE',  ( 1.384514435695538337, -0.6692913385826771977, 0.1292274648535927661 ) ) ;
#57977=DIRECTION ( 'NONE',  ( -5.372046893347524115E-15, 0.000000000000000000, 1.000000000000000000 ) ) ;
#57978=CARTESIAN_POINT ( 'NONE',  ( -0.5446194225721777693, -0.08942795157527998196, 0.3641732283464567121 ) ) ;
#57980=CARTESIAN_POINT ( 'NONE',  ( 0.1246719160104994284, 0.2952755905511810774, -0.1292274648535930714 ) ) ;
#57982=CARTESIAN_POINT ( 'NONE',  ( 0.9973753280839902091, 0.1283753931104746893, -0.1820866141732285504 ) ) ;
#57983=CARTESIAN_POINT ( 'NONE',  ( 0.2230971128608929543, -0.004921259842519870586, -0.3153832671262229437 ) ) ;
#57984=CARTESIAN_POINT ( 'NONE',  ( 0.3083989501312343062, -0.05778040916215560624, -0.4822834645669293319 ) ) ;
#57985=CARTESIAN_POINT ( 'NONE',  ( -1.259842519685038686, -0.1870078740157479769, 0.4822834645669291653 ) ) ;
#57986=CARTESIAN_POINT ( 'NONE',  ( -0.7677165354330699465, -0.4536011799217368745, -0.2665933059059886201 ) ) ;
#57988=CARTESIAN_POINT ( 'NONE',  ( -0.8202099737532799750, 0.2952755905511810774, -0.1292274648535930714 ) ) ;
#57990=( BOUNDED_CURVE ( )  B_SPLINE_CURVE ( 2, ( #49076, #74777, #17128, #42760, #55798, #36868, #62544, #4882, #30556, #56222, #51537, #76820, #13688 ),
 .UNSPECIFIED., .F., .F. ) 
 B_SPLINE_CURVE_WITH_KNOTS ( ( 3, 2, 2, 2, 2, 2, 3 ),
 ( 0.6853969023887781509, 0.6856060606060606633, 0.6893939393939394478, 0.6931818181818182323, 0.6969696969696970168, 0.7007575757575758013, 0.7009667339748582027 ),
 .UNSPECIFIED. ) 
 CURVE ( )  GEOMETRIC_REPRESENTATION_ITEM ( )  RATIONAL_B_SPLINE_CURVE ( ( 0.9964447847208419695, 0.9981185001348091834, 1.000000000000000000, 0.9659258262890683122, 1.000000000000000000, 0.9659258262890683122, 1.000000000000000000, 0.9659258262890683122, 1.000000000000000000, 0.9659258262890683122, 1.000000000000000000, 0.9981185001348101826, 0.9964447847208438569 ) ) 
 REPRESENTATION_ITEM ( '' )  );
#57992=CARTESIAN_POINT ( 'NONE',  ( 0.2690288713910767848, -0.5511811023622048555, -0.09757992244046775898 ) ) ;
#57993=CARTESIAN_POINT ( 'NONE',  ( -0.7020997375328074108, -0.05778040916215522460, 0.4822834645669289988 ) ) ;
#57994=CARTESIAN_POINT ( 'NONE',  ( -1.200787401574802349, -0.5400638737290844871, 0.3530559997133364547 ) ) ;
#57995=CARTESIAN_POINT ( 'NONE',  ( -1.397637795275589623, -0.4536011799217368745, -0.2665933059059886201 ) ) ;
#57996=CARTESIAN_POINT ( 'NONE',  ( 1.555118110236221041, 0.1660481256975883668, -0.3530559997133364547 ) ) ;
#57997=CARTESIAN_POINT ( 'NONE',  ( -0.3083989501312330295, -0.3162353388693409650, -0.4822834645669289433 ) ) ;
#57998=CARTESIAN_POINT ( 'NONE',  ( -0.7152230971128602510, -0.2845877964562159024, 0.3641732283464567677 ) ) ;
#57999=CARTESIAN_POINT ( 'NONE',  ( -1.614173228346456268, -0.5511811023622047445, 6.969142054262312111E-17 ) ) ;
#58000=CARTESIAN_POINT ( 'NONE',  ( 1.351706036745407458, -0.4281496062992127816, -0.4176697321401328100 ) ) ;
#58005=CARTESIAN_POINT ( 'NONE',  ( 1.437007874015748810, 0.07958543189024085140, 0.2665933059059887866 ) ) ;
#58006=CARTESIAN_POINT ( 'NONE',  ( -0.7349081364829390672, 0.2306618581243847221, -0.2411417322834647770 ) ) ;
#58007=CARTESIAN_POINT ( 'NONE',  ( -1.581364829396324945, -0.05778040916215560624, -0.4822834645669293319 ) ) ;
#58009=CARTESIAN_POINT ( 'NONE',  ( 1.653543307086614789, -0.1870078740157479769, 0.3641732283464567677 ) ) ;
#58010=CARTESIAN_POINT ( 'NONE',  ( 0.6299212598425204535, -0.1870078740157480879, -0.4822834645669291653 ) ) ;
#58011=CARTESIAN_POINT ( 'NONE',  ( 0.2165354330708668673, -0.5400638737290844871, 0.3530559997133364547 ) ) ;
#58013=CARTESIAN_POINT ( 'NONE',  ( -0.7426113562972000981, 2.401574803149605586, 0.5309055118110236338 ) ) ;
#58014=CARTESIAN_POINT ( 'NONE',  ( 0.8530183727034126306, -0.004921259842519870586, -0.3153832671262229437 ) ) ;
#58018=ORIENTED_EDGE ( 'NONE', *, *, #21915, .T. ) ;
#58019=CARTESIAN_POINT ( 'NONE',  ( -0.1443569553805768291, 0.05413385826771666132, 0.4176697321401328100 ) ) ;
#58021=CARTESIAN_POINT ( 'NONE',  ( -1.522309711286088607, -0.6046776061558807314, 0.2411417322834647770 ) ) ;
#58022=CARTESIAN_POINT ( 'NONE',  ( 0.6627296587926517768, -0.6692913385826773087, -0.1292274648535924053 ) ) ;
#58023=CARTESIAN_POINT ( 'NONE',  ( 1.089238845144357759, 0.05413385826771626580, -0.4176697321401330321 ) ) ;
#58024=CARTESIAN_POINT ( 'NONE',  ( 1.463254593175853824, 0.2952755905511810774, -0.1292274648535930714 ) ) ;
#58025=CARTESIAN_POINT ( 'NONE',  ( -0.3215223097112853146, -0.05778040916215560624, -0.4822834645669293319 ) ) ;
#58026=CARTESIAN_POINT ( 'NONE',  ( -0.07217847769028813698, -0.3162353388693409650, -0.4822834645669289433 ) ) ;
#58027=CARTESIAN_POINT ( 'NONE',  ( 1.522309711286089939, -0.6046776061558809534, -0.2411417322834644161 ) ) ;
#58029=CARTESIAN_POINT ( 'NONE',  ( 1.489501312335958172, -0.05778040916215560624, -0.4822834645669293319 ) ) ;
#58030=CARTESIAN_POINT ( 'NONE',  ( 1.673228346456693494, 0.1660481256975885056, 0.3530559997133364547 ) ) ;
#58031=CARTESIAN_POINT ( 'NONE',  ( -0.3018372703412066094, 0.05413385826771666132, 0.4176697321401328100 ) ) ;
#58033=CARTESIAN_POINT ( 'NONE',  ( 0.6036745406824154392, 0.1283753931104746893, -0.1820866141732285504 ) ) ;
#58036=ORIENTED_EDGE ( 'NONE', *, *, #12851, .T. ) ;
#58037=CARTESIAN_POINT ( 'NONE',  ( -0.5446194225721777693, -0.2845877964562161244, -0.3641732283464567121 ) ) ;
#58039=CARTESIAN_POINT ( 'NONE',  ( 0.1640419947506569498, -0.05778040916215522460, 0.4822834645669289988 ) ) ;
#58040=CARTESIAN_POINT ( 'NONE',  ( -0.1706036745406816491, -0.4281496062992124485, 0.4176697321401328655 ) ) ;
#58041=CARTESIAN_POINT ( 'NONE',  ( -0.8792650918635160906, 0.05413385826771626580, -0.4176697321401330321 ) ) ;
#58043=CARTESIAN_POINT ( 'NONE',  ( -1.318897637795274802, 0.1660481256975885056, 0.3530559997133364547 ) ) ;
#58044=CARTESIAN_POINT ( 'NONE',  ( -1.614173228346456712, 1.543375672658095610, -0.1372047244094478091 ) ) ;
#58045=CARTESIAN_POINT ( 'NONE',  ( 0.9186351706036751663, -0.5023911411419708095, 0.1820866141732285504 ) ) ;
#58046=CARTESIAN_POINT ( 'NONE',  ( 0.3346456692913393205, -0.5400638737290845981, -0.3530559997133363437 ) ) ;
#58047=CARTESIAN_POINT ( 'NONE',  ( 0.5971128608923891301, 0.2952755905511810774, -0.1292274648535930714 ) ) ;
#58049=CARTESIAN_POINT ( 'NONE',  ( 0.3260583142159772518, 2.726622551019859153E-15, 0.3954974714151457960 ) ) ;
#58052=CARTESIAN_POINT ( 'NONE',  ( -0.3083989501312330295, -0.05778040916215522460, 0.4822834645669289988 ) ) ;
#58055=CARTESIAN_POINT ( 'NONE',  ( -1.325459317585300889, -0.004921259842519576551, 0.3153832671262227771 ) ) ;
#58056=CARTESIAN_POINT ( 'NONE',  ( 1.325459317585302665, 0.05413385826771626580, -0.4176697321401330321 ) ) ;
#58057=CARTESIAN_POINT ( 'NONE',  ( 1.233595800524935227, 0.2306618581243847221, -0.2411417322834647770 ) ) ;
#58058=CARTESIAN_POINT ( 'NONE',  ( 0.3280839895013130669, -0.3690944881889765550, -0.3153832671262227771 ) ) ;
#58059=CARTESIAN_POINT ( 'NONE',  ( 0.6692913385826777528, 0.2952755905511811885, 0.000000000000000000 ) ) ;
#58061=CARTESIAN_POINT ( 'NONE',  ( 0.3149606299212606708, -0.1870078740157480601, -0.3641732283464567677 ) ) ;
#58062=CARTESIAN_POINT ( 'NONE',  ( 0.1574803149606306130, -0.1870078740157479769, 0.4822834645669291653 ) ) ;
#58064=CARTESIAN_POINT ( 'NONE',  ( -1.010498687664041384, -0.4281496062992127816, -0.4176697321401328100 ) ) ;
#58065=CARTESIAN_POINT ( 'NONE',  ( 0.7152230971128614723, -0.2845877964562161244, -0.3641732283464567121 ) ) ;
#58067=CARTESIAN_POINT ( 'NONE',  ( -0.5511811023622041894, -0.1870078740157480879, -0.4822834645669291653 ) ) ;
#58069=CARTESIAN_POINT ( 'NONE',  ( -0.4986876640419939388, 0.1283753931104746893, -0.1820866141732285504 ) ) ;
#58071=CARTESIAN_POINT ( 'NONE',  ( -0.1837270341207343505, -0.6046776061558807314, 0.2411417322834647770 ) ) ;
#58072=CARTESIAN_POINT ( 'NONE',  ( -0.2755905511811015396, -0.6692913385826771977, 8.415575281601705876E-17 ) ) ;
#58073=CARTESIAN_POINT ( 'NONE',  ( 0.5314960629921264834, 0.07958543189024071263, -0.2665933059059888421 ) ) ;
#58075=CARTESIAN_POINT ( 'NONE',  ( -0.1115485564304453947, -0.6692913385826771977, 0.1292274648535927661 ) ) ;
#58077=CARTESIAN_POINT ( 'NONE',  ( 0.8727034120734913358, -0.08942795157527998196, 0.3641732283464567121 ) ) ;
#58078=CARTESIAN_POINT ( 'NONE',  ( 1.305774278215223960, 0.2952755905511810774, -0.1292274648535930714 ) ) ;
#58079=CARTESIAN_POINT ( 'NONE',  ( -1.003937007874015297, -0.4536011799217368745, -0.2665933059059886201 ) ) ;
#58080=CARTESIAN_POINT ( 'NONE',  ( -0.8333333333333323711, -0.5511811023622048555, -0.09757992244046775898 ) ) ;
#58081=CARTESIAN_POINT ( 'NONE',  ( -0.8661417322834640276, -0.1870078740157479769, 0.4822834645669291653 ) ) ;
#58082=CARTESIAN_POINT ( 'NONE',  ( -0.1902887139107604098, -0.6692913385826771977, 0.1292274648535927661 ) ) ;
#58083=CARTESIAN_POINT ( 'NONE',  ( 0.6167979002624679463, -0.004921259842519870586, -0.3153832671262229437 ) ) ;
#58085=CARTESIAN_POINT ( 'NONE',  ( 1.122047244094488860, 0.07958543189024085140, 0.2665933059059887866 ) ) ;
#58087=CARTESIAN_POINT ( 'NONE',  ( 0.8530183727034128527, -0.4281496062992124485, 0.4176697321401328655 ) ) ;
#58089=CARTESIAN_POINT ( 'NONE',  ( -0.2165354330708654795, -0.5400638737290845981, -0.3530559997133363437 ) ) ;
#58091=CARTESIAN_POINT ( 'NONE',  ( -1.712598425196849572, 0.1660481256975885056, 0.3530559997133364547 ) ) ;
#58092=CARTESIAN_POINT ( 'NONE',  ( 0.5314960629921267055, -0.5400638737290844871, 0.3530559997133364547 ) ) ;
#58093=CARTESIAN_POINT ( 'NONE',  ( 0.3083989501312343062, -0.05778040916215560624, -0.4822834645669293319 ) ) ;
#58095=CARTESIAN_POINT ( 'NONE',  ( 0.5577427821522316087, -0.08942795157527998196, 0.3641732283464567121 ) ) ;
#58096=CARTESIAN_POINT ( 'NONE',  ( 0.9645669291338591078, -0.5400638737290845981, -0.3530559997133363437 ) ) ;
#58097=CARTESIAN_POINT ( 'NONE',  ( -0.1968503937007867743, -0.5511811023622047445, 6.969142054262312111E-17 ) ) ;
#58098=CARTESIAN_POINT ( 'NONE',  ( -0.6627296587926501115, 0.2952755905511810774, -0.1292274648535930714 ) ) ;
#58099=CARTESIAN_POINT ( 'NONE',  ( 0.8561328129276796206, 8.471767977567108961E-16, -0.4445507791589058955 ) ) ;
#58100=CARTESIAN_POINT ( 'NONE',  ( -0.2034120734908131112, -0.6692913385826773087, -0.1292274648535924053 ) ) ;
#58101=CARTESIAN_POINT ( 'NONE',  ( -1.417322834645668772, -0.1870078740157480879, -0.4822834645669291653 ) ) ;
#58102=CARTESIAN_POINT ( 'NONE',  ( -0.7480314960629914633, 0.1771653543307087630, 0.000000000000000000 ) ) ;
#58103=CARTESIAN_POINT ( 'NONE',  ( 0.5511811023622054106, -0.1870078740157480879, -0.4822834645669291653 ) ) ;
#58104=CARTESIAN_POINT ( 'NONE',  ( -1.358267716535432434, 0.1660481256975883668, -0.3530559997133364547 ) ) ;
#58105=CARTESIAN_POINT ( 'NONE',  ( -0.5118110236220466680, 0.2952755905511811885, 0.000000000000000000 ) ) ;
#58108=CARTESIAN_POINT ( 'NONE',  ( 1.509186351706037543, -0.4281496062992127816, -0.4176697321401328100 ) ) ;
#58109=CARTESIAN_POINT ( 'NONE',  ( 1.489501312335958172, -0.3162353388693405765, 0.4822834645669290543 ) ) ;
#58112=CARTESIAN_POINT ( 'NONE',  ( -1.286089238845143479, -0.6046776061558807314, 0.2411417322834647770 ) ) ;
#58115=ORIENTED_EDGE ( 'NONE', *, *, #9984, .F. ) ;
#58116=CARTESIAN_POINT ( 'NONE',  ( 0.04593175853018440641, -0.5511811023622046335, 0.09757992244046803654 ) ) ;
#58119=CARTESIAN_POINT ( 'NONE',  ( 0.09842519685039434474, -0.5400638737290845981, -0.3530559997133363437 ) ) ;
#58120=CARTESIAN_POINT ( 'NONE',  ( 0.4002624671916016896, -0.3162353388693409650, -0.4822834645669289433 ) ) ;
#58123=CARTESIAN_POINT ( 'NONE',  ( -0.2755905511811015396, -0.5511811023622047445, 6.969142054262312111E-17 ) ) ;
#58124=CARTESIAN_POINT ( 'NONE',  ( 0.3249695492770460770, 1.223219560026271499E-15, 0.4445507791589056734 ) ) ;
#58125=CARTESIAN_POINT ( 'NONE',  ( 0.9120734908136490793, 0.2952755905511810774, -0.1292274648535930714 ) ) ;
#58126=CARTESIAN_POINT ( 'NONE',  ( 0.8989501312335963501, -0.5511811023622048555, -0.09757992244046775898 ) ) ;
#58127=CARTESIAN_POINT ( 'NONE',  ( -0.6233595800524928121, -0.3162353388693409650, -0.4822834645669289433 ) ) ;
#58129=CARTESIAN_POINT ( 'NONE',  ( -0.9055118110236215490, -0.6692913385826771977, 8.415575281601705876E-17 ) ) ;
#58130=CARTESIAN_POINT ( 'NONE',  ( -1.286089238845143479, -0.5023911411419708095, 0.1820866141732285504 ) ) ;
#58131=CARTESIAN_POINT ( 'NONE',  ( -1.023622047244094002, -0.1870078740157480879, -0.4822834645669291653 ) ) ;
#58132=CARTESIAN_POINT ( 'NONE',  ( 1.496062992125985147, -0.1870078740157479769, 0.4822834645669291653 ) ) ;
#58134=ORIENTED_EDGE ( 'NONE', *, *, #57357, .F. ) ;
#58136=CARTESIAN_POINT ( 'NONE',  ( 0.1181102362204730916, 0.2952755905511811885, 0.000000000000000000 ) ) ;
#58137=ORIENTED_EDGE ( 'NONE', *, *, #31097, .T. ) ;
#58138=CARTESIAN_POINT ( 'NONE',  ( -0.9580052493438311334, -0.4281496062992124485, 0.4176697321401328655 ) ) ;
#58139=CARTESIAN_POINT ( 'NONE',  ( 1.581364829396326277, -0.05778040916215522460, 0.4822834645669289988 ) ) ;
#58140=CARTESIAN_POINT ( 'NONE',  ( 1.102362204724410155, -0.1870078740157479769, 0.4822834645669291653 ) ) ;
#58141=CARTESIAN_POINT ( 'NONE',  ( 0.06561679790026316017, 0.05413385826771626580, -0.4176697321401330321 ) ) ;
#58143=CARTESIAN_POINT ( 'NONE',  ( 0.06561679790026316017, -0.4281496062992124485, 0.4176697321401328655 ) ) ;
#58145=CARTESIAN_POINT ( 'NONE',  ( -1.200787401574802349, 0.1660481256975883668, -0.3530559997133364547 ) ) ;
#58146=CARTESIAN_POINT ( 'NONE',  ( -0.01968503937007793844, 0.1660481256975883668, -0.3530559997133364547 ) ) ;
#58147=CARTESIAN_POINT ( 'NONE',  ( -0.2427821522309703550, -0.2845877964562159024, 0.3641732283464567677 ) ) ;
#58148=CARTESIAN_POINT ( 'NONE',  ( 1.620734908136483465, -0.6692913385826771977, 0.1292274648535927661 ) ) ;
#58149=CARTESIAN_POINT ( 'NONE',  ( 1.463254593175853824, -0.6692913385826771977, 0.1292274648535927661 ) ) ;
#58150=CARTESIAN_POINT ( 'NONE',  ( -0.5971128608923877978, 0.2952755905511811885, 0.1292274648535926551 ) ) ;
#58151=CARTESIAN_POINT ( 'NONE',  ( 0.2489931967792015644, 0.004960608223780119466, 0.3437734562760182411 ) ) ;
#58152=CARTESIAN_POINT ( 'NONE',  ( 1.122047244094488860, 0.1660481256975885056, 0.3530559997133364547 ) ) ;
#58157=CARTESIAN_POINT ( 'NONE',  ( 0.1377952755905518800, 0.1660481256975883668, -0.3530559997133364547 ) ) ;
#58158=CARTESIAN_POINT ( 'NONE',  ( -0.4527559055118102749, 0.07958543189024085140, 0.2665933059059887866 ) ) ;
#58159=CARTESIAN_POINT ( 'NONE',  ( 1.476377952755906442, -0.4536011799217367080, 0.2665933059059888421 ) ) ;
#58162=CARTESIAN_POINT ( 'NONE',  ( 1.594488188976378673, -0.4536011799217368745, -0.2665933059059886201 ) ) ;
#58163=CARTESIAN_POINT ( 'NONE',  ( 1.607611548556431069, 0.2952755905511811885, 0.1292274648535926551 ) ) ;
#58165=CARTESIAN_POINT ( 'NONE',  ( -0.02624671916010428221, -0.6046776061558807314, 0.2411417322834647770 ) ) ;
#58167=CARTESIAN_POINT ( 'NONE',  ( -1.410761154855642463, -0.05778040916215522460, 0.4822834645669289988 ) ) ;
#58168=CARTESIAN_POINT ( 'NONE',  ( 0.2230971128608929543, 0.05413385826771626580, -0.4176697321401330321 ) ) ;
#58170=CARTESIAN_POINT ( 'NONE',  ( 1.679790026246720025, 0.2306618581243848609, 0.2411417322834645549 ) ) ;
#58171=CARTESIAN_POINT ( 'NONE',  ( 1.056430446194226436, -0.6692913385826773087, -0.1292274648535924053 ) ) ;
#58172=CARTESIAN_POINT ( 'NONE',  ( 1.003937007874016407, -0.4536011799217367080, 0.2665933059059888421 ) ) ;
#58173=CARTESIAN_POINT ( 'NONE',  ( 0.8464566929133864326, 0.1012011053420775880, -0.2882089793578257453 ) ) ;
#58174=CARTESIAN_POINT ( 'NONE',  ( 0.9251968503937015864, 0.07958543189024071263, -0.2665933059059888421 ) ) ;
#58175=CARTESIAN_POINT ( 'NONE',  ( -1.279527559055116948, 0.1660481256975883668, -0.3530559997133364547 ) ) ;
#58177=CARTESIAN_POINT ( 'NONE',  ( 1.377952755905512472, 0.2952755905511811885, 0.000000000000000000 ) ) ;
#58179=CARTESIAN_POINT ( 'NONE',  ( 0.8464566929133866546, -0.5400638737290844871, 0.3530559997133364547 ) ) ;
#58182=CARTESIAN_POINT ( 'NONE',  ( 0.3543307086614179147, 0.1771653543307087630, 0.000000000000000000 ) ) ;
#58183=CARTESIAN_POINT ( 'NONE',  ( 0.7086614173228353852, -0.1870078740157479769, 0.4822834645669291653 ) ) ;
#58185=CARTESIAN_POINT ( 'NONE',  ( -1.062992125984250968, 0.1771653543307087630, 0.000000000000000000 ) ) ;
#58186=CARTESIAN_POINT ( 'NONE',  ( -1.213910761154854745, 0.2952755905511810774, -0.1292274648535930714 ) ) ;
#58188=CARTESIAN_POINT ( 'NONE',  ( 1.509186351706037543, 0.05413385826771666132, 0.4176697321401328100 ) ) ;
#58189=EDGE_CURVE ( 'NONE', #54098, #81558, #32028, .T. ) ;
#58190=CARTESIAN_POINT ( 'NONE',  ( -1.036745406824146176, 0.05413385826771626580, -0.4176697321401330321 ) ) ;
#58191=CARTESIAN_POINT ( 'NONE',  ( 0.7611548556430454138, 0.2306618581243847221, -0.2411417322834647770 ) ) ;
#58192=CARTESIAN_POINT ( 'NONE',  ( -1.332020997375327642, -0.08942795157527998196, 0.3641732283464567121 ) ) ;
#58194=CARTESIAN_POINT ( 'NONE',  ( 1.062992125984252745, -0.6692913385826771977, 8.415575281601705876E-17 ) ) ;
#58197=CARTESIAN_POINT ( 'NONE',  ( 1.213910761154856299, 0.2952755905511811885, 0.1292274648535926551 ) ) ;
#58198=CARTESIAN_POINT ( 'NONE',  ( -0.9973753280839886548, -0.5023911411419708095, -0.1820866141732282451 ) ) ;
#58199=CARTESIAN_POINT ( 'NONE',  ( 1.679790026246720025, 0.1283753931104748280, 0.1820866141732283561 ) ) ;
#58200=CARTESIAN_POINT ( 'NONE',  ( -1.233595800524933894, -0.5023911411419708095, -0.1820866141732282451 ) ) ;
#58201=CARTESIAN_POINT ( 'NONE',  ( -0.5052493438320203589, 0.1771653543307087075, -0.09757992244046823083 ) ) ;
#58202=CARTESIAN_POINT ( 'NONE',  ( -1.699475065616797398, 0.1771653543307087630, 0.09757992244046791164 ) ) ;
#58203=CARTESIAN_POINT ( 'NONE',  ( 0.7677165354330716118, -0.4536011799217367080, 0.2665933059059888421 ) ) ;
#58205=CARTESIAN_POINT ( 'NONE',  ( 0.3346456692913393205, -0.5400638737290845981, -0.3530559997133363437 ) ) ;
#58206=CARTESIAN_POINT ( 'NONE',  ( 1.345144356955381593, -0.3162353388693409650, -0.4822834645669289433 ) ) ;
#58207=CARTESIAN_POINT ( 'NONE',  ( -0.1509186351706028884, -0.3162353388693409650, -0.4822834645669289433 ) ) ;
#58208=CARTESIAN_POINT ( 'NONE',  ( 0.7349081364829402885, -0.5023911411419708095, -0.1820866141732282451 ) ) ;
#58209=CARTESIAN_POINT ( 'NONE',  ( -1.646981627296586703, -0.05778040916215522460, 0.4822834645669289988 ) ) ;
#58211=CARTESIAN_POINT ( 'NONE',  ( -1.443569553805773564, 0.2306618581243847221, -0.2411417322834647770 ) ) ;
#58212=CARTESIAN_POINT ( 'NONE',  ( -0.7020997375328076329, -0.3162353388693409650, -0.4822834645669289433 ) ) ;
#58215=CARTESIAN_POINT ( 'NONE',  ( 0.2099737532808405305, 0.2306618581243847221, -0.2411417322834647770 ) ) ;
#58216=CARTESIAN_POINT ( 'NONE',  ( -0.2493438320209966919, -0.4281496062992124485, 0.4176697321401328655 ) ) ;
#58217=CARTESIAN_POINT ( 'NONE',  ( 0.2559055118110243332, -0.5400638737290845981, -0.3530559997133363437 ) ) ;
#58223=CARTESIAN_POINT ( 'NONE',  ( -0.7414698162729651543, 0.1771653543307087075, -0.09757992244046823083 ) ) ;
#58225=CARTESIAN_POINT ( 'NONE',  ( -1.089238845144356427, 0.05413385826771666132, 0.4176697321401328100 ) ) ;
#58227=CARTESIAN_POINT ( 'NONE',  ( 0.5839895013123367340, 0.2952755905511811885, 0.1292274648535926551 ) ) ;
#58228=CARTESIAN_POINT ( 'NONE',  ( 0.08530183727034192087, -0.2845877964562161244, -0.3641732283464567121 ) ) ;
#58229=CARTESIAN_POINT ( 'NONE',  ( 1.194225721784777594, -0.4281496062992127816, -0.4176697321401328100 ) ) ;
#58230=CARTESIAN_POINT ( 'NONE',  ( 0.3871391076115492380, -0.05778040916215560624, -0.4822834645669293319 ) ) ;
#58234=CARTESIAN_POINT ( 'NONE',  ( 1.207349081364829990, 0.2306618581243848609, 0.2411417322834645549 ) ) ;
#58235=CARTESIAN_POINT ( 'NONE',  ( 0.6299212598425204535, -0.1870078740157479769, 0.4822834645669291653 ) ) ;
#58236=CARTESIAN_POINT ( 'NONE',  ( 0.05249343832021075018, 0.2306618581243847221, -0.2411417322834647770 ) ) ;
#58237=CARTESIAN_POINT ( 'NONE',  ( 0.9120734908136489683, -0.5511811023622046335, 0.09757992244046803654 ) ) ;
#58239=CARTESIAN_POINT ( 'NONE',  ( 1.358267716535433323, 0.1660481256975885056, 0.3530559997133364547 ) ) ;
#58241=CARTESIAN_POINT ( 'NONE',  ( 0.2362204724409456558, -0.1870078740157480879, -0.4822834645669291653 ) ) ;
#58242=CARTESIAN_POINT ( 'NONE',  ( 1.240157480314961314, 0.1660481256975883668, -0.3530559997133364547 ) ) ;
#58243=CARTESIAN_POINT ( 'NONE',  ( 0.5577427821522316087, -0.05778040916215522460, 0.4822834645669289988 ) ) ;
#58245=CARTESIAN_POINT ( 'NONE',  ( 1.207349081364829990, 0.1283753931104748280, 0.1820866141732283561 ) ) ;
#58246=CARTESIAN_POINT ( 'NONE',  ( -1.010498687664041384, -0.4281496062992127816, -0.4176697321401328100 ) ) ;
#58247=CARTESIAN_POINT ( 'NONE',  ( -0.8661417322834640276, -0.1870078740157480879, -0.4822834645669291653 ) ) ;
#58248=CARTESIAN_POINT ( 'NONE',  ( 1.069553805774278610, -0.6692913385826771977, 0.1292274648535927661 ) ) ;
#58254=ORIENTED_EDGE ( 'NONE', *, *, #40513, .T. ) ;
#58255=CARTESIAN_POINT ( 'NONE',  ( 1.469816272965879911, -0.6046776061558807314, 0.2411417322834647770 ) ) ;
#58256=CARTESIAN_POINT ( 'NONE',  ( 0.8464566929133865436, 0.07958543189024071263, -0.2665933059059888421 ) ) ;
#58257=CARTESIAN_POINT ( 'NONE',  ( -0.7749820319012115100, 0.000000000000000000, 0.3464511005275205946 ) ) ;
#58262=CARTESIAN_POINT ( 'NONE',  ( -1.246719160104985846, -0.3690944881889765550, -0.3153832671262227771 ) ) ;
#58263=CARTESIAN_POINT ( 'NONE',  ( -1.450131233595799651, -0.5511811023622046335, 0.09757992244046803654 ) ) ;
#58264=CARTESIAN_POINT ( 'NONE',  ( -1.299212598425196097, 0.2952755905511811885, 0.000000000000000000 ) ) ;
#58265=CARTESIAN_POINT ( 'NONE',  ( -0.1181102362204717315, 0.2952755905511811885, 0.000000000000000000 ) ) ;
#58266=CARTESIAN_POINT ( 'NONE',  ( 1.443569553805774897, 0.2306618581243848609, 0.2411417322834645549 ) ) ;
#58267=ORIENTED_EDGE ( 'NONE', *, *, #72340, .T. ) ;
#58271=CARTESIAN_POINT ( 'NONE',  ( -1.614173228346457378, 1.881821177735609085, -0.1372047244094477536 ) ) ;
#58272=CARTESIAN_POINT ( 'NONE',  ( -1.056430446194224881, -0.5511811023622046335, 0.09757992244046803654 ) ) ;
#58273=CARTESIAN_POINT ( 'NONE',  ( -1.404199475065615932, -0.4281496062992127816, -0.4176697321401328100 ) ) ;
#58274=CARTESIAN_POINT ( 'NONE',  ( 0.5314960629921267055, -0.5400638737290844871, 0.3530559997133364547 ) ) ;
#58275=ORIENTED_EDGE ( 'NONE', *, *, #58647, .T. ) ;
#58278=CARTESIAN_POINT ( 'NONE',  ( 1.246719160104987623, 0.05413385826771626580, -0.4176697321401330321 ) ) ;
#58279=CARTESIAN_POINT ( 'NONE',  ( -1.587926509186350810, -0.4281496062992124485, 0.4176697321401328655 ) ) ;
#58281=CARTESIAN_POINT ( 'NONE',  ( -0.2559055118110230564, 0.07958543189024071263, -0.2665933059059888421 ) ) ;
#58282=CARTESIAN_POINT ( 'NONE',  ( -1.443569553805773564, 0.1283753931104746893, -0.1820866141732285504 ) ) ;
#58283=CARTESIAN_POINT ( 'NONE',  ( 0.5611900217179910388, 1.223219560026271499E-15, 0.4445507791589056734 ) ) ;
#58284=CARTESIAN_POINT ( 'NONE',  ( -0.5446194225721777693, -0.08942795157527998196, 0.3641732283464567121 ) ) ;
#58285=CARTESIAN_POINT ( 'NONE',  ( 0.2099737532808405305, 0.1283753931104746893, -0.1820866141732285504 ) ) ;
#58286=ADVANCED_FACE ( 'NONE', ( #26780 ), #34311, .F. ) ;
#58287=CARTESIAN_POINT ( 'NONE',  ( 0.3083989501312343062, -0.3162353388693405765, 0.4822834645669290543 ) ) ;
#58288=CARTESIAN_POINT ( 'NONE',  ( -1.154855643044618851, 0.1283753931104748280, 0.1820866141732283561 ) ) ;
#58290=CARTESIAN_POINT ( 'NONE',  ( 0.6955380577427828781, 0.05413385826771626580, -0.4176697321401330321 ) ) ;
#58292=CARTESIAN_POINT ( 'NONE',  ( -1.522309711286088607, -0.6046776061558807314, 0.2411417322834647770 ) ) ;
#58294=CARTESIAN_POINT ( 'NONE',  ( -0.3674540682414692561, -0.6046776061558809534, -0.2411417322834644161 ) ) ;
#58295=CARTESIAN_POINT ( 'NONE',  ( 0.1706036745406830368, -0.004921259842519576551, 0.3153832671262227771 ) ) ;
#58296=CARTESIAN_POINT ( 'NONE',  ( -0.8858267716535425107, -0.5400638737290844871, 0.3530559997133364547 ) ) ;
#58297=CARTESIAN_POINT ( 'NONE',  ( 0.8005249343832028242, -0.3690944881889765550, -0.3153832671262227771 ) ) ;
#58298=CARTESIAN_POINT ( 'NONE',  ( -0.1246719160104980823, 0.1771653543307087630, 0.09757992244046791164 ) ) ;
#58299=CARTESIAN_POINT ( 'NONE',  ( -0.6430446194225716283, -0.4281496062992124485, 0.4176697321401328655 ) ) ;
#58300=CARTESIAN_POINT ( 'NONE',  ( -1.489501312335957062, -0.05778040916215522460, 0.4822834645669289988 ) ) ;
#58301=CARTESIAN_POINT ( 'NONE',  ( -0.7535225988626923499, 2.401574803149606474, 0.4915354330708645025 ) ) ;
#58302=CARTESIAN_POINT ( 'NONE',  ( 1.292650918635171564, -0.5511811023622048555, -0.09757992244046775898 ) ) ;
#58304=CARTESIAN_POINT ( 'NONE',  ( -1.587926509186350810, 0.05413385826771626580, -0.4176697321401330321 ) ) ;
#58305=CARTESIAN_POINT ( 'NONE',  ( -1.397637795275589623, 0.1660481256975885056, 0.3530559997133364547 ) ) ;
#58308=EDGE_CURVE ( 'NONE', #74503, #57928, #40248, .T. ) ;
#58309=CARTESIAN_POINT ( 'NONE',  ( -0.8530183727034112984, -0.004921259842519576551, 0.3153832671262227771 ) ) ;
#58310=CARTESIAN_POINT ( 'NONE',  ( 0.6299212598425204535, -0.1870078740157479769, 0.4822834645669291653 ) ) ;
#58311=CARTESIAN_POINT ( 'NONE',  ( -1.108923884514435132, -0.2845877964562159024, 0.3641732283464567677 ) ) ;
#58313=CARTESIAN_POINT ( 'NONE',  ( -1.174540682414697335, -0.3162353388693409650, -0.4822834645669289433 ) ) ;
#58314=CARTESIAN_POINT ( 'NONE',  ( 1.062992125984252745, 0.2952755905511811885, 0.000000000000000000 ) ) ;
#58315=CARTESIAN_POINT ( 'NONE',  ( 0.5839895013123367340, 0.2952755905511811885, 0.1292274648535926551 ) ) ;
#58318=CARTESIAN_POINT ( 'NONE',  ( -1.312335958005248715, -0.5023911411419708095, -0.1820866141732282451 ) ) ;
#58323=CARTESIAN_POINT ( 'NONE',  ( 0.4889872687189469325, 1.535433070866141225, -0.4915354330708656683 ) ) ;
#58324=CARTESIAN_POINT ( 'NONE',  ( 0.8923884514435703741, 0.1283753931104748280, 0.1820866141732283561 ) ) ;
#58325=CARTESIAN_POINT ( 'NONE',  ( 0.2821522309711292364, -0.5511811023622046335, 0.09757992244046803654 ) ) ;
#58326=CARTESIAN_POINT ( 'NONE',  ( -0.006561679790025524116, -0.3162353388693405765, 0.4822834645669290543 ) ) ;
#58327=CARTESIAN_POINT ( 'NONE',  ( 1.489501312335958172, -0.05778040916215560624, -0.4822834645669293319 ) ) ;
#58329=CARTESIAN_POINT ( 'NONE',  ( 0.2755905511811031494, 0.1771653543307087630, 0.000000000000000000 ) ) ;
#58330=CARTESIAN_POINT ( 'NONE',  ( -0.8661417322834640276, -0.1870078740157479769, 0.4822834645669291653 ) ) ;
#58331=CARTESIAN_POINT ( 'NONE',  ( -1.128608923884513837, 0.2306618581243847221, -0.2411417322834647770 ) ) ;
#58332=CARTESIAN_POINT ( 'NONE',  ( 0.7611548556430454138, 0.2306618581243847221, -0.2411417322834647770 ) ) ;
#58334=CARTESIAN_POINT ( 'NONE',  ( -0.7611548556430438595, 0.2306618581243848609, 0.2411417322834645549 ) ) ;
#58337=CARTESIAN_POINT ( 'NONE',  ( -1.351706036745406347, 0.05413385826771626580, -0.4176697321401330321 ) ) ;
#58338=CARTESIAN_POINT ( 'NONE',  ( -0.6496062992125976043, 0.1660481256975883668, -0.3530559997133364547 ) ) ;
#58339=CARTESIAN_POINT ( 'NONE',  ( -0.7283464566929126471, -0.4536011799217367080, 0.2665933059059888421 ) ) ;
#58340=CARTESIAN_POINT ( 'NONE',  ( -0.6102362204724400829, -0.5400638737290845981, -0.3530559997133363437 ) ) ;
#58343=ADVANCED_FACE ( 'NONE', ( #41899 ), #37002, .F. ) ;
#58344=CARTESIAN_POINT ( 'NONE',  ( 1.666666666666667185, 0.05413385826771666132, 0.4176697321401328100 ) ) ;
#58345=CARTESIAN_POINT ( 'NONE',  ( -1.056430446194224881, 0.2952755905511810774, -0.1292274648535930714 ) ) ;
#58346=CARTESIAN_POINT ( 'NONE',  ( 0.1771653543307093182, 0.1660481256975885056, 0.3530559997133364547 ) ) ;
#58347=CARTESIAN_POINT ( 'NONE',  ( -0.8202099737532799750, 0.2952755905511810774, -0.1292274648535930714 ) ) ;
#58348=CARTESIAN_POINT ( 'NONE',  ( 0.8136482939632553313, 0.2306618581243848609, 0.2411417322834645549 ) ) ;
#58350=CARTESIAN_POINT ( 'NONE',  ( -0.6299212598425188991, -0.1870078740157480601, -0.3641732283464567677 ) ) ;
#58354=CARTESIAN_POINT ( 'NONE',  ( -1.220472440944881054, 0.8346805926620878280, 0.5309055118110237448 ) ) ;
#58355=CARTESIAN_POINT ( 'NONE',  ( -1.069553805774277722, 0.2952755905511811885, 0.1292274648535926551 ) ) ;
#58356=CARTESIAN_POINT ( 'NONE',  ( -1.371391076115484609, -0.6692913385826771977, 0.1292274648535927661 ) ) ;
#58358=CARTESIAN_POINT ( 'NONE',  ( -1.279527559055116948, -0.5400638737290844871, 0.3530559997133364547 ) ) ;
#58359=CARTESIAN_POINT ( 'NONE',  ( -1.220472440944881054, 0.2952755905511811885, 0.000000000000000000 ) ) ;
#58360=CARTESIAN_POINT ( 'NONE',  ( -1.240157480314959759, -0.5400638737290845981, -0.3530559997133363437 ) ) ;
#58363=CARTESIAN_POINT ( 'NONE',  ( -0.01968503937007793844, 0.07958543189024071263, -0.2665933059059888421 ) ) ;
#58366=CARTESIAN_POINT ( 'NONE',  ( -0.4068241469816267775, -0.004921259842519870586, -0.3153832671262229437 ) ) ;
#58368=CARTESIAN_POINT ( 'NONE',  ( -0.8267716535433065062, 0.2952755905511811885, 0.000000000000000000 ) ) ;
#58369=CARTESIAN_POINT ( 'NONE',  ( 1.233595800524935227, -0.6046776061558807314, 0.2411417322834647770 ) ) ;
#58370=CARTESIAN_POINT ( 'NONE',  ( -0.7020997375328074108, -0.05778040916215522460, 0.4822834645669289988 ) ) ;
#58371=VERTEX_POINT ( 'NONE', #9103 ) ;
#58372=ORIENTED_EDGE ( 'NONE', *, *, #80532, .T. ) ;
#58374=CARTESIAN_POINT ( 'NONE',  ( -0.8530183727034112984, 0.05413385826771666132, 0.4176697321401328100 ) ) ;
#58375=CARTESIAN_POINT ( 'NONE',  ( 1.318897637795276356, 0.1660481256975883668, -0.3530559997133364547 ) ) ;
#58376=CARTESIAN_POINT ( 'NONE',  ( -1.587926509186350810, -0.3690944881889763329, 0.3153832671262228327 ) ) ;
#58377=CARTESIAN_POINT ( 'NONE',  ( -1.305774278215222184, -0.6692913385826773087, -0.1292274648535924053 ) ) ;
#58379=EDGE_CURVE ( 'NONE', #34463, #4617, #19513, .T. ) ;
#58383=CARTESIAN_POINT ( 'NONE',  ( -0.3674540682414689785, 0.2306618581243848609, 0.2411417322834645549 ) ) ;
#58384=CARTESIAN_POINT ( 'NONE',  ( -1.476377952755905110, 0.07958543189024085140, 0.2665933059059887866 ) ) ;
#58385=CARTESIAN_POINT ( 'NONE',  ( -0.8727034120734901146, -0.05778040916215560624, -0.4822834645669293319 ) ) ;
#58387=CARTESIAN_POINT ( 'NONE',  ( -1.102362204724408601, -0.1870078740157479769, 0.4822834645669291653 ) ) ;
#58388=CARTESIAN_POINT ( 'NONE',  ( -0.1968503937007867743, 0.2952755905511811885, 0.000000000000000000 ) ) ;
#58389=CARTESIAN_POINT ( 'NONE',  ( -1.010498687664041384, -0.4281496062992127816, -0.4176697321401328100 ) ) ;
#58390=CARTESIAN_POINT ( 'NONE',  ( -0.3805774278215216522, -0.4281496062992127816, -0.4176697321401328100 ) ) ;
#58391=AXIS2_PLACEMENT_3D ( 'NONE', #82995, #63218, #5150 ) ;
#58393=CARTESIAN_POINT ( 'NONE',  ( 1.036745406824147508, -0.3690944881889765550, -0.3153832671262227771 ) ) ;
#58395=CARTESIAN_POINT ( 'NONE',  ( 0.9580052493438327987, -0.3690944881889765550, -0.3153832671262227771 ) ) ;
#58396=CARTESIAN_POINT ( 'NONE',  ( 1.279527559055118724, 0.07958543189024085140, 0.2665933059059887866 ) ) ;
#58397=CARTESIAN_POINT ( 'NONE',  ( 1.397637795275591177, -0.5400638737290844871, 0.3530559997133364547 ) ) ;
#58398=CARTESIAN_POINT ( 'NONE',  ( 0.2427821522309719648, -0.08942795157527998196, 0.3641732283464567121 ) ) ;
#58400=CARTESIAN_POINT ( 'NONE',  ( -1.062992125984250968, -0.6692913385826771977, 8.415575281601705876E-17 ) ) ;
#58401=CARTESIAN_POINT ( 'NONE',  ( 1.141732283464567566, 0.2952755905511811885, 0.000000000000000000 ) ) ;
#58402=EDGE_CURVE ( 'NONE', #68129, #27226, #22063, .T. ) ;
#58404=CARTESIAN_POINT ( 'NONE',  ( -0.6496062992125976043, 0.07958543189024071263, -0.2665933059059888421 ) ) ;
#58406=CARTESIAN_POINT ( 'NONE',  ( 0.2952755905511819101, 0.1660481256975883668, -0.3530559997133364547 ) ) ;
#58408=CARTESIAN_POINT ( 'NONE',  ( 0.8136482939632553313, 0.1283753931104748280, 0.1820866141732283561 ) ) ;
#58409=CARTESIAN_POINT ( 'NONE',  ( 0.3346456692913390985, 0.07958543189024085140, 0.2665933059059887866 ) ) ;
#58410=CARTESIAN_POINT ( 'NONE',  ( -0.4002624671916004129, -0.3162353388693405765, 0.4822834645669290543 ) ) ;
#58411=CARTESIAN_POINT ( 'NONE',  ( -1.404199475065615932, 0.05413385826771666132, 0.4176697321401328100 ) ) ;
#58412=CARTESIAN_POINT ( 'NONE',  ( -0.6496062992125976043, 0.07958543189024071263, -0.2665933059059888421 ) ) ;
#58414=CARTESIAN_POINT ( 'NONE',  ( 0.5511811023622055217, -0.1870078740157479769, 0.4822834645669291653 ) ) ;
#58415=CARTESIAN_POINT ( 'NONE',  ( -1.030183727034119867, -0.3162353388693405765, 0.4822834645669290543 ) ) ;
#58418=CARTESIAN_POINT ( 'NONE',  ( 0.3740157480314966754, 0.07958543189024071263, -0.2665933059059888421 ) ) ;
#58419=CARTESIAN_POINT ( 'NONE',  ( -0.7086614173228339419, -0.1870078740157479769, 0.4822834645669291653 ) ) ;
#58420=CARTESIAN_POINT ( 'NONE',  ( -1.253280839895012377, -0.3162353388693409650, -0.4822834645669289433 ) ) ;
#58421=CARTESIAN_POINT ( 'NONE',  ( -1.430446194225720724, -0.004921259842519870586, -0.3153832671262229437 ) ) ;
#58423=CARTESIAN_POINT ( 'NONE',  ( -1.082677165354329896, -0.4536011799217368745, -0.2665933059059886201 ) ) ;
#58424=CARTESIAN_POINT ( 'NONE',  ( -1.528871391076114250, 0.1771653543307087075, -0.09757992244046823083 ) ) ;
#58425=CARTESIAN_POINT ( 'NONE',  ( 1.108923884514436242, -0.05778040916215522460, 0.4822834645669289988 ) ) ;
#58429=CARTESIAN_POINT ( 'NONE',  ( 0.5411721830064198935, 8.471767977567108961E-16, -0.4445507791589058955 ) ) ;
#58430=CARTESIAN_POINT ( 'NONE',  ( -1.686351706036744558, 0.2952755905511810774, -0.1292274648535930714 ) ) ;
#58431=CARTESIAN_POINT ( 'NONE',  ( -1.213910761154854745, 0.2952755905511810774, -0.1292274648535930714 ) ) ;
#58432=CARTESIAN_POINT ( 'NONE',  ( 1.377952755905512472, -0.6692913385826771977, 8.415575281601705876E-17 ) ) ;
#58435=CARTESIAN_POINT ( 'NONE',  ( 0.4921259842519691285, -0.5400638737290845981, -0.3530559997133363437 ) ) ;
#58436=CARTESIAN_POINT ( 'NONE',  ( 0.006561679790026889343, -0.3162353388693409650, -0.4822834645669289433 ) ) ;
#58439=CARTESIAN_POINT ( 'NONE',  ( 0.8005249343832027131, -0.004921259842519576551, 0.3153832671262227771 ) ) ;
#58446=CARTESIAN_POINT ( 'NONE',  ( 0.1837270341207354329, 0.2306618581243848609, 0.2411417322834645549 ) ) ;
#58447=CARTESIAN_POINT ( 'NONE',  ( -1.581364829396324945, -0.05778040916215560624, -0.4822834645669293319 ) ) ;
#58448=CARTESIAN_POINT ( 'NONE',  ( 0.7808398950131241190, -0.05778040916215560624, -0.4822834645669293319 ) ) ;
#58449=CARTESIAN_POINT ( 'NONE',  ( 1.095800524934383846, -0.05778040916215560624, -0.4822834645669293319 ) ) ;
#58450=CARTESIAN_POINT ( 'NONE',  ( 1.417322834645670104, -0.1870078740157479769, 0.4822834645669291653 ) ) ;
#58452=CARTESIAN_POINT ( 'NONE',  ( -0.4855643044619415427, 0.05413385826771626580, -0.4176697321401330321 ) ) ;
#58453=CARTESIAN_POINT ( 'NONE',  ( 0.2099737532808405305, 0.2306618581243847221, -0.2411417322834647770 ) ) ;
#58454=CARTESIAN_POINT ( 'NONE',  ( -1.633858267716534529, 0.1660481256975885056, 0.3530559997133364547 ) ) ;
#58455=CARTESIAN_POINT ( 'NONE',  ( 1.312335958005249825, 0.2306618581243847221, -0.2411417322834647770 ) ) ;
#58456=CARTESIAN_POINT ( 'NONE',  ( 1.003937007874016407, -0.5400638737290844871, 0.3530559997133364547 ) ) ;
#58457=CARTESIAN_POINT ( 'NONE',  ( 0.01312335958005323398, 0.05413385826771666132, 0.4176697321401328100 ) ) ;
#58459=CARTESIAN_POINT ( 'NONE',  ( 0.5774278215223104249, 0.1283753931104748280, 0.1820866141732283561 ) ) ;
#58462=ORIENTED_EDGE ( 'NONE', *, *, #49126, .F. ) ;
#58463=CARTESIAN_POINT ( 'NONE',  ( -0.3740157480314953431, -0.4536011799217368745, -0.2665933059059886201 ) ) ;
#58464=CARTESIAN_POINT ( 'NONE',  ( 0.07217847769028949700, -0.3162353388693405765, 0.4822834645669290543 ) ) ;
#58466=CARTESIAN_POINT ( 'NONE',  ( 0.006561679790026889343, -0.05778040916215522460, 0.4822834645669289988 ) ) ;
#58467=CARTESIAN_POINT ( 'NONE',  ( -0.03937007874015669567, -0.6692913385826771977, 8.415575281601705876E-17 ) ) ;
#58468=CARTESIAN_POINT ( 'NONE',  ( -0.8267716535433065062, -0.6692913385826771977, 8.415575281601705876E-17 ) ) ;
#58469=CARTESIAN_POINT ( 'NONE',  ( 1.279527559055118724, -0.4536011799217368745, -0.2665933059059886201 ) ) ;
#58470=CARTESIAN_POINT ( 'NONE',  ( -1.443569553805773564, 0.2306618581243847221, -0.2411417322834647770 ) ) ;
#58472=CARTESIAN_POINT ( 'NONE',  ( 0.9251968503937015864, -0.4536011799217367080, 0.2665933059059888421 ) ) ;
#58473=CARTESIAN_POINT ( 'NONE',  ( 0.2755905511811031494, 0.2952755905511811885, 0.000000000000000000 ) ) ;
#58474=CARTESIAN_POINT ( 'NONE',  ( 0.7545931758530189937, 0.2952755905511810774, -0.1292274648535930714 ) ) ;
#58479=CARTESIAN_POINT ( 'NONE',  ( -0.1902887139107604098, -0.6692913385826771977, 0.1292274648535927661 ) ) ;
#58482=CARTESIAN_POINT ( 'NONE',  ( -1.200787401574802349, -0.4536011799217367080, 0.2665933059059888421 ) ) ;
#58483=CARTESIAN_POINT ( 'NONE',  ( 1.187664041994751285, -0.3162353388693409650, -0.4822834645669289433 ) ) ;
#58484=CARTESIAN_POINT ( 'NONE',  ( 1.456692913385827515, -0.6692913385826771977, 8.415575281601705876E-17 ) ) ;
#58485=CARTESIAN_POINT ( 'NONE',  ( -0.4199475065616791736, -0.5023911411419708095, 0.1820866141732285504 ) ) ;
#58486=CARTESIAN_POINT ( 'NONE',  ( 0.6233595800524939223, -0.3162353388693405765, 0.4822834645669290543 ) ) ;
#58488=CARTESIAN_POINT ( 'NONE',  ( 0.2690288713910767848, 0.1771653543307087630, 0.09757992244046791164 ) ) ;
#58489=CARTESIAN_POINT ( 'NONE',  ( -0.1443569553805768291, 0.05413385826771666132, 0.4176697321401328100 ) ) ;
#58491=CARTESIAN_POINT ( 'NONE',  ( -1.279527559055116948, -0.5400638737290844871, 0.3530559997133364547 ) ) ;
#58493=CARTESIAN_POINT ( 'NONE',  ( 0.3608923884514443348, 0.1771653543307087075, -0.09757992244046823083 ) ) ;
#58495=CARTESIAN_POINT ( 'NONE',  ( -0.7939632545931754048, -0.3162353388693405765, 0.4822834645669290543 ) ) ;
#58496=CARTESIAN_POINT ( 'NONE',  ( -0.3083989501312330295, -0.2845877964562161244, -0.3641732283464567121 ) ) ;
#58497=CARTESIAN_POINT ( 'NONE',  ( -1.306827173596998737, 0.000000000000000000, 0.4445507791589060065 ) ) ;
#58498=CARTESIAN_POINT ( 'NONE',  ( -0.5643044619422565855, 0.05413385826771626580, -0.4176697321401330321 ) ) ;
#58499=CARTESIAN_POINT ( 'NONE',  ( -0.3083989501312330295, -0.3162353388693409650, -0.4822834645669289433 ) ) ;
#58500=CARTESIAN_POINT ( 'NONE',  ( 0.4658792650918640033, -0.2845877964562159024, 0.3641732283464567677 ) ) ;
#58502=CARTESIAN_POINT ( 'NONE',  ( 0.09186351706036827158, 0.05413385826771666132, 0.4176697321401328100 ) ) ;
#58505=CARTESIAN_POINT ( 'NONE',  ( -1.469816272965878357, -0.5023911411419708095, -0.1820866141732282451 ) ) ;
#58506=CARTESIAN_POINT ( 'NONE',  ( 0.6496062992125991586, -0.4536011799217368745, -0.2665933059059886201 ) ) ;
#58507=CARTESIAN_POINT ( 'NONE',  ( 1.601049868766404982, 0.2306618581243848609, 0.2411417322834645549 ) ) ;
#58508=CARTESIAN_POINT ( 'NONE',  ( -0.6758530183727028406, -0.5511811023622048555, -0.09757992244046775898 ) ) ;
#58509=CARTESIAN_POINT ( 'NONE',  ( -1.338582677165353729, -0.1870078740157480601, -0.3641732283464567677 ) ) ;
#58510=CARTESIAN_POINT ( 'NONE',  ( -0.7808398950131222316, -0.3162353388693409650, -0.4822834645669289433 ) ) ;
#58511=CARTESIAN_POINT ( 'NONE',  ( -0.2296587926509179312, -0.3162353388693409650, -0.4822834645669289433 ) ) ;
#58512=CARTESIAN_POINT ( 'NONE',  ( 0.5708661417322842269, 0.07958543189024085140, 0.2665933059059887866 ) ) ;
#58514=CARTESIAN_POINT ( 'NONE',  ( 0.9580052493438326877, -0.004921259842519576551, 0.3153832671262227771 ) ) ;
#58515=CARTESIAN_POINT ( 'NONE',  ( 0.4921259842519691285, -0.5400638737290845981, -0.3530559997133363437 ) ) ;
#58517=CARTESIAN_POINT ( 'NONE',  ( -0.1837270341207343505, -0.6046776061558807314, 0.2411417322834647770 ) ) ;
#58519=CARTESIAN_POINT ( 'NONE',  ( 1.417322834645670104, -0.1870078740157479769, 0.3641732283464567677 ) ) ;
#58520=CARTESIAN_POINT ( 'NONE',  ( 0.6627296587926517768, -0.6692913385826773087, -0.1292274648535924053 ) ) ;
#58521=CARTESIAN_POINT ( 'NONE',  ( 0.09842519685039434474, 0.1660481256975885056, 0.3530559997133364547 ) ) ;
#58522=CARTESIAN_POINT ( 'NONE',  ( 1.112371124080195450, -4.927456884911482678E-16, 0.4445507791589062840 ) ) ;
#58523=CARTESIAN_POINT ( 'NONE',  ( -0.05249343832020911260, 0.1283753931104748280, 0.1820866141732283561 ) ) ;
#58524=CARTESIAN_POINT ( 'NONE',  ( 0.7349081364829403995, 0.2306618581243848609, 0.2411417322834645549 ) ) ;
#58525=CARTESIAN_POINT ( 'NONE',  ( -0.3280839895013117347, -0.3690944881889763329, 0.3153832671262228327 ) ) ;
#58526=CARTESIAN_POINT ( 'NONE',  ( -0.6561679790026240244, 0.2306618581243847221, -0.2411417322834647770 ) ) ;
#58527=CARTESIAN_POINT ( 'NONE',  ( 0.8333333333333340365, 0.2952755905511810219, -0.1292274648535930437 ) ) ;
#58528=CARTESIAN_POINT ( 'NONE',  ( -0.3280839895013117347, -0.4281496062992124485, 0.4176697321401328655 ) ) ;
#58530=CARTESIAN_POINT ( 'NONE',  ( -1.272965879265091305, 0.05413385826771626580, -0.4176697321401330321 ) ) ;
#58531=CARTESIAN_POINT ( 'NONE',  ( -0.5839895013123351797, 0.1771653543307087075, -0.09757992244046823083 ) ) ;
#58532=CARTESIAN_POINT ( 'NONE',  ( -0.07874015748031421014, -0.1870078740157480879, -0.4822834645669291653 ) ) ;
#58533=CARTESIAN_POINT ( 'NONE',  ( -1.456692913385826182, -0.6692913385826771977, 8.415575281601705876E-17 ) ) ;
#58534=CARTESIAN_POINT ( 'NONE',  ( -0.8202099737532799750, 0.2952755905511810774, -0.1292274648535930714 ) ) ;
#58536=CARTESIAN_POINT ( 'NONE',  ( 1.062992125984252745, 0.2952755905511811885, 0.000000000000000000 ) ) ;
#58537=CARTESIAN_POINT ( 'NONE',  ( 1.338582677165355062, -0.1870078740157480879, -0.4822834645669291653 ) ) ;
#58538=CARTESIAN_POINT ( 'NONE',  ( 1.371391076115485941, 0.2952755905511811885, 0.1292274648535926551 ) ) ;
#58540=DIRECTION ( 'NONE',  ( -1.000000000000000000, -3.083952846180990281E-16, 0.000000000000000000 ) ) ;
#58541=CARTESIAN_POINT ( 'NONE',  ( -1.128608923884513837, -0.6046776061558807314, 0.2411417322834647770 ) ) ;
#58543=EDGE_CURVE ( 'NONE', #78494, #10845, #80040, .T. ) ;
#58545=VERTEX_POINT ( 'NONE', #15420 ) ;
#58546=CARTESIAN_POINT ( 'NONE',  ( -0.2296587926509179312, -0.08942795157527998196, 0.3641732283464567121 ) ) ;
#58549=CARTESIAN_POINT ( 'NONE',  ( 0.1509186351706042484, -0.3162353388693405765, 0.4822834645669290543 ) ) ;
#58550=CARTESIAN_POINT ( 'NONE',  ( 0.3149606299212603933, -0.1870078740157479769, 0.4822834645669291653 ) ) ;
#58553=CARTESIAN_POINT ( 'NONE',  ( -0.8923884514435688198, -0.5023911411419708095, 0.1820866141732285504 ) ) ;
#58555=CARTESIAN_POINT ( 'NONE',  ( 0.7020997375328090762, -0.3162353388693405765, 0.4822834645669290543 ) ) ;
#58556=CARTESIAN_POINT ( 'NONE',  ( 0.8464566929133865436, 0.07958543189024071263, -0.2665933059059888421 ) ) ;
#58557=CARTESIAN_POINT ( 'NONE',  ( -0.3477690288713902178, 0.2952755905511810774, -0.1292274648535930714 ) ) ;
#58559=CARTESIAN_POINT ( 'NONE',  ( -0.8398950131233585692, 0.2306618581243848609, 0.2411417322834645549 ) ) ;
#58561=CARTESIAN_POINT ( 'NONE',  ( 1.181102362204725198, -0.1870078740157479769, 0.4822834645669291653 ) ) ;
#58562=CARTESIAN_POINT ( 'NONE',  ( 1.633858267716535639, -0.4536011799217367080, 0.2665933059059888421 ) ) ;
#58565=CARTESIAN_POINT ( 'NONE',  ( -0.1246719160104980823, -0.6692913385826773087, -0.1292274648535924053 ) ) ;
#58566=VERTEX_POINT ( 'NONE', #33933 ) ;
#58568=CARTESIAN_POINT ( 'NONE',  ( -0.6430446194225716283, -0.4281496062992124485, 0.4176697321401328655 ) ) ;
#58569=CARTESIAN_POINT ( 'NONE',  ( 1.220472440944882386, -0.6692913385826771977, 8.415575281601705876E-17 ) ) ;
#58570=CARTESIAN_POINT ( 'NONE',  ( 1.056430446194226436, -0.6692913385826773087, -0.1292274648535924053 ) ) ;
#58571=CARTESIAN_POINT ( 'NONE',  ( 0.4330708661417329575, -0.6692913385826771977, 8.415575281601705876E-17 ) ) ;
#58572=CARTESIAN_POINT ( 'NONE',  ( -0.5708661417322825615, -0.5400638737290844871, 0.3530559997133364547 ) ) ;
#58574=CARTESIAN_POINT ( 'NONE',  ( -0.9973753280839886548, -0.6046776061558809534, -0.2411417322834644161 ) ) ;
#58575=CARTESIAN_POINT ( 'NONE',  ( -0.04593175853018302557, 0.2952755905511811885, 0.1292274648535926551 ) ) ;
#58576=CARTESIAN_POINT ( 'NONE',  ( -0.1377952755905504645, -0.4536011799217368745, -0.2665933059059886201 ) ) ;
#58577=CARTESIAN_POINT ( 'NONE',  ( 1.666666666666667185, 0.05413385826771666132, 0.4176697321401328100 ) ) ;
#58578=CARTESIAN_POINT ( 'NONE',  ( 1.325459317585302665, -0.4281496062992124485, 0.4176697321401328655 ) ) ;
#58579=CARTESIAN_POINT ( 'NONE',  ( -0.3149606299212590610, -0.1870078740157479769, 0.4822834645669291653 ) ) ;
#58581=CARTESIAN_POINT ( 'NONE',  ( 1.194225721784777594, -0.4281496062992127816, -0.4176697321401328100 ) ) ;
#58584=CARTESIAN_POINT ( 'NONE',  ( 0.2887139107611556010, 0.2306618581243847221, -0.2411417322834647770 ) ) ;
#58585=CARTESIAN_POINT ( 'NONE',  ( -0.3412073490813641308, -0.5023911411419708095, 0.1820866141732285504 ) ) ;
#58586=CARTESIAN_POINT ( 'NONE',  ( 1.364829396325460076, 0.1283753931104748280, 0.1820866141732283561 ) ) ;
#58587=CARTESIAN_POINT ( 'NONE',  ( -1.614173228346457378, 0.4410134679336882302, 0.1372047244094476981 ) ) ;
#58589=CARTESIAN_POINT ( 'NONE',  ( 1.561679790026247350, -0.004921259842519870586, -0.3153832671262229437 ) ) ;
#58590=CARTESIAN_POINT ( 'NONE',  ( 1.194225721784777594, -0.4281496062992127816, -0.4176697321401328100 ) ) ;
#58592=CARTESIAN_POINT ( 'NONE',  ( 0.08530183727034192087, -0.3162353388693409650, -0.4822834645669289433 ) ) ;
#58594=CARTESIAN_POINT ( 'NONE',  ( 1.594488188976378673, 0.07958543189024085140, 0.2665933059059887866 ) ) ;
#58595=CARTESIAN_POINT ( 'NONE',  ( 5.463695987328526437E-16, -0.1870078740157479769, 0.4822834645669291653 ) ) ;
#58597=CARTESIAN_POINT ( 'NONE',  ( 1.607611548556431069, -0.6692913385826773087, -0.1292274648535924053 ) ) ;
#58598=CARTESIAN_POINT ( 'NONE',  ( 0.7217847769028878924, -0.4281496062992127816, -0.4176697321401328100 ) ) ;
#58599=CARTESIAN_POINT ( 'NONE',  ( 0.8333333333333340365, -0.5511811023622046335, 0.09757992244046803654 ) ) ;
#58600=CARTESIAN_POINT ( 'NONE',  ( -0.03280839895013062946, 0.2952755905511810219, -0.1292274648535930437 ) ) ;
#58601=CARTESIAN_POINT ( 'NONE',  ( 0.8989501312335964611, 0.1771653543307087630, 0.09757992244046791164 ) ) ;
#58602=CARTESIAN_POINT ( 'NONE',  ( -1.332020997375327642, -0.05778040916215522460, 0.4822834645669289988 ) ) ;
#58604=CARTESIAN_POINT ( 'NONE',  ( 1.325459317585302665, -0.4281496062992124485, 0.4176697321401328655 ) ) ;
#58607=CARTESIAN_POINT ( 'NONE',  ( 0.6955380577427828781, -0.4281496062992124485, 0.4176697321401328655 ) ) ;
#58609=CARTESIAN_POINT ( 'NONE',  ( -0.3812812444996365180, -2.294479370626195693E-15, 0.3464511005275217603 ) ) ;
#58610=CARTESIAN_POINT ( 'NONE',  ( 0.5249343832021003964, 0.1283753931104746893, -0.1820866141732285504 ) ) ;
#58611=CARTESIAN_POINT ( 'NONE',  ( 0.4790026246719168435, -0.3162353388693409650, -0.4822834645669289433 ) ) ;
#58612=CARTESIAN_POINT ( 'NONE',  ( 1.666666666666667185, -0.004921259842519576551, 0.3153832671262227771 ) ) ;
#58613=CARTESIAN_POINT ( 'NONE',  ( -1.017060367454067249, -0.2845877964562161244, -0.3641732283464567121 ) ) ;
#58614=CARTESIAN_POINT ( 'NONE',  ( -0.8530183727034112984, -0.4281496062992127816, -0.4176697321401328100 ) ) ;
#58615=CARTESIAN_POINT ( 'NONE',  ( -1.679790026246718693, 0.2306618581243847221, -0.2411417322834647770 ) ) ;
#58616=CARTESIAN_POINT ( 'NONE',  ( 0.9580052493438327987, -0.4281496062992127816, -0.4176697321401328100 ) ) ;
#58617=CARTESIAN_POINT ( 'NONE',  ( 1.535433070866142558, 0.2952755905511811885, 0.000000000000000000 ) ) ;
#58619=CARTESIAN_POINT ( 'NONE',  ( 0.8661417322834652488, -0.1870078740157480879, -0.4822834645669291653 ) ) ;
#58623=CARTESIAN_POINT ( 'NONE',  ( 1.581364829396326277, -0.3162353388693409650, -0.4822834645669289433 ) ) ;
#58624=CARTESIAN_POINT ( 'NONE',  ( -1.351706036745406347, -0.004921259842519870586, -0.3153832671262229437 ) ) ;
#58625=CARTESIAN_POINT ( 'NONE',  ( 1.049868766404200349, 0.1283753931104748280, 0.1820866141732283561 ) ) ;
#58626=CARTESIAN_POINT ( 'NONE',  ( -1.469816272965878357, 0.1283753931104748280, 0.1820866141732283561 ) ) ;
#58627=CARTESIAN_POINT ( 'NONE',  ( -0.5839895013123351797, -0.5511811023622046335, 0.09757992244046803654 ) ) ;
#58628=CARTESIAN_POINT ( 'NONE',  ( -1.522309711286088607, 0.1283753931104746893, -0.1820866141732285504 ) ) ;
#58629=CARTESIAN_POINT ( 'NONE',  ( 1.102362204724410155, -0.1870078740157479769, 0.3641732283464567677 ) ) ;
#58630=CARTESIAN_POINT ( 'NONE',  ( 0.4986876640419954376, -0.6046776061558809534, -0.2411417322834644161 ) ) ;
#58631=CARTESIAN_POINT ( 'NONE',  ( 1.122047244094488860, 0.1660481256975885056, 0.3530559997133364547 ) ) ;
#58632=CARTESIAN_POINT ( 'NONE',  ( -0.06561679790026180015, 0.05413385826771666132, 0.4176697321401328100 ) ) ;
#58633=CARTESIAN_POINT ( 'NONE',  ( 0.6496062992125991586, 0.07958543189024085140, 0.2665933059059887866 ) ) ;
#58634=CARTESIAN_POINT ( 'NONE',  ( 1.095800524934383846, -0.3162353388693405765, 0.4822834645669290543 ) ) ;
#58635=EDGE_CURVE ( 'NONE', #53475, #12926, #39042, .T. ) ;
#58636=CARTESIAN_POINT ( 'NONE',  ( -0.6299212598425202314, 1.968503937007873628, 0.000000000000000000 ) ) ;
#58637=CARTESIAN_POINT ( 'NONE',  ( -0.6889763779527552368, -0.5400638737290845981, -0.3530559997133363437 ) ) ;
#58640=CARTESIAN_POINT ( 'NONE',  ( 0.08530183727034192087, -0.3162353388693409650, -0.4822834645669289433 ) ) ;
#58641=CARTESIAN_POINT ( 'NONE',  ( -0.2296587926509179312, -0.05778040916215522460, 0.4822834645669289988 ) ) ;
#58642=CARTESIAN_POINT ( 'NONE',  ( 0.1377952755905518800, -0.5400638737290844871, 0.3530559997133364547 ) ) ;
#58647=EDGE_CURVE ( 'NONE', #38771, #53888, #47380, .T. ) ;
#58649=CARTESIAN_POINT ( 'NONE',  ( -1.122047244094487306, -0.4536011799217367080, 0.2665933059059888421 ) ) ;
#58651=CARTESIAN_POINT ( 'NONE',  ( -1.299212598425196097, -0.6692913385826771977, 8.415575281601705876E-17 ) ) ;
#58653=CARTESIAN_POINT ( 'NONE',  ( 0.3477690288713918276, -0.6692913385826773087, -0.1292274648535924053 ) ) ;
#58654=CARTESIAN_POINT ( 'NONE',  ( -0.3346456692913377662, -0.4536011799217367080, 0.2665933059059888421 ) ) ;
#58655=CARTESIAN_POINT ( 'NONE',  ( 1.469816272965879911, 0.2306618581243847221, -0.2411417322834647770 ) ) ;
#58656=CARTESIAN_POINT ( 'NONE',  ( 0.4527559055118117182, -0.5400638737290844871, 0.3530559997133364547 ) ) ;
#58658=VECTOR ( 'NONE', #16702, 39.37007874015748143 ) ;
#58661=CARTESIAN_POINT ( 'NONE',  ( 1.062992125984252745, 0.2952755905511811885, 0.000000000000000000 ) ) ;
#58663=CARTESIAN_POINT ( 'NONE',  ( 0.4921259842519691285, 0.1660481256975885056, 0.3530559997133364547 ) ) ;
#58664=CARTESIAN_POINT ( 'NONE',  ( 0.1312335958005255154, -0.6046776061558807314, 0.2411417322834647770 ) ) ;
#58665=CARTESIAN_POINT ( 'NONE',  ( 1.391076115485564868, 0.2306618581243847221, -0.2411417322834647770 ) ) ;
#58667=CARTESIAN_POINT ( 'NONE',  ( -0.02624671916010428221, -0.6046776061558807314, 0.2411417322834647770 ) ) ;
#58668=CARTESIAN_POINT ( 'NONE',  ( 1.128608923884515169, -0.6046776061558809534, -0.2411417322834644161 ) ) ;
#58669=CARTESIAN_POINT ( 'NONE',  ( 0.2230971128608932319, -0.4281496062992124485, 0.4176697321401328655 ) ) ;
#58670=CARTESIAN_POINT ( 'NONE',  ( 0.9842519685039378130, -0.5511811023622047445, 6.969142054262312111E-17 ) ) ;
#58671=CARTESIAN_POINT ( 'NONE',  ( -0.9120734908136475250, 0.2952755905511811885, 0.1292274648535926551 ) ) ;
#58672=CARTESIAN_POINT ( 'NONE',  ( -1.227034120734907585, 0.2952755905511811885, 0.1292274648535926551 ) ) ;
#58673=CARTESIAN_POINT ( 'NONE',  ( 0.7874015748031503170, -0.1870078740157479769, 0.4822834645669291653 ) ) ;
#58676=ORIENTED_EDGE ( 'NONE', *, *, #81439, .F. ) ;
#58678=ORIENTED_EDGE ( 'NONE', *, *, #56444, .T. ) ;
#58679=CARTESIAN_POINT ( 'NONE',  ( 1.423884514435696413, -0.3162353388693409650, -0.4822834645669289433 ) ) ;
#58680=CARTESIAN_POINT ( 'NONE',  ( 0.8530183727034126306, -0.004921259842519870586, -0.3153832671262229437 ) ) ;
#58682=CARTESIAN_POINT ( 'NONE',  ( -0.09186351706036689768, 0.05413385826771626580, -0.4176697321401330321 ) ) ;
#58683=CARTESIAN_POINT ( 'NONE',  ( -1.363814626685859288, 0.1354692512615922884, -0.3875633260700434568 ) ) ;
#58685=CARTESIAN_POINT ( 'NONE',  ( -1.305774278215222184, 0.1771653543307087630, 0.09757992244046791164 ) ) ;
#58686=CARTESIAN_POINT ( 'NONE',  ( -1.502624671916009680, -0.08942795157528024563, -0.3641732283464568787 ) ) ;
#58688=CARTESIAN_POINT ( 'NONE',  ( -0.4330708661417315697, 0.2952755905511811885, 0.000000000000000000 ) ) ;
#58689=CARTESIAN_POINT ( 'NONE',  ( 1.082677165354331228, -0.5400638737290844871, 0.3530559997133364547 ) ) ;
#58691=CARTESIAN_POINT ( 'NONE',  ( -1.515748031496062076, 0.1660481256975883668, -0.3530559997133364547 ) ) ;
#58692=CARTESIAN_POINT ( 'NONE',  ( 0.5288531115723354992, 1.522331584275770089, 0.5046369196612368047 ) ) ;
#58696=CARTESIAN_POINT ( 'NONE',  ( -0.8136482939632537770, 0.1283753931104746893, -0.1820866141732285504 ) ) ;
#58697=CARTESIAN_POINT ( 'NONE',  ( -1.522309711286088607, -0.6046776061558807314, 0.2411417322834647770 ) ) ;
#58698=CARTESIAN_POINT ( 'NONE',  ( 0.5052493438320218022, -0.6692913385826773087, -0.1292274648535924053 ) ) ;
#58699=VERTEX_POINT ( 'NONE', #35595 ) ;
#58700=CARTESIAN_POINT ( 'NONE',  ( -0.7478466213799872531, 2.204724409448818978, 0.5309055118110236338 ) ) ;
#58702=CARTESIAN_POINT ( 'NONE',  ( 1.358267716535433323, 0.1660481256975885056, 0.3530559997133364547 ) ) ;
#58703=CARTESIAN_POINT ( 'NONE',  ( -1.692913385826770645, 0.2952755905511811885, 0.000000000000000000 ) ) ;
#58705=CARTESIAN_POINT ( 'NONE',  ( -0.9580052493438311334, -0.3690944881889763329, 0.3153832671262228327 ) ) ;
#58707=CARTESIAN_POINT ( 'NONE',  ( -1.423884514435694859, -0.08942795157528024563, -0.3641732283464568787 ) ) ;
#58709=CARTESIAN_POINT ( 'NONE',  ( 0.3543307086614179147, 0.2952755905511811885, 0.000000000000000000 ) ) ;
#58710=CARTESIAN_POINT ( 'NONE',  ( -0.7283464566929126471, -0.4536011799217367080, 0.2665933059059888421 ) ) ;
#58711=CARTESIAN_POINT ( 'NONE',  ( 0.1443569553805781891, -0.3690944881889763329, 0.3153832671262228327 ) ) ;
#58712=CARTESIAN_POINT ( 'NONE',  ( 0.2165354330708668673, 0.1660481256975883668, -0.3530559997133364547 ) ) ;
#58713=CARTESIAN_POINT ( 'NONE',  ( -1.253280839895012377, -0.2845877964562161244, -0.3641732283464567121 ) ) ;
#58715=CARTESIAN_POINT ( 'NONE',  ( 0.7152230971128614723, -0.3162353388693409650, -0.4822834645669289433 ) ) ;
#58716=AXIS2_PLACEMENT_3D ( 'NONE', #70969, #52841, #71807 ) ;
#58718=CARTESIAN_POINT ( 'NONE',  ( -1.548556430446193399, -0.6046776061558809534, -0.2411417322834644161 ) ) ;
#58721=CARTESIAN_POINT ( 'NONE',  ( -0.7939632545931754048, -0.3162353388693405765, 0.4822834645669290543 ) ) ;
#58722=CARTESIAN_POINT ( 'NONE',  ( -0.3477690288713905509, -0.5511811023622046335, 0.09757992244046803654 ) ) ;
#58723=CARTESIAN_POINT ( 'NONE',  ( -0.8070866141732276899, 0.1660481256975883668, -0.3530559997133364547 ) ) ;
#58724=CARTESIAN_POINT ( 'NONE',  ( 0.9973753280839902091, -0.5023911411419708095, 0.1820866141732285504 ) ) ;
#58725=CARTESIAN_POINT ( 'NONE',  ( -0.4133858267716528645, 0.07958543189024071263, -0.2665933059059888421 ) ) ;
#58726=CARTESIAN_POINT ( 'NONE',  ( -0.6758530183727028406, -0.6692913385826773087, -0.1292274648535924053 ) ) ;
#58727=CARTESIAN_POINT ( 'NONE',  ( -1.043307086614172707, 0.1660481256975883668, -0.3530559997133364547 ) ) ;
#58728=CARTESIAN_POINT ( 'NONE',  ( 1.673228346456693494, 0.1660481256975885056, 0.3530559997133364547 ) ) ;
#58730=CARTESIAN_POINT ( 'NONE',  ( 1.430446194225722500, -0.3690944881889765550, -0.3153832671262227771 ) ) ;
#58732=CARTESIAN_POINT ( 'NONE',  ( 0.2559055118110243332, 0.1660481256975885056, 0.3530559997133364547 ) ) ;
#58733=CARTESIAN_POINT ( 'NONE',  ( 1.220472440944882164, 0.2066929133858268208, 4.479895975645240118E-15 ) ) ;
#58734=CARTESIAN_POINT ( 'NONE',  ( -1.660104986876639543, -0.05778040916215560624, -0.4822834645669293319 ) ) ;
#58735=VERTEX_POINT ( 'NONE', #72653 ) ;
#58737=CARTESIAN_POINT ( 'NONE',  ( -1.069553805774277722, -0.5511811023622048555, -0.09757992244046775898 ) ) ;
#58738=CARTESIAN_POINT ( 'NONE',  ( 0.7611548556430451917, -0.6046776061558807314, 0.2411417322834647770 ) ) ;
#58739=CARTESIAN_POINT ( 'NONE',  ( -1.102362204724408601, -0.1870078740157479769, 0.3641732283464567677 ) ) ;
#58741=CARTESIAN_POINT ( 'NONE',  ( -1.128608923884513837, -0.6046776061558807314, 0.2411417322834647770 ) ) ;
#58742=CARTESIAN_POINT ( 'NONE',  ( 0.7939632545931766261, -0.3162353388693409650, -0.4822834645669289433 ) ) ;
#58743=CARTESIAN_POINT ( 'NONE',  ( 0.4527559055118117182, 0.1660481256975883668, -0.3530559997133364547 ) ) ;
#58744=CARTESIAN_POINT ( 'NONE',  ( 1.279527559055118724, 0.1660481256975885056, 0.3530559997133364547 ) ) ;
#58745=CARTESIAN_POINT ( 'NONE',  ( -1.489501312335957062, -0.2845877964562161244, -0.3641732283464567121 ) ) ;
#58750=CARTESIAN_POINT ( 'NONE',  ( 0.9251968503937015864, 0.07958543189024071263, -0.2665933059059888421 ) ) ;
#58751=CARTESIAN_POINT ( 'NONE',  ( 0.4658792650918640033, -0.2845877964562159024, 0.3641732283464567677 ) ) ;
#58752=CARTESIAN_POINT ( 'NONE',  ( 0.006561679790026889343, -0.05778040916215522460, 0.4822834645669289988 ) ) ;
#58753=CARTESIAN_POINT ( 'NONE',  ( 1.292650918635171564, 0.2952755905511811885, 0.1292274648535926551 ) ) ;
#58755=CARTESIAN_POINT ( 'NONE',  ( 0.2230971128608932319, -0.3690944881889763329, 0.3153832671262228327 ) ) ;
#58756=CARTESIAN_POINT ( 'NONE',  ( -0.8398950131233585692, 0.2306618581243848609, 0.2411417322834645549 ) ) ;
#58757=CARTESIAN_POINT ( 'NONE',  ( 1.417322834645670104, -0.1870078740157479769, 0.4822834645669291653 ) ) ;
#58758=CARTESIAN_POINT ( 'NONE',  ( 0.9120734908136490793, 0.2952755905511810774, -0.1292274648535930714 ) ) ;
#58762=ORIENTED_EDGE ( 'NONE', *, *, #29439, .T. ) ;
#58763=CARTESIAN_POINT ( 'NONE',  ( -1.443569553805773564, -0.6046776061558807314, 0.2411417322834647770 ) ) ;
#58764=CARTESIAN_POINT ( 'NONE',  ( -0.6955380577427815458, -0.004921259842519576551, 0.3153832671262227771 ) ) ;
#58765=CARTESIAN_POINT ( 'NONE',  ( -0.5774278215223089816, -0.6046776061558807314, 0.2411417322834647770 ) ) ;
#58768=CARTESIAN_POINT ( 'NONE',  ( -1.548556430446193399, -0.5023911411419708095, -0.1820866141732282451 ) ) ;
#58769=CARTESIAN_POINT ( 'NONE',  ( -1.148293963254592542, -0.6692913385826773087, -0.1292274648535924053 ) ) ;
#58770=CARTESIAN_POINT ( 'NONE',  ( 0.1312335958005255154, -0.6046776061558807314, 0.2411417322834647770 ) ) ;
#58772=CARTESIAN_POINT ( 'NONE',  ( -1.207349081364828436, -0.6046776061558807314, 0.2411417322834647770 ) ) ;
#58774=ADVANCED_FACE ( 'NONE', ( #21308 ), #40660, .F. ) ;
#58776=CARTESIAN_POINT ( 'NONE',  ( 0.4330708661417329575, -0.6692913385826771977, 8.415575281601705876E-17 ) ) ;
#58778=CARTESIAN_POINT ( 'NONE',  ( -0.6627296587926501115, 0.1771653543307087075, -0.09757992244046823083 ) ) ;
#58783=FACE_OUTER_BOUND ( 'NONE', #9994, .T. ) ;
#58785=CARTESIAN_POINT ( 'NONE',  ( -1.187664041994750175, -0.05778040916215560624, -0.4822834645669293319 ) ) ;
#58786=CARTESIAN_POINT ( 'NONE',  ( -1.207349081364828436, -0.6046776061558807314, 0.2411417322834647770 ) ) ;
#58788=CARTESIAN_POINT ( 'NONE',  ( -1.017060367454067249, -0.3162353388693409650, -0.4822834645669289433 ) ) ;
#58789=CARTESIAN_POINT ( 'NONE',  ( -1.174540682414697335, -0.3162353388693409650, -0.4822834645669289433 ) ) ;
#58790=CARTESIAN_POINT ( 'NONE',  ( -1.259842519685038686, -0.1870078740157480879, -0.4822834645669291653 ) ) ;
#58793=CARTESIAN_POINT ( 'NONE',  ( 0.1443569553805781891, -0.004921259842519870586, -0.3153832671262229437 ) ) ;
#58794=CARTESIAN_POINT ( 'NONE',  ( -2.795275590551184575, 0.7874015748031495399, -3.317813449798768424E-16 ) ) ;
#58796=CARTESIAN_POINT ( 'NONE',  ( -0.4790026246719154557, -0.2845877964562159024, 0.3641732283464567677 ) ) ;
#58797=CARTESIAN_POINT ( 'NONE',  ( -0.8136482939632537770, 0.2306618581243847221, -0.2411417322834647770 ) ) ;
#58798=CARTESIAN_POINT ( 'NONE',  ( 0.8989501312335963501, -0.6692913385826773087, -0.1292274648535924053 ) ) ;
#58799=CARTESIAN_POINT ( 'NONE',  ( -0.5446194225721777693, -0.05778040916215522460, 0.4822834645669289988 ) ) ;
#58803=CARTESIAN_POINT ( 'NONE',  ( -0.9908136482939626788, 0.2952755905511811885, 0.1292274648535926551 ) ) ;
#58804=CARTESIAN_POINT ( 'NONE',  ( 1.089238845144357537, -0.4281496062992124485, 0.4176697321401328655 ) ) ;
#58805=CARTESIAN_POINT ( 'NONE',  ( -1.489501312335957062, -0.2845877964562161244, -0.3641732283464567121 ) ) ;
#58812=CARTESIAN_POINT ( 'NONE',  ( -0.2230971128608915943, 0.05413385826771666132, 0.4176697321401328100 ) ) ;
#58813=CARTESIAN_POINT ( 'NONE',  ( -1.312335958005248715, 0.1283753931104748280, 0.1820866141732283561 ) ) ;
#58814=CARTESIAN_POINT ( 'NONE',  ( -0.7217847769028863381, 0.05413385826771626580, -0.4176697321401330321 ) ) ;
#58816=CARTESIAN_POINT ( 'NONE',  ( -1.122047244094487306, -0.5400638737290844871, 0.3530559997133364547 ) ) ;
#58818=CARTESIAN_POINT ( 'NONE',  ( -0.8595800524934373854, -0.3162353388693409650, -0.4822834645669289433 ) ) ;
#58819=CARTESIAN_POINT ( 'NONE',  ( -0.1837270341207343505, -0.6046776061558807314, 0.2411417322834647770 ) ) ;
#58821=CARTESIAN_POINT ( 'NONE',  ( 0.8136482939632553313, 0.1283753931104748280, 0.1820866141732283561 ) ) ;
#58823=CARTESIAN_POINT ( 'NONE',  ( 0.9514435695538062676, -0.2845877964562161244, -0.3641732283464567121 ) ) ;
#58824=CARTESIAN_POINT ( 'NONE',  ( 1.437007874015748810, 0.07958543189024085140, 0.2665933059059887866 ) ) ;
#58825=CARTESIAN_POINT ( 'NONE',  ( 1.332020997375328974, -0.05778040916215560624, -0.4822834645669293319 ) ) ;
#58826=CARTESIAN_POINT ( 'NONE',  ( 0.3280839895013130669, -0.3690944881889765550, -0.3153832671262227771 ) ) ;
#58828=CARTESIAN_POINT ( 'NONE',  ( -1.410761154855641575, -0.3162353388693409650, -0.4822834645669289433 ) ) ;
#58829=CARTESIAN_POINT ( 'NONE',  ( 1.443569553805774897, 0.2306618581243848609, 0.2411417322834645549 ) ) ;
#58831=CARTESIAN_POINT ( 'NONE',  ( -0.6955380577427815458, -0.004921259842519576551, 0.3153832671262227771 ) ) ;
#58832=CARTESIAN_POINT ( 'NONE',  ( -0.4330708661417315697, 0.2952755905511811885, 0.000000000000000000 ) ) ;
#58833=CARTESIAN_POINT ( 'NONE',  ( 0.4658792650918641698, -0.05778040916215560624, -0.4822834645669293319 ) ) ;
#58835=CARTESIAN_POINT ( 'NONE',  ( 0.7480314960629927956, -0.5511811023622047445, 6.969142054262312111E-17 ) ) ;
#58836=CARTESIAN_POINT ( 'NONE',  ( -0.04593175853018302557, -0.5511811023622048555, -0.09757992244046775898 ) ) ;
#58837=CARTESIAN_POINT ( 'NONE',  ( -0.4133858267716528645, -0.5400638737290844871, 0.3530559997133364547 ) ) ;
#58838=CARTESIAN_POINT ( 'NONE',  ( -1.200787401574802349, 0.1660481256975883668, -0.3530559997133364547 ) ) ;
#58839=CARTESIAN_POINT ( 'NONE',  ( -0.8595800524934373854, -0.08942795157527998196, 0.3641732283464567121 ) ) ;
#58840=DIRECTION ( 'NONE',  ( 0.000000000000000000, -1.000000000000000000, 0.000000000000000000 ) ) ;
#58841=CARTESIAN_POINT ( 'NONE',  ( 0.7480314960629927956, 0.2952755905511811885, 0.000000000000000000 ) ) ;
#58842=CARTESIAN_POINT ( 'NONE',  ( -0.9448818897637790704, -0.1870078740157480879, -0.4822834645669291653 ) ) ;
#58845=CARTESIAN_POINT ( 'NONE',  ( 0.2624671916010504757, -0.5023911411419708095, -0.1820866141732282451 ) ) ;
#58846=CARTESIAN_POINT ( 'NONE',  ( -0.8858267716535425107, -0.5400638737290844871, 0.3530559997133364547 ) ) ;
#58847=CONICAL_SURFACE ( 'NONE', #41369, 1.220472440944881942, 0.7853981633974621568 ) ;
#58848=CARTESIAN_POINT ( 'NONE',  ( -1.102362204724408601, -0.1870078740157480879, -0.4822834645669291653 ) ) ;
#58849=CARTESIAN_POINT ( 'NONE',  ( -1.312335958005248715, 0.1283753931104748280, 0.1820866141732283561 ) ) ;
#58851=CARTESIAN_POINT ( 'NONE',  ( -0.7283464566929126471, -0.4536011799217367080, 0.2665933059059888421 ) ) ;
#58853=CARTESIAN_POINT ( 'NONE',  ( 1.220472440944882386, -0.6692913385826771977, 8.415575281601705876E-17 ) ) ;
#58858=CARTESIAN_POINT ( 'NONE',  ( -1.587926509186350810, -0.4281496062992124485, 0.4176697321401328655 ) ) ;
#58859=CARTESIAN_POINT ( 'NONE',  ( -1.371391076115484831, 0.2952755905511810774, -0.1292274648535930714 ) ) ;
#58861=CARTESIAN_POINT ( 'NONE',  ( 1.404199475065617264, -0.4281496062992124485, 0.4176697321401328655 ) ) ;
#58864=CARTESIAN_POINT ( 'NONE',  ( 0.4330708661417329575, 0.2952755905511811885, 0.000000000000000000 ) ) ;
#58865=CARTESIAN_POINT ( 'NONE',  ( -0.3018372703412066094, -0.4281496062992127816, -0.4176697321401328100 ) ) ;
#58867=CARTESIAN_POINT ( 'NONE',  ( 0.06724401132815006898, 1.722984403643211298E-16, -0.3791483426435174331 ) ) ;
#58868=CARTESIAN_POINT ( 'NONE',  ( 0.7283464566929140904, -0.4536011799217368745, -0.2665933059059886201 ) ) ;
#58870=EDGE_LOOP ( 'NONE', ( #6821, #23576, #3734, #44060 ) ) ;
#58873=CARTESIAN_POINT ( 'NONE',  ( 0.1902887139107617975, 0.2952755905511811885, 0.1292274648535926551 ) ) ;
#58874=CARTESIAN_POINT ( 'NONE',  ( 1.482939632545932307, 0.05413385826771626580, -0.4176697321401330321 ) ) ;
#58875=CARTESIAN_POINT ( 'NONE',  ( 0.01968503937007957949, -0.5400638737290845981, -0.3530559997133363437 ) ) ;
#58876=CARTESIAN_POINT ( 'NONE',  ( 1.371391076115485941, 0.2952755905511811885, 0.1292274648535926551 ) ) ;
#58877=CARTESIAN_POINT ( 'NONE',  ( -0.4002624671916004129, -0.3162353388693405765, 0.4822834645669290543 ) ) ;
#58878=CARTESIAN_POINT ( 'NONE',  ( -0.03280839895013062252, -0.6692913385826771977, 0.1292274648535927661 ) ) ;
#58879=CARTESIAN_POINT ( 'NONE',  ( -1.653543307086613234, -0.1870078740157479769, 0.4822834645669291653 ) ) ;
#58880=CARTESIAN_POINT ( 'NONE',  ( 1.358267716535433323, -0.5400638737290845981, -0.3530559997133363437 ) ) ;
#58881=CARTESIAN_POINT ( 'NONE',  ( 1.069553805774278832, 0.2952755905511810774, -0.1292274648535930714 ) ) ;
#58883=CARTESIAN_POINT ( 'NONE',  ( 0.3937007874015754361, -0.1870078740157479769, 0.3641732283464567677 ) ) ;
#58887=CARTESIAN_POINT ( 'NONE',  ( -0.3543307086614165824, -0.5511811023622047445, 6.969142054262312111E-17 ) ) ;
#58888=CARTESIAN_POINT ( 'NONE',  ( -0.02624671916010428221, 0.2306618581243847221, -0.2411417322834647770 ) ) ;
#58889=CARTESIAN_POINT ( 'NONE',  ( 1.586052503253845281, 0.4724409448818907564, -0.1653254495020589354 ) ) ;
#58890=CARTESIAN_POINT ( 'NONE',  ( 0.2427821522309716595, -0.3162353388693409650, -0.4822834645669289433 ) ) ;
#58891=CARTESIAN_POINT ( 'NONE',  ( 0.04593175853018440641, 0.2952755905511810774, -0.1292274648535930714 ) ) ;
#58892=CARTESIAN_POINT ( 'NONE',  ( -0.7742782152230962556, -0.4281496062992127816, -0.4176697321401328100 ) ) ;
#58893=CARTESIAN_POINT ( 'NONE',  ( -0.8136482939632537770, -0.6046776061558807314, 0.2411417322834647770 ) ) ;
#58894=CARTESIAN_POINT ( 'NONE',  ( 1.312335958005250269, -0.5023911411419708095, 0.1820866141732285504 ) ) ;
#58895=CARTESIAN_POINT ( 'NONE',  ( -1.548556430446193399, -0.6046776061558809534, -0.2411417322834644161 ) ) ;
#58896=CARTESIAN_POINT ( 'NONE',  ( -0.3025410870193214197, 0.000000000000000000, 0.3464511005275205946 ) ) ;
#58897=CARTESIAN_POINT ( 'NONE',  ( 0.7939632545931766261, -0.08942795157527998196, 0.3641732283464567121 ) ) ;
#58898=CARTESIAN_POINT ( 'NONE',  ( 0.5052493438320218022, -0.6692913385826773087, -0.1292274648535924053 ) ) ;
#58899=CARTESIAN_POINT ( 'NONE',  ( 0.7611548556430454138, 0.2306618581243847221, -0.2411417322834647770 ) ) ;
#58904=CARTESIAN_POINT ( 'NONE',  ( -0.5249343832020990641, -0.6046776061558809534, -0.2411417322834644161 ) ) ;
#58907=CARTESIAN_POINT ( 'NONE',  ( -1.167979002624671470, -0.004921259842519576551, 0.3153832671262227771 ) ) ;
#58908=CARTESIAN_POINT ( 'NONE',  ( 1.266404199475066328, -0.05778040916215522460, 0.4822834645669289988 ) ) ;
#58909=CONICAL_SURFACE ( 'NONE', #76394, 1.220472440944881942, 0.7853981633974621568 ) ;
#58910=CARTESIAN_POINT ( 'NONE',  ( 0.8595800524934390507, -0.3162353388693405765, 0.4822834645669290543 ) ) ;
#58911=CARTESIAN_POINT ( 'NONE',  ( -0.3674540682414689785, 0.1283753931104748280, 0.1820866141732283561 ) ) ;
#58912=CARTESIAN_POINT ( 'NONE',  ( 0.5380577427821529035, 0.05413385826771626580, -0.4176697321401330321 ) ) ;
#58914=CARTESIAN_POINT ( 'NONE',  ( 0.1968503937007881344, -0.5511811023622047445, 6.969142054262312111E-17 ) ) ;
#58915=CARTESIAN_POINT ( 'NONE',  ( -0.07217847769028813698, -0.3162353388693409650, -0.4822834645669289433 ) ) ;
#58917=CARTESIAN_POINT ( 'NONE',  ( -1.089238845144356427, 0.05413385826771666132, 0.4176697321401328100 ) ) ;
#58918=CARTESIAN_POINT ( 'NONE',  ( 0.5839895013123367340, -0.5511811023622048555, -0.09757992244046775898 ) ) ;
#58920=CARTESIAN_POINT ( 'NONE',  ( -0.8070866141732276899, -0.5400638737290844871, 0.3530559997133364547 ) ) ;
#58921=CARTESIAN_POINT ( 'NONE',  ( -0.4461942257217840213, -0.5023911411419708095, -0.1820866141732282451 ) ) ;
#58923=CARTESIAN_POINT ( 'NONE',  ( -0.7020997375328076329, -0.3162353388693409650, -0.4822834645669289433 ) ) ;
#58924=CARTESIAN_POINT ( 'NONE',  ( -0.7874015748031489847, -0.1870078740157480879, -0.4822834645669291653 ) ) ;
#58925=CARTESIAN_POINT ( 'NONE',  ( -0.1771653543307080136, 0.1660481256975883668, -0.3530559997133364547 ) ) ;
#58928=CARTESIAN_POINT ( 'NONE',  ( -1.555118110236219930, 0.07958543189024085140, 0.2665933059059887866 ) ) ;
#58929=CARTESIAN_POINT ( 'NONE',  ( 0.9186351706036752773, 0.1283753931104746893, -0.1820866141732285504 ) ) ;
#58930=CARTESIAN_POINT ( 'NONE',  ( 1.456692913385827515, 0.2952755905511811885, 0.000000000000000000 ) ) ;
#58931=CARTESIAN_POINT ( 'NONE',  ( -0.8923884514435688198, 0.1283753931104746893, -0.1820866141732285504 ) ) ;
#58933=CARTESIAN_POINT ( 'NONE',  ( -0.9842519685039365918, -0.5511811023622047445, 6.969142054262312111E-17 ) ) ;
#58934=CARTESIAN_POINT ( 'NONE',  ( -0.7414698162729651543, -0.6692913385826771977, 0.1292274648535927661 ) ) ;
#58935=CARTESIAN_POINT ( 'NONE',  ( -0.1968503937007867743, -0.6692913385826771977, 8.415575281601705876E-17 ) ) ;
#58936=CARTESIAN_POINT ( 'NONE',  ( 0.6824146981627303710, -0.5023911411419708095, 0.1820866141732285504 ) ) ;
#58938=CARTESIAN_POINT ( 'NONE',  ( 1.220472440944882386, -0.5511811023622047445, 6.969142054262312111E-17 ) ) ;
#58940=CARTESIAN_POINT ( 'NONE',  ( 0.3608923884514443348, -0.6692913385826771977, 0.1292274648535927661 ) ) ;
#58942=CARTESIAN_POINT ( 'NONE',  ( -0.7874015748031489847, -0.1870078740157479769, 0.4822834645669291653 ) ) ;
#58944=CARTESIAN_POINT ( 'NONE',  ( 1.272965879265092637, -0.004921259842519576551, 0.3153832671262227771 ) ) ;
#58945=CARTESIAN_POINT ( 'NONE',  ( 0.3477690288713918276, -0.6692913385826773087, -0.1292274648535924053 ) ) ;
#58946=CARTESIAN_POINT ( 'NONE',  ( 0.02624671916010564918, -0.6046776061558809534, -0.2411417322834644161 ) ) ;
#58947=CARTESIAN_POINT ( 'NONE',  ( 0.1246719160104994284, 0.1771653543307087075, -0.09757992244046823083 ) ) ;
#58949=CARTESIAN_POINT ( 'NONE',  ( 0.05905511811023709395, -0.4536011799217367080, 0.2665933059059888421 ) ) ;
#58950=CARTESIAN_POINT ( 'NONE',  ( 0.9711286089238851948, -0.6046776061558809534, -0.2411417322834644161 ) ) ;
#58951=CARTESIAN_POINT ( 'NONE',  ( -0.7545931758530177724, 0.1771653543307087630, 0.09757992244046791164 ) ) ;
#58952=CARTESIAN_POINT ( 'NONE',  ( -0.5774278215223089816, -0.6046776061558807314, 0.2411417322834647770 ) ) ;
#58953=CARTESIAN_POINT ( 'NONE',  ( 0.1706036745406830368, 0.009842519685039463617, 0.3409548833797002576 ) ) ;
#58954=ORIENTED_EDGE ( 'NONE', *, *, #43837, .T. ) ;
#58955=CARTESIAN_POINT ( 'NONE',  ( -1.089238845144356427, -0.4281496062992127816, -0.4176697321401328100 ) ) ;
#58956=CARTESIAN_POINT ( 'NONE',  ( -1.056430446194224881, 0.1771653543307087075, -0.09757992244046823083 ) ) ;
#58957=CARTESIAN_POINT ( 'NONE',  ( 0.07874015748031558404, -0.1870078740157480879, -0.4822834645669291653 ) ) ;
#58958=EDGE_CURVE ( 'NONE', #69752, #29072, #44976, .T. ) ;
#58959=CARTESIAN_POINT ( 'NONE',  ( -1.528871391076114250, 0.2952755905511810774, -0.1292274648535930714 ) ) ;
#58960=CARTESIAN_POINT ( 'NONE',  ( -0.8858267716535425107, -0.5400638737290844871, 0.3530559997133364547 ) ) ;
#58962=CARTESIAN_POINT ( 'NONE',  ( -0.9317585301837263412, 0.05413385826771666132, 0.4176697321401328100 ) ) ;
#58963=CARTESIAN_POINT ( 'NONE',  ( 0.7545931758530188826, -0.6692913385826771977, 0.1292274648535927661 ) ) ;
#58964=CARTESIAN_POINT ( 'NONE',  ( 1.397637795275591177, 0.1660481256975883668, -0.3530559997133364547 ) ) ;
#58966=CARTESIAN_POINT ( 'NONE',  ( 1.574803149606299746, -0.1870078740157479769, 0.4822834645669291653 ) ) ;
#58967=CARTESIAN_POINT ( 'NONE',  ( -1.148293963254592542, -0.6692913385826773087, -0.1292274648535924053 ) ) ;
#58970=ORIENTED_EDGE ( 'NONE', *, *, #47715, .F. ) ;
#58971=EDGE_CURVE ( 'NONE', #12926, #48838, #2838, .T. ) ;
#58972=CARTESIAN_POINT ( 'NONE',  ( -0.2559055118110227234, -0.4536011799217367080, 0.2665933059059888421 ) ) ;
#58974=ORIENTED_EDGE ( 'NONE', *, *, #45936, .T. ) ;
#58975=CARTESIAN_POINT ( 'NONE',  ( 0.3805774278215230400, 0.05413385826771626580, -0.4176697321401330321 ) ) ;
#58976=CARTESIAN_POINT ( 'NONE',  ( -0.1509186351706028884, -0.05778040916215522460, 0.4822834645669289988 ) ) ;
#58977=CARTESIAN_POINT ( 'NONE',  ( -0.5708661417322825615, -0.5400638737290844871, 0.3530559997133364547 ) ) ;
#58978=CARTESIAN_POINT ( 'NONE',  ( -1.646051170424378096, -0.1870078740157480046, 1.254653134982923898E-17 ) ) ;
#58979=CARTESIAN_POINT ( 'NONE',  ( -0.8858267716535425107, -0.4536011799217367080, 0.2665933059059888421 ) ) ;
#58980=CARTESIAN_POINT ( 'NONE',  ( 0.4935044252197983150, 1.488513638086841118, -0.5309055118110237448 ) ) ;
#58981=CARTESIAN_POINT ( 'NONE',  ( 0.9186351706036752773, 0.2306618581243847221, -0.2411417322834647770 ) ) ;
#58982=CARTESIAN_POINT ( 'NONE',  ( 0.4527559055118117182, -0.4536011799217367080, 0.2665933059059888421 ) ) ;
#58983=CARTESIAN_POINT ( 'NONE',  ( -0.4855643044619415427, 0.05413385826771626580, -0.4176697321401330321 ) ) ;
#58985=CARTESIAN_POINT ( 'NONE',  ( -0.7349081364829387342, -0.6046776061558807314, 0.2411417322834647770 ) ) ;
#58986=CARTESIAN_POINT ( 'NONE',  ( -1.561679790026246017, -0.004921259842519576551, 0.3153832671262227771 ) ) ;
#58987=CARTESIAN_POINT ( 'NONE',  ( 1.154855643044620184, -0.6046776061558807314, 0.2411417322834647770 ) ) ;
#58988=CARTESIAN_POINT ( 'NONE',  ( 1.489501312335958172, -0.2845877964562159024, 0.3641732283464567677 ) ) ;
#58989=EDGE_LOOP ( 'NONE', ( #18746, #7867, #23974, #34029, #9014, #71838 ) ) ;
#58991=CARTESIAN_POINT ( 'NONE',  ( 0.1115485564304470323, 0.2952755905511811885, 0.1292274648535926551 ) ) ;
#58993=CARTESIAN_POINT ( 'NONE',  ( -0.8858267716535425107, 0.1660481256975883668, -0.3530559997133364547 ) ) ;
#58994=CARTESIAN_POINT ( 'NONE',  ( 1.437007874015748810, 0.1660481256975885056, 0.3530559997133364547 ) ) ;
#58995=CARTESIAN_POINT ( 'NONE',  ( 1.187664041994751285, -0.3162353388693409650, -0.4822834645669289433 ) ) ;
#58996=CARTESIAN_POINT ( 'NONE',  ( 0.3149606299212603933, -0.1870078740157479769, 0.4822834645669291653 ) ) ;
#58997=CARTESIAN_POINT ( 'NONE',  ( -0.2821522309711278487, -0.6692913385826773087, -0.1292274648535924053 ) ) ;
#58999=CARTESIAN_POINT ( 'NONE',  ( -0.9908136482939626788, -0.6692913385826773087, -0.1292274648535924053 ) ) ;
#59001=CARTESIAN_POINT ( 'NONE',  ( -0.7152230971128602510, -0.3162353388693405765, 0.4822834645669290543 ) ) ;
#59002=CARTESIAN_POINT ( 'NONE',  ( 8.195543980992789655E-16, -0.1870078740157480601, -0.3641732283464567677 ) ) ;
#59003=CARTESIAN_POINT ( 'NONE',  ( -0.4624320255261038515, -2.191421614605370878E-15, 0.4445507791589071167 ) ) ;
#59004=CARTESIAN_POINT ( 'NONE',  ( -0.5446194225721777693, -0.3162353388693409650, -0.4822834645669289433 ) ) ;
#59006=CARTESIAN_POINT ( 'NONE',  ( 0.8727034120734912248, -0.3162353388693409650, -0.4822834645669289433 ) ) ;
#59008=VERTEX_POINT ( 'NONE', #56179 ) ;
#59009=CARTESIAN_POINT ( 'NONE',  ( 8.195543980992789655E-16, -0.1870078740157480879, -0.4822834645669291653 ) ) ;
#59010=CARTESIAN_POINT ( 'NONE',  ( -0.2821522309711278487, 0.1771653543307087630, 0.09757992244046791164 ) ) ;
#59011=CARTESIAN_POINT ( 'NONE',  ( 0.8858267716535438430, 0.07958543189024085140, 0.2665933059059887866 ) ) ;
#59015=CARTESIAN_POINT ( 'NONE',  ( 1.364829396325459854, -0.6046776061558809534, -0.2411417322834644161 ) ) ;
#59017=CARTESIAN_POINT ( 'NONE',  ( 5.463695987328526437E-16, -0.1870078740157479769, 0.4822834645669291653 ) ) ;
#59019=CARTESIAN_POINT ( 'NONE',  ( -1.535433070866141225, 0.2952755905511811885, 0.000000000000000000 ) ) ;
#59020=CARTESIAN_POINT ( 'NONE',  ( -0.3543307086614165824, -0.6692913385826771977, 8.415575281601705876E-17 ) ) ;
#59022=CARTESIAN_POINT ( 'NONE',  ( -1.469816272965878357, 0.1283753931104748280, 0.1820866141732283561 ) ) ;
#59023=CARTESIAN_POINT ( 'NONE',  ( 0.7152230971128614723, -0.3162353388693409650, -0.4822834645669289433 ) ) ;
#59024=CARTESIAN_POINT ( 'NONE',  ( 1.017060367454068803, -0.2845877964562159024, 0.3641732283464567677 ) ) ;
#59026=CARTESIAN_POINT ( 'NONE',  ( 0.5380577427821529035, -0.3690944881889763329, 0.3153832671262228327 ) ) ;
#59027=CARTESIAN_POINT ( 'NONE',  ( -1.286089238845143479, 0.2306618581243847221, -0.2411417322834647770 ) ) ;
#59029=CARTESIAN_POINT ( 'NONE',  ( 1.371391076115485941, 0.2952755905511811885, 0.1292274648535926551 ) ) ;
#59031=CARTESIAN_POINT ( 'NONE',  ( 0.8398950131233602345, -0.6046776061558807314, 0.2411417322834647770 ) ) ;
#59032=CARTESIAN_POINT ( 'NONE',  ( -0.7137454485294953965, 2.165354330708661124, -0.4917280318828585184 ) ) ;
#59034=CARTESIAN_POINT ( 'NONE',  ( 0.5971128608923890191, -0.5511811023622046335, 0.09757992244046803654 ) ) ;
#59035=ADVANCED_FACE ( 'NONE', ( #43540 ), #11587, .F. ) ;
#59036=CARTESIAN_POINT ( 'NONE',  ( 0.5839895013123367340, 0.2952755905511811885, 0.1292274648535926551 ) ) ;
#59038=CARTESIAN_POINT ( 'NONE',  ( -0.9317585301837263412, -0.004921259842519576551, 0.3153832671262227771 ) ) ;
#59039=CARTESIAN_POINT ( 'NONE',  ( -0.8727034120734901146, -0.05778040916215560624, -0.4822834645669293319 ) ) ;
#59040=CARTESIAN_POINT ( 'NONE',  ( -1.482939632545930975, -0.4281496062992127816, -0.4176697321401328100 ) ) ;
#59041=CARTESIAN_POINT ( 'NONE',  ( 1.115485564304462551, -0.4281496062992127816, -0.4176697321401328100 ) ) ;
#59042=CARTESIAN_POINT ( 'NONE',  ( 1.456692913385827515, -0.6692913385826771977, 8.415575281601705876E-17 ) ) ;
#59044=CARTESIAN_POINT ( 'NONE',  ( 0.5971128608923890191, -0.6692913385826771977, 0.1292274648535927661 ) ) ;
#59046=CARTESIAN_POINT ( 'NONE',  ( 1.620734908136483465, -0.6692913385826771977, 0.1292274648535927661 ) ) ;
#59047=CARTESIAN_POINT ( 'NONE',  ( 1.351706036745407680, 0.05413385826771666132, 0.4176697321401328100 ) ) ;
#59048=CARTESIAN_POINT ( 'NONE',  ( -1.515748031496062076, 0.07958543189024071263, -0.2665933059059888421 ) ) ;
#59049=CARTESIAN_POINT ( 'NONE',  ( 1.233595800524935227, 0.1283753931104746893, -0.1820866141732285504 ) ) ;
#59050=CARTESIAN_POINT ( 'NONE',  ( -1.141732283464566011, 0.1771653543307087630, 0.000000000000000000 ) ) ;
#59051=CARTESIAN_POINT ( 'NONE',  ( -0.5314960629921250401, 0.07958543189024085140, 0.2665933059059887866 ) ) ;
#59052=CARTESIAN_POINT ( 'NONE',  ( 0.4606732211678793432, 1.929133858267716439, 0.5309055118110234117 ) ) ;
#59053=CARTESIAN_POINT ( 'NONE',  ( 1.089238845144357537, -0.3690944881889763329, 0.3153832671262228327 ) ) ;
#59054=CARTESIAN_POINT ( 'NONE',  ( 0.4658792650918641698, -0.05778040916215560624, -0.4822834645669293319 ) ) ;
#59055=CARTESIAN_POINT ( 'NONE',  ( 1.233595800524935227, -0.6046776061558807314, 0.2411417322834647770 ) ) ;
#59056=CARTESIAN_POINT ( 'NONE',  ( 0.04593175853018440641, -0.6692913385826771977, 0.1292274648535927661 ) ) ;
#59057=CARTESIAN_POINT ( 'NONE',  ( 0.4593175853018379162, -0.3690944881889763329, 0.3153832671262228327 ) ) ;
#59058=CARTESIAN_POINT ( 'NONE',  ( 1.430446194225722500, 0.05413385826771666132, 0.4176697321401328100 ) ) ;
#59060=CARTESIAN_POINT ( 'NONE',  ( -0.3215223097112853146, -0.3162353388693405765, 0.4822834645669290543 ) ) ;
#59062=CARTESIAN_POINT ( 'NONE',  ( 0.03937007874015806264, 0.2066929133858268208, 0.000000000000000000 ) ) ;
#59063=CARTESIAN_POINT ( 'NONE',  ( 0.1968503937007881344, 0.2952755905511811885, 0.000000000000000000 ) ) ;
#59064=CARTESIAN_POINT ( 'NONE',  ( -0.7414698162729651543, -0.6692913385826771977, 0.1292274648535927661 ) ) ;
#59065=CARTESIAN_POINT ( 'NONE',  ( -0.1509186351706028884, -0.05778040916215522460, 0.4822834645669289988 ) ) ;
#59070=CARTESIAN_POINT ( 'NONE',  ( -1.076115485564303809, 0.1283753931104748280, 0.1820866141732283561 ) ) ;
#59072=CARTESIAN_POINT ( 'NONE',  ( -1.167979002624671470, -0.4281496062992127816, -0.4176697321401328100 ) ) ;
#59074=CARTESIAN_POINT ( 'NONE',  ( 0.4790026246719168435, -0.3162353388693409650, -0.4822834645669289433 ) ) ;
#59075=CARTESIAN_POINT ( 'NONE',  ( -0.4068241469816267775, -0.004921259842519870586, -0.3153832671262229437 ) ) ;
#59076=CARTESIAN_POINT ( 'NONE',  ( 1.384514435695538337, -0.6692913385826771977, 0.1292274648535927661 ) ) ;
#59077=CARTESIAN_POINT ( 'NONE',  ( 0.1574803149606306130, -0.1870078740157479769, 0.4822834645669291653 ) ) ;
#59081=CARTESIAN_POINT ( 'NONE',  ( 1.377952755905512472, 0.2952755905511811885, 0.000000000000000000 ) ) ;
#59082=CARTESIAN_POINT ( 'NONE',  ( 0.5446194225721792126, -0.05778040916215560624, -0.4822834645669293319 ) ) ;
#59083=CARTESIAN_POINT ( 'NONE',  ( 0.1574803149606306130, -0.1870078740157479769, 0.4822834645669291653 ) ) ;
#59084=CARTESIAN_POINT ( 'NONE',  ( 1.417322834645670104, -0.1870078740157479769, 0.4822834645669291653 ) ) ;
#59085=CARTESIAN_POINT ( 'NONE',  ( 1.003937007874016407, -0.5400638737290844871, 0.3530559997133364547 ) ) ;
#59087=CARTESIAN_POINT ( 'NONE',  ( 0.1706036745406830368, 0.05413385826771666132, 0.4176697321401328100 ) ) ;
#59088=CARTESIAN_POINT ( 'NONE',  ( 1.167979002624672580, -0.4281496062992124485, 0.4176697321401328655 ) ) ;
#59089=CARTESIAN_POINT ( 'NONE',  ( 0.3674540682414705883, -0.6046776061558807314, 0.2411417322834647770 ) ) ;
#59090=CARTESIAN_POINT ( 'NONE',  ( 1.115485564304462551, -0.3690944881889765550, -0.3153832671262227771 ) ) ;
#59091=CARTESIAN_POINT ( 'NONE',  ( -1.469816272965878357, -0.6046776061558809534, -0.2411417322834644161 ) ) ;
#59092=CARTESIAN_POINT ( 'NONE',  ( -1.469816272965878357, -0.6046776061558809534, -0.2411417322834644161 ) ) ;
#59093=CARTESIAN_POINT ( 'NONE',  ( 0.9580052493438326877, 0.05413385826771666132, 0.4176697321401328100 ) ) ;
#59100=CARTESIAN_POINT ( 'NONE',  ( 0.8070866141732288002, 0.07958543189024085140, 0.2665933059059887866 ) ) ;
#59105=CARTESIAN_POINT ( 'NONE',  ( 1.187664041994751285, -0.3162353388693409650, -0.4822834645669289433 ) ) ;
#59106=CARTESIAN_POINT ( 'NONE',  ( -1.502624671916009680, -0.3162353388693405765, 0.4822834645669290543 ) ) ;
#59107=CARTESIAN_POINT ( 'NONE',  ( -0.2099737532808391705, -0.6046776061558809534, -0.2411417322834644161 ) ) ;
#59108=CARTESIAN_POINT ( 'NONE',  ( 0.9776902887139113929, 0.2952755905511811885, 0.1292274648535926551 ) ) ;
#59110=CARTESIAN_POINT ( 'NONE',  ( -1.614173228346456268, -0.6692913385826771977, 8.415575281601705876E-17 ) ) ;
#59115=CARTESIAN_POINT ( 'NONE',  ( -1.003937007874014853, 0.07958543189024085140, 0.2665933059059887866 ) ) ;
#59117=CARTESIAN_POINT ( 'NONE',  ( 0.8923884514435701520, 0.1539470093639523085, 0.1968503937007873850 ) ) ;
#59118=CARTESIAN_POINT ( 'NONE',  ( 0.6233595800524942554, -0.05778040916215560624, -0.4822834645669293319 ) ) ;
#59119=EDGE_LOOP ( 'NONE', ( #58036, #30186, #74119, #13762 ) ) ;
#59121=CARTESIAN_POINT ( 'NONE',  ( -0.4596682205436332658, 0.004960608223778823628, 0.3437734562760190182 ) ) ;
#59122=CARTESIAN_POINT ( 'NONE',  ( 0.7020997375328090762, -0.3162353388693405765, 0.4822834645669290543 ) ) ;
#59123=CARTESIAN_POINT ( 'NONE',  ( -1.594488188976377563, -0.5400638737290844871, 0.3530559997133364547 ) ) ;
#59125=CARTESIAN_POINT ( 'NONE',  ( -0.7020997375328076329, -0.2845877964562161244, -0.3641732283464567121 ) ) ;
#59126=CARTESIAN_POINT ( 'NONE',  ( 1.660104986876641320, -0.05778040916215522460, 0.4822834645669289988 ) ) ;
#59128=CARTESIAN_POINT ( 'NONE',  ( 0.6430446194225728496, 0.05413385826771666132, 0.4176697321401328100 ) ) ;
#59129=CARTESIAN_POINT ( 'NONE',  ( -1.076115485564303809, -0.5023911411419708095, -0.1820866141732282451 ) ) ;
#59130=CARTESIAN_POINT ( 'NONE',  ( 0.1837270341207354329, 0.1283753931104748280, 0.1820866141732283561 ) ) ;
#59131=CARTESIAN_POINT ( 'NONE',  ( -0.3280839895013117347, -0.4281496062992124485, 0.4176697321401328655 ) ) ;
#59132=CARTESIAN_POINT ( 'NONE',  ( -1.010498687664041384, -0.004921259842519576551, 0.3153832671262227771 ) ) ;
#59134=CARTESIAN_POINT ( 'NONE',  ( 0.6167979002624678353, -0.4281496062992124485, 0.4176697321401328655 ) ) ;
#59136=CARTESIAN_POINT ( 'NONE',  ( -1.469816272965878357, 0.2306618581243848609, 0.2411417322834645549 ) ) ;
#59138=CARTESIAN_POINT ( 'NONE',  ( -0.7545931758530177724, 0.2952755905511811885, 0.1292274648535926551 ) ) ;
#59139=CARTESIAN_POINT ( 'NONE',  ( -0.01968503937007793844, -0.4536011799217367080, 0.2665933059059888421 ) ) ;
#59140=CARTESIAN_POINT ( 'NONE',  ( -1.220472440944881054, -0.6692913385826771977, 8.415575281601705876E-17 ) ) ;
#59141=CARTESIAN_POINT ( 'NONE',  ( 0.8727034120734913358, -0.08942795157527998196, 0.3641732283464567121 ) ) ;
#59142=CARTESIAN_POINT ( 'NONE',  ( -0.9055118110236215490, 0.1771653543307087630, 0.000000000000000000 ) ) ;
#59143=CARTESIAN_POINT ( 'NONE',  ( -1.036745406824146176, 0.05413385826771626580, -0.4176697321401330321 ) ) ;
#59144=CARTESIAN_POINT ( 'NONE',  ( -1.049868766404198794, 0.2306618581243847221, -0.2411417322834647770 ) ) ;
#59146=CARTESIAN_POINT ( 'NONE',  ( -1.430446194225720724, 0.05413385826771626580, -0.4176697321401330321 ) ) ;
#59148=CARTESIAN_POINT ( 'NONE',  ( 0.8727034120734913358, -0.08942795157527998196, 0.3641732283464567121 ) ) ;
#59149=CARTESIAN_POINT ( 'NONE',  ( 0.5446194225721792126, -0.3162353388693405765, 0.4822834645669290543 ) ) ;
#59150=CARTESIAN_POINT ( 'NONE',  ( -1.345144356955379816, -0.3162353388693405765, 0.4822834645669290543 ) ) ;
#59151=CARTESIAN_POINT ( 'NONE',  ( -1.581364829396324945, -0.3162353388693405765, 0.4822834645669290543 ) ) ;
#59152=ORIENTED_EDGE ( 'NONE', *, *, #23233, .F. ) ;
#59154=CARTESIAN_POINT ( 'NONE',  ( -1.397637795275589623, -0.4536011799217368745, -0.2665933059059886201 ) ) ;
#59155=CARTESIAN_POINT ( 'NONE',  ( 0.5446194225721792126, -0.05778040916215560624, -0.4822834645669293319 ) ) ;
#59156=CARTESIAN_POINT ( 'NONE',  ( -1.430446194225721390, -0.3690944881889763329, 0.3153832671262228327 ) ) ;
#59158=CARTESIAN_POINT ( 'NONE',  ( -1.581364829396324945, -0.3162353388693405765, 0.4822834645669290543 ) ) ;
#59159=CARTESIAN_POINT ( 'NONE',  ( 0.8070866141732289112, -0.5400638737290845981, -0.3530559997133363437 ) ) ;
#59160=CARTESIAN_POINT ( 'NONE',  ( 0.6561679790026253567, -0.6046776061558809534, -0.2411417322834644161 ) ) ;
#59161=CARTESIAN_POINT ( 'NONE',  ( 1.128608923884514947, 0.2306618581243848609, 0.2411417322834645549 ) ) ;
#59166=CARTESIAN_POINT ( 'NONE',  ( 0.1377952755905518800, -0.4536011799217367080, 0.2665933059059888421 ) ) ;
#59167=CARTESIAN_POINT ( 'NONE',  ( 0.2624671916010504757, -0.6046776061558809534, -0.2411417322834644161 ) ) ;
#59168=CARTESIAN_POINT ( 'NONE',  ( 1.227034120734908917, -0.6692913385826771977, 0.1292274648535927661 ) ) ;
#59170=CARTESIAN_POINT ( 'NONE',  ( 0.1837270341207357105, -0.5023911411419708095, -0.1820866141732282451 ) ) ;
#59171=CARTESIAN_POINT ( 'NONE',  ( -0.7611548556430438595, -0.6046776061558809534, -0.2411417322834644161 ) ) ;
#59172=CARTESIAN_POINT ( 'NONE',  ( 1.581364829396326277, -0.05778040916215522460, 0.4822834645669289988 ) ) ;
#59173=CARTESIAN_POINT ( 'NONE',  ( 0.3608923884514443348, -0.6692913385826771977, 0.1292274648535927661 ) ) ;
#59175=LINE ( 'NONE', #39826, #82880 ) ;
#59177=ORIENTED_EDGE ( 'NONE', *, *, #56716, .F. ) ;
#59178=CARTESIAN_POINT ( 'NONE',  ( -1.660104986876639543, -0.05778040916215560624, -0.4822834645669293319 ) ) ;
#59180=CARTESIAN_POINT ( 'NONE',  ( -1.253280839895012377, -0.2845877964562161244, -0.3641732283464567121 ) ) ;
#59181=CARTESIAN_POINT ( 'NONE',  ( -1.135170603674539924, 0.2952755905511810774, -0.1292274648535930714 ) ) ;
#59184=CARTESIAN_POINT ( 'NONE',  ( 1.515748031496063408, 0.1660481256975885056, 0.3530559997133364547 ) ) ;
#59185=CARTESIAN_POINT ( 'NONE',  ( -1.181102362204723644, -0.1870078740157480879, -0.4822834645669291653 ) ) ;
#59186=CARTESIAN_POINT ( 'NONE',  ( 0.4396325459317590445, -0.6692913385826771977, 0.1292274648535927661 ) ) ;
#59187=CARTESIAN_POINT ( 'NONE',  ( -1.430446194225720724, 0.05413385826771626580, -0.4176697321401330321 ) ) ;
#59189=CARTESIAN_POINT ( 'NONE',  ( 0.7020997375328090762, -0.05778040916215560624, -0.4822834645669293319 ) ) ;
#59191=CARTESIAN_POINT ( 'NONE',  ( -1.200787401574802349, -0.4536011799217367080, 0.2665933059059888421 ) ) ;
#59195=CARTESIAN_POINT ( 'NONE',  ( -1.528871391076114250, 0.1771653543307087075, -0.09757992244046823083 ) ) ;
#59196=CARTESIAN_POINT ( 'NONE',  ( -1.049868766404198794, 0.2306618581243847221, -0.2411417322834647770 ) ) ;
#59197=CARTESIAN_POINT ( 'NONE',  ( -1.102362204724408601, -0.1870078740157480879, -0.4822834645669291653 ) ) ;
#59199=CARTESIAN_POINT ( 'NONE',  ( -1.555118110236219930, 0.1660481256975885056, 0.3530559997133364547 ) ) ;
#59200=CARTESIAN_POINT ( 'NONE',  ( -1.686351706036744558, 0.2952755905511810774, -0.1292274648535930714 ) ) ;
#59201=CARTESIAN_POINT ( 'NONE',  ( -1.246719160104985846, -0.4281496062992127816, -0.4176697321401328100 ) ) ;
#59203=CARTESIAN_POINT ( 'NONE',  ( 0.1574803149606306130, -0.1870078740157480601, -0.3641732283464567677 ) ) ;
#59204=DIRECTION ( 'NONE',  ( -1.000000000000000000, -3.083952846180989294E-16, 0.000000000000000000 ) ) ;
#59206=CARTESIAN_POINT ( 'NONE',  ( -0.5249343832020990641, -0.5023911411419708095, -0.1820866141732282451 ) ) ;
#59207=CARTESIAN_POINT ( 'NONE',  ( -0.5839895013123351797, -0.6692913385826771977, 0.1292274648535927661 ) ) ;
#59208=CARTESIAN_POINT ( 'NONE',  ( 1.030183727034121421, -0.3162353388693409650, -0.4822834645669289433 ) ) ;
#59209=CARTESIAN_POINT ( 'NONE',  ( -0.8005249343832011588, 0.05413385826771626580, -0.4176697321401330321 ) ) ;
#59210=ORIENTED_EDGE ( 'NONE', *, *, #18560, .F. ) ;
#59212=CARTESIAN_POINT ( 'NONE',  ( -0.9251968503937002541, -0.5400638737290845981, -0.3530559997133363437 ) ) ;
#59213=CARTESIAN_POINT ( 'NONE',  ( 0.6955380577427828781, 0.05413385826771626580, -0.4176697321401330321 ) ) ;
#59214=CARTESIAN_POINT ( 'NONE',  ( -1.391076115485563758, 0.1283753931104748280, 0.1820866141732283561 ) ) ;
#59216=DIRECTION ( 'NONE',  ( -3.096699300667737957E-16, 1.000000000000000000, -0.000000000000000000 ) ) ;
#59220=CARTESIAN_POINT ( 'NONE',  ( -0.1181102362204717315, -0.6692913385826771977, 8.415575281601705876E-17 ) ) ;
#59221=CARTESIAN_POINT ( 'NONE',  ( -1.358267716535432434, -0.4536011799217367080, 0.2665933059059888421 ) ) ;
#59223=CARTESIAN_POINT ( 'NONE',  ( -1.476377952755905110, -0.5400638737290845981, -0.3530559997133363437 ) ) ;
#59225=CARTESIAN_POINT ( 'NONE',  ( -1.450131233595799651, -0.6692913385826771977, 0.1292274648535927661 ) ) ;
#59226=CARTESIAN_POINT ( 'NONE',  ( -0.4724409448818890911, -0.1870078740157479769, 0.4822834645669291653 ) ) ;
#59228=CARTESIAN_POINT ( 'NONE',  ( 0.2493438320209980519, -0.3690944881889765550, -0.3153832671262227771 ) ) ;
#59230=CARTESIAN_POINT ( 'NONE',  ( 0.2362204724409456558, -0.1870078740157479769, 0.3641732283464567677 ) ) ;
#59231=CARTESIAN_POINT ( 'NONE',  ( 1.167979002624672580, -0.004921259842519870586, -0.3153832671262229437 ) ) ;
#59232=CARTESIAN_POINT ( 'NONE',  ( 0.7808398950131240079, -0.3162353388693405765, 0.4822834645669290543 ) ) ;
#59233=CARTESIAN_POINT ( 'NONE',  ( 0.2099737532808405305, -0.5023911411419708095, 0.1820866141732285504 ) ) ;
#59235=CARTESIAN_POINT ( 'NONE',  ( -1.469816272965878357, 0.2306618581243848609, 0.2411417322834645549 ) ) ;
#59236=CARTESIAN_POINT ( 'NONE',  ( 0.02624671916010564918, 0.1283753931104748280, 0.1820866141732283561 ) ) ;
#59237=( BOUNDED_CURVE ( )  B_SPLINE_CURVE ( 2, ( #55884, #49577, #31042, #57117, #5381, #44079, #43247, #68945, #4975, #62631, #37372, #24728, #12116 ),
 .UNSPECIFIED., .F., .F. ) 
 B_SPLINE_CURVE_WITH_KNOTS ( ( 3, 2, 2, 2, 2, 2, 3 ),
 ( 0.7194878114796872115, 0.7196969696969697239, 0.7234848484848485084, 0.7272727272727272929, 0.7310606060606060774, 0.7348484848484848619, 0.7350576430657673743 ),
 .UNSPECIFIED. ) 
 CURVE ( )  GEOMETRIC_REPRESENTATION_ITEM ( )  RATIONAL_B_SPLINE_CURVE ( ( 0.9964447847208419695, 0.9981185001348091834, 1.000000000000000000, 0.9659258262890683122, 1.000000000000000000, 0.9659258262890683122, 1.000000000000000000, 0.9659258262890683122, 1.000000000000000000, 0.9659258262890683122, 1.000000000000000000, 0.9981185001348091834, 0.9964447847208420805 ) ) 
 REPRESENTATION_ITEM ( '' )  );
#59238=DIRECTION ( 'NONE',  ( -0.000000000000000000, -1.000000000000000000, -0.000000000000000000 ) ) ;
#59239=CARTESIAN_POINT ( 'NONE',  ( -0.3280839895013117347, -0.004921259842519870586, -0.3153832671262229437 ) ) ;
#59241=CARTESIAN_POINT ( 'NONE',  ( 0.07874015748031558404, -0.1870078740157479769, 0.4822834645669291653 ) ) ;
#59243=CARTESIAN_POINT ( 'NONE',  ( 1.154855643044620184, 0.1283753931104746893, -0.1820866141732285504 ) ) ;
#59244=CARTESIAN_POINT ( 'NONE',  ( -0.2952755905511804668, 0.07958543189024085140, 0.2665933059059887866 ) ) ;
#59245=CARTESIAN_POINT ( 'NONE',  ( -0.3608923884514428360, 0.2952755905511811885, 0.1292274648535926551 ) ) ;
#59246=CARTESIAN_POINT ( 'NONE',  ( -1.666666666666665853, 0.05413385826771626580, -0.4176697321401330321 ) ) ;
#59247=CARTESIAN_POINT ( 'NONE',  ( -1.299212598425196097, 0.1771653543307087630, 0.000000000000000000 ) ) ;
#59248=CARTESIAN_POINT ( 'NONE',  ( -2.795275590551181910, 1.850393700787402729, -6.635626899597537341E-17 ) ) ;
#59250=CARTESIAN_POINT ( 'NONE',  ( 0.7020997375328090762, -0.3162353388693405765, 0.4822834645669290543 ) ) ;
#59251=VECTOR ( 'NONE', #25128, 39.37007874015748143 ) ;
#59252=CARTESIAN_POINT ( 'NONE',  ( -0.8070866141732276899, 0.1660481256975883668, -0.3530559997133364547 ) ) ;
#59255=CARTESIAN_POINT ( 'NONE',  ( 0.3543307086614179147, 0.1771653543307087630, 0.000000000000000000 ) ) ;
#59256=CARTESIAN_POINT ( 'NONE',  ( -0.9776902887139098386, 0.2952755905511810774, -0.1292274648535930714 ) ) ;
#59257=CARTESIAN_POINT ( 'NONE',  ( -1.259842519685038686, -0.1870078740157480879, -0.4822834645669291653 ) ) ;
#59258=CARTESIAN_POINT ( 'NONE',  ( -1.437007874015747477, 0.07958543189024071263, -0.2665933059059888421 ) ) ;
#59260=CARTESIAN_POINT ( 'NONE',  ( -0.7086614173228339419, -0.1870078740157479769, 0.3641732283464567677 ) ) ;
#59262=CARTESIAN_POINT ( 'NONE',  ( 0.6824146981627303710, 0.2306618581243847221, -0.2411417322834647770 ) ) ;
#59266=CARTESIAN_POINT ( 'NONE',  ( -1.633858267716534529, -0.5400638737290845981, -0.3530559997133363437 ) ) ;
#59267=CARTESIAN_POINT ( 'NONE',  ( -1.194225721784776262, 0.05413385826771626580, -0.4176697321401330321 ) ) ;
#59268=CARTESIAN_POINT ( 'NONE',  ( 1.115485564304462551, 0.05413385826771666132, 0.4176697321401328100 ) ) ;
#59271=EDGE_CURVE ( 'NONE', #17299, #23493, #67087, .T. ) ;
#59272=CARTESIAN_POINT ( 'NONE',  ( 0.4396325459317593221, 0.2952755905511810774, -0.1292274648535930714 ) ) ;
#59273=CARTESIAN_POINT ( 'NONE',  ( -0.3937007874015740483, -0.1870078740157479769, 0.4822834645669291653 ) ) ;
#59276=CARTESIAN_POINT ( 'NONE',  ( 0.6102362204724416372, -0.4536011799217367080, 0.2665933059059888421 ) ) ;
#59281=CARTESIAN_POINT ( 'NONE',  ( 0.09842519685039434474, -0.5400638737290845981, -0.3530559997133363437 ) ) ;
#59282=CARTESIAN_POINT ( 'NONE',  ( 1.476377952755906220, 0.1660481256975883668, -0.3530559997133364547 ) ) ;
#59283=CARTESIAN_POINT ( 'NONE',  ( 0.2559055118110243332, 0.1660481256975885056, 0.3530559997133364547 ) ) ;
#59284=CARTESIAN_POINT ( 'NONE',  ( -0.5577427821522301654, -0.2845877964562159024, 0.3641732283464567677 ) ) ;
#59285=CARTESIAN_POINT ( 'NONE',  ( 1.181102362204725198, -0.1870078740157479769, 0.4822834645669291653 ) ) ;
#59286=CARTESIAN_POINT ( 'NONE',  ( -0.4068241469816264999, -0.4281496062992124485, 0.4176697321401328655 ) ) ;
#59287=CARTESIAN_POINT ( 'NONE',  ( 0.05249343832021075018, 0.2306618581243847221, -0.2411417322834647770 ) ) ;
#59288=CARTESIAN_POINT ( 'NONE',  ( -1.594488188976377119, 0.1660481256975883668, -0.3530559997133364547 ) ) ;
#59289=CARTESIAN_POINT ( 'NONE',  ( 0.7545931758530188826, -0.6692913385826771977, 0.1292274648535927661 ) ) ;
#59291=CARTESIAN_POINT ( 'NONE',  ( 1.332020997375329197, -0.3162353388693405765, 0.4822834645669290543 ) ) ;
#59293=CARTESIAN_POINT ( 'NONE',  ( 0.4330708661417329575, 0.1771653543307087630, 0.000000000000000000 ) ) ;
#59297=CARTESIAN_POINT ( 'NONE',  ( -0.6167979002624665030, -0.004921259842519576551, 0.3153832671262227771 ) ) ;
#59298=CARTESIAN_POINT ( 'NONE',  ( -0.04593175853018302557, 0.2952755905511811885, 0.1292274648535926551 ) ) ;
#59300=CARTESIAN_POINT ( 'NONE',  ( -0.1509186351706028884, -0.05778040916215522460, 0.4822834645669289988 ) ) ;
#59301=CARTESIAN_POINT ( 'NONE',  ( -0.07217847769028813698, -0.3162353388693409650, -0.4822834645669289433 ) ) ;
#59302=CARTESIAN_POINT ( 'NONE',  ( -0.9645669291338575535, 0.1660481256975883668, -0.3530559997133364547 ) ) ;
#59303=CARTESIAN_POINT ( 'NONE',  ( -0.9514435695538050464, -0.3162353388693405765, 0.4822834645669290543 ) ) ;
#59304=CARTESIAN_POINT ( 'NONE',  ( 1.299212598425197429, -0.5511811023622047445, 6.969142054262312111E-17 ) ) ;
#59305=CARTESIAN_POINT ( 'NONE',  ( -1.646981627296586703, -0.05778040916215522460, 0.4822834645669289988 ) ) ;
#59307=CARTESIAN_POINT ( 'NONE',  ( 1.003937007874016185, 0.07958543189024071263, -0.2665933059059888421 ) ) ;
#59308=CARTESIAN_POINT ( 'NONE',  ( 0.4199475065616805614, 0.2306618581243848609, 0.2411417322834645549 ) ) ;
#59309=CARTESIAN_POINT ( 'NONE',  ( 0.2624671916010504757, 0.2306618581243848609, 0.2411417322834645549 ) ) ;
#59315=CARTESIAN_POINT ( 'NONE',  ( -0.3477690288713905509, -0.6692913385826771977, 0.1292274648535927661 ) ) ;
#59318=CARTESIAN_POINT ( 'NONE',  ( -1.233595800524933894, -0.5023911411419708095, -0.1820866141732282451 ) ) ;
#59319=CARTESIAN_POINT ( 'NONE',  ( 0.9645669291338588858, 0.1660481256975885056, 0.3530559997133364547 ) ) ;
#59320=CARTESIAN_POINT ( 'NONE',  ( 1.030183727034121421, -0.05778040916215522460, 0.4822834645669289988 ) ) ;
#59321=CARTESIAN_POINT ( 'NONE',  ( -0.07217847769028787330, -0.08942795157527998196, 0.3641732283464567121 ) ) ;
#59322=CARTESIAN_POINT ( 'NONE',  ( 0.5839895013123367340, -0.6692913385826773087, -0.1292274648535924053 ) ) ;
#59324=CARTESIAN_POINT ( 'NONE',  ( -0.1968503937007867743, 0.1771653543307087630, 0.000000000000000000 ) ) ;
#59325=CARTESIAN_POINT ( 'NONE',  ( 0.03280839895013198948, 0.2952755905511811885, 0.1292274648535926551 ) ) ;
#59327=CARTESIAN_POINT ( 'NONE',  ( -1.587926509186350810, -0.4281496062992124485, 0.4176697321401328655 ) ) ;
#59328=CARTESIAN_POINT ( 'NONE',  ( 0.7020997375328090762, -0.08942795157528024563, -0.3641732283464568787 ) ) ;
#59329=CARTESIAN_POINT ( 'NONE',  ( 1.469816272965879911, -0.5023911411419708095, 0.1820866141732285504 ) ) ;
#59330=CARTESIAN_POINT ( 'NONE',  ( -0.8858267716535425107, 0.1660481256975883668, -0.3530559997133364547 ) ) ;
#59331=CARTESIAN_POINT ( 'NONE',  ( -0.1509186351706028884, -0.2845877964562161244, -0.3641732283464567121 ) ) ;
#59333=CARTESIAN_POINT ( 'NONE',  ( -0.8595800524934373854, -0.3162353388693409650, -0.4822834645669289433 ) ) ;
#59334=CARTESIAN_POINT ( 'NONE',  ( -0.7152230971128602510, -0.3162353388693405765, 0.4822834645669290543 ) ) ;
#59335=CARTESIAN_POINT ( 'NONE',  ( -0.1509186351706028884, -0.3162353388693409650, -0.4822834645669289433 ) ) ;
#59339=CARTESIAN_POINT ( 'NONE',  ( 0.7742782152230979209, -0.004921259842519870586, -0.3153832671262229437 ) ) ;
#59340=CARTESIAN_POINT ( 'NONE',  ( 1.207349081364829990, -0.6046776061558809534, -0.2411417322834644161 ) ) ;
#59341=CARTESIAN_POINT ( 'NONE',  ( -0.7545931758530177724, 0.1771653543307087630, 0.09757992244046791164 ) ) ;
#59342=CARTESIAN_POINT ( 'NONE',  ( -1.233595800524933894, 0.1283753931104748280, 0.1820866141732283561 ) ) ;
#59343=CARTESIAN_POINT ( 'NONE',  ( -0.8202099737532799750, 0.2952755905511810774, -0.1292274648535930714 ) ) ;
#59344=CARTESIAN_POINT ( 'NONE',  ( -0.5183727034120726440, -0.6692913385826773087, -0.1292274648535924053 ) ) ;
#59345=CARTESIAN_POINT ( 'NONE',  ( 0.6233595800524942554, -0.08942795157528024563, -0.3641732283464568787 ) ) ;
#59347=CARTESIAN_POINT ( 'NONE',  ( 1.076115485564305141, -0.5023911411419708095, 0.1820866141732285504 ) ) ;
#59348=CARTESIAN_POINT ( 'NONE',  ( 0.2624671916010504757, 0.2306618581243848609, 0.2411417322834645549 ) ) ;
#59350=CARTESIAN_POINT ( 'NONE',  ( -0.6496062992125976043, -0.5400638737290844871, 0.3530559997133364547 ) ) ;
#59352=CARTESIAN_POINT ( 'NONE',  ( 1.377952755905512472, -0.5511811023622047445, 6.969142054262312111E-17 ) ) ;
#59353=CARTESIAN_POINT ( 'NONE',  ( 0.4002624671916016896, -0.05778040916215522460, 0.4822834645669289988 ) ) ;
#59354=CARTESIAN_POINT ( 'NONE',  ( 0.1509186351706045259, -0.05778040916215560624, -0.4822834645669293319 ) ) ;
#59355=CARTESIAN_POINT ( 'NONE',  ( -0.03937007874015669567, 0.1771653543307087630, 0.000000000000000000 ) ) ;
#59356=CARTESIAN_POINT ( 'NONE',  ( 0.5643044619422579178, 0.009842519685039467087, 0.3409548833797002021 ) ) ;
#59357=CARTESIAN_POINT ( 'NONE',  ( -0.1771653543307080136, 0.07958543189024071263, -0.2665933059059888421 ) ) ;
#59358=CARTESIAN_POINT ( 'NONE',  ( 0.8661417322834653598, -0.1870078740157479769, 0.4822834645669291653 ) ) ;
#59359=CARTESIAN_POINT ( 'NONE',  ( -0.7677165354330699465, 0.07958543189024085140, 0.2665933059059887866 ) ) ;
#59360=CARTESIAN_POINT ( 'NONE',  ( -1.213910761154854745, -0.6692913385826771977, 0.1292274648535927661 ) ) ;
#59363=CARTESIAN_POINT ( 'NONE',  ( -1.318897637795274802, 0.1660481256975885056, 0.3530559997133364547 ) ) ;
#59364=CARTESIAN_POINT ( 'NONE',  ( -1.135170603674539924, -0.5511811023622046335, 0.09757992244046803654 ) ) ;
#59366=CARTESIAN_POINT ( 'NONE',  ( -0.05249343832020938322, -0.6046776061558809534, -0.2411417322834644161 ) ) ;
#59368=CARTESIAN_POINT ( 'NONE',  ( -0.8005249343832011588, 0.05413385826771626580, -0.4176697321401330321 ) ) ;
#59370=CARTESIAN_POINT ( 'NONE',  ( 1.620734908136483465, -0.6692913385826771977, 0.1292274648535927661 ) ) ;
#59371=CARTESIAN_POINT ( 'NONE',  ( 0.7874015748031503170, -0.1870078740157479769, 0.4822834645669291653 ) ) ;
#59372=CARTESIAN_POINT ( 'NONE',  ( 1.036745406824147731, 0.05413385826771666132, 0.4176697321401328100 ) ) ;
#59374=CARTESIAN_POINT ( 'NONE',  ( 1.581364829396326277, -0.05778040916215522460, 0.4822834645669289988 ) ) ;
#59376=CARTESIAN_POINT ( 'NONE',  ( -1.332020997375327642, -0.3162353388693409650, -0.4822834645669289433 ) ) ;
#59379=CARTESIAN_POINT ( 'NONE',  ( -0.6102362204724400829, -0.4536011799217368745, -0.2665933059059886201 ) ) ;
#59382=CARTESIAN_POINT ( 'NONE',  ( 0.3412073490813655186, 0.2306618581243848609, 0.2411417322834645549 ) ) ;
#59383=CARTESIAN_POINT ( 'NONE',  ( 0.03937007874015806264, 0.2952755905511811885, 0.000000000000000000 ) ) ;
#59384=CARTESIAN_POINT ( 'NONE',  ( -0.5446194225721777693, -0.05778040916215522460, 0.4822834645669289988 ) ) ;
#59385=CARTESIAN_POINT ( 'NONE',  ( 1.482939632545932307, -0.4281496062992124485, 0.4176697321401328655 ) ) ;
#59386=CARTESIAN_POINT ( 'NONE',  ( -0.7742782152230962556, -0.3690944881889765550, -0.3153832671262227771 ) ) ;
#59387=CARTESIAN_POINT ( 'NONE',  ( -0.7426113562972006532, 2.209901789876323797, -0.5309055118110235227 ) ) ;
#59388=CARTESIAN_POINT ( 'NONE',  ( 0.8464566929133866546, -0.5400638737290844871, 0.3530559997133364547 ) ) ;
#59389=CARTESIAN_POINT ( 'NONE',  ( 0.5380577427821529035, -0.004921259842519870586, -0.3153832671262229437 ) ) ;
#59390=CARTESIAN_POINT ( 'NONE',  ( -0.2427821522309703550, -0.3162353388693405765, 0.4822834645669290543 ) ) ;
#59392=CARTESIAN_POINT ( 'NONE',  ( -0.6889763779527552368, 0.1660481256975885056, 0.3530559997133364547 ) ) ;
#59393=CARTESIAN_POINT ( 'NONE',  ( -1.633858267716534529, -0.4536011799217368745, -0.2665933059059886201 ) ) ;
#59394=CARTESIAN_POINT ( 'NONE',  ( 1.286089238845145033, -0.6046776061558809534, -0.2411417322834644161 ) ) ;
#59395=CARTESIAN_POINT ( 'NONE',  ( 1.502624671916010790, -0.08942795157527998196, 0.3641732283464567121 ) ) ;
#59398=CARTESIAN_POINT ( 'NONE',  ( 0.01968503937007957949, -0.5400638737290845981, -0.3530559997133363437 ) ) ;
#59400=CARTESIAN_POINT ( 'NONE',  ( -1.122047244094487306, -0.5400638737290844871, 0.3530559997133364547 ) ) ;
#59401=CARTESIAN_POINT ( 'NONE',  ( 1.069553805774278610, -0.6692913385826771977, 0.1292274648535927661 ) ) ;
#59402=CARTESIAN_POINT ( 'NONE',  ( 1.259842519685040019, -0.1870078740157479769, 0.4822834645669291653 ) ) ;
#59404=CARTESIAN_POINT ( 'NONE',  ( 0.4265091863517067039, -0.6692913385826773087, -0.1292274648535924053 ) ) ;
#59405=CARTESIAN_POINT ( 'NONE',  ( -0.3871391076115476282, -0.05778040916215522460, 0.4822834645669289988 ) ) ;
#59407=CARTESIAN_POINT ( 'NONE',  ( -1.299212598425196097, -0.6692913385826771977, 8.415575281601705876E-17 ) ) ;
#59408=CARTESIAN_POINT ( 'NONE',  ( -0.5511811023622038563, -0.1870078740157479769, 0.4822834645669291653 ) ) ;
#59410=CARTESIAN_POINT ( 'NONE',  ( -0.3937007874015740483, -0.1870078740157479769, 0.3641732283464567677 ) ) ;
#59412=CARTESIAN_POINT ( 'NONE',  ( -0.6758530183727028406, -0.6692913385826773087, -0.1292274648535924053 ) ) ;
#59414=CARTESIAN_POINT ( 'NONE',  ( 0.8070866141732288002, 0.1660481256975885056, 0.3530559997133364547 ) ) ;
#59417=( BOUNDED_CURVE ( )  B_SPLINE_CURVE ( 2, ( #50720, #56221, #5695, #37686, #50309, #4881, #75600, #10793, #37284, #63361, #63770, #17127, #42759 ),
 .UNSPECIFIED., .F., .F. ) 
 B_SPLINE_CURVE_WITH_KNOTS ( ( 3, 2, 2, 2, 2, 2, 3 ),
 ( 0.2642401855438917813, 0.2651515151515151381, 0.2689393939393939226, 0.2727272727272727071, 0.2765151515151514916, 0.2803030303030302761, 0.2812143599106537439 ),
 .UNSPECIFIED. ) 
 CURVE ( )  GEOMETRIC_REPRESENTATION_ITEM ( )  RATIONAL_B_SPLINE_CURVE ( ( 0.9875488213027530104, 0.9918020599134685922, 1.000000000000000000, 0.9659258262890683122, 1.000000000000000000, 0.9659258262890683122, 1.000000000000000000, 0.9659258262890683122, 1.000000000000000000, 0.9659258262890683122, 1.000000000000000000, 0.9918020599134677040, 0.9875488213027521223 ) ) 
 REPRESENTATION_ITEM ( '' )  );
#59418=CARTESIAN_POINT ( 'NONE',  ( -0.2755905511811015396, -0.6692913385826771977, 8.415575281601705876E-17 ) ) ;
#59419=CARTESIAN_POINT ( 'NONE',  ( 0.8530183727034128527, -0.3690944881889763329, 0.3153832671262228327 ) ) ;
#59420=CARTESIAN_POINT ( 'NONE',  ( -0.8792650918635160906, 0.009842519685039144428, -0.3409548833797004797 ) ) ;
#59422=CARTESIAN_POINT ( 'NONE',  ( 1.351706036745407680, -0.004921259842519576551, 0.3153832671262227771 ) ) ;
#59423=CARTESIAN_POINT ( 'NONE',  ( 1.122047244094488860, 0.1660481256975885056, 0.3530559997133364547 ) ) ;
#59426=CARTESIAN_POINT ( 'NONE',  ( -0.006561679790025524116, -0.3162353388693405765, 0.4822834645669290543 ) ) ;
#59427=CARTESIAN_POINT ( 'NONE',  ( -1.463254593175852492, 0.2952755905511811885, 0.1292274648535926551 ) ) ;
#59428=CARTESIAN_POINT ( 'NONE',  ( -1.601049868766403650, -0.6046776061558807314, 0.2411417322834647770 ) ) ;
#59429=CARTESIAN_POINT ( 'NONE',  ( -0.04593175853018302557, -0.6692913385826773087, -0.1292274648535924053 ) ) ;
#59431=CARTESIAN_POINT ( 'NONE',  ( 1.220472440944882608, 0.2952755905511811885, 0.000000000000000000 ) ) ;
#59432=CARTESIAN_POINT ( 'NONE',  ( 0.5839895013123367340, -0.6692913385826773087, -0.1292274648535924053 ) ) ;
#59434=CARTESIAN_POINT ( 'NONE',  ( 0.8792650918635177559, -0.004921259842519576551, 0.3153832671262227771 ) ) ;
#59436=CARTESIAN_POINT ( 'NONE',  ( 0.5183727034120741983, -0.5511811023622046335, 0.09757992244046803654 ) ) ;
#59437=CARTESIAN_POINT ( 'NONE',  ( -1.430446194225720724, 0.05413385826771626580, -0.4176697321401330321 ) ) ;
#59440=CARTESIAN_POINT ( 'NONE',  ( 1.161417322834646493, -0.5400638737290844871, 0.3530559997133364547 ) ) ;
#59442=CARTESIAN_POINT ( 'NONE',  ( 0.2821522309711292364, 0.2952755905511810774, -0.1292274648535930714 ) ) ;
#59444=CARTESIAN_POINT ( 'NONE',  ( -0.3277333542595150528, 0.004960608223778509643, -0.3437734562760191848 ) ) ;
#59445=CARTESIAN_POINT ( 'NONE',  ( 0.4921259842519691285, 0.07958543189024085140, 0.2665933059059887866 ) ) ;
#59447=CARTESIAN_POINT ( 'NONE',  ( 0.6364829396325465405, -0.3162353388693409650, -0.4822834645669289433 ) ) ;
#59449=CARTESIAN_POINT ( 'NONE',  ( -0.8858267716535425107, 0.07958543189024071263, -0.2665933059059888421 ) ) ;
#59450=CARTESIAN_POINT ( 'NONE',  ( -1.108923884514435132, -0.3162353388693405765, 0.4822834645669290543 ) ) ;
#59451=CARTESIAN_POINT ( 'NONE',  ( -1.620734908136482577, -0.6692913385826773087, -0.1292274648535924053 ) ) ;
#59452=CARTESIAN_POINT ( 'NONE',  ( 0.5905511811023629321, 0.2952755905511811885, 0.000000000000000000 ) ) ;
#59454=CARTESIAN_POINT ( 'NONE',  ( 1.686351706036745890, 0.2952755905511811885, 0.1292274648535926551 ) ) ;
#59457=CARTESIAN_POINT ( 'NONE',  ( 0.6496062992125991586, 0.1660481256975885056, 0.3530559997133364547 ) ) ;
#59459=CARTESIAN_POINT ( 'NONE',  ( -1.646051170424378096, 0.000000000000000000, 0.3464511005275205946 ) ) ;
#59460=CARTESIAN_POINT ( 'NONE',  ( 1.496062992125985147, -0.1870078740157479769, 0.4822834645669291653 ) ) ;
#59461=CARTESIAN_POINT ( 'NONE',  ( -1.535433070866141225, 0.1771653543307087630, 0.000000000000000000 ) ) ;
#59462=CARTESIAN_POINT ( 'NONE',  ( 1.167979002624672580, -0.3690944881889763329, 0.3153832671262228327 ) ) ;
#59463=CARTESIAN_POINT ( 'NONE',  ( -1.456692913385826182, 0.1771653543307087630, 0.000000000000000000 ) ) ;
#59464=CARTESIAN_POINT ( 'NONE',  ( -0.6889763779527552368, 0.07958543189024085140, 0.2665933059059887866 ) ) ;
#59466=CARTESIAN_POINT ( 'NONE',  ( 0.7217847769028878924, -0.3690944881889765550, -0.3153832671262227771 ) ) ;
#59467=CARTESIAN_POINT ( 'NONE',  ( 0.4330708661417329575, 0.2952755905511811885, 0.000000000000000000 ) ) ;
#59468=CARTESIAN_POINT ( 'NONE',  ( 1.036745406824147508, -0.4281496062992127816, -0.4176697321401328100 ) ) ;
#59469=CARTESIAN_POINT ( 'NONE',  ( 0.2427821522309719648, -0.05778040916215522460, 0.4822834645669289988 ) ) ;
#59470=CARTESIAN_POINT ( 'NONE',  ( 0.09186351706036799403, -0.3690944881889765550, -0.3153832671262227771 ) ) ;
#59471=CARTESIAN_POINT ( 'NONE',  ( 1.148293963254593653, 0.2952755905511810774, -0.1292274648535930714 ) ) ;
#59472=CARTESIAN_POINT ( 'NONE',  ( -0.1698998578625667832, -2.609869883881465018E-15, -0.3464511005275220379 ) ) ;
#59473=CARTESIAN_POINT ( 'NONE',  ( -0.7414698162729651543, 0.2952755905511810774, -0.1292274648535930714 ) ) ;
#59476=CARTESIAN_POINT ( 'NONE',  ( 0.1049868766404206816, -0.6046776061558809534, -0.2411417322834644161 ) ) ;
#59477=CARTESIAN_POINT ( 'NONE',  ( -0.9842519685039360366, 0.2952755905511811885, 0.000000000000000000 ) ) ;
#59478=CARTESIAN_POINT ( 'NONE',  ( -0.01968503937007793844, -0.5400638737290844871, 0.3530559997133364547 ) ) ;
#59484=CARTESIAN_POINT ( 'NONE',  ( -1.220472440944881054, 0.1771653543307087630, 0.000000000000000000 ) ) ;
#59486=CARTESIAN_POINT ( 'NONE',  ( -1.391076115485563758, 0.2306618581243848609, 0.2411417322834645549 ) ) ;
#59488=CARTESIAN_POINT ( 'NONE',  ( 0.4330708661417329575, 0.2952755905511811885, 0.000000000000000000 ) ) ;
#59489=CARTESIAN_POINT ( 'NONE',  ( -0.6758530183727028406, -0.5511811023622048555, -0.09757992244046775898 ) ) ;
#59490=CARTESIAN_POINT ( 'NONE',  ( 0.6889763779527563470, 0.1660481256975883668, -0.3530559997133364547 ) ) ;
#59491=CARTESIAN_POINT ( 'NONE',  ( 0.3477690288713918276, 0.2952755905511811885, 0.1292274648535926551 ) ) ;
#59495=CARTESIAN_POINT ( 'NONE',  ( 1.325459317585302665, -0.4281496062992124485, 0.4176697321401328655 ) ) ;
#59496=CARTESIAN_POINT ( 'NONE',  ( -0.08530183727034056085, -0.05778040916215560624, -0.4822834645669293319 ) ) ;
#59498=CARTESIAN_POINT ( 'NONE',  ( 1.358267716535433323, -0.5400638737290845981, -0.3530559997133363437 ) ) ;
#59499=CARTESIAN_POINT ( 'NONE',  ( 0.9580052493438327987, -0.4281496062992127816, -0.4176697321401328100 ) ) ;
#59501=CARTESIAN_POINT ( 'NONE',  ( 0.2099737532808405305, 0.2306618581243847221, -0.2411417322834647770 ) ) ;
#59502=CARTESIAN_POINT ( 'NONE',  ( 0.8136482939632553313, -0.6046776061558809534, -0.2411417322834644161 ) ) ;
#59503=CARTESIAN_POINT ( 'NONE',  ( -0.2165354330708654795, 0.1660481256975885056, 0.3530559997133364547 ) ) ;
#59504=CARTESIAN_POINT ( 'NONE',  ( 0.7742782152230979209, -0.004921259842519870586, -0.3153832671262229437 ) ) ;
#59505=CARTESIAN_POINT ( 'NONE',  ( -1.181102362204723644, -0.1870078740157480879, -0.4822834645669291653 ) ) ;
#59506=CARTESIAN_POINT ( 'NONE',  ( -1.515748031496062076, 0.1660481256975883668, -0.3530559997133364547 ) ) ;
#59507=CARTESIAN_POINT ( 'NONE',  ( 0.9514435695538062676, -0.05778040916215522460, 0.4822834645669289988 ) ) ;
#59513=CARTESIAN_POINT ( 'NONE',  ( 1.266404199475066328, -0.3162353388693409650, -0.4822834645669289433 ) ) ;
#59514=CARTESIAN_POINT ( 'NONE',  ( 0.8267716535433077274, 0.1771653543307087630, 0.000000000000000000 ) ) ;
#59518=CARTESIAN_POINT ( 'NONE',  ( 1.496062992125984703, -0.1870078740157480879, -0.4822834645669291653 ) ) ;
#59520=CARTESIAN_POINT ( 'NONE',  ( -0.5118110236220466680, -0.6692913385826771977, 8.415575281601705876E-17 ) ) ;
#59521=CARTESIAN_POINT ( 'NONE',  ( 0.8989501312335963501, -0.6692913385826773087, -0.1292274648535924053 ) ) ;
#59523=CARTESIAN_POINT ( 'NONE',  ( -1.450131233595799651, -0.6692913385826771977, 0.1292274648535927661 ) ) ;
#59526=CARTESIAN_POINT ( 'NONE',  ( 1.515748031496063408, 0.07958543189024085140, 0.2665933059059887866 ) ) ;
#59528=CARTESIAN_POINT ( 'NONE',  ( -0.7611548556430438595, -0.5023911411419708095, -0.1820866141732282451 ) ) ;
#59529=CARTESIAN_POINT ( 'NONE',  ( -1.555118110236219930, -0.5400638737290845981, -0.3530559997133363437 ) ) ;
#59530=CARTESIAN_POINT ( 'NONE',  ( 0.5511811023622055217, -0.1870078740157479769, 0.4822834645669291653 ) ) ;
#59531=ORIENTED_EDGE ( 'NONE', *, *, #19583, .T. ) ;
#59532=CARTESIAN_POINT ( 'NONE',  ( 1.535433070866142558, 0.2952755905511811885, 0.000000000000000000 ) ) ;
#59533=DIRECTION ( 'NONE',  ( -3.096699300667737957E-16, 1.000000000000000000, -0.000000000000000000 ) ) ;
#59534=CARTESIAN_POINT ( 'NONE',  ( -0.8858267716535425107, 0.07958543189024071263, -0.2665933059059888421 ) ) ;
#59535=CARTESIAN_POINT ( 'NONE',  ( 1.010498687664042716, -0.4281496062992124485, 0.4176697321401328655 ) ) ;
#59536=CARTESIAN_POINT ( 'NONE',  ( -1.640419947506561060, -0.4281496062992127816, -0.4176697321401328100 ) ) ;
#59539=CARTESIAN_POINT ( 'NONE',  ( -0.6561679790026240244, -0.5023911411419708095, 0.1820866141732285504 ) ) ;
#59540=CARTESIAN_POINT ( 'NONE',  ( 1.581364829396326277, -0.3162353388693409650, -0.4822834645669289433 ) ) ;
#59541=MANIFOLD_SOLID_BREP ( 'Cut-Sweep1', #36623 ) ;
#59542=CARTESIAN_POINT ( 'NONE',  ( 1.436417322834644184, 0.8346805926620878280, -0.3149606299212601157 ) ) ;
#59543=CARTESIAN_POINT ( 'NONE',  ( 0.6233595800524939223, -0.3162353388693405765, 0.4822834645669290543 ) ) ;
#59544=CARTESIAN_POINT ( 'NONE',  ( -1.017060367454067249, -0.08942795157527998196, 0.3641732283464567121 ) ) ;
#59545=CARTESIAN_POINT ( 'NONE',  ( -0.4133858267716528645, 0.07958543189024071263, -0.2665933059059888421 ) ) ;
#59546=CARTESIAN_POINT ( 'NONE',  ( -0.2034120734908131112, -0.6692913385826773087, -0.1292274648535924053 ) ) ;
#59547=CARTESIAN_POINT ( 'NONE',  ( -1.023622047244093558, -0.1870078740157479769, 0.3641732283464567677 ) ) ;
#59549=CARTESIAN_POINT ( 'NONE',  ( 0.8792650918635177559, -0.4281496062992127816, -0.4176697321401328100 ) ) ;
#59550=CARTESIAN_POINT ( 'NONE',  ( 0.8780747636526964328, 6.817843310734658629E-16, 0.3627989612356145588 ) ) ;
#59552=CARTESIAN_POINT ( 'NONE',  ( -0.9580052493438311334, -0.4281496062992124485, 0.4176697321401328655 ) ) ;
#59553=CARTESIAN_POINT ( 'NONE',  ( -0.1837270341207343505, -0.5023911411419708095, 0.1820866141732285504 ) ) ;
#59554=CARTESIAN_POINT ( 'NONE',  ( -1.410761154855641575, -0.3162353388693409650, -0.4822834645669289433 ) ) ;
#59555=CARTESIAN_POINT ( 'NONE',  ( 0.7414698162729663755, 0.1771653543307087630, 0.09757992244046791164 ) ) ;
#59556=CARTESIAN_POINT ( 'NONE',  ( -0.5314960629921254842, -0.4536011799217368745, -0.2665933059059886201 ) ) ;
#59557=CARTESIAN_POINT ( 'NONE',  ( -0.9711286089238838626, -0.6046776061558807314, 0.2411417322834647770 ) ) ;
#59558=CARTESIAN_POINT ( 'NONE',  ( -1.496062992125983815, -0.1870078740157480879, -0.4822834645669291653 ) ) ;
#59559=CARTESIAN_POINT ( 'NONE',  ( -1.594488188976377119, 0.1660481256975883668, -0.3530559997133364547 ) ) ;
#59561=CARTESIAN_POINT ( 'NONE',  ( 0.9317585301837276734, -0.004921259842519870586, -0.3153832671262229437 ) ) ;
#59562=CARTESIAN_POINT ( 'NONE',  ( 0.3280839895013130669, -0.4281496062992127816, -0.4176697321401328100 ) ) ;
#59563=CARTESIAN_POINT ( 'NONE',  ( -1.299212598425196097, 0.2952755905511811885, 0.000000000000000000 ) ) ;
#59564=CARTESIAN_POINT ( 'NONE',  ( 1.246719160104987623, -0.3690944881889763329, 0.3153832671262228327 ) ) ;
#59567=CARTESIAN_POINT ( 'NONE',  ( -1.233595800524933894, -0.5023911411419708095, -0.1820866141732282451 ) ) ;
#59568=CARTESIAN_POINT ( 'NONE',  ( -0.4199475065616791736, -0.6046776061558807314, 0.2411417322834647770 ) ) ;
#59569=CARTESIAN_POINT ( 'NONE',  ( 0.1312335958005255154, -0.6046776061558807314, 0.2411417322834647770 ) ) ;
#59570=CARTESIAN_POINT ( 'NONE',  ( -1.292650918635170010, -0.5511811023622046335, 0.09757992244046803654 ) ) ;
#59572=CARTESIAN_POINT ( 'NONE',  ( -1.332020997375327642, -0.3162353388693409650, -0.4822834645669289433 ) ) ;
#59573=CARTESIAN_POINT ( 'NONE',  ( 0.5905511811023629321, 0.2952755905511811885, 0.000000000000000000 ) ) ;
#59574=CARTESIAN_POINT ( 'NONE',  ( 8.195543980992789655E-16, -0.1870078740157480879, -0.4822834645669291653 ) ) ;
#59575=CARTESIAN_POINT ( 'NONE',  ( 1.174540682414699111, -0.05778040916215560624, -0.4822834645669293319 ) ) ;
#59581=CARTESIAN_POINT ( 'NONE',  ( 0.4330708661417329575, -0.5511811023622047445, 6.969142054262312111E-17 ) ) ;
#59582=CARTESIAN_POINT ( 'NONE',  ( -0.4658792650918627265, -0.05778040916215522460, 0.4822834645669289988 ) ) ;
#59583=CARTESIAN_POINT ( 'NONE',  ( 1.220472440944882386, -0.6692913385826771977, 8.415575281601705876E-17 ) ) ;
#59585=CARTESIAN_POINT ( 'NONE',  ( -0.09842519685039295696, -0.4536011799217367080, 0.2665933059059888421 ) ) ;
#59586=CARTESIAN_POINT ( 'NONE',  ( -1.115485564304461219, 0.05413385826771626580, -0.4176697321401330321 ) ) ;
#59587=CARTESIAN_POINT ( 'NONE',  ( -1.633858267716534529, 0.1660481256975885056, 0.3530559997133364547 ) ) ;
#59592=ORIENTED_EDGE ( 'NONE', *, *, #45224, .T. ) ;
#59594=CARTESIAN_POINT ( 'NONE',  ( 1.548556430446194954, -0.5023911411419708095, 0.1820866141732285504 ) ) ;
#59595=CARTESIAN_POINT ( 'NONE',  ( -1.292650918635170010, 0.1771653543307087075, -0.09757992244046823083 ) ) ;
#59596=CARTESIAN_POINT ( 'NONE',  ( -1.062992125984250968, -0.6692913385826771977, 8.415575281601705876E-17 ) ) ;
#59598=CARTESIAN_POINT ( 'NONE',  ( -1.603475055217291612, 1.267857067133556281, -0.04573490813648263542 ) ) ;
#59599=CARTESIAN_POINT ( 'NONE',  ( 1.332020997375329197, -0.3162353388693405765, 0.4822834645669290543 ) ) ;
#59600=CARTESIAN_POINT ( 'NONE',  ( -1.391076115485563758, 0.2306618581243848609, 0.2411417322834645549 ) ) ;
#59601=CARTESIAN_POINT ( 'NONE',  ( -0.01968503937007793844, -0.5400638737290844871, 0.3530559997133364547 ) ) ;
#59602=CARTESIAN_POINT ( 'NONE',  ( -1.377952755905511140, -0.6692913385826771977, 8.415575281601705876E-17 ) ) ;
#59604=CARTESIAN_POINT ( 'NONE',  ( 0.7611548556430451917, -0.6046776061558807314, 0.2411417322834647770 ) ) ;
#59606=CARTESIAN_POINT ( 'NONE',  ( -1.043307086614172041, -0.4536011799217367080, 0.2665933059059888421 ) ) ;
#59607=VERTEX_POINT ( 'NONE', #60346 ) ;
#59609=ORIENTED_EDGE ( 'NONE', *, *, #77894, .F. ) ;
#59610=CARTESIAN_POINT ( 'NONE',  ( 1.604771003085129211, 1.278209470906375378, 0.1466069496707752828 ) ) ;
#59611=CARTESIAN_POINT ( 'NONE',  ( -0.9251968503937002541, 0.1660481256975885056, 0.3530559997133364547 ) ) ;
#59612=CARTESIAN_POINT ( 'NONE',  ( -1.167979002624671470, 0.05413385826771666132, 0.4176697321401328100 ) ) ;
#59614=CARTESIAN_POINT ( 'NONE',  ( -1.450131233595799651, -0.6692913385826771977, 0.1292274648535927661 ) ) ;
#59615=CARTESIAN_POINT ( 'NONE',  ( -1.482939632545930975, -0.4281496062992127816, -0.4176697321401328100 ) ) ;
#59616=CARTESIAN_POINT ( 'NONE',  ( -1.272965879265091305, 0.05413385826771626580, -0.4176697321401330321 ) ) ;
#59619=CARTESIAN_POINT ( 'NONE',  ( 0.1640419947506569498, -0.2845877964562161244, -0.3641732283464567121 ) ) ;
#59621=CARTESIAN_POINT ( 'NONE',  ( -0.7349081364829390672, 0.1283753931104746893, -0.1820866141732285504 ) ) ;
#59622=CARTESIAN_POINT ( 'NONE',  ( -1.089238845144356427, -0.4281496062992127816, -0.4176697321401328100 ) ) ;
#59623=CARTESIAN_POINT ( 'NONE',  ( 1.010498687664042716, 0.05413385826771626580, -0.4176697321401330321 ) ) ;
#59624=CARTESIAN_POINT ( 'NONE',  ( -0.8792650918635160906, -0.4281496062992124485, 0.4176697321401328655 ) ) ;
#59626=ORIENTED_EDGE ( 'NONE', *, *, #20226, .T. ) ;
#59627=CARTESIAN_POINT ( 'NONE',  ( -1.003937007874014853, 0.1660481256975885056, 0.3530559997133364547 ) ) ;
#59628=CARTESIAN_POINT ( 'NONE',  ( 0.7545931758530188826, -0.6692913385826771977, 0.1292274648535927661 ) ) ;
#59629=CARTESIAN_POINT ( 'NONE',  ( -1.417322834645668772, -0.1870078740157479769, 0.3641732283464567677 ) ) ;
#59634=CARTESIAN_POINT ( 'NONE',  ( -0.5118110236220466680, 0.2952755905511811885, 0.000000000000000000 ) ) ;
#59635=CARTESIAN_POINT ( 'NONE',  ( 1.660104986876641320, -0.05778040916215522460, 0.4822834645669289988 ) ) ;
#59637=CARTESIAN_POINT ( 'NONE',  ( -1.358267716535432434, 0.1660481256975883668, -0.3530559997133364547 ) ) ;
#59639=CARTESIAN_POINT ( 'NONE',  ( -1.443569553805773564, -0.6046776061558807314, 0.2411417322834647770 ) ) ;
#59640=CARTESIAN_POINT ( 'NONE',  ( -0.5839895013123351797, 0.2952755905511810774, -0.1292274648535930714 ) ) ;
#59642=CARTESIAN_POINT ( 'NONE',  ( 0.6561679790026253567, 0.1283753931104748280, 0.1820866141732283561 ) ) ;
#59645=CARTESIAN_POINT ( 'NONE',  ( 0.4068241469816281097, -0.004921259842519576551, 0.3153832671262227771 ) ) ;
#59646=CARTESIAN_POINT ( 'NONE',  ( 1.482939632545932307, -0.004921259842519870586, -0.3153832671262229437 ) ) ;
#59647=CARTESIAN_POINT ( 'NONE',  ( 1.122047244094488860, 0.1660481256975885056, 0.3530559997133364547 ) ) ;
#59648=CARTESIAN_POINT ( 'NONE',  ( 0.1246719160104994284, 0.1771653543307087075, -0.09757992244046823083 ) ) ;
#59650=CARTESIAN_POINT ( 'NONE',  ( -1.141732283464566011, 0.2952755905511811885, 0.000000000000000000 ) ) ;
#59651=CARTESIAN_POINT ( 'NONE',  ( -0.01968503937007793844, -0.4536011799217367080, 0.2665933059059888421 ) ) ;
#59652=CARTESIAN_POINT ( 'NONE',  ( -1.167979002624671470, -0.004921259842519576551, 0.3153832671262227771 ) ) ;
#59654=CARTESIAN_POINT ( 'NONE',  ( -0.2952755905511803003, -0.4536011799217368745, -0.2665933059059886201 ) ) ;
#59656=CARTESIAN_POINT ( 'NONE',  ( -0.1443569553805765515, -0.4281496062992127816, -0.4176697321401328100 ) ) ;
#59658=CARTESIAN_POINT ( 'NONE',  ( 0.7152230971128614723, -0.2845877964562161244, -0.3641732283464567121 ) ) ;
#59659=CARTESIAN_POINT ( 'NONE',  ( -0.2362204724409442680, -0.1870078740157480601, -0.3641732283464567677 ) ) ;
#59660=CARTESIAN_POINT ( 'NONE',  ( -0.1902887139107604098, 0.2952755905511810774, -0.1292274648535930714 ) ) ;
#59661=CARTESIAN_POINT ( 'NONE',  ( -1.581364829396324945, -0.3162353388693405765, 0.4822834645669290543 ) ) ;
#59662=CARTESIAN_POINT ( 'NONE',  ( -1.154855643044618851, 0.1283753931104748280, 0.1820866141732283561 ) ) ;
#59663=DIRECTION ( 'NONE',  ( 0.000000000000000000, 1.000000000000000000, 0.000000000000000000 ) ) ;
#59664=CARTESIAN_POINT ( 'NONE',  ( 0.4790026246719168435, -0.3162353388693409650, -0.4822834645669289433 ) ) ;
#59666=CARTESIAN_POINT ( 'NONE',  ( -0.9711286089238838626, 0.2306618581243847221, -0.2411417322834647770 ) ) ;
#59669=CARTESIAN_POINT ( 'NONE',  ( -0.1968503937007867743, -0.5511811023622047445, 6.969142054262312111E-17 ) ) ;
#59670=CARTESIAN_POINT ( 'NONE',  ( -1.371391076115484609, -0.6692913385826771977, 0.1292274648535927661 ) ) ;
#59671=CARTESIAN_POINT ( 'NONE',  ( -1.620734908136482577, 0.1771653543307087630, 0.09757992244046791164 ) ) ;
#59673=CARTESIAN_POINT ( 'NONE',  ( -0.6758530183727028406, -0.5511811023622048555, -0.09757992244046775898 ) ) ;
#59674=CARTESIAN_POINT ( 'NONE',  ( -0.5411721830064186722, -2.191421614605370878E-15, 0.4445507791589071167 ) ) ;
#59675=CARTESIAN_POINT ( 'NONE',  ( 1.003937007874016185, 0.1660481256975883668, -0.3530559997133364547 ) ) ;
#59679=CARTESIAN_POINT ( 'NONE',  ( -1.640419947506561060, -0.4281496062992127816, -0.4176697321401328100 ) ) ;
#59680=CARTESIAN_POINT ( 'NONE',  ( -1.253280839895012377, -0.05778040916215522460, 0.4822834645669289988 ) ) ;
#59681=CARTESIAN_POINT ( 'NONE',  ( 1.220472440944882386, -0.6692913385826771977, 8.415575281601705876E-17 ) ) ;
#59683=CARTESIAN_POINT ( 'NONE',  ( 1.489501312335958172, -0.2845877964562159024, 0.3641732283464567677 ) ) ;
#59685=CARTESIAN_POINT ( 'NONE',  ( 0.6955380577427828781, -0.4281496062992124485, 0.4176697321401328655 ) ) ;
#59686=CARTESIAN_POINT ( 'NONE',  ( -0.5774278215223089816, -0.6046776061558807314, 0.2411417322834647770 ) ) ;
#59689=CARTESIAN_POINT ( 'NONE',  ( 0.9383202099737536495, -0.2845877964562159024, 0.3641732283464567677 ) ) ;
#59693=CARTESIAN_POINT ( 'NONE',  ( -0.2755905511811018171, 0.2952755905511811885, 0.000000000000000000 ) ) ;
#59694=CARTESIAN_POINT ( 'NONE',  ( 1.187664041994751285, -0.3162353388693409650, -0.4822834645669289433 ) ) ;
#59695=CARTESIAN_POINT ( 'NONE',  ( 0.4068241469816281097, 0.05413385826771666132, 0.4176697321401328100 ) ) ;
#59696=CARTESIAN_POINT ( 'NONE',  ( -0.2362204724409440182, -0.1870078740157479769, 0.3641732283464567677 ) ) ;
#59698=CARTESIAN_POINT ( 'NONE',  ( 1.358267716535433323, 0.1660481256975885056, 0.3530559997133364547 ) ) ;
#59699=CARTESIAN_POINT ( 'NONE',  ( -1.069553805774277722, -0.6692913385826773087, -0.1292274648535924053 ) ) ;
#59700=CARTESIAN_POINT ( 'NONE',  ( -0.04593175853018302557, -0.6692913385826773087, -0.1292274648535924053 ) ) ;
#59701=CARTESIAN_POINT ( 'NONE',  ( -0.7283464566929126471, 0.1660481256975883668, -0.3530559997133364547 ) ) ;
#59702=CARTESIAN_POINT ( 'NONE',  ( 1.187664041994751285, -0.3162353388693409650, -0.4822834645669289433 ) ) ;
#59703=CARTESIAN_POINT ( 'NONE',  ( 0.8333333333333340365, 0.2952755905511810774, -0.1292274648535930714 ) ) ;
#59704=CARTESIAN_POINT ( 'NONE',  ( 1.377952755905512472, 0.2952755905511811885, 0.000000000000000000 ) ) ;
#59706=CARTESIAN_POINT ( 'NONE',  ( 0.01968503937007957949, -0.4536011799217368745, -0.2665933059059886201 ) ) ;
#59710=CARTESIAN_POINT ( 'NONE',  ( -0.3608923884514428360, -0.5511811023622048555, -0.09757992244046775898 ) ) ;
#59711=CARTESIAN_POINT ( 'NONE',  ( 0.1640419947506569498, -0.3162353388693409650, -0.4822834645669289433 ) ) ;
#59713=CARTESIAN_POINT ( 'NONE',  ( -0.3543307086614165824, -0.6692913385826771977, 8.415575281601705876E-17 ) ) ;
#59714=CARTESIAN_POINT ( 'NONE',  ( -0.4068241469816267775, 0.05413385826771626580, -0.4176697321401330321 ) ) ;
#59715=CARTESIAN_POINT ( 'NONE',  ( -0.7939632545931750718, -0.05778040916215560624, -0.4822834645669293319 ) ) ;
#59716=CARTESIAN_POINT ( 'NONE',  ( -0.9973753280839886548, -0.6046776061558809534, -0.2411417322834644161 ) ) ;
#59718=CARTESIAN_POINT ( 'NONE',  ( 1.397637795275591177, 0.07958543189024071263, -0.2665933059059888421 ) ) ;
#59719=CARTESIAN_POINT ( 'NONE',  ( 1.614173228346456712, 0.4410134679336843999, 0.1372047244094478646 ) ) ;
#59721=CARTESIAN_POINT ( 'NONE',  ( 0.4855643044619428750, -0.004921259842519576551, 0.3153832671262227771 ) ) ;
#59722=CARTESIAN_POINT ( 'NONE',  ( 0.4790026246719168435, -0.3162353388693409650, -0.4822834645669289433 ) ) ;
#59723=CARTESIAN_POINT ( 'NONE',  ( 0.4330708661417329575, 0.2952755905511811885, 0.000000000000000000 ) ) ;
#59724=EDGE_LOOP ( 'NONE', ( #27610, #20889, #54952, #34884 ) ) ;
#59726=CARTESIAN_POINT ( 'NONE',  ( -0.5627669687126057863, 0.02791078216816347476, -0.4328096321851898631 ) ) ;
#59729=CARTESIAN_POINT ( 'NONE',  ( -0.6167979002624665030, 0.05413385826771666132, 0.4176697321401328100 ) ) ;
#59733=CARTESIAN_POINT ( 'NONE',  ( 1.640419947506562393, -0.4281496062992124485, 0.4176697321401328655 ) ) ;
#59734=CARTESIAN_POINT ( 'NONE',  ( 0.7480314960629927956, -0.6692913385826771977, 8.415575281601705876E-17 ) ) ;
#59735=CARTESIAN_POINT ( 'NONE',  ( 1.141732283464567788, -0.6692913385826771977, 8.415575281601705876E-17 ) ) ;
#59736=CARTESIAN_POINT ( 'NONE',  ( -0.2821522309711278487, -0.5511811023622048555, -0.09757992244046775898 ) ) ;
#59737=CARTESIAN_POINT ( 'NONE',  ( 0.4986876640419954376, 0.2306618581243848609, 0.2411417322834645549 ) ) ;
#59739=CARTESIAN_POINT ( 'NONE',  ( -0.05249343832020911260, 0.1283753931104748280, 0.1820866141732283561 ) ) ;
#59740=CARTESIAN_POINT ( 'NONE',  ( -0.2230971128608915943, -0.4281496062992127816, -0.4176697321401328100 ) ) ;
#59742=CARTESIAN_POINT ( 'NONE',  ( -1.548556430446193399, 0.2306618581243848609, 0.2411417322834645549 ) ) ;
#59743=CARTESIAN_POINT ( 'NONE',  ( -0.03280839895013062252, -0.5511811023622046335, 0.09757992244046803654 ) ) ;
#59744=CARTESIAN_POINT ( 'NONE',  ( 1.646981627296588035, -0.2845877964562159024, 0.3641732283464567677 ) ) ;
#59745=CARTESIAN_POINT ( 'NONE',  ( -0.8595800524934373854, -0.3162353388693409650, -0.4822834645669289433 ) ) ;
#59746=CARTESIAN_POINT ( 'NONE',  ( -0.7545931758530176614, -0.5511811023622048555, -0.09757992244046775898 ) ) ;
#59747=CARTESIAN_POINT ( 'NONE',  ( 1.600415083108465142, 1.509172534626478823, -0.1324231768467331039 ) ) ;
#59748=CARTESIAN_POINT ( 'NONE',  ( -0.8792650918635160906, 0.05413385826771626580, -0.4176697321401330321 ) ) ;
#59749=CARTESIAN_POINT ( 'NONE',  ( -0.5577427821522301654, -0.3162353388693405765, 0.4822834645669290543 ) ) ;
#59750=CARTESIAN_POINT ( 'NONE',  ( 0.03937007874015833325, -0.6692913385826771977, 8.415575281601705876E-17 ) ) ;
#59754=CARTESIAN_POINT ( 'NONE',  ( 0.9251968503937015864, 0.07958543189024071263, -0.2665933059059888421 ) ) ;
#59755=CARTESIAN_POINT ( 'NONE',  ( 1.548556430446194954, -0.6046776061558807314, 0.2411417322834647770 ) ) ;
#59756=CARTESIAN_POINT ( 'NONE',  ( -1.417322834645668772, -0.1870078740157479769, 0.3641732283464567677 ) ) ;
#59757=CARTESIAN_POINT ( 'NONE',  ( 1.069553805774278832, 0.2952755905511810774, -0.1292274648535930714 ) ) ;
#59758=CARTESIAN_POINT ( 'NONE',  ( -1.122047244094487306, -0.4536011799217367080, 0.2665933059059888421 ) ) ;
#59759=CARTESIAN_POINT ( 'NONE',  ( -0.6496062992125976043, -0.5400638737290844871, 0.3530559997133364547 ) ) ;
#59760=CARTESIAN_POINT ( 'NONE',  ( 0.1509186351706045259, -0.08942795157528024563, -0.3641732283464568787 ) ) ;
#59761=CARTESIAN_POINT ( 'NONE',  ( 1.614173228346457378, 0.2753471884572478157, 0.1372047244094478646 ) ) ;
#59762=CARTESIAN_POINT ( 'NONE',  ( 1.259842519685040019, -0.1870078740157479769, 0.3641732283464567677 ) ) ;
#59764=CARTESIAN_POINT ( 'NONE',  ( 0.4002624671916016896, -0.05778040916215522460, 0.4822834645669289988 ) ) ;
#59766=CARTESIAN_POINT ( 'NONE',  ( -0.7480314960629914633, 0.2952755905511811885, 0.000000000000000000 ) ) ;
#59768=CARTESIAN_POINT ( 'NONE',  ( 0.8267716535433077274, 0.1771653543307087630, 0.000000000000000000 ) ) ;
#59769=CARTESIAN_POINT ( 'NONE',  ( 0.3280839895013130669, -0.4281496062992127816, -0.4176697321401328100 ) ) ;
#59770=CARTESIAN_POINT ( 'NONE',  ( -0.09186351706036663400, -0.4281496062992124485, 0.4176697321401328655 ) ) ;
#59771=CARTESIAN_POINT ( 'NONE',  ( -0.1706036745406816491, -0.004921259842519870586, -0.3153832671262229437 ) ) ;
#59773=CARTESIAN_POINT ( 'NONE',  ( 0.1246719160104994284, 0.1771653543307087075, -0.09757992244046823083 ) ) ;
#59774=CARTESIAN_POINT ( 'NONE',  ( 0.6561679790026253567, -0.6046776061558809534, -0.2411417322834644161 ) ) ;
#59775=CARTESIAN_POINT ( 'NONE',  ( -0.6955380577427815458, -0.3690944881889765550, -0.3153832671262227771 ) ) ;
#59778=CARTESIAN_POINT ( 'NONE',  ( -0.9448818897637790704, -0.1870078740157480879, -0.4822834645669291653 ) ) ;
#59780=ORIENTED_EDGE ( 'NONE', *, *, #12082, .T. ) ;
#59781=CARTESIAN_POINT ( 'NONE',  ( -0.9908136482939626788, -0.5511811023622048555, -0.09757992244046775898 ) ) ;
#59782=CARTESIAN_POINT ( 'NONE',  ( -0.1902887139107604098, -0.6692913385826771977, 0.1292274648535927661 ) ) ;
#59784=CARTESIAN_POINT ( 'NONE',  ( -0.7086614173228339419, -0.1870078740157479769, 0.4822834645669291653 ) ) ;
#59786=CARTESIAN_POINT ( 'NONE',  ( 1.092353285368624860, -4.408777212815537393E-16, -0.4445507791589063395 ) ) ;
#59787=CARTESIAN_POINT ( 'NONE',  ( 1.010498687664042716, 0.05413385826771626580, -0.4176697321401330321 ) ) ;
#59788=CARTESIAN_POINT ( 'NONE',  ( 0.9514435695538062676, -0.3162353388693409650, -0.4822834645669289433 ) ) ;
#59791=CARTESIAN_POINT ( 'NONE',  ( -1.404199475065615932, 0.05413385826771666132, 0.4176697321401328100 ) ) ;
#59795=CARTESIAN_POINT ( 'NONE',  ( -0.7152230971128602510, -0.2845877964562159024, 0.3641732283464567677 ) ) ;
#59798=CARTESIAN_POINT ( 'NONE',  ( 0.7677165354330716118, -0.5400638737290844871, 0.3530559997133364547 ) ) ;
#59799=CARTESIAN_POINT ( 'NONE',  ( 0.02624671916010564918, 0.2306618581243848609, 0.2411417322834645549 ) ) ;
#59800=CARTESIAN_POINT ( 'NONE',  ( -0.4855643044619415427, 0.05413385826771626580, -0.4176697321401330321 ) ) ;
#59801=CARTESIAN_POINT ( 'NONE',  ( 1.351706036745407680, 0.05413385826771666132, 0.4176697321401328100 ) ) ;
#59802=CARTESIAN_POINT ( 'NONE',  ( -0.8792650918635160906, -0.3690944881889763329, 0.3153832671262228327 ) ) ;
#59804=CARTESIAN_POINT ( 'NONE',  ( 0.8858267716535438430, 0.1660481256975885056, 0.3530559997133364547 ) ) ;
#59805=CARTESIAN_POINT ( 'NONE',  ( 0.3805774278215230400, -0.004921259842519870586, -0.3153832671262229437 ) ) ;
#59806=CARTESIAN_POINT ( 'NONE',  ( -0.5446194225721777693, -0.05778040916215522460, 0.4822834645669289988 ) ) ;
#59808=CARTESIAN_POINT ( 'NONE',  ( -1.292650918635170010, 0.2952755905511810774, -0.1292274648535930714 ) ) ;
#59810=CARTESIAN_POINT ( 'NONE',  ( 1.456692913385827515, -0.6692913385826771977, 8.415575281601705876E-17 ) ) ;
#59811=CARTESIAN_POINT ( 'NONE',  ( 1.233595800524935227, 0.1283753931104746893, -0.1820866141732285504 ) ) ;
#59814=CARTESIAN_POINT ( 'NONE',  ( -0.09842519685039295696, -0.5400638737290844871, 0.3530559997133364547 ) ) ;
#59816=CARTESIAN_POINT ( 'NONE',  ( 1.017060367454068581, -0.08942795157528024563, -0.3641732283464568787 ) ) ;
#59817=CARTESIAN_POINT ( 'NONE',  ( -1.095800524934382292, -0.05778040916215522460, 0.4822834645669289988 ) ) ;
#59818=CARTESIAN_POINT ( 'NONE',  ( 1.062992125984252745, -0.6692913385826771977, 8.415575281601705876E-17 ) ) ;
#59819=CARTESIAN_POINT ( 'NONE',  ( 0.7020997375328090762, -0.05778040916215560624, -0.4822834645669293319 ) ) ;
#59820=CARTESIAN_POINT ( 'NONE',  ( 0.2624671916010504757, -0.6046776061558809534, -0.2411417322834644161 ) ) ;
#59821=CARTESIAN_POINT ( 'NONE',  ( -0.5249343832020990641, 0.2306618581243848609, 0.2411417322834645549 ) ) ;
#59823=CARTESIAN_POINT ( 'NONE',  ( -1.384514435695537005, 0.2952755905511811885, 0.1292274648535926551 ) ) ;
#59824=CARTESIAN_POINT ( 'NONE',  ( -0.4527559055118102749, -0.5400638737290845981, -0.3530559997133363437 ) ) ;
#59825=CARTESIAN_POINT ( 'NONE',  ( -0.5118110236220466680, -0.6692913385826771977, 8.415575281601705876E-17 ) ) ;
#59826=CARTESIAN_POINT ( 'NONE',  ( -0.5839895013123351797, -0.5511811023622046335, 0.09757992244046803654 ) ) ;
#59830=CARTESIAN_POINT ( 'NONE',  ( -0.3608923884514428360, -0.6692913385826773087, -0.1292274648535924053 ) ) ;
#59832=CARTESIAN_POINT ( 'NONE',  ( 0.6430446194225728496, 0.05413385826771666132, 0.4176697321401328100 ) ) ;
#59836=CARTESIAN_POINT ( 'NONE',  ( -0.06561679790026180015, 0.05413385826771666132, 0.4176697321401328100 ) ) ;
#59837=CARTESIAN_POINT ( 'NONE',  ( 1.069553805774278832, 0.1771653543307087075, -0.09757992244046823083 ) ) ;
#59838=CARTESIAN_POINT ( 'NONE',  ( 0.6962418744208975774, 2.409604939980833412E-17, -0.3464511005275205946 ) ) ;
#59840=CARTESIAN_POINT ( 'NONE',  ( 1.332020997375329197, -0.2845877964562159024, 0.3641732283464567677 ) ) ;
#59841=CARTESIAN_POINT ( 'NONE',  ( 1.128608923884514947, 0.2306618581243848609, 0.2411417322834645549 ) ) ;
#59844=CARTESIAN_POINT ( 'NONE',  ( -0.2887139107611542133, 0.2306618581243848609, 0.2411417322834645549 ) ) ;
#59845=CARTESIAN_POINT ( 'NONE',  ( -1.528871391076114250, -0.6692913385826771977, 0.1292274648535927661 ) ) ;
#59846=CARTESIAN_POINT ( 'NONE',  ( -1.660104986876639543, -0.05778040916215560624, -0.4822834645669293319 ) ) ;
#59847=CARTESIAN_POINT ( 'NONE',  ( 0.01968503937007930540, 0.1660481256975885056, 0.3530559997133364547 ) ) ;
#59849=CARTESIAN_POINT ( 'NONE',  ( 1.410761154855643795, -0.05778040916215560624, -0.4822834645669293319 ) ) ;
#59850=CARTESIAN_POINT ( 'NONE',  ( 0.4199475065616803948, -0.6046776061558809534, -0.2411417322834644161 ) ) ;
#59851=CARTESIAN_POINT ( 'NONE',  ( 0.7152230971128616943, -0.08942795157527998196, 0.3641732283464567121 ) ) ;
#59853=CARTESIAN_POINT ( 'NONE',  ( 0.4658792650918641698, -0.08942795157528024563, -0.3641732283464568787 ) ) ;
#59854=CARTESIAN_POINT ( 'NONE',  ( -1.043307086614172929, 0.1012011053420775880, -0.2882089793578257453 ) ) ;
#59856=CARTESIAN_POINT ( 'NONE',  ( 0.8661417322834653598, -0.1870078740157479769, 0.4822834645669291653 ) ) ;
#59857=ADVANCED_FACE ( 'NONE', ( #12313 ), #75472, .F. ) ;
#59861=CARTESIAN_POINT ( 'NONE',  ( -0.1115485564304456306, 0.1771653543307087075, -0.09757992244046823083 ) ) ;
#59862=CARTESIAN_POINT ( 'NONE',  ( 0.3280839895013130669, -0.4281496062992127816, -0.4176697321401328100 ) ) ;
#59863=CARTESIAN_POINT ( 'NONE',  ( 1.325459317585302665, -0.3690944881889763329, 0.3153832671262228327 ) ) ;
#59864=CARTESIAN_POINT ( 'NONE',  ( -0.9711286089238838626, -0.5023911411419708095, 0.1820866141732285504 ) ) ;
#59865=CARTESIAN_POINT ( 'NONE',  ( -0.9186351706036736120, 0.2306618581243848609, 0.2411417322834645549 ) ) ;
#59866=CARTESIAN_POINT ( 'NONE',  ( -1.660104986876639543, -0.05778040916215560624, -0.4822834645669293319 ) ) ;
#59867=CARTESIAN_POINT ( 'NONE',  ( 0.3280839895013130669, -0.4281496062992127816, -0.4176697321401328100 ) ) ;
#59868=CARTESIAN_POINT ( 'NONE',  ( 1.410761154855643795, -0.05778040916215560624, -0.4822834645669293319 ) ) ;
#59870=CARTESIAN_POINT ( 'NONE',  ( 0.3871391076115492380, -0.05778040916215560624, -0.4822834645669293319 ) ) ;
#59872=CARTESIAN_POINT ( 'NONE',  ( 1.660104986876641320, -0.05778040916215522460, 0.4822834645669289988 ) ) ;
#59873=CARTESIAN_POINT ( 'NONE',  ( 1.312335958005250269, -0.6046776061558807314, 0.2411417322834647770 ) ) ;
#59874=CARTESIAN_POINT ( 'NONE',  ( -1.581364829396324945, -0.2845877964562159024, 0.3641732283464567677 ) ) ;
#59875=CARTESIAN_POINT ( 'NONE',  ( 1.338582677165355062, -0.1870078740157479769, 0.3641732283464567677 ) ) ;
#59876=CARTESIAN_POINT ( 'NONE',  ( -1.200787401574802349, -0.4536011799217367080, 0.2665933059059888421 ) ) ;
#59877=CARTESIAN_POINT ( 'NONE',  ( -0.8398950131233585692, 0.1283753931104748280, 0.1820866141732283561 ) ) ;
#59879=CARTESIAN_POINT ( 'NONE',  ( 0.6036745406824153282, -0.5023911411419708095, 0.1820866141732285504 ) ) ;
#59880=CARTESIAN_POINT ( 'NONE',  ( -0.08530183727034056085, -0.3162353388693405765, 0.4822834645669290543 ) ) ;
#59881=CARTESIAN_POINT ( 'NONE',  ( 1.102362204724410155, -0.1870078740157479769, 0.4822834645669291653 ) ) ;
#59882=CARTESIAN_POINT ( 'NONE',  ( 0.06561679790026316017, -0.4281496062992124485, 0.4176697321401328655 ) ) ;
#59883=CARTESIAN_POINT ( 'NONE',  ( 0.2624671916010504757, -0.5023911411419708095, -0.1820866141732282451 ) ) ;
#59884=CARTESIAN_POINT ( 'NONE',  ( 1.227034120734908917, -0.6692913385826771977, 0.1292274648535927661 ) ) ;
#59885=LINE ( 'NONE', #14469, #7039 ) ;
#59886=CARTESIAN_POINT ( 'NONE',  ( -1.036745406824146176, 0.05413385826771626580, -0.4176697321401330321 ) ) ;
#59889=CARTESIAN_POINT ( 'NONE',  ( -1.023622047244093558, -0.1870078740157479769, 0.4822834645669291653 ) ) ;
#59890=VECTOR ( 'NONE', #67032, 39.37007874015748854 ) ;
#59892=CARTESIAN_POINT ( 'NONE',  ( -0.1771653543307080136, -0.5400638737290844871, 0.3530559997133364547 ) ) ;
#59898=CARTESIAN_POINT ( 'NONE',  ( -1.272965879265091305, -0.3690944881889763329, 0.3153832671262228327 ) ) ;
#59900=CARTESIAN_POINT ( 'NONE',  ( -1.594488188976377563, -0.5400638737290844871, 0.3530559997133364547 ) ) ;
#59903=CARTESIAN_POINT ( 'NONE',  ( -0.1181102362204717315, -0.6692913385826771977, 8.415575281601705876E-17 ) ) ;
#59904=CARTESIAN_POINT ( 'NONE',  ( -0.5052493438320203589, -0.5511811023622046335, 0.09757992244046803654 ) ) ;
#59905=CARTESIAN_POINT ( 'NONE',  ( 1.049868766404200127, -0.6046776061558809534, -0.2411417322834644161 ) ) ;
#59906=CARTESIAN_POINT ( 'NONE',  ( 0.2493438320209980519, -0.4281496062992127816, -0.4176697321401328100 ) ) ;
#59907=CARTESIAN_POINT ( 'NONE',  ( -0.3049517105654738214, -2.191421614605370878E-15, 0.4445507791589071167 ) ) ;
#59910=CARTESIAN_POINT ( 'NONE',  ( 1.069553805774278832, 0.2952755905511810774, -0.1292274648535930714 ) ) ;
#59911=CARTESIAN_POINT ( 'NONE',  ( 0.1574803149606306130, -0.1870078740157479769, 0.4822834645669291653 ) ) ;
#59912=CARTESIAN_POINT ( 'NONE',  ( -1.220472440944881054, -0.6692913385826771977, 8.415575281601705876E-17 ) ) ;
#59913=CARTESIAN_POINT ( 'NONE',  ( 1.601049868766404982, 0.2306618581243848609, 0.2411417322834645549 ) ) ;
#59914=CARTESIAN_POINT ( 'NONE',  ( 0.9776902887139113929, -0.6692913385826773087, -0.1292274648535924053 ) ) ;
#59916=CARTESIAN_POINT ( 'NONE',  ( 0.01968503937007930540, 0.1660481256975885056, 0.3530559997133364547 ) ) ;
#59917=CARTESIAN_POINT ( 'NONE',  ( 0.6561679790026253567, -0.6046776061558809534, -0.2411417322834644161 ) ) ;
#59918=CARTESIAN_POINT ( 'NONE',  ( -0.1640419947506553400, -0.05778040916215560624, -0.4822834645669293319 ) ) ;
#59919=CARTESIAN_POINT ( 'NONE',  ( 0.6758530183727039509, -0.5511811023622046335, 0.09757992244046803654 ) ) ;
#59920=CARTESIAN_POINT ( 'NONE',  ( -1.135170603674539924, -0.6692913385826771977, 0.1292274648535927661 ) ) ;
#59921=CARTESIAN_POINT ( 'NONE',  ( -1.614173228346456268, -0.6692913385826771977, 8.415575281601705876E-17 ) ) ;
#59922=CARTESIAN_POINT ( 'NONE',  ( 0.7217847769028878924, -0.4281496062992127816, -0.4176697321401328100 ) ) ;
#59925=ORIENTED_EDGE ( 'NONE', *, *, #34284, .F. ) ;
#59927=VERTEX_POINT ( 'NONE', #11494 ) ;
#59928=CARTESIAN_POINT ( 'NONE',  ( 0.9383202099737538715, -0.05778040916215560624, -0.4822834645669293319 ) ) ;
#59929=CARTESIAN_POINT ( 'NONE',  ( 0.3477690288713918276, 0.1771653543307087630, 0.09757992244046791164 ) ) ;
#59937=CARTESIAN_POINT ( 'NONE',  ( -0.4199475065616791736, 0.2306618581243847221, -0.2411417322834647770 ) ) ;
#59938=CARTESIAN_POINT ( 'NONE',  ( 1.220472440944882386, -0.6692913385826771977, 8.415575281601705876E-17 ) ) ;
#59940=CARTESIAN_POINT ( 'NONE',  ( -1.384514435695537005, 0.2952755905511811885, 0.1292274648535926551 ) ) ;
#59943=CARTESIAN_POINT ( 'NONE',  ( 1.561679790026247350, -0.004921259842519870586, -0.3153832671262229437 ) ) ;
#59945=CARTESIAN_POINT ( 'NONE',  ( -1.515748031496062076, -0.4536011799217367080, 0.2665933059059888421 ) ) ;
#59946=CARTESIAN_POINT ( 'NONE',  ( -1.410761154855641575, -0.3162353388693409650, -0.4822834645669289433 ) ) ;
#59947=CARTESIAN_POINT ( 'NONE',  ( 0.1968503937007881344, -0.6692913385826771977, 8.415575281601705876E-17 ) ) ;
#59949=VERTEX_POINT ( 'NONE', #43855 ) ;
#59950=CARTESIAN_POINT ( 'NONE',  ( 1.601049868766404982, -0.6046776061558809534, -0.2411417322834644161 ) ) ;
#59952=CARTESIAN_POINT ( 'NONE',  ( -0.5839895013123351797, 0.1771653543307087075, -0.09757992244046823083 ) ) ;
#59953=CARTESIAN_POINT ( 'NONE',  ( 0.9514435695538062676, -0.3162353388693409650, -0.4822834645669289433 ) ) ;
#59954=CARTESIAN_POINT ( 'NONE',  ( -1.515748031496062076, 0.1660481256975883668, -0.3530559997133364547 ) ) ;
#59956=CARTESIAN_POINT ( 'NONE',  ( -0.9908136482939626788, -0.5511811023622048555, -0.09757992244046775898 ) ) ;
#59957=CARTESIAN_POINT ( 'NONE',  ( -1.509186351706035767, -0.3690944881889763329, 0.3153832671262228327 ) ) ;
#59959=CARTESIAN_POINT ( 'NONE',  ( 0.5905511811023629321, -0.6692913385826771977, 8.415575281601705876E-17 ) ) ;
#59960=CARTESIAN_POINT ( 'NONE',  ( -0.9973753280839886548, 0.1283753931104748280, 0.1820866141732283561 ) ) ;
#59961=CARTESIAN_POINT ( 'NONE',  ( -0.2296587926509179312, -0.2845877964562161244, -0.3641732283464567121 ) ) ;
#59962=CARTESIAN_POINT ( 'NONE',  ( -0.1509186351706028884, -0.05778040916215522460, 0.4822834645669289988 ) ) ;
#59963=CARTESIAN_POINT ( 'NONE',  ( -1.548556430446193399, -0.5023911411419708095, -0.1820866141732282451 ) ) ;
#59965=CARTESIAN_POINT ( 'NONE',  ( 0.5511811023622054106, -0.1870078740157480879, -0.4822834645669291653 ) ) ;
#59966=CARTESIAN_POINT ( 'NONE',  ( 0.4056338187708066201, 5.789745203009502317E-16, 0.3627989612356145588 ) ) ;
#59968=CARTESIAN_POINT ( 'NONE',  ( -0.7283464566929126471, 0.1660481256975883668, -0.3530559997133364547 ) ) ;
#59969=CARTESIAN_POINT ( 'NONE',  ( -0.3346456692913377662, -0.4536011799217367080, 0.2665933059059888421 ) ) ;
#59971=CARTESIAN_POINT ( 'NONE',  ( -1.187664041994749731, -0.3162353388693405765, 0.4822834645669290543 ) ) ;
#59972=CARTESIAN_POINT ( 'NONE',  ( 0.4921259842519691285, -0.4536011799217368745, -0.2665933059059886201 ) ) ;
#59973=CARTESIAN_POINT ( 'NONE',  ( -0.8661417322834640276, -0.1870078740157480601, -0.3641732283464567677 ) ) ;
#59974=CARTESIAN_POINT ( 'NONE',  ( -1.253280839895012377, -0.05778040916215522460, 0.4822834645669289988 ) ) ;
#59975=CARTESIAN_POINT ( 'NONE',  ( -1.601049868766403650, -0.6046776061558807314, 0.2411417322834647770 ) ) ;
#59976=CARTESIAN_POINT ( 'NONE',  ( 1.227034120734908917, 0.2952755905511810774, -0.1292274648535930714 ) ) ;
#59978=CARTESIAN_POINT ( 'NONE',  ( 0.6889763779527566800, -0.4536011799217367080, 0.2665933059059888421 ) ) ;
#59979=CARTESIAN_POINT ( 'NONE',  ( 0.2821522309711292364, 0.2952755905511810774, -0.1292274648535930714 ) ) ;
#59981=CARTESIAN_POINT ( 'NONE',  ( 0.5419760673063064305, 1.535433070866141447, -0.4915354330708657793 ) ) ;
#59982=CARTESIAN_POINT ( 'NONE',  ( 1.528871391076116026, -0.5511811023622048555, -0.09757992244046775898 ) ) ;
#59985=CARTESIAN_POINT ( 'NONE',  ( -1.325459317585300889, -0.004921259842519576551, 0.3153832671262227771 ) ) ;
#59986=CARTESIAN_POINT ( 'NONE',  ( -0.2952755905511803003, -0.5400638737290845981, -0.3530559997133363437 ) ) ;
#59987=CARTESIAN_POINT ( 'NONE',  ( 0.4658792650918640033, -0.3162353388693405765, 0.4822834645669290543 ) ) ;
#59989=CARTESIAN_POINT ( 'NONE',  ( -1.561679790026246017, -0.004921259842519576551, 0.3153832671262227771 ) ) ;
#59991=CARTESIAN_POINT ( 'NONE',  ( -1.246719160104986512, 0.05413385826771666132, 0.4176697321401328100 ) ) ;
#59994=CARTESIAN_POINT ( 'NONE',  ( 0.3215223097112867578, -0.3162353388693409650, -0.4822834645669289433 ) ) ;
#59995=CARTESIAN_POINT ( 'NONE',  ( 0.01312335958005323398, -0.4281496062992127816, -0.4176697321401328100 ) ) ;
#59996=CARTESIAN_POINT ( 'NONE',  ( 1.115485564304462551, 0.05413385826771666132, 0.4176697321401328100 ) ) ;
#60002=CARTESIAN_POINT ( 'NONE',  ( 0.07874015748031558404, -0.1870078740157480601, -0.3641732283464567677 ) ) ;
#60003=CARTESIAN_POINT ( 'NONE',  ( -0.1181102362204717315, 0.2952755905511811885, 0.000000000000000000 ) ) ;
#60004=CARTESIAN_POINT ( 'NONE',  ( 0.8005249343832027131, 0.05413385826771666132, 0.4176697321401328100 ) ) ;
#60006=CARTESIAN_POINT ( 'NONE',  ( -0.03937007874015669567, 0.1771653543307087630, 0.000000000000000000 ) ) ;
#60007=CARTESIAN_POINT ( 'NONE',  ( -1.318897637795274802, 0.1660481256975885056, 0.3530559997133364547 ) ) ;
#60008=CARTESIAN_POINT ( 'NONE',  ( 1.601049868766404982, 0.2306618581243848609, 0.2411417322834645549 ) ) ;
#60014=CARTESIAN_POINT ( 'NONE',  ( 1.535433070866142335, -0.6692913385826771977, 8.415575281601705876E-17 ) ) ;
#60015=CARTESIAN_POINT ( 'NONE',  ( 1.594488188976378673, 0.07958543189024085140, 0.2665933059059887866 ) ) ;
#60016=CARTESIAN_POINT ( 'NONE',  ( -1.076115485564303809, -0.5023911411419708095, -0.1820866141732282451 ) ) ;
#60017=CARTESIAN_POINT ( 'NONE',  ( -0.9908136482939626788, 0.2952755905511811885, 0.1292274648535926551 ) ) ;
#60019=CARTESIAN_POINT ( 'NONE',  ( -2.795275590551183686, 1.299212598425198095, -1.990688069879260956E-16 ) ) ;
#60020=CARTESIAN_POINT ( 'NONE',  ( 1.417322834645670104, -0.1870078740157480879, -0.4822834645669291653 ) ) ;
#60021=CARTESIAN_POINT ( 'NONE',  ( -1.699475065616797398, 0.2952755905511811885, 0.1292274648535926551 ) ) ;
#60022=CARTESIAN_POINT ( 'NONE',  ( -0.2559055118110230564, 0.1660481256975883668, -0.3530559997133364547 ) ) ;
#60023=CARTESIAN_POINT ( 'NONE',  ( -0.3346456692913377662, -0.5400638737290844871, 0.3530559997133364547 ) ) ;
#60024=CARTESIAN_POINT ( 'NONE',  ( -1.233595800524933894, -0.6046776061558809534, -0.2411417322834644161 ) ) ;
#60026=CARTESIAN_POINT ( 'NONE',  ( 0.7545931758530188826, -0.6692913385826771977, 0.1292274648535927661 ) ) ;
#60028=CARTESIAN_POINT ( 'NONE',  ( -1.364829396325458521, -0.5023911411419708095, 0.1820866141732285504 ) ) ;
#60031=ORIENTED_EDGE ( 'NONE', *, *, #28480, .T. ) ;
#60032=LINE ( 'NONE', #8280, #30081 ) ;
#60033=CARTESIAN_POINT ( 'NONE',  ( -1.587926509186350810, -0.4281496062992124485, 0.4176697321401328655 ) ) ;
#60034=CARTESIAN_POINT ( 'NONE',  ( -1.345144356955379816, -0.3162353388693405765, 0.4822834645669290543 ) ) ;
#60036=CARTESIAN_POINT ( 'NONE',  ( -1.601049868766403650, -0.6046776061558807314, 0.2411417322834647770 ) ) ;
#60038=CARTESIAN_POINT ( 'NONE',  ( 0.4593175853018380828, 0.05413385826771626580, -0.4176697321401330321 ) ) ;
#60041=CARTESIAN_POINT ( 'NONE',  ( -0.08530183727034056085, -0.2845877964562159024, 0.3641732283464567677 ) ) ;
#60042=CARTESIAN_POINT ( 'NONE',  ( -0.6561679790026240244, -0.5023911411419708095, 0.1820866141732285504 ) ) ;
#60043=CARTESIAN_POINT ( 'NONE',  ( -1.246719160104985846, -0.4281496062992127816, -0.4176697321401328100 ) ) ;
#60044=CARTESIAN_POINT ( 'NONE',  ( 0.8005249343832027131, 0.05413385826771666132, 0.4176697321401328100 ) ) ;
#60045=CARTESIAN_POINT ( 'NONE',  ( -0.9317585301837263412, -0.4281496062992127816, -0.4176697321401328100 ) ) ;
#60047=VERTEX_POINT ( 'NONE', #64062 ) ;
#60048=CARTESIAN_POINT ( 'NONE',  ( -1.305774278215222184, 0.2952755905511811885, 0.1292274648535926551 ) ) ;
#60049=CARTESIAN_POINT ( 'NONE',  ( -1.607611548556429737, -0.5511811023622046335, 0.09757992244046803654 ) ) ;
#60052=FACE_OUTER_BOUND ( 'NONE', #69750, .T. ) ;
#60056=CARTESIAN_POINT ( 'NONE',  ( -0.3740157480314953431, 0.1660481256975885056, 0.3530559997133364547 ) ) ;
#60057=CARTESIAN_POINT ( 'NONE',  ( -1.305774278215222184, 0.1771653543307087630, 0.09757992244046791164 ) ) ;
#60059=AXIS2_PLACEMENT_3D ( 'NONE', #21021, #7567, #33239 ) ;
#60061=CARTESIAN_POINT ( 'NONE',  ( -0.7461015469959760837, 2.202998601756388730, -0.5309055118110235227 ) ) ;
#60063=CARTESIAN_POINT ( 'NONE',  ( -1.555118110236219930, 0.1660481256975885056, 0.3530559997133364547 ) ) ;
#60064=CARTESIAN_POINT ( 'NONE',  ( -0.3740157480314953431, -0.5400638737290845981, -0.3530559997133363437 ) ) ;
#60066=CARTESIAN_POINT ( 'NONE',  ( 0.5052493438320215802, 0.1771653543307087630, 0.09757992244046791164 ) ) ;
#60067=DIRECTION ( 'NONE',  ( -1.000000000000000000, -2.312964634635742464E-16, 0.000000000000000000 ) ) ;
#60068=CARTESIAN_POINT ( 'NONE',  ( 0.3280839895013130669, -0.3690944881889765550, -0.3153832671262227771 ) ) ;
#60069=CARTESIAN_POINT ( 'NONE',  ( 1.128608923884514947, 0.1283753931104748280, 0.1820866141732283561 ) ) ;
#60070=CARTESIAN_POINT ( 'NONE',  ( 1.154855643044620184, 0.2306618581243847221, -0.2411417322834647770 ) ) ;
#60071=CARTESIAN_POINT ( 'NONE',  ( -0.3412073490813641308, 0.1283753931104746893, -0.1820866141732285504 ) ) ;
#60073=CARTESIAN_POINT ( 'NONE',  ( -1.233595800524933894, -0.6046776061558809534, -0.2411417322834644161 ) ) ;
#60074=CARTESIAN_POINT ( 'NONE',  ( -0.1246719160104980823, 0.1771653543307087630, 0.09757992244046791164 ) ) ;
#60075=CARTESIAN_POINT ( 'NONE',  ( -1.187664041994749731, -0.2845877964562159024, 0.3641732283464567677 ) ) ;
#60077=CARTESIAN_POINT ( 'NONE',  ( -0.7283464566929126471, -0.4536011799217367080, 0.2665933059059888421 ) ) ;
#60080=CARTESIAN_POINT ( 'NONE',  ( -0.1049868766404193215, -0.6046776061558807314, 0.2411417322834647770 ) ) ;
#60081=CARTESIAN_POINT ( 'NONE',  ( 1.653543307086614789, -0.1870078740157479769, 0.3641732283464567677 ) ) ;
#60082=CARTESIAN_POINT ( 'NONE',  ( 0.3740157480314966754, 0.07958543189024071263, -0.2665933059059888421 ) ) ;
#60083=CARTESIAN_POINT ( 'NONE',  ( -0.4133858267716528645, 0.07958543189024071263, -0.2665933059059888421 ) ) ;
#60084=CARTESIAN_POINT ( 'NONE',  ( -0.3280839895013117347, 0.05413385826771626580, -0.4176697321401330321 ) ) ;
#60085=CARTESIAN_POINT ( 'NONE',  ( -1.627296587926508442, -0.6046776061558809534, -0.2411417322834644161 ) ) ;
#60086=CARTESIAN_POINT ( 'NONE',  ( -1.030183727034119867, -0.2845877964562159024, 0.3641732283464567677 ) ) ;
#60088=CARTESIAN_POINT ( 'NONE',  ( 0.4265091863517067594, 0.2952755905511811885, 0.1292274648535926551 ) ) ;
#60092=CARTESIAN_POINT ( 'NONE',  ( -0.2230971128608915943, -0.3690944881889765550, -0.3153832671262227771 ) ) ;
#60093=CARTESIAN_POINT ( 'NONE',  ( -0.05249343832020938322, -0.6046776061558809534, -0.2411417322834644161 ) ) ;
#60094=CARTESIAN_POINT ( 'NONE',  ( -1.607611548556429737, 0.2952755905511810774, -0.1292274648535930714 ) ) ;
#60095=CARTESIAN_POINT ( 'NONE',  ( -1.535433070866141225, -0.5511811023622047445, 6.969142054262312111E-17 ) ) ;
#60096=CARTESIAN_POINT ( 'NONE',  ( 1.351706036745407680, 0.05413385826771666132, 0.4176697321401328100 ) ) ;
#60097=( BOUNDED_SURFACE ( )  B_SPLINE_SURFACE ( 1, 2, ( 
 ( #66133, #21508, #73700, #53482, #72858, #53892, #15206, #9713, #40043, #67379, #61049, #16040, #2574, #79192, #53060, #28651, #34972, #72029, #54311, #47166, #8882, #40867, #2155, #60635, #65729, #14385, #21922, #66549, #34140, #35384, #8062, #33723, #59385, #34558, #72448, #80022, #60224, #28233, #27822, #1743, #79606, #47584, #3399, #29062, #54733, #41283, #27400, #78772, #73278, #8470, #46755, #21096, #59801, #14797, #40454, #15626, #22341, #48001, #41686, #20684, #2986, #66969, #9302, #46336, #81251, #50060, #24389, #81671, #17285, #80438, #23982, #36605, #74108, #48408, #3812, #11787, #55958, #63114, #16454, #10133, #55132, #42099, #67796, #29474, #30292, #17688, #56377, #61464, #29879, #49649, #42913, #22748, #80842, #35797, #23155, #31113, #55541, #48824, #82076, #74525, #62707, #16871, #42508, #75341, #37440, #68210, #75755, #4621, #69434, #69016, #68608, #18097, #43730, #5045, #10547, #30714, #43318, #62283, #11368, #36205, #23566, #10948, #61874, #4215, #49237, #5452, #37025, #74940, #76576, #52122, #32360, #76987, #56781, #31532, #12190, #76168, #7538, #31947, #82480, #58448, #37847, #39089, #18904, #63525, #51702, #13855, #24796, #77830, #64353, #45810, #45393, #19316, #26471, #808, #64770, #57188, #7109, #58022, #13021, #38675, #82890, #83299, #44969, #50464, #70244, #18505, #32779, #70665, #63935, #44554, #20160, #386, #6271, #25621, #6690, #51284, #71508, #44148, #39513, #65202, #69840, #26042, #57608, #5855, #25210, #71090, #50876, #12599, #77404, #19739, #13433, #38258, #73169, #52542, #1233, #34452, #59695, #46654, #47889, #26882, #78251, #20582, #21407, #1640, #41178, #47061, #79089, #14695, #71930, #8368, #60121, #22234, #79917, #73597, #53786, #39941, #14279, #72753, #78671, #59283, #33620, #72347, #46233, #65627, #7958, #66868, #9198, #34871, #15939, #47477, #52956, #40351, #20992, #34034, #2882, #60532, #2472, #53382, #33211, #28131, #15102, #27298, #66030, #2051, #41586, #8779, #67276, #27715, #40758, #66442, #79498, #21813, #15520, #28545, #54201, #58875, #74003, #42402, #68507, #23881, #74836, #30190, #81149, #3291, #55441, #75241, #23464, #55853, #36508, #61354, #10847, #81562, #43217, #49131, #17180, #35689, #68915, #74418, #61773, #10446, #62184, #16763, #4521, #48306, #3708, #75655, #35278, #17585, #29779, #68100, #36102, #11265, #30611, #41994, #10023, #36923, #4114, #42813, #49546, #62600, #56275, #16350, #4942, #81971, #24286, #49958, #17995, #43629, #9609, #60941, #28956, #67688, #54621, #80332, #22647, #29371, #55032, #80739, #23053, #48721, #6585, #44448, #6166, #50366, #25516, #19628, #20052, #31010, #5351, #82380, #5754, #12086, #13329, #51595, #70140, #52017, #69741, #44049, #26357, #69333, #12913, #70985, #32672, #76063, #44858, #18406, #70557, #37743, #25936, #63417, #31424, #38570, #11683, #57086, #82782, #25103, #38982, #58338, #64251, #19210, #700, #32256, #77723, #37340, #76476, #12492, #63828, #83194, #57917, #63013, #77297, #64665, #51181, #56678, #76879, #50776, #281, #18803, #38155, #24697, #31841, #57503, #45289, #7004, #79297, #53588, #21615, #39406, #9407, #29176, #35077, #9820, #73810, #15316, #22452, #35491, #80547, #3095, #60743, #72965, #22859, #28343, #15739, #47693, #16147, #54004, #41794, #2267, #40979, #29583, #71401, #54842, #67075, #79716, #22032, #48520, #67905, #47275, #66661, #74220, #73387, #28759, #67485, #16565, #10242, #27930, #61155, #42210, #3507, #54421, #55246, #80132, #48112, #35913, #61579, #9000, #41393, #3922, #65089, #7427, #34250, #80953, #45705, #13749, #59912, #34672, #60335, #2683, #62822, #56896, #57303, #68321, #42624, #36313, #43026, #49352, #50577, #5564, #24091, #5974, #23678, #81365, #63636, #23268, #50171, #24909, #69948, #29992, #82188, #55655, #24505, #75049, #63224, #17395, #68720, #75867, #48937, #11062, #36720, #62396, #76284, #12303, #18210, #56485, #37959, #43845, #31644, #74638, #30407, #81781, #17799, #37137, #69548, #16981, #31228, #18615, #5156, #10658, #30820, #4734, #11896, #56075, #49761, #61989, #4326, #75461, #43434, #69131, #11482, #37549, #82589 ),
 ( #44258, #46351, #40058, #78369, #64890, #58139, #32062, #7662, #13977, #50986, #33333, #26161, #71208, #51823, #64469, #39634, #19017, #76684, #934, #77527, #13141, #14403, #44665, #70361, #12716, #13551, #51399, #58994, #39207, #45511, #6806, #38376, #508, #26592, #72047, #65745, #8078, #20277, #6392, #64051, #7229, #45086, #25738, #85, #38793, #57722, #77103, #19435, #1350, #27000, #52663, #33741, #65325, #70790, #32477, #19863, #32901, #20701, #83001, #52244, #58569, #25322, #77948, #45927, #71625, #27416, #66151, #74125, #34988, #42116, #53077, #72465, #34157, #78789, #21114, #8488, #9318, #80038, #35400, #40473, #8900, #60652, #79624, #59401, #59818, #14814, #46774, #10150, #34576, #1759, #61065, #2173, #41702, #79209, #27839, #54329, #16471, #53501, #54749, #66986, #48426, #48017, #21941, #29079, #3416, #67395, #21525, #9729, #3002, #15644, #41300, #47184, #2591, #47601, #72876, #15224, #40884, #80455, #66566, #60244, #73295, #28250, #53910, #28668, #22358, #73717, #16056, #22764, #67813, #11800, #69450, #24811, #50074, #55558, #49254, #81267, #36622, #5466, #63128, #37040, #55975, #35816, #62722, #75356, #29490, #3830, #42527, #50478, #11383, #18519, #55149, #48841, #10563, #80860, #23172, #68229, #69032, #56391, #37454, #16888, #68624, #5059, #81687, #61481, #36221, #74542, #61890, #69854, #10964, #4231, #31128, #29895, #18111, #23582, #74956, #30729, #76182, #17302, #56795, #43332, #44162, #24404, #23998, #82495, #42929, #43744, #62300, #4637, #82090, #17704, #75769, #30308, #49666, #32375, #63539, #25637, #46249, #45825, #26060, #19334, #31963, #7556, #71106, #44986, #64369, #45410, #6706, #1249, #31546, #58890, #52557, #33227, #77422, #70684, #44569, #20175, #26488, #5870, #71524, #38691, #403, #58039, #77003, #52139, #57203, #82904, #13449, #51719, #51300, #26898, #25225, #50890, #76590, #19756, #63951, #13870, #39105, #64787, #13038, #18919, #7125, #32797, #78266, #20597, #12205, #58466, #37863, #70260, #12615, #829, #77846, #38273, #39529, #65217, #6288, #57624, #62528, #60138, #15121, #53399, #28564, #7974, #39958, #73187, #40775, #2068, #3308, #65644, #33637, #59300, #2489, #40367, #79936, #28148, #34472, #79106, #27314, #47079, #15537, #60958, #35296, #28973, #9215, #78687, #52973, #53804, #34050, #14712, #72364, #27734, #1657, #21010, #46670, #22251, #47909, #73614, #54640, #2900, #8385, #21425, #59713, #72770, #41602, #15956, #41197, #8796, #71945, #66885, #79517, #66047, #66460, #21832, #80350, #47495, #22663, #34888, #60549, #54220, #67292, #9625, #14297, #81582, #68932, #24304, #29388, #81165, #23899, #68523, #48322, #23069, #3724, #67705, #82396, #23481, #74019, #49974, #55048, #30628, #68119, #80755, #43235, #5368, #16365, #43646, #55869, #37357, #36940, #10864, #18012, #75672, #56293, #48737, #81990, #49565, #4537, #30207, #74434, #74855, #36524, #42011, #61790, #10041, #69349, #62200, #55456, #10464, #11703, #75259, #49148, #17197, #17603, #42830, #63030, #35705, #31029, #61374, #16781, #42419, #36117, #4130, #29795, #56697, #11281, #62618, #4960, #25123, #82799, #65110, #24714, #51613, #26378, #71422, #31441, #299, #57104, #25955, #50793, #64684, #76494, #18821, #77318, #58788, #44468, #70159, #12512, #77742, #13769, #19648, #57935, #39426, #45309, #7448, #33118, #31863, #83213, #19228, #38591, #71004, #50382, #7023, #20073, #64269, #76080, #6603, #38173, #13347, #63847, #25535, #18424, #5772, #6185, #57522, #51200, #76898, #44878, #70577, #39001, #32275, #32691, #12931, #44065, #58358, #720, #52038, #45725, #69757, #12103, #37761, #63436, #34792, #40677, #46978, #27212, #60451, #65948, #53294, #1969, #28048, #8284, #79415, #39850, #52875, #67197, #26796, #66787, #21325, #33950, #59614, #2803, #22154, #33536, #1558, #9122, #27632, #66362, #21734, #28462, #47813, #65541, #8700, #41099, #34371, #79006, #59199, #54123, #15438, #52453, #79837, #72672, #15021, #60036, #2392, #73515, #20494, #78163, #53706, #47397, #14611, #15864, #46148, #71843, #7872, #14193, #41512, #9528, #35200, #1146, #78585, #20911, #40265, #46564 ) ),
 .UNSPECIFIED., .F., .F., .F. ) 
 B_SPLINE_SURFACE_WITH_KNOTS ( ( 2, 2 ),
 ( 3, 2, 2, 2, 2, 2, 2, 2, 2, 2, 2, 2, 2, 2, 2, 2, 2, 2, 2, 2, 2, 2, 2, 2, 2, 2, 2, 2, 2, 2, 2, 2, 2, 2, 2, 2, 2, 2, 2, 2, 2, 2, 2, 2, 2, 2, 2, 2, 2, 2, 2, 2, 2, 2, 2, 2, 2, 2, 2, 2, 2, 2, 2, 2, 2, 2, 2, 2, 2, 2, 2, 2, 2, 2, 2, 2, 2, 2, 2, 2, 2, 2, 2, 2, 2, 2, 2, 2, 2, 2, 2, 2, 2, 2, 2, 2, 2, 2, 2, 2, 2, 2, 2, 2, 2, 2, 2, 2, 2, 2, 2, 2, 2, 2, 2, 2, 2, 2, 2, 2, 2, 2, 2, 2, 2, 2, 2, 2, 2, 2, 2, 2, 2, 2, 2, 2, 2, 2, 2, 2, 2, 2, 2, 2, 2, 2, 2, 2, 2, 2, 2, 2, 2, 2, 2, 2, 2, 2, 2, 2, 2, 2, 2, 2, 2, 2, 2, 2, 2, 2, 2, 2, 2, 2, 2, 2, 2, 2, 2, 2, 2, 2, 2, 2, 2, 2, 2, 2, 2, 2, 2, 2, 2, 2, 2, 2, 2, 2, 2, 2, 2, 2, 2, 2, 2, 2, 2, 2, 2, 2, 2, 2, 2, 2, 2, 2, 2, 2, 2, 2, 2, 2, 2, 2, 2, 2, 2, 2, 2, 2, 2, 2, 2, 2, 2, 2, 2, 2, 2, 2, 2, 2, 2, 2, 2, 2, 2, 2, 2, 2, 2, 2, 2, 2, 2, 3 ),
 ( 0.000000000000000000, 1.000000000000000000 ),
 ( 0.000000000000000000, 0.003787878787878787984, 0.007575757575757575968, 0.01136363636363636395, 0.01515151515151515194, 0.01893939393939393992, 0.02272727272727272790, 0.02651515151515151589, 0.03030303030303030387, 0.03409090909090908839, 0.03787878787878787984, 0.04166666666666666435, 0.04545454545454545581, 0.04924242424242424032, 0.05303030303030303177, 0.05681818181818181629, 0.06060606060606060774, 0.06439393939393939226, 0.06818181818181817677, 0.07196969696969697516, 0.07575757575757575968, 0.07954545454545454419, 0.08333333333333332871, 0.08712121212121212710, 0.09090909090909091161, 0.09469696969696969613, 0.09848484848484848064, 0.1022727272727272790, 0.1060606060606060635, 0.1098484848484848481, 0.1136363636363636326, 0.1174242424242424310, 0.1212121212121212155, 0.1250000000000000000, 0.1287878787878787845, 0.1325757575757575690, 0.1363636363636363535, 0.1401515151515151381, 0.1439393939393939503, 0.1477272727272727348, 0.1515151515151515194, 0.1553030303030303039, 0.1590909090909090884, 0.1628787878787878729, 0.1666666666666666574, 0.1704545454545454419, 0.1742424242424242542, 0.1780303030303030387, 0.1818181818181818232, 0.1856060606060606077, 0.1893939393939393923, 0.1931818181818181768, 0.1969696969696969613, 0.2007575757575757458, 0.2045454545454545581, 0.2083333333333333426, 0.2121212121212121271, 0.2159090909090909116, 0.2196969696969696961, 0.2234848484848484806, 0.2272727272727272652, 0.2310606060606060497, 0.2348484848484848619, 0.2386363636363636465, 0.2424242424242424310, 0.2462121212121212155, 0.2500000000000000000, 0.2537878787878787845, 0.2575757575757575690, 0.2613636363636363535, 0.2651515151515151381, 0.2689393939393939226, 0.2727272727272727071, 0.2765151515151514916, 0.2803030303030302761, 0.2840909090909091161, 0.2878787878787879007, 0.2916666666666666852, 0.2954545454545454697, 0.2992424242424242542, 0.3030303030303030387, 0.3068181818181818232, 0.3106060606060606077, 0.3143939393939393923, 0.3181818181818181768, 0.3219696969696969613, 0.3257575757575757458, 0.3295454545454545303, 0.3333333333333333148, 0.3371212121212120993, 0.3409090909090908839, 0.3446969696969697239, 0.3484848484848485084, 0.3522727272727272929, 0.3560606060606060774, 0.3598484848484848619, 0.3636363636363636465, 0.3674242424242424310, 0.3712121212121212155, 0.3750000000000000000, 0.3787878787878787845, 0.3825757575757575690, 0.3863636363636363535, 0.3901515151515151381, 0.3939393939393939226, 0.3977272727272727071, 0.4015151515151514916, 0.4053030303030302761, 0.4090909090909091161, 0.4128787878787879007, 0.4166666666666666852, 0.4204545454545454697, 0.4242424242424242542, 0.4280303030303030387, 0.4318181818181818232, 0.4356060606060606077, 0.4393939393939393923, 0.4431818181818181768, 0.4469696969696969613, 0.4507575757575757458, 0.4545454545454545303, 0.4583333333333333148, 0.4621212121212120993, 0.4659090909090908839, 0.4696969696969697239, 0.4734848484848485084, 0.4772727272727272929, 0.4810606060606060774, 0.4848484848484848619, 0.4886363636363636465, 0.4924242424242424310, 0.4962121212121212155, 0.5000000000000000000, 0.5037878787878787845, 0.5075757575757575690, 0.5113636363636363535, 0.5151515151515151381, 0.5189393939393939226, 0.5227272727272727071, 0.5265151515151514916, 0.5303030303030302761, 0.5340909090909090606, 0.5378787878787878451, 0.5416666666666666297, 0.5454545454545454142, 0.5492424242424241987, 0.5530303030303029832, 0.5568181818181817677, 0.5606060606060605522, 0.5643939393939394478, 0.5681818181818182323, 0.5719696969696970168, 0.5757575757575758013, 0.5795454545454545858, 0.5833333333333333703, 0.5871212121212121549, 0.5909090909090909394, 0.5946969696969697239, 0.5984848484848485084, 0.6022727272727272929, 0.6060606060606060774, 0.6098484848484848619, 0.6136363636363636465, 0.6174242424242424310, 0.6212121212121212155, 0.6250000000000000000, 0.6287878787878787845, 0.6325757575757575690, 0.6363636363636363535, 0.6401515151515151381, 0.6439393939393939226, 0.6477272727272727071, 0.6515151515151514916, 0.6553030303030302761, 0.6590909090909090606, 0.6628787878787878451, 0.6666666666666666297, 0.6704545454545454142, 0.6742424242424241987, 0.6780303030303029832, 0.6818181818181817677, 0.6856060606060605522, 0.6893939393939394478, 0.6931818181818182323, 0.6969696969696970168, 0.7007575757575758013, 0.7045454545454545858, 0.7083333333333333703, 0.7121212121212121549, 0.7159090909090909394, 0.7196969696969697239, 0.7234848484848485084, 0.7272727272727272929, 0.7310606060606060774, 0.7348484848484848619, 0.7386363636363636465, 0.7424242424242424310, 0.7462121212121212155, 0.7500000000000000000, 0.7537878787878787845, 0.7575757575757575690, 0.7613636363636363535, 0.7651515151515151381, 0.7689393939393939226, 0.7727272727272727071, 0.7765151515151514916, 0.7803030303030302761, 0.7840909090909090606, 0.7878787878787878451, 0.7916666666666666297, 0.7954545454545454142, 0.7992424242424241987, 0.8030303030303029832, 0.8068181818181817677, 0.8106060606060605522, 0.8143939393939394478, 0.8181818181818182323, 0.8219696969696970168, 0.8257575757575758013, 0.8295454545454545858, 0.8333333333333333703, 0.8371212121212121549, 0.8409090909090909394, 0.8446969696969697239, 0.8484848484848485084, 0.8522727272727272929, 0.8560606060606060774, 0.8598484848484848619, 0.8636363636363636465, 0.8674242424242424310, 0.8712121212121212155, 0.8750000000000000000, 0.8787878787878787845, 0.8825757575757575690, 0.8863636363636363535, 0.8901515151515151381, 0.8939393939393939226, 0.8977272727272727071, 0.9015151515151514916, 0.9053030303030302761, 0.9090909090909090606, 0.9128787878787878451, 0.9166666666666666297, 0.9204545454545454142, 0.9242424242424241987, 0.9280303030303029832, 0.9318181818181817677, 0.9356060606060605522, 0.9393939393939394478, 0.9431818181818182323, 0.9469696969696970168, 0.9507575757575758013, 0.9545454545454545858, 0.9583333333333333703, 0.9621212121212121549, 0.9659090909090909394 ),
 .UNSPECIFIED. ) 
 GEOMETRIC_REPRESENTATION_ITEM ( )  RATIONAL_B_SPLINE_SURFACE ( (
 ( 1.000000000000000000, 0.9659258262890683122, 1.000000000000000000, 0.9659258262890683122, 1.000000000000000000, 0.9659258262890683122, 1.000000000000000000, 0.9659258262890683122, 1.000000000000000000, 0.9659258262890683122, 1.000000000000000000, 0.9659258262890683122, 1.000000000000000000, 0.9659258262890683122, 1.000000000000000000, 0.9659258262890683122, 1.000000000000000000, 0.9659258262890683122, 1.000000000000000000, 0.9659258262890683122, 1.000000000000000000, 0.9659258262890683122, 1.000000000000000000, 0.9659258262890683122, 1.000000000000000000, 0.9659258262890683122, 1.000000000000000000, 0.9659258262890683122, 1.000000000000000000, 0.9659258262890683122, 1.000000000000000000, 0.9659258262890683122, 1.000000000000000000, 0.9659258262890683122, 1.000000000000000000, 0.9659258262890683122, 1.000000000000000000, 0.9659258262890683122, 1.000000000000000000, 0.9659258262890683122, 1.000000000000000000, 0.9659258262890683122, 1.000000000000000000, 0.9659258262890683122, 1.000000000000000000, 0.9659258262890683122, 1.000000000000000000, 0.9659258262890683122, 1.000000000000000000, 0.9659258262890683122, 1.000000000000000000, 0.9659258262890683122, 1.000000000000000000, 0.9659258262890683122, 1.000000000000000000, 0.9659258262890683122, 1.000000000000000000, 0.9659258262890683122, 1.000000000000000000, 0.9659258262890683122, 1.000000000000000000, 0.9659258262890683122, 1.000000000000000000, 0.9659258262890683122, 1.000000000000000000, 0.9659258262890683122, 1.000000000000000000, 0.9659258262890683122, 1.000000000000000000, 0.9659258262890683122, 1.000000000000000000, 0.9659258262890683122, 1.000000000000000000, 0.9659258262890683122, 1.000000000000000000, 0.9659258262890683122, 1.000000000000000000, 0.9659258262890683122, 1.000000000000000000, 0.9659258262890683122, 1.000000000000000000, 0.9659258262890683122, 1.000000000000000000, 0.9659258262890683122, 1.000000000000000000, 0.9659258262890683122, 1.000000000000000000, 0.9659258262890683122, 1.000000000000000000, 0.9659258262890683122, 1.000000000000000000, 0.9659258262890683122, 1.000000000000000000, 0.9659258262890683122, 1.000000000000000000, 0.9659258262890683122, 1.000000000000000000, 0.9659258262890683122, 1.000000000000000000, 0.9659258262890683122, 1.000000000000000000, 0.9659258262890683122, 1.000000000000000000, 0.9659258262890683122, 1.000000000000000000, 0.9659258262890683122, 1.000000000000000000, 0.9659258262890683122, 1.000000000000000000, 0.9659258262890683122, 1.000000000000000000, 0.9659258262890683122, 1.000000000000000000, 0.9659258262890683122, 1.000000000000000000, 0.9659258262890683122, 1.000000000000000000, 0.9659258262890683122, 1.000000000000000000, 0.9659258262890683122, 1.000000000000000000, 0.9659258262890683122, 1.000000000000000000, 0.9659258262890683122, 1.000000000000000000, 0.9659258262890683122, 1.000000000000000000, 0.9659258262890683122, 1.000000000000000000, 0.9659258262890683122, 1.000000000000000000, 0.9659258262890683122, 1.000000000000000000, 0.9659258262890683122, 1.000000000000000000, 0.9659258262890683122, 1.000000000000000000, 0.9659258262890683122, 1.000000000000000000, 0.9659258262890683122, 1.000000000000000000, 0.9659258262890683122, 1.000000000000000000, 0.9659258262890683122, 1.000000000000000000, 0.9659258262890683122, 1.000000000000000000, 0.9659258262890683122, 1.000000000000000000, 0.9659258262890683122, 1.000000000000000000, 0.9659258262890683122, 1.000000000000000000, 0.9659258262890683122, 1.000000000000000000, 0.9659258262890683122, 1.000000000000000000, 0.9659258262890683122, 1.000000000000000000, 0.9659258262890683122, 1.000000000000000000, 0.9659258262890683122, 1.000000000000000000, 0.9659258262890683122, 1.000000000000000000, 0.9659258262890683122, 1.000000000000000000, 0.9659258262890683122, 1.000000000000000000, 0.9659258262890683122, 1.000000000000000000, 0.9659258262890683122, 1.000000000000000000, 0.9659258262890683122, 1.000000000000000000, 0.9659258262890683122, 1.000000000000000000, 0.9659258262890683122, 1.000000000000000000, 0.9659258262890683122, 1.000000000000000000, 0.9659258262890683122, 1.000000000000000000, 0.9659258262890683122, 1.000000000000000000, 0.9659258262890683122, 1.000000000000000000, 0.9659258262890683122, 1.000000000000000000, 0.9659258262890683122, 1.000000000000000000, 0.9659258262890683122, 1.000000000000000000, 0.9659258262890683122, 1.000000000000000000, 0.9659258262890683122, 1.000000000000000000, 0.9659258262890683122, 1.000000000000000000, 0.9659258262890683122, 1.000000000000000000, 0.9659258262890683122, 1.000000000000000000, 0.9659258262890683122, 1.000000000000000000, 0.9659258262890683122, 1.000000000000000000, 0.9659258262890683122, 1.000000000000000000, 0.9659258262890683122, 1.000000000000000000, 0.9659258262890683122, 1.000000000000000000, 0.9659258262890683122, 1.000000000000000000, 0.9659258262890683122, 1.000000000000000000, 0.9659258262890683122, 1.000000000000000000, 0.9659258262890683122, 1.000000000000000000, 0.9659258262890683122, 1.000000000000000000, 0.9659258262890683122, 1.000000000000000000, 0.9659258262890683122, 1.000000000000000000, 0.9659258262890683122, 1.000000000000000000, 0.9659258262890683122, 1.000000000000000000, 0.9659258262890683122, 1.000000000000000000, 0.9659258262890683122, 1.000000000000000000, 0.9659258262890683122, 1.000000000000000000, 0.9659258262890683122, 1.000000000000000000, 0.9659258262890683122, 1.000000000000000000, 0.9659258262890683122, 1.000000000000000000, 0.9659258262890683122, 1.000000000000000000, 0.9659258262890683122, 1.000000000000000000, 0.9659258262890683122, 1.000000000000000000, 0.9659258262890683122, 1.000000000000000000, 0.9659258262890683122, 1.000000000000000000, 0.9659258262890683122, 1.000000000000000000, 0.9659258262890683122, 1.000000000000000000, 0.9659258262890683122, 1.000000000000000000, 0.9659258262890683122, 1.000000000000000000, 0.9659258262890683122, 1.000000000000000000, 0.9659258262890683122, 1.000000000000000000, 0.9659258262890683122, 1.000000000000000000, 0.9659258262890683122, 1.000000000000000000, 0.9659258262890683122, 1.000000000000000000, 0.9659258262890683122, 1.000000000000000000, 0.9659258262890683122, 1.000000000000000000, 0.9659258262890683122, 1.000000000000000000, 0.9659258262890683122, 1.000000000000000000, 0.9659258262890683122, 1.000000000000000000, 0.9659258262890683122, 1.000000000000000000, 0.9659258262890683122, 1.000000000000000000, 0.9659258262890683122, 1.000000000000000000, 0.9659258262890683122, 1.000000000000000000, 0.9659258262890683122, 1.000000000000000000, 0.9659258262890683122, 1.000000000000000000, 0.9659258262890683122, 1.000000000000000000, 0.9659258262890683122, 1.000000000000000000, 0.9659258262890683122, 1.000000000000000000, 0.9659258262890683122, 1.000000000000000000, 0.9659258262890683122, 1.000000000000000000, 0.9659258262890683122, 1.000000000000000000, 0.9659258262890683122, 1.000000000000000000, 0.9659258262890683122, 1.000000000000000000, 0.9659258262890683122, 1.000000000000000000, 0.9659258262890683122, 1.000000000000000000, 0.9659258262890683122, 1.000000000000000000, 0.9659258262890683122, 1.000000000000000000, 0.9659258262890683122, 1.000000000000000000, 0.9659258262890683122, 1.000000000000000000, 0.9659258262890683122, 1.000000000000000000, 0.9659258262890683122, 1.000000000000000000, 0.9659258262890683122, 1.000000000000000000, 0.9659258262890683122, 1.000000000000000000, 0.9659258262890683122, 1.000000000000000000, 0.9659258262890683122, 1.000000000000000000, 0.9659258262890683122, 1.000000000000000000, 0.9659258262890683122, 1.000000000000000000, 0.9659258262890683122, 1.000000000000000000, 0.9659258262890683122, 1.000000000000000000, 0.9659258262890683122, 1.000000000000000000, 0.9659258262890683122, 1.000000000000000000, 0.9659258262890683122, 1.000000000000000000, 0.9659258262890683122, 1.000000000000000000, 0.9659258262890683122, 1.000000000000000000, 0.9659258262890683122, 1.000000000000000000, 0.9659258262890683122, 1.000000000000000000, 0.9659258262890683122, 1.000000000000000000, 0.9659258262890683122, 1.000000000000000000, 0.9659258262890683122, 1.000000000000000000, 0.9659258262890683122, 1.000000000000000000, 0.9659258262890683122, 1.000000000000000000, 0.9659258262890683122, 1.000000000000000000, 0.9659258262890683122, 1.000000000000000000, 0.9659258262890683122, 1.000000000000000000, 0.9659258262890683122, 1.000000000000000000, 0.9659258262890683122, 1.000000000000000000, 0.9659258262890683122, 1.000000000000000000, 0.9659258262890683122, 1.000000000000000000, 0.9659258262890683122, 1.000000000000000000, 0.9659258262890683122, 1.000000000000000000, 0.9659258262890683122, 1.000000000000000000, 0.9659258262890683122, 1.000000000000000000, 0.9659258262890683122, 1.000000000000000000, 0.9659258262890683122, 1.000000000000000000, 0.9659258262890683122, 1.000000000000000000, 0.9659258262890683122, 1.000000000000000000, 0.9659258262890683122, 1.000000000000000000, 0.9659258262890683122, 1.000000000000000000, 0.9659258262890683122, 1.000000000000000000, 0.9659258262890683122, 1.000000000000000000, 0.9659258262890683122, 1.000000000000000000, 0.9659258262890683122, 1.000000000000000000, 0.9659258262890683122, 1.000000000000000000, 0.9659258262890683122, 1.000000000000000000, 0.9659258262890683122, 1.000000000000000000, 0.9659258262890683122, 1.000000000000000000, 0.9659258262890683122, 1.000000000000000000, 0.9659258262890683122, 1.000000000000000000, 0.9659258262890683122, 1.000000000000000000, 0.9659258262890683122, 1.000000000000000000, 0.9659258262890683122, 1.000000000000000000, 0.9659258262890683122, 1.000000000000000000, 0.9659258262890683122, 1.000000000000000000, 0.9659258262890683122, 1.000000000000000000, 0.9659258262890683122, 1.000000000000000000, 0.9659258262890683122, 1.000000000000000000, 0.9659258262890683122, 1.000000000000000000, 0.9659258262890683122, 1.000000000000000000, 0.9659258262890683122, 1.000000000000000000, 0.9659258262890683122, 1.000000000000000000, 0.9659258262890683122, 1.000000000000000000, 0.9659258262890683122, 1.000000000000000000, 0.9659258262890683122, 1.000000000000000000, 0.9659258262890683122, 1.000000000000000000, 0.9659258262890683122, 1.000000000000000000, 0.9659258262890683122, 1.000000000000000000, 0.9659258262890683122, 1.000000000000000000, 0.9659258262890683122, 1.000000000000000000, 0.9659258262890683122, 1.000000000000000000, 0.9659258262890683122, 1.000000000000000000, 0.9659258262890683122, 1.000000000000000000, 0.9659258262890683122, 1.000000000000000000, 0.9659258262890683122, 1.000000000000000000, 0.9659258262890683122, 1.000000000000000000, 0.9659258262890683122, 1.000000000000000000, 0.9659258262890683122, 1.000000000000000000, 0.9659258262890683122, 1.000000000000000000, 0.9659258262890683122, 1.000000000000000000, 0.9659258262890683122, 1.000000000000000000, 0.9659258262890683122, 1.000000000000000000, 0.9659258262890683122, 1.000000000000000000, 0.9659258262890683122, 1.000000000000000000, 0.9659258262890683122, 1.000000000000000000, 0.9659258262890683122, 1.000000000000000000, 0.9659258262890683122, 1.000000000000000000, 0.9659258262890683122, 1.000000000000000000, 0.9659258262890683122, 1.000000000000000000, 0.9659258262890683122, 1.000000000000000000, 0.9659258262890683122, 1.000000000000000000, 0.9659258262890683122, 1.000000000000000000, 0.9659258262890683122, 1.000000000000000000, 0.9659258262890683122, 1.000000000000000000, 0.9659258262890683122, 1.000000000000000000, 0.9659258262890683122, 1.000000000000000000),
 ( 1.000000000000000000, 0.9659258262890683122, 1.000000000000000000, 0.9659258262890683122, 1.000000000000000000, 0.9659258262890683122, 1.000000000000000000, 0.9659258262890683122, 1.000000000000000000, 0.9659258262890683122, 1.000000000000000000, 0.9659258262890683122, 1.000000000000000000, 0.9659258262890683122, 1.000000000000000000, 0.9659258262890683122, 1.000000000000000000, 0.9659258262890683122, 1.000000000000000000, 0.9659258262890683122, 1.000000000000000000, 0.9659258262890683122, 1.000000000000000000, 0.9659258262890683122, 1.000000000000000000, 0.9659258262890683122, 1.000000000000000000, 0.9659258262890683122, 1.000000000000000000, 0.9659258262890683122, 1.000000000000000000, 0.9659258262890683122, 1.000000000000000000, 0.9659258262890683122, 1.000000000000000000, 0.9659258262890683122, 1.000000000000000000, 0.9659258262890683122, 1.000000000000000000, 0.9659258262890683122, 1.000000000000000000, 0.9659258262890683122, 1.000000000000000000, 0.9659258262890683122, 1.000000000000000000, 0.9659258262890683122, 1.000000000000000000, 0.9659258262890683122, 1.000000000000000000, 0.9659258262890683122, 1.000000000000000000, 0.9659258262890683122, 1.000000000000000000, 0.9659258262890683122, 1.000000000000000000, 0.9659258262890683122, 1.000000000000000000, 0.9659258262890683122, 1.000000000000000000, 0.9659258262890683122, 1.000000000000000000, 0.9659258262890683122, 1.000000000000000000, 0.9659258262890683122, 1.000000000000000000, 0.9659258262890683122, 1.000000000000000000, 0.9659258262890683122, 1.000000000000000000, 0.9659258262890683122, 1.000000000000000000, 0.9659258262890683122, 1.000000000000000000, 0.9659258262890683122, 1.000000000000000000, 0.9659258262890683122, 1.000000000000000000, 0.9659258262890683122, 1.000000000000000000, 0.9659258262890683122, 1.000000000000000000, 0.9659258262890683122, 1.000000000000000000, 0.9659258262890683122, 1.000000000000000000, 0.9659258262890683122, 1.000000000000000000, 0.9659258262890683122, 1.000000000000000000, 0.9659258262890683122, 1.000000000000000000, 0.9659258262890683122, 1.000000000000000000, 0.9659258262890683122, 1.000000000000000000, 0.9659258262890683122, 1.000000000000000000, 0.9659258262890683122, 1.000000000000000000, 0.9659258262890683122, 1.000000000000000000, 0.9659258262890683122, 1.000000000000000000, 0.9659258262890683122, 1.000000000000000000, 0.9659258262890683122, 1.000000000000000000, 0.9659258262890683122, 1.000000000000000000, 0.9659258262890683122, 1.000000000000000000, 0.9659258262890683122, 1.000000000000000000, 0.9659258262890683122, 1.000000000000000000, 0.9659258262890683122, 1.000000000000000000, 0.9659258262890683122, 1.000000000000000000, 0.9659258262890683122, 1.000000000000000000, 0.9659258262890683122, 1.000000000000000000, 0.9659258262890683122, 1.000000000000000000, 0.9659258262890683122, 1.000000000000000000, 0.9659258262890683122, 1.000000000000000000, 0.9659258262890683122, 1.000000000000000000, 0.9659258262890683122, 1.000000000000000000, 0.9659258262890683122, 1.000000000000000000, 0.9659258262890683122, 1.000000000000000000, 0.9659258262890683122, 1.000000000000000000, 0.9659258262890683122, 1.000000000000000000, 0.9659258262890683122, 1.000000000000000000, 0.9659258262890683122, 1.000000000000000000, 0.9659258262890683122, 1.000000000000000000, 0.9659258262890683122, 1.000000000000000000, 0.9659258262890683122, 1.000000000000000000, 0.9659258262890683122, 1.000000000000000000, 0.9659258262890683122, 1.000000000000000000, 0.9659258262890683122, 1.000000000000000000, 0.9659258262890683122, 1.000000000000000000, 0.9659258262890683122, 1.000000000000000000, 0.9659258262890683122, 1.000000000000000000, 0.9659258262890683122, 1.000000000000000000, 0.9659258262890683122, 1.000000000000000000, 0.9659258262890683122, 1.000000000000000000, 0.9659258262890683122, 1.000000000000000000, 0.9659258262890683122, 1.000000000000000000, 0.9659258262890683122, 1.000000000000000000, 0.9659258262890683122, 1.000000000000000000, 0.9659258262890683122, 1.000000000000000000, 0.9659258262890683122, 1.000000000000000000, 0.9659258262890683122, 1.000000000000000000, 0.9659258262890683122, 1.000000000000000000, 0.9659258262890683122, 1.000000000000000000, 0.9659258262890683122, 1.000000000000000000, 0.9659258262890683122, 1.000000000000000000, 0.9659258262890683122, 1.000000000000000000, 0.9659258262890683122, 1.000000000000000000, 0.9659258262890683122, 1.000000000000000000, 0.9659258262890683122, 1.000000000000000000, 0.9659258262890683122, 1.000000000000000000, 0.9659258262890683122, 1.000000000000000000, 0.9659258262890683122, 1.000000000000000000, 0.9659258262890683122, 1.000000000000000000, 0.9659258262890683122, 1.000000000000000000, 0.9659258262890683122, 1.000000000000000000, 0.9659258262890683122, 1.000000000000000000, 0.9659258262890683122, 1.000000000000000000, 0.9659258262890683122, 1.000000000000000000, 0.9659258262890683122, 1.000000000000000000, 0.9659258262890683122, 1.000000000000000000, 0.9659258262890683122, 1.000000000000000000, 0.9659258262890683122, 1.000000000000000000, 0.9659258262890683122, 1.000000000000000000, 0.9659258262890683122, 1.000000000000000000, 0.9659258262890683122, 1.000000000000000000, 0.9659258262890683122, 1.000000000000000000, 0.9659258262890683122, 1.000000000000000000, 0.9659258262890683122, 1.000000000000000000, 0.9659258262890683122, 1.000000000000000000, 0.9659258262890683122, 1.000000000000000000, 0.9659258262890683122, 1.000000000000000000, 0.9659258262890683122, 1.000000000000000000, 0.9659258262890683122, 1.000000000000000000, 0.9659258262890683122, 1.000000000000000000, 0.9659258262890683122, 1.000000000000000000, 0.9659258262890683122, 1.000000000000000000, 0.9659258262890683122, 1.000000000000000000, 0.9659258262890683122, 1.000000000000000000, 0.9659258262890683122, 1.000000000000000000, 0.9659258262890683122, 1.000000000000000000, 0.9659258262890683122, 1.000000000000000000, 0.9659258262890683122, 1.000000000000000000, 0.9659258262890683122, 1.000000000000000000, 0.9659258262890683122, 1.000000000000000000, 0.9659258262890683122, 1.000000000000000000, 0.9659258262890683122, 1.000000000000000000, 0.9659258262890683122, 1.000000000000000000, 0.9659258262890683122, 1.000000000000000000, 0.9659258262890683122, 1.000000000000000000, 0.9659258262890683122, 1.000000000000000000, 0.9659258262890683122, 1.000000000000000000, 0.9659258262890683122, 1.000000000000000000, 0.9659258262890683122, 1.000000000000000000, 0.9659258262890683122, 1.000000000000000000, 0.9659258262890683122, 1.000000000000000000, 0.9659258262890683122, 1.000000000000000000, 0.9659258262890683122, 1.000000000000000000, 0.9659258262890683122, 1.000000000000000000, 0.9659258262890683122, 1.000000000000000000, 0.9659258262890683122, 1.000000000000000000, 0.9659258262890683122, 1.000000000000000000, 0.9659258262890683122, 1.000000000000000000, 0.9659258262890683122, 1.000000000000000000, 0.9659258262890683122, 1.000000000000000000, 0.9659258262890683122, 1.000000000000000000, 0.9659258262890683122, 1.000000000000000000, 0.9659258262890683122, 1.000000000000000000, 0.9659258262890683122, 1.000000000000000000, 0.9659258262890683122, 1.000000000000000000, 0.9659258262890683122, 1.000000000000000000, 0.9659258262890683122, 1.000000000000000000, 0.9659258262890683122, 1.000000000000000000, 0.9659258262890683122, 1.000000000000000000, 0.9659258262890683122, 1.000000000000000000, 0.9659258262890683122, 1.000000000000000000, 0.9659258262890683122, 1.000000000000000000, 0.9659258262890683122, 1.000000000000000000, 0.9659258262890683122, 1.000000000000000000, 0.9659258262890683122, 1.000000000000000000, 0.9659258262890683122, 1.000000000000000000, 0.9659258262890683122, 1.000000000000000000, 0.9659258262890683122, 1.000000000000000000, 0.9659258262890683122, 1.000000000000000000, 0.9659258262890683122, 1.000000000000000000, 0.9659258262890683122, 1.000000000000000000, 0.9659258262890683122, 1.000000000000000000, 0.9659258262890683122, 1.000000000000000000, 0.9659258262890683122, 1.000000000000000000, 0.9659258262890683122, 1.000000000000000000, 0.9659258262890683122, 1.000000000000000000, 0.9659258262890683122, 1.000000000000000000, 0.9659258262890683122, 1.000000000000000000, 0.9659258262890683122, 1.000000000000000000, 0.9659258262890683122, 1.000000000000000000, 0.9659258262890683122, 1.000000000000000000, 0.9659258262890683122, 1.000000000000000000, 0.9659258262890683122, 1.000000000000000000, 0.9659258262890683122, 1.000000000000000000, 0.9659258262890683122, 1.000000000000000000, 0.9659258262890683122, 1.000000000000000000, 0.9659258262890683122, 1.000000000000000000, 0.9659258262890683122, 1.000000000000000000, 0.9659258262890683122, 1.000000000000000000, 0.9659258262890683122, 1.000000000000000000, 0.9659258262890683122, 1.000000000000000000, 0.9659258262890683122, 1.000000000000000000, 0.9659258262890683122, 1.000000000000000000, 0.9659258262890683122, 1.000000000000000000, 0.9659258262890683122, 1.000000000000000000, 0.9659258262890683122, 1.000000000000000000, 0.9659258262890683122, 1.000000000000000000, 0.9659258262890683122, 1.000000000000000000, 0.9659258262890683122, 1.000000000000000000, 0.9659258262890683122, 1.000000000000000000, 0.9659258262890683122, 1.000000000000000000, 0.9659258262890683122, 1.000000000000000000, 0.9659258262890683122, 1.000000000000000000, 0.9659258262890683122, 1.000000000000000000, 0.9659258262890683122, 1.000000000000000000, 0.9659258262890683122, 1.000000000000000000, 0.9659258262890683122, 1.000000000000000000, 0.9659258262890683122, 1.000000000000000000, 0.9659258262890683122, 1.000000000000000000, 0.9659258262890683122, 1.000000000000000000, 0.9659258262890683122, 1.000000000000000000, 0.9659258262890683122, 1.000000000000000000, 0.9659258262890683122, 1.000000000000000000, 0.9659258262890683122, 1.000000000000000000, 0.9659258262890683122, 1.000000000000000000, 0.9659258262890683122, 1.000000000000000000, 0.9659258262890683122, 1.000000000000000000, 0.9659258262890683122, 1.000000000000000000, 0.9659258262890683122, 1.000000000000000000, 0.9659258262890683122, 1.000000000000000000, 0.9659258262890683122, 1.000000000000000000, 0.9659258262890683122, 1.000000000000000000, 0.9659258262890683122, 1.000000000000000000, 0.9659258262890683122, 1.000000000000000000, 0.9659258262890683122, 1.000000000000000000, 0.9659258262890683122, 1.000000000000000000, 0.9659258262890683122, 1.000000000000000000, 0.9659258262890683122, 1.000000000000000000, 0.9659258262890683122, 1.000000000000000000, 0.9659258262890683122, 1.000000000000000000, 0.9659258262890683122, 1.000000000000000000, 0.9659258262890683122, 1.000000000000000000, 0.9659258262890683122, 1.000000000000000000, 0.9659258262890683122, 1.000000000000000000, 0.9659258262890683122, 1.000000000000000000, 0.9659258262890683122, 1.000000000000000000, 0.9659258262890683122, 1.000000000000000000, 0.9659258262890683122, 1.000000000000000000, 0.9659258262890683122, 1.000000000000000000, 0.9659258262890683122, 1.000000000000000000, 0.9659258262890683122, 1.000000000000000000, 0.9659258262890683122, 1.000000000000000000, 0.9659258262890683122, 1.000000000000000000, 0.9659258262890683122, 1.000000000000000000, 0.9659258262890683122, 1.000000000000000000, 0.9659258262890683122, 1.000000000000000000, 0.9659258262890683122, 1.000000000000000000, 0.9659258262890683122, 1.000000000000000000, 0.9659258262890683122, 1.000000000000000000, 0.9659258262890683122, 1.000000000000000000, 0.9659258262890683122, 1.000000000000000000) ) ) 
 REPRESENTATION_ITEM ( '' )  SURFACE ( )  );
#60098=CARTESIAN_POINT ( 'NONE',  ( -0.5249343832020990641, -0.5023911411419708095, -0.1820866141732282451 ) ) ;
#60103=CARTESIAN_POINT ( 'NONE',  ( 0.9776902887139113929, 0.1771653543307087630, 0.09757992244046791164 ) ) ;
#60104=CARTESIAN_POINT ( 'NONE',  ( -1.725721784776902190, -0.05778040916215522460, 0.4822834645669289988 ) ) ;
#60105=AXIS2_PLACEMENT_3D ( 'NONE', #58978, #37942, #12286 ) ;
#60106=CARTESIAN_POINT ( 'NONE',  ( 1.266404199475066328, -0.05778040916215522460, 0.4822834645669289988 ) ) ;
#60108=CARTESIAN_POINT ( 'NONE',  ( 1.148293963254593875, -0.5511811023622046335, 0.09757992244046803654 ) ) ;
#60109=CARTESIAN_POINT ( 'NONE',  ( 0.1049868766404206816, 0.2306618581243848609, 0.2411417322834645549 ) ) ;
#60110=CARTESIAN_POINT ( 'NONE',  ( -0.4658792650918627265, -0.3162353388693409650, -0.4822834645669289433 ) ) ;
#60111=CARTESIAN_POINT ( 'NONE',  ( 1.581364829396326277, -0.3162353388693409650, -0.4822834645669289433 ) ) ;
#60115=CARTESIAN_POINT ( 'NONE',  ( 0.3674540682414705883, 0.1283753931104746893, -0.1820866141732285504 ) ) ;
#60119=CARTESIAN_POINT ( 'NONE',  ( -0.4068241469816267775, 0.05413385826771626580, -0.4176697321401330321 ) ) ;
#60120=CARTESIAN_POINT ( 'NONE',  ( 1.509186351706037543, -0.4281496062992127816, -0.4176697321401328100 ) ) ;
#60121=CARTESIAN_POINT ( 'NONE',  ( 0.3149606299212606708, -0.1870078740157480879, -0.4822834645669291653 ) ) ;
#60122=CARTESIAN_POINT ( 'NONE',  ( -0.3937007874015740483, -0.1870078740157479769, 0.3641732283464567677 ) ) ;
#60123=CARTESIAN_POINT ( 'NONE',  ( 0.6824146981627303710, -0.6046776061558807314, 0.2411417322834647770 ) ) ;
#60124=CARTESIAN_POINT ( 'NONE',  ( -0.8202099737532799750, 0.2952755905511810774, -0.1292274648535930714 ) ) ;
#60125=CARTESIAN_POINT ( 'NONE',  ( -0.3937007874015740483, -0.1870078740157480879, -0.4822834645669291653 ) ) ;
#60126=CARTESIAN_POINT ( 'NONE',  ( -0.7086614173228339419, -0.1870078740157480879, -0.4822834645669291653 ) ) ;
#60127=CARTESIAN_POINT ( 'NONE',  ( 1.115485564304462551, 0.05413385826771666132, 0.4176697321401328100 ) ) ;
#60128=CARTESIAN_POINT ( 'NONE',  ( 0.7874015748031503170, -0.1870078740157479769, 0.4822834645669291653 ) ) ;
#60129=CARTESIAN_POINT ( 'NONE',  ( 0.7480314960629927956, 0.2952755905511811885, 0.000000000000000000 ) ) ;
#60131=CARTESIAN_POINT ( 'NONE',  ( -0.1115485564304453947, -0.5511811023622046335, 0.09757992244046803654 ) ) ;
#60135=CARTESIAN_POINT ( 'NONE',  ( -1.003937007874015297, -0.4536011799217368745, -0.2665933059059886201 ) ) ;
#60136=CARTESIAN_POINT ( 'NONE',  ( -0.2296587926509179312, -0.05778040916215522460, 0.4822834645669289988 ) ) ;
#60138=CARTESIAN_POINT ( 'NONE',  ( -0.07217847769028813698, -0.3162353388693409650, -0.4822834645669289433 ) ) ;
#60139=CARTESIAN_POINT ( 'NONE',  ( -0.5511811023622041894, -0.1870078740157480879, -0.4822834645669291653 ) ) ;
#60140=CARTESIAN_POINT ( 'NONE',  ( -1.469816272965878357, 0.2306618581243848609, 0.2411417322834645549 ) ) ;
#60141=CARTESIAN_POINT ( 'NONE',  ( -1.417322834645668772, -0.1870078740157479769, 0.4822834645669291653 ) ) ;
#60142=CARTESIAN_POINT ( 'NONE',  ( 1.364829396325460076, 0.1283753931104748280, 0.1820866141732283561 ) ) ;
#60143=CARTESIAN_POINT ( 'NONE',  ( -1.469816272965878357, 0.2306618581243848609, 0.2411417322834645549 ) ) ;
#60145=CARTESIAN_POINT ( 'NONE',  ( 0.4396325459317590445, -0.5511811023622046335, 0.09757992244046803654 ) ) ;
#60146=CARTESIAN_POINT ( 'NONE',  ( 0.1640419947506569498, -0.3162353388693409650, -0.4822834645669289433 ) ) ;
#60147=CARTESIAN_POINT ( 'NONE',  ( 0.3280839895013130669, -0.4281496062992127816, -0.4176697321401328100 ) ) ;
#60153=CARTESIAN_POINT ( 'NONE',  ( -0.6889763779527552368, -0.5400638737290845981, -0.3530559997133363437 ) ) ;
#60156=CARTESIAN_POINT ( 'NONE',  ( -1.443569553805773564, 0.1283753931104746893, -0.1820866141732285504 ) ) ;
#60157=CARTESIAN_POINT ( 'NONE',  ( 0.8530183727034126306, 0.05413385826771626580, -0.4176697321401330321 ) ) ;
#60158=CARTESIAN_POINT ( 'NONE',  ( 1.043307086614173818, 0.1660481256975885056, 0.3530559997133364547 ) ) ;
#60159=CARTESIAN_POINT ( 'NONE',  ( -0.1115485564304453947, -0.5511811023622046335, 0.09757992244046803654 ) ) ;
#60160=CARTESIAN_POINT ( 'NONE',  ( 0.04593175853018440641, 0.2952755905511810774, -0.1292274648535930714 ) ) ;
#60162=CARTESIAN_POINT ( 'NONE',  ( 0.1246719160104994284, 0.1771653543307087075, -0.09757992244046823083 ) ) ;
#60163=CARTESIAN_POINT ( 'NONE',  ( -0.3805774278215216522, -0.4281496062992127816, -0.4176697321401328100 ) ) ;
#60165=CARTESIAN_POINT ( 'NONE',  ( -1.686351706036744558, 0.2952755905511810774, -0.1292274648535930714 ) ) ;
#60166=CARTESIAN_POINT ( 'NONE',  ( 0.2034120734908142214, 0.1771653543307087075, -0.09757992244046823083 ) ) ;
#60167=CARTESIAN_POINT ( 'NONE',  ( -1.056430446194224881, 0.2952755905511810774, -0.1292274648535930714 ) ) ;
#60168=CARTESIAN_POINT ( 'NONE',  ( -0.8792650918635160906, -0.3690944881889763329, 0.3153832671262228327 ) ) ;
#60169=CARTESIAN_POINT ( 'NONE',  ( -0.6955380577427815458, -0.4281496062992127816, -0.4176697321401328100 ) ) ;
#60170=CARTESIAN_POINT ( 'NONE',  ( -0.5380577427821514602, 0.05413385826771666132, 0.4176697321401328100 ) ) ;
#60171=CARTESIAN_POINT ( 'NONE',  ( -0.05905511811023545637, 0.1660481256975885056, 0.3530559997133364547 ) ) ;
#60177=CARTESIAN_POINT ( 'NONE',  ( 0.3280839895013130669, -0.3690944881889765550, -0.3153832671262227771 ) ) ;
#60178=CARTESIAN_POINT ( 'NONE',  ( 1.122047244094488860, 0.1660481256975885056, 0.3530559997133364547 ) ) ;
#60179=CARTESIAN_POINT ( 'NONE',  ( -1.338582677165353729, -0.1870078740157480601, -0.3641732283464567677 ) ) ;
#60180=CARTESIAN_POINT ( 'NONE',  ( 1.318897637795276356, -0.5400638737290844871, 0.3530559997133364547 ) ) ;
#60181=CARTESIAN_POINT ( 'NONE',  ( -1.194225721784776262, -0.004921259842519870586, -0.3153832671262229437 ) ) ;
#60182=ADVANCED_FACE ( 'NONE', ( #31656 ), #49772, .F. ) ;
#60183=CARTESIAN_POINT ( 'NONE',  ( -0.3215223097112853146, -0.3162353388693405765, 0.4822834645669290543 ) ) ;
#60184=CARTESIAN_POINT ( 'NONE',  ( -0.006561679790025524116, -0.08942795157528024563, -0.3641732283464568787 ) ) ;
#60185=CARTESIAN_POINT ( 'NONE',  ( 1.609563999208788898, 0.2869511693896439342, 0.09226456620623516014 ) ) ;
#60186=CARTESIAN_POINT ( 'NONE',  ( 0.6102362204724416372, -0.4536011799217367080, 0.2665933059059888421 ) ) ;
#60187=B_SPLINE_CURVE_WITH_KNOTS ( 'NONE', 3,
 ( #43271, #11317, #50010, #30665, #4165, #4574, #82431 ),
 .UNSPECIFIED., .F., .F.,
 ( 4, 3, 4 ),
 ( 1.734723475976807094E-18, 0.001246230184515552441, 0.002492489877932635954 ),
 .UNSPECIFIED. ) ;
#60188=CARTESIAN_POINT ( 'NONE',  ( 0.3149606299212606708, -0.1870078740157480879, -0.4822834645669291653 ) ) ;
#60190=CARTESIAN_POINT ( 'NONE',  ( -0.5052493438320203589, -0.6692913385826771977, 0.1292274648535927661 ) ) ;
#60192=CARTESIAN_POINT ( 'NONE',  ( 1.181102362204724976, -0.1870078740157480601, -0.3641732283464567677 ) ) ;
#60193=CARTESIAN_POINT ( 'NONE',  ( -0.06561679790026180015, 0.05413385826771666132, 0.4176697321401328100 ) ) ;
#60194=CARTESIAN_POINT ( 'NONE',  ( -0.3740157480314953431, 0.1660481256975885056, 0.3530559997133364547 ) ) ;
#60195=CARTESIAN_POINT ( 'NONE',  ( -0.3215223097112853146, -0.08942795157528024563, -0.3641732283464568787 ) ) ;
#60196=DIRECTION ( 'NONE',  ( -1.000000000000000000, 0.000000000000000000, 0.000000000000000000 ) ) ;
#60197=CARTESIAN_POINT ( 'NONE',  ( 0.03937007874015833325, -0.5511811023622047445, 6.969142054262312111E-17 ) ) ;
#60198=CARTESIAN_POINT ( 'NONE',  ( 0.2952755905511819101, 0.1660481256975883668, -0.3530559997133364547 ) ) ;
#60199=CARTESIAN_POINT ( 'NONE',  ( -0.6430446194225716283, -0.3690944881889763329, 0.3153832671262228327 ) ) ;
#60201=CARTESIAN_POINT ( 'NONE',  ( -1.246719160104985846, -0.4281496062992127816, -0.4176697321401328100 ) ) ;
#60205=CARTESIAN_POINT ( 'NONE',  ( -0.9317585301837263412, -0.004921259842519576551, 0.3153832671262227771 ) ) ;
#60206=CARTESIAN_POINT ( 'NONE',  ( -0.1968503937007867743, -0.6692913385826771977, 8.415575281601705876E-17 ) ) ;
#60208=CARTESIAN_POINT ( 'NONE',  ( -0.6824146981627288167, 0.2306618581243848609, 0.2411417322834645549 ) ) ;
#60210=CARTESIAN_POINT ( 'NONE',  ( 1.496062992125985147, -0.1870078740157479769, 0.4822834645669291653 ) ) ;
#60211=CARTESIAN_POINT ( 'NONE',  ( 0.8267716535433078384, -0.6692913385826771977, 8.415575281601705876E-17 ) ) ;
#60215=CARTESIAN_POINT ( 'NONE',  ( -1.555118110236219930, 0.1660481256975885056, 0.3530559997133364547 ) ) ;
#60218=CARTESIAN_POINT ( 'NONE',  ( -0.3215223097112853146, -0.08942795157528024563, -0.3641732283464568787 ) ) ;
#60220=EDGE_LOOP ( 'NONE', ( #49162, #82201, #15014, #54302 ) ) ;
#60221=CARTESIAN_POINT ( 'NONE',  ( 0.8595800524934390507, -0.05778040916215560624, -0.4822834645669293319 ) ) ;
#60222=CARTESIAN_POINT ( 'NONE',  ( 0.1443569553805781891, -0.4281496062992124485, 0.4176697321401328655 ) ) ;
#60223=CARTESIAN_POINT ( 'NONE',  ( -0.7874015748031489847, -0.1870078740157480879, -0.4822834645669291653 ) ) ;
#60224=CARTESIAN_POINT ( 'NONE',  ( 1.456692913385827515, -0.6692913385826771977, 8.415575281601705876E-17 ) ) ;
#60225=CARTESIAN_POINT ( 'NONE',  ( -0.7414698162729651543, -0.5511811023622046335, 0.09757992244046803654 ) ) ;
#60227=CARTESIAN_POINT ( 'NONE',  ( 0.2821522309711292364, 0.2952755905511810774, -0.1292274648535930714 ) ) ;
#60228=CARTESIAN_POINT ( 'NONE',  ( 0.5708661417322841158, -0.4536011799217368745, -0.2665933059059886201 ) ) ;
#60229=CARTESIAN_POINT ( 'NONE',  ( -0.8333333333333323711, 0.2952755905511811885, 0.1292274648535926551 ) ) ;
#60231=CARTESIAN_POINT ( 'NONE',  ( -1.062992125984250968, -0.6692913385826771977, 8.415575281601705876E-17 ) ) ;
#60233=LINE ( 'NONE', #78780, #73470 ) ;
#60235=CARTESIAN_POINT ( 'NONE',  ( 1.069553805774278832, 0.2952755905511810774, -0.1292274648535930714 ) ) ;
#60236=CARTESIAN_POINT ( 'NONE',  ( 1.161417322834646493, -0.4536011799217367080, 0.2665933059059888421 ) ) ;
#60239=CARTESIAN_POINT ( 'NONE',  ( -0.5052493438320203589, 0.2952755905511810774, -0.1292274648535930714 ) ) ;
#60241=AXIS2_PLACEMENT_3D ( 'NONE', #63592, #31599, #12671 ) ;
#60242=CARTESIAN_POINT ( 'NONE',  ( 0.3149606299212603933, -0.1870078740157479769, 0.3641732283464567677 ) ) ;
#60243=CARTESIAN_POINT ( 'NONE',  ( -1.253280839895012377, -0.05778040916215522460, 0.4822834645669289988 ) ) ;
#60244=CARTESIAN_POINT ( 'NONE',  ( 0.8333333333333340365, 0.2952755905511810774, -0.1292274648535930714 ) ) ;
#60245=CARTESIAN_POINT ( 'NONE',  ( 0.6758530183727039509, 0.2952755905511810774, -0.1292274648535930714 ) ) ;
#60246=CARTESIAN_POINT ( 'NONE',  ( -0.2755905511811018171, 0.2952755905511811885, 0.000000000000000000 ) ) ;
#60247=CARTESIAN_POINT ( 'NONE',  ( -0.3083989501312330295, -0.3162353388693409650, -0.4822834645669289433 ) ) ;
#60249=CARTESIAN_POINT ( 'NONE',  ( -1.502624671916009680, -0.05778040916215560624, -0.4822834645669293319 ) ) ;
#60250=CARTESIAN_POINT ( 'NONE',  ( -0.4986876640419939388, 0.2306618581243847221, -0.2411417322834647770 ) ) ;
#60251=CARTESIAN_POINT ( 'NONE',  ( -0.6627296587926501115, 0.1771653543307087075, -0.09757992244046823083 ) ) ;
#60252=CARTESIAN_POINT ( 'NONE',  ( 1.135170603674541256, -0.6692913385826773087, -0.1292274648535924053 ) ) ;
#60254=CARTESIAN_POINT ( 'NONE',  ( -0.8595800524934373854, -0.3162353388693409650, -0.4822834645669289433 ) ) ;
#60256=CARTESIAN_POINT ( 'NONE',  ( 0.7677165354330716118, -0.5400638737290844871, 0.3530559997133364547 ) ) ;
#60258=LINE ( 'NONE', #23908, #17396 ) ;
#60259=CARTESIAN_POINT ( 'NONE',  ( 0.03937007874015833325, -0.6692913385826771977, 8.415575281601705876E-17 ) ) ;
#60260=CARTESIAN_POINT ( 'NONE',  ( -1.338582677165353729, -0.1870078740157479769, 0.3641732283464567677 ) ) ;
#60261=CARTESIAN_POINT ( 'NONE',  ( 0.9776902887139113929, -0.5511811023622048555, -0.09757992244046775898 ) ) ;
#60264=CARTESIAN_POINT ( 'NONE',  ( 1.266404199475066328, -0.2845877964562161244, -0.3641732283464567121 ) ) ;
#60265=CARTESIAN_POINT ( 'NONE',  ( 1.377952755905512472, -0.6692913385826771977, 8.415575281601705876E-17 ) ) ;
#60267=CARTESIAN_POINT ( 'NONE',  ( -0.2624671916010490880, 0.2306618581243847221, -0.2411417322834647770 ) ) ;
#60269=CARTESIAN_POINT ( 'NONE',  ( 1.509186351706037543, -0.3690944881889765550, -0.3153832671262227771 ) ) ;
#60270=CARTESIAN_POINT ( 'NONE',  ( -0.2230971128608915943, -0.4281496062992127816, -0.4176697321401328100 ) ) ;
#60272=CARTESIAN_POINT ( 'NONE',  ( 1.076115485564305141, 0.2306618581243847221, -0.2411417322834647770 ) ) ;
#60273=CARTESIAN_POINT ( 'NONE',  ( -0.01312335958005186876, -0.4281496062992124485, 0.4176697321401328655 ) ) ;
#60274=CARTESIAN_POINT ( 'NONE',  ( 0.6692913385826778638, -0.5511811023622047445, 6.969142054262312111E-17 ) ) ;
#60276=CARTESIAN_POINT ( 'NONE',  ( 0.4330708661417329575, 0.1771653543307087630, 0.000000000000000000 ) ) ;
#60277=CARTESIAN_POINT ( 'NONE',  ( -1.646981627296586703, -0.05778040916215522460, 0.4822834645669289988 ) ) ;
#60279=CARTESIAN_POINT ( 'NONE',  ( 0.7020997375328090762, -0.3162353388693405765, 0.4822834645669290543 ) ) ;
#60283=CARTESIAN_POINT ( 'NONE',  ( -0.01968503937007793844, -0.4536011799217367080, 0.2665933059059888421 ) ) ;
#60284=CARTESIAN_POINT ( 'NONE',  ( 0.2427821522309719648, -0.05778040916215522460, 0.4822834645669289988 ) ) ;
#60285=CARTESIAN_POINT ( 'NONE',  ( 1.194225721784777594, -0.004921259842519576551, 0.3153832671262227771 ) ) ;
#60286=CARTESIAN_POINT ( 'NONE',  ( -1.377952755905511140, 0.1771653543307087630, 0.000000000000000000 ) ) ;
#60287=CARTESIAN_POINT ( 'NONE',  ( -1.266404199475064773, -0.3162353388693405765, 0.4822834645669290543 ) ) ;
#60288=CARTESIAN_POINT ( 'NONE',  ( 0.6627296587926517768, -0.6692913385826773087, -0.1292274648535924053 ) ) ;
#60289=CARTESIAN_POINT ( 'NONE',  ( 1.443569553805774897, -0.6046776061558809534, -0.2411417322834644161 ) ) ;
#60291=CARTESIAN_POINT ( 'NONE',  ( 0.4068241469816279987, -0.4281496062992127816, -0.4176697321401328100 ) ) ;
#60293=CARTESIAN_POINT ( 'NONE',  ( 1.535433070866142558, 0.2952755905511811885, 0.000000000000000000 ) ) ;
#60294=CARTESIAN_POINT ( 'NONE',  ( 0.9055118110236227702, 0.2952755905511811885, 0.000000000000000000 ) ) ;
#60295=CARTESIAN_POINT ( 'NONE',  ( -1.555118110236219930, 0.07958543189024085140, 0.2665933059059887866 ) ) ;
#60296=CARTESIAN_POINT ( 'NONE',  ( 1.332020997375329197, -0.2845877964562159024, 0.3641732283464567677 ) ) ;
#60297=CARTESIAN_POINT ( 'NONE',  ( 1.423884514435696413, -0.3162353388693409650, -0.4822834645669289433 ) ) ;
#60298=CARTESIAN_POINT ( 'NONE',  ( -0.9251968503937002541, -0.4536011799217368745, -0.2665933059059886201 ) ) ;
#60299=CARTESIAN_POINT ( 'NONE',  ( 1.587926509186352142, 0.05413385826771666132, 0.4176697321401328100 ) ) ;
#60300=CARTESIAN_POINT ( 'NONE',  ( 0.4658792650918640033, -0.2845877964562159024, 0.3641732283464567677 ) ) ;
#60301=CARTESIAN_POINT ( 'NONE',  ( 0.1640419947506569498, -0.3162353388693409650, -0.4822834645669289433 ) ) ;
#60302=CARTESIAN_POINT ( 'NONE',  ( 1.227034120734908917, -0.6692913385826771977, 0.1292274648535927661 ) ) ;
#60303=CARTESIAN_POINT ( 'NONE',  ( -0.3280839895013117347, 0.05413385826771626580, -0.4176697321401330321 ) ) ;
#60305=CARTESIAN_POINT ( 'NONE',  ( 0.1706036745406830368, -0.004921259842519576551, 0.3153832671262227771 ) ) ;
#60306=CARTESIAN_POINT ( 'NONE',  ( 1.082677165354331228, -0.5400638737290844871, 0.3530559997133364547 ) ) ;
#60307=CARTESIAN_POINT ( 'NONE',  ( -1.620734908136482577, 0.2952755905511811885, 0.1292274648535926551 ) ) ;
#60308=CARTESIAN_POINT ( 'NONE',  ( -0.8989501312335946848, 0.2952755905511810774, -0.1292274648535930714 ) ) ;
#60309=CARTESIAN_POINT ( 'NONE',  ( -1.423884514435694859, -0.2845877964562159024, 0.3641732283464567677 ) ) ;
#60311=CARTESIAN_POINT ( 'NONE',  ( -1.193521905106661674, 2.660739321503277841E-15, -0.3464511005275191513 ) ) ;
#60312=CARTESIAN_POINT ( 'NONE',  ( -0.6233595800524928121, -0.3162353388693409650, -0.4822834645669289433 ) ) ;
#60313=CARTESIAN_POINT ( 'NONE',  ( -0.02624671916010428221, -0.6046776061558807314, 0.2411417322834647770 ) ) ;
#60316=ORIENTED_EDGE ( 'NONE', *, *, #68819, .T. ) ;
#60317=CARTESIAN_POINT ( 'NONE',  ( 0.6824146981627303710, -0.5023911411419708095, 0.1820866141732285504 ) ) ;
#60319=CARTESIAN_POINT ( 'NONE',  ( 0.9120734908136489683, -0.6692913385826771977, 0.1292274648535927661 ) ) ;
#60320=CARTESIAN_POINT ( 'NONE',  ( -0.2473181295769223131, 5.952911114587291371E-15, -0.3954985857520045833 ) ) ;
#60321=CARTESIAN_POINT ( 'NONE',  ( -1.476377952755905110, -0.4536011799217368745, -0.2665933059059886201 ) ) ;
#60322=CARTESIAN_POINT ( 'NONE',  ( 1.640419947506562393, -0.4281496062992124485, 0.4176697321401328655 ) ) ;
#60323=CARTESIAN_POINT ( 'NONE',  ( -1.443569553805773564, -0.6046776061558807314, 0.2411417322834647770 ) ) ;
#60325=CARTESIAN_POINT ( 'NONE',  ( 0.1771653543307093182, -0.5400638737290845981, -0.3530559997133363437 ) ) ;
#60326=CARTESIAN_POINT ( 'NONE',  ( -0.3083989501312330295, -0.08942795157527998196, 0.3641732283464567121 ) ) ;
#60328=CARTESIAN_POINT ( 'NONE',  ( 0.9645669291338588858, 0.1660481256975885056, 0.3530559997133364547 ) ) ;
#60329=CARTESIAN_POINT ( 'NONE',  ( -0.03280839895013062252, -0.6692913385826771977, 0.1292274648535927661 ) ) ;
#60331=DIRECTION ( 'NONE',  ( -1.000000000000000000, -3.412570772413389987E-16, 0.000000000000000000 ) ) ;
#60333=CARTESIAN_POINT ( 'NONE',  ( 0.9973753280839902091, -0.6046776061558807314, 0.2411417322834647770 ) ) ;
#60334=CARTESIAN_POINT ( 'NONE',  ( 0.08530183727034192087, -0.3162353388693409650, -0.4822834645669289433 ) ) ;
#60335=CARTESIAN_POINT ( 'NONE',  ( -1.233595800524933894, -0.6046776061558809534, -0.2411417322834644161 ) ) ;
#60336=CARTESIAN_POINT ( 'NONE',  ( -1.627296587926508442, 0.2306618581243848609, 0.2411417322834645549 ) ) ;
#60337=CARTESIAN_POINT ( 'NONE',  ( 0.8923884514435703741, 0.2306618581243848609, 0.2411417322834645549 ) ) ;
#60339=CARTESIAN_POINT ( 'NONE',  ( -0.4265091863517051496, 0.2952755905511810774, -0.1292274648535930714 ) ) ;
#60340=CARTESIAN_POINT ( 'NONE',  ( 0.6299212598425204535, -0.1870078740157480879, -0.4822834645669291653 ) ) ;
#60341=CARTESIAN_POINT ( 'NONE',  ( -0.07874015748031421014, -0.1870078740157479769, 0.4822834645669291653 ) ) ;
#60342=CARTESIAN_POINT ( 'NONE',  ( 0.5380577427821529035, -0.3690944881889763329, 0.3153832671262228327 ) ) ;
#60343=CARTESIAN_POINT ( 'NONE',  ( -1.476377952755905110, -0.5400638737290845981, -0.3530559997133363437 ) ) ;
#60344=CARTESIAN_POINT ( 'NONE',  ( 1.216659146022341931, 1.505269100445303598, 0.5216994034917036283 ) ) ;
#60345=CARTESIAN_POINT ( 'NONE',  ( 0.6364829396325465405, -0.05778040916215522460, 0.4822834645669289988 ) ) ;
#60346=CARTESIAN_POINT ( 'NONE',  ( -1.220472440944878834, 0.4405861044731111953, -0.5309055118110234117 ) ) ;
#60349=VERTEX_POINT ( 'NONE', #24516 ) ;
#60351=CARTESIAN_POINT ( 'NONE',  ( 1.148293963254593875, -0.6692913385826771977, 0.1292274648535927661 ) ) ;
#60352=CARTESIAN_POINT ( 'NONE',  ( 0.4658792650918640033, -0.2845877964562159024, 0.3641732283464567677 ) ) ;
#60358=CARTESIAN_POINT ( 'NONE',  ( -0.8333333333333323711, 0.2952755905511811885, 0.1292274648535926551 ) ) ;
#60359=CARTESIAN_POINT ( 'NONE',  ( -0.6430446194225716283, -0.4281496062992124485, 0.4176697321401328655 ) ) ;
#60360=CARTESIAN_POINT ( 'NONE',  ( 1.187664041994751285, -0.3162353388693409650, -0.4822834645669289433 ) ) ;
#60362=CARTESIAN_POINT ( 'NONE',  ( -1.594488188976377563, -0.5400638737290844871, 0.3530559997133364547 ) ) ;
#60364=CARTESIAN_POINT ( 'NONE',  ( 1.627296587926509996, -0.5023911411419708095, 0.1820866141732285504 ) ) ;
#60366=CARTESIAN_POINT ( 'NONE',  ( -1.384514435695537005, -0.5511811023622048555, -0.09757992244046775898 ) ) ;
#60368=CARTESIAN_POINT ( 'NONE',  ( 0.3412073490813655186, -0.6046776061558809534, -0.2411417322834644161 ) ) ;
#60369=CARTESIAN_POINT ( 'NONE',  ( 1.404199475065617708, 0.05413385826771626580, -0.4176697321401330321 ) ) ;
#60370=CARTESIAN_POINT ( 'NONE',  ( 0.7773926554473647998, 8.471767977567108961E-16, -0.4445507791589058955 ) ) ;
#60371=CARTESIAN_POINT ( 'NONE',  ( -0.8070866141732276899, -0.4536011799217367080, 0.2665933059059888421 ) ) ;
#60372=CARTESIAN_POINT ( 'NONE',  ( 0.6167979002624679463, 0.05413385826771626580, -0.4176697321401330321 ) ) ;
#60373=CARTESIAN_POINT ( 'NONE',  ( 1.489501312335958172, -0.08942795157528024563, -0.3641732283464568787 ) ) ;
#60375=CARTESIAN_POINT ( 'NONE',  ( -0.7349081364829390672, 0.1283753931104746893, -0.1820866141732285504 ) ) ;
#60376=CARTESIAN_POINT ( 'NONE',  ( 1.194225721784777594, 0.05413385826771666132, 0.4176697321401328100 ) ) ;
#60378=CARTESIAN_POINT ( 'NONE',  ( 0.3477690288713918276, 0.2952755905511811885, 0.1292274648535926551 ) ) ;
#60379=CARTESIAN_POINT ( 'NONE',  ( -1.056430446194224881, -0.5511811023622046335, 0.09757992244046803654 ) ) ;
#60380=CARTESIAN_POINT ( 'NONE',  ( -0.3018372703412066094, -0.004921259842519576551, 0.3153832671262227771 ) ) ;
#60381=CARTESIAN_POINT ( 'NONE',  ( -0.3477690288713905509, -0.6692913385826771977, 0.1292274648535927661 ) ) ;
#60382=CARTESIAN_POINT ( 'NONE',  ( -1.410761154855641575, -0.2845877964562161244, -0.3641732283464567121 ) ) ;
#60384=CARTESIAN_POINT ( 'NONE',  ( 0.2296587926509192634, -0.05778040916215560624, -0.4822834645669293319 ) ) ;
#60385=CARTESIAN_POINT ( 'NONE',  ( 0.8768409086929784824, 4.512065407040659715E-16, 0.4118484887281966822 ) ) ;
#60387=CARTESIAN_POINT ( 'NONE',  ( -0.8923884514435688198, 0.2306618581243847221, -0.2411417322834647770 ) ) ;
#60389=CARTESIAN_POINT ( 'NONE',  ( -0.3871391076115479057, -0.2845877964562161244, -0.3641732283464567121 ) ) ;
#60390=CARTESIAN_POINT ( 'NONE',  ( -1.213910761154854745, -0.6692913385826771977, 0.1292274648535927661 ) ) ;
#60391=CARTESIAN_POINT ( 'NONE',  ( 0.2887139107611556010, 0.1283753931104746893, -0.1820866141732285504 ) ) ;
#60392=CARTESIAN_POINT ( 'NONE',  ( -0.6561679790026240244, -0.5023911411419708095, 0.1820866141732285504 ) ) ;
#60393=CARTESIAN_POINT ( 'NONE',  ( -1.089238845144356427, 0.05413385826771666132, 0.4176697321401328100 ) ) ;
#60394=CARTESIAN_POINT ( 'NONE',  ( -1.548556430446193399, 0.2306618581243848609, 0.2411417322834645549 ) ) ;
#60395=CARTESIAN_POINT ( 'NONE',  ( 1.548556430446194954, 0.2306618581243847221, -0.2411417322834647770 ) ) ;
#60397=CARTESIAN_POINT ( 'NONE',  ( 0.8136482939632553313, -0.5023911411419708095, -0.1820866141732282451 ) ) ;
#60398=CARTESIAN_POINT ( 'NONE',  ( 0.5577427821522316087, -0.05778040916215522460, 0.4822834645669289988 ) ) ;
#60399=EDGE_CURVE ( 'NONE', #2588, #58735, #20279, .T. ) ;
#60400=CARTESIAN_POINT ( 'NONE',  ( 0.5288531115724313114, 1.522331584275864680, -0.5046369196611424357 ) ) ;
#60401=CARTESIAN_POINT ( 'NONE',  ( 1.272965879265092637, -0.004921259842519576551, 0.3153832671262227771 ) ) ;
#60404=CARTESIAN_POINT ( 'NONE',  ( -1.122047244094487306, 0.07958543189024071263, -0.2665933059059888421 ) ) ;
#60405=CARTESIAN_POINT ( 'NONE',  ( -0.4133858267716528645, -0.5400638737290844871, 0.3530559997133364547 ) ) ;
#60406=CARTESIAN_POINT ( 'NONE',  ( 0.4461942257217855201, -0.6046776061558807314, 0.2411417322834647770 ) ) ;
#60407=CARTESIAN_POINT ( 'NONE',  ( -1.666666666666665853, -0.004921259842519870586, -0.3153832671262229437 ) ) ;
#60409=CARTESIAN_POINT ( 'NONE',  ( -1.515748031496062076, 0.1660481256975883668, -0.3530559997133364547 ) ) ;
#60410=CARTESIAN_POINT ( 'NONE',  ( 0.5314960629921267055, -0.5400638737290844871, 0.3530559997133364547 ) ) ;
#60411=CARTESIAN_POINT ( 'NONE',  ( -0.1049868766404193215, -0.6046776061558807314, 0.2411417322834647770 ) ) ;
#60412=CARTESIAN_POINT ( 'NONE',  ( 1.312335958005249825, 0.2306618581243847221, -0.2411417322834647770 ) ) ;
#60413=FACE_OUTER_BOUND ( 'NONE', #17410, .T. ) ;
#60419=CARTESIAN_POINT ( 'NONE',  ( -0.05249343832020938322, -0.5023911411419708095, -0.1820866141732282451 ) ) ;
#60420=CARTESIAN_POINT ( 'NONE',  ( -0.5314960629921254842, -0.5400638737290845981, -0.3530559997133363437 ) ) ;
#60421=CARTESIAN_POINT ( 'NONE',  ( 0.8595800524934390507, -0.05778040916215560624, -0.4822834645669293319 ) ) ;
#60423=CARTESIAN_POINT ( 'NONE',  ( -0.2296587926509179312, -0.08942795157527998196, 0.3641732283464567121 ) ) ;
#60424=CARTESIAN_POINT ( 'NONE',  ( -1.062992125984250968, -0.6692913385826771977, 8.415575281601705876E-17 ) ) ;
#60425=CARTESIAN_POINT ( 'NONE',  ( -1.587926509186350810, 0.05413385826771626580, -0.4176697321401330321 ) ) ;
#60430=CARTESIAN_POINT ( 'NONE',  ( 0.9711286089238851948, 0.2306618581243848609, 0.2411417322834645549 ) ) ;
#60431=CARTESIAN_POINT ( 'NONE',  ( -1.489501312335957062, -0.3162353388693409650, -0.4822834645669289433 ) ) ;
#60432=CARTESIAN_POINT ( 'NONE',  ( -1.187664041994749731, -0.2845877964562159024, 0.3641732283464567677 ) ) ;
#60433=CARTESIAN_POINT ( 'NONE',  ( -1.069553805774277722, -0.6692913385826773087, -0.1292274648535924053 ) ) ;
#60436=CARTESIAN_POINT ( 'NONE',  ( 1.240157480314961314, 0.1660481256975883668, -0.3530559997133364547 ) ) ;
#60437=CARTESIAN_POINT ( 'NONE',  ( -1.496062992125983815, -0.1870078740157480879, -0.4822834645669291653 ) ) ;
#60438=CARTESIAN_POINT ( 'NONE',  ( -0.01312335958005186876, -0.4281496062992124485, 0.4176697321401328655 ) ) ;
#60439=CARTESIAN_POINT ( 'NONE',  ( -0.2690288713910754526, 0.2952755905511810774, -0.1292274648535930714 ) ) ;
#60440=CARTESIAN_POINT ( 'NONE',  ( -1.391076115485563314, -0.6046776061558809534, -0.2411417322834644161 ) ) ;
#60442=CARTESIAN_POINT ( 'NONE',  ( 0.3937007874015754361, -0.1870078740157480879, -0.4822834645669291653 ) ) ;
#60444=CARTESIAN_POINT ( 'NONE',  ( -1.351706036745406347, -0.3690944881889763329, 0.3153832671262228327 ) ) ;
#60445=VERTEX_POINT ( 'NONE', #78381 ) ;
#60449=CARTESIAN_POINT ( 'NONE',  ( -1.541994750656167090, 0.2952755905511811885, 0.1292274648535926551 ) ) ;
#60451=CARTESIAN_POINT ( 'NONE',  ( -1.358267716535432434, 0.1660481256975883668, -0.3530559997133364547 ) ) ;
#60453=CARTESIAN_POINT ( 'NONE',  ( -1.013613127888308485, -2.191421614605370878E-15, 0.4445507791589071167 ) ) ;
#60455=EDGE_CURVE ( 'NONE', #50394, #23460, #22489, .T. ) ;
#60457=CARTESIAN_POINT ( 'NONE',  ( -0.4133858267716528645, -0.4536011799217367080, 0.2665933059059888421 ) ) ;
#60458=CARTESIAN_POINT ( 'NONE',  ( -0.5774278215223089816, 0.1283753931104746893, -0.1820866141732285504 ) ) ;
#60459=CARTESIAN_POINT ( 'NONE',  ( -1.410761154855641575, -0.3162353388693409650, -0.4822834645669289433 ) ) ;
#60461=CARTESIAN_POINT ( 'NONE',  ( 1.056430446194226436, -0.6692913385826773087, -0.1292274648535924053 ) ) ;
#60462=CARTESIAN_POINT ( 'NONE',  ( -0.8858267716535425107, -0.5400638737290844871, 0.3530559997133364547 ) ) ;
#60464=CARTESIAN_POINT ( 'NONE',  ( -1.410761154855641575, -0.3162353388693409650, -0.4822834645669289433 ) ) ;
#60465=CARTESIAN_POINT ( 'NONE',  ( -1.606345848754414662, 0.2948621807332563738, 0.02311241260066472514 ) ) ;
#60471=CARTESIAN_POINT ( 'NONE',  ( -0.6233595800524928121, -0.3162353388693409650, -0.4822834645669289433 ) ) ;
#60472=CARTESIAN_POINT ( 'NONE',  ( 1.246719160104987623, 0.05413385826771626580, -0.4176697321401330321 ) ) ;
#60474=CARTESIAN_POINT ( 'NONE',  ( -1.633858267716534529, -0.5400638737290845981, -0.3530559997133363437 ) ) ;
#60476=CARTESIAN_POINT ( 'NONE',  ( -1.377952755905511140, 0.2952755905511811885, 0.000000000000000000 ) ) ;
#60477=CARTESIAN_POINT ( 'NONE',  ( -0.8989501312335946848, 0.2952755905511810774, -0.1292274648535930714 ) ) ;
#60479=CARTESIAN_POINT ( 'NONE',  ( 0.4068241469816279987, -0.3690944881889765550, -0.3153832671262227771 ) ) ;
#60481=CARTESIAN_POINT ( 'NONE',  ( 0.4396325459317593221, 0.1771653543307087075, -0.09757992244046823083 ) ) ;
#60482=CARTESIAN_POINT ( 'NONE',  ( 0.9842519685039375910, 0.1771653543307087630, 0.000000000000000000 ) ) ;
#60483=CARTESIAN_POINT ( 'NONE',  ( 0.9973753280839902091, 0.2306618581243847221, -0.2411417322834647770 ) ) ;
#60485=CARTESIAN_POINT ( 'NONE',  ( -0.4855643044619415427, -0.004921259842519870586, -0.3153832671262229437 ) ) ;
#60487=CARTESIAN_POINT ( 'NONE',  ( -1.253280839895012377, -0.3162353388693409650, -0.4822834645669289433 ) ) ;
#60489=CARTESIAN_POINT ( 'NONE',  ( -1.227034120734907141, -0.5511811023622048555, -0.09757992244046775898 ) ) ;
#60491=CARTESIAN_POINT ( 'NONE',  ( -0.9645669291338575535, 0.07958543189024071263, -0.2665933059059888421 ) ) ;
#60492=CARTESIAN_POINT ( 'NONE',  ( -0.1246719160104980823, -0.6692913385826773087, -0.1292274648535924053 ) ) ;
#60493=CARTESIAN_POINT ( 'NONE',  ( -0.7426113562967729953, 2.199547029020892275, -0.5309055118110235227 ) ) ;
#60495=CARTESIAN_POINT ( 'NONE',  ( 0.5774278215223103139, -0.5023911411419708095, -0.1820866141732282451 ) ) ;
#60496=CARTESIAN_POINT ( 'NONE',  ( -0.4593175853018366950, -0.004921259842519576551, 0.3153832671262227771 ) ) ;
#60497=CARTESIAN_POINT ( 'NONE',  ( -0.8333333333333323711, 0.2952755905511811885, 0.1292274648535926551 ) ) ;
#60500=CARTESIAN_POINT ( 'NONE',  ( -0.02624671916010428221, 0.2306618581243847221, -0.2411417322834647770 ) ) ;
#60502=ADVANCED_BREP_SHAPE_REPRESENTATION ( '', ( #59541, #22098 ), #14119 ) ;
#60505=CARTESIAN_POINT ( 'NONE',  ( 1.404199475065617264, -0.4281496062992124485, 0.4176697321401328655 ) ) ;
#60506=CARTESIAN_POINT ( 'NONE',  ( -0.1706036745406816491, -0.3690944881889763329, 0.3153832671262228327 ) ) ;
#60507=CARTESIAN_POINT ( 'NONE',  ( 5.463695987328526437E-16, -0.1870078740157479769, 0.4822834645669291653 ) ) ;
#60508=CARTESIAN_POINT ( 'NONE',  ( -1.594488188976377119, 0.1660481256975883668, -0.3530559997133364547 ) ) ;
#60509=CARTESIAN_POINT ( 'NONE',  ( 1.646981627296588035, -0.3162353388693405765, 0.4822834645669290543 ) ) ;
#60510=CARTESIAN_POINT ( 'NONE',  ( 1.220472440944882608, 0.2952755905511811885, 0.000000000000000000 ) ) ;
#60511=CARTESIAN_POINT ( 'NONE',  ( -0.6824146981627291497, -0.5023911411419708095, -0.1820866141732282451 ) ) ;
#60516=CARTESIAN_POINT ( 'NONE',  ( 1.351706036745407458, -0.3690944881889765550, -0.3153832671262227771 ) ) ;
#60517=CARTESIAN_POINT ( 'NONE',  ( -1.607611548556429737, -0.6692913385826771977, 0.1292274648535927661 ) ) ;
#60518=CARTESIAN_POINT ( 'NONE',  ( 1.010498687664042716, 0.05413385826771626580, -0.4176697321401330321 ) ) ;
#60520=CARTESIAN_POINT ( 'NONE',  ( 1.122047244094488860, -0.4536011799217368745, -0.2665933059059886201 ) ) ;
#60521=CARTESIAN_POINT ( 'NONE',  ( -0.04593175853018302557, 0.2952755905511811885, 0.1292274648535926551 ) ) ;
#60522=CARTESIAN_POINT ( 'NONE',  ( -0.3477690288713902178, 0.2952755905511810774, -0.1292274648535930714 ) ) ;
#60526=CARTESIAN_POINT ( 'NONE',  ( 0.4330708661417329575, -0.5511811023622047445, 6.969142054262312111E-17 ) ) ;
#60529=ORIENTED_EDGE ( 'NONE', *, *, #40891, .T. ) ;
#60530=CARTESIAN_POINT ( 'NONE',  ( -0.5314960629921254842, -0.5400638737290845981, -0.3530559997133363437 ) ) ;
#60531=CARTESIAN_POINT ( 'NONE',  ( 0.7349081364829402885, -0.6046776061558809534, -0.2411417322834644161 ) ) ;
#60532=CARTESIAN_POINT ( 'NONE',  ( 0.1509186351706045259, -0.05778040916215560624, -0.4822834645669293319 ) ) ;
#60533=CARTESIAN_POINT ( 'NONE',  ( -0.4724409448818890911, -0.1870078740157480601, -0.3641732283464567677 ) ) ;
#60534=CARTESIAN_POINT ( 'NONE',  ( 0.8333333333333340365, -0.6692913385826771977, 0.1292274648535927661 ) ) ;
#60535=CARTESIAN_POINT ( 'NONE',  ( -0.8792650918635160906, -0.4281496062992124485, 0.4176697321401328655 ) ) ;
#60536=CARTESIAN_POINT ( 'NONE',  ( -0.5183727034120726440, -0.6692913385826773087, -0.1292274648535924053 ) ) ;
#60537=CARTESIAN_POINT ( 'NONE',  ( -0.7742782152230965886, 0.05413385826771666132, 0.4176697321401328100 ) ) ;
#60538=CARTESIAN_POINT ( 'NONE',  ( 1.017060367454068581, -0.05778040916215560624, -0.4822834645669293319 ) ) ;
#60539=CARTESIAN_POINT ( 'NONE',  ( 0.7217847769028878924, -0.4281496062992127816, -0.4176697321401328100 ) ) ;
#60540=CARTESIAN_POINT ( 'NONE',  ( 0.8792650918635177559, 0.05413385826771666132, 0.4176697321401328100 ) ) ;
#60542=CARTESIAN_POINT ( 'NONE',  ( 0.2034120734908144990, -0.5511811023622046335, 0.09757992244046803654 ) ) ;
#60546=CARTESIAN_POINT ( 'NONE',  ( -0.9317585301837263412, -0.004921259842519576551, 0.3153832671262227771 ) ) ;
#60547=CARTESIAN_POINT ( 'NONE',  ( -0.4133858267716528645, -0.5400638737290844871, 0.3530559997133364547 ) ) ;
#60549=CARTESIAN_POINT ( 'NONE',  ( -0.4593175853018366950, 0.05413385826771666132, 0.4176697321401328100 ) ) ;
#60550=CARTESIAN_POINT ( 'NONE',  ( -0.2362204724409442680, -0.1870078740157480879, -0.4822834645669291653 ) ) ;
#60551=CARTESIAN_POINT ( 'NONE',  ( -1.443569553805773564, 0.2306618581243847221, -0.2411417322834647770 ) ) ;
#60553=CARTESIAN_POINT ( 'NONE',  ( -1.522309711286088607, 0.2306618581243847221, -0.2411417322834647770 ) ) ;
#60554=CARTESIAN_POINT ( 'NONE',  ( 1.095800524934383846, -0.08942795157528024563, -0.3641732283464568787 ) ) ;
#60557=CARTESIAN_POINT ( 'NONE',  ( 0.3608923884514443348, 0.1771653543307087075, -0.09757992244046823083 ) ) ;
#60558=CARTESIAN_POINT ( 'NONE',  ( -0.01312335958005186876, 0.05413385826771626580, -0.4176697321401330321 ) ) ;
#60559=CARTESIAN_POINT ( 'NONE',  ( 0.4002624671916016896, -0.05778040916215522460, 0.4822834645669289988 ) ) ;
#60562=CARTESIAN_POINT ( 'NONE',  ( -0.5839895013123352907, 0.2066929133858267098, -0.1054918080437494132 ) ) ;
#60563=ORIENTED_EDGE ( 'NONE', *, *, #62867, .F. ) ;
#60566=CARTESIAN_POINT ( 'NONE',  ( -0.4265091863517051496, 0.1771653543307087075, -0.09757992244046823083 ) ) ;
#60567=CARTESIAN_POINT ( 'NONE',  ( -0.5708661417322828946, 0.1660481256975883668, -0.3530559997133364547 ) ) ;
#60570=CARTESIAN_POINT ( 'NONE',  ( 1.614173228346457378, -0.6692913385826771977, 8.415575281601705876E-17 ) ) ;
#60571=CARTESIAN_POINT ( 'NONE',  ( 0.7152230971128614723, -0.3162353388693409650, -0.4822834645669289433 ) ) ;
#60572=CARTESIAN_POINT ( 'NONE',  ( 0.8530183727034128527, -0.4281496062992124485, 0.4176697321401328655 ) ) ;
#60573=CARTESIAN_POINT ( 'NONE',  ( -0.7808398950131222316, -0.2845877964562161244, -0.3641732283464567121 ) ) ;
#60574=CARTESIAN_POINT ( 'NONE',  ( 0.07217847769028949700, -0.05778040916215560624, -0.4822834645669293319 ) ) ;
#60576=CARTESIAN_POINT ( 'NONE',  ( -0.01968503937007793844, 0.07958543189024071263, -0.2665933059059888421 ) ) ;
#60577=CARTESIAN_POINT ( 'NONE',  ( -0.3871391076115479057, -0.3162353388693409650, -0.4822834645669289433 ) ) ;
#60579=CARTESIAN_POINT ( 'NONE',  ( 1.535433070866142335, -0.5511811023622047445, 6.969142054262312111E-17 ) ) ;
#60580=CARTESIAN_POINT ( 'NONE',  ( -0.01968503937007793844, -0.4536011799217367080, 0.2665933059059888421 ) ) ;
#60581=CARTESIAN_POINT ( 'NONE',  ( -0.7426113562971995430, 1.972848275015057995, -0.5309055118110235227 ) ) ;
#60582=CARTESIAN_POINT ( 'NONE',  ( -1.148293963254592542, -0.6692913385826773087, -0.1292274648535924053 ) ) ;
#60584=CARTESIAN_POINT ( 'NONE',  ( -0.8070866141732276899, 0.07958543189024071263, -0.2665933059059888421 ) ) ;
#60586=CARTESIAN_POINT ( 'NONE',  ( -1.082677165354329896, 0.1660481256975885056, 0.3530559997133364547 ) ) ;
#60587=CARTESIAN_POINT ( 'NONE',  ( 0.1377952755905518800, 0.1660481256975883668, -0.3530559997133364547 ) ) ;
#60591=CARTESIAN_POINT ( 'NONE',  ( 0.5249343832021005074, -0.5023911411419708095, 0.1820866141732285504 ) ) ;
#60592=CARTESIAN_POINT ( 'NONE',  ( 0.9186351706036751663, -0.6046776061558807314, 0.2411417322834647770 ) ) ;
#60593=CARTESIAN_POINT ( 'NONE',  ( -1.240157480314959759, 0.07958543189024085140, 0.2665933059059887866 ) ) ;
#60594=( BOUNDED_CURVE ( )  B_SPLINE_CURVE ( 2, ( #69801, #63074, #36985, #12557, #18865, #55916, #38216, #31073, #76124, #56741, #69394, #44514, #23940 ),
 .UNSPECIFIED., .F., .F. ) 
 B_SPLINE_CURVE_WITH_KNOTS ( ( 3, 2, 2, 2, 2, 2, 3 ),
 ( 0.2642401855438917813, 0.2651515151515151381, 0.2689393939393939226, 0.2727272727272727071, 0.2765151515151514916, 0.2803030303030302761, 0.2812143599106537439 ),
 .UNSPECIFIED. ) 
 CURVE ( )  GEOMETRIC_REPRESENTATION_ITEM ( )  RATIONAL_B_SPLINE_CURVE ( ( 0.9875488213027530104, 0.9918020599134685922, 1.000000000000000000, 0.9659258262890683122, 1.000000000000000000, 0.9659258262890683122, 1.000000000000000000, 0.9659258262890683122, 1.000000000000000000, 0.9659258262890683122, 1.000000000000000000, 0.9918020599134677040, 0.9875488213027521223 ) ) 
 REPRESENTATION_ITEM ( '' )  );
#60595=CARTESIAN_POINT ( 'NONE',  ( 1.108923884514436686, -0.3162353388693409650, -0.4822834645669289433 ) ) ;
#60596=CARTESIAN_POINT ( 'NONE',  ( -1.502624671916009680, -0.08942795157528024563, -0.3641732283464568787 ) ) ;
#60597=CARTESIAN_POINT ( 'NONE',  ( -0.3149606299212590610, -0.1870078740157479769, 0.4822834645669291653 ) ) ;
#60598=CARTESIAN_POINT ( 'NONE',  ( 0.2559055118110243332, 0.07958543189024085140, 0.2665933059059887866 ) ) ;
#60599=CARTESIAN_POINT ( 'NONE',  ( 0.5314960629921264834, 0.07958543189024071263, -0.2665933059059888421 ) ) ;
#60601=CARTESIAN_POINT ( 'NONE',  ( 0.1181102362204730916, 0.2952755905511811885, 0.000000000000000000 ) ) ;
#60603=CARTESIAN_POINT ( 'NONE',  ( -0.5118110236220466680, -0.6692913385826771977, 8.415575281601705876E-17 ) ) ;
#60605=CARTESIAN_POINT ( 'NONE',  ( 1.220472440944882386, -0.5511811023622047445, 6.969142054262312111E-17 ) ) ;
#60606=CARTESIAN_POINT ( 'NONE',  ( -0.03937007874015669567, 0.2952755905511811885, 0.000000000000000000 ) ) ;
#60607=CARTESIAN_POINT ( 'NONE',  ( -0.2230971128608915943, 0.05413385826771666132, 0.4176697321401328100 ) ) ;
#60608=CARTESIAN_POINT ( 'NONE',  ( -0.2230971128608915943, -0.004921259842519576551, 0.3153832671262227771 ) ) ;
#60609=CARTESIAN_POINT ( 'NONE',  ( 1.207349081364829990, 0.2306618581243848609, 0.2411417322834645549 ) ) ;
#60610=CARTESIAN_POINT ( 'NONE',  ( -0.3543307086614165824, 0.1771653543307087630, 0.000000000000000000 ) ) ;
#60611=CARTESIAN_POINT ( 'NONE',  ( 0.2230971128608932319, -0.4281496062992124485, 0.4176697321401328655 ) ) ;
#60612=CARTESIAN_POINT ( 'NONE',  ( -0.9120734908136475250, 0.1771653543307087630, 0.09757992244046791164 ) ) ;
#60614=CARTESIAN_POINT ( 'NONE',  ( -1.076115485564303809, -0.6046776061558809534, -0.2411417322834644161 ) ) ;
#60616=ORIENTED_EDGE ( 'NONE', *, *, #70755, .F. ) ;
#60617=CARTESIAN_POINT ( 'NONE',  ( -1.213910761154854745, 0.1771653543307087075, -0.09757992244046823083 ) ) ;
#60618=CARTESIAN_POINT ( 'NONE',  ( -0.4396325459317579898, 0.2952755905511811885, 0.1292274648535926551 ) ) ;
#60620=CARTESIAN_POINT ( 'NONE',  ( -1.338582677165353729, -0.1870078740157479769, 0.4822834645669291653 ) ) ;
#60622=CARTESIAN_POINT ( 'NONE',  ( 1.502624671916010790, -0.05778040916215522460, 0.4822834645669289988 ) ) ;
#60623=CARTESIAN_POINT ( 'NONE',  ( 0.6627296587926517768, -0.6692913385826773087, -0.1292274648535924053 ) ) ;
#60626=CARTESIAN_POINT ( 'NONE',  ( -1.666666666666665853, 0.05413385826771626580, -0.4176697321401330321 ) ) ;
#60629=CARTESIAN_POINT ( 'NONE',  ( -0.6561679790026240244, 0.1283753931104746893, -0.1820866141732285504 ) ) ;
#60632=CARTESIAN_POINT ( 'NONE',  ( 0.9514435695538062676, -0.05778040916215522460, 0.4822834645669289988 ) ) ;
#60633=CARTESIAN_POINT ( 'NONE',  ( 0.08530183727034192087, -0.3162353388693409650, -0.4822834645669289433 ) ) ;
#60634=CARTESIAN_POINT ( 'NONE',  ( -0.6233595800524928121, -0.3162353388693409650, -0.4822834645669289433 ) ) ;
#60635=CARTESIAN_POINT ( 'NONE',  ( 1.541994750656168645, 0.2952755905511810774, -0.1292274648535930714 ) ) ;
#60636=CARTESIAN_POINT ( 'NONE',  ( -1.259842519685038686, -0.1870078740157480601, -0.3641732283464567677 ) ) ;
#60637=DIRECTION ( 'NONE',  ( -1.000000000000000000, -3.096699300667737957E-16, 1.692413147294446216E-16 ) ) ;
#60638=CARTESIAN_POINT ( 'NONE',  ( 0.2755905511811031494, 0.2952755905511811885, 0.000000000000000000 ) ) ;
#60640=CARTESIAN_POINT ( 'NONE',  ( -0.7808398950131222316, -0.3162353388693409650, -0.4822834645669289433 ) ) ;
#60642=CARTESIAN_POINT ( 'NONE',  ( -1.371391076115484609, -0.6692913385826771977, 0.1292274648535927661 ) ) ;
#60644=CARTESIAN_POINT ( 'NONE',  ( 1.089238845144357759, 0.05413385826771626580, -0.4176697321401330321 ) ) ;
#60645=CARTESIAN_POINT ( 'NONE',  ( 1.095800524934383846, -0.08942795157528024563, -0.3641732283464568787 ) ) ;
#60648=CARTESIAN_POINT ( 'NONE',  ( -0.6233595800524928121, -0.3162353388693409650, -0.4822834645669289433 ) ) ;
#60650=CARTESIAN_POINT ( 'NONE',  ( 0.2230971128608929543, -0.004921259842519870586, -0.3153832671262229437 ) ) ;
#60651=CARTESIAN_POINT ( 'NONE',  ( -1.135170603674539924, -0.6692913385826771977, 0.1292274648535927661 ) ) ;
#60652=CARTESIAN_POINT ( 'NONE',  ( 1.082677165354331228, -0.5400638737290844871, 0.3530559997133364547 ) ) ;
#60653=CARTESIAN_POINT ( 'NONE',  ( 1.017060367454068581, -0.05778040916215560624, -0.4822834645669293319 ) ) ;
#60654=EDGE_CURVE ( 'NONE', #80968, #41294, #38803, .T. ) ;
#60655=CARTESIAN_POINT ( 'NONE',  ( -0.2559055118110230564, 0.1660481256975883668, -0.3530559997133364547 ) ) ;
#60656=CARTESIAN_POINT ( 'NONE',  ( -0.9973753280839886548, 0.2306618581243848609, 0.2411417322834645549 ) ) ;
#60658=CARTESIAN_POINT ( 'NONE',  ( -1.528871391076114250, 0.2952755905511810774, -0.1292274648535930714 ) ) ;
#60659=CARTESIAN_POINT ( 'NONE',  ( -0.5314960629921250401, 0.1660481256975885056, 0.3530559997133364547 ) ) ;
#60660=CARTESIAN_POINT ( 'NONE',  ( -0.6758530183727028406, 0.1771653543307087630, 0.09757992244046791164 ) ) ;
#60661=CARTESIAN_POINT ( 'NONE',  ( 1.417322834645670104, -0.1870078740157480879, -0.4822834645669291653 ) ) ;
#60663=CARTESIAN_POINT ( 'NONE',  ( 1.568241469816273659, -0.05778040916215560624, -0.4822834645669293319 ) ) ;
#60664=CARTESIAN_POINT ( 'NONE',  ( -0.8464566929133852113, -0.5400638737290845981, -0.3530559997133363437 ) ) ;
#60666=CARTESIAN_POINT ( 'NONE',  ( 0.8989501312335963501, -0.6692913385826773087, -0.1292274648535924053 ) ) ;
#60668=DIRECTION ( 'NONE',  ( -3.096699300667737957E-16, 1.000000000000000000, -0.000000000000000000 ) ) ;
#60669=CARTESIAN_POINT ( 'NONE',  ( -0.006561679790025524116, -0.05778040916215560624, -0.4822834645669293319 ) ) ;
#60670=CARTESIAN_POINT ( 'NONE',  ( -1.207349081364828436, -0.5023911411419708095, 0.1820866141732285504 ) ) ;
#60671=CARTESIAN_POINT ( 'NONE',  ( 0.9645669291338591078, -0.4536011799217368745, -0.2665933059059886201 ) ) ;
#60673=CARTESIAN_POINT ( 'NONE',  ( 1.141732283464567788, -0.5511811023622047445, 6.969142054262312111E-17 ) ) ;
#60674=CARTESIAN_POINT ( 'NONE',  ( 0.9645669291338588858, 0.1660481256975885056, 0.3530559997133364547 ) ) ;
#60676=CARTESIAN_POINT ( 'NONE',  ( -0.4593175853018366950, 0.05413385826771666132, 0.4176697321401328100 ) ) ;
#60677=CARTESIAN_POINT ( 'NONE',  ( 0.4606732211681152100, 1.541615089183626441, 0.5309055118110234117 ) ) ;
#60678=CARTESIAN_POINT ( 'NONE',  ( 1.397637795275591177, -0.4536011799217367080, 0.2665933059059888421 ) ) ;
#60679=CARTESIAN_POINT ( 'NONE',  ( -0.4461942257217840213, 0.2306618581243848609, 0.2411417322834645549 ) ) ;
#60681=CARTESIAN_POINT ( 'NONE',  ( 1.358267716535433323, 0.1660481256975885056, 0.3530559997133364547 ) ) ;
#60682=CARTESIAN_POINT ( 'NONE',  ( 0.2427821522309716595, -0.3162353388693409650, -0.4822834645669289433 ) ) ;
#60683=CARTESIAN_POINT ( 'NONE',  ( 0.3805774278215230400, -0.3690944881889763329, 0.3153832671262228327 ) ) ;
#60685=CARTESIAN_POINT ( 'NONE',  ( 0.3871391076115493490, -0.2845877964562159024, 0.3641732283464567677 ) ) ;
#60688=CARTESIAN_POINT ( 'NONE',  ( 0.6955380577427828781, -0.4281496062992124485, 0.4176697321401328655 ) ) ;
#60690=CARTESIAN_POINT ( 'NONE',  ( 1.548556430446194954, 0.1283753931104746893, -0.1820866141732285504 ) ) ;
#60692=CARTESIAN_POINT ( 'NONE',  ( -0.02624671916010428221, -0.5023911411419708095, 0.1820866141732285504 ) ) ;
#60693=CARTESIAN_POINT ( 'NONE',  ( 0.07874015748031558404, -0.1870078740157479769, 0.4822834645669291653 ) ) ;
#60694=CARTESIAN_POINT ( 'NONE',  ( 1.482939632545932307, -0.3690944881889763329, 0.3153832671262228327 ) ) ;
#60695=CARTESIAN_POINT ( 'NONE',  ( -1.482939632545930975, -0.3690944881889765550, -0.3153832671262227771 ) ) ;
#60696=CARTESIAN_POINT ( 'NONE',  ( -1.272965879265091305, -0.4281496062992124485, 0.4176697321401328655 ) ) ;
#60698=CARTESIAN_POINT ( 'NONE',  ( 0.3937007874015754361, -0.1870078740157479769, 0.4822834645669291653 ) ) ;
#60699=CARTESIAN_POINT ( 'NONE',  ( 1.240157480314961314, 0.1660481256975883668, -0.3530559997133364547 ) ) ;
#60701=CARTESIAN_POINT ( 'NONE',  ( 0.6233595800524939223, -0.3162353388693405765, 0.4822834645669290543 ) ) ;
#60702=CARTESIAN_POINT ( 'NONE',  ( 1.463254593175853824, -0.6692913385826771977, 0.1292274648535927661 ) ) ;
#60703=CARTESIAN_POINT ( 'NONE',  ( 0.8202099737532814183, -0.6692913385826773087, -0.1292274648535924053 ) ) ;
#60704=CARTESIAN_POINT ( 'NONE',  ( -1.699475065616797398, 0.1771653543307087630, 0.09757992244046791164 ) ) ;
#60705=CARTESIAN_POINT ( 'NONE',  ( 0.6824146981627303710, -0.5023911411419708095, 0.1820866141732285504 ) ) ;
#60706=CARTESIAN_POINT ( 'NONE',  ( 1.673228346456693494, 0.1660481256975885056, 0.3530559997133364547 ) ) ;
#60707=CARTESIAN_POINT ( 'NONE',  ( -0.8858267716535425107, -0.4536011799217367080, 0.2665933059059888421 ) ) ;
#60708=CARTESIAN_POINT ( 'NONE',  ( 0.3937007874015754361, -0.1870078740157480601, -0.3641732283464567677 ) ) ;
#60709=CARTESIAN_POINT ( 'NONE',  ( 0.04593175853018440641, -0.6692913385826771977, 0.1292274648535927661 ) ) ;
#60710=CARTESIAN_POINT ( 'NONE',  ( 0.8398950131233602345, 0.2306618581243847221, -0.2411417322834647770 ) ) ;
#60711=CARTESIAN_POINT ( 'NONE',  ( -0.4461942257217840213, -0.6046776061558809534, -0.2411417322834644161 ) ) ;
#60712=CARTESIAN_POINT ( 'NONE',  ( 0.07874015748031558404, -0.1870078740157480601, -0.3641732283464567677 ) ) ;
#60713=CARTESIAN_POINT ( 'NONE',  ( 0.8989501312335963501, -0.6692913385826773087, -0.1292274648535924053 ) ) ;
#60714=( BOUNDED_CURVE ( )  B_SPLINE_CURVE ( 2, ( #54441, #15758, #14918, #41000, #72158, #65441, #2286, #65850, #2700, #28360, #67095, #7774, #8183 ),
 .UNSPECIFIED., .F., .F. ) 
 B_SPLINE_CURVE_WITH_KNOTS ( ( 3, 2, 2, 2, 2, 2, 3 ),
 ( 0.3096947309984372509, 0.3106060606060606077, 0.3143939393939393923, 0.3181818181818181768, 0.3219696969696969613, 0.3257575757575757458, 0.3266689053651991581 ),
 .UNSPECIFIED. ) 
 CURVE ( )  GEOMETRIC_REPRESENTATION_ITEM ( )  RATIONAL_B_SPLINE_CURVE ( ( 0.9875488213027530104, 0.9918020599134685922, 1.000000000000000000, 0.9659258262890683122, 1.000000000000000000, 0.9659258262890683122, 1.000000000000000000, 0.9659258262890683122, 1.000000000000000000, 0.9659258262890683122, 1.000000000000000000, 0.9918020599134680371, 0.9875488213027523443 ) ) 
 REPRESENTATION_ITEM ( '' )  );
#60716=CARTESIAN_POINT ( 'NONE',  ( -0.8202099737532801971, -0.6692913385826771977, 0.1292274648535927661 ) ) ;
#60720=CARTESIAN_POINT ( 'NONE',  ( -0.6167979002624665030, -0.4281496062992127816, -0.4176697321401328100 ) ) ;
#60721=CARTESIAN_POINT ( 'NONE',  ( -0.3674540682414692561, -0.6046776061558809534, -0.2411417322834644161 ) ) ;
#60724=EDGE_LOOP ( 'NONE', ( #13529, #39086, #50069, #2752, #1097, #16792, #57589, #40653, #74933, #15130, #15619, #64049, #8235, #39796, #25617, #71601, #67701, #76094, #22130, #12316 ) ) ;
#60725=CARTESIAN_POINT ( 'NONE',  ( 0.7742782152230979209, -0.004921259842519870586, -0.3153832671262229437 ) ) ;
#60727=CARTESIAN_POINT ( 'NONE',  ( 1.253280839895013710, -0.3162353388693405765, 0.4822834645669290543 ) ) ;
#60729=CARTESIAN_POINT ( 'NONE',  ( -1.266404199475064773, -0.2845877964562159024, 0.3641732283464567677 ) ) ;
#60730=CARTESIAN_POINT ( 'NONE',  ( 1.561679790026247350, 0.05413385826771626580, -0.4176697321401330321 ) ) ;
#60731=CARTESIAN_POINT ( 'NONE',  ( -1.489501312335957062, -0.3162353388693409650, -0.4822834645669289433 ) ) ;
#60732=CARTESIAN_POINT ( 'NONE',  ( 0.3083989501312343062, -0.05778040916215560624, -0.4822834645669293319 ) ) ;
#60734=CARTESIAN_POINT ( 'NONE',  ( -0.1771653543307080136, 0.1660481256975883668, -0.3530559997133364547 ) ) ;
#60735=CARTESIAN_POINT ( 'NONE',  ( -0.8202099737532801971, -0.5511811023622046335, 0.09757992244046803654 ) ) ;
#60736=CARTESIAN_POINT ( 'NONE',  ( 0.9908136482939640111, 0.2952755905511810774, -0.1292274648535930714 ) ) ;
#60738=CARTESIAN_POINT ( 'NONE',  ( 0.1049868766404206816, -0.6046776061558809534, -0.2411417322834644161 ) ) ;
#60741=CARTESIAN_POINT ( 'NONE',  ( 0.9514435695538062676, -0.3162353388693409650, -0.4822834645669289433 ) ) ;
#60742=CARTESIAN_POINT ( 'NONE',  ( 0.04593175853018440641, 0.2952755905511810774, -0.1292274648535930714 ) ) ;
#60743=CARTESIAN_POINT ( 'NONE',  ( -0.9186351706036736120, -0.6046776061558809534, -0.2411417322834644161 ) ) ;
#60744=CARTESIAN_POINT ( 'NONE',  ( 1.122047244094488860, 0.1660481256975885056, 0.3530559997133364547 ) ) ;
#60745=CARTESIAN_POINT ( 'NONE',  ( 0.9908136482939640111, -0.6692913385826771977, 0.1292274648535927661 ) ) ;
#60747=CARTESIAN_POINT ( 'NONE',  ( -0.4855643044619415427, -0.4281496062992124485, 0.4176697321401328655 ) ) ;
#60748=CARTESIAN_POINT ( 'NONE',  ( 0.4461942257217856311, 0.2306618581243847221, -0.2411417322834647770 ) ) ;
#60749=CARTESIAN_POINT ( 'NONE',  ( 0.06561679790026316017, -0.4281496062992124485, 0.4176697321401328655 ) ) ;
#60750=CARTESIAN_POINT ( 'NONE',  ( 0.9251968503937015864, 0.07958543189024071263, -0.2665933059059888421 ) ) ;
#60751=CARTESIAN_POINT ( 'NONE',  ( -1.213910761154854745, 0.2952755905511810774, -0.1292274648535930714 ) ) ;
#60753=CARTESIAN_POINT ( 'NONE',  ( 0.4986876640419954376, 0.2306618581243848609, 0.2411417322834645549 ) ) ;
#60759=CARTESIAN_POINT ( 'NONE',  ( 0.9448818897637802916, -0.1870078740157480879, -0.4822834645669291653 ) ) ;
#60760=CARTESIAN_POINT ( 'NONE',  ( 0.5380577427821529035, -0.004921259842519870586, -0.3153832671262229437 ) ) ;
#60761=CARTESIAN_POINT ( 'NONE',  ( -1.171093442848938793, -2.191421614605370878E-15, 0.4445507791589071167 ) ) ;
#60767=CARTESIAN_POINT ( 'NONE',  ( -0.8202099737532799750, 0.2952755905511810774, -0.1292274648535930714 ) ) ;
#60768=CARTESIAN_POINT ( 'NONE',  ( -0.7152230971128602510, -0.05778040916215560624, -0.4822834645669293319 ) ) ;
#60769=CARTESIAN_POINT ( 'NONE',  ( 0.5511811023622054106, -0.1870078740157480879, -0.4822834645669291653 ) ) ;
#60770=ORIENTED_EDGE ( 'NONE', *, *, #37751, .T. ) ;
#60771=CARTESIAN_POINT ( 'NONE',  ( 1.312335958005249825, 0.2306618581243847221, -0.2411417322834647770 ) ) ;
#60772=CARTESIAN_POINT ( 'NONE',  ( 1.692913385826772421, 0.1771653543307087630, 0.000000000000000000 ) ) ;
#60774=CARTESIAN_POINT ( 'NONE',  ( -1.586052503253848389, 0.7480314960629931287, -0.1653254495020559933 ) ) ;
#60776=CARTESIAN_POINT ( 'NONE',  ( -1.469816272965878357, 0.1283753931104748280, 0.1820866141732283561 ) ) ;
#60778=CARTESIAN_POINT ( 'NONE',  ( 0.2559055118110243332, 0.1660481256975885056, 0.3530559997133364547 ) ) ;
#60781=CARTESIAN_POINT ( 'NONE',  ( -1.095800524934382292, -0.08942795157527998196, 0.3641732283464567121 ) ) ;
#60782=CARTESIAN_POINT ( 'NONE',  ( 0.6692913385826778638, -0.6692913385826771977, 8.415575281601705876E-17 ) ) ;
#60783=CARTESIAN_POINT ( 'NONE',  ( 1.410761154855643795, -0.2845877964562159024, 0.3641732283464567677 ) ) ;
#60785=CARTESIAN_POINT ( 'NONE',  ( -1.423884514435694859, -0.2845877964562159024, 0.3641732283464567677 ) ) ;
#60786=CARTESIAN_POINT ( 'NONE',  ( 1.515748031496063408, 0.1660481256975885056, 0.3530559997133364547 ) ) ;
#60788=CARTESIAN_POINT ( 'NONE',  ( -0.2493438320209966919, 0.05413385826771626580, -0.4176697321401330321 ) ) ;
#60789=CARTESIAN_POINT ( 'NONE',  ( -1.417322834645668772, -0.1870078740157480601, -0.3641732283464567677 ) ) ;
#60790=CARTESIAN_POINT ( 'NONE',  ( -0.3674540682414692561, -0.5023911411419708095, -0.1820866141732282451 ) ) ;
#60791=CARTESIAN_POINT ( 'NONE',  ( -0.4068241469816267775, 0.05413385826771626580, -0.4176697321401330321 ) ) ;
#60792=CARTESIAN_POINT ( 'NONE',  ( -1.568241469816272105, -0.2845877964562161244, -0.3641732283464567121 ) ) ;
#60794=CARTESIAN_POINT ( 'NONE',  ( 0.2690288713910767848, -0.6692913385826773087, -0.1292274648535924053 ) ) ;
#60796=CARTESIAN_POINT ( 'NONE',  ( -1.102362204724408601, -0.1870078740157479769, 0.4822834645669291653 ) ) ;
#60797=CARTESIAN_POINT ( 'NONE',  ( -0.5971128608923877978, 0.1771653543307087630, 0.09757992244046791164 ) ) ;
#60798=CARTESIAN_POINT ( 'NONE',  ( -1.561679790026246017, -0.4281496062992127816, -0.4176697321401328100 ) ) ;
#60799=CARTESIAN_POINT ( 'NONE',  ( -0.08530183727034056085, -0.3162353388693405765, 0.4822834645669290543 ) ) ;
#60800=CARTESIAN_POINT ( 'NONE',  ( 0.4461942257217856311, 0.1283753931104746893, -0.1820866141732285504 ) ) ;
#60801=CARTESIAN_POINT ( 'NONE',  ( -0.8923884514435688198, 0.1283753931104746893, -0.1820866141732285504 ) ) ;
#60802=CARTESIAN_POINT ( 'NONE',  ( -1.154855643044618851, -0.6046776061558809534, -0.2411417322834644161 ) ) ;
#60803=CARTESIAN_POINT ( 'NONE',  ( -1.391076115485563758, 0.2306618581243848609, 0.2411417322834645549 ) ) ;
#60804=CARTESIAN_POINT ( 'NONE',  ( 1.489501312335958172, -0.3162353388693405765, 0.4822834645669290543 ) ) ;
#60806=CARTESIAN_POINT ( 'NONE',  ( 0.8005249343832028242, -0.3690944881889765550, -0.3153832671262227771 ) ) ;
#60808=CARTESIAN_POINT ( 'NONE',  ( 0.9055118110236227702, 0.2952755905511811885, 0.000000000000000000 ) ) ;
#60809=DIRECTION ( 'NONE',  ( 0.000000000000000000, -1.000000000000000000, 0.000000000000000000 ) ) ;
#60810=CARTESIAN_POINT ( 'NONE',  ( 1.555118110236221041, -0.4536011799217367080, 0.2665933059059888421 ) ) ;
#60811=AXIS2_PLACEMENT_3D ( 'NONE', #9790, #17367, #15708 ) ;
#60813=CARTESIAN_POINT ( 'NONE',  ( -0.9055118110236215490, -0.6692913385826771977, 8.415575281601705876E-17 ) ) ;
#60814=CARTESIAN_POINT ( 'NONE',  ( -0.8005249343832011588, 0.05413385826771626580, -0.4176697321401330321 ) ) ;
#60815=CARTESIAN_POINT ( 'NONE',  ( 0.4330708661417329575, -0.6692913385826771977, 8.415575281601705876E-17 ) ) ;
#60816=CARTESIAN_POINT ( 'NONE',  ( -1.286089238845143479, -0.5023911411419708095, 0.1820866141732285504 ) ) ;
#60818=CARTESIAN_POINT ( 'NONE',  ( -1.286089238845143479, -0.6046776061558807314, 0.2411417322834647770 ) ) ;
#60819=CARTESIAN_POINT ( 'NONE',  ( 0.2887139107611556010, 0.2306618581243847221, -0.2411417322834647770 ) ) ;
#60820=CARTESIAN_POINT ( 'NONE',  ( 0.05249343832021075018, -0.6046776061558807314, 0.2411417322834647770 ) ) ;
#60821=CARTESIAN_POINT ( 'NONE',  ( 0.8398950131233602345, 0.2306618581243847221, -0.2411417322834647770 ) ) ;
#60822=CARTESIAN_POINT ( 'NONE',  ( 1.614173228346457156, 1.496062992125984037, -0.5309055118110239668 ) ) ;
#60828=CARTESIAN_POINT ( 'NONE',  ( -0.2427821522309703550, -0.08942795157528024563, -0.3641732283464568787 ) ) ;
#60829=CARTESIAN_POINT ( 'NONE',  ( -0.2296587926509179312, -0.3162353388693409650, -0.4822834645669289433 ) ) ;
#60830=CARTESIAN_POINT ( 'NONE',  ( 0.6955380577427828781, 0.05413385826771626580, -0.4176697321401330321 ) ) ;
#60832=CARTESIAN_POINT ( 'NONE',  ( 0.1574803149606306130, -0.1870078740157480601, -0.3641732283464567677 ) ) ;
#60833=CARTESIAN_POINT ( 'NONE',  ( -1.325459317585300889, 0.05413385826771666132, 0.4176697321401328100 ) ) ;
#60834=CARTESIAN_POINT ( 'NONE',  ( 1.148293963254593653, 0.2952755905511810774, -0.1292274648535930714 ) ) ;
#60837=CARTESIAN_POINT ( 'NONE',  ( 1.204164820379012069, 1.535433070866141447, -0.4915354330708657793 ) ) ;
#60838=ORIENTED_EDGE ( 'NONE', *, *, #39775, .T. ) ;
#60839=ORIENTED_EDGE ( 'NONE', *, *, #65705, .T. ) ;
#60840=CARTESIAN_POINT ( 'NONE',  ( 1.036745406824147508, -0.4281496062992127816, -0.4176697321401328100 ) ) ;
#60841=CARTESIAN_POINT ( 'NONE',  ( -1.627296587926508442, -0.6046776061558809534, -0.2411417322834644161 ) ) ;
#60842=CARTESIAN_POINT ( 'NONE',  ( -1.207349081364828436, -0.5023911411419708095, 0.1820866141732285504 ) ) ;
#60843=CARTESIAN_POINT ( 'NONE',  ( -1.233595800524933894, -0.6046776061558809534, -0.2411417322834644161 ) ) ;
#60845=DIRECTION ( 'NONE',  ( 0.000000000000000000, 0.000000000000000000, 1.000000000000000000 ) ) ;
#60846=CARTESIAN_POINT ( 'NONE',  ( 1.430446194225722500, -0.4281496062992127816, -0.4176697321401328100 ) ) ;
#60847=CARTESIAN_POINT ( 'NONE',  ( -1.627296587926508442, -0.6046776061558809534, -0.2411417322834644161 ) ) ;
#60848=CARTESIAN_POINT ( 'NONE',  ( -0.1771653543307080136, -0.5400638737290844871, 0.3530559997133364547 ) ) ;
#60849=CARTESIAN_POINT ( 'NONE',  ( -0.4986876640419942164, -0.6046776061558807314, 0.2411417322834647770 ) ) ;
#60850=CARTESIAN_POINT ( 'NONE',  ( -1.496062992125983815, -0.1870078740157479769, 0.4822834645669291653 ) ) ;
#60852=CARTESIAN_POINT ( 'NONE',  ( 0.3674540682414705883, 0.2306618581243847221, -0.2411417322834647770 ) ) ;
#60854=CARTESIAN_POINT ( 'NONE',  ( -1.437007874015747477, 0.07958543189024071263, -0.2665933059059888421 ) ) ;
#60859=CARTESIAN_POINT ( 'NONE',  ( -1.535433070866141225, 0.2952755905511811885, 0.000000000000000000 ) ) ;
#60861=CARTESIAN_POINT ( 'NONE',  ( 1.607611548556431069, -0.5511811023622048555, -0.09757992244046775898 ) ) ;
#60862=CARTESIAN_POINT ( 'NONE',  ( -1.555118110236219930, 0.1660481256975885056, 0.3530559997133364547 ) ) ;
#60867=CARTESIAN_POINT ( 'NONE',  ( -0.4790026246719152336, -0.08942795157528024563, -0.3641732283464568787 ) ) ;
#60868=CARTESIAN_POINT ( 'NONE',  ( -0.6036745406824141069, 0.1283753931104748280, 0.1820866141732283561 ) ) ;
#60869=CARTESIAN_POINT ( 'NONE',  ( -1.286089238845143479, 0.2306618581243847221, -0.2411417322834647770 ) ) ;
#60870=CARTESIAN_POINT ( 'NONE',  ( 0.6824146981627303710, 0.2306618581243847221, -0.2411417322834647770 ) ) ;
#60871=CARTESIAN_POINT ( 'NONE',  ( -1.023622047244093558, -0.1870078740157479769, 0.4822834645669291653 ) ) ;
#60874=EDGE_CURVE ( 'NONE', #81247, #21404, #45939, .T. ) ;
#60875=CARTESIAN_POINT ( 'NONE',  ( -1.502624671916009680, -0.3162353388693405765, 0.4822834645669290543 ) ) ;
#60879=CARTESIAN_POINT ( 'NONE',  ( -1.604771003085130321, 1.044625174762916719, -0.1466069496707741726 ) ) ;
#60883=CARTESIAN_POINT ( 'NONE',  ( -0.6299212598425188991, -0.1870078740157480879, -0.4822834645669291653 ) ) ;
#60884=CARTESIAN_POINT ( 'NONE',  ( 1.286089238845145033, -0.6046776061558809534, -0.2411417322834644161 ) ) ;
#60886=CARTESIAN_POINT ( 'NONE',  ( -1.614173228346456268, -0.6692913385826771977, 8.415575281601705876E-17 ) ) ;
#60888=CARTESIAN_POINT ( 'NONE',  ( -1.332020997375327642, -0.3162353388693409650, -0.4822834645669289433 ) ) ;
#60889=CARTESIAN_POINT ( 'NONE',  ( -0.7020997375328076329, -0.3162353388693409650, -0.4822834645669289433 ) ) ;
#60891=CARTESIAN_POINT ( 'NONE',  ( 0.2952755905511816326, -0.4536011799217367080, 0.2665933059059888421 ) ) ;
#60893=CARTESIAN_POINT ( 'NONE',  ( 0.1181102362204730916, 0.1771653543307087630, 0.000000000000000000 ) ) ;
#60894=CARTESIAN_POINT ( 'NONE',  ( 1.148293963254593653, 0.1771653543307087075, -0.09757992244046823083 ) ) ;
#60895=CARTESIAN_POINT ( 'NONE',  ( 0.9251968503937015864, -0.5400638737290844871, 0.3530559997133364547 ) ) ;
#60896=CARTESIAN_POINT ( 'NONE',  ( -0.1706036745406816491, -0.004921259842519870586, -0.3153832671262229437 ) ) ;
#60898=CARTESIAN_POINT ( 'NONE',  ( 1.469816272965879911, 0.2306618581243847221, -0.2411417322834647770 ) ) ;
#60900=CARTESIAN_POINT ( 'NONE',  ( -1.272965879265091305, -0.004921259842519870586, -0.3153832671262229437 ) ) ;
#60903=CARTESIAN_POINT ( 'NONE',  ( -0.1706036745406816491, 0.05413385826771626580, -0.4176697321401330321 ) ) ;
#60905=CARTESIAN_POINT ( 'NONE',  ( 0.6627296587926515548, 0.1771653543307087630, 0.09757992244046791164 ) ) ;
#60906=CARTESIAN_POINT ( 'NONE',  ( -0.09842519685039295696, 0.07958543189024071263, -0.2665933059059888421 ) ) ;
#60907=CARTESIAN_POINT ( 'NONE',  ( -0.6102362204724400829, -0.5400638737290845981, -0.3530559997133363437 ) ) ;
#60908=CARTESIAN_POINT ( 'NONE',  ( 0.6986524979670498681, 8.471767977567108961E-16, -0.4445507791589058955 ) ) ;
#60910=CARTESIAN_POINT ( 'NONE',  ( 0.09186351706036827158, 0.05413385826771666132, 0.4176697321401328100 ) ) ;
#60913=CARTESIAN_POINT ( 'NONE',  ( 0.2262115530851599166, 8.471767977567108961E-16, -0.4445507791589058955 ) ) ;
#60914=CARTESIAN_POINT ( 'NONE',  ( -0.4330708661417315697, 0.1771653543307087630, 0.000000000000000000 ) ) ;
#60915=CARTESIAN_POINT ( 'NONE',  ( 0.05249343832021075018, 0.2306618581243847221, -0.2411417322834647770 ) ) ;
#60916=CARTESIAN_POINT ( 'NONE',  ( -1.410761154855641575, -0.3162353388693409650, -0.4822834645669289433 ) ) ;
#60917=CARTESIAN_POINT ( 'NONE',  ( -1.627296587926508442, 0.1283753931104748280, 0.1820866141732283561 ) ) ;
#60918=CARTESIAN_POINT ( 'NONE',  ( 1.279527559055118724, -0.5400638737290845981, -0.3530559997133363437 ) ) ;
#60919=CARTESIAN_POINT ( 'NONE',  ( -1.325459317585300889, 0.05413385826771666132, 0.4176697321401328100 ) ) ;
#60920=CARTESIAN_POINT ( 'NONE',  ( -0.5905511811023615998, 0.1771653543307087630, 0.000000000000000000 ) ) ;
#60923=AXIS2_PLACEMENT_3D ( 'NONE', #35523, #15769, #29614 ) ;
#60925=CARTESIAN_POINT ( 'NONE',  ( 1.528871391076116026, 0.1771653543307087630, 0.09757992244046791164 ) ) ;
#60926=CARTESIAN_POINT ( 'NONE',  ( 1.115485564304462551, -0.004921259842519576551, 0.3153832671262227771 ) ) ;
#60927=CARTESIAN_POINT ( 'NONE',  ( -1.692913385826770645, 0.2952755905511811885, 0.000000000000000000 ) ) ;
#60928=CARTESIAN_POINT ( 'NONE',  ( 0.7349081364829402885, -0.6046776061558809534, -0.2411417322834644161 ) ) ;
#60930=CARTESIAN_POINT ( 'NONE',  ( 1.325459317585302665, -0.3690944881889763329, 0.3153832671262228327 ) ) ;
#60931=CARTESIAN_POINT ( 'NONE',  ( 0.2165354330708668673, -0.5400638737290844871, 0.3530559997133364547 ) ) ;
#60932=CARTESIAN_POINT ( 'NONE',  ( -0.9251968503937002541, -0.5400638737290845981, -0.3530559997133363437 ) ) ;
#60936=CARTESIAN_POINT ( 'NONE',  ( 0.4199475065616803948, -0.5023911411419708095, -0.1820866141732282451 ) ) ;
#60940=CARTESIAN_POINT ( 'NONE',  ( -0.5839895013123351797, 0.2952755905511810774, -0.1292274648535930714 ) ) ;
#60941=CARTESIAN_POINT ( 'NONE',  ( -0.3346456692913377662, 0.1660481256975883668, -0.3530559997133364547 ) ) ;
#60942=CARTESIAN_POINT ( 'NONE',  ( -0.1837270341207340729, 0.1283753931104746893, -0.1820866141732285504 ) ) ;
#60943=CARTESIAN_POINT ( 'NONE',  ( 0.6102362204724416372, 0.1660481256975883668, -0.3530559997133364547 ) ) ;
#60944=CARTESIAN_POINT ( 'NONE',  ( -1.003937007874014853, 0.1660481256975885056, 0.3530559997133364547 ) ) ;
#60945=CARTESIAN_POINT ( 'NONE',  ( -0.1968503937007867743, -0.6692913385826771977, 8.415575281601705876E-17 ) ) ;
#60946=CARTESIAN_POINT ( 'NONE',  ( 1.069553805774278610, -0.6692913385826771977, 0.1292274648535927661 ) ) ;
#60947=CARTESIAN_POINT ( 'NONE',  ( 1.036745406824147508, -0.4281496062992127816, -0.4176697321401328100 ) ) ;
#60948=EDGE_CURVE ( 'NONE', #34118, #80835, #72151, .T. ) ;
#60949=CARTESIAN_POINT ( 'NONE',  ( 0.8595800524934390507, -0.3162353388693405765, 0.4822834645669290543 ) ) ;
#60951=CARTESIAN_POINT ( 'NONE',  ( 0.1902887139107617975, -0.5511811023622048555, -0.09757992244046775898 ) ) ;
#60955=CARTESIAN_POINT ( 'NONE',  ( -1.069553805774277722, 0.1771653543307087630, 0.09757992244046791164 ) ) ;
#60956=CARTESIAN_POINT ( 'NONE',  ( -0.5971128608923877978, -0.6692913385826773087, -0.1292274648535924053 ) ) ;
#60958=CARTESIAN_POINT ( 'NONE',  ( -0.2165354330708654795, -0.5400638737290845981, -0.3530559997133363437 ) ) ;
#60959=CARTESIAN_POINT ( 'NONE',  ( -0.6167979002624665030, 0.05413385826771666132, 0.4176697321401328100 ) ) ;
#60960=CARTESIAN_POINT ( 'NONE',  ( -1.148293963254592542, 0.2952755905511811885, 0.1292274648535926551 ) ) ;
#60961=CARTESIAN_POINT ( 'NONE',  ( -1.305774278215222184, -0.6692913385826773087, -0.1292274648535924053 ) ) ;
#60962=CARTESIAN_POINT ( 'NONE',  ( 0.8661417322834653598, -0.1870078740157479769, 0.3641732283464567677 ) ) ;
#60965=CARTESIAN_POINT ( 'NONE',  ( 0.3674540682414705883, 0.1283753931104746893, -0.1820866141732285504 ) ) ;
#60966=CARTESIAN_POINT ( 'NONE',  ( 0.02624671916010564918, -0.6046776061558809534, -0.2411417322834644161 ) ) ;
#60967=CARTESIAN_POINT ( 'NONE',  ( 0.3346456692913393205, -0.5400638737290845981, -0.3530559997133363437 ) ) ;
#60971=EDGE_LOOP ( 'NONE', ( #53800, #48747, #40217, #19240 ) ) ;
#60974=CARTESIAN_POINT ( 'NONE',  ( -0.7611548556430438595, 0.1283753931104748280, 0.1820866141732283561 ) ) ;
#60975=CARTESIAN_POINT ( 'NONE',  ( -1.128608923884513837, -0.6046776061558807314, 0.2411417322834647770 ) ) ;
#60977=EDGE_CURVE ( 'NONE', #3487, #38656, #11759, .T. ) ;
#60979=CARTESIAN_POINT ( 'NONE',  ( -1.574803149606298192, -0.1870078740157480601, -0.3641732283464567677 ) ) ;
#60980=CARTESIAN_POINT ( 'NONE',  ( 0.8202099737532813073, 0.2952755905511811885, 0.1292274648535926551 ) ) ;
#60981=CARTESIAN_POINT ( 'NONE',  ( 0.4986876640419954376, -0.6046776061558809534, -0.2411417322834644161 ) ) ;
#60982=CARTESIAN_POINT ( 'NONE',  ( -0.5839895013123351797, -0.5511811023622046335, 0.09757992244046803654 ) ) ;
#60983=CARTESIAN_POINT ( 'NONE',  ( 0.09842519685039434474, -0.5400638737290845981, -0.3530559997133363437 ) ) ;
#60985=CARTESIAN_POINT ( 'NONE',  ( -0.2230971128608915943, -0.004921259842519576551, 0.3153832671262227771 ) ) ;
#60986=CARTESIAN_POINT ( 'NONE',  ( -0.4461942257217840213, 0.2306618581243848609, 0.2411417322834645549 ) ) ;
#60989=CARTESIAN_POINT ( 'NONE',  ( 1.522309711286089939, -0.5023911411419708095, -0.1820866141732282451 ) ) ;
#60990=CARTESIAN_POINT ( 'NONE',  ( -0.09186351706036689768, -0.004921259842519870586, -0.3153832671262229437 ) ) ;
#60991=CARTESIAN_POINT ( 'NONE',  ( 1.574803149606299746, -0.1870078740157480601, -0.3641732283464567677 ) ) ;
#60992=CARTESIAN_POINT ( 'NONE',  ( -0.9842519685039365918, -0.6692913385826771977, 8.415575281601705876E-17 ) ) ;
#60993=CARTESIAN_POINT ( 'NONE',  ( -0.8923884514435688198, -0.5023911411419708095, 0.1820866141732285504 ) ) ;
#60995=CARTESIAN_POINT ( 'NONE',  ( -1.200787401574802349, 0.1660481256975883668, -0.3530559997133364547 ) ) ;
#60996=CARTESIAN_POINT ( 'NONE',  ( -0.3543307086614165824, 0.2952755905511811885, 0.000000000000000000 ) ) ;
#60997=EDGE_CURVE ( 'NONE', #19450, #82899, #83190, .T. ) ;
#60998=CARTESIAN_POINT ( 'NONE',  ( 0.4396325459317593221, 0.2952755905511810774, -0.1292274648535930714 ) ) ;
#61001=CARTESIAN_POINT ( 'NONE',  ( 0.3477690288713918276, -0.5511811023622048555, -0.09757992244046775898 ) ) ;
#61002=CARTESIAN_POINT ( 'NONE',  ( 1.003937007874016185, 0.1660481256975883668, -0.3530559997133364547 ) ) ;
#61003=CARTESIAN_POINT ( 'NONE',  ( -1.364829396325458521, 0.1283753931104746893, -0.1820866141732285504 ) ) ;
#61004=CARTESIAN_POINT ( 'NONE',  ( 1.082677165354331228, 0.1660481256975883668, -0.3530559997133364547 ) ) ;
#61005=CARTESIAN_POINT ( 'NONE',  ( -1.430446194225721390, -0.3690944881889763329, 0.3153832671262228327 ) ) ;
#61006=CARTESIAN_POINT ( 'NONE',  ( -0.4068241469816267775, 0.05413385826771626580, -0.4176697321401330321 ) ) ;
#61007=CARTESIAN_POINT ( 'NONE',  ( 0.1640419947506569498, -0.2845877964562161244, -0.3641732283464567121 ) ) ;
#61008=CARTESIAN_POINT ( 'NONE',  ( -0.8761506516392493227, -2.567464376874931580E-15, -0.4445507791589072832 ) ) ;
#61009=CARTESIAN_POINT ( 'NONE',  ( 0.4790026246719167324, -0.08942795157527998196, 0.3641732283464567121 ) ) ;
#61010=CARTESIAN_POINT ( 'NONE',  ( -0.1968503937007867743, 0.2952755905511811885, 0.000000000000000000 ) ) ;
#61012=CARTESIAN_POINT ( 'NONE',  ( -1.089238845144356427, 0.05413385826771666132, 0.4176697321401328100 ) ) ;
#61014=CARTESIAN_POINT ( 'NONE',  ( 0.9514435695538062676, -0.08942795157527998196, 0.3641732283464567121 ) ) ;
#61015=CARTESIAN_POINT ( 'NONE',  ( 0.006561679790026889343, -0.3162353388693409650, -0.4822834645669289433 ) ) ;
#61016=CARTESIAN_POINT ( 'NONE',  ( -0.1049868766404193215, -0.6046776061558807314, 0.2411417322834647770 ) ) ;
#61017=CARTESIAN_POINT ( 'NONE',  ( -0.2427821522309703550, -0.2845877964562159024, 0.3641732283464567677 ) ) ;
#61019=CARTESIAN_POINT ( 'NONE',  ( -0.3280839895013117347, -0.004921259842519870586, -0.3153832671262229437 ) ) ;
#61020=CARTESIAN_POINT ( 'NONE',  ( 0.4855643044619430415, -0.4281496062992127816, -0.4176697321401328100 ) ) ;
#61022=CARTESIAN_POINT ( 'NONE',  ( -1.240157480314959759, 0.07958543189024085140, 0.2665933059059887866 ) ) ;
#61024=CARTESIAN_POINT ( 'NONE',  ( -1.049868766404198794, -0.6046776061558807314, 0.2411417322834647770 ) ) ;
#61027=AXIS2_PLACEMENT_3D ( 'NONE', #39178, #64862, #58540 ) ;
#61028=ADVANCED_FACE ( 'NONE', ( #72727 ), #64194, .F. ) ;
#61029=CARTESIAN_POINT ( 'NONE',  ( -1.646981627296586703, -0.2845877964562161244, -0.3641732283464567121 ) ) ;
#61030=CARTESIAN_POINT ( 'NONE',  ( -0.5708661417322828946, 0.1660481256975883668, -0.3530559997133364547 ) ) ;
#61032=CARTESIAN_POINT ( 'NONE',  ( -1.325459317585300889, 0.05413385826771666132, 0.4176697321401328100 ) ) ;
#61035=CARTESIAN_POINT ( 'NONE',  ( 1.541994750656168645, 0.2952755905511810774, -0.1292274648535930714 ) ) ;
#61036=CARTESIAN_POINT ( 'NONE',  ( 0.9055118110236227702, 0.2952755905511811885, 0.000000000000000000 ) ) ;
#61039=CARTESIAN_POINT ( 'NONE',  ( -1.620734908136482577, -0.6692913385826773087, -0.1292274648535924053 ) ) ;
#61042=CARTESIAN_POINT ( 'NONE',  ( -0.6496062992125976043, 0.07958543189024071263, -0.2665933059059888421 ) ) ;
#61045=ORIENTED_EDGE ( 'NONE', *, *, #63677, .F. ) ;
#61046=CARTESIAN_POINT ( 'NONE',  ( 0.8202099737532813073, 0.2952755905511811885, 0.1292274648535926551 ) ) ;
#61047=CARTESIAN_POINT ( 'NONE',  ( -0.4461942257217840213, 0.2306618581243848609, 0.2411417322834645549 ) ) ;
#61048=CARTESIAN_POINT ( 'NONE',  ( -1.167979002624671470, 0.05413385826771666132, 0.4176697321401328100 ) ) ;
#61049=CARTESIAN_POINT ( 'NONE',  ( 1.627296587926509996, -0.6046776061558807314, 0.2411417322834647770 ) ) ;
#61050=CARTESIAN_POINT ( 'NONE',  ( -1.220472440944881054, -0.5511811023622047445, 6.969142054262312111E-17 ) ) ;
#61052=CARTESIAN_POINT ( 'NONE',  ( 0.4330708661417329575, 0.2952755905511811885, 0.000000000000000000 ) ) ;
#61053=CARTESIAN_POINT ( 'NONE',  ( -0.7677165354330699465, -0.5400638737290845981, -0.3530559997133363437 ) ) ;
#61055=CARTESIAN_POINT ( 'NONE',  ( -1.384514435695537005, -0.6692913385826773087, -0.1292274648535924053 ) ) ;
#61057=CARTESIAN_POINT ( 'NONE',  ( 0.9186351706036752773, 0.2306618581243847221, -0.2411417322834647770 ) ) ;
#61058=CARTESIAN_POINT ( 'NONE',  ( 1.443569553805774897, -0.5023911411419708095, -0.1820866141732282451 ) ) ;
#61061=CARTESIAN_POINT ( 'NONE',  ( -0.3412073490813641308, 0.2306618581243847221, -0.2411417322834647770 ) ) ;
#61062=EDGE_LOOP ( 'NONE', ( #46054, #222, #77737, #27188 ) ) ;
#61063=CARTESIAN_POINT ( 'NONE',  ( 0.5708661417322841158, -0.4536011799217368745, -0.2665933059059886201 ) ) ;
#61064=CARTESIAN_POINT ( 'NONE',  ( -1.299212598425196097, -0.6692913385826771977, 8.415575281601705876E-17 ) ) ;
#61065=CARTESIAN_POINT ( 'NONE',  ( 1.023622047244095112, -0.1870078740157480879, -0.4822834645669291653 ) ) ;
#61066=CARTESIAN_POINT ( 'NONE',  ( 0.8792650918635177559, -0.4281496062992127816, -0.4176697321401328100 ) ) ;
#61067=CARTESIAN_POINT ( 'NONE',  ( -0.02624671916010428221, -0.6046776061558807314, 0.2411417322834647770 ) ) ;
#61069=CARTESIAN_POINT ( 'NONE',  ( -0.5905511811023613777, -0.6692913385826771977, 8.415575281601705876E-17 ) ) ;
#61071=CARTESIAN_POINT ( 'NONE',  ( -1.679790026246718693, 0.2306618581243847221, -0.2411417322834647770 ) ) ;
#61072=CARTESIAN_POINT ( 'NONE',  ( -1.003937007874014853, 0.1660481256975885056, 0.3530559997133364547 ) ) ;
#61073=CARTESIAN_POINT ( 'NONE',  ( 1.148293963254593875, -0.6692913385826771977, 0.1292274648535927661 ) ) ;
#61074=CARTESIAN_POINT ( 'NONE',  ( 1.397637795275591177, 0.1660481256975883668, -0.3530559997133364547 ) ) ;
#61075=CARTESIAN_POINT ( 'NONE',  ( -1.030183727034119867, -0.05778040916215560624, -0.4822834645669293319 ) ) ;
#61076=B_SPLINE_CURVE_WITH_KNOTS ( 'NONE', 3,
 ( #21989, #23221, #48891, #47650 ),
 .UNSPECIFIED., .F., .F.,
 ( 4, 4 ),
 ( 3.210432057660995851E-07, 0.001287787053612144111 ),
 .UNSPECIFIED. ) ;
#61078=CARTESIAN_POINT ( 'NONE',  ( 0.2099737532808405305, 0.2306618581243847221, -0.2411417322834647770 ) ) ;
#61080=CARTESIAN_POINT ( 'NONE',  ( -0.5446194225721777693, -0.05778040916215522460, 0.4822834645669289988 ) ) ;
#61081=CARTESIAN_POINT ( 'NONE',  ( 1.594488188976378673, -0.5400638737290845981, -0.3530559997133363437 ) ) ;
#61082=CARTESIAN_POINT ( 'NONE',  ( 0.5643044619422579178, -0.004921259842519576551, 0.3153832671262227771 ) ) ;
#61083=CARTESIAN_POINT ( 'NONE',  ( 1.200787401574803681, -0.5400638737290845981, -0.3530559997133363437 ) ) ;
#61085=CARTESIAN_POINT ( 'NONE',  ( 1.017060367454068803, -0.2845877964562159024, 0.3641732283464567677 ) ) ;
#61086=CARTESIAN_POINT ( 'NONE',  ( 0.8595800524934390507, -0.05778040916215560624, -0.4822834645669293319 ) ) ;
#61088=CARTESIAN_POINT ( 'NONE',  ( -0.5118110236220466680, -0.6692913385826771977, 8.415575281601705876E-17 ) ) ;
#61090=CARTESIAN_POINT ( 'NONE',  ( 1.272965879265092637, -0.004921259842519576551, 0.3153832671262227771 ) ) ;
#61091=CARTESIAN_POINT ( 'NONE',  ( -0.5511811023622041894, -0.1870078740157480879, -0.4822834645669291653 ) ) ;
#61093=CARTESIAN_POINT ( 'NONE',  ( 1.272965879265092637, -0.4281496062992127816, -0.4176697321401328100 ) ) ;
#61094=CARTESIAN_POINT ( 'NONE',  ( 0.2296587926509192634, -0.05778040916215560624, -0.4822834645669293319 ) ) ;
#61095=CARTESIAN_POINT ( 'NONE',  ( 0.4002624671916016896, -0.08942795157527998196, 0.3641732283464567121 ) ) ;
#61097=CARTESIAN_POINT ( 'NONE',  ( -0.05249343832020911260, 0.1283753931104748280, 0.1820866141732283561 ) ) ;
#61098=CARTESIAN_POINT ( 'NONE',  ( -1.555118110236219930, -0.5400638737290845981, -0.3530559997133363437 ) ) ;
#61100=CARTESIAN_POINT ( 'NONE',  ( 0.7939632545931766261, -0.3162353388693409650, -0.4822834645669289433 ) ) ;
#61102=CARTESIAN_POINT ( 'NONE',  ( 1.437007874015748810, -0.4536011799217368745, -0.2665933059059886201 ) ) ;
#61103=CARTESIAN_POINT ( 'NONE',  ( 2.795275590551181466, 1.023622047244095556, -2.156651478620225655E-16 ) ) ;
#61104=CARTESIAN_POINT ( 'NONE',  ( -0.1312335958005241554, 0.1283753931104748280, 0.1820866141732283561 ) ) ;
#61105=AXIS2_PLACEMENT_3D ( 'NONE', #29988, #80543, #67481 ) ;
#61106=CARTESIAN_POINT ( 'NONE',  ( 0.3149606299212606708, -0.1870078740157480879, -0.4822834645669291653 ) ) ;
#61107=CARTESIAN_POINT ( 'NONE',  ( 1.469816272965879911, -0.5023911411419708095, 0.1820866141732285504 ) ) ;
#61108=CARTESIAN_POINT ( 'NONE',  ( -1.233595800524933894, 0.1283753931104748280, 0.1820866141732283561 ) ) ;
#61109=CARTESIAN_POINT ( 'NONE',  ( -1.417322834645668772, -0.1870078740157479769, 0.4822834645669291653 ) ) ;
#61110=CARTESIAN_POINT ( 'NONE',  ( 0.6955380577427828781, -0.4281496062992124485, 0.4176697321401328655 ) ) ;
#61111=CARTESIAN_POINT ( 'NONE',  ( 1.253280839895013710, -0.05778040916215560624, -0.4822834645669293319 ) ) ;
#61113=CARTESIAN_POINT ( 'NONE',  ( 0.1312335958005255154, -0.6046776061558807314, 0.2411417322834647770 ) ) ;
#61114=CARTESIAN_POINT ( 'NONE',  ( 1.312335958005250269, -0.6046776061558807314, 0.2411417322834647770 ) ) ;
#61115=CARTESIAN_POINT ( 'NONE',  ( 0.8398950131233602345, -0.6046776061558807314, 0.2411417322834647770 ) ) ;
#61116=CARTESIAN_POINT ( 'NONE',  ( -1.686351706036744558, 0.1771653543307087075, -0.09757992244046823083 ) ) ;
#61117=CARTESIAN_POINT ( 'NONE',  ( 0.9120734908136490793, 0.1771653543307087075, -0.09757992244046823083 ) ) ;
#61118=CARTESIAN_POINT ( 'NONE',  ( 1.489501312335958172, -0.3162353388693405765, 0.4822834645669290543 ) ) ;
#61119=EDGE_CURVE ( 'NONE', #33739, #72166, #25181, .T. ) ;
#61120=CARTESIAN_POINT ( 'NONE',  ( 0.3543307086614179147, 0.1771653543307087630, 0.000000000000000000 ) ) ;
#61121=CARTESIAN_POINT ( 'NONE',  ( 0.2034120734908144990, -0.6692913385826771977, 0.1292274648535927661 ) ) ;
#61122=CARTESIAN_POINT ( 'NONE',  ( 0.5774278215223103139, -0.6046776061558809534, -0.2411417322834644161 ) ) ;
#61123=CARTESIAN_POINT ( 'NONE',  ( -0.3083989501312330295, -0.3162353388693409650, -0.4822834645669289433 ) ) ;
#61124=CARTESIAN_POINT ( 'NONE',  ( -0.01312335958005186876, -0.3690944881889763329, 0.3153832671262228327 ) ) ;
#61125=CARTESIAN_POINT ( 'NONE',  ( 0.8136482939632553313, 0.2306618581243848609, 0.2411417322834645549 ) ) ;
#61127=CARTESIAN_POINT ( 'NONE',  ( -1.128608923884513837, -0.6046776061558807314, 0.2411417322834647770 ) ) ;
#61129=CARTESIAN_POINT ( 'NONE',  ( 1.586052503253845281, 1.299212598425198095, -0.1653254495020587411 ) ) ;
#61131=CARTESIAN_POINT ( 'NONE',  ( -1.036745406824146176, -0.4281496062992124485, 0.4176697321401328655 ) ) ;
#61132=CARTESIAN_POINT ( 'NONE',  ( -0.3280839895013117347, -0.4281496062992124485, 0.4176697321401328655 ) ) ;
#61136=CARTESIAN_POINT ( 'NONE',  ( 0.8005249343832028242, -0.3690944881889765550, -0.3153832671262227771 ) ) ;
#61138=CARTESIAN_POINT ( 'NONE',  ( 1.240157480314961314, -0.5400638737290844871, 0.3530559997133364547 ) ) ;
#61140=CARTESIAN_POINT ( 'NONE',  ( -0.2469196488504575571, 5.952911114587291371E-15, -0.4118484887281962381 ) ) ;
#61141=CARTESIAN_POINT ( 'NONE',  ( -1.548556430446193399, 0.1283753931104748280, 0.1820866141732283561 ) ) ;
#61142=CARTESIAN_POINT ( 'NONE',  ( 1.601049868766404982, -0.6046776061558809534, -0.2411417322834644161 ) ) ;
#61143=CARTESIAN_POINT ( 'NONE',  ( -1.568241469816272105, -0.05778040916215522460, 0.4822834645669289988 ) ) ;
#61144=CARTESIAN_POINT ( 'NONE',  ( 0.5511811023622055217, -0.1870078740157479769, 0.4822834645669291653 ) ) ;
#61146=CARTESIAN_POINT ( 'NONE',  ( -0.01968503937007793844, 0.1660481256975883668, -0.3530559997133364547 ) ) ;
#61147=CARTESIAN_POINT ( 'NONE',  ( -0.7545931758530177724, 0.1771653543307087630, 0.09757992244046791164 ) ) ;
#61148=CARTESIAN_POINT ( 'NONE',  ( 1.030183727034121421, -0.3162353388693409650, -0.4822834645669289433 ) ) ;
#61149=CARTESIAN_POINT ( 'NONE',  ( -0.2034120734908131112, -0.6692913385826773087, -0.1292274648535924053 ) ) ;
#61150=CARTESIAN_POINT ( 'NONE',  ( 0.5249343832021003964, 0.2306618581243847221, -0.2411417322834647770 ) ) ;
#61153=CARTESIAN_POINT ( 'NONE',  ( 0.9908136482939640111, -0.6692913385826771977, 0.1292274648535927661 ) ) ;
#61154=CARTESIAN_POINT ( 'NONE',  ( -0.01312335958005186876, -0.4281496062992124485, 0.4176697321401328655 ) ) ;
#61155=CARTESIAN_POINT ( 'NONE',  ( -1.102362204724408601, -0.1870078740157480879, -0.4822834645669291653 ) ) ;
#61157=CARTESIAN_POINT ( 'NONE',  ( 1.017060367454068581, -0.05778040916215560624, -0.4822834645669293319 ) ) ;
#61158=CARTESIAN_POINT ( 'NONE',  ( 0.2690288713910767848, 0.2952755905511811885, 0.1292274648535926551 ) ) ;
#61160=CARTESIAN_POINT ( 'NONE',  ( -0.2296587926509179312, -0.3162353388693409650, -0.4822834645669289433 ) ) ;
#61161=CARTESIAN_POINT ( 'NONE',  ( 0.5839895013123367340, 0.2952755905511811885, 0.1292274648535926551 ) ) ;
#61162=CARTESIAN_POINT ( 'NONE',  ( -0.1246719160104980823, -0.6692913385826773087, -0.1292274648535924053 ) ) ;
#61163=CARTESIAN_POINT ( 'NONE',  ( 0.5971128608923891301, 0.1771653543307087075, -0.09757992244046823083 ) ) ;
#61164=CARTESIAN_POINT ( 'NONE',  ( -1.692913385826770645, 0.2952755905511811885, 0.000000000000000000 ) ) ;
#61166=CARTESIAN_POINT ( 'NONE',  ( 0.1574803149606306130, -0.1870078740157479769, 0.4822834645669291653 ) ) ;
#61169=ORIENTED_EDGE ( 'NONE', *, *, #2754, .T. ) ;
#61171=CARTESIAN_POINT ( 'NONE',  ( 1.207349081364829990, 0.2306618581243848609, 0.2411417322834645549 ) ) ;
#61172=CARTESIAN_POINT ( 'NONE',  ( 0.6167979002624678353, -0.3690944881889763329, 0.3153832671262228327 ) ) ;
#61173=CARTESIAN_POINT ( 'NONE',  ( 0.9563780557770535928, -8.614921172258640174E-17, 0.3791475997938231202 ) ) ;
#61176=CARTESIAN_POINT ( 'NONE',  ( 0.4556365110581300226, 1.773775493389249114, -0.5309055118110237448 ) ) ;
#61180=CARTESIAN_POINT ( 'NONE',  ( 0.9251968503937015864, -0.5400638737290844871, 0.3530559997133364547 ) ) ;
#61181=CARTESIAN_POINT ( 'NONE',  ( -0.9580052493438311334, 0.05413385826771626580, -0.4176697321401330321 ) ) ;
#61182=CARTESIAN_POINT ( 'NONE',  ( -0.7611548556430438595, 0.2306618581243848609, 0.2411417322834645549 ) ) ;
#61183=CARTESIAN_POINT ( 'NONE',  ( 0.8267716535433077274, 0.2952755905511811885, 0.000000000000000000 ) ) ;
#61184=CARTESIAN_POINT ( 'NONE',  ( 1.482939632545932307, 0.05413385826771626580, -0.4176697321401330321 ) ) ;
#61185=CARTESIAN_POINT ( 'NONE',  ( 1.686351706036745890, 0.1771653543307087630, 0.09757992244046791164 ) ) ;
#61186=CARTESIAN_POINT ( 'NONE',  ( 1.410761154855643795, -0.08942795157528024563, -0.3641732283464568787 ) ) ;
#61188=CARTESIAN_POINT ( 'NONE',  ( -1.404199475065615932, -0.3690944881889765550, -0.3153832671262227771 ) ) ;
#61190=CARTESIAN_POINT ( 'NONE',  ( 0.02624671916010564918, -0.6046776061558809534, -0.2411417322834644161 ) ) ;
#61191=CARTESIAN_POINT ( 'NONE',  ( 1.627296587926509996, -0.6046776061558807314, 0.2411417322834647770 ) ) ;
#61192=DIRECTION ( 'NONE',  ( 0.000000000000000000, 0.000000000000000000, -1.000000000000000000 ) ) ;
#61193=CARTESIAN_POINT ( 'NONE',  ( -1.115485564304461219, -0.3690944881889763329, 0.3153832671262228327 ) ) ;
#61194=CARTESIAN_POINT ( 'NONE',  ( 0.2821522309711292364, 0.2952755905511810774, -0.1292274648535930714 ) ) ;
#61195=CARTESIAN_POINT ( 'NONE',  ( 1.469816272965879911, 0.1283753931104746893, -0.1820866141732285504 ) ) ;
#61197=CARTESIAN_POINT ( 'NONE',  ( -1.135170603674539924, -0.5511811023622046335, 0.09757992244046803654 ) ) ;
#61198=CARTESIAN_POINT ( 'NONE',  ( 1.220472440944882608, 0.2952755905511811885, 0.000000000000000000 ) ) ;
#61200=CARTESIAN_POINT ( 'NONE',  ( -0.006561679790025524116, -0.3162353388693405765, 0.4822834645669290543 ) ) ;
#61201=CARTESIAN_POINT ( 'NONE',  ( -1.358267716535432434, -0.4536011799217367080, 0.2665933059059888421 ) ) ;
#61202=CARTESIAN_POINT ( 'NONE',  ( -0.6167979002624665030, 0.05413385826771666132, 0.4176697321401328100 ) ) ;
#61203=CARTESIAN_POINT ( 'NONE',  ( -1.614173228346455824, 0.1771653543307087630, 0.000000000000000000 ) ) ;
#61205=CARTESIAN_POINT ( 'NONE',  ( 0.4593175853018379162, -0.4281496062992124485, 0.4176697321401328655 ) ) ;
#61207=CARTESIAN_POINT ( 'NONE',  ( 1.581364829396326277, -0.05778040916215522460, 0.4822834645669289988 ) ) ;
#61210=CARTESIAN_POINT ( 'NONE',  ( -1.233595800524933894, 0.2306618581243848609, 0.2411417322834645549 ) ) ;
#61211=CARTESIAN_POINT ( 'NONE',  ( -0.4593175853018366950, -0.004921259842519576551, 0.3153832671262227771 ) ) ;
#61212=CARTESIAN_POINT ( 'NONE',  ( -1.646051170424378096, 0.4405861044731112508, 0.3149606299212598381 ) ) ;
#61213=CARTESIAN_POINT ( 'NONE',  ( 0.1574803149606306130, -0.1870078740157480879, -0.4822834645669291653 ) ) ;
#61214=CARTESIAN_POINT ( 'NONE',  ( 0.5183727034120741983, -0.5511811023622046335, 0.09757992244046803654 ) ) ;
#61215=CARTESIAN_POINT ( 'NONE',  ( -0.9448818897637790704, -0.1870078740157479769, 0.3641732283464567677 ) ) ;
#61216=CARTESIAN_POINT ( 'NONE',  ( -1.502624671916009680, -0.05778040916215560624, -0.4822834645669293319 ) ) ;
#61217=CARTESIAN_POINT ( 'NONE',  ( -1.404199475065615932, 0.05413385826771666132, 0.4176697321401328100 ) ) ;
#61218=ADVANCED_FACE ( 'NONE', ( #73142 ), #26163, .F. ) ;
#61219=CARTESIAN_POINT ( 'NONE',  ( 1.476377952755906442, -0.5400638737290844871, 0.3530559997133364547 ) ) ;
#61220=CARTESIAN_POINT ( 'NONE',  ( -1.586052503253849055, 0.4724409448818907564, -0.1653254495020551051 ) ) ;
#61221=CARTESIAN_POINT ( 'NONE',  ( 0.4527559055118117182, 0.07958543189024071263, -0.2665933059059888421 ) ) ;
#61222=CARTESIAN_POINT ( 'NONE',  ( 0.7874015748031503170, -0.1870078740157480879, -0.4822834645669291653 ) ) ;
#61224=CARTESIAN_POINT ( 'NONE',  ( 1.535433070866142335, -0.5511811023622047445, 6.969142054262312111E-17 ) ) ;
#61227=CARTESIAN_POINT ( 'NONE',  ( -1.148293963254592542, 0.2952755905511811885, 0.1292274648535926551 ) ) ;
#61228=CARTESIAN_POINT ( 'NONE',  ( -0.8661417322834640276, -0.1870078740157479769, 0.4822834645669291653 ) ) ;
#61229=CARTESIAN_POINT ( 'NONE',  ( 0.4002624671916016896, -0.3162353388693409650, -0.4822834645669289433 ) ) ;
#61230=CARTESIAN_POINT ( 'NONE',  ( -1.719160104986876103, -0.004921259842519576551, 0.3153832671262227771 ) ) ;
#61232=CARTESIAN_POINT ( 'NONE',  ( 1.056430446194226436, -0.6692913385826773087, -0.1292274648535924053 ) ) ;
#61233=CARTESIAN_POINT ( 'NONE',  ( -1.699475065616797398, 0.2952755905511811885, 0.1292274648535926551 ) ) ;
#61234=CARTESIAN_POINT ( 'NONE',  ( 0.3740157480314966754, -0.5400638737290844871, 0.3530559997133364547 ) ) ;
#61235=CARTESIAN_POINT ( 'NONE',  ( 0.6496062992125991586, 0.1660481256975885056, 0.3530559997133364547 ) ) ;
#61242=CARTESIAN_POINT ( 'NONE',  ( -0.1968503937007867743, -0.5511811023622047445, 6.969142054262312111E-17 ) ) ;
#61243=CARTESIAN_POINT ( 'NONE',  ( -0.2952755905511804668, 0.1660481256975885056, 0.3530559997133364547 ) ) ;
#61244=CARTESIAN_POINT ( 'NONE',  ( 0.7677165354330716118, -0.5400638737290844871, 0.3530559997133364547 ) ) ;
#61246=CARTESIAN_POINT ( 'NONE',  ( -0.07874015748031421014, -0.1870078740157479769, 0.3641732283464567677 ) ) ;
#61247=CARTESIAN_POINT ( 'NONE',  ( -1.305774278215222184, 0.2952755905511811885, 0.1292274648535926551 ) ) ;
#61248=CARTESIAN_POINT ( 'NONE',  ( 1.010498687664042716, 0.05413385826771626580, -0.4176697321401330321 ) ) ;
#61251=DIRECTION ( 'NONE',  ( -3.096699300667737957E-16, 1.000000000000000000, -0.000000000000000000 ) ) ;
#61253=CARTESIAN_POINT ( 'NONE',  ( 0.8202099737532813073, 0.2952755905511811885, 0.1292274648535926551 ) ) ;
#61254=CARTESIAN_POINT ( 'NONE',  ( 1.312335958005249825, 0.1283753931104746893, -0.1820866141732285504 ) ) ;
#61255=CARTESIAN_POINT ( 'NONE',  ( -1.522309711286088607, -0.5023911411419708095, 0.1820866141732285504 ) ) ;
#61256=CARTESIAN_POINT ( 'NONE',  ( 1.535433070866142335, -0.6692913385826771977, 8.415575281601705876E-17 ) ) ;
#61259=CARTESIAN_POINT ( 'NONE',  ( 1.384514435695538559, 0.2952755905511810774, -0.1292274648535930714 ) ) ;
#61260=CARTESIAN_POINT ( 'NONE',  ( -1.732283464566928277, -0.1870078740157479769, 0.4822834645669291653 ) ) ;
#61261=CARTESIAN_POINT ( 'NONE',  ( 0.03280839895013198948, 0.2952755905511811885, 0.1292274648535926551 ) ) ;
#61262=CARTESIAN_POINT ( 'NONE',  ( -0.7742782152230965886, 0.05413385826771666132, 0.4176697321401328100 ) ) ;
#61263=CARTESIAN_POINT ( 'NONE',  ( 1.437007874015748810, 0.1660481256975885056, 0.3530559997133364547 ) ) ;
#61265=CARTESIAN_POINT ( 'NONE',  ( 0.01968503937007930540, 0.1660481256975885056, 0.3530559997133364547 ) ) ;
#61267=CARTESIAN_POINT ( 'NONE',  ( 1.515748031496063408, 0.1660481256975885056, 0.3530559997133364547 ) ) ;
#61268=VERTEX_POINT ( 'NONE', #75852 ) ;
#61270=ORIENTED_EDGE ( 'NONE', *, *, #37699, .F. ) ;
#61273=CARTESIAN_POINT ( 'NONE',  ( -1.712598425196849572, 0.1660481256975885056, 0.3530559997133364547 ) ) ;
#61275=CARTESIAN_POINT ( 'NONE',  ( 0.5631141337314363726, 7.053449127088339072E-16, 0.3627989612356146698 ) ) ;
#61277=CARTESIAN_POINT ( 'NONE',  ( -0.9973753280839886548, 0.2306618581243848609, 0.2411417322834645549 ) ) ;
#61280=CARTESIAN_POINT ( 'NONE',  ( -0.1115485564304453947, -0.5511811023622046335, 0.09757992244046803654 ) ) ;
#61281=EDGE_CURVE ( 'NONE', #47808, #1757, #8976, .T. ) ;
#61282=CARTESIAN_POINT ( 'NONE',  ( -0.8989501312335946848, 0.1771653543307087075, -0.09757992244046823083 ) ) ;
#61283=CARTESIAN_POINT ( 'NONE',  ( -1.345144356955379816, -0.3162353388693405765, 0.4822834645669290543 ) ) ;
#61284=CARTESIAN_POINT ( 'NONE',  ( 0.5708661417322841158, -0.5400638737290845981, -0.3530559997133363437 ) ) ;
#61285=CARTESIAN_POINT ( 'NONE',  ( -1.240157480314959759, -0.5400638737290845981, -0.3530559997133363437 ) ) ;
#61287=EDGE_LOOP ( 'NONE', ( #4341, #43639, #26297, #31206, #64464, #45101, #47981, #76258, #45922, #61350, #67918, #75337, #75626, #32453, #40862, #68206, #69267, #54323, #5578, #81147, #1363 ) ) ;
#61288=CARTESIAN_POINT ( 'NONE',  ( -1.469816272965878357, 0.2306618581243848609, 0.2411417322834645549 ) ) ;
#61289=CARTESIAN_POINT ( 'NONE',  ( -1.604771003085129211, 2.104981124449682550, -0.1466069496707751996 ) ) ;
#61294=CARTESIAN_POINT ( 'NONE',  ( -0.9120734908136475250, -0.6692913385826773087, -0.1292274648535924053 ) ) ;
#61295=CARTESIAN_POINT ( 'NONE',  ( 1.581364829396326277, -0.3162353388693409650, -0.4822834645669289433 ) ) ;
#61296=CARTESIAN_POINT ( 'NONE',  ( -1.719160104986876103, 0.05413385826771666132, 0.4176697321401328100 ) ) ;
#61298=CARTESIAN_POINT ( 'NONE',  ( 1.522309711286089939, 0.2306618581243848609, 0.2411417322834645549 ) ) ;
#61299=CARTESIAN_POINT ( 'NONE',  ( -1.017060367454067249, -0.3162353388693409650, -0.4822834645669289433 ) ) ;
#61301=CARTESIAN_POINT ( 'NONE',  ( -0.09186351706036689768, -0.004921259842519870586, -0.3153832671262229437 ) ) ;
#61303=CARTESIAN_POINT ( 'NONE',  ( -0.05905511811023545637, 0.07958543189024085140, 0.2665933059059887866 ) ) ;
#61304=CARTESIAN_POINT ( 'NONE',  ( 0.9514435695538062676, -0.08942795157527998196, 0.3641732283464567121 ) ) ;
#61305=CARTESIAN_POINT ( 'NONE',  ( 0.3674540682414705883, 0.2306618581243847221, -0.2411417322834647770 ) ) ;
#61307=CARTESIAN_POINT ( 'NONE',  ( -0.2362204724409440182, -0.1870078740157479769, 0.3641732283464567677 ) ) ;
#61309=CARTESIAN_POINT ( 'NONE',  ( -1.515748031496062076, -0.5400638737290844871, 0.3530559997133364547 ) ) ;
#61310=VECTOR ( 'NONE', #26825, 39.37007874015748143 ) ;
#61311=CARTESIAN_POINT ( 'NONE',  ( -1.318897637795274802, 0.07958543189024085140, 0.2665933059059887866 ) ) ;
#61314=CARTESIAN_POINT ( 'NONE',  ( 0.1706036745406830368, 0.05413385826771666132, 0.4176697321401328100 ) ) ;
#61315=CARTESIAN_POINT ( 'NONE',  ( -0.4658792650918627265, -0.3162353388693409650, -0.4822834645669289433 ) ) ;
#61317=CARTESIAN_POINT ( 'NONE',  ( 0.4921259842519691285, 0.07958543189024085140, 0.2665933059059887866 ) ) ;
#61318=CARTESIAN_POINT ( 'NONE',  ( -0.06561679790026180015, -0.4281496062992127816, -0.4176697321401328100 ) ) ;
#61319=CARTESIAN_POINT ( 'NONE',  ( -0.7414698162729651543, -0.6692913385826771977, 0.1292274648535927661 ) ) ;
#61322=CARTESIAN_POINT ( 'NONE',  ( 0.07874015748031558404, -0.1870078740157479769, 0.4822834645669291653 ) ) ;
#61324=CARTESIAN_POINT ( 'NONE',  ( -1.586052503253847501, 1.299212598425198095, -0.1653254495020571035 ) ) ;
#61325=CARTESIAN_POINT ( 'NONE',  ( -0.2099737532808391705, -0.5023911411419708095, -0.1820866141732282451 ) ) ;
#61327=CARTESIAN_POINT ( 'NONE',  ( -0.3871391076115479057, -0.3162353388693409650, -0.4822834645669289433 ) ) ;
#61328=CARTESIAN_POINT ( 'NONE',  ( -1.509186351706035767, -0.3690944881889763329, 0.3153832671262228327 ) ) ;
#61329=CARTESIAN_POINT ( 'NONE',  ( 1.502624671916010790, -0.05778040916215522460, 0.4822834645669289988 ) ) ;
#61330=CARTESIAN_POINT ( 'NONE',  ( -1.476377952755905110, 0.1660481256975885056, 0.3530559997133364547 ) ) ;
#61331=CARTESIAN_POINT ( 'NONE',  ( -0.8136482939632537770, -0.5023911411419708095, 0.1820866141732285504 ) ) ;
#61335=CARTESIAN_POINT ( 'NONE',  ( 1.404199475065617708, -0.004921259842519870586, -0.3153832671262229437 ) ) ;
#61337=CARTESIAN_POINT ( 'NONE',  ( 1.259842519685040019, -0.1870078740157479769, 0.3641732283464567677 ) ) ;
#61338=CARTESIAN_POINT ( 'NONE',  ( 1.043307086614173818, -0.5400638737290845981, -0.3530559997133363437 ) ) ;
#61339=CARTESIAN_POINT ( 'NONE',  ( -1.712598425196849572, 0.1660481256975885056, 0.3530559997133364547 ) ) ;
#61340=CARTESIAN_POINT ( 'NONE',  ( 0.8858267716535438430, -0.5400638737290845981, -0.3530559997133363437 ) ) ;
#61342=CARTESIAN_POINT ( 'NONE',  ( 1.187664041994751285, -0.08942795157527998196, 0.3641732283464567121 ) ) ;
#61344=CARTESIAN_POINT ( 'NONE',  ( 0.09842519685039434474, 0.1660481256975885056, 0.3530559997133364547 ) ) ;
#61345=CARTESIAN_POINT ( 'NONE',  ( -0.6824146981627288167, 0.2306618581243848609, 0.2411417322834645549 ) ) ;
#61349=CARTESIAN_POINT ( 'NONE',  ( 0.4855643044619428750, -0.004921259842519576551, 0.3153832671262227771 ) ) ;
#61350=ORIENTED_EDGE ( 'NONE', *, *, #2281, .F. ) ;
#61353=CARTESIAN_POINT ( 'NONE',  ( -0.5643044619422565855, 0.05413385826771626580, -0.4176697321401330321 ) ) ;
#61354=CARTESIAN_POINT ( 'NONE',  ( -0.07217847769028787330, -0.05778040916215522460, 0.4822834645669289988 ) ) ;
#61355=CARTESIAN_POINT ( 'NONE',  ( -0.1574803149606292529, -0.1870078740157480879, -0.4822834645669291653 ) ) ;
#61356=CARTESIAN_POINT ( 'NONE',  ( 0.6167979002624679463, 0.05413385826771626580, -0.4176697321401330321 ) ) ;
#61357=CARTESIAN_POINT ( 'NONE',  ( -0.8070866141732276899, 0.1660481256975883668, -0.3530559997133364547 ) ) ;
#61358=CARTESIAN_POINT ( 'NONE',  ( -0.4527559055118102749, 0.1660481256975885056, 0.3530559997133364547 ) ) ;
#61359=CARTESIAN_POINT ( 'NONE',  ( 0.9776902887139113929, 0.2952755905511811885, 0.1292274648535926551 ) ) ;
#61361=CARTESIAN_POINT ( 'NONE',  ( 0.2952755905511816326, -0.5400638737290844871, 0.3530559997133364547 ) ) ;
#61362=CARTESIAN_POINT ( 'NONE',  ( 0.9514435695538062676, -0.3162353388693409650, -0.4822834645669289433 ) ) ;
#61365=CARTESIAN_POINT ( 'NONE',  ( -0.1902887139107604098, 0.1771653543307087075, -0.09757992244046823083 ) ) ;
#61366=ORIENTED_EDGE ( 'NONE', *, *, #74915, .F. ) ;
#61369=CARTESIAN_POINT ( 'NONE',  ( -0.8661417322834640276, -0.1870078740157480601, -0.3641732283464567677 ) ) ;
#61372=CARTESIAN_POINT ( 'NONE',  ( -0.5643044619422565855, -0.4281496062992124485, 0.4176697321401328655 ) ) ;
#61373=CARTESIAN_POINT ( 'NONE',  ( 0.7759054087898769048, 2.575861430505332611E-15, -0.3791475997938230091 ) ) ;
#61374=CARTESIAN_POINT ( 'NONE',  ( -0.8464566929133852113, -0.5400638737290845981, -0.3530559997133363437 ) ) ;
#61375=CARTESIAN_POINT ( 'NONE',  ( -0.5183727034120726440, -0.6692913385826773087, -0.1292274648535924053 ) ) ;
#61377=CARTESIAN_POINT ( 'NONE',  ( -1.095800524934382292, -0.3162353388693409650, -0.4822834645669289433 ) ) ;
#61378=CARTESIAN_POINT ( 'NONE',  ( -1.423884514435694859, -0.3162353388693405765, 0.4822834645669290543 ) ) ;
#61379=CARTESIAN_POINT ( 'NONE',  ( 0.7677165354330716118, 0.07958543189024071263, -0.2665933059059888421 ) ) ;
#61382=CARTESIAN_POINT ( 'NONE',  ( 0.6299212598425204535, -0.1870078740157479769, 0.3641732283464567677 ) ) ;
#61383=CARTESIAN_POINT ( 'NONE',  ( -0.03937007874015669567, 0.2952755905511811885, 0.000000000000000000 ) ) ;
#61384=CARTESIAN_POINT ( 'NONE',  ( -0.2165354330708654795, 0.1660481256975885056, 0.3530559997133364547 ) ) ;
#61387=FACE_OUTER_BOUND ( 'NONE', #61062, .T. ) ;
#61388=ORIENTED_EDGE ( 'NONE', *, *, #20062, .F. ) ;
#61390=CARTESIAN_POINT ( 'NONE',  ( -0.7874015748031492068, 2.204724409448818978, 0.000000000000000000 ) ) ;
#61391=CARTESIAN_POINT ( 'NONE',  ( -0.5643044619422565855, -0.004921259842519870586, -0.3153832671262229437 ) ) ;
#61392=CARTESIAN_POINT ( 'NONE',  ( -0.8923884514435688198, 0.2306618581243847221, -0.2411417322834647770 ) ) ;
#61395=CARTESIAN_POINT ( 'NONE',  ( 1.594488188976378673, -0.5400638737290845981, -0.3530559997133363437 ) ) ;
#61396=CARTESIAN_POINT ( 'NONE',  ( 0.4593175853018379162, -0.4281496062992124485, 0.4176697321401328655 ) ) ;
#61397=CARTESIAN_POINT ( 'NONE',  ( 0.5774278215223104249, 0.2306618581243848609, 0.2411417322834645549 ) ) ;
#61398=CARTESIAN_POINT ( 'NONE',  ( -0.7349081364829387342, -0.5023911411419708095, 0.1820866141732285504 ) ) ;
#61399=CARTESIAN_POINT ( 'NONE',  ( -0.03937007874015669567, -0.6692913385826771977, 8.415575281601705876E-17 ) ) ;
#61401=CARTESIAN_POINT ( 'NONE',  ( -0.5774278215223089816, 0.2306618581243847221, -0.2411417322834647770 ) ) ;
#61403=CARTESIAN_POINT ( 'NONE',  ( 1.095800524934383846, -0.2845877964562159024, 0.3641732283464567677 ) ) ;
#61404=CARTESIAN_POINT ( 'NONE',  ( 0.2690288713910767848, -0.5511811023622048555, -0.09757992244046775898 ) ) ;
#61405=CARTESIAN_POINT ( 'NONE',  ( 1.305774278215223960, -0.5511811023622046335, 0.09757992244046803654 ) ) ;
#61406=CARTESIAN_POINT ( 'NONE',  ( -1.338582677165353729, -0.1870078740157480879, -0.4822834645669291653 ) ) ;
#61407=CARTESIAN_POINT ( 'NONE',  ( -0.5643044619422565855, -0.3690944881889763329, 0.3153832671262228327 ) ) ;
#61409=CARTESIAN_POINT ( 'NONE',  ( -1.148293963254592542, -0.6692913385826773087, -0.1292274648535924053 ) ) ;
#61410=CARTESIAN_POINT ( 'NONE',  ( -0.6036745406824141069, -0.6046776061558809534, -0.2411417322834644161 ) ) ;
#61411=CARTESIAN_POINT ( 'NONE',  ( 0.4593175853018380828, 0.05413385826771626580, -0.4176697321401330321 ) ) ;
#61414=CARTESIAN_POINT ( 'NONE',  ( 0.5183727034120741983, -0.5511811023622046335, 0.09757992244046803654 ) ) ;
#61415=CARTESIAN_POINT ( 'NONE',  ( 0.8661417322834652488, -0.1870078740157480879, -0.4822834645669291653 ) ) ;
#61416=CARTESIAN_POINT ( 'NONE',  ( -1.154855643044618851, -0.5023911411419708095, -0.1820866141732282451 ) ) ;
#61417=CARTESIAN_POINT ( 'NONE',  ( 1.233595800524935227, 0.2306618581243847221, -0.2411417322834647770 ) ) ;
#61418=CARTESIAN_POINT ( 'NONE',  ( -1.404199475065615932, -0.004921259842519576551, 0.3153832671262227771 ) ) ;
#61419=CARTESIAN_POINT ( 'NONE',  ( -1.469816272965878357, -0.6046776061558809534, -0.2411417322834644161 ) ) ;
#61420=CARTESIAN_POINT ( 'NONE',  ( -0.7808398950131225646, -0.05778040916215522460, 0.4822834645669289988 ) ) ;
#61421=CARTESIAN_POINT ( 'NONE',  ( 8.195543980992789655E-16, -0.1870078740157480601, -0.3641732283464567677 ) ) ;
#61423=CARTESIAN_POINT ( 'NONE',  ( 0.5249343832021003964, 0.1283753931104746893, -0.1820866141732285504 ) ) ;
#61426=CARTESIAN_POINT ( 'NONE',  ( 0.02624671916010564918, -0.6046776061558809534, -0.2411417322834644161 ) ) ;
#61428=CARTESIAN_POINT ( 'NONE',  ( -1.115485564304461219, -0.4281496062992124485, 0.4176697321401328655 ) ) ;
#61431=CARTESIAN_POINT ( 'NONE',  ( 0.8923884514435701520, -0.5023911411419708095, -0.1820866141732282451 ) ) ;
#61432=CARTESIAN_POINT ( 'NONE',  ( -0.1509186351706028884, -0.3162353388693409650, -0.4822834645669289433 ) ) ;
#61433=MECHANICAL_DESIGN_GEOMETRIC_PRESENTATION_REPRESENTATION('',(#72196),#64135);
#61435=CARTESIAN_POINT ( 'NONE',  ( -0.2887139107611542133, -0.6046776061558809534, -0.2411417322834644161 ) ) ;
#61436=CARTESIAN_POINT ( 'NONE',  ( -0.5774278215223089816, -0.5023911411419708095, 0.1820866141732285504 ) ) ;
#61437=CARTESIAN_POINT ( 'NONE',  ( 0.9842519685039375910, 0.2066929133858268208, 0.000000000000000000 ) ) ;
#61438=CARTESIAN_POINT ( 'NONE',  ( -0.5511811023622038563, -0.1870078740157479769, 0.3641732283464567677 ) ) ;
#61439=CARTESIAN_POINT ( 'NONE',  ( 0.3937007874015754361, -0.1870078740157479769, 0.4822834645669291653 ) ) ;
#61440=CARTESIAN_POINT ( 'NONE',  ( -1.286089238845143479, -0.5023911411419708095, 0.1820866141732285504 ) ) ;
#61442=CARTESIAN_POINT ( 'NONE',  ( -1.417322834645668772, -0.1870078740157480879, -0.4822834645669291653 ) ) ;
#61445=CARTESIAN_POINT ( 'NONE',  ( -1.437007874015747477, -0.4536011799217367080, 0.2665933059059888421 ) ) ;
#61446=CARTESIAN_POINT ( 'NONE',  ( -0.6430446194225716283, -0.4281496062992124485, 0.4176697321401328655 ) ) ;
#61447=CARTESIAN_POINT ( 'NONE',  ( -1.358267716535432434, -0.5400638737290844871, 0.3530559997133364547 ) ) ;
#61449=LINE ( 'NONE', #41269, #12234 ) ;
#61450=CARTESIAN_POINT ( 'NONE',  ( 1.325459317585302665, -0.4281496062992124485, 0.4176697321401328655 ) ) ;
#61451=CARTESIAN_POINT ( 'NONE',  ( 0.2690288713910767848, 0.2952755905511811885, 0.1292274648535926551 ) ) ;
#61455=CARTESIAN_POINT ( 'NONE',  ( 1.541994750656168645, -0.5511811023622046335, 0.09757992244046803654 ) ) ;
#61458=CARTESIAN_POINT ( 'NONE',  ( -1.062992125984250968, -0.5511811023622047445, 6.969142054262312111E-17 ) ) ;
#61460=ORIENTED_EDGE ( 'NONE', *, *, #60948, .F. ) ;
#61461=CARTESIAN_POINT ( 'NONE',  ( 0.8530183727034126306, 0.05413385826771626580, -0.4176697321401330321 ) ) ;
#61462=CARTESIAN_POINT ( 'NONE',  ( -0.2034120734908131112, -0.6692913385826773087, -0.1292274648535924053 ) ) ;
#61463=CARTESIAN_POINT ( 'NONE',  ( -1.279527559055116948, 0.1660481256975883668, -0.3530559997133364547 ) ) ;
#61464=CARTESIAN_POINT ( 'NONE',  ( 1.122047244094488860, -0.5400638737290845981, -0.3530559997133363437 ) ) ;
#61465=CARTESIAN_POINT ( 'NONE',  ( -1.174540682414697335, -0.08942795157527998196, 0.3641732283464567121 ) ) ;
#61466=CARTESIAN_POINT ( 'NONE',  ( 0.08907927694007038155, -1.094630224652485432E-15, 0.4281993546915535687 ) ) ;
#61467=CARTESIAN_POINT ( 'NONE',  ( 0.2165354330708668673, -0.5400638737290844871, 0.3530559997133364547 ) ) ;
#61468=CARTESIAN_POINT ( 'NONE',  ( -0.7611548556430438595, -0.6046776061558809534, -0.2411417322834644161 ) ) ;
#61470=CARTESIAN_POINT ( 'NONE',  ( -1.167979002624671470, 0.05413385826771666132, 0.4176697321401328100 ) ) ;
#61472=CARTESIAN_POINT ( 'NONE',  ( 1.076115485564305141, 0.2306618581243847221, -0.2411417322834647770 ) ) ;
#61474=CARTESIAN_POINT ( 'NONE',  ( 1.286089238845145033, -0.5023911411419708095, -0.1820866141732282451 ) ) ;
#61475=ORIENTED_EDGE ( 'NONE', *, *, #46438, .F. ) ;
#61477=CARTESIAN_POINT ( 'NONE',  ( -0.4921259842519677963, 0.1660481256975883668, -0.3530559997133364547 ) ) ;
#61479=CARTESIAN_POINT ( 'NONE',  ( 0.4593175853018379162, -0.3690944881889763329, 0.3153832671262228327 ) ) ;
#61480=CARTESIAN_POINT ( 'NONE',  ( -1.496062992125983815, -0.1870078740157480879, -0.4822834645669291653 ) ) ;
#61481=CARTESIAN_POINT ( 'NONE',  ( 0.5446194225721792126, -0.05778040916215560624, -0.4822834645669293319 ) ) ;
#61482=CARTESIAN_POINT ( 'NONE',  ( 0.8727034120734912248, -0.3162353388693409650, -0.4822834645669289433 ) ) ;
#61483=CARTESIAN_POINT ( 'NONE',  ( -0.1837270341207343505, -0.6046776061558807314, 0.2411417322834647770 ) ) ;
#61485=CARTESIAN_POINT ( 'NONE',  ( -0.9317585301837263412, -0.4281496062992127816, -0.4176697321401328100 ) ) ;
#61488=CARTESIAN_POINT ( 'NONE',  ( -1.437007874015747477, -0.5400638737290844871, 0.3530559997133364547 ) ) ;
#61489=CARTESIAN_POINT ( 'NONE',  ( -0.9120734908136475250, -0.6692913385826773087, -0.1292274648535924053 ) ) ;
#61490=CARTESIAN_POINT ( 'NONE',  ( 1.122047244094488860, -0.5400638737290845981, -0.3530559997133363437 ) ) ;
#61491=CARTESIAN_POINT ( 'NONE',  ( 1.594488188976378673, -0.5400638737290845981, -0.3530559997133363437 ) ) ;
#61493=CARTESIAN_POINT ( 'NONE',  ( -1.056430446194224881, 0.2952755905511810774, -0.1292274648535930714 ) ) ;
#61495=CARTESIAN_POINT ( 'NONE',  ( 0.4724409448818904789, -0.1870078740157479769, 0.4822834645669291653 ) ) ;
#61497=CARTESIAN_POINT ( 'NONE',  ( -0.5708661417322825615, -0.5400638737290844871, 0.3530559997133364547 ) ) ;
#61499=CARTESIAN_POINT ( 'NONE',  ( -1.627296587926508442, 0.1283753931104748280, 0.1820866141732283561 ) ) ;
#61500=CARTESIAN_POINT ( 'NONE',  ( 0.6758530183727039509, -0.5511811023622046335, 0.09757992244046803654 ) ) ;
#61501=CARTESIAN_POINT ( 'NONE',  ( 1.233595800524935227, -0.6046776061558807314, 0.2411417322834647770 ) ) ;
#61503=CARTESIAN_POINT ( 'NONE',  ( 0.7086614173228353852, -0.1870078740157479769, 0.3641732283464567677 ) ) ;
#61505=CARTESIAN_POINT ( 'NONE',  ( 0.6496062992125991586, 0.1660481256975885056, 0.3530559997133364547 ) ) ;
#61507=CARTESIAN_POINT ( 'NONE',  ( -0.5774278215223089816, 0.2306618581243847221, -0.2411417322834647770 ) ) ;
#61509=CARTESIAN_POINT ( 'NONE',  ( 1.299212598425197429, 0.1771653543307087630, 0.000000000000000000 ) ) ;
#61510=CARTESIAN_POINT ( 'NONE',  ( -0.7086614173228339419, -0.1870078740157480879, -0.4822834645669291653 ) ) ;
#61512=CARTESIAN_POINT ( 'NONE',  ( 0.1312335958005255154, -0.6046776061558807314, 0.2411417322834647770 ) ) ;
#61513=CARTESIAN_POINT ( 'NONE',  ( -1.135170603674539924, 0.2952755905511810219, -0.1292274648535930437 ) ) ;
#61514=CARTESIAN_POINT ( 'NONE',  ( -0.02624671916010428221, -0.6046776061558807314, 0.2411417322834647770 ) ) ;
#61515=CARTESIAN_POINT ( 'NONE',  ( 0.4199475065616805614, 0.1283753931104748280, 0.1820866141732283561 ) ) ;
#61517=CARTESIAN_POINT ( 'NONE',  ( 0.1377952755905518800, 0.07958543189024071263, -0.2665933059059888421 ) ) ;
#61518=CARTESIAN_POINT ( 'NONE',  ( 0.8398950131233602345, 0.1283753931104746893, -0.1820866141732285504 ) ) ;
#61519=CARTESIAN_POINT ( 'NONE',  ( -1.049868766404198794, 0.1539470093639521697, -0.1968503937007875793 ) ) ;
#61521=CARTESIAN_POINT ( 'NONE',  ( 0.6889763779527566800, -0.5400638737290844871, 0.3530559997133364547 ) ) ;
#61523=CARTESIAN_POINT ( 'NONE',  ( 1.633858267716535639, -0.4536011799217367080, 0.2665933059059888421 ) ) ;
#61524=CARTESIAN_POINT ( 'NONE',  ( 0.1115485564304470184, 0.2952755905511811885, 0.1292274648535926551 ) ) ;
#61525=CARTESIAN_POINT ( 'NONE',  ( 0.1771653543307093182, 0.07958543189024085140, 0.2665933059059887866 ) ) ;
#61526=CARTESIAN_POINT ( 'NONE',  ( 0.2230971128608932319, -0.4281496062992124485, 0.4176697321401328655 ) ) ;
#61527=CARTESIAN_POINT ( 'NONE',  ( 1.299212598425197429, -0.5511811023622047445, 6.969142054262312111E-17 ) ) ;
#61528=CARTESIAN_POINT ( 'NONE',  ( -1.227034120734907585, 0.1771653543307087630, 0.09757992244046791164 ) ) ;
#61529=CARTESIAN_POINT ( 'NONE',  ( -1.364829396325458521, 0.2306618581243847221, -0.2411417322834647770 ) ) ;
#61530=CARTESIAN_POINT ( 'NONE',  ( 0.2690288713910767848, 0.2952755905511811885, 0.1292274648535926551 ) ) ;
#61532=CARTESIAN_POINT ( 'NONE',  ( 1.148293963254593875, -0.6692913385826771977, 0.1292274648535927661 ) ) ;
#61534=CARTESIAN_POINT ( 'NONE',  ( 0.1115485564304467270, -0.6692913385826773087, -0.1292274648535924053 ) ) ;
#61535=CARTESIAN_POINT ( 'NONE',  ( 1.377952755905512472, 0.2952755905511811885, 0.000000000000000000 ) ) ;
#61536=CARTESIAN_POINT ( 'NONE',  ( 0.8858267716535438430, 0.1660481256975885056, 0.3530559997133364547 ) ) ;
#61538=CARTESIAN_POINT ( 'NONE',  ( 0.9973753280839902091, -0.5023911411419708095, 0.1820866141732285504 ) ) ;
#61539=CARTESIAN_POINT ( 'NONE',  ( 1.607611548556431069, -0.6692913385826773087, -0.1292274648535924053 ) ) ;
#61541=CARTESIAN_POINT ( 'NONE',  ( 0.1837270341207354329, 0.1283753931104748280, 0.1820866141732283561 ) ) ;
#61542=CARTESIAN_POINT ( 'NONE',  ( 0.1115485564304470323, 0.2952755905511811885, 0.1292274648535926551 ) ) ;
#61543=CARTESIAN_POINT ( 'NONE',  ( 0.6430446194225728496, 0.05413385826771666132, 0.4176697321401328100 ) ) ;
#61544=CARTESIAN_POINT ( 'NONE',  ( -0.4855643044619415427, 0.05413385826771626580, -0.4176697321401330321 ) ) ;
#61546=CARTESIAN_POINT ( 'NONE',  ( -0.4396325459317579898, 0.1771653543307087630, 0.09757992244046791164 ) ) ;
#61547=CARTESIAN_POINT ( 'NONE',  ( 0.6496062992125991586, 0.1660481256975885056, 0.3530559997133364547 ) ) ;
#61549=CARTESIAN_POINT ( 'NONE',  ( 1.043307086614173818, 0.07958543189024085140, 0.2665933059059887866 ) ) ;
#61551=CARTESIAN_POINT ( 'NONE',  ( -1.092353285368623750, -2.191421614605370878E-15, 0.4445507791589071167 ) ) ;
#61553=CARTESIAN_POINT ( 'NONE',  ( -1.220472440944882830, 0.2066929133858268208, 2.389277853677468338E-14 ) ) ;
#61554=VECTOR ( 'NONE', #46308, 39.37007874015748143 ) ;
#61555=CARTESIAN_POINT ( 'NONE',  ( -1.194225721784776262, -0.4281496062992124485, 0.4176697321401328655 ) ) ;
#61556=CARTESIAN_POINT ( 'NONE',  ( -0.4790026246719154557, -0.3162353388693405765, 0.4822834645669290543 ) ) ;
#61560=CARTESIAN_POINT ( 'NONE',  ( 0.2755905511811031494, 0.1771653543307087630, 0.000000000000000000 ) ) ;
#61562=CARTESIAN_POINT ( 'NONE',  ( 0.8989501312335963501, -0.6692913385826773087, -0.1292274648535924053 ) ) ;
#61564=CARTESIAN_POINT ( 'NONE',  ( 1.013613127888309595, -4.408777212815537393E-16, -0.4445507791589063395 ) ) ;
#61566=DIRECTION ( 'NONE',  ( 0.000000000000000000, 0.000000000000000000, 1.000000000000000000 ) ) ;
#61567=CARTESIAN_POINT ( 'NONE',  ( 1.384514435695538337, -0.5511811023622046335, 0.09757992244046803654 ) ) ;
#61568=CARTESIAN_POINT ( 'NONE',  ( 0.4790026246719168435, -0.3162353388693409650, -0.4822834645669289433 ) ) ;
#61570=CARTESIAN_POINT ( 'NONE',  ( 0.04593175853018440641, -0.6692913385826771977, 0.1292274648535927661 ) ) ;
#61571=CARTESIAN_POINT ( 'NONE',  ( -1.089238845144356427, -0.004921259842519576551, 0.3153832671262227771 ) ) ;
#61572=CARTESIAN_POINT ( 'NONE',  ( 0.4461942257217855201, -0.6046776061558807314, 0.2411417322834647770 ) ) ;
#61573=CARTESIAN_POINT ( 'NONE',  ( 0.04593175853018440641, 0.2952755905511810774, -0.1292274648535930714 ) ) ;
#61577=CARTESIAN_POINT ( 'NONE',  ( 0.9711286089238851948, -0.6046776061558809534, -0.2411417322834644161 ) ) ;
#61578=CARTESIAN_POINT ( 'NONE',  ( -0.1443569553805768291, 0.05413385826771666132, 0.4176697321401328100 ) ) ;
#61579=CARTESIAN_POINT ( 'NONE',  ( -1.154855643044618851, 0.2306618581243848609, 0.2411417322834645549 ) ) ;
#61580=CARTESIAN_POINT ( 'NONE',  ( 1.108923884514436242, -0.05778040916215522460, 0.4822834645669289988 ) ) ;
#61581=CARTESIAN_POINT ( 'NONE',  ( 0.4790026246719168435, -0.3162353388693409650, -0.4822834645669289433 ) ) ;
#61583=CARTESIAN_POINT ( 'NONE',  ( -0.3543307086614165824, -0.6692913385826771977, 8.415575281601705876E-17 ) ) ;
#61584=CARTESIAN_POINT ( 'NONE',  ( 0.2690288713910767848, 0.2952755905511811885, 0.1292274648535926551 ) ) ;
#61585=CARTESIAN_POINT ( 'NONE',  ( -0.3674540682414689785, 0.2306618581243848609, 0.2411417322834645549 ) ) ;
#61586=CARTESIAN_POINT ( 'NONE',  ( 0.1902887139107617975, -0.5511811023622048555, -0.09757992244046775898 ) ) ;
#61587=CARTESIAN_POINT ( 'NONE',  ( -1.633858267716534529, -0.5400638737290845981, -0.3530559997133363437 ) ) ;
#61589=CARTESIAN_POINT ( 'NONE',  ( 0.2887139107611556010, -0.6046776061558807314, 0.2411417322834647770 ) ) ;
#61591=CARTESIAN_POINT ( 'NONE',  ( 1.371391076115485719, -0.6692913385826773087, -0.1292274648535924053 ) ) ;
#61594=EDGE_LOOP ( 'NONE', ( #53053, #47595, #6406, #9640 ) ) ;
#61595=CARTESIAN_POINT ( 'NONE',  ( 0.5446194225721792126, -0.3162353388693405765, 0.4822834645669290543 ) ) ;
#61596=CARTESIAN_POINT ( 'NONE',  ( 0.6233595800524939223, -0.2845877964562159024, 0.3641732283464567677 ) ) ;
#61598=CARTESIAN_POINT ( 'NONE',  ( 2.795275590551181466, 2.165354330708662012, 0.000000000000000000 ) ) ;
#61601=CARTESIAN_POINT ( 'NONE',  ( 0.7190005367825900162, -6.840088175765282460E-16, 0.4281993546915531246 ) ) ;
#61605=CARTESIAN_POINT ( 'NONE',  ( 0.8202099737532813073, 0.2952755905511811885, 0.1292274648535926551 ) ) ;
#61606=CARTESIAN_POINT ( 'NONE',  ( -0.6167979002624665030, -0.4281496062992127816, -0.4176697321401328100 ) ) ;
#61607=CARTESIAN_POINT ( 'NONE',  ( -0.5314960629921254842, -0.5400638737290845981, -0.3530559997133363437 ) ) ;
#61608=CARTESIAN_POINT ( 'NONE',  ( 0.7545931758530188826, -0.6692913385826771977, 0.1292274648535927661 ) ) ;
#61609=CARTESIAN_POINT ( 'NONE',  ( 1.443569553805774897, 0.2306618581243848609, 0.2411417322834645549 ) ) ;
#61612=CARTESIAN_POINT ( 'NONE',  ( 1.417322834645670104, -0.1870078740157480601, -0.3641732283464567677 ) ) ;
#61614=CARTESIAN_POINT ( 'NONE',  ( -1.410761154855641575, -0.2845877964562161244, -0.3641732283464567121 ) ) ;
#61616=CARTESIAN_POINT ( 'NONE',  ( 0.2952755905511819101, 0.1660481256975883668, -0.3530559997133364547 ) ) ;
#61617=CARTESIAN_POINT ( 'NONE',  ( 1.200787401574803681, 0.1660481256975885056, 0.3530559997133364547 ) ) ;
#61619=CARTESIAN_POINT ( 'NONE',  ( -1.227034120734907585, 0.1771653543307087630, 0.09757992244046791164 ) ) ;
#61620=CARTESIAN_POINT ( 'NONE',  ( 0.3608923884514443348, -0.6692913385826771977, 0.1292274648535927661 ) ) ;
#61621=CARTESIAN_POINT ( 'NONE',  ( 1.095800524934383846, -0.2845877964562159024, 0.3641732283464567677 ) ) ;
#61623=CARTESIAN_POINT ( 'NONE',  ( -1.305774278215222184, -0.5511811023622048555, -0.09757992244046775898 ) ) ;
#61624=CARTESIAN_POINT ( 'NONE',  ( 1.312335958005250269, -0.6046776061558807314, 0.2411417322834647770 ) ) ;
#61626=CARTESIAN_POINT ( 'NONE',  ( -0.2690288713910754526, 0.1771653543307087075, -0.09757992244046823083 ) ) ;
#61627=CARTESIAN_POINT ( 'NONE',  ( -0.2624671916010490880, 0.2306618581243847221, -0.2411417322834647770 ) ) ;
#61628=CARTESIAN_POINT ( 'NONE',  ( -1.437007874015747477, 0.07958543189024071263, -0.2665933059059888421 ) ) ;
#61629=CARTESIAN_POINT ( 'NONE',  ( -0.6299212598425188991, -0.1870078740157479769, 0.4822834645669291653 ) ) ;
#61630=CARTESIAN_POINT ( 'NONE',  ( -1.404199475065615932, -0.3690944881889765550, -0.3153832671262227771 ) ) ;
#61633=CARTESIAN_POINT ( 'NONE',  ( -1.646051170424378096, 0.000000000000000000, -0.3464511005275205946 ) ) ;
#61634=CARTESIAN_POINT ( 'NONE',  ( 1.463254593175853824, 0.2952755905511810774, -0.1292274648535930714 ) ) ;
#61636=CARTESIAN_POINT ( 'NONE',  ( -1.345144356955379816, -0.05778040916215560624, -0.4822834645669293319 ) ) ;
#61637=CARTESIAN_POINT ( 'NONE',  ( -1.069553805774277722, -0.5511811023622048555, -0.09757992244046775898 ) ) ;
#61638=CARTESIAN_POINT ( 'NONE',  ( -0.7808398950131225646, -0.08942795157527998196, 0.3641732283464567121 ) ) ;
#61640=CARTESIAN_POINT ( 'NONE',  ( 0.1968503937007881344, -0.6692913385826771977, 8.415575281601705876E-17 ) ) ;
#61641=CARTESIAN_POINT ( 'NONE',  ( 0.6036745406824154392, 0.1283753931104746893, -0.1820866141732285504 ) ) ;
#61642=CARTESIAN_POINT ( 'NONE',  ( -1.227034120734907585, 0.1771653543307087630, 0.09757992244046791164 ) ) ;
#61643=CARTESIAN_POINT ( 'NONE',  ( -1.561679790026246017, 0.05413385826771666132, 0.4176697321401328100 ) ) ;
#61644=CARTESIAN_POINT ( 'NONE',  ( 1.220472440944882386, -0.5511811023622047445, 6.969142054262312111E-17 ) ) ;
#61645=CARTESIAN_POINT ( 'NONE',  ( 1.351706036745407680, 0.05413385826771666132, 0.4176697321401328100 ) ) ;
#61647=CARTESIAN_POINT ( 'NONE',  ( 0.2821522309711292364, 0.1771653543307087075, -0.09757992244046823083 ) ) ;
#61648=CARTESIAN_POINT ( 'NONE',  ( 1.062992125984252745, 0.2952755905511811885, 0.000000000000000000 ) ) ;
#61650=CARTESIAN_POINT ( 'NONE',  ( 1.076115485564305141, -0.5023911411419708095, 0.1820866141732285504 ) ) ;
#61652=CARTESIAN_POINT ( 'NONE',  ( -1.371391076115484609, -0.6692913385826771977, 0.1292274648535927661 ) ) ;
#61653=CARTESIAN_POINT ( 'NONE',  ( -0.7086614173228339419, -0.1870078740157479769, 0.4822834645669291653 ) ) ;
#61654=CARTESIAN_POINT ( 'NONE',  ( 0.01968503937007930540, 0.1660481256975885056, 0.3530559997133364547 ) ) ;
#61657=CARTESIAN_POINT ( 'NONE',  ( 0.9251968503937015864, -0.5400638737290844871, 0.3530559997133364547 ) ) ;
#61658=CARTESIAN_POINT ( 'NONE',  ( 1.371391076115485719, -0.5511811023622048555, -0.09757992244046775898 ) ) ;
#61659=CARTESIAN_POINT ( 'NONE',  ( -0.07874015748031421014, -0.1870078740157479769, 0.4822834645669291653 ) ) ;
#61660=CARTESIAN_POINT ( 'NONE',  ( 0.7020997375328090762, -0.05778040916215560624, -0.4822834645669293319 ) ) ;
#61666=CARTESIAN_POINT ( 'NONE',  ( -0.2821522309711278487, 0.1771653543307087630, 0.09757992244046791164 ) ) ;
#61667=CARTESIAN_POINT ( 'NONE',  ( -0.5643044619422565855, 0.05413385826771626580, -0.4176697321401330321 ) ) ;
#61668=CARTESIAN_POINT ( 'NONE',  ( 0.8398950131233602345, 0.2306618581243847221, -0.2411417322834647770 ) ) ;
#61670=CARTESIAN_POINT ( 'NONE',  ( -0.5839895013123351797, -0.5511811023622046335, 0.09757992244046803654 ) ) ;
#61671=CARTESIAN_POINT ( 'NONE',  ( -1.443569553805773564, 0.2306618581243847221, -0.2411417322834647770 ) ) ;
#61672=CARTESIAN_POINT ( 'NONE',  ( 1.246719160104987623, -0.4281496062992124485, 0.4176697321401328655 ) ) ;
#61675=CARTESIAN_POINT ( 'NONE',  ( 2.787279214012418738, 0.000000000000000000, 0.000000000000000000 ) ) ;
#61677=CARTESIAN_POINT ( 'NONE',  ( 0.9514435695538062676, -0.05778040916215522460, 0.4822834645669289988 ) ) ;
#61678=CARTESIAN_POINT ( 'NONE',  ( 1.279527559055118724, 0.07958543189024085140, 0.2665933059059887866 ) ) ;
#61679=CARTESIAN_POINT ( 'NONE',  ( -1.653543307086613234, -0.1870078740157479769, 0.3641732283464567677 ) ) ;
#61680=CARTESIAN_POINT ( 'NONE',  ( -1.581364829396324945, -0.05778040916215560624, -0.4822834645669293319 ) ) ;
#61683=CARTESIAN_POINT ( 'NONE',  ( 0.6299212598425204535, -0.1870078740157480879, -0.4822834645669291653 ) ) ;
#61684=CARTESIAN_POINT ( 'NONE',  ( -1.528871391076114250, 0.2952755905511810774, -0.1292274648535930714 ) ) ;
#61685=CARTESIAN_POINT ( 'NONE',  ( -0.6102362204724400829, 0.1660481256975885056, 0.3530559997133364547 ) ) ;
#61686=CARTESIAN_POINT ( 'NONE',  ( -0.6299212598425188991, -0.1870078740157479769, 0.4822834645669291653 ) ) ;
#61687=CARTESIAN_POINT ( 'NONE',  ( 1.469816272965879911, 0.2306618581243847221, -0.2411417322834647770 ) ) ;
#61689=EDGE_CURVE ( 'NONE', #56464, #24808, #74614, .T. ) ;
#61690=CARTESIAN_POINT ( 'NONE',  ( 0.2821522309711292364, -0.6692913385826771977, 0.1292274648535927661 ) ) ;
#61692=CARTESIAN_POINT ( 'NONE',  ( -1.607611548556429737, 0.1771653543307087075, -0.09757992244046823083 ) ) ;
#61697=CARTESIAN_POINT ( 'NONE',  ( -1.522309711286088607, 0.2306618581243847221, -0.2411417322834647770 ) ) ;
#61699=CARTESIAN_POINT ( 'NONE',  ( 0.5615202218219601527, -1.094630224652485432E-15, 0.4281993546915535687 ) ) ;
#61701=CARTESIAN_POINT ( 'NONE',  ( 0.4068241469816281097, 0.05413385826771666132, 0.4176697321401328100 ) ) ;
#61704=CARTESIAN_POINT ( 'NONE',  ( -0.1640419947506553400, -0.08942795157528024563, -0.3641732283464568787 ) ) ;
#61705=CARTESIAN_POINT ( 'NONE',  ( -1.233595800524933894, 0.1283753931104748280, 0.1820866141732283561 ) ) ;
#61706=CARTESIAN_POINT ( 'NONE',  ( -1.594488188976377119, 0.1660481256975883668, -0.3530559997133364547 ) ) ;
#61707=CARTESIAN_POINT ( 'NONE',  ( 0.3215223097112867578, -0.05778040916215522460, 0.4822834645669289988 ) ) ;
#61708=CARTESIAN_POINT ( 'NONE',  ( -1.515748031496062076, -0.5400638737290844871, 0.3530559997133364547 ) ) ;
#61711=CARTESIAN_POINT ( 'NONE',  ( -1.509186351706035767, -0.4281496062992124485, 0.4176697321401328655 ) ) ;
#61715=( BOUNDED_CURVE ( )  B_SPLINE_CURVE ( 2, ( #62365, #35051, #67877, #68691, #36286, #74191, #4703, #22424, #67458, #55217, #28733, #35464, #61551 ),
 .UNSPECIFIED., .F., .F. ) 
 B_SPLINE_CURVE_WITH_KNOTS ( ( 3, 2, 2, 2, 2, 2, 3 ),
 ( 0.7642401855438917258, 0.7651515151515151381, 0.7689393939393939226, 0.7727272727272727071, 0.7765151515151514916, 0.7803030303030302761, 0.7812143599106537994 ),
 .UNSPECIFIED. ) 
 CURVE ( )  GEOMETRIC_REPRESENTATION_ITEM ( )  RATIONAL_B_SPLINE_CURVE ( ( 0.9875488213027523443, 0.9918020599134680371, 1.000000000000000000, 0.9659258262890683122, 1.000000000000000000, 0.9659258262890683122, 1.000000000000000000, 0.9659258262890683122, 1.000000000000000000, 0.9659258262890683122, 1.000000000000000000, 0.9918020599134671489, 0.9875488213027514561 ) ) 
 REPRESENTATION_ITEM ( '' )  );
#61717=CARTESIAN_POINT ( 'NONE',  ( -0.8923884514435688198, -0.6046776061558807314, 0.2411417322834647770 ) ) ;
#61718=CARTESIAN_POINT ( 'NONE',  ( 1.391076115485564868, 0.2306618581243847221, -0.2411417322834647770 ) ) ;
#61719=CARTESIAN_POINT ( 'NONE',  ( -1.515748031496062076, 0.1660481256975883668, -0.3530559997133364547 ) ) ;
#61721=AXIS2_PLACEMENT_3D ( 'NONE', #6188, #50796, #44471 ) ;
#61722=CARTESIAN_POINT ( 'NONE',  ( -1.732283464566928277, -0.1870078740157479769, 0.4822834645669291653 ) ) ;
#61723=CARTESIAN_POINT ( 'NONE',  ( -0.6561679790026240244, -0.6046776061558807314, 0.2411417322834647770 ) ) ;
#61725=CARTESIAN_POINT ( 'NONE',  ( 0.07874015748031558404, -0.1870078740157480601, -0.3641732283464567677 ) ) ;
#61727=CARTESIAN_POINT ( 'NONE',  ( -0.06561679790026180015, -0.004921259842519576551, 0.3153832671262227771 ) ) ;
#61728=CARTESIAN_POINT ( 'NONE',  ( 0.6167979002624678353, -0.3690944881889763329, 0.3153832671262228327 ) ) ;
#61729=CARTESIAN_POINT ( 'NONE',  ( 0.5774278215223103139, -0.6046776061558809534, -0.2411417322834644161 ) ) ;
#61730=CARTESIAN_POINT ( 'NONE',  ( -0.1968503937007867743, 0.1771653543307087630, 0.000000000000000000 ) ) ;
#61732=CARTESIAN_POINT ( 'NONE',  ( -1.587926509186350810, 0.05413385826771626580, -0.4176697321401330321 ) ) ;
#61733=CARTESIAN_POINT ( 'NONE',  ( -1.102362204724408601, -0.1870078740157480879, -0.4822834645669291653 ) ) ;
#61735=CARTESIAN_POINT ( 'NONE',  ( -0.06561679790026180015, -0.4281496062992127816, -0.4176697321401328100 ) ) ;
#61736=CARTESIAN_POINT ( 'NONE',  ( -0.3871391076115476282, -0.05778040916215522460, 0.4822834645669289988 ) ) ;
#61737=CARTESIAN_POINT ( 'NONE',  ( 1.561679790026247350, -0.004921259842519870586, -0.3153832671262229437 ) ) ;
#61738=CARTESIAN_POINT ( 'NONE',  ( -0.01968503937007793844, -0.4536011799217367080, 0.2665933059059888421 ) ) ;
#61739=CARTESIAN_POINT ( 'NONE',  ( -0.1443569553805768291, 0.05413385826771666132, 0.4176697321401328100 ) ) ;
#61740=CARTESIAN_POINT ( 'NONE',  ( -0.5314960629921250401, 0.1660481256975885056, 0.3530559997133364547 ) ) ;
#61743=CARTESIAN_POINT ( 'NONE',  ( 0.1115485564304470323, 0.2952755905511811885, 0.1292274648535926551 ) ) ;
#61744=ORIENTED_EDGE ( 'NONE', *, *, #1251, .T. ) ;
#61746=CARTESIAN_POINT ( 'NONE',  ( 1.548556430446194954, -0.6046776061558807314, 0.2411417322834647770 ) ) ;
#61747=CARTESIAN_POINT ( 'NONE',  ( -0.6167979002624665030, -0.004921259842519576551, 0.3153832671262227771 ) ) ;
#61748=CARTESIAN_POINT ( 'NONE',  ( -0.7349081364829390672, 0.2306618581243847221, -0.2411417322834647770 ) ) ;
#61749=CARTESIAN_POINT ( 'NONE',  ( 1.305774278215223960, -0.6692913385826771977, 0.1292274648535927661 ) ) ;
#61750=CARTESIAN_POINT ( 'NONE',  ( 1.377952755905512472, 0.2952755905511811885, 0.000000000000000000 ) ) ;
#61751=CARTESIAN_POINT ( 'NONE',  ( -1.587926509186350810, 0.05413385826771626580, -0.4176697321401330321 ) ) ;
#61752=CARTESIAN_POINT ( 'NONE',  ( -1.062992125984250968, 0.1771653543307087630, 0.000000000000000000 ) ) ;
#61756=CARTESIAN_POINT ( 'NONE',  ( 1.601049868766404982, -0.5023911411419708095, -0.1820866141732282451 ) ) ;
#61757=CARTESIAN_POINT ( 'NONE',  ( 1.108923884514436242, -0.08942795157527998196, 0.3641732283464567121 ) ) ;
#61758=CARTESIAN_POINT ( 'NONE',  ( 0.5446194225721792126, -0.05778040916215560624, -0.4822834645669293319 ) ) ;
#61759=CARTESIAN_POINT ( 'NONE',  ( -1.673228346456691717, 0.1660481256975883668, -0.3530559997133364547 ) ) ;
#61760=CARTESIAN_POINT ( 'NONE',  ( 0.9711286089238851948, 0.2306618581243848609, 0.2411417322834645549 ) ) ;
#61762=CARTESIAN_POINT ( 'NONE',  ( 1.384514435695538559, 0.1771653543307087075, -0.09757992244046823083 ) ) ;
#61763=CARTESIAN_POINT ( 'NONE',  ( 0.1312335958005257930, 0.2306618581243847221, -0.2411417322834647770 ) ) ;
#61764=CARTESIAN_POINT ( 'NONE',  ( -0.8792650918635160906, -0.4281496062992124485, 0.4176697321401328655 ) ) ;
#61765=CARTESIAN_POINT ( 'NONE',  ( 1.207349081364829990, 0.2306618581243848609, 0.2411417322834645549 ) ) ;
#61768=CARTESIAN_POINT ( 'NONE',  ( 0.3937007874015754361, -0.1870078740157480601, -0.3641732283464567677 ) ) ;
#61772=CARTESIAN_POINT ( 'NONE',  ( -0.8530183727034112984, -0.4281496062992127816, -0.4176697321401328100 ) ) ;
#61773=CARTESIAN_POINT ( 'NONE',  ( -0.1312335958005241554, -0.6046776061558809534, -0.2411417322834644161 ) ) ;
#61774=CARTESIAN_POINT ( 'NONE',  ( -0.2493438320209966919, -0.4281496062992124485, 0.4176697321401328655 ) ) ;
#61775=CARTESIAN_POINT ( 'NONE',  ( 0.7874015748031503170, -0.1870078740157480879, -0.4822834645669291653 ) ) ;
#61776=CARTESIAN_POINT ( 'NONE',  ( -1.345144356955379816, -0.3162353388693405765, 0.4822834645669290543 ) ) ;
#61777=CARTESIAN_POINT ( 'NONE',  ( -0.4986876640419942164, -0.6046776061558807314, 0.2411417322834647770 ) ) ;
#61778=CARTESIAN_POINT ( 'NONE',  ( 0.7414698162729663755, -0.6692913385826773087, -0.1292274648535924053 ) ) ;
#61779=CARTESIAN_POINT ( 'NONE',  ( 0.3149606299212603933, -0.1870078740157479769, 0.4822834645669291653 ) ) ;
#61780=CARTESIAN_POINT ( 'NONE',  ( 0.8005249343832028242, -0.4281496062992127816, -0.4176697321401328100 ) ) ;
#61783=CARTESIAN_POINT ( 'NONE',  ( -0.4265091863517051496, -0.5511811023622046335, 0.09757992244046803654 ) ) ;
#61787=CARTESIAN_POINT ( 'NONE',  ( -1.200787401574802349, 0.07958543189024071263, -0.2665933059059888421 ) ) ;
#61788=CARTESIAN_POINT ( 'NONE',  ( -0.5118110236220466680, 0.2952755905511811885, 0.000000000000000000 ) ) ;
#61789=DIRECTION ( 'NONE',  ( 0.000000000000000000, 0.000000000000000000, 1.000000000000000000 ) ) ;
#61790=CARTESIAN_POINT ( 'NONE',  ( -0.7480314960629914633, 0.2952755905511811885, 0.000000000000000000 ) ) ;
#61791=CARTESIAN_POINT ( 'NONE',  ( -0.6758530183727028406, -0.6692913385826773087, -0.1292274648535924053 ) ) ;
#61792=CARTESIAN_POINT ( 'NONE',  ( -1.397637795275589623, -0.5400638737290845981, -0.3530559997133363437 ) ) ;
#61793=CARTESIAN_POINT ( 'NONE',  ( -1.509186351706035767, 0.05413385826771626580, -0.4176697321401330321 ) ) ;
#61794=CARTESIAN_POINT ( 'NONE',  ( 0.9383202099737538715, -0.08942795157528024563, -0.3641732283464568787 ) ) ;
#61797=CARTESIAN_POINT ( 'NONE',  ( 0.2296587926509192634, -0.08942795157528024563, -0.3641732283464568787 ) ) ;
#61798=CARTESIAN_POINT ( 'NONE',  ( -0.2559055118110227234, -0.5400638737290844871, 0.3530559997133364547 ) ) ;
#61799=CARTESIAN_POINT ( 'NONE',  ( 0.1246719160104994284, 0.2952755905511810774, -0.1292274648535930714 ) ) ;
#61800=ORIENTED_EDGE ( 'NONE', *, *, #47629, .T. ) ;
#61805=CARTESIAN_POINT ( 'NONE',  ( 1.614173228346457378, 0.4410134679336836783, -0.1372047244094476148 ) ) ;
#61806=CARTESIAN_POINT ( 'NONE',  ( -0.7480314960629914633, 0.1771653543307087630, 0.000000000000000000 ) ) ;
#61807=CARTESIAN_POINT ( 'NONE',  ( -0.8202099737532801971, -0.6692913385826771977, 0.1292274648535927661 ) ) ;
#61811=CARTESIAN_POINT ( 'NONE',  ( 1.417322834645670104, -0.1870078740157480879, -0.4822834645669291653 ) ) ;
#61812=CARTESIAN_POINT ( 'NONE',  ( 0.3543307086614179147, 0.2952755905511811885, 0.000000000000000000 ) ) ;
#61813=CARTESIAN_POINT ( 'NONE',  ( 0.5643044619422579178, 0.05413385826771666132, 0.4176697321401328100 ) ) ;
#61814=CARTESIAN_POINT ( 'NONE',  ( -0.8333333333333323711, 0.1771653543307087630, 0.09757992244046791164 ) ) ;
#61815=CARTESIAN_POINT ( 'NONE',  ( -0.1049868766404193215, 0.2306618581243847221, -0.2411417322834647770 ) ) ;
#61817=CARTESIAN_POINT ( 'NONE',  ( -0.4527559055118102749, 0.1660481256975885056, 0.3530559997133364547 ) ) ;
#61819=CARTESIAN_POINT ( 'NONE',  ( 1.456692913385827515, 0.1771653543307087630, 0.000000000000000000 ) ) ;
#61820=CARTESIAN_POINT ( 'NONE',  ( -0.1312335958005241554, 0.1283753931104748280, 0.1820866141732283561 ) ) ;
#61821=CARTESIAN_POINT ( 'NONE',  ( 1.069553805774278832, 0.1771653543307087075, -0.09757992244046823083 ) ) ;
#61822=CARTESIAN_POINT ( 'NONE',  ( -1.240157480314959759, 0.1660481256975885056, 0.3530559997133364547 ) ) ;
#61823=EDGE_CURVE ( 'NONE', #59927, #42372, #41867, .T. ) ;
#61824=CARTESIAN_POINT ( 'NONE',  ( -0.9908136482939626788, 0.1771653543307087630, 0.09757992244046791164 ) ) ;
#61825=CARTESIAN_POINT ( 'NONE',  ( -2.795275590551184131, 1.023622047244095556, -2.654250759839014936E-16 ) ) ;
#61826=CARTESIAN_POINT ( 'NONE',  ( -1.181102362204723644, -0.1870078740157480879, -0.4822834645669291653 ) ) ;
#61827=CARTESIAN_POINT ( 'NONE',  ( -0.2559055118110227234, -0.5400638737290844871, 0.3530559997133364547 ) ) ;
#61828=CARTESIAN_POINT ( 'NONE',  ( 0.3937007874015754361, -0.1870078740157479769, 0.4822834645669291653 ) ) ;
#61831=CARTESIAN_POINT ( 'NONE',  ( 0.3543307086614181922, -0.5511811023622047445, 6.969142054262312111E-17 ) ) ;
#61832=CARTESIAN_POINT ( 'NONE',  ( -1.568241469816272105, -0.08942795157527998196, 0.3641732283464567121 ) ) ;
#61833=CARTESIAN_POINT ( 'NONE',  ( 0.6889763779527566800, -0.5400638737290844871, 0.3530559997133364547 ) ) ;
#61834=CARTESIAN_POINT ( 'NONE',  ( -1.607611548556429737, -0.5511811023622046335, 0.09757992244046803654 ) ) ;
#61835=CARTESIAN_POINT ( 'NONE',  ( 1.233595800524935227, -0.5023911411419708095, 0.1820866141732285504 ) ) ;
#61836=CARTESIAN_POINT ( 'NONE',  ( -0.8464566929133852113, -0.5400638737290845981, -0.3530559997133363437 ) ) ;
#61837=CARTESIAN_POINT ( 'NONE',  ( -0.09186351706036663400, -0.3690944881889763329, 0.3153832671262228327 ) ) ;
#61838=DIRECTION ( 'NONE',  ( 1.000000000000000000, 3.083952846180989294E-16, 0.000000000000000000 ) ) ;
#61839=CARTESIAN_POINT ( 'NONE',  ( 0.6758530183727039509, 0.1771653543307087075, -0.09757992244046823083 ) ) ;
#61840=CARTESIAN_POINT ( 'NONE',  ( -0.07217847769028787330, -0.05778040916215522460, 0.4822834645669289988 ) ) ;
#61844=CARTESIAN_POINT ( 'NONE',  ( 0.7152230971128614723, -0.2845877964562161244, -0.3641732283464567121 ) ) ;
#61845=CARTESIAN_POINT ( 'NONE',  ( 0.2427821522309719648, -0.05778040916215522460, 0.4822834645669289988 ) ) ;
#61846=CARTESIAN_POINT ( 'NONE',  ( -0.8136482939632537770, 0.2306618581243847221, -0.2411417322834647770 ) ) ;
#61847=CARTESIAN_POINT ( 'NONE',  ( -0.4790026246719152336, -0.08942795157528024563, -0.3641732283464568787 ) ) ;
#61849=CARTESIAN_POINT ( 'NONE',  ( -0.4002624671916004129, -0.2845877964562159024, 0.3641732283464567677 ) ) ;
#61850=CARTESIAN_POINT ( 'NONE',  ( 0.4396325459317593221, 0.2952755905511810774, -0.1292274648535930714 ) ) ;
#61851=CARTESIAN_POINT ( 'NONE',  ( -1.036745406824146176, -0.004921259842519870586, -0.3153832671262229437 ) ) ;
#61853=CARTESIAN_POINT ( 'NONE',  ( 1.541994750656168645, -0.6692913385826771977, 0.1292274648535927661 ) ) ;
#61856=CARTESIAN_POINT ( 'NONE',  ( -1.332020997375327642, -0.2845877964562161244, -0.3641732283464567121 ) ) ;
#61857=CARTESIAN_POINT ( 'NONE',  ( -0.6561679790026240244, -0.6046776061558807314, 0.2411417322834647770 ) ) ;
#61858=CARTESIAN_POINT ( 'NONE',  ( -1.279527559055116948, 0.1660481256975883668, -0.3530559997133364547 ) ) ;
#61861=CARTESIAN_POINT ( 'NONE',  ( 1.548556430446194954, 0.2306618581243847221, -0.2411417322834647770 ) ) ;
#61862=CARTESIAN_POINT ( 'NONE',  ( 0.3083989501312343062, -0.05778040916215560624, -0.4822834645669293319 ) ) ;
#61865=CARTESIAN_POINT ( 'NONE',  ( 1.476377952755906220, 0.07958543189024071263, -0.2665933059059888421 ) ) ;
#61867=ORIENTED_EDGE ( 'NONE', *, *, #37700, .T. ) ;
#61868=CARTESIAN_POINT ( 'NONE',  ( -0.8792650918635160906, -0.3690944881889763329, 0.3153832671262228327 ) ) ;
#61871=CARTESIAN_POINT ( 'NONE',  ( 0.4724409448818904789, -0.1870078740157479769, 0.4822834645669291653 ) ) ;
#61872=CARTESIAN_POINT ( 'NONE',  ( -0.5577427821522301654, -0.05778040916215560624, -0.4822834645669293319 ) ) ;
#61873=CARTESIAN_POINT ( 'NONE',  ( -0.9514435695538050464, -0.05778040916215560624, -0.4822834645669293319 ) ) ;
#61874=CARTESIAN_POINT ( 'NONE',  ( 0.8923884514435703741, 0.2306618581243848609, 0.2411417322834645549 ) ) ;
#61875=CARTESIAN_POINT ( 'NONE',  ( -1.227034120734907141, -0.5511811023622048555, -0.09757992244046775898 ) ) ;
#61877=CARTESIAN_POINT ( 'NONE',  ( 0.2427821522309719648, -0.05778040916215522460, 0.4822834645669289988 ) ) ;
#61878=CARTESIAN_POINT ( 'NONE',  ( -0.9711286089238838626, 0.2306618581243847221, -0.2411417322834647770 ) ) ;
#61880=CARTESIAN_POINT ( 'NONE',  ( 1.548556430446194954, -0.6046776061558807314, 0.2411417322834647770 ) ) ;
#61883=CARTESIAN_POINT ( 'NONE',  ( 0.9383202099737538715, -0.08942795157528024563, -0.3641732283464568787 ) ) ;
#61886=CARTESIAN_POINT ( 'NONE',  ( -0.3805774278215216522, 0.05413385826771666132, 0.4176697321401328100 ) ) ;
#61888=CARTESIAN_POINT ( 'NONE',  ( 0.5052493438320215802, 0.1771653543307087630, 0.09757992244046791164 ) ) ;
#61889=CARTESIAN_POINT ( 'NONE',  ( -1.476377952755905110, -0.5400638737290845981, -0.3530559997133363437 ) ) ;
#61890=CARTESIAN_POINT ( 'NONE',  ( 0.5249343832021003964, 0.2306618581243847221, -0.2411417322834647770 ) ) ;
#61891=CARTESIAN_POINT ( 'NONE',  ( 0.5249343832021003964, 0.2306618581243847221, -0.2411417322834647770 ) ) ;
#61892=CARTESIAN_POINT ( 'NONE',  ( -0.006561679790025524116, -0.3162353388693405765, 0.4822834645669290543 ) ) ;
#61894=CARTESIAN_POINT ( 'NONE',  ( -0.6627296587926501115, 0.2952755905511810774, -0.1292274648535930714 ) ) ;
#61896=CARTESIAN_POINT ( 'NONE',  ( 1.482939632545932307, -0.004921259842519870586, -0.3153832671262229437 ) ) ;
#61897=CARTESIAN_POINT ( 'NONE',  ( -1.102362204724408601, -0.1870078740157480879, -0.4822834645669291653 ) ) ;
#61898=CARTESIAN_POINT ( 'NONE',  ( 1.266404199475066328, -0.3162353388693409650, -0.4822834645669289433 ) ) ;
#61899=CARTESIAN_POINT ( 'NONE',  ( 1.240157480314961314, 0.1660481256975883668, -0.3530559997133364547 ) ) ;
#61902=CARTESIAN_POINT ( 'NONE',  ( -0.8136482939632537770, -0.6046776061558807314, 0.2411417322834647770 ) ) ;
#61904=CARTESIAN_POINT ( 'NONE',  ( 0.1312335958005255154, -0.6046776061558807314, 0.2411417322834647770 ) ) ;
#61906=CARTESIAN_POINT ( 'NONE',  ( -0.6758530183727028406, 0.2952755905511811885, 0.1292274648535926551 ) ) ;
#61907=CARTESIAN_POINT ( 'NONE',  ( 1.614173228346457378, -0.6692913385826771977, 8.415575281601705876E-17 ) ) ;
#61908=CARTESIAN_POINT ( 'NONE',  ( 0.6364829396325465405, -0.2845877964562161244, -0.3641732283464567121 ) ) ;
#61909=CARTESIAN_POINT ( 'NONE',  ( 1.167979002624672580, 0.05413385826771626580, -0.4176697321401330321 ) ) ;
#61911=CARTESIAN_POINT ( 'NONE',  ( 0.9448818897637802916, -0.1870078740157480601, -0.3641732283464567677 ) ) ;
#61912=CARTESIAN_POINT ( 'NONE',  ( 0.8727034120734912248, -0.3162353388693409650, -0.4822834645669289433 ) ) ;
#61914=CARTESIAN_POINT ( 'NONE',  ( -0.7086614173228339419, -0.1870078740157480879, -0.4822834645669291653 ) ) ;
#61916=CARTESIAN_POINT ( 'NONE',  ( 1.358267716535433323, -0.4536011799217368745, -0.2665933059059886201 ) ) ;
#61917=CARTESIAN_POINT ( 'NONE',  ( -0.4068241469816267775, 0.05413385826771626580, -0.4176697321401330321 ) ) ;
#61918=CARTESIAN_POINT ( 'NONE',  ( 0.2296587926509192634, -0.05778040916215560624, -0.4822834645669293319 ) ) ;
#61920=CARTESIAN_POINT ( 'NONE',  ( 0.2624671916010504757, -0.6046776061558809534, -0.2411417322834644161 ) ) ;
#61921=EDGE_CURVE ( 'NONE', #5694, #57471, #73036, .T. ) ;
#61922=CARTESIAN_POINT ( 'NONE',  ( -0.03937007874015669567, 0.1771653543307087630, 0.000000000000000000 ) ) ;
#61924=CARTESIAN_POINT ( 'NONE',  ( 0.09842519685039434474, 0.07958543189024085140, 0.2665933059059887866 ) ) ;
#61925=CARTESIAN_POINT ( 'NONE',  ( 0.9383202099737536495, -0.2845877964562159024, 0.3641732283464567677 ) ) ;
#61928=CARTESIAN_POINT ( 'NONE',  ( 0.4265091863517067594, 0.2952755905511811885, 0.1292274648535926551 ) ) ;
#61930=CARTESIAN_POINT ( 'NONE',  ( 1.528871391076116026, 0.1771653543307087630, 0.09757992244046791164 ) ) ;
#61932=CARTESIAN_POINT ( 'NONE',  ( -0.2690288713910754526, 0.1771653543307087075, -0.09757992244046823083 ) ) ;
#61933=CARTESIAN_POINT ( 'NONE',  ( 0.1902887139107617975, -0.6692913385826773087, -0.1292274648535924053 ) ) ;
#61934=CARTESIAN_POINT ( 'NONE',  ( 0.9383202099737538715, -0.08942795157528024563, -0.3641732283464568787 ) ) ;
#61935=CARTESIAN_POINT ( 'NONE',  ( -1.194225721784776262, -0.004921259842519870586, -0.3153832671262229437 ) ) ;
#61936=CARTESIAN_POINT ( 'NONE',  ( -1.633858267716534529, -0.5400638737290845981, -0.3530559997133363437 ) ) ;
#61937=CARTESIAN_POINT ( 'NONE',  ( 0.1377952755905518800, 0.1660481256975883668, -0.3530559997133364547 ) ) ;
#61938=CARTESIAN_POINT ( 'NONE',  ( 1.089238845144357759, 0.05413385826771626580, -0.4176697321401330321 ) ) ;
#61939=( BOUNDED_CURVE ( )  B_SPLINE_CURVE ( 2, ( #48553, #3123, #67105, #67515, #42652, #3953, #62019 ),
 .UNSPECIFIED., .F., .F. ) 
 B_SPLINE_CURVE_WITH_KNOTS ( ( 3, 2, 2, 3 ),
 ( 0.1363636363636364923, 0.1401515151515152213, 0.1439393939393939503, 0.1441485521566764350 ),
 .UNSPECIFIED. ) 
 CURVE ( )  GEOMETRIC_REPRESENTATION_ITEM ( )  RATIONAL_B_SPLINE_CURVE ( ( 0.9999999999999987788, 0.9659258262890695335, 1.000000000000000000, 0.9659258262890683122, 1.000000000000000000, 0.9981185001348095165, 0.9964447847208426357 ) ) 
 REPRESENTATION_ITEM ( '' )  );
#61940=EDGE_CURVE ( 'NONE', #55671, #73693, #34142, .T. ) ;
#61942=CARTESIAN_POINT ( 'NONE',  ( 0.07217847769028949700, -0.05778040916215560624, -0.4822834645669293319 ) ) ;
#61943=CARTESIAN_POINT ( 'NONE',  ( 1.220472440944882608, 0.2952755905511811885, 0.000000000000000000 ) ) ;
#61944=CARTESIAN_POINT ( 'NONE',  ( 0.8923884514435703741, 0.2306618581243848609, 0.2411417322834645549 ) ) ;
#61947=CARTESIAN_POINT ( 'NONE',  ( 0.7217847769028878924, -0.004921259842519576551, 0.3153832671262227771 ) ) ;
#61948=CARTESIAN_POINT ( 'NONE',  ( 1.548556430446194954, 0.2306618581243847221, -0.2411417322834647770 ) ) ;
#61949=CARTESIAN_POINT ( 'NONE',  ( 0.2099737532808405305, 0.1283753931104746893, -0.1820866141732285504 ) ) ;
#61950=CARTESIAN_POINT ( 'NONE',  ( -0.2427821522309703550, -0.3162353388693405765, 0.4822834645669290543 ) ) ;
#61951=CARTESIAN_POINT ( 'NONE',  ( 0.5183727034120741983, 0.2952755905511810774, -0.1292274648535930714 ) ) ;
#61952=CARTESIAN_POINT ( 'NONE',  ( -0.5708661417322825615, -0.5400638737290844871, 0.3530559997133364547 ) ) ;
#61954=CARTESIAN_POINT ( 'NONE',  ( -0.2362204724409442680, -0.1870078740157480601, -0.3641732283464567677 ) ) ;
#61956=CARTESIAN_POINT ( 'NONE',  ( 0.6889763779527563470, 0.1660481256975883668, -0.3530559997133364547 ) ) ;
#61957=CARTESIAN_POINT ( 'NONE',  ( 0.8267716535433078384, -0.5511811023622047445, 6.969142054262312111E-17 ) ) ;
#61959=CARTESIAN_POINT ( 'NONE',  ( 0.4330708661417329575, 1.805669738366188382, 0.000000000000000000 ) ) ;
#61962=CARTESIAN_POINT ( 'NONE',  ( -1.404199475065615932, -0.4281496062992127816, -0.4176697321401328100 ) ) ;
#61963=CARTESIAN_POINT ( 'NONE',  ( -0.4002624671916004129, -0.05778040916215560624, -0.4822834645669293319 ) ) ;
#61967=ORIENTED_EDGE ( 'NONE', *, *, #55092, .F. ) ;
#61968=CARTESIAN_POINT ( 'NONE',  ( 0.2493438320209980519, -0.004921259842519576551, 0.3153832671262227771 ) ) ;
#61970=CARTESIAN_POINT ( 'NONE',  ( 0.9514435695538062676, -0.05778040916215522460, 0.4822834645669289988 ) ) ;
#61974=CARTESIAN_POINT ( 'NONE',  ( -1.607611548556429737, -0.5511811023622046335, 0.09757992244046803654 ) ) ;
#61977=CARTESIAN_POINT ( 'NONE',  ( 1.233595800524935227, -0.5023911411419708095, 0.1820866141732285504 ) ) ;
#61978=CARTESIAN_POINT ( 'NONE',  ( 0.6167979002624679463, 0.05413385826771626580, -0.4176697321401330321 ) ) ;
#61980=CARTESIAN_POINT ( 'NONE',  ( -0.2034120734908128059, 0.2952755905511811885, 0.1292274648535926551 ) ) ;
#61981=CARTESIAN_POINT ( 'NONE',  ( -1.082677165354329896, 0.07958543189024085140, 0.2665933059059887866 ) ) ;
#61982=CARTESIAN_POINT ( 'NONE',  ( 0.2887139107611556010, -0.6046776061558807314, 0.2411417322834647770 ) ) ;
#61983=CARTESIAN_POINT ( 'NONE',  ( 0.09842519685039434474, -0.5400638737290845981, -0.3530559997133363437 ) ) ;
#61987=CARTESIAN_POINT ( 'NONE',  ( 0.6430446194225729606, -0.4281496062992127816, -0.4176697321401328100 ) ) ;
#61988=CARTESIAN_POINT ( 'NONE',  ( -0.2230971128608915943, -0.4281496062992127816, -0.4176697321401328100 ) ) ;
#61989=CARTESIAN_POINT ( 'NONE',  ( -1.607611548556429737, 0.2952755905511810774, -0.1292274648535930714 ) ) ;
#61990=CARTESIAN_POINT ( 'NONE',  ( 1.253280839895013710, -0.3162353388693405765, 0.4822834645669290543 ) ) ;
#61991=CARTESIAN_POINT ( 'NONE',  ( 0.3937007874015754361, -0.1870078740157479769, 0.4822834645669291653 ) ) ;
#61993=CARTESIAN_POINT ( 'NONE',  ( -0.3346456692913377662, -0.5400638737290844871, 0.3530559997133364547 ) ) ;
#61994=CARTESIAN_POINT ( 'NONE',  ( 0.09842519685039434474, 0.1660481256975885056, 0.3530559997133364547 ) ) ;
#61995=CARTESIAN_POINT ( 'NONE',  ( -0.3215223097112853146, -0.05778040916215560624, -0.4822834645669293319 ) ) ;
#61996=CARTESIAN_POINT ( 'NONE',  ( 0.4986876640419954376, -0.5023911411419708095, -0.1820866141732282451 ) ) ;
#61997=CARTESIAN_POINT ( 'NONE',  ( -1.574803149606298636, -0.1870078740157479769, 0.4822834645669291653 ) ) ;
#61999=CARTESIAN_POINT ( 'NONE',  ( 0.5380577427821529035, 0.05413385826771626580, -0.4176697321401330321 ) ) ;
#62002=CARTESIAN_POINT ( 'NONE',  ( 1.496062992125984703, -0.1870078740157480879, -0.4822834645669291653 ) ) ;
#62005=ORIENTED_EDGE ( 'NONE', *, *, #10455, .T. ) ;
#62006=CARTESIAN_POINT ( 'NONE',  ( 0.5774278215223104249, 0.2306618581243848609, 0.2411417322834645549 ) ) ;
#62007=CARTESIAN_POINT ( 'NONE',  ( 0.09186351706036799403, -0.3690944881889765550, -0.3153832671262227771 ) ) ;
#62011=ADVANCED_FACE ( 'NONE', ( #10135 ), #74527, .F. ) ;
#62013=CARTESIAN_POINT ( 'NONE',  ( 0.5643044619422579178, -0.4281496062992127816, -0.4176697321401328100 ) ) ;
#62014=CARTESIAN_POINT ( 'NONE',  ( -0.9120734908136475250, -0.6692913385826773087, -0.1292274648535924053 ) ) ;
#62015=CARTESIAN_POINT ( 'NONE',  ( -0.8792650918635160906, 0.05413385826771626580, -0.4176697321401330321 ) ) ;
#62016=CARTESIAN_POINT ( 'NONE',  ( 0.8398950131233602345, 0.2306618581243847221, -0.2411417322834647770 ) ) ;
#62018=CARTESIAN_POINT ( 'NONE',  ( 1.181102362204724976, -0.1870078740157480879, -0.4822834645669291653 ) ) ;
#62019=CARTESIAN_POINT ( 'NONE',  ( 1.193521905106662784, 3.421639014772782816E-16, 0.3464511005275203726 ) ) ;
#62021=CARTESIAN_POINT ( 'NONE',  ( 1.141732283464567788, -0.5511811023622047445, 6.969142054262312111E-17 ) ) ;
#62022=CARTESIAN_POINT ( 'NONE',  ( -0.7414698162729651543, -0.6692913385826771977, 0.1292274648535927661 ) ) ;
#62023=CARTESIAN_POINT ( 'NONE',  ( -1.646981627296586703, -0.08942795157527998196, 0.3641732283464567121 ) ) ;
#62025=CARTESIAN_POINT ( 'NONE',  ( 1.595398199321655497, 0.7585570207896586981, 0.1559797534342493297 ) ) ;
#62026=CARTESIAN_POINT ( 'NONE',  ( -0.3543307086614165824, 0.2952755905511811885, 0.000000000000000000 ) ) ;
#62027=CARTESIAN_POINT ( 'NONE',  ( 1.194225721784777594, 0.05413385826771666132, 0.4176697321401328100 ) ) ;
#62028=CARTESIAN_POINT ( 'NONE',  ( -0.7213048234621840527, 1.923042554663772385, 0.5309055118110236338 ) ) ;
#62029=CARTESIAN_POINT ( 'NONE',  ( -0.9776902887139098386, -0.5511811023622046335, 0.09757992244046803654 ) ) ;
#62030=CARTESIAN_POINT ( 'NONE',  ( 0.2624671916010504757, 0.2306618581243848609, 0.2411417322834645549 ) ) ;
#62031=CARTESIAN_POINT ( 'NONE',  ( 0.7414698162729663755, -0.5511811023622048555, -0.09757992244046775898 ) ) ;
#62033=CARTESIAN_POINT ( 'NONE',  ( -1.062992125984250968, 0.1771653543307087630, 0.000000000000000000 ) ) ;
#62034=CARTESIAN_POINT ( 'NONE',  ( 1.272965879265092637, -0.4281496062992127816, -0.4176697321401328100 ) ) ;
#62036=CARTESIAN_POINT ( 'NONE',  ( -0.07217847769028813698, -0.2845877964562161244, -0.3641732283464567121 ) ) ;
#62037=CARTESIAN_POINT ( 'NONE',  ( -0.1443569553805768291, 0.05413385826771666132, 0.4176697321401328100 ) ) ;
#62038=CARTESIAN_POINT ( 'NONE',  ( -1.187664041994749731, -0.2845877964562159024, 0.3641732283464567677 ) ) ;
#62039=CARTESIAN_POINT ( 'NONE',  ( -0.7283464566929126471, 0.1660481256975883668, -0.3530559997133364547 ) ) ;
#62040=CARTESIAN_POINT ( 'NONE',  ( 1.423884514435696413, -0.3162353388693409650, -0.4822834645669289433 ) ) ;
#62042=CARTESIAN_POINT ( 'NONE',  ( -0.7217847769028863381, -0.3690944881889763329, 0.3153832671262228327 ) ) ;
#62043=PLANE ( 'NONE',  #54763 ) ;
#62044=CARTESIAN_POINT ( 'NONE',  ( 1.437007874015748810, 0.1660481256975885056, 0.3530559997133364547 ) ) ;
#62046=CARTESIAN_POINT ( 'NONE',  ( -1.213910761154854745, 0.2952755905511810774, -0.1292274648535930714 ) ) ;
#62047=CARTESIAN_POINT ( 'NONE',  ( -1.200787401574802349, -0.4536011799217367080, 0.2665933059059888421 ) ) ;
#62048=CARTESIAN_POINT ( 'NONE',  ( -0.7349081364829390672, 0.1283753931104746893, -0.1820866141732285504 ) ) ;
#62050=CARTESIAN_POINT ( 'NONE',  ( -0.1312335958005241554, -0.6046776061558809534, -0.2411417322834644161 ) ) ;
#62051=CARTESIAN_POINT ( 'NONE',  ( -0.03937007874015669567, 0.1771653543307087630, 0.000000000000000000 ) ) ;
#62052=CARTESIAN_POINT ( 'NONE',  ( -1.299212598425196097, -0.5511811023622047445, 6.969142054262312111E-17 ) ) ;
#62053=CARTESIAN_POINT ( 'NONE',  ( -1.286089238845143479, -0.6046776061558807314, 0.2411417322834647770 ) ) ;
#62054=CARTESIAN_POINT ( 'NONE',  ( 1.437007874015748810, 0.07958543189024085140, 0.2665933059059887866 ) ) ;
#62055=CARTESIAN_POINT ( 'NONE',  ( 0.7677165354330716118, 0.1660481256975883668, -0.3530559997133364547 ) ) ;
#62057=CARTESIAN_POINT ( 'NONE',  ( 0.3805774278215230400, -0.3690944881889763329, 0.3153832671262228327 ) ) ;
#62058=CARTESIAN_POINT ( 'NONE',  ( 0.8070866141732289112, -0.5400638737290845981, -0.3530559997133363437 ) ) ;
#62059=CARTESIAN_POINT ( 'NONE',  ( 1.128608923884514947, 0.1283753931104748280, 0.1820866141732283561 ) ) ;
#62060=ORIENTED_EDGE ( 'NONE', *, *, #13149, .F. ) ;
#62061=CARTESIAN_POINT ( 'NONE',  ( -1.049868766404198794, -0.6046776061558807314, 0.2411417322834647770 ) ) ;
#62062=CARTESIAN_POINT ( 'NONE',  ( -0.9448818897637790704, -0.1870078740157480879, -0.4822834645669291653 ) ) ;
#62063=CARTESIAN_POINT ( 'NONE',  ( 0.01312335958005323398, 0.05413385826771666132, 0.4176697321401328100 ) ) ;
#62066=CARTESIAN_POINT ( 'NONE',  ( 0.7152230971128614723, -0.3162353388693409650, -0.4822834645669289433 ) ) ;
#62067=CARTESIAN_POINT ( 'NONE',  ( 1.377952755905512472, -0.5511811023622047445, 6.969142054262312111E-17 ) ) ;
#62068=CARTESIAN_POINT ( 'NONE',  ( 0.1771653543307093182, -0.5400638737290845981, -0.3530559997133363437 ) ) ;
#62069=CARTESIAN_POINT ( 'NONE',  ( 0.6758530183727039509, 0.2952755905511810774, -0.1292274648535930714 ) ) ;
#62076=CARTESIAN_POINT ( 'NONE',  ( -0.4986876640419942164, -0.5023911411419708095, 0.1820866141732285504 ) ) ;
#62077=CARTESIAN_POINT ( 'NONE',  ( -0.7152230971128602510, -0.05778040916215560624, -0.4822834645669293319 ) ) ;
#62078=CARTESIAN_POINT ( 'NONE',  ( 0.3805774278215230400, 0.05413385826771626580, -0.4176697321401330321 ) ) ;
#62080=CARTESIAN_POINT ( 'NONE',  ( -1.522309711286088607, -0.6046776061558807314, 0.2411417322834647770 ) ) ;
#62081=CARTESIAN_POINT ( 'NONE',  ( 1.115485564304462551, 0.05413385826771666132, 0.4176697321401328100 ) ) ;
#62084=CARTESIAN_POINT ( 'NONE',  ( 1.122047244094488860, 0.1660481256975885056, 0.3530559997133364547 ) ) ;
#62085=CARTESIAN_POINT ( 'NONE',  ( 0.8202099737532813073, 0.2952755905511811885, 0.1292274648535926551 ) ) ;
#62086=CARTESIAN_POINT ( 'NONE',  ( 0.6627296587926515548, 0.2952755905511811885, 0.1292274648535926551 ) ) ;
#62087=CARTESIAN_POINT ( 'NONE',  ( 1.259842519685040019, -0.1870078740157479769, 0.3641732283464567677 ) ) ;
#62088=CARTESIAN_POINT ( 'NONE',  ( -1.535433070866141225, -0.5511811023622047445, 6.969142054262312111E-17 ) ) ;
#62089=CARTESIAN_POINT ( 'NONE',  ( -1.646981627296586703, -0.05778040916215522460, 0.4822834645669289988 ) ) ;
#62091=CARTESIAN_POINT ( 'NONE',  ( -1.614173228346457378, 1.267785121476993293, 0.1372047244094476981 ) ) ;
#62092=CARTESIAN_POINT ( 'NONE',  ( 0.8267716535433078384, -0.6692913385826771977, 8.415575281601705876E-17 ) ) ;
#62093=FACE_OUTER_BOUND ( 'NONE', #60971, .T. ) ;
#62094=CARTESIAN_POINT ( 'NONE',  ( -0.5774278215223089816, 0.2306618581243847221, -0.2411417322834647770 ) ) ;
#62095=CARTESIAN_POINT ( 'NONE',  ( -0.6364829396325453192, -0.3162353388693405765, 0.4822834645669290543 ) ) ;
#62096=CARTESIAN_POINT ( 'NONE',  ( 1.417322834645670104, -0.1870078740157479769, 0.4822834645669291653 ) ) ;
#62098=CARTESIAN_POINT ( 'NONE',  ( 0.3543307086614179147, 0.2952755905511811885, 0.000000000000000000 ) ) ;
#62100=CARTESIAN_POINT ( 'NONE',  ( 1.568241469816273659, -0.05778040916215560624, -0.4822834645669293319 ) ) ;
#62105=CARTESIAN_POINT ( 'NONE',  ( 1.194225721784777594, -0.3690944881889765550, -0.3153832671262227771 ) ) ;
#62107=DIRECTION ( 'NONE',  ( 1.000000000000000000, -0.000000000000000000, -0.000000000000000000 ) ) ;
#62109=LINE ( 'NONE', #62523, #4678 ) ;
#62112=CARTESIAN_POINT ( 'NONE',  ( -0.3149606299212590610, -0.1870078740157480601, -0.3641732283464567677 ) ) ;
#62113=CARTESIAN_POINT ( 'NONE',  ( -1.036745406824146176, -0.004921259842519870586, -0.3153832671262229437 ) ) ;
#62114=CARTESIAN_POINT ( 'NONE',  ( -1.528871391076114250, -0.6692913385826771977, 0.1292274648535927661 ) ) ;
#62115=CARTESIAN_POINT ( 'NONE',  ( 0.6758530183727039509, 0.2952755905511810774, -0.1292274648535930714 ) ) ;
#62116=CARTESIAN_POINT ( 'NONE',  ( -1.509186351706035767, -0.4281496062992124485, 0.4176697321401328655 ) ) ;
#62119=CARTESIAN_POINT ( 'NONE',  ( 1.502624671916010790, -0.3162353388693409650, -0.4822834645669289433 ) ) ;
#62123=( BOUNDED_SURFACE ( )  B_SPLINE_SURFACE ( 1, 2, ( 
 ( #65005, #76798, #13255, #12832, #19129, #51101, #71319, #31761, #50696, #13668, #1454, #76393, #12414, #71736, #38904, #44368, #32592, #52353, #38072, #20390, #51937, #39320, #64584, #57423, #77642, #6921, #33439, #46042, #200, #83117, #26276, #25435, #44778, #70475, #58255, #6507, #38489, #14091, #39743, #19545, #26698, #58679, #7341, #25852, #620, #64173, #19974, #1044, #32177, #51512, #45203, #45625, #33009, #78060, #65439, #48128, #46875, #28358, #27946, #54020, #8181, #9423, #33847, #28775, #73825, #59513, #2698, #52774, #1867, #14916, #15333, #40998, #72981, #66678, #61171, #9015, #78899, #34688, #67501, #78482, #9836, #41809, #21220, #60351, #35507, #27111, #34268, #46462, #72569, #79313, #16163, #20806, #67092, #80148, #79731, #22048, #8596, #21632, #72156, #27529, #2284, #14511, #53184, #47708, #22468, #40164, #65848, #35092, #15755, #73404, #41408, #40576, #66257, #47292, #60759, #59928, #53605, #3110, #54437, #18225, #5172, #42639, #43451, #55672, #24108, #42225, #75064, #36737, #17412, #37154, #54858, #4751, #69149, #37565, #56501, #24521, #43862, #80563, #48954, #74236, #43042, #30836, #11500, #49777, #10258, #50187, #30425, #35928, #29600, #16997, #82203, #68336, #75884, #81797, #55261, #56092, #80971, #3523, #10675, #74655, #36331, #62838, #48536, #29191, #68738, #62413, #69563, #11080, #11911, #23284, #62006, #4342, #75477, #22874, #30009, #61595, #16580, #81381, #67920, #23695, #49368, #3941, #17818, #6824, #951, #57738, #63239, #45944, #70806, #18630, #38809, #44680, #26607, #50592, #7246, #32493, #31245, #5579, #56911, #51840, #45528, #19451, #71642, #13158, #71226, #38390, #32918, #13993, #26178, #100, #77545, #82607, #52259, #57320, #58584, #77965, #13570, #24925, #37976, #45102, #51001, #64068, #19879, #25754, #76301, #44274, #64486, #6407, #76700, #20295, #69964, #12318, #63651, #51416, #31661, #39224, #77118, #58157, #70376, #5990, #83016, #525, #25339, #19033, #12731, #32077, #64909, #65758, #2189, #1774, #8091, #40071, #60259, #20716, #39650, #2608, #73736, #48034, #59009, #60669, #27857, #65341, #21540, #41319, #1364, #9333, #40900, #28265, #59836, #7676, #66581, #79224, #80055, #35004, #72479, #33347, #15240, #22374, #27016, #52677, #33755, #78385, #14828, #66166, #72891, #53927, #15659, #46367, #21131, #54345, #53517, #8917, #47201, #73311, #72061, #34594, #79639, #14419, #3017, #28684, #59418, #27432, #53094, #78804, #21957, #67001, #47616, #46788, #40488, #8506, #34172, #48441, #42132, #29505, #44482, #55166, #18837, #12119, #67827, #69775, #10165, #51216, #80875, #3845, #23187, #50807, #55574, #48858, #9744, #38187, #12526, #42542, #76508, #25138, #37777, #74558, #36236, #80469, #81284, #70173, #16071, #61080, #35415, #29093, #35831, #61497, #63862, #6199, #16903, #17317, #68244, #42945, #22781, #82814, #74141, #31877, #57537, #16486, #74971, #41717, #10579, #61906, #4248, #29910, #23599, #49269, #67410, #63452, #5788, #31458, #83228, #3430, #25549, #54764, #57120, #26812, #33965, #1982, #737, #12946, #71018, #45740, #40278, #27645, #33550, #46579, #7463, #46162, #58374, #71436, #14624, #51628, #52052, #65961, #57948, #39440, #72277, #6617, #70592, #59212, #65555, #65128, #52470, #8297, #44893, #13783, #33133, #32708, #26394, #58803, #76912, #59627, #78600, #77757, #1573, #1161, #14208, #32288, #38604, #19242, #78178, #20508, #27227, #71858, #64282, #315, #39864, #25969, #20090, #7886, #52888, #77332, #19661, #20924, #45323, #13362, #39015, #64699, #7038, #41524, #3227, #67209, #3640, #21339, #54552, #9954, #4051, #22991, #74353, #10380, #46992, #15452, #40689, #9543, #80677, #35625, #16284, #60048, #16697, #80267, #2404, #79427, #66799, #48656, #9134, #54970, #48244, #21746, #22583, #47411, #53307, #34805, #41111, #60464, #29308, #35212, #2815, #72685, #42338, #68035, #79850, #36038, #61288, #73940, #28475, #73527, #34383, #60875, #61711, #79020, #15033, #66375, #8712, #73100, #54135, #28062, #53719, #22167, #41929, #47826, #67622, #15876, #28892, #68446, #75998, #12020, #10786, #17931, #55379, #36446, #23814 ),
 ( #43567, #24221, #63353, #69677, #43156, #57022, #69268, #5687, #81085, #17116, #4462, #49069, #68852, #36859, #75592, #37275, #50300, #62119, #75179, #31356, #42751, #56209, #11615, #81909, #24634, #23402, #62950, #30947, #29717, #74768, #30127, #55791, #49486, #49892, #11200, #18340, #81497, #17523, #62533, #5286, #4871, #30544, #37676, #56614, #82314, #43980, #35061, #23250, #16547, #47677, #74201, #73372, #55637, #3079, #9391, #60727, #55227, #61138, #28743, #15301, #42603, #16964, #48093, #80934, #29565, #42192, #80116, #41775, #2668, #3490, #48919, #21599, #66645, #40963, #34655, #41377, #15721, #74620, #68305, #67058, #22841, #22434, #48500, #28327, #3905, #53989, #10641, #36296, #79701, #80529, #47260, #22017, #54404, #9803, #35474, #67468, #29156, #72950, #54825, #73793, #67887, #61970, #8982, #4309, #29973, #16129, #10225, #60319, #35892, #61562, #17378, #75442, #50152, #44646, #6371, #37940, #50967, #11877, #50558, #62803, #75848, #18997, #56054, #56468, #70343, #62376, #43823, #76664, #11043, #75033, #63617, #69928, #69527, #56877, #64031, #4714, #18190, #12697, #37119, #5137, #37529, #32043, #38356, #82982, #30802, #5954, #63205, #18596, #43008, #31623, #12284, #5544, #82570, #81346, #30388, #31209, #23661, #82169, #24485, #24889, #49332, #68702, #25302, #76261, #57285, #44239, #36702, #81763, #24073, #49742, #17781, #43415, #69113, #11461, #14382, #8467, #27397, #78769, #14794, #25719, #19842, #45067, #71605, #1740, #40040, #20681, #64449, #21093, #58975, #6785, #486, #71188, #53057, #13530, #59382, #52645, #26141, #26980, #51802, #57702, #39186, #45491, #64870, #8059, #13958, #7210, #51379, #46752, #72445, #915, #33720, #65726, #78349, #32880, #77928, #38772, #39615, #40451, #65, #19416, #77084, #70770, #77507, #58549, #66130, #13120, #26572, #1331, #52225, #46333, #32457, #58119, #20259, #45908, #65304, #7643, #33313, #72026, #66774, #44978, #22141, #79825, #6279, #9107, #58457, #70252, #52129, #73075, #31955, #41085, #72657, #34357, #7117, #12607, #15007, #26479, #28450, #34780, #19747, #38265, #46965, #54109, #63942, #83307, #13030, #57616, #45402, #13441, #21312, #8687, #47384, #51292, #51711, #2790, #25629, #76995, #817, #38683, #79401, #78992, #32788, #77412, #19326, #70673, #40664, #64361, #6698, #60439, #71098, #2378, #32367, #66348, #58031, #394, #26052, #39097, #64779, #60023, #28035, #53693, #21720, #15424, #68828, #36015, #56183, #29691, #49460, #67185, #17500, #49044, #10762, #68010, #47799, #74741, #4027, #4846, #43130, #80652, #81886, #23376, #30521, #41500, #60849, #73916, #9515, #22965, #74326, #81060, #68422, #23789, #28865, #29282, #62508, #35188, #73503, #55354, #17089, #4437, #42726, #54946, #36422, #11175, #61686, #62095, #15851, #3616, #80242, #3201, #9928, #54527, #16256, #48631, #22558, #75155, #30103, #36835, #42312, #48220, #41903, #55765, #67597, #81472, #16673, #35599, #61262, #10355, #51092, #75567, #24197, #17908, #12824, #6498, #63740, #32584, #31753, #32168, #82695, #51504, #58247, #70467, #18718, #38481, #43544, #45194, #18315, #77208, #19537, #57824, #69243, #82291, #6079, #11997, #25014, #64165, #44360, #11591, #37251, #25427, #50687, #37651, #38896, #62926, #5260, #30924, #56590, #83108, #5666, #70897, #24610, #13247, #76789, #50277, #49867, #75975, #191, #25844, #57415, #43957, #19121, #64575, #76385, #6912, #69653, #63328, #70051, #31333, #56998, #12406, #38064, #44770, #53597, #8589, #51929, #58672, #40157, #71729, #1447, #14909, #78475, #19966, #77634, #1859, #27104, #14084, #15326, #45617, #71311, #13658, #72148, #52346, #34260, #14504, #46455, #65432, #39311, #34681, #65841, #78053, #64999, #21624, #7765, #40569, #26691, #8174, #46034, #20382, #1037, #39736, #33431, #79306, #59092, #612, #9009, #7334, #47284, #33839, #26268, #59506, #2276, #33002, #72974, #27521, #46868, #20799, #52766, #53177, #78892, #40991, #66670, #21213, #72562, #66250, #59921, #27939, #73398, #3104, #22042, #35501, #3516, #10251, #80962, #36324, #41402, #41803, #75058, #47702, #2692, #42219, #35922, #16990, #67915 ) ),
 .UNSPECIFIED., .F., .F., .F. ) 
 B_SPLINE_SURFACE_WITH_KNOTS ( ( 2, 2 ),
 ( 3, 2, 2, 2, 2, 2, 2, 2, 2, 2, 2, 2, 2, 2, 2, 2, 2, 2, 2, 2, 2, 2, 2, 2, 2, 2, 2, 2, 2, 2, 2, 2, 2, 2, 2, 2, 2, 2, 2, 2, 2, 2, 2, 2, 2, 2, 2, 2, 2, 2, 2, 2, 2, 2, 2, 2, 2, 2, 2, 2, 2, 2, 2, 2, 2, 2, 2, 2, 2, 2, 2, 2, 2, 2, 2, 2, 2, 2, 2, 2, 2, 2, 2, 2, 2, 2, 2, 2, 2, 2, 2, 2, 2, 2, 2, 2, 2, 2, 2, 2, 2, 2, 2, 2, 2, 2, 2, 2, 2, 2, 2, 2, 2, 2, 2, 2, 2, 2, 2, 2, 2, 2, 2, 2, 2, 2, 2, 2, 2, 2, 2, 2, 2, 2, 2, 2, 2, 2, 2, 2, 2, 2, 2, 2, 2, 2, 2, 2, 2, 2, 2, 2, 2, 2, 2, 2, 2, 2, 2, 2, 2, 2, 2, 2, 2, 2, 2, 2, 2, 2, 2, 2, 2, 2, 2, 2, 2, 2, 2, 2, 2, 2, 2, 2, 2, 2, 2, 2, 2, 2, 2, 2, 2, 2, 2, 2, 2, 2, 2, 2, 2, 2, 2, 2, 2, 2, 2, 2, 2, 2, 2, 2, 2, 2, 2, 2, 2, 2, 2, 2, 2, 2, 2, 2, 2, 2, 2, 2, 2, 2, 2, 2, 2, 2, 2, 2, 2, 2, 2, 2, 2, 2, 2, 2, 2, 2, 2, 2, 2, 2, 2, 2, 2, 2, 2, 3 ),
 ( 0.000000000000000000, 1.000000000000000000 ),
 ( 0.000000000000000000, 0.003787878787878787984, 0.007575757575757575968, 0.01136363636363636395, 0.01515151515151515194, 0.01893939393939393992, 0.02272727272727272790, 0.02651515151515151589, 0.03030303030303030387, 0.03409090909090908839, 0.03787878787878787984, 0.04166666666666666435, 0.04545454545454545581, 0.04924242424242424032, 0.05303030303030303177, 0.05681818181818181629, 0.06060606060606060774, 0.06439393939393939226, 0.06818181818181817677, 0.07196969696969697516, 0.07575757575757575968, 0.07954545454545454419, 0.08333333333333332871, 0.08712121212121212710, 0.09090909090909091161, 0.09469696969696969613, 0.09848484848484848064, 0.1022727272727272790, 0.1060606060606060635, 0.1098484848484848481, 0.1136363636363636326, 0.1174242424242424310, 0.1212121212121212155, 0.1250000000000000000, 0.1287878787878787845, 0.1325757575757575690, 0.1363636363636363535, 0.1401515151515151381, 0.1439393939393939503, 0.1477272727272727348, 0.1515151515151515194, 0.1553030303030303039, 0.1590909090909090884, 0.1628787878787878729, 0.1666666666666666574, 0.1704545454545454419, 0.1742424242424242542, 0.1780303030303030387, 0.1818181818181818232, 0.1856060606060606077, 0.1893939393939393923, 0.1931818181818181768, 0.1969696969696969613, 0.2007575757575757458, 0.2045454545454545581, 0.2083333333333333426, 0.2121212121212121271, 0.2159090909090909116, 0.2196969696969696961, 0.2234848484848484806, 0.2272727272727272652, 0.2310606060606060497, 0.2348484848484848619, 0.2386363636363636465, 0.2424242424242424310, 0.2462121212121212155, 0.2500000000000000000, 0.2537878787878787845, 0.2575757575757575690, 0.2613636363636363535, 0.2651515151515151381, 0.2689393939393939226, 0.2727272727272727071, 0.2765151515151514916, 0.2803030303030302761, 0.2840909090909091161, 0.2878787878787879007, 0.2916666666666666852, 0.2954545454545454697, 0.2992424242424242542, 0.3030303030303030387, 0.3068181818181818232, 0.3106060606060606077, 0.3143939393939393923, 0.3181818181818181768, 0.3219696969696969613, 0.3257575757575757458, 0.3295454545454545303, 0.3333333333333333148, 0.3371212121212120993, 0.3409090909090908839, 0.3446969696969697239, 0.3484848484848485084, 0.3522727272727272929, 0.3560606060606060774, 0.3598484848484848619, 0.3636363636363636465, 0.3674242424242424310, 0.3712121212121212155, 0.3750000000000000000, 0.3787878787878787845, 0.3825757575757575690, 0.3863636363636363535, 0.3901515151515151381, 0.3939393939393939226, 0.3977272727272727071, 0.4015151515151514916, 0.4053030303030302761, 0.4090909090909091161, 0.4128787878787879007, 0.4166666666666666852, 0.4204545454545454697, 0.4242424242424242542, 0.4280303030303030387, 0.4318181818181818232, 0.4356060606060606077, 0.4393939393939393923, 0.4431818181818181768, 0.4469696969696969613, 0.4507575757575757458, 0.4545454545454545303, 0.4583333333333333148, 0.4621212121212120993, 0.4659090909090908839, 0.4696969696969697239, 0.4734848484848485084, 0.4772727272727272929, 0.4810606060606060774, 0.4848484848484848619, 0.4886363636363636465, 0.4924242424242424310, 0.4962121212121212155, 0.5000000000000000000, 0.5037878787878787845, 0.5075757575757575690, 0.5113636363636363535, 0.5151515151515151381, 0.5189393939393939226, 0.5227272727272727071, 0.5265151515151514916, 0.5303030303030302761, 0.5340909090909090606, 0.5378787878787878451, 0.5416666666666666297, 0.5454545454545454142, 0.5492424242424241987, 0.5530303030303029832, 0.5568181818181817677, 0.5606060606060605522, 0.5643939393939394478, 0.5681818181818182323, 0.5719696969696970168, 0.5757575757575758013, 0.5795454545454545858, 0.5833333333333333703, 0.5871212121212121549, 0.5909090909090909394, 0.5946969696969697239, 0.5984848484848485084, 0.6022727272727272929, 0.6060606060606060774, 0.6098484848484848619, 0.6136363636363636465, 0.6174242424242424310, 0.6212121212121212155, 0.6250000000000000000, 0.6287878787878787845, 0.6325757575757575690, 0.6363636363636363535, 0.6401515151515151381, 0.6439393939393939226, 0.6477272727272727071, 0.6515151515151514916, 0.6553030303030302761, 0.6590909090909090606, 0.6628787878787878451, 0.6666666666666666297, 0.6704545454545454142, 0.6742424242424241987, 0.6780303030303029832, 0.6818181818181817677, 0.6856060606060605522, 0.6893939393939394478, 0.6931818181818182323, 0.6969696969696970168, 0.7007575757575758013, 0.7045454545454545858, 0.7083333333333333703, 0.7121212121212121549, 0.7159090909090909394, 0.7196969696969697239, 0.7234848484848485084, 0.7272727272727272929, 0.7310606060606060774, 0.7348484848484848619, 0.7386363636363636465, 0.7424242424242424310, 0.7462121212121212155, 0.7500000000000000000, 0.7537878787878787845, 0.7575757575757575690, 0.7613636363636363535, 0.7651515151515151381, 0.7689393939393939226, 0.7727272727272727071, 0.7765151515151514916, 0.7803030303030302761, 0.7840909090909090606, 0.7878787878787878451, 0.7916666666666666297, 0.7954545454545454142, 0.7992424242424241987, 0.8030303030303029832, 0.8068181818181817677, 0.8106060606060605522, 0.8143939393939394478, 0.8181818181818182323, 0.8219696969696970168, 0.8257575757575758013, 0.8295454545454545858, 0.8333333333333333703, 0.8371212121212121549, 0.8409090909090909394, 0.8446969696969697239, 0.8484848484848485084, 0.8522727272727272929, 0.8560606060606060774, 0.8598484848484848619, 0.8636363636363636465, 0.8674242424242424310, 0.8712121212121212155, 0.8750000000000000000, 0.8787878787878787845, 0.8825757575757575690, 0.8863636363636363535, 0.8901515151515151381, 0.8939393939393939226, 0.8977272727272727071, 0.9015151515151514916, 0.9053030303030302761, 0.9090909090909090606, 0.9128787878787878451, 0.9166666666666666297, 0.9204545454545454142, 0.9242424242424241987, 0.9280303030303029832, 0.9318181818181817677, 0.9356060606060605522, 0.9393939393939394478, 0.9431818181818182323, 0.9469696969696970168, 0.9507575757575758013, 0.9545454545454545858, 0.9583333333333333703, 0.9621212121212121549, 0.9659090909090909394 ),
 .UNSPECIFIED. ) 
 GEOMETRIC_REPRESENTATION_ITEM ( )  RATIONAL_B_SPLINE_SURFACE ( (
 ( 1.000000000000000000, 0.9659258262890683122, 1.000000000000000000, 0.9659258262890683122, 1.000000000000000000, 0.9659258262890683122, 1.000000000000000000, 0.9659258262890683122, 1.000000000000000000, 0.9659258262890683122, 1.000000000000000000, 0.9659258262890683122, 1.000000000000000000, 0.9659258262890683122, 1.000000000000000000, 0.9659258262890683122, 1.000000000000000000, 0.9659258262890683122, 1.000000000000000000, 0.9659258262890683122, 1.000000000000000000, 0.9659258262890683122, 1.000000000000000000, 0.9659258262890683122, 1.000000000000000000, 0.9659258262890683122, 1.000000000000000000, 0.9659258262890683122, 1.000000000000000000, 0.9659258262890683122, 1.000000000000000000, 0.9659258262890683122, 1.000000000000000000, 0.9659258262890683122, 1.000000000000000000, 0.9659258262890683122, 1.000000000000000000, 0.9659258262890683122, 1.000000000000000000, 0.9659258262890683122, 1.000000000000000000, 0.9659258262890683122, 1.000000000000000000, 0.9659258262890683122, 1.000000000000000000, 0.9659258262890683122, 1.000000000000000000, 0.9659258262890683122, 1.000000000000000000, 0.9659258262890683122, 1.000000000000000000, 0.9659258262890683122, 1.000000000000000000, 0.9659258262890683122, 1.000000000000000000, 0.9659258262890683122, 1.000000000000000000, 0.9659258262890683122, 1.000000000000000000, 0.9659258262890683122, 1.000000000000000000, 0.9659258262890683122, 1.000000000000000000, 0.9659258262890683122, 1.000000000000000000, 0.9659258262890683122, 1.000000000000000000, 0.9659258262890683122, 1.000000000000000000, 0.9659258262890683122, 1.000000000000000000, 0.9659258262890683122, 1.000000000000000000, 0.9659258262890683122, 1.000000000000000000, 0.9659258262890683122, 1.000000000000000000, 0.9659258262890683122, 1.000000000000000000, 0.9659258262890683122, 1.000000000000000000, 0.9659258262890683122, 1.000000000000000000, 0.9659258262890683122, 1.000000000000000000, 0.9659258262890683122, 1.000000000000000000, 0.9659258262890683122, 1.000000000000000000, 0.9659258262890683122, 1.000000000000000000, 0.9659258262890683122, 1.000000000000000000, 0.9659258262890683122, 1.000000000000000000, 0.9659258262890683122, 1.000000000000000000, 0.9659258262890683122, 1.000000000000000000, 0.9659258262890683122, 1.000000000000000000, 0.9659258262890683122, 1.000000000000000000, 0.9659258262890683122, 1.000000000000000000, 0.9659258262890683122, 1.000000000000000000, 0.9659258262890683122, 1.000000000000000000, 0.9659258262890683122, 1.000000000000000000, 0.9659258262890683122, 1.000000000000000000, 0.9659258262890683122, 1.000000000000000000, 0.9659258262890683122, 1.000000000000000000, 0.9659258262890683122, 1.000000000000000000, 0.9659258262890683122, 1.000000000000000000, 0.9659258262890683122, 1.000000000000000000, 0.9659258262890683122, 1.000000000000000000, 0.9659258262890683122, 1.000000000000000000, 0.9659258262890683122, 1.000000000000000000, 0.9659258262890683122, 1.000000000000000000, 0.9659258262890683122, 1.000000000000000000, 0.9659258262890683122, 1.000000000000000000, 0.9659258262890683122, 1.000000000000000000, 0.9659258262890683122, 1.000000000000000000, 0.9659258262890683122, 1.000000000000000000, 0.9659258262890683122, 1.000000000000000000, 0.9659258262890683122, 1.000000000000000000, 0.9659258262890683122, 1.000000000000000000, 0.9659258262890683122, 1.000000000000000000, 0.9659258262890683122, 1.000000000000000000, 0.9659258262890683122, 1.000000000000000000, 0.9659258262890683122, 1.000000000000000000, 0.9659258262890683122, 1.000000000000000000, 0.9659258262890683122, 1.000000000000000000, 0.9659258262890683122, 1.000000000000000000, 0.9659258262890683122, 1.000000000000000000, 0.9659258262890683122, 1.000000000000000000, 0.9659258262890683122, 1.000000000000000000, 0.9659258262890683122, 1.000000000000000000, 0.9659258262890683122, 1.000000000000000000, 0.9659258262890683122, 1.000000000000000000, 0.9659258262890683122, 1.000000000000000000, 0.9659258262890683122, 1.000000000000000000, 0.9659258262890683122, 1.000000000000000000, 0.9659258262890683122, 1.000000000000000000, 0.9659258262890683122, 1.000000000000000000, 0.9659258262890683122, 1.000000000000000000, 0.9659258262890683122, 1.000000000000000000, 0.9659258262890683122, 1.000000000000000000, 0.9659258262890683122, 1.000000000000000000, 0.9659258262890683122, 1.000000000000000000, 0.9659258262890683122, 1.000000000000000000, 0.9659258262890683122, 1.000000000000000000, 0.9659258262890683122, 1.000000000000000000, 0.9659258262890683122, 1.000000000000000000, 0.9659258262890683122, 1.000000000000000000, 0.9659258262890683122, 1.000000000000000000, 0.9659258262890683122, 1.000000000000000000, 0.9659258262890683122, 1.000000000000000000, 0.9659258262890683122, 1.000000000000000000, 0.9659258262890683122, 1.000000000000000000, 0.9659258262890683122, 1.000000000000000000, 0.9659258262890683122, 1.000000000000000000, 0.9659258262890683122, 1.000000000000000000, 0.9659258262890683122, 1.000000000000000000, 0.9659258262890683122, 1.000000000000000000, 0.9659258262890683122, 1.000000000000000000, 0.9659258262890683122, 1.000000000000000000, 0.9659258262890683122, 1.000000000000000000, 0.9659258262890683122, 1.000000000000000000, 0.9659258262890683122, 1.000000000000000000, 0.9659258262890683122, 1.000000000000000000, 0.9659258262890683122, 1.000000000000000000, 0.9659258262890683122, 1.000000000000000000, 0.9659258262890683122, 1.000000000000000000, 0.9659258262890683122, 1.000000000000000000, 0.9659258262890683122, 1.000000000000000000, 0.9659258262890683122, 1.000000000000000000, 0.9659258262890683122, 1.000000000000000000, 0.9659258262890683122, 1.000000000000000000, 0.9659258262890683122, 1.000000000000000000, 0.9659258262890683122, 1.000000000000000000, 0.9659258262890683122, 1.000000000000000000, 0.9659258262890683122, 1.000000000000000000, 0.9659258262890683122, 1.000000000000000000, 0.9659258262890683122, 1.000000000000000000, 0.9659258262890683122, 1.000000000000000000, 0.9659258262890683122, 1.000000000000000000, 0.9659258262890683122, 1.000000000000000000, 0.9659258262890683122, 1.000000000000000000, 0.9659258262890683122, 1.000000000000000000, 0.9659258262890683122, 1.000000000000000000, 0.9659258262890683122, 1.000000000000000000, 0.9659258262890683122, 1.000000000000000000, 0.9659258262890683122, 1.000000000000000000, 0.9659258262890683122, 1.000000000000000000, 0.9659258262890683122, 1.000000000000000000, 0.9659258262890683122, 1.000000000000000000, 0.9659258262890683122, 1.000000000000000000, 0.9659258262890683122, 1.000000000000000000, 0.9659258262890683122, 1.000000000000000000, 0.9659258262890683122, 1.000000000000000000, 0.9659258262890683122, 1.000000000000000000, 0.9659258262890683122, 1.000000000000000000, 0.9659258262890683122, 1.000000000000000000, 0.9659258262890683122, 1.000000000000000000, 0.9659258262890683122, 1.000000000000000000, 0.9659258262890683122, 1.000000000000000000, 0.9659258262890683122, 1.000000000000000000, 0.9659258262890683122, 1.000000000000000000, 0.9659258262890683122, 1.000000000000000000, 0.9659258262890683122, 1.000000000000000000, 0.9659258262890683122, 1.000000000000000000, 0.9659258262890683122, 1.000000000000000000, 0.9659258262890683122, 1.000000000000000000, 0.9659258262890683122, 1.000000000000000000, 0.9659258262890683122, 1.000000000000000000, 0.9659258262890683122, 1.000000000000000000, 0.9659258262890683122, 1.000000000000000000, 0.9659258262890683122, 1.000000000000000000, 0.9659258262890683122, 1.000000000000000000, 0.9659258262890683122, 1.000000000000000000, 0.9659258262890683122, 1.000000000000000000, 0.9659258262890683122, 1.000000000000000000, 0.9659258262890683122, 1.000000000000000000, 0.9659258262890683122, 1.000000000000000000, 0.9659258262890683122, 1.000000000000000000, 0.9659258262890683122, 1.000000000000000000, 0.9659258262890683122, 1.000000000000000000, 0.9659258262890683122, 1.000000000000000000, 0.9659258262890683122, 1.000000000000000000, 0.9659258262890683122, 1.000000000000000000, 0.9659258262890683122, 1.000000000000000000, 0.9659258262890683122, 1.000000000000000000, 0.9659258262890683122, 1.000000000000000000, 0.9659258262890683122, 1.000000000000000000, 0.9659258262890683122, 1.000000000000000000, 0.9659258262890683122, 1.000000000000000000, 0.9659258262890683122, 1.000000000000000000, 0.9659258262890683122, 1.000000000000000000, 0.9659258262890683122, 1.000000000000000000, 0.9659258262890683122, 1.000000000000000000, 0.9659258262890683122, 1.000000000000000000, 0.9659258262890683122, 1.000000000000000000, 0.9659258262890683122, 1.000000000000000000, 0.9659258262890683122, 1.000000000000000000, 0.9659258262890683122, 1.000000000000000000, 0.9659258262890683122, 1.000000000000000000, 0.9659258262890683122, 1.000000000000000000, 0.9659258262890683122, 1.000000000000000000, 0.9659258262890683122, 1.000000000000000000, 0.9659258262890683122, 1.000000000000000000, 0.9659258262890683122, 1.000000000000000000, 0.9659258262890683122, 1.000000000000000000, 0.9659258262890683122, 1.000000000000000000, 0.9659258262890683122, 1.000000000000000000, 0.9659258262890683122, 1.000000000000000000, 0.9659258262890683122, 1.000000000000000000, 0.9659258262890683122, 1.000000000000000000, 0.9659258262890683122, 1.000000000000000000, 0.9659258262890683122, 1.000000000000000000, 0.9659258262890683122, 1.000000000000000000, 0.9659258262890683122, 1.000000000000000000, 0.9659258262890683122, 1.000000000000000000, 0.9659258262890683122, 1.000000000000000000, 0.9659258262890683122, 1.000000000000000000, 0.9659258262890683122, 1.000000000000000000, 0.9659258262890683122, 1.000000000000000000, 0.9659258262890683122, 1.000000000000000000, 0.9659258262890683122, 1.000000000000000000, 0.9659258262890683122, 1.000000000000000000, 0.9659258262890683122, 1.000000000000000000, 0.9659258262890683122, 1.000000000000000000, 0.9659258262890683122, 1.000000000000000000, 0.9659258262890683122, 1.000000000000000000, 0.9659258262890683122, 1.000000000000000000, 0.9659258262890683122, 1.000000000000000000, 0.9659258262890683122, 1.000000000000000000, 0.9659258262890683122, 1.000000000000000000, 0.9659258262890683122, 1.000000000000000000, 0.9659258262890683122, 1.000000000000000000, 0.9659258262890683122, 1.000000000000000000, 0.9659258262890683122, 1.000000000000000000, 0.9659258262890683122, 1.000000000000000000, 0.9659258262890683122, 1.000000000000000000, 0.9659258262890683122, 1.000000000000000000, 0.9659258262890683122, 1.000000000000000000, 0.9659258262890683122, 1.000000000000000000, 0.9659258262890683122, 1.000000000000000000, 0.9659258262890683122, 1.000000000000000000, 0.9659258262890683122, 1.000000000000000000, 0.9659258262890683122, 1.000000000000000000, 0.9659258262890683122, 1.000000000000000000, 0.9659258262890683122, 1.000000000000000000, 0.9659258262890683122, 1.000000000000000000, 0.9659258262890683122, 1.000000000000000000, 0.9659258262890683122, 1.000000000000000000, 0.9659258262890683122, 1.000000000000000000, 0.9659258262890683122, 1.000000000000000000, 0.9659258262890683122, 1.000000000000000000, 0.9659258262890683122, 1.000000000000000000, 0.9659258262890683122, 1.000000000000000000, 0.9659258262890683122, 1.000000000000000000, 0.9659258262890683122, 1.000000000000000000, 0.9659258262890683122, 1.000000000000000000, 0.9659258262890683122, 1.000000000000000000, 0.9659258262890683122, 1.000000000000000000, 0.9659258262890683122, 1.000000000000000000, 0.9659258262890683122, 1.000000000000000000, 0.9659258262890683122, 1.000000000000000000),
 ( 1.000000000000000000, 0.9659258262890683122, 1.000000000000000000, 0.9659258262890683122, 1.000000000000000000, 0.9659258262890683122, 1.000000000000000000, 0.9659258262890683122, 1.000000000000000000, 0.9659258262890683122, 1.000000000000000000, 0.9659258262890683122, 1.000000000000000000, 0.9659258262890683122, 1.000000000000000000, 0.9659258262890683122, 1.000000000000000000, 0.9659258262890683122, 1.000000000000000000, 0.9659258262890683122, 1.000000000000000000, 0.9659258262890683122, 1.000000000000000000, 0.9659258262890683122, 1.000000000000000000, 0.9659258262890683122, 1.000000000000000000, 0.9659258262890683122, 1.000000000000000000, 0.9659258262890683122, 1.000000000000000000, 0.9659258262890683122, 1.000000000000000000, 0.9659258262890683122, 1.000000000000000000, 0.9659258262890683122, 1.000000000000000000, 0.9659258262890683122, 1.000000000000000000, 0.9659258262890683122, 1.000000000000000000, 0.9659258262890683122, 1.000000000000000000, 0.9659258262890683122, 1.000000000000000000, 0.9659258262890683122, 1.000000000000000000, 0.9659258262890683122, 1.000000000000000000, 0.9659258262890683122, 1.000000000000000000, 0.9659258262890683122, 1.000000000000000000, 0.9659258262890683122, 1.000000000000000000, 0.9659258262890683122, 1.000000000000000000, 0.9659258262890683122, 1.000000000000000000, 0.9659258262890683122, 1.000000000000000000, 0.9659258262890683122, 1.000000000000000000, 0.9659258262890683122, 1.000000000000000000, 0.9659258262890683122, 1.000000000000000000, 0.9659258262890683122, 1.000000000000000000, 0.9659258262890683122, 1.000000000000000000, 0.9659258262890683122, 1.000000000000000000, 0.9659258262890683122, 1.000000000000000000, 0.9659258262890683122, 1.000000000000000000, 0.9659258262890683122, 1.000000000000000000, 0.9659258262890683122, 1.000000000000000000, 0.9659258262890683122, 1.000000000000000000, 0.9659258262890683122, 1.000000000000000000, 0.9659258262890683122, 1.000000000000000000, 0.9659258262890683122, 1.000000000000000000, 0.9659258262890683122, 1.000000000000000000, 0.9659258262890683122, 1.000000000000000000, 0.9659258262890683122, 1.000000000000000000, 0.9659258262890683122, 1.000000000000000000, 0.9659258262890683122, 1.000000000000000000, 0.9659258262890683122, 1.000000000000000000, 0.9659258262890683122, 1.000000000000000000, 0.9659258262890683122, 1.000000000000000000, 0.9659258262890683122, 1.000000000000000000, 0.9659258262890683122, 1.000000000000000000, 0.9659258262890683122, 1.000000000000000000, 0.9659258262890683122, 1.000000000000000000, 0.9659258262890683122, 1.000000000000000000, 0.9659258262890683122, 1.000000000000000000, 0.9659258262890683122, 1.000000000000000000, 0.9659258262890683122, 1.000000000000000000, 0.9659258262890683122, 1.000000000000000000, 0.9659258262890683122, 1.000000000000000000, 0.9659258262890683122, 1.000000000000000000, 0.9659258262890683122, 1.000000000000000000, 0.9659258262890683122, 1.000000000000000000, 0.9659258262890683122, 1.000000000000000000, 0.9659258262890683122, 1.000000000000000000, 0.9659258262890683122, 1.000000000000000000, 0.9659258262890683122, 1.000000000000000000, 0.9659258262890683122, 1.000000000000000000, 0.9659258262890683122, 1.000000000000000000, 0.9659258262890683122, 1.000000000000000000, 0.9659258262890683122, 1.000000000000000000, 0.9659258262890683122, 1.000000000000000000, 0.9659258262890683122, 1.000000000000000000, 0.9659258262890683122, 1.000000000000000000, 0.9659258262890683122, 1.000000000000000000, 0.9659258262890683122, 1.000000000000000000, 0.9659258262890683122, 1.000000000000000000, 0.9659258262890683122, 1.000000000000000000, 0.9659258262890683122, 1.000000000000000000, 0.9659258262890683122, 1.000000000000000000, 0.9659258262890683122, 1.000000000000000000, 0.9659258262890683122, 1.000000000000000000, 0.9659258262890683122, 1.000000000000000000, 0.9659258262890683122, 1.000000000000000000, 0.9659258262890683122, 1.000000000000000000, 0.9659258262890683122, 1.000000000000000000, 0.9659258262890683122, 1.000000000000000000, 0.9659258262890683122, 1.000000000000000000, 0.9659258262890683122, 1.000000000000000000, 0.9659258262890683122, 1.000000000000000000, 0.9659258262890683122, 1.000000000000000000, 0.9659258262890683122, 1.000000000000000000, 0.9659258262890683122, 1.000000000000000000, 0.9659258262890683122, 1.000000000000000000, 0.9659258262890683122, 1.000000000000000000, 0.9659258262890683122, 1.000000000000000000, 0.9659258262890683122, 1.000000000000000000, 0.9659258262890683122, 1.000000000000000000, 0.9659258262890683122, 1.000000000000000000, 0.9659258262890683122, 1.000000000000000000, 0.9659258262890683122, 1.000000000000000000, 0.9659258262890683122, 1.000000000000000000, 0.9659258262890683122, 1.000000000000000000, 0.9659258262890683122, 1.000000000000000000, 0.9659258262890683122, 1.000000000000000000, 0.9659258262890683122, 1.000000000000000000, 0.9659258262890683122, 1.000000000000000000, 0.9659258262890683122, 1.000000000000000000, 0.9659258262890683122, 1.000000000000000000, 0.9659258262890683122, 1.000000000000000000, 0.9659258262890683122, 1.000000000000000000, 0.9659258262890683122, 1.000000000000000000, 0.9659258262890683122, 1.000000000000000000, 0.9659258262890683122, 1.000000000000000000, 0.9659258262890683122, 1.000000000000000000, 0.9659258262890683122, 1.000000000000000000, 0.9659258262890683122, 1.000000000000000000, 0.9659258262890683122, 1.000000000000000000, 0.9659258262890683122, 1.000000000000000000, 0.9659258262890683122, 1.000000000000000000, 0.9659258262890683122, 1.000000000000000000, 0.9659258262890683122, 1.000000000000000000, 0.9659258262890683122, 1.000000000000000000, 0.9659258262890683122, 1.000000000000000000, 0.9659258262890683122, 1.000000000000000000, 0.9659258262890683122, 1.000000000000000000, 0.9659258262890683122, 1.000000000000000000, 0.9659258262890683122, 1.000000000000000000, 0.9659258262890683122, 1.000000000000000000, 0.9659258262890683122, 1.000000000000000000, 0.9659258262890683122, 1.000000000000000000, 0.9659258262890683122, 1.000000000000000000, 0.9659258262890683122, 1.000000000000000000, 0.9659258262890683122, 1.000000000000000000, 0.9659258262890683122, 1.000000000000000000, 0.9659258262890683122, 1.000000000000000000, 0.9659258262890683122, 1.000000000000000000, 0.9659258262890683122, 1.000000000000000000, 0.9659258262890683122, 1.000000000000000000, 0.9659258262890683122, 1.000000000000000000, 0.9659258262890683122, 1.000000000000000000, 0.9659258262890683122, 1.000000000000000000, 0.9659258262890683122, 1.000000000000000000, 0.9659258262890683122, 1.000000000000000000, 0.9659258262890683122, 1.000000000000000000, 0.9659258262890683122, 1.000000000000000000, 0.9659258262890683122, 1.000000000000000000, 0.9659258262890683122, 1.000000000000000000, 0.9659258262890683122, 1.000000000000000000, 0.9659258262890683122, 1.000000000000000000, 0.9659258262890683122, 1.000000000000000000, 0.9659258262890683122, 1.000000000000000000, 0.9659258262890683122, 1.000000000000000000, 0.9659258262890683122, 1.000000000000000000, 0.9659258262890683122, 1.000000000000000000, 0.9659258262890683122, 1.000000000000000000, 0.9659258262890683122, 1.000000000000000000, 0.9659258262890683122, 1.000000000000000000, 0.9659258262890683122, 1.000000000000000000, 0.9659258262890683122, 1.000000000000000000, 0.9659258262890683122, 1.000000000000000000, 0.9659258262890683122, 1.000000000000000000, 0.9659258262890683122, 1.000000000000000000, 0.9659258262890683122, 1.000000000000000000, 0.9659258262890683122, 1.000000000000000000, 0.9659258262890683122, 1.000000000000000000, 0.9659258262890683122, 1.000000000000000000, 0.9659258262890683122, 1.000000000000000000, 0.9659258262890683122, 1.000000000000000000, 0.9659258262890683122, 1.000000000000000000, 0.9659258262890683122, 1.000000000000000000, 0.9659258262890683122, 1.000000000000000000, 0.9659258262890683122, 1.000000000000000000, 0.9659258262890683122, 1.000000000000000000, 0.9659258262890683122, 1.000000000000000000, 0.9659258262890683122, 1.000000000000000000, 0.9659258262890683122, 1.000000000000000000, 0.9659258262890683122, 1.000000000000000000, 0.9659258262890683122, 1.000000000000000000, 0.9659258262890683122, 1.000000000000000000, 0.9659258262890683122, 1.000000000000000000, 0.9659258262890683122, 1.000000000000000000, 0.9659258262890683122, 1.000000000000000000, 0.9659258262890683122, 1.000000000000000000, 0.9659258262890683122, 1.000000000000000000, 0.9659258262890683122, 1.000000000000000000, 0.9659258262890683122, 1.000000000000000000, 0.9659258262890683122, 1.000000000000000000, 0.9659258262890683122, 1.000000000000000000, 0.9659258262890683122, 1.000000000000000000, 0.9659258262890683122, 1.000000000000000000, 0.9659258262890683122, 1.000000000000000000, 0.9659258262890683122, 1.000000000000000000, 0.9659258262890683122, 1.000000000000000000, 0.9659258262890683122, 1.000000000000000000, 0.9659258262890683122, 1.000000000000000000, 0.9659258262890683122, 1.000000000000000000, 0.9659258262890683122, 1.000000000000000000, 0.9659258262890683122, 1.000000000000000000, 0.9659258262890683122, 1.000000000000000000, 0.9659258262890683122, 1.000000000000000000, 0.9659258262890683122, 1.000000000000000000, 0.9659258262890683122, 1.000000000000000000, 0.9659258262890683122, 1.000000000000000000, 0.9659258262890683122, 1.000000000000000000, 0.9659258262890683122, 1.000000000000000000, 0.9659258262890683122, 1.000000000000000000, 0.9659258262890683122, 1.000000000000000000, 0.9659258262890683122, 1.000000000000000000, 0.9659258262890683122, 1.000000000000000000, 0.9659258262890683122, 1.000000000000000000, 0.9659258262890683122, 1.000000000000000000, 0.9659258262890683122, 1.000000000000000000, 0.9659258262890683122, 1.000000000000000000, 0.9659258262890683122, 1.000000000000000000, 0.9659258262890683122, 1.000000000000000000, 0.9659258262890683122, 1.000000000000000000, 0.9659258262890683122, 1.000000000000000000, 0.9659258262890683122, 1.000000000000000000, 0.9659258262890683122, 1.000000000000000000, 0.9659258262890683122, 1.000000000000000000, 0.9659258262890683122, 1.000000000000000000, 0.9659258262890683122, 1.000000000000000000, 0.9659258262890683122, 1.000000000000000000, 0.9659258262890683122, 1.000000000000000000, 0.9659258262890683122, 1.000000000000000000, 0.9659258262890683122, 1.000000000000000000, 0.9659258262890683122, 1.000000000000000000, 0.9659258262890683122, 1.000000000000000000, 0.9659258262890683122, 1.000000000000000000, 0.9659258262890683122, 1.000000000000000000, 0.9659258262890683122, 1.000000000000000000, 0.9659258262890683122, 1.000000000000000000, 0.9659258262890683122, 1.000000000000000000, 0.9659258262890683122, 1.000000000000000000, 0.9659258262890683122, 1.000000000000000000, 0.9659258262890683122, 1.000000000000000000, 0.9659258262890683122, 1.000000000000000000, 0.9659258262890683122, 1.000000000000000000, 0.9659258262890683122, 1.000000000000000000, 0.9659258262890683122, 1.000000000000000000, 0.9659258262890683122, 1.000000000000000000, 0.9659258262890683122, 1.000000000000000000, 0.9659258262890683122, 1.000000000000000000, 0.9659258262890683122, 1.000000000000000000, 0.9659258262890683122, 1.000000000000000000, 0.9659258262890683122, 1.000000000000000000, 0.9659258262890683122, 1.000000000000000000, 0.9659258262890683122, 1.000000000000000000, 0.9659258262890683122, 1.000000000000000000, 0.9659258262890683122, 1.000000000000000000, 0.9659258262890683122, 1.000000000000000000, 0.9659258262890683122, 1.000000000000000000) ) ) 
 REPRESENTATION_ITEM ( '' )  SURFACE ( )  );
#62124=CARTESIAN_POINT ( 'NONE',  ( 1.614173228346456712, 0.000000000000000000, 0.5309055118110233007 ) ) ;
#62125=CARTESIAN_POINT ( 'NONE',  ( -0.8333333333333323711, 0.2952755905511811885, 0.1292274648535926551 ) ) ;
#62126=CARTESIAN_POINT ( 'NONE',  ( 1.358267716535433323, 0.1660481256975885056, 0.3530559997133364547 ) ) ;
#62127=DIRECTION ( 'NONE',  ( 1.000000000000000000, 0.000000000000000000, 0.000000000000000000 ) ) ;
#62128=CARTESIAN_POINT ( 'NONE',  ( -1.011202504342156416, -2.294479370626195693E-15, 0.3464511005275217603 ) ) ;
#62129=CARTESIAN_POINT ( 'NONE',  ( 1.450131233595801428, -0.6692913385826773087, -0.1292274648535924053 ) ) ;
#62130=CARTESIAN_POINT ( 'NONE',  ( -0.8727034120734901146, -0.05778040916215560624, -0.4822834645669293319 ) ) ;
#62132=CARTESIAN_POINT ( 'NONE',  ( 0.07217847769028949700, -0.08942795157528024563, -0.3641732283464568787 ) ) ;
#62134=CARTESIAN_POINT ( 'NONE',  ( -0.1640419947506553400, -0.08942795157528024563, -0.3641732283464568787 ) ) ;
#62135=CARTESIAN_POINT ( 'NONE',  ( 0.5249343832021003964, 0.1283753931104746893, -0.1820866141732285504 ) ) ;
#62136=CARTESIAN_POINT ( 'NONE',  ( 0.6102362204724416372, -0.5400638737290844871, 0.3530559997133364547 ) ) ;
#62138=CARTESIAN_POINT ( 'NONE',  ( -0.8792650918635160906, -0.3690944881889763329, 0.3153832671262228327 ) ) ;
#62140=CARTESIAN_POINT ( 'NONE',  ( 1.430446194225722500, 0.05413385826771666132, 0.4176697321401328100 ) ) ;
#62141=CARTESIAN_POINT ( 'NONE',  ( -0.8727034120734901146, -0.3162353388693405765, 0.4822834645669290543 ) ) ;
#62143=CARTESIAN_POINT ( 'NONE',  ( -0.1181102362204717315, 0.2952755905511811885, 0.000000000000000000 ) ) ;
#62144=CARTESIAN_POINT ( 'NONE',  ( -0.6758530183727028406, 0.2952755905511811885, 0.1292274648535926551 ) ) ;
#62145=CARTESIAN_POINT ( 'NONE',  ( 1.305774278215223960, -0.5511811023622046335, 0.09757992244046803654 ) ) ;
#62146=CARTESIAN_POINT ( 'NONE',  ( 0.1968503937007881344, 0.1771653543307087630, 0.000000000000000000 ) ) ;
#62147=CARTESIAN_POINT ( 'NONE',  ( -0.3608923884514428360, -0.6692913385826773087, -0.1292274648535924053 ) ) ;
#62148=CARTESIAN_POINT ( 'NONE',  ( -0.6627296587926501115, 0.2952755905511810774, -0.1292274648535930714 ) ) ;
#62150=CARTESIAN_POINT ( 'NONE',  ( 1.548556430446194954, 0.1283753931104746893, -0.1820866141732285504 ) ) ;
#62151=CARTESIAN_POINT ( 'NONE',  ( 0.1443569553805781891, 0.05413385826771626580, -0.4176697321401330321 ) ) ;
#62155=CARTESIAN_POINT ( 'NONE',  ( 1.089238845144357537, -0.4281496062992124485, 0.4176697321401328655 ) ) ;
#62156=CARTESIAN_POINT ( 'NONE',  ( -0.5511811023622041894, -0.1870078740157480601, -0.3641732283464567677 ) ) ;
#62157=CARTESIAN_POINT ( 'NONE',  ( -0.6824146981627291497, -0.6046776061558809534, -0.2411417322834644161 ) ) ;
#62158=CARTESIAN_POINT ( 'NONE',  ( 1.364829396325460076, 0.2306618581243848609, 0.2411417322834645549 ) ) ;
#62159=CARTESIAN_POINT ( 'NONE',  ( 0.7939632545931766261, -0.3162353388693409650, -0.4822834645669289433 ) ) ;
#62160=CARTESIAN_POINT ( 'NONE',  ( 1.220472440944879056, 0.8346805926620878280, 0.5309055118110235227 ) ) ;
#62161=CARTESIAN_POINT ( 'NONE',  ( -1.135170603674539924, -0.5511811023622046335, 0.09757992244046803654 ) ) ;
#62163=EDGE_CURVE ( 'NONE', #49328, #47474, #36607, .T. ) ;
#62166=CARTESIAN_POINT ( 'NONE',  ( 1.450131233595801428, -0.5511811023622048555, -0.09757992244046775898 ) ) ;
#62167=CARTESIAN_POINT ( 'NONE',  ( 0.5643044619422579178, -0.3690944881889765550, -0.3153832671262227771 ) ) ;
#62168=CARTESIAN_POINT ( 'NONE',  ( 0.5577427821522314977, -0.3162353388693409650, -0.4822834645669289433 ) ) ;
#62171=CARTESIAN_POINT ( 'NONE',  ( 0.8923884514435703741, 0.1283753931104748280, 0.1820866141732283561 ) ) ;
#62172=CARTESIAN_POINT ( 'NONE',  ( -0.1902887139107604098, 0.2952755905511810774, -0.1292274648535930714 ) ) ;
#62173=CARTESIAN_POINT ( 'NONE',  ( -0.8858267716535425107, -0.5400638737290844871, 0.3530559997133364547 ) ) ;
#62174=CARTESIAN_POINT ( 'NONE',  ( 1.141732283464567788, -0.6692913385826771977, 8.415575281601705876E-17 ) ) ;
#62175=B_SPLINE_CURVE_WITH_KNOTS ( 'NONE', 3,
 ( #46256, #19762, #77008, #58044 ),
 .UNSPECIFIED., .F., .F.,
 ( 4, 4 ),
 ( 3.210432057752138185E-07, 0.001287787053612062362 ),
 .UNSPECIFIED. ) ;
#62178=CARTESIAN_POINT ( 'NONE',  ( 0.05249343832021075018, 0.1283753931104746893, -0.1820866141732285504 ) ) ;
#62181=VERTEX_POINT ( 'NONE', #68610 ) ;
#62183=CARTESIAN_POINT ( 'NONE',  ( -0.7349081364829390672, 0.2306618581243847221, -0.2411417322834647770 ) ) ;
#62184=CARTESIAN_POINT ( 'NONE',  ( -0.1443569553805765515, -0.4281496062992127816, -0.4176697321401328100 ) ) ;
#62185=CARTESIAN_POINT ( 'NONE',  ( -0.4461942257217840213, -0.6046776061558809534, -0.2411417322834644161 ) ) ;
#62186=CARTESIAN_POINT ( 'NONE',  ( 0.3937007874015754361, -0.1870078740157479769, 0.4822834645669291653 ) ) ;
#62187=CARTESIAN_POINT ( 'NONE',  ( -0.2821522309711278487, -0.6692913385826773087, -0.1292274648535924053 ) ) ;
#62188=CARTESIAN_POINT ( 'NONE',  ( -1.423884514435694859, -0.05778040916215560624, -0.4822834645669293319 ) ) ;
#62189=CARTESIAN_POINT ( 'NONE',  ( -0.9580052493438311334, -0.4281496062992124485, 0.4176697321401328655 ) ) ;
#62190=CARTESIAN_POINT ( 'NONE',  ( 0.8530183727034126306, 0.05413385826771626580, -0.4176697321401330321 ) ) ;
#62191=CARTESIAN_POINT ( 'NONE',  ( 0.6167979002624678353, -0.4281496062992124485, 0.4176697321401328655 ) ) ;
#62193=CARTESIAN_POINT ( 'NONE',  ( -0.2690288713910754526, -0.5511811023622046335, 0.09757992244046803654 ) ) ;
#62194=EDGE_LOOP ( 'NONE', ( #2799, #69330, #20922, #27802 ) ) ;
#62197=CARTESIAN_POINT ( 'NONE',  ( -1.292650918635170010, -0.5511811023622046335, 0.09757992244046803654 ) ) ;
#62198=CARTESIAN_POINT ( 'NONE',  ( -0.3805774278215216522, 0.05413385826771666132, 0.4176697321401328100 ) ) ;
#62199=CARTESIAN_POINT ( 'NONE',  ( 0.7763038905084337360, 2.575861430505332611E-15, -0.3954974714151464621 ) ) ;
#62200=CARTESIAN_POINT ( 'NONE',  ( -0.7677165354330699465, 0.1660481256975885056, 0.3530559997133364547 ) ) ;
#62201=CARTESIAN_POINT ( 'NONE',  ( -0.7874015748031489847, -0.1870078740157479769, 0.4822834645669291653 ) ) ;
#62202=CARTESIAN_POINT ( 'NONE',  ( -1.502624671916009680, -0.3162353388693405765, 0.4822834645669290543 ) ) ;
#62204=CARTESIAN_POINT ( 'NONE',  ( 1.122047244094488860, -0.4536011799217368745, -0.2665933059059886201 ) ) ;
#62207=CARTESIAN_POINT ( 'NONE',  ( -0.07217847769028813698, -0.2845877964562161244, -0.3641732283464567121 ) ) ;
#62208=CARTESIAN_POINT ( 'NONE',  ( -0.5183727034120726440, 0.2952755905511811885, 0.1292274648535926551 ) ) ;
#62210=CARTESIAN_POINT ( 'NONE',  ( -0.1115485564304453947, -0.6692913385826771977, 0.1292274648535927661 ) ) ;
#62211=ORIENTED_EDGE ( 'NONE', *, *, #53641, .T. ) ;
#62213=CARTESIAN_POINT ( 'NONE',  ( 0.2473181295769235899, 2.056812631849083806E-16, 0.3954985857520053605 ) ) ;
#62214=ORIENTED_EDGE ( 'NONE', *, *, #52674, .T. ) ;
#62217=CARTESIAN_POINT ( 'NONE',  ( -0.7349081364829390672, 0.1283753931104746893, -0.1820866141732285504 ) ) ;
#62218=CARTESIAN_POINT ( 'NONE',  ( -1.174540682414697335, -0.3162353388693409650, -0.4822834645669289433 ) ) ;
#62220=CARTESIAN_POINT ( 'NONE',  ( -0.7233831536535466622, 2.176714048050540473, 0.5048085489443566720 ) ) ;
#62222=CARTESIAN_POINT ( 'NONE',  ( 1.279527559055118724, -0.5400638737290845981, -0.3530559997133363437 ) ) ;
#62223=CARTESIAN_POINT ( 'NONE',  ( 0.4068241469816279987, -0.4281496062992127816, -0.4176697321401328100 ) ) ;
#62224=CARTESIAN_POINT ( 'NONE',  ( 0.5708661417322842269, 0.1660481256975885056, 0.3530559997133364547 ) ) ;
#62225=CARTESIAN_POINT ( 'NONE',  ( -0.5511811023622038563, -0.1870078740157479769, 0.3641732283464567677 ) ) ;
#62226=CARTESIAN_POINT ( 'NONE',  ( -0.4396325459317579898, 0.2952755905511811885, 0.1292274648535926551 ) ) ;
#62228=CARTESIAN_POINT ( 'NONE',  ( -1.010498687664041384, -0.4281496062992127816, -0.4176697321401328100 ) ) ;
#62230=CARTESIAN_POINT ( 'NONE',  ( 1.437007874015748810, 0.07958543189024085140, 0.2665933059059887866 ) ) ;
#62231=CARTESIAN_POINT ( 'NONE',  ( -0.3937007874015740483, -0.1870078740157480601, -0.3641732283464567677 ) ) ;
#62233=CARTESIAN_POINT ( 'NONE',  ( 1.286089238845145033, -0.5023911411419708095, -0.1820866141732282451 ) ) ;
#62234=CARTESIAN_POINT ( 'NONE',  ( 1.607611548556431069, 0.1771653543307087630, 0.09757992244046791164 ) ) ;
#62235=CARTESIAN_POINT ( 'NONE',  ( -1.122047244094487306, 0.07958543189024071263, -0.2665933059059888421 ) ) ;
#62236=CARTESIAN_POINT ( 'NONE',  ( 1.594488188976378673, 0.1660481256975885056, 0.3530559997133364547 ) ) ;
#62237=CARTESIAN_POINT ( 'NONE',  ( -1.332020997375327642, -0.3162353388693409650, -0.4822834645669289433 ) ) ;
#62238=CARTESIAN_POINT ( 'NONE',  ( -0.2427821522309703550, -0.3162353388693405765, 0.4822834645669290543 ) ) ;
#62240=CARTESIAN_POINT ( 'NONE',  ( -0.2493438320209966919, -0.3690944881889763329, 0.3153832671262228327 ) ) ;
#62241=CARTESIAN_POINT ( 'NONE',  ( -1.509186351706035767, -0.004921259842519870586, -0.3153832671262229437 ) ) ;
#62242=CARTESIAN_POINT ( 'NONE',  ( 0.8858267716535438430, 0.1660481256975885056, 0.3530559997133364547 ) ) ;
#62243=CARTESIAN_POINT ( 'NONE',  ( -1.476377952755905110, -0.4536011799217368745, -0.2665933059059886201 ) ) ;
#62244=CONICAL_SURFACE ( 'NONE', #19208, 1.181102362204724310, 0.7853981633974621568 ) ;
#62245=CARTESIAN_POINT ( 'NONE',  ( 1.220472440944882386, -0.5511811023622047445, 6.969142054262312111E-17 ) ) ;
#62246=CARTESIAN_POINT ( 'NONE',  ( -0.9120734908136475250, 0.2952755905511811885, 0.1292274648535926551 ) ) ;
#62247=CARTESIAN_POINT ( 'NONE',  ( -0.3674540682414689785, 0.1283753931104748280, 0.1820866141732283561 ) ) ;
#62249=CARTESIAN_POINT ( 'NONE',  ( 0.09842519685039434474, -0.4536011799217368745, -0.2665933059059886201 ) ) ;
#62250=CARTESIAN_POINT ( 'NONE',  ( -0.2821522309711278487, -0.6692913385826773087, -0.1292274648535924053 ) ) ;
#62252=EDGE_CURVE ( 'NONE', #38980, #55534, #12805, .T. ) ;
#62254=CARTESIAN_POINT ( 'NONE',  ( 0.4921259842519691285, 0.07958543189024085140, 0.2665933059059887866 ) ) ;
#62255=CARTESIAN_POINT ( 'NONE',  ( -0.2230971128608915943, 0.05413385826771666132, 0.4176697321401328100 ) ) ;
#62256=CARTESIAN_POINT ( 'NONE',  ( -0.5905511811023613777, -0.6692913385826771977, 8.415575281601705876E-17 ) ) ;
#62257=CARTESIAN_POINT ( 'NONE',  ( -0.8530183727034112984, -0.004921259842519576551, 0.3153832671262227771 ) ) ;
#62259=CARTESIAN_POINT ( 'NONE',  ( -0.5971128608923877978, -0.5511811023622048555, -0.09757992244046775898 ) ) ;
#62260=CARTESIAN_POINT ( 'NONE',  ( -0.1377952755905504645, -0.5400638737290845981, -0.3530559997133363437 ) ) ;
#62261=CARTESIAN_POINT ( 'NONE',  ( -1.089238845144356427, -0.004921259842519576551, 0.3153832671262227771 ) ) ;
#62262=CARTESIAN_POINT ( 'NONE',  ( -1.482939632545930975, 0.05413385826771666132, 0.4176697321401328100 ) ) ;
#62263=CARTESIAN_POINT ( 'NONE',  ( 0.4613432605871740089, 1.990046790791744833E-15, -0.3954974714151458515 ) ) ;
#62264=ORIENTED_EDGE ( 'NONE', *, *, #47242, .T. ) ;
#62265=CARTESIAN_POINT ( 'NONE',  ( -1.522309711286088607, 0.1283753931104746893, -0.1820866141732285504 ) ) ;
#62266=CARTESIAN_POINT ( 'NONE',  ( -0.4133858267716528645, 0.1660481256975883668, -0.3530559997133364547 ) ) ;
#62267=CARTESIAN_POINT ( 'NONE',  ( -1.010498687664041384, 0.05413385826771666132, 0.4176697321401328100 ) ) ;
#62270=CARTESIAN_POINT ( 'NONE',  ( 0.9580052493438327987, -0.4281496062992127816, -0.4176697321401328100 ) ) ;
#62271=CARTESIAN_POINT ( 'NONE',  ( 0.5183727034120741983, -0.6692913385826771977, 0.1292274648535927661 ) ) ;
#62274=CARTESIAN_POINT ( 'NONE',  ( 0.9842519685039375910, 0.1771653543307087630, 0.000000000000000000 ) ) ;
#62277=CARTESIAN_POINT ( 'NONE',  ( -0.8136482939632537770, 0.1283753931104746893, -0.1820866141732285504 ) ) ;
#62279=ORIENTED_EDGE ( 'NONE', *, *, #12089, .F. ) ;
#62280=CARTESIAN_POINT ( 'NONE',  ( 0.4002624671916016896, -0.3162353388693409650, -0.4822834645669289433 ) ) ;
#62281=CARTESIAN_POINT ( 'NONE',  ( -0.3149606299212590610, -0.1870078740157479769, 0.4822834645669291653 ) ) ;
#62282=CARTESIAN_POINT ( 'NONE',  ( -1.259842519685038686, -0.1870078740157480879, -0.4822834645669291653 ) ) ;
#62283=CARTESIAN_POINT ( 'NONE',  ( 0.9251968503937015864, 0.1660481256975883668, -0.3530559997133364547 ) ) ;
#62285=CARTESIAN_POINT ( 'NONE',  ( -1.456692913385826182, 0.1771653543307087630, 0.000000000000000000 ) ) ;
#62287=CARTESIAN_POINT ( 'NONE',  ( -0.09842519685039295696, -0.5400638737290844871, 0.3530559997133364547 ) ) ;
#62288=CARTESIAN_POINT ( 'NONE',  ( -1.305774278215222184, 0.2952755905511811885, 0.1292274648535926551 ) ) ;
#62291=CARTESIAN_POINT ( 'NONE',  ( 1.572991167713778227, 1.535433070866141447, -0.1227090857360983167 ) ) ;
#62293=CARTESIAN_POINT ( 'NONE',  ( 0.7874015748031503170, -0.1870078740157480601, -0.3641732283464567677 ) ) ;
#62296=CARTESIAN_POINT ( 'NONE',  ( -1.017060367454067249, -0.05778040916215522460, 0.4822834645669289988 ) ) ;
#62297=ORIENTED_EDGE ( 'NONE', *, *, #80383, .T. ) ;
#62298=CARTESIAN_POINT ( 'NONE',  ( -0.006561679790025524116, -0.2845877964562159024, 0.3641732283464567677 ) ) ;
#62299=CARTESIAN_POINT ( 'NONE',  ( -1.463254593175852492, -0.6692913385826773087, -0.1292274648535924053 ) ) ;
#62300=CARTESIAN_POINT ( 'NONE',  ( 0.3937007874015754361, -0.1870078740157480879, -0.4822834645669291653 ) ) ;
#62301=CARTESIAN_POINT ( 'NONE',  ( 0.6233595800524939223, -0.3162353388693405765, 0.4822834645669290543 ) ) ;
#62302=CARTESIAN_POINT ( 'NONE',  ( -0.6036745406824141069, 0.2306618581243848609, 0.2411417322834645549 ) ) ;
#62304=CARTESIAN_POINT ( 'NONE',  ( -0.6496062992125976043, 0.1660481256975883668, -0.3530559997133364547 ) ) ;
#62306=CARTESIAN_POINT ( 'NONE',  ( 1.305774278215223960, 0.1771653543307087075, -0.09757992244046823083 ) ) ;
#62307=CARTESIAN_POINT ( 'NONE',  ( -0.8530183727034112984, 0.05413385826771666132, 0.4176697321401328100 ) ) ;
#62308=CARTESIAN_POINT ( 'NONE',  ( 0.9317585301837276734, 0.05413385826771626580, -0.4176697321401330321 ) ) ;
#62309=CARTESIAN_POINT ( 'NONE',  ( 1.227034120734908917, 0.2952755905511810774, -0.1292274648535930714 ) ) ;
#62311=CARTESIAN_POINT ( 'NONE',  ( -1.417322834645668772, -0.1870078740157479769, 0.4822834645669291653 ) ) ;
#62313=CARTESIAN_POINT ( 'NONE',  ( 0.3215223097112867578, -0.05778040916215522460, 0.4822834645669289988 ) ) ;
#62315=CARTESIAN_POINT ( 'NONE',  ( -1.574803149606298192, -0.1870078740157480601, -0.3641732283464567677 ) ) ;
#62316=CARTESIAN_POINT ( 'NONE',  ( 0.6627296587926517768, -0.5511811023622048555, -0.09757992244046775898 ) ) ;
#62317=CARTESIAN_POINT ( 'NONE',  ( 0.7874015748031503170, -0.1870078740157479769, 0.4822834645669291653 ) ) ;
#62319=CARTESIAN_POINT ( 'NONE',  ( 0.7545931758530189937, 0.1771653543307087075, -0.09757992244046823083 ) ) ;
#62320=CARTESIAN_POINT ( 'NONE',  ( 0.8989501312335963501, -0.6692913385826773087, -0.1292274648535924053 ) ) ;
#62322=CARTESIAN_POINT ( 'NONE',  ( -0.8595800524934373854, -0.3162353388693409650, -0.4822834645669289433 ) ) ;
#62324=CARTESIAN_POINT ( 'NONE',  ( 1.043307086614173818, -0.4536011799217368745, -0.2665933059059886201 ) ) ;
#62325=CARTESIAN_POINT ( 'NONE',  ( -0.4724409448818890911, -0.1870078740157479769, 0.4822834645669291653 ) ) ;
#62326=CARTESIAN_POINT ( 'NONE',  ( -0.05249343832020938322, -0.6046776061558809534, -0.2411417322834644161 ) ) ;
#62328=CARTESIAN_POINT ( 'NONE',  ( -0.4855643044619415427, -0.4281496062992124485, 0.4176697321401328655 ) ) ;
#62329=CARTESIAN_POINT ( 'NONE',  ( 0.2755905511811031494, 0.1771653543307087630, 0.000000000000000000 ) ) ;
#62331=CARTESIAN_POINT ( 'NONE',  ( 0.1837270341207357105, -0.5023911411419708095, -0.1820866141732282451 ) ) ;
#62332=CARTESIAN_POINT ( 'NONE',  ( 0.9186351706036751663, -0.5023911411419708095, 0.1820866141732285504 ) ) ;
#62335=CARTESIAN_POINT ( 'NONE',  ( 0.3543307086614181922, -0.6692913385826771977, 8.415575281601705876E-17 ) ) ;
#62337=CARTESIAN_POINT ( 'NONE',  ( 0.2238009295390077091, 2.409604939980833412E-17, -0.3464511005275205946 ) ) ;
#62338=CARTESIAN_POINT ( 'NONE',  ( 0.2230971128608929543, 0.05413385826771626580, -0.4176697321401330321 ) ) ;
#62339=CARTESIAN_POINT ( 'NONE',  ( -0.2296587926509179312, -0.2845877964562161244, -0.3641732283464567121 ) ) ;
#62340=CARTESIAN_POINT ( 'NONE',  ( -0.1443569553805768291, -0.004921259842519576551, 0.3153832671262227771 ) ) ;
#62341=CARTESIAN_POINT ( 'NONE',  ( -0.3346456692913377662, 0.1660481256975883668, -0.3530559997133364547 ) ) ;
#62342=CARTESIAN_POINT ( 'NONE',  ( 0.8989501312335964611, 0.1771653543307087630, 0.09757992244046791164 ) ) ;
#62343=CARTESIAN_POINT ( 'NONE',  ( -1.660104986876639543, -0.08942795157528024563, -0.3641732283464568787 ) ) ;
#62344=CARTESIAN_POINT ( 'NONE',  ( 1.305774278215223960, 0.1771653543307087075, -0.09757992244046823083 ) ) ;
#62346=CARTESIAN_POINT ( 'NONE',  ( 0.2099737532808405305, -0.6046776061558807314, 0.2411417322834647770 ) ) ;
#62347=CARTESIAN_POINT ( 'NONE',  ( 1.154855643044620184, -0.6046776061558807314, 0.2411417322834647770 ) ) ;
#62349=CARTESIAN_POINT ( 'NONE',  ( 0.02624671916010564918, 0.2306618581243848609, 0.2411417322834645549 ) ) ;
#62350=CARTESIAN_POINT ( 'NONE',  ( 1.286089238845145033, -0.6046776061558809534, -0.2411417322834644161 ) ) ;
#62351=CARTESIAN_POINT ( 'NONE',  ( 0.5971128608923891301, 0.2952755905511810774, -0.1292274648535930714 ) ) ;
#62353=CARTESIAN_POINT ( 'NONE',  ( 0.7808398950131241190, -0.08942795157528024563, -0.3641732283464568787 ) ) ;
#62354=CARTESIAN_POINT ( 'NONE',  ( 1.122047244094488860, -0.5400638737290845981, -0.3530559997133363437 ) ) ;
#62355=CARTESIAN_POINT ( 'NONE',  ( 5.463695987328526437E-16, -0.1870078740157479769, 0.3641732283464567677 ) ) ;
#62357=CARTESIAN_POINT ( 'NONE',  ( -0.1837270341207340729, 0.2306618581243847221, -0.2411417322834647770 ) ) ;
#62358=CARTESIAN_POINT ( 'NONE',  ( 0.3608923884514443348, 0.2952755905511810774, -0.1292274648535930714 ) ) ;
#62359=CARTESIAN_POINT ( 'NONE',  ( -0.7020997375328074108, -0.05778040916215522460, 0.4822834645669289988 ) ) ;
#62360=CARTESIAN_POINT ( 'NONE',  ( -0.3805774278215216522, -0.3690944881889765550, -0.3153832671262227771 ) ) ;
#62361=CARTESIAN_POINT ( 'NONE',  ( 0.7152230971128614723, -0.3162353388693409650, -0.4822834645669289433 ) ) ;
#62362=CARTESIAN_POINT ( 'NONE',  ( 0.9776902887139113929, -0.5511811023622048555, -0.09757992244046775898 ) ) ;
#62363=CARTESIAN_POINT ( 'NONE',  ( 0.2624671916010504757, 0.2306618581243848609, 0.2411417322834645549 ) ) ;
#62365=CARTESIAN_POINT ( 'NONE',  ( -1.033630966599879297, -2.567464376874931580E-15, -0.4445507791589072832 ) ) ;
#62367=CARTESIAN_POINT ( 'NONE',  ( 1.528871391076116026, 0.2952755905511811885, 0.1292274648535926551 ) ) ;
#62369=CARTESIAN_POINT ( 'NONE',  ( -1.200787401574802349, -0.5400638737290844871, 0.3530559997133364547 ) ) ;
#62370=CARTESIAN_POINT ( 'NONE',  ( -0.4986876640419942164, -0.6046776061558807314, 0.2411417322834647770 ) ) ;
#62373=EDGE_LOOP ( 'NONE', ( #27548, #24229, #2697, #23339 ) ) ;
#62374=CARTESIAN_POINT ( 'NONE',  ( 0.1902887139107617975, -0.5511811023622048555, -0.09757992244046775898 ) ) ;
#62376=CARTESIAN_POINT ( 'NONE',  ( 0.7939632545931766261, -0.05778040916215522460, 0.4822834645669289988 ) ) ;
#62380=CARTESIAN_POINT ( 'NONE',  ( 1.049868766404200349, 0.2306618581243848609, 0.2411417322834645549 ) ) ;
#62382=CARTESIAN_POINT ( 'NONE',  ( 1.240157480314961314, -0.4536011799217367080, 0.2665933059059888421 ) ) ;
#62383=CARTESIAN_POINT ( 'NONE',  ( -0.01312335958005186876, 0.05413385826771626580, -0.4176697321401330321 ) ) ;
#62385=CARTESIAN_POINT ( 'NONE',  ( -0.2821522309711278487, -0.6692913385826773087, -0.1292274648535924053 ) ) ;
#62386=CARTESIAN_POINT ( 'NONE',  ( -1.108923884514435132, -0.2845877964562159024, 0.3641732283464567677 ) ) ;
#62387=CARTESIAN_POINT ( 'NONE',  ( 0.5577427821522314977, -0.3162353388693409650, -0.4822834645669289433 ) ) ;
#62388=CARTESIAN_POINT ( 'NONE',  ( -0.6627296587926503335, -0.6692913385826771977, 0.1292274648535927661 ) ) ;
#62394=CARTESIAN_POINT ( 'NONE',  ( 0.3871391076115493490, -0.3162353388693405765, 0.4822834645669290543 ) ) ;
#62395=CARTESIAN_POINT ( 'NONE',  ( -0.3149606299212590610, -0.1870078740157479769, 0.4822834645669291653 ) ) ;
#62396=CARTESIAN_POINT ( 'NONE',  ( -1.450131233595799651, 0.2952755905511810774, -0.1292274648535930714 ) ) ;
#62397=CARTESIAN_POINT ( 'NONE',  ( 0.9251968503937015864, -0.5400638737290844871, 0.3530559997133364547 ) ) ;
#62398=CARTESIAN_POINT ( 'NONE',  ( 0.6233595800524942554, -0.05778040916215560624, -0.4822834645669293319 ) ) ;
#62400=CARTESIAN_POINT ( 'NONE',  ( -0.9580052493438311334, -0.4281496062992124485, 0.4176697321401328655 ) ) ;
#62401=CARTESIAN_POINT ( 'NONE',  ( 0.2952755905511819101, 0.1660481256975883668, -0.3530559997133364547 ) ) ;
#62402=CARTESIAN_POINT ( 'NONE',  ( -0.3280839895013117347, 0.05413385826771626580, -0.4176697321401330321 ) ) ;
#62403=CARTESIAN_POINT ( 'NONE',  ( 0.2230971128608932319, -0.3690944881889763329, 0.3153832671262228327 ) ) ;
#62404=CARTESIAN_POINT ( 'NONE',  ( 1.692913385826772421, 0.1771653543307087630, 0.000000000000000000 ) ) ;
#62406=CARTESIAN_POINT ( 'NONE',  ( 0.4396325459317590445, -0.6692913385826771977, 0.1292274648535927661 ) ) ;
#62407=DIRECTION ( 'NONE',  ( -0.000000000000000000, 1.000000000000000000, -0.000000000000000000 ) ) ;
#62408=CARTESIAN_POINT ( 'NONE',  ( 1.410761154855643795, -0.3162353388693405765, 0.4822834645669290543 ) ) ;
#62413=CARTESIAN_POINT ( 'NONE',  ( 0.6102362204724416372, 0.1660481256975883668, -0.3530559997133364547 ) ) ;
#62414=CARTESIAN_POINT ( 'NONE',  ( 0.2559055118110243332, -0.4536011799217368745, -0.2665933059059886201 ) ) ;
#62422=CARTESIAN_POINT ( 'NONE',  ( 0.4855643044619428750, 0.05413385826771666132, 0.4176697321401328100 ) ) ;
#62423=CARTESIAN_POINT ( 'NONE',  ( -1.253280839895012377, -0.3162353388693409650, -0.4822834645669289433 ) ) ;
#62424=CARTESIAN_POINT ( 'NONE',  ( -1.049868766404198794, 0.2306618581243847221, -0.2411417322834647770 ) ) ;
#62425=CARTESIAN_POINT ( 'NONE',  ( 0.5577427821522314977, -0.3162353388693409650, -0.4822834645669289433 ) ) ;
#62426=CARTESIAN_POINT ( 'NONE',  ( 1.325459317585302665, 0.05413385826771626580, -0.4176697321401330321 ) ) ;
#62427=CARTESIAN_POINT ( 'NONE',  ( 1.410761154855643795, -0.08942795157528024563, -0.3641732283464568787 ) ) ;
#62428=CARTESIAN_POINT ( 'NONE',  ( 1.082677165354331228, 0.07958543189024071263, -0.2665933059059888421 ) ) ;
#62429=CARTESIAN_POINT ( 'NONE',  ( -0.6627296587926501115, 0.2952755905511810774, -0.1292274648535930714 ) ) ;
#62431=CARTESIAN_POINT ( 'NONE',  ( 1.410761154855643795, -0.05778040916215560624, -0.4822834645669293319 ) ) ;
#62434=CARTESIAN_POINT ( 'NONE',  ( -0.4199475065616791736, -0.6046776061558807314, 0.2411417322834647770 ) ) ;
#62435=CARTESIAN_POINT ( 'NONE',  ( 0.9711286089238851948, -0.6046776061558809534, -0.2411417322834644161 ) ) ;
#62436=CARTESIAN_POINT ( 'NONE',  ( -0.7137454485294953965, 2.793565526369265584, 0.4917280318828574082 ) ) ;
#62437=CARTESIAN_POINT ( 'NONE',  ( -1.010498687664041384, -0.3690944881889765550, -0.3153832671262227771 ) ) ;
#62438=CARTESIAN_POINT ( 'NONE',  ( 0.4002624671916016896, -0.05778040916215522460, 0.4822834645669289988 ) ) ;
#62439=CARTESIAN_POINT ( 'NONE',  ( 0.9055118110236227702, -0.5511811023622047445, 6.969142054262312111E-17 ) ) ;
#62442=CARTESIAN_POINT ( 'NONE',  ( -1.410761154855642463, -0.08942795157527998196, 0.3641732283464567121 ) ) ;
#62443=CARTESIAN_POINT ( 'NONE',  ( 0.8398950131233602345, -0.6046776061558807314, 0.2411417322834647770 ) ) ;
#62445=CARTESIAN_POINT ( 'NONE',  ( -0.5052493438320203589, -0.5511811023622046335, 0.09757992244046803654 ) ) ;
#62446=CARTESIAN_POINT ( 'NONE',  ( -0.2296587926509179312, -0.3162353388693409650, -0.4822834645669289433 ) ) ;
#62447=CARTESIAN_POINT ( 'NONE',  ( -1.181102362204723644, -0.1870078740157479769, 0.3641732283464567677 ) ) ;
#62448=CARTESIAN_POINT ( 'NONE',  ( -0.5708661417322828946, 0.1660481256975883668, -0.3530559997133364547 ) ) ;
#62449=CARTESIAN_POINT ( 'NONE',  ( 1.213910761154856299, 0.2952755905511811885, 0.1292274648535926551 ) ) ;
#62451=CARTESIAN_POINT ( 'NONE',  ( -0.8595800524934373854, -0.08942795157527998196, 0.3641732283464567121 ) ) ;
#62453=CARTESIAN_POINT ( 'NONE',  ( 1.358267716535433323, -0.5400638737290845981, -0.3530559997133363437 ) ) ;
#62455=CARTESIAN_POINT ( 'NONE',  ( -1.371391076115484831, 0.2952755905511810774, -0.1292274648535930714 ) ) ;
#62456=CARTESIAN_POINT ( 'NONE',  ( -1.482939632545930975, -0.004921259842519576551, 0.3153832671262227771 ) ) ;
#62458=CARTESIAN_POINT ( 'NONE',  ( -0.5708661417322828946, 0.07958543189024071263, -0.2665933059059888421 ) ) ;
#62459=CARTESIAN_POINT ( 'NONE',  ( 0.7993346172249373716, 1.763362281772084768E-16, 0.3627985898453514602 ) ) ;
#62460=CARTESIAN_POINT ( 'NONE',  ( -0.3805774278215216522, 0.05413385826771666132, 0.4176697321401328100 ) ) ;
#62461=CARTESIAN_POINT ( 'NONE',  ( 0.03280839895013198948, -0.5511811023622048555, -0.09757992244046775898 ) ) ;
#62462=CARTESIAN_POINT ( 'NONE',  ( -1.003937007874015297, -0.4536011799217368745, -0.2665933059059886201 ) ) ;
#62463=CARTESIAN_POINT ( 'NONE',  ( -1.509186351706035767, 0.05413385826771626580, -0.4176697321401330321 ) ) ;
#62464=CARTESIAN_POINT ( 'NONE',  ( 1.423884514435696191, -0.08942795157527998196, 0.3641732283464567121 ) ) ;
#62465=CARTESIAN_POINT ( 'NONE',  ( 1.023622047244095334, -0.1870078740157479769, 0.4822834645669291653 ) ) ;
#62467=CARTESIAN_POINT ( 'NONE',  ( 0.3543307086614181922, -0.5511811023622047445, 6.969142054262312111E-17 ) ) ;
#62468=CARTESIAN_POINT ( 'NONE',  ( 0.1968503937007881344, 0.2952755905511811885, 0.000000000000000000 ) ) ;
#62469=CARTESIAN_POINT ( 'NONE',  ( 1.003937007874016407, -0.5400638737290844871, 0.3530559997133364547 ) ) ;
#62470=CARTESIAN_POINT ( 'NONE',  ( 0.8595800524934390507, -0.08942795157528024563, -0.3641732283464568787 ) ) ;
#62472=CARTESIAN_POINT ( 'NONE',  ( -1.194225721784776262, -0.4281496062992124485, 0.4176697321401328655 ) ) ;
#62474=CARTESIAN_POINT ( 'NONE',  ( -0.7677165354330699465, -0.5400638737290845981, -0.3530559997133363437 ) ) ;
#62475=CARTESIAN_POINT ( 'NONE',  ( -0.1312335958005241554, 0.2306618581243848609, 0.2411417322834645549 ) ) ;
#62478=CARTESIAN_POINT ( 'NONE',  ( 0.2493438320209980519, -0.4281496062992127816, -0.4176697321401328100 ) ) ;
#62479=CARTESIAN_POINT ( 'NONE',  ( 1.561679790026247350, -0.3690944881889763329, 0.3153832671262228327 ) ) ;
#62480=CARTESIAN_POINT ( 'NONE',  ( -0.08530183727034056085, -0.3162353388693405765, 0.4822834645669290543 ) ) ;
#62481=CARTESIAN_POINT ( 'NONE',  ( 0.8727034120734912248, -0.3162353388693409650, -0.4822834645669289433 ) ) ;
#62488=CARTESIAN_POINT ( 'NONE',  ( -0.6561679790026240244, -0.5023911411419708095, 0.1820866141732285504 ) ) ;
#62489=CARTESIAN_POINT ( 'NONE',  ( -0.8070866141732276899, -0.5400638737290844871, 0.3530559997133364547 ) ) ;
#62490=CARTESIAN_POINT ( 'NONE',  ( 0.3674540682414705883, 0.2306618581243847221, -0.2411417322834647770 ) ) ;
#62492=CARTESIAN_POINT ( 'NONE',  ( 0.9055118110236227702, 0.2952755905511811885, 0.000000000000000000 ) ) ;
#62493=CARTESIAN_POINT ( 'NONE',  ( -1.627296587926508442, 0.2306618581243848609, 0.2411417322834645549 ) ) ;
#62494=CARTESIAN_POINT ( 'NONE',  ( 1.286089238845145033, 0.2306618581243848609, 0.2411417322834645549 ) ) ;
#62497=CARTESIAN_POINT ( 'NONE',  ( -1.646051170424378096, -0.1870078740157480046, 1.254653134982923898E-17 ) ) ;
#62498=CARTESIAN_POINT ( 'NONE',  ( 0.8989501312335963501, -0.6692913385826773087, -0.1292274648535924053 ) ) ;
#62499=CARTESIAN_POINT ( 'NONE',  ( 0.4724409448818904789, -0.1870078740157479769, 0.4822834645669291653 ) ) ;
#62500=CARTESIAN_POINT ( 'NONE',  ( 1.345144356955381593, -0.2845877964562161244, -0.3641732283464567121 ) ) ;
#62501=CARTESIAN_POINT ( 'NONE',  ( -1.601049868766403650, 0.1283753931104746893, -0.1820866141732285504 ) ) ;
#62502=CARTESIAN_POINT ( 'NONE',  ( -1.437007874015747477, 0.1660481256975883668, -0.3530559997133364547 ) ) ;
#62504=CARTESIAN_POINT ( 'NONE',  ( -1.586052503253847501, 1.299212598425198095, 0.1653254495020568260 ) ) ;
#62505=CARTESIAN_POINT ( 'NONE',  ( 0.6889763779527566800, -0.5400638737290844871, 0.3530559997133364547 ) ) ;
#62506=CARTESIAN_POINT ( 'NONE',  ( 1.555118110236221041, 0.07958543189024071263, -0.2665933059059888421 ) ) ;
#62507=CARTESIAN_POINT ( 'NONE',  ( -0.3871391076115479057, -0.3162353388693409650, -0.4822834645669289433 ) ) ;
#62508=CARTESIAN_POINT ( 'NONE',  ( -0.5643044619422565855, 0.05413385826771626580, -0.4176697321401330321 ) ) ;
#62509=CARTESIAN_POINT ( 'NONE',  ( 1.391076115485564868, -0.6046776061558807314, 0.2411417322834647770 ) ) ;
#62513=CARTESIAN_POINT ( 'NONE',  ( 1.601049868766404982, -0.6046776061558809534, -0.2411417322834644161 ) ) ;
#62516=VERTEX_POINT ( 'NONE', #69436 ) ;
#62517=LINE ( 'NONE', #16682, #26043 ) ;
#62518=CARTESIAN_POINT ( 'NONE',  ( 1.581364829396326277, -0.08942795157527998196, 0.3641732283464567121 ) ) ;
#62520=CARTESIAN_POINT ( 'NONE',  ( 0.5618802787717186442, 7.570362723507360306E-16, 0.4118484887281971263 ) ) ;
#62521=CARTESIAN_POINT ( 'NONE',  ( -0.09186351706036689768, 0.009842519685039144428, -0.3409548833797004797 ) ) ;
#62522=B_SPLINE_CURVE_WITH_KNOTS ( 'NONE', 3,
 ( #69074, #57240, #57662, #18957, #12244, #18556, #56017 ),
 .UNSPECIFIED., .F., .F.,
 ( 4, 3, 4 ),
 ( 1.910166083080835130E-17, 0.001246230184515546152, 0.002492489877932653301 ),
 .UNSPECIFIED. ) ;
#62523=CARTESIAN_POINT ( 'NONE',  ( -1.220472440944878834, 2.401574803149606474, -0.5309055118110234117 ) ) ;
#62526=CARTESIAN_POINT ( 'NONE',  ( -0.8661417322834640276, -0.1870078740157479769, 0.3641732283464567677 ) ) ;
#62527=CARTESIAN_POINT ( 'NONE',  ( -1.220472440944881054, 0.1771653543307087630, 0.000000000000000000 ) ) ;
#62528=CARTESIAN_POINT ( 'NONE',  ( -0.06561679790026180015, -0.4281496062992127816, -0.4176697321401328100 ) ) ;
#62529=CARTESIAN_POINT ( 'NONE',  ( 0.6364829396325465405, -0.05778040916215522460, 0.4822834645669289988 ) ) ;
#62530=CARTESIAN_POINT ( 'NONE',  ( -1.213910761154854745, -0.6692913385826771977, 0.1292274648535927661 ) ) ;
#62533=CARTESIAN_POINT ( 'NONE',  ( 1.364829396325459854, -0.6046776061558809534, -0.2411417322834644161 ) ) ;
#62537=CARTESIAN_POINT ( 'NONE',  ( -0.01241954290193713825, 2.784432375088962958E-17, -0.3464511005275205946 ) ) ;
#62538=CARTESIAN_POINT ( 'NONE',  ( -0.3412073490813641308, 0.1283753931104746893, -0.1820866141732285504 ) ) ;
#62540=CARTESIAN_POINT ( 'NONE',  ( -1.266404199475064773, -0.05778040916215560624, -0.4822834645669293319 ) ) ;
#62541=CARTESIAN_POINT ( 'NONE',  ( 1.174540682414699111, -0.3162353388693405765, 0.4822834645669290543 ) ) ;
#62544=CARTESIAN_POINT ( 'NONE',  ( 0.6692913385826777528, 0.2066929133858268208, 0.000000000000000000 ) ) ;
#62545=EDGE_CURVE ( 'NONE', #74234, #1651, #37476, .T. ) ;
#62546=CARTESIAN_POINT ( 'NONE',  ( 1.686351706036745890, 0.2952755905511811885, 0.1292274648535926551 ) ) ;
#62547=CARTESIAN_POINT ( 'NONE',  ( -1.279527559055116948, -0.5400638737290844871, 0.3530559997133364547 ) ) ;
#62550=CARTESIAN_POINT ( 'NONE',  ( -0.07217847769028813698, -0.2845877964562161244, -0.3641732283464567121 ) ) ;
#62553=CARTESIAN_POINT ( 'NONE',  ( -0.1574803149606292529, -0.1870078740157480601, -0.3641732283464567677 ) ) ;
#62554=CARTESIAN_POINT ( 'NONE',  ( 0.6496062992125991586, 0.07958543189024085140, 0.2665933059059887866 ) ) ;
#62555=CARTESIAN_POINT ( 'NONE',  ( 0.6036745406824153282, -0.6046776061558807314, 0.2411417322834647770 ) ) ;
#62556=CARTESIAN_POINT ( 'NONE',  ( -0.9055118110236215490, -0.5511811023622047445, 6.969142054262312111E-17 ) ) ;
#62558=CARTESIAN_POINT ( 'NONE',  ( 1.417322834645670104, -0.1870078740157479769, 0.4822834645669291653 ) ) ;
#62559=CARTESIAN_POINT ( 'NONE',  ( -1.082677165354329896, -0.5400638737290845981, -0.3530559997133363437 ) ) ;
#62561=CARTESIAN_POINT ( 'NONE',  ( 0.1837270341207354329, 0.2306618581243848609, 0.2411417322834645549 ) ) ;
#62562=CARTESIAN_POINT ( 'NONE',  ( -0.6692913385826764205, 0.2952755905511811885, 0.000000000000000000 ) ) ;
#62563=CARTESIAN_POINT ( 'NONE',  ( 1.286089238845145033, -0.5023911411419708095, -0.1820866141732282451 ) ) ;
#62564=CARTESIAN_POINT ( 'NONE',  ( 0.05249343832021075018, 0.1283753931104746893, -0.1820866141732285504 ) ) ;
#62565=CARTESIAN_POINT ( 'NONE',  ( -0.1312335958005241554, 0.2306618581243848609, 0.2411417322834645549 ) ) ;
#62566=CARTESIAN_POINT ( 'NONE',  ( -1.043307086614172041, -0.5400638737290844871, 0.3530559997133364547 ) ) ;
#62567=DIRECTION ( 'NONE',  ( 0.000000000000000000, -1.000000000000000000, 0.000000000000000000 ) ) ;
#62568=CARTESIAN_POINT ( 'NONE',  ( 1.594488188976378673, -0.4536011799217368745, -0.2665933059059886201 ) ) ;
#62569=CARTESIAN_POINT ( 'NONE',  ( -0.1115485564304453947, -0.6692913385826771977, 0.1292274648535927661 ) ) ;
#62572=CARTESIAN_POINT ( 'NONE',  ( 1.017060367454068581, -0.05778040916215560624, -0.4822834645669293319 ) ) ;
#62573=CARTESIAN_POINT ( 'NONE',  ( -0.8070866141732276899, -0.4536011799217367080, 0.2665933059059888421 ) ) ;
#62574=CARTESIAN_POINT ( 'NONE',  ( -0.6758530183727028406, -0.6692913385826773087, -0.1292274648535924053 ) ) ;
#62575=CARTESIAN_POINT ( 'NONE',  ( 1.266404199475066328, -0.3162353388693409650, -0.4822834645669289433 ) ) ;
#62576=CARTESIAN_POINT ( 'NONE',  ( 0.7086614173228353852, -0.1870078740157479769, 0.4822834645669291653 ) ) ;
#62578=CARTESIAN_POINT ( 'NONE',  ( -1.187664041994750175, -0.08942795157528024563, -0.3641732283464568787 ) ) ;
#62583=CARTESIAN_POINT ( 'NONE',  ( 1.561679790026247350, -0.004921259842519870586, -0.3153832671262229437 ) ) ;
#62584=CARTESIAN_POINT ( 'NONE',  ( 0.6561679790026253567, 0.1283753931104748280, 0.1820866141732283561 ) ) ;
#62585=CARTESIAN_POINT ( 'NONE',  ( 0.4199475065616803948, -0.6046776061558809534, -0.2411417322834644161 ) ) ;
#62588=CARTESIAN_POINT ( 'NONE',  ( 0.8595800524934390507, -0.2845877964562159024, 0.3641732283464567677 ) ) ;
#62589=CARTESIAN_POINT ( 'NONE',  ( -0.4002624671916004129, -0.3162353388693405765, 0.4822834645669290543 ) ) ;
#62590=CARTESIAN_POINT ( 'NONE',  ( -0.7414698162729651543, -0.6692913385826771977, 0.1292274648535927661 ) ) ;
#62591=CARTESIAN_POINT ( 'NONE',  ( 1.102362204724410155, -0.1870078740157480879, -0.4822834645669291653 ) ) ;
#62595=CARTESIAN_POINT ( 'NONE',  ( -0.2362204724409442680, -0.1870078740157480601, -0.3641732283464567677 ) ) ;
#62599=CARTESIAN_POINT ( 'NONE',  ( -0.9317585301837263412, 0.05413385826771666132, 0.4176697321401328100 ) ) ;
#62600=CARTESIAN_POINT ( 'NONE',  ( -0.2690288713910754526, -0.6692913385826771977, 0.1292274648535927661 ) ) ;
#62601=CARTESIAN_POINT ( 'NONE',  ( -0.4986876640419939388, 0.2306618581243847221, -0.2411417322834647770 ) ) ;
#62603=CARTESIAN_POINT ( 'NONE',  ( 0.4921259842519691285, -0.5400638737290845981, -0.3530559997133363437 ) ) ;
#62604=CARTESIAN_POINT ( 'NONE',  ( -0.4527559055118102749, -0.5400638737290845981, -0.3530559997133363437 ) ) ;
#62605=CARTESIAN_POINT ( 'NONE',  ( -1.364829396325458521, -0.6046776061558807314, 0.2411417322834647770 ) ) ;
#62606=CARTESIAN_POINT ( 'NONE',  ( -0.6299212598425188991, -0.1870078740157479769, 0.4822834645669291653 ) ) ;
#62607=CARTESIAN_POINT ( 'NONE',  ( 0.9580052493438326877, 0.05413385826771666132, 0.4176697321401328100 ) ) ;
#62608=( BOUNDED_SURFACE ( )  B_SPLINE_SURFACE ( 1, 2, ( 
 ( #69300, #24252, #10815, #11231, #50333, #55410, #4491, #12053, #81116, #36892, #37710, #42370, #16729, #37307, #17961, #62568, #75623, #63383, #68069, #43598, #62981, #36475, #62150, #5320, #29339, #56645, #23433, #49098, #74802, #30159, #26323, #44413, #77264, #38949, #19593, #39369, #57055, #6968, #45670, #39792, #58730, #26744, #46093, #82747, #51148, #76441, #45255, #33060, #71366, #51984, #12459, #52399, #32639, #38120, #31808, #19176, #1093, #44824, #7392, #668, #57468, #58302, #77689, #70107, #12878, #76842, #70522, #65054, #70952, #78108, #13297, #83162, #57881, #32223, #20439, #13715, #20019, #64218, #25900, #63795, #64632, #71785, #5719, #50743, #25069, #18770, #25481, #38537, #14140, #31389, #6552, #6133, #248, #51560, #46508, #47758, #72208, #67141, #28824, #14561, #41043, #7819, #40213, #53236, #53653, #79361, #27993, #21680, #16214, #47341, #33895, #73031, #22517, #33486, #48178, #80199, #59561, #15381, #73874, #65487, #72618, #1505, #1916, #34317, #54488, #59148, #22097, #35144, #66728, #9065, #28408, #2337, #27157, #34737, #60397, #52821, #60806, #14966, #78531, #2748, #20856, #65895, #8231, #27579, #78952, #40623, #8645, #54066, #79782, #41457, #21270, #46925, #66306, #59978, #73456, #15806, #9470, #3160, #49422, #37205, #10312, #35977, #81023, #43092, #50238, #23335, #74286, #67553, #42690, #75528, #75934, #49005, #56552, #43502, #68789, #62886, #36383, #41861, #24572, #75117, #80612, #17462, #74704, #5221, #29242, #69200, #11134, #9888, #35557, #61221, #30479, #24160, #81434, #3575, #36791, #49828, #17049, #11549, #54906, #4802, #62057, #56143, #22923, #17868, #62467, #29652, #48589, #30885, #16630, #42272, #23749, #68387, #67969, #4395, #82253, #61647, #3988, #81848, #10726, #55314, #30063, #55724, #69613, #37614, #6459, #70013, #27369, #33286, #64123, #83068, #56960, #53454, #1305, #12368, #63289, #40423, #25389, #33694, #44323, #58947, #63702, #38027, #18678, #40014, #82657, #18275, #65701, #43916, #27794, #5629, #66104, #26954, #11959, #52617, #21068, #31296, #72418, #78323, #53030, #76753, #46726, #24972, #8031, #12784, #59355, #50644, #1714, #20654, #6041, #76348, #78743, #31713, #57373, #46307, #51052, #19083, #72001, #14767, #44732, #70428, #14357, #38441, #8440, #34110, #59771, #2126, #15178, #67351, #47555, #3783, #9684, #41660, #60608, #34531, #29851, #61017, #73247, #40835, #16842, #2957, #10102, #21891, #35355, #41256, #15596, #79575, #16425, #60195, #79162, #42071, #21479, #4188, #66520, #42476, #3368, #47137, #29032, #80814, #8852, #48797, #80409, #67766, #16014, #72828, #22721, #54703, #36174, #74495, #28622, #2546, #48380, #61847, #28204, #53863, #66942, #9274, #54280, #22310, #74079, #35766, #55105, #34945, #79996, #10520, #47973, #73672, #61436, #29446, #23129, #68181, #50850, #23952, #49620, #11338, #56754, #63906, #36998, #4593, #81222, #56348, #5829, #6242, #62677, #70215, #57162, #82454, #76550, #50032, #55514, #38229, #63087, #10921, #31087, #5019, #18878, #42885, #82861, #24769, #23538, #49207, #74911, #44122, #37819, #11761, #17257, #31502, #68580, #36578, #62257, #30264, #75314, #81644, #25183, #44527, #17661, #50438, #82049, #76139, #55928, #63495, #43292, #12571, #68989, #30687, #18480, #24362, #75729, #18069, #43704, #69407, #37415, #5425, #69814, #12163, #359, #13829, #72322, #57580, #14668, #46626, #26016, #65175, #40326, #66004, #39062, #51257, #51674, #781, #78644, #31919, #71902, #1615, #45783, #1206, #13407, #26442, #52932, #6661, #7083, #20967, #12992, #77803, #27271, #44938, #25594, #14254, #20556, #20135, #7512, #83271, #76959, #52095, #71482, #71063, #64745, #39488, #19287, #33180, #58849, #70636, #38648, #26856, #52515, #64325, #78223, #46208, #39912, #65600, #32333, #7932, #33593, #57995, #77378, #19709, #45368, #32754, #58421, #59258, #22209, #35664, #48281, #54598, #15076, #29347, #9584, #40734, #34430, #21789, #61328, #47451, #9999, #3268, #60095, #35253, #28929, #47036, #15495, #79473, #73146, #41969, #47866, #3682, #22622, #2857, #27692, #59671, #60917, #34846, #41153, #23029, #2026 ),
 ( #66841, #67662, #73570, #9175, #53355, #55006, #80714, #60509, #48695, #16325, #80307, #28521, #54177, #72730, #15915, #74393, #42377, #79066, #21382, #66418, #28108, #2450, #16737, #8343, #53762, #73979, #79891, #34009, #8754, #41563, #67252, #69717, #31399, #74811, #43606, #10420, #17156, #55829, #56251, #81947, #30585, #24260, #18780, #49933, #36483, #75631, #25079, #36078, #50753, #82758, #62158, #17969, #76453, #68076, #75216, #4086, #4499, #36899, #57064, #61749, #24673, #37719, #69308, #37316, #49523, #62575, #5728, #42789, #43193, #29754, #49105, #11658, #63393, #81124, #55417, #50341, #56654, #62989, #5328, #23441, #68484, #4917, #30986, #23856, #17561, #82355, #10823, #76038, #18383, #30166, #81537, #44024, #12061, #68889, #11239, #77700, #58314, #78119, #12469, #45681, #1104, #78545, #14151, #65498, #1517, #38131, #6562, #31818, #679, #71798, #26755, #7404, #51158, #7830, #71377, #44423, #27171, #51995, #83172, #20030, #25911, #33497, #57478, #39807, #13727, #63805, #70118, #6144, #33075, #52410, #26334, #52833, #39381, #20452, #19604, #59159, #25492, #58742, #38959, #46105, #76853, #19186, #65066, #32234, #44835, #70533, #12889, #38548, #64228, #57892, #45266, #259, #64643, #51571, #77274, #70962, #13307, #6980, #32649, #14573, #72222, #40225, #9079, #72630, #28835, #34750, #66743, #2350, #59573, #54918, #2761, #14978, #65907, #41873, #28006, #35159, #46938, #60410, #66319, #40637, #21283, #41470, #1929, #20870, #67155, #46523, #29254, #8243, #67567, #28420, #33909, #54080, #22527, #27592, #73886, #22111, #9484, #41055, #53252, #47771, #79795, #61234, #16226, #53666, #78964, #73472, #3589, #8658, #34329, #59994, #79373, #21692, #47355, #15821, #60819, #80212, #73044, #15393, #35571, #3171, #54499, #48189, #9899, #37221, #4815, #75946, #49018, #74715, #36394, #81859, #5640, #62068, #29664, #22936, #81446, #30897, #31307, #4407, #11971, #82265, #24171, #18287, #75128, #30493, #68398, #80624, #5233, #48602, #55326, #36804, #10737, #23763, #11562, #17473, #16644, #74298, #49840, #49434, #30075, #37626, #42284, #67982, #10327, #68800, #17064, #56564, #11145, #43104, #55738, #35989, #61659, #62480, #42701, #4000, #43932, #56156, #62898, #23347, #75539, #17879, #43513, #81035, #69213, #24583, #50250, #69626, #63302, #65399, #76360, #78023, #45164, #7736, #38865, #58641, #18692, #26662, #58216, #19938, #77179, #56971, #582, #13219, #14053, #52316, #6469, #82669, #32553, #39707, #50660, #70026, #83079, #44335, #32139, #163, #6883, #77605, #32973, #38037, #38451, #71699, #12379, #24984, #64546, #26236, #13629, #51898, #20351, #25400, #51064, #12795, #45587, #63712, #64137, #6052, #31724, #57796, #7304, #57387, #25816, #76764, #1009, #71280, #46003, #51476, #19094, #44743, #39281, #70438, #64968, #19510, #70870, #20771, #60720, #60312, #1419, #33402, #27075, #22010, #15713, #72943, #41768, #40956, #41370, #8560, #3069, #67461, #79693, #27909, #47670, #52734, #67051, #59064, #40542, #78445, #27490, #2243, #80108, #46424, #73364, #28736, #47254, #2661, #14882, #53568, #54396, #8147, #34228, #22427, #14475, #79277, #48085, #72116, #40128, #9384, #35054, #21592, #8973, #73786, #65814, #15295, #66636, #72534, #66222, #34648, #33812, #28320, #53981, #16122, #59477, #1830, #53147, #78860, #21186, #46840, #59889, #43406, #61131, #11036, #49735, #43815, #62795, #30794, #50144, #3482, #55220, #80519, #23654, #37111, #75434, #56047, #16540, #56460, #36694, #42185, #35885, #23242, #5130, #48912, #11454, #4707, #61555, #62369, #30380, #48493, #16956, #80927, #74612, #69106, #49324, #42596, #29149, #82162, #24478, #36289, #75841, #17774, #81756, #68298, #29965, #74194, #75026, #18183, #9795, #54818, #22834, #67880, #29557, #3898, #35467, #10217, #10634, #24066, #61962, #4302, #55630, #81339, #17371, #43001, #68694, #76254, #45059, #11870, #18589, #57277, #57695, #57, #32036, #25711, #20251, #51371, #37933, #77074, #26563, #37522, #52217, #906, #63610, #19408, #77920, #76657, #477, #12275, #70761, #31616, #5947, #69921, #6777, #50550, #69520, #32449, #63196 ) ),
 .UNSPECIFIED., .F., .F., .F. ) 
 B_SPLINE_SURFACE_WITH_KNOTS ( ( 2, 2 ),
 ( 3, 2, 2, 2, 2, 2, 2, 2, 2, 2, 2, 2, 2, 2, 2, 2, 2, 2, 2, 2, 2, 2, 2, 2, 2, 2, 2, 2, 2, 2, 2, 2, 2, 2, 2, 2, 2, 2, 2, 2, 2, 2, 2, 2, 2, 2, 2, 2, 2, 2, 2, 2, 2, 2, 2, 2, 2, 2, 2, 2, 2, 2, 2, 2, 2, 2, 2, 2, 2, 2, 2, 2, 2, 2, 2, 2, 2, 2, 2, 2, 2, 2, 2, 2, 2, 2, 2, 2, 2, 2, 2, 2, 2, 2, 2, 2, 2, 2, 2, 2, 2, 2, 2, 2, 2, 2, 2, 2, 2, 2, 2, 2, 2, 2, 2, 2, 2, 2, 2, 2, 2, 2, 2, 2, 2, 2, 2, 2, 2, 2, 2, 2, 2, 2, 2, 2, 2, 2, 2, 2, 2, 2, 2, 2, 2, 2, 2, 2, 2, 2, 2, 2, 2, 2, 2, 2, 2, 2, 2, 2, 2, 2, 2, 2, 2, 2, 2, 2, 2, 2, 2, 2, 2, 2, 2, 2, 2, 2, 2, 2, 2, 2, 2, 2, 2, 2, 2, 2, 2, 2, 2, 2, 2, 2, 2, 2, 2, 2, 2, 2, 2, 2, 2, 2, 2, 2, 2, 2, 2, 2, 2, 2, 2, 2, 2, 2, 2, 2, 2, 2, 2, 2, 2, 2, 2, 2, 2, 2, 2, 2, 2, 2, 2, 2, 2, 2, 2, 2, 2, 2, 2, 2, 2, 2, 2, 2, 2, 2, 2, 2, 2, 2, 2, 2, 2, 3 ),
 ( 0.000000000000000000, 1.000000000000000000 ),
 ( 0.000000000000000000, 0.003787878787878787984, 0.007575757575757575968, 0.01136363636363636395, 0.01515151515151515194, 0.01893939393939393992, 0.02272727272727272790, 0.02651515151515151589, 0.03030303030303030387, 0.03409090909090908839, 0.03787878787878787984, 0.04166666666666666435, 0.04545454545454545581, 0.04924242424242424032, 0.05303030303030303177, 0.05681818181818181629, 0.06060606060606060774, 0.06439393939393939226, 0.06818181818181817677, 0.07196969696969697516, 0.07575757575757575968, 0.07954545454545454419, 0.08333333333333332871, 0.08712121212121212710, 0.09090909090909091161, 0.09469696969696969613, 0.09848484848484848064, 0.1022727272727272790, 0.1060606060606060635, 0.1098484848484848481, 0.1136363636363636326, 0.1174242424242424310, 0.1212121212121212155, 0.1250000000000000000, 0.1287878787878787845, 0.1325757575757575690, 0.1363636363636363535, 0.1401515151515151381, 0.1439393939393939503, 0.1477272727272727348, 0.1515151515151515194, 0.1553030303030303039, 0.1590909090909090884, 0.1628787878787878729, 0.1666666666666666574, 0.1704545454545454419, 0.1742424242424242542, 0.1780303030303030387, 0.1818181818181818232, 0.1856060606060606077, 0.1893939393939393923, 0.1931818181818181768, 0.1969696969696969613, 0.2007575757575757458, 0.2045454545454545581, 0.2083333333333333426, 0.2121212121212121271, 0.2159090909090909116, 0.2196969696969696961, 0.2234848484848484806, 0.2272727272727272652, 0.2310606060606060497, 0.2348484848484848619, 0.2386363636363636465, 0.2424242424242424310, 0.2462121212121212155, 0.2500000000000000000, 0.2537878787878787845, 0.2575757575757575690, 0.2613636363636363535, 0.2651515151515151381, 0.2689393939393939226, 0.2727272727272727071, 0.2765151515151514916, 0.2803030303030302761, 0.2840909090909091161, 0.2878787878787879007, 0.2916666666666666852, 0.2954545454545454697, 0.2992424242424242542, 0.3030303030303030387, 0.3068181818181818232, 0.3106060606060606077, 0.3143939393939393923, 0.3181818181818181768, 0.3219696969696969613, 0.3257575757575757458, 0.3295454545454545303, 0.3333333333333333148, 0.3371212121212120993, 0.3409090909090908839, 0.3446969696969697239, 0.3484848484848485084, 0.3522727272727272929, 0.3560606060606060774, 0.3598484848484848619, 0.3636363636363636465, 0.3674242424242424310, 0.3712121212121212155, 0.3750000000000000000, 0.3787878787878787845, 0.3825757575757575690, 0.3863636363636363535, 0.3901515151515151381, 0.3939393939393939226, 0.3977272727272727071, 0.4015151515151514916, 0.4053030303030302761, 0.4090909090909091161, 0.4128787878787879007, 0.4166666666666666852, 0.4204545454545454697, 0.4242424242424242542, 0.4280303030303030387, 0.4318181818181818232, 0.4356060606060606077, 0.4393939393939393923, 0.4431818181818181768, 0.4469696969696969613, 0.4507575757575757458, 0.4545454545454545303, 0.4583333333333333148, 0.4621212121212120993, 0.4659090909090908839, 0.4696969696969697239, 0.4734848484848485084, 0.4772727272727272929, 0.4810606060606060774, 0.4848484848484848619, 0.4886363636363636465, 0.4924242424242424310, 0.4962121212121212155, 0.5000000000000000000, 0.5037878787878787845, 0.5075757575757575690, 0.5113636363636363535, 0.5151515151515151381, 0.5189393939393939226, 0.5227272727272727071, 0.5265151515151514916, 0.5303030303030302761, 0.5340909090909090606, 0.5378787878787878451, 0.5416666666666666297, 0.5454545454545454142, 0.5492424242424241987, 0.5530303030303029832, 0.5568181818181817677, 0.5606060606060605522, 0.5643939393939394478, 0.5681818181818182323, 0.5719696969696970168, 0.5757575757575758013, 0.5795454545454545858, 0.5833333333333333703, 0.5871212121212121549, 0.5909090909090909394, 0.5946969696969697239, 0.5984848484848485084, 0.6022727272727272929, 0.6060606060606060774, 0.6098484848484848619, 0.6136363636363636465, 0.6174242424242424310, 0.6212121212121212155, 0.6250000000000000000, 0.6287878787878787845, 0.6325757575757575690, 0.6363636363636363535, 0.6401515151515151381, 0.6439393939393939226, 0.6477272727272727071, 0.6515151515151514916, 0.6553030303030302761, 0.6590909090909090606, 0.6628787878787878451, 0.6666666666666666297, 0.6704545454545454142, 0.6742424242424241987, 0.6780303030303029832, 0.6818181818181817677, 0.6856060606060605522, 0.6893939393939394478, 0.6931818181818182323, 0.6969696969696970168, 0.7007575757575758013, 0.7045454545454545858, 0.7083333333333333703, 0.7121212121212121549, 0.7159090909090909394, 0.7196969696969697239, 0.7234848484848485084, 0.7272727272727272929, 0.7310606060606060774, 0.7348484848484848619, 0.7386363636363636465, 0.7424242424242424310, 0.7462121212121212155, 0.7500000000000000000, 0.7537878787878787845, 0.7575757575757575690, 0.7613636363636363535, 0.7651515151515151381, 0.7689393939393939226, 0.7727272727272727071, 0.7765151515151514916, 0.7803030303030302761, 0.7840909090909090606, 0.7878787878787878451, 0.7916666666666666297, 0.7954545454545454142, 0.7992424242424241987, 0.8030303030303029832, 0.8068181818181817677, 0.8106060606060605522, 0.8143939393939394478, 0.8181818181818182323, 0.8219696969696970168, 0.8257575757575758013, 0.8295454545454545858, 0.8333333333333333703, 0.8371212121212121549, 0.8409090909090909394, 0.8446969696969697239, 0.8484848484848485084, 0.8522727272727272929, 0.8560606060606060774, 0.8598484848484848619, 0.8636363636363636465, 0.8674242424242424310, 0.8712121212121212155, 0.8750000000000000000, 0.8787878787878787845, 0.8825757575757575690, 0.8863636363636363535, 0.8901515151515151381, 0.8939393939393939226, 0.8977272727272727071, 0.9015151515151514916, 0.9053030303030302761, 0.9090909090909090606, 0.9128787878787878451, 0.9166666666666666297, 0.9204545454545454142, 0.9242424242424241987, 0.9280303030303029832, 0.9318181818181817677, 0.9356060606060605522, 0.9393939393939394478, 0.9431818181818182323, 0.9469696969696970168, 0.9507575757575758013, 0.9545454545454545858, 0.9583333333333333703, 0.9621212121212121549, 0.9659090909090909394 ),
 .UNSPECIFIED. ) 
 GEOMETRIC_REPRESENTATION_ITEM ( )  RATIONAL_B_SPLINE_SURFACE ( (
 ( 1.000000000000000000, 0.9659258262890683122, 1.000000000000000000, 0.9659258262890683122, 1.000000000000000000, 0.9659258262890683122, 1.000000000000000000, 0.9659258262890683122, 1.000000000000000000, 0.9659258262890683122, 1.000000000000000000, 0.9659258262890683122, 1.000000000000000000, 0.9659258262890683122, 1.000000000000000000, 0.9659258262890683122, 1.000000000000000000, 0.9659258262890683122, 1.000000000000000000, 0.9659258262890683122, 1.000000000000000000, 0.9659258262890683122, 1.000000000000000000, 0.9659258262890683122, 1.000000000000000000, 0.9659258262890683122, 1.000000000000000000, 0.9659258262890683122, 1.000000000000000000, 0.9659258262890683122, 1.000000000000000000, 0.9659258262890683122, 1.000000000000000000, 0.9659258262890683122, 1.000000000000000000, 0.9659258262890683122, 1.000000000000000000, 0.9659258262890683122, 1.000000000000000000, 0.9659258262890683122, 1.000000000000000000, 0.9659258262890683122, 1.000000000000000000, 0.9659258262890683122, 1.000000000000000000, 0.9659258262890683122, 1.000000000000000000, 0.9659258262890683122, 1.000000000000000000, 0.9659258262890683122, 1.000000000000000000, 0.9659258262890683122, 1.000000000000000000, 0.9659258262890683122, 1.000000000000000000, 0.9659258262890683122, 1.000000000000000000, 0.9659258262890683122, 1.000000000000000000, 0.9659258262890683122, 1.000000000000000000, 0.9659258262890683122, 1.000000000000000000, 0.9659258262890683122, 1.000000000000000000, 0.9659258262890683122, 1.000000000000000000, 0.9659258262890683122, 1.000000000000000000, 0.9659258262890683122, 1.000000000000000000, 0.9659258262890683122, 1.000000000000000000, 0.9659258262890683122, 1.000000000000000000, 0.9659258262890683122, 1.000000000000000000, 0.9659258262890683122, 1.000000000000000000, 0.9659258262890683122, 1.000000000000000000, 0.9659258262890683122, 1.000000000000000000, 0.9659258262890683122, 1.000000000000000000, 0.9659258262890683122, 1.000000000000000000, 0.9659258262890683122, 1.000000000000000000, 0.9659258262890683122, 1.000000000000000000, 0.9659258262890683122, 1.000000000000000000, 0.9659258262890683122, 1.000000000000000000, 0.9659258262890683122, 1.000000000000000000, 0.9659258262890683122, 1.000000000000000000, 0.9659258262890683122, 1.000000000000000000, 0.9659258262890683122, 1.000000000000000000, 0.9659258262890683122, 1.000000000000000000, 0.9659258262890683122, 1.000000000000000000, 0.9659258262890683122, 1.000000000000000000, 0.9659258262890683122, 1.000000000000000000, 0.9659258262890683122, 1.000000000000000000, 0.9659258262890683122, 1.000000000000000000, 0.9659258262890683122, 1.000000000000000000, 0.9659258262890683122, 1.000000000000000000, 0.9659258262890683122, 1.000000000000000000, 0.9659258262890683122, 1.000000000000000000, 0.9659258262890683122, 1.000000000000000000, 0.9659258262890683122, 1.000000000000000000, 0.9659258262890683122, 1.000000000000000000, 0.9659258262890683122, 1.000000000000000000, 0.9659258262890683122, 1.000000000000000000, 0.9659258262890683122, 1.000000000000000000, 0.9659258262890683122, 1.000000000000000000, 0.9659258262890683122, 1.000000000000000000, 0.9659258262890683122, 1.000000000000000000, 0.9659258262890683122, 1.000000000000000000, 0.9659258262890683122, 1.000000000000000000, 0.9659258262890683122, 1.000000000000000000, 0.9659258262890683122, 1.000000000000000000, 0.9659258262890683122, 1.000000000000000000, 0.9659258262890683122, 1.000000000000000000, 0.9659258262890683122, 1.000000000000000000, 0.9659258262890683122, 1.000000000000000000, 0.9659258262890683122, 1.000000000000000000, 0.9659258262890683122, 1.000000000000000000, 0.9659258262890683122, 1.000000000000000000, 0.9659258262890683122, 1.000000000000000000, 0.9659258262890683122, 1.000000000000000000, 0.9659258262890683122, 1.000000000000000000, 0.9659258262890683122, 1.000000000000000000, 0.9659258262890683122, 1.000000000000000000, 0.9659258262890683122, 1.000000000000000000, 0.9659258262890683122, 1.000000000000000000, 0.9659258262890683122, 1.000000000000000000, 0.9659258262890683122, 1.000000000000000000, 0.9659258262890683122, 1.000000000000000000, 0.9659258262890683122, 1.000000000000000000, 0.9659258262890683122, 1.000000000000000000, 0.9659258262890683122, 1.000000000000000000, 0.9659258262890683122, 1.000000000000000000, 0.9659258262890683122, 1.000000000000000000, 0.9659258262890683122, 1.000000000000000000, 0.9659258262890683122, 1.000000000000000000, 0.9659258262890683122, 1.000000000000000000, 0.9659258262890683122, 1.000000000000000000, 0.9659258262890683122, 1.000000000000000000, 0.9659258262890683122, 1.000000000000000000, 0.9659258262890683122, 1.000000000000000000, 0.9659258262890683122, 1.000000000000000000, 0.9659258262890683122, 1.000000000000000000, 0.9659258262890683122, 1.000000000000000000, 0.9659258262890683122, 1.000000000000000000, 0.9659258262890683122, 1.000000000000000000, 0.9659258262890683122, 1.000000000000000000, 0.9659258262890683122, 1.000000000000000000, 0.9659258262890683122, 1.000000000000000000, 0.9659258262890683122, 1.000000000000000000, 0.9659258262890683122, 1.000000000000000000, 0.9659258262890683122, 1.000000000000000000, 0.9659258262890683122, 1.000000000000000000, 0.9659258262890683122, 1.000000000000000000, 0.9659258262890683122, 1.000000000000000000, 0.9659258262890683122, 1.000000000000000000, 0.9659258262890683122, 1.000000000000000000, 0.9659258262890683122, 1.000000000000000000, 0.9659258262890683122, 1.000000000000000000, 0.9659258262890683122, 1.000000000000000000, 0.9659258262890683122, 1.000000000000000000, 0.9659258262890683122, 1.000000000000000000, 0.9659258262890683122, 1.000000000000000000, 0.9659258262890683122, 1.000000000000000000, 0.9659258262890683122, 1.000000000000000000, 0.9659258262890683122, 1.000000000000000000, 0.9659258262890683122, 1.000000000000000000, 0.9659258262890683122, 1.000000000000000000, 0.9659258262890683122, 1.000000000000000000, 0.9659258262890683122, 1.000000000000000000, 0.9659258262890683122, 1.000000000000000000, 0.9659258262890683122, 1.000000000000000000, 0.9659258262890683122, 1.000000000000000000, 0.9659258262890683122, 1.000000000000000000, 0.9659258262890683122, 1.000000000000000000, 0.9659258262890683122, 1.000000000000000000, 0.9659258262890683122, 1.000000000000000000, 0.9659258262890683122, 1.000000000000000000, 0.9659258262890683122, 1.000000000000000000, 0.9659258262890683122, 1.000000000000000000, 0.9659258262890683122, 1.000000000000000000, 0.9659258262890683122, 1.000000000000000000, 0.9659258262890683122, 1.000000000000000000, 0.9659258262890683122, 1.000000000000000000, 0.9659258262890683122, 1.000000000000000000, 0.9659258262890683122, 1.000000000000000000, 0.9659258262890683122, 1.000000000000000000, 0.9659258262890683122, 1.000000000000000000, 0.9659258262890683122, 1.000000000000000000, 0.9659258262890683122, 1.000000000000000000, 0.9659258262890683122, 1.000000000000000000, 0.9659258262890683122, 1.000000000000000000, 0.9659258262890683122, 1.000000000000000000, 0.9659258262890683122, 1.000000000000000000, 0.9659258262890683122, 1.000000000000000000, 0.9659258262890683122, 1.000000000000000000, 0.9659258262890683122, 1.000000000000000000, 0.9659258262890683122, 1.000000000000000000, 0.9659258262890683122, 1.000000000000000000, 0.9659258262890683122, 1.000000000000000000, 0.9659258262890683122, 1.000000000000000000, 0.9659258262890683122, 1.000000000000000000, 0.9659258262890683122, 1.000000000000000000, 0.9659258262890683122, 1.000000000000000000, 0.9659258262890683122, 1.000000000000000000, 0.9659258262890683122, 1.000000000000000000, 0.9659258262890683122, 1.000000000000000000, 0.9659258262890683122, 1.000000000000000000, 0.9659258262890683122, 1.000000000000000000, 0.9659258262890683122, 1.000000000000000000, 0.9659258262890683122, 1.000000000000000000, 0.9659258262890683122, 1.000000000000000000, 0.9659258262890683122, 1.000000000000000000, 0.9659258262890683122, 1.000000000000000000, 0.9659258262890683122, 1.000000000000000000, 0.9659258262890683122, 1.000000000000000000, 0.9659258262890683122, 1.000000000000000000, 0.9659258262890683122, 1.000000000000000000, 0.9659258262890683122, 1.000000000000000000, 0.9659258262890683122, 1.000000000000000000, 0.9659258262890683122, 1.000000000000000000, 0.9659258262890683122, 1.000000000000000000, 0.9659258262890683122, 1.000000000000000000, 0.9659258262890683122, 1.000000000000000000, 0.9659258262890683122, 1.000000000000000000, 0.9659258262890683122, 1.000000000000000000, 0.9659258262890683122, 1.000000000000000000, 0.9659258262890683122, 1.000000000000000000, 0.9659258262890683122, 1.000000000000000000, 0.9659258262890683122, 1.000000000000000000, 0.9659258262890683122, 1.000000000000000000, 0.9659258262890683122, 1.000000000000000000, 0.9659258262890683122, 1.000000000000000000, 0.9659258262890683122, 1.000000000000000000, 0.9659258262890683122, 1.000000000000000000, 0.9659258262890683122, 1.000000000000000000, 0.9659258262890683122, 1.000000000000000000, 0.9659258262890683122, 1.000000000000000000, 0.9659258262890683122, 1.000000000000000000, 0.9659258262890683122, 1.000000000000000000, 0.9659258262890683122, 1.000000000000000000, 0.9659258262890683122, 1.000000000000000000, 0.9659258262890683122, 1.000000000000000000, 0.9659258262890683122, 1.000000000000000000, 0.9659258262890683122, 1.000000000000000000, 0.9659258262890683122, 1.000000000000000000, 0.9659258262890683122, 1.000000000000000000, 0.9659258262890683122, 1.000000000000000000, 0.9659258262890683122, 1.000000000000000000, 0.9659258262890683122, 1.000000000000000000, 0.9659258262890683122, 1.000000000000000000, 0.9659258262890683122, 1.000000000000000000, 0.9659258262890683122, 1.000000000000000000, 0.9659258262890683122, 1.000000000000000000, 0.9659258262890683122, 1.000000000000000000, 0.9659258262890683122, 1.000000000000000000, 0.9659258262890683122, 1.000000000000000000, 0.9659258262890683122, 1.000000000000000000, 0.9659258262890683122, 1.000000000000000000, 0.9659258262890683122, 1.000000000000000000, 0.9659258262890683122, 1.000000000000000000, 0.9659258262890683122, 1.000000000000000000, 0.9659258262890683122, 1.000000000000000000, 0.9659258262890683122, 1.000000000000000000, 0.9659258262890683122, 1.000000000000000000, 0.9659258262890683122, 1.000000000000000000, 0.9659258262890683122, 1.000000000000000000, 0.9659258262890683122, 1.000000000000000000, 0.9659258262890683122, 1.000000000000000000, 0.9659258262890683122, 1.000000000000000000, 0.9659258262890683122, 1.000000000000000000, 0.9659258262890683122, 1.000000000000000000, 0.9659258262890683122, 1.000000000000000000, 0.9659258262890683122, 1.000000000000000000, 0.9659258262890683122, 1.000000000000000000, 0.9659258262890683122, 1.000000000000000000, 0.9659258262890683122, 1.000000000000000000, 0.9659258262890683122, 1.000000000000000000, 0.9659258262890683122, 1.000000000000000000, 0.9659258262890683122, 1.000000000000000000, 0.9659258262890683122, 1.000000000000000000, 0.9659258262890683122, 1.000000000000000000, 0.9659258262890683122, 1.000000000000000000, 0.9659258262890683122, 1.000000000000000000, 0.9659258262890683122, 1.000000000000000000, 0.9659258262890683122, 1.000000000000000000, 0.9659258262890683122, 1.000000000000000000, 0.9659258262890683122, 1.000000000000000000, 0.9659258262890683122, 1.000000000000000000, 0.9659258262890683122, 1.000000000000000000, 0.9659258262890683122, 1.000000000000000000, 0.9659258262890683122, 1.000000000000000000, 0.9659258262890683122, 1.000000000000000000),
 ( 1.000000000000000000, 0.9659258262890683122, 1.000000000000000000, 0.9659258262890683122, 1.000000000000000000, 0.9659258262890683122, 1.000000000000000000, 0.9659258262890683122, 1.000000000000000000, 0.9659258262890683122, 1.000000000000000000, 0.9659258262890683122, 1.000000000000000000, 0.9659258262890683122, 1.000000000000000000, 0.9659258262890683122, 1.000000000000000000, 0.9659258262890683122, 1.000000000000000000, 0.9659258262890683122, 1.000000000000000000, 0.9659258262890683122, 1.000000000000000000, 0.9659258262890683122, 1.000000000000000000, 0.9659258262890683122, 1.000000000000000000, 0.9659258262890683122, 1.000000000000000000, 0.9659258262890683122, 1.000000000000000000, 0.9659258262890683122, 1.000000000000000000, 0.9659258262890683122, 1.000000000000000000, 0.9659258262890683122, 1.000000000000000000, 0.9659258262890683122, 1.000000000000000000, 0.9659258262890683122, 1.000000000000000000, 0.9659258262890683122, 1.000000000000000000, 0.9659258262890683122, 1.000000000000000000, 0.9659258262890683122, 1.000000000000000000, 0.9659258262890683122, 1.000000000000000000, 0.9659258262890683122, 1.000000000000000000, 0.9659258262890683122, 1.000000000000000000, 0.9659258262890683122, 1.000000000000000000, 0.9659258262890683122, 1.000000000000000000, 0.9659258262890683122, 1.000000000000000000, 0.9659258262890683122, 1.000000000000000000, 0.9659258262890683122, 1.000000000000000000, 0.9659258262890683122, 1.000000000000000000, 0.9659258262890683122, 1.000000000000000000, 0.9659258262890683122, 1.000000000000000000, 0.9659258262890683122, 1.000000000000000000, 0.9659258262890683122, 1.000000000000000000, 0.9659258262890683122, 1.000000000000000000, 0.9659258262890683122, 1.000000000000000000, 0.9659258262890683122, 1.000000000000000000, 0.9659258262890683122, 1.000000000000000000, 0.9659258262890683122, 1.000000000000000000, 0.9659258262890683122, 1.000000000000000000, 0.9659258262890683122, 1.000000000000000000, 0.9659258262890683122, 1.000000000000000000, 0.9659258262890683122, 1.000000000000000000, 0.9659258262890683122, 1.000000000000000000, 0.9659258262890683122, 1.000000000000000000, 0.9659258262890683122, 1.000000000000000000, 0.9659258262890683122, 1.000000000000000000, 0.9659258262890683122, 1.000000000000000000, 0.9659258262890683122, 1.000000000000000000, 0.9659258262890683122, 1.000000000000000000, 0.9659258262890683122, 1.000000000000000000, 0.9659258262890683122, 1.000000000000000000, 0.9659258262890683122, 1.000000000000000000, 0.9659258262890683122, 1.000000000000000000, 0.9659258262890683122, 1.000000000000000000, 0.9659258262890683122, 1.000000000000000000, 0.9659258262890683122, 1.000000000000000000, 0.9659258262890683122, 1.000000000000000000, 0.9659258262890683122, 1.000000000000000000, 0.9659258262890683122, 1.000000000000000000, 0.9659258262890683122, 1.000000000000000000, 0.9659258262890683122, 1.000000000000000000, 0.9659258262890683122, 1.000000000000000000, 0.9659258262890683122, 1.000000000000000000, 0.9659258262890683122, 1.000000000000000000, 0.9659258262890683122, 1.000000000000000000, 0.9659258262890683122, 1.000000000000000000, 0.9659258262890683122, 1.000000000000000000, 0.9659258262890683122, 1.000000000000000000, 0.9659258262890683122, 1.000000000000000000, 0.9659258262890683122, 1.000000000000000000, 0.9659258262890683122, 1.000000000000000000, 0.9659258262890683122, 1.000000000000000000, 0.9659258262890683122, 1.000000000000000000, 0.9659258262890683122, 1.000000000000000000, 0.9659258262890683122, 1.000000000000000000, 0.9659258262890683122, 1.000000000000000000, 0.9659258262890683122, 1.000000000000000000, 0.9659258262890683122, 1.000000000000000000, 0.9659258262890683122, 1.000000000000000000, 0.9659258262890683122, 1.000000000000000000, 0.9659258262890683122, 1.000000000000000000, 0.9659258262890683122, 1.000000000000000000, 0.9659258262890683122, 1.000000000000000000, 0.9659258262890683122, 1.000000000000000000, 0.9659258262890683122, 1.000000000000000000, 0.9659258262890683122, 1.000000000000000000, 0.9659258262890683122, 1.000000000000000000, 0.9659258262890683122, 1.000000000000000000, 0.9659258262890683122, 1.000000000000000000, 0.9659258262890683122, 1.000000000000000000, 0.9659258262890683122, 1.000000000000000000, 0.9659258262890683122, 1.000000000000000000, 0.9659258262890683122, 1.000000000000000000, 0.9659258262890683122, 1.000000000000000000, 0.9659258262890683122, 1.000000000000000000, 0.9659258262890683122, 1.000000000000000000, 0.9659258262890683122, 1.000000000000000000, 0.9659258262890683122, 1.000000000000000000, 0.9659258262890683122, 1.000000000000000000, 0.9659258262890683122, 1.000000000000000000, 0.9659258262890683122, 1.000000000000000000, 0.9659258262890683122, 1.000000000000000000, 0.9659258262890683122, 1.000000000000000000, 0.9659258262890683122, 1.000000000000000000, 0.9659258262890683122, 1.000000000000000000, 0.9659258262890683122, 1.000000000000000000, 0.9659258262890683122, 1.000000000000000000, 0.9659258262890683122, 1.000000000000000000, 0.9659258262890683122, 1.000000000000000000, 0.9659258262890683122, 1.000000000000000000, 0.9659258262890683122, 1.000000000000000000, 0.9659258262890683122, 1.000000000000000000, 0.9659258262890683122, 1.000000000000000000, 0.9659258262890683122, 1.000000000000000000, 0.9659258262890683122, 1.000000000000000000, 0.9659258262890683122, 1.000000000000000000, 0.9659258262890683122, 1.000000000000000000, 0.9659258262890683122, 1.000000000000000000, 0.9659258262890683122, 1.000000000000000000, 0.9659258262890683122, 1.000000000000000000, 0.9659258262890683122, 1.000000000000000000, 0.9659258262890683122, 1.000000000000000000, 0.9659258262890683122, 1.000000000000000000, 0.9659258262890683122, 1.000000000000000000, 0.9659258262890683122, 1.000000000000000000, 0.9659258262890683122, 1.000000000000000000, 0.9659258262890683122, 1.000000000000000000, 0.9659258262890683122, 1.000000000000000000, 0.9659258262890683122, 1.000000000000000000, 0.9659258262890683122, 1.000000000000000000, 0.9659258262890683122, 1.000000000000000000, 0.9659258262890683122, 1.000000000000000000, 0.9659258262890683122, 1.000000000000000000, 0.9659258262890683122, 1.000000000000000000, 0.9659258262890683122, 1.000000000000000000, 0.9659258262890683122, 1.000000000000000000, 0.9659258262890683122, 1.000000000000000000, 0.9659258262890683122, 1.000000000000000000, 0.9659258262890683122, 1.000000000000000000, 0.9659258262890683122, 1.000000000000000000, 0.9659258262890683122, 1.000000000000000000, 0.9659258262890683122, 1.000000000000000000, 0.9659258262890683122, 1.000000000000000000, 0.9659258262890683122, 1.000000000000000000, 0.9659258262890683122, 1.000000000000000000, 0.9659258262890683122, 1.000000000000000000, 0.9659258262890683122, 1.000000000000000000, 0.9659258262890683122, 1.000000000000000000, 0.9659258262890683122, 1.000000000000000000, 0.9659258262890683122, 1.000000000000000000, 0.9659258262890683122, 1.000000000000000000, 0.9659258262890683122, 1.000000000000000000, 0.9659258262890683122, 1.000000000000000000, 0.9659258262890683122, 1.000000000000000000, 0.9659258262890683122, 1.000000000000000000, 0.9659258262890683122, 1.000000000000000000, 0.9659258262890683122, 1.000000000000000000, 0.9659258262890683122, 1.000000000000000000, 0.9659258262890683122, 1.000000000000000000, 0.9659258262890683122, 1.000000000000000000, 0.9659258262890683122, 1.000000000000000000, 0.9659258262890683122, 1.000000000000000000, 0.9659258262890683122, 1.000000000000000000, 0.9659258262890683122, 1.000000000000000000, 0.9659258262890683122, 1.000000000000000000, 0.9659258262890683122, 1.000000000000000000, 0.9659258262890683122, 1.000000000000000000, 0.9659258262890683122, 1.000000000000000000, 0.9659258262890683122, 1.000000000000000000, 0.9659258262890683122, 1.000000000000000000, 0.9659258262890683122, 1.000000000000000000, 0.9659258262890683122, 1.000000000000000000, 0.9659258262890683122, 1.000000000000000000, 0.9659258262890683122, 1.000000000000000000, 0.9659258262890683122, 1.000000000000000000, 0.9659258262890683122, 1.000000000000000000, 0.9659258262890683122, 1.000000000000000000, 0.9659258262890683122, 1.000000000000000000, 0.9659258262890683122, 1.000000000000000000, 0.9659258262890683122, 1.000000000000000000, 0.9659258262890683122, 1.000000000000000000, 0.9659258262890683122, 1.000000000000000000, 0.9659258262890683122, 1.000000000000000000, 0.9659258262890683122, 1.000000000000000000, 0.9659258262890683122, 1.000000000000000000, 0.9659258262890683122, 1.000000000000000000, 0.9659258262890683122, 1.000000000000000000, 0.9659258262890683122, 1.000000000000000000, 0.9659258262890683122, 1.000000000000000000, 0.9659258262890683122, 1.000000000000000000, 0.9659258262890683122, 1.000000000000000000, 0.9659258262890683122, 1.000000000000000000, 0.9659258262890683122, 1.000000000000000000, 0.9659258262890683122, 1.000000000000000000, 0.9659258262890683122, 1.000000000000000000, 0.9659258262890683122, 1.000000000000000000, 0.9659258262890683122, 1.000000000000000000, 0.9659258262890683122, 1.000000000000000000, 0.9659258262890683122, 1.000000000000000000, 0.9659258262890683122, 1.000000000000000000, 0.9659258262890683122, 1.000000000000000000, 0.9659258262890683122, 1.000000000000000000, 0.9659258262890683122, 1.000000000000000000, 0.9659258262890683122, 1.000000000000000000, 0.9659258262890683122, 1.000000000000000000, 0.9659258262890683122, 1.000000000000000000, 0.9659258262890683122, 1.000000000000000000, 0.9659258262890683122, 1.000000000000000000, 0.9659258262890683122, 1.000000000000000000, 0.9659258262890683122, 1.000000000000000000, 0.9659258262890683122, 1.000000000000000000, 0.9659258262890683122, 1.000000000000000000, 0.9659258262890683122, 1.000000000000000000, 0.9659258262890683122, 1.000000000000000000, 0.9659258262890683122, 1.000000000000000000, 0.9659258262890683122, 1.000000000000000000, 0.9659258262890683122, 1.000000000000000000, 0.9659258262890683122, 1.000000000000000000, 0.9659258262890683122, 1.000000000000000000, 0.9659258262890683122, 1.000000000000000000, 0.9659258262890683122, 1.000000000000000000, 0.9659258262890683122, 1.000000000000000000, 0.9659258262890683122, 1.000000000000000000, 0.9659258262890683122, 1.000000000000000000, 0.9659258262890683122, 1.000000000000000000, 0.9659258262890683122, 1.000000000000000000, 0.9659258262890683122, 1.000000000000000000, 0.9659258262890683122, 1.000000000000000000, 0.9659258262890683122, 1.000000000000000000, 0.9659258262890683122, 1.000000000000000000, 0.9659258262890683122, 1.000000000000000000, 0.9659258262890683122, 1.000000000000000000, 0.9659258262890683122, 1.000000000000000000, 0.9659258262890683122, 1.000000000000000000, 0.9659258262890683122, 1.000000000000000000, 0.9659258262890683122, 1.000000000000000000, 0.9659258262890683122, 1.000000000000000000, 0.9659258262890683122, 1.000000000000000000, 0.9659258262890683122, 1.000000000000000000, 0.9659258262890683122, 1.000000000000000000, 0.9659258262890683122, 1.000000000000000000, 0.9659258262890683122, 1.000000000000000000, 0.9659258262890683122, 1.000000000000000000, 0.9659258262890683122, 1.000000000000000000, 0.9659258262890683122, 1.000000000000000000, 0.9659258262890683122, 1.000000000000000000, 0.9659258262890683122, 1.000000000000000000, 0.9659258262890683122, 1.000000000000000000, 0.9659258262890683122, 1.000000000000000000, 0.9659258262890683122, 1.000000000000000000, 0.9659258262890683122, 1.000000000000000000, 0.9659258262890683122, 1.000000000000000000) ) ) 
 REPRESENTATION_ITEM ( '' )  SURFACE ( )  );
#62610=CARTESIAN_POINT ( 'NONE',  ( -0.5446194225721777693, -0.08942795157527998196, 0.3641732283464567121 ) ) ;
#62611=ORIENTED_EDGE ( 'NONE', *, *, #16161, .F. ) ;
#62614=CARTESIAN_POINT ( 'NONE',  ( -1.450131233595799651, -0.5511811023622046335, 0.09757992244046803654 ) ) ;
#62615=CARTESIAN_POINT ( 'NONE',  ( -0.9645669291338575535, 0.1660481256975883668, -0.3530559997133364547 ) ) ;
#62616=CARTESIAN_POINT ( 'NONE',  ( -0.9383202099737524282, -0.3162353388693409650, -0.4822834645669289433 ) ) ;
#62618=CARTESIAN_POINT ( 'NONE',  ( -0.8989501312335946848, 0.2952755905511810774, -0.1292274648535930714 ) ) ;
#62619=CARTESIAN_POINT ( 'NONE',  ( -0.7480314960629914633, 0.2952755905511811885, 0.000000000000000000 ) ) ;
#62621=CARTESIAN_POINT ( 'NONE',  ( -1.712598425196849572, 0.1660481256975885056, 0.3530559997133364547 ) ) ;
#62622=CARTESIAN_POINT ( 'NONE',  ( 0.6364829396325465405, -0.2845877964562161244, -0.3641732283464567121 ) ) ;
#62625=CARTESIAN_POINT ( 'NONE',  ( 0.1902887139107617975, 0.1771653543307087630, 0.09757992244046791164 ) ) ;
#62626=CARTESIAN_POINT ( 'NONE',  ( -0.4921259842519677963, 0.1660481256975883668, -0.3530559997133364547 ) ) ;
#62628=CARTESIAN_POINT ( 'NONE',  ( -0.07217847769028787330, -0.05778040916215522460, 0.4822834645669289988 ) ) ;
#62631=CARTESIAN_POINT ( 'NONE',  ( -0.8464566929133849893, 0.1012011053420777407, 0.2882089793578256898 ) ) ;
#62635=CARTESIAN_POINT ( 'NONE',  ( -1.332020997375327642, -0.2845877964562161244, -0.3641732283464567121 ) ) ;
#62636=CARTESIAN_POINT ( 'NONE',  ( -0.7611548556430438595, 0.2306618581243848609, 0.2411417322834645549 ) ) ;
#62640=CARTESIAN_POINT ( 'NONE',  ( 1.463254593175853824, -0.6692913385826771977, 0.1292274648535927661 ) ) ;
#62641=CARTESIAN_POINT ( 'NONE',  ( 0.6496062992125991586, 0.1660481256975885056, 0.3530559997133364547 ) ) ;
#62642=CARTESIAN_POINT ( 'NONE',  ( 0.3805774278215230400, -0.4281496062992124485, 0.4176697321401328655 ) ) ;
#62643=CARTESIAN_POINT ( 'NONE',  ( -1.233595800524933894, -0.5023911411419708095, -0.1820866141732282451 ) ) ;
#62645=VECTOR ( 'NONE', #24439, 39.37007874015748143 ) ;
#62646=CARTESIAN_POINT ( 'NONE',  ( -0.4068241469816267775, 0.05413385826771626580, -0.4176697321401330321 ) ) ;
#62648=CARTESIAN_POINT ( 'NONE',  ( -0.7152230971128602510, -0.05778040916215560624, -0.4822834645669293319 ) ) ;
#62651=CARTESIAN_POINT ( 'NONE',  ( 1.423884514435696191, -0.08942795157527998196, 0.3641732283464567121 ) ) ;
#62652=CARTESIAN_POINT ( 'NONE',  ( -0.5052493438320203589, -0.5511811023622046335, 0.09757992244046803654 ) ) ;
#62653=CARTESIAN_POINT ( 'NONE',  ( 1.128608923884515169, -0.5023911411419708095, -0.1820866141732282451 ) ) ;
#62654=CARTESIAN_POINT ( 'NONE',  ( -1.627296587926508442, -0.6046776061558809534, -0.2411417322834644161 ) ) ;
#62655=CARTESIAN_POINT ( 'NONE',  ( -1.161417322834644716, 0.07958543189024085140, 0.2665933059059887866 ) ) ;
#62657=CARTESIAN_POINT ( 'NONE',  ( 0.4396325459317593221, 0.1771653543307087075, -0.09757992244046823083 ) ) ;
#62658=CARTESIAN_POINT ( 'NONE',  ( -0.2296587926509179312, -0.05778040916215522460, 0.4822834645669289988 ) ) ;
#62661=CARTESIAN_POINT ( 'NONE',  ( 0.07874015748031558404, -0.1870078740157479769, 0.3641732283464567677 ) ) ;
#62662=CARTESIAN_POINT ( 'NONE',  ( -1.646981627296586703, -0.2845877964562161244, -0.3641732283464567121 ) ) ;
#62663=CARTESIAN_POINT ( 'NONE',  ( 0.7020997375328090762, -0.3162353388693405765, 0.4822834645669290543 ) ) ;
#62665=CARTESIAN_POINT ( 'NONE',  ( 1.568241469816273437, -0.2845877964562159024, 0.3641732283464567677 ) ) ;
#62666=CARTESIAN_POINT ( 'NONE',  ( -1.108923884514435132, -0.3162353388693405765, 0.4822834645669290543 ) ) ;
#62667=CARTESIAN_POINT ( 'NONE',  ( -0.3805774278215216522, -0.004921259842519576551, 0.3153832671262227771 ) ) ;
#62668=CARTESIAN_POINT ( 'NONE',  ( 1.436417322834645516, 0.4405861044731112508, -0.3149606299212598381 ) ) ;
#62669=CARTESIAN_POINT ( 'NONE',  ( 0.3477690288713918276, 0.1771653543307087630, 0.09757992244046791164 ) ) ;
#62670=CARTESIAN_POINT ( 'NONE',  ( -1.240157480314959759, 0.1660481256975885056, 0.3530559997133364547 ) ) ;
#62671=CARTESIAN_POINT ( 'NONE',  ( -0.3346456692913377662, 0.1660481256975883668, -0.3530559997133364547 ) ) ;
#62674=CARTESIAN_POINT ( 'NONE',  ( 0.4658792650918640033, -0.2845877964562159024, 0.3641732283464567677 ) ) ;
#62675=CARTESIAN_POINT ( 'NONE',  ( -0.4199475065616791736, -0.6046776061558807314, 0.2411417322834647770 ) ) ;
#62676=CARTESIAN_POINT ( 'NONE',  ( -0.6955380577427815458, 0.05413385826771666132, 0.4176697321401328100 ) ) ;
#62677=CARTESIAN_POINT ( 'NONE',  ( -0.6824146981627288167, 0.1283753931104748280, 0.1820866141732283561 ) ) ;
#62679=CARTESIAN_POINT ( 'NONE',  ( -0.02624671916010428221, 0.2306618581243847221, -0.2411417322834647770 ) ) ;
#62680=CARTESIAN_POINT ( 'NONE',  ( -1.049868766404198794, 0.1283753931104746893, -0.1820866141732285504 ) ) ;
#62681=CARTESIAN_POINT ( 'NONE',  ( -1.535433070866141225, -0.6692913385826771977, 8.415575281601705876E-17 ) ) ;
#62682=CARTESIAN_POINT ( 'NONE',  ( 0.2230971128608929543, 0.009842519685039144428, -0.3409548833797004797 ) ) ;
#62684=CARTESIAN_POINT ( 'NONE',  ( -1.384514435695537005, 0.1771653543307087630, 0.09757992244046791164 ) ) ;
#62685=CARTESIAN_POINT ( 'NONE',  ( -1.410761154855642463, -0.05778040916215522460, 0.4822834645669289988 ) ) ;
#62686=CARTESIAN_POINT ( 'NONE',  ( -1.043307086614172707, 0.1660481256975883668, -0.3530559997133364547 ) ) ;
#62687=CARTESIAN_POINT ( 'NONE',  ( 1.561679790026247350, -0.4281496062992124485, 0.4176697321401328655 ) ) ;
#62690=CARTESIAN_POINT ( 'NONE',  ( 1.095800524934383846, -0.05778040916215560624, -0.4822834645669293319 ) ) ;
#62691=CARTESIAN_POINT ( 'NONE',  ( 0.6364829396325465405, -0.3162353388693409650, -0.4822834645669289433 ) ) ;
#62694=AXIS2_PLACEMENT_3D ( 'NONE', #37319, #62991, #22624 ) ;
#62697=CARTESIAN_POINT ( 'NONE',  ( 1.377952755905512472, -0.5511811023622047445, 6.969142054262312111E-17 ) ) ;
#62700=CARTESIAN_POINT ( 'NONE',  ( -0.8595800524934373854, -0.08942795157527998196, 0.3641732283464567121 ) ) ;
#62703=CARTESIAN_POINT ( 'NONE',  ( 0.5708661417322841158, -0.5400638737290845981, -0.3530559997133363437 ) ) ;
#62704=CARTESIAN_POINT ( 'NONE',  ( -0.5971128608923877978, 0.2952755905511811885, 0.1292274648535926551 ) ) ;
#62706=CARTESIAN_POINT ( 'NONE',  ( -1.299212598425196097, 0.2952755905511811885, 0.000000000000000000 ) ) ;
#62707=CARTESIAN_POINT ( 'NONE',  ( 1.036745406824147731, 0.05413385826771666132, 0.4176697321401328100 ) ) ;
#62708=CARTESIAN_POINT ( 'NONE',  ( -1.620734908136482577, 0.1771653543307087630, 0.09757992244046791164 ) ) ;
#62710=CARTESIAN_POINT ( 'NONE',  ( -0.09186351706036663400, -0.4281496062992124485, 0.4176697321401328655 ) ) ;
#62711=CARTESIAN_POINT ( 'NONE',  ( -1.364829396325458521, -0.6046776061558807314, 0.2411417322834647770 ) ) ;
#62712=CARTESIAN_POINT ( 'NONE',  ( -1.607611548556429737, 0.2952755905511810774, -0.1292274648535930714 ) ) ;
#62715=CARTESIAN_POINT ( 'NONE',  ( 0.6627296587926517768, -0.5511811023622048555, -0.09757992244046775898 ) ) ;
#62719=CARTESIAN_POINT ( 'NONE',  ( 0.1771653543307093182, 0.07958543189024085140, 0.2665933059059887866 ) ) ;
#62721=CARTESIAN_POINT ( 'NONE',  ( -1.646981627296586703, -0.3162353388693409650, -0.4822834645669289433 ) ) ;
#62722=CARTESIAN_POINT ( 'NONE',  ( 0.6824146981627303710, 0.2306618581243847221, -0.2411417322834647770 ) ) ;
#62723=CARTESIAN_POINT ( 'NONE',  ( 0.4593175853018379162, -0.4281496062992124485, 0.4176697321401328655 ) ) ;
#62724=CARTESIAN_POINT ( 'NONE',  ( -0.4855643044619415427, -0.4281496062992124485, 0.4176697321401328655 ) ) ;
#62726=CARTESIAN_POINT ( 'NONE',  ( -1.404199475065615932, -0.4281496062992127816, -0.4176697321401328100 ) ) ;
#62728=CARTESIAN_POINT ( 'NONE',  ( 1.417322834645670104, -0.1870078740157479769, 0.3641732283464567677 ) ) ;
#62729=CARTESIAN_POINT ( 'NONE',  ( -1.227034120734907141, -0.6692913385826773087, -0.1292274648535924053 ) ) ;
#62730=CARTESIAN_POINT ( 'NONE',  ( 0.6824146981627303710, -0.6046776061558807314, 0.2411417322834647770 ) ) ;
#62731=CARTESIAN_POINT ( 'NONE',  ( 1.056430446194226658, 0.2952755905511811885, 0.1292274648535926551 ) ) ;
#62733=CARTESIAN_POINT ( 'NONE',  ( -1.227034120734907585, 0.2952755905511811885, 0.1292274648535926551 ) ) ;
#62735=B_SPLINE_CURVE_WITH_KNOTS ( 'NONE', 3,
 ( #82171, #24487, #37531, #63207, #31211, #56879, #82572 ),
 .UNSPECIFIED., .F., .F.,
 ( 4, 3, 4 ),
 ( 6.162975822039154730E-33, 0.001246232571205221906, 0.002492492258783241162 ),
 .UNSPECIFIED. ) ;
#62736=CARTESIAN_POINT ( 'NONE',  ( 0.09186351706036799403, -0.4281496062992127816, -0.4176697321401328100 ) ) ;
#62738=ADVANCED_FACE ( 'NONE', ( #45395 ), #361, .F. ) ;
#62740=CARTESIAN_POINT ( 'NONE',  ( -1.561679790026246017, -0.3690944881889765550, -0.3153832671262227771 ) ) ;
#62741=CARTESIAN_POINT ( 'NONE',  ( 0.4265091863517067594, 0.1771653543307087630, 0.09757992244046791164 ) ) ;
#62742=CARTESIAN_POINT ( 'NONE',  ( 0.8530183727034126306, 0.05413385826771626580, -0.4176697321401330321 ) ) ;
#62744=CARTESIAN_POINT ( 'NONE',  ( 0.7742782152230979209, -0.004921259842519870586, -0.3153832671262229437 ) ) ;
#62745=CARTESIAN_POINT ( 'NONE',  ( 0.5511811023622054106, -0.1870078740157480879, -0.4822834645669291653 ) ) ;
#62748=CARTESIAN_POINT ( 'NONE',  ( -0.6561679790026240244, -0.6046776061558807314, 0.2411417322834647770 ) ) ;
#62750=CARTESIAN_POINT ( 'NONE',  ( 0.9317585301837276734, -0.3690944881889763329, 0.3153832671262228327 ) ) ;
#62751=CARTESIAN_POINT ( 'NONE',  ( 0.05249343832021075018, 0.2306618581243847221, -0.2411417322834647770 ) ) ;
#62753=CARTESIAN_POINT ( 'NONE',  ( -0.1181102362204717315, 0.2952755905511811885, 0.000000000000000000 ) ) ;
#62754=CARTESIAN_POINT ( 'NONE',  ( 0.2034120734908144990, -0.5511811023622046335, 0.09757992244046803654 ) ) ;
#62756=CARTESIAN_POINT ( 'NONE',  ( -0.3871391076115479057, -0.3162353388693409650, -0.4822834645669289433 ) ) ;
#62757=CARTESIAN_POINT ( 'NONE',  ( 0.5774278215223103139, -0.5023911411419708095, -0.1820866141732282451 ) ) ;
#62761=CARTESIAN_POINT ( 'NONE',  ( 0.3412073490813655186, -0.6046776061558809534, -0.2411417322834644161 ) ) ;
#62765=CARTESIAN_POINT ( 'NONE',  ( 1.194225721784777594, -0.004921259842519576551, 0.3153832671262227771 ) ) ;
#62766=CARTESIAN_POINT ( 'NONE',  ( -0.4790026246719154557, -0.2845877964562159024, 0.3641732283464567677 ) ) ;
#62767=CARTESIAN_POINT ( 'NONE',  ( -0.9317585301837263412, -0.004921259842519576551, 0.3153832671262227771 ) ) ;
#62768=CARTESIAN_POINT ( 'NONE',  ( -0.1377952755905504645, -0.5400638737290845981, -0.3530559997133363437 ) ) ;
#62769=CARTESIAN_POINT ( 'NONE',  ( 0.2821522309711292364, -0.6692913385826771977, 0.1292274648535927661 ) ) ;
#62770=CARTESIAN_POINT ( 'NONE',  ( 0.9776902887139113929, -0.5511811023622048555, -0.09757992244046775898 ) ) ;
#62771=CARTESIAN_POINT ( 'NONE',  ( -1.574803149606298636, -0.1870078740157479769, 0.3641732283464567677 ) ) ;
#62772=CARTESIAN_POINT ( 'NONE',  ( 1.601049868766404982, 0.1283753931104748280, 0.1820866141732283561 ) ) ;
#62773=CARTESIAN_POINT ( 'NONE',  ( 0.5839895013123367340, 0.2952755905511811885, 0.1292274648535926551 ) ) ;
#62775=CARTESIAN_POINT ( 'NONE',  ( 0.1837270341207354329, 0.2306618581243848609, 0.2411417322834645549 ) ) ;
#62777=CARTESIAN_POINT ( 'NONE',  ( 0.9776902887139113929, -0.6692913385826773087, -0.1292274648535924053 ) ) ;
#62778=CARTESIAN_POINT ( 'NONE',  ( 0.4658792650918641698, -0.05778040916215560624, -0.4822834645669293319 ) ) ;
#62780=CARTESIAN_POINT ( 'NONE',  ( 0.2755905511811031494, 0.1771653543307087630, 0.000000000000000000 ) ) ;
#62781=CARTESIAN_POINT ( 'NONE',  ( 1.056430446194226658, 0.2952755905511811885, 0.1292274648535926551 ) ) ;
#62782=CARTESIAN_POINT ( 'NONE',  ( 0.01312335958005323398, -0.004921259842519576551, 0.3153832671262227771 ) ) ;
#62783=CARTESIAN_POINT ( 'NONE',  ( -0.4002624671916004129, -0.3162353388693405765, 0.4822834645669290543 ) ) ;
#62784=CARTESIAN_POINT ( 'NONE',  ( 0.2493438320209980519, -0.4281496062992127816, -0.4176697321401328100 ) ) ;
#62785=CARTESIAN_POINT ( 'NONE',  ( -0.8202099737532799750, 0.2952755905511810774, -0.1292274648535930714 ) ) ;
#62786=CARTESIAN_POINT ( 'NONE',  ( -0.3543307086614165824, -0.5511811023622047445, 6.969142054262312111E-17 ) ) ;
#62787=CARTESIAN_POINT ( 'NONE',  ( 0.4986876640419954376, 0.2306618581243848609, 0.2411417322834645549 ) ) ;
#62788=CARTESIAN_POINT ( 'NONE',  ( 0.9448818897637802916, -0.1870078740157480601, -0.3641732283464567677 ) ) ;
#62789=CARTESIAN_POINT ( 'NONE',  ( -0.3805774278215216522, 0.05413385826771666132, 0.4176697321401328100 ) ) ;
#62790=CARTESIAN_POINT ( 'NONE',  ( 1.168329637866469151, 0.004960608223778500969, -0.3437734562760191848 ) ) ;
#62791=CARTESIAN_POINT ( 'NONE',  ( -0.6365311798329505999, 1.942272084518551489, 0.5177672855601881396 ) ) ;
#62793=CARTESIAN_POINT ( 'NONE',  ( 1.640419947506562393, -0.4281496062992124485, 0.4176697321401328655 ) ) ;
#62795=CARTESIAN_POINT ( 'NONE',  ( -1.062992125984250968, -0.6692913385826771977, 8.415575281601705876E-17 ) ) ;
#62796=CARTESIAN_POINT ( 'NONE',  ( -0.8727034120734901146, -0.05778040916215560624, -0.4822834645669293319 ) ) ;
#62797=( BOUNDED_CURVE ( )  B_SPLINE_CURVE ( 1, ( #29049, #47990 ),
 .UNSPECIFIED., .F., .F. ) 
 B_SPLINE_CURVE_WITH_KNOTS ( ( 2, 2 ),
 ( 3.469446951953614189E-18, 0.002000000000000001776 ),
 .UNSPECIFIED. ) 
 CURVE ( )  GEOMETRIC_REPRESENTATION_ITEM ( )  RATIONAL_B_SPLINE_CURVE ( ( 0.9875488213027527884, 0.9875488213027527884 ) ) 
 REPRESENTATION_ITEM ( '' )  );
#62801=CARTESIAN_POINT ( 'NONE',  ( 0.4133858267716541968, 0.07958543189024085140, 0.2665933059059887866 ) ) ;
#62803=CARTESIAN_POINT ( 'NONE',  ( 0.8333333333333340365, 0.2952755905511810774, -0.1292274648535930714 ) ) ;
#62806=CARTESIAN_POINT ( 'NONE',  ( -1.594488188976377563, -0.4536011799217367080, 0.2665933059059888421 ) ) ;
#62807=CARTESIAN_POINT ( 'NONE',  ( 1.325459317585302665, -0.4281496062992124485, 0.4176697321401328655 ) ) ;
#62808=CARTESIAN_POINT ( 'NONE',  ( 1.450131233595801428, 0.1771653543307087630, 0.09757992244046791164 ) ) ;
#62809=CARTESIAN_POINT ( 'NONE',  ( -0.02624671916010428221, 0.2306618581243847221, -0.2411417322834647770 ) ) ;
#62811=CARTESIAN_POINT ( 'NONE',  ( -0.4855643044619415427, 0.05413385826771626580, -0.4176697321401330321 ) ) ;
#62812=CARTESIAN_POINT ( 'NONE',  ( -1.187664041994750175, -0.08942795157528024563, -0.3641732283464568787 ) ) ;
#62813=CARTESIAN_POINT ( 'NONE',  ( 0.4396325459317590445, -0.6692913385826771977, 0.1292274648535927661 ) ) ;
#62814=CARTESIAN_POINT ( 'NONE',  ( -0.3280839895013117347, -0.4281496062992124485, 0.4176697321401328655 ) ) ;
#62815=CARTESIAN_POINT ( 'NONE',  ( -1.220472440944878834, 2.401574803149606474, -0.5309055118110234117 ) ) ;
#62820=CARTESIAN_POINT ( 'NONE',  ( 0.5052493438320218022, -0.6692913385826773087, -0.1292274648535924053 ) ) ;
#62821=CARTESIAN_POINT ( 'NONE',  ( -0.3608923884514428360, -0.6692913385826773087, -0.1292274648535924053 ) ) ;
#62822=CARTESIAN_POINT ( 'NONE',  ( -1.246719160104985846, -0.4281496062992127816, -0.4176697321401328100 ) ) ;
#62823=CARTESIAN_POINT ( 'NONE',  ( 0.8005249343832027131, 0.05413385826771666132, 0.4176697321401328100 ) ) ;
#62824=CARTESIAN_POINT ( 'NONE',  ( 0.6167979002624679463, 0.05413385826771626580, -0.4176697321401330321 ) ) ;
#62826=CARTESIAN_POINT ( 'NONE',  ( -0.7414698162729651543, 0.2952755905511810774, -0.1292274648535930714 ) ) ;
#62827=CARTESIAN_POINT ( 'NONE',  ( 0.05249343832021075018, -0.6046776061558807314, 0.2411417322834647770 ) ) ;
#62828=CARTESIAN_POINT ( 'NONE',  ( -0.5839895013123351797, -0.6692913385826771977, 0.1292274648535927661 ) ) ;
#62829=CARTESIAN_POINT ( 'NONE',  ( 0.2559055118110243332, 0.07958543189024085140, 0.2665933059059887866 ) ) ;
#62830=CYLINDRICAL_SURFACE ( 'NONE', #35574, 1.181102362204724310 ) ;
#62832=CARTESIAN_POINT ( 'NONE',  ( -0.1115485564304456306, 0.2952755905511810774, -0.1292274648535930714 ) ) ;
#62834=CARTESIAN_POINT ( 'NONE',  ( -1.607611548556429737, 0.2952755905511810774, -0.1292274648535930714 ) ) ;
#62837=VERTEX_POINT ( 'NONE', #56031 ) ;
#62838=CARTESIAN_POINT ( 'NONE',  ( 0.6364829396325465405, -0.3162353388693409650, -0.4822834645669289433 ) ) ;
#62839=CARTESIAN_POINT ( 'NONE',  ( 0.02624671916010564918, 0.1283753931104748280, 0.1820866141732283561 ) ) ;
#62841=FACE_OUTER_BOUND ( 'NONE', #33515, .T. ) ;
#62844=CARTESIAN_POINT ( 'NONE',  ( 0.2821522309711292364, -0.6692913385826771977, 0.1292274648535927661 ) ) ;
#62845=CARTESIAN_POINT ( 'NONE',  ( -1.167979002624671470, 0.05413385826771666132, 0.4176697321401328100 ) ) ;
#62846=CARTESIAN_POINT ( 'NONE',  ( -1.095800524934382292, -0.05778040916215522460, 0.4822834645669289988 ) ) ;
#62847=CARTESIAN_POINT ( 'NONE',  ( 0.1640419947506569498, -0.05778040916215522460, 0.4822834645669289988 ) ) ;
#62848=CARTESIAN_POINT ( 'NONE',  ( 1.043307086614173818, -0.5400638737290845981, -0.3530559997133363437 ) ) ;
#62849=CARTESIAN_POINT ( 'NONE',  ( 1.469816272965879911, -0.5023911411419708095, 0.1820866141732285504 ) ) ;
#62850=CARTESIAN_POINT ( 'NONE',  ( 1.299212598425197429, -0.5511811023622047445, 6.969142054262312111E-17 ) ) ;
#62851=CARTESIAN_POINT ( 'NONE',  ( -1.036745406824146176, -0.4281496062992124485, 0.4176697321401328655 ) ) ;
#62853=CARTESIAN_POINT ( 'NONE',  ( 1.568241469816273659, -0.05778040916215560624, -0.4822834645669293319 ) ) ;
#62855=CARTESIAN_POINT ( 'NONE',  ( -0.1049868766404193215, -0.6046776061558807314, 0.2411417322834647770 ) ) ;
#62856=CARTESIAN_POINT ( 'NONE',  ( 1.043307086614173818, 0.1660481256975885056, 0.3530559997133364547 ) ) ;
#62858=CARTESIAN_POINT ( 'NONE',  ( -1.384514435695537005, 0.1771653543307087630, 0.09757992244046791164 ) ) ;
#62859=CARTESIAN_POINT ( 'NONE',  ( 0.2690288713910767848, 0.2952755905511811885, 0.1292274648535926551 ) ) ;
#62860=CARTESIAN_POINT ( 'NONE',  ( 0.8333333333333340365, 0.1771653543307087075, -0.09757992244046823083 ) ) ;
#62862=CARTESIAN_POINT ( 'NONE',  ( 0.7939632545931766261, -0.3162353388693409650, -0.4822834645669289433 ) ) ;
#62863=CARTESIAN_POINT ( 'NONE',  ( -0.4824498642376744417, -2.567464376874931580E-15, -0.4445507791589072832 ) ) ;
#62864=CARTESIAN_POINT ( 'NONE',  ( -0.6430446194225716283, -0.3690944881889763329, 0.3153832671262228327 ) ) ;
#62865=CARTESIAN_POINT ( 'NONE',  ( -0.4724409448818890911, -0.1870078740157479769, 0.4822834645669291653 ) ) ;
#62866=CARTESIAN_POINT ( 'NONE',  ( 1.450131233595801428, -0.6692913385826773087, -0.1292274648535924053 ) ) ;
#62867=EDGE_CURVE ( 'NONE', #22548, #34118, #81106, .T. ) ;
#62868=CARTESIAN_POINT ( 'NONE',  ( -0.6955380577427815458, -0.4281496062992127816, -0.4176697321401328100 ) ) ;
#62869=CARTESIAN_POINT ( 'NONE',  ( 1.364829396325460076, 0.2306618581243848609, 0.2411417322834645549 ) ) ;
#62871=CARTESIAN_POINT ( 'NONE',  ( -1.056430446194224881, -0.5511811023622046335, 0.09757992244046803654 ) ) ;
#62872=CARTESIAN_POINT ( 'NONE',  ( -0.7137454485294953965, 2.244094488188976388, 0.4917280318828573527 ) ) ;
#62873=CARTESIAN_POINT ( 'NONE',  ( 1.345144356955381593, -0.3162353388693409650, -0.4822834645669289433 ) ) ;
#62874=CIRCLE ( 'NONE', #25242, 1.220472440944881942 ) ;
#62876=CARTESIAN_POINT ( 'NONE',  ( -0.09115970038225217065, 2.409604939980833412E-17, -0.3464511005275205946 ) ) ;
#62877=CARTESIAN_POINT ( 'NONE',  ( -1.469816272965878357, 0.1283753931104748280, 0.1820866141732283561 ) ) ;
#62878=CARTESIAN_POINT ( 'NONE',  ( -0.9055118110236215490, 0.1771653543307087630, 0.000000000000000000 ) ) ;
#62879=CARTESIAN_POINT ( 'NONE',  ( 0.7988977408164235072, -1.206088964116209378E-16, 0.3791475997938230647 ) ) ;
#62880=CARTESIAN_POINT ( 'NONE',  ( -0.2165354330708654795, 0.1660481256975885056, 0.3530559997133364547 ) ) ;
#62881=CARTESIAN_POINT ( 'NONE',  ( 0.01968503937007957949, -0.4536011799217368745, -0.2665933059059886201 ) ) ;
#62882=CARTESIAN_POINT ( 'NONE',  ( -1.187664041994750175, -0.08942795157528024563, -0.3641732283464568787 ) ) ;
#62883=CARTESIAN_POINT ( 'NONE',  ( 1.417322834645670104, -0.1870078740157479769, 0.3641732283464567677 ) ) ;
#62884=CARTESIAN_POINT ( 'NONE',  ( 1.095800524934383846, -0.05778040916215560624, -0.4822834645669293319 ) ) ;
#62885=CARTESIAN_POINT ( 'NONE',  ( 1.555118110236221041, -0.5400638737290844871, 0.3530559997133364547 ) ) ;
#62886=CARTESIAN_POINT ( 'NONE',  ( 0.5446194225721792126, -0.2845877964562159024, 0.3641732283464567677 ) ) ;
#62887=CARTESIAN_POINT ( 'NONE',  ( 0.4593175853018380828, 0.05413385826771626580, -0.4176697321401330321 ) ) ;
#62888=CARTESIAN_POINT ( 'NONE',  ( 0.8792650918635177559, -0.3690944881889765550, -0.3153832671262227771 ) ) ;
#62890=CARTESIAN_POINT ( 'NONE',  ( -1.010498687664041384, 0.05413385826771666132, 0.4176697321401328100 ) ) ;
#62892=CARTESIAN_POINT ( 'NONE',  ( -1.338582677165353729, -0.1870078740157479769, 0.4822834645669291653 ) ) ;
#62893=CARTESIAN_POINT ( 'NONE',  ( -0.03280839895013062252, -0.6692913385826771977, 0.1292274648535927661 ) ) ;
#62896=CARTESIAN_POINT ( 'NONE',  ( 0.4921259842519691285, 0.1660481256975885056, 0.3530559997133364547 ) ) ;
#62897=CARTESIAN_POINT ( 'NONE',  ( 1.555118110236221041, -0.4536011799217367080, 0.2665933059059888421 ) ) ;
#62898=CARTESIAN_POINT ( 'NONE',  ( -0.1181102362204717315, -0.6692913385826771977, 8.415575281601705876E-17 ) ) ;
#62899=CARTESIAN_POINT ( 'NONE',  ( 0.2887139107611556010, -0.6046776061558807314, 0.2411417322834647770 ) ) ;
#62905=CARTESIAN_POINT ( 'NONE',  ( -0.4002624671916004129, -0.08942795157528024563, -0.3641732283464568787 ) ) ;
#62906=CARTESIAN_POINT ( 'NONE',  ( -0.7545931758530177724, 0.2952755905511811885, 0.1292274648535926551 ) ) ;
#62907=CARTESIAN_POINT ( 'NONE',  ( 0.2690288713910767848, -0.6692913385826773087, -0.1292274648535924053 ) ) ;
#62910=CARTESIAN_POINT ( 'NONE',  ( 1.017060367454068803, -0.3162353388693405765, 0.4822834645669290543 ) ) ;
#62912=CARTESIAN_POINT ( 'NONE',  ( -1.509186351706035767, -0.4281496062992124485, 0.4176697321401328655 ) ) ;
#62913=CARTESIAN_POINT ( 'NONE',  ( 0.8923884514435701520, -0.6046776061558809534, -0.2411417322834644161 ) ) ;
#62916=CARTESIAN_POINT ( 'NONE',  ( 1.587926509186352586, -0.4281496062992127816, -0.4176697321401328100 ) ) ;
#62917=CARTESIAN_POINT ( 'NONE',  ( 0.9120734908136489683, -0.6692913385826771977, 0.1292274648535927661 ) ) ;
#62918=CARTESIAN_POINT ( 'NONE',  ( 0.6955380577427828781, 0.05413385826771626580, -0.4176697321401330321 ) ) ;
#62919=CARTESIAN_POINT ( 'NONE',  ( 1.036745406824147508, -0.3690944881889765550, -0.3153832671262227771 ) ) ;
#62920=CARTESIAN_POINT ( 'NONE',  ( -1.627296587926508442, 0.1283753931104748280, 0.1820866141732283561 ) ) ;
#62921=CARTESIAN_POINT ( 'NONE',  ( -1.443569553805773564, 0.2306618581243847221, -0.2411417322834647770 ) ) ;
#62923=CARTESIAN_POINT ( 'NONE',  ( 0.6955380577427828781, -0.4281496062992124485, 0.4176697321401328655 ) ) ;
#62924=CARTESIAN_POINT ( 'NONE',  ( 1.633858267716535639, -0.4536011799217367080, 0.2665933059059888421 ) ) ;
#62925=CARTESIAN_POINT ( 'NONE',  ( -0.3083989501312330295, -0.05778040916215522460, 0.4822834645669289988 ) ) ;
#62926=CARTESIAN_POINT ( 'NONE',  ( -1.017060367454067249, -0.3162353388693409650, -0.4822834645669289433 ) ) ;
#62927=CARTESIAN_POINT ( 'NONE',  ( 1.017060367454068581, -0.05778040916215560624, -0.4822834645669293319 ) ) ;
#62932=CARTESIAN_POINT ( 'NONE',  ( -1.476377952755905110, 0.07958543189024085140, 0.2665933059059887866 ) ) ;
#62935=ORIENTED_EDGE ( 'NONE', *, *, #8539, .F. ) ;
#62937=CARTESIAN_POINT ( 'NONE',  ( 1.338582677165355062, -0.1870078740157480601, -0.3641732283464567677 ) ) ;
#62939=CARTESIAN_POINT ( 'NONE',  ( 1.371391076115485941, 0.1771653543307087630, 0.09757992244046791164 ) ) ;
#62941=DIRECTION ( 'NONE',  ( -1.000000000000000000, 0.000000000000000000, 0.000000000000000000 ) ) ;
#62944=CARTESIAN_POINT ( 'NONE',  ( -0.8267716535433065062, 0.1771653543307087630, 0.000000000000000000 ) ) ;
#62945=CARTESIAN_POINT ( 'NONE',  ( -1.207349081364828880, 0.1283753931104746893, -0.1820866141732285504 ) ) ;
#62946=CARTESIAN_POINT ( 'NONE',  ( -1.410761154855641575, -0.3162353388693409650, -0.4822834645669289433 ) ) ;
#62947=CARTESIAN_POINT ( 'NONE',  ( 0.1181102362204730916, -0.6692913385826771977, 8.415575281601705876E-17 ) ) ;
#62948=CARTESIAN_POINT ( 'NONE',  ( -1.423884514435694859, -0.05778040916215560624, -0.4822834645669293319 ) ) ;
#62950=CARTESIAN_POINT ( 'NONE',  ( 1.443569553805774897, 0.2306618581243848609, 0.2411417322834645549 ) ) ;
#62955=CARTESIAN_POINT ( 'NONE',  ( -0.3740157480314953431, 0.07958543189024085140, 0.2665933059059887866 ) ) ;
#62956=CARTESIAN_POINT ( 'NONE',  ( -1.200787401574802349, -0.5400638737290844871, 0.3530559997133364547 ) ) ;
#62957=CARTESIAN_POINT ( 'NONE',  ( 0.8923884514435703741, 0.2306618581243848609, 0.2411417322834645549 ) ) ;
#62961=CARTESIAN_POINT ( 'NONE',  ( -1.673228346456691717, 0.1660481256975883668, -0.3530559997133364547 ) ) ;
#62962=CARTESIAN_POINT ( 'NONE',  ( -1.220472440944881054, 0.2952755905511811885, 0.000000000000000000 ) ) ;
#62964=CARTESIAN_POINT ( 'NONE',  ( 0.1771653543307093182, 0.07958543189024085140, 0.2665933059059887866 ) ) ;
#62966=CARTESIAN_POINT ( 'NONE',  ( -0.5708661417322825615, -0.4536011799217367080, 0.2665933059059888421 ) ) ;
#62967=CARTESIAN_POINT ( 'NONE',  ( 0.6299212598425204535, -0.1870078740157479769, 0.3641732283464567677 ) ) ;
#62968=CARTESIAN_POINT ( 'NONE',  ( 0.5052493438320215802, 0.2952755905511811885, 0.1292274648535926551 ) ) ;
#62969=CARTESIAN_POINT ( 'NONE',  ( -0.5577427821522301654, -0.2845877964562159024, 0.3641732283464567677 ) ) ;
#62971=CARTESIAN_POINT ( 'NONE',  ( 1.318897637795276356, 0.1660481256975883668, -0.3530559997133364547 ) ) ;
#62972=CARTESIAN_POINT ( 'NONE',  ( -1.174540682414697335, -0.05778040916215522460, 0.4822834645669289988 ) ) ;
#62974=CARTESIAN_POINT ( 'NONE',  ( -0.01968503937007793844, -0.5400638737290844871, 0.3530559997133364547 ) ) ;
#62975=CARTESIAN_POINT ( 'NONE',  ( -0.4133858267716528645, -0.5400638737290844871, 0.3530559997133364547 ) ) ;
#62976=CARTESIAN_POINT ( 'NONE',  ( 1.233595800524935227, 0.1283753931104746893, -0.1820866141732285504 ) ) ;
#62977=CARTESIAN_POINT ( 'NONE',  ( 0.2099737532808405305, 0.1283753931104746893, -0.1820866141732285504 ) ) ;
#62978=CARTESIAN_POINT ( 'NONE',  ( -0.02624671916010428221, -0.6046776061558807314, 0.2411417322834647770 ) ) ;
#62979=CARTESIAN_POINT ( 'NONE',  ( -1.154855643044618851, 0.2306618581243848609, 0.2411417322834645549 ) ) ;
#62981=CARTESIAN_POINT ( 'NONE',  ( 1.561679790026247350, -0.004921259842519870586, -0.3153832671262229437 ) ) ;
#62982=CARTESIAN_POINT ( 'NONE',  ( -0.2165354330708654795, 0.1660481256975885056, 0.3530559997133364547 ) ) ;
#62983=CARTESIAN_POINT ( 'NONE',  ( -1.246719160104986512, 0.05413385826771666132, 0.4176697321401328100 ) ) ;
#62984=ORIENTED_EDGE ( 'NONE', *, *, #28526, .F. ) ;
#62986=CARTESIAN_POINT ( 'NONE',  ( 1.082677165354331228, -0.5400638737290844871, 0.3530559997133364547 ) ) ;
#62987=CARTESIAN_POINT ( 'NONE',  ( -0.6692913385826764205, -0.5511811023622047445, 6.969142054262312111E-17 ) ) ;
#62988=CARTESIAN_POINT ( 'NONE',  ( -0.5708661417322828946, 0.1660481256975883668, -0.3530559997133364547 ) ) ;
#62989=CARTESIAN_POINT ( 'NONE',  ( 1.187664041994751285, -0.05778040916215522460, 0.4822834645669289988 ) ) ;
#62990=CARTESIAN_POINT ( 'NONE',  ( 1.102362204724410155, -0.1870078740157480879, -0.4822834645669291653 ) ) ;
#62991=DIRECTION ( 'NONE',  ( 0.000000000000000000, -1.000000000000000000, 0.000000000000000000 ) ) ;
#62992=CARTESIAN_POINT ( 'NONE',  ( -1.089238845144356427, -0.004921259842519576551, 0.3153832671262227771 ) ) ;
#62997=CARTESIAN_POINT ( 'NONE',  ( 1.076115485564305141, 0.1283753931104746893, -0.1820866141732285504 ) ) ;
#62998=CARTESIAN_POINT ( 'NONE',  ( 0.5708661417322841158, -0.4536011799217368745, -0.2665933059059886201 ) ) ;
#62999=CARTESIAN_POINT ( 'NONE',  ( 0.4986876640419954376, 0.2306618581243848609, 0.2411417322834645549 ) ) ;
#63002=CARTESIAN_POINT ( 'NONE',  ( 0.6955380577427828781, -0.3690944881889763329, 0.3153832671262228327 ) ) ;
#63003=CARTESIAN_POINT ( 'NONE',  ( -0.1837270341207340729, 0.2306618581243847221, -0.2411417322834647770 ) ) ;
#63004=CARTESIAN_POINT ( 'NONE',  ( -1.049868766404198794, -0.6046776061558807314, 0.2411417322834647770 ) ) ;
#63005=CARTESIAN_POINT ( 'NONE',  ( 1.115485564304462551, -0.4281496062992127816, -0.4176697321401328100 ) ) ;
#63008=CARTESIAN_POINT ( 'NONE',  ( 0.1181102362204730916, -0.5511811023622047445, 6.969142054262312111E-17 ) ) ;
#63012=CARTESIAN_POINT ( 'NONE',  ( -0.7020997375328076329, -0.3162353388693409650, -0.4822834645669289433 ) ) ;
#63013=CARTESIAN_POINT ( 'NONE',  ( -0.7283464566929126471, -0.5400638737290844871, 0.3530559997133364547 ) ) ;
#63014=CARTESIAN_POINT ( 'NONE',  ( -0.1902887139107604098, 0.2952755905511810774, -0.1292274648535930714 ) ) ;
#63015=CARTESIAN_POINT ( 'NONE',  ( 0.2624671916010504757, 0.2306618581243848609, 0.2411417322834645549 ) ) ;
#63017=CARTESIAN_POINT ( 'NONE',  ( -0.5971128608923877978, -0.6692913385826773087, -0.1292274648535924053 ) ) ;
#63018=CARTESIAN_POINT ( 'NONE',  ( -1.253280839895012377, -0.3162353388693409650, -0.4822834645669289433 ) ) ;
#63019=CARTESIAN_POINT ( 'NONE',  ( -0.9842519685039365918, -0.6692913385826771977, 8.415575281601705876E-17 ) ) ;
#63020=CARTESIAN_POINT ( 'NONE',  ( 0.9120734908136489683, -0.6692913385826771977, 0.1292274648535927661 ) ) ;
#63022=CARTESIAN_POINT ( 'NONE',  ( -0.4461942257217840213, -0.5023911411419708095, -0.1820866141732282451 ) ) ;
#63025=ORIENTED_EDGE ( 'NONE', *, *, #31934, .F. ) ;
#63026=CARTESIAN_POINT ( 'NONE',  ( -1.167979002624671470, -0.3690944881889765550, -0.3153832671262227771 ) ) ;
#63027=CARTESIAN_POINT ( 'NONE',  ( -1.141732283464566011, 0.2952755905511811885, 0.000000000000000000 ) ) ;
#63028=CARTESIAN_POINT ( 'NONE',  ( -0.9514435695538050464, -0.05778040916215560624, -0.4822834645669293319 ) ) ;
#63030=CARTESIAN_POINT ( 'NONE',  ( -0.8267716535433065062, -0.6692913385826771977, 8.415575281601705876E-17 ) ) ;
#63031=CARTESIAN_POINT ( 'NONE',  ( -0.7939632545931754048, -0.3162353388693405765, 0.4822834645669290543 ) ) ;
#63032=CARTESIAN_POINT ( 'NONE',  ( -1.594488188976377119, 0.1660481256975883668, -0.3530559997133364547 ) ) ;
#63034=CARTESIAN_POINT ( 'NONE',  ( 0.5446194225721792126, -0.2845877964562159024, 0.3641732283464567677 ) ) ;
#63037=CARTESIAN_POINT ( 'NONE',  ( 0.06561679790026316017, -0.004921259842519870586, -0.3153832671262229437 ) ) ;
#63038=CARTESIAN_POINT ( 'NONE',  ( -0.4133858267716528645, -0.5400638737290844871, 0.3530559997133364547 ) ) ;
#63039=CARTESIAN_POINT ( 'NONE',  ( 1.476377952755906220, 0.1660481256975883668, -0.3530559997133364547 ) ) ;
#63040=CARTESIAN_POINT ( 'NONE',  ( -0.09186351706036663400, -0.4281496062992124485, 0.4176697321401328655 ) ) ;
#63046=CARTESIAN_POINT ( 'NONE',  ( -1.312335958005248715, -0.5023911411419708095, -0.1820866141732282451 ) ) ;
#63047=CARTESIAN_POINT ( 'NONE',  ( -1.581364829396324945, -0.3162353388693405765, 0.4822834645669290543 ) ) ;
#63052=CARTESIAN_POINT ( 'NONE',  ( 1.233595800524935227, 0.2306618581243847221, -0.2411417322834647770 ) ) ;
#63053=CARTESIAN_POINT ( 'NONE',  ( 0.6167979002624678353, -0.4281496062992124485, 0.4176697321401328655 ) ) ;
#63054=CARTESIAN_POINT ( 'NONE',  ( 0.2887139107611556010, 0.2306618581243847221, -0.2411417322834647770 ) ) ;
#63055=CARTESIAN_POINT ( 'NONE',  ( -1.240157480314959759, -0.4536011799217368745, -0.2665933059059886201 ) ) ;
#63056=CARTESIAN_POINT ( 'NONE',  ( -0.4265091863517051496, 0.2952755905511810774, -0.1292274648535930714 ) ) ;
#63058=CARTESIAN_POINT ( 'NONE',  ( -1.036745406824146176, 0.05413385826771626580, -0.4176697321401330321 ) ) ;
#63059=EDGE_CURVE ( 'NONE', #44871, #33221, #35451, .T. ) ;
#63061=CARTESIAN_POINT ( 'NONE',  ( 1.286089238845145033, 0.1283753931104748280, 0.1820866141732283561 ) ) ;
#63062=CARTESIAN_POINT ( 'NONE',  ( -0.2690288713910754526, 0.1771653543307087075, -0.09757992244046823083 ) ) ;
#63063=CARTESIAN_POINT ( 'NONE',  ( 1.089238845144357759, -0.004921259842519870586, -0.3153832671262229437 ) ) ;
#63064=CARTESIAN_POINT ( 'NONE',  ( -1.397637795275589623, 0.1660481256975885056, 0.3530559997133364547 ) ) ;
#63065=CARTESIAN_POINT ( 'NONE',  ( -1.233595800524933894, -0.5023911411419708095, -0.1820866141732282451 ) ) ;
#63067=CARTESIAN_POINT ( 'NONE',  ( 0.7217847769028878924, -0.004921259842519576551, 0.3153832671262227771 ) ) ;
#63068=CARTESIAN_POINT ( 'NONE',  ( -1.036745406824146176, -0.4281496062992124485, 0.4176697321401328655 ) ) ;
#63071=CARTESIAN_POINT ( 'NONE',  ( -0.09186351706036663400, -0.3690944881889763329, 0.3153832671262228327 ) ) ;
#63072=CARTESIAN_POINT ( 'NONE',  ( -1.548556430446193399, 0.1283753931104748280, 0.1820866141732283561 ) ) ;
#63073=CARTESIAN_POINT ( 'NONE',  ( 0.7152230971128616943, -0.05778040916215522460, 0.4822834645669289988 ) ) ;
#63074=CARTESIAN_POINT ( 'NONE',  ( 0.6970755509724333443, 0.02791078216816508459, -0.4328096321851889194 ) ) ;
#63075=CARTESIAN_POINT ( 'NONE',  ( 1.194225721784777594, -0.3690944881889765550, -0.3153832671262227771 ) ) ;
#63076=CARTESIAN_POINT ( 'NONE',  ( -0.9776902887139098386, -0.6692913385826771977, 0.1292274648535927661 ) ) ;
#63077=CARTESIAN_POINT ( 'NONE',  ( -0.09842519685039295696, -0.4536011799217367080, 0.2665933059059888421 ) ) ;
#63078=DIRECTION ( 'NONE',  ( 1.000000000000000000, -0.000000000000000000, -0.000000000000000000 ) ) ;
#63079=CARTESIAN_POINT ( 'NONE',  ( 0.1246719160104994284, -0.5511811023622046335, 0.09757992244046803654 ) ) ;
#63080=CARTESIAN_POINT ( 'NONE',  ( -0.9908136482939626788, -0.6692913385826773087, -0.1292274648535924053 ) ) ;
#63081=CARTESIAN_POINT ( 'NONE',  ( -0.6102362204724400829, -0.5400638737290845981, -0.3530559997133363437 ) ) ;
#63084=CARTESIAN_POINT ( 'NONE',  ( 0.4790026246719167324, -0.08942795157527998196, 0.3641732283464567121 ) ) ;
#63085=CARTESIAN_POINT ( 'NONE',  ( -0.2362204724409440182, -0.1870078740157479769, 0.4822834645669291653 ) ) ;
#63086=CARTESIAN_POINT ( 'NONE',  ( -0.8005249343832011588, 0.05413385826771626580, -0.4176697321401330321 ) ) ;
#63087=CARTESIAN_POINT ( 'NONE',  ( -0.7349081364829387342, -0.5023911411419708095, 0.1820866141732285504 ) ) ;
#63089=CARTESIAN_POINT ( 'NONE',  ( -0.2099737532808391705, 0.2306618581243848609, 0.2411417322834645549 ) ) ;
#63090=AXIS2_PLACEMENT_3D ( 'NONE', #26605, #45525, #7673 ) ;
#63091=CARTESIAN_POINT ( 'NONE',  ( -1.620734908136482577, -0.5511811023622048555, -0.09757992244046775898 ) ) ;
#63092=CARTESIAN_POINT ( 'NONE',  ( 1.614173228346457378, 0.2952755905511811885, 0.000000000000000000 ) ) ;
#63096=CARTESIAN_POINT ( 'NONE',  ( -1.450131233595799651, -0.6692913385826771977, 0.1292274648535927661 ) ) ;
#63097=CARTESIAN_POINT ( 'NONE',  ( -1.049868766404198794, 0.2306618581243847221, -0.2411417322834647770 ) ) ;
#63098=CARTESIAN_POINT ( 'NONE',  ( 1.509186351706037543, -0.4281496062992127816, -0.4176697321401328100 ) ) ;
#63100=CARTESIAN_POINT ( 'NONE',  ( 0.1450607720586929161, 2.784432375088962958E-17, -0.3464511005275205946 ) ) ;
#63101=CARTESIAN_POINT ( 'NONE',  ( 0.8070866141732289112, -0.5400638737290845981, -0.3530559997133363437 ) ) ;
#63102=CARTESIAN_POINT ( 'NONE',  ( 0.4068241469816281097, 0.05413385826771666132, 0.4176697321401328100 ) ) ;
#63105=CARTESIAN_POINT ( 'NONE',  ( 1.082677165354331228, -0.4536011799217367080, 0.2665933059059888421 ) ) ;
#63106=EDGE_CURVE ( 'NONE', #6972, #71206, #51835, .T. ) ;
#63108=ORIENTED_EDGE ( 'NONE', *, *, #58635, .T. ) ;
#63111=CARTESIAN_POINT ( 'NONE',  ( 0.5839895013123367340, -0.6692913385826773087, -0.1292274648535924053 ) ) ;
#63112=CARTESIAN_POINT ( 'NONE',  ( -0.8267716535433065062, -0.6692913385826771977, 8.415575281601705876E-17 ) ) ;
#63113=CARTESIAN_POINT ( 'NONE',  ( 1.541994750656168645, -0.6692913385826771977, 0.1292274648535927661 ) ) ;
#63114=CARTESIAN_POINT ( 'NONE',  ( 1.187664041994751285, -0.05778040916215522460, 0.4822834645669289988 ) ) ;
#63115=CARTESIAN_POINT ( 'NONE',  ( 1.535433070866142558, 0.2952755905511811885, 0.000000000000000000 ) ) ;
#63117=CARTESIAN_POINT ( 'NONE',  ( -0.2427821522309703550, -0.3162353388693405765, 0.4822834645669290543 ) ) ;
#63118=CARTESIAN_POINT ( 'NONE',  ( -1.292650918635170010, 0.2952755905511810774, -0.1292274648535930714 ) ) ;
#63119=CARTESIAN_POINT ( 'NONE',  ( -1.601049868766403650, 0.2306618581243847221, -0.2411417322834647770 ) ) ;
#63122=CARTESIAN_POINT ( 'NONE',  ( 0.8595800524934390507, -0.2845877964562159024, 0.3641732283464567677 ) ) ;
#63126=CARTESIAN_POINT ( 'NONE',  ( -0.1377952755905504645, 0.07958543189024085140, 0.2665933059059887866 ) ) ;
#63128=CARTESIAN_POINT ( 'NONE',  ( 0.7086614173228352742, -0.1870078740157480879, -0.4822834645669291653 ) ) ;
#63129=CARTESIAN_POINT ( 'NONE',  ( 0.2690288713910767848, -0.6692913385826773087, -0.1292274648535924053 ) ) ;
#63130=CARTESIAN_POINT ( 'NONE',  ( -0.4133858267716528645, 0.1660481256975883668, -0.3530559997133364547 ) ) ;
#63132=CARTESIAN_POINT ( 'NONE',  ( -1.213910761154854745, -0.6692913385826771977, 0.1292274648535927661 ) ) ;
#63134=CARTESIAN_POINT ( 'NONE',  ( 1.200787401574803681, -0.4536011799217368745, -0.2665933059059886201 ) ) ;
#63135=CARTESIAN_POINT ( 'NONE',  ( -1.561679790026246017, -0.4281496062992127816, -0.4176697321401328100 ) ) ;
#63136=CARTESIAN_POINT ( 'NONE',  ( 1.003937007874016407, -0.5400638737290844871, 0.3530559997133364547 ) ) ;
#63137=CARTESIAN_POINT ( 'NONE',  ( 0.9776902887139113929, -0.6692913385826773087, -0.1292274648535924053 ) ) ;
#63139=CARTESIAN_POINT ( 'NONE',  ( -1.377952755905511140, 0.2952755905511811885, 0.000000000000000000 ) ) ;
#63141=CARTESIAN_POINT ( 'NONE',  ( -0.1574803149606292529, -0.1870078740157479769, 0.4822834645669291653 ) ) ;
#63144=CARTESIAN_POINT ( 'NONE',  ( 1.351706036745407680, 0.05413385826771666132, 0.4176697321401328100 ) ) ;
#63145=CARTESIAN_POINT ( 'NONE',  ( 0.09186351706036827158, -0.004921259842519576551, 0.3153832671262227771 ) ) ;
#63146=CARTESIAN_POINT ( 'NONE',  ( 0.7611548556430451917, -0.6046776061558807314, 0.2411417322834647770 ) ) ;
#63148=CARTESIAN_POINT ( 'NONE',  ( 0.7283464566929143125, 0.07958543189024085140, 0.2665933059059887866 ) ) ;
#63149=CARTESIAN_POINT ( 'NONE',  ( 0.3215223097112867578, -0.05778040916215522460, 0.4822834645669289988 ) ) ;
#63151=CARTESIAN_POINT ( 'NONE',  ( -0.7939632545931754048, -0.3162353388693405765, 0.4822834645669290543 ) ) ;
#63154=CARTESIAN_POINT ( 'NONE',  ( 1.141732283464567566, 0.1771653543307087630, 0.000000000000000000 ) ) ;
#63156=CARTESIAN_POINT ( 'NONE',  ( -0.4330708661417315697, 0.2952755905511811885, 0.000000000000000000 ) ) ;
#63158=CARTESIAN_POINT ( 'NONE',  ( -0.08530183727034056085, -0.2845877964562159024, 0.3641732283464567677 ) ) ;
#63160=CARTESIAN_POINT ( 'NONE',  ( -0.5183727034120726440, -0.6692913385826773087, -0.1292274648535924053 ) ) ;
#63161=CARTESIAN_POINT ( 'NONE',  ( 0.6824146981627303710, 0.1283753931104746893, -0.1820866141732285504 ) ) ;
#63162=B_SPLINE_CURVE_WITH_KNOTS ( 'NONE', 3,
 ( #18470, #37406, #75306, #36989 ),
 .UNSPECIFIED., .F., .F.,
 ( 4, 4 ),
 ( 1.999999999897049408E-07, 0.006970199999999935128 ),
 .UNSPECIFIED. ) ;
#63164=CARTESIAN_POINT ( 'NONE',  ( 0.3477690288713918276, -0.6692913385826773087, -0.1292274648535924053 ) ) ;
#63165=CARTESIAN_POINT ( 'NONE',  ( 1.253280839895013710, -0.08942795157528024563, -0.3641732283464568787 ) ) ;
#63166=FACE_OUTER_BOUND ( 'NONE', #12505, .T. ) ;
#63167=CARTESIAN_POINT ( 'NONE',  ( -0.2624671916010490880, 0.1283753931104746893, -0.1820866141732285504 ) ) ;
#63168=CARTESIAN_POINT ( 'NONE',  ( -0.5577427821522301654, -0.08942795157528024563, -0.3641732283464568787 ) ) ;
#63169=CARTESIAN_POINT ( 'NONE',  ( -0.3018372703412066094, -0.4281496062992127816, -0.4176697321401328100 ) ) ;
#63170=CARTESIAN_POINT ( 'NONE',  ( 0.1312335958005255154, -0.6046776061558807314, 0.2411417322834647770 ) ) ;
#63171=CARTESIAN_POINT ( 'NONE',  ( 0.8530183727034128527, -0.3690944881889763329, 0.3153832671262228327 ) ) ;
#63173=CARTESIAN_POINT ( 'NONE',  ( 1.443569553805774897, 0.1283753931104748280, 0.1820866141732283561 ) ) ;
#63174=CARTESIAN_POINT ( 'NONE',  ( 0.9448818897637802916, -0.1870078740157480879, -0.4822834645669291653 ) ) ;
#63175=DIRECTION ( 'NONE',  ( -1.000000000000000000, -3.469446951953613696E-16, 0.000000000000000000 ) ) ;
#63176=CARTESIAN_POINT ( 'NONE',  ( -0.4265091863517051496, 0.2952755905511810774, -0.1292274648535930714 ) ) ;
#63178=CARTESIAN_POINT ( 'NONE',  ( 0.8202099737532814183, -0.6692913385826773087, -0.1292274648535924053 ) ) ;
#63179=CARTESIAN_POINT ( 'NONE',  ( 0.7020997375328090762, -0.3162353388693405765, 0.4822834645669290543 ) ) ;
#63181=CARTESIAN_POINT ( 'NONE',  ( 0.3477690288713918276, -0.5511811023622048555, -0.09757992244046775898 ) ) ;
#63182=CARTESIAN_POINT ( 'NONE',  ( 1.286089238845145033, -0.6046776061558809534, -0.2411417322834644161 ) ) ;
#63183=CARTESIAN_POINT ( 'NONE',  ( -0.02624671916010428221, -0.5023911411419708095, 0.1820866141732285504 ) ) ;
#63184=CARTESIAN_POINT ( 'NONE',  ( -0.4921259842519677963, 0.1660481256975883668, -0.3530559997133364547 ) ) ;
#63186=CARTESIAN_POINT ( 'NONE',  ( 0.3674540682414705883, 0.2306618581243847221, -0.2411417322834647770 ) ) ;
#63187=CARTESIAN_POINT ( 'NONE',  ( -0.6167979002624665030, -0.4281496062992127816, -0.4176697321401328100 ) ) ;
#63188=CARTESIAN_POINT ( 'NONE',  ( -0.2755905511811018171, 0.1771653543307087630, 0.000000000000000000 ) ) ;
#63189=CARTESIAN_POINT ( 'NONE',  ( 0.3871391076115492380, -0.05778040916215560624, -0.4822834645669293319 ) ) ;
#63190=CARTESIAN_POINT ( 'NONE',  ( 0.7874015748031503170, -0.1870078740157480601, -0.3641732283464567677 ) ) ;
#63191=CARTESIAN_POINT ( 'NONE',  ( -0.4527559055118102749, -0.5400638737290845981, -0.3530559997133363437 ) ) ;
#63192=CARTESIAN_POINT ( 'NONE',  ( 1.114781747626347963, 3.405574981839577511E-16, 0.3464511005275203726 ) ) ;
#63193=CARTESIAN_POINT ( 'NONE',  ( -0.9324623468618411515, 0.000000000000000000, 0.3464511005275205946 ) ) ;
#63194=CARTESIAN_POINT ( 'NONE',  ( 1.397637795275591177, -0.5400638737290844871, 0.3530559997133364547 ) ) ;
#63196=CARTESIAN_POINT ( 'NONE',  ( -1.653543307086613234, -0.1870078740157479769, 0.4822834645669291653 ) ) ;
#63197=CARTESIAN_POINT ( 'NONE',  ( -0.9842519685039365918, -0.6692913385826771977, 8.415575281601705876E-17 ) ) ;
#63202=CARTESIAN_POINT ( 'NONE',  ( 0.2887139107611556010, 0.1283753931104746893, -0.1820866141732285504 ) ) ;
#63205=CARTESIAN_POINT ( 'NONE',  ( 0.6561679790026253567, 0.2306618581243848609, 0.2411417322834645549 ) ) ;
#63207=CARTESIAN_POINT ( 'NONE',  ( -0.5622787594981818460, -5.582469467804009507E-15, -0.3954985857520081360 ) ) ;
#63208=CARTESIAN_POINT ( 'NONE',  ( -0.4724409448818890911, -0.1870078740157480601, -0.3641732283464567677 ) ) ;
#63210=CARTESIAN_POINT ( 'NONE',  ( 1.299212598425197429, -0.6692913385826771977, 8.415575281601705876E-17 ) ) ;
#63211=CARTESIAN_POINT ( 'NONE',  ( 0.9973753280839902091, 0.1283753931104746893, -0.1820866141732285504 ) ) ;
#63212=CARTESIAN_POINT ( 'NONE',  ( -0.1706036745406816491, 0.05413385826771626580, -0.4176697321401330321 ) ) ;
#63214=CARTESIAN_POINT ( 'NONE',  ( -0.5971128608923877978, -0.6692913385826773087, -0.1292274648535924053 ) ) ;
#63215=CARTESIAN_POINT ( 'NONE',  ( -1.345144356955379816, -0.08942795157528024563, -0.3641732283464568787 ) ) ;
#63216=CARTESIAN_POINT ( 'NONE',  ( -0.3871391076115479057, -0.3162353388693409650, -0.4822834645669289433 ) ) ;
#63217=CARTESIAN_POINT ( 'NONE',  ( -1.614173228346457378, 1.055049524192299693, 0.1372047244094476981 ) ) ;
#63218=DIRECTION ( 'NONE',  ( -1.196716813021146393E-16, 0.7071067811865616726, -0.7071067811865334729 ) ) ;
#63221=CARTESIAN_POINT ( 'NONE',  ( 0.6167979002624679463, 0.05413385826771626580, -0.4176697321401330321 ) ) ;
#63223=CARTESIAN_POINT ( 'NONE',  ( -0.2624671916010490880, 0.2306618581243847221, -0.2411417322834647770 ) ) ;
#63224=CARTESIAN_POINT ( 'NONE',  ( -1.404199475065615932, -0.4281496062992127816, -0.4176697321401328100 ) ) ;
#63225=CARTESIAN_POINT ( 'NONE',  ( 0.5511811023622054106, -0.1870078740157480879, -0.4822834645669291653 ) ) ;
#63226=CARTESIAN_POINT ( 'NONE',  ( -0.05905511811023545637, 0.1660481256975885056, 0.3530559997133364547 ) ) ;
#63228=CARTESIAN_POINT ( 'NONE',  ( -0.9776902887139098386, -0.6692913385826771977, 0.1292274648535927661 ) ) ;
#63229=CARTESIAN_POINT ( 'NONE',  ( 0.2493438320209980519, 0.05413385826771666132, 0.4176697321401328100 ) ) ;
#63230=CARTESIAN_POINT ( 'NONE',  ( -0.2952755905511803003, -0.5400638737290845981, -0.3530559997133363437 ) ) ;
#63231=CARTESIAN_POINT ( 'NONE',  ( 0.2952755905511819101, 0.07958543189024071263, -0.2665933059059888421 ) ) ;
#63233=CARTESIAN_POINT ( 'NONE',  ( -0.02624671916010428221, -0.6046776061558807314, 0.2411417322834647770 ) ) ;
#63234=CARTESIAN_POINT ( 'NONE',  ( -2.787279214012418738, 0.000000000000000000, 0.000000000000000000 ) ) ;
#63235=CARTESIAN_POINT ( 'NONE',  ( 1.581364829396326277, -0.05778040916215522460, 0.4822834645669289988 ) ) ;
#63239=CARTESIAN_POINT ( 'NONE',  ( 0.4724409448818904789, -0.1870078740157480879, -0.4822834645669291653 ) ) ;
#63240=CARTESIAN_POINT ( 'NONE',  ( 0.07217847769028949700, -0.08942795157528024563, -0.3641732283464568787 ) ) ;
#63241=CARTESIAN_POINT ( 'NONE',  ( 1.266404199475066328, -0.2845877964562161244, -0.3641732283464567121 ) ) ;
#63247=CARTESIAN_POINT ( 'NONE',  ( 0.2690288713910767848, -0.6692913385826773087, -0.1292274648535924053 ) ) ;
#63248=CARTESIAN_POINT ( 'NONE',  ( -1.161417322834644716, 0.1660481256975885056, 0.3530559997133364547 ) ) ;
#63249=CARTESIAN_POINT ( 'NONE',  ( -1.345144356955379816, -0.05778040916215560624, -0.4822834645669293319 ) ) ;
#63250=CARTESIAN_POINT ( 'NONE',  ( 0.1443569553805781891, -0.4281496062992124485, 0.4176697321401328655 ) ) ;
#63251=CARTESIAN_POINT ( 'NONE',  ( 0.8989501312335963501, -0.6692913385826773087, -0.1292274648535924053 ) ) ;
#63252=CARTESIAN_POINT ( 'NONE',  ( 1.476377952755906442, -0.4536011799217367080, 0.2665933059059888421 ) ) ;
#63253=CARTESIAN_POINT ( 'NONE',  ( 0.7349081364829403995, 0.1283753931104748280, 0.1820866141732283561 ) ) ;
#63254=CARTESIAN_POINT ( 'NONE',  ( -1.043307086614172041, -0.5400638737290844871, 0.3530559997133364547 ) ) ;
#63256=CARTESIAN_POINT ( 'NONE',  ( -1.568241469816272105, -0.2845877964562161244, -0.3641732283464567121 ) ) ;
#63258=CARTESIAN_POINT ( 'NONE',  ( 1.023622047244095334, -0.1870078740157479769, 0.4822834645669291653 ) ) ;
#63260=CARTESIAN_POINT ( 'NONE',  ( -1.522309711286088607, 0.1283753931104746893, -0.1820866141732285504 ) ) ;
#63261=CARTESIAN_POINT ( 'NONE',  ( 0.07874015748031558404, -0.1870078740157479769, 0.4822834645669291653 ) ) ;
#63262=CARTESIAN_POINT ( 'NONE',  ( 0.8070866141732288002, 0.07958543189024085140, 0.2665933059059887866 ) ) ;
#63263=CARTESIAN_POINT ( 'NONE',  ( -1.692913385826770645, 0.1771653543307087630, 0.000000000000000000 ) ) ;
#63264=CARTESIAN_POINT ( 'NONE',  ( 1.023622047244095334, -0.1870078740157479769, 0.4822834645669291653 ) ) ;
#63266=CARTESIAN_POINT ( 'NONE',  ( -0.3674540682414692561, -0.5023911411419708095, -0.1820866141732282451 ) ) ;
#63267=CARTESIAN_POINT ( 'NONE',  ( -0.5971128608923877978, 0.2952755905511811885, 0.1292274648535926551 ) ) ;
#63268=CARTESIAN_POINT ( 'NONE',  ( 1.423884514435696413, -0.3162353388693409650, -0.4822834645669289433 ) ) ;
#63269=CARTESIAN_POINT ( 'NONE',  ( -1.003937007874015297, -0.5400638737290845981, -0.3530559997133363437 ) ) ;
#63271=CARTESIAN_POINT ( 'NONE',  ( 1.450131233595801428, -0.6692913385826773087, -0.1292274648535924053 ) ) ;
#63273=B_SPLINE_CURVE_WITH_KNOTS ( 'NONE', 3,
 ( #56702, #43240, #25540, #81995 ),
 .UNSPECIFIED., .F., .F.,
 ( 4, 4 ),
 ( 1.040834085586084411E-17, 0.001346657832031600320 ),
 .UNSPECIFIED. ) ;
#63274=CARTESIAN_POINT ( 'NONE',  ( -1.194225721784776262, -0.3690944881889763329, 0.3153832671262228327 ) ) ;
#63276=CARTESIAN_POINT ( 'NONE',  ( 1.141732283464567566, 0.2952755905511811885, 0.000000000000000000 ) ) ;
#63278=CARTESIAN_POINT ( 'NONE',  ( -1.515748031496062076, 0.1660481256975883668, -0.3530559997133364547 ) ) ;
#63279=CARTESIAN_POINT ( 'NONE',  ( -1.633858267716534529, 0.07958543189024085140, 0.2665933059059887866 ) ) ;
#63280=CARTESIAN_POINT ( 'NONE',  ( -1.181102362204723644, -0.1870078740157480601, -0.3641732283464567677 ) ) ;
#63281=( BOUNDED_CURVE ( )  B_SPLINE_CURVE ( 2, ( #39760, #14108, #6939, #20410, #32611, #65456, #7788, #33455, #59117, #1474, #27128, #52792, #78502 ),
 .UNSPECIFIED., .F., .F. ) 
 B_SPLINE_CURVE_WITH_KNOTS ( ( 3, 2, 2, 2, 2, 2, 3 ),
 ( 0.2194878114796872115, 0.2196969696969696961, 0.2234848484848484806, 0.2272727272727272652, 0.2310606060606060497, 0.2348484848484848619, 0.2350576430657673466 ),
 .UNSPECIFIED. ) 
 CURVE ( )  GEOMETRIC_REPRESENTATION_ITEM ( )  RATIONAL_B_SPLINE_CURVE ( ( 0.9964447847208424136, 0.9981185001348094055, 1.000000000000000000, 0.9659258262890683122, 1.000000000000000000, 0.9659258262890683122, 1.000000000000000000, 0.9659258262890683122, 1.000000000000000000, 0.9659258262890683122, 1.000000000000000000, 0.9981185001348095165, 0.9964447847208426357 ) ) 
 REPRESENTATION_ITEM ( '' )  );
#63282=CARTESIAN_POINT ( 'NONE',  ( 1.541994750656168645, 0.1771653543307087075, -0.09757992244046823083 ) ) ;
#63283=CARTESIAN_POINT ( 'NONE',  ( -0.5118110236220466680, 0.2952755905511811885, 0.000000000000000000 ) ) ;
#63284=CARTESIAN_POINT ( 'NONE',  ( 0.07217847769028949700, -0.2845877964562159024, 0.3641732283464567677 ) ) ;
#63285=CARTESIAN_POINT ( 'NONE',  ( -1.450131233595799651, -0.5511811023622046335, 0.09757992244046803654 ) ) ;
#63286=CARTESIAN_POINT ( 'NONE',  ( 1.259842519685040019, -0.1870078740157479769, 0.3641732283464567677 ) ) ;
#63287=CARTESIAN_POINT ( 'NONE',  ( 0.9645669291338591078, -0.5400638737290845981, -0.3530559997133363437 ) ) ;
#63288=CARTESIAN_POINT ( 'NONE',  ( 1.535433070866142335, -0.6692913385826771977, 8.415575281601705876E-17 ) ) ;
#63289=CARTESIAN_POINT ( 'NONE',  ( 0.1574803149606306130, -0.1870078740157480601, -0.3641732283464567677 ) ) ;
#63290=CARTESIAN_POINT ( 'NONE',  ( 0.5380577427821529035, -0.4281496062992124485, 0.4176697321401328655 ) ) ;
#63292=CARTESIAN_POINT ( 'NONE',  ( 1.187664041994751285, -0.2845877964562161244, -0.3641732283464567121 ) ) ;
#63294=CARTESIAN_POINT ( 'NONE',  ( -1.489501312335957062, -0.05778040916215522460, 0.4822834645669289988 ) ) ;
#63296=CARTESIAN_POINT ( 'NONE',  ( -1.423884514435694859, -0.05778040916215560624, -0.4822834645669293319 ) ) ;
#63297=CARTESIAN_POINT ( 'NONE',  ( -0.2034120734908131112, -0.6692913385826773087, -0.1292274648535924053 ) ) ;
#63300=CARTESIAN_POINT ( 'NONE',  ( 0.3740157480314966754, 0.1660481256975883668, -0.3530559997133364547 ) ) ;
#63301=CARTESIAN_POINT ( 'NONE',  ( 1.017060367454068581, -0.08942795157528024563, -0.3641732283464568787 ) ) ;
#63302=CARTESIAN_POINT ( 'NONE',  ( -0.1837270341207340729, 0.2306618581243847221, -0.2411417322834647770 ) ) ;
#63303=CARTESIAN_POINT ( 'NONE',  ( 0.4724409448818904789, -0.1870078740157479769, 0.4822834645669291653 ) ) ;
#63307=CARTESIAN_POINT ( 'NONE',  ( -0.4824498642376744417, -2.567464376874931580E-15, -0.4445507791589072832 ) ) ;
#63309=CARTESIAN_POINT ( 'NONE',  ( -0.5446194225721777693, -0.2845877964562161244, -0.3641732283464567121 ) ) ;
#63310=CARTESIAN_POINT ( 'NONE',  ( -0.5971128608923877978, 0.2952755905511811885, 0.1292274648535926551 ) ) ;
#63312=B_SPLINE_CURVE_WITH_KNOTS ( 'NONE', 3,
 ( #12699, #25721, #38358, #32045 ),
 .UNSPECIFIED., .F., .F.,
 ( 4, 4 ),
 ( 3.593986969204291827E-07, 0.001287825409103274298 ),
 .UNSPECIFIED. ) ;
#63313=CARTESIAN_POINT ( 'NONE',  ( 0.7808398950131241190, -0.05778040916215560624, -0.4822834645669293319 ) ) ;
#63314=CARTESIAN_POINT ( 'NONE',  ( -1.404199475065615932, -0.4281496062992127816, -0.4176697321401328100 ) ) ;
#63315=CARTESIAN_POINT ( 'NONE',  ( 0.9514435695538062676, -0.05778040916215522460, 0.4822834645669289988 ) ) ;
#63318=CARTESIAN_POINT ( 'NONE',  ( 1.627296587926509996, -0.6046776061558807314, 0.2411417322834647770 ) ) ;
#63319=CARTESIAN_POINT ( 'NONE',  ( 0.8267716535433077274, 0.2952755905511811885, 0.000000000000000000 ) ) ;
#63320=CARTESIAN_POINT ( 'NONE',  ( 0.6758530183727039509, 0.2952755905511810774, -0.1292274648535930714 ) ) ;
#63321=CARTESIAN_POINT ( 'NONE',  ( 0.9908136482939640111, 0.1771653543307087075, -0.09757992244046823083 ) ) ;
#63322=CARTESIAN_POINT ( 'NONE',  ( 1.450131233595801428, -0.6692913385826773087, -0.1292274648535924053 ) ) ;
#63325=CARTESIAN_POINT ( 'NONE',  ( 0.8595800524934390507, -0.3162353388693405765, 0.4822834645669290543 ) ) ;
#63326=CARTESIAN_POINT ( 'NONE',  ( 1.673228346456693494, 0.07958543189024085140, 0.2665933059059887866 ) ) ;
#63327=CARTESIAN_POINT ( 'NONE',  ( -0.4068241469816267775, 0.05413385826771626580, -0.4176697321401330321 ) ) ;
#63328=CARTESIAN_POINT ( 'NONE',  ( -1.161417322834644716, -0.5400638737290845981, -0.3530559997133363437 ) ) ;
#63330=CARTESIAN_POINT ( 'NONE',  ( 1.010498687664042716, 0.05413385826771626580, -0.4176697321401330321 ) ) ;
#63334=CARTESIAN_POINT ( 'NONE',  ( 1.391076115485564868, 0.2306618581243847221, -0.2411417322834647770 ) ) ;
#63335=ORIENTED_EDGE ( 'NONE', *, *, #10620, .T. ) ;
#63337=ORIENTED_EDGE ( 'NONE', *, *, #22330, .F. ) ;
#63338=CARTESIAN_POINT ( 'NONE',  ( -1.604771003085130765, 0.4514378173630708146, 0.1466069496707738118 ) ) ;
#63339=CARTESIAN_POINT ( 'NONE',  ( 1.515748031496063186, -0.4536011799217368745, -0.2665933059059886201 ) ) ;
#63341=CARTESIAN_POINT ( 'NONE',  ( 1.377952755905512472, 0.1771653543307087630, 0.000000000000000000 ) ) ;
#63342=CARTESIAN_POINT ( 'NONE',  ( 0.6192220670824153395, 2.084810923686589862E-15, -0.4118477457932985253 ) ) ;
#63344=CARTESIAN_POINT ( 'NONE',  ( 0.4330708661417329575, 1.726086921369708538, 0.000000000000000000 ) ) ;
#63346=CARTESIAN_POINT ( 'NONE',  ( -0.5314960629921250401, 0.07958543189024085140, 0.2665933059059887866 ) ) ;
#63347=CARTESIAN_POINT ( 'NONE',  ( -1.587926509186350810, -0.3690944881889763329, 0.3153832671262228327 ) ) ;
#63348=CARTESIAN_POINT ( 'NONE',  ( -1.174540682414697335, -0.05778040916215522460, 0.4822834645669289988 ) ) ;
#63349=CARTESIAN_POINT ( 'NONE',  ( 0.04593175853018440641, 0.2952755905511810774, -0.1292274648535930714 ) ) ;
#63350=CARTESIAN_POINT ( 'NONE',  ( 1.607611548556431069, 0.2952755905511811885, 0.1292274648535926551 ) ) ;
#63353=CARTESIAN_POINT ( 'NONE',  ( 1.601049868766404982, 0.2306618581243848609, 0.2411417322834645549 ) ) ;
#63356=CARTESIAN_POINT ( 'NONE',  ( 1.586052503253845281, 1.023622047244095556, -0.1653254495020587966 ) ) ;
#63357=CARTESIAN_POINT ( 'NONE',  ( -0.4002624671916004129, -0.2845877964562159024, 0.3641732283464567677 ) ) ;
#63358=CARTESIAN_POINT ( 'NONE',  ( -1.246719160104985846, -0.4281496062992127816, -0.4176697321401328100 ) ) ;
#63359=CARTESIAN_POINT ( 'NONE',  ( 0.8530183727034128527, -0.4281496062992124485, 0.4176697321401328655 ) ) ;
#63360=ORIENTED_EDGE ( 'NONE', *, *, #78140, .T. ) ;
#63361=CARTESIAN_POINT ( 'NONE',  ( 0.7283464566929142014, 0.1660481256975885056, 0.3530559997133364547 ) ) ;
#63363=CARTESIAN_POINT ( 'NONE',  ( 1.102362204724410155, -0.1870078740157480879, -0.4822834645669291653 ) ) ;
#63364=CARTESIAN_POINT ( 'NONE',  ( -1.023622047244094002, -0.1870078740157480879, -0.4822834645669291653 ) ) ;
#63366=CARTESIAN_POINT ( 'NONE',  ( -0.2230971128608915943, -0.3690944881889765550, -0.3153832671262227771 ) ) ;
#63368=CARTESIAN_POINT ( 'NONE',  ( -0.3477690288713902178, 0.1771653543307087075, -0.09757992244046823083 ) ) ;
#63369=CARTESIAN_POINT ( 'NONE',  ( 0.5052493438320215802, 0.1771653543307087630, 0.09757992244046791164 ) ) ;
#63370=CARTESIAN_POINT ( 'NONE',  ( 0.3280839895013130669, 0.05413385826771666132, 0.4176697321401328100 ) ) ;
#63371=CARTESIAN_POINT ( 'NONE',  ( -0.5774278215223089816, -0.5023911411419708095, 0.1820866141732285504 ) ) ;
#63373=CARTESIAN_POINT ( 'NONE',  ( 1.220472440944882386, -0.6692913385826771977, 8.415575281601705876E-17 ) ) ;
#63374=CARTESIAN_POINT ( 'NONE',  ( -0.9055118110236215490, -0.6692913385826771977, 8.415575281601705876E-17 ) ) ;
#63376=CARTESIAN_POINT ( 'NONE',  ( -0.3805774278215216522, -0.4281496062992127816, -0.4176697321401328100 ) ) ;
#63377=CARTESIAN_POINT ( 'NONE',  ( -0.7545931758530176614, -0.6692913385826773087, -0.1292274648535924053 ) ) ;
#63378=CARTESIAN_POINT ( 'NONE',  ( 1.377952755905512472, 0.1771653543307087630, 0.000000000000000000 ) ) ;
#63379=CARTESIAN_POINT ( 'NONE',  ( 0.1181102362204730916, -0.5511811023622047445, 6.969142054262312111E-17 ) ) ;
#63380=CARTESIAN_POINT ( 'NONE',  ( -0.4986876640419942164, -0.6046776061558807314, 0.2411417322834647770 ) ) ;
#63381=CARTESIAN_POINT ( 'NONE',  ( -1.227034120734907141, -0.6692913385826773087, -0.1292274648535924053 ) ) ;
#63382=CARTESIAN_POINT ( 'NONE',  ( -0.7270051398050848546, 2.375327444609086402, 0.4916655823645582069 ) ) ;
#63383=CARTESIAN_POINT ( 'NONE',  ( 1.581364829396326277, -0.2845877964562161244, -0.3641732283464567121 ) ) ;
#63384=CARTESIAN_POINT ( 'NONE',  ( -0.4199475065616791736, -0.6046776061558807314, 0.2411417322834647770 ) ) ;
#63386=CARTESIAN_POINT ( 'NONE',  ( -1.135170603674539924, -0.6692913385826771977, 0.1292274648535927661 ) ) ;
#63389=CARTESIAN_POINT ( 'NONE',  ( 1.272965879265092637, 0.05413385826771666132, 0.4176697321401328100 ) ) ;
#63390=CARTESIAN_POINT ( 'NONE',  ( -0.7349081364829390672, 0.1283753931104746893, -0.1820866141732285504 ) ) ;
#63392=CARTESIAN_POINT ( 'NONE',  ( -0.9055118110236215490, 0.2952755905511811885, 0.000000000000000000 ) ) ;
#63393=CARTESIAN_POINT ( 'NONE',  ( 1.220472440944882608, 0.2952755905511811885, 0.000000000000000000 ) ) ;
#63394=CARTESIAN_POINT ( 'NONE',  ( 0.8792650918635177559, 0.05413385826771666132, 0.4176697321401328100 ) ) ;
#63396=CARTESIAN_POINT ( 'NONE',  ( -1.272965879265091305, -0.3690944881889763329, 0.3153832671262228327 ) ) ;
#63401=CARTESIAN_POINT ( 'NONE',  ( 1.266404199475066328, -0.2845877964562161244, -0.3641732283464567121 ) ) ;
#63402=CARTESIAN_POINT ( 'NONE',  ( 0.9251968503937015864, -0.4536011799217367080, 0.2665933059059888421 ) ) ;
#63403=CARTESIAN_POINT ( 'NONE',  ( 0.4658792650918640033, -0.3162353388693405765, 0.4822834645669290543 ) ) ;
#63404=CARTESIAN_POINT ( 'NONE',  ( 0.4606732211678724598, 1.763126522798933227, -0.5309055118110237448 ) ) ;
#63406=CARTESIAN_POINT ( 'NONE',  ( 0.9908136482939640111, -0.5511811023622046335, 0.09757992244046803654 ) ) ;
#63407=( BOUNDED_SURFACE ( )  B_SPLINE_SURFACE ( 1, 2, ( 
 ( #31331, #11995, #10760, #63326, #57413, #44358, #17906, #43955, #43128, #62924, #23787, #56996, #17498, #17087, #56588, #75973, #49458, #69651, #37649, #81470, #5258, #62506, #82693, #49865, #11173, #30922, #36833, #4435, #24195, #38062, #25012, #81884, #43542, #36420, #42724, #69241, #50685, #4844, #30519, #18313, #70049, #76383, #82289, #12404, #68420, #63738, #75565, #56181, #31751, #23374, #49042, #74739, #77632, #25425, #78473, #38479, #51090, #64997, #38894, #20797, #76787, #6910, #26266, #46453, #19119, #32582, #14082, #51927, #65839, #1445, #189, #77206, #72146, #14502, #58245, #6496, #8172, #64163, #13656, #40155, #39734, #44768, #33837, #70895, #33429, #32166, #7332, #33000, #59090, #70465, #83106, #19535, #12822, #78051, #65430, #13245, #57822, #25842, #51502, #45192, #64573, #610, #19964, #46032, #45615, #71309, #39309, #27102, #58670, #1035, #20380, #26689, #52344, #71727, #7763, #52764, #21622, #60750, #14907, #47282, #67082, #72560, #10249, #74227, #3102, #54429, #80139, #2690, #2274, #42218, #72972, #53175, #67913, #47700, #28767, #80554, #73396, #40989, #48119, #15746, #59504, #16572, #40567, #41801, #22040, #22461, #73817, #66248, #27937, #15324, #16154, #53595, #67492, #9414, #41400, #59919, #35084, #1857, #66668, #35499, #79304, #27519, #22866, #21211, #9828, #3514, #8587, #61163, #29183, #54851, #48527, #78890, #46866, #34258, #9007, #34679, #60342, #28350, #54011, #79723, #30828, #69555, #61996, #82599, #24916, #76291, #49359, #23275, #43441, #16988, #18217, #50584, #5571, #69956, #29999, #43033, #36727, #68729, #4333, #55663, #5164, #69139, #75468, #36322, #17808, #35920, #75056, #11903, #81372, #18622, #56903, #80960, #11490, #63231, #68328, #75875, #37144, #37557, #44265, #62829, #56493, #82195, #24512, #23685, #62403, #31236, #49768, #50180, #43852, #61586, #17403, #3932, #29590, #55253, #11069, #48945, #74646, #42631, #10666, #4742, #30415, #56083, #81788, #24099, #13150, #19443, #38382, #6398, #33340, #27009, #45093, #19025, #78377, #76691, #26169, #52670, #52251, #63643, #59002, #92, #45934, #44673, #19870, #45520, #71633, #83008, #7669, #32068, #37967, #7236, #26599, #25745, #25329, #12723, #70368, #20708, #64059, #1357, #31653, #58576, #46361, #50993, #70797, #13985, #77110, #51408, #32910, #12310, #71215, #64476, #57729, #38800, #6813, #13558, #32484, #58147, #39214, #516, #5982, #57310, #64899, #941, #77957, #51830, #77535, #20285, #39641, #65332, #48025, #15232, #2599, #28676, #40892, #34164, #47608, #66573, #16064, #80047, #59410, #41307, #72883, #21949, #28257, #27423, #46781, #40480, #73303, #53918, #79631, #66993, #72472, #54337, #22366, #73725, #8498, #33748, #34583, #1766, #9325, #72054, #3009, #14411, #66158, #53508, #21532, #27847, #14821, #59826, #40065, #65752, #47191, #2180, #8085, #79216, #15651, #53085, #78797, #8907, #21121, #60251, #34995, #60660, #71484, #13831, #14256, #51260, #59260, #57998, #6245, #58851, #78225, #77380, #76962, #64328, #12995, #20969, #38651, #52934, #83274, #26858, #1617, #19291, #71065, #65603, #45370, #19711, #1208, #14671, #39490, #32756, #44942, #6664, #26018, #65177, #70639, #51677, #7514, #32336, #63909, #78647, #33183, #52517, #20558, #7085, #362, #46628, #13409, #57583, #72324, #52097, #46210, #27273, #77806, #39064, #71905, #20137, #31922, #25597, #64747, #39914, #26444, #7934, #33595, #58423, #784, #45785, #52302, #13613, #33387, #78008, #7719, #78845, #59050, #20758, #1404, #64530, #34213, #77589, #6867, #46408, #20336, #59876, #32536, #45988, #65384, #2230, #58200, #71684, #53134, #27060, #21578, #40529, #39267, #53555, #27895, #78430, #72102, #1814, #14460, #64949, #39693, #8547, #52719, #65799, #33798, #72519, #7289, #79263, #47240, #72930, #14036, #26221, #40112, #19923, #21172, #38850, #568, #51884, #32959, #8133, #59463, #27476, #58626, #993, #45573, #71266, #46827, #26648, #14867, #66208, #29136, #29950, #55206, #66621, #36276, #3055, #48897, #21995, #22822, #48480, #74599, #2647, #10619, #9370, #40942, #10204, #29544, #28721, #28304, #15700, #47656 ),
 ( #67448, #79678, #41357, #60706, #16528, #53966, #54384, #74181, #73352, #49309, #55614, #42172, #35873, #61539, #41753, #67038, #81325, #80094, #8959, #23639, #3470, #67867, #61948, #54803, #22414, #3884, #80507, #15281, #34633, #35041, #80914, #61118, #23227, #16942, #48071, #73773, #16109, #42583, #9782, #68284, #4288, #60297, #35453, #56850, #75010, #30782, #50946, #75417, #32020, #12673, #36678, #50535, #18974, #24050, #31601, #82548, #76643, #70318, #38332, #5115, #11440, #37507, #63182, #68680, #57680, #82960, #64008, #17761, #50127, #12260, #25278, #5520, #44216, #69906, #44623, #69092, #6349, #11022, #63594, #5929, #81741, #31186, #18573, #30366, #42, #57261, #25695, #62354, #17357, #42985, #4692, #69505, #37917, #37096, #24867, #43392, #56033, #62781, #49721, #76239, #56443, #82146, #24461, #75827, #18168, #43801, #11854, #8034, #77904, #45467, #58950, #58096, #6761, #52200, #66107, #53033, #26547, #71581, #64427, #45044, #13932, #33698, #71165, #461, #46310, #46729, #59358, #1308, #33289, #64846, #26117, #45883, #7184, #20235, #1717, #39589, #26957, #65278, #77059, #72421, #32433, #19392, #52620, #32855, #14770, #70745, #58524, #7617, #40426, #13097, #889, #65704, #78326, #34113, #78746, #51778, #8443, #77483, #59774, #13505, #20657, #19818, #39161, #27372, #21071, #2129, #38750, #72004, #14360, #40017, #51356, #48383, #34533, #41259, #79578, #74498, #10523, #66523, #68184, #15599, #47140, #35769, #66945, #16845, #61020, #8855, #42479, #10105, #16428, #15181, #67769, #61850, #23132, #22313, #74082, #47557, #67354, #28207, #61439, #21894, #21482, #3371, #29035, #53866, #42074, #3786, #2549, #41663, #9277, #29449, #54283, #73250, #35358, #60198, #34948, #28625, #36177, #55108, #2960, #47976, #40838, #72831, #73675, #80817, #60611, #79999, #22724, #48800, #27797, #54706, #9687, #16017, #80412, #53457, #79165, #56350, #44124, #24364, #69409, #82051, #29854, #82863, #42888, #55517, #11763, #43294, #25185, #81225, #11340, #30689, #50852, #23541, #37000, #18482, #50034, #70217, #5831, #4596, #18880, #30267, #76552, #23954, #62679, #10924, #49622, #69816, #12165, #44529, #49210, #75316, #5021, #68583, #37821, #24771, #36581, #17663, #55931, #12574, #38231, #62260, #4191, #68991, #74914, #63497, #75731, #17260, #37417, #81646, #18071, #43706, #63089, #5427, #31089, #56756, #82456, #31504, #50440, #76141, #57164, #2345, #15388, #78959, #34324, #59986, #66735, #57997, #9074, #57582, #53661, #79368, #70638, #21278, #8653, #28001, #19289, #54075, #47350, #21687, #51259, #73039, #15816, #60405, #59568, #41050, #1512, #46933, #64327, #34745, #27166, #83273, #14973, #66314, #6663, #2756, #28415, #38650, #72625, #20865, #79790, #8238, #52828, #40632, #12994, #44941, #65902, #22106, #47766, #40220, #1924, #76961, #25596, #27587, #73464, #78540, #32335, #63908, #6244, #31921, #46515, #72217, #14568, #33904, #53244, #54912, #10318, #81440, #61653, #23341, #35983, #67150, #36798, #80205, #9479, #49012, #80618, #62474, #35154, #48596, #67976, #4809, #60814, #74292, #55732, #3994, #24165, #43098, #41868, #56150, #67562, #30485, #61228, #16638, #48184, #3581, #23754, #49428, #81854, #3166, #29248, #42278, #22522, #75122, #62062, #73881, #22930, #9894, #49834, #75533, #16221, #41465, #29658, #28830, #17467, #55320, #54494, #74709, #35565, #81029, #17055, #42695, #68392, #10731, #36388, #4401, #68794, #30069, #11139, #76354, #38445, #51470, #31718, #70432, #12789, #19504, #11965, #45158, #11556, #6463, #32133, #24577, #57378, #83073, #31301, #75940, #12373, #56965, #70020, #57790, #38031, #25394, #63706, #43507, #13213, #56558, #69207, #51058, #82663, #38859, #37213, #24978, #44329, #64540, #62892, #50651, #157, #6046, #577, #70862, #18281, #32547, #43923, #6877, #37620, #18686, #50244, #63296, #25810, #77173, #58211, #5227, #5634, #76758, #82259, #26231, #64128, #69620, #19088, #44737, #51894, #17873, #30891, #34642, #65394, #13624, #2239, #33397, #40951, #27485, #72939, #15291, #7729, #14048, #40122, #65809, #71275, #60307, #27904, #66631, #20346, #52729, #14878 ) ),
 .UNSPECIFIED., .F., .F., .F. ) 
 B_SPLINE_SURFACE_WITH_KNOTS ( ( 2, 2 ),
 ( 3, 2, 2, 2, 2, 2, 2, 2, 2, 2, 2, 2, 2, 2, 2, 2, 2, 2, 2, 2, 2, 2, 2, 2, 2, 2, 2, 2, 2, 2, 2, 2, 2, 2, 2, 2, 2, 2, 2, 2, 2, 2, 2, 2, 2, 2, 2, 2, 2, 2, 2, 2, 2, 2, 2, 2, 2, 2, 2, 2, 2, 2, 2, 2, 2, 2, 2, 2, 2, 2, 2, 2, 2, 2, 2, 2, 2, 2, 2, 2, 2, 2, 2, 2, 2, 2, 2, 2, 2, 2, 2, 2, 2, 2, 2, 2, 2, 2, 2, 2, 2, 2, 2, 2, 2, 2, 2, 2, 2, 2, 2, 2, 2, 2, 2, 2, 2, 2, 2, 2, 2, 2, 2, 2, 2, 2, 2, 2, 2, 2, 2, 2, 2, 2, 2, 2, 2, 2, 2, 2, 2, 2, 2, 2, 2, 2, 2, 2, 2, 2, 2, 2, 2, 2, 2, 2, 2, 2, 2, 2, 2, 2, 2, 2, 2, 2, 2, 2, 2, 2, 2, 2, 2, 2, 2, 2, 2, 2, 2, 2, 2, 2, 2, 2, 2, 2, 2, 2, 2, 2, 2, 2, 2, 2, 2, 2, 2, 2, 2, 2, 2, 2, 2, 2, 2, 2, 2, 2, 2, 2, 2, 2, 2, 2, 2, 2, 2, 2, 2, 2, 2, 2, 2, 2, 2, 2, 2, 2, 2, 2, 2, 2, 2, 2, 2, 2, 2, 2, 2, 2, 2, 2, 2, 2, 2, 2, 2, 2, 2, 2, 2, 2, 2, 2, 2, 3 ),
 ( 0.000000000000000000, 1.000000000000000000 ),
 ( 0.000000000000000000, 0.003787878787878787984, 0.007575757575757575968, 0.01136363636363636395, 0.01515151515151515194, 0.01893939393939393992, 0.02272727272727272790, 0.02651515151515151589, 0.03030303030303030387, 0.03409090909090908839, 0.03787878787878787984, 0.04166666666666666435, 0.04545454545454545581, 0.04924242424242424032, 0.05303030303030303177, 0.05681818181818181629, 0.06060606060606060774, 0.06439393939393939226, 0.06818181818181817677, 0.07196969696969697516, 0.07575757575757575968, 0.07954545454545454419, 0.08333333333333332871, 0.08712121212121212710, 0.09090909090909091161, 0.09469696969696969613, 0.09848484848484848064, 0.1022727272727272790, 0.1060606060606060635, 0.1098484848484848481, 0.1136363636363636326, 0.1174242424242424310, 0.1212121212121212155, 0.1250000000000000000, 0.1287878787878787845, 0.1325757575757575690, 0.1363636363636363535, 0.1401515151515151381, 0.1439393939393939503, 0.1477272727272727348, 0.1515151515151515194, 0.1553030303030303039, 0.1590909090909090884, 0.1628787878787878729, 0.1666666666666666574, 0.1704545454545454419, 0.1742424242424242542, 0.1780303030303030387, 0.1818181818181818232, 0.1856060606060606077, 0.1893939393939393923, 0.1931818181818181768, 0.1969696969696969613, 0.2007575757575757458, 0.2045454545454545581, 0.2083333333333333426, 0.2121212121212121271, 0.2159090909090909116, 0.2196969696969696961, 0.2234848484848484806, 0.2272727272727272652, 0.2310606060606060497, 0.2348484848484848619, 0.2386363636363636465, 0.2424242424242424310, 0.2462121212121212155, 0.2500000000000000000, 0.2537878787878787845, 0.2575757575757575690, 0.2613636363636363535, 0.2651515151515151381, 0.2689393939393939226, 0.2727272727272727071, 0.2765151515151514916, 0.2803030303030302761, 0.2840909090909091161, 0.2878787878787879007, 0.2916666666666666852, 0.2954545454545454697, 0.2992424242424242542, 0.3030303030303030387, 0.3068181818181818232, 0.3106060606060606077, 0.3143939393939393923, 0.3181818181818181768, 0.3219696969696969613, 0.3257575757575757458, 0.3295454545454545303, 0.3333333333333333148, 0.3371212121212120993, 0.3409090909090908839, 0.3446969696969697239, 0.3484848484848485084, 0.3522727272727272929, 0.3560606060606060774, 0.3598484848484848619, 0.3636363636363636465, 0.3674242424242424310, 0.3712121212121212155, 0.3750000000000000000, 0.3787878787878787845, 0.3825757575757575690, 0.3863636363636363535, 0.3901515151515151381, 0.3939393939393939226, 0.3977272727272727071, 0.4015151515151514916, 0.4053030303030302761, 0.4090909090909091161, 0.4128787878787879007, 0.4166666666666666852, 0.4204545454545454697, 0.4242424242424242542, 0.4280303030303030387, 0.4318181818181818232, 0.4356060606060606077, 0.4393939393939393923, 0.4431818181818181768, 0.4469696969696969613, 0.4507575757575757458, 0.4545454545454545303, 0.4583333333333333148, 0.4621212121212120993, 0.4659090909090908839, 0.4696969696969697239, 0.4734848484848485084, 0.4772727272727272929, 0.4810606060606060774, 0.4848484848484848619, 0.4886363636363636465, 0.4924242424242424310, 0.4962121212121212155, 0.5000000000000000000, 0.5037878787878787845, 0.5075757575757575690, 0.5113636363636363535, 0.5151515151515151381, 0.5189393939393939226, 0.5227272727272727071, 0.5265151515151514916, 0.5303030303030302761, 0.5340909090909090606, 0.5378787878787878451, 0.5416666666666666297, 0.5454545454545454142, 0.5492424242424241987, 0.5530303030303029832, 0.5568181818181817677, 0.5606060606060605522, 0.5643939393939394478, 0.5681818181818182323, 0.5719696969696970168, 0.5757575757575758013, 0.5795454545454545858, 0.5833333333333333703, 0.5871212121212121549, 0.5909090909090909394, 0.5946969696969697239, 0.5984848484848485084, 0.6022727272727272929, 0.6060606060606060774, 0.6098484848484848619, 0.6136363636363636465, 0.6174242424242424310, 0.6212121212121212155, 0.6250000000000000000, 0.6287878787878787845, 0.6325757575757575690, 0.6363636363636363535, 0.6401515151515151381, 0.6439393939393939226, 0.6477272727272727071, 0.6515151515151514916, 0.6553030303030302761, 0.6590909090909090606, 0.6628787878787878451, 0.6666666666666666297, 0.6704545454545454142, 0.6742424242424241987, 0.6780303030303029832, 0.6818181818181817677, 0.6856060606060605522, 0.6893939393939394478, 0.6931818181818182323, 0.6969696969696970168, 0.7007575757575758013, 0.7045454545454545858, 0.7083333333333333703, 0.7121212121212121549, 0.7159090909090909394, 0.7196969696969697239, 0.7234848484848485084, 0.7272727272727272929, 0.7310606060606060774, 0.7348484848484848619, 0.7386363636363636465, 0.7424242424242424310, 0.7462121212121212155, 0.7500000000000000000, 0.7537878787878787845, 0.7575757575757575690, 0.7613636363636363535, 0.7651515151515151381, 0.7689393939393939226, 0.7727272727272727071, 0.7765151515151514916, 0.7803030303030302761, 0.7840909090909090606, 0.7878787878787878451, 0.7916666666666666297, 0.7954545454545454142, 0.7992424242424241987, 0.8030303030303029832, 0.8068181818181817677, 0.8106060606060605522, 0.8143939393939394478, 0.8181818181818182323, 0.8219696969696970168, 0.8257575757575758013, 0.8295454545454545858, 0.8333333333333333703, 0.8371212121212121549, 0.8409090909090909394, 0.8446969696969697239, 0.8484848484848485084, 0.8522727272727272929, 0.8560606060606060774, 0.8598484848484848619, 0.8636363636363636465, 0.8674242424242424310, 0.8712121212121212155, 0.8750000000000000000, 0.8787878787878787845, 0.8825757575757575690, 0.8863636363636363535, 0.8901515151515151381, 0.8939393939393939226, 0.8977272727272727071, 0.9015151515151514916, 0.9053030303030302761, 0.9090909090909090606, 0.9128787878787878451, 0.9166666666666666297, 0.9204545454545454142, 0.9242424242424241987, 0.9280303030303029832, 0.9318181818181817677, 0.9356060606060605522, 0.9393939393939394478, 0.9431818181818182323, 0.9469696969696970168, 0.9507575757575758013, 0.9545454545454545858, 0.9583333333333333703, 0.9621212121212121549, 0.9659090909090909394 ),
 .UNSPECIFIED. ) 
 GEOMETRIC_REPRESENTATION_ITEM ( )  RATIONAL_B_SPLINE_SURFACE ( (
 ( 1.000000000000000000, 0.9659258262890683122, 1.000000000000000000, 0.9659258262890683122, 1.000000000000000000, 0.9659258262890683122, 1.000000000000000000, 0.9659258262890683122, 1.000000000000000000, 0.9659258262890683122, 1.000000000000000000, 0.9659258262890683122, 1.000000000000000000, 0.9659258262890683122, 1.000000000000000000, 0.9659258262890683122, 1.000000000000000000, 0.9659258262890683122, 1.000000000000000000, 0.9659258262890683122, 1.000000000000000000, 0.9659258262890683122, 1.000000000000000000, 0.9659258262890683122, 1.000000000000000000, 0.9659258262890683122, 1.000000000000000000, 0.9659258262890683122, 1.000000000000000000, 0.9659258262890683122, 1.000000000000000000, 0.9659258262890683122, 1.000000000000000000, 0.9659258262890683122, 1.000000000000000000, 0.9659258262890683122, 1.000000000000000000, 0.9659258262890683122, 1.000000000000000000, 0.9659258262890683122, 1.000000000000000000, 0.9659258262890683122, 1.000000000000000000, 0.9659258262890683122, 1.000000000000000000, 0.9659258262890683122, 1.000000000000000000, 0.9659258262890683122, 1.000000000000000000, 0.9659258262890683122, 1.000000000000000000, 0.9659258262890683122, 1.000000000000000000, 0.9659258262890683122, 1.000000000000000000, 0.9659258262890683122, 1.000000000000000000, 0.9659258262890683122, 1.000000000000000000, 0.9659258262890683122, 1.000000000000000000, 0.9659258262890683122, 1.000000000000000000, 0.9659258262890683122, 1.000000000000000000, 0.9659258262890683122, 1.000000000000000000, 0.9659258262890683122, 1.000000000000000000, 0.9659258262890683122, 1.000000000000000000, 0.9659258262890683122, 1.000000000000000000, 0.9659258262890683122, 1.000000000000000000, 0.9659258262890683122, 1.000000000000000000, 0.9659258262890683122, 1.000000000000000000, 0.9659258262890683122, 1.000000000000000000, 0.9659258262890683122, 1.000000000000000000, 0.9659258262890683122, 1.000000000000000000, 0.9659258262890683122, 1.000000000000000000, 0.9659258262890683122, 1.000000000000000000, 0.9659258262890683122, 1.000000000000000000, 0.9659258262890683122, 1.000000000000000000, 0.9659258262890683122, 1.000000000000000000, 0.9659258262890683122, 1.000000000000000000, 0.9659258262890683122, 1.000000000000000000, 0.9659258262890683122, 1.000000000000000000, 0.9659258262890683122, 1.000000000000000000, 0.9659258262890683122, 1.000000000000000000, 0.9659258262890683122, 1.000000000000000000, 0.9659258262890683122, 1.000000000000000000, 0.9659258262890683122, 1.000000000000000000, 0.9659258262890683122, 1.000000000000000000, 0.9659258262890683122, 1.000000000000000000, 0.9659258262890683122, 1.000000000000000000, 0.9659258262890683122, 1.000000000000000000, 0.9659258262890683122, 1.000000000000000000, 0.9659258262890683122, 1.000000000000000000, 0.9659258262890683122, 1.000000000000000000, 0.9659258262890683122, 1.000000000000000000, 0.9659258262890683122, 1.000000000000000000, 0.9659258262890683122, 1.000000000000000000, 0.9659258262890683122, 1.000000000000000000, 0.9659258262890683122, 1.000000000000000000, 0.9659258262890683122, 1.000000000000000000, 0.9659258262890683122, 1.000000000000000000, 0.9659258262890683122, 1.000000000000000000, 0.9659258262890683122, 1.000000000000000000, 0.9659258262890683122, 1.000000000000000000, 0.9659258262890683122, 1.000000000000000000, 0.9659258262890683122, 1.000000000000000000, 0.9659258262890683122, 1.000000000000000000, 0.9659258262890683122, 1.000000000000000000, 0.9659258262890683122, 1.000000000000000000, 0.9659258262890683122, 1.000000000000000000, 0.9659258262890683122, 1.000000000000000000, 0.9659258262890683122, 1.000000000000000000, 0.9659258262890683122, 1.000000000000000000, 0.9659258262890683122, 1.000000000000000000, 0.9659258262890683122, 1.000000000000000000, 0.9659258262890683122, 1.000000000000000000, 0.9659258262890683122, 1.000000000000000000, 0.9659258262890683122, 1.000000000000000000, 0.9659258262890683122, 1.000000000000000000, 0.9659258262890683122, 1.000000000000000000, 0.9659258262890683122, 1.000000000000000000, 0.9659258262890683122, 1.000000000000000000, 0.9659258262890683122, 1.000000000000000000, 0.9659258262890683122, 1.000000000000000000, 0.9659258262890683122, 1.000000000000000000, 0.9659258262890683122, 1.000000000000000000, 0.9659258262890683122, 1.000000000000000000, 0.9659258262890683122, 1.000000000000000000, 0.9659258262890683122, 1.000000000000000000, 0.9659258262890683122, 1.000000000000000000, 0.9659258262890683122, 1.000000000000000000, 0.9659258262890683122, 1.000000000000000000, 0.9659258262890683122, 1.000000000000000000, 0.9659258262890683122, 1.000000000000000000, 0.9659258262890683122, 1.000000000000000000, 0.9659258262890683122, 1.000000000000000000, 0.9659258262890683122, 1.000000000000000000, 0.9659258262890683122, 1.000000000000000000, 0.9659258262890683122, 1.000000000000000000, 0.9659258262890683122, 1.000000000000000000, 0.9659258262890683122, 1.000000000000000000, 0.9659258262890683122, 1.000000000000000000, 0.9659258262890683122, 1.000000000000000000, 0.9659258262890683122, 1.000000000000000000, 0.9659258262890683122, 1.000000000000000000, 0.9659258262890683122, 1.000000000000000000, 0.9659258262890683122, 1.000000000000000000, 0.9659258262890683122, 1.000000000000000000, 0.9659258262890683122, 1.000000000000000000, 0.9659258262890683122, 1.000000000000000000, 0.9659258262890683122, 1.000000000000000000, 0.9659258262890683122, 1.000000000000000000, 0.9659258262890683122, 1.000000000000000000, 0.9659258262890683122, 1.000000000000000000, 0.9659258262890683122, 1.000000000000000000, 0.9659258262890683122, 1.000000000000000000, 0.9659258262890683122, 1.000000000000000000, 0.9659258262890683122, 1.000000000000000000, 0.9659258262890683122, 1.000000000000000000, 0.9659258262890683122, 1.000000000000000000, 0.9659258262890683122, 1.000000000000000000, 0.9659258262890683122, 1.000000000000000000, 0.9659258262890683122, 1.000000000000000000, 0.9659258262890683122, 1.000000000000000000, 0.9659258262890683122, 1.000000000000000000, 0.9659258262890683122, 1.000000000000000000, 0.9659258262890683122, 1.000000000000000000, 0.9659258262890683122, 1.000000000000000000, 0.9659258262890683122, 1.000000000000000000, 0.9659258262890683122, 1.000000000000000000, 0.9659258262890683122, 1.000000000000000000, 0.9659258262890683122, 1.000000000000000000, 0.9659258262890683122, 1.000000000000000000, 0.9659258262890683122, 1.000000000000000000, 0.9659258262890683122, 1.000000000000000000, 0.9659258262890683122, 1.000000000000000000, 0.9659258262890683122, 1.000000000000000000, 0.9659258262890683122, 1.000000000000000000, 0.9659258262890683122, 1.000000000000000000, 0.9659258262890683122, 1.000000000000000000, 0.9659258262890683122, 1.000000000000000000, 0.9659258262890683122, 1.000000000000000000, 0.9659258262890683122, 1.000000000000000000, 0.9659258262890683122, 1.000000000000000000, 0.9659258262890683122, 1.000000000000000000, 0.9659258262890683122, 1.000000000000000000, 0.9659258262890683122, 1.000000000000000000, 0.9659258262890683122, 1.000000000000000000, 0.9659258262890683122, 1.000000000000000000, 0.9659258262890683122, 1.000000000000000000, 0.9659258262890683122, 1.000000000000000000, 0.9659258262890683122, 1.000000000000000000, 0.9659258262890683122, 1.000000000000000000, 0.9659258262890683122, 1.000000000000000000, 0.9659258262890683122, 1.000000000000000000, 0.9659258262890683122, 1.000000000000000000, 0.9659258262890683122, 1.000000000000000000, 0.9659258262890683122, 1.000000000000000000, 0.9659258262890683122, 1.000000000000000000, 0.9659258262890683122, 1.000000000000000000, 0.9659258262890683122, 1.000000000000000000, 0.9659258262890683122, 1.000000000000000000, 0.9659258262890683122, 1.000000000000000000, 0.9659258262890683122, 1.000000000000000000, 0.9659258262890683122, 1.000000000000000000, 0.9659258262890683122, 1.000000000000000000, 0.9659258262890683122, 1.000000000000000000, 0.9659258262890683122, 1.000000000000000000, 0.9659258262890683122, 1.000000000000000000, 0.9659258262890683122, 1.000000000000000000, 0.9659258262890683122, 1.000000000000000000, 0.9659258262890683122, 1.000000000000000000, 0.9659258262890683122, 1.000000000000000000, 0.9659258262890683122, 1.000000000000000000, 0.9659258262890683122, 1.000000000000000000, 0.9659258262890683122, 1.000000000000000000, 0.9659258262890683122, 1.000000000000000000, 0.9659258262890683122, 1.000000000000000000, 0.9659258262890683122, 1.000000000000000000, 0.9659258262890683122, 1.000000000000000000, 0.9659258262890683122, 1.000000000000000000, 0.9659258262890683122, 1.000000000000000000, 0.9659258262890683122, 1.000000000000000000, 0.9659258262890683122, 1.000000000000000000, 0.9659258262890683122, 1.000000000000000000, 0.9659258262890683122, 1.000000000000000000, 0.9659258262890683122, 1.000000000000000000, 0.9659258262890683122, 1.000000000000000000, 0.9659258262890683122, 1.000000000000000000, 0.9659258262890683122, 1.000000000000000000, 0.9659258262890683122, 1.000000000000000000, 0.9659258262890683122, 1.000000000000000000, 0.9659258262890683122, 1.000000000000000000, 0.9659258262890683122, 1.000000000000000000, 0.9659258262890683122, 1.000000000000000000, 0.9659258262890683122, 1.000000000000000000, 0.9659258262890683122, 1.000000000000000000, 0.9659258262890683122, 1.000000000000000000, 0.9659258262890683122, 1.000000000000000000, 0.9659258262890683122, 1.000000000000000000, 0.9659258262890683122, 1.000000000000000000, 0.9659258262890683122, 1.000000000000000000, 0.9659258262890683122, 1.000000000000000000, 0.9659258262890683122, 1.000000000000000000, 0.9659258262890683122, 1.000000000000000000, 0.9659258262890683122, 1.000000000000000000, 0.9659258262890683122, 1.000000000000000000, 0.9659258262890683122, 1.000000000000000000, 0.9659258262890683122, 1.000000000000000000, 0.9659258262890683122, 1.000000000000000000, 0.9659258262890683122, 1.000000000000000000, 0.9659258262890683122, 1.000000000000000000, 0.9659258262890683122, 1.000000000000000000, 0.9659258262890683122, 1.000000000000000000, 0.9659258262890683122, 1.000000000000000000, 0.9659258262890683122, 1.000000000000000000, 0.9659258262890683122, 1.000000000000000000, 0.9659258262890683122, 1.000000000000000000, 0.9659258262890683122, 1.000000000000000000, 0.9659258262890683122, 1.000000000000000000, 0.9659258262890683122, 1.000000000000000000, 0.9659258262890683122, 1.000000000000000000, 0.9659258262890683122, 1.000000000000000000, 0.9659258262890683122, 1.000000000000000000, 0.9659258262890683122, 1.000000000000000000, 0.9659258262890683122, 1.000000000000000000, 0.9659258262890683122, 1.000000000000000000, 0.9659258262890683122, 1.000000000000000000, 0.9659258262890683122, 1.000000000000000000, 0.9659258262890683122, 1.000000000000000000, 0.9659258262890683122, 1.000000000000000000, 0.9659258262890683122, 1.000000000000000000, 0.9659258262890683122, 1.000000000000000000, 0.9659258262890683122, 1.000000000000000000, 0.9659258262890683122, 1.000000000000000000, 0.9659258262890683122, 1.000000000000000000, 0.9659258262890683122, 1.000000000000000000, 0.9659258262890683122, 1.000000000000000000, 0.9659258262890683122, 1.000000000000000000, 0.9659258262890683122, 1.000000000000000000, 0.9659258262890683122, 1.000000000000000000, 0.9659258262890683122, 1.000000000000000000, 0.9659258262890683122, 1.000000000000000000, 0.9659258262890683122, 1.000000000000000000, 0.9659258262890683122, 1.000000000000000000, 0.9659258262890683122, 1.000000000000000000, 0.9659258262890683122, 1.000000000000000000),
 ( 1.000000000000000000, 0.9659258262890683122, 1.000000000000000000, 0.9659258262890683122, 1.000000000000000000, 0.9659258262890683122, 1.000000000000000000, 0.9659258262890683122, 1.000000000000000000, 0.9659258262890683122, 1.000000000000000000, 0.9659258262890683122, 1.000000000000000000, 0.9659258262890683122, 1.000000000000000000, 0.9659258262890683122, 1.000000000000000000, 0.9659258262890683122, 1.000000000000000000, 0.9659258262890683122, 1.000000000000000000, 0.9659258262890683122, 1.000000000000000000, 0.9659258262890683122, 1.000000000000000000, 0.9659258262890683122, 1.000000000000000000, 0.9659258262890683122, 1.000000000000000000, 0.9659258262890683122, 1.000000000000000000, 0.9659258262890683122, 1.000000000000000000, 0.9659258262890683122, 1.000000000000000000, 0.9659258262890683122, 1.000000000000000000, 0.9659258262890683122, 1.000000000000000000, 0.9659258262890683122, 1.000000000000000000, 0.9659258262890683122, 1.000000000000000000, 0.9659258262890683122, 1.000000000000000000, 0.9659258262890683122, 1.000000000000000000, 0.9659258262890683122, 1.000000000000000000, 0.9659258262890683122, 1.000000000000000000, 0.9659258262890683122, 1.000000000000000000, 0.9659258262890683122, 1.000000000000000000, 0.9659258262890683122, 1.000000000000000000, 0.9659258262890683122, 1.000000000000000000, 0.9659258262890683122, 1.000000000000000000, 0.9659258262890683122, 1.000000000000000000, 0.9659258262890683122, 1.000000000000000000, 0.9659258262890683122, 1.000000000000000000, 0.9659258262890683122, 1.000000000000000000, 0.9659258262890683122, 1.000000000000000000, 0.9659258262890683122, 1.000000000000000000, 0.9659258262890683122, 1.000000000000000000, 0.9659258262890683122, 1.000000000000000000, 0.9659258262890683122, 1.000000000000000000, 0.9659258262890683122, 1.000000000000000000, 0.9659258262890683122, 1.000000000000000000, 0.9659258262890683122, 1.000000000000000000, 0.9659258262890683122, 1.000000000000000000, 0.9659258262890683122, 1.000000000000000000, 0.9659258262890683122, 1.000000000000000000, 0.9659258262890683122, 1.000000000000000000, 0.9659258262890683122, 1.000000000000000000, 0.9659258262890683122, 1.000000000000000000, 0.9659258262890683122, 1.000000000000000000, 0.9659258262890683122, 1.000000000000000000, 0.9659258262890683122, 1.000000000000000000, 0.9659258262890683122, 1.000000000000000000, 0.9659258262890683122, 1.000000000000000000, 0.9659258262890683122, 1.000000000000000000, 0.9659258262890683122, 1.000000000000000000, 0.9659258262890683122, 1.000000000000000000, 0.9659258262890683122, 1.000000000000000000, 0.9659258262890683122, 1.000000000000000000, 0.9659258262890683122, 1.000000000000000000, 0.9659258262890683122, 1.000000000000000000, 0.9659258262890683122, 1.000000000000000000, 0.9659258262890683122, 1.000000000000000000, 0.9659258262890683122, 1.000000000000000000, 0.9659258262890683122, 1.000000000000000000, 0.9659258262890683122, 1.000000000000000000, 0.9659258262890683122, 1.000000000000000000, 0.9659258262890683122, 1.000000000000000000, 0.9659258262890683122, 1.000000000000000000, 0.9659258262890683122, 1.000000000000000000, 0.9659258262890683122, 1.000000000000000000, 0.9659258262890683122, 1.000000000000000000, 0.9659258262890683122, 1.000000000000000000, 0.9659258262890683122, 1.000000000000000000, 0.9659258262890683122, 1.000000000000000000, 0.9659258262890683122, 1.000000000000000000, 0.9659258262890683122, 1.000000000000000000, 0.9659258262890683122, 1.000000000000000000, 0.9659258262890683122, 1.000000000000000000, 0.9659258262890683122, 1.000000000000000000, 0.9659258262890683122, 1.000000000000000000, 0.9659258262890683122, 1.000000000000000000, 0.9659258262890683122, 1.000000000000000000, 0.9659258262890683122, 1.000000000000000000, 0.9659258262890683122, 1.000000000000000000, 0.9659258262890683122, 1.000000000000000000, 0.9659258262890683122, 1.000000000000000000, 0.9659258262890683122, 1.000000000000000000, 0.9659258262890683122, 1.000000000000000000, 0.9659258262890683122, 1.000000000000000000, 0.9659258262890683122, 1.000000000000000000, 0.9659258262890683122, 1.000000000000000000, 0.9659258262890683122, 1.000000000000000000, 0.9659258262890683122, 1.000000000000000000, 0.9659258262890683122, 1.000000000000000000, 0.9659258262890683122, 1.000000000000000000, 0.9659258262890683122, 1.000000000000000000, 0.9659258262890683122, 1.000000000000000000, 0.9659258262890683122, 1.000000000000000000, 0.9659258262890683122, 1.000000000000000000, 0.9659258262890683122, 1.000000000000000000, 0.9659258262890683122, 1.000000000000000000, 0.9659258262890683122, 1.000000000000000000, 0.9659258262890683122, 1.000000000000000000, 0.9659258262890683122, 1.000000000000000000, 0.9659258262890683122, 1.000000000000000000, 0.9659258262890683122, 1.000000000000000000, 0.9659258262890683122, 1.000000000000000000, 0.9659258262890683122, 1.000000000000000000, 0.9659258262890683122, 1.000000000000000000, 0.9659258262890683122, 1.000000000000000000, 0.9659258262890683122, 1.000000000000000000, 0.9659258262890683122, 1.000000000000000000, 0.9659258262890683122, 1.000000000000000000, 0.9659258262890683122, 1.000000000000000000, 0.9659258262890683122, 1.000000000000000000, 0.9659258262890683122, 1.000000000000000000, 0.9659258262890683122, 1.000000000000000000, 0.9659258262890683122, 1.000000000000000000, 0.9659258262890683122, 1.000000000000000000, 0.9659258262890683122, 1.000000000000000000, 0.9659258262890683122, 1.000000000000000000, 0.9659258262890683122, 1.000000000000000000, 0.9659258262890683122, 1.000000000000000000, 0.9659258262890683122, 1.000000000000000000, 0.9659258262890683122, 1.000000000000000000, 0.9659258262890683122, 1.000000000000000000, 0.9659258262890683122, 1.000000000000000000, 0.9659258262890683122, 1.000000000000000000, 0.9659258262890683122, 1.000000000000000000, 0.9659258262890683122, 1.000000000000000000, 0.9659258262890683122, 1.000000000000000000, 0.9659258262890683122, 1.000000000000000000, 0.9659258262890683122, 1.000000000000000000, 0.9659258262890683122, 1.000000000000000000, 0.9659258262890683122, 1.000000000000000000, 0.9659258262890683122, 1.000000000000000000, 0.9659258262890683122, 1.000000000000000000, 0.9659258262890683122, 1.000000000000000000, 0.9659258262890683122, 1.000000000000000000, 0.9659258262890683122, 1.000000000000000000, 0.9659258262890683122, 1.000000000000000000, 0.9659258262890683122, 1.000000000000000000, 0.9659258262890683122, 1.000000000000000000, 0.9659258262890683122, 1.000000000000000000, 0.9659258262890683122, 1.000000000000000000, 0.9659258262890683122, 1.000000000000000000, 0.9659258262890683122, 1.000000000000000000, 0.9659258262890683122, 1.000000000000000000, 0.9659258262890683122, 1.000000000000000000, 0.9659258262890683122, 1.000000000000000000, 0.9659258262890683122, 1.000000000000000000, 0.9659258262890683122, 1.000000000000000000, 0.9659258262890683122, 1.000000000000000000, 0.9659258262890683122, 1.000000000000000000, 0.9659258262890683122, 1.000000000000000000, 0.9659258262890683122, 1.000000000000000000, 0.9659258262890683122, 1.000000000000000000, 0.9659258262890683122, 1.000000000000000000, 0.9659258262890683122, 1.000000000000000000, 0.9659258262890683122, 1.000000000000000000, 0.9659258262890683122, 1.000000000000000000, 0.9659258262890683122, 1.000000000000000000, 0.9659258262890683122, 1.000000000000000000, 0.9659258262890683122, 1.000000000000000000, 0.9659258262890683122, 1.000000000000000000, 0.9659258262890683122, 1.000000000000000000, 0.9659258262890683122, 1.000000000000000000, 0.9659258262890683122, 1.000000000000000000, 0.9659258262890683122, 1.000000000000000000, 0.9659258262890683122, 1.000000000000000000, 0.9659258262890683122, 1.000000000000000000, 0.9659258262890683122, 1.000000000000000000, 0.9659258262890683122, 1.000000000000000000, 0.9659258262890683122, 1.000000000000000000, 0.9659258262890683122, 1.000000000000000000, 0.9659258262890683122, 1.000000000000000000, 0.9659258262890683122, 1.000000000000000000, 0.9659258262890683122, 1.000000000000000000, 0.9659258262890683122, 1.000000000000000000, 0.9659258262890683122, 1.000000000000000000, 0.9659258262890683122, 1.000000000000000000, 0.9659258262890683122, 1.000000000000000000, 0.9659258262890683122, 1.000000000000000000, 0.9659258262890683122, 1.000000000000000000, 0.9659258262890683122, 1.000000000000000000, 0.9659258262890683122, 1.000000000000000000, 0.9659258262890683122, 1.000000000000000000, 0.9659258262890683122, 1.000000000000000000, 0.9659258262890683122, 1.000000000000000000, 0.9659258262890683122, 1.000000000000000000, 0.9659258262890683122, 1.000000000000000000, 0.9659258262890683122, 1.000000000000000000, 0.9659258262890683122, 1.000000000000000000, 0.9659258262890683122, 1.000000000000000000, 0.9659258262890683122, 1.000000000000000000, 0.9659258262890683122, 1.000000000000000000, 0.9659258262890683122, 1.000000000000000000, 0.9659258262890683122, 1.000000000000000000, 0.9659258262890683122, 1.000000000000000000, 0.9659258262890683122, 1.000000000000000000, 0.9659258262890683122, 1.000000000000000000, 0.9659258262890683122, 1.000000000000000000, 0.9659258262890683122, 1.000000000000000000, 0.9659258262890683122, 1.000000000000000000, 0.9659258262890683122, 1.000000000000000000, 0.9659258262890683122, 1.000000000000000000, 0.9659258262890683122, 1.000000000000000000, 0.9659258262890683122, 1.000000000000000000, 0.9659258262890683122, 1.000000000000000000, 0.9659258262890683122, 1.000000000000000000, 0.9659258262890683122, 1.000000000000000000, 0.9659258262890683122, 1.000000000000000000, 0.9659258262890683122, 1.000000000000000000, 0.9659258262890683122, 1.000000000000000000, 0.9659258262890683122, 1.000000000000000000, 0.9659258262890683122, 1.000000000000000000, 0.9659258262890683122, 1.000000000000000000, 0.9659258262890683122, 1.000000000000000000, 0.9659258262890683122, 1.000000000000000000, 0.9659258262890683122, 1.000000000000000000, 0.9659258262890683122, 1.000000000000000000, 0.9659258262890683122, 1.000000000000000000, 0.9659258262890683122, 1.000000000000000000, 0.9659258262890683122, 1.000000000000000000, 0.9659258262890683122, 1.000000000000000000, 0.9659258262890683122, 1.000000000000000000, 0.9659258262890683122, 1.000000000000000000, 0.9659258262890683122, 1.000000000000000000, 0.9659258262890683122, 1.000000000000000000, 0.9659258262890683122, 1.000000000000000000, 0.9659258262890683122, 1.000000000000000000, 0.9659258262890683122, 1.000000000000000000, 0.9659258262890683122, 1.000000000000000000, 0.9659258262890683122, 1.000000000000000000, 0.9659258262890683122, 1.000000000000000000, 0.9659258262890683122, 1.000000000000000000, 0.9659258262890683122, 1.000000000000000000, 0.9659258262890683122, 1.000000000000000000, 0.9659258262890683122, 1.000000000000000000, 0.9659258262890683122, 1.000000000000000000, 0.9659258262890683122, 1.000000000000000000, 0.9659258262890683122, 1.000000000000000000, 0.9659258262890683122, 1.000000000000000000, 0.9659258262890683122, 1.000000000000000000, 0.9659258262890683122, 1.000000000000000000, 0.9659258262890683122, 1.000000000000000000, 0.9659258262890683122, 1.000000000000000000, 0.9659258262890683122, 1.000000000000000000, 0.9659258262890683122, 1.000000000000000000, 0.9659258262890683122, 1.000000000000000000, 0.9659258262890683122, 1.000000000000000000, 0.9659258262890683122, 1.000000000000000000, 0.9659258262890683122, 1.000000000000000000, 0.9659258262890683122, 1.000000000000000000, 0.9659258262890683122, 1.000000000000000000) ) ) 
 REPRESENTATION_ITEM ( '' )  SURFACE ( )  );
#63408=CARTESIAN_POINT ( 'NONE',  ( -0.2887139107611542133, -0.6046776061558809534, -0.2411417322834644161 ) ) ;
#63409=CARTESIAN_POINT ( 'NONE',  ( -1.338582677165353729, -0.1870078740157479769, 0.4822834645669291653 ) ) ;
#63410=CARTESIAN_POINT ( 'NONE',  ( 1.364829396325460076, 0.2306618581243848609, 0.2411417322834645549 ) ) ;
#63413=CARTESIAN_POINT ( 'NONE',  ( -0.2034120734908131112, -0.5511811023622048555, -0.09757992244046775898 ) ) ;
#63416=CARTESIAN_POINT ( 'NONE',  ( -0.8005249343832013809, -0.4281496062992124485, 0.4176697321401328655 ) ) ;
#63417=CARTESIAN_POINT ( 'NONE',  ( -0.5971128608923877978, -0.6692913385826773087, -0.1292274648535924053 ) ) ;
#63418=CARTESIAN_POINT ( 'NONE',  ( -0.8464566929133852113, 0.07958543189024085140, 0.2665933059059887866 ) ) ;
#63419=CARTESIAN_POINT ( 'NONE',  ( -0.5905511811023613777, -0.6692913385826771977, 8.415575281601705876E-17 ) ) ;
#63420=CARTESIAN_POINT ( 'NONE',  ( 0.3149606299212606708, -0.1870078740157480879, -0.4822834645669291653 ) ) ;
#63421=CARTESIAN_POINT ( 'NONE',  ( -0.2887139107611542133, -0.6046776061558809534, -0.2411417322834644161 ) ) ;
#63422=CARTESIAN_POINT ( 'NONE',  ( -1.410761154855641575, -0.3162353388693409650, -0.4822834645669289433 ) ) ;
#63423=CARTESIAN_POINT ( 'NONE',  ( -0.8005249343832013809, -0.4281496062992124485, 0.4176697321401328655 ) ) ;
#63424=CARTESIAN_POINT ( 'NONE',  ( 0.6496062992125991586, 0.1660481256975885056, 0.3530559997133364547 ) ) ;
#63428=CARTESIAN_POINT ( 'NONE',  ( -0.3346456692913377662, 0.07958543189024071263, -0.2665933059059888421 ) ) ;
#63431=ORIENTED_EDGE ( 'NONE', *, *, #34823, .T. ) ;
#63432=CARTESIAN_POINT ( 'NONE',  ( -1.325459317585300889, -0.3690944881889765550, -0.3153832671262227771 ) ) ;
#63433=CARTESIAN_POINT ( 'NONE',  ( -1.246719160104985846, -0.4281496062992127816, -0.4176697321401328100 ) ) ;
#63434=CARTESIAN_POINT ( 'NONE',  ( -0.7677165354330699465, -0.5400638737290845981, -0.3530559997133363437 ) ) ;
#63436=CARTESIAN_POINT ( 'NONE',  ( -1.325459317585300889, -0.4281496062992127816, -0.4176697321401328100 ) ) ;
#63437=CARTESIAN_POINT ( 'NONE',  ( -1.003937007874015297, -0.5400638737290845981, -0.3530559997133363437 ) ) ;
#63438=CARTESIAN_POINT ( 'NONE',  ( -1.581364829396324945, -0.05778040916215560624, -0.4822834645669293319 ) ) ;
#63439=CARTESIAN_POINT ( 'NONE',  ( -1.719160104986876103, 0.05413385826771666132, 0.4176697321401328100 ) ) ;
#63440=CARTESIAN_POINT ( 'NONE',  ( 0.3674540682414705883, -0.5023911411419708095, 0.1820866141732285504 ) ) ;
#63443=CARTESIAN_POINT ( 'NONE',  ( 0.08530183727034192087, -0.2845877964562161244, -0.3641732283464567121 ) ) ;
#63444=CARTESIAN_POINT ( 'NONE',  ( -0.4855643044619415427, 0.05413385826771626580, -0.4176697321401330321 ) ) ;
#63445=CARTESIAN_POINT ( 'NONE',  ( 1.456692913385827515, 0.2952755905511811885, 0.000000000000000000 ) ) ;
#63446=CARTESIAN_POINT ( 'NONE',  ( -0.3412073490813641308, 0.2306618581243847221, -0.2411417322834647770 ) ) ;
#63450=ORIENTED_EDGE ( 'NONE', *, *, #62163, .F. ) ;
#63452=CARTESIAN_POINT ( 'NONE',  ( -0.7152230971128602510, -0.3162353388693405765, 0.4822834645669290543 ) ) ;
#63454=CARTESIAN_POINT ( 'NONE',  ( 1.351706036745407458, -0.4281496062992127816, -0.4176697321401328100 ) ) ;
#63455=CARTESIAN_POINT ( 'NONE',  ( -0.9580052493438311334, -0.3690944881889763329, 0.3153832671262228327 ) ) ;
#63456=CARTESIAN_POINT ( 'NONE',  ( -1.377952755905511140, 0.2952755905511811885, 0.000000000000000000 ) ) ;
#63461=CARTESIAN_POINT ( 'NONE',  ( 1.128608923884515169, -0.6046776061558809534, -0.2411417322834644161 ) ) ;
#63463=CARTESIAN_POINT ( 'NONE',  ( 0.05905511811023709395, -0.5400638737290844871, 0.3530559997133364547 ) ) ;
#63464=CARTESIAN_POINT ( 'NONE',  ( -1.194225721784776262, -0.3690944881889763329, 0.3153832671262228327 ) ) ;
#63465=CARTESIAN_POINT ( 'NONE',  ( -0.2034120734908131112, -0.6692913385826773087, -0.1292274648535924053 ) ) ;
#63468=CARTESIAN_POINT ( 'NONE',  ( -0.7480314960629914633, 0.2952755905511811885, 0.000000000000000000 ) ) ;
#63470=CARTESIAN_POINT ( 'NONE',  ( 0.6889763779527563470, 0.07958543189024071263, -0.2665933059059888421 ) ) ;
#63471=CARTESIAN_POINT ( 'NONE',  ( -0.2165354330708654795, -0.4536011799217368745, -0.2665933059059886201 ) ) ;
#63472=CARTESIAN_POINT ( 'NONE',  ( 0.8070866141732289112, -0.4536011799217368745, -0.2665933059059886201 ) ) ;
#63473=CARTESIAN_POINT ( 'NONE',  ( -1.607611548556429737, -0.6692913385826771977, 0.1292274648535927661 ) ) ;
#63474=CARTESIAN_POINT ( 'NONE',  ( 1.371391076115485719, -0.6692913385826773087, -0.1292274648535924053 ) ) ;
#63475=CARTESIAN_POINT ( 'NONE',  ( 0.4921259842519691285, -0.4536011799217368745, -0.2665933059059886201 ) ) ;
#63476=CARTESIAN_POINT ( 'NONE',  ( -0.9973753280839886548, 0.2306618581243848609, 0.2411417322834645549 ) ) ;
#63477=CARTESIAN_POINT ( 'NONE',  ( 1.266404199475066328, -0.05778040916215522460, 0.4822834645669289988 ) ) ;
#63480=CARTESIAN_POINT ( 'NONE',  ( -0.1049868766404193215, -0.5023911411419708095, 0.1820866141732285504 ) ) ;
#63481=CARTESIAN_POINT ( 'NONE',  ( 0.1674892343164159914, -2.191421614605370878E-15, 0.4445507791589071167 ) ) ;
#63482=CARTESIAN_POINT ( 'NONE',  ( 0.3280839895013130669, -0.4281496062992127816, -0.4176697321401328100 ) ) ;
#63484=CARTESIAN_POINT ( 'NONE',  ( 1.482939632545932307, -0.004921259842519870586, -0.3153832671262229437 ) ) ;
#63485=CARTESIAN_POINT ( 'NONE',  ( -1.463254593175852492, -0.6692913385826773087, -0.1292274648535924053 ) ) ;
#63486=CARTESIAN_POINT ( 'NONE',  ( -0.4461942257217840213, -0.5023911411419708095, -0.1820866141732282451 ) ) ;
#63488=CARTESIAN_POINT ( 'NONE',  ( -1.003937007874015297, -0.5400638737290845981, -0.3530559997133363437 ) ) ;
#63489=CARTESIAN_POINT ( 'NONE',  ( -0.7152230971128602510, -0.3162353388693405765, 0.4822834645669290543 ) ) ;
#63492=CARTESIAN_POINT ( 'NONE',  ( 0.5314960629921264834, 0.07958543189024071263, -0.2665933059059888421 ) ) ;
#63493=CARTESIAN_POINT ( 'NONE',  ( -0.5183727034120726440, 0.2952755905511811885, 0.1292274648535926551 ) ) ;
#63494=CARTESIAN_POINT ( 'NONE',  ( -0.6364829396325453192, -0.05778040916215560624, -0.4822834645669293319 ) ) ;
#63495=CARTESIAN_POINT ( 'NONE',  ( -0.9251968503937002541, -0.4536011799217368745, -0.2665933059059886201 ) ) ;
#63496=CARTESIAN_POINT ( 'NONE',  ( 0.6199123404867349363, 8.471767977567108961E-16, -0.4445507791589058955 ) ) ;
#63497=CARTESIAN_POINT ( 'NONE',  ( -0.1640419947506553400, -0.05778040916215560624, -0.4822834645669293319 ) ) ;
#63498=B_SPLINE_CURVE_WITH_KNOTS ( 'NONE', 3,
 ( #9816, #54417, #41389, #16977, #54838, #80128, #74216 ),
 .UNSPECIFIED., .F., .F.,
 ( 4, 3, 4 ),
 ( 1.735570302229820823E-18, 0.001246230184515536828, 0.002492489877932635954 ),
 .UNSPECIFIED. ) ;
#63499=PLANE ( 'NONE',  #65666 ) ;
#63500=CARTESIAN_POINT ( 'NONE',  ( 1.089238845144357537, -0.4281496062992124485, 0.4176697321401328655 ) ) ;
#63506=CARTESIAN_POINT ( 'NONE',  ( -1.358267716535432434, 0.1660481256975883668, -0.3530559997133364547 ) ) ;
#63508=CARTESIAN_POINT ( 'NONE',  ( -0.6889763779527552368, -0.5400638737290845981, -0.3530559997133363437 ) ) ;
#63510=CARTESIAN_POINT ( 'NONE',  ( 1.469816272965879911, 0.2306618581243847221, -0.2411417322834647770 ) ) ;
#63513=CARTESIAN_POINT ( 'NONE',  ( 1.017060367454068803, -0.3162353388693405765, 0.4822834645669290543 ) ) ;
#63514=CARTESIAN_POINT ( 'NONE',  ( 0.08530183727034192087, -0.05778040916215522460, 0.4822834645669289988 ) ) ;
#63517=CARTESIAN_POINT ( 'NONE',  ( 1.305774278215223960, 0.1771653543307087075, -0.09757992244046823083 ) ) ;
#63519=EDGE_LOOP ( 'NONE', ( #31941, #62005, #49757, #68445, #68110 ) ) ;
#63522=CARTESIAN_POINT ( 'NONE',  ( 0.5971128608923890191, -0.6692913385826771977, 0.1292274648535927661 ) ) ;
#63523=CARTESIAN_POINT ( 'NONE',  ( -0.7349081364829390672, 0.2306618581243847221, -0.2411417322834647770 ) ) ;
#63524=CARTESIAN_POINT ( 'NONE',  ( 1.568241469816273437, -0.3162353388693405765, 0.4822834645669290543 ) ) ;
#63525=CARTESIAN_POINT ( 'NONE',  ( 0.7545931758530189937, 0.2952755905511810774, -0.1292274648535930714 ) ) ;
#63526=CARTESIAN_POINT ( 'NONE',  ( -1.509186351706035767, -0.3690944881889763329, 0.3153832671262228327 ) ) ;
#63527=CARTESIAN_POINT ( 'NONE',  ( 1.614173228346457378, 0.2952755905511811885, 0.000000000000000000 ) ) ;
#63528=CARTESIAN_POINT ( 'NONE',  ( -0.1968503937007867743, 0.2952755905511811885, 0.000000000000000000 ) ) ;
#63529=CARTESIAN_POINT ( 'NONE',  ( -1.463254593175852492, 0.2952755905511811885, 0.1292274648535926551 ) ) ;
#63530=CARTESIAN_POINT ( 'NONE',  ( 1.587926509186352142, 0.05413385826771666132, 0.4176697321401328100 ) ) ;
#63533=CARTESIAN_POINT ( 'NONE',  ( 0.7677165354330716118, 0.07958543189024071263, -0.2665933059059888421 ) ) ;
#63534=ORIENTED_EDGE ( 'NONE', *, *, #46886, .T. ) ;
#63536=ORIENTED_EDGE ( 'NONE', *, *, #24986, .T. ) ;
#63537=CARTESIAN_POINT ( 'NONE',  ( -0.2230971128608915943, -0.3690944881889765550, -0.3153832671262227771 ) ) ;
#63539=CARTESIAN_POINT ( 'NONE',  ( 0.3412073490813655186, 0.2306618581243848609, 0.2411417322834645549 ) ) ;
#63540=CARTESIAN_POINT ( 'NONE',  ( 0.4199475065616803948, -0.6046776061558809534, -0.2411417322834644161 ) ) ;
#63541=CARTESIAN_POINT ( 'NONE',  ( -0.6364829396325453192, -0.3162353388693405765, 0.4822834645669290543 ) ) ;
#63543=CARTESIAN_POINT ( 'NONE',  ( -1.049868766404198794, -0.6046776061558807314, 0.2411417322834647770 ) ) ;
#63545=CARTESIAN_POINT ( 'NONE',  ( 1.515748031496063186, -0.4536011799217368745, -0.2665933059059886201 ) ) ;
#63546=CARTESIAN_POINT ( 'NONE',  ( 0.7152230971128616943, -0.05778040916215522460, 0.4822834645669289988 ) ) ;
#63547=CARTESIAN_POINT ( 'NONE',  ( 1.161417322834646493, -0.5400638737290844871, 0.3530559997133364547 ) ) ;
#63549=CARTESIAN_POINT ( 'NONE',  ( -1.312335958005248715, -0.6046776061558809534, -0.2411417322834644161 ) ) ;
#63552=CARTESIAN_POINT ( 'NONE',  ( -0.3018372703412066094, 0.05413385826771666132, 0.4176697321401328100 ) ) ;
#63556=CARTESIAN_POINT ( 'NONE',  ( 1.095800524934383846, -0.3162353388693405765, 0.4822834645669290543 ) ) ;
#63557=CARTESIAN_POINT ( 'NONE',  ( 1.259842519685040019, -0.1870078740157480879, -0.4822834645669291653 ) ) ;
#63558=CARTESIAN_POINT ( 'NONE',  ( 0.07217847769028949700, -0.2845877964562159024, 0.3641732283464567677 ) ) ;
#63559=CARTESIAN_POINT ( 'NONE',  ( 0.7152230971128614723, -0.3162353388693409650, -0.4822834645669289433 ) ) ;
#63561=CARTESIAN_POINT ( 'NONE',  ( 0.3346456692913393205, -0.4536011799217368745, -0.2665933059059886201 ) ) ;
#63562=CARTESIAN_POINT ( 'NONE',  ( 0.2624671916010504757, -0.6046776061558809534, -0.2411417322834644161 ) ) ;
#63563=CONICAL_SURFACE ( 'NONE', #60923, 1.181102362204724310, 0.7853981633974621568 ) ;
#63565=CARTESIAN_POINT ( 'NONE',  ( -0.8858267716535425107, 0.1660481256975883668, -0.3530559997133364547 ) ) ;
#63566=CARTESIAN_POINT ( 'NONE',  ( 1.036745406824147508, -0.3690944881889765550, -0.3153832671262227771 ) ) ;
#63567=DIRECTION ( 'NONE',  ( 1.000000000000000000, 0.000000000000000000, 0.000000000000000000 ) ) ;
#63568=CARTESIAN_POINT ( 'NONE',  ( -0.4265091863517051496, 0.2952755905511810774, -0.1292274648535930714 ) ) ;
#63569=CARTESIAN_POINT ( 'NONE',  ( 0.1049868766404206816, 0.1283753931104748280, 0.1820866141732283561 ) ) ;
#63571=CARTESIAN_POINT ( 'NONE',  ( -0.3083989501312330295, -0.05778040916215522460, 0.4822834645669289988 ) ) ;
#63572=CARTESIAN_POINT ( 'NONE',  ( 0.2624671916010504757, -0.5023911411419708095, -0.1820866141732282451 ) ) ;
#63574=CARTESIAN_POINT ( 'NONE',  ( 0.2296587926509192634, -0.3162353388693405765, 0.4822834645669290543 ) ) ;
#63575=CARTESIAN_POINT ( 'NONE',  ( 1.115485564304462551, -0.3690944881889765550, -0.3153832671262227771 ) ) ;
#63576=CARTESIAN_POINT ( 'NONE',  ( 0.3817677560323445296, -4.069555009745408348E-17, -0.3627989612356148363 ) ) ;
#63577=CARTESIAN_POINT ( 'NONE',  ( -0.3083989501312330295, -0.08942795157527998196, 0.3641732283464567121 ) ) ;
#63579=CARTESIAN_POINT ( 'NONE',  ( -0.8595800524934373854, -0.2845877964562161244, -0.3641732283464567121 ) ) ;
#63580=CARTESIAN_POINT ( 'NONE',  ( -0.1312335958005241554, -0.6046776061558809534, -0.2411417322834644161 ) ) ;
#63581=CARTESIAN_POINT ( 'NONE',  ( -0.1049868766404193215, 0.2306618581243847221, -0.2411417322834647770 ) ) ;
#63582=CARTESIAN_POINT ( 'NONE',  ( 1.023622047244095334, -0.1870078740157479769, 0.3641732283464567677 ) ) ;
#63584=CARTESIAN_POINT ( 'NONE',  ( 1.515748031496063186, -0.4536011799217368745, -0.2665933059059886201 ) ) ;
#63585=EDGE_CURVE ( 'NONE', #29291, #74748, #15813, .T. ) ;
#63586=CARTESIAN_POINT ( 'NONE',  ( 0.9580052493438327987, -0.4281496062992127816, -0.4176697321401328100 ) ) ;
#63588=CARTESIAN_POINT ( 'NONE',  ( -0.3280839895013117347, -0.4281496062992124485, 0.4176697321401328655 ) ) ;
#63590=CARTESIAN_POINT ( 'NONE',  ( 0.8727034120734913358, -0.05778040916215522460, 0.4822834645669289988 ) ) ;
#63591=CARTESIAN_POINT ( 'NONE',  ( 0.5380577427821529035, -0.4281496062992124485, 0.4176697321401328655 ) ) ;
#63592=CARTESIAN_POINT ( 'NONE',  ( 2.795275590551181466, 1.299212598425198095, -1.617488608965169241E-16 ) ) ;
#63593=CARTESIAN_POINT ( 'NONE',  ( 0.2230971128608932319, -0.3690944881889763329, 0.3153832671262228327 ) ) ;
#63594=CARTESIAN_POINT ( 'NONE',  ( 1.181102362204725198, -0.1870078740157479769, 0.4822834645669291653 ) ) ;
#63595=CARTESIAN_POINT ( 'NONE',  ( -0.1902887139107604098, -0.5511811023622046335, 0.09757992244046803654 ) ) ;
#63596=CARTESIAN_POINT ( 'NONE',  ( -0.2362204724409440182, -0.1870078740157479769, 0.4822834645669291653 ) ) ;
#63598=CARTESIAN_POINT ( 'NONE',  ( 0.3477690288713918276, 0.2952755905511811885, 0.1292274648535926551 ) ) ;
#63599=CARTESIAN_POINT ( 'NONE',  ( -0.9317585301837263412, -0.4281496062992127816, -0.4176697321401328100 ) ) ;
#63600=VECTOR ( 'NONE', #77048, 39.37007874015748143 ) ;
#63601=CARTESIAN_POINT ( 'NONE',  ( -0.7020997375328076329, -0.2845877964562161244, -0.3641732283464567121 ) ) ;
#63602=CARTESIAN_POINT ( 'NONE',  ( 0.5839895013123367340, -0.6692913385826773087, -0.1292274648535924053 ) ) ;
#63603=CARTESIAN_POINT ( 'NONE',  ( -1.187664041994750175, -0.05778040916215560624, -0.4822834645669293319 ) ) ;
#63604=CARTESIAN_POINT ( 'NONE',  ( -0.5446194225721777693, -0.05778040916215522460, 0.4822834645669289988 ) ) ;
#63606=CARTESIAN_POINT ( 'NONE',  ( -0.6575345472713096662, 1.929133858267489954, 0.5309055118110236338 ) ) ;
#63607=CARTESIAN_POINT ( 'NONE',  ( 1.377952755905512472, -0.6692913385826771977, 8.415575281601705876E-17 ) ) ;
#63608=CARTESIAN_POINT ( 'NONE',  ( 1.423884514435696413, -0.3162353388693409650, -0.4822834645669289433 ) ) ;
#63610=CARTESIAN_POINT ( 'NONE',  ( -1.561679790026246017, -0.4281496062992127816, -0.4176697321401328100 ) ) ;
#63611=CARTESIAN_POINT ( 'NONE',  ( -0.8398950131233589023, -0.6046776061558809534, -0.2411417322834644161 ) ) ;
#63614=EDGE_LOOP ( 'NONE', ( #197, #78245, #37544, #8860, #35090, #42824, #74122 ) ) ;
#63615=CARTESIAN_POINT ( 'NONE',  ( -0.1771653543307080136, 0.07958543189024071263, -0.2665933059059888421 ) ) ;
#63617=CARTESIAN_POINT ( 'NONE',  ( 0.7611548556430451917, -0.6046776061558807314, 0.2411417322834647770 ) ) ;
#63620=CARTESIAN_POINT ( 'NONE',  ( -0.6496062992125976043, 0.07958543189024071263, -0.2665933059059888421 ) ) ;
#63622=CARTESIAN_POINT ( 'NONE',  ( 1.384514435695538559, 0.2952755905511810774, -0.1292274648535930714 ) ) ;
#63623=CARTESIAN_POINT ( 'NONE',  ( 1.010498687664042716, -0.004921259842519870586, -0.3153832671262229437 ) ) ;
#63624=CARTESIAN_POINT ( 'NONE',  ( 0.1246719160104994284, 0.2952755905511810774, -0.1292274648535930714 ) ) ;
#63626=CARTESIAN_POINT ( 'NONE',  ( -0.2493438320209966919, -0.4281496062992124485, 0.4176697321401328655 ) ) ;
#63627=CARTESIAN_POINT ( 'NONE',  ( -1.141732283464566011, -0.5511811023622047445, 6.969142054262312111E-17 ) ) ;
#63628=CARTESIAN_POINT ( 'NONE',  ( -0.4002624671916004129, -0.05778040916215560624, -0.4822834645669293319 ) ) ;
#63629=CARTESIAN_POINT ( 'NONE',  ( 1.587926509186352586, -0.4281496062992127816, -0.4176697321401328100 ) ) ;
#63633=CARTESIAN_POINT ( 'NONE',  ( 0.2755905511811031494, 0.2952755905511811885, 0.000000000000000000 ) ) ;
#63635=CARTESIAN_POINT ( 'NONE',  ( -0.9776902887139098386, -0.6692913385826771977, 0.1292274648535927661 ) ) ;
#63636=CARTESIAN_POINT ( 'NONE',  ( -1.338582677165353729, -0.1870078740157479769, 0.4822834645669291653 ) ) ;
#63637=CARTESIAN_POINT ( 'NONE',  ( 0.8464566929133865436, 0.1660481256975883668, -0.3530559997133364547 ) ) ;
#63638=CARTESIAN_POINT ( 'NONE',  ( -0.05249343832020911260, 0.2306618581243848609, 0.2411417322834645549 ) ) ;
#63640=CARTESIAN_POINT ( 'NONE',  ( -0.7808398950131225646, -0.05778040916215522460, 0.4822834645669289988 ) ) ;
#63641=CARTESIAN_POINT ( 'NONE',  ( -0.3083989501312330295, -0.3162353388693409650, -0.4822834645669289433 ) ) ;
#63642=CARTESIAN_POINT ( 'NONE',  ( -0.9120734908136475250, -0.6692913385826773087, -0.1292274648535924053 ) ) ;
#63643=CARTESIAN_POINT ( 'NONE',  ( 0.006561679790026889343, -0.2845877964562161244, -0.3641732283464567121 ) ) ;
#63645=CARTESIAN_POINT ( 'NONE',  ( -0.08530183727034056085, -0.05778040916215560624, -0.4822834645669293319 ) ) ;
#63647=CARTESIAN_POINT ( 'NONE',  ( 1.338582677165355062, -0.1870078740157480879, -0.4822834645669291653 ) ) ;
#63650=EDGE_LOOP ( 'NONE', ( #37310, #62279, #46557, #61270 ) ) ;
#63651=CARTESIAN_POINT ( 'NONE',  ( 0.1706036745406830368, -0.4281496062992127816, -0.4176697321401328100 ) ) ;
#63652=CARTESIAN_POINT ( 'NONE',  ( 0.07874015748031558404, -0.1870078740157480601, -0.3641732283464567677 ) ) ;
#63653=CARTESIAN_POINT ( 'NONE',  ( 1.489501312335958172, -0.2845877964562159024, 0.3641732283464567677 ) ) ;
#63654=CARTESIAN_POINT ( 'NONE',  ( 1.603475055217291612, 0.5037964761735346242, -0.04573490813648244807 ) ) ;
#63657=CARTESIAN_POINT ( 'NONE',  ( 1.640419947506562393, -0.3690944881889763329, 0.3153832671262228327 ) ) ;
#63658=CARTESIAN_POINT ( 'NONE',  ( -1.614173228346455824, 0.2952755905511811885, 0.000000000000000000 ) ) ;
#63660=CARTESIAN_POINT ( 'NONE',  ( 0.6364829396325465405, -0.05778040916215522460, 0.4822834645669289988 ) ) ;
#63661=CARTESIAN_POINT ( 'NONE',  ( -1.207349081364828436, -0.6046776061558807314, 0.2411417322834647770 ) ) ;
#63663=CARTESIAN_POINT ( 'NONE',  ( -1.253280839895012377, -0.05778040916215522460, 0.4822834645669289988 ) ) ;
#63664=CARTESIAN_POINT ( 'NONE',  ( 0.3215223097112867578, -0.05778040916215522460, 0.4822834645669289988 ) ) ;
#63665=CARTESIAN_POINT ( 'NONE',  ( 1.141732283464567566, 0.2952755905511811885, 0.000000000000000000 ) ) ;
#63666=CARTESIAN_POINT ( 'NONE',  ( 1.515748031496063408, 0.07958543189024085140, 0.2665933059059887866 ) ) ;
#63667=CARTESIAN_POINT ( 'NONE',  ( 0.9645669291338591078, -0.4536011799217368745, -0.2665933059059886201 ) ) ;
#63668=CARTESIAN_POINT ( 'NONE',  ( -0.7349081364829387342, -0.6046776061558807314, 0.2411417322834647770 ) ) ;
#63670=CARTESIAN_POINT ( 'NONE',  ( 1.692913385826772421, 0.2952755905511811885, 0.000000000000000000 ) ) ;
#63672=CARTESIAN_POINT ( 'NONE',  ( 0.8923884514435703741, 0.2306618581243848609, 0.2411417322834645549 ) ) ;
#63674=CARTESIAN_POINT ( 'NONE',  ( -1.443569553805773564, -0.5023911411419708095, 0.1820866141732285504 ) ) ;
#63675=CARTESIAN_POINT ( 'NONE',  ( 0.04593175853018440641, -0.6692913385826771977, 0.1292274648535927661 ) ) ;
#63676=CARTESIAN_POINT ( 'NONE',  ( 0.9645669291338588858, 0.07958543189024085140, 0.2665933059059887866 ) ) ;
#63677=EDGE_CURVE ( 'NONE', #4124, #9295, #54817, .T. ) ;
#63680=CARTESIAN_POINT ( 'NONE',  ( 1.010498687664042716, -0.4281496062992124485, 0.4176697321401328655 ) ) ;
#63681=CARTESIAN_POINT ( 'NONE',  ( -0.4840268112322907434, 0.02791078216816347476, -0.4328096321851898631 ) ) ;
#63682=CARTESIAN_POINT ( 'NONE',  ( -0.3280839895013117347, -0.3690944881889763329, 0.3153832671262228327 ) ) ;
#63683=CARTESIAN_POINT ( 'NONE',  ( -0.5643044619422565855, 0.05413385826771626580, -0.4176697321401330321 ) ) ;
#63684=CARTESIAN_POINT ( 'NONE',  ( 1.535433070866142558, 0.2952755905511811885, 0.000000000000000000 ) ) ;
#63685=CARTESIAN_POINT ( 'NONE',  ( -1.049868766404198794, 0.2306618581243847221, -0.2411417322834647770 ) ) ;
#63686=CARTESIAN_POINT ( 'NONE',  ( 1.443569553805774897, -0.6046776061558809534, -0.2411417322834644161 ) ) ;
#63688=CARTESIAN_POINT ( 'NONE',  ( -1.187664041994749731, -0.2845877964562159024, 0.3641732283464567677 ) ) ;
#63689=CARTESIAN_POINT ( 'NONE',  ( -0.7233831536535030304, 2.232734770847148997, 0.5048085489442963869 ) ) ;
#63690=CARTESIAN_POINT ( 'NONE',  ( 1.174540682414699111, -0.05778040916215560624, -0.4822834645669293319 ) ) ;
#63692=CARTESIAN_POINT ( 'NONE',  ( -1.725721784776902190, -0.05778040916215522460, 0.4822834645669289988 ) ) ;
#63693=CARTESIAN_POINT ( 'NONE',  ( 1.673228346456693494, 0.1660481256975885056, 0.3530559997133364547 ) ) ;
#63694=CARTESIAN_POINT ( 'NONE',  ( -1.194225721784776262, -0.004921259842519870586, -0.3153832671262229437 ) ) ;
#63695=CARTESIAN_POINT ( 'NONE',  ( 1.170763242744970123, 4.257495641787552160E-16, -0.4281993546915526805 ) ) ;
#63696=CARTESIAN_POINT ( 'NONE',  ( -0.5905511811023613777, -0.6692913385826771977, 8.415575281601705876E-17 ) ) ;
#63697=CARTESIAN_POINT ( 'NONE',  ( 0.07874015748031558404, -0.1870078740157479769, 0.3641732283464567677 ) ) ;
#63698=CARTESIAN_POINT ( 'NONE',  ( -1.574803149606298636, -0.1870078740157479769, 0.3641732283464567677 ) ) ;
#63699=CARTESIAN_POINT ( 'NONE',  ( 0.8661417322834652488, -0.1870078740157480601, -0.3641732283464567677 ) ) ;
#63700=CARTESIAN_POINT ( 'NONE',  ( 0.8792650918635177559, 0.05413385826771666132, 0.4176697321401328100 ) ) ;
#63701=CARTESIAN_POINT ( 'NONE',  ( 1.502624671916010790, -0.3162353388693409650, -0.4822834645669289433 ) ) ;
#63702=CARTESIAN_POINT ( 'NONE',  ( 0.1181102362204730916, 0.1771653543307087630, 0.000000000000000000 ) ) ;
#63703=CARTESIAN_POINT ( 'NONE',  ( 0.5643044619422579178, 0.05413385826771666132, 0.4176697321401328100 ) ) ;
#63704=CARTESIAN_POINT ( 'NONE',  ( 0.6692913385826777528, 0.1771653543307087630, 0.000000000000000000 ) ) ;
#63705=CARTESIAN_POINT ( 'NONE',  ( -1.653543307086613234, -0.1870078740157479769, 0.4822834645669291653 ) ) ;
#63706=CARTESIAN_POINT ( 'NONE',  ( -1.259842519685038686, -0.1870078740157480879, -0.4822834645669291653 ) ) ;
#63707=CARTESIAN_POINT ( 'NONE',  ( -0.3412073490813641308, -0.6046776061558807314, 0.2411417322834647770 ) ) ;
#63710=CARTESIAN_POINT ( 'NONE',  ( 0.5314960629921264834, 0.1660481256975883668, -0.3530559997133364547 ) ) ;
#63711=CARTESIAN_POINT ( 'NONE',  ( 1.154855643044620184, 0.1283753931104746893, -0.1820866141732285504 ) ) ;
#63712=CARTESIAN_POINT ( 'NONE',  ( -0.4790026246719152336, -0.05778040916215560624, -0.4822834645669293319 ) ) ;
#63713=CARTESIAN_POINT ( 'NONE',  ( 0.3871391076115492380, -0.05778040916215560624, -0.4822834645669293319 ) ) ;
#63717=CARTESIAN_POINT ( 'NONE',  ( 2.795275590551181910, 1.805669738366189048, 0.000000000000000000 ) ) ;
#63720=CARTESIAN_POINT ( 'NONE',  ( -0.3608923884514428360, -0.5511811023622048555, -0.09757992244046775898 ) ) ;
#63721=CARTESIAN_POINT ( 'NONE',  ( -1.095800524934382292, -0.05778040916215522460, 0.4822834645669289988 ) ) ;
#63723=CARTESIAN_POINT ( 'NONE',  ( 0.6496062992125991586, -0.5400638737290845981, -0.3530559997133363437 ) ) ;
#63724=CARTESIAN_POINT ( 'NONE',  ( 1.417322834645670104, -0.1870078740157479769, 0.4822834645669291653 ) ) ;
#63725=CARTESIAN_POINT ( 'NONE',  ( 0.7349081364829402885, -0.6046776061558809534, -0.2411417322834644161 ) ) ;
#63728=CARTESIAN_POINT ( 'NONE',  ( 1.673228346456693494, 0.1660481256975885056, 0.3530559997133364547 ) ) ;
#63729=CARTESIAN_POINT ( 'NONE',  ( 0.4855643044619428750, 0.05413385826771666132, 0.4176697321401328100 ) ) ;
#63730=CARTESIAN_POINT ( 'NONE',  ( 0.7414698162729663755, -0.6692913385826773087, -0.1292274648535924053 ) ) ;
#63732=CARTESIAN_POINT ( 'NONE',  ( 0.7414698162729663755, -0.5511811023622048555, -0.09757992244046775898 ) ) ;
#63733=CARTESIAN_POINT ( 'NONE',  ( 1.108923884514436686, -0.3162353388693409650, -0.4822834645669289433 ) ) ;
#63735=CARTESIAN_POINT ( 'NONE',  ( 0.3608923884514443348, 0.2952755905511810774, -0.1292274648535930714 ) ) ;
#63736=CARTESIAN_POINT ( 'NONE',  ( 0.9908136482939640111, -0.6692913385826771977, 0.1292274648535927661 ) ) ;
#63737=CARTESIAN_POINT ( 'NONE',  ( 0.2559055118110243332, 0.1660481256975885056, 0.3530559997133364547 ) ) ;
#63738=CARTESIAN_POINT ( 'NONE',  ( 1.397637795275591177, 0.07958543189024071263, -0.2665933059059888421 ) ) ;
#63739=CARTESIAN_POINT ( 'NONE',  ( -0.8661417322834640276, -0.1870078740157480879, -0.4822834645669291653 ) ) ;
#63740=CARTESIAN_POINT ( 'NONE',  ( -0.8267716535433065062, -0.6692913385826771977, 8.415575281601705876E-17 ) ) ;
#63741=CARTESIAN_POINT ( 'NONE',  ( 1.351706036745407458, -0.4281496062992127816, -0.4176697321401328100 ) ) ;
#63745=EDGE_LOOP ( 'NONE', ( #20155, #42523, #5379, #80931, #58676, #28023, #16348, #2341, #63025, #506, #46895, #13119, #76390, #54631, #69617, #26392, #19126, #33846, #75862, #43574, #53907 ) ) ;
#63749=CARTESIAN_POINT ( 'NONE',  ( 1.437007874015748810, 0.07958543189024085140, 0.2665933059059887866 ) ) ;
#63751=CARTESIAN_POINT ( 'NONE',  ( 1.227034120734908917, 0.1771653543307087075, -0.09757992244046823083 ) ) ;
#63755=CARTESIAN_POINT ( 'NONE',  ( -0.5511811023622038563, -0.1870078740157479769, 0.3641732283464567677 ) ) ;
#63756=CARTESIAN_POINT ( 'NONE',  ( -1.568241469816272105, -0.08942795157527998196, 0.3641732283464567121 ) ) ;
#63757=CARTESIAN_POINT ( 'NONE',  ( -1.404199475065615932, -0.4281496062992127816, -0.4176697321401328100 ) ) ;
#63758=CARTESIAN_POINT ( 'NONE',  ( 0.2952755905511816326, -0.5400638737290844871, 0.3530559997133364547 ) ) ;
#63759=CARTESIAN_POINT ( 'NONE',  ( 1.594488188976378673, 0.1660481256975885056, 0.3530559997133364547 ) ) ;
#63765=CARTESIAN_POINT ( 'NONE',  ( -0.6167979002624665030, -0.3690944881889765550, -0.3153832671262227771 ) ) ;
#63767=CARTESIAN_POINT ( 'NONE',  ( -1.148293963254592542, 0.2952755905511811885, 0.1292274648535926551 ) ) ;
#63768=CARTESIAN_POINT ( 'NONE',  ( 1.049868766404200349, 0.2306618581243848609, 0.2411417322834645549 ) ) ;
#63770=CARTESIAN_POINT ( 'NONE',  ( 0.7217847769028878924, 0.05413385826771666132, 0.4176697321401328100 ) ) ;
#63771=CARTESIAN_POINT ( 'NONE',  ( -1.595398199321657051, 0.7585570207896576989, 0.1559797534342473035 ) ) ;
#63772=CARTESIAN_POINT ( 'NONE',  ( 1.082677165354331228, 0.1660481256975883668, -0.3530559997133364547 ) ) ;
#63773=CARTESIAN_POINT ( 'NONE',  ( -1.345144356955379816, -0.05778040916215560624, -0.4822834645669293319 ) ) ;
#63775=EDGE_CURVE ( 'NONE', #29190, #69836, #48781, .T. ) ;
#63776=CARTESIAN_POINT ( 'NONE',  ( -0.4986876640419942164, -0.5023911411419708095, 0.1820866141732285504 ) ) ;
#63779=CARTESIAN_POINT ( 'NONE',  ( -0.6955380577427815458, -0.004921259842519576551, 0.3153832671262227771 ) ) ;
#63780=CARTESIAN_POINT ( 'NONE',  ( 0.2230971128608929543, -0.004921259842519870586, -0.3153832671262229437 ) ) ;
#63781=CARTESIAN_POINT ( 'NONE',  ( 0.01312335958005323398, 0.05413385826771666132, 0.4176697321401328100 ) ) ;
#63782=CARTESIAN_POINT ( 'NONE',  ( -0.7939632545931750718, -0.08942795157528024563, -0.3641732283464568787 ) ) ;
#63784=CARTESIAN_POINT ( 'NONE',  ( 1.286089238845145033, 0.2306618581243848609, 0.2411417322834645549 ) ) ;
#63785=CARTESIAN_POINT ( 'NONE',  ( -1.272965879265091305, 0.05413385826771626580, -0.4176697321401330321 ) ) ;
#63787=CARTESIAN_POINT ( 'NONE',  ( -0.1640419947506555343, -0.3162353388693405765, 0.4822834645669290543 ) ) ;
#63788=CARTESIAN_POINT ( 'NONE',  ( -0.9776902887139098386, 0.2952755905511810774, -0.1292274648535930714 ) ) ;
#63789=CARTESIAN_POINT ( 'NONE',  ( 1.207349081364829990, 0.1283753931104748280, 0.1820866141732283561 ) ) ;
#63791=CARTESIAN_POINT ( 'NONE',  ( -0.1902887139107604098, -0.5511811023622046335, 0.09757992244046803654 ) ) ;
#63792=CARTESIAN_POINT ( 'NONE',  ( -0.4527559055118102749, 0.1660481256975885056, 0.3530559997133364547 ) ) ;
#63793=CARTESIAN_POINT ( 'NONE',  ( -1.259842519685038686, -0.1870078740157480879, -0.4822834645669291653 ) ) ;
#63795=CARTESIAN_POINT ( 'NONE',  ( 1.174540682414699111, -0.2845877964562159024, 0.3641732283464567677 ) ) ;
#63796=CARTESIAN_POINT ( 'NONE',  ( -0.3937007874015740483, -0.1870078740157479769, 0.4822834645669291653 ) ) ;
#63797=CARTESIAN_POINT ( 'NONE',  ( -1.699475065616797398, 0.2952755905511811885, 0.1292274648535926551 ) ) ;
#63800=CARTESIAN_POINT ( 'NONE',  ( -0.9448818897637790704, -0.1870078740157480601, -0.3641732283464567677 ) ) ;
#63801=CARTESIAN_POINT ( 'NONE',  ( 1.187664041994751285, -0.3162353388693409650, -0.4822834645669289433 ) ) ;
#63802=CARTESIAN_POINT ( 'NONE',  ( -1.049868766404198794, 0.1283753931104746893, -0.1820866141732285504 ) ) ;
#63804=CARTESIAN_POINT ( 'NONE',  ( -1.115485564304461219, -0.4281496062992124485, 0.4176697321401328655 ) ) ;
#63805=CARTESIAN_POINT ( 'NONE',  ( 0.8727034120734913358, -0.05778040916215522460, 0.4822834645669289988 ) ) ;
#63806=CARTESIAN_POINT ( 'NONE',  ( 0.9645669291338591078, -0.5400638737290845981, -0.3530559997133363437 ) ) ;
#63807=CARTESIAN_POINT ( 'NONE',  ( 1.482939632545932307, 0.05413385826771626580, -0.4176697321401330321 ) ) ;
#63808=CARTESIAN_POINT ( 'NONE',  ( -1.601049868766403650, -0.5023911411419708095, 0.1820866141732285504 ) ) ;
#63813=CARTESIAN_POINT ( 'NONE',  ( 1.305774278215223960, -0.5511811023622046335, 0.09757992244046803654 ) ) ;
#63814=CARTESIAN_POINT ( 'NONE',  ( 0.7086614173228352742, -0.1870078740157480601, -0.3641732283464567677 ) ) ;
#63815=CARTESIAN_POINT ( 'NONE',  ( 0.1312335958005255154, -0.6046776061558807314, 0.2411417322834647770 ) ) ;
#63816=CARTESIAN_POINT ( 'NONE',  ( 1.581364829396326277, -0.05778040916215522460, 0.4822834645669289988 ) ) ;
#63818=CARTESIAN_POINT ( 'NONE',  ( 0.8464566929133866546, -0.4536011799217367080, 0.2665933059059888421 ) ) ;
#63819=CARTESIAN_POINT ( 'NONE',  ( -0.4855643044619415427, 0.05413385826771626580, -0.4176697321401330321 ) ) ;
#63820=CARTESIAN_POINT ( 'NONE',  ( -1.377952755905511140, -0.6692913385826771977, 8.415575281601705876E-17 ) ) ;
#63821=CARTESIAN_POINT ( 'NONE',  ( 1.049868766404200349, 0.2306618581243848609, 0.2411417322834645549 ) ) ;
#63823=CARTESIAN_POINT ( 'NONE',  ( -0.7773926554473638006, -2.191421614605370878E-15, 0.4445507791589071167 ) ) ;
#63825=ORIENTED_EDGE ( 'NONE', *, *, #30136, .F. ) ;
#63826=CARTESIAN_POINT ( 'NONE',  ( -1.299212598425196097, -0.6692913385826771977, 8.415575281601705876E-17 ) ) ;
#63828=CARTESIAN_POINT ( 'NONE',  ( -0.7086614173228339419, -0.1870078740157479769, 0.4822834645669291653 ) ) ;
#63829=CARTESIAN_POINT ( 'NONE',  ( -0.7086614173228339419, -0.1870078740157479769, 0.3641732283464567677 ) ) ;
#63830=CARTESIAN_POINT ( 'NONE',  ( -0.9186351706036736120, -0.6046776061558809534, -0.2411417322834644161 ) ) ;
#63833=CARTESIAN_POINT ( 'NONE',  ( -0.2559055118110227234, -0.5400638737290844871, 0.3530559997133364547 ) ) ;
#63834=CARTESIAN_POINT ( 'NONE',  ( 1.614173228346457378, 0.2952755905511811885, 0.000000000000000000 ) ) ;
#63835=CARTESIAN_POINT ( 'NONE',  ( -0.9514435695538050464, -0.3162353388693405765, 0.4822834645669290543 ) ) ;
#63836=CARTESIAN_POINT ( 'NONE',  ( 0.3937007874015754361, -0.1870078740157480879, -0.4822834645669291653 ) ) ;
#63837=CARTESIAN_POINT ( 'NONE',  ( -0.8727034120734901146, -0.3162353388693405765, 0.4822834645669290543 ) ) ;
#63839=CARTESIAN_POINT ( 'NONE',  ( -0.8202099737532799750, 0.1771653543307087075, -0.09757992244046823083 ) ) ;
#63843=CARTESIAN_POINT ( 'NONE',  ( -1.607611548556429737, -0.5511811023622046335, 0.09757992244046803654 ) ) ;
#63844=CARTESIAN_POINT ( 'NONE',  ( -1.174540682414697335, -0.05778040916215522460, 0.4822834645669289988 ) ) ;
#63845=CARTESIAN_POINT ( 'NONE',  ( -0.8792650918635160906, -0.4281496062992124485, 0.4176697321401328655 ) ) ;
#63847=CARTESIAN_POINT ( 'NONE',  ( -1.181102362204723644, -0.1870078740157480879, -0.4822834645669291653 ) ) ;
#63848=CARTESIAN_POINT ( 'NONE',  ( -1.391076115485563758, 0.2306618581243848609, 0.2411417322834645549 ) ) ;
#63849=CARTESIAN_POINT ( 'NONE',  ( 2.795275590551181466, 1.968503937007874960, 0.000000000000000000 ) ) ;
#63850=FACE_OUTER_BOUND ( 'NONE', #10147, .T. ) ;
#63852=CARTESIAN_POINT ( 'NONE',  ( 0.5511811023622055217, -0.1870078740157479769, 0.3641732283464567677 ) ) ;
#63855=CARTESIAN_POINT ( 'NONE',  ( -0.5708661417322828946, 0.07958543189024071263, -0.2665933059059888421 ) ) ;
#63856=CARTESIAN_POINT ( 'NONE',  ( -0.9580052493438311334, 0.05413385826771626580, -0.4176697321401330321 ) ) ;
#63857=CARTESIAN_POINT ( 'NONE',  ( 1.489501312335958172, -0.05778040916215560624, -0.4822834645669293319 ) ) ;
#63858=CARTESIAN_POINT ( 'NONE',  ( -0.3149606299212590610, -0.1870078740157480879, -0.4822834645669291653 ) ) ;
#63862=CARTESIAN_POINT ( 'NONE',  ( -0.5774278215223089816, -0.6046776061558807314, 0.2411417322834647770 ) ) ;
#63863=CARTESIAN_POINT ( 'NONE',  ( 1.377952755905512472, -0.6692913385826771977, 8.415575281601705876E-17 ) ) ;
#63864=CARTESIAN_POINT ( 'NONE',  ( -1.259842519685038686, -0.1870078740157479769, 0.3641732283464567677 ) ) ;
#63865=CARTESIAN_POINT ( 'NONE',  ( -1.253280839895012377, -0.05778040916215522460, 0.4822834645669289988 ) ) ;
#63870=CARTESIAN_POINT ( 'NONE',  ( 0.1181102362204730916, 0.2952755905511811885, 0.000000000000000000 ) ) ;
#63871=CARTESIAN_POINT ( 'NONE',  ( -1.036745406824146176, -0.3690944881889763329, 0.3153832671262228327 ) ) ;
#63872=CARTESIAN_POINT ( 'NONE',  ( -0.1968503937007867743, -0.6692913385826771977, 8.415575281601705876E-17 ) ) ;
#63874=CARTESIAN_POINT ( 'NONE',  ( -0.7611548556430438595, 0.2306618581243848609, 0.2411417322834645549 ) ) ;
#63875=CARTESIAN_POINT ( 'NONE',  ( -0.9842519685039365918, -0.6692913385826771977, 8.415575281601705876E-17 ) ) ;
#63877=CARTESIAN_POINT ( 'NONE',  ( 0.9580052493438326877, -0.004921259842519576551, 0.3153832671262227771 ) ) ;
#63878=CARTESIAN_POINT ( 'NONE',  ( -0.9448818897637790704, -0.1870078740157479769, 0.3641732283464567677 ) ) ;
#63879=CARTESIAN_POINT ( 'NONE',  ( 0.8333333333333340365, -0.5511811023622046335, 0.09757992244046803654 ) ) ;
#63880=CARTESIAN_POINT ( 'NONE',  ( -1.686351706036744558, 0.2952755905511810774, -0.1292274648535930714 ) ) ;
#63881=CARTESIAN_POINT ( 'NONE',  ( 1.515748031496063186, -0.5400638737290845981, -0.3530559997133363437 ) ) ;
#63883=CARTESIAN_POINT ( 'NONE',  ( 0.5774278215223104249, 0.1283753931104748280, 0.1820866141732283561 ) ) ;
#63885=CARTESIAN_POINT ( 'NONE',  ( -0.8530183727034112984, 0.05413385826771666132, 0.4176697321401328100 ) ) ;
#63886=CARTESIAN_POINT ( 'NONE',  ( 1.305774278215223960, 0.2952755905511810774, -0.1292274648535930714 ) ) ;
#63888=CARTESIAN_POINT ( 'NONE',  ( -0.2427821522309703550, -0.2845877964562159024, 0.3641732283464567677 ) ) ;
#63890=CARTESIAN_POINT ( 'NONE',  ( 0.3805774278215230400, -0.4281496062992124485, 0.4176697321401328655 ) ) ;
#63892=CARTESIAN_POINT ( 'NONE',  ( 1.017060367454068581, -0.08942795157528024563, -0.3641732283464568787 ) ) ;
#63893=CARTESIAN_POINT ( 'NONE',  ( 0.1640419947506569498, -0.08942795157527998196, 0.3641732283464567121 ) ) ;
#63894=CARTESIAN_POINT ( 'NONE',  ( 0.2427821522309719648, -0.05778040916215522460, 0.4822834645669289988 ) ) ;
#63895=CARTESIAN_POINT ( 'NONE',  ( -1.358267716535432434, 0.1660481256975883668, -0.3530559997133364547 ) ) ;
#63896=CARTESIAN_POINT ( 'NONE',  ( -0.8333333333333323711, 0.1771653543307087630, 0.09757992244046791164 ) ) ;
#63899=CARTESIAN_POINT ( 'NONE',  ( -0.3543307086614165824, 0.2952755905511811885, 0.000000000000000000 ) ) ;
#63901=( BOUNDED_CURVE ( )  B_SPLINE_CURVE ( 2, ( #78401, #71658, #20311, #77563, #38824, #58600, #19897, #14010, #45962, #52277, #542, #13586, #25772 ),
 .UNSPECIFIED., .F., .F. ) 
 B_SPLINE_CURVE_WITH_KNOTS ( ( 3, 2, 2, 2, 2, 2, 3 ),
 ( 0.4915129128166190742, 0.4924242424242424310, 0.4962121212121212155, 0.5000000000000000000, 0.5037878787878787845, 0.5075757575757575690, 0.5084870871833810924 ),
 .UNSPECIFIED. ) 
 CURVE ( )  GEOMETRIC_REPRESENTATION_ITEM ( )  RATIONAL_B_SPLINE_CURVE ( ( 0.9875488213027530104, 0.9918020599134685922, 1.000000000000000000, 0.9659258262890683122, 1.000000000000000000, 0.9659258262890683122, 1.000000000000000000, 0.9659258262890683122, 1.000000000000000000, 0.9659258262890683122, 1.000000000000000000, 0.9918020599134671489, 0.9875488213027514561 ) ) 
 REPRESENTATION_ITEM ( '' )  );
#63903=CARTESIAN_POINT ( 'NONE',  ( 0.3871391076115492380, -0.08942795157528024563, -0.3641732283464568787 ) ) ;
#63904=CARTESIAN_POINT ( 'NONE',  ( -0.4658792650918627265, -0.3162353388693409650, -0.4822834645669289433 ) ) ;
#63905=CARTESIAN_POINT ( 'NONE',  ( -1.174540682414697335, -0.05778040916215522460, 0.4822834645669289988 ) ) ;
#63906=CARTESIAN_POINT ( 'NONE',  ( -0.6364829396325453192, -0.08942795157528024563, -0.3641732283464568787 ) ) ;
#63908=CARTESIAN_POINT ( 'NONE',  ( -0.6364829396325453192, -0.05778040916215560624, -0.4822834645669293319 ) ) ;
#63909=CARTESIAN_POINT ( 'NONE',  ( -0.9186351706036736120, -0.5023911411419708095, -0.1820866141732282451 ) ) ;
#63910=CARTESIAN_POINT ( 'NONE',  ( -1.423884514435694859, -0.2845877964562159024, 0.3641732283464567677 ) ) ;
#63911=CARTESIAN_POINT ( 'NONE',  ( 1.187664041994751285, -0.3162353388693409650, -0.4822834645669289433 ) ) ;
#63916=CARTESIAN_POINT ( 'NONE',  ( -1.345144356955379816, -0.05778040916215560624, -0.4822834645669293319 ) ) ;
#63917=CARTESIAN_POINT ( 'NONE',  ( -1.017060367454067249, -0.3162353388693409650, -0.4822834645669289433 ) ) ;
#63918=EDGE_CURVE ( 'NONE', #66254, #10557, #64978, .T. ) ;
#63919=CARTESIAN_POINT ( 'NONE',  ( -1.568241469816272105, -0.3162353388693409650, -0.4822834645669289433 ) ) ;
#63923=CARTESIAN_POINT ( 'NONE',  ( 0.9186351706036752773, 0.2306618581243847221, -0.2411417322834647770 ) ) ;
#63924=CARTESIAN_POINT ( 'NONE',  ( -0.01968503937007793844, 0.1660481256975883668, -0.3530559997133364547 ) ) ;
#63925=CARTESIAN_POINT ( 'NONE',  ( -0.6986524979670485358, -2.191421614605370878E-15, 0.4445507791589071167 ) ) ;
#63927=CARTESIAN_POINT ( 'NONE',  ( 1.161417322834646271, 0.07958543189024071263, -0.2665933059059888421 ) ) ;
#63929=ORIENTED_EDGE ( 'NONE', *, *, #28395, .T. ) ;
#63932=CARTESIAN_POINT ( 'NONE',  ( 0.04593175853018440641, 0.2952755905511810774, -0.1292274648535930714 ) ) ;
#63933=CARTESIAN_POINT ( 'NONE',  ( -0.9055118110236215490, 0.2952755905511811885, 0.000000000000000000 ) ) ;
#63934=CARTESIAN_POINT ( 'NONE',  ( -1.535433070866141225, -0.6692913385826771977, 8.415575281601705876E-17 ) ) ;
#63935=CARTESIAN_POINT ( 'NONE',  ( 0.5905511811023629321, 0.2952755905511811885, 0.000000000000000000 ) ) ;
#63936=CARTESIAN_POINT ( 'NONE',  ( -1.627296587926508442, 0.1283753931104748280, 0.1820866141732283561 ) ) ;
#63937=CARTESIAN_POINT ( 'NONE',  ( 1.358267716535433323, -0.5400638737290845981, -0.3530559997133363437 ) ) ;
#63938=CARTESIAN_POINT ( 'NONE',  ( -0.6561679790026240244, 0.2306618581243847221, -0.2411417322834647770 ) ) ;
#63939=CARTESIAN_POINT ( 'NONE',  ( -1.161417322834644716, 0.1660481256975885056, 0.3530559997133364547 ) ) ;
#63940=CARTESIAN_POINT ( 'NONE',  ( 1.410761154855643795, -0.3162353388693405765, 0.4822834645669290543 ) ) ;
#63941=CARTESIAN_POINT ( 'NONE',  ( 1.666666666666667185, 0.05413385826771666132, 0.4176697321401328100 ) ) ;
#63942=CARTESIAN_POINT ( 'NONE',  ( -0.1049868766404193215, 0.2306618581243847221, -0.2411417322834647770 ) ) ;
#63944=CARTESIAN_POINT ( 'NONE',  ( 0.5183727034120741983, -0.5511811023622046335, 0.09757992244046803654 ) ) ;
#63945=ORIENTED_EDGE ( 'NONE', *, *, #75955, .F. ) ;
#63948=CARTESIAN_POINT ( 'NONE',  ( -0.08530183727034056085, -0.08942795157528024563, -0.3641732283464568787 ) ) ;
#63951=CARTESIAN_POINT ( 'NONE',  ( 0.07874015748031558404, -0.1870078740157480879, -0.4822834645669291653 ) ) ;
#63952=CARTESIAN_POINT ( 'NONE',  ( -0.09186351706036689768, 0.05413385826771626580, -0.4176697321401330321 ) ) ;
#63953=CARTESIAN_POINT ( 'NONE',  ( -0.7742782152230965886, 0.05413385826771666132, 0.4176697321401328100 ) ) ;
#63955=CARTESIAN_POINT ( 'NONE',  ( -1.207349081364828436, -0.6046776061558807314, 0.2411417322834647770 ) ) ;
#63957=CARTESIAN_POINT ( 'NONE',  ( 0.7217847769028878924, -0.3690944881889765550, -0.3153832671262227771 ) ) ;
#63958=CARTESIAN_POINT ( 'NONE',  ( 1.089238845144357759, 0.05413385826771626580, -0.4176697321401330321 ) ) ;
#63959=CARTESIAN_POINT ( 'NONE',  ( 0.9711286089238851948, -0.6046776061558809534, -0.2411417322834644161 ) ) ;
#63961=CARTESIAN_POINT ( 'NONE',  ( -1.325459317585300889, -0.4281496062992127816, -0.4176697321401328100 ) ) ;
#63964=CARTESIAN_POINT ( 'NONE',  ( 0.05905511811023681640, 0.1660481256975883668, -0.3530559997133364547 ) ) ;
#63967=CARTESIAN_POINT ( 'NONE',  ( 1.233595800524935227, -0.6046776061558807314, 0.2411417322834647770 ) ) ;
#63969=CARTESIAN_POINT ( 'NONE',  ( 1.246719160104987623, 0.05413385826771626580, -0.4176697321401330321 ) ) ;
#63970=CARTESIAN_POINT ( 'NONE',  ( 0.2034120734908144990, -0.5511811023622046335, 0.09757992244046803654 ) ) ;
#63971=CARTESIAN_POINT ( 'NONE',  ( 0.9055118110236227702, -0.6692913385826771977, 8.415575281601705876E-17 ) ) ;
#63973=CARTESIAN_POINT ( 'NONE',  ( 0.1509186351706045259, -0.08942795157528024563, -0.3641732283464568787 ) ) ;
#63974=CARTESIAN_POINT ( 'NONE',  ( 0.1771653543307093182, 0.1660481256975885056, 0.3530559997133364547 ) ) ;
#63976=CARTESIAN_POINT ( 'NONE',  ( -1.246719160104986512, 0.05413385826771666132, 0.4176697321401328100 ) ) ;
#63977=CARTESIAN_POINT ( 'NONE',  ( 0.9973753280839902091, 0.1283753931104746893, -0.1820866141732285504 ) ) ;
#63979=CARTESIAN_POINT ( 'NONE',  ( -0.4527559055118102749, 0.1660481256975885056, 0.3530559997133364547 ) ) ;
#63980=CARTESIAN_POINT ( 'NONE',  ( -0.3149606299212590610, -0.1870078740157480601, -0.3641732283464567677 ) ) ;
#63982=CARTESIAN_POINT ( 'NONE',  ( -0.4199475065616791736, 0.2306618581243847221, -0.2411417322834647770 ) ) ;
#63983=CARTESIAN_POINT ( 'NONE',  ( 0.4199475065616803948, -0.5023911411419708095, -0.1820866141732282451 ) ) ;
#63984=EDGE_CURVE ( 'NONE', #32456, #32791, #15179, .T. ) ;
#63986=CARTESIAN_POINT ( 'NONE',  ( -0.01312335958005186876, 0.05413385826771626580, -0.4176697321401330321 ) ) ;
#63988=CARTESIAN_POINT ( 'NONE',  ( 1.213910761154856299, 0.1771653543307087630, 0.09757992244046791164 ) ) ;
#63990=CARTESIAN_POINT ( 'NONE',  ( -0.8202099737532801971, -0.5511811023622046335, 0.09757992244046803654 ) ) ;
#63991=CARTESIAN_POINT ( 'NONE',  ( -0.8136482939632537770, -0.5023911411419708095, 0.1820866141732285504 ) ) ;
#63992=CARTESIAN_POINT ( 'NONE',  ( -0.2821522309711278487, -0.6692913385826773087, -0.1292274648535924053 ) ) ;
#63993=CARTESIAN_POINT ( 'NONE',  ( -0.03937007874015669567, -0.6692913385826771977, 8.415575281601705876E-17 ) ) ;
#63994=CARTESIAN_POINT ( 'NONE',  ( 0.4855643044619430415, -0.3690944881889765550, -0.3153832671262227771 ) ) ;
#63996=CARTESIAN_POINT ( 'NONE',  ( 1.391076115485564868, -0.5023911411419708095, 0.1820866141732285504 ) ) ;
#63997=CARTESIAN_POINT ( 'NONE',  ( 0.7742782152230979209, 0.05413385826771626580, -0.4176697321401330321 ) ) ;
#63999=CARTESIAN_POINT ( 'NONE',  ( -0.2427821522309703550, -0.05778040916215560624, -0.4822834645669293319 ) ) ;
#64001=CARTESIAN_POINT ( 'NONE',  ( -1.476377952755905110, -0.5400638737290845981, -0.3530559997133363437 ) ) ;
#64003=CARTESIAN_POINT ( 'NONE',  ( 0.8858267716535438430, 0.1660481256975885056, 0.3530559997133364547 ) ) ;
#64005=CARTESIAN_POINT ( 'NONE',  ( 0.4002624671916016896, -0.05778040916215522460, 0.4822834645669289988 ) ) ;
#64007=CARTESIAN_POINT ( 'NONE',  ( 0.2034120734908144990, -0.5511811023622046335, 0.09757992244046803654 ) ) ;
#64008=CARTESIAN_POINT ( 'NONE',  ( 1.259842519685040019, -0.1870078740157480879, -0.4822834645669291653 ) ) ;
#64009=CARTESIAN_POINT ( 'NONE',  ( -0.2887139107611542133, 0.1283753931104748280, 0.1820866141732283561 ) ) ;
#64010=CARTESIAN_POINT ( 'NONE',  ( -0.6036745406824141069, -0.6046776061558809534, -0.2411417322834644161 ) ) ;
#64011=CARTESIAN_POINT ( 'NONE',  ( 0.8530183727034126306, 0.05413385826771626580, -0.4176697321401330321 ) ) ;
#64012=CARTESIAN_POINT ( 'NONE',  ( 0.2821522309711292364, -0.6692913385826771977, 0.1292274648535927661 ) ) ;
#64013=CARTESIAN_POINT ( 'NONE',  ( -0.9842519685039360366, 0.2952755905511811885, 0.000000000000000000 ) ) ;
#64014=CARTESIAN_POINT ( 'NONE',  ( -0.6299212598425188991, -0.1870078740157479769, 0.3641732283464567677 ) ) ;
#64015=CARTESIAN_POINT ( 'NONE',  ( 0.1968503937007881344, 0.2952755905511811885, 0.000000000000000000 ) ) ;
#64016=CARTESIAN_POINT ( 'NONE',  ( -1.194225721784776262, 0.05413385826771626580, -0.4176697321401330321 ) ) ;
#64017=CARTESIAN_POINT ( 'NONE',  ( -0.2427821522309703550, -0.3162353388693405765, 0.4822834645669290543 ) ) ;
#64018=CARTESIAN_POINT ( 'NONE',  ( 1.167979002624672580, 0.009842519685039144428, -0.3409548833797004797 ) ) ;
#64020=CARTESIAN_POINT ( 'NONE',  ( 1.548556430446194954, -0.6046776061558807314, 0.2411417322834647770 ) ) ;
#64021=CARTESIAN_POINT ( 'NONE',  ( 1.476377952755906442, -0.5400638737290844871, 0.3530559997133364547 ) ) ;
#64022=CARTESIAN_POINT ( 'NONE',  ( 0.6962418744208975774, 2.409604939980833412E-17, -0.3464511005275205946 ) ) ;
#64024=CONICAL_SURFACE ( 'NONE', #25023, 1.181102362204724310, 0.7853981633974621568 ) ;
#64025=CARTESIAN_POINT ( 'NONE',  ( -0.8070866141732276899, -0.5400638737290844871, 0.3530559997133364547 ) ) ;
#64029=CARTESIAN_POINT ( 'NONE',  ( -0.1246719160104980823, -0.5511811023622048555, -0.09757992244046775898 ) ) ;
#64031=CARTESIAN_POINT ( 'NONE',  ( 0.7349081364829402885, -0.6046776061558809534, -0.2411417322834644161 ) ) ;
#64032=EDGE_CURVE ( 'NONE', #44871, #53395, #40836, .T. ) ;
#64035=CARTESIAN_POINT ( 'NONE',  ( -0.2493438320209966919, -0.3690944881889763329, 0.3153832671262228327 ) ) ;
#64037=CARTESIAN_POINT ( 'NONE',  ( 1.391076115485564868, 0.2306618581243847221, -0.2411417322834647770 ) ) ;
#64038=CARTESIAN_POINT ( 'NONE',  ( 0.8727034120734912248, -0.2845877964562161244, -0.3641732283464567121 ) ) ;
#64039=CARTESIAN_POINT ( 'NONE',  ( 0.07217847769028949700, -0.3162353388693405765, 0.4822834645669290543 ) ) ;
#64041=CARTESIAN_POINT ( 'NONE',  ( -0.9842519685039360366, 0.2952755905511811885, 0.000000000000000000 ) ) ;
#64042=CARTESIAN_POINT ( 'NONE',  ( -1.292650918635170010, -0.5511811023622046335, 0.09757992244046803654 ) ) ;
#64043=CARTESIAN_POINT ( 'NONE',  ( -0.5774278215223089816, 0.2306618581243847221, -0.2411417322834647770 ) ) ;
#64048=CARTESIAN_POINT ( 'NONE',  ( 0.4002624671916016896, -0.05778040916215522460, 0.4822834645669289988 ) ) ;
#64049=ORIENTED_EDGE ( 'NONE', *, *, #35375, .T. ) ;
#64050=CARTESIAN_POINT ( 'NONE',  ( -0.7808398950131225646, -0.05778040916215522460, 0.4822834645669289988 ) ) ;
#64051=CARTESIAN_POINT ( 'NONE',  ( 1.358267716535433323, -0.5400638737290845981, -0.3530559997133363437 ) ) ;
#64052=EDGE_CURVE ( 'NONE', #5951, #54436, #22801, .T. ) ;
#64053=CARTESIAN_POINT ( 'NONE',  ( 0.5314960629921264834, 0.1660481256975883668, -0.3530559997133364547 ) ) ;
#64054=CARTESIAN_POINT ( 'NONE',  ( -0.1443569553805765515, -0.4281496062992127816, -0.4176697321401328100 ) ) ;
#64056=CARTESIAN_POINT ( 'NONE',  ( -0.7874015748031489847, -0.1870078740157479769, 0.4822834645669291653 ) ) ;
#64057=CARTESIAN_POINT ( 'NONE',  ( -0.3412073490813641308, 0.2306618581243847221, -0.2411417322834647770 ) ) ;
#64059=CARTESIAN_POINT ( 'NONE',  ( -0.1181102362204717315, -0.5511811023622047445, 6.969142054262312111E-17 ) ) ;
#64061=CARTESIAN_POINT ( 'NONE',  ( 0.06561679790026316017, 0.05413385826771626580, -0.4176697321401330321 ) ) ;
#64062=CARTESIAN_POINT ( 'NONE',  ( -1.220472440944882386, 0.000000000000000000, -0.3464511005275204836 ) ) ;
#64063=CARTESIAN_POINT ( 'NONE',  ( 0.9448818897637802916, -0.1870078740157479769, 0.4822834645669291653 ) ) ;
#64064=CARTESIAN_POINT ( 'NONE',  ( 0.4855643044619428750, 0.009842519685039463617, 0.3409548833797002576 ) ) ;
#64066=ORIENTED_EDGE ( 'NONE', *, *, #48987, .T. ) ;
#64068=CARTESIAN_POINT ( 'NONE',  ( 0.2427821522309719648, -0.05778040916215522460, 0.4822834645669289988 ) ) ;
#64069=CARTESIAN_POINT ( 'NONE',  ( -0.3805774278215216522, -0.3690944881889765550, -0.3153832671262227771 ) ) ;
#64072=CARTESIAN_POINT ( 'NONE',  ( 1.240157480314961314, 0.07958543189024071263, -0.2665933059059888421 ) ) ;
#64076=CARTESIAN_POINT ( 'NONE',  ( 1.437007874015748810, -0.4536011799217368745, -0.2665933059059886201 ) ) ;
#64077=CARTESIAN_POINT ( 'NONE',  ( -1.463254593175852492, 0.2952755905511811885, 0.1292274648535926551 ) ) ;
#64080=CARTESIAN_POINT ( 'NONE',  ( 0.1115485564304467270, -0.6692913385826773087, -0.1292274648535924053 ) ) ;
#64081=CARTESIAN_POINT ( 'NONE',  ( -1.391076115485563314, -0.6046776061558809534, -0.2411417322834644161 ) ) ;
#64082=CARTESIAN_POINT ( 'NONE',  ( -1.010498687664041384, -0.4281496062992127816, -0.4176697321401328100 ) ) ;
#64083=CARTESIAN_POINT ( 'NONE',  ( 0.3871391076115492380, -0.05778040916215560624, -0.4822834645669293319 ) ) ;
#64085=CARTESIAN_POINT ( 'NONE',  ( -1.555118110236219930, -0.4536011799217368745, -0.2665933059059886201 ) ) ;
#64086=CARTESIAN_POINT ( 'NONE',  ( 0.9120734908136489683, -0.6692913385826771977, 0.1292274648535927661 ) ) ;
#64087=CARTESIAN_POINT ( 'NONE',  ( 0.7808398950131241190, -0.08942795157528024563, -0.3641732283464568787 ) ) ;
#64089=CARTESIAN_POINT ( 'NONE',  ( 0.6233595800524942554, -0.08942795157528024563, -0.3641732283464568787 ) ) ;
#64090=CARTESIAN_POINT ( 'NONE',  ( -1.456692913385826182, 0.2952755905511811885, 0.000000000000000000 ) ) ;
#64091=ADVANCED_FACE ( 'NONE', ( #45881 ), #58847, .F. ) ;
#64093=CARTESIAN_POINT ( 'NONE',  ( 1.259842519685040019, -0.1870078740157480879, -0.4822834645669291653 ) ) ;
#64095=CARTESIAN_POINT ( 'NONE',  ( 0.6233595800524942554, -0.05778040916215560624, -0.4822834645669293319 ) ) ;
#64097=CARTESIAN_POINT ( 'NONE',  ( -1.528871391076114250, 0.1771653543307087075, -0.09757992244046823083 ) ) ;
#64098=CARTESIAN_POINT ( 'NONE',  ( 0.1115485564304470323, 0.2952755905511811885, 0.1292274648535926551 ) ) ;
#64099=CARTESIAN_POINT ( 'NONE',  ( 0.4593175853018379162, -0.3690944881889763329, 0.3153832671262228327 ) ) ;
#64101=CARTESIAN_POINT ( 'NONE',  ( 1.076115485564305141, 0.2306618581243847221, -0.2411417322834647770 ) ) ;
#64103=CARTESIAN_POINT ( 'NONE',  ( -0.3149606299212590610, -0.1870078740157479769, 0.3641732283464567677 ) ) ;
#64104=CARTESIAN_POINT ( 'NONE',  ( -0.6364829396325453192, -0.3162353388693405765, 0.4822834645669290543 ) ) ;
#64105=CARTESIAN_POINT ( 'NONE',  ( -1.620734908136482577, 0.1771653543307087630, 0.09757992244046791164 ) ) ;
#64106=CARTESIAN_POINT ( 'NONE',  ( -1.207349081364828880, 0.2306618581243847221, -0.2411417322834647770 ) ) ;
#64107=CARTESIAN_POINT ( 'NONE',  ( 1.017060367454068803, -0.3162353388693405765, 0.4822834645669290543 ) ) ;
#64109=CARTESIAN_POINT ( 'NONE',  ( -1.240157480314959759, -0.4536011799217368745, -0.2665933059059886201 ) ) ;
#64112=CARTESIAN_POINT ( 'NONE',  ( 0.8727034120734912248, -0.3162353388693409650, -0.4822834645669289433 ) ) ;
#64114=CARTESIAN_POINT ( 'NONE',  ( -1.660104986876639543, -0.05778040916215560624, -0.4822834645669293319 ) ) ;
#64115=CARTESIAN_POINT ( 'NONE',  ( -1.437007874015747477, 0.07958543189024071263, -0.2665933059059888421 ) ) ;
#64116=CARTESIAN_POINT ( 'NONE',  ( -0.8267716535433065062, -0.5511811023622047445, 6.969142054262312111E-17 ) ) ;
#64117=CARTESIAN_POINT ( 'NONE',  ( 1.660104986876641320, -0.08942795157527998196, 0.3641732283464567121 ) ) ;
#64118=CARTESIAN_POINT ( 'NONE',  ( -0.4330708661417315697, -0.6692913385826771977, 8.415575281601705876E-17 ) ) ;
#64119=CARTESIAN_POINT ( 'NONE',  ( -0.4658792650918627265, -0.2845877964562161244, -0.3641732283464567121 ) ) ;
#64120=CARTESIAN_POINT ( 'NONE',  ( -1.430446194225721390, -0.3690944881889763329, 0.3153832671262228327 ) ) ;
#64121=CARTESIAN_POINT ( 'NONE',  ( 0.9645669291338588858, 0.07958543189024085140, 0.2665933059059887866 ) ) ;
#64122=CARTESIAN_POINT ( 'NONE',  ( 0.4265091863517067594, 0.2952755905511811885, 0.1292274648535926551 ) ) ;
#64123=CARTESIAN_POINT ( 'NONE',  ( 0.1968503937007881344, -0.5511811023622047445, 6.969142054262312111E-17 ) ) ;
#64124=CARTESIAN_POINT ( 'NONE',  ( 0.3412073490813655186, -0.6046776061558809534, -0.2411417322834644161 ) ) ;
#64125=CARTESIAN_POINT ( 'NONE',  ( 0.5643044619422579178, -0.3690944881889765550, -0.3153832671262227771 ) ) ;
#64126=AXIS2_PLACEMENT_3D ( 'NONE', #67470, #9804, #35476 ) ;
#64127=CARTESIAN_POINT ( 'NONE',  ( -1.541994750656167090, -0.6692913385826773087, -0.1292274648535924053 ) ) ;
#64128=CARTESIAN_POINT ( 'NONE',  ( -1.482939632545930975, 0.05413385826771666132, 0.4176697321401328100 ) ) ;
#64129=CARTESIAN_POINT ( 'NONE',  ( -0.3937007874015740483, -0.1870078740157480879, -0.4822834645669291653 ) ) ;
#64130=AXIS2_PLACEMENT_3D ( 'NONE', #21865, #73648, #22697 ) ;
#64133=CARTESIAN_POINT ( 'NONE',  ( 0.4396325459317590445, -0.6692913385826771977, 0.1292274648535927661 ) ) ;
#64134=CARTESIAN_POINT ( 'NONE',  ( 1.062992125984252745, -0.5511811023622047445, 6.969142054262312111E-17 ) ) ;
#64135=( GEOMETRIC_REPRESENTATION_CONTEXT ( 3 ) GLOBAL_UNCERTAINTY_ASSIGNED_CONTEXT ( ( #15894 ) ) GLOBAL_UNIT_ASSIGNED_CONTEXT ( ( #28354, #23279, #80143 ) ) REPRESENTATION_CONTEXT ( 'NONE', 'WORKASPACE' ) );
#64136=CIRCLE ( 'NONE', #49350, 1.220472440944881942 ) ;
#64137=CARTESIAN_POINT ( 'NONE',  ( -0.4855643044619415427, 0.05413385826771626580, -0.4176697321401330321 ) ) ;
#64138=CARTESIAN_POINT ( 'NONE',  ( 0.3543307086614179147, 0.2952755905511811885, 0.000000000000000000 ) ) ;
#64144=CARTESIAN_POINT ( 'NONE',  ( -0.8398950131233589023, -0.5023911411419708095, -0.1820866141732282451 ) ) ;
#64145=CARTESIAN_POINT ( 'NONE',  ( -1.154855643044618851, -0.6046776061558809534, -0.2411417322834644161 ) ) ;
#64147=CARTESIAN_POINT ( 'NONE',  ( 1.056430446194226658, 0.2952755905511811885, 0.1292274648535926551 ) ) ;
#64148=CARTESIAN_POINT ( 'NONE',  ( 1.246719160104987623, -0.4281496062992124485, 0.4176697321401328655 ) ) ;
#64149=CARTESIAN_POINT ( 'NONE',  ( 0.5708661417322841158, -0.5400638737290845981, -0.3530559997133363437 ) ) ;
#64153=CARTESIAN_POINT ( 'NONE',  ( 1.660104986876641320, -0.05778040916215522460, 0.4822834645669289988 ) ) ;
#64154=CARTESIAN_POINT ( 'NONE',  ( 0.5249343832021003964, 0.2306618581243847221, -0.2411417322834647770 ) ) ;
#64156=CARTESIAN_POINT ( 'NONE',  ( 0.1181102362204730916, -0.6692913385826771977, 8.415575281601705876E-17 ) ) ;
#64157=CARTESIAN_POINT ( 'NONE',  ( 0.6364829396325465405, -0.08942795157527998196, 0.3641732283464567121 ) ) ;
#64158=CARTESIAN_POINT ( 'NONE',  ( 1.174540682414699111, -0.3162353388693405765, 0.4822834645669290543 ) ) ;
#64160=CARTESIAN_POINT ( 'NONE',  ( 0.3018372703412079971, -0.4281496062992124485, 0.4176697321401328655 ) ) ;
#64161=CARTESIAN_POINT ( 'NONE',  ( 0.9645669291338591078, -0.5400638737290845981, -0.3530559997133363437 ) ) ;
#64162=CARTESIAN_POINT ( 'NONE',  ( 0.3018372703412079971, 0.05413385826771626580, -0.4176697321401330321 ) ) ;
#64163=CARTESIAN_POINT ( 'NONE',  ( 1.187664041994751285, -0.08942795157527998196, 0.3641732283464567121 ) ) ;
#64164=CARTESIAN_POINT ( 'NONE',  ( -0.9908136482939626788, -0.6692913385826773087, -0.1292274648535924053 ) ) ;
#64165=CARTESIAN_POINT ( 'NONE',  ( -0.9645669291338575535, -0.5400638737290844871, 0.3530559997133364547 ) ) ;
#64166=CARTESIAN_POINT ( 'NONE',  ( 1.338582677165355062, -0.1870078740157480879, -0.4822834645669291653 ) ) ;
#64173=CARTESIAN_POINT ( 'NONE',  ( 1.397637795275591177, 0.1660481256975883668, -0.3530559997133364547 ) ) ;
#64174=CARTESIAN_POINT ( 'NONE',  ( 0.8792650918635177559, -0.3690944881889765550, -0.3153832671262227771 ) ) ;
#64176=CARTESIAN_POINT ( 'NONE',  ( 1.246719160104987623, -0.004921259842519870586, -0.3153832671262229437 ) ) ;
#64177=CARTESIAN_POINT ( 'NONE',  ( 0.6188235755478038724, 2.084810923686589862E-15, -0.3954974714151459625 ) ) ;
#64181=CARTESIAN_POINT ( 'NONE',  ( -0.7808398950131222316, -0.2845877964562161244, -0.3641732283464567121 ) ) ;
#64182=CARTESIAN_POINT ( 'NONE',  ( -1.430446194225721390, -0.3690944881889763329, 0.3153832671262228327 ) ) ;
#64183=CARTESIAN_POINT ( 'NONE',  ( -1.227034120734907141, -0.6692913385826773087, -0.1292274648535924053 ) ) ;
#64184=CARTESIAN_POINT ( 'NONE',  ( -0.04593175853018302557, -0.6692913385826773087, -0.1292274648535924053 ) ) ;
#64185=CARTESIAN_POINT ( 'NONE',  ( 1.476377952755906220, 0.1660481256975883668, -0.3530559997133364547 ) ) ;
#64187=CARTESIAN_POINT ( 'NONE',  ( -1.128608923884513837, 0.1539470093639521697, -0.1968503937007875793 ) ) ;
#64189=LINE ( 'NONE', #6524, #47863 ) ;
#64190=DIRECTION ( 'NONE',  ( 0.000000000000000000, 0.000000000000000000, 1.000000000000000000 ) ) ;
#64191=CARTESIAN_POINT ( 'NONE',  ( -0.8005249343832011588, -0.004921259842519870586, -0.3153832671262229437 ) ) ;
#64192=CARTESIAN_POINT ( 'NONE',  ( -1.181102362204723644, -0.1870078740157479769, 0.4822834645669291653 ) ) ;
#64193=CARTESIAN_POINT ( 'NONE',  ( 0.8727034120734913358, -0.05778040916215522460, 0.4822834645669289988 ) ) ;
#64194=CONICAL_SURFACE ( 'NONE', #76282, 1.220472440944881942, 0.7853981633974621568 ) ;
#64196=DIRECTION ( 'NONE',  ( -1.000000000000000000, 0.000000000000000000, 0.000000000000000000 ) ) ;
#64198=CARTESIAN_POINT ( 'NONE',  ( 1.017060367454068803, -0.3162353388693405765, 0.4822834645669290543 ) ) ;
#64199=CARTESIAN_POINT ( 'NONE',  ( -1.312335958005248715, -0.6046776061558809534, -0.2411417322834644161 ) ) ;
#64201=CARTESIAN_POINT ( 'NONE',  ( -0.5118110236220466680, -0.5511811023622047445, 6.969142054262312111E-17 ) ) ;
#64203=CARTESIAN_POINT ( 'NONE',  ( -0.6233595800524928121, -0.2845877964562161244, -0.3641732283464567121 ) ) ;
#64204=CARTESIAN_POINT ( 'NONE',  ( 0.2362204724409456558, -0.1870078740157480601, -0.3641732283464567677 ) ) ;
#64205=CARTESIAN_POINT ( 'NONE',  ( 0.1049868766404206816, -0.6046776061558809534, -0.2411417322834644161 ) ) ;
#64206=CARTESIAN_POINT ( 'NONE',  ( -1.338582677165353729, -0.1870078740157479769, 0.3641732283464567677 ) ) ;
#64208=CARTESIAN_POINT ( 'NONE',  ( 1.049868766404200127, -0.6046776061558809534, -0.2411417322834644161 ) ) ;
#64209=CARTESIAN_POINT ( 'NONE',  ( -1.463254593175852492, 0.2952755905511811885, 0.1292274648535926551 ) ) ;
#64211=CARTESIAN_POINT ( 'NONE',  ( -0.5380577427821514602, -0.4281496062992127816, -0.4176697321401328100 ) ) ;
#64212=CARTESIAN_POINT ( 'NONE',  ( -0.8005249343832011588, 0.05413385826771626580, -0.4176697321401330321 ) ) ;
#64213=CARTESIAN_POINT ( 'NONE',  ( 0.6299212598425204535, -0.1870078740157480601, -0.3641732283464567677 ) ) ;
#64214=CARTESIAN_POINT ( 'NONE',  ( -0.2624671916010490880, 0.1283753931104746893, -0.1820866141732285504 ) ) ;
#64215=CARTESIAN_POINT ( 'NONE',  ( -0.4396325459317579898, 0.2952755905511811885, 0.1292274648535926551 ) ) ;
#64216=CARTESIAN_POINT ( 'NONE',  ( -1.345144356955379816, -0.3162353388693405765, 0.4822834645669290543 ) ) ;
#64218=CARTESIAN_POINT ( 'NONE',  ( 1.187664041994751285, -0.08942795157527998196, 0.3641732283464567121 ) ) ;
#64219=CARTESIAN_POINT ( 'NONE',  ( -0.09842519685039295696, -0.5400638737290844871, 0.3530559997133364547 ) ) ;
#64220=CARTESIAN_POINT ( 'NONE',  ( -1.528871391076114250, 0.2952755905511810774, -0.1292274648535930714 ) ) ;
#64223=CARTESIAN_POINT ( 'NONE',  ( -0.8267716535433065062, 0.1771653543307087630, 0.000000000000000000 ) ) ;
#64224=CARTESIAN_POINT ( 'NONE',  ( 0.9448818897637802916, -0.1870078740157479769, 0.4822834645669291653 ) ) ;
#64225=CARTESIAN_POINT ( 'NONE',  ( -1.141732283464566011, -0.5511811023622047445, 6.969142054262312111E-17 ) ) ;
#64227=CARTESIAN_POINT ( 'NONE',  ( -0.8398950131233589023, -0.6046776061558809534, -0.2411417322834644161 ) ) ;
#64228=CARTESIAN_POINT ( 'NONE',  ( 0.7217847769028878924, 0.05413385826771666132, 0.4176697321401328100 ) ) ;
#64229=CARTESIAN_POINT ( 'NONE',  ( 0.5708661417322842269, 0.1660481256975885056, 0.3530559997133364547 ) ) ;
#64230=CARTESIAN_POINT ( 'NONE',  ( 1.430446194225722500, 0.05413385826771666132, 0.4176697321401328100 ) ) ;
#64231=CARTESIAN_POINT ( 'NONE',  ( -1.515748031496062076, 0.07958543189024071263, -0.2665933059059888421 ) ) ;
#64236=CARTESIAN_POINT ( 'NONE',  ( 1.056430446194226658, 0.1771653543307087630, 0.09757992244046791164 ) ) ;
#64237=CARTESIAN_POINT ( 'NONE',  ( 0.4002624671916016896, -0.2845877964562161244, -0.3641732283464567121 ) ) ;
#64238=CARTESIAN_POINT ( 'NONE',  ( 0.2755905511811031494, -0.6692913385826771977, 8.415575281601705876E-17 ) ) ;
#64239=CARTESIAN_POINT ( 'NONE',  ( 1.174540682414699111, -0.05778040916215560624, -0.4822834645669293319 ) ) ;
#64241=CARTESIAN_POINT ( 'NONE',  ( 0.3740157480314966754, -0.4536011799217367080, 0.2665933059059888421 ) ) ;
#64242=CARTESIAN_POINT ( 'NONE',  ( -0.8267716535433065062, 0.2952755905511811885, 0.000000000000000000 ) ) ;
#64243=CARTESIAN_POINT ( 'NONE',  ( -1.417322834645668772, -0.1870078740157480879, -0.4822834645669291653 ) ) ;
#64244=CARTESIAN_POINT ( 'NONE',  ( 0.9383202099737538715, -0.05778040916215560624, -0.4822834645669293319 ) ) ;
#64249=EDGE_LOOP ( 'NONE', ( #27110, #66763, #54910, #3074, #51608, #22150, #39421 ) ) ;
#64250=CARTESIAN_POINT ( 'NONE',  ( -1.174540682414697335, -0.3162353388693409650, -0.4822834645669289433 ) ) ;
#64251=CARTESIAN_POINT ( 'NONE',  ( -0.6561679790026240244, 0.2306618581243847221, -0.2411417322834647770 ) ) ;
#64252=CARTESIAN_POINT ( 'NONE',  ( -0.7939632545931750718, -0.08942795157528024563, -0.3641732283464568787 ) ) ;
#64253=CARTESIAN_POINT ( 'NONE',  ( -0.7939632545931750718, -0.05778040916215560624, -0.4822834645669293319 ) ) ;
#64256=CARTESIAN_POINT ( 'NONE',  ( 1.692913385826772421, 0.2952755905511811885, 0.000000000000000000 ) ) ;
#64257=CARTESIAN_POINT ( 'NONE',  ( -1.135170603674539924, -0.6692913385826771977, 0.1292274648535927661 ) ) ;
#64258=CARTESIAN_POINT ( 'NONE',  ( 0.4593175853018379162, -0.4281496062992124485, 0.4176697321401328655 ) ) ;
#64259=CARTESIAN_POINT ( 'NONE',  ( -0.6955380577427815458, 0.05413385826771666132, 0.4176697321401328100 ) ) ;
#64261=CARTESIAN_POINT ( 'NONE',  ( -0.7217847769028863381, -0.3690944881889763329, 0.3153832671262228327 ) ) ;
#64265=CARTESIAN_POINT ( 'NONE',  ( -1.515748031496062076, 0.07958543189024071263, -0.2665933059059888421 ) ) ;
#64266=CARTESIAN_POINT ( 'NONE',  ( -1.220472440944881054, -0.6692913385826771977, 8.415575281601705876E-17 ) ) ;
#64267=CARTESIAN_POINT ( 'NONE',  ( -0.9055118110236215490, -0.6692913385826771977, 8.415575281601705876E-17 ) ) ;
#64269=CARTESIAN_POINT ( 'NONE',  ( -1.148293963254592542, -0.6692913385826773087, -0.1292274648535924053 ) ) ;
#64270=CARTESIAN_POINT ( 'NONE',  ( -1.345144356955379816, -0.05778040916215560624, -0.4822834645669293319 ) ) ;
#64271=CARTESIAN_POINT ( 'NONE',  ( -0.8464566929133852113, 0.1660481256975885056, 0.3530559997133364547 ) ) ;
#64272=CARTESIAN_POINT ( 'NONE',  ( 0.3543307086614181922, -0.5511811023622047445, 6.969142054262312111E-17 ) ) ;
#64273=CARTESIAN_POINT ( 'NONE',  ( 1.614173228346456712, 0.4410134679336843999, 0.1372047244094478646 ) ) ;
#64275=CARTESIAN_POINT ( 'NONE',  ( -0.4461942257217840213, 0.1283753931104748280, 0.1820866141732283561 ) ) ;
#64276=CARTESIAN_POINT ( 'NONE',  ( -0.6692913385826764205, 0.2952755905511811885, 0.000000000000000000 ) ) ;
#64277=CARTESIAN_POINT ( 'NONE',  ( 1.207349081364829990, -0.6046776061558809534, -0.2411417322834644161 ) ) ;
#64278=CARTESIAN_POINT ( 'NONE',  ( -0.6299212598425188991, -0.1870078740157480879, -0.4822834645669291653 ) ) ;
#64279=EDGE_LOOP ( 'NONE', ( #60616, #15202, #27626, #5268, #41489, #80417, #82087, #33294, #26709, #16731, #28244, #67359, #10770, #57021, #13267, #50336, #71184, #9522, #31109, #74032, #28952, #59609, #58462, #5348, #62984, #73511, #49660, #18207, #75735, #77842 ) ) ;
#64282=CARTESIAN_POINT ( 'NONE',  ( -1.089238845144356427, -0.4281496062992127816, -0.4176697321401328100 ) ) ;
#64283=CARTESIAN_POINT ( 'NONE',  ( 1.181102362204724976, -0.1870078740157480879, -0.4822834645669291653 ) ) ;
#64284=CARTESIAN_POINT ( 'NONE',  ( -1.036745406824146176, -0.004921259842519870586, -0.3153832671262229437 ) ) ;
#64285=CARTESIAN_POINT ( 'NONE',  ( -1.594488188976377563, -0.5400638737290844871, 0.3530559997133364547 ) ) ;
#64290=CARTESIAN_POINT ( 'NONE',  ( 0.2952755905511819101, 0.1660481256975883668, -0.3530559997133364547 ) ) ;
#64291=CARTESIAN_POINT ( 'NONE',  ( -0.9645669291338575535, 0.07958543189024071263, -0.2665933059059888421 ) ) ;
#64292=CARTESIAN_POINT ( 'NONE',  ( -0.7742782152230965886, 0.05413385826771666132, 0.4176697321401328100 ) ) ;
#64294=CARTESIAN_POINT ( 'NONE',  ( -1.272965879265091305, -0.4281496062992124485, 0.4176697321401328655 ) ) ;
#64295=CARTESIAN_POINT ( 'NONE',  ( -0.8530183727034112984, -0.4281496062992127816, -0.4176697321401328100 ) ) ;
#64296=CARTESIAN_POINT ( 'NONE',  ( -0.1640419947506555343, -0.3162353388693405765, 0.4822834645669290543 ) ) ;
#64298=CARTESIAN_POINT ( 'NONE',  ( 0.8530183727034126306, -0.004921259842519870586, -0.3153832671262229437 ) ) ;
#64299=CARTESIAN_POINT ( 'NONE',  ( -0.6496062992125976043, -0.4536011799217367080, 0.2665933059059888421 ) ) ;
#64301=CARTESIAN_POINT ( 'NONE',  ( 0.5511811023622055217, -0.1870078740157479769, 0.3641732283464567677 ) ) ;
#64302=CARTESIAN_POINT ( 'NONE',  ( 1.259842519685040019, -0.1870078740157479769, 0.3641732283464567677 ) ) ;
#64303=CARTESIAN_POINT ( 'NONE',  ( 1.240157480314961314, -0.5400638737290844871, 0.3530559997133364547 ) ) ;
#64304=CARTESIAN_POINT ( 'NONE',  ( 0.1377952755905518800, 0.07958543189024071263, -0.2665933059059888421 ) ) ;
#64306=CARTESIAN_POINT ( 'NONE',  ( -0.9645669291338575535, 0.1660481256975883668, -0.3530559997133364547 ) ) ;
#64307=CARTESIAN_POINT ( 'NONE',  ( 1.286089238845145033, 0.2306618581243848609, 0.2411417322834645549 ) ) ;
#64309=CARTESIAN_POINT ( 'NONE',  ( -0.4396325459317577122, -0.5511811023622048555, -0.09757992244046775898 ) ) ;
#64311=CARTESIAN_POINT ( 'NONE',  ( 0.3412073490813655186, -0.6046776061558809534, -0.2411417322834644161 ) ) ;
#64313=CARTESIAN_POINT ( 'NONE',  ( 0.8464566929133865436, 0.07958543189024071263, -0.2665933059059888421 ) ) ;
#64314=CARTESIAN_POINT ( 'NONE',  ( 0.2165354330708668673, 0.07958543189024071263, -0.2665933059059888421 ) ) ;
#64315=CARTESIAN_POINT ( 'NONE',  ( -0.01968503937007793844, 0.1660481256975883668, -0.3530559997133364547 ) ) ;
#64316=CARTESIAN_POINT ( 'NONE',  ( -1.174540682414697335, -0.3162353388693409650, -0.4822834645669289433 ) ) ;
#64317=CARTESIAN_POINT ( 'NONE',  ( -0.9055118110236215490, -0.5511811023622047445, 6.969142054262312111E-17 ) ) ;
#64319=CARTESIAN_POINT ( 'NONE',  ( -0.5446194225721777693, -0.05778040916215522460, 0.4822834645669289988 ) ) ;
#64322=CARTESIAN_POINT ( 'NONE',  ( 0.2755905511811031494, -0.5511811023622047445, 6.969142054262312111E-17 ) ) ;
#64323=CARTESIAN_POINT ( 'NONE',  ( -0.6758530183727028406, 0.2952755905511811885, 0.1292274648535926551 ) ) ;
#64324=CARTESIAN_POINT ( 'NONE',  ( -1.220472440944881054, -0.6692913385826771977, 8.415575281601705876E-17 ) ) ;
#64325=CARTESIAN_POINT ( 'NONE',  ( -1.345144356955379816, -0.2845877964562159024, 0.3641732283464567677 ) ) ;
#64326=CARTESIAN_POINT ( 'NONE',  ( 1.633858267716535639, -0.5400638737290844871, 0.3530559997133364547 ) ) ;
#64327=CARTESIAN_POINT ( 'NONE',  ( -0.4461942257217840213, -0.6046776061558809534, -0.2411417322834644161 ) ) ;
#64328=CARTESIAN_POINT ( 'NONE',  ( -0.7545931758530176614, -0.5511811023622048555, -0.09757992244046775898 ) ) ;
#64329=CARTESIAN_POINT ( 'NONE',  ( -1.548556430446193399, 0.1283753931104748280, 0.1820866141732283561 ) ) ;
#64330=CARTESIAN_POINT ( 'NONE',  ( 1.417322834645670104, -0.1870078740157479769, 0.4822834645669291653 ) ) ;
#64333=ORIENTED_EDGE ( 'NONE', *, *, #43698, .T. ) ;
#64335=CARTESIAN_POINT ( 'NONE',  ( -1.377952755905511140, 0.2952755905511811885, 0.000000000000000000 ) ) ;
#64336=CARTESIAN_POINT ( 'NONE',  ( -0.8267716535433065062, -0.6692913385826771977, 8.415575281601705876E-17 ) ) ;
#64337=CARTESIAN_POINT ( 'NONE',  ( -1.561679790026246017, -0.4281496062992127816, -0.4176697321401328100 ) ) ;
#64339=CARTESIAN_POINT ( 'NONE',  ( 1.437007874015748810, -0.4536011799217368745, -0.2665933059059886201 ) ) ;
#64341=CARTESIAN_POINT ( 'NONE',  ( 0.4199475065616805614, 0.2306618581243848609, 0.2411417322834645549 ) ) ;
#64342=CARTESIAN_POINT ( 'NONE',  ( -0.1312335958005241554, -0.6046776061558809534, -0.2411417322834644161 ) ) ;
#64343=CARTESIAN_POINT ( 'NONE',  ( -0.6962418744208963561, -2.294479370626195693E-15, 0.3464511005275217603 ) ) ;
#64344=CARTESIAN_POINT ( 'NONE',  ( -0.6415071261929207180, 0.02791078216816347476, -0.4328096321851898631 ) ) ;
#64345=CARTESIAN_POINT ( 'NONE',  ( 0.8989501312335963501, -0.5511811023622048555, -0.09757992244046775898 ) ) ;
#64347=VERTEX_POINT ( 'NONE', #28205 ) ;
#64350=CARTESIAN_POINT ( 'NONE',  ( -0.1246719160104980823, 0.2952755905511811885, 0.1292274648535926551 ) ) ;
#64351=CARTESIAN_POINT ( 'NONE',  ( -0.6496062992125976043, -0.5400638737290844871, 0.3530559997133364547 ) ) ;
#64352=CARTESIAN_POINT ( 'NONE',  ( -1.456692913385826182, 0.2952755905511811885, 0.000000000000000000 ) ) ;
#64353=CARTESIAN_POINT ( 'NONE',  ( 0.7217847769028878924, 0.05413385826771666132, 0.4176697321401328100 ) ) ;
#64354=CARTESIAN_POINT ( 'NONE',  ( 1.633858267716535639, -0.5400638737290844871, 0.3530559997133364547 ) ) ;
#64355=CARTESIAN_POINT ( 'NONE',  ( 1.391076115485564868, -0.6046776061558807314, 0.2411417322834647770 ) ) ;
#64356=CARTESIAN_POINT ( 'NONE',  ( -0.5380577427821514602, 0.05413385826771666132, 0.4176697321401328100 ) ) ;
#64357=CARTESIAN_POINT ( 'NONE',  ( 0.4724409448818904789, -0.1870078740157479769, 0.4822834645669291653 ) ) ;
#64358=CARTESIAN_POINT ( 'NONE',  ( 1.509186351706037543, -0.4281496062992127816, -0.4176697321401328100 ) ) ;
#64359=CARTESIAN_POINT ( 'NONE',  ( 1.272965879265092637, 0.05413385826771666132, 0.4176697321401328100 ) ) ;
#64360=CARTESIAN_POINT ( 'NONE',  ( 1.541994750656168645, 0.2952755905511810774, -0.1292274648535930714 ) ) ;
#64361=CARTESIAN_POINT ( 'NONE',  ( -0.2559055118110230564, 0.1660481256975883668, -0.3530559997133364547 ) ) ;
#64363=CARTESIAN_POINT ( 'NONE',  ( 0.5643044619422579178, -0.004921259842519576551, 0.3153832671262227771 ) ) ;
#64367=CARTESIAN_POINT ( 'NONE',  ( -0.5052493438320203589, -0.5511811023622046335, 0.09757992244046803654 ) ) ;
#64369=CARTESIAN_POINT ( 'NONE',  ( 0.2755905511811031494, -0.6692913385826771977, 8.415575281601705876E-17 ) ) ;
#64370=CARTESIAN_POINT ( 'NONE',  ( 0.07217847769028949700, -0.05778040916215560624, -0.4822834645669293319 ) ) ;
#64371=CARTESIAN_POINT ( 'NONE',  ( -0.9383202099737524282, -0.05778040916215522460, 0.4822834645669289988 ) ) ;
#64373=CARTESIAN_POINT ( 'NONE',  ( -1.056430446194224881, -0.6692913385826771977, 0.1292274648535927661 ) ) ;
#64375=CARTESIAN_POINT ( 'NONE',  ( 0.8595800524934390507, -0.08942795157528024563, -0.3641732283464568787 ) ) ;
#64376=CARTESIAN_POINT ( 'NONE',  ( 0.6692913385826778638, -0.6692913385826771977, 8.415575281601705876E-17 ) ) ;
#64377=CARTESIAN_POINT ( 'NONE',  ( 0.8464566929133866546, -0.5400638737290844871, 0.3530559997133364547 ) ) ;
#64378=EDGE_CURVE ( 'NONE', #73939, #72992, #62874, .T. ) ;
#64380=CARTESIAN_POINT ( 'NONE',  ( -1.627296587926508442, -0.6046776061558809534, -0.2411417322834644161 ) ) ;
#64383=CARTESIAN_POINT ( 'NONE',  ( 0.07217847769028949700, -0.05778040916215560624, -0.4822834645669293319 ) ) ;
#64386=CARTESIAN_POINT ( 'NONE',  ( -1.318897637795274802, 0.07958543189024085140, 0.2665933059059887866 ) ) ;
#64387=CARTESIAN_POINT ( 'NONE',  ( 1.148293963254593653, 0.2952755905511810774, -0.1292274648535930714 ) ) ;
#64388=CARTESIAN_POINT ( 'NONE',  ( 1.410761154855643795, -0.05778040916215560624, -0.4822834645669293319 ) ) ;
#64389=CARTESIAN_POINT ( 'NONE',  ( 0.3740157480314966754, -0.4536011799217367080, 0.2665933059059888421 ) ) ;
#64390=CARTESIAN_POINT ( 'NONE',  ( 0.5052493438320215802, 0.2952755905511811885, 0.1292274648535926551 ) ) ;
#64392=CARTESIAN_POINT ( 'NONE',  ( 0.3412073490813655186, -0.5023911411419708095, -0.1820866141732282451 ) ) ;
#64393=CARTESIAN_POINT ( 'NONE',  ( -0.07874015748031421014, -0.1870078740157480879, -0.4822834645669291653 ) ) ;
#64395=CARTESIAN_POINT ( 'NONE',  ( -1.148293963254592542, -0.6692913385826773087, -0.1292274648535924053 ) ) ;
#64396=CARTESIAN_POINT ( 'NONE',  ( 0.5577427821522314977, -0.2845877964562161244, -0.3641732283464567121 ) ) ;
#64397=CARTESIAN_POINT ( 'NONE',  ( 0.4849061582275022153, 1.805669738366188382, 0.4921425059946344938 ) ) ;
#64398=CARTESIAN_POINT ( 'NONE',  ( -0.7020997375328076329, -0.3162353388693409650, -0.4822834645669289433 ) ) ;
#64399=CARTESIAN_POINT ( 'NONE',  ( -0.4593175853018364174, -0.3690944881889765550, -0.3153832671262227771 ) ) ;
#64401=CARTESIAN_POINT ( 'NONE',  ( -0.3477690288713905509, -0.6692913385826771977, 0.1292274648535927661 ) ) ;
#64402=CARTESIAN_POINT ( 'NONE',  ( -0.2690288713910754526, -0.6692913385826771977, 0.1292274648535927661 ) ) ;
#64403=CARTESIAN_POINT ( 'NONE',  ( 0.4265091863517067039, -0.5511811023622048555, -0.09757992244046775898 ) ) ;
#64405=CARTESIAN_POINT ( 'NONE',  ( -0.1443569553805765515, -0.4281496062992127816, -0.4176697321401328100 ) ) ;
#64408=CARTESIAN_POINT ( 'NONE',  ( 0.8792650918635177559, -0.004921259842519576551, 0.3153832671262227771 ) ) ;
#64409=CARTESIAN_POINT ( 'NONE',  ( 1.332020997375328974, -0.05778040916215560624, -0.4822834645669293319 ) ) ;
#64410=CARTESIAN_POINT ( 'NONE',  ( -0.8661417322834640276, -0.1870078740157480601, -0.3641732283464567677 ) ) ;
#64411=CARTESIAN_POINT ( 'NONE',  ( -0.6889763779527552368, -0.4536011799217368745, -0.2665933059059886201 ) ) ;
#64412=CARTESIAN_POINT ( 'NONE',  ( -0.7480314960629914633, -0.6692913385826771977, 8.415575281601705876E-17 ) ) ;
#64413=CARTESIAN_POINT ( 'NONE',  ( 0.01312335958005323398, 0.05413385826771666132, 0.4176697321401328100 ) ) ;
#64414=CARTESIAN_POINT ( 'NONE',  ( 0.7349081364829403995, 0.1283753931104748280, 0.1820866141732283561 ) ) ;
#64415=CARTESIAN_POINT ( 'NONE',  ( 1.614173228346457156, 1.929133858267716661, -0.5309055118110239668 ) ) ;
#64416=CARTESIAN_POINT ( 'NONE',  ( 1.207349081364829990, -0.5023911411419708095, -0.1820866141732282451 ) ) ;
#64417=CARTESIAN_POINT ( 'NONE',  ( 0.6102362204724416372, 0.1660481256975883668, -0.3530559997133364547 ) ) ;
#64419=CARTESIAN_POINT ( 'NONE',  ( -0.09842519685039295696, 0.1660481256975883668, -0.3530559997133364547 ) ) ;
#64421=CARTESIAN_POINT ( 'NONE',  ( 1.587926509186352142, -0.004921259842519576551, 0.3153832671262227771 ) ) ;
#64422=CARTESIAN_POINT ( 'NONE',  ( 1.082677165354331228, 0.1660481256975883668, -0.3530559997133364547 ) ) ;
#64424=CARTESIAN_POINT ( 'NONE',  ( 0.3412073490813655186, -0.6046776061558809534, -0.2411417322834644161 ) ) ;
#64426=CARTESIAN_POINT ( 'NONE',  ( 0.2624671916010504757, 0.1283753931104748280, 0.1820866141732283561 ) ) ;
#64427=CARTESIAN_POINT ( 'NONE',  ( 0.9186351706036752773, 0.2306618581243847221, -0.2411417322834647770 ) ) ;
#64428=CARTESIAN_POINT ( 'NONE',  ( -0.1509186351706028884, -0.08942795157527998196, 0.3641732283464567121 ) ) ;
#64429=CARTESIAN_POINT ( 'NONE',  ( -0.7677165354330699465, -0.5400638737290845981, -0.3530559997133363437 ) ) ;
#64431=CARTESIAN_POINT ( 'NONE',  ( -0.2559055118110230564, 0.1660481256975883668, -0.3530559997133364547 ) ) ;
#64432=CARTESIAN_POINT ( 'NONE',  ( -1.404199475065615932, -0.4281496062992127816, -0.4176697321401328100 ) ) ;
#64433=CARTESIAN_POINT ( 'NONE',  ( -0.7677165354330699465, 0.07958543189024085140, 0.2665933059059887866 ) ) ;
#64434=CARTESIAN_POINT ( 'NONE',  ( 0.2099737532808405305, 0.2306618581243847221, -0.2411417322834647770 ) ) ;
#64435=CARTESIAN_POINT ( 'NONE',  ( -1.108923884514435132, -0.3162353388693405765, 0.4822834645669290543 ) ) ;
#64436=CARTESIAN_POINT ( 'NONE',  ( -0.2165354330708654795, 0.1660481256975885056, 0.3530559997133364547 ) ) ;
#64438=CARTESIAN_POINT ( 'NONE',  ( 1.266404199475066328, -0.05778040916215522460, 0.4822834645669289988 ) ) ;
#64439=CARTESIAN_POINT ( 'NONE',  ( 1.338582677165355062, -0.1870078740157479769, 0.4822834645669291653 ) ) ;
#64441=CARTESIAN_POINT ( 'NONE',  ( 0.4849061582275024929, 1.726086921369708538, -0.4921425059946356040 ) ) ;
#64442=CARTESIAN_POINT ( 'NONE',  ( -0.9776902887139098386, -0.6692913385826771977, 0.1292274648535927661 ) ) ;
#64446=CARTESIAN_POINT ( 'NONE',  ( -0.2427821522309703550, -0.2845877964562159024, 0.3641732283464567677 ) ) ;
#64449=CARTESIAN_POINT ( 'NONE',  ( 0.3937007874015754361, -0.1870078740157480879, -0.4822834645669291653 ) ) ;
#64450=CARTESIAN_POINT ( 'NONE',  ( 0.6430446194225728496, 0.05413385826771666132, 0.4176697321401328100 ) ) ;
#64451=DIRECTION ( 'NONE',  ( 0.000000000000000000, -1.000000000000000000, 0.000000000000000000 ) ) ;
#64452=CARTESIAN_POINT ( 'NONE',  ( -0.5392480709929732274, -4.055231247046636510E-15, 0.3627989612356165572 ) ) ;
#64453=CARTESIAN_POINT ( 'NONE',  ( -0.4330708661417315697, -0.5511811023622047445, 6.969142054262312111E-17 ) ) ;
#64454=CARTESIAN_POINT ( 'NONE',  ( 0.3543307086614179147, 0.2952755905511811885, 0.000000000000000000 ) ) ;
#64455=CARTESIAN_POINT ( 'NONE',  ( 0.8595800524934390507, -0.3162353388693405765, 0.4822834645669290543 ) ) ;
#64456=CARTESIAN_POINT ( 'NONE',  ( 0.9055118110236227702, -0.5511811023622047445, 6.969142054262312111E-17 ) ) ;
#64457=CARTESIAN_POINT ( 'NONE',  ( -0.6036745406824141069, -0.6046776061558809534, -0.2411417322834644161 ) ) ;
#64459=CARTESIAN_POINT ( 'NONE',  ( -0.8464566929133852113, 0.1660481256975885056, 0.3530559997133364547 ) ) ;
#64460=CARTESIAN_POINT ( 'NONE',  ( -1.213910761154854745, 0.1771653543307087075, -0.09757992244046823083 ) ) ;
#64461=CARTESIAN_POINT ( 'NONE',  ( -1.010498687664041384, -0.4281496062992127816, -0.4176697321401328100 ) ) ;
#64462=CARTESIAN_POINT ( 'NONE',  ( 1.200787401574803681, 0.1660481256975885056, 0.3530559997133364547 ) ) ;
#64464=ORIENTED_EDGE ( 'NONE', *, *, #37751, .F. ) ;
#64466=CARTESIAN_POINT ( 'NONE',  ( 0.1968503937007881344, -0.6692913385826771977, 8.415575281601705876E-17 ) ) ;
#64468=CARTESIAN_POINT ( 'NONE',  ( -0.9186351706036736120, 0.2306618581243848609, 0.2411417322834645549 ) ) ;
#64469=CARTESIAN_POINT ( 'NONE',  ( 1.522309711286089939, -0.6046776061558809534, -0.2411417322834644161 ) ) ;
#64470=CARTESIAN_POINT ( 'NONE',  ( 1.430446194225722500, 0.05413385826771666132, 0.4176697321401328100 ) ) ;
#64471=CARTESIAN_POINT ( 'NONE',  ( 0.5971128608923890191, -0.6692913385826771977, 0.1292274648535927661 ) ) ;
#64472=CARTESIAN_POINT ( 'NONE',  ( 0.1771653543307093182, -0.5400638737290845981, -0.3530559997133363437 ) ) ;
#64474=CARTESIAN_POINT ( 'NONE',  ( -1.069553805774277722, 0.2952755905511811885, 0.1292274648535926551 ) ) ;
#64475=CARTESIAN_POINT ( 'NONE',  ( -0.03280839895013062252, 0.2952755905511810774, -0.1292274648535930714 ) ) ;
#64476=CARTESIAN_POINT ( 'NONE',  ( -0.2034120734908128059, 0.1771653543307087630, 0.09757992244046791164 ) ) ;
#64478=EDGE_CURVE ( 'NONE', #64485, #4208, #74127, .T. ) ;
#64479=CARTESIAN_POINT ( 'NONE',  ( -0.2230971128608915943, -0.4281496062992127816, -0.4176697321401328100 ) ) ;
#64480=CARTESIAN_POINT ( 'NONE',  ( 0.2690288713910768403, 0.2066929133858267931, 0.1054918080437490802 ) ) ;
#64481=CARTESIAN_POINT ( 'NONE',  ( 1.200787401574803681, -0.5400638737290845981, -0.3530559997133363437 ) ) ;
#64482=FACE_OUTER_BOUND ( 'NONE', #54231, .T. ) ;
#64485=VERTEX_POINT ( 'NONE', #80815 ) ;
#64486=CARTESIAN_POINT ( 'NONE',  ( 0.2099737532808405305, -0.6046776061558807314, 0.2411417322834647770 ) ) ;
#64487=CARTESIAN_POINT ( 'NONE',  ( -0.4002624671916004129, -0.08942795157528024563, -0.3641732283464568787 ) ) ;
#64488=CARTESIAN_POINT ( 'NONE',  ( 1.515748031496063408, 0.07958543189024085140, 0.2665933059059887866 ) ) ;
#64489=LINE ( 'NONE', #12321, #3483 ) ;
#64491=CARTESIAN_POINT ( 'NONE',  ( 1.666666666666667185, -0.004921259842519576551, 0.3153832671262227771 ) ) ;
#64492=CARTESIAN_POINT ( 'NONE',  ( 1.574803149606299746, -0.1870078740157479769, 0.4822834645669291653 ) ) ;
#64494=CARTESIAN_POINT ( 'NONE',  ( 0.2493438320209980519, -0.4281496062992127816, -0.4176697321401328100 ) ) ;
#64496=CARTESIAN_POINT ( 'NONE',  ( -1.417322834645668772, -0.1870078740157479769, 0.4822834645669291653 ) ) ;
#64497=CARTESIAN_POINT ( 'NONE',  ( 0.3149606299212603933, -0.1870078740157479769, 0.4822834645669291653 ) ) ;
#64499=CARTESIAN_POINT ( 'NONE',  ( 1.522309711286089939, 0.2306618581243848609, 0.2411417322834645549 ) ) ;
#64500=CARTESIAN_POINT ( 'NONE',  ( 0.8202099737532813073, 0.2952755905511811885, 0.1292274648535926551 ) ) ;
#64501=CARTESIAN_POINT ( 'NONE',  ( 1.135170603674541256, -0.5511811023622048555, -0.09757992244046775898 ) ) ;
#64502=DIRECTION ( 'NONE',  ( 0.000000000000000000, 0.000000000000000000, 1.000000000000000000 ) ) ;
#64503=CARTESIAN_POINT ( 'NONE',  ( 0.9448818897637802916, -0.1870078740157480601, -0.3641732283464567677 ) ) ;
#64504=CARTESIAN_POINT ( 'NONE',  ( -1.404199475065615932, -0.4281496062992127816, -0.4176697321401328100 ) ) ;
#64506=CARTESIAN_POINT ( 'NONE',  ( 0.9776902887139113929, -0.6692913385826773087, -0.1292274648535924053 ) ) ;
#64509=EDGE_CURVE ( 'NONE', #22644, #8180, #3784, .T. ) ;
#64510=CARTESIAN_POINT ( 'NONE',  ( 0.5708661417322842269, 0.1660481256975885056, 0.3530559997133364547 ) ) ;
#64512=CARTESIAN_POINT ( 'NONE',  ( -1.706036745406823485, 0.1283753931104748280, 0.1820866141732283561 ) ) ;
#64513=CARTESIAN_POINT ( 'NONE',  ( 0.6364829396325465405, -0.08942795157527998196, 0.3641732283464567121 ) ) ;
#64514=CARTESIAN_POINT ( 'NONE',  ( 0.5905511811023629321, 0.2952755905511811885, 0.000000000000000000 ) ) ;
#64516=CARTESIAN_POINT ( 'NONE',  ( -0.8267716535433065062, -0.5511811023622047445, 6.969142054262312111E-17 ) ) ;
#64517=CARTESIAN_POINT ( 'NONE',  ( -0.5183727034120726440, -0.6692913385826773087, -0.1292274648535924053 ) ) ;
#64518=CARTESIAN_POINT ( 'NONE',  ( -1.601049868766403650, 0.1283753931104746893, -0.1820866141732285504 ) ) ;
#64519=CARTESIAN_POINT ( 'NONE',  ( -1.030183727034119867, -0.05778040916215560624, -0.4822834645669293319 ) ) ;
#64520=CARTESIAN_POINT ( 'NONE',  ( 0.9120734908136490793, 0.2952755905511810774, -0.1292274648535930714 ) ) ;
#64522=CARTESIAN_POINT ( 'NONE',  ( -1.174540682414697335, -0.08942795157527998196, 0.3641732283464567121 ) ) ;
#64524=CARTESIAN_POINT ( 'NONE',  ( 0.9973753280839902091, 0.2306618581243847221, -0.2411417322834647770 ) ) ;
#64526=CARTESIAN_POINT ( 'NONE',  ( -1.699475065616797398, 0.2952755905511811885, 0.1292274648535926551 ) ) ;
#64527=CARTESIAN_POINT ( 'NONE',  ( 1.292650918635171564, -0.6692913385826773087, -0.1292274648535924053 ) ) ;
#64528=CARTESIAN_POINT ( 'NONE',  ( -1.115485564304461219, -0.3690944881889763329, 0.3153832671262228327 ) ) ;
#64529=CARTESIAN_POINT ( 'NONE',  ( 1.666666666666667185, -0.004921259842519576551, 0.3153832671262227771 ) ) ;
#64530=CARTESIAN_POINT ( 'NONE',  ( -1.161417322834644716, 0.07958543189024085140, 0.2665933059059887866 ) ) ;
#64531=CARTESIAN_POINT ( 'NONE',  ( -0.4855643044619415427, -0.004921259842519870586, -0.3153832671262229437 ) ) ;
#64532=CARTESIAN_POINT ( 'NONE',  ( -1.364829396325458521, 0.1283753931104746893, -0.1820866141732285504 ) ) ;
#64533=CARTESIAN_POINT ( 'NONE',  ( 0.7742782152230978099, -0.3690944881889763329, 0.3153832671262228327 ) ) ;
#64534=CARTESIAN_POINT ( 'NONE',  ( 0.3543307086614181922, -0.6692913385826771977, 8.415575281601705876E-17 ) ) ;
#64535=CARTESIAN_POINT ( 'NONE',  ( 1.528871391076116026, -0.6692913385826773087, -0.1292274648535924053 ) ) ;
#64536=CARTESIAN_POINT ( 'NONE',  ( -0.09186351706036663400, -0.4281496062992124485, 0.4176697321401328655 ) ) ;
#64538=CARTESIAN_POINT ( 'NONE',  ( 0.6824146981627303710, 0.1283753931104746893, -0.1820866141732285504 ) ) ;
#64539=CARTESIAN_POINT ( 'NONE',  ( -1.574803149606298192, -0.1870078740157480879, -0.4822834645669291653 ) ) ;
#64540=CARTESIAN_POINT ( 'NONE',  ( -1.332020997375327642, -0.05778040916215522460, 0.4822834645669289988 ) ) ;
#64541=CARTESIAN_POINT ( 'NONE',  ( -0.5774278215223089816, 0.2306618581243847221, -0.2411417322834647770 ) ) ;
#64544=CARTESIAN_POINT ( 'NONE',  ( 0.05249343832021075018, 0.2306618581243847221, -0.2411417322834647770 ) ) ;
#64545=CARTESIAN_POINT ( 'NONE',  ( 1.108923884514436242, -0.08942795157527998196, 0.3641732283464567121 ) ) ;
#64546=CARTESIAN_POINT ( 'NONE',  ( -0.4199475065616791736, -0.6046776061558807314, 0.2411417322834647770 ) ) ;
#64547=CARTESIAN_POINT ( 'NONE',  ( 0.5511811023622054106, -0.1870078740157480879, -0.4822834645669291653 ) ) ;
#64553=CARTESIAN_POINT ( 'NONE',  ( -1.082677165354329896, 0.07958543189024085140, 0.2665933059059887866 ) ) ;
#64555=CARTESIAN_POINT ( 'NONE',  ( -1.213910761154854745, 0.2952755905511810774, -0.1292274648535930714 ) ) ;
#64557=EDGE_CURVE ( 'NONE', #38656, #68129, #22982, .T. ) ;
#64558=CARTESIAN_POINT ( 'NONE',  ( 0.5052493438320218022, -0.6692913385826773087, -0.1292274648535924053 ) ) ;
#64559=CARTESIAN_POINT ( 'NONE',  ( 1.122047244094488860, 0.1660481256975885056, 0.3530559997133364547 ) ) ;
#64560=CARTESIAN_POINT ( 'NONE',  ( 0.7086614173228352742, -0.1870078740157480879, -0.4822834645669291653 ) ) ;
#64564=CARTESIAN_POINT ( 'NONE',  ( 1.220472440944882608, 0.2952755905511811885, 0.000000000000000000 ) ) ;
#64565=CARTESIAN_POINT ( 'NONE',  ( 0.3871391076115492380, -0.05778040916215560624, -0.4822834645669293319 ) ) ;
#64566=CARTESIAN_POINT ( 'NONE',  ( 0.2755905511811031494, -0.6692913385826771977, 8.415575281601705876E-17 ) ) ;
#64567=CARTESIAN_POINT ( 'NONE',  ( 0.6299212598425204535, -0.1870078740157479769, 0.3641732283464567677 ) ) ;
#64568=CARTESIAN_POINT ( 'NONE',  ( 1.148293963254593875, -0.6692913385826771977, 0.1292274648535927661 ) ) ;
#64570=CARTESIAN_POINT ( 'NONE',  ( -0.08530183727034056085, -0.05778040916215560624, -0.4822834645669293319 ) ) ;
#64571=CARTESIAN_POINT ( 'NONE',  ( 0.9186351706036752773, 0.2306618581243847221, -0.2411417322834647770 ) ) ;
#64572=CARTESIAN_POINT ( 'NONE',  ( 0.5905511811023629321, 0.2952755905511811885, 0.000000000000000000 ) ) ;
#64573=CARTESIAN_POINT ( 'NONE',  ( 1.036745406824147731, -0.004921259842519576551, 0.3153832671262227771 ) ) ;
#64574=CARTESIAN_POINT ( 'NONE',  ( -0.7808398950131225646, -0.05778040916215522460, 0.4822834645669289988 ) ) ;
#64575=CARTESIAN_POINT ( 'NONE',  ( -1.135170603674539924, -0.6692913385826771977, 0.1292274648535927661 ) ) ;
#64576=CARTESIAN_POINT ( 'NONE',  ( 1.154855643044620184, 0.2306618581243847221, -0.2411417322834647770 ) ) ;
#64583=ORIENTED_EDGE ( 'NONE', *, *, #17800, .F. ) ;
#64584=CARTESIAN_POINT ( 'NONE',  ( 1.548556430446194954, 0.2306618581243847221, -0.2411417322834647770 ) ) ;
#64585=CARTESIAN_POINT ( 'NONE',  ( 1.108923884514436242, -0.08942795157527998196, 0.3641732283464567121 ) ) ;
#64587=CARTESIAN_POINT ( 'NONE',  ( 1.305774278215223960, -0.5511811023622046335, 0.09757992244046803654 ) ) ;
#64588=DIRECTION ( 'NONE',  ( -1.000000000000000000, -3.083952846180990281E-16, 0.000000000000000000 ) ) ;
#64592=CARTESIAN_POINT ( 'NONE',  ( -0.9711286089238838626, 0.1283753931104746893, -0.1820866141732285504 ) ) ;
#64593=CARTESIAN_POINT ( 'NONE',  ( 1.594488188976378673, 0.1660481256975885056, 0.3530559997133364547 ) ) ;
#64594=CARTESIAN_POINT ( 'NONE',  ( -1.154855643044618851, 0.2306618581243848609, 0.2411417322834645549 ) ) ;
#64595=CARTESIAN_POINT ( 'NONE',  ( 0.2165354330708668673, 0.1660481256975883668, -0.3530559997133364547 ) ) ;
#64596=CARTESIAN_POINT ( 'NONE',  ( -1.607611548556429737, 0.2952755905511810774, -0.1292274648535930714 ) ) ;
#64603=CARTESIAN_POINT ( 'NONE',  ( -0.9776902887139098386, 0.1771653543307087075, -0.09757992244046823083 ) ) ;
#64604=CARTESIAN_POINT ( 'NONE',  ( 0.5774278215223104249, 0.2306618581243848609, 0.2411417322834645549 ) ) ;
#64606=LINE ( 'NONE', #65459, #588 ) ;
#64607=CARTESIAN_POINT ( 'NONE',  ( -1.220472440944881720, 0.8346805926620878280, 0.5309055118110233007 ) ) ;
#64608=CARTESIAN_POINT ( 'NONE',  ( 1.272965879265092637, -0.4281496062992127816, -0.4176697321401328100 ) ) ;
#64609=CARTESIAN_POINT ( 'NONE',  ( -1.679790026246718693, 0.2306618581243847221, -0.2411417322834647770 ) ) ;
#64611=CARTESIAN_POINT ( 'NONE',  ( -0.3346456692913377662, -0.4536011799217367080, 0.2665933059059888421 ) ) ;
#64612=CARTESIAN_POINT ( 'NONE',  ( -1.292650918635170010, 0.1771653543307087075, -0.09757992244046823083 ) ) ;
#64613=DIRECTION ( 'NONE',  ( -3.096699300667737957E-16, 1.000000000000000000, -0.000000000000000000 ) ) ;
#64614=CARTESIAN_POINT ( 'NONE',  ( -0.4265091863517051496, -0.5511811023622046335, 0.09757992244046803654 ) ) ;
#64615=CARTESIAN_POINT ( 'NONE',  ( 0.2034120734908142214, 0.1771653543307087075, -0.09757992244046823083 ) ) ;
#64617=CARTESIAN_POINT ( 'NONE',  ( 0.03280839895013198948, 0.2952755905511811885, 0.1292274648535926551 ) ) ;
#64618=CARTESIAN_POINT ( 'NONE',  ( -1.036745406824146176, -0.3690944881889763329, 0.3153832671262228327 ) ) ;
#64620=CARTESIAN_POINT ( 'NONE',  ( 1.135170603674541256, 0.2952755905511811885, 0.1292274648535926551 ) ) ;
#64621=CARTESIAN_POINT ( 'NONE',  ( -1.279527559055116948, 0.1660481256975883668, -0.3530559997133364547 ) ) ;
#64623=CARTESIAN_POINT ( 'NONE',  ( -0.2427821522309703550, -0.05778040916215560624, -0.4822834645669293319 ) ) ;
#64624=CARTESIAN_POINT ( 'NONE',  ( 0.4396325459317590445, -0.5511811023622046335, 0.09757992244046803654 ) ) ;
#64626=CARTESIAN_POINT ( 'NONE',  ( -1.069553805774277722, -0.6692913385826773087, -0.1292274648535924053 ) ) ;
#64627=CARTESIAN_POINT ( 'NONE',  ( 0.6889763779527566800, -0.4536011799217367080, 0.2665933059059888421 ) ) ;
#64628=CARTESIAN_POINT ( 'NONE',  ( -0.1640419947506555343, -0.2845877964562159024, 0.3641732283464567677 ) ) ;
#64629=CARTESIAN_POINT ( 'NONE',  ( -0.8202099737532801971, -0.6692913385826771977, 0.1292274648535927661 ) ) ;
#64630=CARTESIAN_POINT ( 'NONE',  ( -1.640419947506561060, 0.05413385826771666132, 0.4176697321401328100 ) ) ;
#64631=CARTESIAN_POINT ( 'NONE',  ( -0.7402641841139966372, 2.388450810264987734, 0.4916013665244731712 ) ) ;
#64632=CARTESIAN_POINT ( 'NONE',  ( 1.167979002624672580, -0.3690944881889763329, 0.3153832671262228327 ) ) ;
#64634=CARTESIAN_POINT ( 'NONE',  ( -1.338582677165353729, -0.1870078740157479769, 0.4822834645669291653 ) ) ;
#64635=CARTESIAN_POINT ( 'NONE',  ( -1.430446194225721390, -0.4281496062992124485, 0.4176697321401328655 ) ) ;
#64638=CARTESIAN_POINT ( 'NONE',  ( -0.8202099737532799750, 0.1771653543307087075, -0.09757992244046823083 ) ) ;
#64639=CARTESIAN_POINT ( 'NONE',  ( 0.6102362204724416372, -0.5400638737290844871, 0.3530559997133364547 ) ) ;
#64640=CARTESIAN_POINT ( 'NONE',  ( -1.115485564304461219, -0.3690944881889763329, 0.3153832671262228327 ) ) ;
#64642=CARTESIAN_POINT ( 'NONE',  ( -1.062992125984250968, 0.2952755905511811885, 0.000000000000000000 ) ) ;
#64643=CARTESIAN_POINT ( 'NONE',  ( 0.6955380577427828781, -0.4281496062992124485, 0.4176697321401328655 ) ) ;
#64644=CARTESIAN_POINT ( 'NONE',  ( 0.4199475065616805614, 0.2306618581243848609, 0.2411417322834645549 ) ) ;
#64646=CARTESIAN_POINT ( 'NONE',  ( -1.646981627296586703, -0.2845877964562161244, -0.3641732283464567121 ) ) ;
#64650=FACE_OUTER_BOUND ( 'NONE', #19032, .T. ) ;
#64651=CARTESIAN_POINT ( 'NONE',  ( 1.200787401574803681, 0.07958543189024085140, 0.2665933059059887866 ) ) ;
#64652=CARTESIAN_POINT ( 'NONE',  ( 0.2427821522309716595, -0.2845877964562161244, -0.3641732283464567121 ) ) ;
#64653=CARTESIAN_POINT ( 'NONE',  ( 0.03937007874015806264, 0.2952755905511811885, 0.000000000000000000 ) ) ;
#64654=CARTESIAN_POINT ( 'NONE',  ( 1.259842519685040019, -0.1870078740157479769, 0.4822834645669291653 ) ) ;
#64656=CARTESIAN_POINT ( 'NONE',  ( 0.4790026246719168435, -0.2845877964562161244, -0.3641732283464567121 ) ) ;
#64657=CARTESIAN_POINT ( 'NONE',  ( -0.8923884514435688198, -0.6046776061558807314, 0.2411417322834647770 ) ) ;
#64658=CARTESIAN_POINT ( 'NONE',  ( -1.397637795275589623, -0.5400638737290845981, -0.3530559997133363437 ) ) ;
#64659=CARTESIAN_POINT ( 'NONE',  ( 0.7939632545931766261, -0.3162353388693409650, -0.4822834645669289433 ) ) ;
#64664=CARTESIAN_POINT ( 'NONE',  ( -1.194225721784776262, 0.05413385826771626580, -0.4176697321401330321 ) ) ;
#64665=CARTESIAN_POINT ( 'NONE',  ( -0.7414698162729651543, -0.6692913385826771977, 0.1292274648535927661 ) ) ;
#64666=CARTESIAN_POINT ( 'NONE',  ( -0.6299212598425188991, -0.1870078740157480601, -0.3641732283464567677 ) ) ;
#64667=CARTESIAN_POINT ( 'NONE',  ( -0.9317585301837263412, -0.4281496062992127816, -0.4176697321401328100 ) ) ;
#64670=CARTESIAN_POINT ( 'NONE',  ( 1.555118110236221041, 0.1660481256975883668, -0.3530559997133364547 ) ) ;
#64671=CARTESIAN_POINT ( 'NONE',  ( -1.246719160104986512, 0.05413385826771666132, 0.4176697321401328100 ) ) ;
#64672=CARTESIAN_POINT ( 'NONE',  ( 0.1574803149606306130, -0.1870078740157479769, 0.4822834645669291653 ) ) ;
#64673=CARTESIAN_POINT ( 'NONE',  ( -0.6692913385826764205, 0.2952755905511811885, 0.000000000000000000 ) ) ;
#64674=CARTESIAN_POINT ( 'NONE',  ( 0.4921259842519691285, 0.1660481256975885056, 0.3530559997133364547 ) ) ;
#64676=CARTESIAN_POINT ( 'NONE',  ( -1.023622047244093558, -0.1870078740157479769, 0.3641732283464567677 ) ) ;
#64677=ORIENTED_EDGE ( 'NONE', *, *, #51203, .F. ) ;
#64679=ORIENTED_EDGE ( 'NONE', *, *, #38011, .T. ) ;
#64681=CARTESIAN_POINT ( 'NONE',  ( -1.299212598425196097, -0.6692913385826771977, 8.415575281601705876E-17 ) ) ;
#64682=CARTESIAN_POINT ( 'NONE',  ( -1.246719160104985846, -0.4281496062992127816, -0.4176697321401328100 ) ) ;
#64684=CARTESIAN_POINT ( 'NONE',  ( -0.9908136482939626788, -0.6692913385826773087, -0.1292274648535924053 ) ) ;
#64685=CARTESIAN_POINT ( 'NONE',  ( -1.272965879265091305, -0.4281496062992124485, 0.4176697321401328655 ) ) ;
#64686=CARTESIAN_POINT ( 'NONE',  ( -1.332020997375327642, -0.05778040916215522460, 0.4822834645669289988 ) ) ;
#64687=CARTESIAN_POINT ( 'NONE',  ( -0.3833616679418195283, -1.094630224652485432E-15, 0.4281993546915541238 ) ) ;
#64689=CARTESIAN_POINT ( 'NONE',  ( -0.02624671916010428221, 0.1283753931104746893, -0.1820866141732285504 ) ) ;
#64692=CARTESIAN_POINT ( 'NONE',  ( -0.3215223097112853146, -0.2845877964562159024, 0.3641732283464567677 ) ) ;
#64693=CARTESIAN_POINT ( 'NONE',  ( -0.7939632545931750718, -0.05778040916215560624, -0.4822834645669293319 ) ) ;
#64694=CARTESIAN_POINT ( 'NONE',  ( 1.345144356955381593, -0.3162353388693409650, -0.4822834645669289433 ) ) ;
#64695=CARTESIAN_POINT ( 'NONE',  ( -0.6036745406824141069, -0.6046776061558809534, -0.2411417322834644161 ) ) ;
#64699=CARTESIAN_POINT ( 'NONE',  ( -1.174540682414697335, -0.05778040916215522460, 0.4822834645669289988 ) ) ;
#64700=CARTESIAN_POINT ( 'NONE',  ( 1.338582677165355062, -0.1870078740157480879, -0.4822834645669291653 ) ) ;
#64701=CARTESIAN_POINT ( 'NONE',  ( -1.423884514435694859, -0.2845877964562159024, 0.3641732283464567677 ) ) ;
#64702=CARTESIAN_POINT ( 'NONE',  ( -1.332020997375327642, -0.3162353388693409650, -0.4822834645669289433 ) ) ;
#64707=CARTESIAN_POINT ( 'NONE',  ( -0.07217847769028787330, -0.05778040916215522460, 0.4822834645669289988 ) ) ;
#64708=CARTESIAN_POINT ( 'NONE',  ( -1.574803149606298192, -0.1870078740157480601, -0.3641732283464567677 ) ) ;
#64709=CARTESIAN_POINT ( 'NONE',  ( -0.8530183727034112984, -0.4281496062992127816, -0.4176697321401328100 ) ) ;
#64711=CARTESIAN_POINT ( 'NONE',  ( -1.377952755905511140, 0.2952755905511811885, 0.000000000000000000 ) ) ;
#64712=CARTESIAN_POINT ( 'NONE',  ( -0.2262115530851587786, -2.191421614605370878E-15, 0.4445507791589071167 ) ) ;
#64713=CARTESIAN_POINT ( 'NONE',  ( -1.056430446194224881, 0.2952755905511810774, -0.1292274648535930714 ) ) ;
#64714=CARTESIAN_POINT ( 'NONE',  ( -0.3412073490813641308, -0.6046776061558807314, 0.2411417322834647770 ) ) ;
#64716=CARTESIAN_POINT ( 'NONE',  ( 0.9711286089238851948, 0.1283753931104748280, 0.1820866141732283561 ) ) ;
#64718=CARTESIAN_POINT ( 'NONE',  ( 0.7414698162729663755, 0.1771653543307087630, 0.09757992244046791164 ) ) ;
#64719=CARTESIAN_POINT ( 'NONE',  ( 1.292650918635171564, 0.1771653543307087630, 0.09757992244046791164 ) ) ;
#64721=CARTESIAN_POINT ( 'NONE',  ( 1.437007874015748810, 0.1660481256975885056, 0.3530559997133364547 ) ) ;
#64723=CARTESIAN_POINT ( 'NONE',  ( 0.2821522309711292364, 0.1771653543307087075, -0.09757992244046823083 ) ) ;
#64725=CARTESIAN_POINT ( 'NONE',  ( -1.056430446194224881, -0.6692913385826771977, 0.1292274648535927661 ) ) ;
#64726=CARTESIAN_POINT ( 'NONE',  ( 1.371391076115485719, -0.6692913385826773087, -0.1292274648535924053 ) ) ;
#64728=CARTESIAN_POINT ( 'NONE',  ( -0.5380577427821514602, -0.004921259842519576551, 0.3153832671262227771 ) ) ;
#64731=CARTESIAN_POINT ( 'NONE',  ( 0.2755905511811031494, 0.2952755905511811885, 0.000000000000000000 ) ) ;
#64732=DIRECTION ( 'NONE',  ( -1.000000000000000000, -2.312964634635742464E-16, 0.000000000000000000 ) ) ;
#64733=CARTESIAN_POINT ( 'NONE',  ( 0.7742782152230978099, -0.3690944881889763329, 0.3153832671262228327 ) ) ;
#64734=CARTESIAN_POINT ( 'NONE',  ( 0.1049868766404206816, -0.5023911411419708095, -0.1820866141732282451 ) ) ;
#64735=CARTESIAN_POINT ( 'NONE',  ( -0.2362204724409440182, -0.1870078740157479769, 0.4822834645669291653 ) ) ;
#64736=CARTESIAN_POINT ( 'NONE',  ( -1.325459317585300889, -0.4281496062992127816, -0.4176697321401328100 ) ) ;
#64737=CARTESIAN_POINT ( 'NONE',  ( -0.5839895013123351797, -0.5511811023622046335, 0.09757992244046803654 ) ) ;
#64739=CARTESIAN_POINT ( 'NONE',  ( -0.9908136482939626788, 0.2952755905511811885, 0.1292274648535926551 ) ) ;
#64742=CARTESIAN_POINT ( 'NONE',  ( -0.006561679790025524116, -0.2845877964562159024, 0.3641732283464567677 ) ) ;
#64743=CARTESIAN_POINT ( 'NONE',  ( -0.7217847769028863381, -0.4281496062992124485, 0.4176697321401328655 ) ) ;
#64744=CARTESIAN_POINT ( 'NONE',  ( -0.9186351706036736120, -0.6046776061558809534, -0.2411417322834644161 ) ) ;
#64745=CARTESIAN_POINT ( 'NONE',  ( -1.286089238845143479, 0.1283753931104746893, -0.1820866141732285504 ) ) ;
#64747=CARTESIAN_POINT ( 'NONE',  ( -1.049868766404198794, -0.5023911411419708095, 0.1820866141732285504 ) ) ;
#64748=CARTESIAN_POINT ( 'NONE',  ( -1.522309711286088607, 0.1283753931104746893, -0.1820866141732285504 ) ) ;
#64749=CARTESIAN_POINT ( 'NONE',  ( 1.161417322834646271, 0.1660481256975883668, -0.3530559997133364547 ) ) ;
#64754=CARTESIAN_POINT ( 'NONE',  ( 1.541994750656168645, -0.5511811023622046335, 0.09757992244046803654 ) ) ;
#64755=CARTESIAN_POINT ( 'NONE',  ( -1.227034120734907585, 0.2952755905511811885, 0.1292274648535926551 ) ) ;
#64756=CARTESIAN_POINT ( 'NONE',  ( 1.443569553805774897, 0.2306618581243848609, 0.2411417322834645549 ) ) ;
#64758=CARTESIAN_POINT ( 'NONE',  ( 1.587926509186352586, -0.3690944881889765550, -0.3153832671262227771 ) ) ;
#64759=CARTESIAN_POINT ( 'NONE',  ( 0.5839895013123367340, 0.2952755905511811885, 0.1292274648535926551 ) ) ;
#64760=CARTESIAN_POINT ( 'NONE',  ( 0.1574803149606306130, -0.1870078740157480879, -0.4822834645669291653 ) ) ;
#64763=CARTESIAN_POINT ( 'NONE',  ( 0.8923884514435701520, -0.5023911411419708095, -0.1820866141732282451 ) ) ;
#64765=ORIENTED_EDGE ( 'NONE', *, *, #40849, .T. ) ;
#64768=CARTESIAN_POINT ( 'NONE',  ( 0.1574803149606306130, -0.1870078740157479769, 0.4822834645669291653 ) ) ;
#64769=CARTESIAN_POINT ( 'NONE',  ( -1.555118110236219930, -0.5400638737290845981, -0.3530559997133363437 ) ) ;
#64770=CARTESIAN_POINT ( 'NONE',  ( 0.6824146981627303710, -0.6046776061558807314, 0.2411417322834647770 ) ) ;
#64771=CARTESIAN_POINT ( 'NONE',  ( 1.384514435695538559, 0.2952755905511810774, -0.1292274648535930714 ) ) ;
#64772=CARTESIAN_POINT ( 'NONE',  ( 1.469816272965879911, 0.2306618581243847221, -0.2411417322834647770 ) ) ;
#64773=CARTESIAN_POINT ( 'NONE',  ( -0.4461942257217840213, -0.6046776061558809534, -0.2411417322834644161 ) ) ;
#64774=CARTESIAN_POINT ( 'NONE',  ( -0.01968503937007793844, -0.5400638737290844871, 0.3530559997133364547 ) ) ;
#64775=CARTESIAN_POINT ( 'NONE',  ( 1.607611548556431069, 0.2952755905511811885, 0.1292274648535926551 ) ) ;
#64776=AXIS2_PLACEMENT_3D ( 'NONE', #75430, #50956, #76653 ) ;
#64777=CARTESIAN_POINT ( 'NONE',  ( 1.404199475065617264, -0.4281496062992124485, 0.4176697321401328655 ) ) ;
#64778=CARTESIAN_POINT ( 'NONE',  ( 1.371391076115485941, 0.2952755905511811885, 0.1292274648535926551 ) ) ;
#64779=CARTESIAN_POINT ( 'NONE',  ( -0.3280839895013117347, -0.4281496062992124485, 0.4176697321401328655 ) ) ;
#64781=CARTESIAN_POINT ( 'NONE',  ( 0.3871391076115493490, -0.2845877964562159024, 0.3641732283464567677 ) ) ;
#64785=CARTESIAN_POINT ( 'NONE',  ( -0.5643044619422565855, -0.004921259842519870586, -0.3153832671262229437 ) ) ;
#64787=CARTESIAN_POINT ( 'NONE',  ( 0.05905511811023681640, 0.1660481256975883668, -0.3530559997133364547 ) ) ;
#64788=CARTESIAN_POINT ( 'NONE',  ( 0.1049868766404206816, -0.6046776061558809534, -0.2411417322834644161 ) ) ;
#64789=CARTESIAN_POINT ( 'NONE',  ( -1.056430446194224881, 0.2952755905511810774, -0.1292274648535930714 ) ) ;
#64791=CARTESIAN_POINT ( 'NONE',  ( -1.561679790026246017, -0.4281496062992127816, -0.4176697321401328100 ) ) ;
#64793=CARTESIAN_POINT ( 'NONE',  ( 0.7874015748031503170, -0.1870078740157479769, 0.3641732283464567677 ) ) ;
#64794=CARTESIAN_POINT ( 'NONE',  ( 0.3018372703412079971, 0.05413385826771626580, -0.4176697321401330321 ) ) ;
#64795=CARTESIAN_POINT ( 'NONE',  ( 0.8727034120734913358, -0.05778040916215522460, 0.4822834645669289988 ) ) ;
#64797=CARTESIAN_POINT ( 'NONE',  ( -1.673228346456691717, 0.1660481256975883668, -0.3530559997133364547 ) ) ;
#64800=CARTESIAN_POINT ( 'NONE',  ( -0.1837270341207343505, -0.6046776061558807314, 0.2411417322834647770 ) ) ;
#64803=CARTESIAN_POINT ( 'NONE',  ( -1.259842519685038686, -0.1870078740157480601, -0.3641732283464567677 ) ) ;
#64804=CARTESIAN_POINT ( 'NONE',  ( 1.167979002624672580, 0.05413385826771626580, -0.4176697321401330321 ) ) ;
#64805=CARTESIAN_POINT ( 'NONE',  ( 1.358267716535433323, 0.1660481256975885056, 0.3530559997133364547 ) ) ;
#64806=CARTESIAN_POINT ( 'NONE',  ( 0.1837270341207357105, -0.5023911411419708095, -0.1820866141732282451 ) ) ;
#64807=CARTESIAN_POINT ( 'NONE',  ( 0.3477690288713918276, 0.2952755905511811885, 0.1292274648535926551 ) ) ;
#64809=CARTESIAN_POINT ( 'NONE',  ( 0.3871391076115493490, -0.2845877964562159024, 0.3641732283464567677 ) ) ;
#64810=CARTESIAN_POINT ( 'NONE',  ( -0.1377952755905504645, 0.1660481256975885056, 0.3530559997133364547 ) ) ;
#64812=CARTESIAN_POINT ( 'NONE',  ( -1.423884514435694859, -0.3162353388693405765, 0.4822834645669290543 ) ) ;
#64813=CARTESIAN_POINT ( 'NONE',  ( 0.6561679790026253567, 0.1283753931104748280, 0.1820866141732283561 ) ) ;
#64815=CARTESIAN_POINT ( 'NONE',  ( -0.7283464566929126471, 0.1660481256975883668, -0.3530559997133364547 ) ) ;
#64816=CARTESIAN_POINT ( 'NONE',  ( -0.1181102362204717315, -0.5511811023622047445, 6.969142054262312111E-17 ) ) ;
#64818=CARTESIAN_POINT ( 'NONE',  ( -0.9383202099737524282, -0.05778040916215522460, 0.4822834645669289988 ) ) ;
#64819=CARTESIAN_POINT ( 'NONE',  ( -0.2230971128608915943, 0.05413385826771666132, 0.4176697321401328100 ) ) ;
#64820=CARTESIAN_POINT ( 'NONE',  ( 0.2230971128608929543, -0.004921259842519870586, -0.3153832671262229437 ) ) ;
#64823=CARTESIAN_POINT ( 'NONE',  ( -0.02624671916010428221, 0.2306618581243847221, -0.2411417322834647770 ) ) ;
#64827=CARTESIAN_POINT ( 'NONE',  ( 0.7939632545931766261, -0.2845877964562161244, -0.3641732283464567121 ) ) ;
#64828=CARTESIAN_POINT ( 'NONE',  ( 1.555118110236221041, -0.5400638737290844871, 0.3530559997133364547 ) ) ;
#64829=CARTESIAN_POINT ( 'NONE',  ( -0.7808398950131225646, -0.08942795157527998196, 0.3641732283464567121 ) ) ;
#64830=CARTESIAN_POINT ( 'NONE',  ( -1.351706036745406347, -0.004921259842519870586, -0.3153832671262229437 ) ) ;
#64832=CARTESIAN_POINT ( 'NONE',  ( -0.7742782152230962556, -0.4281496062992127816, -0.4176697321401328100 ) ) ;
#64833=CARTESIAN_POINT ( 'NONE',  ( -0.1312335958005241554, 0.2306618581243848609, 0.2411417322834645549 ) ) ;
#64834=CARTESIAN_POINT ( 'NONE',  ( 0.3608923884514443348, -0.5511811023622046335, 0.09757992244046803654 ) ) ;
#64836=CARTESIAN_POINT ( 'NONE',  ( 0.9973753280839902091, 0.1283753931104746893, -0.1820866141732285504 ) ) ;
#64837=CARTESIAN_POINT ( 'NONE',  ( 0.1377952755905518800, 0.1660481256975883668, -0.3530559997133364547 ) ) ;
#64838=CARTESIAN_POINT ( 'NONE',  ( -1.436417322834644850, 0.4405861044731111953, 0.3149606299212598381 ) ) ;
#64839=CARTESIAN_POINT ( 'NONE',  ( -0.3477690288713905509, -0.6692913385826771977, 0.1292274648535927661 ) ) ;
#64841=CARTESIAN_POINT ( 'NONE',  ( 1.469816272965879911, 0.1283753931104746893, -0.1820866141732285504 ) ) ;
#64842=CARTESIAN_POINT ( 'NONE',  ( 0.6561679790026253567, -0.6046776061558809534, -0.2411417322834644161 ) ) ;
#64843=CARTESIAN_POINT ( 'NONE',  ( 0.2034120734908144990, -0.6692913385826771977, 0.1292274648535927661 ) ) ;
#64844=CARTESIAN_POINT ( 'NONE',  ( 1.114295247146197099, 1.650914051239646151E-16, 0.3627985898453514046 ) ) ;
#64845=CARTESIAN_POINT ( 'NONE',  ( 0.006561679790026889343, -0.2845877964562161244, -0.3641732283464567121 ) ) ;
#64846=CARTESIAN_POINT ( 'NONE',  ( 0.8464566929133866546, -0.5400638737290844871, 0.3530559997133364547 ) ) ;
#64847=CARTESIAN_POINT ( 'NONE',  ( -0.3805774278215216522, -0.3690944881889765550, -0.3153832671262227771 ) ) ;
#64848=CARTESIAN_POINT ( 'NONE',  ( -0.6364829396325453192, -0.05778040916215560624, -0.4822834645669293319 ) ) ;
#64849=CARTESIAN_POINT ( 'NONE',  ( 0.8136482939632553313, 0.2306618581243848609, 0.2411417322834645549 ) ) ;
#64850=CARTESIAN_POINT ( 'NONE',  ( -0.2755905511811018171, 0.2952755905511811885, 0.000000000000000000 ) ) ;
#64851=VERTEX_POINT ( 'NONE', #63496 ) ;
#64852=CARTESIAN_POINT ( 'NONE',  ( -1.141732283464566011, 0.2952755905511811885, 0.000000000000000000 ) ) ;
#64853=CARTESIAN_POINT ( 'NONE',  ( -0.8136482939632537770, -0.5023911411419708095, 0.1820866141732285504 ) ) ;
#64854=CARTESIAN_POINT ( 'NONE',  ( 0.1377952755905518800, -0.5400638737290844871, 0.3530559997133364547 ) ) ;
#64855=CARTESIAN_POINT ( 'NONE',  ( -1.213910761154854745, 0.2952755905511810774, -0.1292274648535930714 ) ) ;
#64856=CARTESIAN_POINT ( 'NONE',  ( -0.7349081364829387342, -0.6046776061558807314, 0.2411417322834647770 ) ) ;
#64859=CARTESIAN_POINT ( 'NONE',  ( 1.437007874015748810, 0.1660481256975885056, 0.3530559997133364547 ) ) ;
#64860=CARTESIAN_POINT ( 'NONE',  ( 1.181102362204725198, -0.1870078740157479769, 0.4822834645669291653 ) ) ;
#64862=DIRECTION ( 'NONE',  ( -3.096699300667737957E-16, 1.000000000000000000, -0.000000000000000000 ) ) ;
#64863=CARTESIAN_POINT ( 'NONE',  ( -1.279527559055116948, -0.5400638737290844871, 0.3530559997133364547 ) ) ;
#64867=CARTESIAN_POINT ( 'NONE',  ( -0.1115485564304453947, -0.5511811023622046335, 0.09757992244046803654 ) ) ;
#64870=CARTESIAN_POINT ( 'NONE',  ( 0.2887139107611556010, -0.6046776061558807314, 0.2411417322834647770 ) ) ;
#64871=CARTESIAN_POINT ( 'NONE',  ( 0.4068241469816279987, -0.4281496062992127816, -0.4176697321401328100 ) ) ;
#64874=CARTESIAN_POINT ( 'NONE',  ( -0.9317585301837263412, -0.3690944881889765550, -0.3153832671262227771 ) ) ;
#64876=CARTESIAN_POINT ( 'NONE',  ( 0.6233595800524942554, -0.05778040916215560624, -0.4822834645669293319 ) ) ;
#64877=CARTESIAN_POINT ( 'NONE',  ( 0.9186351706036751663, -0.5023911411419708095, 0.1820866141732285504 ) ) ;
#64878=CARTESIAN_POINT ( 'NONE',  ( -0.3083989501312330295, -0.3162353388693409650, -0.4822834645669289433 ) ) ;
#64880=CARTESIAN_POINT ( 'NONE',  ( -0.9448818897637790704, -0.1870078740157480879, -0.4822834645669291653 ) ) ;
#64882=CARTESIAN_POINT ( 'NONE',  ( -0.8530183727034112984, -0.4281496062992127816, -0.4176697321401328100 ) ) ;
#64883=CARTESIAN_POINT ( 'NONE',  ( 1.292650918635171564, -0.6692913385826773087, -0.1292274648535924053 ) ) ;
#64884=CARTESIAN_POINT ( 'NONE',  ( 1.640419947506562393, -0.3690944881889763329, 0.3153832671262228327 ) ) ;
#64885=ORIENTED_EDGE ( 'NONE', *, *, #24432, .T. ) ;
#64887=CARTESIAN_POINT ( 'NONE',  ( -0.2099737532808391705, 0.2306618581243848609, 0.2411417322834645549 ) ) ;
#64889=CARTESIAN_POINT ( 'NONE',  ( -0.7545931758530177724, 0.2952755905511811885, 0.1292274648535926551 ) ) ;
#64890=CARTESIAN_POINT ( 'NONE',  ( 1.587926509186352142, 0.05413385826771666132, 0.4176697321401328100 ) ) ;
#64891=CARTESIAN_POINT ( 'NONE',  ( 1.384514435695538337, -0.6692913385826771977, 0.1292274648535927661 ) ) ;
#64892=CARTESIAN_POINT ( 'NONE',  ( 0.3083989501312343062, -0.3162353388693405765, 0.4822834645669290543 ) ) ;
#64895=CARTESIAN_POINT ( 'NONE',  ( -0.3412073490813641308, 0.2306618581243847221, -0.2411417322834647770 ) ) ;
#64897=CARTESIAN_POINT ( 'NONE',  ( -1.358267716535432434, 0.1660481256975883668, -0.3530559997133364547 ) ) ;
#64898=CARTESIAN_POINT ( 'NONE',  ( -0.01312335958005186876, 0.05413385826771626580, -0.4176697321401330321 ) ) ;
#64899=CARTESIAN_POINT ( 'NONE',  ( -0.2755905511811015396, -0.5511811023622047445, 6.969142054262312111E-17 ) ) ;
#64900=CARTESIAN_POINT ( 'NONE',  ( 1.601049868766404982, -0.6046776061558809534, -0.2411417322834644161 ) ) ;
#64901=CARTESIAN_POINT ( 'NONE',  ( 1.410761154855643795, -0.05778040916215560624, -0.4822834645669293319 ) ) ;
#64902=CARTESIAN_POINT ( 'NONE',  ( -0.3280839895013117347, -0.4281496062992124485, 0.4176697321401328655 ) ) ;
#64904=CARTESIAN_POINT ( 'NONE',  ( 1.233595800524935227, -0.6046776061558807314, 0.2411417322834647770 ) ) ;
#64906=ORIENTED_EDGE ( 'NONE', *, *, #42986, .T. ) ;
#64909=CARTESIAN_POINT ( 'NONE',  ( 0.07874015748031558404, -0.1870078740157479769, 0.4822834645669291653 ) ) ;
#64910=CARTESIAN_POINT ( 'NONE',  ( -0.2099737532808391705, -0.5023911411419708095, -0.1820866141732282451 ) ) ;
#64911=CARTESIAN_POINT ( 'NONE',  ( 1.496062992125985147, -0.1870078740157479769, 0.3641732283464567677 ) ) ;
#64915=CARTESIAN_POINT ( 'NONE',  ( 1.240157480314961314, -0.5400638737290844871, 0.3530559997133364547 ) ) ;
#64917=CARTESIAN_POINT ( 'NONE',  ( -0.03937007874015669567, -0.6692913385826771977, 8.415575281601705876E-17 ) ) ;
#64918=CARTESIAN_POINT ( 'NONE',  ( -1.627296587926508442, 0.2306618581243848609, 0.2411417322834645549 ) ) ;
#64919=CARTESIAN_POINT ( 'NONE',  ( -1.437007874015747477, -0.5400638737290844871, 0.3530559997133364547 ) ) ;
#64920=CARTESIAN_POINT ( 'NONE',  ( -0.1443569553805768291, 0.05413385826771666132, 0.4176697321401328100 ) ) ;
#64922=CARTESIAN_POINT ( 'NONE',  ( 1.666666666666667185, 0.05413385826771666132, 0.4176697321401328100 ) ) ;
#64923=CARTESIAN_POINT ( 'NONE',  ( 0.7020997375328090762, -0.05778040916215560624, -0.4822834645669293319 ) ) ;
#64924=CARTESIAN_POINT ( 'NONE',  ( 1.036745406824147731, -0.004921259842519576551, 0.3153832671262227771 ) ) ;
#64926=CARTESIAN_POINT ( 'NONE',  ( 0.9711286089238851948, -0.5023911411419708095, -0.1820866141732282451 ) ) ;
#64927=CARTESIAN_POINT ( 'NONE',  ( -1.122047244094487306, 0.1660481256975883668, -0.3530559997133364547 ) ) ;
#64929=CARTESIAN_POINT ( 'NONE',  ( 1.076115485564305141, 0.2306618581243847221, -0.2411417322834647770 ) ) ;
#64931=CARTESIAN_POINT ( 'NONE',  ( 0.8727034120734913358, -0.05778040916215522460, 0.4822834645669289988 ) ) ;
#64933=CARTESIAN_POINT ( 'NONE',  ( 0.2887139107611556010, -0.5023911411419708095, 0.1820866141732285504 ) ) ;
#64934=CARTESIAN_POINT ( 'NONE',  ( 0.5446194225721792126, -0.3162353388693405765, 0.4822834645669290543 ) ) ;
#64936=CARTESIAN_POINT ( 'NONE',  ( -1.135170603674539924, -0.5511811023622046335, 0.09757992244046803654 ) ) ;
#64937=CARTESIAN_POINT ( 'NONE',  ( -1.056430446194224881, 0.2952755905511810774, -0.1292274648535930714 ) ) ;
#64938=CARTESIAN_POINT ( 'NONE',  ( 1.305774278215223960, -0.6692913385826771977, 0.1292274648535927661 ) ) ;
#64939=CARTESIAN_POINT ( 'NONE',  ( -1.404199475065615932, 0.05413385826771666132, 0.4176697321401328100 ) ) ;
#64940=CARTESIAN_POINT ( 'NONE',  ( 1.043307086614173818, 0.1660481256975885056, 0.3530559997133364547 ) ) ;
#64941=CARTESIAN_POINT ( 'NONE',  ( -1.456692913385826182, 0.1771653543307087630, 0.000000000000000000 ) ) ;
#64943=CARTESIAN_POINT ( 'NONE',  ( 1.003937007874016185, 0.1660481256975883668, -0.3530559997133364547 ) ) ;
#64945=CARTESIAN_POINT ( 'NONE',  ( 1.614173228346457378, -0.6692913385826771977, 8.415575281601705876E-17 ) ) ;
#64946=CARTESIAN_POINT ( 'NONE',  ( 1.187664041994751285, -0.05778040916215522460, 0.4822834645669289988 ) ) ;
#64947=CARTESIAN_POINT ( 'NONE',  ( -1.325459317585300889, -0.3690944881889765550, -0.3153832671262227771 ) ) ;
#64948=CARTESIAN_POINT ( 'NONE',  ( 1.371391076115485941, 0.1771653543307087630, 0.09757992244046791164 ) ) ;
#64949=CARTESIAN_POINT ( 'NONE',  ( -1.318897637795274802, 0.07958543189024085140, 0.2665933059059887866 ) ) ;
#64950=CARTESIAN_POINT ( 'NONE',  ( -0.5643044619422565855, -0.3690944881889763329, 0.3153832671262228327 ) ) ;
#64951=CARTESIAN_POINT ( 'NONE',  ( -1.437007874015747477, -0.4536011799217367080, 0.2665933059059888421 ) ) ;
#64952=CARTESIAN_POINT ( 'NONE',  ( 0.8398950131233602345, 0.1283753931104746893, -0.1820866141732285504 ) ) ;
#64953=B_SPLINE_CURVE_WITH_KNOTS ( 'NONE', 3,
 ( #50106, #75803, #18145, #44913, #40297, #39885, #65147 ),
 .UNSPECIFIED., .F., .F.,
 ( 4, 3, 4 ),
 ( 5.551115123125782702E-17, 0.001246230184515582365, 0.002492489877932689731 ),
 .UNSPECIFIED. ) ;
#64954=CONICAL_SURFACE ( 'NONE', #28671, 3.582677165354330562, 0.7853981633974415066 ) ;
#64955=CARTESIAN_POINT ( 'NONE',  ( 0.5971128608923891301, 0.2952755905511810774, -0.1292274648535930714 ) ) ;
#64956=CARTESIAN_POINT ( 'NONE',  ( 1.043307086614173818, -0.5400638737290845981, -0.3530559997133363437 ) ) ;
#64957=CARTESIAN_POINT ( 'NONE',  ( 0.1640419947506569498, -0.3162353388693409650, -0.4822834645669289433 ) ) ;
#64958=ADVANCED_FACE ( 'NONE', ( #31920 ), #44528, .F. ) ;
#64959=CARTESIAN_POINT ( 'NONE',  ( 0.4527559055118117182, -0.4536011799217367080, 0.2665933059059888421 ) ) ;
#64960=CARTESIAN_POINT ( 'NONE',  ( -1.456692913385826182, 0.2952755905511811885, 0.000000000000000000 ) ) ;
#64962=EDGE_CURVE ( 'NONE', #82322, #23151, #12993, .T. ) ;
#64963=CARTESIAN_POINT ( 'NONE',  ( 2.795275590551181910, 1.568468489416428469, 0.000000000000000000 ) ) ;
#64964=CARTESIAN_POINT ( 'NONE',  ( -0.4265091863517051496, 0.2952755905511810774, -0.1292274648535930714 ) ) ;
#64966=CARTESIAN_POINT ( 'NONE',  ( 0.01241954290193841674, 0.000000000000000000, 0.3464511005275205946 ) ) ;
#64967=CARTESIAN_POINT ( 'NONE',  ( 0.1443569553805781891, -0.4281496062992124485, 0.4176697321401328655 ) ) ;
#64968=CARTESIAN_POINT ( 'NONE',  ( -0.5905511811023613777, -0.6692913385826771977, 8.415575281601705876E-17 ) ) ;
#64969=CARTESIAN_POINT ( 'NONE',  ( 0.02624671916010564918, 0.2306618581243848609, 0.2411417322834645549 ) ) ;
#64975=CARTESIAN_POINT ( 'NONE',  ( -0.8923884514435688198, 0.1283753931104746893, -0.1820866141732285504 ) ) ;
#64977=CARTESIAN_POINT ( 'NONE',  ( -1.259842519685038686, -0.1870078740157479769, 0.4822834645669291653 ) ) ;
#64978=B_SPLINE_CURVE_WITH_KNOTS ( 'NONE', 3,
 ( #20655, #64844, #1715, #65702, #7182, #32853, #58522 ),
 .UNSPECIFIED., .F., .F.,
 ( 4, 3, 4 ),
 ( 7.703719777548943412E-34, 0.001246230184515573257, 0.002492489877932650266 ),
 .UNSPECIFIED. ) ;
#64980=CARTESIAN_POINT ( 'NONE',  ( 0.6299212598425204535, -0.1870078740157480879, -0.4822834645669291653 ) ) ;
#64981=CARTESIAN_POINT ( 'NONE',  ( -0.09186351706036689768, -0.004921259842519870586, -0.3153832671262229437 ) ) ;
#64983=CARTESIAN_POINT ( 'NONE',  ( 1.266404199475066328, -0.05778040916215522460, 0.4822834645669289988 ) ) ;
#64984=CARTESIAN_POINT ( 'NONE',  ( 0.5314960629921264834, 0.1660481256975883668, -0.3530559997133364547 ) ) ;
#64988=CARTESIAN_POINT ( 'NONE',  ( 1.318897637795276356, -0.5400638737290844871, 0.3530559997133364547 ) ) ;
#64989=CARTESIAN_POINT ( 'NONE',  ( 0.3149606299212603933, -0.1870078740157479769, 0.4822834645669291653 ) ) ;
#64990=CARTESIAN_POINT ( 'NONE',  ( 0.2887139107611556010, -0.6046776061558807314, 0.2411417322834647770 ) ) ;
#64991=CARTESIAN_POINT ( 'NONE',  ( 1.404199475065617708, 0.05413385826771626580, -0.4176697321401330321 ) ) ;
#64993=CARTESIAN_POINT ( 'NONE',  ( 0.1377952755905518800, -0.5400638737290844871, 0.3530559997133364547 ) ) ;
#64994=CARTESIAN_POINT ( 'NONE',  ( 1.181102362204725198, -0.1870078740157479769, 0.4822834645669291653 ) ) ;
#64995=CARTESIAN_POINT ( 'NONE',  ( 0.3740157480314966754, -0.5400638737290844871, 0.3530559997133364547 ) ) ;
#64997=CARTESIAN_POINT ( 'NONE',  ( 1.318897637795276356, -0.4536011799217367080, 0.2665933059059888421 ) ) ;
#64998=CARTESIAN_POINT ( 'NONE',  ( -1.003937007874015297, -0.5400638737290845981, -0.3530559997133363437 ) ) ;
#64999=CARTESIAN_POINT ( 'NONE',  ( -1.391076115485563758, 0.2306618581243848609, 0.2411417322834645549 ) ) ;
#65000=CARTESIAN_POINT ( 'NONE',  ( 0.9251968503937015864, -0.5400638737290844871, 0.3530559997133364547 ) ) ;
#65002=ORIENTED_EDGE ( 'NONE', *, *, #29379, .F. ) ;
#65005=CARTESIAN_POINT ( 'NONE',  ( 1.692913385826772421, 0.2952755905511811885, 0.000000000000000000 ) ) ;
#65006=CARTESIAN_POINT ( 'NONE',  ( 0.9055118110236227702, -0.5511811023622047445, 6.969142054262312111E-17 ) ) ;
#65007=DIRECTION ( 'NONE',  ( -3.096699300667737957E-16, 1.000000000000000000, -0.000000000000000000 ) ) ;
#65012=CARTESIAN_POINT ( 'NONE',  ( -1.102362204724408601, -0.1870078740157480601, -0.3641732283464567677 ) ) ;
#65013=CARTESIAN_POINT ( 'NONE',  ( 1.581364829396326277, -0.05778040916215522460, 0.4822834645669289988 ) ) ;
#65014=CARTESIAN_POINT ( 'NONE',  ( -1.653543307086613234, -0.1870078740157479769, 0.4822834645669291653 ) ) ;
#65015=CARTESIAN_POINT ( 'NONE',  ( -0.3280839895013117347, -0.4281496062992124485, 0.4176697321401328655 ) ) ;
#65016=CARTESIAN_POINT ( 'NONE',  ( -1.614173228346455824, 0.2952755905511811885, 0.000000000000000000 ) ) ;
#65018=CARTESIAN_POINT ( 'NONE',  ( -1.430446194225721390, -0.4281496062992124485, 0.4176697321401328655 ) ) ;
#65023=CARTESIAN_POINT ( 'NONE',  ( -0.7480314960629914633, -0.5511811023622047445, 6.969142054262312111E-17 ) ) ;
#65024=CARTESIAN_POINT ( 'NONE',  ( -1.646981627296586703, -0.05778040916215522460, 0.4822834645669289988 ) ) ;
#65025=CARTESIAN_POINT ( 'NONE',  ( 0.5577427821522316087, -0.05778040916215522460, 0.4822834645669289988 ) ) ;
#65028=CARTESIAN_POINT ( 'NONE',  ( 1.586052503253845503, 0.4724409448818907564, 0.1653254495020587411 ) ) ;
#65029=CARTESIAN_POINT ( 'NONE',  ( 1.220472440944882608, 0.2952755905511811885, 0.000000000000000000 ) ) ;
#65030=CARTESIAN_POINT ( 'NONE',  ( 1.548556430446194954, -0.5023911411419708095, 0.1820866141732285504 ) ) ;
#65032=CARTESIAN_POINT ( 'NONE',  ( -0.4724409448818890911, -0.1870078740157479769, 0.3641732283464567677 ) ) ;
#65033=CARTESIAN_POINT ( 'NONE',  ( -1.561679790026246017, -0.3690944881889765550, -0.3153832671262227771 ) ) ;
#65035=CARTESIAN_POINT ( 'NONE',  ( 0.2952755905511816326, -0.5400638737290844871, 0.3530559997133364547 ) ) ;
#65036=CARTESIAN_POINT ( 'NONE',  ( -0.9317585301837263412, -0.3690944881889765550, -0.3153832671262227771 ) ) ;
#65037=CARTESIAN_POINT ( 'NONE',  ( 0.2624671916010504757, -0.5023911411419708095, -0.1820866141732282451 ) ) ;
#65038=CARTESIAN_POINT ( 'NONE',  ( 0.09842519685039434474, -0.5400638737290845981, -0.3530559997133363437 ) ) ;
#65039=CARTESIAN_POINT ( 'NONE',  ( -1.240157480314959759, -0.4536011799217368745, -0.2665933059059886201 ) ) ;
#65041=CARTESIAN_POINT ( 'NONE',  ( 0.7414698162729663755, -0.6692913385826773087, -0.1292274648535924053 ) ) ;
#65043=CARTESIAN_POINT ( 'NONE',  ( -1.633858267716534529, 0.1660481256975885056, 0.3530559997133364547 ) ) ;
#65045=CARTESIAN_POINT ( 'NONE',  ( -0.4855643044619415427, -0.4281496062992124485, 0.4176697321401328655 ) ) ;
#65046=CARTESIAN_POINT ( 'NONE',  ( 0.1509186351706042484, -0.2845877964562159024, 0.3641732283464567677 ) ) ;
#65047=CARTESIAN_POINT ( 'NONE',  ( -1.062992125984250968, -0.6692913385826771977, 8.415575281601705876E-17 ) ) ;
#65048=CARTESIAN_POINT ( 'NONE',  ( 0.8923884514435703741, 0.1283753931104748280, 0.1820866141732283561 ) ) ;
#65049=CARTESIAN_POINT ( 'NONE',  ( -0.2099737532808391705, -0.5023911411419708095, -0.1820866141732282451 ) ) ;
#65050=CARTESIAN_POINT ( 'NONE',  ( -0.5643044619422565855, 0.05413385826771626580, -0.4176697321401330321 ) ) ;
#65051=CARTESIAN_POINT ( 'NONE',  ( -1.318897637795274802, -0.5400638737290845981, -0.3530559997133363437 ) ) ;
#65052=CARTESIAN_POINT ( 'NONE',  ( 1.679790026246720025, 0.2306618581243848609, 0.2411417322834645549 ) ) ;
#65053=CARTESIAN_POINT ( 'NONE',  ( 1.062992125984252523, 0.2066929133858268208, 0.000000000000000000 ) ) ;
#65054=CARTESIAN_POINT ( 'NONE',  ( 1.253280839895013710, -0.08942795157528024563, -0.3641732283464568787 ) ) ;
#65056=CARTESIAN_POINT ( 'NONE',  ( 0.3083989501312343062, -0.05778040916215560624, -0.4822834645669293319 ) ) ;
#65057=CARTESIAN_POINT ( 'NONE',  ( -1.627296587926508442, 0.2306618581243848609, 0.2411417322834645549 ) ) ;
#65058=CARTESIAN_POINT ( 'NONE',  ( -1.437007874015747477, -0.5400638737290844871, 0.3530559997133364547 ) ) ;
#65061=CARTESIAN_POINT ( 'NONE',  ( -0.6955380577427815458, -0.004921259842519576551, 0.3153832671262227771 ) ) ;
#65062=CARTESIAN_POINT ( 'NONE',  ( 0.8530183727034126306, 0.05413385826771626580, -0.4176697321401330321 ) ) ;
#65063=CARTESIAN_POINT ( 'NONE',  ( -0.9055118110236215490, 0.1771653543307087630, 0.000000000000000000 ) ) ;
#65065=CARTESIAN_POINT ( 'NONE',  ( -1.200787401574802349, 0.1660481256975883668, -0.3530559997133364547 ) ) ;
#65066=CARTESIAN_POINT ( 'NONE',  ( 0.7611548556430454138, 0.2306618581243847221, -0.2411417322834647770 ) ) ;
#65067=CARTESIAN_POINT ( 'NONE',  ( 0.5183727034120741983, -0.6692913385826771977, 0.1292274648535927661 ) ) ;
#65069=CARTESIAN_POINT ( 'NONE',  ( -1.712598425196849572, 0.07958543189024085140, 0.2665933059059887866 ) ) ;
#65075=CARTESIAN_POINT ( 'NONE',  ( 0.8727034120734913358, -0.08942795157527998196, 0.3641732283464567121 ) ) ;
#65076=CARTESIAN_POINT ( 'NONE',  ( 0.2034120734908142214, 0.1771653543307087075, -0.09757992244046823083 ) ) ;
#65077=CARTESIAN_POINT ( 'NONE',  ( 0.03280839895013198948, 0.2952755905511811885, 0.1292274648535926551 ) ) ;
#65078=CARTESIAN_POINT ( 'NONE',  ( 1.115485564304462551, 0.05413385826771666132, 0.4176697321401328100 ) ) ;
#65080=CARTESIAN_POINT ( 'NONE',  ( 0.5839895013123367340, 0.1771653543307087630, 0.09757992244046791164 ) ) ;
#65081=CARTESIAN_POINT ( 'NONE',  ( -0.6692913385826764205, 0.2952755905511811885, 0.000000000000000000 ) ) ;
#65082=CARTESIAN_POINT ( 'NONE',  ( 1.430446194225722500, 0.05413385826771666132, 0.4176697321401328100 ) ) ;
#65083=CARTESIAN_POINT ( 'NONE',  ( 0.9776902887139113929, -0.6692913385826773087, -0.1292274648535924053 ) ) ;
#65085=CARTESIAN_POINT ( 'NONE',  ( 1.171093442848939681, -8.644661201599092366E-16, -0.4445507791589066171 ) ) ;
#65086=VERTEX_POINT ( 'NONE', #14255 ) ;
#65088=CARTESIAN_POINT ( 'NONE',  ( -1.332020997375327642, -0.3162353388693409650, -0.4822834645669289433 ) ) ;
#65089=CARTESIAN_POINT ( 'NONE',  ( -1.181102362204723644, -0.1870078740157479769, 0.4822834645669291653 ) ) ;
#65090=CARTESIAN_POINT ( 'NONE',  ( -0.8595800524934373854, -0.08942795157527998196, 0.3641732283464567121 ) ) ;
#65091=CARTESIAN_POINT ( 'NONE',  ( -0.5708661417322825615, -0.5400638737290844871, 0.3530559997133364547 ) ) ;
#65094=CARTESIAN_POINT ( 'NONE',  ( 1.601049868766404982, -0.6046776061558809534, -0.2411417322834644161 ) ) ;
#65095=CARTESIAN_POINT ( 'NONE',  ( -1.437007874015747477, -0.5400638737290844871, 0.3530559997133364547 ) ) ;
#65096=CARTESIAN_POINT ( 'NONE',  ( 0.4330708661417329575, -0.6692913385826771977, 8.415575281601705876E-17 ) ) ;
#65097=B_SPLINE_CURVE_WITH_KNOTS ( 'NONE', 3,
 ( #53959, #3049, #54378, #68278 ),
 .UNSPECIFIED., .F., .F.,
 ( 4, 4 ),
 ( 1.999999999910059834E-07, 0.006970199999999934261 ),
 .UNSPECIFIED. ) ;
#65098=CARTESIAN_POINT ( 'NONE',  ( -0.9055118110236215490, -0.6692913385826771977, 8.415575281601705876E-17 ) ) ;
#65100=CARTESIAN_POINT ( 'NONE',  ( 0.5577427821522314977, -0.3162353388693409650, -0.4822834645669289433 ) ) ;
#65102=CARTESIAN_POINT ( 'NONE',  ( -0.6889763779527552368, 0.07958543189024085140, 0.2665933059059887866 ) ) ;
#65103=ORIENTED_EDGE ( 'NONE', *, *, #37312, .F. ) ;
#65106=CARTESIAN_POINT ( 'NONE',  ( -1.555118110236219930, 0.07958543189024085140, 0.2665933059059887866 ) ) ;
#65107=CARTESIAN_POINT ( 'NONE',  ( -1.174540682414697335, -0.3162353388693409650, -0.4822834645669289433 ) ) ;
#65108=CARTESIAN_POINT ( 'NONE',  ( -1.213910761154854745, -0.6692913385826771977, 0.1292274648535927661 ) ) ;
#65110=CARTESIAN_POINT ( 'NONE',  ( -0.9251968503937002541, 0.1660481256975885056, 0.3530559997133364547 ) ) ;
#65111=CARTESIAN_POINT ( 'NONE',  ( -1.240157480314959759, 0.1660481256975885056, 0.3530559997133364547 ) ) ;
#65112=CARTESIAN_POINT ( 'NONE',  ( -1.627296587926508442, 0.2306618581243848609, 0.2411417322834645549 ) ) ;
#65113=DIRECTION ( 'NONE',  ( 0.000000000000000000, -1.000000000000000000, 0.000000000000000000 ) ) ;
#65114=EDGE_CURVE ( 'NONE', #44445, #60047, #46209, .T. ) ;
#65115=LINE ( 'NONE', #724, #25402 ) ;
#65116=CARTESIAN_POINT ( 'NONE',  ( 0.1837270341207357105, -0.5023911411419708095, -0.1820866141732282451 ) ) ;
#65119=CARTESIAN_POINT ( 'NONE',  ( -0.2493438320209966919, -0.004921259842519870586, -0.3153832671262229437 ) ) ;
#65121=CARTESIAN_POINT ( 'NONE',  ( -0.9120734908136475250, -0.6692913385826773087, -0.1292274648535924053 ) ) ;
#65123=CARTESIAN_POINT ( 'NONE',  ( 0.8530183727034126306, 0.05413385826771626580, -0.4176697321401330321 ) ) ;
#65124=CARTESIAN_POINT ( 'NONE',  ( -0.3346456692913377662, 0.1660481256975883668, -0.3530559997133364547 ) ) ;
#65126=ORIENTED_EDGE ( 'NONE', *, *, #8539, .T. ) ;
#65128=CARTESIAN_POINT ( 'NONE',  ( -0.9383202099737524282, -0.3162353388693409650, -0.4822834645669289433 ) ) ;
#65129=CARTESIAN_POINT ( 'NONE',  ( 1.200787401574803681, -0.5400638737290845981, -0.3530559997133363437 ) ) ;
#65130=CARTESIAN_POINT ( 'NONE',  ( -1.384514435695537005, 0.1771653543307087630, 0.09757992244046791164 ) ) ;
#65131=CARTESIAN_POINT ( 'NONE',  ( -1.620734908136482577, -0.6692913385826773087, -0.1292274648535924053 ) ) ;
#65136=CARTESIAN_POINT ( 'NONE',  ( -0.2427821522309703550, -0.3162353388693405765, 0.4822834645669290543 ) ) ;
#65137=CARTESIAN_POINT ( 'NONE',  ( 1.692913385826772421, 0.2952755905511811885, 0.000000000000000000 ) ) ;
#65138=CARTESIAN_POINT ( 'NONE',  ( -0.6692913385826764205, -0.6692913385826771977, 8.415575281601705876E-17 ) ) ;
#65140=CARTESIAN_POINT ( 'NONE',  ( -1.167979002624671470, -0.4281496062992127816, -0.4176697321401328100 ) ) ;
#65142=CARTESIAN_POINT ( 'NONE',  ( -1.102362204724408601, -0.1870078740157479769, 0.4822834645669291653 ) ) ;
#65143=CARTESIAN_POINT ( 'NONE',  ( -0.5052493438320203589, -0.6692913385826771977, 0.1292274648535927661 ) ) ;
#65146=CARTESIAN_POINT ( 'NONE',  ( 0.8333333333333340365, 0.1771653543307087075, -0.09757992244046823083 ) ) ;
#65147=CARTESIAN_POINT ( 'NONE',  ( -1.112371124080194340, -2.567464376874931580E-15, -0.4445507791589072832 ) ) ;
#65148=CARTESIAN_POINT ( 'NONE',  ( 0.6036745406824154392, 0.1283753931104746893, -0.1820866141732285504 ) ) ;
#65149=CARTESIAN_POINT ( 'NONE',  ( 1.351706036745407458, -0.3690944881889765550, -0.3153832671262227771 ) ) ;
#65150=CARTESIAN_POINT ( 'NONE',  ( 1.220472440944882386, -0.6692913385826771977, 8.415575281601705876E-17 ) ) ;
#65151=CARTESIAN_POINT ( 'NONE',  ( 0.07874015748031558404, -0.1870078740157479769, 0.3641732283464567677 ) ) ;
#65153=CARTESIAN_POINT ( 'NONE',  ( -1.095800524934382292, -0.3162353388693409650, -0.4822834645669289433 ) ) ;
#65154=CARTESIAN_POINT ( 'NONE',  ( 1.227034120734908917, -0.6692913385826771977, 0.1292274648535927661 ) ) ;
#65155=( BOUNDED_CURVE ( )  B_SPLINE_CURVE ( 1, ( #42274, #3990 ),
 .UNSPECIFIED., .F., .F. ) 
 B_SPLINE_CURVE_WITH_KNOTS ( ( 2, 2 ),
 ( 4.770489558936219510E-18, 0.002000000000000006981 ),
 .UNSPECIFIED. ) 
 CURVE ( )  GEOMETRIC_REPRESENTATION_ITEM ( )  RATIONAL_B_SPLINE_CURVE ( ( 0.9875488213027530104, 0.9875488213027530104 ) ) 
 REPRESENTATION_ITEM ( '' )  );
#65157=CARTESIAN_POINT ( 'NONE',  ( -0.6889763779527552368, 0.07958543189024085140, 0.2665933059059887866 ) ) ;
#65158=CARTESIAN_POINT ( 'NONE',  ( 0.01000891935578606708, -2.191421614605370878E-15, 0.4445507791589071167 ) ) ;
#65159=CARTESIAN_POINT ( 'NONE',  ( 0.4068241469816281097, 0.05413385826771666132, 0.4176697321401328100 ) ) ;
#65160=CYLINDRICAL_SURFACE ( 'NONE', #53250, 2.362204724409449064 ) ;
#65162=CARTESIAN_POINT ( 'NONE',  ( 0.7611548556430451917, -0.5023911411419708095, 0.1820866141732285504 ) ) ;
#65163=CARTESIAN_POINT ( 'NONE',  ( 0.3215223097112867578, -0.08942795157527998196, 0.3641732283464567121 ) ) ;
#65164=CARTESIAN_POINT ( 'NONE',  ( -0.4593175853018364174, -0.4281496062992127816, -0.4176697321401328100 ) ) ;
#65165=CARTESIAN_POINT ( 'NONE',  ( -1.181102362204723644, -0.1870078740157480879, -0.4822834645669291653 ) ) ;
#65166=CARTESIAN_POINT ( 'NONE',  ( -0.8464566929133852113, 0.07958543189024085140, 0.2665933059059887866 ) ) ;
#65168=CARTESIAN_POINT ( 'NONE',  ( 0.5774278215223104249, 0.2306618581243848609, 0.2411417322834645549 ) ) ;
#65169=CARTESIAN_POINT ( 'NONE',  ( -0.7414698162729651543, -0.6692913385826771977, 0.1292274648535927661 ) ) ;
#65172=CARTESIAN_POINT ( 'NONE',  ( 0.1246719160104994284, -0.5511811023622046335, 0.09757992244046803654 ) ) ;
#65173=CARTESIAN_POINT ( 'NONE',  ( -0.6496062992125976043, 0.1660481256975883668, -0.3530559997133364547 ) ) ;
#65174=CARTESIAN_POINT ( 'NONE',  ( -1.292650918635170010, 0.2952755905511810774, -0.1292274648535930714 ) ) ;
#65175=CARTESIAN_POINT ( 'NONE',  ( -1.069553805774277722, -0.5511811023622048555, -0.09757992244046775898 ) ) ;
#65177=CARTESIAN_POINT ( 'NONE',  ( -0.8858267716535425107, -0.4536011799217367080, 0.2665933059059888421 ) ) ;
#65178=CARTESIAN_POINT ( 'NONE',  ( -0.7283464566929126471, 0.1012011053420775880, -0.2882089793578257453 ) ) ;
#65179=CARTESIAN_POINT ( 'NONE',  ( 1.286089238845145033, 0.2306618581243848609, 0.2411417322834645549 ) ) ;
#65185=CARTESIAN_POINT ( 'NONE',  ( -1.601049868766403650, -0.6046776061558807314, 0.2411417322834647770 ) ) ;
#65186=CARTESIAN_POINT ( 'NONE',  ( -1.220472440944881054, 0.2952755905511811885, 0.000000000000000000 ) ) ;
#65187=CARTESIAN_POINT ( 'NONE',  ( 1.069553805774278610, -0.6692913385826771977, 0.1292274648535927661 ) ) ;
#65189=CARTESIAN_POINT ( 'NONE',  ( 1.620734908136483465, -0.5511811023622046335, 0.09757992244046803654 ) ) ;
#65190=CARTESIAN_POINT ( 'NONE',  ( 0.4002624671916016896, -0.05778040916215522460, 0.4822834645669289988 ) ) ;
#65191=CARTESIAN_POINT ( 'NONE',  ( -0.1049868766404193215, -0.6046776061558807314, 0.2411417322834647770 ) ) ;
#65194=CARTESIAN_POINT ( 'NONE',  ( 0.7808398950131240079, -0.2845877964562159024, 0.3641732283464567677 ) ) ;
#65200=CARTESIAN_POINT ( 'NONE',  ( -0.05905511811023545637, -0.5400638737290845981, -0.3530559997133363437 ) ) ;
#65201=CARTESIAN_POINT ( 'NONE',  ( 1.463254593175853824, 0.2952755905511810774, -0.1292274648535930714 ) ) ;
#65202=CARTESIAN_POINT ( 'NONE',  ( 0.5183727034120741983, -0.6692913385826771977, 0.1292274648535927661 ) ) ;
#65203=CARTESIAN_POINT ( 'NONE',  ( 1.174540682414699111, -0.3162353388693405765, 0.4822834645669290543 ) ) ;
#65204=CARTESIAN_POINT ( 'NONE',  ( -0.3412073490813641308, 0.2306618581243847221, -0.2411417322834647770 ) ) ;
#65205=CARTESIAN_POINT ( 'NONE',  ( 0.1509186351706042484, -0.3162353388693405765, 0.4822834645669290543 ) ) ;
#65206=CARTESIAN_POINT ( 'NONE',  ( -1.496062992125983815, -0.1870078740157479769, 0.4822834645669291653 ) ) ;
#65207=CARTESIAN_POINT ( 'NONE',  ( 1.391076115485564868, -0.6046776061558807314, 0.2411417322834647770 ) ) ;
#65208=CARTESIAN_POINT ( 'NONE',  ( 1.272965879265092637, -0.4281496062992127816, -0.4176697321401328100 ) ) ;
#65210=CARTESIAN_POINT ( 'NONE',  ( 0.2427821522309719648, -0.08942795157527998196, 0.3641732283464567121 ) ) ;
#65214=CARTESIAN_POINT ( 'NONE',  ( -0.4265091863517051496, 0.1771653543307087075, -0.09757992244046823083 ) ) ;
#65215=CARTESIAN_POINT ( 'NONE',  ( 0.03280839895013198948, -0.6692913385826773087, -0.1292274648535924053 ) ) ;
#65217=CARTESIAN_POINT ( 'NONE',  ( -0.04593175853018302557, -0.6692913385826773087, -0.1292274648535924053 ) ) ;
#65218=CARTESIAN_POINT ( 'NONE',  ( 0.09842519685039434474, -0.5400638737290845981, -0.3530559997133363437 ) ) ;
#65219=CARTESIAN_POINT ( 'NONE',  ( -0.6889763779527552368, 0.1660481256975885056, 0.3530559997133364547 ) ) ;
#65220=ADVANCED_FACE ( 'NONE', ( #72323 ), #28882, .F. ) ;
#65221=CARTESIAN_POINT ( 'NONE',  ( -1.082677165354329896, 0.1660481256975885056, 0.3530559997133364547 ) ) ;
#65222=CARTESIAN_POINT ( 'NONE',  ( 1.489501312335958172, -0.2845877964562159024, 0.3641732283464567677 ) ) ;
#65225=CARTESIAN_POINT ( 'NONE',  ( 0.9514435695538062676, -0.08942795157527998196, 0.3641732283464567121 ) ) ;
#65226=CARTESIAN_POINT ( 'NONE',  ( 0.5183727034120741983, -0.6692913385826771977, 0.1292274648535927661 ) ) ;
#65227=CARTESIAN_POINT ( 'NONE',  ( 0.6758530183727039509, -0.6692913385826771977, 0.1292274648535927661 ) ) ;
#65229=CARTESIAN_POINT ( 'NONE',  ( -1.633858267716534529, -0.5400638737290845981, -0.3530559997133363437 ) ) ;
#65233=CARTESIAN_POINT ( 'NONE',  ( -0.3805774278215216522, -0.4281496062992127816, -0.4176697321401328100 ) ) ;
#65236=CARTESIAN_POINT ( 'NONE',  ( -1.194225721784776262, -0.3690944881889763329, 0.3153832671262228327 ) ) ;
#65237=CARTESIAN_POINT ( 'NONE',  ( 1.496062992125984703, -0.1870078740157480879, -0.4822834645669291653 ) ) ;
#65238=CARTESIAN_POINT ( 'NONE',  ( 0.8136482939632553313, -0.6046776061558809534, -0.2411417322834644161 ) ) ;
#65239=CARTESIAN_POINT ( 'NONE',  ( -0.2559055118110227234, -0.4536011799217367080, 0.2665933059059888421 ) ) ;
#65240=CARTESIAN_POINT ( 'NONE',  ( 0.4133858267716541968, -0.5400638737290845981, -0.3530559997133363437 ) ) ;
#65242=CARTESIAN_POINT ( 'NONE',  ( 0.3018372703412079971, -0.004921259842519870586, -0.3153832671262229437 ) ) ;
#65243=CARTESIAN_POINT ( 'NONE',  ( -0.1902887139107604098, -0.6692913385826771977, 0.1292274648535927661 ) ) ;
#65245=CARTESIAN_POINT ( 'NONE',  ( -1.062992125984250968, 0.2952755905511811885, 0.000000000000000000 ) ) ;
#65247=CARTESIAN_POINT ( 'NONE',  ( 0.5643044619422579178, -0.3690944881889765550, -0.3153832671262227771 ) ) ;
#65248=CARTESIAN_POINT ( 'NONE',  ( 0.3346456692913390985, 0.1012011053420777407, 0.2882089793578257453 ) ) ;
#65249=CARTESIAN_POINT ( 'NONE',  ( -0.8727034120734901146, -0.05778040916215560624, -0.4822834645669293319 ) ) ;
#65250=CARTESIAN_POINT ( 'NONE',  ( -0.2427821522309703550, -0.2845877964562159024, 0.3641732283464567677 ) ) ;
#65251=CARTESIAN_POINT ( 'NONE',  ( -1.614173228346456712, 0.4410134679336886188, -0.1372047244094478091 ) ) ;
#65252=CARTESIAN_POINT ( 'NONE',  ( -0.7742782152230965886, 0.05413385826771666132, 0.4176697321401328100 ) ) ;
#65253=CARTESIAN_POINT ( 'NONE',  ( -0.7480314960629914633, -0.6692913385826771977, 8.415575281601705876E-17 ) ) ;
#65254=CARTESIAN_POINT ( 'NONE',  ( 0.5249343832021003964, 0.1283753931104746893, -0.1820866141732285504 ) ) ;
#65256=CARTESIAN_POINT ( 'NONE',  ( -0.1640419947506553400, -0.05778040916215560624, -0.4822834645669293319 ) ) ;
#65260=CARTESIAN_POINT ( 'NONE',  ( 0.8267716535433078384, -0.5511811023622047445, 6.969142054262312111E-17 ) ) ;
#65261=CARTESIAN_POINT ( 'NONE',  ( 1.345144356955381593, -0.3162353388693409650, -0.4822834645669289433 ) ) ;
#65262=CARTESIAN_POINT ( 'NONE',  ( -0.7939632545931754048, -0.2845877964562159024, 0.3641732283464567677 ) ) ;
#65263=CARTESIAN_POINT ( 'NONE',  ( -1.161417322834644716, -0.4536011799217368745, -0.2665933059059886201 ) ) ;
#65264=CARTESIAN_POINT ( 'NONE',  ( -0.8005249343832011588, 0.05413385826771626580, -0.4176697321401330321 ) ) ;
#65265=CARTESIAN_POINT ( 'NONE',  ( -0.2165354330708654795, -0.5400638737290845981, -0.3530559997133363437 ) ) ;
#65266=CARTESIAN_POINT ( 'NONE',  ( 0.5446194225721792126, -0.2845877964562159024, 0.3641732283464567677 ) ) ;
#65268=CARTESIAN_POINT ( 'NONE',  ( 1.036745406824147508, -0.3690944881889765550, -0.3153832671262227771 ) ) ;
#65269=CARTESIAN_POINT ( 'NONE',  ( 0.4265091863517067594, 0.2952755905511811885, 0.1292274648535926551 ) ) ;
#65271=CARTESIAN_POINT ( 'NONE',  ( -0.5314960629921254842, -0.5400638737290845981, -0.3530559997133363437 ) ) ;
#65273=CARTESIAN_POINT ( 'NONE',  ( 1.522309711286089939, -0.5023911411419708095, -0.1820866141732282451 ) ) ;
#65274=CARTESIAN_POINT ( 'NONE',  ( 0.5643044619422579178, 0.05413385826771666132, 0.4176697321401328100 ) ) ;
#65275=CARTESIAN_POINT ( 'NONE',  ( 0.1246719160104994284, 0.2952755905511810774, -0.1292274648535930714 ) ) ;
#65277=CARTESIAN_POINT ( 'NONE',  ( 0.09842519685039434474, 0.07958543189024085140, 0.2665933059059887866 ) ) ;
#65278=CARTESIAN_POINT ( 'NONE',  ( 0.7939632545931766261, -0.3162353388693409650, -0.4822834645669289433 ) ) ;
#65279=CARTESIAN_POINT ( 'NONE',  ( -0.6299212598425188991, -0.1870078740157479769, 0.3641732283464567677 ) ) ;
#65280=CARTESIAN_POINT ( 'NONE',  ( -0.6758530183727028406, 0.2952755905511811885, 0.1292274648535926551 ) ) ;
#65282=CARTESIAN_POINT ( 'NONE',  ( -0.3543307086614165824, -0.6692913385826771977, 8.415575281601705876E-17 ) ) ;
#65285=CARTESIAN_POINT ( 'NONE',  ( -1.181102362204723644, -0.1870078740157479769, 0.4822834645669291653 ) ) ;
#65286=CARTESIAN_POINT ( 'NONE',  ( -1.286089238845143479, -0.5023911411419708095, 0.1820866141732285504 ) ) ;
#65287=CARTESIAN_POINT ( 'NONE',  ( -0.1246719160104980823, 0.2952755905511811885, 0.1292274648535926551 ) ) ;
#65289=CARTESIAN_POINT ( 'NONE',  ( -0.7152230971128602510, -0.3162353388693405765, 0.4822834645669290543 ) ) ;
#65291=CARTESIAN_POINT ( 'NONE',  ( 1.082677165354331228, 0.1660481256975883391, -0.3530559997133364547 ) ) ;
#65292=CARTESIAN_POINT ( 'NONE',  ( 0.8464566929133865436, 0.1660481256975883668, -0.3530559997133364547 ) ) ;
#65293=CARTESIAN_POINT ( 'NONE',  ( 1.404199475065617708, 0.05413385826771626580, -0.4176697321401330321 ) ) ;
#65296=CARTESIAN_POINT ( 'NONE',  ( -1.384514435695537005, 0.2952755905511811885, 0.1292274648535926551 ) ) ;
#65300=ORIENTED_EDGE ( 'NONE', *, *, #14652, .T. ) ;
#65301=CARTESIAN_POINT ( 'NONE',  ( -0.1574803149606292529, -0.1870078740157480601, -0.3641732283464567677 ) ) ;
#65304=CARTESIAN_POINT ( 'NONE',  ( 0.07874015748031558404, -0.1870078740157480879, -0.4822834645669291653 ) ) ;
#65305=CARTESIAN_POINT ( 'NONE',  ( -0.1443569553805768291, 0.05413385826771666132, 0.4176697321401328100 ) ) ;
#65306=CARTESIAN_POINT ( 'NONE',  ( -0.6036745406824141069, -0.6046776061558809534, -0.2411417322834644161 ) ) ;
#65308=CARTESIAN_POINT ( 'NONE',  ( -0.7283464566929126471, -0.4536011799217367080, 0.2665933059059888421 ) ) ;
#65310=CARTESIAN_POINT ( 'NONE',  ( 0.9514435695538062676, -0.3162353388693409650, -0.4822834645669289433 ) ) ;
#65311=CARTESIAN_POINT ( 'NONE',  ( 0.5839895013123367340, -0.5511811023622048555, -0.09757992244046775898 ) ) ;
#65312=CARTESIAN_POINT ( 'NONE',  ( -0.4724409448818890911, -0.1870078740157480879, -0.4822834645669291653 ) ) ;
#65314=CARTESIAN_POINT ( 'NONE',  ( -0.8005249343832011588, 0.05413385826771626580, -0.4176697321401330321 ) ) ;
#65317=CARTESIAN_POINT ( 'NONE',  ( 1.509186351706037543, 0.05413385826771666132, 0.4176697321401328100 ) ) ;
#65321=CARTESIAN_POINT ( 'NONE',  ( -0.05249343832020911260, 0.2306618581243848609, 0.2411417322834645549 ) ) ;
#65324=CARTESIAN_POINT ( 'NONE',  ( -0.8398950131233589023, -0.6046776061558809534, -0.2411417322834644161 ) ) ;
#65325=CARTESIAN_POINT ( 'NONE',  ( 1.272965879265092637, 0.05413385826771666132, 0.4176697321401328100 ) ) ;
#65326=CARTESIAN_POINT ( 'NONE',  ( 1.410761154855643795, -0.3162353388693405765, 0.4822834645669290543 ) ) ;
#65327=CARTESIAN_POINT ( 'NONE',  ( 0.1640419947506569498, -0.05778040916215522460, 0.4822834645669289988 ) ) ;
#65328=CARTESIAN_POINT ( 'NONE',  ( -0.1968503937007867743, 0.2952755905511811885, 0.000000000000000000 ) ) ;
#65330=CARTESIAN_POINT ( 'NONE',  ( -1.397637795275589623, 0.1660481256975885056, 0.3530559997133364547 ) ) ;
#65331=CARTESIAN_POINT ( 'NONE',  ( -0.2034120734908128059, 0.2952755905511811885, 0.1292274648535926551 ) ) ;
#65332=CARTESIAN_POINT ( 'NONE',  ( -0.3215223097112853146, -0.08942795157528024563, -0.3641732283464568787 ) ) ;
#65333=CARTESIAN_POINT ( 'NONE',  ( -1.603475055217291612, 0.7166759647713525361, -0.04573490813648263542 ) ) ;
#65334=CARTESIAN_POINT ( 'NONE',  ( 1.358267716535433323, 0.1660481256975885056, 0.3530559997133364547 ) ) ;
#65335=CARTESIAN_POINT ( 'NONE',  ( -0.6167979002624665030, 0.05413385826771666132, 0.4176697321401328100 ) ) ;
#65336=CARTESIAN_POINT ( 'NONE',  ( 0.2952755905511819101, 0.1012011053420775880, -0.2882089793578256898 ) ) ;
#65337=CARTESIAN_POINT ( 'NONE',  ( 1.174540682414699111, -0.05778040916215560624, -0.4822834645669293319 ) ) ;
#65338=CARTESIAN_POINT ( 'NONE',  ( -0.3049517105654738214, -2.191421614605370878E-15, 0.4445507791589071167 ) ) ;
#65339=( BOUNDED_SURFACE ( )  B_SPLINE_SURFACE ( 1, 2, ( 
 ( #18103, #76174, #70672, #58030, #63941, #76994, #37855, #76582, #5458, #44154, #44977, #82081, #82487, #13028, #5051, #12606, #83306, #18910, #44561, #6278, #38264, #12197, #82896, #64360, #30720, #69846, #31538, #31120, #56787, #70251, #57194, #23989, #50882, #31954, #6697, #19325, #24802, #49656, #25628, #56383, #24396, #50066, #75761, #43736, #51291, #69441, #11793, #20999, #59704, #64778, #8376, #26889, #1239, #393, #65635, #59291, #40358, #7965, #79097, #52128, #77837, #39520, #1648, #8787, #65208, #32787, #26051, #52548, #34041, #34460, #7545, #15111, #2059, #27305, #21416, #78257, #51710, #66451, #33627, #39096, #52964, #33218, #47070, #71097, #27723, #78678, #20166, #816, #71515, #26478, #66037, #39949, #77411, #46661, #53390, #58881, #72761, #19746, #72355, #20588, #14703, #45401, #40766, #13440, #7116, #58456, #45816, #13861, #46240, #71936, #14285, #41593, #22242, #61362, #53795, #28139, #74010, #67283, #54211, #10454, #79507, #2480, #21823, #3299, #60540, #29378, #28963, #60949, #47897, #73178, #4121, #80341, #2891, #47485, #36109, #79926, #61780, #15528, #54628, #28555, #34879, #9206, #67696, #41186, #60129, #74425, #66876, #73605, #9616, #15947, #35287, #22654, #48313, #16357, #35696, #42002, #10032, #42410, #3715, #55039, #80746, #23060, #48728, #16772, #68107, #20441, #33897, #9066, #77690, #34738, #66729, #46094, #1918, #60398, #2749, #59149, #71367, #71787, #20857, #15382, #51985, #8647, #21681, #65896, #21271, #33487, #46509, #73032, #26745, #27159, #41044, #33061, #40625, #2338, #46926, #72619, #34318, #66307, #40214, #27580, #20020, #45671, #72210, #14562, #7820, #1506, #8232, #13716, #59562, #53237, #39370, #65056, #78953, #14967, #7393, #59979, #27994, #53654, #79362, #58732, #47343, #1094, #52400, #78109, #14141, #39793, #65488, #52822, #78533, #26933, #21868, #15575, #72806, #41639, #40812, #41233, #8419, #60587, #67330, #79555, #27769, #47533, #1284, #8831, #2937, #53842, #66497, #66920, #52594, #8009, #15155, #21459, #59750, #14748, #73224, #78301, #20633, #34508, #2104, #46705, #47948, #46284, #71980, #14334, #47117, #1692, #9252, #60171, #79142, #40402, #39992, #33263, #2526, #27350, #65682, #73650, #21046, #15992, #33673, #28184, #78721, #59335, #53008, #34924, #72399, #58925, #66083, #34087, #53434, #28601, #79974, #54258, #22287, #62658, #23519, #62238, #74473, #61827, #30667, #67745, #68156, #82029, #74056, #81622, #43273, #4576, #30247, #49603, #23935, #81204, #68560, #56330, #60996, #4167, #29831, #48774, #16820, #49188, #18051, #74891, #17237, #50012, #24343, #55494, #55910, #48358, #42867, #10903, #36561, #68970, #3345, #75297, #17641, #43684, #4999, #75710, #9663, #29009, #55082, #80387, #11319, #36978, #35333, #54675, #16403, #22699, #42049, #10078, #35742, #23106, #61410, #42456, #3759, #29424, #80791, #10500, #36154, #82839, #44507, #57142, #25161, #19689, #25574, #51239, #5405, #31067, #56736, #12551, #45347, #77358, #6640, #70196, #6223, #50419, #76938, #71043, #20115, #82433, #24751, #76119, #5811, #12142, #13388, #7064, #31481, #70616, #38210, #50829, #63885, #76531, #31899, #39040, #32733, #18460, #44919, #11741, #44103, #18859, #57560, #83251, #19266, #12971, #69387, #38628, #37799, #64306, #26421, #37396, #52074, #760, #63476, #32312, #77781, #57975, #340, #25996, #63068, #69796, #51653, #64725, #58400, #79043, #2837, #54158, #52910, #65153, #39891, #14647, #9156, #79873, #2428, #15475, #59650, #15056, #27251, #40304, #66823, #20533, #20948, #34829, #26836, #34405, #79450, #40712, #66397, #28084, #60073, #33988, #21362, #60487, #13808, #65984, #8322, #1596, #78624, #2006, #45762, #27668, #53334, #28500, #71461, #47015, #8735, #1185, #72709, #53742, #21770, #47432, #39467, #73125, #41132, #7490, #33159, #58828, #52494, #78203, #7912, #46185, #71882, #14231, #65578, #33573, #59235, #46605, #72301, #54577, #48264, #35648, #49506, #61309, #23838, #17139, #73961, #42771, #75199, #3666, #80698, #9979, #29329, #55810, #61732, #4069, #41545, #67234, #9564, #48679, #81517, #30149, #68467, #23011, #42358 ),
 ( #54990, #16718, #41950, #68056, #17543, #68872, #28913, #81105, #47847, #80290, #74374, #10403, #36060, #29736, #55399, #56233, #35235, #43175, #23422, #30568, #49088, #11220, #60898, #36880, #74788, #10805, #36465, #22190, #62140, #4479, #62558, #4893, #73553, #15897, #3250, #22604, #16307, #67645, #24654, #43588, #57044, #25057, #31795, #19164, #57871, #62971, #6542, #50732, #82738, #81931, #63784, #57458, #38525, #6123, #77253, #50322, #76019, #37698, #83151, #6957, #63373, #30968, #24242, #76431, #32212, #32627, #5708, #13287, #237, #25471, #19582, #18759, #49915, #64620, #51137, #37296, #76832, #31379, #45242, #69289, #25889, #44814, #75613, #17951, #11636, #70510, #64208, #38108, #5309, #12868, #51549, #44403, #70942, #56635, #38939, #70095, #82336, #18361, #44005, #69698, #12042, #12449, #66294, #26312, #33046, #14548, #46495, #1492, #39779, #14953, #77678, #51970, #59549, #27145, #71773, #73018, #20008, #45659, #71355, #72191, #26733, #8633, #40200, #20843, #65473, #13701, #9049, #65883, #52387, #39357, #15369, #46080, #41030, #65041, #8219, #20427, #1080, #58715, #78934, #7378, #58290, #21257, #655, #66716, #78096, #33883, #7807, #21668, #14126, #2321, #1904, #33472, #59134, #52809, #46911, #40611, #27565, #78519, #53224, #34304, #72606, #27981, #59965, #53640, #79347, #47327, #2733, #11428, #5508, #56431, #67953, #43787, #28394, #9457, #74272, #22907, #61205, #16201, #75812, #54053, #79767, #37083, #3562, #48165, #50521, #22084, #47743, #73441, #48575, #3147, #69493, #16616, #80599, #41848, #15791, #69894, #42258, #28810, #41443, #76227, #22502, #18561, #67127, #62769, #80187, #60794, #35130, #82133, #54474, #34724, #24447, #60384, #44204, #73860, #56837, #5103, #67538, #30770, #37495, #9875, #31171, #50115, #18155, #54894, #35544, #11842, #63170, #29227, #82535, #24853, #46295, #71151, #78311, #5915, #25266, #38319, #57244, #70729, #38736, #45453, #32842, #71568, #76630, #20221, #64413, #13083, #12248, #77467, #13492, #52186, #19804, #7601, #63993, #6334, #51342, #39148, #20642, #77046, #44609, #37904, #6748, #45870, #63581, #19378, #26943, #13919, #64833, #33275, #32420, #31589, #82948, #7171, #45030, #50932, #32007, #58082, #58935, #18961, #77890, #65265, #26103, #58511, #448, #51765, #1293, #70305, #874, #52604, #12658, #26533, #39575, #57667, #29, #25682, #60597, #60183, #47543, #9673, #40003, #66507, #8841, #27780, #79152, #28193, #80397, #53851, #79564, #29020, #61006, #40822, #9263, #27358, #2535, #21879, #73233, #22296, #65691, #15584, #28611, #22710, #41649, #35344, #54686, #8019, #34096, #59344, #41243, #16002, #54268, #34934, #78732, #3355, #66930, #21055, #14756, #2114, #67340, #53443, #73661, #2946, #40411, #79983, #71990, #21468, #47126, #59759, #72816, #47957, #14343, #33682, #1701, #53017, #46715, #15166, #72407, #66092, #8428, #34517, #68568, #29434, #4583, #82036, #82441, #10089, #67755, #61420, #68166, #74483, #75718, #69396, #10509, #49609, #49197, #36162, #42875, #61836, #10910, #50019, #11748, #55093, #23942, #74067, #80801, #4177, #36568, #62246, #30254, #55918, #48368, #81631, #16830, #75304, #5414, #16413, #31075, #63076, #42466, #17648, #56743, #42060, #35754, #3770, #43280, #29840, #55504, #48786, #68979, #23118, #81212, #11327, #23527, #74898, #17246, #37404, #36987, #62666, #5006, #18058, #30676, #43691, #56337, #24350, #44929, #24758, #51664, #64316, #65165, #20125, #57570, #58838, #350, #7501, #18468, #37807, #50840, #69803, #83262, #51248, #57985, #45357, #770, #5819, #32744, #76950, #25584, #50426, #6650, #26007, #64736, #32323, #45772, #76540, #18868, #63895, #77368, #33170, #6233, #57151, #76126, #19277, #58411, #44111, #31909, #39478, #26432, #19700, #71471, #70626, #12151, #63485, #71054, #31490, #13398, #12982, #13819, #82850, #52083, #39051, #25171, #44517, #70204, #7074, #77792, #12562, #38220, #38638, #9166, #59661, #28511, #9574, #47442, #79056, #73136, #52504, #60085, #54168, #21780, #34417, #34838, #78213, #59246, #40723, #72720, #27681, #65995, #41143, #20545, #46197, #2439, #53346, #14659 ) ),
 .UNSPECIFIED., .F., .F., .F. ) 
 B_SPLINE_SURFACE_WITH_KNOTS ( ( 2, 2 ),
 ( 3, 2, 2, 2, 2, 2, 2, 2, 2, 2, 2, 2, 2, 2, 2, 2, 2, 2, 2, 2, 2, 2, 2, 2, 2, 2, 2, 2, 2, 2, 2, 2, 2, 2, 2, 2, 2, 2, 2, 2, 2, 2, 2, 2, 2, 2, 2, 2, 2, 2, 2, 2, 2, 2, 2, 2, 2, 2, 2, 2, 2, 2, 2, 2, 2, 2, 2, 2, 2, 2, 2, 2, 2, 2, 2, 2, 2, 2, 2, 2, 2, 2, 2, 2, 2, 2, 2, 2, 2, 2, 2, 2, 2, 2, 2, 2, 2, 2, 2, 2, 2, 2, 2, 2, 2, 2, 2, 2, 2, 2, 2, 2, 2, 2, 2, 2, 2, 2, 2, 2, 2, 2, 2, 2, 2, 2, 2, 2, 2, 2, 2, 2, 2, 2, 2, 2, 2, 2, 2, 2, 2, 2, 2, 2, 2, 2, 2, 2, 2, 2, 2, 2, 2, 2, 2, 2, 2, 2, 2, 2, 2, 2, 2, 2, 2, 2, 2, 2, 2, 2, 2, 2, 2, 2, 2, 2, 2, 2, 2, 2, 2, 2, 2, 2, 2, 2, 2, 2, 2, 2, 2, 2, 2, 2, 2, 2, 2, 2, 2, 2, 2, 2, 2, 2, 2, 2, 2, 2, 2, 2, 2, 2, 2, 2, 2, 2, 2, 2, 2, 2, 2, 2, 2, 2, 2, 2, 2, 2, 2, 2, 2, 2, 2, 2, 2, 2, 2, 2, 2, 2, 2, 2, 2, 2, 2, 2, 2, 2, 2, 2, 2, 2, 2, 2, 2, 3 ),
 ( 0.000000000000000000, 1.000000000000000000 ),
 ( 0.000000000000000000, 0.003787878787878787984, 0.007575757575757575968, 0.01136363636363636395, 0.01515151515151515194, 0.01893939393939393992, 0.02272727272727272790, 0.02651515151515151589, 0.03030303030303030387, 0.03409090909090908839, 0.03787878787878787984, 0.04166666666666666435, 0.04545454545454545581, 0.04924242424242424032, 0.05303030303030303177, 0.05681818181818181629, 0.06060606060606060774, 0.06439393939393939226, 0.06818181818181817677, 0.07196969696969697516, 0.07575757575757575968, 0.07954545454545454419, 0.08333333333333332871, 0.08712121212121212710, 0.09090909090909091161, 0.09469696969696969613, 0.09848484848484848064, 0.1022727272727272790, 0.1060606060606060635, 0.1098484848484848481, 0.1136363636363636326, 0.1174242424242424310, 0.1212121212121212155, 0.1250000000000000000, 0.1287878787878787845, 0.1325757575757575690, 0.1363636363636363535, 0.1401515151515151381, 0.1439393939393939503, 0.1477272727272727348, 0.1515151515151515194, 0.1553030303030303039, 0.1590909090909090884, 0.1628787878787878729, 0.1666666666666666574, 0.1704545454545454419, 0.1742424242424242542, 0.1780303030303030387, 0.1818181818181818232, 0.1856060606060606077, 0.1893939393939393923, 0.1931818181818181768, 0.1969696969696969613, 0.2007575757575757458, 0.2045454545454545581, 0.2083333333333333426, 0.2121212121212121271, 0.2159090909090909116, 0.2196969696969696961, 0.2234848484848484806, 0.2272727272727272652, 0.2310606060606060497, 0.2348484848484848619, 0.2386363636363636465, 0.2424242424242424310, 0.2462121212121212155, 0.2500000000000000000, 0.2537878787878787845, 0.2575757575757575690, 0.2613636363636363535, 0.2651515151515151381, 0.2689393939393939226, 0.2727272727272727071, 0.2765151515151514916, 0.2803030303030302761, 0.2840909090909091161, 0.2878787878787879007, 0.2916666666666666852, 0.2954545454545454697, 0.2992424242424242542, 0.3030303030303030387, 0.3068181818181818232, 0.3106060606060606077, 0.3143939393939393923, 0.3181818181818181768, 0.3219696969696969613, 0.3257575757575757458, 0.3295454545454545303, 0.3333333333333333148, 0.3371212121212120993, 0.3409090909090908839, 0.3446969696969697239, 0.3484848484848485084, 0.3522727272727272929, 0.3560606060606060774, 0.3598484848484848619, 0.3636363636363636465, 0.3674242424242424310, 0.3712121212121212155, 0.3750000000000000000, 0.3787878787878787845, 0.3825757575757575690, 0.3863636363636363535, 0.3901515151515151381, 0.3939393939393939226, 0.3977272727272727071, 0.4015151515151514916, 0.4053030303030302761, 0.4090909090909091161, 0.4128787878787879007, 0.4166666666666666852, 0.4204545454545454697, 0.4242424242424242542, 0.4280303030303030387, 0.4318181818181818232, 0.4356060606060606077, 0.4393939393939393923, 0.4431818181818181768, 0.4469696969696969613, 0.4507575757575757458, 0.4545454545454545303, 0.4583333333333333148, 0.4621212121212120993, 0.4659090909090908839, 0.4696969696969697239, 0.4734848484848485084, 0.4772727272727272929, 0.4810606060606060774, 0.4848484848484848619, 0.4886363636363636465, 0.4924242424242424310, 0.4962121212121212155, 0.5000000000000000000, 0.5037878787878787845, 0.5075757575757575690, 0.5113636363636363535, 0.5151515151515151381, 0.5189393939393939226, 0.5227272727272727071, 0.5265151515151514916, 0.5303030303030302761, 0.5340909090909090606, 0.5378787878787878451, 0.5416666666666666297, 0.5454545454545454142, 0.5492424242424241987, 0.5530303030303029832, 0.5568181818181817677, 0.5606060606060605522, 0.5643939393939394478, 0.5681818181818182323, 0.5719696969696970168, 0.5757575757575758013, 0.5795454545454545858, 0.5833333333333333703, 0.5871212121212121549, 0.5909090909090909394, 0.5946969696969697239, 0.5984848484848485084, 0.6022727272727272929, 0.6060606060606060774, 0.6098484848484848619, 0.6136363636363636465, 0.6174242424242424310, 0.6212121212121212155, 0.6250000000000000000, 0.6287878787878787845, 0.6325757575757575690, 0.6363636363636363535, 0.6401515151515151381, 0.6439393939393939226, 0.6477272727272727071, 0.6515151515151514916, 0.6553030303030302761, 0.6590909090909090606, 0.6628787878787878451, 0.6666666666666666297, 0.6704545454545454142, 0.6742424242424241987, 0.6780303030303029832, 0.6818181818181817677, 0.6856060606060605522, 0.6893939393939394478, 0.6931818181818182323, 0.6969696969696970168, 0.7007575757575758013, 0.7045454545454545858, 0.7083333333333333703, 0.7121212121212121549, 0.7159090909090909394, 0.7196969696969697239, 0.7234848484848485084, 0.7272727272727272929, 0.7310606060606060774, 0.7348484848484848619, 0.7386363636363636465, 0.7424242424242424310, 0.7462121212121212155, 0.7500000000000000000, 0.7537878787878787845, 0.7575757575757575690, 0.7613636363636363535, 0.7651515151515151381, 0.7689393939393939226, 0.7727272727272727071, 0.7765151515151514916, 0.7803030303030302761, 0.7840909090909090606, 0.7878787878787878451, 0.7916666666666666297, 0.7954545454545454142, 0.7992424242424241987, 0.8030303030303029832, 0.8068181818181817677, 0.8106060606060605522, 0.8143939393939394478, 0.8181818181818182323, 0.8219696969696970168, 0.8257575757575758013, 0.8295454545454545858, 0.8333333333333333703, 0.8371212121212121549, 0.8409090909090909394, 0.8446969696969697239, 0.8484848484848485084, 0.8522727272727272929, 0.8560606060606060774, 0.8598484848484848619, 0.8636363636363636465, 0.8674242424242424310, 0.8712121212121212155, 0.8750000000000000000, 0.8787878787878787845, 0.8825757575757575690, 0.8863636363636363535, 0.8901515151515151381, 0.8939393939393939226, 0.8977272727272727071, 0.9015151515151514916, 0.9053030303030302761, 0.9090909090909090606, 0.9128787878787878451, 0.9166666666666666297, 0.9204545454545454142, 0.9242424242424241987, 0.9280303030303029832, 0.9318181818181817677, 0.9356060606060605522, 0.9393939393939394478, 0.9431818181818182323, 0.9469696969696970168, 0.9507575757575758013, 0.9545454545454545858, 0.9583333333333333703, 0.9621212121212121549, 0.9659090909090909394 ),
 .UNSPECIFIED. ) 
 GEOMETRIC_REPRESENTATION_ITEM ( )  RATIONAL_B_SPLINE_SURFACE ( (
 ( 1.000000000000000000, 0.9659258262890683122, 1.000000000000000000, 0.9659258262890683122, 1.000000000000000000, 0.9659258262890683122, 1.000000000000000000, 0.9659258262890683122, 1.000000000000000000, 0.9659258262890683122, 1.000000000000000000, 0.9659258262890683122, 1.000000000000000000, 0.9659258262890683122, 1.000000000000000000, 0.9659258262890683122, 1.000000000000000000, 0.9659258262890683122, 1.000000000000000000, 0.9659258262890683122, 1.000000000000000000, 0.9659258262890683122, 1.000000000000000000, 0.9659258262890683122, 1.000000000000000000, 0.9659258262890683122, 1.000000000000000000, 0.9659258262890683122, 1.000000000000000000, 0.9659258262890683122, 1.000000000000000000, 0.9659258262890683122, 1.000000000000000000, 0.9659258262890683122, 1.000000000000000000, 0.9659258262890683122, 1.000000000000000000, 0.9659258262890683122, 1.000000000000000000, 0.9659258262890683122, 1.000000000000000000, 0.9659258262890683122, 1.000000000000000000, 0.9659258262890683122, 1.000000000000000000, 0.9659258262890683122, 1.000000000000000000, 0.9659258262890683122, 1.000000000000000000, 0.9659258262890683122, 1.000000000000000000, 0.9659258262890683122, 1.000000000000000000, 0.9659258262890683122, 1.000000000000000000, 0.9659258262890683122, 1.000000000000000000, 0.9659258262890683122, 1.000000000000000000, 0.9659258262890683122, 1.000000000000000000, 0.9659258262890683122, 1.000000000000000000, 0.9659258262890683122, 1.000000000000000000, 0.9659258262890683122, 1.000000000000000000, 0.9659258262890683122, 1.000000000000000000, 0.9659258262890683122, 1.000000000000000000, 0.9659258262890683122, 1.000000000000000000, 0.9659258262890683122, 1.000000000000000000, 0.9659258262890683122, 1.000000000000000000, 0.9659258262890683122, 1.000000000000000000, 0.9659258262890683122, 1.000000000000000000, 0.9659258262890683122, 1.000000000000000000, 0.9659258262890683122, 1.000000000000000000, 0.9659258262890683122, 1.000000000000000000, 0.9659258262890683122, 1.000000000000000000, 0.9659258262890683122, 1.000000000000000000, 0.9659258262890683122, 1.000000000000000000, 0.9659258262890683122, 1.000000000000000000, 0.9659258262890683122, 1.000000000000000000, 0.9659258262890683122, 1.000000000000000000, 0.9659258262890683122, 1.000000000000000000, 0.9659258262890683122, 1.000000000000000000, 0.9659258262890683122, 1.000000000000000000, 0.9659258262890683122, 1.000000000000000000, 0.9659258262890683122, 1.000000000000000000, 0.9659258262890683122, 1.000000000000000000, 0.9659258262890683122, 1.000000000000000000, 0.9659258262890683122, 1.000000000000000000, 0.9659258262890683122, 1.000000000000000000, 0.9659258262890683122, 1.000000000000000000, 0.9659258262890683122, 1.000000000000000000, 0.9659258262890683122, 1.000000000000000000, 0.9659258262890683122, 1.000000000000000000, 0.9659258262890683122, 1.000000000000000000, 0.9659258262890683122, 1.000000000000000000, 0.9659258262890683122, 1.000000000000000000, 0.9659258262890683122, 1.000000000000000000, 0.9659258262890683122, 1.000000000000000000, 0.9659258262890683122, 1.000000000000000000, 0.9659258262890683122, 1.000000000000000000, 0.9659258262890683122, 1.000000000000000000, 0.9659258262890683122, 1.000000000000000000, 0.9659258262890683122, 1.000000000000000000, 0.9659258262890683122, 1.000000000000000000, 0.9659258262890683122, 1.000000000000000000, 0.9659258262890683122, 1.000000000000000000, 0.9659258262890683122, 1.000000000000000000, 0.9659258262890683122, 1.000000000000000000, 0.9659258262890683122, 1.000000000000000000, 0.9659258262890683122, 1.000000000000000000, 0.9659258262890683122, 1.000000000000000000, 0.9659258262890683122, 1.000000000000000000, 0.9659258262890683122, 1.000000000000000000, 0.9659258262890683122, 1.000000000000000000, 0.9659258262890683122, 1.000000000000000000, 0.9659258262890683122, 1.000000000000000000, 0.9659258262890683122, 1.000000000000000000, 0.9659258262890683122, 1.000000000000000000, 0.9659258262890683122, 1.000000000000000000, 0.9659258262890683122, 1.000000000000000000, 0.9659258262890683122, 1.000000000000000000, 0.9659258262890683122, 1.000000000000000000, 0.9659258262890683122, 1.000000000000000000, 0.9659258262890683122, 1.000000000000000000, 0.9659258262890683122, 1.000000000000000000, 0.9659258262890683122, 1.000000000000000000, 0.9659258262890683122, 1.000000000000000000, 0.9659258262890683122, 1.000000000000000000, 0.9659258262890683122, 1.000000000000000000, 0.9659258262890683122, 1.000000000000000000, 0.9659258262890683122, 1.000000000000000000, 0.9659258262890683122, 1.000000000000000000, 0.9659258262890683122, 1.000000000000000000, 0.9659258262890683122, 1.000000000000000000, 0.9659258262890683122, 1.000000000000000000, 0.9659258262890683122, 1.000000000000000000, 0.9659258262890683122, 1.000000000000000000, 0.9659258262890683122, 1.000000000000000000, 0.9659258262890683122, 1.000000000000000000, 0.9659258262890683122, 1.000000000000000000, 0.9659258262890683122, 1.000000000000000000, 0.9659258262890683122, 1.000000000000000000, 0.9659258262890683122, 1.000000000000000000, 0.9659258262890683122, 1.000000000000000000, 0.9659258262890683122, 1.000000000000000000, 0.9659258262890683122, 1.000000000000000000, 0.9659258262890683122, 1.000000000000000000, 0.9659258262890683122, 1.000000000000000000, 0.9659258262890683122, 1.000000000000000000, 0.9659258262890683122, 1.000000000000000000, 0.9659258262890683122, 1.000000000000000000, 0.9659258262890683122, 1.000000000000000000, 0.9659258262890683122, 1.000000000000000000, 0.9659258262890683122, 1.000000000000000000, 0.9659258262890683122, 1.000000000000000000, 0.9659258262890683122, 1.000000000000000000, 0.9659258262890683122, 1.000000000000000000, 0.9659258262890683122, 1.000000000000000000, 0.9659258262890683122, 1.000000000000000000, 0.9659258262890683122, 1.000000000000000000, 0.9659258262890683122, 1.000000000000000000, 0.9659258262890683122, 1.000000000000000000, 0.9659258262890683122, 1.000000000000000000, 0.9659258262890683122, 1.000000000000000000, 0.9659258262890683122, 1.000000000000000000, 0.9659258262890683122, 1.000000000000000000, 0.9659258262890683122, 1.000000000000000000, 0.9659258262890683122, 1.000000000000000000, 0.9659258262890683122, 1.000000000000000000, 0.9659258262890683122, 1.000000000000000000, 0.9659258262890683122, 1.000000000000000000, 0.9659258262890683122, 1.000000000000000000, 0.9659258262890683122, 1.000000000000000000, 0.9659258262890683122, 1.000000000000000000, 0.9659258262890683122, 1.000000000000000000, 0.9659258262890683122, 1.000000000000000000, 0.9659258262890683122, 1.000000000000000000, 0.9659258262890683122, 1.000000000000000000, 0.9659258262890683122, 1.000000000000000000, 0.9659258262890683122, 1.000000000000000000, 0.9659258262890683122, 1.000000000000000000, 0.9659258262890683122, 1.000000000000000000, 0.9659258262890683122, 1.000000000000000000, 0.9659258262890683122, 1.000000000000000000, 0.9659258262890683122, 1.000000000000000000, 0.9659258262890683122, 1.000000000000000000, 0.9659258262890683122, 1.000000000000000000, 0.9659258262890683122, 1.000000000000000000, 0.9659258262890683122, 1.000000000000000000, 0.9659258262890683122, 1.000000000000000000, 0.9659258262890683122, 1.000000000000000000, 0.9659258262890683122, 1.000000000000000000, 0.9659258262890683122, 1.000000000000000000, 0.9659258262890683122, 1.000000000000000000, 0.9659258262890683122, 1.000000000000000000, 0.9659258262890683122, 1.000000000000000000, 0.9659258262890683122, 1.000000000000000000, 0.9659258262890683122, 1.000000000000000000, 0.9659258262890683122, 1.000000000000000000, 0.9659258262890683122, 1.000000000000000000, 0.9659258262890683122, 1.000000000000000000, 0.9659258262890683122, 1.000000000000000000, 0.9659258262890683122, 1.000000000000000000, 0.9659258262890683122, 1.000000000000000000, 0.9659258262890683122, 1.000000000000000000, 0.9659258262890683122, 1.000000000000000000, 0.9659258262890683122, 1.000000000000000000, 0.9659258262890683122, 1.000000000000000000, 0.9659258262890683122, 1.000000000000000000, 0.9659258262890683122, 1.000000000000000000, 0.9659258262890683122, 1.000000000000000000, 0.9659258262890683122, 1.000000000000000000, 0.9659258262890683122, 1.000000000000000000, 0.9659258262890683122, 1.000000000000000000, 0.9659258262890683122, 1.000000000000000000, 0.9659258262890683122, 1.000000000000000000, 0.9659258262890683122, 1.000000000000000000, 0.9659258262890683122, 1.000000000000000000, 0.9659258262890683122, 1.000000000000000000, 0.9659258262890683122, 1.000000000000000000, 0.9659258262890683122, 1.000000000000000000, 0.9659258262890683122, 1.000000000000000000, 0.9659258262890683122, 1.000000000000000000, 0.9659258262890683122, 1.000000000000000000, 0.9659258262890683122, 1.000000000000000000, 0.9659258262890683122, 1.000000000000000000, 0.9659258262890683122, 1.000000000000000000, 0.9659258262890683122, 1.000000000000000000, 0.9659258262890683122, 1.000000000000000000, 0.9659258262890683122, 1.000000000000000000, 0.9659258262890683122, 1.000000000000000000, 0.9659258262890683122, 1.000000000000000000, 0.9659258262890683122, 1.000000000000000000, 0.9659258262890683122, 1.000000000000000000, 0.9659258262890683122, 1.000000000000000000, 0.9659258262890683122, 1.000000000000000000, 0.9659258262890683122, 1.000000000000000000, 0.9659258262890683122, 1.000000000000000000, 0.9659258262890683122, 1.000000000000000000, 0.9659258262890683122, 1.000000000000000000, 0.9659258262890683122, 1.000000000000000000, 0.9659258262890683122, 1.000000000000000000, 0.9659258262890683122, 1.000000000000000000, 0.9659258262890683122, 1.000000000000000000, 0.9659258262890683122, 1.000000000000000000, 0.9659258262890683122, 1.000000000000000000, 0.9659258262890683122, 1.000000000000000000, 0.9659258262890683122, 1.000000000000000000, 0.9659258262890683122, 1.000000000000000000, 0.9659258262890683122, 1.000000000000000000, 0.9659258262890683122, 1.000000000000000000, 0.9659258262890683122, 1.000000000000000000, 0.9659258262890683122, 1.000000000000000000, 0.9659258262890683122, 1.000000000000000000, 0.9659258262890683122, 1.000000000000000000, 0.9659258262890683122, 1.000000000000000000, 0.9659258262890683122, 1.000000000000000000, 0.9659258262890683122, 1.000000000000000000, 0.9659258262890683122, 1.000000000000000000, 0.9659258262890683122, 1.000000000000000000, 0.9659258262890683122, 1.000000000000000000, 0.9659258262890683122, 1.000000000000000000, 0.9659258262890683122, 1.000000000000000000, 0.9659258262890683122, 1.000000000000000000, 0.9659258262890683122, 1.000000000000000000, 0.9659258262890683122, 1.000000000000000000, 0.9659258262890683122, 1.000000000000000000, 0.9659258262890683122, 1.000000000000000000, 0.9659258262890683122, 1.000000000000000000, 0.9659258262890683122, 1.000000000000000000, 0.9659258262890683122, 1.000000000000000000, 0.9659258262890683122, 1.000000000000000000, 0.9659258262890683122, 1.000000000000000000, 0.9659258262890683122, 1.000000000000000000, 0.9659258262890683122, 1.000000000000000000, 0.9659258262890683122, 1.000000000000000000, 0.9659258262890683122, 1.000000000000000000, 0.9659258262890683122, 1.000000000000000000, 0.9659258262890683122, 1.000000000000000000, 0.9659258262890683122, 1.000000000000000000, 0.9659258262890683122, 1.000000000000000000, 0.9659258262890683122, 1.000000000000000000, 0.9659258262890683122, 1.000000000000000000, 0.9659258262890683122, 1.000000000000000000, 0.9659258262890683122, 1.000000000000000000, 0.9659258262890683122, 1.000000000000000000),
 ( 1.000000000000000000, 0.9659258262890683122, 1.000000000000000000, 0.9659258262890683122, 1.000000000000000000, 0.9659258262890683122, 1.000000000000000000, 0.9659258262890683122, 1.000000000000000000, 0.9659258262890683122, 1.000000000000000000, 0.9659258262890683122, 1.000000000000000000, 0.9659258262890683122, 1.000000000000000000, 0.9659258262890683122, 1.000000000000000000, 0.9659258262890683122, 1.000000000000000000, 0.9659258262890683122, 1.000000000000000000, 0.9659258262890683122, 1.000000000000000000, 0.9659258262890683122, 1.000000000000000000, 0.9659258262890683122, 1.000000000000000000, 0.9659258262890683122, 1.000000000000000000, 0.9659258262890683122, 1.000000000000000000, 0.9659258262890683122, 1.000000000000000000, 0.9659258262890683122, 1.000000000000000000, 0.9659258262890683122, 1.000000000000000000, 0.9659258262890683122, 1.000000000000000000, 0.9659258262890683122, 1.000000000000000000, 0.9659258262890683122, 1.000000000000000000, 0.9659258262890683122, 1.000000000000000000, 0.9659258262890683122, 1.000000000000000000, 0.9659258262890683122, 1.000000000000000000, 0.9659258262890683122, 1.000000000000000000, 0.9659258262890683122, 1.000000000000000000, 0.9659258262890683122, 1.000000000000000000, 0.9659258262890683122, 1.000000000000000000, 0.9659258262890683122, 1.000000000000000000, 0.9659258262890683122, 1.000000000000000000, 0.9659258262890683122, 1.000000000000000000, 0.9659258262890683122, 1.000000000000000000, 0.9659258262890683122, 1.000000000000000000, 0.9659258262890683122, 1.000000000000000000, 0.9659258262890683122, 1.000000000000000000, 0.9659258262890683122, 1.000000000000000000, 0.9659258262890683122, 1.000000000000000000, 0.9659258262890683122, 1.000000000000000000, 0.9659258262890683122, 1.000000000000000000, 0.9659258262890683122, 1.000000000000000000, 0.9659258262890683122, 1.000000000000000000, 0.9659258262890683122, 1.000000000000000000, 0.9659258262890683122, 1.000000000000000000, 0.9659258262890683122, 1.000000000000000000, 0.9659258262890683122, 1.000000000000000000, 0.9659258262890683122, 1.000000000000000000, 0.9659258262890683122, 1.000000000000000000, 0.9659258262890683122, 1.000000000000000000, 0.9659258262890683122, 1.000000000000000000, 0.9659258262890683122, 1.000000000000000000, 0.9659258262890683122, 1.000000000000000000, 0.9659258262890683122, 1.000000000000000000, 0.9659258262890683122, 1.000000000000000000, 0.9659258262890683122, 1.000000000000000000, 0.9659258262890683122, 1.000000000000000000, 0.9659258262890683122, 1.000000000000000000, 0.9659258262890683122, 1.000000000000000000, 0.9659258262890683122, 1.000000000000000000, 0.9659258262890683122, 1.000000000000000000, 0.9659258262890683122, 1.000000000000000000, 0.9659258262890683122, 1.000000000000000000, 0.9659258262890683122, 1.000000000000000000, 0.9659258262890683122, 1.000000000000000000, 0.9659258262890683122, 1.000000000000000000, 0.9659258262890683122, 1.000000000000000000, 0.9659258262890683122, 1.000000000000000000, 0.9659258262890683122, 1.000000000000000000, 0.9659258262890683122, 1.000000000000000000, 0.9659258262890683122, 1.000000000000000000, 0.9659258262890683122, 1.000000000000000000, 0.9659258262890683122, 1.000000000000000000, 0.9659258262890683122, 1.000000000000000000, 0.9659258262890683122, 1.000000000000000000, 0.9659258262890683122, 1.000000000000000000, 0.9659258262890683122, 1.000000000000000000, 0.9659258262890683122, 1.000000000000000000, 0.9659258262890683122, 1.000000000000000000, 0.9659258262890683122, 1.000000000000000000, 0.9659258262890683122, 1.000000000000000000, 0.9659258262890683122, 1.000000000000000000, 0.9659258262890683122, 1.000000000000000000, 0.9659258262890683122, 1.000000000000000000, 0.9659258262890683122, 1.000000000000000000, 0.9659258262890683122, 1.000000000000000000, 0.9659258262890683122, 1.000000000000000000, 0.9659258262890683122, 1.000000000000000000, 0.9659258262890683122, 1.000000000000000000, 0.9659258262890683122, 1.000000000000000000, 0.9659258262890683122, 1.000000000000000000, 0.9659258262890683122, 1.000000000000000000, 0.9659258262890683122, 1.000000000000000000, 0.9659258262890683122, 1.000000000000000000, 0.9659258262890683122, 1.000000000000000000, 0.9659258262890683122, 1.000000000000000000, 0.9659258262890683122, 1.000000000000000000, 0.9659258262890683122, 1.000000000000000000, 0.9659258262890683122, 1.000000000000000000, 0.9659258262890683122, 1.000000000000000000, 0.9659258262890683122, 1.000000000000000000, 0.9659258262890683122, 1.000000000000000000, 0.9659258262890683122, 1.000000000000000000, 0.9659258262890683122, 1.000000000000000000, 0.9659258262890683122, 1.000000000000000000, 0.9659258262890683122, 1.000000000000000000, 0.9659258262890683122, 1.000000000000000000, 0.9659258262890683122, 1.000000000000000000, 0.9659258262890683122, 1.000000000000000000, 0.9659258262890683122, 1.000000000000000000, 0.9659258262890683122, 1.000000000000000000, 0.9659258262890683122, 1.000000000000000000, 0.9659258262890683122, 1.000000000000000000, 0.9659258262890683122, 1.000000000000000000, 0.9659258262890683122, 1.000000000000000000, 0.9659258262890683122, 1.000000000000000000, 0.9659258262890683122, 1.000000000000000000, 0.9659258262890683122, 1.000000000000000000, 0.9659258262890683122, 1.000000000000000000, 0.9659258262890683122, 1.000000000000000000, 0.9659258262890683122, 1.000000000000000000, 0.9659258262890683122, 1.000000000000000000, 0.9659258262890683122, 1.000000000000000000, 0.9659258262890683122, 1.000000000000000000, 0.9659258262890683122, 1.000000000000000000, 0.9659258262890683122, 1.000000000000000000, 0.9659258262890683122, 1.000000000000000000, 0.9659258262890683122, 1.000000000000000000, 0.9659258262890683122, 1.000000000000000000, 0.9659258262890683122, 1.000000000000000000, 0.9659258262890683122, 1.000000000000000000, 0.9659258262890683122, 1.000000000000000000, 0.9659258262890683122, 1.000000000000000000, 0.9659258262890683122, 1.000000000000000000, 0.9659258262890683122, 1.000000000000000000, 0.9659258262890683122, 1.000000000000000000, 0.9659258262890683122, 1.000000000000000000, 0.9659258262890683122, 1.000000000000000000, 0.9659258262890683122, 1.000000000000000000, 0.9659258262890683122, 1.000000000000000000, 0.9659258262890683122, 1.000000000000000000, 0.9659258262890683122, 1.000000000000000000, 0.9659258262890683122, 1.000000000000000000, 0.9659258262890683122, 1.000000000000000000, 0.9659258262890683122, 1.000000000000000000, 0.9659258262890683122, 1.000000000000000000, 0.9659258262890683122, 1.000000000000000000, 0.9659258262890683122, 1.000000000000000000, 0.9659258262890683122, 1.000000000000000000, 0.9659258262890683122, 1.000000000000000000, 0.9659258262890683122, 1.000000000000000000, 0.9659258262890683122, 1.000000000000000000, 0.9659258262890683122, 1.000000000000000000, 0.9659258262890683122, 1.000000000000000000, 0.9659258262890683122, 1.000000000000000000, 0.9659258262890683122, 1.000000000000000000, 0.9659258262890683122, 1.000000000000000000, 0.9659258262890683122, 1.000000000000000000, 0.9659258262890683122, 1.000000000000000000, 0.9659258262890683122, 1.000000000000000000, 0.9659258262890683122, 1.000000000000000000, 0.9659258262890683122, 1.000000000000000000, 0.9659258262890683122, 1.000000000000000000, 0.9659258262890683122, 1.000000000000000000, 0.9659258262890683122, 1.000000000000000000, 0.9659258262890683122, 1.000000000000000000, 0.9659258262890683122, 1.000000000000000000, 0.9659258262890683122, 1.000000000000000000, 0.9659258262890683122, 1.000000000000000000, 0.9659258262890683122, 1.000000000000000000, 0.9659258262890683122, 1.000000000000000000, 0.9659258262890683122, 1.000000000000000000, 0.9659258262890683122, 1.000000000000000000, 0.9659258262890683122, 1.000000000000000000, 0.9659258262890683122, 1.000000000000000000, 0.9659258262890683122, 1.000000000000000000, 0.9659258262890683122, 1.000000000000000000, 0.9659258262890683122, 1.000000000000000000, 0.9659258262890683122, 1.000000000000000000, 0.9659258262890683122, 1.000000000000000000, 0.9659258262890683122, 1.000000000000000000, 0.9659258262890683122, 1.000000000000000000, 0.9659258262890683122, 1.000000000000000000, 0.9659258262890683122, 1.000000000000000000, 0.9659258262890683122, 1.000000000000000000, 0.9659258262890683122, 1.000000000000000000, 0.9659258262890683122, 1.000000000000000000, 0.9659258262890683122, 1.000000000000000000, 0.9659258262890683122, 1.000000000000000000, 0.9659258262890683122, 1.000000000000000000, 0.9659258262890683122, 1.000000000000000000, 0.9659258262890683122, 1.000000000000000000, 0.9659258262890683122, 1.000000000000000000, 0.9659258262890683122, 1.000000000000000000, 0.9659258262890683122, 1.000000000000000000, 0.9659258262890683122, 1.000000000000000000, 0.9659258262890683122, 1.000000000000000000, 0.9659258262890683122, 1.000000000000000000, 0.9659258262890683122, 1.000000000000000000, 0.9659258262890683122, 1.000000000000000000, 0.9659258262890683122, 1.000000000000000000, 0.9659258262890683122, 1.000000000000000000, 0.9659258262890683122, 1.000000000000000000, 0.9659258262890683122, 1.000000000000000000, 0.9659258262890683122, 1.000000000000000000, 0.9659258262890683122, 1.000000000000000000, 0.9659258262890683122, 1.000000000000000000, 0.9659258262890683122, 1.000000000000000000, 0.9659258262890683122, 1.000000000000000000, 0.9659258262890683122, 1.000000000000000000, 0.9659258262890683122, 1.000000000000000000, 0.9659258262890683122, 1.000000000000000000, 0.9659258262890683122, 1.000000000000000000, 0.9659258262890683122, 1.000000000000000000, 0.9659258262890683122, 1.000000000000000000, 0.9659258262890683122, 1.000000000000000000, 0.9659258262890683122, 1.000000000000000000, 0.9659258262890683122, 1.000000000000000000, 0.9659258262890683122, 1.000000000000000000, 0.9659258262890683122, 1.000000000000000000, 0.9659258262890683122, 1.000000000000000000, 0.9659258262890683122, 1.000000000000000000, 0.9659258262890683122, 1.000000000000000000, 0.9659258262890683122, 1.000000000000000000, 0.9659258262890683122, 1.000000000000000000, 0.9659258262890683122, 1.000000000000000000, 0.9659258262890683122, 1.000000000000000000, 0.9659258262890683122, 1.000000000000000000, 0.9659258262890683122, 1.000000000000000000, 0.9659258262890683122, 1.000000000000000000, 0.9659258262890683122, 1.000000000000000000, 0.9659258262890683122, 1.000000000000000000, 0.9659258262890683122, 1.000000000000000000, 0.9659258262890683122, 1.000000000000000000, 0.9659258262890683122, 1.000000000000000000, 0.9659258262890683122, 1.000000000000000000, 0.9659258262890683122, 1.000000000000000000, 0.9659258262890683122, 1.000000000000000000, 0.9659258262890683122, 1.000000000000000000, 0.9659258262890683122, 1.000000000000000000, 0.9659258262890683122, 1.000000000000000000, 0.9659258262890683122, 1.000000000000000000, 0.9659258262890683122, 1.000000000000000000, 0.9659258262890683122, 1.000000000000000000, 0.9659258262890683122, 1.000000000000000000, 0.9659258262890683122, 1.000000000000000000, 0.9659258262890683122, 1.000000000000000000, 0.9659258262890683122, 1.000000000000000000, 0.9659258262890683122, 1.000000000000000000, 0.9659258262890683122, 1.000000000000000000, 0.9659258262890683122, 1.000000000000000000, 0.9659258262890683122, 1.000000000000000000, 0.9659258262890683122, 1.000000000000000000, 0.9659258262890683122, 1.000000000000000000, 0.9659258262890683122, 1.000000000000000000, 0.9659258262890683122, 1.000000000000000000, 0.9659258262890683122, 1.000000000000000000) ) ) 
 REPRESENTATION_ITEM ( '' )  SURFACE ( )  );
#65341=CARTESIAN_POINT ( 'NONE',  ( -0.01968503937007793844, 0.1660481256975883668, -0.3530559997133364547 ) ) ;
#65342=CARTESIAN_POINT ( 'NONE',  ( -0.2493438320209966919, -0.004921259842519870586, -0.3153832671262229437 ) ) ;
#65343=CARTESIAN_POINT ( 'NONE',  ( 1.010498687664042716, -0.3690944881889763329, 0.3153832671262228327 ) ) ;
#65344=CARTESIAN_POINT ( 'NONE',  ( -1.603475055217291612, 0.7793870273546337213, -0.04573490813648262154 ) ) ;
#65346=CARTESIAN_POINT ( 'NONE',  ( 1.692913385826772421, 0.1771653543307087630, 0.000000000000000000 ) ) ;
#65347=CARTESIAN_POINT ( 'NONE',  ( 1.036745406824147508, -0.4281496062992127816, -0.4176697321401328100 ) ) ;
#65349=CARTESIAN_POINT ( 'NONE',  ( 0.01312335958005323398, 0.05413385826771666132, 0.4176697321401328100 ) ) ;
#65351=CARTESIAN_POINT ( 'NONE',  ( -1.404199475065615932, 0.05413385826771666132, 0.4176697321401328100 ) ) ;
#65352=CARTESIAN_POINT ( 'NONE',  ( -0.1181102362204717315, 0.2952755905511811885, 0.000000000000000000 ) ) ;
#65354=CARTESIAN_POINT ( 'NONE',  ( 1.627296587926509996, -0.6046776061558807314, 0.2411417322834647770 ) ) ;
#65355=CARTESIAN_POINT ( 'NONE',  ( 0.5446194225721792126, -0.05778040916215560624, -0.4822834645669293319 ) ) ;
#65356=CARTESIAN_POINT ( 'NONE',  ( 1.154855643044620184, -0.5023911411419708095, 0.1820866141732285504 ) ) ;
#65358=CARTESIAN_POINT ( 'NONE',  ( 0.2230971128608932319, -0.3690944881889763329, 0.3153832671262228327 ) ) ;
#65359=CARTESIAN_POINT ( 'NONE',  ( -1.351706036745406347, -0.4281496062992124485, 0.4176697321401328655 ) ) ;
#65361=CARTESIAN_POINT ( 'NONE',  ( 0.9908136482939640111, -0.6692913385826771977, 0.1292274648535927661 ) ) ;
#65362=CONICAL_SURFACE ( 'NONE', #46517, 1.220472440944883497, 0.7853981633974691512 ) ;
#65366=CARTESIAN_POINT ( 'NONE',  ( 0.7152230971128616943, -0.05778040916215522460, 0.4822834645669289988 ) ) ;
#65369=CARTESIAN_POINT ( 'NONE',  ( 0.4199475065616803948, -0.5023911411419708095, -0.1820866141732282451 ) ) ;
#65370=CARTESIAN_POINT ( 'NONE',  ( 0.7217847769028878924, 0.05413385826771666132, 0.4176697321401328100 ) ) ;
#65372=CARTESIAN_POINT ( 'NONE',  ( -1.141732283464566011, -0.5511811023622047445, 6.969142054262312111E-17 ) ) ;
#65373=CARTESIAN_POINT ( 'NONE',  ( -1.122047244094487306, -0.5400638737290844871, 0.3530559997133364547 ) ) ;
#65374=CARTESIAN_POINT ( 'NONE',  ( -1.358267716535432434, 0.1660481256975883668, -0.3530559997133364547 ) ) ;
#65375=CARTESIAN_POINT ( 'NONE',  ( 0.9776902887139113929, -0.6692913385826773087, -0.1292274648535924053 ) ) ;
#65376=CARTESIAN_POINT ( 'NONE',  ( 1.476377952755906442, -0.5400638737290844871, 0.3530559997133364547 ) ) ;
#65378=CARTESIAN_POINT ( 'NONE',  ( 0.5380577427821529035, 0.05413385826771626580, -0.4176697321401330321 ) ) ;
#65381=CARTESIAN_POINT ( 'NONE',  ( 1.410761154855643795, -0.05778040916215560624, -0.4822834645669293319 ) ) ;
#65382=CARTESIAN_POINT ( 'NONE',  ( -1.371391076115484831, 0.1771653543307087075, -0.09757992244046823083 ) ) ;
#65383=CARTESIAN_POINT ( 'NONE',  ( 1.423884514435696413, -0.2845877964562161244, -0.3641732283464567121 ) ) ;
#65384=CARTESIAN_POINT ( 'NONE',  ( -1.220472440944881054, -0.5511811023622047445, 6.969142054262312111E-17 ) ) ;
#65385=CARTESIAN_POINT ( 'NONE',  ( -0.3215223097112853146, -0.08942795157528024563, -0.3641732283464568787 ) ) ;
#65387=CARTESIAN_POINT ( 'NONE',  ( 0.9448818897637802916, -0.1870078740157479769, 0.3641732283464567677 ) ) ;
#65388=CARTESIAN_POINT ( 'NONE',  ( 0.5314960629921267055, -0.5400638737290844871, 0.3530559997133364547 ) ) ;
#65389=CARTESIAN_POINT ( 'NONE',  ( 1.148293963254593653, 0.2952755905511810774, -0.1292274648535930714 ) ) ;
#65390=CARTESIAN_POINT ( 'NONE',  ( 0.1509186351706045259, -0.05778040916215560624, -0.4822834645669293319 ) ) ;
#65391=CARTESIAN_POINT ( 'NONE',  ( 0.4986876640419954376, 0.1283753931104748280, 0.1820866141732283561 ) ) ;
#65392=B_SPLINE_CURVE_WITH_KNOTS ( 'NONE', 3,
 ( #58257, #12010, #5677, #34270, #73409, #46464, #14093 ),
 .UNSPECIFIED., .F., .F.,
 ( 4, 3, 4 ),
 ( 1.561251128379126385E-17, 0.001246230184515555693, 0.002492489877932649398 ),
 .UNSPECIFIED. ) ;
#65393=CARTESIAN_POINT ( 'NONE',  ( 1.069553805774278610, -0.6692913385826771977, 0.1292274648535927661 ) ) ;
#65394=CARTESIAN_POINT ( 'NONE',  ( -1.535433070866141225, -0.6692913385826771977, 8.415575281601705876E-17 ) ) ;
#65395=CARTESIAN_POINT ( 'NONE',  ( -0.6758530183727028406, -0.6692913385826773087, -0.1292274648535924053 ) ) ;
#65397=CARTESIAN_POINT ( 'NONE',  ( 0.05905511811023680946, 0.1012011053420775880, -0.2882089793578257453 ) ) ;
#65398=CARTESIAN_POINT ( 'NONE',  ( 0.1246719160104994284, -0.6692913385826771977, 0.1292274648535927661 ) ) ;
#65399=CARTESIAN_POINT ( 'NONE',  ( -0.1902887139107604098, 0.2952755905511810774, -0.1292274648535930714 ) ) ;
#65400=CARTESIAN_POINT ( 'NONE',  ( 0.1246719160104994284, -0.6692913385826771977, 0.1292274648535927661 ) ) ;
#65405=CARTESIAN_POINT ( 'NONE',  ( -0.9908136482939626788, -0.5511811023622048555, -0.09757992244046775898 ) ) ;
#65407=CARTESIAN_POINT ( 'NONE',  ( -1.108923884514435132, -0.3162353388693405765, 0.4822834645669290543 ) ) ;
#65409=CARTESIAN_POINT ( 'NONE',  ( 0.4002624671916016896, -0.05778040916215522460, 0.4822834645669289988 ) ) ;
#65410=CARTESIAN_POINT ( 'NONE',  ( -0.6364829396325453192, -0.2845877964562159024, 0.3641732283464567677 ) ) ;
#65411=CARTESIAN_POINT ( 'NONE',  ( 1.404199475065617264, -0.4281496062992124485, 0.4176697321401328655 ) ) ;
#65412=EDGE_CURVE ( 'NONE', #82979, #44891, #82854, .T. ) ;
#65413=CARTESIAN_POINT ( 'NONE',  ( 0.3674540682414705883, 0.2306618581243847221, -0.2411417322834647770 ) ) ;
#65418=CARTESIAN_POINT ( 'NONE',  ( 1.259842519685040019, -0.1870078740157480879, -0.4822834645669291653 ) ) ;
#65421=CARTESIAN_POINT ( 'NONE',  ( 0.2821522309711292364, -0.6692913385826771977, 0.1292274648535927661 ) ) ;
#65422=CARTESIAN_POINT ( 'NONE',  ( 0.3740157480314966754, 0.1660481256975883668, -0.3530559997133364547 ) ) ;
#65423=CARTESIAN_POINT ( 'NONE',  ( 1.522309711286089939, -0.6046776061558809534, -0.2411417322834644161 ) ) ;
#65424=CARTESIAN_POINT ( 'NONE',  ( 0.8136482939632553313, -0.6046776061558809534, -0.2411417322834644161 ) ) ;
#65427=CARTESIAN_POINT ( 'NONE',  ( -0.1377952755905504645, 0.1660481256975885056, 0.3530559997133364547 ) ) ;
#65428=CARTESIAN_POINT ( 'NONE',  ( 1.030183727034121421, -0.05778040916215522460, 0.4822834645669289988 ) ) ;
#65429=CARTESIAN_POINT ( 'NONE',  ( 0.5971128608923891301, 0.2952755905511810774, -0.1292274648535930714 ) ) ;
#65430=CARTESIAN_POINT ( 'NONE',  ( 1.076115485564305141, 0.1283753931104746893, -0.1820866141732285504 ) ) ;
#65431=CARTESIAN_POINT ( 'NONE',  ( -0.7480314960629914633, 0.2952755905511811885, 0.000000000000000000 ) ) ;
#65432=CARTESIAN_POINT ( 'NONE',  ( -1.358267716535432434, 0.1660481256975883668, -0.3530559997133364547 ) ) ;
#65433=CARTESIAN_POINT ( 'NONE',  ( 0.9055118110236227702, -0.6692913385826771977, 8.415575281601705876E-17 ) ) ;
#65439=CARTESIAN_POINT ( 'NONE',  ( 1.338582677165355062, -0.1870078740157479769, 0.4822834645669291653 ) ) ;
#65440=CARTESIAN_POINT ( 'NONE',  ( 0.7874015748031503170, -0.1870078740157479769, 0.3641732283464567677 ) ) ;
#65441=CARTESIAN_POINT ( 'NONE',  ( 0.5971128608923891301, 0.2952755905511810219, -0.1292274648535930437 ) ) ;
#65442=CARTESIAN_POINT ( 'NONE',  ( -0.08874907683609993547, 8.471767977567108961E-16, -0.4445507791589058955 ) ) ;
#65445=CARTESIAN_POINT ( 'NONE',  ( 1.122047244094488860, 0.1660481256975885056, 0.3530559997133364547 ) ) ;
#65447=CARTESIAN_POINT ( 'NONE',  ( -0.4396325459317579898, 0.2952755905511811885, 0.1292274648535926551 ) ) ;
#65448=CARTESIAN_POINT ( 'NONE',  ( 1.272965879265092637, 0.05413385826771666132, 0.4176697321401328100 ) ) ;
#65449=ORIENTED_EDGE ( 'NONE', *, *, #19008, .T. ) ;
#65451=CARTESIAN_POINT ( 'NONE',  ( -1.673228346456691717, 0.1660481256975883668, -0.3530559997133364547 ) ) ;
#65454=CARTESIAN_POINT ( 'NONE',  ( 1.614173228346456712, 1.496062992125984037, -0.1372047244094476703 ) ) ;
#65455=CARTESIAN_POINT ( 'NONE',  ( -0.9645669291338575535, 0.07958543189024071263, -0.2665933059059888421 ) ) ;
#65456=CARTESIAN_POINT ( 'NONE',  ( 0.9120734908136490793, 0.2066929133858267098, -0.1054918080437494132 ) ) ;
#65457=CARTESIAN_POINT ( 'NONE',  ( 0.6889763779527566800, -0.5400638737290844871, 0.3530559997133364547 ) ) ;
#65459=CARTESIAN_POINT ( 'NONE',  ( -1.614173228346456712, 2.401574803149606474, 0.1372047244094477536 ) ) ;
#65461=CARTESIAN_POINT ( 'NONE',  ( 0.8792650918635177559, 0.05413385826771666132, 0.4176697321401328100 ) ) ;
#65462=CARTESIAN_POINT ( 'NONE',  ( -1.509186351706035767, 0.05413385826771626580, -0.4176697321401330321 ) ) ;
#65464=CARTESIAN_POINT ( 'NONE',  ( -0.8923884514435688198, 0.1283753931104746893, -0.1820866141732285504 ) ) ;
#65465=CARTESIAN_POINT ( 'NONE',  ( 1.686351706036745890, 0.2952755905511811885, 0.1292274648535926551 ) ) ;
#65467=CARTESIAN_POINT ( 'NONE',  ( 0.2755905511811031494, -0.6692913385826771977, 8.415575281601705876E-17 ) ) ;
#65468=CARTESIAN_POINT ( 'NONE',  ( -0.9711286089238838626, 0.1283753931104746893, -0.1820866141732285504 ) ) ;
#65469=CARTESIAN_POINT ( 'NONE',  ( 0.1902887139107617975, 0.1771653543307087630, 0.09757992244046791164 ) ) ;
#65470=CARTESIAN_POINT ( 'NONE',  ( -0.4527559055118102749, 0.1660481256975885056, 0.3530559997133364547 ) ) ;
#65471=CARTESIAN_POINT ( 'NONE',  ( -1.299212598425196097, 0.1771653543307087630, 0.000000000000000000 ) ) ;
#65473=CARTESIAN_POINT ( 'NONE',  ( 0.8005249343832027131, 0.05413385826771666132, 0.4176697321401328100 ) ) ;
#65475=CARTESIAN_POINT ( 'NONE',  ( -1.338582677165353729, -0.1870078740157479769, 0.4822834645669291653 ) ) ;
#65478=CARTESIAN_POINT ( 'NONE',  ( -0.6692913385826764205, -0.6692913385826771977, 8.415575281601705876E-17 ) ) ;
#65479=CARTESIAN_POINT ( 'NONE',  ( -0.2952755905511804668, 0.07958543189024085140, 0.2665933059059887866 ) ) ;
#65480=CARTESIAN_POINT ( 'NONE',  ( -1.227034120734907141, -0.6692913385826773087, -0.1292274648535924053 ) ) ;
#65481=CARTESIAN_POINT ( 'NONE',  ( 0.8989501312335964611, 0.1771653543307087630, 0.09757992244046791164 ) ) ;
#65482=CARTESIAN_POINT ( 'NONE',  ( -0.4265091863517051496, 0.1771653543307087075, -0.09757992244046823083 ) ) ;
#65483=CARTESIAN_POINT ( 'NONE',  ( -1.187664041994750175, -0.05778040916215560624, -0.4822834645669293319 ) ) ;
#65484=CARTESIAN_POINT ( 'NONE',  ( -0.9711286089238838626, -0.6046776061558807314, 0.2411417322834647770 ) ) ;
#65485=CARTESIAN_POINT ( 'NONE',  ( 1.686351706036745890, 0.2952755905511811885, 0.1292274648535926551 ) ) ;
#65486=CARTESIAN_POINT ( 'NONE',  ( 1.036041590146032698, 3.421639014772782816E-16, 0.3464511005275203726 ) ) ;
#65487=CARTESIAN_POINT ( 'NONE',  ( 0.9120734908136490793, 0.1771653543307087075, -0.09757992244046823083 ) ) ;
#65488=CARTESIAN_POINT ( 'NONE',  ( 0.2099737532808405305, -0.6046776061558807314, 0.2411417322834647770 ) ) ;
#65489=CARTESIAN_POINT ( 'NONE',  ( -1.305774278215222184, 0.2952755905511811885, 0.1292274648535926551 ) ) ;
#65490=CARTESIAN_POINT ( 'NONE',  ( -1.384514435695537005, 0.2952755905511811885, 0.1292274648535926551 ) ) ;
#65491=VERTEX_POINT ( 'NONE', #28300 ) ;
#65493=CARTESIAN_POINT ( 'NONE',  ( -0.7545931758530176614, -0.5511811023622048555, -0.09757992244046775898 ) ) ;
#65494=CARTESIAN_POINT ( 'NONE',  ( 0.5643044619422579178, -0.4281496062992127816, -0.4176697321401328100 ) ) ;
#65495=CARTESIAN_POINT ( 'NONE',  ( -1.259842519685038686, -0.1870078740157479769, 0.3641732283464567677 ) ) ;
#65497=CARTESIAN_POINT ( 'NONE',  ( -1.574803149606298636, -0.1870078740157479769, 0.4822834645669291653 ) ) ;
#65498=CARTESIAN_POINT ( 'NONE',  ( 1.017060367454068803, -0.3162353388693405765, 0.4822834645669290543 ) ) ;
#65499=CARTESIAN_POINT ( 'NONE',  ( 0.4855643044619430415, -0.4281496062992127816, -0.4176697321401328100 ) ) ;
#65500=CARTESIAN_POINT ( 'NONE',  ( 1.233595800524935227, -0.6046776061558807314, 0.2411417322834647770 ) ) ;
#65504=CARTESIAN_POINT ( 'NONE',  ( 1.112371124080195450, -4.927456884911482678E-16, 0.4445507791589062840 ) ) ;
#65505=CARTESIAN_POINT ( 'NONE',  ( 0.1574803149606306130, -0.1870078740157479769, 0.3641732283464567677 ) ) ;
#65506=CARTESIAN_POINT ( 'NONE',  ( 0.01968503937007930540, 0.1660481256975885056, 0.3530559997133364547 ) ) ;
#65507=CARTESIAN_POINT ( 'NONE',  ( 1.089238845144357537, -0.4281496062992124485, 0.4176697321401328655 ) ) ;
#65509=CARTESIAN_POINT ( 'NONE',  ( 0.3805774278215230400, -0.3690944881889763329, 0.3153832671262228327 ) ) ;
#65510=CARTESIAN_POINT ( 'NONE',  ( -0.5774278215223089816, -0.6046776061558807314, 0.2411417322834647770 ) ) ;
#65511=CARTESIAN_POINT ( 'NONE',  ( -1.555118110236219930, -0.5400638737290845981, -0.3530559997133363437 ) ) ;
#65512=CARTESIAN_POINT ( 'NONE',  ( 0.8727034120734913358, -0.05778040916215522460, 0.4822834645669289988 ) ) ;
#65515=B_SPLINE_CURVE_WITH_KNOTS ( 'NONE', 3,
 ( #45729, #39429, #65545, #72267 ),
 .UNSPECIFIED., .F., .F.,
 ( 4, 4 ),
 ( 3.210432057730626195E-07, 0.001287787053611998828 ),
 .UNSPECIFIED. ) ;
#65516=( BOUNDED_CURVE ( )  B_SPLINE_CURVE ( 1, ( #75432, #56866 ),
 .UNSPECIFIED., .F., .F. ) 
 B_SPLINE_CURVE_WITH_KNOTS ( ( 2, 2 ),
 ( 0.000000000000000000, 0.002000000000000011317 ),
 .UNSPECIFIED. ) 
 CURVE ( )  GEOMETRIC_REPRESENTATION_ITEM ( )  RATIONAL_B_SPLINE_CURVE ( ( 0.9875488213027514561, 0.9875488213027514561 ) ) 
 REPRESENTATION_ITEM ( '' )  );
#65519=CARTESIAN_POINT ( 'NONE',  ( -1.423884514435694859, -0.3162353388693405765, 0.4822834645669290543 ) ) ;
#65520=CARTESIAN_POINT ( 'NONE',  ( -1.115485564304461219, -0.004921259842519870586, -0.3153832671262229437 ) ) ;
#65521=CARTESIAN_POINT ( 'NONE',  ( -1.023622047244093558, -0.1870078740157479769, 0.4822834645669291653 ) ) ;
#65524=CARTESIAN_POINT ( 'NONE',  ( 1.522309711286089939, 0.2306618581243848609, 0.2411417322834645549 ) ) ;
#65525=CARTESIAN_POINT ( 'NONE',  ( -1.095800524934382292, -0.05778040916215522460, 0.4822834645669289988 ) ) ;
#65526=CARTESIAN_POINT ( 'NONE',  ( 0.3477690288713918276, 0.2952755905511811885, 0.1292274648535926551 ) ) ;
#65527=CARTESIAN_POINT ( 'NONE',  ( -1.161417322834644716, 0.1660481256975885056, 0.3530559997133364547 ) ) ;
#65529=CARTESIAN_POINT ( 'NONE',  ( 0.7152230971128614723, -0.3162353388693409650, -0.4822834645669289433 ) ) ;
#65531=CARTESIAN_POINT ( 'NONE',  ( -0.7742782152230962556, -0.3690944881889765550, -0.3153832671262227771 ) ) ;
#65532=EDGE_LOOP ( 'NONE', ( #46063, #7769, #72566, #83015 ) ) ;
#65536=CARTESIAN_POINT ( 'NONE',  ( -1.522309711286088607, 0.1283753931104746893, -0.1820866141732285504 ) ) ;
#65538=CARTESIAN_POINT ( 'NONE',  ( -0.9908136482939626788, -0.6692913385826773087, -0.1292274648535924053 ) ) ;
#65539=CARTESIAN_POINT ( 'NONE',  ( -1.502624671916009680, -0.3162353388693405765, 0.4822834645669290543 ) ) ;
#65541=CARTESIAN_POINT ( 'NONE',  ( -1.522309711286088607, 0.2306618581243847221, -0.2411417322834647770 ) ) ;
#65542=CARTESIAN_POINT ( 'NONE',  ( -1.233595800524933894, 0.2306618581243848609, 0.2411417322834645549 ) ) ;
#65543=CARTESIAN_POINT ( 'NONE',  ( -1.463254593175852492, 0.2952755905511811885, 0.1292274648535926551 ) ) ;
#65544=CARTESIAN_POINT ( 'NONE',  ( -1.614173228346457378, 1.818966223839196372, 0.1372047244094476981 ) ) ;
#65545=CARTESIAN_POINT ( 'NONE',  ( -1.604771003085130321, 0.7270283685441725208, -0.1466069496707743391 ) ) ;
#65546=CARTESIAN_POINT ( 'NONE',  ( 0.2034120734908144990, -0.5511811023622046335, 0.09757992244046803654 ) ) ;
#65547=CARTESIAN_POINT ( 'NONE',  ( 2.795275590551181910, 1.900312960331935086, 0.000000000000000000 ) ) ;
#65549=CARTESIAN_POINT ( 'NONE',  ( -0.5118110236220466680, -0.5511811023622047445, 6.969142054262312111E-17 ) ) ;
#65550=CARTESIAN_POINT ( 'NONE',  ( -0.6233595800524928121, -0.3162353388693409650, -0.4822834645669289433 ) ) ;
#65551=CARTESIAN_POINT ( 'NONE',  ( 0.9251968503937015864, -0.5400638737290844871, 0.3530559997133364547 ) ) ;
#65552=CARTESIAN_POINT ( 'NONE',  ( -0.9973753280839886548, 0.2306618581243848609, 0.2411417322834645549 ) ) ;
#65554=ORIENTED_EDGE ( 'NONE', *, *, #81347, .T. ) ;
#65555=CARTESIAN_POINT ( 'NONE',  ( -0.9317585301837263412, -0.4281496062992127816, -0.4176697321401328100 ) ) ;
#65556=CARTESIAN_POINT ( 'NONE',  ( 0.7677165354330716118, -0.5400638737290844871, 0.3530559997133364547 ) ) ;
#65557=CARTESIAN_POINT ( 'NONE',  ( -1.522309711286088607, 0.1283753931104746893, -0.1820866141732285504 ) ) ;
#65562=CARTESIAN_POINT ( 'NONE',  ( -0.1443569553805765515, -0.4281496062992127816, -0.4176697321401328100 ) ) ;
#65563=CARTESIAN_POINT ( 'NONE',  ( -1.404199475065615932, -0.3690944881889765550, -0.3153832671262227771 ) ) ;
#65564=CARTESIAN_POINT ( 'NONE',  ( -0.7152230971128602510, -0.05778040916215560624, -0.4822834645669293319 ) ) ;
#65566=CARTESIAN_POINT ( 'NONE',  ( -1.463254593175852492, -0.6692913385826773087, -0.1292274648535924053 ) ) ;
#65568=CARTESIAN_POINT ( 'NONE',  ( -1.154855643044618851, -0.6046776061558809534, -0.2411417322834644161 ) ) ;
#65569=CARTESIAN_POINT ( 'NONE',  ( -0.4133858267716528645, 0.1660481256975883668, -0.3530559997133364547 ) ) ;
#65571=CARTESIAN_POINT ( 'NONE',  ( 0.2624671916010504757, -0.5023911411419708095, -0.1820866141732282451 ) ) ;
#65573=CARTESIAN_POINT ( 'NONE',  ( 0.5183727034120741983, -0.5511811023622046335, 0.09757992244046803654 ) ) ;
#65574=CARTESIAN_POINT ( 'NONE',  ( 1.509186351706037543, -0.3690944881889765550, -0.3153832671262227771 ) ) ;
#65575=CARTESIAN_POINT ( 'NONE',  ( 0.9842519685039375910, 0.2952755905511811885, 0.000000000000000000 ) ) ;
#65576=CARTESIAN_POINT ( 'NONE',  ( 0.2887139107611556010, 0.1283753931104746893, -0.1820866141732285504 ) ) ;
#65578=CARTESIAN_POINT ( 'NONE',  ( -1.456692913385826182, 0.2952755905511811885, 0.000000000000000000 ) ) ;
#65579=CARTESIAN_POINT ( 'NONE',  ( -0.1706036745406816491, -0.3690944881889763329, 0.3153832671262228327 ) ) ;
#65581=CARTESIAN_POINT ( 'NONE',  ( -0.5118110236220466680, 0.1771653543307087630, 0.000000000000000000 ) ) ;
#65583=CARTESIAN_POINT ( 'NONE',  ( -0.4624320255261038515, -2.191421614605370878E-15, 0.4445507791589071167 ) ) ;
#65584=CARTESIAN_POINT ( 'NONE',  ( -0.2559055118110227234, -0.5400638737290844871, 0.3530559997133364547 ) ) ;
#65586=CARTESIAN_POINT ( 'NONE',  ( 1.115485564304462551, -0.004921259842519576551, 0.3153832671262227771 ) ) ;
#65587=CARTESIAN_POINT ( 'NONE',  ( 0.2427821522309716595, -0.2845877964562161244, -0.3641732283464567121 ) ) ;
#65588=CARTESIAN_POINT ( 'NONE',  ( -0.3543307086614165824, 0.2952755905511811885, 0.000000000000000000 ) ) ;
#65589=DIRECTION ( 'NONE',  ( 0.000000000000000000, -1.000000000000000000, 0.000000000000000000 ) ) ;
#65590=CARTESIAN_POINT ( 'NONE',  ( -0.8923884514435688198, -0.5023911411419708095, 0.1820866141732285504 ) ) ;
#65591=CARTESIAN_POINT ( 'NONE',  ( -1.646051170424378096, 0.8346805926620876059, 0.5309055118110233007 ) ) ;
#65592=CARTESIAN_POINT ( 'NONE',  ( 0.7152230971128616943, -0.05778040916215522460, 0.4822834645669289988 ) ) ;
#65593=CARTESIAN_POINT ( 'NONE',  ( -0.7480314960629914633, -0.6692913385826771977, 8.415575281601705876E-17 ) ) ;
#65596=CARTESIAN_POINT ( 'NONE',  ( 0.05249343832021075018, 0.1283753931104746893, -0.1820866141732285504 ) ) ;
#65597=CARTESIAN_POINT ( 'NONE',  ( -0.6167979002624665030, -0.4281496062992127816, -0.4176697321401328100 ) ) ;
#65599=CARTESIAN_POINT ( 'NONE',  ( -1.167979002624671470, 0.05413385826771666132, 0.4176697321401328100 ) ) ;
#65600=CARTESIAN_POINT ( 'NONE',  ( -1.371391076115484609, -0.5511811023622046335, 0.09757992244046803654 ) ) ;
#65602=EDGE_CURVE ( 'NONE', #1230, #33111, #8129, .T. ) ;
#65603=CARTESIAN_POINT ( 'NONE',  ( -0.8202099737532799750, 0.1771653543307087075, -0.09757992244046823083 ) ) ;
#65604=DIRECTION ( 'NONE',  ( 0.000000000000000000, 0.000000000000000000, 1.000000000000000000 ) ) ;
#65605=CARTESIAN_POINT ( 'NONE',  ( 0.7545931758530188826, -0.6692913385826771977, 0.1292274648535927661 ) ) ;
#65608=ORIENTED_EDGE ( 'NONE', *, *, #31972, .T. ) ;
#65609=ADVANCED_FACE ( 'NONE', ( #1810 ), #57365, .F. ) ;
#65611=CARTESIAN_POINT ( 'NONE',  ( 1.417322834645670104, -0.1870078740157479769, 0.3641732283464567677 ) ) ;
#65612=CARTESIAN_POINT ( 'NONE',  ( -1.207349081364828880, 0.2306618581243847221, -0.2411417322834647770 ) ) ;
#65613=CARTESIAN_POINT ( 'NONE',  ( 1.246719160104987623, -0.4281496062992124485, 0.4176697321401328655 ) ) ;
#65615=CARTESIAN_POINT ( 'NONE',  ( 1.522309711286089939, 0.1283753931104748280, 0.1820866141732283561 ) ) ;
#65616=CARTESIAN_POINT ( 'NONE',  ( 0.6692913385826778638, -0.6692913385826771977, 8.415575281601705876E-17 ) ) ;
#65617=CARTESIAN_POINT ( 'NONE',  ( -0.2427821522309703550, -0.3162353388693405765, 0.4822834645669290543 ) ) ;
#65620=CARTESIAN_POINT ( 'NONE',  ( 0.6299212598425204535, -0.1870078740157479769, 0.3641732283464567677 ) ) ;
#65625=CARTESIAN_POINT ( 'NONE',  ( -0.08530183727034056085, -0.05778040916215560624, -0.4822834645669293319 ) ) ;
#65626=CARTESIAN_POINT ( 'NONE',  ( 1.299212598425197429, 0.2952755905511811885, 0.000000000000000000 ) ) ;
#65627=CARTESIAN_POINT ( 'NONE',  ( 0.2296587926509192634, -0.3162353388693405765, 0.4822834645669290543 ) ) ;
#65628=CARTESIAN_POINT ( 'NONE',  ( -0.5380577427821514602, -0.004921259842519576551, 0.3153832671262227771 ) ) ;
#65629=CARTESIAN_POINT ( 'NONE',  ( 1.391076115485564868, 0.2306618581243847221, -0.2411417322834647770 ) ) ;
#65630=CARTESIAN_POINT ( 'NONE',  ( -0.3149606299212590610, -0.1870078740157480879, -0.4822834645669291653 ) ) ;
#65631=CARTESIAN_POINT ( 'NONE',  ( -0.01312335958005186876, -0.4281496062992124485, 0.4176697321401328655 ) ) ;
#65632=CARTESIAN_POINT ( 'NONE',  ( -1.515748031496062076, -0.5400638737290844871, 0.3530559997133364547 ) ) ;
#65633=CARTESIAN_POINT ( 'NONE',  ( 1.469816272965879911, 0.2306618581243847221, -0.2411417322834647770 ) ) ;
#65635=CARTESIAN_POINT ( 'NONE',  ( 1.338582677165355062, -0.1870078740157479769, 0.4822834645669291653 ) ) ;
#65637=CARTESIAN_POINT ( 'NONE',  ( 0.4921259842519691285, -0.4536011799217368745, -0.2665933059059886201 ) ) ;
#65641=CARTESIAN_POINT ( 'NONE',  ( -0.2755905511811018171, 0.1771653543307087630, 0.000000000000000000 ) ) ;
#65642=CARTESIAN_POINT ( 'NONE',  ( 0.01312335958005323398, -0.4281496062992127816, -0.4176697321401328100 ) ) ;
#65644=CARTESIAN_POINT ( 'NONE',  ( -0.1377952755905504645, 0.1660481256975885056, 0.3530559997133364547 ) ) ;
#65645=CARTESIAN_POINT ( 'NONE',  ( -0.05905511811023545637, -0.5400638737290845981, -0.3530559997133363437 ) ) ;
#65646=CARTESIAN_POINT ( 'NONE',  ( -0.9908136482939626788, 0.2952755905511811885, 0.1292274648535926551 ) ) ;
#65647=CARTESIAN_POINT ( 'NONE',  ( -0.8464566929133852113, -0.5400638737290845981, -0.3530559997133363437 ) ) ;
#65649=CARTESIAN_POINT ( 'NONE',  ( 1.233595800524935227, 0.1283753931104746893, -0.1820866141732285504 ) ) ;
#65650=CARTESIAN_POINT ( 'NONE',  ( -1.515748031496062076, -0.5400638737290844871, 0.3530559997133364547 ) ) ;
#65652=CARTESIAN_POINT ( 'NONE',  ( 1.102362204724410155, -0.1870078740157479769, 0.3641732283464567677 ) ) ;
#65653=CARTESIAN_POINT ( 'NONE',  ( 0.3805774278215230400, -0.4281496062992124485, 0.4176697321401328655 ) ) ;
#65654=CARTESIAN_POINT ( 'NONE',  ( 0.3740157480314966754, -0.5400638737290844871, 0.3530559997133364547 ) ) ;
#65656=CARTESIAN_POINT ( 'NONE',  ( -1.653543307086613234, -0.1870078740157480879, -0.4822834645669291653 ) ) ;
#65659=CARTESIAN_POINT ( 'NONE',  ( -0.5577427821522301654, -0.05778040916215560624, -0.4822834645669293319 ) ) ;
#65664=CARTESIAN_POINT ( 'NONE',  ( -1.095800524934382292, -0.2845877964562161244, -0.3641732283464567121 ) ) ;
#65665=CARTESIAN_POINT ( 'NONE',  ( 0.9973753280839902091, 0.2306618581243847221, -0.2411417322834647770 ) ) ;
#65666=AXIS2_PLACEMENT_3D ( 'NONE', #44125, #5832, #57165 ) ;
#65667=CARTESIAN_POINT ( 'NONE',  ( 1.049868766404200349, 0.2306618581243848609, 0.2411417322834645549 ) ) ;
#65668=CARTESIAN_POINT ( 'NONE',  ( -0.06561679790026180015, -0.004921259842519576551, 0.3153832671262227771 ) ) ;
#65669=CARTESIAN_POINT ( 'NONE',  ( 0.5249343832021003964, 0.2306618581243847221, -0.2411417322834647770 ) ) ;
#65671=CARTESIAN_POINT ( 'NONE',  ( -0.2690288713910754526, -0.5511811023622046335, 0.09757992244046803654 ) ) ;
#65672=CARTESIAN_POINT ( 'NONE',  ( 0.05905511811023681640, 0.1660481256975883668, -0.3530559997133364547 ) ) ;
#65674=CARTESIAN_POINT ( 'NONE',  ( -1.305774278215222184, -0.6692913385826773087, -0.1292274648535924053 ) ) ;
#65675=CARTESIAN_POINT ( 'NONE',  ( 0.6496062992125991586, 0.07958543189024085140, 0.2665933059059887866 ) ) ;
#65676=CARTESIAN_POINT ( 'NONE',  ( 1.482939632545932307, -0.3690944881889763329, 0.3153832671262228327 ) ) ;
#65677=CARTESIAN_POINT ( 'NONE',  ( -0.8661417322834640276, -0.1870078740157480879, -0.4822834645669291653 ) ) ;
#65678=CARTESIAN_POINT ( 'NONE',  ( -0.2230971128608915943, -0.004921259842519576551, 0.3153832671262227771 ) ) ;
#65680=CARTESIAN_POINT ( 'NONE',  ( -0.7217847769028863381, 0.05413385826771626580, -0.4176697321401330321 ) ) ;
#65681=CARTESIAN_POINT ( 'NONE',  ( -0.5971128608923877978, -0.6692913385826773087, -0.1292274648535924053 ) ) ;
#65682=CARTESIAN_POINT ( 'NONE',  ( -0.1049868766404193215, -0.6046776061558807314, 0.2411417322834647770 ) ) ;
#65685=CARTESIAN_POINT ( 'NONE',  ( -1.574803149606298636, -0.1870078740157479769, 0.3641732283464567677 ) ) ;
#65686=CARTESIAN_POINT ( 'NONE',  ( 0.8595800524934390507, -0.2845877964562159024, 0.3641732283464567677 ) ) ;
#65687=CARTESIAN_POINT ( 'NONE',  ( 1.384514435695538337, -0.6692913385826771977, 0.1292274648535927661 ) ) ;
#65688=CARTESIAN_POINT ( 'NONE',  ( -0.6496062992125976043, -0.4536011799217367080, 0.2665933059059888421 ) ) ;
#65689=CARTESIAN_POINT ( 'NONE',  ( -1.200787401574802349, 0.07958543189024071263, -0.2665933059059888421 ) ) ;
#65690=CARTESIAN_POINT ( 'NONE',  ( -0.6889763779527552368, 0.1660481256975885056, 0.3530559997133364547 ) ) ;
#65691=CARTESIAN_POINT ( 'NONE',  ( -0.4593175853018366950, 0.05413385826771666132, 0.4176697321401328100 ) ) ;
#65692=CARTESIAN_POINT ( 'NONE',  ( 0.5118110236220480003, -0.5511811023622047445, 6.969142054262312111E-17 ) ) ;
#65693=CARTESIAN_POINT ( 'NONE',  ( 1.266404199475066328, -0.08942795157527998196, 0.3641732283464567121 ) ) ;
#65694=CARTESIAN_POINT ( 'NONE',  ( 0.4396325459317593221, 0.2952755905511810774, -0.1292274648535930714 ) ) ;
#65695=CYLINDRICAL_SURFACE ( 'NONE', #19567, 0.3937007874015748254 ) ;
#65696=CARTESIAN_POINT ( 'NONE',  ( -0.4855643044619415427, -0.4281496062992124485, 0.4176697321401328655 ) ) ;
#65698=CARTESIAN_POINT ( 'NONE',  ( 1.568241469816273437, -0.2845877964562159024, 0.3641732283464567677 ) ) ;
#65699=CARTESIAN_POINT ( 'NONE',  ( 0.5971128608923891301, 0.2952755905511810774, -0.1292274648535930714 ) ) ;
#65700=CARTESIAN_POINT ( 'NONE',  ( 0.3215223097112867578, -0.3162353388693409650, -0.4822834645669289433 ) ) ;
#65701=CARTESIAN_POINT ( 'NONE',  ( 0.07874015748031558404, -0.1870078740157479769, 0.3641732283464567677 ) ) ;
#65702=CARTESIAN_POINT ( 'NONE',  ( 1.113459889019126514, -1.206088964116209378E-16, 0.3954974714151466841 ) ) ;
#65703=CARTESIAN_POINT ( 'NONE',  ( 0.01312335958005323398, -0.3690944881889765550, -0.3153832671262227771 ) ) ;
#65704=CARTESIAN_POINT ( 'NONE',  ( 0.7020997375328090762, -0.3162353388693405765, 0.4822834645669290543 ) ) ;
#65705=EDGE_CURVE ( 'NONE', #53888, #30109, #71904, .T. ) ;
#65706=CARTESIAN_POINT ( 'NONE',  ( -0.5708661417322828946, 0.07958543189024071263, -0.2665933059059888421 ) ) ;
#65707=CARTESIAN_POINT ( 'NONE',  ( -0.8989501312335946848, -0.6692913385826771977, 0.1292274648535927661 ) ) ;
#65710=CARTESIAN_POINT ( 'NONE',  ( -1.076115485564303809, -0.6046776061558809534, -0.2411417322834644161 ) ) ;
#65711=CARTESIAN_POINT ( 'NONE',  ( -1.095800524934382292, -0.08942795157527998196, 0.3641732283464567121 ) ) ;
#65712=CARTESIAN_POINT ( 'NONE',  ( -0.1837270341207343505, -0.6046776061558807314, 0.2411417322834647770 ) ) ;
#65713=CARTESIAN_POINT ( 'NONE',  ( -1.666666666666665853, 0.05413385826771626580, -0.4176697321401330321 ) ) ;
#65714=CARTESIAN_POINT ( 'NONE',  ( -0.6496062992125976043, 0.1660481256975883668, -0.3530559997133364547 ) ) ;
#65716=CARTESIAN_POINT ( 'NONE',  ( 1.627296587926509996, -0.6046776061558807314, 0.2411417322834647770 ) ) ;
#65717=CARTESIAN_POINT ( 'NONE',  ( 0.8136482939632553313, 0.2306618581243848609, 0.2411417322834645549 ) ) ;
#65718=CARTESIAN_POINT ( 'NONE',  ( 0.8202099737532814183, -0.6692913385826773087, -0.1292274648535924053 ) ) ;
#65720=CARTESIAN_POINT ( 'NONE',  ( -1.154855643044618851, -0.6046776061558809534, -0.2411417322834644161 ) ) ;
#65722=ORIENTED_EDGE ( 'NONE', *, *, #67683, .T. ) ;
#65723=CARTESIAN_POINT ( 'NONE',  ( -0.5774278215223089816, -0.5023911411419708095, 0.1820866141732285504 ) ) ;
#65726=CARTESIAN_POINT ( 'NONE',  ( 0.2296587926509192634, -0.05778040916215560624, -0.4822834645669293319 ) ) ;
#65727=CARTESIAN_POINT ( 'NONE',  ( -0.1706036745406816491, -0.4281496062992124485, 0.4176697321401328655 ) ) ;
#65728=CARTESIAN_POINT ( 'NONE',  ( -0.6824146981627288167, 0.2306618581243848609, 0.2411417322834645549 ) ) ;
#65729=CARTESIAN_POINT ( 'NONE',  ( 1.535433070866142558, 0.2952755905511811885, 0.000000000000000000 ) ) ;
#65730=CARTESIAN_POINT ( 'NONE',  ( -1.003937007874014853, 0.07958543189024085140, 0.2665933059059887866 ) ) ;
#65732=CARTESIAN_POINT ( 'NONE',  ( 0.6758530183727039509, -0.6692913385826771977, 0.1292274648535927661 ) ) ;
#65733=CARTESIAN_POINT ( 'NONE',  ( 0.6561679790026253567, 0.1283753931104748280, 0.1820866141732283561 ) ) ;
#65734=CARTESIAN_POINT ( 'NONE',  ( -0.4133858267716528645, -0.5400638737290844871, 0.3530559997133364547 ) ) ;
#65736=CARTESIAN_POINT ( 'NONE',  ( -0.8923884514435688198, -0.6046776061558807314, 0.2411417322834647770 ) ) ;
#65737=CARTESIAN_POINT ( 'NONE',  ( -1.568241469816272105, -0.08942795157527998196, 0.3641732283464567121 ) ) ;
#65738=CARTESIAN_POINT ( 'NONE',  ( 1.358267716535433323, 0.1660481256975885056, 0.3530559997133364547 ) ) ;
#65739=CARTESIAN_POINT ( 'NONE',  ( 1.601049868766404982, -0.5023911411419708095, -0.1820866141732282451 ) ) ;
#65742=CARTESIAN_POINT ( 'NONE',  ( 0.09186351706036827158, 0.05413385826771666132, 0.4176697321401328100 ) ) ;
#65744=CARTESIAN_POINT ( 'NONE',  ( -1.056430446194224881, 0.2952755905511810774, -0.1292274648535930714 ) ) ;
#65745=CARTESIAN_POINT ( 'NONE',  ( 1.384514435695538337, -0.6692913385826771977, 0.1292274648535927661 ) ) ;
#65746=CARTESIAN_POINT ( 'NONE',  ( 1.174540682414699111, -0.05778040916215560624, -0.4822834645669293319 ) ) ;
#65747=CARTESIAN_POINT ( 'NONE',  ( 0.3477690288713918276, 0.2952755905511811885, 0.1292274648535926551 ) ) ;
#65748=CARTESIAN_POINT ( 'NONE',  ( -0.4593175853018364174, -0.4281496062992127816, -0.4176697321401328100 ) ) ;
#65750=CARTESIAN_POINT ( 'NONE',  ( -1.227034120734907585, 0.2952755905511811885, 0.1292274648535926551 ) ) ;
#65751=CARTESIAN_POINT ( 'NONE',  ( -0.4002624671916004129, -0.3162353388693405765, 0.4822834645669290543 ) ) ;
#65752=CARTESIAN_POINT ( 'NONE',  ( -0.5971128608923877978, -0.5511811023622048555, -0.09757992244046775898 ) ) ;
#65753=CARTESIAN_POINT ( 'NONE',  ( -2.795275590551185907, 0.4724409448818907564, -3.981376139758521912E-16 ) ) ;
#65754=CARTESIAN_POINT ( 'NONE',  ( -0.4790026246719154557, -0.3162353388693405765, 0.4822834645669290543 ) ) ;
#65756=CARTESIAN_POINT ( 'NONE',  ( 0.5905511811023629321, -0.6692913385826771977, 8.415575281601705876E-17 ) ) ;
#65758=CARTESIAN_POINT ( 'NONE',  ( 0.07217847769028949700, -0.3162353388693405765, 0.4822834645669290543 ) ) ;
#65759=CARTESIAN_POINT ( 'NONE',  ( -0.3018372703412066094, -0.004921259842519576551, 0.3153832671262227771 ) ) ;
#65760=CARTESIAN_POINT ( 'NONE',  ( 1.174540682414699111, -0.2845877964562159024, 0.3641732283464567677 ) ) ;
#65761=CARTESIAN_POINT ( 'NONE',  ( -0.8858267716535425107, 0.1012011053420775880, -0.2882089793578257453 ) ) ;
#65763=CARTESIAN_POINT ( 'NONE',  ( 0.9776902887139113929, -0.5511811023622048555, -0.09757992244046775898 ) ) ;
#65765=CARTESIAN_POINT ( 'NONE',  ( 1.312335958005249825, 0.2306618581243847221, -0.2411417322834647770 ) ) ;
#65767=CARTESIAN_POINT ( 'NONE',  ( 0.06561679790026316017, 0.05413385826771626580, -0.4176697321401330321 ) ) ;
#65769=CARTESIAN_POINT ( 'NONE',  ( 1.568241469816273437, -0.2845877964562159024, 0.3641732283464567677 ) ) ;
#65770=CARTESIAN_POINT ( 'NONE',  ( -0.3477690288713905509, -0.6692913385826771977, 0.1292274648535927661 ) ) ;
#65772=CARTESIAN_POINT ( 'NONE',  ( -1.522309711286088607, -0.5023911411419708095, 0.1820866141732285504 ) ) ;
#65773=CARTESIAN_POINT ( 'NONE',  ( 0.6496062992125991586, 0.1660481256975885056, 0.3530559997133364547 ) ) ;
#65774=CARTESIAN_POINT ( 'NONE',  ( 0.9580052493438327987, -0.3690944881889765550, -0.3153832671262227771 ) ) ;
#65775=CARTESIAN_POINT ( 'NONE',  ( 0.8070866141732288002, 0.1012011053420777407, 0.2882089793578257453 ) ) ;
#65776=CARTESIAN_POINT ( 'NONE',  ( 0.5774278215223104249, 0.1283753931104748280, 0.1820866141732283561 ) ) ;
#65777=CARTESIAN_POINT ( 'NONE',  ( -1.312335958005248715, 0.2306618581243848609, 0.2411417322834645549 ) ) ;
#65779=CARTESIAN_POINT ( 'NONE',  ( 1.207349081364829990, 0.2306618581243848609, 0.2411417322834645549 ) ) ;
#65781=CARTESIAN_POINT ( 'NONE',  ( 0.2952755905511819101, 0.1660481256975883668, -0.3530559997133364547 ) ) ;
#65783=CARTESIAN_POINT ( 'NONE',  ( -0.8478501267249378692, 2.401574803149606474, 0.8478501267249375362 ) ) ;
#65784=CARTESIAN_POINT ( 'NONE',  ( 0.3149606299212603933, -0.1870078740157479769, 0.3641732283464567677 ) ) ;
#65785=CARTESIAN_POINT ( 'NONE',  ( 0.4199475065616805614, 0.2306618581243848609, 0.2411417322834645549 ) ) ;
#65787=CARTESIAN_POINT ( 'NONE',  ( -1.069553805774277722, 0.1771653543307087630, 0.09757992244046791164 ) ) ;
#65788=CARTESIAN_POINT ( 'NONE',  ( -1.200787401574802349, 0.1660481256975883668, -0.3530559997133364547 ) ) ;
#65789=CARTESIAN_POINT ( 'NONE',  ( -1.364829396325458521, 0.2306618581243847221, -0.2411417322834647770 ) ) ;
#65790=CARTESIAN_POINT ( 'NONE',  ( 0.6496062992125991586, -0.5400638737290845981, -0.3530559997133363437 ) ) ;
#65791=CARTESIAN_POINT ( 'NONE',  ( -1.574803149606298192, -0.1870078740157480601, -0.3641732283464567677 ) ) ;
#65793=CARTESIAN_POINT ( 'NONE',  ( 0.7349081364829402885, -0.6046776061558809534, -0.2411417322834644161 ) ) ;
#65796=CARTESIAN_POINT ( 'NONE',  ( 1.443569553805774897, -0.6046776061558809534, -0.2411417322834644161 ) ) ;
#65797=CARTESIAN_POINT ( 'NONE',  ( -1.299212598425196097, -0.5511811023622047445, 6.969142054262312111E-17 ) ) ;
#65798=CARTESIAN_POINT ( 'NONE',  ( 1.095800524934383846, -0.08942795157528024563, -0.3641732283464568787 ) ) ;
#65799=CARTESIAN_POINT ( 'NONE',  ( -1.345144356955379816, -0.2845877964562159024, 0.3641732283464567677 ) ) ;
#65800=CARTESIAN_POINT ( 'NONE',  ( -0.7545931758530176614, -0.5511811023622048555, -0.09757992244046775898 ) ) ;
#65803=CARTESIAN_POINT ( 'NONE',  ( 0.3083989501312343062, -0.2845877964562159024, 0.3641732283464567677 ) ) ;
#65804=CARTESIAN_POINT ( 'NONE',  ( 0.5708661417322842269, 0.1660481256975885056, 0.3530559997133364547 ) ) ;
#65805=CARTESIAN_POINT ( 'NONE',  ( 1.253280839895013710, -0.3162353388693405765, 0.4822834645669290543 ) ) ;
#65806=CARTESIAN_POINT ( 'NONE',  ( -0.1049868766404193215, -0.6046776061558807314, 0.2411417322834647770 ) ) ;
#65807=CARTESIAN_POINT ( 'NONE',  ( -0.04593175853018302557, -0.5511811023622048555, -0.09757992244046775898 ) ) ;
#65808=CARTESIAN_POINT ( 'NONE',  ( 1.404199475065617264, -0.4281496062992124485, 0.4176697321401328655 ) ) ;
#65809=CARTESIAN_POINT ( 'NONE',  ( -1.607611548556429737, 0.2952755905511810774, -0.1292274648535930714 ) ) ;
#65810=CARTESIAN_POINT ( 'NONE',  ( -1.062992125984250968, 0.2952755905511811885, 0.000000000000000000 ) ) ;
#65812=CARTESIAN_POINT ( 'NONE',  ( 0.05249343832021075018, 0.1539470093639521697, -0.1968503937007875793 ) ) ;
#65813=CARTESIAN_POINT ( 'NONE',  ( 0.006561679790026889343, -0.05778040916215522460, 0.4822834645669289988 ) ) ;
#65814=CARTESIAN_POINT ( 'NONE',  ( -0.9186351706036736120, -0.6046776061558809534, -0.2411417322834644161 ) ) ;
#65815=CARTESIAN_POINT ( 'NONE',  ( 0.1312335958005255154, -0.6046776061558807314, 0.2411417322834647770 ) ) ;
#65820=CARTESIAN_POINT ( 'NONE',  ( -0.8070866141732276899, -0.4536011799217367080, 0.2665933059059888421 ) ) ;
#65822=CARTESIAN_POINT ( 'NONE',  ( 1.614173228346457378, 0.1771653543307087630, 0.000000000000000000 ) ) ;
#65824=CARTESIAN_POINT ( 'NONE',  ( 0.5577427821522316087, -0.05778040916215522460, 0.4822834645669289988 ) ) ;
#65825=CARTESIAN_POINT ( 'NONE',  ( -0.3674540682414692561, -0.5023911411419708095, -0.1820866141732282451 ) ) ;
#65826=CARTESIAN_POINT ( 'NONE',  ( 1.017060367454068581, -0.05778040916215560624, -0.4822834645669293319 ) ) ;
#65827=CARTESIAN_POINT ( 'NONE',  ( 0.4986876640419954376, 0.2306618581243848609, 0.2411417322834645549 ) ) ;
#65831=CARTESIAN_POINT ( 'NONE',  ( 1.423884514435696413, -0.3162353388693409650, -0.4822834645669289433 ) ) ;
#65832=CARTESIAN_POINT ( 'NONE',  ( -0.09842519685039295696, 0.1660481256975883668, -0.3530559997133364547 ) ) ;
#65833=CARTESIAN_POINT ( 'NONE',  ( -1.548556430446193399, -0.6046776061558809534, -0.2411417322834644161 ) ) ;
#65834=CARTESIAN_POINT ( 'NONE',  ( 0.9645669291338591078, -0.5400638737290845981, -0.3530559997133363437 ) ) ;
#65836=CARTESIAN_POINT ( 'NONE',  ( -0.03280839895013062252, -0.6692913385826771977, 0.1292274648535927661 ) ) ;
#65837=CARTESIAN_POINT ( 'NONE',  ( 0.8398950131233602345, -0.6046776061558807314, 0.2411417322834647770 ) ) ;
#65838=CARTESIAN_POINT ( 'NONE',  ( -0.2034120734908128059, 0.2952755905511811885, 0.1292274648535926551 ) ) ;
#65839=CARTESIAN_POINT ( 'NONE',  ( 1.246719160104987623, -0.004921259842519870586, -0.3153832671262229437 ) ) ;
#65840=CARTESIAN_POINT ( 'NONE',  ( -1.371391076115484831, 0.2952755905511810774, -0.1292274648535930714 ) ) ;
#65841=CARTESIAN_POINT ( 'NONE',  ( -1.377952755905511140, 0.2952755905511811885, 0.000000000000000000 ) ) ;
#65842=CARTESIAN_POINT ( 'NONE',  ( 0.8005249343832027131, 0.05413385826771666132, 0.4176697321401328100 ) ) ;
#65845=VERTEX_POINT ( 'NONE', #16748 ) ;
#65848=CARTESIAN_POINT ( 'NONE',  ( 0.9973753280839902091, -0.6046776061558807314, 0.2411417322834647770 ) ) ;
#65849=CARTESIAN_POINT ( 'NONE',  ( 1.141732283464567566, 0.1771653543307087630, 0.000000000000000000 ) ) ;
#65850=CARTESIAN_POINT ( 'NONE',  ( 0.5839895013123366230, 0.2952755905511811885, 0.1292274648535926551 ) ) ;
#65854=CARTESIAN_POINT ( 'NONE',  ( 1.332020997375328974, -0.05778040916215560624, -0.4822834645669293319 ) ) ;
#65856=CARTESIAN_POINT ( 'NONE',  ( -0.4593175853018366950, 0.05413385826771666132, 0.4176697321401328100 ) ) ;
#65857=CARTESIAN_POINT ( 'NONE',  ( 1.246719160104987623, -0.4281496062992124485, 0.4176697321401328655 ) ) ;
#65858=EDGE_LOOP ( 'NONE', ( #45490, #21642, #8277, #18835 ) ) ;
#65859=CARTESIAN_POINT ( 'NONE',  ( -1.377952755905511140, 0.2952755905511811885, 0.000000000000000000 ) ) ;
#65862=FACE_OUTER_BOUND ( 'NONE', #76444, .T. ) ;
#65863=DIRECTION ( 'NONE',  ( -1.000000000000000000, -3.469446951953613696E-16, 0.000000000000000000 ) ) ;
#65864=CARTESIAN_POINT ( 'NONE',  ( -0.9514435695538050464, -0.08942795157528024563, -0.3641732283464568787 ) ) ;
#65865=CARTESIAN_POINT ( 'NONE',  ( -1.515748031496062076, -0.5400638737290844871, 0.3530559997133364547 ) ) ;
#65866=CARTESIAN_POINT ( 'NONE',  ( 0.4855643044619430415, -0.4281496062992127816, -0.4176697321401328100 ) ) ;
#65868=FACE_OUTER_BOUND ( 'NONE', #68132, .T. ) ;
#65869=FACE_OUTER_BOUND ( 'NONE', #65532, .T. ) ;
#65870=CARTESIAN_POINT ( 'NONE',  ( -0.8595800524934373854, -0.2845877964562161244, -0.3641732283464567121 ) ) ;
#65871=CARTESIAN_POINT ( 'NONE',  ( 0.7086614173228353852, -0.1870078740157479769, 0.4822834645669291653 ) ) ;
#65872=CARTESIAN_POINT ( 'NONE',  ( -1.601049868766403650, -0.6046776061558807314, 0.2411417322834647770 ) ) ;
#65874=CARTESIAN_POINT ( 'NONE',  ( -0.6692913385826764205, -0.5511811023622047445, 6.969142054262312111E-17 ) ) ;
#65875=CARTESIAN_POINT ( 'NONE',  ( 1.601049868766404982, -0.6046776061558809534, -0.2411417322834644161 ) ) ;
#65876=CARTESIAN_POINT ( 'NONE',  ( 0.4824498642376759960, 1.223219560026271499E-15, 0.4445507791589056734 ) ) ;
#65877=CARTESIAN_POINT ( 'NONE',  ( 0.5839895013123367340, -0.6692913385826773087, -0.1292274648535924053 ) ) ;
#65878=CARTESIAN_POINT ( 'NONE',  ( -0.8989501312335946848, -0.5511811023622046335, 0.09757992244046803654 ) ) ;
#65879=CARTESIAN_POINT ( 'NONE',  ( -0.3477690288713905509, -0.5511811023622046335, 0.09757992244046803654 ) ) ;
#65880=CARTESIAN_POINT ( 'NONE',  ( -0.1181102362204717315, 0.2952755905511811885, 0.000000000000000000 ) ) ;
#65881=CARTESIAN_POINT ( 'NONE',  ( -1.167979002624671470, -0.004921259842519576551, 0.3153832671262227771 ) ) ;
#65883=CARTESIAN_POINT ( 'NONE',  ( 0.7808398950131240079, -0.3162353388693405765, 0.4822834645669290543 ) ) ;
#65885=CARTESIAN_POINT ( 'NONE',  ( 0.4061203303035133549, 3.421639014772782816E-16, 0.3464511005275203726 ) ) ;
#65887=CARTESIAN_POINT ( 'NONE',  ( -0.8464566929133852113, -0.5400638737290845981, -0.3530559997133363437 ) ) ;
#65888=CARTESIAN_POINT ( 'NONE',  ( -0.07874015748031421014, -0.1870078740157480601, -0.3641732283464567677 ) ) ;
#65889=CARTESIAN_POINT ( 'NONE',  ( -1.174540682414697335, -0.05778040916215522460, 0.4822834645669289988 ) ) ;
#65890=CARTESIAN_POINT ( 'NONE',  ( 0.9645669291338591078, -0.4536011799217368745, -0.2665933059059886201 ) ) ;
#65891=CARTESIAN_POINT ( 'NONE',  ( -0.7742782152230965886, -0.004921259842519576551, 0.3153832671262227771 ) ) ;
#65892=CARTESIAN_POINT ( 'NONE',  ( -1.023622047244094002, -0.1870078740157480879, -0.4822834645669291653 ) ) ;
#65893=CARTESIAN_POINT ( 'NONE',  ( -1.660104986876639543, -0.05778040916215560624, -0.4822834645669293319 ) ) ;
#65894=CARTESIAN_POINT ( 'NONE',  ( -1.528871391076114250, -0.6692913385826771977, 0.1292274648535927661 ) ) ;
#65895=CARTESIAN_POINT ( 'NONE',  ( 0.7677165354330716118, 0.07958543189024071263, -0.2665933059059888421 ) ) ;
#65896=CARTESIAN_POINT ( 'NONE',  ( 0.4921259842519691285, -0.5400638737290845981, -0.3530559997133363437 ) ) ;
#65897=CARTESIAN_POINT ( 'NONE',  ( -1.443569553805773564, 0.2306618581243847221, -0.2411417322834647770 ) ) ;
#65898=CARTESIAN_POINT ( 'NONE',  ( 1.384514435695538337, -0.5511811023622046335, 0.09757992244046803654 ) ) ;
#65901=CARTESIAN_POINT ( 'NONE',  ( -1.227034120734907141, -0.5511811023622048555, -0.09757992244046775898 ) ) ;
#65902=CARTESIAN_POINT ( 'NONE',  ( -0.5643044619422565855, -0.4281496062992124485, 0.4176697321401328655 ) ) ;
#65903=CARTESIAN_POINT ( 'NONE',  ( 0.8989501312335963501, -0.6692913385826773087, -0.1292274648535924053 ) ) ;
#65904=CARTESIAN_POINT ( 'NONE',  ( -1.332020997375327642, -0.2845877964562161244, -0.3641732283464567121 ) ) ;
#65906=CARTESIAN_POINT ( 'NONE',  ( -1.620734908136482577, -0.6692913385826773087, -0.1292274648535924053 ) ) ;
#65907=CARTESIAN_POINT ( 'NONE',  ( 0.5643044619422579178, 0.05413385826771666132, 0.4176697321401328100 ) ) ;
#65908=CARTESIAN_POINT ( 'NONE',  ( 0.6036745406824154392, 0.2306618581243847221, -0.2411417322834647770 ) ) ;
#65909=CARTESIAN_POINT ( 'NONE',  ( 1.318897637795276356, 0.1660481256975883668, -0.3530559997133364547 ) ) ;
#65915=CARTESIAN_POINT ( 'NONE',  ( 0.1640419947506569498, -0.08942795157527998196, 0.3641732283464567121 ) ) ;
#65916=CARTESIAN_POINT ( 'NONE',  ( -0.4330708661417315697, 0.2952755905511811885, 0.000000000000000000 ) ) ;
#65917=CARTESIAN_POINT ( 'NONE',  ( 1.286089238845145033, 0.2306618581243848609, 0.2411417322834645549 ) ) ;
#65919=CARTESIAN_POINT ( 'NONE',  ( 0.2690288713910767848, 0.1771653543307087630, 0.09757992244046791164 ) ) ;
#65920=CARTESIAN_POINT ( 'NONE',  ( -0.7349081364829387342, -0.6046776061558807314, 0.2411417322834647770 ) ) ;
#65921=CARTESIAN_POINT ( 'NONE',  ( 1.456692913385827515, 0.2952755905511811885, 0.000000000000000000 ) ) ;
#65922=CARTESIAN_POINT ( 'NONE',  ( 0.5643044619422579178, 0.05413385826771666132, 0.4176697321401328100 ) ) ;
#65927=CARTESIAN_POINT ( 'NONE',  ( -1.574803149606298636, -0.1870078740157479769, 0.4822834645669291653 ) ) ;
#65928=CARTESIAN_POINT ( 'NONE',  ( -1.108923884514435132, -0.08942795157528024563, -0.3641732283464568787 ) ) ;
#65929=CARTESIAN_POINT ( 'NONE',  ( -1.181102362204723644, -0.1870078740157479769, 0.4822834645669291653 ) ) ;
#65931=CARTESIAN_POINT ( 'NONE',  ( 1.614173228346456712, 2.401574803149606474, -0.1372047244094476703 ) ) ;
#65932=CARTESIAN_POINT ( 'NONE',  ( 1.541994750656168645, 0.2952755905511810774, -0.1292274648535930714 ) ) ;
#65933=CARTESIAN_POINT ( 'NONE',  ( -1.384514435695537005, 0.2952755905511811885, 0.1292274648535926551 ) ) ;
#65934=CARTESIAN_POINT ( 'NONE',  ( -0.1049868766404193215, 0.2306618581243847221, -0.2411417322834647770 ) ) ;
#65936=CARTESIAN_POINT ( 'NONE',  ( -1.082677165354329896, -0.5400638737290845981, -0.3530559997133363437 ) ) ;
#65938=CARTESIAN_POINT ( 'NONE',  ( 0.5774278215223103139, -0.6046776061558809534, -0.2411417322834644161 ) ) ;
#65940=CARTESIAN_POINT ( 'NONE',  ( -1.049868766404198794, -0.5023911411419708095, 0.1820866141732285504 ) ) ;
#65945=CARTESIAN_POINT ( 'NONE',  ( -0.9448818897637790704, -0.1870078740157479769, 0.4822834645669291653 ) ) ;
#65946=CARTESIAN_POINT ( 'NONE',  ( -1.509186351706035767, -0.4281496062992124485, 0.4176697321401328655 ) ) ;
#65948=CARTESIAN_POINT ( 'NONE',  ( -1.364829396325458521, 0.2306618581243847221, -0.2411417322834647770 ) ) ;
#65949=CARTESIAN_POINT ( 'NONE',  ( -1.502624671916009680, -0.05778040916215560624, -0.4822834645669293319 ) ) ;
#65950=CARTESIAN_POINT ( 'NONE',  ( -1.299212598425196097, 0.2952755905511811885, 0.000000000000000000 ) ) ;
#65951=CARTESIAN_POINT ( 'NONE',  ( -0.7773926554473638006, -2.191421614605370878E-15, 0.4445507791589071167 ) ) ;
#65953=CARTESIAN_POINT ( 'NONE',  ( 0.1968503937007881344, -0.5511811023622047445, 6.969142054262312111E-17 ) ) ;
#65955=CARTESIAN_POINT ( 'NONE',  ( -0.6167979002624665030, -0.004921259842519576551, 0.3153832671262227771 ) ) ;
#65956=CARTESIAN_POINT ( 'NONE',  ( -1.240157480314959759, -0.5400638737290845981, -0.3530559997133363437 ) ) ;
#65957=CARTESIAN_POINT ( 'NONE',  ( 1.135170603674541256, 0.2952755905511811885, 0.1292274648535926551 ) ) ;
#65958=CARTESIAN_POINT ( 'NONE',  ( -1.122047244094487306, 0.1660481256975883668, -0.3530559997133364547 ) ) ;
#65960=VERTEX_POINT ( 'NONE', #68899 ) ;
#65961=CARTESIAN_POINT ( 'NONE',  ( -0.8858267716535425107, -0.5400638737290844871, 0.3530559997133364547 ) ) ;
#65962=CARTESIAN_POINT ( 'NONE',  ( 0.9711286089238851948, 0.2306618581243848609, 0.2411417322834645549 ) ) ;
#65963=CARTESIAN_POINT ( 'NONE',  ( -1.679790026246718693, 0.1283753931104746893, -0.1820866141732285504 ) ) ;
#65964=CARTESIAN_POINT ( 'NONE',  ( -1.706036745406823485, 0.2306618581243848609, 0.2411417322834645549 ) ) ;
#65969=CARTESIAN_POINT ( 'NONE',  ( -0.4986876640419939388, 0.2306618581243847221, -0.2411417322834647770 ) ) ;
#65970=CARTESIAN_POINT ( 'NONE',  ( -1.548556430446193399, -0.5023911411419708095, -0.1820866141732282451 ) ) ;
#65972=CARTESIAN_POINT ( 'NONE',  ( -1.332020997375327642, -0.3162353388693409650, -0.4822834645669289433 ) ) ;
#65974=CARTESIAN_POINT ( 'NONE',  ( -1.528871391076114250, 0.2952755905511810774, -0.1292274648535930714 ) ) ;
#65975=CARTESIAN_POINT ( 'NONE',  ( -0.4461942257217840213, 0.2306618581243848609, 0.2411417322834645549 ) ) ;
#65977=CARTESIAN_POINT ( 'NONE',  ( 0.6233595800524939223, -0.2845877964562159024, 0.3641732283464567677 ) ) ;
#65979=CARTESIAN_POINT ( 'NONE',  ( 0.4330708661417329575, 0.1771653543307087630, 0.000000000000000000 ) ) ;
#65980=CARTESIAN_POINT ( 'NONE',  ( 1.417322834645670104, -0.1870078740157479769, 0.3641732283464567677 ) ) ;
#65981=CARTESIAN_POINT ( 'NONE',  ( 0.7611548556430451917, -0.6046776061558807314, 0.2411417322834647770 ) ) ;
#65982=CARTESIAN_POINT ( 'NONE',  ( 0.3215223097112867578, -0.2845877964562161244, -0.3641732283464567121 ) ) ;
#65984=CARTESIAN_POINT ( 'NONE',  ( -1.266404199475064773, -0.05778040916215560624, -0.4822834645669293319 ) ) ;
#65985=CARTESIAN_POINT ( 'NONE',  ( -0.1509186351706028884, -0.08942795157527998196, 0.3641732283464567121 ) ) ;
#65986=CARTESIAN_POINT ( 'NONE',  ( -1.082677165354329896, -0.4536011799217368745, -0.2665933059059886201 ) ) ;
#65988=CARTESIAN_POINT ( 'NONE',  ( -0.4265091863517051496, -0.5511811023622046335, 0.09757992244046803654 ) ) ;
#65990=CARTESIAN_POINT ( 'NONE',  ( 0.09186351706036827158, 0.05413385826771666132, 0.4176697321401328100 ) ) ;
#65992=CARTESIAN_POINT ( 'NONE',  ( 0.4790026246719167324, -0.08942795157527998196, 0.3641732283464567121 ) ) ;
#65993=CARTESIAN_POINT ( 'NONE',  ( -0.3346456692913377662, -0.4536011799217367080, 0.2665933059059888421 ) ) ;
#65994=CARTESIAN_POINT ( 'NONE',  ( -0.4068241469816264999, -0.4281496062992124485, 0.4176697321401328655 ) ) ;
#65995=CARTESIAN_POINT ( 'NONE',  ( -1.692913385826770645, 0.2952755905511811885, 0.000000000000000000 ) ) ;
#65996=CARTESIAN_POINT ( 'NONE',  ( -1.122047244094487306, 0.07958543189024071263, -0.2665933059059888421 ) ) ;
#65997=DIRECTION ( 'NONE',  ( -1.000000000000000000, -3.050063254464715288E-16, 0.000000000000000000 ) ) ;
#65998=CARTESIAN_POINT ( 'NONE',  ( 0.5183727034120741983, -0.6692913385826771977, 0.1292274648535927661 ) ) ;
#65999=CARTESIAN_POINT ( 'NONE',  ( -0.9251968503937002541, -0.5400638737290845981, -0.3530559997133363437 ) ) ;
#66002=CARTESIAN_POINT ( 'NONE',  ( -0.3805774278215216522, -0.3690944881889765550, -0.3153832671262227771 ) ) ;
#66003=CARTESIAN_POINT ( 'NONE',  ( 2.787279214012418738, 1.496062992125984481, 0.000000000000000000 ) ) ;
#66004=CARTESIAN_POINT ( 'NONE',  ( -1.082677165354329896, -0.4536011799217368745, -0.2665933059059886201 ) ) ;
#66005=CARTESIAN_POINT ( 'NONE',  ( 1.601049868766404982, -0.6046776061558809534, -0.2411417322834644161 ) ) ;
#66007=CARTESIAN_POINT ( 'NONE',  ( -0.8202099737532801971, -0.5511811023622046335, 0.09757992244046803654 ) ) ;
#66008=CARTESIAN_POINT ( 'NONE',  ( -0.7210809602247715278, -2.613618158232546091E-15, -0.3464511005275220379 ) ) ;
#66009=CARTESIAN_POINT ( 'NONE',  ( 0.8595800524934390507, -0.05778040916215560624, -0.4822834645669293319 ) ) ;
#66015=CARTESIAN_POINT ( 'NONE',  ( -1.692913385826770645, 0.2952755905511811885, 0.000000000000000000 ) ) ;
#66016=CARTESIAN_POINT ( 'NONE',  ( -1.089238845144356427, 0.05413385826771666132, 0.4176697321401328100 ) ) ;
#66017=CARTESIAN_POINT ( 'NONE',  ( 1.128608923884514947, 0.2306618581243848609, 0.2411417322834645549 ) ) ;
#66019=CARTESIAN_POINT ( 'NONE',  ( 1.502624671916010790, -0.08942795157527998196, 0.3641732283464567121 ) ) ;
#66021=CARTESIAN_POINT ( 'NONE',  ( 0.4593175853018380828, 0.05413385826771626580, -0.4176697321401330321 ) ) ;
#66022=CARTESIAN_POINT ( 'NONE',  ( -0.1902887139107604098, 0.2952755905511810774, -0.1292274648535930714 ) ) ;
#66023=CARTESIAN_POINT ( 'NONE',  ( 1.502624671916010790, -0.05778040916215522460, 0.4822834645669289988 ) ) ;
#66024=CARTESIAN_POINT ( 'NONE',  ( 0.8267716535433077274, 0.1771653543307087630, 0.000000000000000000 ) ) ;
#66028=CARTESIAN_POINT ( 'NONE',  ( -0.2690288713910754526, 0.2952755905511810774, -0.1292274648535930714 ) ) ;
#66029=CARTESIAN_POINT ( 'NONE',  ( 1.318897637795276356, 0.1660481256975883668, -0.3530559997133364547 ) ) ;
#66030=CARTESIAN_POINT ( 'NONE',  ( 0.1049868766404206816, 0.2306618581243848609, 0.2411417322834645549 ) ) ;
#66031=CARTESIAN_POINT ( 'NONE',  ( -0.5183727034120726440, 0.1771653543307087630, 0.09757992244046791164 ) ) ;
#66032=CARTESIAN_POINT ( 'NONE',  ( 1.286089238845145033, -0.6046776061558809534, -0.2411417322834644161 ) ) ;
#66033=CARTESIAN_POINT ( 'NONE',  ( -1.102362204724408601, -0.1870078740157480879, -0.4822834645669291653 ) ) ;
#66034=CARTESIAN_POINT ( 'NONE',  ( 0.03937007874015806264, 0.2952755905511811885, 0.000000000000000000 ) ) ;
#66035=CARTESIAN_POINT ( 'NONE',  ( 1.515748031496063186, -0.5400638737290845981, -0.3530559997133363437 ) ) ;
#66036=CARTESIAN_POINT ( 'NONE',  ( 1.003937007874016185, 0.1660481256975883668, -0.3530559997133364547 ) ) ;
#66037=CARTESIAN_POINT ( 'NONE',  ( 1.102362204724410155, -0.1870078740157480879, -0.4822834645669291653 ) ) ;
#66040=CARTESIAN_POINT ( 'NONE',  ( 0.05905511811023709395, -0.4536011799217367080, 0.2665933059059888421 ) ) ;
#66044=CARTESIAN_POINT ( 'NONE',  ( -0.3215223097112853146, -0.2845877964562159024, 0.3641732283464567677 ) ) ;
#66045=CARTESIAN_POINT ( 'NONE',  ( 0.04593175853018440641, -0.6692913385826771977, 0.1292274648535927661 ) ) ;
#66047=CARTESIAN_POINT ( 'NONE',  ( -0.4133858267716528645, 0.1660481256975883668, -0.3530559997133364547 ) ) ;
#66048=CARTESIAN_POINT ( 'NONE',  ( -0.3674540682414692561, -0.6046776061558809534, -0.2411417322834644161 ) ) ;
#66049=ADVANCED_FACE ( 'NONE', ( #81958 ), #50831, .F. ) ;
#66050=CARTESIAN_POINT ( 'NONE',  ( -0.7152230971128602510, -0.3162353388693405765, 0.4822834645669290543 ) ) ;
#66051=CARTESIAN_POINT ( 'NONE',  ( -1.003937007874015297, -0.5400638737290845981, -0.3530559997133363437 ) ) ;
#66052=CARTESIAN_POINT ( 'NONE',  ( 1.509186351706037543, -0.004921259842519576551, 0.3153832671262227771 ) ) ;
#66055=CARTESIAN_POINT ( 'NONE',  ( 0.4002624671916016896, -0.2845877964562161244, -0.3641732283464567121 ) ) ;
#66056=CARTESIAN_POINT ( 'NONE',  ( 0.4265091863517067594, 0.2952755905511811885, 0.1292274648535926551 ) ) ;
#66057=CARTESIAN_POINT ( 'NONE',  ( 0.5183727034120741983, -0.6692913385826771977, 0.1292274648535927661 ) ) ;
#66060=CARTESIAN_POINT ( 'NONE',  ( 0.3249695492770460770, 1.223219560026271499E-15, 0.4445507791589056734 ) ) ;
#66063=CARTESIAN_POINT ( 'NONE',  ( -0.5446194225721777693, -0.3162353388693409650, -0.4822834645669289433 ) ) ;
#66066=CARTESIAN_POINT ( 'NONE',  ( -1.364829396325458521, -0.5023911411419708095, 0.1820866141732285504 ) ) ;
#66067=CARTESIAN_POINT ( 'NONE',  ( 0.9251968503937015864, -0.5400638737290844871, 0.3530559997133364547 ) ) ;
#66068=CARTESIAN_POINT ( 'NONE',  ( 0.8267716535433078384, -0.6692913385826771977, 8.415575281601705876E-17 ) ) ;
#66069=CARTESIAN_POINT ( 'NONE',  ( -0.1377952755905504645, -0.4536011799217368745, -0.2665933059059886201 ) ) ;
#66070=CARTESIAN_POINT ( 'NONE',  ( 0.5314960629921264834, 0.1660481256975883668, -0.3530559997133364547 ) ) ;
#66072=CARTESIAN_POINT ( 'NONE',  ( -0.1771653543307080136, 0.07958543189024071263, -0.2665933059059888421 ) ) ;
#66073=CARTESIAN_POINT ( 'NONE',  ( -0.05249343832020938322, -0.6046776061558809534, -0.2411417322834644161 ) ) ;
#66075=CARTESIAN_POINT ( 'NONE',  ( -1.561679790026246017, 0.05413385826771666132, 0.4176697321401328100 ) ) ;
#66076=CARTESIAN_POINT ( 'NONE',  ( 0.4855643044619428750, -0.004921259842519576551, 0.3153832671262227771 ) ) ;
#66077=CARTESIAN_POINT ( 'NONE',  ( 1.509186351706037543, -0.004921259842519576551, 0.3153832671262227771 ) ) ;
#66078=CARTESIAN_POINT ( 'NONE',  ( -0.7217847769028863381, 0.05413385826771626580, -0.4176697321401330321 ) ) ;
#66079=CARTESIAN_POINT ( 'NONE',  ( -0.7152230971128602510, -0.2845877964562159024, 0.3641732283464567677 ) ) ;
#66081=CARTESIAN_POINT ( 'NONE',  ( -0.8530183727034112984, -0.4281496062992127816, -0.4176697321401328100 ) ) ;
#66082=CARTESIAN_POINT ( 'NONE',  ( -0.6889763779527552368, 0.1660481256975885056, 0.3530559997133364547 ) ) ;
#66083=CARTESIAN_POINT ( 'NONE',  ( -0.1837270341207340729, 0.2306618581243847221, -0.2411417322834647770 ) ) ;
#66087=CARTESIAN_POINT ( 'NONE',  ( 0.8005249343832028242, -0.3690944881889765550, -0.3153832671262227771 ) ) ;
#66089=CARTESIAN_POINT ( 'NONE',  ( 1.187664041994751285, -0.3162353388693409650, -0.4822834645669289433 ) ) ;
#66090=CARTESIAN_POINT ( 'NONE',  ( -1.312335958005248715, -0.5023911411419708095, -0.1820866141732282451 ) ) ;
#66091=CARTESIAN_POINT ( 'NONE',  ( -1.292650918635170010, -0.5511811023622046335, 0.09757992244046803654 ) ) ;
#66092=CARTESIAN_POINT ( 'NONE',  ( -0.7152230971128602510, -0.05778040916215560624, -0.4822834645669293319 ) ) ;
#66093=CARTESIAN_POINT ( 'NONE',  ( -0.04593175853018302557, 0.1771653543307087630, 0.09757992244046791164 ) ) ;
#66095=CARTESIAN_POINT ( 'NONE',  ( 0.9120734908136489683, -0.5511811023622046335, 0.09757992244046803654 ) ) ;
#66097=CARTESIAN_POINT ( 'NONE',  ( 0.2427821522309719648, -0.05778040916215522460, 0.4822834645669289988 ) ) ;
#66099=CARTESIAN_POINT ( 'NONE',  ( -0.4921259842519677963, -0.5400638737290844871, 0.3530559997133364547 ) ) ;
#66101=CARTESIAN_POINT ( 'NONE',  ( 1.496062992125984703, -0.1870078740157480601, -0.3641732283464567677 ) ) ;
#66102=CARTESIAN_POINT ( 'NONE',  ( 0.3543307086614181922, -0.6692913385826771977, 8.415575281601705876E-17 ) ) ;
#66103=CARTESIAN_POINT ( 'NONE',  ( -0.01968503937007793844, 0.1660481256975883668, -0.3530559997133364547 ) ) ;
#66104=CARTESIAN_POINT ( 'NONE',  ( 0.05249343832021075018, -0.5023911411419708095, 0.1820866141732285504 ) ) ;
#66106=CARTESIAN_POINT ( 'NONE',  ( -0.1115485564304453947, -0.5511811023622046335, 0.09757992244046803654 ) ) ;
#66107=CARTESIAN_POINT ( 'NONE',  ( 0.9448818897637802916, -0.1870078740157480879, -0.4822834645669291653 ) ) ;
#66108=CARTESIAN_POINT ( 'NONE',  ( -0.7742782152230965886, -0.004921259842519576551, 0.3153832671262227771 ) ) ;
#66110=CARTESIAN_POINT ( 'NONE',  ( -1.154855643044618851, 0.2306618581243848609, 0.2411417322834645549 ) ) ;
#66111=CARTESIAN_POINT ( 'NONE',  ( -0.8561328129276786214, -2.191421614605370878E-15, 0.4445507791589071167 ) ) ;
#66112=VERTEX_POINT ( 'NONE', #63404 ) ;
#66113=CARTESIAN_POINT ( 'NONE',  ( -1.056430446194224881, -0.6692913385826771977, 0.1292274648535927661 ) ) ;
#66114=CARTESIAN_POINT ( 'NONE',  ( -1.003937007874015297, -0.4536011799217368745, -0.2665933059059886201 ) ) ;
#66115=CARTESIAN_POINT ( 'NONE',  ( 0.02624671916010564918, 0.2306618581243848609, 0.2411417322834645549 ) ) ;
#66117=CARTESIAN_POINT ( 'NONE',  ( -0.9514435695538050464, -0.05778040916215560624, -0.4822834645669293319 ) ) ;
#66119=CARTESIAN_POINT ( 'NONE',  ( 1.594488188976378673, -0.5400638737290845981, -0.3530559997133363437 ) ) ;
#66120=CARTESIAN_POINT ( 'NONE',  ( 1.062992125984252745, -0.6692913385826771977, 8.415575281601705876E-17 ) ) ;
#66121=CARTESIAN_POINT ( 'NONE',  ( 0.9711286089238851948, -0.6046776061558809534, -0.2411417322834644161 ) ) ;
#66122=CARTESIAN_POINT ( 'NONE',  ( -0.3025410870193214197, 0.000000000000000000, 0.3464511005275205946 ) ) ;
#66123=CARTESIAN_POINT ( 'NONE',  ( 1.561679790026247350, -0.4281496062992124485, 0.4176697321401328655 ) ) ;
#66124=CARTESIAN_POINT ( 'NONE',  ( -1.299212598425196097, -0.6692913385826771977, 8.415575281601705876E-17 ) ) ;
#66127=CARTESIAN_POINT ( 'NONE',  ( -0.6299212598425188991, -0.1870078740157480601, -0.3641732283464567677 ) ) ;
#66130=CARTESIAN_POINT ( 'NONE',  ( 0.1443569553805781891, -0.4281496062992124485, 0.4176697321401328655 ) ) ;
#66131=CARTESIAN_POINT ( 'NONE',  ( 0.1312335958005255154, -0.6046776061558807314, 0.2411417322834647770 ) ) ;
#66132=CARTESIAN_POINT ( 'NONE',  ( -0.8398950131233585692, 0.2306618581243848609, 0.2411417322834645549 ) ) ;
#66133=CARTESIAN_POINT ( 'NONE',  ( 1.692913385826772421, 0.2952755905511811885, 0.000000000000000000 ) ) ;
#66134=CARTESIAN_POINT ( 'NONE',  ( -1.049868766404198794, -0.5023911411419708095, 0.1820866141732285504 ) ) ;
#66136=CARTESIAN_POINT ( 'NONE',  ( 0.6167979002624679463, 0.05413385826771626580, -0.4176697321401330321 ) ) ;
#66137=CARTESIAN_POINT ( 'NONE',  ( 0.5971128608923890191, -0.5511811023622046335, 0.09757992244046803654 ) ) ;
#66138=CARTESIAN_POINT ( 'NONE',  ( -0.4593175853018364174, -0.4281496062992127816, -0.4176697321401328100 ) ) ;
#66140=CARTESIAN_POINT ( 'NONE',  ( -1.194225721784776262, -0.4281496062992124485, 0.4176697321401328655 ) ) ;
#66142=( BOUNDED_CURVE ( )  B_SPLINE_CURVE ( 2, ( #51658, #57564, #19694, #71465, #71048, #7068, #58832, #52078, #78207, #39471, #1190, #20539, #65583 ),
 .UNSPECIFIED., .F., .F. ) 
 B_SPLINE_CURVE_WITH_KNOTS ( ( 3, 2, 2, 2, 2, 2, 3 ),
 ( 0.5824220037257099580, 0.5833333333333333703, 0.5871212121212121549, 0.5909090909090909394, 0.5946969696969697239, 0.5984848484848485084, 0.5993961780924720317 ),
 .UNSPECIFIED. ) 
 CURVE ( )  GEOMETRIC_REPRESENTATION_ITEM ( )  RATIONAL_B_SPLINE_CURVE ( ( 0.9875488213027523443, 0.9918020599134680371, 1.000000000000000000, 0.9659258262890683122, 1.000000000000000000, 0.9659258262890683122, 1.000000000000000000, 0.9659258262890683122, 1.000000000000000000, 0.9659258262890683122, 1.000000000000000000, 0.9918020599134671489, 0.9875488213027514561 ) ) 
 REPRESENTATION_ITEM ( '' )  );
#66143=CARTESIAN_POINT ( 'NONE',  ( 1.325459317585302665, -0.4281496062992124485, 0.4176697321401328655 ) ) ;
#66147=CARTESIAN_POINT ( 'NONE',  ( 0.1902887139107617975, -0.6692913385826773087, -0.1292274648535924053 ) ) ;
#66149=CARTESIAN_POINT ( 'NONE',  ( 0.9251968503937015864, -0.4536011799217367080, 0.2665933059059888421 ) ) ;
#66150=CARTESIAN_POINT ( 'NONE',  ( -1.312335958005248715, -0.6046776061558809534, -0.2411417322834644161 ) ) ;
#66151=CARTESIAN_POINT ( 'NONE',  ( 1.181102362204724976, -0.1870078740157480879, -0.4822834645669291653 ) ) ;
#66152=CARTESIAN_POINT ( 'NONE',  ( 0.6692913385826777528, 0.2952755905511811885, 0.000000000000000000 ) ) ;
#66153=CARTESIAN_POINT ( 'NONE',  ( 0.3805774278215230400, 0.05413385826771626580, -0.4176697321401330321 ) ) ;
#66154=CARTESIAN_POINT ( 'NONE',  ( -0.2755905511811015396, -0.6692913385826771977, 8.415575281601705876E-17 ) ) ;
#66156=CARTESIAN_POINT ( 'NONE',  ( -1.272965879265091305, -0.4281496062992124485, 0.4176697321401328655 ) ) ;
#66157=CARTESIAN_POINT ( 'NONE',  ( -0.4658792650918627265, -0.3162353388693409650, -0.4822834645669289433 ) ) ;
#66158=CARTESIAN_POINT ( 'NONE',  ( -0.5511811023622038563, -0.1870078740157479769, 0.3641732283464567677 ) ) ;
#66159=CARTESIAN_POINT ( 'NONE',  ( 1.692913385826772421, 0.2952755905511811885, 0.000000000000000000 ) ) ;
#66160=CARTESIAN_POINT ( 'NONE',  ( 1.646981627296588035, -0.3162353388693405765, 0.4822834645669290543 ) ) ;
#66161=CARTESIAN_POINT ( 'NONE',  ( -0.3805774278215216522, -0.4281496062992127816, -0.4176697321401328100 ) ) ;
#66163=CARTESIAN_POINT ( 'NONE',  ( 0.8398950131233602345, 0.2306618581243847221, -0.2411417322834647770 ) ) ;
#66165=DIRECTION ( 'NONE',  ( 0.000000000000000000, -1.000000000000000000, -0.000000000000000000 ) ) ;
#66166=CARTESIAN_POINT ( 'NONE',  ( -0.1640419947506553400, -0.05778040916215560624, -0.4822834645669293319 ) ) ;
#66167=CARTESIAN_POINT ( 'NONE',  ( 1.207349081364829990, 0.1283753931104748280, 0.1820866141732283561 ) ) ;
#66170=CARTESIAN_POINT ( 'NONE',  ( 1.036745406824147731, -0.004921259842519576551, 0.3153832671262227771 ) ) ;
#66171=ADVANCED_FACE ( 'NONE', ( #43618 ), #31568, .F. ) ;
#66172=CARTESIAN_POINT ( 'NONE',  ( 1.023622047244095112, -0.1870078740157480879, -0.4822834645669291653 ) ) ;
#66175=CARTESIAN_POINT ( 'NONE',  ( -0.3346456692913377662, -0.5400638737290844871, 0.3530559997133364547 ) ) ;
#66176=CARTESIAN_POINT ( 'NONE',  ( -1.489501312335957062, -0.05778040916215522460, 0.4822834645669289988 ) ) ;
#66177=CARTESIAN_POINT ( 'NONE',  ( -1.548556430446193399, 0.2306618581243848609, 0.2411417322834645549 ) ) ;
#66178=CARTESIAN_POINT ( 'NONE',  ( -0.3018372703412066094, 0.05413385826771666132, 0.4176697321401328100 ) ) ;
#66179=EDGE_CURVE ( 'NONE', #32176, #32475, #45371, .T. ) ;
#66181=CARTESIAN_POINT ( 'NONE',  ( 1.240157480314961314, 0.1660481256975883668, -0.3530559997133364547 ) ) ;
#66182=CARTESIAN_POINT ( 'NONE',  ( 0.6167979002624678353, -0.4281496062992124485, 0.4176697321401328655 ) ) ;
#66183=CONICAL_SURFACE ( 'NONE', #25825, 1.220472440944881942, 0.7853981633974621568 ) ;
#66184=CARTESIAN_POINT ( 'NONE',  ( 0.4855643044619430415, -0.3690944881889765550, -0.3153832671262227771 ) ) ;
#66186=CARTESIAN_POINT ( 'NONE',  ( 0.4068241469816281097, -0.004921259842519576551, 0.3153832671262227771 ) ) ;
#66189=CARTESIAN_POINT ( 'NONE',  ( 0.5905511811023629321, 0.2952755905511811885, 0.000000000000000000 ) ) ;
#66192=CARTESIAN_POINT ( 'NONE',  ( -0.7977407017645437026, -5.134928753749862370E-15, -0.4281989832122469752 ) ) ;
#66193=CARTESIAN_POINT ( 'NONE',  ( -0.01312335958005186876, -0.3690944881889763329, 0.3153832671262228327 ) ) ;
#66194=CARTESIAN_POINT ( 'NONE',  ( 0.3412073490813655186, -0.6046776061558809534, -0.2411417322834644161 ) ) ;
#66195=CARTESIAN_POINT ( 'NONE',  ( 1.660104986876641320, -0.08942795157527998196, 0.3641732283464567121 ) ) ;
#66196=CARTESIAN_POINT ( 'NONE',  ( -1.023622047244094002, -0.1870078740157480601, -0.3641732283464567677 ) ) ;
#66197=CARTESIAN_POINT ( 'NONE',  ( -0.8595800524934373854, -0.3162353388693409650, -0.4822834645669289433 ) ) ;
#66198=CARTESIAN_POINT ( 'NONE',  ( -1.594488188976377563, -0.5400638737290844871, 0.3530559997133364547 ) ) ;
#66199=CARTESIAN_POINT ( 'NONE',  ( 0.4658792650918641698, -0.05778040916215560624, -0.4822834645669293319 ) ) ;
#66200=CARTESIAN_POINT ( 'NONE',  ( 1.640419947506562393, -0.4281496062992124485, 0.4176697321401328655 ) ) ;
#66202=CARTESIAN_POINT ( 'NONE',  ( 0.4265091863517067039, -0.6692913385826773087, -0.1292274648535924053 ) ) ;
#66205=CARTESIAN_POINT ( 'NONE',  ( 1.430446194225722500, -0.4281496062992127816, -0.4176697321401328100 ) ) ;
#66206=CARTESIAN_POINT ( 'NONE',  ( -1.266404199475064773, -0.2845877964562159024, 0.3641732283464567677 ) ) ;
#66207=CARTESIAN_POINT ( 'NONE',  ( 1.253280839895013710, -0.08942795157528024563, -0.3641732283464568787 ) ) ;
#66208=CARTESIAN_POINT ( 'NONE',  ( -1.515748031496062076, -0.4536011799217367080, 0.2665933059059888421 ) ) ;
#66209=CARTESIAN_POINT ( 'NONE',  ( -0.7939632545931750718, -0.08942795157528024563, -0.3641732283464568787 ) ) ;
#66210=CARTESIAN_POINT ( 'NONE',  ( 1.535433070866142335, -0.6692913385826771977, 8.415575281601705876E-17 ) ) ;
#66211=CARTESIAN_POINT ( 'NONE',  ( 0.4330708661417329575, -0.5511811023622047445, 6.969142054262312111E-17 ) ) ;
#66212=CARTESIAN_POINT ( 'NONE',  ( -0.07217847769028787330, -0.05778040916215522460, 0.4822834645669289988 ) ) ;
#66213=CARTESIAN_POINT ( 'NONE',  ( 0.9514435695538062676, -0.05778040916215522460, 0.4822834645669289988 ) ) ;
#66214=CARTESIAN_POINT ( 'NONE',  ( 0.1837270341207357105, -0.6046776061558809534, -0.2411417322834644161 ) ) ;
#66215=CARTESIAN_POINT ( 'NONE',  ( 0.2296587926509192634, -0.08942795157528024563, -0.3641732283464568787 ) ) ;
#66216=CARTESIAN_POINT ( 'NONE',  ( 1.154855643044620184, 0.2306618581243847221, -0.2411417322834647770 ) ) ;
#66217=CARTESIAN_POINT ( 'NONE',  ( -0.1706036745406816491, 0.009842519685039147898, -0.3409548833797004797 ) ) ;
#66218=CARTESIAN_POINT ( 'NONE',  ( -0.7808398950131225646, -0.05778040916215522460, 0.4822834645669289988 ) ) ;
#66219=B_SPLINE_CURVE_WITH_KNOTS ( 'NONE', 3,
 ( #24859, #50938, #18161, #24454 ),
 .UNSPECIFIED., .F., .F.,
 ( 4, 4 ),
 ( 1.999999999897049408E-07, 0.006970199999999935128 ),
 .UNSPECIFIED. ) ;
#66221=CARTESIAN_POINT ( 'NONE',  ( 0.04593175853018440641, 0.2066929133858267098, -0.1054918080437494132 ) ) ;
#66222=CARTESIAN_POINT ( 'NONE',  ( -0.9448818897637790704, -0.1870078740157480879, -0.4822834645669291653 ) ) ;
#66223=CARTESIAN_POINT ( 'NONE',  ( 0.08530183727034192087, -0.3162353388693409650, -0.4822834645669289433 ) ) ;
#66228=CYLINDRICAL_SURFACE ( 'NONE', #68171, 0.3937007874015748254 ) ;
#66229=CARTESIAN_POINT ( 'NONE',  ( -1.312335958005248715, -0.5023911411419708095, -0.1820866141732282451 ) ) ;
#66231=CARTESIAN_POINT ( 'NONE',  ( 1.601049868766404982, 0.1283753931104748280, 0.1820866141732283561 ) ) ;
#66233=CARTESIAN_POINT ( 'NONE',  ( 0.3412073490813655186, -0.6046776061558809534, -0.2411417322834644161 ) ) ;
#66234=CARTESIAN_POINT ( 'NONE',  ( -0.3477690288713905509, -0.5511811023622046335, 0.09757992244046803654 ) ) ;
#66235=CARTESIAN_POINT ( 'NONE',  ( 0.7874015748031503170, -0.1870078740157479769, 0.4822834645669291653 ) ) ;
#66236=CARTESIAN_POINT ( 'NONE',  ( 0.4593175853018379162, -0.4281496062992124485, 0.4176697321401328655 ) ) ;
#66240=CARTESIAN_POINT ( 'NONE',  ( 1.240157480314961314, 0.1660481256975883668, -0.3530559997133364547 ) ) ;
#66241=CARTESIAN_POINT ( 'NONE',  ( -0.1115485564304456306, 0.2952755905511810774, -0.1292274648535930714 ) ) ;
#66242=CARTESIAN_POINT ( 'NONE',  ( 1.476377952755906220, 0.1660481256975883668, -0.3530559997133364547 ) ) ;
#66243=CARTESIAN_POINT ( 'NONE',  ( 0.8858267716535438430, 0.1660481256975885056, 0.3530559997133364547 ) ) ;
#66245=CARTESIAN_POINT ( 'NONE',  ( 0.1902887139107617975, 0.2952755905511811885, 0.1292274648535926551 ) ) ;
#66246=CARTESIAN_POINT ( 'NONE',  ( 0.7939632545931766261, -0.3162353388693409650, -0.4822834645669289433 ) ) ;
#66247=CARTESIAN_POINT ( 'NONE',  ( 0.07874015748031558404, -0.1870078740157479769, 0.4822834645669291653 ) ) ;
#66248=CARTESIAN_POINT ( 'NONE',  ( 0.7283464566929143125, 0.07958543189024085140, 0.2665933059059887866 ) ) ;
#66249=CARTESIAN_POINT ( 'NONE',  ( -1.272965879265091305, -0.4281496062992124485, 0.4176697321401328655 ) ) ;
#66250=CARTESIAN_POINT ( 'NONE',  ( -1.607611548556429737, -0.6692913385826771977, 0.1292274648535927661 ) ) ;
#66251=CARTESIAN_POINT ( 'NONE',  ( 0.7152230971128614723, -0.3162353388693409650, -0.4822834645669289433 ) ) ;
#66254=VERTEX_POINT ( 'NONE', #24772 ) ;
#66257=CARTESIAN_POINT ( 'NONE',  ( 0.9580052493438327987, -0.4281496062992127816, -0.4176697321401328100 ) ) ;
#66258=CARTESIAN_POINT ( 'NONE',  ( 0.3412073490813655186, 0.1283753931104748280, 0.1820866141732283561 ) ) ;
#66262=ADVANCED_FACE ( 'NONE', ( #50441 ), #63499, .F. ) ;
#66263=CARTESIAN_POINT ( 'NONE',  ( 1.227034120734908917, -0.6692913385826771977, 0.1292274648535927661 ) ) ;
#66264=CARTESIAN_POINT ( 'NONE',  ( -1.535433070866141225, -0.6692913385826771977, 8.415575281601705876E-17 ) ) ;
#66266=CARTESIAN_POINT ( 'NONE',  ( -0.3608923884514428360, -0.6692913385826773087, -0.1292274648535924053 ) ) ;
#66267=CARTESIAN_POINT ( 'NONE',  ( 1.062992125984252745, -0.6692913385826771977, 8.415575281601705876E-17 ) ) ;
#66269=CARTESIAN_POINT ( 'NONE',  ( -1.732283464566928277, -0.1870078740157479769, 0.4822834645669291653 ) ) ;
#66272=CARTESIAN_POINT ( 'NONE',  ( -1.595398199321657051, 0.7585570207896574768, -0.1559797534342474146 ) ) ;
#66274=CARTESIAN_POINT ( 'NONE',  ( -1.299212598425196097, 0.1771653543307087630, 0.000000000000000000 ) ) ;
#66275=CARTESIAN_POINT ( 'NONE',  ( -1.548556430446193399, -0.6046776061558809534, -0.2411417322834644161 ) ) ;
#66276=CARTESIAN_POINT ( 'NONE',  ( 0.6364829396325465405, -0.3162353388693409650, -0.4822834645669289433 ) ) ;
#66278=CARTESIAN_POINT ( 'NONE',  ( 1.410761154855643795, -0.05778040916215560624, -0.4822834645669293319 ) ) ;
#66280=CARTESIAN_POINT ( 'NONE',  ( -0.7414698162729651543, 0.1771653543307087075, -0.09757992244046823083 ) ) ;
#66281=CARTESIAN_POINT ( 'NONE',  ( 0.8267716535433078384, -0.6692913385826771977, 8.415575281601705876E-17 ) ) ;
#66282=CARTESIAN_POINT ( 'NONE',  ( 1.594488188976378673, 0.07958543189024085140, 0.2665933059059887866 ) ) ;
#66285=CARTESIAN_POINT ( 'NONE',  ( -0.9842519685039365918, -0.5511811023622047445, 6.969142054262312111E-17 ) ) ;
#66286=CARTESIAN_POINT ( 'NONE',  ( -1.502624671916009680, -0.2845877964562159024, 0.3641732283464567677 ) ) ;
#66288=CARTESIAN_POINT ( 'NONE',  ( 0.6102362204724416372, -0.5400638737290844871, 0.3530559997133364547 ) ) ;
#66289=CARTESIAN_POINT ( 'NONE',  ( -1.069553805774277722, -0.5511811023622048555, -0.09757992244046775898 ) ) ;
#66290=CARTESIAN_POINT ( 'NONE',  ( -0.2230971128608915943, -0.3690944881889765550, -0.3153832671262227771 ) ) ;
#66291=CARTESIAN_POINT ( 'NONE',  ( -0.1574803149606292529, -0.1870078740157479769, 0.4822834645669291653 ) ) ;
#66292=CARTESIAN_POINT ( 'NONE',  ( 1.601049868766404982, -0.6046776061558809534, -0.2411417322834644161 ) ) ;
#66294=CARTESIAN_POINT ( 'NONE',  ( 0.9448818897637802916, -0.1870078740157479769, 0.4822834645669291653 ) ) ;
#66297=CARTESIAN_POINT ( 'NONE',  ( -0.7152230971128602510, -0.05778040916215560624, -0.4822834645669293319 ) ) ;
#66298=CARTESIAN_POINT ( 'NONE',  ( -0.09186351706036689768, -0.004921259842519870586, -0.3153832671262229437 ) ) ;
#66299=CARTESIAN_POINT ( 'NONE',  ( -1.515748031496062076, -0.5400638737290844871, 0.3530559997133364547 ) ) ;
#66300=CARTESIAN_POINT ( 'NONE',  ( 0.3805774278215230400, -0.3690944881889763329, 0.3153832671262228327 ) ) ;
#66301=CARTESIAN_POINT ( 'NONE',  ( -0.5839895013123351797, 0.1771653543307087075, -0.09757992244046823083 ) ) ;
#66302=CARTESIAN_POINT ( 'NONE',  ( -1.207349081364828880, 0.2306618581243847221, -0.2411417322834647770 ) ) ;
#66303=CARTESIAN_POINT ( 'NONE',  ( -1.607611548556429737, -0.6692913385826771977, 0.1292274648535927661 ) ) ;
#66304=CARTESIAN_POINT ( 'NONE',  ( 1.601049868766404982, -0.6046776061558809534, -0.2411417322834644161 ) ) ;
#66305=CARTESIAN_POINT ( 'NONE',  ( -0.7080320533160967544, 1.900312960331933976, 0.5309055118110236338 ) ) ;
#66306=CARTESIAN_POINT ( 'NONE',  ( 0.6955380577427828781, -0.3690944881889763329, 0.3153832671262228327 ) ) ;
#66307=CARTESIAN_POINT ( 'NONE',  ( 0.4002624671916016896, -0.05778040916215522460, 0.4822834645669289988 ) ) ;
#66308=CARTESIAN_POINT ( 'NONE',  ( -1.463254593175852492, 0.2952755905511811885, 0.1292274648535926551 ) ) ;
#66309=CARTESIAN_POINT ( 'NONE',  ( 1.469816272965879911, 0.1283753931104746893, -0.1820866141732285504 ) ) ;
#66311=B_SPLINE_CURVE_WITH_KNOTS ( 'NONE', 3,
 ( #31388, #6967, #667, #25068, #6551, #31807, #51559 ),
 .UNSPECIFIED., .F., .F.,
 ( 4, 3, 4 ),
 ( 6.162975822039154730E-33, 0.001246232571205312329, 0.002492492258783241162 ),
 .UNSPECIFIED. ) ;
#66313=CARTESIAN_POINT ( 'NONE',  ( -1.161417322834644716, 0.07958543189024085140, 0.2665933059059887866 ) ) ;
#66314=CARTESIAN_POINT ( 'NONE',  ( -0.4790026246719152336, -0.05778040916215560624, -0.4822834645669293319 ) ) ;
#66315=CARTESIAN_POINT ( 'NONE',  ( 0.1509186351706042484, -0.3162353388693405765, 0.4822834645669290543 ) ) ;
#66316=CARTESIAN_POINT ( 'NONE',  ( -1.469816272965878357, -0.5023911411419708095, -0.1820866141732282451 ) ) ;
#66318=CARTESIAN_POINT ( 'NONE',  ( -1.351706036745406347, 0.05413385826771626580, -0.4176697321401330321 ) ) ;
#66319=CARTESIAN_POINT ( 'NONE',  ( 0.5249343832021005074, -0.6046776061558807314, 0.2411417322834647770 ) ) ;
#66320=CARTESIAN_POINT ( 'NONE',  ( 0.1837270341207357105, -0.6046776061558809534, -0.2411417322834644161 ) ) ;
#66321=CARTESIAN_POINT ( 'NONE',  ( 1.272965879265092637, 0.05413385826771666132, 0.4176697321401328100 ) ) ;
#66325=B_SPLINE_CURVE_WITH_KNOTS ( 'NONE', 3,
 ( #47921, #9227, #10054, #41615 ),
 .UNSPECIFIED., .F., .F.,
 ( 4, 4 ),
 ( 3.593986969192262371E-07, 0.001287825409103183008 ),
 .UNSPECIFIED. ) ;
#66328=CARTESIAN_POINT ( 'NONE',  ( -0.01968503937007793844, -0.4536011799217367080, 0.2665933059059888421 ) ) ;
#66329=CARTESIAN_POINT ( 'NONE',  ( -0.2887139107611542133, 0.2306618581243848609, 0.2411417322834645549 ) ) ;
#66330=CARTESIAN_POINT ( 'NONE',  ( 0.8070866141732288002, 0.1660481256975885056, 0.3530559997133364547 ) ) ;
#66332=CARTESIAN_POINT ( 'NONE',  ( -0.2099737532808391705, 0.1283753931104748280, 0.1820866141732283561 ) ) ;
#66333=CARTESIAN_POINT ( 'NONE',  ( -1.299212598425196097, 0.2952755905511811885, 0.000000000000000000 ) ) ;
#66334=CARTESIAN_POINT ( 'NONE',  ( -1.594488188976377119, 0.1660481256975883668, -0.3530559997133364547 ) ) ;
#66337=ORIENTED_EDGE ( 'NONE', *, *, #29846, .F. ) ;
#66339=CARTESIAN_POINT ( 'NONE',  ( 1.272965879265092637, 0.05413385826771666132, 0.4176697321401328100 ) ) ;
#66340=CIRCLE ( 'NONE', #74399, 2.362204724409449064 ) ;
#66341=CARTESIAN_POINT ( 'NONE',  ( -1.679790026246718693, 0.2306618581243847221, -0.2411417322834647770 ) ) ;
#66342=CARTESIAN_POINT ( 'NONE',  ( -1.351706036745406347, -0.3690944881889763329, 0.3153832671262228327 ) ) ;
#66343=CARTESIAN_POINT ( 'NONE',  ( -1.371391076115484609, -0.6692913385826771977, 0.1292274648535927661 ) ) ;
#66346=CARTESIAN_POINT ( 'NONE',  ( 1.043307086614173818, 0.1660481256975885056, 0.3530559997133364547 ) ) ;
#66347=CARTESIAN_POINT ( 'NONE',  ( 0.1181102362204730916, -0.6692913385826771977, 8.415575281601705876E-17 ) ) ;
#66348=CARTESIAN_POINT ( 'NONE',  ( -0.2952755905511804668, 0.1660481256975885056, 0.3530559997133364547 ) ) ;
#66349=CARTESIAN_POINT ( 'NONE',  ( -1.220472440944881054, -0.6692913385826771977, 8.415575281601705876E-17 ) ) ;
#66351=EDGE_CURVE ( 'NONE', #66780, #9475, #43779, .T. ) ;
#66352=CARTESIAN_POINT ( 'NONE',  ( 0.5643044619422579178, -0.4281496062992127816, -0.4176697321401328100 ) ) ;
#66354=CARTESIAN_POINT ( 'NONE',  ( -1.358267716535432434, -0.4536011799217367080, 0.2665933059059888421 ) ) ;
#66355=VERTEX_POINT ( 'NONE', #59674 ) ;
#66359=CARTESIAN_POINT ( 'NONE',  ( -1.220472440944881054, 0.2952755905511811885, 0.000000000000000000 ) ) ;
#66360=CARTESIAN_POINT ( 'NONE',  ( -1.154855643044618851, 0.2306618581243848609, 0.2411417322834645549 ) ) ;
#66362=CARTESIAN_POINT ( 'NONE',  ( -1.496062992125983815, -0.1870078740157480879, -0.4822834645669291653 ) ) ;
#66363=CARTESIAN_POINT ( 'NONE',  ( -1.581364829396324945, -0.3162353388693405765, 0.4822834645669290543 ) ) ;
#66368=CARTESIAN_POINT ( 'NONE',  ( -0.07217847769028787330, -0.08942795157527998196, 0.3641732283464567121 ) ) ;
#66369=CARTESIAN_POINT ( 'NONE',  ( -0.6364829396325453192, -0.2845877964562159024, 0.3641732283464567677 ) ) ;
#66370=CARTESIAN_POINT ( 'NONE',  ( -1.259842519685038686, -0.1870078740157480879, -0.4822834645669291653 ) ) ;
#66371=CARTESIAN_POINT ( 'NONE',  ( 1.095800524934383846, -0.3162353388693405765, 0.4822834645669290543 ) ) ;
#66372=CARTESIAN_POINT ( 'NONE',  ( -1.102362204724408601, -0.1870078740157480879, -0.4822834645669291653 ) ) ;
#66375=CARTESIAN_POINT ( 'NONE',  ( -1.528871391076114250, -0.6692913385826771977, 0.1292274648535927661 ) ) ;
#66376=CARTESIAN_POINT ( 'NONE',  ( -1.712598425196849572, 0.07958543189024085140, 0.2665933059059887866 ) ) ;
#66377=CARTESIAN_POINT ( 'NONE',  ( -1.627296587926508442, -0.6046776061558809534, -0.2411417322834644161 ) ) ;
#66379=DIRECTION ( 'NONE',  ( 1.000000000000000000, -0.000000000000000000, -0.000000000000000000 ) ) ;
#66382=CARTESIAN_POINT ( 'NONE',  ( -0.5183727034120726440, 0.2952755905511811885, 0.1292274648535926551 ) ) ;
#66383=CARTESIAN_POINT ( 'NONE',  ( -1.509186351706035767, -0.3690944881889763329, 0.3153832671262228327 ) ) ;
#66386=CARTESIAN_POINT ( 'NONE',  ( -1.496062992125983815, -0.1870078740157480879, -0.4822834645669291653 ) ) ;
#66387=CARTESIAN_POINT ( 'NONE',  ( -0.4921259842519677963, -0.5400638737290844871, 0.3530559997133364547 ) ) ;
#66389=CARTESIAN_POINT ( 'NONE',  ( 0.3674540682414705883, 0.1283753931104746893, -0.1820866141732285504 ) ) ;
#66390=DIRECTION ( 'NONE',  ( 0.000000000000000000, 1.000000000000000000, 0.000000000000000000 ) ) ;
#66392=CARTESIAN_POINT ( 'NONE',  ( 0.4002624671916016896, -0.08942795157527998196, 0.3641732283464567121 ) ) ;
#66393=CARTESIAN_POINT ( 'NONE',  ( 0.8595800524934390507, -0.08942795157528024563, -0.3641732283464568787 ) ) ;
#66394=CARTESIAN_POINT ( 'NONE',  ( 0.8530183727034126306, 0.05413385826771626580, -0.4176697321401330321 ) ) ;
#66395=CARTESIAN_POINT ( 'NONE',  ( -0.1574803149606292529, -0.1870078740157480601, -0.3641732283464567677 ) ) ;
#66397=CARTESIAN_POINT ( 'NONE',  ( -1.220472440944881054, -0.6692913385826771977, 8.415575281601705876E-17 ) ) ;
#66398=CARTESIAN_POINT ( 'NONE',  ( 0.09842519685039434474, -0.4536011799217368745, -0.2665933059059886201 ) ) ;
#66399=CARTESIAN_POINT ( 'NONE',  ( -1.128608923884513837, 0.1283753931104746893, -0.1820866141732285504 ) ) ;
#66401=CARTESIAN_POINT ( 'NONE',  ( -0.7742782152230962556, -0.3690944881889765550, -0.3153832671262227771 ) ) ;
#66403=CARTESIAN_POINT ( 'NONE',  ( -0.1640419947506553400, -0.05778040916215560624, -0.4822834645669293319 ) ) ;
#66404=CARTESIAN_POINT ( 'NONE',  ( 1.633858267716535639, -0.4536011799217367080, 0.2665933059059888421 ) ) ;
#66406=CARTESIAN_POINT ( 'NONE',  ( 0.6758530183727039509, 0.1771653543307087075, -0.09757992244046823083 ) ) ;
#66407=CARTESIAN_POINT ( 'NONE',  ( -0.2624671916010490880, 0.1283753931104746893, -0.1820866141732285504 ) ) ;
#66408=CARTESIAN_POINT ( 'NONE',  ( -0.3149606299212590610, -0.1870078740157480879, -0.4822834645669291653 ) ) ;
#66410=CARTESIAN_POINT ( 'NONE',  ( -1.213910761154854745, -0.5511811023622046335, 0.09757992244046803654 ) ) ;
#66412=CARTESIAN_POINT ( 'NONE',  ( 0.7742782152230979209, 0.05413385826771626580, -0.4176697321401330321 ) ) ;
#66415=DIRECTION ( 'NONE',  ( -1.000000000000000000, -3.412570772413390973E-16, 0.000000000000000000 ) ) ;
#66416=CARTESIAN_POINT ( 'NONE',  ( -0.2559055118110230564, 0.07958543189024071263, -0.2665933059059888421 ) ) ;
#66417=CARTESIAN_POINT ( 'NONE',  ( -1.581364829396324945, -0.05778040916215560624, -0.4822834645669293319 ) ) ;
#66418=CARTESIAN_POINT ( 'NONE',  ( 1.568241469816273659, -0.05778040916215560624, -0.4822834645669293319 ) ) ;
#66419=CARTESIAN_POINT ( 'NONE',  ( 1.391076115485564868, 0.2306618581243847221, -0.2411417322834647770 ) ) ;
#66420=CARTESIAN_POINT ( 'NONE',  ( -0.5380577427821514602, -0.3690944881889765550, -0.3153832671262227771 ) ) ;
#66421=CARTESIAN_POINT ( 'NONE',  ( -1.090866038711135744, -2.570477104772672414E-15, 0.3791475997938242304 ) ) ;
#66422=CARTESIAN_POINT ( 'NONE',  ( 0.7677165354330716118, -0.5400638737290844871, 0.3530559997133364547 ) ) ;
#66425=EDGE_CURVE ( 'NONE', #30161, #7970, #26656, .T. ) ;
#66427=CARTESIAN_POINT ( 'NONE',  ( 1.476377952755906220, 0.07958543189024071263, -0.2665933059059888421 ) ) ;
#66428=CARTESIAN_POINT ( 'NONE',  ( -1.338582677165353729, -0.1870078740157480879, -0.4822834645669291653 ) ) ;
#66429=CARTESIAN_POINT ( 'NONE',  ( 1.286089238845145033, 0.2306618581243848609, 0.2411417322834645549 ) ) ;
#66431=CARTESIAN_POINT ( 'NONE',  ( 1.102362204724410155, -0.1870078740157480601, -0.3641732283464567677 ) ) ;
#66432=CARTESIAN_POINT ( 'NONE',  ( 0.1181102362204730916, 0.2952755905511811885, 0.000000000000000000 ) ) ;
#66433=CARTESIAN_POINT ( 'NONE',  ( -0.4855643044619415427, 0.05413385826771626580, -0.4176697321401330321 ) ) ;
#66434=CARTESIAN_POINT ( 'NONE',  ( 1.620734908136483465, -0.6692913385826771977, 0.1292274648535927661 ) ) ;
#66436=CARTESIAN_POINT ( 'NONE',  ( 0.1902887139107617975, 0.1771653543307087630, 0.09757992244046791164 ) ) ;
#66440=CARTESIAN_POINT ( 'NONE',  ( -0.2821522309711278487, 0.2952755905511811885, 0.1292274648535926551 ) ) ;
#66441=CARTESIAN_POINT ( 'NONE',  ( 1.377952755905512472, -0.6692913385826771977, 8.415575281601705876E-17 ) ) ;
#66442=CARTESIAN_POINT ( 'NONE',  ( 0.05905511811023709395, -0.5400638737290844871, 0.3530559997133364547 ) ) ;
#66443=CARTESIAN_POINT ( 'NONE',  ( -0.2230971128608915943, -0.004921259842519576551, 0.3153832671262227771 ) ) ;
#66445=CARTESIAN_POINT ( 'NONE',  ( 1.194225721784777594, 0.05413385826771666132, 0.4176697321401328100 ) ) ;
#66446=CARTESIAN_POINT ( 'NONE',  ( -0.8661417322834640276, -0.1870078740157479769, 0.4822834645669291653 ) ) ;
#66447=CARTESIAN_POINT ( 'NONE',  ( -0.1574803149606292529, -0.1870078740157479769, 0.4822834645669291653 ) ) ;
#66448=CARTESIAN_POINT ( 'NONE',  ( -0.7808398950131225646, -0.05778040916215522460, 0.4822834645669289988 ) ) ;
#66449=CARTESIAN_POINT ( 'NONE',  ( 1.174540682414699111, -0.05778040916215560624, -0.4822834645669293319 ) ) ;
#66450=CARTESIAN_POINT ( 'NONE',  ( 1.089238845144357537, -0.4281496062992124485, 0.4176697321401328655 ) ) ;
#66451=CARTESIAN_POINT ( 'NONE',  ( 1.187664041994751285, -0.05778040916215522460, 0.4822834645669289988 ) ) ;
#66453=CARTESIAN_POINT ( 'NONE',  ( 0.1312335958005257930, 0.1283753931104746893, -0.1820866141732285504 ) ) ;
#66454=EDGE_LOOP ( 'NONE', ( #66732, #45720, #1476, #48535 ) ) ;
#66457=CARTESIAN_POINT ( 'NONE',  ( -0.9448818897637790704, -0.1870078740157479769, 0.3641732283464567677 ) ) ;
#66458=CARTESIAN_POINT ( 'NONE',  ( -0.1574803149606292529, -0.1870078740157480879, -0.4822834645669291653 ) ) ;
#66460=CARTESIAN_POINT ( 'NONE',  ( -0.4199475065616791736, 0.2306618581243847221, -0.2411417322834647770 ) ) ;
#66461=CARTESIAN_POINT ( 'NONE',  ( -0.5249343832020990641, -0.6046776061558809534, -0.2411417322834644161 ) ) ;
#66462=CARTESIAN_POINT ( 'NONE',  ( -0.8858267716535425107, -0.5400638737290844871, 0.3530559997133364547 ) ) ;
#66463=CARTESIAN_POINT ( 'NONE',  ( -1.358267716535432434, 0.1660481256975883668, -0.3530559997133364547 ) ) ;
#66464=CIRCLE ( 'NONE', #46312, 3.582677165354332338 ) ;
#66465=CARTESIAN_POINT ( 'NONE',  ( 1.528871391076116026, 0.1771653543307087630, 0.09757992244046791164 ) ) ;
#66466=DIRECTION ( 'NONE',  ( -0.7071067811865495711, 0.000000000000000000, 0.7071067811865454633 ) ) ;
#66468=CARTESIAN_POINT ( 'NONE',  ( 0.2952755905511816326, -0.4536011799217367080, 0.2665933059059888421 ) ) ;
#66469=CARTESIAN_POINT ( 'NONE',  ( -0.04593175853018302557, 0.2952755905511811885, 0.1292274648535926551 ) ) ;
#66470=CARTESIAN_POINT ( 'NONE',  ( 0.3805774278215230400, -0.4281496062992124485, 0.4176697321401328655 ) ) ;
#66476=CARTESIAN_POINT ( 'NONE',  ( -0.6036745406824141069, 0.2306618581243848609, 0.2411417322834645549 ) ) ;
#66479=CARTESIAN_POINT ( 'NONE',  ( -1.601049868766403650, 0.1283753931104746893, -0.1820866141732285504 ) ) ;
#66480=CARTESIAN_POINT ( 'NONE',  ( 1.043307086614173818, -0.5400638737290845981, -0.3530559997133363437 ) ) ;
#66481=CARTESIAN_POINT ( 'NONE',  ( 0.8464566929133866546, -0.5400638737290844871, 0.3530559997133364547 ) ) ;
#66482=CARTESIAN_POINT ( 'NONE',  ( -0.2755905511811015396, -0.5511811023622047445, 6.969142054262312111E-17 ) ) ;
#66483=CARTESIAN_POINT ( 'NONE',  ( 0.2427821522309716595, -0.3162353388693409650, -0.4822834645669289433 ) ) ;
#66485=CARTESIAN_POINT ( 'NONE',  ( -0.04593175853018302557, 0.1771653543307087630, 0.09757992244046791164 ) ) ;
#66486=CARTESIAN_POINT ( 'NONE',  ( -0.3280839895013117347, -0.4281496062992124485, 0.4176697321401328655 ) ) ;
#66488=CARTESIAN_POINT ( 'NONE',  ( -1.607611548556429737, -0.6692913385826771977, 0.1292274648535927661 ) ) ;
#66489=CARTESIAN_POINT ( 'NONE',  ( 0.2624671916010504757, -0.5023911411419708095, -0.1820866141732282451 ) ) ;
#66490=CARTESIAN_POINT ( 'NONE',  ( -0.7330015572057683171, 1.982446682556143758, -0.5178628694646268960 ) ) ;
#66491=CARTESIAN_POINT ( 'NONE',  ( -1.017060367454067249, -0.3162353388693409650, -0.4822834645669289433 ) ) ;
#66493=CARTESIAN_POINT ( 'NONE',  ( -0.5511811023622038563, -0.1870078740157479769, 0.3641732283464567677 ) ) ;
#66495=CARTESIAN_POINT ( 'NONE',  ( -0.6758530183727028406, -0.6692913385826773087, -0.1292274648535924053 ) ) ;
#66496=CARTESIAN_POINT ( 'NONE',  ( -0.4593175853018364174, -0.4281496062992127816, -0.4176697321401328100 ) ) ;
#66497=CARTESIAN_POINT ( 'NONE',  ( 0.07874015748031558404, -0.1870078740157479769, 0.4822834645669291653 ) ) ;
#66501=CARTESIAN_POINT ( 'NONE',  ( 0.3018372703412079971, -0.004921259842519870586, -0.3153832671262229437 ) ) ;
#66502=CARTESIAN_POINT ( 'NONE',  ( 1.076115485564305141, -0.6046776061558807314, 0.2411417322834647770 ) ) ;
#66503=CARTESIAN_POINT ( 'NONE',  ( -1.253280839895012377, -0.08942795157527998196, 0.3641732283464567121 ) ) ;
#66504=( BOUNDED_CURVE ( )  B_SPLINE_CURVE ( 2, ( #66122, #8458, #42088, #21496, #15613, #66958, #29463, #34128, #9702, #2562, #15194, #28220, #16029 ),
 .UNSPECIFIED., .F., .F. ) 
 B_SPLINE_CURVE_WITH_KNOTS ( ( 3, 2, 2, 2, 2, 2, 3 ),
 ( 0.4126696296615054438, 0.4128787878787879562, 0.4166666666666667407, 0.4204545454545455252, 0.4242424242424243097, 0.4280303030303030942, 0.4282394612475854956 ),
 .UNSPECIFIED. ) 
 CURVE ( )  GEOMETRIC_REPRESENTATION_ITEM ( )  RATIONAL_B_SPLINE_CURVE ( ( 0.9964447847208419695, 0.9981185001348091834, 1.000000000000000000, 0.9659258262890683122, 1.000000000000000000, 0.9659258262890683122, 1.000000000000000000, 0.9659258262890683122, 1.000000000000000000, 0.9659258262890683122, 1.000000000000000000, 0.9981185001348101826, 0.9964447847208438569 ) ) 
 REPRESENTATION_ITEM ( '' )  );
#66505=CARTESIAN_POINT ( 'NONE',  ( 1.049868766404200349, 0.2306618581243848609, 0.2411417322834645549 ) ) ;
#66506=CARTESIAN_POINT ( 'NONE',  ( -1.220472440944881054, 0.1771653543307087630, 0.000000000000000000 ) ) ;
#66507=CARTESIAN_POINT ( 'NONE',  ( -0.3477690288713905509, -0.6692913385826771977, 0.1292274648535927661 ) ) ;
#66508=CARTESIAN_POINT ( 'NONE',  ( 0.2362204724409456558, -0.1870078740157479769, 0.3641732283464567677 ) ) ;
#66509=CARTESIAN_POINT ( 'NONE',  ( 1.607547226907515947, 0.2919332483279780122, 0.05801724265248875412 ) ) ;
#66510=CARTESIAN_POINT ( 'NONE',  ( 0.6692913385826777528, 0.1771653543307087630, 0.000000000000000000 ) ) ;
#66512=CARTESIAN_POINT ( 'NONE',  ( 0.1509186351706045259, -0.05778040916215560624, -0.4822834645669293319 ) ) ;
#66513=EDGE_CURVE ( 'NONE', #77522, #48621, #20712, .T. ) ;
#66515=CARTESIAN_POINT ( 'NONE',  ( -0.6364829396325453192, -0.3162353388693405765, 0.4822834645669290543 ) ) ;
#66517=CARTESIAN_POINT ( 'NONE',  ( 1.233595800524935227, -0.5023911411419708095, 0.1820866141732285504 ) ) ;
#66518=CARTESIAN_POINT ( 'NONE',  ( 0.6430446194225729606, -0.4281496062992127816, -0.4176697321401328100 ) ) ;
#66519=CARTESIAN_POINT ( 'NONE',  ( -0.3871391076115476282, -0.05778040916215522460, 0.4822834645669289988 ) ) ;
#66520=CARTESIAN_POINT ( 'NONE',  ( -0.3543307086614165824, 0.1771653543307087630, 0.000000000000000000 ) ) ;
#66521=DIRECTION ( 'NONE',  ( -0.7071067811865489050, -2.189697074797801291E-16, 0.7071067811865460184 ) ) ;
#66522=CARTESIAN_POINT ( 'NONE',  ( 0.1115485564304470323, 0.1771653543307087630, 0.09757992244046791164 ) ) ;
#66523=CARTESIAN_POINT ( 'NONE',  ( 0.5314960629921267055, -0.5400638737290844871, 0.3530559997133364547 ) ) ;
#66524=CARTESIAN_POINT ( 'NONE',  ( -0.5643044619422565855, -0.004921259842519870586, -0.3153832671262229437 ) ) ;
#66527=CARTESIAN_POINT ( 'NONE',  ( -1.194225721784776262, -0.4281496062992124485, 0.4176697321401328655 ) ) ;
#66530=CARTESIAN_POINT ( 'NONE',  ( -1.253280839895012377, -0.08942795157527998196, 0.3641732283464567121 ) ) ;
#66531=CARTESIAN_POINT ( 'NONE',  ( -0.2362204724409442680, -0.1870078740157480879, -0.4822834645669291653 ) ) ;
#66532=CARTESIAN_POINT ( 'NONE',  ( -1.502624671916009680, -0.05778040916215560624, -0.4822834645669293319 ) ) ;
#66533=CARTESIAN_POINT ( 'NONE',  ( -0.9776902887139098386, 0.2952755905511810774, -0.1292274648535930714 ) ) ;
#66535=CARTESIAN_POINT ( 'NONE',  ( 1.174540682414699111, -0.3162353388693405765, 0.4822834645669290543 ) ) ;
#66536=CARTESIAN_POINT ( 'NONE',  ( 1.049868766404200349, 0.2306618581243848609, 0.2411417322834645549 ) ) ;
#66537=DIRECTION ( 'NONE',  ( 1.000000000000000000, 0.000000000000000000, -0.000000000000000000 ) ) ;
#66538=CARTESIAN_POINT ( 'NONE',  ( 1.456692913385827515, 0.2952755905511811885, 0.000000000000000000 ) ) ;
#66540=CARTESIAN_POINT ( 'NONE',  ( -1.305774278215222184, -0.6692913385826773087, -0.1292274648535924053 ) ) ;
#66543=CARTESIAN_POINT ( 'NONE',  ( -0.5446194225721777693, -0.08942795157527998196, 0.3641732283464567121 ) ) ;
#66545=EDGE_LOOP ( 'NONE', ( #25866, #50857, #6703, #70554 ) ) ;
#66546=CARTESIAN_POINT ( 'NONE',  ( 0.8005249343832027131, 0.05413385826771666132, 0.4176697321401328100 ) ) ;
#66547=CARTESIAN_POINT ( 'NONE',  ( -0.09186351706036689768, 0.05413385826771626580, -0.4176697321401330321 ) ) ;
#66548=CARTESIAN_POINT ( 'NONE',  ( -0.8792650918635160906, -0.4281496062992124485, 0.4176697321401328655 ) ) ;
#66549=CARTESIAN_POINT ( 'NONE',  ( 1.515748031496063408, 0.1660481256975885056, 0.3530559997133364547 ) ) ;
#66550=CARTESIAN_POINT ( 'NONE',  ( -0.7349081364829387342, -0.5023911411419708095, 0.1820866141732285504 ) ) ;
#66552=CARTESIAN_POINT ( 'NONE',  ( 0.4527559055118117182, 0.1660481256975883668, -0.3530559997133364547 ) ) ;
#66553=CARTESIAN_POINT ( 'NONE',  ( 0.5249343832021003964, 0.1283753931104746893, -0.1820866141732285504 ) ) ;
#66554=CARTESIAN_POINT ( 'NONE',  ( -1.030183727034119867, -0.3162353388693405765, 0.4822834645669290543 ) ) ;
#66556=CARTESIAN_POINT ( 'NONE',  ( -1.240157480314959759, -0.5400638737290845981, -0.3530559997133363437 ) ) ;
#66558=CARTESIAN_POINT ( 'NONE',  ( 0.9973753280839902091, -0.6046776061558807314, 0.2411417322834647770 ) ) ;
#66559=CARTESIAN_POINT ( 'NONE',  ( 1.187664041994751285, -0.08942795157527998196, 0.3641732283464567121 ) ) ;
#66562=CARTESIAN_POINT ( 'NONE',  ( -0.4724409448818890911, -0.1870078740157480879, -0.4822834645669291653 ) ) ;
#66564=CARTESIAN_POINT ( 'NONE',  ( 0.4724409448818904789, -0.1870078740157479769, 0.3641732283464567677 ) ) ;
#66565=CARTESIAN_POINT ( 'NONE',  ( -1.318897637795274802, -0.5400638737290845981, -0.3530559997133363437 ) ) ;
#66566=CARTESIAN_POINT ( 'NONE',  ( 0.8398950131233602345, 0.2306618581243847221, -0.2411417322834647770 ) ) ;
#66567=CARTESIAN_POINT ( 'NONE',  ( 0.8595800524934390507, -0.05778040916215560624, -0.4822834645669293319 ) ) ;
#66568=CARTESIAN_POINT ( 'NONE',  ( -0.2165354330708654795, -0.5400638737290845981, -0.3530559997133363437 ) ) ;
#66569=CARTESIAN_POINT ( 'NONE',  ( -0.4921259842519677963, 0.1660481256975883668, -0.3530559997133364547 ) ) ;
#66571=CARTESIAN_POINT ( 'NONE',  ( -1.548556430446193399, 0.2306618581243848609, 0.2411417322834645549 ) ) ;
#66572=CARTESIAN_POINT ( 'NONE',  ( -0.8070866141732276899, 0.1660481256975883668, -0.3530559997133364547 ) ) ;
#66573=CARTESIAN_POINT ( 'NONE',  ( -0.3740157480314953431, 0.07958543189024085140, 0.2665933059059887866 ) ) ;
#66574=CARTESIAN_POINT ( 'NONE',  ( 1.384514435695538559, 0.2952755905511810774, -0.1292274648535930714 ) ) ;
#66575=CARTESIAN_POINT ( 'NONE',  ( 1.581364829396326277, -0.3162353388693409650, -0.4822834645669289433 ) ) ;
#66576=CARTESIAN_POINT ( 'NONE',  ( -0.5774278215223089816, 0.2306618581243847221, -0.2411417322834647770 ) ) ;
#66578=CARTESIAN_POINT ( 'NONE',  ( 0.8595800524934390507, -0.05778040916215560624, -0.4822834645669293319 ) ) ;
#66581=CARTESIAN_POINT ( 'NONE',  ( -0.07874015748031421014, -0.1870078740157479769, 0.4822834645669291653 ) ) ;
#66582=CARTESIAN_POINT ( 'NONE',  ( -1.325459317585300889, -0.004921259842519576551, 0.3153832671262227771 ) ) ;
#66583=CARTESIAN_POINT ( 'NONE',  ( 1.200787401574803681, 0.07958543189024085140, 0.2665933059059887866 ) ) ;
#66586=CARTESIAN_POINT ( 'NONE',  ( 1.207349081364829990, 0.1283753931104748280, 0.1820866141732283561 ) ) ;
#66587=CARTESIAN_POINT ( 'NONE',  ( 1.397637795275591177, -0.5400638737290844871, 0.3530559997133364547 ) ) ;
#66588=AXIS2_PLACEMENT_3D ( 'NONE', #8683, #34353, #53689 ) ;
#66590=CARTESIAN_POINT ( 'NONE',  ( -0.1968503937007867743, -0.6692913385826771977, 8.415575281601705876E-17 ) ) ;
#66592=CARTESIAN_POINT ( 'NONE',  ( 1.213910761154856299, -0.5511811023622048555, -0.09757992244046775898 ) ) ;
#66593=CARTESIAN_POINT ( 'NONE',  ( -0.1377952755905504645, 0.1660481256975885056, 0.3530559997133364547 ) ) ;
#66596=CARTESIAN_POINT ( 'NONE',  ( 1.325459317585302665, -0.4281496062992124485, 0.4176697321401328655 ) ) ;
#66597=CARTESIAN_POINT ( 'NONE',  ( 0.4855643044619428750, 0.05413385826771666132, 0.4176697321401328100 ) ) ;
#66598=CARTESIAN_POINT ( 'NONE',  ( 0.4527559055118117182, 0.07958543189024071263, -0.2665933059059888421 ) ) ;
#66600=CARTESIAN_POINT ( 'NONE',  ( 0.3280839895013130669, -0.3690944881889765550, -0.3153832671262227771 ) ) ;
#66601=CARTESIAN_POINT ( 'NONE',  ( -1.594488188976377119, 0.1660481256975883668, -0.3530559997133364547 ) ) ;
#66603=CARTESIAN_POINT ( 'NONE',  ( 0.7545931758530189937, 0.2952755905511810774, -0.1292274648535930714 ) ) ;
#66605=CARTESIAN_POINT ( 'NONE',  ( 0.8761506516392508770, -4.927456884911482678E-16, 0.4445507791589062840 ) ) ;
#66607=CARTESIAN_POINT ( 'NONE',  ( -0.1181102362204717315, 0.1771653543307087630, 0.000000000000000000 ) ) ;
#66608=CARTESIAN_POINT ( 'NONE',  ( -0.09186351706036663400, -0.4281496062992124485, 0.4176697321401328655 ) ) ;
#66609=CARTESIAN_POINT ( 'NONE',  ( 1.430446194225722500, -0.3690944881889765550, -0.3153832671262227771 ) ) ;
#66610=CARTESIAN_POINT ( 'NONE',  ( -1.469816272965878357, -0.5023911411419708095, -0.1820866141732282451 ) ) ;
#66611=CARTESIAN_POINT ( 'NONE',  ( -1.240157480314959759, 0.1660481256975885056, 0.3530559997133364547 ) ) ;
#66612=CARTESIAN_POINT ( 'NONE',  ( 0.5380577427821529035, -0.4281496062992124485, 0.4176697321401328655 ) ) ;
#66613=CARTESIAN_POINT ( 'NONE',  ( 1.469816272965879911, -0.6046776061558807314, 0.2411417322834647770 ) ) ;
#66614=CARTESIAN_POINT ( 'NONE',  ( 2.795275590551181910, 1.568468489416428469, 0.000000000000000000 ) ) ;
#66615=CARTESIAN_POINT ( 'NONE',  ( 0.4527559055118117182, -0.5400638737290844871, 0.3530559997133364547 ) ) ;
#66617=CARTESIAN_POINT ( 'NONE',  ( 1.555118110236221041, 0.1660481256975883668, -0.3530559997133364547 ) ) ;
#66618=CARTESIAN_POINT ( 'NONE',  ( 1.082677165354331228, 0.1660481256975883668, -0.3530559997133364547 ) ) ;
#66619=CARTESIAN_POINT ( 'NONE',  ( -1.463254593175852492, -0.5511811023622048555, -0.09757992244046775898 ) ) ;
#66620=CARTESIAN_POINT ( 'NONE',  ( 1.227034120734908917, 0.1771653543307087075, -0.09757992244046823083 ) ) ;
#66621=CARTESIAN_POINT ( 'NONE',  ( -1.541994750656167090, -0.5511811023622048555, -0.09757992244046775898 ) ) ;
#66622=CARTESIAN_POINT ( 'NONE',  ( -0.8727034120734901146, -0.2845877964562159024, 0.3641732283464567677 ) ) ;
#66623=CARTESIAN_POINT ( 'NONE',  ( 1.502624671916010790, -0.3162353388693409650, -0.4822834645669289433 ) ) ;
#66624=CARTESIAN_POINT ( 'NONE',  ( 0.5708661417322841158, -0.4536011799217368745, -0.2665933059059886201 ) ) ;
#66625=CARTESIAN_POINT ( 'NONE',  ( 0.2624671916010504757, 0.2306618581243848609, 0.2411417322834645549 ) ) ;
#66626=CARTESIAN_POINT ( 'NONE',  ( 1.246719160104987623, -0.4281496062992124485, 0.4176697321401328655 ) ) ;
#66627=CARTESIAN_POINT ( 'NONE',  ( -0.5577427821522301654, -0.3162353388693405765, 0.4822834645669290543 ) ) ;
#66628=CARTESIAN_POINT ( 'NONE',  ( 0.2559055118110243332, -0.4536011799217368745, -0.2665933059059886201 ) ) ;
#66629=CARTESIAN_POINT ( 'NONE',  ( 1.167979002624672580, 0.05413385826771626580, -0.4176697321401330321 ) ) ;
#66631=CARTESIAN_POINT ( 'NONE',  ( -1.633858267716534529, 0.1660481256975885056, 0.3530559997133364547 ) ) ;
#66632=CARTESIAN_POINT ( 'NONE',  ( -0.8530183727034112984, -0.4281496062992127816, -0.4176697321401328100 ) ) ;
#66633=CARTESIAN_POINT ( 'NONE',  ( -1.456692913385826182, -0.5511811023622047445, 6.969142054262312111E-17 ) ) ;
#66636=CARTESIAN_POINT ( 'NONE',  ( -0.9317585301837263412, -0.4281496062992127816, -0.4176697321401328100 ) ) ;
#66637=AXIS2_PLACEMENT_3D ( 'NONE', #27849, #15653, #9327 ) ;
#66638=CARTESIAN_POINT ( 'NONE',  ( -0.05905511811023545637, -0.5400638737290845981, -0.3530559997133363437 ) ) ;
#66643=CARTESIAN_POINT ( 'NONE',  ( 0.8333333333333340365, -0.5511811023622046335, 0.09757992244046803654 ) ) ;
#66645=CARTESIAN_POINT ( 'NONE',  ( 1.141732283464567566, 0.2952755905511811885, 0.000000000000000000 ) ) ;
#66646=CARTESIAN_POINT ( 'NONE',  ( -1.646051170424378096, -0.1870078740157480046, 1.254653134982923898E-17 ) ) ;
#66647=ADVANCED_FACE ( 'NONE', ( #71906 ), #58909, .F. ) ;
#66648=CARTESIAN_POINT ( 'NONE',  ( -1.200787401574802349, 0.07958543189024071263, -0.2665933059059888421 ) ) ;
#66649=CARTESIAN_POINT ( 'NONE',  ( 1.410761154855643795, -0.05778040916215560624, -0.4822834645669293319 ) ) ;
#66650=CARTESIAN_POINT ( 'NONE',  ( -1.423884514435694859, -0.3162353388693405765, 0.4822834645669290543 ) ) ;
#66652=CARTESIAN_POINT ( 'NONE',  ( -0.1377952755905504645, -0.5400638737290845981, -0.3530559997133363437 ) ) ;
#66653=CARTESIAN_POINT ( 'NONE',  ( -0.4527559055118102749, 0.07958543189024085140, 0.2665933059059887866 ) ) ;
#66654=CARTESIAN_POINT ( 'NONE',  ( 0.7414698162729663755, -0.6692913385826773087, -0.1292274648535924053 ) ) ;
#66655=CARTESIAN_POINT ( 'NONE',  ( 0.3149606299212603933, -0.1870078740157479769, 0.4822834645669291653 ) ) ;
#66659=CARTESIAN_POINT ( 'NONE',  ( 0.7677165354330716118, 0.1660481256975883668, -0.3530559997133364547 ) ) ;
#66660=CARTESIAN_POINT ( 'NONE',  ( 0.01312335958005323398, 0.05413385826771666132, 0.4176697321401328100 ) ) ;
#66661=CARTESIAN_POINT ( 'NONE',  ( -1.049868766404198794, -0.6046776061558807314, 0.2411417322834647770 ) ) ;
#66662=CARTESIAN_POINT ( 'NONE',  ( 1.410761154855643795, -0.3162353388693405765, 0.4822834645669290543 ) ) ;
#66663=CARTESIAN_POINT ( 'NONE',  ( 1.010498687664042716, -0.4281496062992124485, 0.4176697321401328655 ) ) ;
#66665=CARTESIAN_POINT ( 'NONE',  ( -0.1706036745406816491, -0.4281496062992124485, 0.4176697321401328655 ) ) ;
#66666=CARTESIAN_POINT ( 'NONE',  ( 0.4658792650918641698, -0.05778040916215560624, -0.4822834645669293319 ) ) ;
#66667=CARTESIAN_POINT ( 'NONE',  ( -0.1049868766404193215, -0.6046776061558807314, 0.2411417322834647770 ) ) ;
#66668=CARTESIAN_POINT ( 'NONE',  ( 0.6561679790026253567, -0.5023911411419708095, -0.1820866141732282451 ) ) ;
#66669=CARTESIAN_POINT ( 'NONE',  ( -1.548556430446193399, 0.2306618581243848609, 0.2411417322834645549 ) ) ;
#66670=CARTESIAN_POINT ( 'NONE',  ( -1.587926509186350810, -0.4281496062992124485, 0.4176697321401328655 ) ) ;
#66671=CARTESIAN_POINT ( 'NONE',  ( 0.5511811023622054106, -0.1870078740157480879, -0.4822834645669291653 ) ) ;
#66673=EDGE_CURVE ( 'NONE', #44273, #81026, #16602, .T. ) ;
#66678=CARTESIAN_POINT ( 'NONE',  ( 1.213910761154856299, 0.2952755905511811885, 0.1292274648535926551 ) ) ;
#66679=CARTESIAN_POINT ( 'NONE',  ( 0.3543307086614179147, 0.1771653543307087630, 0.000000000000000000 ) ) ;
#66683=FACE_OUTER_BOUND ( 'NONE', #60220, .T. ) ;
#66687=CARTESIAN_POINT ( 'NONE',  ( -1.627296587926508442, 0.2306618581243848609, 0.2411417322834645549 ) ) ;
#66688=CARTESIAN_POINT ( 'NONE',  ( -0.4133858267716528645, 0.1660481256975883668, -0.3530559997133364547 ) ) ;
#66689=CARTESIAN_POINT ( 'NONE',  ( 1.227034120734908917, -0.6692913385826771977, 0.1292274648535927661 ) ) ;
#66691=CARTESIAN_POINT ( 'NONE',  ( 1.614173228346457378, 0.2952755905511811885, 0.000000000000000000 ) ) ;
#66692=CARTESIAN_POINT ( 'NONE',  ( 1.594488188976378673, -0.4536011799217368745, -0.2665933059059886201 ) ) ;
#66695=DIRECTION ( 'NONE',  ( 0.000000000000000000, 1.000000000000000000, 0.000000000000000000 ) ) ;
#66696=CARTESIAN_POINT ( 'NONE',  ( -1.266404199475064773, -0.08942795157528024563, -0.3641732283464568787 ) ) ;
#66697=ADVANCED_FACE ( 'NONE', ( #27174 ), #78548, .F. ) ;
#66698=CARTESIAN_POINT ( 'NONE',  ( 1.586052503253845503, 0.7480314960629931287, 0.1653254495020587966 ) ) ;
#66699=CARTESIAN_POINT ( 'NONE',  ( 0.01312335958005323398, -0.4281496062992127816, -0.4176697321401328100 ) ) ;
#66701=CARTESIAN_POINT ( 'NONE',  ( 1.430446194225722500, -0.4281496062992127816, -0.4176697321401328100 ) ) ;
#66703=CARTESIAN_POINT ( 'NONE',  ( -0.8989501312335946848, 0.1771653543307087075, -0.09757992244046823083 ) ) ;
#66704=CARTESIAN_POINT ( 'NONE',  ( 0.6496062992125991586, -0.5400638737290845981, -0.3530559997133363437 ) ) ;
#66705=CARTESIAN_POINT ( 'NONE',  ( 1.227034120734908917, -0.5511811023622046335, 0.09757992244046803654 ) ) ;
#66707=CARTESIAN_POINT ( 'NONE',  ( -0.7086614173228339419, -0.1870078740157480601, -0.3641732283464567677 ) ) ;
#66708=CARTESIAN_POINT ( 'NONE',  ( 1.207349081364829990, 0.2306618581243848609, 0.2411417322834645549 ) ) ;
#66710=CARTESIAN_POINT ( 'NONE',  ( 0.3740157480314966754, 0.1660481256975883668, -0.3530559997133364547 ) ) ;
#66711=CARTESIAN_POINT ( 'NONE',  ( -0.7349081364829387342, -0.5023911411419708095, 0.1820866141732285504 ) ) ;
#66712=CARTESIAN_POINT ( 'NONE',  ( -0.4527559055118102749, 0.07958543189024085140, 0.2665933059059887866 ) ) ;
#66713=CARTESIAN_POINT ( 'NONE',  ( -0.2624671916010490880, 0.2306618581243847221, -0.2411417322834647770 ) ) ;
#66714=CARTESIAN_POINT ( 'NONE',  ( -1.482939632545930975, -0.004921259842519576551, 0.3153832671262227771 ) ) ;
#66716=CARTESIAN_POINT ( 'NONE',  ( 0.6758530183727039509, 0.2952755905511810774, -0.1292274648535930714 ) ) ;
#66719=CARTESIAN_POINT ( 'NONE',  ( -0.9055118110236215490, 0.2952755905511811885, 0.000000000000000000 ) ) ;
#66720=CARTESIAN_POINT ( 'NONE',  ( -0.03937007874015669567, -0.5511811023622047445, 6.969142054262312111E-17 ) ) ;
#66721=CARTESIAN_POINT ( 'NONE',  ( -1.450131233595799651, 0.2952755905511810774, -0.1292274648535930714 ) ) ;
#66722=CARTESIAN_POINT ( 'NONE',  ( 0.4855643044619430415, -0.3690944881889765550, -0.3153832671262227771 ) ) ;
#66723=CARTESIAN_POINT ( 'NONE',  ( -0.5380577427821514602, -0.3690944881889765550, -0.3153832671262227771 ) ) ;
#66724=CARTESIAN_POINT ( 'NONE',  ( -0.9383202099737524282, -0.05778040916215522460, 0.4822834645669289988 ) ) ;
#66725=CARTESIAN_POINT ( 'NONE',  ( -1.515748031496062076, 0.1660481256975883668, -0.3530559997133364547 ) ) ;
#66726=CARTESIAN_POINT ( 'NONE',  ( 1.207349081364829990, 0.2306618581243848609, 0.2411417322834645549 ) ) ;
#66727=DIRECTION ( 'NONE',  ( -0.000000000000000000, 1.000000000000000000, -0.000000000000000000 ) ) ;
#66728=CARTESIAN_POINT ( 'NONE',  ( 0.8530183727034128527, -0.3690944881889763329, 0.3153832671262228327 ) ) ;
#66729=CARTESIAN_POINT ( 'NONE',  ( 0.5774278215223104249, 0.2306618581243848609, 0.2411417322834645549 ) ) ;
#66730=LINE ( 'NONE', #31189, #12490 ) ;
#66731=CARTESIAN_POINT ( 'NONE',  ( 1.338582677165355062, -0.1870078740157480601, -0.3641732283464567677 ) ) ;
#66732=ORIENTED_EDGE ( 'NONE', *, *, #70646, .T. ) ;
#66734=CARTESIAN_POINT ( 'NONE',  ( -1.207349081364828436, -0.5023911411419708095, 0.1820866141732285504 ) ) ;
#66735=CARTESIAN_POINT ( 'NONE',  ( -0.3018372703412066094, -0.4281496062992127816, -0.4176697321401328100 ) ) ;
#66736=CARTESIAN_POINT ( 'NONE',  ( 0.3674540682414705883, 0.2306618581243847221, -0.2411417322834647770 ) ) ;
#66738=CARTESIAN_POINT ( 'NONE',  ( -1.397637795275589623, 0.07958543189024085140, 0.2665933059059887866 ) ) ;
#66740=CARTESIAN_POINT ( 'NONE',  ( -1.443569553805773564, -0.6046776061558807314, 0.2411417322834647770 ) ) ;
#66743=CARTESIAN_POINT ( 'NONE',  ( 0.6036745406824154392, 0.2306618581243847221, -0.2411417322834647770 ) ) ;
#66744=CARTESIAN_POINT ( 'NONE',  ( 0.01968503937007957949, -0.5400638737290845981, -0.3530559997133363437 ) ) ;
#66745=CARTESIAN_POINT ( 'NONE',  ( 1.122047244094488860, 0.1660481256975885056, 0.3530559997133364547 ) ) ;
#66746=PLANE ( 'NONE',  #29162 ) ;
#66753=CARTESIAN_POINT ( 'NONE',  ( -0.06561679790026180015, -0.3690944881889765550, -0.3153832671262227771 ) ) ;
#66754=CARTESIAN_POINT ( 'NONE',  ( -0.4921259842519677963, -0.5400638737290844871, 0.3530559997133364547 ) ) ;
#66755=CARTESIAN_POINT ( 'NONE',  ( 0.8923884514435701520, -0.6046776061558809534, -0.2411417322834644161 ) ) ;
#66757=CARTESIAN_POINT ( 'NONE',  ( -0.1706036745406816491, -0.004921259842519870586, -0.3153832671262229437 ) ) ;
#66758=CARTESIAN_POINT ( 'NONE',  ( -0.9514435695538050464, -0.05778040916215560624, -0.4822834645669293319 ) ) ;
#66759=CARTESIAN_POINT ( 'NONE',  ( 1.489501312335958172, -0.05778040916215560624, -0.4822834645669293319 ) ) ;
#66763=ORIENTED_EDGE ( 'NONE', *, *, #82446, .F. ) ;
#66765=CARTESIAN_POINT ( 'NONE',  ( 0.9842519685039375910, 0.2952755905511811885, 0.000000000000000000 ) ) ;
#66766=CARTESIAN_POINT ( 'NONE',  ( 1.496062992125984703, -0.1870078740157480601, -0.3641732283464567677 ) ) ;
#66767=CARTESIAN_POINT ( 'NONE',  ( -1.062992125984250968, -0.5511811023622047445, 6.969142054262312111E-17 ) ) ;
#66768=CARTESIAN_POINT ( 'NONE',  ( -1.128608923884513837, 0.2306618581243847221, -0.2411417322834647770 ) ) ;
#66770=CARTESIAN_POINT ( 'NONE',  ( -1.010849322905837955, 0.004960608223778821026, 0.3437734562760189072 ) ) ;
#66771=CARTESIAN_POINT ( 'NONE',  ( 1.292650918635171564, -0.6692913385826773087, -0.1292274648535924053 ) ) ;
#66772=CARTESIAN_POINT ( 'NONE',  ( -1.581364829396324945, -0.3162353388693405765, 0.4822834645669290543 ) ) ;
#66773=CARTESIAN_POINT ( 'NONE',  ( 0.09186351706036799403, -0.4281496062992127816, -0.4176697321401328100 ) ) ;
#66774=CARTESIAN_POINT ( 'NONE',  ( 0.05249343832021075018, 0.2306618581243847221, -0.2411417322834647770 ) ) ;
#66775=CARTESIAN_POINT ( 'NONE',  ( -1.108923884514435132, -0.05778040916215560624, -0.4822834645669293319 ) ) ;
#66777=CARTESIAN_POINT ( 'NONE',  ( 0.3871391076115492380, -0.05778040916215560624, -0.4822834645669293319 ) ) ;
#66779=CARTESIAN_POINT ( 'NONE',  ( -1.108923884514435132, -0.08942795157528024563, -0.3641732283464568787 ) ) ;
#66780=VERTEX_POINT ( 'NONE', #41473 ) ;
#66783=CARTESIAN_POINT ( 'NONE',  ( 1.595398199321655275, 1.288687073698532526, 0.1559797534342495240 ) ) ;
#66784=CARTESIAN_POINT ( 'NONE',  ( -1.417322834645668772, -0.1870078740157479769, 0.4822834645669291653 ) ) ;
#66785=CARTESIAN_POINT ( 'NONE',  ( -1.522309711286088607, -0.6046776061558807314, 0.2411417322834647770 ) ) ;
#66787=CARTESIAN_POINT ( 'NONE',  ( -1.430446194225721390, -0.4281496062992124485, 0.4176697321401328655 ) ) ;
#66788=CARTESIAN_POINT ( 'NONE',  ( -1.522309711286088607, 0.2306618581243847221, -0.2411417322834647770 ) ) ;
#66790=DIRECTION ( 'NONE',  ( 0.000000000000000000, 1.000000000000000000, 0.000000000000000000 ) ) ;
#66792=CARTESIAN_POINT ( 'NONE',  ( -0.3018372703412066094, -0.3690944881889765550, -0.3153832671262227771 ) ) ;
#66793=CARTESIAN_POINT ( 'NONE',  ( -0.6430446194225716283, -0.3690944881889763329, 0.3153832671262228327 ) ) ;
#66794=CARTESIAN_POINT ( 'NONE',  ( -1.338582677165353729, -0.1870078740157479769, 0.4822834645669291653 ) ) ;
#66795=CARTESIAN_POINT ( 'NONE',  ( 0.9842519685039375910, 0.2952755905511811885, 0.000000000000000000 ) ) ;
#66796=CARTESIAN_POINT ( 'NONE',  ( -1.056430446194224881, -0.6692913385826771977, 0.1292274648535927661 ) ) ;
#66798=ORIENTED_EDGE ( 'NONE', *, *, #75407, .F. ) ;
#66799=CARTESIAN_POINT ( 'NONE',  ( -1.338582677165353729, -0.1870078740157479769, 0.4822834645669291653 ) ) ;
#66801=CARTESIAN_POINT ( 'NONE',  ( -1.686351706036744558, 0.2952755905511810774, -0.1292274648535930714 ) ) ;
#66807=CARTESIAN_POINT ( 'NONE',  ( -0.3543307086614165824, 0.2952755905511811885, 0.000000000000000000 ) ) ;
#66808=CARTESIAN_POINT ( 'NONE',  ( 1.272965879265092637, -0.4281496062992127816, -0.4176697321401328100 ) ) ;
#66811=CARTESIAN_POINT ( 'NONE',  ( -1.220472440944882386, 0.000000000000000000, -0.4445507791589061175 ) ) ;
#66813=CARTESIAN_POINT ( 'NONE',  ( -1.233595800524933894, 0.2306618581243848609, 0.2411417322834645549 ) ) ;
#66814=CARTESIAN_POINT ( 'NONE',  ( -0.9383202099737524282, -0.05778040916215522460, 0.4822834645669289988 ) ) ;
#66816=CARTESIAN_POINT ( 'NONE',  ( 0.3608923884514443348, 0.1771653543307087075, -0.09757992244046823083 ) ) ;
#66818=CARTESIAN_POINT ( 'NONE',  ( 0.5118110236220480003, -0.5511811023622047445, 6.969142054262312111E-17 ) ) ;
#66819=CARTESIAN_POINT ( 'NONE',  ( 0.9251968503937015864, -0.4536011799217367080, 0.2665933059059888421 ) ) ;
#66820=CARTESIAN_POINT ( 'NONE',  ( 0.9711286089238851948, 0.2306618581243848609, 0.2411417322834645549 ) ) ;
#66821=CARTESIAN_POINT ( 'NONE',  ( -0.1443569553805765515, -0.3690944881889765550, -0.3153832671262227771 ) ) ;
#66823=CARTESIAN_POINT ( 'NONE',  ( -1.167979002624671470, 0.05413385826771666132, 0.4176697321401328100 ) ) ;
#66824=CARTESIAN_POINT ( 'NONE',  ( -0.1574803149606292529, -0.1870078740157479769, 0.3641732283464567677 ) ) ;
#66825=CARTESIAN_POINT ( 'NONE',  ( -1.292650918635170010, 0.1771653543307087075, -0.09757992244046823083 ) ) ;
#66827=CARTESIAN_POINT ( 'NONE',  ( -0.8792650918635160906, -0.3690944881889763329, 0.3153832671262228327 ) ) ;
#66828=CARTESIAN_POINT ( 'NONE',  ( -0.1837270341207340729, 0.2306618581243847221, -0.2411417322834647770 ) ) ;
#66830=CARTESIAN_POINT ( 'NONE',  ( 0.3280839895013130669, -0.004921259842519576551, 0.3153832671262227771 ) ) ;
#66831=CARTESIAN_POINT ( 'NONE',  ( -0.3477690288713905509, -0.5511811023622046335, 0.09757992244046803654 ) ) ;
#66832=CARTESIAN_POINT ( 'NONE',  ( -0.8661417322834640276, -0.1870078740157479769, 0.4822834645669291653 ) ) ;
#66835=CARTESIAN_POINT ( 'NONE',  ( 0.6167979002624679463, 0.05413385826771626580, -0.4176697321401330321 ) ) ;
#66837=CARTESIAN_POINT ( 'NONE',  ( 1.443569553805774897, 0.2306618581243848609, 0.2411417322834645549 ) ) ;
#66838=CARTESIAN_POINT ( 'NONE',  ( -0.4002624671916004129, -0.08942795157528024563, -0.3641732283464568787 ) ) ;
#66839=CARTESIAN_POINT ( 'NONE',  ( -0.1640419947506555343, -0.3162353388693405765, 0.4822834645669290543 ) ) ;
#66840=CARTESIAN_POINT ( 'NONE',  ( -1.351706036745406347, -0.4281496062992124485, 0.4176697321401328655 ) ) ;
#66841=CARTESIAN_POINT ( 'NONE',  ( 1.692913385826772421, 0.2952755905511811885, 0.000000000000000000 ) ) ;
#66842=CARTESIAN_POINT ( 'NONE',  ( 1.207349081364829990, 0.2306618581243848609, 0.2411417322834645549 ) ) ;
#66843=CARTESIAN_POINT ( 'NONE',  ( -0.4986876640419942164, -0.5023911411419708095, 0.1820866141732285504 ) ) ;
#66845=EDGE_CURVE ( 'NONE', #50773, #39166, #65516, .T. ) ;
#66849=CARTESIAN_POINT ( 'NONE',  ( 1.338582677165355062, -0.1870078740157480601, -0.3641732283464567677 ) ) ;
#66850=CARTESIAN_POINT ( 'NONE',  ( -1.574803149606298636, -0.1870078740157479769, 0.4822834645669291653 ) ) ;
#66852=CARTESIAN_POINT ( 'NONE',  ( 1.003937007874016185, 0.1660481256975883668, -0.3530559997133364547 ) ) ;
#66854=CARTESIAN_POINT ( 'NONE',  ( 1.194225721784777594, -0.004921259842519576551, 0.3153832671262227771 ) ) ;
#66855=CARTESIAN_POINT ( 'NONE',  ( -0.03937007874015669567, 0.2952755905511811885, 0.000000000000000000 ) ) ;
#66856=CARTESIAN_POINT ( 'NONE',  ( -0.3674540682414689785, 0.2306618581243848609, 0.2411417322834645549 ) ) ;
#66862=CARTESIAN_POINT ( 'NONE',  ( 0.2821522309711292364, -0.5511811023622046335, 0.09757992244046803654 ) ) ;
#66863=EDGE_LOOP ( 'NONE', ( #27744, #27609, #55029, #31338 ) ) ;
#66866=CARTESIAN_POINT ( 'NONE',  ( -0.2296587926509179312, -0.3162353388693409650, -0.4822834645669289433 ) ) ;
#66867=CARTESIAN_POINT ( 'NONE',  ( 1.410761154855643795, -0.3162353388693405765, 0.4822834645669290543 ) ) ;
#66868=CARTESIAN_POINT ( 'NONE',  ( 0.2165354330708668673, -0.5400638737290844871, 0.3530559997133364547 ) ) ;
#66869=CARTESIAN_POINT ( 'NONE',  ( -0.4330708661417315697, -0.5511811023622047445, 6.969142054262312111E-17 ) ) ;
#66870=CARTESIAN_POINT ( 'NONE',  ( 0.7480314960629927956, 0.2952755905511811885, 0.000000000000000000 ) ) ;
#66871=CARTESIAN_POINT ( 'NONE',  ( -1.010498687664041384, 0.05413385826771666132, 0.4176697321401328100 ) ) ;
#66872=CARTESIAN_POINT ( 'NONE',  ( -0.2952755905511804668, 0.1660481256975885056, 0.3530559997133364547 ) ) ;
#66873=CARTESIAN_POINT ( 'NONE',  ( -0.8792650918635160906, 0.05413385826771626580, -0.4176697321401330321 ) ) ;
#66874=CARTESIAN_POINT ( 'NONE',  ( 1.292650918635171564, 0.2952755905511811885, 0.1292274648535926551 ) ) ;
#66875=CARTESIAN_POINT ( 'NONE',  ( 0.7677165354330716118, -0.5400638737290844871, 0.3530559997133364547 ) ) ;
#66876=CARTESIAN_POINT ( 'NONE',  ( 0.7349081364829403995, 0.2306618581243848609, 0.2411417322834645549 ) ) ;
#66878=CARTESIAN_POINT ( 'NONE',  ( -0.1246719160104980823, -0.5511811023622048555, -0.09757992244046775898 ) ) ;
#66879=ORIENTED_EDGE ( 'NONE', *, *, #74381, .T. ) ;
#66882=CARTESIAN_POINT ( 'NONE',  ( -0.8464566929133852113, -0.4536011799217368745, -0.2665933059059886201 ) ) ;
#66883=CARTESIAN_POINT ( 'NONE',  ( 0.1049868766404206816, 0.2306618581243848609, 0.2411417322834645549 ) ) ;
#66885=CARTESIAN_POINT ( 'NONE',  ( -0.4002624671916004129, -0.05778040916215560624, -0.4822834645669293319 ) ) ;
#66886=CARTESIAN_POINT ( 'NONE',  ( -0.4658792650918627265, -0.05778040916215522460, 0.4822834645669289988 ) ) ;
#66887=CARTESIAN_POINT ( 'NONE',  ( -1.286089238845143479, 0.2306618581243847221, -0.2411417322834647770 ) ) ;
#66888=CARTESIAN_POINT ( 'NONE',  ( -1.351706036745406347, 0.05413385826771626580, -0.4176697321401330321 ) ) ;
#66889=CARTESIAN_POINT ( 'NONE',  ( 0.7808398950131241190, -0.08942795157528024563, -0.3641732283464568787 ) ) ;
#66892=CARTESIAN_POINT ( 'NONE',  ( 0.3871391076115492380, -0.08942795157528024563, -0.3641732283464568787 ) ) ;
#66893=CARTESIAN_POINT ( 'NONE',  ( -0.05249343832020911260, 0.2306618581243848609, 0.2411417322834645549 ) ) ;
#66894=CARTESIAN_POINT ( 'NONE',  ( 0.4396325459317593221, 0.2952755905511810774, -0.1292274648535930714 ) ) ;
#66898=ORIENTED_EDGE ( 'NONE', *, *, #1215, .F. ) ;
#66901=CARTESIAN_POINT ( 'NONE',  ( -0.3937007874015740483, -0.1870078740157480879, -0.4822834645669291653 ) ) ;
#66904=CARTESIAN_POINT ( 'NONE',  ( 1.679790026246720025, 0.2306618581243848609, 0.2411417322834645549 ) ) ;
#66905=CARTESIAN_POINT ( 'NONE',  ( 0.8267716535433077274, 0.2952755905511811885, 0.000000000000000000 ) ) ;
#66906=CARTESIAN_POINT ( 'NONE',  ( 0.7611548556430454138, 0.2306618581243847221, -0.2411417322834647770 ) ) ;
#66907=CARTESIAN_POINT ( 'NONE',  ( -0.1312335958005241554, -0.5023911411419708095, -0.1820866141732282451 ) ) ;
#66908=CARTESIAN_POINT ( 'NONE',  ( -0.1377952755905504645, 0.1660481256975885056, 0.3530559997133364547 ) ) ;
#66910=CARTESIAN_POINT ( 'NONE',  ( -0.1181102362204717315, -0.5511811023622047445, 6.969142054262312111E-17 ) ) ;
#66911=CARTESIAN_POINT ( 'NONE',  ( -0.5905511811023615998, 0.2952755905511811885, 0.000000000000000000 ) ) ;
#66913=CARTESIAN_POINT ( 'NONE',  ( -1.712598425196849572, 0.1660481256975885056, 0.3530559997133364547 ) ) ;
#66914=CARTESIAN_POINT ( 'NONE',  ( -0.02624671916010428221, -0.5023911411419708095, 0.1820866141732285504 ) ) ;
#66915=CARTESIAN_POINT ( 'NONE',  ( 1.476377952755906442, -0.4536011799217367080, 0.2665933059059888421 ) ) ;
#66916=CARTESIAN_POINT ( 'NONE',  ( -1.128608923884513837, -0.6046776061558807314, 0.2411417322834647770 ) ) ;
#66917=CARTESIAN_POINT ( 'NONE',  ( -0.7808398950131222316, -0.2845877964562161244, -0.3641732283464567121 ) ) ;
#66918=CARTESIAN_POINT ( 'NONE',  ( -1.036041590146031366, -2.613618158232546091E-15, -0.3464511005275220379 ) ) ;
#66919=CARTESIAN_POINT ( 'NONE',  ( -1.259842519685038686, -0.1870078740157479769, 0.4822834645669291653 ) ) ;
#66920=CARTESIAN_POINT ( 'NONE',  ( 0.07217847769028949700, -0.3162353388693405765, 0.4822834645669290543 ) ) ;
#66925=CARTESIAN_POINT ( 'NONE',  ( 0.4921259842519691285, -0.4536011799217368745, -0.2665933059059886201 ) ) ;
#66926=CARTESIAN_POINT ( 'NONE',  ( 0.8398950131233602345, 0.2306618581243847221, -0.2411417322834647770 ) ) ;
#66927=CARTESIAN_POINT ( 'NONE',  ( -1.292650918635170010, -0.5511811023622046335, 0.09757992244046803654 ) ) ;
#66928=CARTESIAN_POINT ( 'NONE',  ( 1.272965879265092637, -0.4281496062992127816, -0.4176697321401328100 ) ) ;
#66929=CARTESIAN_POINT ( 'NONE',  ( -1.463254593175852492, -0.5511811023622048555, -0.09757992244046775898 ) ) ;
#66930=CARTESIAN_POINT ( 'NONE',  ( -0.5643044619422565855, 0.05413385826771626580, -0.4176697321401330321 ) ) ;
#66931=CARTESIAN_POINT ( 'NONE',  ( 0.2034120734908144990, -0.5511811023622046335, 0.09757992244046803654 ) ) ;
#66932=CARTESIAN_POINT ( 'NONE',  ( 1.363814626685862175, 0.1354692512615924549, -0.3875633260700433458 ) ) ;
#66933=CARTESIAN_POINT ( 'NONE',  ( 0.6561679790026253567, 0.1283753931104748280, 0.1820866141732283561 ) ) ;
#66934=CARTESIAN_POINT ( 'NONE',  ( -0.05905511811023545637, 0.1660481256975885056, 0.3530559997133364547 ) ) ;
#66937=CARTESIAN_POINT ( 'NONE',  ( -0.5643044619422565855, 0.05413385826771626580, -0.4176697321401330321 ) ) ;
#66939=CARTESIAN_POINT ( 'NONE',  ( 0.9120734908136489683, -0.5511811023622046335, 0.09757992244046803654 ) ) ;
#66940=CARTESIAN_POINT ( 'NONE',  ( -0.006561679790025524116, -0.05778040916215560624, -0.4822834645669293319 ) ) ;
#66941=CARTESIAN_POINT ( 'NONE',  ( -0.3018372703412066094, -0.4281496062992127816, -0.4176697321401328100 ) ) ;
#66942=CARTESIAN_POINT ( 'NONE',  ( -0.4986876640419939388, 0.1283753931104746893, -0.1820866141732285504 ) ) ;
#66943=CARTESIAN_POINT ( 'NONE',  ( 0.9576546141020361169, 0.004960608223778963273, 0.3437734562760189072 ) ) ;
#66944=CARTESIAN_POINT ( 'NONE',  ( -0.6430446194225712953, -0.004921259842519870586, -0.3153832671262229437 ) ) ;
#66945=CARTESIAN_POINT ( 'NONE',  ( 0.4986876640419954376, -0.6046776061558809534, -0.2411417322834644161 ) ) ;
#66946=CARTESIAN_POINT ( 'NONE',  ( -0.8923884514435688198, 0.1283753931104746893, -0.1820866141732285504 ) ) ;
#66948=CARTESIAN_POINT ( 'NONE',  ( -1.167979002624671470, 0.05413385826771666132, 0.4176697321401328100 ) ) ;
#66949=CARTESIAN_POINT ( 'NONE',  ( -0.8558026128237093966, -1.094630224652485432E-15, 0.4281993546915541238 ) ) ;
#66951=CARTESIAN_POINT ( 'NONE',  ( -1.181102362204723644, -0.1870078740157480601, -0.3641732283464567677 ) ) ;
#66952=CARTESIAN_POINT ( 'NONE',  ( -0.2690288713910754526, 0.2952755905511810774, -0.1292274648535930714 ) ) ;
#66953=CARTESIAN_POINT ( 'NONE',  ( -1.712598425196849572, 0.1660481256975885056, 0.3530559997133364547 ) ) ;
#66954=CARTESIAN_POINT ( 'NONE',  ( -0.9842519685039360366, 0.2952755905511811885, 0.000000000000000000 ) ) ;
#66956=CARTESIAN_POINT ( 'NONE',  ( 1.515748031496063408, 0.1660481256975885056, 0.3530559997133364547 ) ) ;
#66957=CARTESIAN_POINT ( 'NONE',  ( 0.7349081364829403995, 0.2306618581243848609, 0.2411417322834645549 ) ) ;
#66958=CARTESIAN_POINT ( 'NONE',  ( -0.2821522309711278487, 0.2066929133858267931, 0.1054918080437490802 ) ) ;
#66960=CARTESIAN_POINT ( 'NONE',  ( -1.561679790026246017, 0.05413385826771666132, 0.4176697321401328100 ) ) ;
#66963=CARTESIAN_POINT ( 'NONE',  ( -0.5249343832020990641, 0.1283753931104748280, 0.1820866141732283561 ) ) ;
#66966=CARTESIAN_POINT ( 'NONE',  ( 0.6692913385826777528, 0.2952755905511811885, 0.000000000000000000 ) ) ;
#66967=CARTESIAN_POINT ( 'NONE',  ( 0.2165354330708668673, 0.1660481256975883668, -0.3530559997133364547 ) ) ;
#66968=CARTESIAN_POINT ( 'NONE',  ( -0.5314960629921250401, 0.1660481256975885056, 0.3530559997133364547 ) ) ;
#66969=CARTESIAN_POINT ( 'NONE',  ( 1.292650918635171564, -0.6692913385826773087, -0.1292274648535924053 ) ) ;
#66970=CARTESIAN_POINT ( 'NONE',  ( -1.450131233595799651, 0.1771653543307087075, -0.09757992244046823083 ) ) ;
#66972=CARTESIAN_POINT ( 'NONE',  ( 0.3149606299212606708, -0.1870078740157480879, -0.4822834645669291653 ) ) ;
#66973=CARTESIAN_POINT ( 'NONE',  ( -0.7414698162729651543, -0.6692913385826771977, 0.1292274648535927661 ) ) ;
#66975=CARTESIAN_POINT ( 'NONE',  ( -1.450131233595799651, 0.2952755905511810774, -0.1292274648535930714 ) ) ;
#66976=CARTESIAN_POINT ( 'NONE',  ( 1.306827173596997183, 0.000000000000000000, 0.4445507791589062285 ) ) ;
#66977=CARTESIAN_POINT ( 'NONE',  ( 0.9711286089238851948, -0.6046776061558809534, -0.2411417322834644161 ) ) ;
#66978=CARTESIAN_POINT ( 'NONE',  ( 1.430446194225722500, -0.3690944881889765550, -0.3153832671262227771 ) ) ;
#66981=CARTESIAN_POINT ( 'NONE',  ( -0.3280839895013117347, 0.05413385826771626580, -0.4176697321401330321 ) ) ;
#66982=VERTEX_POINT ( 'NONE', #30378 ) ;
#66984=CARTESIAN_POINT ( 'NONE',  ( 0.2559055118110243332, -0.4536011799217368745, -0.2665933059059886201 ) ) ;
#66985=CARTESIAN_POINT ( 'NONE',  ( -1.194225721784776262, 0.05413385826771626580, -0.4176697321401330321 ) ) ;
#66986=CARTESIAN_POINT ( 'NONE',  ( 0.9645669291338588858, 0.1660481256975885056, 0.3530559997133364547 ) ) ;
#66987=CARTESIAN_POINT ( 'NONE',  ( 0.7742782152230978099, -0.4281496062992124485, 0.4176697321401328655 ) ) ;
#66988=CARTESIAN_POINT ( 'NONE',  ( -0.05249343832020938322, -0.6046776061558809534, -0.2411417322834644161 ) ) ;
#66989=CARTESIAN_POINT ( 'NONE',  ( -0.8989501312335946848, -0.6692913385826771977, 0.1292274648535927661 ) ) ;
#66991=CARTESIAN_POINT ( 'NONE',  ( -1.443569553805773564, -0.6046776061558807314, 0.2411417322834647770 ) ) ;
#66992=CARTESIAN_POINT ( 'NONE',  ( -0.5577427821522301654, -0.3162353388693405765, 0.4822834645669290543 ) ) ;
#66993=CARTESIAN_POINT ( 'NONE',  ( -0.4658792650918627265, -0.2845877964562161244, -0.3641732283464567121 ) ) ;
#66994=CARTESIAN_POINT ( 'NONE',  ( 1.437007874015748810, -0.5400638737290845981, -0.3530559997133363437 ) ) ;
#66995=CARTESIAN_POINT ( 'NONE',  ( 1.522309711286089939, 0.2306618581243848609, 0.2411417322834645549 ) ) ;
#66996=CARTESIAN_POINT ( 'NONE',  ( -1.082677165354329896, 0.1660481256975885056, 0.3530559997133364547 ) ) ;
#66998=CARTESIAN_POINT ( 'NONE',  ( 0.7545931758530188826, -0.6692913385826771977, 0.1292274648535927661 ) ) ;
#67000=CARTESIAN_POINT ( 'NONE',  ( 0.4606732211678797317, 2.793565526369266028, -0.5309055118110236338 ) ) ;
#67001=CARTESIAN_POINT ( 'NONE',  ( -0.3083989501312330295, -0.3162353388693409650, -0.4822834645669289433 ) ) ;
#67002=CARTESIAN_POINT ( 'NONE',  ( -1.135170603674539924, 0.1771653543307087075, -0.09757992244046823083 ) ) ;
#67003=CARTESIAN_POINT ( 'NONE',  ( 1.003937007874016407, -0.4536011799217367080, 0.2665933059059888421 ) ) ;
#67005=CARTESIAN_POINT ( 'NONE',  ( 1.240157480314961314, 0.07958543189024071263, -0.2665933059059888421 ) ) ;
#67006=CARTESIAN_POINT ( 'NONE',  ( 0.7414698162729663755, -0.6692913385826773087, -0.1292274648535924053 ) ) ;
#67008=CARTESIAN_POINT ( 'NONE',  ( -0.2755905511811018171, 0.2952755905511811885, 0.000000000000000000 ) ) ;
#67010=CARTESIAN_POINT ( 'NONE',  ( 1.522309711286089939, -0.5023911411419708095, -0.1820866141732282451 ) ) ;
#67011=CARTESIAN_POINT ( 'NONE',  ( -0.6167979002624665030, 0.05413385826771666132, 0.4176697321401328100 ) ) ;
#67013=CARTESIAN_POINT ( 'NONE',  ( 1.384514435695538559, 0.2952755905511810774, -0.1292274648535930714 ) ) ;
#67014=CARTESIAN_POINT ( 'NONE',  ( 0.05249343832021075018, 0.2306618581243847221, -0.2411417322834647770 ) ) ;
#67015=CARTESIAN_POINT ( 'NONE',  ( 0.5052493438320218022, -0.5511811023622048555, -0.09757992244046775898 ) ) ;
#67017=CARTESIAN_POINT ( 'NONE',  ( 0.3083989501312343062, -0.08942795157528024563, -0.3641732283464568787 ) ) ;
#67018=CARTESIAN_POINT ( 'NONE',  ( -1.640419947506561060, 0.05413385826771666132, 0.4176697321401328100 ) ) ;
#67020=CARTESIAN_POINT ( 'NONE',  ( 0.7086614173228353852, -0.1870078740157479769, 0.4822834645669291653 ) ) ;
#67022=CARTESIAN_POINT ( 'NONE',  ( 1.620734908136483465, -0.5511811023622046335, 0.09757992244046803654 ) ) ;
#67024=CARTESIAN_POINT ( 'NONE',  ( -0.1640419947506555343, -0.2845877964562159024, 0.3641732283464567677 ) ) ;
#67025=CARTESIAN_POINT ( 'NONE',  ( 0.03280839895013198948, -0.6692913385826773087, -0.1292274648535924053 ) ) ;
#67027=CARTESIAN_POINT ( 'NONE',  ( 1.404199475065617708, -0.004921259842519870586, -0.3153832671262229437 ) ) ;
#67028=CARTESIAN_POINT ( 'NONE',  ( -1.351706036745406347, -0.004921259842519870586, -0.3153832671262229437 ) ) ;
#67029=CARTESIAN_POINT ( 'NONE',  ( -1.292650918635170010, -0.6692913385826771977, 0.1292274648535927661 ) ) ;
#67030=CARTESIAN_POINT ( 'NONE',  ( 0.6233595800524942554, -0.05778040916215560624, -0.4822834645669293319 ) ) ;
#67031=CARTESIAN_POINT ( 'NONE',  ( 1.108923884514436686, -0.3162353388693409650, -0.4822834645669289433 ) ) ;
#67032=DIRECTION ( 'NONE',  ( -0.2810846377148183417, 0.6785983445458432239, 0.6785983445458515506 ) ) ;
#67033=CARTESIAN_POINT ( 'NONE',  ( 0.7677165354330716118, -0.5400638737290844871, 0.3530559997133364547 ) ) ;
#67034=CARTESIAN_POINT ( 'NONE',  ( 1.430446194225722500, -0.4281496062992127816, -0.4176697321401328100 ) ) ;
#67035=CARTESIAN_POINT ( 'NONE',  ( 1.036745406824147731, 0.05413385826771666132, 0.4176697321401328100 ) ) ;
#67036=CARTESIAN_POINT ( 'NONE',  ( -1.706036745406823485, 0.1283753931104748280, 0.1820866141732283561 ) ) ;
#67037=CARTESIAN_POINT ( 'NONE',  ( 0.6692913385826778638, -0.5511811023622047445, 6.969142054262312111E-17 ) ) ;
#67038=CARTESIAN_POINT ( 'NONE',  ( 1.594488188976378673, -0.5400638737290845981, -0.3530559997133363437 ) ) ;
#67039=CARTESIAN_POINT ( 'NONE',  ( -0.9514435695538050464, -0.08942795157528024563, -0.3641732283464568787 ) ) ;
#67040=CARTESIAN_POINT ( 'NONE',  ( 0.4068241469816279987, -0.3690944881889765550, -0.3153832671262227771 ) ) ;
#67041=CARTESIAN_POINT ( 'NONE',  ( 0.08530183727034192087, -0.05778040916215522460, 0.4822834645669289988 ) ) ;
#67042=CARTESIAN_POINT ( 'NONE',  ( 0.7020997375328090762, -0.05778040916215560624, -0.4822834645669293319 ) ) ;
#67043=CARTESIAN_POINT ( 'NONE',  ( -0.1968503937007867743, 0.2952755905511811885, 0.000000000000000000 ) ) ;
#67044=CARTESIAN_POINT ( 'NONE',  ( 0.02624671916010564918, 0.1283753931104748280, 0.1820866141732283561 ) ) ;
#67045=CARTESIAN_POINT ( 'NONE',  ( 1.102362204724410155, -0.1870078740157479769, 0.4822834645669291653 ) ) ;
#67047=CARTESIAN_POINT ( 'NONE',  ( -1.089238845144356427, 0.05413385826771666132, 0.4176697321401328100 ) ) ;
#67051=CARTESIAN_POINT ( 'NONE',  ( -0.7349081364829387342, -0.6046776061558807314, 0.2411417322834647770 ) ) ;
#67052=CARTESIAN_POINT ( 'NONE',  ( -0.6102362204724400829, 0.1660481256975885056, 0.3530559997133364547 ) ) ;
#67055=ORIENTED_EDGE ( 'NONE', *, *, #28103, .T. ) ;
#67056=CARTESIAN_POINT ( 'NONE',  ( 0.6889763779527566800, -0.4536011799217367080, 0.2665933059059888421 ) ) ;
#67058=CARTESIAN_POINT ( 'NONE',  ( 1.095800524934383846, -0.3162353388693405765, 0.4822834645669290543 ) ) ;
#67059=CARTESIAN_POINT ( 'NONE',  ( -0.2481535038101752855, 4.694981358611540289E-15, -0.3627989612356130045 ) ) ;
#67060=CARTESIAN_POINT ( 'NONE',  ( -1.437007874015747477, -0.4536011799217367080, 0.2665933059059888421 ) ) ;
#67061=CARTESIAN_POINT ( 'NONE',  ( 1.660104986876641320, -0.05778040916215522460, 0.4822834645669289988 ) ) ;
#67063=CARTESIAN_POINT ( 'NONE',  ( -1.397637795275589623, 0.1660481256975885056, 0.3530559997133364547 ) ) ;
#67065=CARTESIAN_POINT ( 'NONE',  ( 0.1837270341207357105, -0.6046776061558809534, -0.2411417322834644161 ) ) ;
#67066=CARTESIAN_POINT ( 'NONE',  ( -0.2887139107611542133, 0.1283753931104748280, 0.1820866141732283561 ) ) ;
#67067=CARTESIAN_POINT ( 'NONE',  ( 0.9514435695538062676, -0.05778040916215522460, 0.4822834645669289988 ) ) ;
#67068=CARTESIAN_POINT ( 'NONE',  ( 0.01312335958005323398, 0.05413385826771666132, 0.4176697321401328100 ) ) ;
#67069=EDGE_CURVE ( 'NONE', #80835, #53475, #12648, .T. ) ;
#67070=CARTESIAN_POINT ( 'NONE',  ( 0.4986876640419954376, 0.2306618581243848609, 0.2411417322834645549 ) ) ;
#67073=CARTESIAN_POINT ( 'NONE',  ( 0.7349081364829403995, 0.2306618581243848609, 0.2411417322834645549 ) ) ;
#67074=CARTESIAN_POINT ( 'NONE',  ( 0.1115485564304467270, -0.6692913385826773087, -0.1292274648535924053 ) ) ;
#67075=CARTESIAN_POINT ( 'NONE',  ( -1.010498687664041384, 0.05413385826771666132, 0.4176697321401328100 ) ) ;
#67076=CARTESIAN_POINT ( 'NONE',  ( 1.076115485564305141, -0.6046776061558807314, 0.2411417322834647770 ) ) ;
#67077=CARTESIAN_POINT ( 'NONE',  ( 1.062992125984252745, 0.2952755905511811885, 0.000000000000000000 ) ) ;
#67079=CARTESIAN_POINT ( 'NONE',  ( -0.1968503937007867743, -0.6692913385826771977, 8.415575281601705876E-17 ) ) ;
#67080=CARTESIAN_POINT ( 'NONE',  ( 0.4527559055118117182, 0.1660481256975883668, -0.3530559997133364547 ) ) ;
#67081=CARTESIAN_POINT ( 'NONE',  ( 0.1049868766404206816, 0.2306618581243848609, 0.2411417322834645549 ) ) ;
#67082=CARTESIAN_POINT ( 'NONE',  ( 0.9055118110236227702, 0.1771653543307087630, 0.000000000000000000 ) ) ;
#67083=CARTESIAN_POINT ( 'NONE',  ( -1.187664041994750175, -0.05778040916215560624, -0.4822834645669293319 ) ) ;
#67085=CARTESIAN_POINT ( 'NONE',  ( 0.4068241469816279987, -0.4281496062992127816, -0.4176697321401328100 ) ) ;
#67087=B_SPLINE_CURVE_WITH_KNOTS ( 'NONE', 3,
 ( #77636, #20801, #1039, #40571 ),
 .UNSPECIFIED., .F., .F.,
 ( 4, 4 ),
 ( 0.000000000000000000, 0.001421551995671103573 ),
 .UNSPECIFIED. ) ;
#67091=ORIENTED_EDGE ( 'NONE', *, *, #37822, .T. ) ;
#67092=CARTESIAN_POINT ( 'NONE',  ( 1.089238845144357759, 0.05413385826771626580, -0.4176697321401330321 ) ) ;
#67093=CARTESIAN_POINT ( 'NONE',  ( 0.5183727034120741983, 0.1771653543307087075, -0.09757992244046823083 ) ) ;
#67095=CARTESIAN_POINT ( 'NONE',  ( 0.5643044619422579178, 0.05413385826771666132, 0.4176697321401328100 ) ) ;
#67096=ADVANCED_FACE ( 'NONE', ( #60413 ), #66746, .F. ) ;
#67100=CARTESIAN_POINT ( 'NONE',  ( -0.7677165354330699465, -0.5400638737290845981, -0.3530559997133363437 ) ) ;
#67101=CARTESIAN_POINT ( 'NONE',  ( -0.7349081364829390672, 0.2306618581243847221, -0.2411417322834647770 ) ) ;
#67102=CARTESIAN_POINT ( 'NONE',  ( 0.6955380577427828781, 0.05413385826771626580, -0.4176697321401330321 ) ) ;
#67103=ORIENTED_EDGE ( 'NONE', *, *, #18560, .T. ) ;
#67104=CARTESIAN_POINT ( 'NONE',  ( 1.397637795275591177, -0.5400638737290844871, 0.3530559997133364547 ) ) ;
#67105=CARTESIAN_POINT ( 'NONE',  ( 1.207349081364829990, 0.1539470093639523085, 0.1968503937007873850 ) ) ;
#67106=CARTESIAN_POINT ( 'NONE',  ( 1.535433070866142558, 0.1771653543307087630, 0.000000000000000000 ) ) ;
#67108=CARTESIAN_POINT ( 'NONE',  ( -1.450131233595799651, 0.1771653543307087075, -0.09757992244046823083 ) ) ;
#67110=CARTESIAN_POINT ( 'NONE',  ( 0.2165354330708668673, -0.5400638737290844871, 0.3530559997133364547 ) ) ;
#67111=CARTESIAN_POINT ( 'NONE',  ( 1.397637795275591177, 0.1660481256975883668, -0.3530559997133364547 ) ) ;
#67113=CARTESIAN_POINT ( 'NONE',  ( -1.017060367454067249, -0.2845877964562161244, -0.3641732283464567121 ) ) ;
#67114=CARTESIAN_POINT ( 'NONE',  ( 0.7611548556430454138, 0.2306618581243847221, -0.2411417322834647770 ) ) ;
#67115=CARTESIAN_POINT ( 'NONE',  ( 1.266404199475066328, -0.08942795157527998196, 0.3641732283464567121 ) ) ;
#67117=CARTESIAN_POINT ( 'NONE',  ( -0.9251968503937002541, 0.07958543189024085140, 0.2665933059059887866 ) ) ;
#67118=CARTESIAN_POINT ( 'NONE',  ( 1.476377952755906442, -0.5400638737290844871, 0.3530559997133364547 ) ) ;
#67120=CARTESIAN_POINT ( 'NONE',  ( -0.2755905511811018171, 0.2952755905511811885, 0.000000000000000000 ) ) ;
#67121=EDGE_CURVE ( 'NONE', #81558, #5170, #40186, .T. ) ;
#67122=CARTESIAN_POINT ( 'NONE',  ( -1.548556430446193399, -0.5023911411419708095, -0.1820866141732282451 ) ) ;
#67123=CARTESIAN_POINT ( 'NONE',  ( -0.2034120734908131112, -0.5511811023622048555, -0.09757992244046775898 ) ) ;
#67124=CARTESIAN_POINT ( 'NONE',  ( -0.1837270341207343505, -0.6046776061558807314, 0.2411417322834647770 ) ) ;
#67125=CARTESIAN_POINT ( 'NONE',  ( -1.430446194225720724, -0.004921259842519870586, -0.3153832671262229437 ) ) ;
#67127=CARTESIAN_POINT ( 'NONE',  ( 0.2887139107611556010, -0.6046776061558807314, 0.2411417322834647770 ) ) ;
#67128=CARTESIAN_POINT ( 'NONE',  ( 0.4037097067573611753, 1.223219560026271499E-15, 0.4445507791589056734 ) ) ;
#67130=CARTESIAN_POINT ( 'NONE',  ( -1.167979002624671470, -0.4281496062992127816, -0.4176697321401328100 ) ) ;
#67132=CARTESIAN_POINT ( 'NONE',  ( -0.03280839895013062252, -0.5511811023622046335, 0.09757992244046803654 ) ) ;
#67133=CARTESIAN_POINT ( 'NONE',  ( -1.496062992125983815, -0.1870078740157479769, 0.4822834645669291653 ) ) ;
#67134=CARTESIAN_POINT ( 'NONE',  ( 0.01968503937007957949, -0.5400638737290845981, -0.3530559997133363437 ) ) ;
#67135=CARTESIAN_POINT ( 'NONE',  ( 0.5971128608923891301, 0.1771653543307087075, -0.09757992244046823083 ) ) ;
#67136=CARTESIAN_POINT ( 'NONE',  ( -0.6692913385826764205, -0.5511811023622047445, 6.969142054262312111E-17 ) ) ;
#67137=CARTESIAN_POINT ( 'NONE',  ( -0.9317585301837263412, 0.05413385826771666132, 0.4176697321401328100 ) ) ;
#67138=CARTESIAN_POINT ( 'NONE',  ( -1.666666666666665853, 0.05413385826771626580, -0.4176697321401330321 ) ) ;
#67139=CARTESIAN_POINT ( 'NONE',  ( 1.469816272965879911, -0.6046776061558807314, 0.2411417322834647770 ) ) ;
#67141=CARTESIAN_POINT ( 'NONE',  ( 1.056430446194226658, 0.1771653543307087630, 0.09757992244046791164 ) ) ;
#67142=CARTESIAN_POINT ( 'NONE',  ( 0.7283464566929143125, 0.1660481256975885056, 0.3530559997133364547 ) ) ;
#67143=CARTESIAN_POINT ( 'NONE',  ( -1.614173228346457378, 0.7166040191147894367, 0.1372047244094476981 ) ) ;
#67144=CARTESIAN_POINT ( 'NONE',  ( 1.561679790026247350, -0.3690944881889763329, 0.3153832671262228327 ) ) ;
#67146=CARTESIAN_POINT ( 'NONE',  ( -0.8136482939632537770, 0.2306618581243847221, -0.2411417322834647770 ) ) ;
#67147=ADVANCED_FACE ( 'NONE', ( #49733 ), #34797, .F. ) ;
#67149=CARTESIAN_POINT ( 'NONE',  ( -1.391076115485563314, -0.5023911411419708095, -0.1820866141732282451 ) ) ;
#67150=CARTESIAN_POINT ( 'NONE',  ( -0.7283464566929126471, -0.5400638737290844871, 0.3530559997133364547 ) ) ;
#67151=CARTESIAN_POINT ( 'NONE',  ( 0.1443569553805781891, -0.4281496062992124485, 0.4176697321401328655 ) ) ;
#67152=CARTESIAN_POINT ( 'NONE',  ( -1.351706036745406347, -0.004921259842519870586, -0.3153832671262229437 ) ) ;
#67154=CARTESIAN_POINT ( 'NONE',  ( -1.338582677165353729, -0.1870078740157480879, -0.4822834645669291653 ) ) ;
#67155=CARTESIAN_POINT ( 'NONE',  ( 0.4855643044619430415, -0.4281496062992127816, -0.4176697321401328100 ) ) ;
#67156=CARTESIAN_POINT ( 'NONE',  ( 0.09842519685039434474, 0.1660481256975885056, 0.3530559997133364547 ) ) ;
#67157=CARTESIAN_POINT ( 'NONE',  ( 0.9514435695538062676, -0.05778040916215522460, 0.4822834645669289988 ) ) ;
#67158=DIRECTION ( 'NONE',  ( 3.386413887818973075E-16, -0.7071067811865519026, 0.7071067811865432429 ) ) ;
#67162=CARTESIAN_POINT ( 'NONE',  ( -1.604771003085130099, 1.002618919725274838, -0.1466069496707743947 ) ) ;
#67164=CARTESIAN_POINT ( 'NONE',  ( 0.006561679790026889343, -0.08942795157527998196, 0.3641732283464567121 ) ) ;
#67165=CARTESIAN_POINT ( 'NONE',  ( -0.3280839895013117347, -0.4281496062992124485, 0.4176697321401328655 ) ) ;
#67166=CARTESIAN_POINT ( 'NONE',  ( 0.7808398950131240079, -0.3162353388693405765, 0.4822834645669290543 ) ) ;
#67168=CARTESIAN_POINT ( 'NONE',  ( -0.1443569553805765515, -0.3690944881889765550, -0.3153832671262227771 ) ) ;
#67170=CARTESIAN_POINT ( 'NONE',  ( -1.122047244094487306, 0.1660481256975883668, -0.3530559997133364547 ) ) ;
#67171=CARTESIAN_POINT ( 'NONE',  ( 1.233595800524935227, -0.6046776061558807314, 0.2411417322834647770 ) ) ;
#67174=CARTESIAN_POINT ( 'NONE',  ( 1.113948071074811752, 0.02791078216816225699, 0.4328096321851905293 ) ) ;
#67177=CARTESIAN_POINT ( 'NONE',  ( 1.174540682414699111, -0.05778040916215560624, -0.4822834645669293319 ) ) ;
#67178=CARTESIAN_POINT ( 'NONE',  ( 1.574803149606299746, -0.1870078740157479769, 0.3641732283464567677 ) ) ;
#67179=CARTESIAN_POINT ( 'NONE',  ( -0.9973753280839886548, 0.1283753931104748280, 0.1820866141732283561 ) ) ;
#67180=CARTESIAN_POINT ( 'NONE',  ( -0.9645669291338575535, 0.1660481256975883668, -0.3530559997133364547 ) ) ;
#67182=CARTESIAN_POINT ( 'NONE',  ( 1.135170603674541256, -0.6692913385826773087, -0.1292274648535924053 ) ) ;
#67184=CARTESIAN_POINT ( 'NONE',  ( 0.06561679790026316017, 0.05413385826771626580, -0.4176697321401330321 ) ) ;
#67185=CARTESIAN_POINT ( 'NONE',  ( -0.4002624671916004129, -0.05778040916215560624, -0.4822834645669293319 ) ) ;
#67186=CARTESIAN_POINT ( 'NONE',  ( -1.548556430446193399, -0.6046776061558809534, -0.2411417322834644161 ) ) ;
#67188=CARTESIAN_POINT ( 'NONE',  ( 0.3805774278215230400, 0.05413385826771626580, -0.4176697321401330321 ) ) ;
#67190=CARTESIAN_POINT ( 'NONE',  ( -1.417322834645668772, -0.1870078740157480601, -0.3641732283464567677 ) ) ;
#67195=CARTESIAN_POINT ( 'NONE',  ( -1.423884514435694859, -0.3162353388693405765, 0.4822834645669290543 ) ) ;
#67197=CARTESIAN_POINT ( 'NONE',  ( -1.417322834645668772, -0.1870078740157479769, 0.4822834645669291653 ) ) ;
#67200=CARTESIAN_POINT ( 'NONE',  ( -0.3608923884514428360, 0.2952755905511811885, 0.1292274648535926551 ) ) ;
#67202=CARTESIAN_POINT ( 'NONE',  ( -0.4002624671916004129, -0.2845877964562159024, 0.3641732283464567677 ) ) ;
#67203=CARTESIAN_POINT ( 'NONE',  ( -0.9645669291338575535, -0.4536011799217367080, 0.2665933059059888421 ) ) ;
#67204=CARTESIAN_POINT ( 'NONE',  ( -1.213910761154854745, -0.6692913385826771977, 0.1292274648535927661 ) ) ;
#67205=CARTESIAN_POINT ( 'NONE',  ( 0.6955380577427828781, 0.05413385826771626580, -0.4176697321401330321 ) ) ;
#67206=CARTESIAN_POINT ( 'NONE',  ( -0.8530183727034112984, 0.05413385826771666132, 0.4176697321401328100 ) ) ;
#67208=ORIENTED_EDGE ( 'NONE', *, *, #74915, .T. ) ;
#67209=CARTESIAN_POINT ( 'NONE',  ( -1.200787401574802349, -0.5400638737290844871, 0.3530559997133364547 ) ) ;
#67213=CARTESIAN_POINT ( 'NONE',  ( -0.7426113562972000981, 2.362204724409448620, -0.5309055118110235227 ) ) ;
#67216=CARTESIAN_POINT ( 'NONE',  ( -0.7480314960629914633, -0.6692913385826771977, 8.415575281601705876E-17 ) ) ;
#67217=CARTESIAN_POINT ( 'NONE',  ( 1.338582677165355062, -0.1870078740157479769, 0.4822834645669291653 ) ) ;
#67219=CARTESIAN_POINT ( 'NONE',  ( 0.7210809602247731931, 4.888820689338890882E-16, 0.3464511005275202615 ) ) ;
#67222=CARTESIAN_POINT ( 'NONE',  ( -1.358267716535432434, 0.1660481256975883668, -0.3530559997133364547 ) ) ;
#67223=CARTESIAN_POINT ( 'NONE',  ( -0.9448818897637790704, -0.1870078740157479769, 0.4822834645669291653 ) ) ;
#67225=B_SPLINE_CURVE_WITH_KNOTS ( 'NONE', 3,
 ( #55674, #50189, #61173, #75886, #16582, #42227, #80973 ),
 .UNSPECIFIED., .F., .F.,
 ( 4, 3, 4 ),
 ( 5.204170427930420513E-18, 0.001246230184515574775, 0.002492489877932649832 ),
 .UNSPECIFIED. ) ;
#67226=CARTESIAN_POINT ( 'NONE',  ( 0.3149606299212603933, -0.1870078740157479769, 0.3641732283464567677 ) ) ;
#67229=CARTESIAN_POINT ( 'NONE',  ( 0.2559055118110243332, 0.07958543189024085140, 0.2665933059059887866 ) ) ;
#67230=CARTESIAN_POINT ( 'NONE',  ( 1.135170603674541256, 0.1771653543307087630, 0.09757992244046791164 ) ) ;
#67231=CARTESIAN_POINT ( 'NONE',  ( 0.8923884514435701520, -0.6046776061558809534, -0.2411417322834644161 ) ) ;
#67232=CARTESIAN_POINT ( 'NONE',  ( -0.2230971128608915943, -0.004921259842519576551, 0.3153832671262227771 ) ) ;
#67234=CARTESIAN_POINT ( 'NONE',  ( -1.607611548556429737, 0.2952755905511810774, -0.1292274648535930714 ) ) ;
#67235=CARTESIAN_POINT ( 'NONE',  ( -1.240157480314959759, -0.4536011799217368745, -0.2665933059059886201 ) ) ;
#67237=CARTESIAN_POINT ( 'NONE',  ( -0.9186351706036736120, -0.5023911411419708095, -0.1820866141732282451 ) ) ;
#67238=CARTESIAN_POINT ( 'NONE',  ( -0.07874015748031421014, -0.1870078740157479769, 0.4822834645669291653 ) ) ;
#67240=CARTESIAN_POINT ( 'NONE',  ( 0.7020997375328090762, -0.08942795157528024563, -0.3641732283464568787 ) ) ;
#67241=CARTESIAN_POINT ( 'NONE',  ( -0.06561679790026180015, -0.3690944881889765550, -0.3153832671262227771 ) ) ;
#67242=CARTESIAN_POINT ( 'NONE',  ( -0.9186351706036736120, -0.6046776061558809534, -0.2411417322834644161 ) ) ;
#67243=LINE ( 'NONE', #28097, #57322 ) ;
#67245=CARTESIAN_POINT ( 'NONE',  ( 0.2427821522309719648, -0.05778040916215522460, 0.4822834645669289988 ) ) ;
#67248=CARTESIAN_POINT ( 'NONE',  ( 1.463254593175853824, 0.2952755905511810774, -0.1292274648535930714 ) ) ;
#67249=CARTESIAN_POINT ( 'NONE',  ( -0.4068241469816267775, -0.004921259842519870586, -0.3153832671262229437 ) ) ;
#67250=CARTESIAN_POINT ( 'NONE',  ( -0.2296587926509179312, -0.3162353388693409650, -0.4822834645669289433 ) ) ;
#67251=CARTESIAN_POINT ( 'NONE',  ( -1.541994750656167090, -0.6692913385826773087, -0.1292274648535924053 ) ) ;
#67252=CARTESIAN_POINT ( 'NONE',  ( 1.496062992125985147, -0.1870078740157479769, 0.4822834645669291653 ) ) ;
#67253=CARTESIAN_POINT ( 'NONE',  ( 1.456692913385827515, -0.6692913385826771977, 8.415575281601705876E-17 ) ) ;
#67254=CARTESIAN_POINT ( 'NONE',  ( -0.7677165354330699465, 0.07958543189024085140, 0.2665933059059887866 ) ) ;
#67259=CARTESIAN_POINT ( 'NONE',  ( 1.541994750656168645, 0.1771653543307087075, -0.09757992244046823083 ) ) ;
#67260=CARTESIAN_POINT ( 'NONE',  ( 1.154855643044620184, 0.1283753931104746893, -0.1820866141732285504 ) ) ;
#67261=CARTESIAN_POINT ( 'NONE',  ( 0.4461942257217855756, 0.1539470093639521697, -0.1968503937007875793 ) ) ;
#67262=CARTESIAN_POINT ( 'NONE',  ( 0.7742782152230978099, -0.4281496062992124485, 0.4176697321401328655 ) ) ;
#67264=CARTESIAN_POINT ( 'NONE',  ( 1.082677165354331228, 0.07958543189024071263, -0.2665933059059888421 ) ) ;
#67265=CARTESIAN_POINT ( 'NONE',  ( -0.09842519685039295696, -0.5400638737290844871, 0.3530559997133364547 ) ) ;
#67266=CARTESIAN_POINT ( 'NONE',  ( -0.2362204724409440182, -0.1870078740157479769, 0.4822834645669291653 ) ) ;
#67267=CARTESIAN_POINT ( 'NONE',  ( 1.692913385826772421, 0.2952755905511811885, 0.000000000000000000 ) ) ;
#67270=CARTESIAN_POINT ( 'NONE',  ( 0.3805774278215230400, -0.004921259842519870586, -0.3153832671262229437 ) ) ;
#67273=ORIENTED_EDGE ( 'NONE', *, *, #19808, .T. ) ;
#67274=CARTESIAN_POINT ( 'NONE',  ( -0.4265091863517051496, 0.2952755905511810774, -0.1292274648535930714 ) ) ;
#67275=CARTESIAN_POINT ( 'NONE',  ( 0.7874015748031503170, -0.1870078740157479769, 0.4822834645669291653 ) ) ;
#67276=CARTESIAN_POINT ( 'NONE',  ( 0.07874015748031558404, -0.1870078740157479769, 0.4822834645669291653 ) ) ;
#67277=CARTESIAN_POINT ( 'NONE',  ( -0.2624671916010490880, -0.5023911411419708095, 0.1820866141732285504 ) ) ;
#67278=CARTESIAN_POINT ( 'NONE',  ( 0.7152230971128616943, -0.05778040916215522460, 0.4822834645669289988 ) ) ;
#67279=CARTESIAN_POINT ( 'NONE',  ( -0.9645669291338575535, 0.1660481256975883668, -0.3530559997133364547 ) ) ;
#67280=CARTESIAN_POINT ( 'NONE',  ( -0.4724409448818890911, -0.1870078740157479769, 0.4822834645669291653 ) ) ;
#67281=CARTESIAN_POINT ( 'NONE',  ( 0.9908136482939640111, 0.2952755905511810774, -0.1292274648535930714 ) ) ;
#67282=CARTESIAN_POINT ( 'NONE',  ( 0.9842519685039375910, 0.2952755905511811885, 0.000000000000000000 ) ) ;
#67283=CARTESIAN_POINT ( 'NONE',  ( 0.9251968503937015864, 0.1660481256975883668, -0.3530559997133364547 ) ) ;
#67285=CARTESIAN_POINT ( 'NONE',  ( -0.02624671916010428221, 0.1283753931104746893, -0.1820866141732285504 ) ) ;
#67289=CARTESIAN_POINT ( 'NONE',  ( -0.9514435695538050464, -0.2845877964562159024, 0.3641732283464567677 ) ) ;
#67290=CARTESIAN_POINT ( 'NONE',  ( -0.4593175853018364174, -0.4281496062992127816, -0.4176697321401328100 ) ) ;
#67292=CARTESIAN_POINT ( 'NONE',  ( -0.4724409448818890911, -0.1870078740157479769, 0.4822834645669291653 ) ) ;
#67293=CARTESIAN_POINT ( 'NONE',  ( -0.5643044619422565855, 0.05413385826771626580, -0.4176697321401330321 ) ) ;
#67294=CARTESIAN_POINT ( 'NONE',  ( -1.371391076115484609, -0.6692913385826771977, 0.1292274648535927661 ) ) ;
#67295=CARTESIAN_POINT ( 'NONE',  ( -1.601049868766403650, -0.6046776061558807314, 0.2411417322834647770 ) ) ;
#67296=CARTESIAN_POINT ( 'NONE',  ( 0.9120734908136490793, 0.1771653543307087075, -0.09757992244046823083 ) ) ;
#67298=CARTESIAN_POINT ( 'NONE',  ( -1.614173228346456712, 2.362204724409448620, 0.1372047244094477536 ) ) ;
#67299=CARTESIAN_POINT ( 'NONE',  ( 0.4593175853018379162, -0.3690944881889763329, 0.3153832671262228327 ) ) ;
#67300=CARTESIAN_POINT ( 'NONE',  ( 0.2559055118110243332, 0.1660481256975885056, 0.3530559997133364547 ) ) ;
#67301=CARTESIAN_POINT ( 'NONE',  ( 0.2427821522309719648, -0.05778040916215522460, 0.4822834645669289988 ) ) ;
#67302=ORIENTED_EDGE ( 'NONE', *, *, #78140, .F. ) ;
#67304=DIRECTION ( 'NONE',  ( 0.000000000000000000, 0.000000000000000000, -1.000000000000000000 ) ) ;
#67308=CARTESIAN_POINT ( 'NONE',  ( -0.6561679790026240244, -0.5023911411419708095, 0.1820866141732285504 ) ) ;
#67309=CARTESIAN_POINT ( 'NONE',  ( -1.056430446194224881, 0.2952755905511810774, -0.1292274648535930714 ) ) ;
#67312=CARTESIAN_POINT ( 'NONE',  ( 1.555118110236221041, 0.1660481256975883668, -0.3530559997133364547 ) ) ;
#67313=CARTESIAN_POINT ( 'NONE',  ( 1.049868766404200127, -0.6046776061558809534, -0.2411417322834644161 ) ) ;
#67314=CARTESIAN_POINT ( 'NONE',  ( 0.3215223097112867578, -0.3162353388693409650, -0.4822834645669289433 ) ) ;
#67315=CARTESIAN_POINT ( 'NONE',  ( -0.5314960629921250401, 0.07958543189024085140, 0.2665933059059887866 ) ) ;
#67316=CARTESIAN_POINT ( 'NONE',  ( 0.2230971128608929543, 0.05413385826771626580, -0.4176697321401330321 ) ) ;
#67318=CARTESIAN_POINT ( 'NONE',  ( -0.1443569553805765515, -0.3690944881889765550, -0.3153832671262227771 ) ) ;
#67319=CARTESIAN_POINT ( 'NONE',  ( -0.6627296587926503335, -0.6692913385826771977, 0.1292274648535927661 ) ) ;
#67322=CARTESIAN_POINT ( 'NONE',  ( -1.568241469816272105, -0.05778040916215522460, 0.4822834645669289988 ) ) ;
#67323=CARTESIAN_POINT ( 'NONE',  ( 0.1181102362204730916, -0.5511811023622047445, 6.969142054262312111E-17 ) ) ;
#67324=CARTESIAN_POINT ( 'NONE',  ( 1.607611548556431069, -0.5511811023622048555, -0.09757992244046775898 ) ) ;
#67325=CARTESIAN_POINT ( 'NONE',  ( -1.030183727034119867, -0.05778040916215560624, -0.4822834645669293319 ) ) ;
#67326=AXIS2_PLACEMENT_3D ( 'NONE', #51206, #11708, #12937 ) ;
#67327=CARTESIAN_POINT ( 'NONE',  ( -0.7349081364829387342, -0.5023911411419708095, 0.1820866141732285504 ) ) ;
#67328=CARTESIAN_POINT ( 'NONE',  ( -1.035118193396259434, 5.987370802660155681E-15, -0.3791483426435156567 ) ) ;
#67329=CARTESIAN_POINT ( 'NONE',  ( -1.194225721784776262, 0.05413385826771626580, -0.4176697321401330321 ) ) ;
#67330=CARTESIAN_POINT ( 'NONE',  ( 0.1312335958005257930, 0.2306618581243847221, -0.2411417322834647770 ) ) ;
#67332=CARTESIAN_POINT ( 'NONE',  ( 0.1902887139107617975, -0.6692913385826773087, -0.1292274648535924053 ) ) ;
#67335=CARTESIAN_POINT ( 'NONE',  ( 0.2099737532808405305, -0.5023911411419708095, 0.1820866141732285504 ) ) ;
#67336=CARTESIAN_POINT ( 'NONE',  ( 1.017060367454068581, -0.05778040916215560624, -0.4822834645669293319 ) ) ;
#67337=CARTESIAN_POINT ( 'NONE',  ( -1.233595800524933894, 0.1283753931104748280, 0.1820866141732283561 ) ) ;
#67338=CARTESIAN_POINT ( 'NONE',  ( 1.043307086614173818, 0.1660481256975885056, 0.3530559997133364547 ) ) ;
#67339=CARTESIAN_POINT ( 'NONE',  ( -1.692913385826770645, 0.1771653543307087630, 0.000000000000000000 ) ) ;
#67340=CARTESIAN_POINT ( 'NONE',  ( -0.5905511811023615998, 0.2952755905511811885, 0.000000000000000000 ) ) ;
#67341=CARTESIAN_POINT ( 'NONE',  ( 0.3477690288713918276, -0.5511811023622048555, -0.09757992244046775898 ) ) ;
#67342=CARTESIAN_POINT ( 'NONE',  ( 1.606165476768023126, 0.2953034477953545567, -0.04641075316546838109 ) ) ;
#67343=CARTESIAN_POINT ( 'NONE',  ( 0.4593175853018379162, -0.3690944881889763329, 0.3153832671262228327 ) ) ;
#67344=CARTESIAN_POINT ( 'NONE',  ( -0.1706036745406816491, 0.05413385826771626580, -0.4176697321401330321 ) ) ;
#67346=CARTESIAN_POINT ( 'NONE',  ( -0.9448818897637790704, -0.1870078740157479769, 0.4822834645669291653 ) ) ;
#67348=CARTESIAN_POINT ( 'NONE',  ( 1.154855643044620184, 0.1283753931104746893, -0.1820866141732285504 ) ) ;
#67349=CARTESIAN_POINT ( 'NONE',  ( 0.2099737532808405305, -0.6046776061558807314, 0.2411417322834647770 ) ) ;
#67350=CARTESIAN_POINT ( 'NONE',  ( -0.3608923884514428360, 0.2952755905511811885, 0.1292274648535926551 ) ) ;
#67351=CARTESIAN_POINT ( 'NONE',  ( -0.1902887139107604098, 0.1771653543307087075, -0.09757992244046823083 ) ) ;
#67352=CARTESIAN_POINT ( 'NONE',  ( 0.9908136482939640111, 0.2066929133858267098, -0.1054918080437494132 ) ) ;
#67353=CARTESIAN_POINT ( 'NONE',  ( -0.5905511811023613777, -0.5511811023622047445, 6.969142054262312111E-17 ) ) ;
#67354=CARTESIAN_POINT ( 'NONE',  ( 0.4068241469816281097, 0.05413385826771666132, 0.4176697321401328100 ) ) ;
#67355=CARTESIAN_POINT ( 'NONE',  ( -1.305774278215222184, -0.5511811023622048555, -0.09757992244046775898 ) ) ;
#67357=CARTESIAN_POINT ( 'NONE',  ( -0.9973753280839886548, 0.2306618581243848609, 0.2411417322834645549 ) ) ;
#67358=CARTESIAN_POINT ( 'NONE',  ( 0.8542087009142342868, -6.211426067506147994E-17, -0.3627989612356148363 ) ) ;
#67359=ORIENTED_EDGE ( 'NONE', *, *, #58958, .F. ) ;
#67360=CARTESIAN_POINT ( 'NONE',  ( -1.712598425196849572, 0.07958543189024085140, 0.2665933059059887866 ) ) ;
#67361=CARTESIAN_POINT ( 'NONE',  ( -0.5643044619422565855, 0.05413385826771626580, -0.4176697321401330321 ) ) ;
#67362=B_SPLINE_CURVE_WITH_KNOTS ( 'NONE', 3,
 ( #13969, #26583, #46343, #40051 ),
 .UNSPECIFIED., .F., .F.,
 ( 4, 4 ),
 ( 3.210432057725814518E-07, 0.001287787053612126330 ),
 .UNSPECIFIED. ) ;
#67364=CARTESIAN_POINT ( 'NONE',  ( -1.253280839895012377, -0.3162353388693409650, -0.4822834645669289433 ) ) ;
#67366=CARTESIAN_POINT ( 'NONE',  ( 1.574803149606299746, -0.1870078740157480879, -0.4822834645669291653 ) ) ;
#67367=CARTESIAN_POINT ( 'NONE',  ( 1.010498687664042716, -0.4281496062992124485, 0.4176697321401328655 ) ) ;
#67369=CARTESIAN_POINT ( 'NONE',  ( 1.306827173596997183, 0.000000000000000000, 0.4445507791589062285 ) ) ;
#67370=CARTESIAN_POINT ( 'NONE',  ( 1.410761154855643795, -0.2845877964562159024, 0.3641732283464567677 ) ) ;
#67372=ORIENTED_EDGE ( 'NONE', *, *, #49490, .T. ) ;
#67373=CARTESIAN_POINT ( 'NONE',  ( -0.3018372703412066094, -0.3690944881889765550, -0.3153832671262227771 ) ) ;
#67376=CARTESIAN_POINT ( 'NONE',  ( 0.7152230971128614723, -0.3162353388693409650, -0.4822834645669289433 ) ) ;
#67377=CARTESIAN_POINT ( 'NONE',  ( -0.2493438320209966919, 0.05413385826771626580, -0.4176697321401330321 ) ) ;
#67378=CARTESIAN_POINT ( 'NONE',  ( -0.9448818897637790704, -0.1870078740157480879, -0.4822834645669291653 ) ) ;
#67379=CARTESIAN_POINT ( 'NONE',  ( 1.633858267716535639, -0.5400638737290844871, 0.3530559997133364547 ) ) ;
#67380=CARTESIAN_POINT ( 'NONE',  ( -1.115485564304461219, -0.004921259842519870586, -0.3153832671262229437 ) ) ;
#67381=CARTESIAN_POINT ( 'NONE',  ( 0.3937007874015754361, -0.1870078740157479769, 0.4822834645669291653 ) ) ;
#67383=CARTESIAN_POINT ( 'NONE',  ( -0.7217847769028863381, -0.4281496062992124485, 0.4176697321401328655 ) ) ;
#67385=CARTESIAN_POINT ( 'NONE',  ( -1.305774278215222184, 0.2952755905511811885, 0.1292274648535926551 ) ) ;
#67387=CARTESIAN_POINT ( 'NONE',  ( 1.095800524934383846, -0.05778040916215560624, -0.4822834645669293319 ) ) ;
#67388=CARTESIAN_POINT ( 'NONE',  ( 1.069553805774278832, 0.1771653543307087075, -0.09757992244046823083 ) ) ;
#67391=CARTESIAN_POINT ( 'NONE',  ( -0.5314960629921250401, 0.1660481256975885056, 0.3530559997133364547 ) ) ;
#67392=ORIENTED_EDGE ( 'NONE', *, *, #5222, .F. ) ;
#67393=CARTESIAN_POINT ( 'NONE',  ( 0.4265091863517067039, -0.5511811023622048555, -0.09757992244046775898 ) ) ;
#67394=CARTESIAN_POINT ( 'NONE',  ( -1.213910761154854745, 0.2952755905511810774, -0.1292274648535930714 ) ) ;
#67395=CARTESIAN_POINT ( 'NONE',  ( 0.9251968503937015864, -0.5400638737290844871, 0.3530559997133364547 ) ) ;
#67396=CARTESIAN_POINT ( 'NONE',  ( 0.9383202099737536495, -0.3162353388693405765, 0.4822834645669290543 ) ) ;
#67397=CARTESIAN_POINT ( 'NONE',  ( -0.3346456692913377662, -0.5400638737290844871, 0.3530559997133364547 ) ) ;
#67399=CARTESIAN_POINT ( 'NONE',  ( -0.7545931758530176614, -0.6692913385826773087, -0.1292274648535924053 ) ) ;
#67401=CARTESIAN_POINT ( 'NONE',  ( -1.515748031496062076, 0.1660481256975883668, -0.3530559997133364547 ) ) ;
#67402=CARTESIAN_POINT ( 'NONE',  ( -0.6430446194225712953, 0.05413385826771626580, -0.4176697321401330321 ) ) ;
#67403=CARTESIAN_POINT ( 'NONE',  ( 1.194225721784777594, 0.05413385826771666132, 0.4176697321401328100 ) ) ;
#67405=CARTESIAN_POINT ( 'NONE',  ( 1.410761154855643795, -0.05778040916215560624, -0.4822834645669293319 ) ) ;
#67406=CARTESIAN_POINT ( 'NONE',  ( -0.7480314960629914633, 0.2952755905511811885, 0.000000000000000000 ) ) ;
#67407=CARTESIAN_POINT ( 'NONE',  ( 0.7349081364829402885, -0.6046776061558809534, -0.2411417322834644161 ) ) ;
#67410=CARTESIAN_POINT ( 'NONE',  ( -0.7086614173228339419, -0.1870078740157479769, 0.4822834645669291653 ) ) ;
#67411=CARTESIAN_POINT ( 'NONE',  ( -1.181102362204723644, -0.1870078740157479769, 0.3641732283464567677 ) ) ;
#67412=CARTESIAN_POINT ( 'NONE',  ( 0.6233595800524942554, -0.08942795157528024563, -0.3641732283464568787 ) ) ;
#67414=CARTESIAN_POINT ( 'NONE',  ( 1.056430446194226658, 0.1771653543307087630, 0.09757992244046791164 ) ) ;
#67415=CARTESIAN_POINT ( 'NONE',  ( 0.9383202099737536495, -0.3162353388693405765, 0.4822834645669290543 ) ) ;
#67418=CARTESIAN_POINT ( 'NONE',  ( -0.3608923884514428360, -0.6692913385826773087, -0.1292274648535924053 ) ) ;
#67420=CARTESIAN_POINT ( 'NONE',  ( 1.338582677165355062, -0.1870078740157480601, -0.3641732283464567677 ) ) ;
#67421=CARTESIAN_POINT ( 'NONE',  ( -0.4330708661417315697, 0.2952755905511811885, 0.000000000000000000 ) ) ;
#67423=CARTESIAN_POINT ( 'NONE',  ( 1.417322834645670104, -0.1870078740157480879, -0.4822834645669291653 ) ) ;
#67424=CARTESIAN_POINT ( 'NONE',  ( -0.07874015748031421014, -0.1870078740157480879, -0.4822834645669291653 ) ) ;
#67425=CARTESIAN_POINT ( 'NONE',  ( 0.6299212598425204535, -0.1870078740157480601, -0.3641732283464567677 ) ) ;
#67427=CARTESIAN_POINT ( 'NONE',  ( 0.09186351706036827158, -0.004921259842519576551, 0.3153832671262227771 ) ) ;
#67428=DIRECTION ( 'NONE',  ( -0.000000000000000000, -1.000000000000000000, -0.000000000000000000 ) ) ;
#67430=CARTESIAN_POINT ( 'NONE',  ( 0.5511811023622055217, -0.1870078740157479769, 0.4822834645669291653 ) ) ;
#67434=CARTESIAN_POINT ( 'NONE',  ( 0.2034120734908142214, 0.1771653543307087075, -0.09757992244046823083 ) ) ;
#67435=CARTESIAN_POINT ( 'NONE',  ( 0.1509186351706045259, -0.05778040916215560624, -0.4822834645669293319 ) ) ;
#67436=CARTESIAN_POINT ( 'NONE',  ( 1.279527559055118724, -0.4536011799217368745, -0.2665933059059886201 ) ) ;
#67437=CARTESIAN_POINT ( 'NONE',  ( -1.154855643044618851, -0.5023911411419708095, -0.1820866141732282451 ) ) ;
#67438=CARTESIAN_POINT ( 'NONE',  ( -1.496062992125983815, -0.1870078740157480879, -0.4822834645669291653 ) ) ;
#67440=CARTESIAN_POINT ( 'NONE',  ( 0.5708661417322842269, 0.1660481256975885056, 0.3530559997133364547 ) ) ;
#67441=CARTESIAN_POINT ( 'NONE',  ( 1.338582677165355062, -0.1870078740157479769, 0.4822834645669291653 ) ) ;
#67443=CARTESIAN_POINT ( 'NONE',  ( 0.2165354330708668673, 0.1660481256975883668, -0.3530559997133364547 ) ) ;
#67444=CARTESIAN_POINT ( 'NONE',  ( 1.207349081364829990, 0.2306618581243848609, 0.2411417322834645549 ) ) ;
#67445=CARTESIAN_POINT ( 'NONE',  ( 1.076115485564305141, 0.2306618581243847221, -0.2411417322834647770 ) ) ;
#67447=CARTESIAN_POINT ( 'NONE',  ( 0.9711286089238851948, -0.5023911411419708095, -0.1820866141732282451 ) ) ;
#67448=CARTESIAN_POINT ( 'NONE',  ( 1.692913385826772421, 0.2952755905511811885, 0.000000000000000000 ) ) ;
#67449=CARTESIAN_POINT ( 'NONE',  ( -0.8333333333333323711, 0.1771653543307087630, 0.09757992244046791164 ) ) ;
#67450=CARTESIAN_POINT ( 'NONE',  ( 0.3674540682414705883, 0.1283753931104746893, -0.1820866141732285504 ) ) ;
#67451=CARTESIAN_POINT ( 'NONE',  ( 0.01968503937007957949, -0.5400638737290845981, -0.3530559997133363437 ) ) ;
#67452=CARTESIAN_POINT ( 'NONE',  ( 0.8136482939632553313, 0.2306618581243848609, 0.2411417322834645549 ) ) ;
#67453=CARTESIAN_POINT ( 'NONE',  ( -0.2952755905511803003, -0.5400638737290845981, -0.3530559997133363437 ) ) ;
#67454=CARTESIAN_POINT ( 'NONE',  ( 0.2362204724409456558, -0.1870078740157480601, -0.3641732283464567677 ) ) ;
#67455=CARTESIAN_POINT ( 'NONE',  ( 0.8005249343832027131, 0.05413385826771666132, 0.4176697321401328100 ) ) ;
#67456=FACE_OUTER_BOUND ( 'NONE', #3413, .T. ) ;
#67457=CARTESIAN_POINT ( 'NONE',  ( -1.049868766404198794, 0.2306618581243847221, -0.2411417322834647770 ) ) ;
#67458=CARTESIAN_POINT ( 'NONE',  ( -1.076115485564303809, 0.2306618581243848609, 0.2411417322834645549 ) ) ;
#67460=CARTESIAN_POINT ( 'NONE',  ( 1.012922870834582101, 2.412178165100495768E-16, -0.4118484887281966822 ) ) ;
#67461=CARTESIAN_POINT ( 'NONE',  ( -0.7020997375328074108, -0.05778040916215522460, 0.4822834645669289988 ) ) ;
#67462=CARTESIAN_POINT ( 'NONE',  ( -0.6627296587926503335, -0.6692913385826771977, 0.1292274648535927661 ) ) ;
#67466=CARTESIAN_POINT ( 'NONE',  ( 0.8792650918635177559, -0.004921259842519576551, 0.3153832671262227771 ) ) ;
#67468=CARTESIAN_POINT ( 'NONE',  ( 0.9908136482939640111, 0.2952755905511810774, -0.1292274648535930714 ) ) ;
#67470=CARTESIAN_POINT ( 'NONE',  ( 2.795275590551181910, 1.535433070866142335, 0.000000000000000000 ) ) ;
#67471=CARTESIAN_POINT ( 'NONE',  ( -1.318897637795274802, -0.4536011799217368745, -0.2665933059059886201 ) ) ;
#67472=CARTESIAN_POINT ( 'NONE',  ( 2.795275590551181910, 1.771653543307087242, 0.000000000000000000 ) ) ;
#67473=CARTESIAN_POINT ( 'NONE',  ( -1.515748031496062076, 0.1660481256975883668, -0.3530559997133364547 ) ) ;
#67474=CARTESIAN_POINT ( 'NONE',  ( 0.2690288713910767848, 0.2952755905511811885, 0.1292274648535926551 ) ) ;
#67476=CARTESIAN_POINT ( 'NONE',  ( 0.08530183727034192087, -0.05778040916215522460, 0.4822834645669289988 ) ) ;
#67477=CARTESIAN_POINT ( 'NONE',  ( -0.9317585301837263412, -0.004921259842519576551, 0.3153832671262227771 ) ) ;
#67478=CARTESIAN_POINT ( 'NONE',  ( 0.8858267716535438430, -0.5400638737290845981, -0.3530559997133363437 ) ) ;
#67479=CARTESIAN_POINT ( 'NONE',  ( -0.2099737532808391705, -0.6046776061558809534, -0.2411417322834644161 ) ) ;
#67480=CARTESIAN_POINT ( 'NONE',  ( 0.4921259842519691841, 0.1660481256975885056, 0.3530559997133364547 ) ) ;
#67481=DIRECTION ( 'NONE',  ( -1.000000000000000000, -3.412570772413390973E-16, 0.000000000000000000 ) ) ;
#67483=CARTESIAN_POINT ( 'NONE',  ( 0.8727034120734913358, -0.05778040916215522460, 0.4822834645669289988 ) ) ;
#67484=CARTESIAN_POINT ( 'NONE',  ( 0.07874015748031558404, -0.1870078740157480879, -0.4822834645669291653 ) ) ;
#67485=CARTESIAN_POINT ( 'NONE',  ( -1.076115485564303809, -0.6046776061558809534, -0.2411417322834644161 ) ) ;
#67486=CARTESIAN_POINT ( 'NONE',  ( 1.292650918635171564, 0.2952755905511811885, 0.1292274648535926551 ) ) ;
#67487=CARTESIAN_POINT ( 'NONE',  ( 0.5971128608923891301, 0.2952755905511810774, -0.1292274648535930714 ) ) ;
#67489=CARTESIAN_POINT ( 'NONE',  ( -0.4593175853018366950, 0.05413385826771666132, 0.4176697321401328100 ) ) ;
#67490=CARTESIAN_POINT ( 'NONE',  ( 0.6364829396325465405, -0.3162353388693409650, -0.4822834645669289433 ) ) ;
#67491=CARTESIAN_POINT ( 'NONE',  ( 0.08530183727034192087, -0.05778040916215522460, 0.4822834645669289988 ) ) ;
#67492=CARTESIAN_POINT ( 'NONE',  ( 0.6955380577427828781, -0.3690944881889763329, 0.3153832671262228327 ) ) ;
#67493=CARTESIAN_POINT ( 'NONE',  ( -1.437007874015747477, -0.5400638737290844871, 0.3530559997133364547 ) ) ;
#67495=CARTESIAN_POINT ( 'NONE',  ( 0.2034120734908142214, 0.2952755905511810774, -0.1292274648535930714 ) ) ;
#67500=ORIENTED_EDGE ( 'NONE', *, *, #72060, .T. ) ;
#67501=CARTESIAN_POINT ( 'NONE',  ( 1.181102362204725198, -0.1870078740157479769, 0.4822834645669291653 ) ) ;
#67502=CARTESIAN_POINT ( 'NONE',  ( 0.6561679790026253567, 0.1283753931104748280, 0.1820866141732283561 ) ) ;
#67509=CARTESIAN_POINT ( 'NONE',  ( 1.049868766404200127, -0.6046776061558809534, -0.2411417322834644161 ) ) ;
#67510=CARTESIAN_POINT ( 'NONE',  ( -1.003937007874014853, 0.1660481256975885056, 0.3530559997133364547 ) ) ;
#67511=CARTESIAN_POINT ( 'NONE',  ( -0.8595800524934373854, -0.3162353388693409650, -0.4822834645669289433 ) ) ;
#67512=CARTESIAN_POINT ( 'NONE',  ( 0.5446194225721792126, -0.05778040916215560624, -0.4822834645669293319 ) ) ;
#67513=ORIENTED_EDGE ( 'NONE', *, *, #34562, .T. ) ;
#67514=CARTESIAN_POINT ( 'NONE',  ( 1.292650918635171564, 0.2952755905511811885, 0.1292274648535926551 ) ) ;
#67515=CARTESIAN_POINT ( 'NONE',  ( 1.200787401574803681, 0.1012011053420777407, 0.2882089793578256898 ) ) ;
#67517=CARTESIAN_POINT ( 'NONE',  ( 1.548556430446194954, 0.1283753931104746893, -0.1820866141732285504 ) ) ;
#67518=LINE ( 'NONE', #35943, #54637 ) ;
#67519=CARTESIAN_POINT ( 'NONE',  ( -1.246719160104985846, -0.3690944881889765550, -0.3153832671262227771 ) ) ;
#67520=DIRECTION ( 'NONE',  ( -0.7071067811865489050, -0.000000000000000000, 0.7071067811865460184 ) ) ;
#67521=CARTESIAN_POINT ( 'NONE',  ( 0.07217847769028949700, -0.3162353388693405765, 0.4822834645669290543 ) ) ;
#67523=CARTESIAN_POINT ( 'NONE',  ( -1.220472440944881054, 2.401574803149606474, 0.5309055118110237448 ) ) ;
#67524=CARTESIAN_POINT ( 'NONE',  ( -1.220472440944881054, 0.1771653543307087630, 0.000000000000000000 ) ) ;
#67525=CARTESIAN_POINT ( 'NONE',  ( 0.2034120734908144990, -0.6692913385826771977, 0.1292274648535927661 ) ) ;
#67526=CARTESIAN_POINT ( 'NONE',  ( 1.292650918635171564, 0.1771653543307087630, 0.09757992244046791164 ) ) ;
#67528=CARTESIAN_POINT ( 'NONE',  ( -1.272965879265091305, -0.3690944881889763329, 0.3153832671262228327 ) ) ;
#67529=CARTESIAN_POINT ( 'NONE',  ( 1.351706036745407680, 0.05413385826771666132, 0.4176697321401328100 ) ) ;
#67531=CARTESIAN_POINT ( 'NONE',  ( -0.3543307086614165824, -0.6692913385826771977, 8.415575281601705876E-17 ) ) ;
#67532=CARTESIAN_POINT ( 'NONE',  ( -1.489501312335957062, -0.08942795157527998196, 0.3641732283464567121 ) ) ;
#67533=CARTESIAN_POINT ( 'NONE',  ( -0.2362204724409442680, -0.1870078740157480601, -0.3641732283464567677 ) ) ;
#67534=ADVANCED_FACE ( 'NONE', ( #64650 ), #27177, .F. ) ;
#67535=CARTESIAN_POINT ( 'NONE',  ( -0.8661417322834640276, -0.1870078740157480879, -0.4822834645669291653 ) ) ;
#67536=CARTESIAN_POINT ( 'NONE',  ( -1.561679790026246017, -0.3690944881889765550, -0.3153832671262227771 ) ) ;
#67538=CARTESIAN_POINT ( 'NONE',  ( 0.1968503937007881344, 0.2952755905511811885, 0.000000000000000000 ) ) ;
#67543=CARTESIAN_POINT ( 'NONE',  ( -1.030183727034119867, -0.05778040916215560624, -0.4822834645669293319 ) ) ;
#67544=CARTESIAN_POINT ( 'NONE',  ( -0.6102362204724400829, 0.07958543189024085140, 0.2665933059059887866 ) ) ;
#67545=CARTESIAN_POINT ( 'NONE',  ( -0.4852136692201448609, 0.004960608223778509643, -0.3437734562760191848 ) ) ;
#67546=CARTESIAN_POINT ( 'NONE',  ( -0.1377952755905504645, -0.5400638737290845981, -0.3530559997133363437 ) ) ;
#67547=CARTESIAN_POINT ( 'NONE',  ( 0.2559055118110243332, 0.07958543189024085140, 0.2665933059059887866 ) ) ;
#67548=CARTESIAN_POINT ( 'NONE',  ( -1.240157480314959759, 0.07958543189024085140, 0.2665933059059887866 ) ) ;
#67549=CARTESIAN_POINT ( 'NONE',  ( -1.443569553805773564, -0.6046776061558807314, 0.2411417322834647770 ) ) ;
#67550=CARTESIAN_POINT ( 'NONE',  ( -1.463254593175852492, -0.6692913385826773087, -0.1292274648535924053 ) ) ;
#67551=CARTESIAN_POINT ( 'NONE',  ( 1.541994750656168645, 0.2952755905511810774, -0.1292274648535930714 ) ) ;
#67553=CARTESIAN_POINT ( 'NONE',  ( 0.5971128608923891301, 0.1771653543307087075, -0.09757992244046823083 ) ) ;
#67554=CARTESIAN_POINT ( 'NONE',  ( 0.7939632545931766261, -0.3162353388693409650, -0.4822834645669289433 ) ) ;
#67555=CARTESIAN_POINT ( 'NONE',  ( -1.586052503253848611, 0.7480314960629931287, 0.1653254495020559378 ) ) ;
#67556=CARTESIAN_POINT ( 'NONE',  ( 1.437007874015748810, 0.07958543189024085140, 0.2665933059059887866 ) ) ;
#67560=CARTESIAN_POINT ( 'NONE',  ( -1.062992125984250968, -0.6692913385826771977, 8.415575281601705876E-17 ) ) ;
#67562=CARTESIAN_POINT ( 'NONE',  ( -0.8530183727034112984, 0.05413385826771666132, 0.4176697321401328100 ) ) ;
#67563=CARTESIAN_POINT ( 'NONE',  ( 0.4593175853018379162, -0.4281496062992124485, 0.4176697321401328655 ) ) ;
#67564=CARTESIAN_POINT ( 'NONE',  ( -1.391076115485563758, 0.1283753931104748280, 0.1820866141732283561 ) ) ;
#67566=CARTESIAN_POINT ( 'NONE',  ( 1.338582677165355062, -0.1870078740157480601, -0.3641732283464567677 ) ) ;
#67567=CARTESIAN_POINT ( 'NONE',  ( 0.4593175853018380828, 0.05413385826771626580, -0.4176697321401330321 ) ) ;
#67568=CARTESIAN_POINT ( 'NONE',  ( 0.6889763779527563470, 0.1660481256975883668, -0.3530559997133364547 ) ) ;
#67569=CARTESIAN_POINT ( 'NONE',  ( -1.614173228346456712, 1.267785121476993737, -0.1372047244094478091 ) ) ;
#67575=CARTESIAN_POINT ( 'NONE',  ( 0.03937007874015806264, 0.1771653543307087630, 0.000000000000000000 ) ) ;
#67576=CARTESIAN_POINT ( 'NONE',  ( -0.2559055118110230564, 0.1660481256975883668, -0.3530559997133364547 ) ) ;
#67577=CARTESIAN_POINT ( 'NONE',  ( 0.8333333333333340365, 0.2952755905511810774, -0.1292274648535930714 ) ) ;
#67579=CARTESIAN_POINT ( 'NONE',  ( -0.1115485564304453947, -0.5511811023622046335, 0.09757992244046803654 ) ) ;
#67580=CARTESIAN_POINT ( 'NONE',  ( -1.266404199475064773, -0.05778040916215560624, -0.4822834645669293319 ) ) ;
#67581=CARTESIAN_POINT ( 'NONE',  ( 1.043307086614173818, -0.5400638737290845981, -0.3530559997133363437 ) ) ;
#67588=CARTESIAN_POINT ( 'NONE',  ( 0.8398950131233602345, 0.2306618581243847221, -0.2411417322834647770 ) ) ;
#67589=CARTESIAN_POINT ( 'NONE',  ( 1.561679790026247350, -0.3690944881889763329, 0.3153832671262228327 ) ) ;
#67590=CARTESIAN_POINT ( 'NONE',  ( -1.463254593175852492, 0.1771653543307087630, 0.09757992244046791164 ) ) ;
#67591=CARTESIAN_POINT ( 'NONE',  ( -1.463254593175852492, 0.2952755905511811885, 0.1292274648535926551 ) ) ;
#67593=DIRECTION ( 'NONE',  ( -1.000000000000000000, 0.000000000000000000, 0.000000000000000000 ) ) ;
#67594=CARTESIAN_POINT ( 'NONE',  ( 1.141732283464567788, -0.6692913385826771977, 8.415575281601705876E-17 ) ) ;
#67595=CARTESIAN_POINT ( 'NONE',  ( -1.725721784776902190, -0.05778040916215522460, 0.4822834645669289988 ) ) ;
#67596=CARTESIAN_POINT ( 'NONE',  ( -0.04593175853018302557, -0.6692913385826773087, -0.1292274648535924053 ) ) ;
#67597=CARTESIAN_POINT ( 'NONE',  ( -0.7480314960629914633, 0.2952755905511811885, 0.000000000000000000 ) ) ;
#67598=CARTESIAN_POINT ( 'NONE',  ( 1.528871391076116026, -0.6692913385826773087, -0.1292274648535924053 ) ) ;
#67600=CARTESIAN_POINT ( 'NONE',  ( 0.1509186351706042484, -0.3162353388693405765, 0.4822834645669290543 ) ) ;
#67602=CARTESIAN_POINT ( 'NONE',  ( -1.062992125984250968, -0.5511811023622047445, 6.969142054262312111E-17 ) ) ;
#67605=EDGE_LOOP ( 'NONE', ( #77653, #72667, #11183, #74950 ) ) ;
#67607=CARTESIAN_POINT ( 'NONE',  ( -1.620734908136482577, -0.6692913385826773087, -0.1292274648535924053 ) ) ;
#67609=CARTESIAN_POINT ( 'NONE',  ( 1.640419947506562393, -0.3690944881889763329, 0.3153832671262228327 ) ) ;
#67611=CARTESIAN_POINT ( 'NONE',  ( 0.4396325459317593221, 0.2952755905511810219, -0.1292274648535930437 ) ) ;
#67615=CARTESIAN_POINT ( 'NONE',  ( -0.4527559055118102749, -0.4536011799217368745, -0.2665933059059886201 ) ) ;
#67616=CARTESIAN_POINT ( 'NONE',  ( -0.7742782152230965886, -0.004921259842519576551, 0.3153832671262227771 ) ) ;
#67617=CARTESIAN_POINT ( 'NONE',  ( -1.200787401574802349, -0.5400638737290844871, 0.3530559997133364547 ) ) ;
#67618=CARTESIAN_POINT ( 'NONE',  ( 0.5380577427821529035, 0.05413385826771626580, -0.4176697321401330321 ) ) ;
#67619=CARTESIAN_POINT ( 'NONE',  ( -1.469816272965878357, 0.2306618581243848609, 0.2411417322834645549 ) ) ;
#67622=CARTESIAN_POINT ( 'NONE',  ( -1.587926509186350810, 0.05413385826771626580, -0.4176697321401330321 ) ) ;
#67631=CARTESIAN_POINT ( 'NONE',  ( -0.7217847769028863381, -0.4281496062992124485, 0.4176697321401328655 ) ) ;
#67632=CARTESIAN_POINT ( 'NONE',  ( 1.502624671916010790, -0.05778040916215522460, 0.4822834645669289988 ) ) ;
#67633=DIRECTION ( 'NONE',  ( 0.000000000000000000, 0.000000000000000000, 1.000000000000000000 ) ) ;
#67635=CARTESIAN_POINT ( 'NONE',  ( -1.351706036745406347, 0.05413385826771626580, -0.4176697321401330321 ) ) ;
#67636=CARTESIAN_POINT ( 'NONE',  ( -1.010498687664041384, -0.4281496062992127816, -0.4176697321401328100 ) ) ;
#67638=CARTESIAN_POINT ( 'NONE',  ( 0.04593175853018440641, 0.1771653543307087075, -0.09757992244046823083 ) ) ;
#67640=CARTESIAN_POINT ( 'NONE',  ( -0.03937007874015669567, 0.1771653543307087630, 0.000000000000000000 ) ) ;
#67641=CARTESIAN_POINT ( 'NONE',  ( 0.8530183727034126306, -0.004921259842519870586, -0.3153832671262229437 ) ) ;
#67642=CARTESIAN_POINT ( 'NONE',  ( 0.4199475065616803948, -0.6046776061558809534, -0.2411417322834644161 ) ) ;
#67643=CARTESIAN_POINT ( 'NONE',  ( -0.1181102362204717315, -0.5511811023622047445, 6.969142054262312111E-17 ) ) ;
#67645=CARTESIAN_POINT ( 'NONE',  ( 1.371391076115485719, -0.6692913385826773087, -0.1292274648535924053 ) ) ;
#67646=CARTESIAN_POINT ( 'NONE',  ( -1.430446194225720724, -0.004921259842519870586, -0.3153832671262229437 ) ) ;
#67648=CARTESIAN_POINT ( 'NONE',  ( 0.1771653543307093182, 0.1660481256975885056, 0.3530559997133364547 ) ) ;
#67649=CARTESIAN_POINT ( 'NONE',  ( -0.4986876640419939388, 0.2306618581243847221, -0.2411417322834647770 ) ) ;
#67651=CARTESIAN_POINT ( 'NONE',  ( 0.5052493438320215802, 0.1771653543307087630, 0.09757992244046791164 ) ) ;
#67652=CARTESIAN_POINT ( 'NONE',  ( -0.4068241469816267775, 0.05413385826771626580, -0.4176697321401330321 ) ) ;
#67653=CARTESIAN_POINT ( 'NONE',  ( -0.5380577427821514602, 0.05413385826771666132, 0.4176697321401328100 ) ) ;
#67657=CARTESIAN_POINT ( 'NONE',  ( 0.03937007874015833325, -0.6692913385826771977, 8.415575281601705876E-17 ) ) ;
#67659=CARTESIAN_POINT ( 'NONE',  ( -1.614173228346457378, 1.330640075373402897, -0.1372047244094477536 ) ) ;
#67660=CARTESIAN_POINT ( 'NONE',  ( -0.06561679790026180015, -0.3690944881889765550, -0.3153832671262227771 ) ) ;
#67661=CARTESIAN_POINT ( 'NONE',  ( -0.5971128608923877978, 0.2952755905511811885, 0.1292274648535926551 ) ) ;
#67662=CARTESIAN_POINT ( 'NONE',  ( 1.686351706036745890, 0.2952755905511811885, 0.1292274648535926551 ) ) ;
#67663=CARTESIAN_POINT ( 'NONE',  ( 1.312335958005250269, -0.6046776061558807314, 0.2411417322834647770 ) ) ;
#67665=CARTESIAN_POINT ( 'NONE',  ( -0.4855643044619415427, -0.3690944881889763329, 0.3153832671262228327 ) ) ;
#67670=CARTESIAN_POINT ( 'NONE',  ( 1.548556430446194954, 0.1283753931104746893, -0.1820866141732285504 ) ) ;
#67671=CARTESIAN_POINT ( 'NONE',  ( 0.9908136482939640111, 0.1771653543307087075, -0.09757992244046823083 ) ) ;
#67672=CARTESIAN_POINT ( 'NONE',  ( 0.9120734908136489683, -0.6692913385826771977, 0.1292274648535927661 ) ) ;
#67673=CARTESIAN_POINT ( 'NONE',  ( 0.4199475065616804503, 0.1539470093639523085, 0.1968503937007873850 ) ) ;
#67674=CARTESIAN_POINT ( 'NONE',  ( 0.9973753280839902091, 0.2306618581243847221, -0.2411417322834647770 ) ) ;
#67676=CARTESIAN_POINT ( 'NONE',  ( 1.017060367454068803, -0.2845877964562159024, 0.3641732283464567677 ) ) ;
#67677=CARTESIAN_POINT ( 'NONE',  ( -0.06561679790026180015, 0.05413385826771666132, 0.4176697321401328100 ) ) ;
#67678=CARTESIAN_POINT ( 'NONE',  ( -0.6299212598425188991, -0.1870078740157480879, -0.4822834645669291653 ) ) ;
#67679=CARTESIAN_POINT ( 'NONE',  ( -0.4600214019799515053, 0.000000000000000000, 0.3464511005275205946 ) ) ;
#67682=CARTESIAN_POINT ( 'NONE',  ( 0.3740157480314966754, 0.07958543189024071263, -0.2665933059059888421 ) ) ;
#67683=EDGE_CURVE ( 'NONE', #10557, #68129, #34291, .T. ) ;
#67687=CARTESIAN_POINT ( 'NONE',  ( -0.3018372703412066094, 0.05413385826771666132, 0.4176697321401328100 ) ) ;
#67688=CARTESIAN_POINT ( 'NONE',  ( -0.3477690288713902178, 0.2952755905511810774, -0.1292274648535930714 ) ) ;
#67689=CARTESIAN_POINT ( 'NONE',  ( -0.4265091863517051496, -0.6692913385826771977, 0.1292274648535927661 ) ) ;
#67690=CARTESIAN_POINT ( 'NONE',  ( 0.9055118110236227702, 0.2952755905511811885, 0.000000000000000000 ) ) ;
#67692=CARTESIAN_POINT ( 'NONE',  ( -0.9251968503937002541, -0.5400638737290845981, -0.3530559997133363437 ) ) ;
#67693=CARTESIAN_POINT ( 'NONE',  ( -0.3215223097112853146, -0.3162353388693405765, 0.4822834645669290543 ) ) ;
#67694=CARTESIAN_POINT ( 'NONE',  ( 1.332020997375328974, -0.05778040916215560624, -0.4822834645669293319 ) ) ;
#67695=CARTESIAN_POINT ( 'NONE',  ( 0.8267716535433077274, 0.2952755905511811885, 0.000000000000000000 ) ) ;
#67696=CARTESIAN_POINT ( 'NONE',  ( 0.7611548556430454138, 0.2306618581243847221, -0.2411417322834647770 ) ) ;
#67698=CARTESIAN_POINT ( 'NONE',  ( 0.02624671916010564918, -0.5023911411419708095, -0.1820866141732282451 ) ) ;
#67701=ORIENTED_EDGE ( 'NONE', *, *, #39397, .T. ) ;
#67702=CARTESIAN_POINT ( 'NONE',  ( -0.7414698162729651543, 0.1771653543307087075, -0.09757992244046823083 ) ) ;
#67703=CARTESIAN_POINT ( 'NONE',  ( -0.3740157480314953431, 0.1660481256975885056, 0.3530559997133364547 ) ) ;
#67705=CARTESIAN_POINT ( 'NONE',  ( -0.5577427821522301654, -0.05778040916215560624, -0.4822834645669293319 ) ) ;
#67706=CARTESIAN_POINT ( 'NONE',  ( -0.2755905511811018171, 0.2952755905511811885, 0.000000000000000000 ) ) ;
#67707=CARTESIAN_POINT ( 'NONE',  ( -1.299212598425196097, 0.2952755905511811885, 0.000000000000000000 ) ) ;
#67708=CARTESIAN_POINT ( 'NONE',  ( -1.377952755905511140, 0.2952755905511811885, 0.000000000000000000 ) ) ;
#67709=CARTESIAN_POINT ( 'NONE',  ( 0.8858267716535438430, 0.07958543189024085140, 0.2665933059059887866 ) ) ;
#67712=CARTESIAN_POINT ( 'NONE',  ( 0.5905511811023629321, -0.5511811023622047445, 6.969142054262312111E-17 ) ) ;
#67713=AXIS2_PLACEMENT_3D ( 'NONE', #56745, #63078, #23529 ) ;
#67714=CARTESIAN_POINT ( 'NONE',  ( -0.1312335958005241554, -0.6046776061558809534, -0.2411417322834644161 ) ) ;
#67715=CARTESIAN_POINT ( 'NONE',  ( -0.1837270341207340729, 0.2306618581243847221, -0.2411417322834647770 ) ) ;
#67718=CARTESIAN_POINT ( 'NONE',  ( -0.6036745406824141069, 0.2306618581243848609, 0.2411417322834645549 ) ) ;
#67719=EDGE_LOOP ( 'NONE', ( #37350, #24220, #48805, #45081 ) ) ;
#67722=CARTESIAN_POINT ( 'NONE',  ( -0.8923884514435688198, 0.1283753931104746893, -0.1820866141732285504 ) ) ;
#67723=CARTESIAN_POINT ( 'NONE',  ( -1.154855643044618851, -0.6046776061558809534, -0.2411417322834644161 ) ) ;
#67727=CARTESIAN_POINT ( 'NONE',  ( -1.496062992125983815, -0.1870078740157479769, 0.3641732283464567677 ) ) ;
#67728=CARTESIAN_POINT ( 'NONE',  ( 0.2427821522309716595, -0.3162353388693409650, -0.4822834645669289433 ) ) ;
#67729=CARTESIAN_POINT ( 'NONE',  ( 0.6233595800524942554, -0.05778040916215560624, -0.4822834645669293319 ) ) ;
#67730=CARTESIAN_POINT ( 'NONE',  ( -0.4855643044619415427, -0.004921259842519870586, -0.3153832671262229437 ) ) ;
#67731=CARTESIAN_POINT ( 'NONE',  ( -0.05905511811023545637, -0.5400638737290845981, -0.3530559997133363437 ) ) ;
#67733=CARTESIAN_POINT ( 'NONE',  ( -0.4921259842519677963, 0.07958543189024071263, -0.2665933059059888421 ) ) ;
#67734=CARTESIAN_POINT ( 'NONE',  ( -0.5314960629921254842, -0.5400638737290845981, -0.3530559997133363437 ) ) ;
#67738=CARTESIAN_POINT ( 'NONE',  ( -1.719160104986876103, 0.05413385826771666132, 0.4176697321401328100 ) ) ;
#67739=CARTESIAN_POINT ( 'NONE',  ( -0.05905511811023545637, -0.4536011799217368745, -0.2665933059059886201 ) ) ;
#67740=CARTESIAN_POINT ( 'NONE',  ( 1.003937007874016407, -0.4536011799217367080, 0.2665933059059888421 ) ) ;
#67741=CARTESIAN_POINT ( 'NONE',  ( -1.318897637795274802, -0.5400638737290845981, -0.3530559997133363437 ) ) ;
#67742=CARTESIAN_POINT ( 'NONE',  ( -0.8202099737532799750, 0.1771653543307087075, -0.09757992244046823083 ) ) ;
#67743=CARTESIAN_POINT ( 'NONE',  ( 1.614173228346456712, 1.496062992125984037, -0.1372047244094476703 ) ) ;
#67744=CARTESIAN_POINT ( 'NONE',  ( -1.003937007874015297, -0.5400638737290845981, -0.3530559997133363437 ) ) ;
#67745=CARTESIAN_POINT ( 'NONE',  ( -0.2690288713910754526, -0.6692913385826771977, 0.1292274648535927661 ) ) ;
#67746=CARTESIAN_POINT ( 'NONE',  ( 0.2559055118110243332, 0.1660481256975885056, 0.3530559997133364547 ) ) ;
#67749=CARTESIAN_POINT ( 'NONE',  ( 0.3149606299212606708, -0.1870078740157480601, -0.3641732283464567677 ) ) ;
#67750=CARTESIAN_POINT ( 'NONE',  ( 1.030183727034121421, -0.3162353388693409650, -0.4822834645669289433 ) ) ;
#67751=CARTESIAN_POINT ( 'NONE',  ( -1.076115485564303809, 0.1283753931104748280, 0.1820866141732283561 ) ) ;
#67752=CARTESIAN_POINT ( 'NONE',  ( 1.148293963254593875, -0.6692913385826771977, 0.1292274648535927661 ) ) ;
#67753=CARTESIAN_POINT ( 'NONE',  ( -1.620734908136482577, -0.5511811023622048555, -0.09757992244046775898 ) ) ;
#67754=CARTESIAN_POINT ( 'NONE',  ( 1.594488188976378673, 0.07958543189024085140, 0.2665933059059887866 ) ) ;
#67755=CARTESIAN_POINT ( 'NONE',  ( -0.7742782152230965886, 0.05413385826771666132, 0.4176697321401328100 ) ) ;
#67756=CARTESIAN_POINT ( 'NONE',  ( 0.03280839895013198948, -0.5511811023622048555, -0.09757992244046775898 ) ) ;
#67758=CARTESIAN_POINT ( 'NONE',  ( 0.5971128608923890191, -0.5511811023622046335, 0.09757992244046803654 ) ) ;
#67759=CARTESIAN_POINT ( 'NONE',  ( 0.01312335958005323398, -0.4281496062992127816, -0.4176697321401328100 ) ) ;
#67761=CARTESIAN_POINT ( 'NONE',  ( -1.286089238845143479, -0.6046776061558807314, 0.2411417322834647770 ) ) ;
#67763=CARTESIAN_POINT ( 'NONE',  ( 1.010498687664042716, -0.004921259842519870586, -0.3153832671262229437 ) ) ;
#67764=CARTESIAN_POINT ( 'NONE',  ( -0.07217847769028787330, -0.05778040916215522460, 0.4822834645669289988 ) ) ;
#67765=CARTESIAN_POINT ( 'NONE',  ( -0.4068241469816264999, -0.4281496062992124485, 0.4176697321401328655 ) ) ;
#67766=CARTESIAN_POINT ( 'NONE',  ( -0.4133858267716528645, -0.4536011799217367080, 0.2665933059059888421 ) ) ;
#67768=CARTESIAN_POINT ( 'NONE',  ( -0.3018372703412066094, -0.3690944881889765550, -0.3153832671262227771 ) ) ;
#67769=CARTESIAN_POINT ( 'NONE',  ( 0.4461942257217856311, 0.2306618581243847221, -0.2411417322834647770 ) ) ;
#67770=CARTESIAN_POINT ( 'NONE',  ( -0.9973753280839886548, -0.5023911411419708095, -0.1820866141732282451 ) ) ;
#67772=CARTESIAN_POINT ( 'NONE',  ( -1.240157480314959759, -0.5400638737290845981, -0.3530559997133363437 ) ) ;
#67774=ORIENTED_EDGE ( 'NONE', *, *, #21915, .F. ) ;
#67775=CARTESIAN_POINT ( 'NONE',  ( -1.719160104986876103, -0.004921259842519576551, 0.3153832671262227771 ) ) ;
#67776=CARTESIAN_POINT ( 'NONE',  ( -0.3346456692913377662, -0.5400638737290844871, 0.3530559997133364547 ) ) ;
#67778=CARTESIAN_POINT ( 'NONE',  ( -1.122047244094487306, 0.1660481256975883668, -0.3530559997133364547 ) ) ;
#67781=CARTESIAN_POINT ( 'NONE',  ( 1.482939632545932307, -0.4281496062992124485, 0.4176697321401328655 ) ) ;
#67782=CARTESIAN_POINT ( 'NONE',  ( 0.2952755905511819101, 0.1660481256975883668, -0.3530559997133364547 ) ) ;
#67785=CARTESIAN_POINT ( 'NONE',  ( 1.594488188976378673, 0.07958543189024085140, 0.2665933059059887866 ) ) ;
#67786=EDGE_CURVE ( 'NONE', #38903, #28439, #266, .T. ) ;
#67789=CARTESIAN_POINT ( 'NONE',  ( -0.9776902887139098386, 0.1771653543307087075, -0.09757992244046823083 ) ) ;
#67793=CARTESIAN_POINT ( 'NONE',  ( 0.9908136482939640111, 0.2952755905511810774, -0.1292274648535930714 ) ) ;
#67794=CARTESIAN_POINT ( 'NONE',  ( -0.1902887139107604098, -0.6692913385826771977, 0.1292274648535927661 ) ) ;
#67795=CARTESIAN_POINT ( 'NONE',  ( -1.240157480314959759, -0.5400638737290845981, -0.3530559997133363437 ) ) ;
#67796=CARTESIAN_POINT ( 'NONE',  ( 1.154855643044620184, -0.6046776061558807314, 0.2411417322834647770 ) ) ;
#67797=CARTESIAN_POINT ( 'NONE',  ( -1.312335958005248715, 0.1283753931104748280, 0.1820866141732283561 ) ) ;
#67798=CARTESIAN_POINT ( 'NONE',  ( 0.08874907683610111508, -2.191421614605370878E-15, 0.4445507791589071167 ) ) ;
#67799=CARTESIAN_POINT ( 'NONE',  ( 0.3083989501312343062, -0.05778040916215560624, -0.4822834645669293319 ) ) ;
#67800=CARTESIAN_POINT ( 'NONE',  ( -0.7283464566929126471, -0.5400638737290844871, 0.3530559997133364547 ) ) ;
#67802=CARTESIAN_POINT ( 'NONE',  ( -1.351706036745406347, -0.4281496062992124485, 0.4176697321401328655 ) ) ;
#67804=CARTESIAN_POINT ( 'NONE',  ( 1.030183727034121421, -0.05778040916215522460, 0.4822834645669289988 ) ) ;
#67806=CARTESIAN_POINT ( 'NONE',  ( 1.404199475065617708, -0.004921259842519870586, -0.3153832671262229437 ) ) ;
#67809=CARTESIAN_POINT ( 'NONE',  ( -0.4330708661417315697, -0.6692913385826771977, 8.415575281601705876E-17 ) ) ;
#67811=CARTESIAN_POINT ( 'NONE',  ( 0.3280839895013130669, -0.004921259842519576551, 0.3153832671262227771 ) ) ;
#67812=CARTESIAN_POINT ( 'NONE',  ( -1.568241469816272105, -0.05778040916215522460, 0.4822834645669289988 ) ) ;
#67813=CARTESIAN_POINT ( 'NONE',  ( 0.7742782152230978099, -0.4281496062992124485, 0.4176697321401328655 ) ) ;
#67814=CARTESIAN_POINT ( 'NONE',  ( 0.8005249343832027131, 0.05413385826771666132, 0.4176697321401328100 ) ) ;
#67815=CARTESIAN_POINT ( 'NONE',  ( -0.01968503937007793844, -0.5400638737290844871, 0.3530559997133364547 ) ) ;
#67817=CARTESIAN_POINT ( 'NONE',  ( -0.8398950131233585692, 0.2306618581243848609, 0.2411417322834645549 ) ) ;
#67819=CARTESIAN_POINT ( 'NONE',  ( -1.692913385826770645, 0.2952755905511811885, 0.000000000000000000 ) ) ;
#67820=CARTESIAN_POINT ( 'NONE',  ( -0.9186351706036736120, -0.6046776061558809534, -0.2411417322834644161 ) ) ;
#67821=CARTESIAN_POINT ( 'NONE',  ( 1.456692913385827515, -0.6692913385826771977, 8.415575281601705876E-17 ) ) ;
#67822=CARTESIAN_POINT ( 'NONE',  ( 1.633858267716535639, -0.5400638737290844871, 0.3530559997133364547 ) ) ;
#67823=CARTESIAN_POINT ( 'NONE',  ( -0.9776902887139098386, -0.6692913385826771977, 0.1292274648535927661 ) ) ;
#67825=CARTESIAN_POINT ( 'NONE',  ( 0.1509186351706042484, -0.3162353388693405765, 0.4822834645669290543 ) ) ;
#67827=CARTESIAN_POINT ( 'NONE',  ( -0.3937007874015740483, -0.1870078740157479769, 0.4822834645669291653 ) ) ;
#67828=CARTESIAN_POINT ( 'NONE',  ( -1.437007874015747477, 0.07958543189024071263, -0.2665933059059888421 ) ) ;
#67829=CARTESIAN_POINT ( 'NONE',  ( 0.5971128608923891301, 0.1771653543307087075, -0.09757992244046823083 ) ) ;
#67830=CARTESIAN_POINT ( 'NONE',  ( 1.456692913385827515, 0.2952755905511811885, 0.000000000000000000 ) ) ;
#67832=CARTESIAN_POINT ( 'NONE',  ( 0.6036745406824154392, 0.1283753931104746893, -0.1820866141732285504 ) ) ;
#67833=CARTESIAN_POINT ( 'NONE',  ( 0.8661417322834652488, -0.1870078740157480879, -0.4822834645669291653 ) ) ;
#67835=CARTESIAN_POINT ( 'NONE',  ( -0.5708661417322828946, 0.1660481256975883668, -0.3530559997133364547 ) ) ;
#67837=CARTESIAN_POINT ( 'NONE',  ( 1.456692913385827515, 0.1771653543307087630, 0.000000000000000000 ) ) ;
#67838=CARTESIAN_POINT ( 'NONE',  ( -0.5183727034120726440, -0.6692913385826773087, -0.1292274648535924053 ) ) ;
#67840=CARTESIAN_POINT ( 'NONE',  ( 1.227034120734908917, 0.2952755905511810774, -0.1292274648535930714 ) ) ;
#67841=CARTESIAN_POINT ( 'NONE',  ( 0.1181102362204730916, -0.6692913385826771977, 8.415575281601705876E-17 ) ) ;
#67842=CARTESIAN_POINT ( 'NONE',  ( 0.3477690288713918276, -0.5511811023622048555, -0.09757992244046775898 ) ) ;
#67843=CARTESIAN_POINT ( 'NONE',  ( 0.8537221893815273299, 2.409604939980833412E-17, -0.3464511005275205946 ) ) ;
#67844=CARTESIAN_POINT ( 'NONE',  ( 0.01312335958005323398, -0.3690944881889765550, -0.3153832671262227771 ) ) ;
#67845=CARTESIAN_POINT ( 'NONE',  ( 0.7677165354330716118, -0.4536011799217367080, 0.2665933059059888421 ) ) ;
#67846=CARTESIAN_POINT ( 'NONE',  ( -1.587926509186350810, 0.05413385826771626580, -0.4176697321401330321 ) ) ;
#67848=CARTESIAN_POINT ( 'NONE',  ( 0.7611548556430454138, 0.2306618581243847221, -0.2411417322834647770 ) ) ;
#67850=CARTESIAN_POINT ( 'NONE',  ( 1.456692913385827515, -0.5511811023622047445, 6.969142054262312111E-17 ) ) ;
#67852=CARTESIAN_POINT ( 'NONE',  ( 0.2165354330708668673, 0.07958543189024071263, -0.2665933059059888421 ) ) ;
#67854=CARTESIAN_POINT ( 'NONE',  ( 0.1771653543307093182, -0.5400638737290845981, -0.3530559997133363437 ) ) ;
#67855=CARTESIAN_POINT ( 'NONE',  ( 1.305774278215223960, -0.5511811023622046335, 0.09757992244046803654 ) ) ;
#67856=CARTESIAN_POINT ( 'NONE',  ( -1.318897637795274802, -0.4536011799217368745, -0.2665933059059886201 ) ) ;
#67857=CARTESIAN_POINT ( 'NONE',  ( -1.286089238845143479, -0.6046776061558807314, 0.2411417322834647770 ) ) ;
#67858=CARTESIAN_POINT ( 'NONE',  ( 0.1640419947506569498, -0.3162353388693409650, -0.4822834645669289433 ) ) ;
#67859=CARTESIAN_POINT ( 'NONE',  ( 1.017060367454068803, -0.3162353388693405765, 0.4822834645669290543 ) ) ;
#67862=CARTESIAN_POINT ( 'NONE',  ( 0.1706036745406830368, 0.05413385826771666132, 0.4176697321401328100 ) ) ;
#67863=CARTESIAN_POINT ( 'NONE',  ( 1.108923884514436686, -0.3162353388693409650, -0.4822834645669289433 ) ) ;
#67864=CARTESIAN_POINT ( 'NONE',  ( 1.056430446194226658, 0.2952755905511811885, 0.1292274648535926551 ) ) ;
#67865=DIRECTION ( 'NONE',  ( 0.000000000000000000, -1.000000000000000000, 0.000000000000000000 ) ) ;
#67866=CARTESIAN_POINT ( 'NONE',  ( 0.6102362204724416372, 0.07958543189024071263, -0.2665933059059888421 ) ) ;
#67867=CARTESIAN_POINT ( 'NONE',  ( 1.555118110236221041, 0.1660481256975883668, -0.3530559997133364547 ) ) ;
#67868=CARTESIAN_POINT ( 'NONE',  ( 0.2493438320209980519, -0.3690944881889765550, -0.3153832671262227771 ) ) ;
#67869=CARTESIAN_POINT ( 'NONE',  ( 0.2427821522309719648, -0.05778040916215522460, 0.4822834645669289988 ) ) ;
#67870=CARTESIAN_POINT ( 'NONE',  ( 0.7217847769028878924, -0.4281496062992127816, -0.4176697321401328100 ) ) ;
#67871=CARTESIAN_POINT ( 'NONE',  ( -0.3412073490813641308, 0.2306618581243847221, -0.2411417322834647770 ) ) ;
#67872=CARTESIAN_POINT ( 'NONE',  ( -0.07874015748031421014, -0.1870078740157480601, -0.3641732283464567677 ) ) ;
#67873=CARTESIAN_POINT ( 'NONE',  ( 0.9317585301837276734, -0.4281496062992124485, 0.4176697321401328655 ) ) ;
#67874=CARTESIAN_POINT ( 'NONE',  ( 0.8661417322834653598, -0.1870078740157479769, 0.3641732283464567677 ) ) ;
#67877=CARTESIAN_POINT ( 'NONE',  ( -1.036745406824146176, 0.05413385826771626580, -0.4176697321401330321 ) ) ;
#67880=CARTESIAN_POINT ( 'NONE',  ( -1.358267716535432434, -0.5400638737290844871, 0.3530559997133364547 ) ) ;
#67881=CARTESIAN_POINT ( 'NONE',  ( -0.4133858267716528645, 0.1660481256975883668, -0.3530559997133364547 ) ) ;
#67884=ORIENTED_EDGE ( 'NONE', *, *, #27570, .T. ) ;
#67885=CARTESIAN_POINT ( 'NONE',  ( 0.1443569553805781891, -0.004921259842519870586, -0.3153832671262229437 ) ) ;
#67887=CARTESIAN_POINT ( 'NONE',  ( 0.9580052493438326877, 0.05413385826771666132, 0.4176697321401328100 ) ) ;
#67891=CARTESIAN_POINT ( 'NONE',  ( -1.174540682414697335, -0.2845877964562161244, -0.3641732283464567121 ) ) ;
#67892=CARTESIAN_POINT ( 'NONE',  ( 1.679790026246720025, 0.2306618581243848609, 0.2411417322834645549 ) ) ;
#67893=CARTESIAN_POINT ( 'NONE',  ( 1.522309711286089939, -0.5023911411419708095, -0.1820866141732282451 ) ) ;
#67894=CARTESIAN_POINT ( 'NONE',  ( 0.5839895013123367340, 0.2952755905511811885, 0.1292274648535926551 ) ) ;
#67896=CARTESIAN_POINT ( 'NONE',  ( 0.03937007874015833325, -0.6692913385826771977, 8.415575281601705876E-17 ) ) ;
#67897=CARTESIAN_POINT ( 'NONE',  ( -1.062992125984250968, 0.1771653543307087630, 0.000000000000000000 ) ) ;
#67898=CARTESIAN_POINT ( 'NONE',  ( 0.4593175853018379162, -0.4281496062992124485, 0.4176697321401328655 ) ) ;
#67899=CARTESIAN_POINT ( 'NONE',  ( -0.07874015748031421014, -0.1870078740157480879, -0.4822834645669291653 ) ) ;
#67900=CARTESIAN_POINT ( 'NONE',  ( 0.5314960629921265944, 0.1660481256975883391, -0.3530559997133364547 ) ) ;
#67903=CARTESIAN_POINT ( 'NONE',  ( 0.7020997375328090762, -0.3162353388693405765, 0.4822834645669290543 ) ) ;
#67904=CARTESIAN_POINT ( 'NONE',  ( -0.3083989501312330295, -0.05778040916215522460, 0.4822834645669289988 ) ) ;
#67905=CARTESIAN_POINT ( 'NONE',  ( -1.036745406824146176, -0.4281496062992124485, 0.4176697321401328655 ) ) ;
#67907=CARTESIAN_POINT ( 'NONE',  ( 1.174540682414699111, -0.05778040916215560624, -0.4822834645669293319 ) ) ;
#67908=CARTESIAN_POINT ( 'NONE',  ( 0.6430446194225729606, -0.4281496062992127816, -0.4176697321401328100 ) ) ;
#67910=CARTESIAN_POINT ( 'NONE',  ( -0.5446194225721777693, -0.3162353388693409650, -0.4822834645669289433 ) ) ;
#67911=CARTESIAN_POINT ( 'NONE',  ( 0.4002624671916016896, -0.05778040916215522460, 0.4822834645669289988 ) ) ;
#67912=CARTESIAN_POINT ( 'NONE',  ( -0.3543307086614165824, 0.2952755905511811885, 0.000000000000000000 ) ) ;
#67913=CARTESIAN_POINT ( 'NONE',  ( 0.8267716535433078384, -0.5511811023622047445, 6.969142054262312111E-17 ) ) ;
#67914=CARTESIAN_POINT ( 'NONE',  ( 1.666666666666667185, -0.004921259842519576551, 0.3153832671262227771 ) ) ;
#67915=CARTESIAN_POINT ( 'NONE',  ( -1.732283464566928277, -0.1870078740157479769, 0.4822834645669291653 ) ) ;
#67916=CARTESIAN_POINT ( 'NONE',  ( 0.3608923884514443348, 0.2952755905511810774, -0.1292274648535930714 ) ) ;
#67918=ORIENTED_EDGE ( 'NONE', *, *, #7540, .F. ) ;
#67920=CARTESIAN_POINT ( 'NONE',  ( 0.5249343832021005074, -0.6046776061558807314, 0.2411417322834647770 ) ) ;
#67921=CARTESIAN_POINT ( 'NONE',  ( 0.6496062992125991586, 0.07958543189024085140, 0.2665933059059887866 ) ) ;
#67922=DIRECTION ( 'NONE',  ( 0.000000000000000000, 0.000000000000000000, -1.000000000000000000 ) ) ;
#67927=CARTESIAN_POINT ( 'NONE',  ( 0.9842519685039375910, 0.2952755905511811885, 0.000000000000000000 ) ) ;
#67928=CARTESIAN_POINT ( 'NONE',  ( -0.9251968503937002541, -0.5400638737290845981, -0.3530559997133363437 ) ) ;
#67929=CARTESIAN_POINT ( 'NONE',  ( -0.7020997375328076329, -0.3162353388693409650, -0.4822834645669289433 ) ) ;
#67930=CARTESIAN_POINT ( 'NONE',  ( 0.5052493438320215802, 0.2952755905511811885, 0.1292274648535926551 ) ) ;
#67931=CARTESIAN_POINT ( 'NONE',  ( 1.568241469816273437, -0.3162353388693405765, 0.4822834645669290543 ) ) ;
#67932=CARTESIAN_POINT ( 'NONE',  ( -1.168682819302786058, -2.294479370626195693E-15, 0.3464511005275217603 ) ) ;
#67934=CARTESIAN_POINT ( 'NONE',  ( 1.332020997375329197, -0.2845877964562159024, 0.3641732283464567677 ) ) ;
#67936=CARTESIAN_POINT ( 'NONE',  ( -1.181102362204723644, -0.1870078740157479769, 0.3641732283464567677 ) ) ;
#67938=CARTESIAN_POINT ( 'NONE',  ( 0.09842519685039434474, 0.1660481256975885056, 0.3530559997133364547 ) ) ;
#67939=CARTESIAN_POINT ( 'NONE',  ( 1.253280839895013710, -0.05778040916215560624, -0.4822834645669293319 ) ) ;
#67941=CARTESIAN_POINT ( 'NONE',  ( -1.279527559055116948, -0.4536011799217367080, 0.2665933059059888421 ) ) ;
#67942=CARTESIAN_POINT ( 'NONE',  ( 0.4265091863517067594, 0.2952755905511811885, 0.1292274648535926551 ) ) ;
#67943=CARTESIAN_POINT ( 'NONE',  ( 1.338582677165355062, -0.1870078740157480601, -0.3641732283464567677 ) ) ;
#67945=CARTESIAN_POINT ( 'NONE',  ( -1.036745406824146176, -0.004921259842519870586, -0.3153832671262229437 ) ) ;
#67946=CARTESIAN_POINT ( 'NONE',  ( 1.496062992125985147, -0.1870078740157479769, 0.4822834645669291653 ) ) ;
#67948=CARTESIAN_POINT ( 'NONE',  ( -0.3805774278215216522, -0.4281496062992127816, -0.4176697321401328100 ) ) ;
#67949=CARTESIAN_POINT ( 'NONE',  ( -1.469816272965878357, 0.1283753931104748280, 0.1820866141732283561 ) ) ;
#67950=CARTESIAN_POINT ( 'NONE',  ( -0.7808398950131225646, -0.05778040916215522460, 0.4822834645669289988 ) ) ;
#67951=CARTESIAN_POINT ( 'NONE',  ( -1.509186351706035767, -0.3690944881889763329, 0.3153832671262228327 ) ) ;
#67953=CARTESIAN_POINT ( 'NONE',  ( 0.4986876640419954376, 0.2306618581243848609, 0.2411417322834645549 ) ) ;
#67954=LINE ( 'NONE', #34411, #18475 ) ;
#67955=CARTESIAN_POINT ( 'NONE',  ( 1.384514435695538337, -0.6692913385826771977, 0.1292274648535927661 ) ) ;
#67958=CARTESIAN_POINT ( 'NONE',  ( -1.332020997375327642, -0.3162353388693409650, -0.4822834645669289433 ) ) ;
#67959=CARTESIAN_POINT ( 'NONE',  ( -1.108923884514435132, -0.08942795157528024563, -0.3641732283464568787 ) ) ;
#67960=CARTESIAN_POINT ( 'NONE',  ( -0.5314960629921254842, -0.4536011799217368745, -0.2665933059059886201 ) ) ;
#67961=CARTESIAN_POINT ( 'NONE',  ( -0.5384083780239481420, 0.004960608223778821026, 0.3437734562760189072 ) ) ;
#67962=CARTESIAN_POINT ( 'NONE',  ( 0.2362204724409456558, -0.1870078740157479769, 0.4822834645669291653 ) ) ;
#67963=CARTESIAN_POINT ( 'NONE',  ( 0.4002624671916016896, -0.08942795157527998196, 0.3641732283464567121 ) ) ;
#67964=CARTESIAN_POINT ( 'NONE',  ( -0.9842519685039365918, -0.5511811023622047445, 6.969142054262312111E-17 ) ) ;
#67965=CARTESIAN_POINT ( 'NONE',  ( -1.437007874015747477, -0.5400638737290844871, 0.3530559997133364547 ) ) ;
#67966=CARTESIAN_POINT ( 'NONE',  ( 1.541994750656168645, -0.5511811023622046335, 0.09757992244046803654 ) ) ;
#67967=CARTESIAN_POINT ( 'NONE',  ( 1.377952755905512472, 0.2952755905511811885, 0.000000000000000000 ) ) ;
#67969=CARTESIAN_POINT ( 'NONE',  ( 0.3018372703412079971, -0.004921259842519870586, -0.3153832671262229437 ) ) ;
#67970=CARTESIAN_POINT ( 'NONE',  ( 0.9842519685039378130, -0.6692913385826771977, 8.415575281601705876E-17 ) ) ;
#67971=CARTESIAN_POINT ( 'NONE',  ( -1.604771003085130543, 0.7270283685441724097, 0.1466069496707740338 ) ) ;
#67972=CARTESIAN_POINT ( 'NONE',  ( 1.017060367454068581, -0.08942795157528024563, -0.3641732283464568787 ) ) ;
#67973=ORIENTED_EDGE ( 'NONE', *, *, #5358, .T. ) ;
#67974=CARTESIAN_POINT ( 'NONE',  ( -1.286089238845143479, 0.2306618581243847221, -0.2411417322834647770 ) ) ;
#67975=EDGE_CURVE ( 'NONE', #80562, #43140, #1470, .T. ) ;
#67976=CARTESIAN_POINT ( 'NONE',  ( -0.7874015748031489847, -0.1870078740157480879, -0.4822834645669291653 ) ) ;
#67977=CARTESIAN_POINT ( 'NONE',  ( 0.04593175853018440641, 0.2952755905511810774, -0.1292274648535930714 ) ) ;
#67980=CARTESIAN_POINT ( 'NONE',  ( 1.049868766404200127, -0.6046776061558809534, -0.2411417322834644161 ) ) ;
#67981=CARTESIAN_POINT ( 'NONE',  ( -1.725721784776902190, -0.05778040916215522460, 0.4822834645669289988 ) ) ;
#67982=CARTESIAN_POINT ( 'NONE',  ( -0.01968503937007793844, 0.1660481256975883668, -0.3530559997133364547 ) ) ;
#67983=CARTESIAN_POINT ( 'NONE',  ( 0.7480314960629927956, -0.6692913385826771977, 8.415575281601705876E-17 ) ) ;
#67989=CARTESIAN_POINT ( 'NONE',  ( -0.2559055118110230564, 0.07958543189024071263, -0.2665933059059888421 ) ) ;
#67990=CARTESIAN_POINT ( 'NONE',  ( -0.7939632545931754048, -0.3162353388693405765, 0.4822834645669290543 ) ) ;
#67991=CARTESIAN_POINT ( 'NONE',  ( 0.6758530183727039509, 0.2952755905511810774, -0.1292274648535930714 ) ) ;
#67993=CARTESIAN_POINT ( 'NONE',  ( -0.3412073490813641308, 0.1283753931104746893, -0.1820866141732285504 ) ) ;
#67994=CARTESIAN_POINT ( 'NONE',  ( 1.614173228346457378, 0.2952755905511811885, 0.000000000000000000 ) ) ;
#67995=CARTESIAN_POINT ( 'NONE',  ( 1.076115485564305141, -0.6046776061558807314, 0.2411417322834647770 ) ) ;
#67998=FACE_OUTER_BOUND ( 'NONE', #63650, .T. ) ;
#68000=ORIENTED_EDGE ( 'NONE', *, *, #17343, .T. ) ;
#68001=CARTESIAN_POINT ( 'NONE',  ( 1.148293963254593653, 0.2952755905511810774, -0.1292274648535930714 ) ) ;
#68002=CARTESIAN_POINT ( 'NONE',  ( 1.141732283464567566, 0.1771653543307087630, 0.000000000000000000 ) ) ;
#68003=CARTESIAN_POINT ( 'NONE',  ( -1.430446194225720724, -0.004921259842519870586, -0.3153832671262229437 ) ) ;
#68004=CARTESIAN_POINT ( 'NONE',  ( -1.417322834645668772, -0.1870078740157480879, -0.4822834645669291653 ) ) ;
#68006=CARTESIAN_POINT ( 'NONE',  ( -0.9776902887139098386, 0.2066929133858267098, -0.1054918080437494132 ) ) ;
#68007=CARTESIAN_POINT ( 'NONE',  ( 1.108923884514436686, -0.3162353388693409650, -0.4822834645669289433 ) ) ;
#68008=CARTESIAN_POINT ( 'NONE',  ( -1.587926509186350810, -0.4281496062992124485, 0.4176697321401328655 ) ) ;
#68009=CARTESIAN_POINT ( 'NONE',  ( -0.5052493438320203589, -0.6692913385826771977, 0.1292274648535927661 ) ) ;
#68010=CARTESIAN_POINT ( 'NONE',  ( -0.4265091863517051496, 0.2952755905511810774, -0.1292274648535930714 ) ) ;
#68012=CARTESIAN_POINT ( 'NONE',  ( 1.535433070866142335, -0.6692913385826771977, 8.415575281601705876E-17 ) ) ;
#68014=CARTESIAN_POINT ( 'NONE',  ( 0.1968503937007881344, 0.2952755905511811885, 0.000000000000000000 ) ) ;
#68016=CARTESIAN_POINT ( 'NONE',  ( -1.574803149606298192, -0.1870078740157480601, -0.3641732283464567677 ) ) ;
#68020=CARTESIAN_POINT ( 'NONE',  ( -0.05905511811023543556, 0.1012011053420777407, 0.2882089793578256898 ) ) ;
#68022=CARTESIAN_POINT ( 'NONE',  ( -1.404199475065615932, 0.05413385826771666132, 0.4176697321401328100 ) ) ;
#68028=CARTESIAN_POINT ( 'NONE',  ( -0.1246719160104980823, -0.5511811023622048555, -0.09757992244046775898 ) ) ;
#68029=CARTESIAN_POINT ( 'NONE',  ( -1.128608923884513837, -0.5023911411419708095, 0.1820866141732285504 ) ) ;
#68030=CARTESIAN_POINT ( 'NONE',  ( -1.509186351706035767, -0.4281496062992124485, 0.4176697321401328655 ) ) ;
#68031=CARTESIAN_POINT ( 'NONE',  ( 0.3346456692913390985, 0.1660481256975885056, 0.3530559997133364547 ) ) ;
#68032=CARTESIAN_POINT ( 'NONE',  ( -1.489501312335957062, -0.05778040916215522460, 0.4822834645669289988 ) ) ;
#68035=CARTESIAN_POINT ( 'NONE',  ( -1.450131233595799651, 0.2952755905511810774, -0.1292274648535930714 ) ) ;
#68040=ADVANCED_FACE ( 'NONE', ( #52741 ), #66228, .F. ) ;
#68042=CARTESIAN_POINT ( 'NONE',  ( -0.6692913385826764205, 0.2952755905511811885, 0.000000000000000000 ) ) ;
#68043=CARTESIAN_POINT ( 'NONE',  ( 1.522309711286089939, 0.2306618581243848609, 0.2411417322834645549 ) ) ;
#68044=CARTESIAN_POINT ( 'NONE',  ( -1.568241469816272105, -0.05778040916215522460, 0.4822834645669289988 ) ) ;
#68045=DIRECTION ( 'NONE',  ( 0.000000000000000000, 0.000000000000000000, -1.000000000000000000 ) ) ;
#68046=CARTESIAN_POINT ( 'NONE',  ( -1.660104986876639543, -0.05778040916215560624, -0.4822834645669293319 ) ) ;
#68047=CARTESIAN_POINT ( 'NONE',  ( -0.7086614173228339419, -0.1870078740157480879, -0.4822834645669291653 ) ) ;
#68049=CARTESIAN_POINT ( 'NONE',  ( 0.2296587926509192634, -0.08942795157528024563, -0.3641732283464568787 ) ) ;
#68051=CARTESIAN_POINT ( 'NONE',  ( -0.01312335958005186876, -0.004921259842519870586, -0.3153832671262229437 ) ) ;
#68052=CARTESIAN_POINT ( 'NONE',  ( 0.7677165354330716118, -0.4536011799217367080, 0.2665933059059888421 ) ) ;
#68053=CARTESIAN_POINT ( 'NONE',  ( 0.4790026246719167324, -0.05778040916215522460, 0.4822834645669289988 ) ) ;
#68054=CARTESIAN_POINT ( 'NONE',  ( -0.2427821522309703550, -0.2845877964562159024, 0.3641732283464567677 ) ) ;
#68056=CARTESIAN_POINT ( 'NONE',  ( 1.594488188976378673, 0.1660481256975885056, 0.3530559997133364547 ) ) ;
#68058=CARTESIAN_POINT ( 'NONE',  ( -1.003937007874014853, 0.1660481256975885056, 0.3530559997133364547 ) ) ;
#68061=VECTOR ( 'NONE', #77822, 39.37007874015748143 ) ;
#68062=CARTESIAN_POINT ( 'NONE',  ( 0.2296587926509192634, -0.05778040916215560624, -0.4822834645669293319 ) ) ;
#68063=CARTESIAN_POINT ( 'NONE',  ( -0.5774278215223089816, -0.6046776061558807314, 0.2411417322834647770 ) ) ;
#68064=FACE_OUTER_BOUND ( 'NONE', #54856, .T. ) ;
#68065=CARTESIAN_POINT ( 'NONE',  ( 0.02624671916010564918, 0.1283753931104748280, 0.1820866141732283561 ) ) ;
#68066=CARTESIAN_POINT ( 'NONE',  ( -0.2493438320209966919, 0.05413385826771626580, -0.4176697321401330321 ) ) ;
#68067=CARTESIAN_POINT ( 'NONE',  ( -0.5708661417322825615, -0.5400638737290844871, 0.3530559997133364547 ) ) ;
#68068=FACE_OUTER_BOUND ( 'NONE', #61287, .T. ) ;
#68069=CARTESIAN_POINT ( 'NONE',  ( 1.574803149606299746, -0.1870078740157480601, -0.3641732283464567677 ) ) ;
#68070=CARTESIAN_POINT ( 'NONE',  ( 0.2690288713910767848, 0.2952755905511811885, 0.1292274648535926551 ) ) ;
#68072=CARTESIAN_POINT ( 'NONE',  ( 1.522309711286089939, -0.6046776061558809534, -0.2411417322834644161 ) ) ;
#68073=CARTESIAN_POINT ( 'NONE',  ( -0.8005249343832013809, -0.3690944881889763329, 0.3153832671262228327 ) ) ;
#68075=CARTESIAN_POINT ( 'NONE',  ( -0.6955380577427815458, -0.4281496062992127816, -0.4176697321401328100 ) ) ;
#68076=CARTESIAN_POINT ( 'NONE',  ( 1.345144356955381593, -0.05778040916215522460, 0.4822834645669289988 ) ) ;
#68077=CARTESIAN_POINT ( 'NONE',  ( 1.233595800524935227, 0.2306618581243847221, -0.2411417322834647770 ) ) ;
#68079=CARTESIAN_POINT ( 'NONE',  ( -1.010498687664041384, -0.3690944881889765550, -0.3153832671262227771 ) ) ;
#68083=CARTESIAN_POINT ( 'NONE',  ( -0.7480314960629922405, 2.001539355558159983, 0.000000000000000000 ) ) ;
#68084=CARTESIAN_POINT ( 'NONE',  ( 1.062992125984252745, -0.5511811023622047445, 6.969142054262312111E-17 ) ) ;
#68085=CARTESIAN_POINT ( 'NONE',  ( 0.8727034120734912248, -0.3162353388693409650, -0.4822834645669289433 ) ) ;
#68086=CARTESIAN_POINT ( 'NONE',  ( -1.640419947506561060, -0.4281496062992127816, -0.4176697321401328100 ) ) ;
#68087=CARTESIAN_POINT ( 'NONE',  ( 0.8661417322834652488, -0.1870078740157480879, -0.4822834645669291653 ) ) ;
#68089=CARTESIAN_POINT ( 'NONE',  ( 1.220472440944882608, 0.1771653543307087630, 0.000000000000000000 ) ) ;
#68090=CARTESIAN_POINT ( 'NONE',  ( 0.2296587926509192634, -0.3162353388693405765, 0.4822834645669290543 ) ) ;
#68091=CARTESIAN_POINT ( 'NONE',  ( -0.9514435695538050464, -0.05778040916215560624, -0.4822834645669293319 ) ) ;
#68092=CARTESIAN_POINT ( 'NONE',  ( 1.292650918635171564, -0.6692913385826773087, -0.1292274648535924053 ) ) ;
#68095=CARTESIAN_POINT ( 'NONE',  ( 0.4593175853018379162, -0.3690944881889763329, 0.3153832671262228327 ) ) ;
#68099=CARTESIAN_POINT ( 'NONE',  ( -0.6758530183727028406, -0.6692913385826773087, -0.1292274648535924053 ) ) ;
#68100=CARTESIAN_POINT ( 'NONE',  ( -0.2034120734908128059, 0.2952755905511811885, 0.1292274648535926551 ) ) ;
#68101=CARTESIAN_POINT ( 'NONE',  ( -0.5052493438320203589, 0.2952755905511810774, -0.1292274648535930714 ) ) ;
#68102=CARTESIAN_POINT ( 'NONE',  ( 0.9251968503937015864, 0.1660481256975883668, -0.3530559997133364547 ) ) ;
#68103=CARTESIAN_POINT ( 'NONE',  ( -1.292650918635170010, 0.2952755905511810774, -0.1292274648535930714 ) ) ;
#68104=CARTESIAN_POINT ( 'NONE',  ( -0.3674540682414692561, -0.6046776061558809534, -0.2411417322834644161 ) ) ;
#68105=CARTESIAN_POINT ( 'NONE',  ( 1.338582677165355062, -0.1870078740157480879, -0.4822834645669291653 ) ) ;
#68106=CARTESIAN_POINT ( 'NONE',  ( 0.4724409448818904789, -0.1870078740157479769, 0.4822834645669291653 ) ) ;
#68107=CARTESIAN_POINT ( 'NONE',  ( 0.6167979002624679463, 0.05413385826771626580, -0.4176697321401330321 ) ) ;
#68109=CARTESIAN_POINT ( 'NONE',  ( -0.6036745406824141069, -0.5023911411419708095, -0.1820866141732282451 ) ) ;
#68110=ORIENTED_EDGE ( 'NONE', *, *, #54370, .T. ) ;
#68114=CARTESIAN_POINT ( 'NONE',  ( -0.9120734908136475250, 0.1771653543307087630, 0.09757992244046791164 ) ) ;
#68116=AXIS2_PLACEMENT_3D ( 'NONE', #13634, #9291, #34962 ) ;
#68117=CARTESIAN_POINT ( 'NONE',  ( -0.2755905511811015396, -0.6692913385826771977, 8.415575281601705876E-17 ) ) ;
#68119=CARTESIAN_POINT ( 'NONE',  ( -0.6036745406824141069, 0.2306618581243848609, 0.2411417322834645549 ) ) ;
#68120=CARTESIAN_POINT ( 'NONE',  ( -1.043307086614172707, 0.1660481256975883668, -0.3530559997133364547 ) ) ;
#68121=CARTESIAN_POINT ( 'NONE',  ( -1.377952755905511140, -0.6692913385826771977, 8.415575281601705876E-17 ) ) ;
#68122=CARTESIAN_POINT ( 'NONE',  ( -1.450131233595799651, -0.6692913385826771977, 0.1292274648535927661 ) ) ;
#68123=CARTESIAN_POINT ( 'NONE',  ( 0.7414698162729663755, 0.1771653543307087630, 0.09757992244046791164 ) ) ;
#68124=LINE ( 'NONE', #29393, #72659 ) ;
#68126=CARTESIAN_POINT ( 'NONE',  ( 0.2427821522309716595, -0.2845877964562161244, -0.3641732283464567121 ) ) ;
#68127=CARTESIAN_POINT ( 'NONE',  ( 0.01968503937007957949, -0.5400638737290845981, -0.3530559997133363437 ) ) ;
#68128=CARTESIAN_POINT ( 'NONE',  ( -0.2493438320209966919, -0.4281496062992124485, 0.4176697321401328655 ) ) ;
#68129=VERTEX_POINT ( 'NONE', #80117 ) ;
#68132=EDGE_LOOP ( 'NONE', ( #43990, #35699, #40021, #72589 ) ) ;
#68134=CARTESIAN_POINT ( 'NONE',  ( 1.548556430446194954, -0.6046776061558807314, 0.2411417322834647770 ) ) ;
#68135=CARTESIAN_POINT ( 'NONE',  ( -0.6036745406824141069, 0.1283753931104748280, 0.1820866141732283561 ) ) ;
#68136=CARTESIAN_POINT ( 'NONE',  ( -1.102362204724408601, -0.1870078740157479769, 0.4822834645669291653 ) ) ;
#68140=CARTESIAN_POINT ( 'NONE',  ( 1.692913385826772421, 0.2952755905511811885, 0.000000000000000000 ) ) ;
#68141=CARTESIAN_POINT ( 'NONE',  ( 0.3674540682414705883, 0.2306618581243847221, -0.2411417322834647770 ) ) ;
#68142=CARTESIAN_POINT ( 'NONE',  ( 0.6102362204724416372, 0.1660481256975883668, -0.3530559997133364547 ) ) ;
#68143=CARTESIAN_POINT ( 'NONE',  ( -0.6233595800524928121, -0.2845877964562161244, -0.3641732283464567121 ) ) ;
#68144=CARTESIAN_POINT ( 'NONE',  ( -0.09186351706036689768, 0.05413385826771626580, -0.4176697321401330321 ) ) ;
#68147=CARTESIAN_POINT ( 'NONE',  ( -0.6430446194225716283, -0.4281496062992124485, 0.4176697321401328655 ) ) ;
#68149=CARTESIAN_POINT ( 'NONE',  ( 1.187664041994751285, -0.2845877964562161244, -0.3641732283464567121 ) ) ;
#68150=CARTESIAN_POINT ( 'NONE',  ( 0.06561679790026316017, -0.004921259842519870586, -0.3153832671262229437 ) ) ;
#68151=CARTESIAN_POINT ( 'NONE',  ( 1.292650918635171564, -0.5511811023622048555, -0.09757992244046775898 ) ) ;
#68152=CARTESIAN_POINT ( 'NONE',  ( -1.279527559055116948, -0.5400638737290844871, 0.3530559997133364547 ) ) ;
#68153=CARTESIAN_POINT ( 'NONE',  ( -1.082677165354329896, -0.4536011799217368745, -0.2665933059059886201 ) ) ;
#68154=DIRECTION ( 'NONE',  ( -1.000000000000000000, 0.000000000000000000, 1.692413147294446216E-16 ) ) ;
#68155=CARTESIAN_POINT ( 'NONE',  ( -0.9908136482939626788, -0.6692913385826773087, -0.1292274648535924053 ) ) ;
#68156=CARTESIAN_POINT ( 'NONE',  ( -0.2755905511811015396, -0.6692913385826771977, 8.415575281601705876E-17 ) ) ;
#68157=CARTESIAN_POINT ( 'NONE',  ( 0.4527559055118117182, 0.1660481256975883668, -0.3530559997133364547 ) ) ;
#68159=CARTESIAN_POINT ( 'NONE',  ( 1.091663011964304930, -3.876714527516387216E-16, -0.4118477457932991359 ) ) ;
#68160=CARTESIAN_POINT ( 'NONE',  ( 0.1377952755905518800, 0.07958543189024071263, -0.2665933059059888421 ) ) ;
#68161=CARTESIAN_POINT ( 'NONE',  ( -1.515748031496062076, 0.07958543189024071263, -0.2665933059059888421 ) ) ;
#68162=EDGE_CURVE ( 'NONE', #22548, #36796, #3080, .T. ) ;
#68163=CARTESIAN_POINT ( 'NONE',  ( 0.7939632545931766261, -0.3162353388693409650, -0.4822834645669289433 ) ) ;
#68165=CARTESIAN_POINT ( 'NONE',  ( 1.312335958005249825, 0.1283753931104746893, -0.1820866141732285504 ) ) ;
#68166=CARTESIAN_POINT ( 'NONE',  ( -0.7874015748031489847, -0.1870078740157479769, 0.4822834645669291653 ) ) ;
#68167=CARTESIAN_POINT ( 'NONE',  ( -0.07874015748031421014, -0.1870078740157479769, 0.3641732283464567677 ) ) ;
#68169=CARTESIAN_POINT ( 'NONE',  ( 0.7939632545931766261, -0.08942795157527998196, 0.3641732283464567121 ) ) ;
#68171=AXIS2_PLACEMENT_3D ( 'NONE', #66646, #80531, #72540 ) ;
#68172=CARTESIAN_POINT ( 'NONE',  ( -0.2230971128608915943, 0.05413385826771666132, 0.4176697321401328100 ) ) ;
#68174=VECTOR ( 'NONE', #68154, 39.37007874015748143 ) ;
#68176=CARTESIAN_POINT ( 'NONE',  ( 0.8398950131233602345, 0.1283753931104746893, -0.1820866141732285504 ) ) ;
#68177=CARTESIAN_POINT ( 'NONE',  ( 0.02624671916010564918, -0.6046776061558809534, -0.2411417322834644161 ) ) ;
#68180=CARTESIAN_POINT ( 'NONE',  ( -0.4855643044619415427, 0.05413385826771626580, -0.4176697321401330321 ) ) ;
#68181=CARTESIAN_POINT ( 'NONE',  ( -0.5971128608923877978, -0.5511811023622048555, -0.09757992244046775898 ) ) ;
#68182=CARTESIAN_POINT ( 'NONE',  ( 0.9580052493438326877, 0.009842519685039463617, 0.3409548833797002576 ) ) ;
#68183=CARTESIAN_POINT ( 'NONE',  ( -0.5774278215223089816, -0.5023911411419708095, 0.1820866141732285504 ) ) ;
#68184=CARTESIAN_POINT ( 'NONE',  ( 0.5249343832021005074, -0.6046776061558807314, 0.2411417322834647770 ) ) ;
#68185=CARTESIAN_POINT ( 'NONE',  ( -1.003937007874015297, -0.4536011799217368745, -0.2665933059059886201 ) ) ;
#68187=CARTESIAN_POINT ( 'NONE',  ( -1.397637795275589623, -0.5400638737290845981, -0.3530559997133363437 ) ) ;
#68190=CARTESIAN_POINT ( 'NONE',  ( -1.423884514435694859, -0.2845877964562159024, 0.3641732283464567677 ) ) ;
#68191=CARTESIAN_POINT ( 'NONE',  ( -0.4790026246719154557, -0.3162353388693405765, 0.4822834645669290543 ) ) ;
#68193=CARTESIAN_POINT ( 'NONE',  ( -1.069553805774277722, -0.6692913385826773087, -0.1292274648535924053 ) ) ;
#68196=CARTESIAN_POINT ( 'NONE',  ( 1.384514435695538559, 0.2952755905511810774, -0.1292274648535930714 ) ) ;
#68197=CARTESIAN_POINT ( 'NONE',  ( 0.4527559055118117182, 0.1660481256975883668, -0.3530559997133364547 ) ) ;
#68200=CARTESIAN_POINT ( 'NONE',  ( 1.502624671916010790, -0.2845877964562161244, -0.3641732283464567121 ) ) ;
#68203=EDGE_CURVE ( 'NONE', #24205, #35380, #21191, .T. ) ;
#68204=CARTESIAN_POINT ( 'NONE',  ( -0.7480314960629914633, -0.5511811023622047445, 6.969142054262312111E-17 ) ) ;
#68206=ORIENTED_EDGE ( 'NONE', *, *, #4912, .F. ) ;
#68207=CARTESIAN_POINT ( 'NONE',  ( 1.017060367454068581, -0.05778040916215560624, -0.4822834645669293319 ) ) ;
#68208=CARTESIAN_POINT ( 'NONE',  ( -0.4068241469816267775, 0.05413385826771626580, -0.4176697321401330321 ) ) ;
#68209=CARTESIAN_POINT ( 'NONE',  ( -1.056430446194224881, -0.6692913385826771977, 0.1292274648535927661 ) ) ;
#68210=CARTESIAN_POINT ( 'NONE',  ( 1.003937007874016407, -0.5400638737290844871, 0.3530559997133364547 ) ) ;
#68211=CARTESIAN_POINT ( 'NONE',  ( -1.194225721784776262, -0.3690944881889763329, 0.3153832671262228327 ) ) ;
#68213=CARTESIAN_POINT ( 'NONE',  ( 0.1509186351706045259, -0.05778040916215560624, -0.4822834645669293319 ) ) ;
#68214=CARTESIAN_POINT ( 'NONE',  ( -0.9514435695538050464, -0.05778040916215560624, -0.4822834645669293319 ) ) ;
#68217=CARTESIAN_POINT ( 'NONE',  ( 1.535433070866142335, -0.6692913385826771977, 8.415575281601705876E-17 ) ) ;
#68220=CARTESIAN_POINT ( 'NONE',  ( 0.8858267716535438430, 0.1660481256975885056, 0.3530559997133364547 ) ) ;
#68222=CARTESIAN_POINT ( 'NONE',  ( 0.9908136482939640111, -0.5511811023622046335, 0.09757992244046803654 ) ) ;
#68225=CARTESIAN_POINT ( 'NONE',  ( -0.3149606299212590610, -0.1870078740157480879, -0.4822834645669291653 ) ) ;
#68227=CARTESIAN_POINT ( 'NONE',  ( 0.4855643044619428750, -0.004921259842519576551, 0.3153832671262227771 ) ) ;
#68228=CARTESIAN_POINT ( 'NONE',  ( -1.706036745406823485, 0.2306618581243848609, 0.2411417322834645549 ) ) ;
#68229=CARTESIAN_POINT ( 'NONE',  ( 0.5971128608923890191, -0.6692913385826771977, 0.1292274648535927661 ) ) ;
#68230=CARTESIAN_POINT ( 'NONE',  ( 0.3215223097112867578, -0.05778040916215522460, 0.4822834645669289988 ) ) ;
#68231=CARTESIAN_POINT ( 'NONE',  ( -0.06561679790026180015, -0.4281496062992127816, -0.4176697321401328100 ) ) ;
#68233=CARTESIAN_POINT ( 'NONE',  ( -0.9580052493438311334, 0.05413385826771626580, -0.4176697321401330321 ) ) ;
#68235=CARTESIAN_POINT ( 'NONE',  ( 1.581364829396326277, -0.08942795157527998196, 0.3641732283464567121 ) ) ;
#68236=CARTESIAN_POINT ( 'NONE',  ( -1.141732283464566011, 0.2952755905511811885, 0.000000000000000000 ) ) ;
#68237=CARTESIAN_POINT ( 'NONE',  ( 1.371391076115485941, 0.2952755905511811885, 0.1292274648535926551 ) ) ;
#68238=CARTESIAN_POINT ( 'NONE',  ( 1.358267716535433323, 0.1660481256975885056, 0.3530559997133364547 ) ) ;
#68240=CARTESIAN_POINT ( 'NONE',  ( -0.8070866141732276899, -0.5400638737290844871, 0.3530559997133364547 ) ) ;
#68242=CARTESIAN_POINT ( 'NONE',  ( 0.09842519685039434474, -0.5400638737290845981, -0.3530559997133363437 ) ) ;
#68244=CARTESIAN_POINT ( 'NONE',  ( -0.6036745406824141069, -0.6046776061558809534, -0.2411417322834644161 ) ) ;
#68246=CARTESIAN_POINT ( 'NONE',  ( 1.686351706036745890, 0.2952755905511811885, 0.1292274648535926551 ) ) ;
#68247=CARTESIAN_POINT ( 'NONE',  ( 0.7152230971128616943, -0.08942795157527998196, 0.3641732283464567121 ) ) ;
#68248=CARTESIAN_POINT ( 'NONE',  ( 1.345144356955381593, -0.3162353388693409650, -0.4822834645669289433 ) ) ;
#68250=CARTESIAN_POINT ( 'NONE',  ( 0.5643044619422579178, -0.004921259842519576551, 0.3153832671262227771 ) ) ;
#68251=CARTESIAN_POINT ( 'NONE',  ( 0.9973753280839902091, 0.2306618581243847221, -0.2411417322834647770 ) ) ;
#68253=CARTESIAN_POINT ( 'NONE',  ( -0.5905511811023615998, 0.2952755905511811885, 0.000000000000000000 ) ) ;
#68255=CARTESIAN_POINT ( 'NONE',  ( 1.148293963254593653, 0.1771653543307087075, -0.09757992244046823083 ) ) ;
#68256=CARTESIAN_POINT ( 'NONE',  ( -0.7020997375328076329, -0.3162353388693409650, -0.4822834645669289433 ) ) ;
#68257=CARTESIAN_POINT ( 'NONE',  ( 0.2034120734908142214, 0.2952755905511810774, -0.1292274648535930714 ) ) ;
#68258=CARTESIAN_POINT ( 'NONE',  ( 0.1312335958005257930, 0.1539470093639521697, -0.1968503937007875793 ) ) ;
#68259=CARTESIAN_POINT ( 'NONE',  ( 0.2362204724409456558, -0.1870078740157480879, -0.4822834645669291653 ) ) ;
#68260=CARTESIAN_POINT ( 'NONE',  ( -0.01312335958005186876, -0.004921259842519870586, -0.3153832671262229437 ) ) ;
#68262=CARTESIAN_POINT ( 'NONE',  ( 0.06561679790026316017, -0.3690944881889763329, 0.3153832671262228327 ) ) ;
#68263=CARTESIAN_POINT ( 'NONE',  ( 0.6167979002624678353, -0.3690944881889763329, 0.3153832671262228327 ) ) ;
#68266=CARTESIAN_POINT ( 'NONE',  ( 0.3149606299212606708, -0.1870078740157480879, -0.4822834645669291653 ) ) ;
#68269=CARTESIAN_POINT ( 'NONE',  ( 0.09032602383071736130, 0.02791078216816225699, 0.4328096321851905293 ) ) ;
#68270=CARTESIAN_POINT ( 'NONE',  ( -0.4986876640419942164, -0.5023911411419708095, 0.1820866141732285504 ) ) ;
#68271=EDGE_CURVE ( 'NONE', #9475, #76877, #2249, .T. ) ;
#68272=CARTESIAN_POINT ( 'NONE',  ( 0.2493438320209980519, 0.05413385826771666132, 0.4176697321401328100 ) ) ;
#68273=CARTESIAN_POINT ( 'NONE',  ( 0.9842519685039378130, -0.5511811023622047445, 6.969142054262312111E-17 ) ) ;
#68274=CARTESIAN_POINT ( 'NONE',  ( -1.489501312335957062, -0.2845877964562161244, -0.3641732283464567121 ) ) ;
#68275=CARTESIAN_POINT ( 'NONE',  ( -1.607611548556429737, -0.6692913385826771977, 0.1292274648535927661 ) ) ;
#68276=CARTESIAN_POINT ( 'NONE',  ( 0.1509186351706045259, -0.05778040916215560624, -0.4822834645669293319 ) ) ;
#68277=CARTESIAN_POINT ( 'NONE',  ( 1.259842519685040019, -0.1870078740157480879, -0.4822834645669291653 ) ) ;
#68278=CARTESIAN_POINT ( 'NONE',  ( 1.614173228346457378, 0.7794589730112001513, -0.1372047244094476148 ) ) ;
#68279=CARTESIAN_POINT ( 'NONE',  ( 0.2296587926509192634, -0.05778040916215560624, -0.4822834645669293319 ) ) ;
#68280=CARTESIAN_POINT ( 'NONE',  ( 1.509186351706037543, 0.05413385826771666132, 0.4176697321401328100 ) ) ;
#68281=CARTESIAN_POINT ( 'NONE',  ( 1.161417322834646493, -0.5400638737290844871, 0.3530559997133364547 ) ) ;
#68283=CARTESIAN_POINT ( 'NONE',  ( 0.7742782152230979209, -0.004921259842519870586, -0.3153832671262229437 ) ) ;
#68284=CARTESIAN_POINT ( 'NONE',  ( 1.437007874015748810, -0.5400638737290845981, -0.3530559997133363437 ) ) ;
#68285=CARTESIAN_POINT ( 'NONE',  ( -0.1049868766404193215, 0.1283753931104746893, -0.1820866141732285504 ) ) ;
#68286=CARTESIAN_POINT ( 'NONE',  ( -0.1443569553805765515, -0.4281496062992127816, -0.4176697321401328100 ) ) ;
#68287=CARTESIAN_POINT ( 'NONE',  ( 0.8792650918635177559, -0.4281496062992127816, -0.4176697321401328100 ) ) ;
#68288=CARTESIAN_POINT ( 'NONE',  ( -0.5446194225721777693, -0.05778040916215522460, 0.4822834645669289988 ) ) ;
#68290=CARTESIAN_POINT ( 'NONE',  ( -0.3477690288713905509, -0.5511811023622046335, 0.09757992244046803654 ) ) ;
#68291=CARTESIAN_POINT ( 'NONE',  ( 0.9645669291338588858, 0.1660481256975885056, 0.3530559997133364547 ) ) ;
#68292=CARTESIAN_POINT ( 'NONE',  ( 0.8005249343832028242, -0.3690944881889765550, -0.3153832671262227771 ) ) ;
#68295=CARTESIAN_POINT ( 'NONE',  ( 1.614173228346457378, 0.2952755905511811885, 0.000000000000000000 ) ) ;
#68298=CARTESIAN_POINT ( 'NONE',  ( -1.305774278215222184, 0.2952755905511811885, 0.1292274648535926551 ) ) ;
#68299=CARTESIAN_POINT ( 'NONE',  ( -0.3740157480314953431, -0.5400638737290845981, -0.3530559997133363437 ) ) ;
#68303=CARTESIAN_POINT ( 'NONE',  ( 0.4068241469816281097, -0.004921259842519576551, 0.3153832671262227771 ) ) ;
#68305=CARTESIAN_POINT ( 'NONE',  ( 1.102362204724410155, -0.1870078740157479769, 0.4822834645669291653 ) ) ;
#68309=CARTESIAN_POINT ( 'NONE',  ( 1.246719160104987623, -0.3690944881889763329, 0.3153832671262228327 ) ) ;
#68310=CARTESIAN_POINT ( 'NONE',  ( 0.4658792650918641698, -0.05778040916215560624, -0.4822834645669293319 ) ) ;
#68312=CARTESIAN_POINT ( 'NONE',  ( -0.03280839895013062252, 0.2952755905511810774, -0.1292274648535930714 ) ) ;
#68313=CARTESIAN_POINT ( 'NONE',  ( -0.8792650918635160906, -0.004921259842519870586, -0.3153832671262229437 ) ) ;
#68314=CARTESIAN_POINT ( 'NONE',  ( 0.3018372703412079971, -0.4281496062992124485, 0.4176697321401328655 ) ) ;
#68315=CARTESIAN_POINT ( 'NONE',  ( 0.1443569553805781891, -0.4281496062992124485, 0.4176697321401328655 ) ) ;
#68316=DIRECTION ( 'NONE',  ( 0.000000000000000000, 1.000000000000000000, 0.000000000000000000 ) ) ;
#68319=CARTESIAN_POINT ( 'NONE',  ( 0.6692913385826778638, -0.6692913385826771977, 8.415575281601705876E-17 ) ) ;
#68320=CARTESIAN_POINT ( 'NONE',  ( -0.2427821522309703550, -0.05778040916215560624, -0.4822834645669293319 ) ) ;
#68321=CARTESIAN_POINT ( 'NONE',  ( -1.266404199475064773, -0.05778040916215560624, -0.4822834645669293319 ) ) ;
#68322=CARTESIAN_POINT ( 'NONE',  ( 0.9580052493438326877, 0.05413385826771666132, 0.4176697321401328100 ) ) ;
#68323=CARTESIAN_POINT ( 'NONE',  ( 0.6364829396325465405, -0.3162353388693409650, -0.4822834645669289433 ) ) ;
#68325=CARTESIAN_POINT ( 'NONE',  ( -0.1574803149606292529, -0.1870078740157479769, 0.4822834645669291653 ) ) ;
#68326=CARTESIAN_POINT ( 'NONE',  ( 0.1181102362204730916, 0.2952755905511811885, 0.000000000000000000 ) ) ;
#68327=CARTESIAN_POINT ( 'NONE',  ( -0.4068241469816264999, -0.4281496062992124485, 0.4176697321401328655 ) ) ;
#68328=CARTESIAN_POINT ( 'NONE',  ( 0.2887139107611556010, 0.1283753931104746893, -0.1820866141732285504 ) ) ;
#68329=CARTESIAN_POINT ( 'NONE',  ( 1.686351706036745890, 0.1771653543307087630, 0.09757992244046791164 ) ) ;
#68331=CARTESIAN_POINT ( 'NONE',  ( 0.4461942257217855201, -0.6046776061558807314, 0.2411417322834647770 ) ) ;
#68332=CARTESIAN_POINT ( 'NONE',  ( 1.568241469816273437, -0.3162353388693405765, 0.4822834645669290543 ) ) ;
#68334=EDGE_LOOP ( 'NONE', ( #15071, #44159, #50148, #52015 ) ) ;
#68336=CARTESIAN_POINT ( 'NONE',  ( 0.7020997375328090762, -0.3162353388693405765, 0.4822834645669290543 ) ) ;
#68337=CARTESIAN_POINT ( 'NONE',  ( 0.2690288713910767848, -0.5511811023622048555, -0.09757992244046775898 ) ) ;
#68341=DIRECTION ( 'NONE',  ( 0.8050726085550550248, 2.493067783899190563E-16, -0.5931762764595016613 ) ) ;
#68342=CARTESIAN_POINT ( 'NONE',  ( 0.3046215029598646207, 2.057429365980579055E-15, -0.4281989832122139461 ) ) ;
#68344=CARTESIAN_POINT ( 'NONE',  ( 0.4527559055118117182, -0.5400638737290844871, 0.3530559997133364547 ) ) ;
#68345=CARTESIAN_POINT ( 'NONE',  ( -0.8661417322834640276, -0.1870078740157479769, 0.4822834645669291653 ) ) ;
#68346=CARTESIAN_POINT ( 'NONE',  ( -0.8661417322834640276, -0.1870078740157480879, -0.4822834645669291653 ) ) ;
#68347=CARTESIAN_POINT ( 'NONE',  ( 0.6102362204724416372, -0.5400638737290844871, 0.3530559997133364547 ) ) ;
#68348=CARTESIAN_POINT ( 'NONE',  ( 1.502624671916010790, -0.3162353388693409650, -0.4822834645669289433 ) ) ;
#68349=CARTESIAN_POINT ( 'NONE',  ( 1.601049868766404982, -0.5023911411419708095, -0.1820866141732282451 ) ) ;
#68351=CARTESIAN_POINT ( 'NONE',  ( 1.305774278215223960, -0.5511811023622046335, 0.09757992244046803654 ) ) ;
#68352=CARTESIAN_POINT ( 'NONE',  ( -0.8661417322834640276, -0.1870078740157479769, 0.4822834645669291653 ) ) ;
#68353=CARTESIAN_POINT ( 'NONE',  ( 1.555118110236221041, 0.1660481256975883668, -0.3530559997133364547 ) ) ;
#68354=( BOUNDED_CURVE ( )  B_SPLINE_CURVE ( 1, ( #24990, #43109 ),
 .UNSPECIFIED., .F., .F. ) 
 B_SPLINE_CURVE_WITH_KNOTS ( ( 2, 2 ),
 ( 3.469446951953614189E-18, 0.002000000000000006981 ),
 .UNSPECIFIED. ) 
 CURVE ( )  GEOMETRIC_REPRESENTATION_ITEM ( )  RATIONAL_B_SPLINE_CURVE ( ( 0.9875488213027523443, 0.9875488213027523443 ) ) 
 REPRESENTATION_ITEM ( '' )  );
#68356=CARTESIAN_POINT ( 'NONE',  ( 0.1771653543307093182, -0.5400638737290845981, -0.3530559997133363437 ) ) ;
#68357=CARTESIAN_POINT ( 'NONE',  ( 1.003937007874016407, -0.5400638737290844871, 0.3530559997133364547 ) ) ;
#68358=CARTESIAN_POINT ( 'NONE',  ( -1.614173228346457378, 1.543375672658094944, 0.1372047244094476981 ) ) ;
#68359=CARTESIAN_POINT ( 'NONE',  ( -1.371391076115484831, 0.1771653543307087075, -0.09757992244046823083 ) ) ;
#68360=CARTESIAN_POINT ( 'NONE',  ( 0.1837270341207357105, -0.6046776061558809534, -0.2411417322834644161 ) ) ;
#68361=CARTESIAN_POINT ( 'NONE',  ( 1.128608923884514947, 0.1283753931104748280, 0.1820866141732283561 ) ) ;
#68362=EDGE_CURVE ( 'NONE', #47808, #60445, #5481, .T. ) ;
#68364=CARTESIAN_POINT ( 'NONE',  ( -1.030183727034119867, -0.08942795157528024563, -0.3641732283464568787 ) ) ;
#68365=CARTESIAN_POINT ( 'NONE',  ( 1.384514435695538559, 0.2952755905511810774, -0.1292274648535930714 ) ) ;
#68367=CARTESIAN_POINT ( 'NONE',  ( -0.2624671916010490880, 0.1283753931104746893, -0.1820866141732285504 ) ) ;
#68368=CARTESIAN_POINT ( 'NONE',  ( -0.2034120734908131112, -0.6692913385826773087, -0.1292274648535924053 ) ) ;
#68369=CARTESIAN_POINT ( 'NONE',  ( -1.148293963254592542, 0.1771653543307087630, 0.09757992244046791164 ) ) ;
#68370=CARTESIAN_POINT ( 'NONE',  ( -0.6430446194225716283, -0.4281496062992124485, 0.4176697321401328655 ) ) ;
#68371=CARTESIAN_POINT ( 'NONE',  ( 1.430446194225722500, -0.4281496062992127816, -0.4176697321401328100 ) ) ;
#68374=CARTESIAN_POINT ( 'NONE',  ( 1.305774278215223960, 0.2952755905511810774, -0.1292274648535930714 ) ) ;
#68376=CARTESIAN_POINT ( 'NONE',  ( -1.010498687664041384, -0.4281496062992127816, -0.4176697321401328100 ) ) ;
#68377=CARTESIAN_POINT ( 'NONE',  ( -1.128608923884513837, 0.1283753931104746893, -0.1820866141732285504 ) ) ;
#68378=CARTESIAN_POINT ( 'NONE',  ( -0.5052493438320203589, -0.5511811023622046335, 0.09757992244046803654 ) ) ;
#68379=CARTESIAN_POINT ( 'NONE',  ( -0.5387615594602663815, -2.294479370626195693E-15, 0.3464511005275217603 ) ) ;
#68380=CARTESIAN_POINT ( 'NONE',  ( 0.01312335958005323398, -0.4281496062992127816, -0.4176697321401328100 ) ) ;
#68381=CARTESIAN_POINT ( 'NONE',  ( -0.1443569553805765515, -0.3690944881889765550, -0.3153832671262227771 ) ) ;
#68382=CARTESIAN_POINT ( 'NONE',  ( -1.122047244094487306, -0.4536011799217367080, 0.2665933059059888421 ) ) ;
#68383=CARTESIAN_POINT ( 'NONE',  ( -1.686351706036744558, 0.2952755905511810774, -0.1292274648535930714 ) ) ;
#68384=CARTESIAN_POINT ( 'NONE',  ( 1.496062992125984703, -0.1870078740157480601, -0.3641732283464567677 ) ) ;
#68385=CARTESIAN_POINT ( 'NONE',  ( 0.8923884514435703741, 0.2306618581243848609, 0.2411417322834645549 ) ) ;
#68387=CARTESIAN_POINT ( 'NONE',  ( 0.3083989501312343062, -0.08942795157528024563, -0.3641732283464568787 ) ) ;
#68388=CARTESIAN_POINT ( 'NONE',  ( 0.9973753280839902091, -0.6046776061558807314, 0.2411417322834647770 ) ) ;
#68389=CARTESIAN_POINT ( 'NONE',  ( 1.049868766404200127, -0.5023911411419708095, -0.1820866141732282451 ) ) ;
#68391=CARTESIAN_POINT ( 'NONE',  ( -1.391076115485563314, -0.6046776061558809534, -0.2411417322834644161 ) ) ;
#68392=CARTESIAN_POINT ( 'NONE',  ( -1.062992125984250968, -0.6692913385826771977, 8.415575281601705876E-17 ) ) ;
#68393=CARTESIAN_POINT ( 'NONE',  ( -0.006561679790025524116, -0.3162353388693405765, 0.4822834645669290543 ) ) ;
#68396=CARTESIAN_POINT ( 'NONE',  ( 0.7283464566929140904, -0.5400638737290845981, -0.3530559997133363437 ) ) ;
#68397=CARTESIAN_POINT ( 'NONE',  ( 1.568241469816273437, -0.2845877964562159024, 0.3641732283464567677 ) ) ;
#68398=CARTESIAN_POINT ( 'NONE',  ( 0.09186351706036827158, 0.05413385826771666132, 0.4176697321401328100 ) ) ;
#68399=CARTESIAN_POINT ( 'NONE',  ( 0.9186351706036751663, -0.6046776061558807314, 0.2411417322834647770 ) ) ;
#68404=CARTESIAN_POINT ( 'NONE',  ( -0.4133858267716528645, 0.07958543189024071263, -0.2665933059059888421 ) ) ;
#68405=CARTESIAN_POINT ( 'NONE',  ( -0.8333333333333323711, -0.6692913385826773087, -0.1292274648535924053 ) ) ;
#68406=CARTESIAN_POINT ( 'NONE',  ( 0.3871391076115492380, -0.05778040916215560624, -0.4822834645669293319 ) ) ;
#68408=CARTESIAN_POINT ( 'NONE',  ( -1.653543307086613234, -0.1870078740157479769, 0.4822834645669291653 ) ) ;
#68409=CARTESIAN_POINT ( 'NONE',  ( 1.292650918635171564, 0.2952755905511811885, 0.1292274648535926551 ) ) ;
#68413=CARTESIAN_POINT ( 'NONE',  ( 1.082677165354331228, -0.5400638737290844871, 0.3530559997133364547 ) ) ;
#68414=CARTESIAN_POINT ( 'NONE',  ( 1.318897637795276356, 0.07958543189024071263, -0.2665933059059888421 ) ) ;
#68415=CARTESIAN_POINT ( 'NONE',  ( 1.522309711286089939, 0.2306618581243848609, 0.2411417322834645549 ) ) ;
#68416=CARTESIAN_POINT ( 'NONE',  ( -1.423884514435694859, -0.05778040916215560624, -0.4822834645669293319 ) ) ;
#68419=CARTESIAN_POINT ( 'NONE',  ( 0.8070866141732289112, -0.5400638737290845981, -0.3530559997133363437 ) ) ;
#68420=CARTESIAN_POINT ( 'NONE',  ( 1.404199475065617708, -0.004921259842519870586, -0.3153832671262229437 ) ) ;
#68421=CARTESIAN_POINT ( 'NONE',  ( -0.6889763779527552368, -0.5400638737290845981, -0.3530559997133363437 ) ) ;
#68422=CARTESIAN_POINT ( 'NONE',  ( -0.5380577427821514602, -0.4281496062992127816, -0.4176697321401328100 ) ) ;
#68423=CARTESIAN_POINT ( 'NONE',  ( -1.653543307086613234, -0.1870078740157479769, 0.4822834645669291653 ) ) ;
#68425=CARTESIAN_POINT ( 'NONE',  ( 0.2362204724409456558, -0.1870078740157480879, -0.4822834645669291653 ) ) ;
#68427=CARTESIAN_POINT ( 'NONE',  ( -1.496062992125983815, -0.1870078740157479769, 0.3641732283464567677 ) ) ;
#68432=CARTESIAN_POINT ( 'NONE',  ( -1.430446194225721390, -0.4281496062992124485, 0.4176697321401328655 ) ) ;
#68434=CARTESIAN_POINT ( 'NONE',  ( 1.574803149606299746, -0.1870078740157480601, -0.3641732283464567677 ) ) ;
#68435=CARTESIAN_POINT ( 'NONE',  ( -0.09842519685039295696, 0.1012011053420775880, -0.2882089793578257453 ) ) ;
#68436=LINE ( 'NONE', #18731, #54422 ) ;
#68439=CARTESIAN_POINT ( 'NONE',  ( -0.1181102362204717315, -0.5511811023622047445, 6.969142054262312111E-17 ) ) ;
#68440=CARTESIAN_POINT ( 'NONE',  ( -1.364829396325458521, 0.1283753931104746893, -0.1820866141732285504 ) ) ;
#68441=CARTESIAN_POINT ( 'NONE',  ( -1.482939632545930975, 0.05413385826771666132, 0.4176697321401328100 ) ) ;
#68442=CARTESIAN_POINT ( 'NONE',  ( 0.5971128608923890191, -0.6692913385826771977, 0.1292274648535927661 ) ) ;
#68443=CARTESIAN_POINT ( 'NONE',  ( -1.345144356955379816, -0.3162353388693405765, 0.4822834645669290543 ) ) ;
#68445=ORIENTED_EDGE ( 'NONE', *, *, #39193, .T. ) ;
#68446=CARTESIAN_POINT ( 'NONE',  ( -1.607611548556429737, 0.2952755905511810774, -0.1292274648535930714 ) ) ;
#68447=CARTESIAN_POINT ( 'NONE',  ( 1.614173228346456712, 0.4405861044731111953, 0.1372047244094478646 ) ) ;
#68452=CARTESIAN_POINT ( 'NONE',  ( -0.7545931758530176614, -0.6692913385826773087, -0.1292274648535924053 ) ) ;
#68453=CARTESIAN_POINT ( 'NONE',  ( 1.496062992125985147, -0.1870078740157479769, 0.4822834645669291653 ) ) ;
#68455=CARTESIAN_POINT ( 'NONE',  ( 1.614173228346457378, 0.9921945702958886448, -0.1372047244094476148 ) ) ;
#68457=CARTESIAN_POINT ( 'NONE',  ( -1.699475065616797398, 0.2952755905511811885, 0.1292274648535926551 ) ) ;
#68458=CARTESIAN_POINT ( 'NONE',  ( -0.7217847769028863381, 0.05413385826771626580, -0.4176697321401330321 ) ) ;
#68460=CARTESIAN_POINT ( 'NONE',  ( -0.07874015748031421014, -0.1870078740157480601, -0.3641732283464567677 ) ) ;
#68462=CARTESIAN_POINT ( 'NONE',  ( -0.1706036745406816491, -0.004921259842519870586, -0.3153832671262229437 ) ) ;
#68463=CARTESIAN_POINT ( 'NONE',  ( 0.5839895013123367340, -0.5511811023622048555, -0.09757992244046775898 ) ) ;
#68464=CARTESIAN_POINT ( 'NONE',  ( 0.4002624671916016896, -0.3162353388693409650, -0.4822834645669289433 ) ) ;
#68465=CARTESIAN_POINT ( 'NONE',  ( -0.8595800524934373854, -0.08942795157527998196, 0.3641732283464567121 ) ) ;
#68467=CARTESIAN_POINT ( 'NONE',  ( -1.640419947506561060, 0.05413385826771666132, 0.4176697321401328100 ) ) ;
#68468=CARTESIAN_POINT ( 'NONE',  ( -1.148293963254592542, 0.2952755905511811885, 0.1292274648535926551 ) ) ;
#68470=CARTESIAN_POINT ( 'NONE',  ( -0.03280839895013062252, -0.6692913385826771977, 0.1292274648535927661 ) ) ;
#68471=CARTESIAN_POINT ( 'NONE',  ( -0.6627296587926501115, 0.2952755905511810774, -0.1292274648535930714 ) ) ;
#68472=CARTESIAN_POINT ( 'NONE',  ( 1.358267716535433323, 0.07958543189024085140, 0.2665933059059887866 ) ) ;
#68473=CARTESIAN_POINT ( 'NONE',  ( 0.1246719160104994284, -0.5511811023622046335, 0.09757992244046803654 ) ) ;
#68474=CARTESIAN_POINT ( 'NONE',  ( -0.4265091863517051496, 0.2952755905511810774, -0.1292274648535930714 ) ) ;
#68475=CARTESIAN_POINT ( 'NONE',  ( -0.8267716535433065062, 0.2952755905511811885, 0.000000000000000000 ) ) ;
#68478=CARTESIAN_POINT ( 'NONE',  ( 0.3083989501312343062, -0.05778040916215560624, -0.4822834645669293319 ) ) ;
#68479=ORIENTED_EDGE ( 'NONE', *, *, #80156, .F. ) ;
#68481=CARTESIAN_POINT ( 'NONE',  ( 1.062992125984252745, -0.6692913385826771977, 8.415575281601705876E-17 ) ) ;
#68482=CARTESIAN_POINT ( 'NONE',  ( -0.6036745406824141069, 0.1283753931104748280, 0.1820866141732283561 ) ) ;
#68483=CARTESIAN_POINT ( 'NONE',  ( -0.7611548556430438595, 0.2306618581243848609, 0.2411417322834645549 ) ) ;
#68484=CARTESIAN_POINT ( 'NONE',  ( 1.167979002624672580, -0.4281496062992124485, 0.4176697321401328655 ) ) ;
#68485=CARTESIAN_POINT ( 'NONE',  ( 0.8333333333333340365, -0.6692913385826771977, 0.1292274648535927661 ) ) ;
#68486=CARTESIAN_POINT ( 'NONE',  ( -1.535433070866141225, -0.6692913385826771977, 8.415575281601705876E-17 ) ) ;
#68487=CARTESIAN_POINT ( 'NONE',  ( -1.082677165354329896, 0.07958543189024085140, 0.2665933059059887866 ) ) ;
#68491=CARTESIAN_POINT ( 'NONE',  ( 1.489501312335958172, -0.2845877964562159024, 0.3641732283464567677 ) ) ;
#68492=CARTESIAN_POINT ( 'NONE',  ( 1.003937007874016185, 0.07958543189024071263, -0.2665933059059888421 ) ) ;
#68493=CARTESIAN_POINT ( 'NONE',  ( 0.6889763779527563470, 0.1660481256975883668, -0.3530559997133364547 ) ) ;
#68494=CARTESIAN_POINT ( 'NONE',  ( 0.4600214019799526155, 2.784432375088962958E-17, -0.3464511005275205946 ) ) ;
#68496=CARTESIAN_POINT ( 'NONE',  ( 0.6430446194225729606, -0.3690944881889765550, -0.3153832671262227771 ) ) ;
#68497=CARTESIAN_POINT ( 'NONE',  ( -0.2362204724409440182, -0.1870078740157479769, 0.4822834645669291653 ) ) ;
#68498=CARTESIAN_POINT ( 'NONE',  ( -0.7742782152230962556, -0.4281496062992127816, -0.4176697321401328100 ) ) ;
#68499=CARTESIAN_POINT ( 'NONE',  ( 1.377952755905512472, 0.2952755905511811885, 0.000000000000000000 ) ) ;
#68502=CARTESIAN_POINT ( 'NONE',  ( 0.09842519685039434474, -0.4536011799217368745, -0.2665933059059886201 ) ) ;
#68506=CARTESIAN_POINT ( 'NONE',  ( -1.023622047244094002, -0.1870078740157480879, -0.4822834645669291653 ) ) ;
#68507=CARTESIAN_POINT ( 'NONE',  ( 8.195543980992789655E-16, -0.1870078740157480879, -0.4822834645669291653 ) ) ;
#68508=CARTESIAN_POINT ( 'NONE',  ( -0.2099737532808391705, 0.2306618581243848609, 0.2411417322834645549 ) ) ;
#68509=CARTESIAN_POINT ( 'NONE',  ( 0.7020997375328090762, -0.3162353388693405765, 0.4822834645669290543 ) ) ;
#68510=CARTESIAN_POINT ( 'NONE',  ( -0.2690288713910754526, -0.6692913385826771977, 0.1292274648535927661 ) ) ;
#68511=CARTESIAN_POINT ( 'NONE',  ( -1.384514435695537005, -0.6692913385826773087, -0.1292274648535924053 ) ) ;
#68512=CARTESIAN_POINT ( 'NONE',  ( -0.5708661417322828946, 0.1660481256975883668, -0.3530559997133364547 ) ) ;
#68513=CARTESIAN_POINT ( 'NONE',  ( 0.8333333333333340365, 0.2952755905511810774, -0.1292274648535930714 ) ) ;
#68514=CARTESIAN_POINT ( 'NONE',  ( 0.6692913385826777528, 0.2952755905511811885, 0.000000000000000000 ) ) ;
#68516=CARTESIAN_POINT ( 'NONE',  ( -0.4133858267716528645, -0.4536011799217367080, 0.2665933059059888421 ) ) ;
#68517=VERTEX_POINT ( 'NONE', #41776 ) ;
#68519=ORIENTED_EDGE ( 'NONE', *, *, #4442, .T. ) ;
#68520=CARTESIAN_POINT ( 'NONE',  ( -1.076115485564303809, 0.1283753931104748280, 0.1820866141732283561 ) ) ;
#68521=CARTESIAN_POINT ( 'NONE',  ( -0.5905511811023613777, -0.6692913385826771977, 8.415575281601705876E-17 ) ) ;
#68523=CARTESIAN_POINT ( 'NONE',  ( -0.5314960629921254842, -0.5400638737290845981, -0.3530559997133363437 ) ) ;
#68524=CARTESIAN_POINT ( 'NONE',  ( -0.7152230971128602510, -0.05778040916215560624, -0.4822834645669293319 ) ) ;
#68525=CARTESIAN_POINT ( 'NONE',  ( -1.463254593175852492, 0.2952755905511811885, 0.1292274648535926551 ) ) ;
#68526=CARTESIAN_POINT ( 'NONE',  ( -1.706036745406823485, 0.2306618581243848609, 0.2411417322834645549 ) ) ;
#68527=CARTESIAN_POINT ( 'NONE',  ( 0.8792650918635177559, -0.004921259842519576551, 0.3153832671262227771 ) ) ;
#68530=CARTESIAN_POINT ( 'NONE',  ( 0.1706036745406830368, -0.004921259842519576551, 0.3153832671262227771 ) ) ;
#68531=CARTESIAN_POINT ( 'NONE',  ( -0.4330708661417315697, -0.6692913385826771977, 8.415575281601705876E-17 ) ) ;
#68532=PLANE ( 'NONE',  #49623 ) ;
#68533=CARTESIAN_POINT ( 'NONE',  ( -0.2427821522309703550, -0.3162353388693405765, 0.4822834645669290543 ) ) ;
#68540=CARTESIAN_POINT ( 'NONE',  ( -0.7414698162729651543, 0.1771653543307087075, -0.09757992244046823083 ) ) ;
#68541=CARTESIAN_POINT ( 'NONE',  ( -0.7939632545931754048, -0.3162353388693405765, 0.4822834645669290543 ) ) ;
#68545=CARTESIAN_POINT ( 'NONE',  ( 1.194225721784777594, 0.05413385826771666132, 0.4176697321401328100 ) ) ;
#68546=CARTESIAN_POINT ( 'NONE',  ( 0.3083989501312343062, -0.3162353388693405765, 0.4822834645669290543 ) ) ;
#68547=CARTESIAN_POINT ( 'NONE',  ( 0.6036745406824154392, 0.2306618581243847221, -0.2411417322834647770 ) ) ;
#68548=CARTESIAN_POINT ( 'NONE',  ( -0.5446194225721777693, -0.08942795157527998196, 0.3641732283464567121 ) ) ;
#68549=CARTESIAN_POINT ( 'NONE',  ( -0.1902887139107604098, -0.6692913385826771977, 0.1292274648535927661 ) ) ;
#68551=CARTESIAN_POINT ( 'NONE',  ( -0.7086614173228339419, -0.1870078740157480879, -0.4822834645669291653 ) ) ;
#68553=CARTESIAN_POINT ( 'NONE',  ( 1.358267716535433323, -0.4536011799217368745, -0.2665933059059886201 ) ) ;
#68554=CARTESIAN_POINT ( 'NONE',  ( -0.3740157480314953431, -0.4536011799217368745, -0.2665933059059886201 ) ) ;
#68555=CARTESIAN_POINT ( 'NONE',  ( 1.154855643044620184, -0.5023911411419708095, 0.1820866141732285504 ) ) ;
#68556=CARTESIAN_POINT ( 'NONE',  ( -1.712598425196849572, 0.1660481256975885056, 0.3530559997133364547 ) ) ;
#68557=CARTESIAN_POINT ( 'NONE',  ( -1.154855643044618851, 0.1283753931104748280, 0.1820866141732283561 ) ) ;
#68559=CARTESIAN_POINT ( 'NONE',  ( -1.318897637795274802, -0.5400638737290845981, -0.3530559997133363437 ) ) ;
#68560=CARTESIAN_POINT ( 'NONE',  ( -0.3412073490813641308, 0.2306618581243847221, -0.2411417322834647770 ) ) ;
#68563=CARTESIAN_POINT ( 'NONE',  ( -0.09842519685039295696, -0.4536011799217367080, 0.2665933059059888421 ) ) ;
#68564=CARTESIAN_POINT ( 'NONE',  ( -1.620734908136482577, -0.5511811023622048555, -0.09757992244046775898 ) ) ;
#68565=CARTESIAN_POINT ( 'NONE',  ( 0.5577427821522316087, -0.05778040916215522460, 0.4822834645669289988 ) ) ;
#68566=CARTESIAN_POINT ( 'NONE',  ( -1.535433070866141225, 0.1771653543307087630, 0.000000000000000000 ) ) ;
#68567=CARTESIAN_POINT ( 'NONE',  ( 1.397637795275591177, -0.4536011799217367080, 0.2665933059059888421 ) ) ;
#68568=CARTESIAN_POINT ( 'NONE',  ( -0.7349081364829390672, 0.2306618581243847221, -0.2411417322834647770 ) ) ;
#68569=CARTESIAN_POINT ( 'NONE',  ( -0.2427821522309703550, -0.2845877964562159024, 0.3641732283464567677 ) ) ;
#68570=CARTESIAN_POINT ( 'NONE',  ( -0.8785612751854012803, -2.613618158232546091E-15, -0.3464511005275220379 ) ) ;
#68571=CARTESIAN_POINT ( 'NONE',  ( 0.1312335958005255154, -0.5023911411419708095, 0.1820866141732285504 ) ) ;
#68572=EDGE_CURVE ( 'NONE', #28439, #79831, #42610, .T. ) ;
#68573=CARTESIAN_POINT ( 'NONE',  ( -0.2887139107611542133, -0.6046776061558809534, -0.2411417322834644161 ) ) ;
#68575=EDGE_CURVE ( 'NONE', #50999, #18885, #42871, .T. ) ;
#68577=CARTESIAN_POINT ( 'NONE',  ( 0.6036745406824153282, -0.5023911411419708095, 0.1820866141732285504 ) ) ;
#68578=CARTESIAN_POINT ( 'NONE',  ( -0.5118110236220466680, 0.2952755905511811885, 0.000000000000000000 ) ) ;
#68579=CARTESIAN_POINT ( 'NONE',  ( -0.6036745406824141069, -0.6046776061558809534, -0.2411417322834644161 ) ) ;
#68580=CARTESIAN_POINT ( 'NONE',  ( -0.8398950131233585692, 0.1283753931104748280, 0.1820866141732283561 ) ) ;
#68581=CARTESIAN_POINT ( 'NONE',  ( 2.787279214012418738, 1.535433070866142113, 0.000000000000000000 ) ) ;
#68582=CARTESIAN_POINT ( 'NONE',  ( -0.5380577427821514602, -0.004921259842519576551, 0.3153832671262227771 ) ) ;
#68583=CARTESIAN_POINT ( 'NONE',  ( -0.08530183727034056085, -0.3162353388693405765, 0.4822834645669290543 ) ) ;
#68584=CARTESIAN_POINT ( 'NONE',  ( -0.9711286089238838626, -0.5023911411419708095, 0.1820866141732285504 ) ) ;
#68586=CARTESIAN_POINT ( 'NONE',  ( -1.541994750656167090, -0.6692913385826773087, -0.1292274648535924053 ) ) ;
#68589=CARTESIAN_POINT ( 'NONE',  ( -1.633858267716534529, -0.4536011799217368745, -0.2665933059059886201 ) ) ;
#68590=CARTESIAN_POINT ( 'NONE',  ( -0.4658792650918627265, -0.05778040916215522460, 0.4822834645669289988 ) ) ;
#68591=CARTESIAN_POINT ( 'NONE',  ( -1.154855643044618851, 0.2306618581243848609, 0.2411417322834645549 ) ) ;
#68595=CARTESIAN_POINT ( 'NONE',  ( 0.8792650918635177559, 0.05413385826771666132, 0.4176697321401328100 ) ) ;
#68596=CARTESIAN_POINT ( 'NONE',  ( 0.4921259842519691285, -0.5400638737290845981, -0.3530559997133363437 ) ) ;
#68599=CARTESIAN_POINT ( 'NONE',  ( 0.9973753280839902091, 0.1283753931104746893, -0.1820866141732285504 ) ) ;
#68602=CARTESIAN_POINT ( 'NONE',  ( -0.8858267716535425107, -0.4536011799217367080, 0.2665933059059888421 ) ) ;
#68605=CARTESIAN_POINT ( 'NONE',  ( 0.5577427821522314977, -0.3162353388693409650, -0.4822834645669289433 ) ) ;
#68606=CARTESIAN_POINT ( 'NONE',  ( -0.5905511811023615998, 0.2952755905511811885, 0.000000000000000000 ) ) ;
#68607=CARTESIAN_POINT ( 'NONE',  ( -0.9842519685039360366, 0.2952755905511811885, 0.000000000000000000 ) ) ;
#68608=CARTESIAN_POINT ( 'NONE',  ( 0.9711286089238851948, -0.6046776061558809534, -0.2411417322834644161 ) ) ;
#68609=CARTESIAN_POINT ( 'NONE',  ( -1.437007874015747477, 0.07958543189024071263, -0.2665933059059888421 ) ) ;
#68610=CARTESIAN_POINT ( 'NONE',  ( -1.614173228346457378, 0.9921945702958913094, 0.1372047244094476981 ) ) ;
#68611=CARTESIAN_POINT ( 'NONE',  ( 0.05905511811023709395, -0.5400638737290844871, 0.3530559997133364547 ) ) ;
#68612=CARTESIAN_POINT ( 'NONE',  ( -1.049868766404198794, -0.6046776061558807314, 0.2411417322834647770 ) ) ;
#68614=CARTESIAN_POINT ( 'NONE',  ( -1.594488188976377119, 0.1660481256975883668, -0.3530559997133364547 ) ) ;
#68617=CARTESIAN_POINT ( 'NONE',  ( 0.8005249343832028242, -0.3690944881889765550, -0.3153832671262227771 ) ) ;
#68618=ORIENTED_EDGE ( 'NONE', *, *, #80156, .T. ) ;
#68620=CARTESIAN_POINT ( 'NONE',  ( -1.030183727034119867, -0.3162353388693405765, 0.4822834645669290543 ) ) ;
#68621=ORIENTED_EDGE ( 'NONE', *, *, #81623, .F. ) ;
#68622=CARTESIAN_POINT ( 'NONE',  ( 5.463695987328526437E-16, -0.1870078740157479769, 0.3641732283464567677 ) ) ;
#68623=CARTESIAN_POINT ( 'NONE',  ( -1.515748031496062076, 0.1660481256975883668, -0.3530559997133364547 ) ) ;
#68624=CARTESIAN_POINT ( 'NONE',  ( 0.5643044619422579178, -0.4281496062992127816, -0.4176697321401328100 ) ) ;
#68625=CARTESIAN_POINT ( 'NONE',  ( 0.5577427821522314977, -0.3162353388693409650, -0.4822834645669289433 ) ) ;
#68626=CARTESIAN_POINT ( 'NONE',  ( -0.7874015748031489847, -0.1870078740157479769, 0.4822834645669291653 ) ) ;
#68628=CARTESIAN_POINT ( 'NONE',  ( -0.8005249343832011588, 0.05413385826771626580, -0.4176697321401330321 ) ) ;
#68630=CARTESIAN_POINT ( 'NONE',  ( 1.325459317585302665, -0.004921259842519870586, -0.3153832671262229437 ) ) ;
#68631=CARTESIAN_POINT ( 'NONE',  ( -0.9776902887139098386, 0.2952755905511810774, -0.1292274648535930714 ) ) ;
#68632=CARTESIAN_POINT ( 'NONE',  ( 1.049868766404200349, 0.2306618581243848609, 0.2411417322834645549 ) ) ;
#68633=CARTESIAN_POINT ( 'NONE',  ( 1.391076115485564868, 0.2306618581243847221, -0.2411417322834647770 ) ) ;
#68636=CARTESIAN_POINT ( 'NONE',  ( -1.469816272965878357, -0.6046776061558809534, -0.2411417322834644161 ) ) ;
#68638=CARTESIAN_POINT ( 'NONE',  ( 0.3346456692913390985, 0.1660481256975885056, 0.3530559997133364547 ) ) ;
#68640=CARTESIAN_POINT ( 'NONE',  ( -1.417322834645668772, -0.1870078740157480601, -0.3641732283464567677 ) ) ;
#68641=CARTESIAN_POINT ( 'NONE',  ( 0.5118110236220480003, -0.5511811023622047445, 6.969142054262312111E-17 ) ) ;
#68642=CARTESIAN_POINT ( 'NONE',  ( 1.095800524934383846, -0.3162353388693405765, 0.4822834645669290543 ) ) ;
#68644=CARTESIAN_POINT ( 'NONE',  ( 0.6299212598425204535, -0.1870078740157480601, -0.3641732283464567677 ) ) ;
#68645=EDGE_CURVE ( 'NONE', #19973, #19878, #39623, .T. ) ;
#68646=CARTESIAN_POINT ( 'NONE',  ( 0.7086614173228352742, -0.1870078740157480879, -0.4822834645669291653 ) ) ;
#68648=CARTESIAN_POINT ( 'NONE',  ( -0.8398950131233589023, -0.6046776061558809534, -0.2411417322834644161 ) ) ;
#68649=CARTESIAN_POINT ( 'NONE',  ( -1.646051170424378096, 0.000000000000000000, -0.3464511005275205946 ) ) ;
#68650=CARTESIAN_POINT ( 'NONE',  ( 1.089238845144357537, -0.3690944881889763329, 0.3153832671262228327 ) ) ;
#68651=CARTESIAN_POINT ( 'NONE',  ( -0.6036745406824141069, 0.2306618581243848609, 0.2411417322834645549 ) ) ;
#68652=CARTESIAN_POINT ( 'NONE',  ( 0.1902887139107617975, 0.2952755905511811885, 0.1292274648535926551 ) ) ;
#68655=CARTESIAN_POINT ( 'NONE',  ( 0.1640419947506569498, -0.05778040916215522460, 0.4822834645669289988 ) ) ;
#68656=CARTESIAN_POINT ( 'NONE',  ( 0.006561679790026889343, -0.2845877964562161244, -0.3641732283464567121 ) ) ;
#68658=CARTESIAN_POINT ( 'NONE',  ( 0.1115485564304470323, 0.1771653543307087630, 0.09757992244046791164 ) ) ;
#68659=CARTESIAN_POINT ( 'NONE',  ( 0.8727034120734912248, -0.2845877964562161244, -0.3641732283464567121 ) ) ;
#68663=CARTESIAN_POINT ( 'NONE',  ( 0.1837270341207357105, -0.6046776061558809534, -0.2411417322834644161 ) ) ;
#68665=CARTESIAN_POINT ( 'NONE',  ( 1.607611548556431069, -0.5511811023622048555, -0.09757992244046775898 ) ) ;
#68667=CARTESIAN_POINT ( 'NONE',  ( -0.3215223097112853146, -0.2845877964562159024, 0.3641732283464567677 ) ) ;
#68668=CARTESIAN_POINT ( 'NONE',  ( -0.4921259842519677963, 0.1660481256975883668, -0.3530559997133364547 ) ) ;
#68669=CARTESIAN_POINT ( 'NONE',  ( 0.8267716535433078384, -0.5511811023622047445, 6.969142054262312111E-17 ) ) ;
#68671=CARTESIAN_POINT ( 'NONE',  ( 1.318897637795276356, 0.07958543189024071263, -0.2665933059059888421 ) ) ;
#68672=CARTESIAN_POINT ( 'NONE',  ( 0.01312335958005323398, -0.4281496062992127816, -0.4176697321401328100 ) ) ;
#68673=CARTESIAN_POINT ( 'NONE',  ( 0.9908136482939640111, -0.6692913385826771977, 0.1292274648535927661 ) ) ;
#68675=CARTESIAN_POINT ( 'NONE',  ( 0.2821522309711292364, -0.6692913385826771977, 0.1292274648535927661 ) ) ;
#68676=CARTESIAN_POINT ( 'NONE',  ( 1.161417322834646493, -0.5400638737290844871, 0.3530559997133364547 ) ) ;
#68677=CARTESIAN_POINT ( 'NONE',  ( 0.5052493438320218022, -0.6692913385826773087, -0.1292274648535924053 ) ) ;
#68679=CARTESIAN_POINT ( 'NONE',  ( 0.8398950131233602345, -0.5023911411419708095, 0.1820866141732285504 ) ) ;
#68680=CARTESIAN_POINT ( 'NONE',  ( 1.279527559055118724, -0.5400638737290845981, -0.3530559997133363437 ) ) ;
#68681=CARTESIAN_POINT ( 'NONE',  ( 0.05249343832021075018, 0.1283753931104746893, -0.1820866141732285504 ) ) ;
#68682=CARTESIAN_POINT ( 'NONE',  ( -0.2296587926509179312, -0.05778040916215522460, 0.4822834645669289988 ) ) ;
#68683=CARTESIAN_POINT ( 'NONE',  ( 0.4790026246719167324, -0.05778040916215522460, 0.4822834645669289988 ) ) ;
#68684=CARTESIAN_POINT ( 'NONE',  ( -0.6496062992125976043, 0.1660481256975883668, -0.3530559997133364547 ) ) ;
#68685=CARTESIAN_POINT ( 'NONE',  ( -0.3215223097112853146, -0.2845877964562159024, 0.3641732283464567677 ) ) ;
#68686=VECTOR ( 'NONE', #80258, 39.37007874015748143 ) ;
#68687=CARTESIAN_POINT ( 'NONE',  ( 0.6299212598425204535, -0.1870078740157479769, 0.4822834645669291653 ) ) ;
#68688=CARTESIAN_POINT ( 'NONE',  ( 1.122047244094488860, -0.4536011799217368745, -0.2665933059059886201 ) ) ;
#68689=CARTESIAN_POINT ( 'NONE',  ( -0.04593175853018302557, 0.2952755905511811885, 0.1292274648535926551 ) ) ;
#68691=CARTESIAN_POINT ( 'NONE',  ( -1.043307086614172929, 0.1660481256975883391, -0.3530559997133364547 ) ) ;
#68692=CARTESIAN_POINT ( 'NONE',  ( 1.568241469816273437, -0.3162353388693405765, 0.4822834645669290543 ) ) ;
#68694=CARTESIAN_POINT ( 'NONE',  ( -1.443569553805773564, 0.2306618581243847221, -0.2411417322834647770 ) ) ;
#68695=CARTESIAN_POINT ( 'NONE',  ( -0.3608923884514428360, -0.6692913385826773087, -0.1292274648535924053 ) ) ;
#68696=( BOUNDED_SURFACE ( )  B_SPLINE_SURFACE ( 1, 2, ( 
 ( #39790, #65485, #65052, #58728, #1091, #27155, #7817, #52819, #78530, #20854, #72206, #14559, #27577, #53234, #66304, #57879, #2335, #54486, #74284, #80197, #54904, #35555, #60395, #67551, #80610, #42270, #47756, #15804, #10310, #73454, #41455, #60804, #9468, #61219, #67139, #3573, #47339, #34735, #74702, #34315, #16628, #28822, #35142, #3158, #35975, #29650, #41041, #9063, #67967, #22515, #73872, #29240, #61645, #55312, #48176, #17047, #16212, #41859, #9886, #42688, #22921, #48587, #3986, #81021, #73029, #23333, #49003, #27991, #53651, #79359, #8643, #59976, #21678, #15379, #66726, #2746, #28406, #54064, #79780, #22095, #30061, #4393, #81432, #4800, #11132, #12366, #50642, #69198, #51050, #68787, #56141, #62884, #30477, #5219, #70011, #31711, #75115, #43914, #17460, #69611, #36789, #24970, #62465, #43090, #37612, #19081, #81846, #24158, #49826, #38025, #57371, #63287, #18273, #83066, #11957, #25387, #76751, #75526, #43500, #30883, #82251, #5627, #68385, #76346, #63700, #24570, #36381, #50236, #17866, #31294, #11547, #37203, #10724, #49420, #56550, #75932, #56958, #82655, #18676, #44321, #6039, #62055, #55722, #23747, #27064, #7293, #7723, #71689, #13207, #20340, #33392, #78435, #572, #51889, #46412, #26225, #77593, #13617, #45577, #14040, #19927, #39697, #149, #70856, #27480, #70426, #52723, #64955, #71270, #39271, #72106, #65804, #77167, #45153, #20762, #32963, #26652, #65388, #14464, #8137, #998, #53138, #58630, #52306, #78012, #78849, #45992, #59054, #40116, #33802, #25804, #1408, #59467, #64122, #6457, #32127, #1819, #44730, #12782, #38439, #57785, #51465, #19499, #38854, #64534, #6871, #32540, #58205, #34217, #40946, #47245, #48482, #3472, #22000, #3886, #21582, #8963, #15703, #66625, #41360, #22824, #67869, #27898, #80098, #53559, #22417, #72934, #61121, #15286, #79267, #73776, #55208, #34637, #60301, #2651, #74183, #10207, #16112, #54387, #35875, #48074, #61542, #29546, #28308, #79683, #67041, #35044, #41756, #21176, #29139, #16530, #60709, #72523, #3058, #53970, #67451, #47660, #73355, #46831, #2234, #9373, #28726, #9785, #54805, #35456, #14872, #80509, #42175, #40533, #66212, #8551, #59880, #16944, #48900, #82148, #24053, #11024, #12262, #74601, #42586, #68286, #69094, #49311, #5523, #11442, #43394, #62357, #36278, #56035, #24464, #69908, #44218, #37920, #68682, #63596, #61950, #37098, #42988, #23641, #81327, #36681, #10622, #4290, #29952, #31188, #56853, #82551, #5933, #11856, #17359, #4694, #30368, #81743, #50537, #24869, #50129, #17763, #80916, #75829, #62783, #55617, #75013, #49723, #31603, #56446, #23229, #75420, #5117, #30784, #18170, #43803, #69507, #37509, #63184, #76241, #18575, #6763, #32858, #77485, #57263, #32022, #12676, #76645, #8036, #32435, #82962, #58952, #38335, #39592, #77061, #64010, #52202, #14362, #25280, #52623, #64848, #26959, #18976, #58526, #58098, #1310, #65280, #57682, #7619, #892, #13507, #39163, #44, #463, #19820, #50948, #70747, #44625, #33292, #71167, #64429, #19395, #78328, #26549, #26120, #51781, #7186, #45469, #46313, #70321, #77906, #20237, #45885, #71583, #13934, #38752, #6351, #20659, #72006, #40019, #65707, #25697, #45046, #51358, #13099, #79582, #79168, #59778, #34116, #72834, #53037, #72424, #27375, #41666, #9690, #67357, #22727, #47979, #53460, #47144, #21485, #34536, #3375, #61024, #34951, #53869, #33700, #60614, #73254, #78749, #1719, #40429, #48386, #9280, #16431, #21074, #46732, #8446, #14774, #66110, #2132, #66948, #54286, #35361, #27800, #66527, #2963, #21897, #59360, #15184, #40841, #8858, #67772, #60201, #2552, #29038, #28210, #16020, #47560, #15602, #28629, #74085, #41262, #54709, #80003, #80415, #22316, #73679, #42077, #37419, #18073, #10526, #75733, #68993, #49625, #75318, #68187, #36583, #30270, #61442, #23545, #44126, #43708, #23957, #17263, #29857, #5430, #11343, #42892, #62262, #43296, #4598, #82458, #10110, #55933, #17665, #37003, #62681, #68586, #42483, #69411, #24366, #3789, #11765, #81648, #5023, #30691, #74918, #50036, #29453, #55111, #56354, #82053, #49213, #24773, #80820 ),
 ( #63092, #48803, #36181, #76143, #35772, #31091, #56758, #10927, #50442, #18484, #23135, #61853, #4194, #74501, #16849, #55520, #81228, #71486, #7516, #26020, #52519, #6666, #38653, #32338, #78227, #364, #51679, #13833, #39492, #50854, #64330, #77382, #5833, #31506, #57166, #12997, #45787, #77808, #7087, #44944, #58000, #76554, #19713, #20139, #20560, #82865, #25187, #18882, #6247, #12576, #65179, #52099, #70641, #69818, #70220, #57585, #45372, #31924, #71067, #33184, #58853, #44531, #13411, #38233, #39066, #63911, #26446, #83276, #25599, #64749, #12167, #51262, #76964, #19293, #1210, #26860, #32758, #58425, #37824, #786, #63500, #55736, #53360, #21386, #40738, #61232, #67980, #81444, #3998, #17060, #3586, #14258, #29252, #59675, #10323, #20971, #47041, #36392, #27275, #46630, #72326, #14673, #78649, #52936, #40330, #61657, #54916, #35987, #35569, #39916, #8758, #29662, #80622, #55324, #74296, #66009, #22934, #81033, #23345, #2030, #79070, #15080, #48600, #46212, #16642, #42282, #49016, #42699, #8347, #66422, #74713, #65605, #7936, #33597, #72734, #68396, #10735, #62066, #4405, #30073, #34013, #71907, #59262, #1619, #27696, #43102, #36802, #43511, #49838, #51062, #6050, #24581, #6467, #24169, #11560, #18285, #69211, #43928, #25398, #70436, #30489, #82667, #56154, #24982, #75537, #63710, #17877, #81857, #76358, #57794, #37217, #62896, #5231, #76762, #12793, #18690, #56969, #38449, #50656, #64133, #32137, #30895, #82263, #69624, #37624, #44333, #23759, #31722, #19092, #63300, #75126, #5638, #56562, #70024, #50248, #75944, #49432, #4813, #11969, #31305, #12377, #38035, #57383, #83077, #44741, #17471, #68798, #11143, #62478, #1008, #52733, #26661, #33401, #14052, #58215, #71698, #59063, #78444, #19937, #71279, #46423, #45586, #13628, #7303, #64967, #39706, #39280, #65398, #13217, #581, #59476, #25814, #27074, #58640, #32972, #52315, #72115, #40127, #64544, #6881, #20770, #78022, #20350, #7734, #14473, #65813, #46002, #1829, #1418, #8146, #33811, #27489, #77177, #161, #51474, #19508, #45162, #70867, #38863, #32551, #26235, #51897, #77603, #82525, #77036, #31161, #56828, #44195, #76214, #18952, #24843, #70294, #30760, #18143, #58071, #17737, #57656, #12239, #50510, #18550, #19368, #13069, #24437, #75801, #18, #69885, #57234, #12646, #45018, #38724, #31578, #437, #37895, #63571, #5906, #26092, #82935, #25257, #70718, #64401, #56422, #50921, #76621, #11416, #37071, #62756, #44599, #51332, #25672, #38308, #63982, #6319, #82122, #31996, #6737, #75391, #5092, #50104, #43777, #11833, #69480, #32408, #43366, #69066, #37486, #63160, #5499, #46282, #71556, #71978, #53432, #15153, #58498, #27348, #862, #53006, #52174, #8417, #77877, #26519, #21044, #2524, #45858, #20208, #13905, #21457, #40810, #46703, #1690, #66495, #78719, #8829, #60169, #58923, #26931, #14332, #65680, #72396, #51752, #34085, #47115, #8007, #19790, #33671, #65252, #14746, #39563, #52592, #34506, #32830, #7589, #33261, #1282, #78299, #20631, #39990, #66081, #59333, #40400, #77455, #59748, #2102, #27767, #72804, #45442, #79140, #71138, #13480, #39137, #64818, #7159, #35332, #3344, #22698, #42048, #48773, #36560, #68155, #81203, #67744, #79553, #10077, #41638, #74472, #2936, #29008, #17236, #9251, #28600, #54257, #79973, #60586, #34923, #22286, #42455, #35741, #16819, #16402, #21866, #74055, #10499, #61409, #36153, #55081, #47947, #3758, #61826, #4166, #67329, #60995, #29830, #9662, #54674, #80386, #48357, #80790, #29423, #23105, #66919, #73649, #10902, #53840, #55493, #23518, #49187, #74890, #42866, #68559, #15991, #62237, #28182, #47531, #73222, #15573, #41232, #34279, #65859, #59940, #39332, #53197, #46473, #20403, #79324, #2296, #65018, #21643, #14523, #59523, #40175, #52786, #27956, #7353, #33022, #72580, #8193, #1467, #2709, #58691, #1056, #26710, #1880, #39754, #47303, #27540, #33859, #78495, #52366, #72167, #14928, #60362, #34699, #28370, #59110, #54031, #78073, #78910, #33450, #14102, #71749, #27122, #46055, #65451, #7782, #72993, #53615, #20818, #15346, #21231, #46887, #40587, #66269 ) ),
 .UNSPECIFIED., .F., .F., .F. ) 
 B_SPLINE_SURFACE_WITH_KNOTS ( ( 2, 2 ),
 ( 3, 2, 2, 2, 2, 2, 2, 2, 2, 2, 2, 2, 2, 2, 2, 2, 2, 2, 2, 2, 2, 2, 2, 2, 2, 2, 2, 2, 2, 2, 2, 2, 2, 2, 2, 2, 2, 2, 2, 2, 2, 2, 2, 2, 2, 2, 2, 2, 2, 2, 2, 2, 2, 2, 2, 2, 2, 2, 2, 2, 2, 2, 2, 2, 2, 2, 2, 2, 2, 2, 2, 2, 2, 2, 2, 2, 2, 2, 2, 2, 2, 2, 2, 2, 2, 2, 2, 2, 2, 2, 2, 2, 2, 2, 2, 2, 2, 2, 2, 2, 2, 2, 2, 2, 2, 2, 2, 2, 2, 2, 2, 2, 2, 2, 2, 2, 2, 2, 2, 2, 2, 2, 2, 2, 2, 2, 2, 2, 2, 2, 2, 2, 2, 2, 2, 2, 2, 2, 2, 2, 2, 2, 2, 2, 2, 2, 2, 2, 2, 2, 2, 2, 2, 2, 2, 2, 2, 2, 2, 2, 2, 2, 2, 2, 2, 2, 2, 2, 2, 2, 2, 2, 2, 2, 2, 2, 2, 2, 2, 2, 2, 2, 2, 2, 2, 2, 2, 2, 2, 2, 2, 2, 2, 2, 2, 2, 2, 2, 2, 2, 2, 2, 2, 2, 2, 2, 2, 2, 2, 2, 2, 2, 2, 2, 2, 2, 2, 2, 2, 2, 2, 2, 2, 2, 2, 2, 2, 2, 2, 2, 2, 2, 2, 2, 2, 2, 2, 2, 2, 2, 2, 2, 2, 2, 2, 2, 2, 2, 2, 2, 2, 2, 2, 2, 2, 3 ),
 ( 0.000000000000000000, 1.000000000000000000 ),
 ( 0.000000000000000000, 0.003787878787878787984, 0.007575757575757575968, 0.01136363636363636395, 0.01515151515151515194, 0.01893939393939393992, 0.02272727272727272790, 0.02651515151515151589, 0.03030303030303030387, 0.03409090909090908839, 0.03787878787878787984, 0.04166666666666666435, 0.04545454545454545581, 0.04924242424242424032, 0.05303030303030303177, 0.05681818181818181629, 0.06060606060606060774, 0.06439393939393939226, 0.06818181818181817677, 0.07196969696969697516, 0.07575757575757575968, 0.07954545454545454419, 0.08333333333333332871, 0.08712121212121212710, 0.09090909090909091161, 0.09469696969696969613, 0.09848484848484848064, 0.1022727272727272790, 0.1060606060606060635, 0.1098484848484848481, 0.1136363636363636326, 0.1174242424242424310, 0.1212121212121212155, 0.1250000000000000000, 0.1287878787878787845, 0.1325757575757575690, 0.1363636363636363535, 0.1401515151515151381, 0.1439393939393939503, 0.1477272727272727348, 0.1515151515151515194, 0.1553030303030303039, 0.1590909090909090884, 0.1628787878787878729, 0.1666666666666666574, 0.1704545454545454419, 0.1742424242424242542, 0.1780303030303030387, 0.1818181818181818232, 0.1856060606060606077, 0.1893939393939393923, 0.1931818181818181768, 0.1969696969696969613, 0.2007575757575757458, 0.2045454545454545581, 0.2083333333333333426, 0.2121212121212121271, 0.2159090909090909116, 0.2196969696969696961, 0.2234848484848484806, 0.2272727272727272652, 0.2310606060606060497, 0.2348484848484848619, 0.2386363636363636465, 0.2424242424242424310, 0.2462121212121212155, 0.2500000000000000000, 0.2537878787878787845, 0.2575757575757575690, 0.2613636363636363535, 0.2651515151515151381, 0.2689393939393939226, 0.2727272727272727071, 0.2765151515151514916, 0.2803030303030302761, 0.2840909090909091161, 0.2878787878787879007, 0.2916666666666666852, 0.2954545454545454697, 0.2992424242424242542, 0.3030303030303030387, 0.3068181818181818232, 0.3106060606060606077, 0.3143939393939393923, 0.3181818181818181768, 0.3219696969696969613, 0.3257575757575757458, 0.3295454545454545303, 0.3333333333333333148, 0.3371212121212120993, 0.3409090909090908839, 0.3446969696969697239, 0.3484848484848485084, 0.3522727272727272929, 0.3560606060606060774, 0.3598484848484848619, 0.3636363636363636465, 0.3674242424242424310, 0.3712121212121212155, 0.3750000000000000000, 0.3787878787878787845, 0.3825757575757575690, 0.3863636363636363535, 0.3901515151515151381, 0.3939393939393939226, 0.3977272727272727071, 0.4015151515151514916, 0.4053030303030302761, 0.4090909090909091161, 0.4128787878787879007, 0.4166666666666666852, 0.4204545454545454697, 0.4242424242424242542, 0.4280303030303030387, 0.4318181818181818232, 0.4356060606060606077, 0.4393939393939393923, 0.4431818181818181768, 0.4469696969696969613, 0.4507575757575757458, 0.4545454545454545303, 0.4583333333333333148, 0.4621212121212120993, 0.4659090909090908839, 0.4696969696969697239, 0.4734848484848485084, 0.4772727272727272929, 0.4810606060606060774, 0.4848484848484848619, 0.4886363636363636465, 0.4924242424242424310, 0.4962121212121212155, 0.5000000000000000000, 0.5037878787878787845, 0.5075757575757575690, 0.5113636363636363535, 0.5151515151515151381, 0.5189393939393939226, 0.5227272727272727071, 0.5265151515151514916, 0.5303030303030302761, 0.5340909090909090606, 0.5378787878787878451, 0.5416666666666666297, 0.5454545454545454142, 0.5492424242424241987, 0.5530303030303029832, 0.5568181818181817677, 0.5606060606060605522, 0.5643939393939394478, 0.5681818181818182323, 0.5719696969696970168, 0.5757575757575758013, 0.5795454545454545858, 0.5833333333333333703, 0.5871212121212121549, 0.5909090909090909394, 0.5946969696969697239, 0.5984848484848485084, 0.6022727272727272929, 0.6060606060606060774, 0.6098484848484848619, 0.6136363636363636465, 0.6174242424242424310, 0.6212121212121212155, 0.6250000000000000000, 0.6287878787878787845, 0.6325757575757575690, 0.6363636363636363535, 0.6401515151515151381, 0.6439393939393939226, 0.6477272727272727071, 0.6515151515151514916, 0.6553030303030302761, 0.6590909090909090606, 0.6628787878787878451, 0.6666666666666666297, 0.6704545454545454142, 0.6742424242424241987, 0.6780303030303029832, 0.6818181818181817677, 0.6856060606060605522, 0.6893939393939394478, 0.6931818181818182323, 0.6969696969696970168, 0.7007575757575758013, 0.7045454545454545858, 0.7083333333333333703, 0.7121212121212121549, 0.7159090909090909394, 0.7196969696969697239, 0.7234848484848485084, 0.7272727272727272929, 0.7310606060606060774, 0.7348484848484848619, 0.7386363636363636465, 0.7424242424242424310, 0.7462121212121212155, 0.7500000000000000000, 0.7537878787878787845, 0.7575757575757575690, 0.7613636363636363535, 0.7651515151515151381, 0.7689393939393939226, 0.7727272727272727071, 0.7765151515151514916, 0.7803030303030302761, 0.7840909090909090606, 0.7878787878787878451, 0.7916666666666666297, 0.7954545454545454142, 0.7992424242424241987, 0.8030303030303029832, 0.8068181818181817677, 0.8106060606060605522, 0.8143939393939394478, 0.8181818181818182323, 0.8219696969696970168, 0.8257575757575758013, 0.8295454545454545858, 0.8333333333333333703, 0.8371212121212121549, 0.8409090909090909394, 0.8446969696969697239, 0.8484848484848485084, 0.8522727272727272929, 0.8560606060606060774, 0.8598484848484848619, 0.8636363636363636465, 0.8674242424242424310, 0.8712121212121212155, 0.8750000000000000000, 0.8787878787878787845, 0.8825757575757575690, 0.8863636363636363535, 0.8901515151515151381, 0.8939393939393939226, 0.8977272727272727071, 0.9015151515151514916, 0.9053030303030302761, 0.9090909090909090606, 0.9128787878787878451, 0.9166666666666666297, 0.9204545454545454142, 0.9242424242424241987, 0.9280303030303029832, 0.9318181818181817677, 0.9356060606060605522, 0.9393939393939394478, 0.9431818181818182323, 0.9469696969696970168, 0.9507575757575758013, 0.9545454545454545858, 0.9583333333333333703, 0.9621212121212121549, 0.9659090909090909394 ),
 .UNSPECIFIED. ) 
 GEOMETRIC_REPRESENTATION_ITEM ( )  RATIONAL_B_SPLINE_SURFACE ( (
 ( 1.000000000000000000, 0.9659258262890683122, 1.000000000000000000, 0.9659258262890683122, 1.000000000000000000, 0.9659258262890683122, 1.000000000000000000, 0.9659258262890683122, 1.000000000000000000, 0.9659258262890683122, 1.000000000000000000, 0.9659258262890683122, 1.000000000000000000, 0.9659258262890683122, 1.000000000000000000, 0.9659258262890683122, 1.000000000000000000, 0.9659258262890683122, 1.000000000000000000, 0.9659258262890683122, 1.000000000000000000, 0.9659258262890683122, 1.000000000000000000, 0.9659258262890683122, 1.000000000000000000, 0.9659258262890683122, 1.000000000000000000, 0.9659258262890683122, 1.000000000000000000, 0.9659258262890683122, 1.000000000000000000, 0.9659258262890683122, 1.000000000000000000, 0.9659258262890683122, 1.000000000000000000, 0.9659258262890683122, 1.000000000000000000, 0.9659258262890683122, 1.000000000000000000, 0.9659258262890683122, 1.000000000000000000, 0.9659258262890683122, 1.000000000000000000, 0.9659258262890683122, 1.000000000000000000, 0.9659258262890683122, 1.000000000000000000, 0.9659258262890683122, 1.000000000000000000, 0.9659258262890683122, 1.000000000000000000, 0.9659258262890683122, 1.000000000000000000, 0.9659258262890683122, 1.000000000000000000, 0.9659258262890683122, 1.000000000000000000, 0.9659258262890683122, 1.000000000000000000, 0.9659258262890683122, 1.000000000000000000, 0.9659258262890683122, 1.000000000000000000, 0.9659258262890683122, 1.000000000000000000, 0.9659258262890683122, 1.000000000000000000, 0.9659258262890683122, 1.000000000000000000, 0.9659258262890683122, 1.000000000000000000, 0.9659258262890683122, 1.000000000000000000, 0.9659258262890683122, 1.000000000000000000, 0.9659258262890683122, 1.000000000000000000, 0.9659258262890683122, 1.000000000000000000, 0.9659258262890683122, 1.000000000000000000, 0.9659258262890683122, 1.000000000000000000, 0.9659258262890683122, 1.000000000000000000, 0.9659258262890683122, 1.000000000000000000, 0.9659258262890683122, 1.000000000000000000, 0.9659258262890683122, 1.000000000000000000, 0.9659258262890683122, 1.000000000000000000, 0.9659258262890683122, 1.000000000000000000, 0.9659258262890683122, 1.000000000000000000, 0.9659258262890683122, 1.000000000000000000, 0.9659258262890683122, 1.000000000000000000, 0.9659258262890683122, 1.000000000000000000, 0.9659258262890683122, 1.000000000000000000, 0.9659258262890683122, 1.000000000000000000, 0.9659258262890683122, 1.000000000000000000, 0.9659258262890683122, 1.000000000000000000, 0.9659258262890683122, 1.000000000000000000, 0.9659258262890683122, 1.000000000000000000, 0.9659258262890683122, 1.000000000000000000, 0.9659258262890683122, 1.000000000000000000, 0.9659258262890683122, 1.000000000000000000, 0.9659258262890683122, 1.000000000000000000, 0.9659258262890683122, 1.000000000000000000, 0.9659258262890683122, 1.000000000000000000, 0.9659258262890683122, 1.000000000000000000, 0.9659258262890683122, 1.000000000000000000, 0.9659258262890683122, 1.000000000000000000, 0.9659258262890683122, 1.000000000000000000, 0.9659258262890683122, 1.000000000000000000, 0.9659258262890683122, 1.000000000000000000, 0.9659258262890683122, 1.000000000000000000, 0.9659258262890683122, 1.000000000000000000, 0.9659258262890683122, 1.000000000000000000, 0.9659258262890683122, 1.000000000000000000, 0.9659258262890683122, 1.000000000000000000, 0.9659258262890683122, 1.000000000000000000, 0.9659258262890683122, 1.000000000000000000, 0.9659258262890683122, 1.000000000000000000, 0.9659258262890683122, 1.000000000000000000, 0.9659258262890683122, 1.000000000000000000, 0.9659258262890683122, 1.000000000000000000, 0.9659258262890683122, 1.000000000000000000, 0.9659258262890683122, 1.000000000000000000, 0.9659258262890683122, 1.000000000000000000, 0.9659258262890683122, 1.000000000000000000, 0.9659258262890683122, 1.000000000000000000, 0.9659258262890683122, 1.000000000000000000, 0.9659258262890683122, 1.000000000000000000, 0.9659258262890683122, 1.000000000000000000, 0.9659258262890683122, 1.000000000000000000, 0.9659258262890683122, 1.000000000000000000, 0.9659258262890683122, 1.000000000000000000, 0.9659258262890683122, 1.000000000000000000, 0.9659258262890683122, 1.000000000000000000, 0.9659258262890683122, 1.000000000000000000, 0.9659258262890683122, 1.000000000000000000, 0.9659258262890683122, 1.000000000000000000, 0.9659258262890683122, 1.000000000000000000, 0.9659258262890683122, 1.000000000000000000, 0.9659258262890683122, 1.000000000000000000, 0.9659258262890683122, 1.000000000000000000, 0.9659258262890683122, 1.000000000000000000, 0.9659258262890683122, 1.000000000000000000, 0.9659258262890683122, 1.000000000000000000, 0.9659258262890683122, 1.000000000000000000, 0.9659258262890683122, 1.000000000000000000, 0.9659258262890683122, 1.000000000000000000, 0.9659258262890683122, 1.000000000000000000, 0.9659258262890683122, 1.000000000000000000, 0.9659258262890683122, 1.000000000000000000, 0.9659258262890683122, 1.000000000000000000, 0.9659258262890683122, 1.000000000000000000, 0.9659258262890683122, 1.000000000000000000, 0.9659258262890683122, 1.000000000000000000, 0.9659258262890683122, 1.000000000000000000, 0.9659258262890683122, 1.000000000000000000, 0.9659258262890683122, 1.000000000000000000, 0.9659258262890683122, 1.000000000000000000, 0.9659258262890683122, 1.000000000000000000, 0.9659258262890683122, 1.000000000000000000, 0.9659258262890683122, 1.000000000000000000, 0.9659258262890683122, 1.000000000000000000, 0.9659258262890683122, 1.000000000000000000, 0.9659258262890683122, 1.000000000000000000, 0.9659258262890683122, 1.000000000000000000, 0.9659258262890683122, 1.000000000000000000, 0.9659258262890683122, 1.000000000000000000, 0.9659258262890683122, 1.000000000000000000, 0.9659258262890683122, 1.000000000000000000, 0.9659258262890683122, 1.000000000000000000, 0.9659258262890683122, 1.000000000000000000, 0.9659258262890683122, 1.000000000000000000, 0.9659258262890683122, 1.000000000000000000, 0.9659258262890683122, 1.000000000000000000, 0.9659258262890683122, 1.000000000000000000, 0.9659258262890683122, 1.000000000000000000, 0.9659258262890683122, 1.000000000000000000, 0.9659258262890683122, 1.000000000000000000, 0.9659258262890683122, 1.000000000000000000, 0.9659258262890683122, 1.000000000000000000, 0.9659258262890683122, 1.000000000000000000, 0.9659258262890683122, 1.000000000000000000, 0.9659258262890683122, 1.000000000000000000, 0.9659258262890683122, 1.000000000000000000, 0.9659258262890683122, 1.000000000000000000, 0.9659258262890683122, 1.000000000000000000, 0.9659258262890683122, 1.000000000000000000, 0.9659258262890683122, 1.000000000000000000, 0.9659258262890683122, 1.000000000000000000, 0.9659258262890683122, 1.000000000000000000, 0.9659258262890683122, 1.000000000000000000, 0.9659258262890683122, 1.000000000000000000, 0.9659258262890683122, 1.000000000000000000, 0.9659258262890683122, 1.000000000000000000, 0.9659258262890683122, 1.000000000000000000, 0.9659258262890683122, 1.000000000000000000, 0.9659258262890683122, 1.000000000000000000, 0.9659258262890683122, 1.000000000000000000, 0.9659258262890683122, 1.000000000000000000, 0.9659258262890683122, 1.000000000000000000, 0.9659258262890683122, 1.000000000000000000, 0.9659258262890683122, 1.000000000000000000, 0.9659258262890683122, 1.000000000000000000, 0.9659258262890683122, 1.000000000000000000, 0.9659258262890683122, 1.000000000000000000, 0.9659258262890683122, 1.000000000000000000, 0.9659258262890683122, 1.000000000000000000, 0.9659258262890683122, 1.000000000000000000, 0.9659258262890683122, 1.000000000000000000, 0.9659258262890683122, 1.000000000000000000, 0.9659258262890683122, 1.000000000000000000, 0.9659258262890683122, 1.000000000000000000, 0.9659258262890683122, 1.000000000000000000, 0.9659258262890683122, 1.000000000000000000, 0.9659258262890683122, 1.000000000000000000, 0.9659258262890683122, 1.000000000000000000, 0.9659258262890683122, 1.000000000000000000, 0.9659258262890683122, 1.000000000000000000, 0.9659258262890683122, 1.000000000000000000, 0.9659258262890683122, 1.000000000000000000, 0.9659258262890683122, 1.000000000000000000, 0.9659258262890683122, 1.000000000000000000, 0.9659258262890683122, 1.000000000000000000, 0.9659258262890683122, 1.000000000000000000, 0.9659258262890683122, 1.000000000000000000, 0.9659258262890683122, 1.000000000000000000, 0.9659258262890683122, 1.000000000000000000, 0.9659258262890683122, 1.000000000000000000, 0.9659258262890683122, 1.000000000000000000, 0.9659258262890683122, 1.000000000000000000, 0.9659258262890683122, 1.000000000000000000, 0.9659258262890683122, 1.000000000000000000, 0.9659258262890683122, 1.000000000000000000, 0.9659258262890683122, 1.000000000000000000, 0.9659258262890683122, 1.000000000000000000, 0.9659258262890683122, 1.000000000000000000, 0.9659258262890683122, 1.000000000000000000, 0.9659258262890683122, 1.000000000000000000, 0.9659258262890683122, 1.000000000000000000, 0.9659258262890683122, 1.000000000000000000, 0.9659258262890683122, 1.000000000000000000, 0.9659258262890683122, 1.000000000000000000, 0.9659258262890683122, 1.000000000000000000, 0.9659258262890683122, 1.000000000000000000, 0.9659258262890683122, 1.000000000000000000, 0.9659258262890683122, 1.000000000000000000, 0.9659258262890683122, 1.000000000000000000, 0.9659258262890683122, 1.000000000000000000, 0.9659258262890683122, 1.000000000000000000, 0.9659258262890683122, 1.000000000000000000, 0.9659258262890683122, 1.000000000000000000, 0.9659258262890683122, 1.000000000000000000, 0.9659258262890683122, 1.000000000000000000, 0.9659258262890683122, 1.000000000000000000, 0.9659258262890683122, 1.000000000000000000, 0.9659258262890683122, 1.000000000000000000, 0.9659258262890683122, 1.000000000000000000, 0.9659258262890683122, 1.000000000000000000, 0.9659258262890683122, 1.000000000000000000, 0.9659258262890683122, 1.000000000000000000, 0.9659258262890683122, 1.000000000000000000, 0.9659258262890683122, 1.000000000000000000, 0.9659258262890683122, 1.000000000000000000, 0.9659258262890683122, 1.000000000000000000, 0.9659258262890683122, 1.000000000000000000, 0.9659258262890683122, 1.000000000000000000, 0.9659258262890683122, 1.000000000000000000, 0.9659258262890683122, 1.000000000000000000, 0.9659258262890683122, 1.000000000000000000, 0.9659258262890683122, 1.000000000000000000, 0.9659258262890683122, 1.000000000000000000, 0.9659258262890683122, 1.000000000000000000, 0.9659258262890683122, 1.000000000000000000, 0.9659258262890683122, 1.000000000000000000, 0.9659258262890683122, 1.000000000000000000, 0.9659258262890683122, 1.000000000000000000, 0.9659258262890683122, 1.000000000000000000, 0.9659258262890683122, 1.000000000000000000, 0.9659258262890683122, 1.000000000000000000, 0.9659258262890683122, 1.000000000000000000, 0.9659258262890683122, 1.000000000000000000, 0.9659258262890683122, 1.000000000000000000, 0.9659258262890683122, 1.000000000000000000, 0.9659258262890683122, 1.000000000000000000, 0.9659258262890683122, 1.000000000000000000, 0.9659258262890683122, 1.000000000000000000, 0.9659258262890683122, 1.000000000000000000, 0.9659258262890683122, 1.000000000000000000, 0.9659258262890683122, 1.000000000000000000, 0.9659258262890683122, 1.000000000000000000, 0.9659258262890683122, 1.000000000000000000, 0.9659258262890683122, 1.000000000000000000, 0.9659258262890683122, 1.000000000000000000, 0.9659258262890683122, 1.000000000000000000, 0.9659258262890683122, 1.000000000000000000, 0.9659258262890683122, 1.000000000000000000),
 ( 1.000000000000000000, 0.9659258262890683122, 1.000000000000000000, 0.9659258262890683122, 1.000000000000000000, 0.9659258262890683122, 1.000000000000000000, 0.9659258262890683122, 1.000000000000000000, 0.9659258262890683122, 1.000000000000000000, 0.9659258262890683122, 1.000000000000000000, 0.9659258262890683122, 1.000000000000000000, 0.9659258262890683122, 1.000000000000000000, 0.9659258262890683122, 1.000000000000000000, 0.9659258262890683122, 1.000000000000000000, 0.9659258262890683122, 1.000000000000000000, 0.9659258262890683122, 1.000000000000000000, 0.9659258262890683122, 1.000000000000000000, 0.9659258262890683122, 1.000000000000000000, 0.9659258262890683122, 1.000000000000000000, 0.9659258262890683122, 1.000000000000000000, 0.9659258262890683122, 1.000000000000000000, 0.9659258262890683122, 1.000000000000000000, 0.9659258262890683122, 1.000000000000000000, 0.9659258262890683122, 1.000000000000000000, 0.9659258262890683122, 1.000000000000000000, 0.9659258262890683122, 1.000000000000000000, 0.9659258262890683122, 1.000000000000000000, 0.9659258262890683122, 1.000000000000000000, 0.9659258262890683122, 1.000000000000000000, 0.9659258262890683122, 1.000000000000000000, 0.9659258262890683122, 1.000000000000000000, 0.9659258262890683122, 1.000000000000000000, 0.9659258262890683122, 1.000000000000000000, 0.9659258262890683122, 1.000000000000000000, 0.9659258262890683122, 1.000000000000000000, 0.9659258262890683122, 1.000000000000000000, 0.9659258262890683122, 1.000000000000000000, 0.9659258262890683122, 1.000000000000000000, 0.9659258262890683122, 1.000000000000000000, 0.9659258262890683122, 1.000000000000000000, 0.9659258262890683122, 1.000000000000000000, 0.9659258262890683122, 1.000000000000000000, 0.9659258262890683122, 1.000000000000000000, 0.9659258262890683122, 1.000000000000000000, 0.9659258262890683122, 1.000000000000000000, 0.9659258262890683122, 1.000000000000000000, 0.9659258262890683122, 1.000000000000000000, 0.9659258262890683122, 1.000000000000000000, 0.9659258262890683122, 1.000000000000000000, 0.9659258262890683122, 1.000000000000000000, 0.9659258262890683122, 1.000000000000000000, 0.9659258262890683122, 1.000000000000000000, 0.9659258262890683122, 1.000000000000000000, 0.9659258262890683122, 1.000000000000000000, 0.9659258262890683122, 1.000000000000000000, 0.9659258262890683122, 1.000000000000000000, 0.9659258262890683122, 1.000000000000000000, 0.9659258262890683122, 1.000000000000000000, 0.9659258262890683122, 1.000000000000000000, 0.9659258262890683122, 1.000000000000000000, 0.9659258262890683122, 1.000000000000000000, 0.9659258262890683122, 1.000000000000000000, 0.9659258262890683122, 1.000000000000000000, 0.9659258262890683122, 1.000000000000000000, 0.9659258262890683122, 1.000000000000000000, 0.9659258262890683122, 1.000000000000000000, 0.9659258262890683122, 1.000000000000000000, 0.9659258262890683122, 1.000000000000000000, 0.9659258262890683122, 1.000000000000000000, 0.9659258262890683122, 1.000000000000000000, 0.9659258262890683122, 1.000000000000000000, 0.9659258262890683122, 1.000000000000000000, 0.9659258262890683122, 1.000000000000000000, 0.9659258262890683122, 1.000000000000000000, 0.9659258262890683122, 1.000000000000000000, 0.9659258262890683122, 1.000000000000000000, 0.9659258262890683122, 1.000000000000000000, 0.9659258262890683122, 1.000000000000000000, 0.9659258262890683122, 1.000000000000000000, 0.9659258262890683122, 1.000000000000000000, 0.9659258262890683122, 1.000000000000000000, 0.9659258262890683122, 1.000000000000000000, 0.9659258262890683122, 1.000000000000000000, 0.9659258262890683122, 1.000000000000000000, 0.9659258262890683122, 1.000000000000000000, 0.9659258262890683122, 1.000000000000000000, 0.9659258262890683122, 1.000000000000000000, 0.9659258262890683122, 1.000000000000000000, 0.9659258262890683122, 1.000000000000000000, 0.9659258262890683122, 1.000000000000000000, 0.9659258262890683122, 1.000000000000000000, 0.9659258262890683122, 1.000000000000000000, 0.9659258262890683122, 1.000000000000000000, 0.9659258262890683122, 1.000000000000000000, 0.9659258262890683122, 1.000000000000000000, 0.9659258262890683122, 1.000000000000000000, 0.9659258262890683122, 1.000000000000000000, 0.9659258262890683122, 1.000000000000000000, 0.9659258262890683122, 1.000000000000000000, 0.9659258262890683122, 1.000000000000000000, 0.9659258262890683122, 1.000000000000000000, 0.9659258262890683122, 1.000000000000000000, 0.9659258262890683122, 1.000000000000000000, 0.9659258262890683122, 1.000000000000000000, 0.9659258262890683122, 1.000000000000000000, 0.9659258262890683122, 1.000000000000000000, 0.9659258262890683122, 1.000000000000000000, 0.9659258262890683122, 1.000000000000000000, 0.9659258262890683122, 1.000000000000000000, 0.9659258262890683122, 1.000000000000000000, 0.9659258262890683122, 1.000000000000000000, 0.9659258262890683122, 1.000000000000000000, 0.9659258262890683122, 1.000000000000000000, 0.9659258262890683122, 1.000000000000000000, 0.9659258262890683122, 1.000000000000000000, 0.9659258262890683122, 1.000000000000000000, 0.9659258262890683122, 1.000000000000000000, 0.9659258262890683122, 1.000000000000000000, 0.9659258262890683122, 1.000000000000000000, 0.9659258262890683122, 1.000000000000000000, 0.9659258262890683122, 1.000000000000000000, 0.9659258262890683122, 1.000000000000000000, 0.9659258262890683122, 1.000000000000000000, 0.9659258262890683122, 1.000000000000000000, 0.9659258262890683122, 1.000000000000000000, 0.9659258262890683122, 1.000000000000000000, 0.9659258262890683122, 1.000000000000000000, 0.9659258262890683122, 1.000000000000000000, 0.9659258262890683122, 1.000000000000000000, 0.9659258262890683122, 1.000000000000000000, 0.9659258262890683122, 1.000000000000000000, 0.9659258262890683122, 1.000000000000000000, 0.9659258262890683122, 1.000000000000000000, 0.9659258262890683122, 1.000000000000000000, 0.9659258262890683122, 1.000000000000000000, 0.9659258262890683122, 1.000000000000000000, 0.9659258262890683122, 1.000000000000000000, 0.9659258262890683122, 1.000000000000000000, 0.9659258262890683122, 1.000000000000000000, 0.9659258262890683122, 1.000000000000000000, 0.9659258262890683122, 1.000000000000000000, 0.9659258262890683122, 1.000000000000000000, 0.9659258262890683122, 1.000000000000000000, 0.9659258262890683122, 1.000000000000000000, 0.9659258262890683122, 1.000000000000000000, 0.9659258262890683122, 1.000000000000000000, 0.9659258262890683122, 1.000000000000000000, 0.9659258262890683122, 1.000000000000000000, 0.9659258262890683122, 1.000000000000000000, 0.9659258262890683122, 1.000000000000000000, 0.9659258262890683122, 1.000000000000000000, 0.9659258262890683122, 1.000000000000000000, 0.9659258262890683122, 1.000000000000000000, 0.9659258262890683122, 1.000000000000000000, 0.9659258262890683122, 1.000000000000000000, 0.9659258262890683122, 1.000000000000000000, 0.9659258262890683122, 1.000000000000000000, 0.9659258262890683122, 1.000000000000000000, 0.9659258262890683122, 1.000000000000000000, 0.9659258262890683122, 1.000000000000000000, 0.9659258262890683122, 1.000000000000000000, 0.9659258262890683122, 1.000000000000000000, 0.9659258262890683122, 1.000000000000000000, 0.9659258262890683122, 1.000000000000000000, 0.9659258262890683122, 1.000000000000000000, 0.9659258262890683122, 1.000000000000000000, 0.9659258262890683122, 1.000000000000000000, 0.9659258262890683122, 1.000000000000000000, 0.9659258262890683122, 1.000000000000000000, 0.9659258262890683122, 1.000000000000000000, 0.9659258262890683122, 1.000000000000000000, 0.9659258262890683122, 1.000000000000000000, 0.9659258262890683122, 1.000000000000000000, 0.9659258262890683122, 1.000000000000000000, 0.9659258262890683122, 1.000000000000000000, 0.9659258262890683122, 1.000000000000000000, 0.9659258262890683122, 1.000000000000000000, 0.9659258262890683122, 1.000000000000000000, 0.9659258262890683122, 1.000000000000000000, 0.9659258262890683122, 1.000000000000000000, 0.9659258262890683122, 1.000000000000000000, 0.9659258262890683122, 1.000000000000000000, 0.9659258262890683122, 1.000000000000000000, 0.9659258262890683122, 1.000000000000000000, 0.9659258262890683122, 1.000000000000000000, 0.9659258262890683122, 1.000000000000000000, 0.9659258262890683122, 1.000000000000000000, 0.9659258262890683122, 1.000000000000000000, 0.9659258262890683122, 1.000000000000000000, 0.9659258262890683122, 1.000000000000000000, 0.9659258262890683122, 1.000000000000000000, 0.9659258262890683122, 1.000000000000000000, 0.9659258262890683122, 1.000000000000000000, 0.9659258262890683122, 1.000000000000000000, 0.9659258262890683122, 1.000000000000000000, 0.9659258262890683122, 1.000000000000000000, 0.9659258262890683122, 1.000000000000000000, 0.9659258262890683122, 1.000000000000000000, 0.9659258262890683122, 1.000000000000000000, 0.9659258262890683122, 1.000000000000000000, 0.9659258262890683122, 1.000000000000000000, 0.9659258262890683122, 1.000000000000000000, 0.9659258262890683122, 1.000000000000000000, 0.9659258262890683122, 1.000000000000000000, 0.9659258262890683122, 1.000000000000000000, 0.9659258262890683122, 1.000000000000000000, 0.9659258262890683122, 1.000000000000000000, 0.9659258262890683122, 1.000000000000000000, 0.9659258262890683122, 1.000000000000000000, 0.9659258262890683122, 1.000000000000000000, 0.9659258262890683122, 1.000000000000000000, 0.9659258262890683122, 1.000000000000000000, 0.9659258262890683122, 1.000000000000000000, 0.9659258262890683122, 1.000000000000000000, 0.9659258262890683122, 1.000000000000000000, 0.9659258262890683122, 1.000000000000000000, 0.9659258262890683122, 1.000000000000000000, 0.9659258262890683122, 1.000000000000000000, 0.9659258262890683122, 1.000000000000000000, 0.9659258262890683122, 1.000000000000000000, 0.9659258262890683122, 1.000000000000000000, 0.9659258262890683122, 1.000000000000000000, 0.9659258262890683122, 1.000000000000000000, 0.9659258262890683122, 1.000000000000000000, 0.9659258262890683122, 1.000000000000000000, 0.9659258262890683122, 1.000000000000000000, 0.9659258262890683122, 1.000000000000000000, 0.9659258262890683122, 1.000000000000000000, 0.9659258262890683122, 1.000000000000000000, 0.9659258262890683122, 1.000000000000000000, 0.9659258262890683122, 1.000000000000000000, 0.9659258262890683122, 1.000000000000000000, 0.9659258262890683122, 1.000000000000000000, 0.9659258262890683122, 1.000000000000000000, 0.9659258262890683122, 1.000000000000000000, 0.9659258262890683122, 1.000000000000000000, 0.9659258262890683122, 1.000000000000000000, 0.9659258262890683122, 1.000000000000000000, 0.9659258262890683122, 1.000000000000000000, 0.9659258262890683122, 1.000000000000000000, 0.9659258262890683122, 1.000000000000000000, 0.9659258262890683122, 1.000000000000000000, 0.9659258262890683122, 1.000000000000000000, 0.9659258262890683122, 1.000000000000000000, 0.9659258262890683122, 1.000000000000000000, 0.9659258262890683122, 1.000000000000000000, 0.9659258262890683122, 1.000000000000000000, 0.9659258262890683122, 1.000000000000000000, 0.9659258262890683122, 1.000000000000000000, 0.9659258262890683122, 1.000000000000000000, 0.9659258262890683122, 1.000000000000000000, 0.9659258262890683122, 1.000000000000000000, 0.9659258262890683122, 1.000000000000000000, 0.9659258262890683122, 1.000000000000000000, 0.9659258262890683122, 1.000000000000000000, 0.9659258262890683122, 1.000000000000000000, 0.9659258262890683122, 1.000000000000000000, 0.9659258262890683122, 1.000000000000000000, 0.9659258262890683122, 1.000000000000000000) ) ) 
 REPRESENTATION_ITEM ( '' )  SURFACE ( )  );
#68700=CARTESIAN_POINT ( 'NONE',  ( 0.2230971128608932319, -0.3690944881889763329, 0.3153832671262228327 ) ) ;
#68702=CARTESIAN_POINT ( 'NONE',  ( 0.5577427821522314977, -0.3162353388693409650, -0.4822834645669289433 ) ) ;
#68705=CARTESIAN_POINT ( 'NONE',  ( -1.732283464566928277, -0.1870078740157479769, 0.3641732283464567677 ) ) ;
#68707=CARTESIAN_POINT ( 'NONE',  ( 1.227034120734908917, 0.2952755905511810774, -0.1292274648535930714 ) ) ;
#68708=CARTESIAN_POINT ( 'NONE',  ( 1.154855643044620184, 0.1283753931104746893, -0.1820866141732285504 ) ) ;
#68709=CARTESIAN_POINT ( 'NONE',  ( 0.02624671916010564918, -0.6046776061558809534, -0.2411417322834644161 ) ) ;
#68711=CARTESIAN_POINT ( 'NONE',  ( -0.3543307086614165824, 0.2952755905511811885, 0.000000000000000000 ) ) ;
#68712=CARTESIAN_POINT ( 'NONE',  ( -1.017060367454067249, -0.2845877964562161244, -0.3641732283464567121 ) ) ;
#68713=CARTESIAN_POINT ( 'NONE',  ( 0.2427821522309716595, -0.3162353388693409650, -0.4822834645669289433 ) ) ;
#68714=CARTESIAN_POINT ( 'NONE',  ( 0.1377952755905518800, -0.5400638737290844871, 0.3530559997133364547 ) ) ;
#68715=CARTESIAN_POINT ( 'NONE',  ( -1.193035393573954606, -4.754953748228849300E-15, -0.3627989612356167792 ) ) ;
#68718=CARTESIAN_POINT ( 'NONE',  ( 0.3018372703412079971, 0.05413385826771626580, -0.4176697321401330321 ) ) ;
#68719=CARTESIAN_POINT ( 'NONE',  ( -0.4527559055118102749, 0.1660481256975885056, 0.3530559997133364547 ) ) ;
#68720=CARTESIAN_POINT ( 'NONE',  ( -1.417322834645668772, -0.1870078740157480879, -0.4822834645669291653 ) ) ;
#68722=CARTESIAN_POINT ( 'NONE',  ( 1.207349081364829990, -0.6046776061558809534, -0.2411417322834644161 ) ) ;
#68723=CARTESIAN_POINT ( 'NONE',  ( 0.4921259842519691285, -0.5400638737290845981, -0.3530559997133363437 ) ) ;
#68725=CARTESIAN_POINT ( 'NONE',  ( -0.9383202099737524282, -0.05778040916215522460, 0.4822834645669289988 ) ) ;
#68726=CARTESIAN_POINT ( 'NONE',  ( 0.1509186351706045259, -0.05778040916215560624, -0.4822834645669293319 ) ) ;
#68727=CARTESIAN_POINT ( 'NONE',  ( -0.4396325459317577122, -0.6692913385826773087, -0.1292274648535924053 ) ) ;
#68729=CARTESIAN_POINT ( 'NONE',  ( 0.4002624671916016896, -0.08942795157527998196, 0.3641732283464567121 ) ) ;
#68730=CARTESIAN_POINT ( 'NONE',  ( -1.699475065616797398, 0.2952755905511811885, 0.1292274648535926551 ) ) ;
#68732=CARTESIAN_POINT ( 'NONE',  ( 0.1837270341207354329, 0.2306618581243848609, 0.2411417322834645549 ) ) ;
#68734=CARTESIAN_POINT ( 'NONE',  ( 1.377952755905512472, -0.6692913385826771977, 8.415575281601705876E-17 ) ) ;
#68738=CARTESIAN_POINT ( 'NONE',  ( 0.6167979002624679463, 0.05413385826771626580, -0.4176697321401330321 ) ) ;
#68739=CARTESIAN_POINT ( 'NONE',  ( 0.2230971128608929543, -0.004921259842519870586, -0.3153832671262229437 ) ) ;
#68741=CARTESIAN_POINT ( 'NONE',  ( -1.604771003085130099, 1.595806277125121797, 0.1466069496707745612 ) ) ;
#68746=CARTESIAN_POINT ( 'NONE',  ( 0.4068241469816279987, -0.4281496062992127816, -0.4176697321401328100 ) ) ;
#68747=CARTESIAN_POINT ( 'NONE',  ( -0.6692913385826764205, 0.2952755905511811885, 0.000000000000000000 ) ) ;
#68748=CARTESIAN_POINT ( 'NONE',  ( -1.338582677165353729, -0.1870078740157480879, -0.4822834645669291653 ) ) ;
#68749=CARTESIAN_POINT ( 'NONE',  ( 0.8464566929133865436, 0.1660481256975883668, -0.3530559997133364547 ) ) ;
#68751=CARTESIAN_POINT ( 'NONE',  ( 1.541994750656168645, -0.6692913385826771977, 0.1292274648535927661 ) ) ;
#68752=CARTESIAN_POINT ( 'NONE',  ( 1.568241469816273659, -0.08942795157528024563, -0.3641732283464568787 ) ) ;
#68753=CARTESIAN_POINT ( 'NONE',  ( 1.089238845144357759, -0.004921259842519870586, -0.3153832671262229437 ) ) ;
#68754=CARTESIAN_POINT ( 'NONE',  ( -0.8530183727034112984, 0.05413385826771666132, 0.4176697321401328100 ) ) ;
#68756=CARTESIAN_POINT ( 'NONE',  ( 1.496062992125985147, -0.1870078740157479769, 0.4822834645669291653 ) ) ;
#68758=CARTESIAN_POINT ( 'NONE',  ( -0.2952755905511803003, -0.5400638737290845981, -0.3530559997133363437 ) ) ;
#68759=CARTESIAN_POINT ( 'NONE',  ( 1.135170603674541256, -0.6692913385826773087, -0.1292274648535924053 ) ) ;
#68761=CARTESIAN_POINT ( 'NONE',  ( -1.207349081364828880, 0.1283753931104746893, -0.1820866141732285504 ) ) ;
#68762=CARTESIAN_POINT ( 'NONE',  ( 0.3477690288713918276, -0.6692913385826773087, -0.1292274648535924053 ) ) ;
#68763=CARTESIAN_POINT ( 'NONE',  ( 1.003937007874016185, 0.07958543189024071263, -0.2665933059059888421 ) ) ;
#68765=CARTESIAN_POINT ( 'NONE',  ( -1.279527559055116948, -0.4536011799217367080, 0.2665933059059888421 ) ) ;
#68766=CARTESIAN_POINT ( 'NONE',  ( 0.7677165354330716118, 0.1660481256975883668, -0.3530559997133364547 ) ) ;
#68768=CARTESIAN_POINT ( 'NONE',  ( -0.4199475065616791736, 0.1283753931104746893, -0.1820866141732285504 ) ) ;
#68769=CARTESIAN_POINT ( 'NONE',  ( -0.2099737532808391705, -0.6046776061558809534, -0.2411417322834644161 ) ) ;
#68770=CARTESIAN_POINT ( 'NONE',  ( -1.154855643044618851, 0.1283753931104748280, 0.1820866141732283561 ) ) ;
#68771=CARTESIAN_POINT ( 'NONE',  ( -0.8202099737532801971, -0.6692913385826771977, 0.1292274648535927661 ) ) ;
#68772=CARTESIAN_POINT ( 'NONE',  ( 1.220472440944882608, 0.2952755905511811885, 0.000000000000000000 ) ) ;
#68774=CARTESIAN_POINT ( 'NONE',  ( -1.023622047244093558, -0.1870078740157479769, 0.3641732283464567677 ) ) ;
#68776=CARTESIAN_POINT ( 'NONE',  ( 1.299212598425197429, 0.2952755905511811885, 0.000000000000000000 ) ) ;
#68778=CARTESIAN_POINT ( 'NONE',  ( -1.181102362204723644, -0.1870078740157480879, -0.4822834645669291653 ) ) ;
#68779=CARTESIAN_POINT ( 'NONE',  ( -1.220472440944881054, -0.5511811023622047445, 6.969142054262312111E-17 ) ) ;
#68780=CARTESIAN_POINT ( 'NONE',  ( -0.4330708661417315697, 0.1771653543307087630, 0.000000000000000000 ) ) ;
#68781=FACE_OUTER_BOUND ( 'NONE', #63614, .T. ) ;
#68782=CARTESIAN_POINT ( 'NONE',  ( -0.05249343832020911260, 0.2306618581243848609, 0.2411417322834645549 ) ) ;
#68783=CARTESIAN_POINT ( 'NONE',  ( -0.1312335958005241554, -0.5023911411419708095, -0.1820866141732282451 ) ) ;
#68784=CARTESIAN_POINT ( 'NONE',  ( -1.292650918635170010, -0.5511811023622046335, 0.09757992244046803654 ) ) ;
#68785=CARTESIAN_POINT ( 'NONE',  ( -1.666666666666665853, 0.05413385826771626580, -0.4176697321401330321 ) ) ;
#68786=CARTESIAN_POINT ( 'NONE',  ( 1.181102362204724976, -0.1870078740157480601, -0.3641732283464567677 ) ) ;
#68787=CARTESIAN_POINT ( 'NONE',  ( 1.108923884514436686, -0.3162353388693409650, -0.4822834645669289433 ) ) ;
#68789=CARTESIAN_POINT ( 'NONE',  ( 0.5511811023622055217, -0.1870078740157479769, 0.3641732283464567677 ) ) ;
#68790=CARTESIAN_POINT ( 'NONE',  ( 1.089238845144357759, 0.05413385826771626580, -0.4176697321401330321 ) ) ;
#68791=CARTESIAN_POINT ( 'NONE',  ( 0.8398950131233602345, 0.1283753931104746893, -0.1820866141732285504 ) ) ;
#68792=ORIENTED_EDGE ( 'NONE', *, *, #82940, .F. ) ;
#68793=CARTESIAN_POINT ( 'NONE',  ( -1.003937007874014853, 0.1660481256975885056, 0.3530559997133364547 ) ) ;
#68794=CARTESIAN_POINT ( 'NONE',  ( -1.089238845144356427, -0.4281496062992127816, -0.4176697321401328100 ) ) ;
#68795=CARTESIAN_POINT ( 'NONE',  ( -0.2296587926509179312, -0.3162353388693409650, -0.4822834645669289433 ) ) ;
#68798=CARTESIAN_POINT ( 'NONE',  ( 0.2624671916010504757, -0.6046776061558809534, -0.2411417322834644161 ) ) ;
#68799=CARTESIAN_POINT ( 'NONE',  ( -1.666666666666665853, 0.05413385826771626580, -0.4176697321401330321 ) ) ;
#68800=CARTESIAN_POINT ( 'NONE',  ( -0.03280839895013062252, 0.2952755905511810774, -0.1292274648535930714 ) ) ;
#68801=CARTESIAN_POINT ( 'NONE',  ( 0.9383202099737536495, -0.3162353388693405765, 0.4822834645669290543 ) ) ;
#68807=CARTESIAN_POINT ( 'NONE',  ( -0.6364829396325453192, -0.2845877964562159024, 0.3641732283464567677 ) ) ;
#68808=CARTESIAN_POINT ( 'NONE',  ( -0.9055118110236215490, 0.2952755905511811885, 0.000000000000000000 ) ) ;
#68809=CARTESIAN_POINT ( 'NONE',  ( 0.4790026246719167324, -0.05778040916215522460, 0.4822834645669289988 ) ) ;
#68812=CARTESIAN_POINT ( 'NONE',  ( 1.062992125984252745, 0.2952755905511811885, 0.000000000000000000 ) ) ;
#68813=CARTESIAN_POINT ( 'NONE',  ( -1.594488188976377119, 0.1660481256975883668, -0.3530559997133364547 ) ) ;
#68814=CARTESIAN_POINT ( 'NONE',  ( 1.332020997375328974, -0.05778040916215560624, -0.4822834645669293319 ) ) ;
#68818=CARTESIAN_POINT ( 'NONE',  ( 1.082677165354331228, -0.5400638737290844871, 0.3530559997133364547 ) ) ;
#68819=EDGE_CURVE ( 'NONE', #70238, #23460, #51667, .T. ) ;
#68820=CARTESIAN_POINT ( 'NONE',  ( 0.6299212598425204535, -0.1870078740157479769, 0.4822834645669291653 ) ) ;
#68821=CARTESIAN_POINT ( 'NONE',  ( 1.430446194225722500, -0.004921259842519576551, 0.3153832671262227771 ) ) ;
#68822=CARTESIAN_POINT ( 'NONE',  ( -1.581364829396324945, -0.08942795157528024563, -0.3641732283464568787 ) ) ;
#68823=CARTESIAN_POINT ( 'NONE',  ( -1.568241469816272105, -0.3162353388693409650, -0.4822834645669289433 ) ) ;
#68825=CARTESIAN_POINT ( 'NONE',  ( 0.9251968503937015864, 0.1660481256975883668, -0.3530559997133364547 ) ) ;
#68826=DIRECTION ( 'NONE',  ( 0.000000000000000000, -1.000000000000000000, 0.000000000000000000 ) ) ;
#68827=CARTESIAN_POINT ( 'NONE',  ( -0.3412073490813641308, -0.6046776061558807314, 0.2411417322834647770 ) ) ;
#68828=CARTESIAN_POINT ( 'NONE',  ( -0.3674540682414692561, -0.6046776061558809534, -0.2411417322834644161 ) ) ;
#68829=CARTESIAN_POINT ( 'NONE',  ( 1.515748031496063186, -0.5400638737290845981, -0.3530559997133363437 ) ) ;
#68834=CARTESIAN_POINT ( 'NONE',  ( 1.666666666666667185, 0.05413385826771666132, 0.4176697321401328100 ) ) ;
#68837=VERTEX_POINT ( 'NONE', #11879 ) ;
#68839=CARTESIAN_POINT ( 'NONE',  ( 1.253280839895013710, -0.2845877964562159024, 0.3641732283464567677 ) ) ;
#68841=CARTESIAN_POINT ( 'NONE',  ( 0.5636006452641431075, 3.421639014772782816E-16, 0.3464511005275203726 ) ) ;
#68842=CARTESIAN_POINT ( 'NONE',  ( 0.4847769261806178509, 1.968503937007873850, 0.4915354330708653907 ) ) ;
#68846=CARTESIAN_POINT ( 'NONE',  ( -0.6496062992125976043, 0.07958543189024071263, -0.2665933059059888421 ) ) ;
#68847=CARTESIAN_POINT ( 'NONE',  ( -1.076115485564303809, 0.1283753931104748280, 0.1820866141732283561 ) ) ;
#68848=CARTESIAN_POINT ( 'NONE',  ( 0.7152230971128614723, -0.3162353388693409650, -0.4822834645669289433 ) ) ;
#68849=CARTESIAN_POINT ( 'NONE',  ( -1.200787401574802349, -0.5400638737290844871, 0.3530559997133364547 ) ) ;
#68852=CARTESIAN_POINT ( 'NONE',  ( 1.535433070866142335, -0.6692913385826771977, 8.415575281601705876E-17 ) ) ;
#68855=CARTESIAN_POINT ( 'NONE',  ( -1.586052503253847057, 1.574803149606300412, 0.1653254495020574921 ) ) ;
#68857=CARTESIAN_POINT ( 'NONE',  ( -0.7086614173228339419, -0.1870078740157479769, 0.4822834645669291653 ) ) ;
#68858=CARTESIAN_POINT ( 'NONE',  ( 1.227034120734908917, 0.2952755905511810774, -0.1292274648535930714 ) ) ;
#68859=FACE_OUTER_BOUND ( 'NONE', #73273, .T. ) ;
#68861=CARTESIAN_POINT ( 'NONE',  ( -1.640419947506561060, -0.4281496062992127816, -0.4176697321401328100 ) ) ;
#68862=CARTESIAN_POINT ( 'NONE',  ( -1.325459317585300889, -0.4281496062992127816, -0.4176697321401328100 ) ) ;
#68864=CARTESIAN_POINT ( 'NONE',  ( 0.01968503937007930540, 0.07958543189024085140, 0.2665933059059887866 ) ) ;
#68866=CARTESIAN_POINT ( 'NONE',  ( -0.08530183727034056085, -0.2845877964562159024, 0.3641732283464567677 ) ) ;
#68867=CARTESIAN_POINT ( 'NONE',  ( 0.4265091863517067039, -0.5511811023622048555, -0.09757992244046775898 ) ) ;
#68868=CARTESIAN_POINT ( 'NONE',  ( 0.3871391076115492380, -0.05778040916215560624, -0.4822834645669293319 ) ) ;
#68870=CARTESIAN_POINT ( 'NONE',  ( -0.5905511811023613777, -0.5511811023622047445, 6.969142054262312111E-17 ) ) ;
#68872=CARTESIAN_POINT ( 'NONE',  ( 1.581364829396326277, -0.05778040916215522460, 0.4822834645669289988 ) ) ;
#68873=CARTESIAN_POINT ( 'NONE',  ( -0.8202099737532799750, 0.2952755905511810774, -0.1292274648535930714 ) ) ;
#68875=CARTESIAN_POINT ( 'NONE',  ( -0.1443569553805768291, 0.05413385826771666132, 0.4176697321401328100 ) ) ;
#68876=CARTESIAN_POINT ( 'NONE',  ( -0.7020997375328074108, -0.05778040916215522460, 0.4822834645669289988 ) ) ;
#68877=CARTESIAN_POINT ( 'NONE',  ( 1.161417322834646493, -0.4536011799217367080, 0.2665933059059888421 ) ) ;
#68878=CARTESIAN_POINT ( 'NONE',  ( 0.03280839895013198948, 0.1771653543307087630, 0.09757992244046791164 ) ) ;
#68879=CARTESIAN_POINT ( 'NONE',  ( -0.3083989501312330295, -0.05778040916215522460, 0.4822834645669289988 ) ) ;
#68880=CARTESIAN_POINT ( 'NONE',  ( -0.9514435695538050464, -0.05778040916215560624, -0.4822834645669293319 ) ) ;
#68881=CARTESIAN_POINT ( 'NONE',  ( 1.614173228346457378, 0.7166040191147859950, -0.1372047244094476148 ) ) ;
#68883=CARTESIAN_POINT ( 'NONE',  ( -0.4724409448818890911, -0.1870078740157480879, -0.4822834645669291653 ) ) ;
#68886=CARTESIAN_POINT ( 'NONE',  ( 1.043307086614173818, -0.5400638737290845981, -0.3530559997133363437 ) ) ;
#68887=CARTESIAN_POINT ( 'NONE',  ( -0.8464566929133852113, -0.4536011799217368745, -0.2665933059059886201 ) ) ;
#68888=CARTESIAN_POINT ( 'NONE',  ( -0.5905511811023615998, 0.2952755905511811885, 0.000000000000000000 ) ) ;
#68889=CARTESIAN_POINT ( 'NONE',  ( 1.082677165354331228, 0.1660481256975883668, -0.3530559997133364547 ) ) ;
#68890=CARTESIAN_POINT ( 'NONE',  ( 0.7677165354330716118, 0.1660481256975883668, -0.3530559997133364547 ) ) ;
#68891=CARTESIAN_POINT ( 'NONE',  ( -1.489501312335957062, -0.05778040916215522460, 0.4822834645669289988 ) ) ;
#68892=CARTESIAN_POINT ( 'NONE',  ( -1.003937007874015297, -0.4536011799217368745, -0.2665933059059886201 ) ) ;
#68896=CARTESIAN_POINT ( 'NONE',  ( 1.568241469816273659, -0.08942795157528024563, -0.3641732283464568787 ) ) ;
#68897=CARTESIAN_POINT ( 'NONE',  ( 0.8070866141732288002, 0.07958543189024085140, 0.2665933059059887866 ) ) ;
#68898=CARTESIAN_POINT ( 'NONE',  ( 0.3543307086614179147, 0.2952755905511811885, 0.000000000000000000 ) ) ;
#68899=CARTESIAN_POINT ( 'NONE',  ( -1.614173228346456712, 2.094556775020298467, -0.1372047244094478091 ) ) ;
#68901=CARTESIAN_POINT ( 'NONE',  ( 0.6167979002624679463, -0.004921259842519870586, -0.3153832671262229437 ) ) ;
#68903=CARTESIAN_POINT ( 'NONE',  ( -0.5183727034120726440, 0.2952755905511811885, 0.1292274648535926551 ) ) ;
#68904=CARTESIAN_POINT ( 'NONE',  ( -0.8333333333333323711, 0.2952755905511811885, 0.1292274648535926551 ) ) ;
#68905=CARTESIAN_POINT ( 'NONE',  ( 1.128608923884515169, -0.6046776061558809534, -0.2411417322834644161 ) ) ;
#68908=CARTESIAN_POINT ( 'NONE',  ( -0.2690288713910754526, 0.1771653543307087075, -0.09757992244046823083 ) ) ;
#68914=CARTESIAN_POINT ( 'NONE',  ( -1.049868766404198794, 0.2306618581243847221, -0.2411417322834647770 ) ) ;
#68915=CARTESIAN_POINT ( 'NONE',  ( -0.1181102362204717315, -0.6692913385826771977, 8.415575281601705876E-17 ) ) ;
#68916=CARTESIAN_POINT ( 'NONE',  ( -0.2427821522309703550, -0.3162353388693405765, 0.4822834645669290543 ) ) ;
#68917=CARTESIAN_POINT ( 'NONE',  ( 0.4199475065616805614, 0.2306618581243848609, 0.2411417322834645549 ) ) ;
#68918=CARTESIAN_POINT ( 'NONE',  ( -0.4330708661417315697, -0.6692913385826771977, 8.415575281601705876E-17 ) ) ;
#68919=CARTESIAN_POINT ( 'NONE',  ( -1.174540682414697335, -0.05778040916215522460, 0.4822834645669289988 ) ) ;
#68920=CARTESIAN_POINT ( 'NONE',  ( -0.9186351706036736120, 0.2306618581243848609, 0.2411417322834645549 ) ) ;
#68921=CARTESIAN_POINT ( 'NONE',  ( 0.8792650918635177559, -0.4281496062992127816, -0.4176697321401328100 ) ) ;
#68922=CARTESIAN_POINT ( 'NONE',  ( 0.5118110236220478892, 0.2952755905511811885, 0.000000000000000000 ) ) ;
#68924=CARTESIAN_POINT ( 'NONE',  ( -0.2493438320209966919, -0.3690944881889763329, 0.3153832671262228327 ) ) ;
#68927=ORIENTED_EDGE ( 'NONE', *, *, #60948, .T. ) ;
#68928=CARTESIAN_POINT ( 'NONE',  ( -1.371391076115484831, 0.1771653543307087075, -0.09757992244046823083 ) ) ;
#68929=CARTESIAN_POINT ( 'NONE',  ( -1.010498687664041384, 0.05413385826771666132, 0.4176697321401328100 ) ) ;
#68930=CARTESIAN_POINT ( 'NONE',  ( -0.7742782152230962556, -0.4281496062992127816, -0.4176697321401328100 ) ) ;
#68932=CARTESIAN_POINT ( 'NONE',  ( -0.4986876640419942164, -0.6046776061558807314, 0.2411417322834647770 ) ) ;
#68933=CARTESIAN_POINT ( 'NONE',  ( -0.7545931758530177724, 0.2952755905511811885, 0.1292274648535926551 ) ) ;
#68935=CARTESIAN_POINT ( 'NONE',  ( -1.640419947506561060, -0.4281496062992127816, -0.4176697321401328100 ) ) ;
#68936=CARTESIAN_POINT ( 'NONE',  ( 0.5052493438320218022, -0.5511811023622048555, -0.09757992244046775898 ) ) ;
#68939=CARTESIAN_POINT ( 'NONE',  ( -0.03937007874015669567, -0.5511811023622047445, 6.969142054262312111E-17 ) ) ;
#68940=CARTESIAN_POINT ( 'NONE',  ( -0.2624671916010490880, -0.6046776061558807314, 0.2411417322834647770 ) ) ;
#68941=LINE ( 'NONE', #72890, #16076 ) ;
#68942=CARTESIAN_POINT ( 'NONE',  ( -0.05249343832020911260, 0.2306618581243848609, 0.2411417322834645549 ) ) ;
#68945=CARTESIAN_POINT ( 'NONE',  ( -0.8333333333333321491, 0.2066929133858267931, 0.1054918080437490802 ) ) ;
#68949=CARTESIAN_POINT ( 'NONE',  ( -0.8333333333333323711, -0.5511811023622048555, -0.09757992244046775898 ) ) ;
#68950=CARTESIAN_POINT ( 'NONE',  ( -0.8661417322834640276, -0.1870078740157480879, -0.4822834645669291653 ) ) ;
#68954=CARTESIAN_POINT ( 'NONE',  ( 1.253280839895013710, -0.05778040916215560624, -0.4822834645669293319 ) ) ;
#68955=CARTESIAN_POINT ( 'NONE',  ( 0.5183727034120741983, 0.2952755905511810774, -0.1292274648535930714 ) ) ;
#68956=CARTESIAN_POINT ( 'NONE',  ( 0.3937007874015754361, -0.1870078740157479769, 0.4822834645669291653 ) ) ;
#68957=CARTESIAN_POINT ( 'NONE',  ( -0.9711286089238838626, 0.1283753931104746893, -0.1820866141732285504 ) ) ;
#68958=CARTESIAN_POINT ( 'NONE',  ( -0.3083989501312330295, -0.05778040916215522460, 0.4822834645669289988 ) ) ;
#68960=CARTESIAN_POINT ( 'NONE',  ( -0.8202099737532801971, -0.6692913385826771977, 0.1292274648535927661 ) ) ;
#68962=CARTESIAN_POINT ( 'NONE',  ( 1.135170603674541256, 0.1771653543307087630, 0.09757992244046791164 ) ) ;
#68963=CARTESIAN_POINT ( 'NONE',  ( -0.4921259842519677963, -0.4536011799217367080, 0.2665933059059888421 ) ) ;
#68965=CARTESIAN_POINT ( 'NONE',  ( 1.364829396325460076, 0.1283753931104748280, 0.1820866141732283561 ) ) ;
#68966=CARTESIAN_POINT ( 'NONE',  ( 1.601049868766404982, 0.1283753931104748280, 0.1820866141732283561 ) ) ;
#68967=CARTESIAN_POINT ( 'NONE',  ( -1.017060367454067249, -0.08942795157527998196, 0.3641732283464567121 ) ) ;
#68968=LINE ( 'NONE', #16818, #68174 ) ;
#68969=CARTESIAN_POINT ( 'NONE',  ( 0.4986876640419954376, -0.5023911411419708095, -0.1820866141732282451 ) ) ;
#68970=CARTESIAN_POINT ( 'NONE',  ( -0.4658792650918627265, -0.3162353388693409650, -0.4822834645669289433 ) ) ;
#68971=CARTESIAN_POINT ( 'NONE',  ( -2.787279214012418738, 2.401574803149606474, 0.000000000000000000 ) ) ;
#68972=CARTESIAN_POINT ( 'NONE',  ( -0.2034120734908128059, 0.1771653543307087630, 0.09757992244046791164 ) ) ;
#68974=CARTESIAN_POINT ( 'NONE',  ( 0.8464566929133866546, -0.5400638737290844871, 0.3530559997133364547 ) ) ;
#68978=CARTESIAN_POINT ( 'NONE',  ( 1.279527559055118724, 0.07958543189024085140, 0.2665933059059887866 ) ) ;
#68979=CARTESIAN_POINT ( 'NONE',  ( -1.049868766404198794, 0.2306618581243847221, -0.2411417322834647770 ) ) ;
#68980=CARTESIAN_POINT ( 'NONE',  ( -0.3740157480314953431, 0.07958543189024085140, 0.2665933059059887866 ) ) ;
#68982=CARTESIAN_POINT ( 'NONE',  ( 0.1574803149606306130, -0.1870078740157479769, 0.3641732283464567677 ) ) ;
#68983=CARTESIAN_POINT ( 'NONE',  ( -0.4593175853018364174, -0.4281496062992127816, -0.4176697321401328100 ) ) ;
#68986=CARTESIAN_POINT ( 'NONE',  ( 0.7611548556430451917, -0.5023911411419708095, 0.1820866141732285504 ) ) ;
#68987=CARTESIAN_POINT ( 'NONE',  ( -0.3937007874015740483, -0.1870078740157479769, 0.4822834645669291653 ) ) ;
#68988=CARTESIAN_POINT ( 'NONE',  ( -0.6496062992125976043, 0.1660481256975883668, -0.3530559997133364547 ) ) ;
#68989=CARTESIAN_POINT ( 'NONE',  ( -0.9448818897637790704, -0.1870078740157480601, -0.3641732283464567677 ) ) ;
#68991=CARTESIAN_POINT ( 'NONE',  ( -0.1509186351706028884, -0.3162353388693409650, -0.4822834645669289433 ) ) ;
#68992=CARTESIAN_POINT ( 'NONE',  ( -1.095800524934382292, -0.08942795157527998196, 0.3641732283464567121 ) ) ;
#68993=CARTESIAN_POINT ( 'NONE',  ( -1.377952755905511140, -0.6692913385826771977, 8.415575281601705876E-17 ) ) ;
#68996=CARTESIAN_POINT ( 'NONE',  ( -1.463254593175852492, -0.5511811023622048555, -0.09757992244046775898 ) ) ;
#68997=CARTESIAN_POINT ( 'NONE',  ( -1.555118110236219930, 0.1660481256975885056, 0.3530559997133364547 ) ) ;
#68998=CARTESIAN_POINT ( 'NONE',  ( -0.9120734908136475250, 0.2952755905511811885, 0.1292274648535926551 ) ) ;
#69000=CARTESIAN_POINT ( 'NONE',  ( -1.620734908136482577, 0.2952755905511811885, 0.1292274648535926551 ) ) ;
#69003=CARTESIAN_POINT ( 'NONE',  ( 1.108923884514436686, -0.3162353388693409650, -0.4822834645669289433 ) ) ;
#69004=CARTESIAN_POINT ( 'NONE',  ( 0.5774278215223104249, 0.2306618581243848609, 0.2411417322834645549 ) ) ;
#69007=CARTESIAN_POINT ( 'NONE',  ( 1.135170603674541256, 0.1771653543307087630, 0.09757992244046791164 ) ) ;
#69010=CARTESIAN_POINT ( 'NONE',  ( -0.7611548556430438595, -0.5023911411419708095, -0.1820866141732282451 ) ) ;
#69013=CARTESIAN_POINT ( 'NONE',  ( 0.5511811023622054106, -0.1870078740157480879, -0.4822834645669291653 ) ) ;
#69014=CARTESIAN_POINT ( 'NONE',  ( -0.3346456692913377662, -0.5400638737290844871, 0.3530559997133364547 ) ) ;
#69015=CARTESIAN_POINT ( 'NONE',  ( -1.102362204724408601, -0.1870078740157480879, -0.4822834645669291653 ) ) ;
#69016=CARTESIAN_POINT ( 'NONE',  ( 0.9776902887139113929, -0.6692913385826773087, -0.1292274648535924053 ) ) ;
#69018=CARTESIAN_POINT ( 'NONE',  ( -1.607611548556429737, 0.1771653543307087075, -0.09757992244046823083 ) ) ;
#69020=CARTESIAN_POINT ( 'NONE',  ( -0.1640419947506553400, -0.05778040916215560624, -0.4822834645669293319 ) ) ;
#69021=CARTESIAN_POINT ( 'NONE',  ( -1.253280839895012377, -0.3162353388693409650, -0.4822834645669289433 ) ) ;
#69022=CARTESIAN_POINT ( 'NONE',  ( -1.561679790026246017, -0.4281496062992127816, -0.4176697321401328100 ) ) ;
#69025=CARTESIAN_POINT ( 'NONE',  ( 0.9842519685039378130, -0.5511811023622047445, 6.969142054262312111E-17 ) ) ;
#69026=ORIENTED_EDGE ( 'NONE', *, *, #66425, .T. ) ;
#69028=CARTESIAN_POINT ( 'NONE',  ( -0.7874015748031489847, -0.1870078740157480879, -0.4822834645669291653 ) ) ;
#69030=CARTESIAN_POINT ( 'NONE',  ( -0.01312335958005186876, -0.3690944881889763329, 0.3153832671262228327 ) ) ;
#69032=CARTESIAN_POINT ( 'NONE',  ( 0.5905511811023629321, -0.6692913385826771977, 8.415575281601705876E-17 ) ) ;
#69033=CARTESIAN_POINT ( 'NONE',  ( 0.4002624671916016896, -0.3162353388693409650, -0.4822834645669289433 ) ) ;
#69034=CARTESIAN_POINT ( 'NONE',  ( -0.4002624671916004129, -0.05778040916215560624, -0.4822834645669293319 ) ) ;
#69035=AXIS2_PLACEMENT_3D ( 'NONE', #12810, #30911, #11985 ) ;
#69037=CARTESIAN_POINT ( 'NONE',  ( -1.364829396325458521, -0.6046776061558807314, 0.2411417322834647770 ) ) ;
#69039=CARTESIAN_POINT ( 'NONE',  ( 1.351706036745407458, -0.3690944881889765550, -0.3153832671262227771 ) ) ;
#69040=CARTESIAN_POINT ( 'NONE',  ( -1.207349081364828436, -0.6046776061558807314, 0.2411417322834647770 ) ) ;
#69041=CARTESIAN_POINT ( 'NONE',  ( 0.7217847769028878924, 0.05413385826771666132, 0.4176697321401328100 ) ) ;
#69042=CARTESIAN_POINT ( 'NONE',  ( 1.108923884514436686, -0.3162353388693409650, -0.4822834645669289433 ) ) ;
#69043=EDGE_CURVE ( 'NONE', #78537, #40878, #62735, .T. ) ;
#69045=CARTESIAN_POINT ( 'NONE',  ( -1.213910761154854745, 0.2952755905511810774, -0.1292274648535930714 ) ) ;
#69047=CARTESIAN_POINT ( 'NONE',  ( 0.2559055118110243332, -0.5400638737290845981, -0.3530559997133363437 ) ) ;
#69050=CARTESIAN_POINT ( 'NONE',  ( -1.397637795275589623, -0.4536011799217368745, -0.2665933059059886201 ) ) ;
#69051=CARTESIAN_POINT ( 'NONE',  ( 0.4658792650918641698, -0.08942795157528024563, -0.3641732283464568787 ) ) ;
#69052=CARTESIAN_POINT ( 'NONE',  ( 1.017060367454068581, -0.05778040916215560624, -0.4822834645669293319 ) ) ;
#69054=CARTESIAN_POINT ( 'NONE',  ( 0.8005249343832028242, -0.3690944881889765550, -0.3153832671262227771 ) ) ;
#69055=CARTESIAN_POINT ( 'NONE',  ( 0.3871391076115492380, -0.05778040916215560624, -0.4822834645669293319 ) ) ;
#69057=CARTESIAN_POINT ( 'NONE',  ( -0.7349081364829390672, 0.2306618581243847221, -0.2411417322834647770 ) ) ;
#69060=CARTESIAN_POINT ( 'NONE',  ( 1.108923884514436242, -0.08942795157527998196, 0.3641732283464567121 ) ) ;
#69061=CARTESIAN_POINT ( 'NONE',  ( 0.01968503937007930540, 0.1660481256975885056, 0.3530559997133364547 ) ) ;
#69062=CARTESIAN_POINT ( 'NONE',  ( 0.1181102362204730916, 0.2066929133858268208, 0.000000000000000000 ) ) ;
#69063=CARTESIAN_POINT ( 'NONE',  ( -0.1246719160104980823, 0.2952755905511811885, 0.1292274648535926551 ) ) ;
#69064=CARTESIAN_POINT ( 'NONE',  ( -0.06561679790026180015, -0.004921259842519576551, 0.3153832671262227771 ) ) ;
#69066=CARTESIAN_POINT ( 'NONE',  ( -0.5052493438320203589, -0.6692913385826771977, 0.1292274648535927661 ) ) ;
#69067=CARTESIAN_POINT ( 'NONE',  ( 0.7480314960629927956, -0.5511811023622047445, 6.969142054262312111E-17 ) ) ;
#69070=CARTESIAN_POINT ( 'NONE',  ( 0.4921259842519691285, -0.5400638737290845981, -0.3530559997133363437 ) ) ;
#69073=CARTESIAN_POINT ( 'NONE',  ( 1.246719160104987623, -0.004921259842519870586, -0.3153832671262229437 ) ) ;
#69074=CARTESIAN_POINT ( 'NONE',  ( -0.1698998578625667832, -2.609869883881465018E-15, -0.3464511005275220379 ) ) ;
#69075=CARTESIAN_POINT ( 'NONE',  ( -0.2165354330708654795, -0.4536011799217368745, -0.2665933059059886201 ) ) ;
#69076=CARTESIAN_POINT ( 'NONE',  ( -0.9120734908136475250, 0.1771653543307087630, 0.09757992244046791164 ) ) ;
#69077=CARTESIAN_POINT ( 'NONE',  ( -0.1246719160104980823, -0.6692913385826773087, -0.1292274648535924053 ) ) ;
#69078=CARTESIAN_POINT ( 'NONE',  ( 1.036745406824147731, -0.004921259842519576551, 0.3153832671262227771 ) ) ;
#69080=CARTESIAN_POINT ( 'NONE',  ( -1.660104986876639543, -0.05778040916215560624, -0.4822834645669293319 ) ) ;
#69082=CARTESIAN_POINT ( 'NONE',  ( 0.03937007874015833325, -0.6692913385826771977, 8.415575281601705876E-17 ) ) ;
#69084=CARTESIAN_POINT ( 'NONE',  ( 0.5577427821522316087, -0.05778040916215522460, 0.4822834645669289988 ) ) ;
#69086=CARTESIAN_POINT ( 'NONE',  ( 0.2755905511811031494, -0.6692913385826771977, 8.415575281601705876E-17 ) ) ;
#69088=CARTESIAN_POINT ( 'NONE',  ( 0.6824146981627303710, -0.6046776061558807314, 0.2411417322834647770 ) ) ;
#69089=CARTESIAN_POINT ( 'NONE',  ( 0.6824146981627303710, -0.6046776061558807314, 0.2411417322834647770 ) ) ;
#69091=CARTESIAN_POINT ( 'NONE',  ( 0.2821522309711292364, 0.1771653543307087075, -0.09757992244046823083 ) ) ;
#69092=CARTESIAN_POINT ( 'NONE',  ( 1.200787401574803681, 0.1660481256975885056, 0.3530559997133364547 ) ) ;
#69093=CARTESIAN_POINT ( 'NONE',  ( 0.006561679790026889343, -0.08942795157527998196, 0.3641732283464567121 ) ) ;
#69094=CARTESIAN_POINT ( 'NONE',  ( -0.1509186351706028884, -0.3162353388693409650, -0.4822834645669289433 ) ) ;
#69095=CARTESIAN_POINT ( 'NONE',  ( 0.3018372703412079971, -0.4281496062992124485, 0.4176697321401328655 ) ) ;
#69096=CARTESIAN_POINT ( 'NONE',  ( -0.7808398950131222316, -0.3162353388693409650, -0.4822834645669289433 ) ) ;
#69097=CARTESIAN_POINT ( 'NONE',  ( -0.4658792650918627265, -0.08942795157527998196, 0.3641732283464567121 ) ) ;
#69098=CARTESIAN_POINT ( 'NONE',  ( 1.010498687664042716, 0.05413385826771626580, -0.4176697321401330321 ) ) ;
#69099=CARTESIAN_POINT ( 'NONE',  ( 1.135170603674541256, -0.5511811023622048555, -0.09757992244046775898 ) ) ;
#69100=CARTESIAN_POINT ( 'NONE',  ( 0.2034120734908144990, -0.6692913385826771977, 0.1292274648535927661 ) ) ;
#69104=CARTESIAN_POINT ( 'NONE',  ( 1.614173228346457378, -0.6692913385826771977, 8.415575281601705876E-17 ) ) ;
#69106=CARTESIAN_POINT ( 'NONE',  ( -1.240157480314959759, -0.5400638737290845981, -0.3530559997133363437 ) ) ;
#69107=CARTESIAN_POINT ( 'NONE',  ( -0.8595800524934373854, -0.3162353388693409650, -0.4822834645669289433 ) ) ;
#69111=CARTESIAN_POINT ( 'NONE',  ( 0.5118110236220480003, -0.5511811023622047445, 6.969142054262312111E-17 ) ) ;
#69113=CARTESIAN_POINT ( 'NONE',  ( 0.4855643044619428750, 0.05413385826771666132, 0.4176697321401328100 ) ) ;
#69115=CARTESIAN_POINT ( 'NONE',  ( 0.9564677561141817774, 0.02791078216816225699, 0.4328096321851905293 ) ) ;
#69117=CARTESIAN_POINT ( 'NONE',  ( 1.181102362204725198, -0.1870078740157479769, 0.4822834645669291653 ) ) ;
#69118=CARTESIAN_POINT ( 'NONE',  ( 1.200787401574803681, -0.4536011799217368745, -0.2665933059059886201 ) ) ;
#69119=CARTESIAN_POINT ( 'NONE',  ( -0.09186351706036663400, -0.4281496062992124485, 0.4176697321401328655 ) ) ;
#69121=CARTESIAN_POINT ( 'NONE',  ( -0.4658792650918627265, -0.3162353388693409650, -0.4822834645669289433 ) ) ;
#69122=CARTESIAN_POINT ( 'NONE',  ( -0.7939632545931754048, -0.2845877964562159024, 0.3641732283464567677 ) ) ;
#69123=CARTESIAN_POINT ( 'NONE',  ( 0.2755905511811031494, -0.6692913385826771977, 8.415575281601705876E-17 ) ) ;
#69124=CARTESIAN_POINT ( 'NONE',  ( -0.2821522309711278487, 0.2952755905511811885, 0.1292274648535926551 ) ) ;
#69125=CARTESIAN_POINT ( 'NONE',  ( 1.614173228346457378, -0.6692913385826771977, 8.415575281601705876E-17 ) ) ;
#69127=EDGE_LOOP ( 'NONE', ( #30981, #81068, #11652, #16578 ) ) ;
#69129=CARTESIAN_POINT ( 'NONE',  ( 0.5183727034120741983, -0.6692913385826771977, 0.1292274648535927661 ) ) ;
#69130=CARTESIAN_POINT ( 'NONE',  ( -0.3280839895013117347, -0.4281496062992124485, 0.4176697321401328655 ) ) ;
#69131=CARTESIAN_POINT ( 'NONE',  ( -1.633858267716534529, 0.1660481256975885056, 0.3530559997133364547 ) ) ;
#69132=CARTESIAN_POINT ( 'NONE',  ( 0.7611548556430451917, -0.6046776061558807314, 0.2411417322834647770 ) ) ;
#69133=CARTESIAN_POINT ( 'NONE',  ( 0.5643044619422579178, 0.05413385826771666132, 0.4176697321401328100 ) ) ;
#69135=CARTESIAN_POINT ( 'NONE',  ( -0.6889763779527552368, -0.5400638737290845981, -0.3530559997133363437 ) ) ;
#69136=CARTESIAN_POINT ( 'NONE',  ( 0.1574803149606306130, -0.1870078740157480879, -0.4822834645669291653 ) ) ;
#69137=CARTESIAN_POINT ( 'NONE',  ( -0.2755905511811015396, -0.6692913385826771977, 8.415575281601705876E-17 ) ) ;
#69139=CARTESIAN_POINT ( 'NONE',  ( 0.3740157480314966754, -0.4536011799217367080, 0.2665933059059888421 ) ) ;
#69140=CARTESIAN_POINT ( 'NONE',  ( -1.719160104986876103, 0.05413385826771666132, 0.4176697321401328100 ) ) ;
#69142=ADVANCED_FACE ( 'NONE', ( #57704 ), #67, .F. ) ;
#69143=CARTESIAN_POINT ( 'NONE',  ( -0.1771653543307080136, -0.5400638737290844871, 0.3530559997133364547 ) ) ;
#69145=CARTESIAN_POINT ( 'NONE',  ( 1.469816272965879911, 0.2306618581243847221, -0.2411417322834647770 ) ) ;
#69148=ORIENTED_EDGE ( 'NONE', *, *, #12912, .T. ) ;
#69149=CARTESIAN_POINT ( 'NONE',  ( 0.8267716535433078384, -0.6692913385826771977, 8.415575281601705876E-17 ) ) ;
#69150=CARTESIAN_POINT ( 'NONE',  ( -0.05249343832020938322, -0.5023911411419708095, -0.1820866141732282451 ) ) ;
#69152=CARTESIAN_POINT ( 'NONE',  ( -1.614173228346457378, 1.606230626554505658, 0.1372047244094476981 ) ) ;
#69157=CARTESIAN_POINT ( 'NONE',  ( 0.3346456692913390985, 0.1660481256975885056, 0.3530559997133364547 ) ) ;
#69158=CARTESIAN_POINT ( 'NONE',  ( -1.318897637795274802, 0.1660481256975885056, 0.3530559997133364547 ) ) ;
#69159=CARTESIAN_POINT ( 'NONE',  ( -1.233595800524933894, 0.2306618581243848609, 0.2411417322834645549 ) ) ;
#69160=CARTESIAN_POINT ( 'NONE',  ( 0.3674540682414705883, 0.2306618581243847221, -0.2411417322834647770 ) ) ;
#69161=CARTESIAN_POINT ( 'NONE',  ( 1.128608923884514947, 0.2306618581243848609, 0.2411417322834645549 ) ) ;
#69162=CARTESIAN_POINT ( 'NONE',  ( 1.463254593175853824, -0.5511811023622046335, 0.09757992244046803654 ) ) ;
#69163=CARTESIAN_POINT ( 'NONE',  ( 1.345144356955381593, -0.08942795157527998196, 0.3641732283464567121 ) ) ;
#69164=CARTESIAN_POINT ( 'NONE',  ( -1.010498687664041384, 0.05413385826771666132, 0.4176697321401328100 ) ) ;
#69166=CARTESIAN_POINT ( 'NONE',  ( 1.607611548556431069, -0.6692913385826773087, -0.1292274648535924053 ) ) ;
#69168=CARTESIAN_POINT ( 'NONE',  ( -0.1377952755905504645, -0.5400638737290845981, -0.3530559997133363437 ) ) ;
#69169=CARTESIAN_POINT ( 'NONE',  ( 1.095800524934383846, -0.05778040916215560624, -0.4822834645669293319 ) ) ;
#69171=CARTESIAN_POINT ( 'NONE',  ( -1.391076115485563758, 0.1283753931104748280, 0.1820866141732283561 ) ) ;
#69172=CARTESIAN_POINT ( 'NONE',  ( 0.2952755905511819101, 0.1660481256975883668, -0.3530559997133364547 ) ) ;
#69173=CARTESIAN_POINT ( 'NONE',  ( 0.8005249343832027131, -0.004921259842519576551, 0.3153832671262227771 ) ) ;
#69174=CARTESIAN_POINT ( 'NONE',  ( -1.338582677165353729, -0.1870078740157480601, -0.3641732283464567677 ) ) ;
#69175=CARTESIAN_POINT ( 'NONE',  ( 1.128608923884515169, -0.6046776061558809534, -0.2411417322834644161 ) ) ;
#69176=CARTESIAN_POINT ( 'NONE',  ( -0.5411721830064186722, -2.191421614605370878E-15, 0.4445507791589071167 ) ) ;
#69177=CARTESIAN_POINT ( 'NONE',  ( -0.5839895013123351797, 0.1771653543307087075, -0.09757992244046823083 ) ) ;
#69178=CARTESIAN_POINT ( 'NONE',  ( -0.8070866141732276899, -0.5400638737290844871, 0.3530559997133364547 ) ) ;
#69179=CARTESIAN_POINT ( 'NONE',  ( 1.469816272965879911, -0.6046776061558807314, 0.2411417322834647770 ) ) ;
#69180=CARTESIAN_POINT ( 'NONE',  ( -0.7611548556430438595, 0.2306618581243848609, 0.2411417322834645549 ) ) ;
#69181=CARTESIAN_POINT ( 'NONE',  ( 1.561679790026247350, 0.05413385826771626580, -0.4176697321401330321 ) ) ;
#69183=CARTESIAN_POINT ( 'NONE',  ( -0.7480314960629914633, -0.5511811023622047445, 6.969142054262312111E-17 ) ) ;
#69185=B_SPLINE_CURVE_WITH_KNOTS ( 'NONE', 3,
 ( #18566, #49714, #5513, #44209 ),
 .UNSPECIFIED., .F., .F.,
 ( 4, 4 ),
 ( 3.210432057660995851E-07, 0.001287787053612100526 ),
 .UNSPECIFIED. ) ;
#69186=CARTESIAN_POINT ( 'NONE',  ( 1.266404199475066328, -0.05778040916215522460, 0.4822834645669289988 ) ) ;
#69188=CARTESIAN_POINT ( 'NONE',  ( -0.09023630363247998887, 1.809133623825372073E-16, -0.3791483426435173776 ) ) ;
#69189=CARTESIAN_POINT ( 'NONE',  ( 1.666666666666667185, 0.05413385826771666132, 0.4176697321401328100 ) ) ;
#69190=CARTESIAN_POINT ( 'NONE',  ( -1.161417322834644716, -0.4536011799217368745, -0.2665933059059886201 ) ) ;
#69193=CARTESIAN_POINT ( 'NONE',  ( 0.7998211177050879028, 0.000000000000000000, 0.3464511005275205946 ) ) ;
#69194=CARTESIAN_POINT ( 'NONE',  ( -0.4724409448818890911, -0.1870078740157480879, -0.4822834645669291653 ) ) ;
#69195=CARTESIAN_POINT ( 'NONE',  ( 0.1246719160104994284, 0.1771653543307087075, -0.09757992244046823083 ) ) ;
#69196=CARTESIAN_POINT ( 'NONE',  ( -0.9776902887139098386, -0.5511811023622046335, 0.09757992244046803654 ) ) ;
#69197=CARTESIAN_POINT ( 'NONE',  ( 1.410761154855643795, -0.2845877964562159024, 0.3641732283464567677 ) ) ;
#69198=CARTESIAN_POINT ( 'NONE',  ( 1.122047244094488860, -0.5400638737290845981, -0.3530559997133363437 ) ) ;
#69200=CARTESIAN_POINT ( 'NONE',  ( 0.4790026246719168435, -0.2845877964562161244, -0.3641732283464567121 ) ) ;
#69202=CARTESIAN_POINT ( 'NONE',  ( 0.4396325459317593221, 0.2952755905511810774, -0.1292274648535930714 ) ) ;
#69204=CARTESIAN_POINT ( 'NONE',  ( 0.8989501312335963501, -0.5511811023622048555, -0.09757992244046775898 ) ) ;
#69206=CARTESIAN_POINT ( 'NONE',  ( -1.240157480314959759, -0.5400638737290845981, -0.3530559997133363437 ) ) ;
#69207=CARTESIAN_POINT ( 'NONE',  ( -1.286089238845143479, 0.2306618581243847221, -0.2411417322834647770 ) ) ;
#69208=CARTESIAN_POINT ( 'NONE',  ( 5.463695987328526437E-16, -0.1870078740157479769, 0.4822834645669291653 ) ) ;
#69209=DIRECTION ( 'NONE',  ( -1.000000000000000000, 0.000000000000000000, 0.000000000000000000 ) ) ;
#69211=CARTESIAN_POINT ( 'NONE',  ( 0.5905511811023629321, -0.6692913385826771977, 8.415575281601705876E-17 ) ) ;
#69212=CARTESIAN_POINT ( 'NONE',  ( -1.627296587926508442, -0.6046776061558809534, -0.2411417322834644161 ) ) ;
#69213=CARTESIAN_POINT ( 'NONE',  ( -0.1574803149606292529, -0.1870078740157480879, -0.4822834645669291653 ) ) ;
#69214=CARTESIAN_POINT ( 'NONE',  ( 0.1837270341207354329, 0.2306618581243848609, 0.2411417322834645549 ) ) ;
#69219=DIRECTION ( 'NONE',  ( 3.096699300667737957E-16, -1.000000000000000000, 0.000000000000000000 ) ) ;
#69221=CARTESIAN_POINT ( 'NONE',  ( -0.3805774278215216522, -0.3690944881889765550, -0.3153832671262227771 ) ) ;
#69222=CARTESIAN_POINT ( 'NONE',  ( -0.5446194225721777693, -0.3162353388693409650, -0.4822834645669289433 ) ) ;
#69223=CARTESIAN_POINT ( 'NONE',  ( 0.3083989501312343062, -0.3162353388693405765, 0.4822834645669290543 ) ) ;
#69226=CARTESIAN_POINT ( 'NONE',  ( 0.7611548556430454138, 0.2306618581243847221, -0.2411417322834647770 ) ) ;
#69227=CARTESIAN_POINT ( 'NONE',  ( 1.515748031496063186, -0.5400638737290845981, -0.3530559997133363437 ) ) ;
#69228=CARTESIAN_POINT ( 'NONE',  ( 0.6889763779527563470, 0.1660481256975883668, -0.3530559997133364547 ) ) ;
#69231=CARTESIAN_POINT ( 'NONE',  ( 1.653543307086614789, -0.1870078740157479769, 0.4822834645669291653 ) ) ;
#69232=CARTESIAN_POINT ( 'NONE',  ( 0.7217847769028878924, -0.4281496062992127816, -0.4176697321401328100 ) ) ;
#69233=CARTESIAN_POINT ( 'NONE',  ( 0.4658792650918640033, -0.3162353388693405765, 0.4822834645669290543 ) ) ;
#69235=CARTESIAN_POINT ( 'NONE',  ( 1.108923884514436242, -0.08942795157527998196, 0.3641732283464567121 ) ) ;
#69236=CARTESIAN_POINT ( 'NONE',  ( -1.555118110236219930, -0.4536011799217368745, -0.2665933059059886201 ) ) ;
#69237=CARTESIAN_POINT ( 'NONE',  ( -1.496062992125983815, -0.1870078740157479769, 0.4822834645669291653 ) ) ;
#69239=CARTESIAN_POINT ( 'NONE',  ( -2.787279214012418738, 0.000000000000000000, 0.000000000000000000 ) ) ;
#69240=CARTESIAN_POINT ( 'NONE',  ( 0.8333333333333340365, -0.6692913385826771977, 0.1292274648535927661 ) ) ;
#69241=CARTESIAN_POINT ( 'NONE',  ( 1.463254593175853824, -0.5511811023622046335, 0.09757992244046803654 ) ) ;
#69242=CARTESIAN_POINT ( 'NONE',  ( -0.5839895013123351797, 0.2952755905511810774, -0.1292274648535930714 ) ) ;
#69243=CARTESIAN_POINT ( 'NONE',  ( -0.9317585301837263412, 0.05413385826771666132, 0.4176697321401328100 ) ) ;
#69244=CARTESIAN_POINT ( 'NONE',  ( 1.213910761154856299, -0.6692913385826773087, -0.1292274648535924053 ) ) ;
#69245=B_SPLINE_CURVE_WITH_KNOTS ( 'NONE', 3,
 ( #35216, #60879, #3230, #43984 ),
 .UNSPECIFIED., .F., .F.,
 ( 4, 4 ),
 ( 3.593986969204291827E-07, 0.001287825409103184960 ),
 .UNSPECIFIED. ) ;
#69249=EDGE_CURVE ( 'NONE', #4549, #9936, #45298, .T. ) ;
#69250=CARTESIAN_POINT ( 'NONE',  ( 1.640419947506562393, -0.4281496062992124485, 0.4176697321401328655 ) ) ;
#69253=ORIENTED_EDGE ( 'NONE', *, *, #64052, .T. ) ;
#69255=CARTESIAN_POINT ( 'NONE',  ( 1.456692913385827515, 0.1771653543307087630, 0.000000000000000000 ) ) ;
#69257=CARTESIAN_POINT ( 'NONE',  ( 1.692913385826772421, 0.1771653543307087630, 0.000000000000000000 ) ) ;
#69258=CARTESIAN_POINT ( 'NONE',  ( -0.1443569553805768291, 0.009842519685039463617, 0.3409548833797002576 ) ) ;
#69262=CARTESIAN_POINT ( 'NONE',  ( -0.9055118110236215490, -0.5511811023622047445, 6.969142054262312111E-17 ) ) ;
#69263=CARTESIAN_POINT ( 'NONE',  ( -1.213910761154854745, 0.1771653543307087075, -0.09757992244046823083 ) ) ;
#69264=CARTESIAN_POINT ( 'NONE',  ( -1.286089238845143479, 0.2306618581243847221, -0.2411417322834647770 ) ) ;
#69265=CARTESIAN_POINT ( 'NONE',  ( 0.2887139107611556010, -0.6046776061558807314, 0.2411417322834647770 ) ) ;
#69266=CARTESIAN_POINT ( 'NONE',  ( -1.397637795275589623, -0.5400638737290845981, -0.3530559997133363437 ) ) ;
#69267=ORIENTED_EDGE ( 'NONE', *, *, #9067, .F. ) ;
#69268=CARTESIAN_POINT ( 'NONE',  ( 1.574803149606299746, -0.1870078740157479769, 0.4822834645669291653 ) ) ;
#69269=CARTESIAN_POINT ( 'NONE',  ( -1.161417322834644716, 0.1012011053420777407, 0.2882089793578256898 ) ) ;
#69272=CARTESIAN_POINT ( 'NONE',  ( -0.6430446194225712953, -0.004921259842519870586, -0.3153832671262229437 ) ) ;
#69273=CARTESIAN_POINT ( 'NONE',  ( -1.056430446194224881, -0.6692913385826771977, 0.1292274648535927661 ) ) ;
#69274=CARTESIAN_POINT ( 'NONE',  ( 1.207349081364829990, 0.2306618581243848609, 0.2411417322834645549 ) ) ;
#69278=CARTESIAN_POINT ( 'NONE',  ( -1.603475055217291612, 1.606158680897942670, 0.04573490813648253134 ) ) ;
#69279=CARTESIAN_POINT ( 'NONE',  ( 1.568241469816273659, -0.05778040916215560624, -0.4822834645669293319 ) ) ;
#69280=CARTESIAN_POINT ( 'NONE',  ( -1.404199475065615932, 0.05413385826771666132, 0.4176697321401328100 ) ) ;
#69282=CARTESIAN_POINT ( 'NONE',  ( 0.1902887139107617975, 0.1771653543307087630, 0.09757992244046791164 ) ) ;
#69284=CARTESIAN_POINT ( 'NONE',  ( -0.2559055118110227234, -0.4536011799217367080, 0.2665933059059888421 ) ) ;
#69285=CARTESIAN_POINT ( 'NONE',  ( 0.3674540682414705883, 0.1283753931104746893, -0.1820866141732285504 ) ) ;
#69286=CARTESIAN_POINT ( 'NONE',  ( 0.7283464566929140904, -0.5400638737290845981, -0.3530559997133363437 ) ) ;
#69287=CARTESIAN_POINT ( 'NONE',  ( -0.6496062992125976043, 0.07958543189024071263, -0.2665933059059888421 ) ) ;
#69289=CARTESIAN_POINT ( 'NONE',  ( 1.095800524934383846, -0.3162353388693405765, 0.4822834645669290543 ) ) ;
#69290=CARTESIAN_POINT ( 'NONE',  ( -1.108923884514435132, -0.05778040916215560624, -0.4822834645669293319 ) ) ;
#69292=CARTESIAN_POINT ( 'NONE',  ( 0.2230971128608929543, 0.05413385826771626580, -0.4176697321401330321 ) ) ;
#69293=EDGE_CURVE ( 'NONE', #42318, #55143, #25587, .T. ) ;
#69294=CARTESIAN_POINT ( 'NONE',  ( -0.3215223097112853146, -0.05778040916215560624, -0.4822834645669293319 ) ) ;
#69295=CARTESIAN_POINT ( 'NONE',  ( 1.404199475065617708, -0.004921259842519870586, -0.3153832671262229437 ) ) ;
#69296=CARTESIAN_POINT ( 'NONE',  ( 0.2493438320209980519, -0.3690944881889765550, -0.3153832671262227771 ) ) ;
#69297=CARTESIAN_POINT ( 'NONE',  ( -0.1377952755905504645, 0.1660481256975885056, 0.3530559997133364547 ) ) ;
#69298=CARTESIAN_POINT ( 'NONE',  ( -1.128608923884513837, 0.2306618581243847221, -0.2411417322834647770 ) ) ;
#69300=CARTESIAN_POINT ( 'NONE',  ( 1.692913385826772421, 0.1771653543307087630, 0.000000000000000000 ) ) ;
#69301=CARTESIAN_POINT ( 'NONE',  ( -0.2230971128608915943, 0.05413385826771666132, 0.4176697321401328100 ) ) ;
#69302=CARTESIAN_POINT ( 'NONE',  ( -1.102362204724408601, -0.1870078740157479769, 0.4822834645669291653 ) ) ;
#69305=CARTESIAN_POINT ( 'NONE',  ( 0.9711286089238851948, 0.2306618581243848609, 0.2411417322834645549 ) ) ;
#69306=CARTESIAN_POINT ( 'NONE',  ( -0.5183727034120726440, -0.5511811023622048555, -0.09757992244046775898 ) ) ;
#69307=CARTESIAN_POINT ( 'NONE',  ( -0.5839895013123351797, 0.2952755905511810774, -0.1292274648535930714 ) ) ;
#69308=CARTESIAN_POINT ( 'NONE',  ( 1.286089238845145033, -0.6046776061558809534, -0.2411417322834644161 ) ) ;
#69309=CARTESIAN_POINT ( 'NONE',  ( 0.8530183727034128527, -0.4281496062992124485, 0.4176697321401328655 ) ) ;
#69311=CARTESIAN_POINT ( 'NONE',  ( -1.259842519685038686, -0.1870078740157479769, 0.3641732283464567677 ) ) ;
#69316=CARTESIAN_POINT ( 'NONE',  ( 1.286089238845145033, -0.5023911411419708095, -0.1820866141732282451 ) ) ;
#69317=CARTESIAN_POINT ( 'NONE',  ( 0.9120734908136489683, -0.5511811023622046335, 0.09757992244046803654 ) ) ;
#69318=CARTESIAN_POINT ( 'NONE',  ( 0.6824146981627303710, 0.2306618581243847221, -0.2411417322834647770 ) ) ;
#69321=CARTESIAN_POINT ( 'NONE',  ( 0.9514435695538062676, -0.2845877964562161244, -0.3641732283464567121 ) ) ;
#69322=( BOUNDED_CURVE ( )  B_SPLINE_CURVE ( 2, ( #63192, #37106, #13106, #11449, #44226, #45054, #70329, #81750, #51366, #18178, #64018, #62790, #37928 ),
 .UNSPECIFIED., .F., .F. ) 
 B_SPLINE_CURVE_WITH_KNOTS ( ( 3, 2, 2, 2, 2, 2, 3 ),
 ( 0.8217605387524145044, 0.8219696969696970168, 0.8257575757575758013, 0.8295454545454545858, 0.8333333333333333703, 0.8371212121212121549, 0.8373303703384946672 ),
 .UNSPECIFIED. ) 
 CURVE ( )  GEOMETRIC_REPRESENTATION_ITEM ( )  RATIONAL_B_SPLINE_CURVE ( ( 0.9964447847208419695, 0.9981185001348091834, 1.000000000000000000, 0.9659258262890683122, 1.000000000000000000, 0.9659258262890683122, 1.000000000000000000, 0.9659258262890683122, 1.000000000000000000, 0.9659258262890683122, 1.000000000000000000, 0.9981185001348091834, 0.9964447847208420805 ) ) 
 REPRESENTATION_ITEM ( '' )  );
#69323=CARTESIAN_POINT ( 'NONE',  ( -0.1509186351706028884, -0.3162353388693409650, -0.4822834645669289433 ) ) ;
#69324=CARTESIAN_POINT ( 'NONE',  ( -1.305774278215222184, 0.2952755905511811885, 0.1292274648535926551 ) ) ;
#69325=CARTESIAN_POINT ( 'NONE',  ( 1.082677165354331228, 0.1660481256975883668, -0.3530559997133364547 ) ) ;
#69329=CARTESIAN_POINT ( 'NONE',  ( 0.01968503937007930540, 0.07958543189024085140, 0.2665933059059887866 ) ) ;
#69330=ORIENTED_EDGE ( 'NONE', *, *, #29978, .F. ) ;
#69332=CARTESIAN_POINT ( 'NONE',  ( -0.9776902887139098386, -0.6692913385826771977, 0.1292274648535927661 ) ) ;
#69333=CARTESIAN_POINT ( 'NONE',  ( -0.5314960629921250401, 0.1660481256975885056, 0.3530559997133364547 ) ) ;
#69334=CARTESIAN_POINT ( 'NONE',  ( -0.3740157480314953431, 0.1660481256975885056, 0.3530559997133364547 ) ) ;
#69335=CARTESIAN_POINT ( 'NONE',  ( 0.4265091863517067594, 0.2952755905511811885, 0.1292274648535926551 ) ) ;
#69336=CARTESIAN_POINT ( 'NONE',  ( -0.5446194225721777693, -0.05778040916215522460, 0.4822834645669289988 ) ) ;
#69337=CARTESIAN_POINT ( 'NONE',  ( -1.502624671916009680, -0.3162353388693405765, 0.4822834645669290543 ) ) ;
#69338=CARTESIAN_POINT ( 'NONE',  ( -0.7742782152230965886, 0.05413385826771666132, 0.4176697321401328100 ) ) ;
#69339=CARTESIAN_POINT ( 'NONE',  ( 0.5643044619422579178, -0.4281496062992127816, -0.4176697321401328100 ) ) ;
#69341=CARTESIAN_POINT ( 'NONE',  ( -0.2362204724409440182, -0.1870078740157479769, 0.3641732283464567677 ) ) ;
#69345=CARTESIAN_POINT ( 'NONE',  ( -1.154855643044618851, -0.5023911411419708095, -0.1820866141732282451 ) ) ;
#69346=CARTESIAN_POINT ( 'NONE',  ( -0.9251968503937002541, -0.5400638737290845981, -0.3530559997133363437 ) ) ;
#69347=CARTESIAN_POINT ( 'NONE',  ( -0.8398950131233585692, 0.2306618581243848609, 0.2411417322834645549 ) ) ;
#69349=CARTESIAN_POINT ( 'NONE',  ( -0.7611548556430438595, 0.2306618581243848609, 0.2411417322834645549 ) ) ;
#69350=CARTESIAN_POINT ( 'NONE',  ( -0.9908136482939626788, -0.6692913385826773087, -0.1292274648535924053 ) ) ;
#69351=CARTESIAN_POINT ( 'NONE',  ( -1.541994750656167090, -0.6692913385826773087, -0.1292274648535924053 ) ) ;
#69353=CARTESIAN_POINT ( 'NONE',  ( 0.7020997375328090762, -0.2845877964562159024, 0.3641732283464567677 ) ) ;
#69356=CARTESIAN_POINT ( 'NONE',  ( 0.2230971128608929543, -0.004921259842519870586, -0.3153832671262229437 ) ) ;
#69357=CARTESIAN_POINT ( 'NONE',  ( -0.3149606299212590610, -0.1870078740157480879, -0.4822834645669291653 ) ) ;
#69358=CARTESIAN_POINT ( 'NONE',  ( 1.351706036745407458, -0.4281496062992127816, -0.4176697321401328100 ) ) ;
#69359=CARTESIAN_POINT ( 'NONE',  ( -0.006561679790025524116, -0.05778040916215560624, -0.4822834645669293319 ) ) ;
#69360=VERTEX_POINT ( 'NONE', #32460 ) ;
#69362=CARTESIAN_POINT ( 'NONE',  ( 0.2469196488504588338, 2.056812631849083806E-16, 0.4118484887281962381 ) ) ;
#69365=CARTESIAN_POINT ( 'NONE',  ( -0.1474713956048439301, -2.191421614605370878E-15, 0.4445507791589071167 ) ) ;
#69366=CARTESIAN_POINT ( 'NONE',  ( -1.181102362204723644, -0.1870078740157480601, -0.3641732283464567677 ) ) ;
#69367=CARTESIAN_POINT ( 'NONE',  ( -1.548556430446193399, 0.2306618581243848609, 0.2411417322834645549 ) ) ;
#69371=CARTESIAN_POINT ( 'NONE',  ( 1.476377952755906442, -0.5400638737290844871, 0.3530559997133364547 ) ) ;
#69373=CARTESIAN_POINT ( 'NONE',  ( 0.3149606299212603933, -0.1870078740157479769, 0.4822834645669291653 ) ) ;
#69374=CARTESIAN_POINT ( 'NONE',  ( 0.2821522309711292364, 0.2952755905511810774, -0.1292274648535930714 ) ) ;
#69375=CARTESIAN_POINT ( 'NONE',  ( -0.9514435695538050464, -0.08942795157528024563, -0.3641732283464568787 ) ) ;
#69376=CARTESIAN_POINT ( 'NONE',  ( -0.1509186351706028884, -0.05778040916215522460, 0.4822834645669289988 ) ) ;
#69378=CARTESIAN_POINT ( 'NONE',  ( -0.9908136482939626788, -0.6692913385826773087, -0.1292274648535924053 ) ) ;
#69380=CARTESIAN_POINT ( 'NONE',  ( 1.450131233595801428, 0.1771653543307087630, 0.09757992244046791164 ) ) ;
#69381=CARTESIAN_POINT ( 'NONE',  ( -0.2559055118110230564, 0.07958543189024071263, -0.2665933059059888421 ) ) ;
#69382=CARTESIAN_POINT ( 'NONE',  ( 1.174540682414699111, -0.2845877964562159024, 0.3641732283464567677 ) ) ;
#69383=CARTESIAN_POINT ( 'NONE',  ( -1.541994750656167090, 0.2952755905511811885, 0.1292274648535926551 ) ) ;
#69384=CARTESIAN_POINT ( 'NONE',  ( -1.187664041994749731, -0.2845877964562159024, 0.3641732283464567677 ) ) ;
#69385=CARTESIAN_POINT ( 'NONE',  ( 0.4687286201624460968, 1.750728371878951917, 0.5180200956804293932 ) ) ;
#69386=CARTESIAN_POINT ( 'NONE',  ( 0.6627296587926517768, -0.5511811023622048555, -0.09757992244046775898 ) ) ;
#69387=CARTESIAN_POINT ( 'NONE',  ( -0.9448818897637790704, -0.1870078740157480879, -0.4822834645669291653 ) ) ;
#69390=CARTESIAN_POINT ( 'NONE',  ( -0.07874015748031421014, -0.1870078740157479769, 0.3641732283464567677 ) ) ;
#69391=CARTESIAN_POINT ( 'NONE',  ( -1.476377952755905110, -0.4536011799217368745, -0.2665933059059886201 ) ) ;
#69393=CARTESIAN_POINT ( 'NONE',  ( 0.7086614173228353852, -0.1870078740157479769, 0.4822834645669291653 ) ) ;
#69394=CARTESIAN_POINT ( 'NONE',  ( 0.6430446194225728496, 0.05413385826771666132, 0.4176697321401328100 ) ) ;
#69395=CARTESIAN_POINT ( 'NONE',  ( 1.410761154855643795, -0.2845877964562159024, 0.3641732283464567677 ) ) ;
#69396=CARTESIAN_POINT ( 'NONE',  ( -0.8070866141732276899, -0.5400638737290844871, 0.3530559997133364547 ) ) ;
#69397=CARTESIAN_POINT ( 'NONE',  ( -0.2230971128608915943, -0.004921259842519576551, 0.3153832671262227771 ) ) ;
#69398=CARTESIAN_POINT ( 'NONE',  ( -0.7330015572057683171, 1.982446682556143980, 0.5178628694646268960 ) ) ;
#69399=CARTESIAN_POINT ( 'NONE',  ( 0.3543307086614179147, 0.1771653543307087630, 0.000000000000000000 ) ) ;
#69400=CARTESIAN_POINT ( 'NONE',  ( -1.102362204724408601, -0.1870078740157479769, 0.4822834645669291653 ) ) ;
#69401=CARTESIAN_POINT ( 'NONE',  ( -0.5643044619422565855, -0.4281496062992124485, 0.4176697321401328655 ) ) ;
#69404=CARTESIAN_POINT ( 'NONE',  ( 0.4593175853018379162, -0.3690944881889763329, 0.3153832671262228327 ) ) ;
#69405=CARTESIAN_POINT ( 'NONE',  ( -0.4790026246719152336, -0.05778040916215560624, -0.4822834645669293319 ) ) ;
#69406=CARTESIAN_POINT ( 'NONE',  ( -0.7414698162729651543, -0.6692913385826771977, 0.1292274648535927661 ) ) ;
#69407=CARTESIAN_POINT ( 'NONE',  ( -0.9908136482939626788, 0.1771653543307087630, 0.09757992244046791164 ) ) ;
#69409=CARTESIAN_POINT ( 'NONE',  ( 0.1312335958005257930, 0.2306618581243847221, -0.2411417322834647770 ) ) ;
#69410=CARTESIAN_POINT ( 'NONE',  ( -1.574803149606298636, -0.1870078740157479769, 0.3641732283464567677 ) ) ;
#69411=CARTESIAN_POINT ( 'NONE',  ( -1.555118110236219930, -0.5400638737290845981, -0.3530559997133363437 ) ) ;
#69415=CARTESIAN_POINT ( 'NONE',  ( -1.430446194225721390, -0.4281496062992124485, 0.4176697321401328655 ) ) ;
#69416=CARTESIAN_POINT ( 'NONE',  ( -0.9580052493438311334, -0.4281496062992124485, 0.4176697321401328655 ) ) ;
#69417=CARTESIAN_POINT ( 'NONE',  ( 1.541994750656168645, -0.6692913385826771977, 0.1292274648535927661 ) ) ;
#69420=CARTESIAN_POINT ( 'NONE',  ( 1.141732283464567788, -0.6692913385826771977, 8.415575281601705876E-17 ) ) ;
#69421=CARTESIAN_POINT ( 'NONE',  ( 0.5839895013123367340, 0.2952755905511811885, 0.1292274648535926551 ) ) ;
#69426=CARTESIAN_POINT ( 'NONE',  ( 1.187664041994751285, -0.2845877964562161244, -0.3641732283464567121 ) ) ;
#69431=CARTESIAN_POINT ( 'NONE',  ( 0.4855643044619428750, 0.05413385826771666132, 0.4176697321401328100 ) ) ;
#69432=CARTESIAN_POINT ( 'NONE',  ( -0.6299212598425188991, -0.1870078740157479769, 0.4822834645669291653 ) ) ;
#69433=CARTESIAN_POINT ( 'NONE',  ( 1.548556430446194954, -0.6046776061558807314, 0.2411417322834647770 ) ) ;
#69434=CARTESIAN_POINT ( 'NONE',  ( 0.9842519685039378130, -0.6692913385826771977, 8.415575281601705876E-17 ) ) ;
#69435=CARTESIAN_POINT ( 'NONE',  ( 1.679790026246720025, 0.2306618581243848609, 0.2411417322834645549 ) ) ;
#69436=CARTESIAN_POINT ( 'NONE',  ( -1.306827173596996738, 0.000000000000000000, -0.4445507791589060620 ) ) ;
#69437=CARTESIAN_POINT ( 'NONE',  ( 0.07874015748031558404, -0.1870078740157479769, 0.4822834645669291653 ) ) ;
#69438=CARTESIAN_POINT ( 'NONE',  ( -1.135170603674539924, 0.2952755905511810774, -0.1292274648535930714 ) ) ;
#69439=CARTESIAN_POINT ( 'NONE',  ( -1.509186351706035767, -0.4281496062992124485, 0.4176697321401328655 ) ) ;
#69441=CARTESIAN_POINT ( 'NONE',  ( 1.397637795275591177, 0.1660481256975883668, -0.3530559997133364547 ) ) ;
#69443=CARTESIAN_POINT ( 'NONE',  ( 0.9645669291338591078, -0.4536011799217368745, -0.2665933059059886201 ) ) ;
#69446=ORIENTED_EDGE ( 'NONE', *, *, #46038, .F. ) ;
#69447=CARTESIAN_POINT ( 'NONE',  ( 0.03937007874015806264, 0.1771653543307087630, 0.000000000000000000 ) ) ;
#69450=CARTESIAN_POINT ( 'NONE',  ( 0.7611548556430451917, -0.6046776061558807314, 0.2411417322834647770 ) ) ;
#69451=CARTESIAN_POINT ( 'NONE',  ( 0.4658792650918640033, -0.3162353388693405765, 0.4822834645669290543 ) ) ;
#69452=CARTESIAN_POINT ( 'NONE',  ( -0.5446194225721777693, -0.3162353388693409650, -0.4822834645669289433 ) ) ;
#69454=CARTESIAN_POINT ( 'NONE',  ( -1.003937007874014853, 0.1660481256975885056, 0.3530559997133364547 ) ) ;
#69456=CARTESIAN_POINT ( 'NONE',  ( 1.358267716535433323, -0.4536011799217368745, -0.2665933059059886201 ) ) ;
#69457=CARTESIAN_POINT ( 'NONE',  ( -0.9317585301837263412, -0.4281496062992127816, -0.4176697321401328100 ) ) ;
#69458=CARTESIAN_POINT ( 'NONE',  ( 0.8792650918635177559, 0.05413385826771666132, 0.4176697321401328100 ) ) ;
#69459=CARTESIAN_POINT ( 'NONE',  ( 0.9973753280839902091, -0.6046776061558807314, 0.2411417322834647770 ) ) ;
#69461=CARTESIAN_POINT ( 'NONE',  ( -1.305774278215222184, -0.6692913385826773087, -0.1292274648535924053 ) ) ;
#69463=CARTESIAN_POINT ( 'NONE',  ( 0.4133858267716541968, -0.5400638737290845981, -0.3530559997133363437 ) ) ;
#69466=CARTESIAN_POINT ( 'NONE',  ( 1.312335958005250269, -0.6046776061558807314, 0.2411417322834647770 ) ) ;
#69467=CARTESIAN_POINT ( 'NONE',  ( 0.2099737532808405305, -0.5023911411419708095, 0.1820866141732285504 ) ) ;
#69468=CARTESIAN_POINT ( 'NONE',  ( 0.8136482939632553313, 0.2306618581243848609, 0.2411417322834645549 ) ) ;
#69470=CARTESIAN_POINT ( 'NONE',  ( 0.8858267716535438430, 0.07958543189024085140, 0.2665933059059887866 ) ) ;
#69471=CARTESIAN_POINT ( 'NONE',  ( 0.4199475065616803948, -0.6046776061558809534, -0.2411417322834644161 ) ) ;
#69473=CARTESIAN_POINT ( 'NONE',  ( -0.8989501312335946848, 0.2952755905511810774, -0.1292274648535930714 ) ) ;
#69475=CARTESIAN_POINT ( 'NONE',  ( 0.7677165354330716118, -0.4536011799217367080, 0.2665933059059888421 ) ) ;
#69476=CARTESIAN_POINT ( 'NONE',  ( 0.09186351706036827158, 0.009842519685039467087, 0.3409548833797002021 ) ) ;
#69477=CARTESIAN_POINT ( 'NONE',  ( -0.3608923884514428360, -0.6692913385826773087, -0.1292274648535924053 ) ) ;
#69478=CARTESIAN_POINT ( 'NONE',  ( 0.1246719160104994284, 0.1771653543307087075, -0.09757992244046823083 ) ) ;
#69480=CARTESIAN_POINT ( 'NONE',  ( -0.4855643044619415427, -0.4281496062992124485, 0.4176697321401328655 ) ) ;
#69481=CARTESIAN_POINT ( 'NONE',  ( 0.5577427821522314977, -0.2845877964562161244, -0.3641732283464567121 ) ) ;
#69484=CARTESIAN_POINT ( 'NONE',  ( 0.3018372703412079971, 0.05413385826771626580, -0.4176697321401330321 ) ) ;
#69485=EDGE_CURVE ( 'NONE', #19643, #38994, #63312, .T. ) ;
#69488=CARTESIAN_POINT ( 'NONE',  ( 1.069553805774278832, 0.1771653543307087075, -0.09757992244046823083 ) ) ;
#69489=CARTESIAN_POINT ( 'NONE',  ( 0.1771653543307093459, 0.1660481256975885056, 0.3530559997133364547 ) ) ;
#69490=CARTESIAN_POINT ( 'NONE',  ( -0.5052493438320203589, -0.5511811023622046335, 0.09757992244046803654 ) ) ;
#69491=CARTESIAN_POINT ( 'NONE',  ( -0.6627296587926503335, -0.5511811023622046335, 0.09757992244046803654 ) ) ;
#69492=CARTESIAN_POINT ( 'NONE',  ( -0.3674540682414689785, 0.2306618581243848609, 0.2411417322834645549 ) ) ;
#69493=CARTESIAN_POINT ( 'NONE',  ( 0.3674540682414705883, 0.2306618581243847221, -0.2411417322834647770 ) ) ;
#69494=CARTESIAN_POINT ( 'NONE',  ( 0.9055118110236227702, 0.1771653543307087630, 0.000000000000000000 ) ) ;
#69496=CARTESIAN_POINT ( 'NONE',  ( 1.456692913385827515, 0.1771653543307087630, 0.000000000000000000 ) ) ;
#69497=CARTESIAN_POINT ( 'NONE',  ( 0.8398950131233602345, -0.6046776061558807314, 0.2411417322834647770 ) ) ;
#69499=CARTESIAN_POINT ( 'NONE',  ( -0.4199475065616791736, 0.2306618581243847221, -0.2411417322834647770 ) ) ;
#69501=CARTESIAN_POINT ( 'NONE',  ( 0.8595800524934390507, -0.3162353388693405765, 0.4822834645669290543 ) ) ;
#69502=CARTESIAN_POINT ( 'NONE',  ( 0.6496062992125991586, -0.5400638737290845981, -0.3530559997133363437 ) ) ;
#69504=CARTESIAN_POINT ( 'NONE',  ( 0.5118110236220480003, -0.5511811023622047445, 6.969142054262312111E-17 ) ) ;
#69505=CARTESIAN_POINT ( 'NONE',  ( 1.095800524934383846, -0.05778040916215560624, -0.4822834645669293319 ) ) ;
#69506=CARTESIAN_POINT ( 'NONE',  ( 0.09186351706036799403, -0.3690944881889765550, -0.3153832671262227771 ) ) ;
#69507=CARTESIAN_POINT ( 'NONE',  ( -0.4790026246719152336, -0.05778040916215560624, -0.4822834645669293319 ) ) ;
#69509=CARTESIAN_POINT ( 'NONE',  ( 0.1312335958005255154, -0.6046776061558807314, 0.2411417322834647770 ) ) ;
#69510=CARTESIAN_POINT ( 'NONE',  ( -0.9514435695538050464, -0.05778040916215560624, -0.4822834645669293319 ) ) ;
#69511=CARTESIAN_POINT ( 'NONE',  ( -0.1443569553805768291, -0.004921259842519576551, 0.3153832671262227771 ) ) ;
#69512=CARTESIAN_POINT ( 'NONE',  ( 0.5183727034120741983, 0.2952755905511810774, -0.1292274648535930714 ) ) ;
#69513=CARTESIAN_POINT ( 'NONE',  ( 0.7939632545931766261, -0.2845877964562161244, -0.3641732283464567121 ) ) ;
#69514=CARTESIAN_POINT ( 'NONE',  ( -0.4133858267716528645, -0.5400638737290844871, 0.3530559997133364547 ) ) ;
#69517=CARTESIAN_POINT ( 'NONE',  ( 1.220472440944882386, -0.6692913385826771977, 8.415575281601705876E-17 ) ) ;
#69518=CARTESIAN_POINT ( 'NONE',  ( 1.561679790026247350, 0.05413385826771626580, -0.4176697321401330321 ) ) ;
#69520=CARTESIAN_POINT ( 'NONE',  ( -1.640419947506561060, 0.05413385826771666132, 0.4176697321401328100 ) ) ;
#69521=CARTESIAN_POINT ( 'NONE',  ( -0.7283464566929126471, 0.1660481256975883668, -0.3530559997133364547 ) ) ;
#69524=ORIENTED_EDGE ( 'NONE', *, *, #29978, .T. ) ;
#69525=CARTESIAN_POINT ( 'NONE',  ( 0.3346456692913393205, -0.4536011799217368745, -0.2665933059059886201 ) ) ;
#69527=CARTESIAN_POINT ( 'NONE',  ( 0.7480314960629927956, -0.6692913385826771977, 8.415575281601705876E-17 ) ) ;
#69530=CARTESIAN_POINT ( 'NONE',  ( -0.4396325459317577122, -0.5511811023622048555, -0.09757992244046775898 ) ) ;
#69532=CARTESIAN_POINT ( 'NONE',  ( 0.9776902887139113929, -0.6692913385826773087, -0.1292274648535924053 ) ) ;
#69533=CARTESIAN_POINT ( 'NONE',  ( 1.528871391076116026, -0.5511811023622048555, -0.09757992244046775898 ) ) ;
#69534=CARTESIAN_POINT ( 'NONE',  ( 0.07874015748031558404, -0.1870078740157479769, 0.4822834645669291653 ) ) ;
#69536=CARTESIAN_POINT ( 'NONE',  ( -0.5839895013123351797, -0.6692913385826771977, 0.1292274648535927661 ) ) ;
#69537=CARTESIAN_POINT ( 'NONE',  ( -1.496062992125983815, -0.1870078740157480601, -0.3641732283464567677 ) ) ;
#69538=CARTESIAN_POINT ( 'NONE',  ( -0.4461942257217840213, 0.2306618581243848609, 0.2411417322834645549 ) ) ;
#69539=DIRECTION ( 'NONE',  ( 0.000000000000000000, -1.000000000000000000, -0.000000000000000000 ) ) ;
#69542=ORIENTED_EDGE ( 'NONE', *, *, #57357, .T. ) ;
#69544=CARTESIAN_POINT ( 'NONE',  ( 0.2559055118110243332, 0.1660481256975885056, 0.3530559997133364547 ) ) ;
#69547=CARTESIAN_POINT ( 'NONE',  ( -0.5380577427821514602, -0.4281496062992127816, -0.4176697321401328100 ) ) ;
#69548=CARTESIAN_POINT ( 'NONE',  ( -1.535433070866141225, -0.6692913385826771977, 8.415575281601705876E-17 ) ) ;
#69549=CARTESIAN_POINT ( 'NONE',  ( 0.8136482939632553313, 0.2306618581243848609, 0.2411417322834645549 ) ) ;
#69550=CARTESIAN_POINT ( 'NONE',  ( 0.1837270341207357105, -0.6046776061558809534, -0.2411417322834644161 ) ) ;
#69552=CARTESIAN_POINT ( 'NONE',  ( -0.6036745406824141069, 0.2306618581243848609, 0.2411417322834645549 ) ) ;
#69553=CARTESIAN_POINT ( 'NONE',  ( 0.1771653543307093182, -0.5400638737290845981, -0.3530559997133363437 ) ) ;
#69554=CARTESIAN_POINT ( 'NONE',  ( -0.6364829396325453192, -0.05778040916215560624, -0.4822834645669293319 ) ) ;
#69555=CARTESIAN_POINT ( 'NONE',  ( 0.5052493438320218022, -0.5511811023622048555, -0.09757992244046775898 ) ) ;
#69557=CARTESIAN_POINT ( 'NONE',  ( 0.02624671916010564918, 0.2306618581243848609, 0.2411417322834645549 ) ) ;
#69559=CARTESIAN_POINT ( 'NONE',  ( 1.587926509186352142, 0.05413385826771666132, 0.4176697321401328100 ) ) ;
#69563=CARTESIAN_POINT ( 'NONE',  ( 0.6036745406824154392, 0.2306618581243847221, -0.2411417322834647770 ) ) ;
#69564=CARTESIAN_POINT ( 'NONE',  ( -0.03937007874015669567, -0.5511811023622047445, 6.969142054262312111E-17 ) ) ;
#69565=CARTESIAN_POINT ( 'NONE',  ( 1.345144356955381593, -0.08942795157527998196, 0.3641732283464567121 ) ) ;
#69571=CARTESIAN_POINT ( 'NONE',  ( 0.3280839895013130669, 0.05413385826771666132, 0.4176697321401328100 ) ) ;
#69572=CARTESIAN_POINT ( 'NONE',  ( -1.364829396325458521, -0.6046776061558807314, 0.2411417322834647770 ) ) ;
#69573=CARTESIAN_POINT ( 'NONE',  ( -1.299212598425196097, -0.6692913385826771977, 8.415575281601705876E-17 ) ) ;
#69574=CARTESIAN_POINT ( 'NONE',  ( 0.4658792650918640033, -0.3162353388693405765, 0.4822834645669290543 ) ) ;
#69575=CARTESIAN_POINT ( 'NONE',  ( 1.003937007874016185, 0.1660481256975883668, -0.3530559997133364547 ) ) ;
#69576=CARTESIAN_POINT ( 'NONE',  ( 1.377952755905512472, 0.1771653543307087630, 0.000000000000000000 ) ) ;
#69578=CARTESIAN_POINT ( 'NONE',  ( 1.148293963254593875, -0.5511811023622046335, 0.09757992244046803654 ) ) ;
#69579=CARTESIAN_POINT ( 'NONE',  ( -0.9842519685039360366, 0.2952755905511811885, 0.000000000000000000 ) ) ;
#69581=CARTESIAN_POINT ( 'NONE',  ( 1.509186351706037543, 0.05413385826771666132, 0.4176697321401328100 ) ) ;
#69583=CARTESIAN_POINT ( 'NONE',  ( -0.2559055118110227234, -0.5400638737290844871, 0.3530559997133364547 ) ) ;
#69584=CARTESIAN_POINT ( 'NONE',  ( 0.9448818897637802916, -0.1870078740157480879, -0.4822834645669291653 ) ) ;
#69585=CARTESIAN_POINT ( 'NONE',  ( -1.614173228346457378, 1.267785121476993293, 0.1372047244094476981 ) ) ;
#69586=CARTESIAN_POINT ( 'NONE',  ( -1.541994750656167090, 0.1771653543307087630, 0.09757992244046791164 ) ) ;
#69587=CARTESIAN_POINT ( 'NONE',  ( 0.1181102362204730916, 0.2952755905511811885, 0.000000000000000000 ) ) ;
#69588=CARTESIAN_POINT ( 'NONE',  ( 0.6758530183727039509, 0.1771653543307087075, -0.09757992244046823083 ) ) ;
#69589=CARTESIAN_POINT ( 'NONE',  ( -1.496062992125983815, -0.1870078740157480601, -0.3641732283464567677 ) ) ;
#69590=CARTESIAN_POINT ( 'NONE',  ( 1.043307086614173818, 0.1660481256975885056, 0.3530559997133364547 ) ) ;
#69592=CARTESIAN_POINT ( 'NONE',  ( -0.3937007874015740483, -0.1870078740157480601, -0.3641732283464567677 ) ) ;
#69593=CARTESIAN_POINT ( 'NONE',  ( -0.7283464566929126471, 0.1660481256975883668, -0.3530559997133364547 ) ) ;
#69594=CARTESIAN_POINT ( 'NONE',  ( 1.430446194225722500, -0.4281496062992127816, -0.4176697321401328100 ) ) ;
#69595=CARTESIAN_POINT ( 'NONE',  ( -0.9580052493438311334, -0.4281496062992124485, 0.4176697321401328655 ) ) ;
#69596=CARTESIAN_POINT ( 'NONE',  ( 1.391076115485564868, 0.2306618581243847221, -0.2411417322834647770 ) ) ;
#69598=CARTESIAN_POINT ( 'NONE',  ( -1.181102362204723644, -0.1870078740157479769, 0.3641732283464567677 ) ) ;
#69600=CARTESIAN_POINT ( 'NONE',  ( 1.233595800524935227, -0.6046776061558807314, 0.2411417322834647770 ) ) ;
#69601=VECTOR ( 'NONE', #67865, 39.37007874015748143 ) ;
#69603=CARTESIAN_POINT ( 'NONE',  ( -1.450131233595799651, -0.6692913385826771977, 0.1292274648535927661 ) ) ;
#69604=CARTESIAN_POINT ( 'NONE',  ( -1.371391076115484609, -0.5511811023622046335, 0.09757992244046803654 ) ) ;
#69605=CARTESIAN_POINT ( 'NONE',  ( -1.062992125984250968, 0.1771653543307087630, 0.000000000000000000 ) ) ;
#69607=CARTESIAN_POINT ( 'NONE',  ( -0.4855643044619415427, 0.05413385826771626580, -0.4176697321401330321 ) ) ;
#69608=CARTESIAN_POINT ( 'NONE',  ( -0.09842519685039295696, -0.4536011799217367080, 0.2665933059059888421 ) ) ;
#69609=CARTESIAN_POINT ( 'NONE',  ( -1.384514435695537005, 0.1771653543307087630, 0.09757992244046791164 ) ) ;
#69610=CARTESIAN_POINT ( 'NONE',  ( 1.279527559055118724, 0.07958543189024085140, 0.2665933059059887866 ) ) ;
#69611=CARTESIAN_POINT ( 'NONE',  ( 1.043307086614173818, 0.1660481256975885056, 0.3530559997133364547 ) ) ;
#69612=CARTESIAN_POINT ( 'NONE',  ( 1.496062992125984703, -0.1870078740157480879, -0.4822834645669291653 ) ) ;
#69613=CARTESIAN_POINT ( 'NONE',  ( 0.2362204724409456558, -0.1870078740157479769, 0.3641732283464567677 ) ) ;
#69614=CARTESIAN_POINT ( 'NONE',  ( 0.3280839895013130669, -0.4281496062992127816, -0.4176697321401328100 ) ) ;
#69616=CARTESIAN_POINT ( 'NONE',  ( 1.181102362204724976, -0.1870078740157480601, -0.3641732283464567677 ) ) ;
#69617=ORIENTED_EDGE ( 'NONE', *, *, #35805, .F. ) ;
#69618=CARTESIAN_POINT ( 'NONE',  ( 1.463254593175853824, 0.2952755905511810774, -0.1292274648535930714 ) ) ;
#69619=EDGE_CURVE ( 'NONE', #22657, #11962, #39805, .T. ) ;
#69620=CARTESIAN_POINT ( 'NONE',  ( -1.489501312335957062, -0.05778040916215522460, 0.4822834645669289988 ) ) ;
#69621=CARTESIAN_POINT ( 'NONE',  ( -0.2821522309711278487, 0.2952755905511811885, 0.1292274648535926551 ) ) ;
#69624=CARTESIAN_POINT ( 'NONE',  ( 0.4133858267716541968, -0.5400638737290845981, -0.3530559997133363437 ) ) ;
#69625=CARTESIAN_POINT ( 'NONE',  ( 1.115485564304462551, -0.004921259842519576551, 0.3153832671262227771 ) ) ;
#69626=CARTESIAN_POINT ( 'NONE',  ( -0.1771653543307080136, 0.1660481256975883668, -0.3530559997133364547 ) ) ;
#69627=CARTESIAN_POINT ( 'NONE',  ( 0.4527559055118117182, -0.5400638737290844871, 0.3530559997133364547 ) ) ;
#69633=CARTESIAN_POINT ( 'NONE',  ( -0.3543307086614165824, -0.5511811023622047445, 6.969142054262312111E-17 ) ) ;
#69634=CARTESIAN_POINT ( 'NONE',  ( -0.9317585301837263412, 0.05413385826771666132, 0.4176697321401328100 ) ) ;
#69636=CARTESIAN_POINT ( 'NONE',  ( 0.9711286089238851948, -0.6046776061558809534, -0.2411417322834644161 ) ) ;
#69638=CARTESIAN_POINT ( 'NONE',  ( -1.515748031496062076, -0.5400638737290844871, 0.3530559997133364547 ) ) ;
#69639=CARTESIAN_POINT ( 'NONE',  ( 0.7874015748031503170, -0.1870078740157479769, 0.4822834645669291653 ) ) ;
#69643=EDGE_CURVE ( 'NONE', #66355, #46160, #38263, .T. ) ;
#69644=CARTESIAN_POINT ( 'NONE',  ( 1.089238845144357537, -0.4281496062992124485, 0.4176697321401328655 ) ) ;
#69645=CARTESIAN_POINT ( 'NONE',  ( 0.3805774278215230400, 0.05413385826771626580, -0.4176697321401330321 ) ) ;
#69646=CARTESIAN_POINT ( 'NONE',  ( 1.377952755905512472, -0.5511811023622047445, 6.969142054262312111E-17 ) ) ;
#69647=CARTESIAN_POINT ( 'NONE',  ( 1.266404199475066328, -0.3162353388693409650, -0.4822834645669289433 ) ) ;
#69649=CARTESIAN_POINT ( 'NONE',  ( -1.604771003085130321, 1.278209470906376932, 0.1466069496707743947 ) ) ;
#69650=CARTESIAN_POINT ( 'NONE',  ( 0.8661417322834653598, -0.1870078740157479769, 0.4822834645669291653 ) ) ;
#69651=CARTESIAN_POINT ( 'NONE',  ( 1.581364829396326277, -0.2845877964562161244, -0.3641732283464567121 ) ) ;
#69652=CARTESIAN_POINT ( 'NONE',  ( -0.4921259842519677963, -0.5400638737290844871, 0.3530559997133364547 ) ) ;
#69653=CARTESIAN_POINT ( 'NONE',  ( -1.154855643044618851, -0.6046776061558809534, -0.2411417322834644161 ) ) ;
#69654=CARTESIAN_POINT ( 'NONE',  ( 1.194225721784777594, -0.4281496062992127816, -0.4176697321401328100 ) ) ;
#69658=CARTESIAN_POINT ( 'NONE',  ( 1.430446194225722500, -0.4281496062992127816, -0.4176697321401328100 ) ) ;
#69662=CARTESIAN_POINT ( 'NONE',  ( -0.02624671916010427875, 0.1539470093639521697, -0.1968503937007875793 ) ) ;
#69663=VECTOR ( 'NONE', #43707, 39.37007874015748143 ) ;
#69664=CARTESIAN_POINT ( 'NONE',  ( 1.397637795275591177, -0.4536011799217367080, 0.2665933059059888421 ) ) ;
#69666=CARTESIAN_POINT ( 'NONE',  ( 1.423884514435696413, -0.2845877964562161244, -0.3641732283464567121 ) ) ;
#69667=CARTESIAN_POINT ( 'NONE',  ( -1.646051170424378096, 0.4405861044731112508, -0.5309055118110234117 ) ) ;
#69671=CARTESIAN_POINT ( 'NONE',  ( -0.6430446194225712953, -0.004921259842519870586, -0.3153832671262229437 ) ) ;
#69672=CARTESIAN_POINT ( 'NONE',  ( -1.305774278215222184, -0.5511811023622048555, -0.09757992244046775898 ) ) ;
#69673=CARTESIAN_POINT ( 'NONE',  ( -1.161417322834644716, 0.1660481256975885056, 0.3530559997133364547 ) ) ;
#69674=CARTESIAN_POINT ( 'NONE',  ( 0.1968503937007881344, 0.2952755905511811885, 0.000000000000000000 ) ) ;
#69675=CARTESIAN_POINT ( 'NONE',  ( -1.633858267716534529, 0.1660481256975885056, 0.3530559997133364547 ) ) ;
#69677=CARTESIAN_POINT ( 'NONE',  ( 1.594488188976378673, 0.1660481256975885056, 0.3530559997133364547 ) ) ;
#69681=DIRECTION ( 'NONE',  ( -3.096699300667737957E-16, 1.000000000000000000, -0.000000000000000000 ) ) ;
#69682=CARTESIAN_POINT ( 'NONE',  ( -0.4724409448818890911, -0.1870078740157480601, -0.3641732283464567677 ) ) ;
#69683=CARTESIAN_POINT ( 'NONE',  ( -1.312335958005248715, 0.2306618581243848609, 0.2411417322834645549 ) ) ;
#69684=CARTESIAN_POINT ( 'NONE',  ( 0.9776902887139113929, -0.6692913385826773087, -0.1292274648535924053 ) ) ;
#69688=CARTESIAN_POINT ( 'NONE',  ( 1.371391076115485941, 0.2952755905511811885, 0.1292274648535926551 ) ) ;
#69689=CARTESIAN_POINT ( 'NONE',  ( -1.076115485564303809, 0.2306618581243848609, 0.2411417322834645549 ) ) ;
#69691=CARTESIAN_POINT ( 'NONE',  ( -0.2099737532808391705, -0.5023911411419708095, -0.1820866141732282451 ) ) ;
#69693=CARTESIAN_POINT ( 'NONE',  ( -0.5511811023622038563, -0.1870078740157479769, 0.3641732283464567677 ) ) ;
#69694=CARTESIAN_POINT ( 'NONE',  ( 0.7020997375328090762, -0.08942795157528024563, -0.3641732283464568787 ) ) ;
#69695=CARTESIAN_POINT ( 'NONE',  ( 0.08530183727034192087, -0.3162353388693409650, -0.4822834645669289433 ) ) ;
#69696=CARTESIAN_POINT ( 'NONE',  ( -0.6627296587926501115, 0.1771653543307087075, -0.09757992244046823083 ) ) ;
#69698=CARTESIAN_POINT ( 'NONE',  ( 0.9645669291338588858, 0.1660481256975885056, 0.3530559997133364547 ) ) ;
#69699=ADVANCED_FACE ( 'NONE', ( #39189 ), #60097, .F. ) ;
#69700=CARTESIAN_POINT ( 'NONE',  ( -1.122047244094487306, 0.1660481256975883668, -0.3530559997133364547 ) ) ;
#69702=CARTESIAN_POINT ( 'NONE',  ( -0.1968503937007867743, -0.6692913385826771977, 8.415575281601705876E-17 ) ) ;
#69703=CARTESIAN_POINT ( 'NONE',  ( -0.8202099737532799750, 0.2952755905511810774, -0.1292274648535930714 ) ) ;
#69704=CARTESIAN_POINT ( 'NONE',  ( 1.181102362204725198, -0.1870078740157479769, 0.3641732283464567677 ) ) ;
#69705=CARTESIAN_POINT ( 'NONE',  ( 0.1115485564304467270, -0.5511811023622048555, -0.09757992244046775898 ) ) ;
#69706=CARTESIAN_POINT ( 'NONE',  ( -0.5577427821522301654, -0.05778040916215560624, -0.4822834645669293319 ) ) ;
#69707=CARTESIAN_POINT ( 'NONE',  ( -1.148293963254592542, 0.2952755905511811885, 0.1292274648535926551 ) ) ;
#69708=CARTESIAN_POINT ( 'NONE',  ( 0.3937007874015751585, 1.535433070866141447, 0.000000000000000000 ) ) ;
#69710=CARTESIAN_POINT ( 'NONE',  ( -0.3740157480314953431, 0.1660481256975885056, 0.3530559997133364547 ) ) ;
#69711=CARTESIAN_POINT ( 'NONE',  ( -0.9514435695538050464, -0.3162353388693405765, 0.4822834645669290543 ) ) ;
#69714=CARTESIAN_POINT ( 'NONE',  ( 1.200787401574803681, -0.5400638737290845981, -0.3530559997133363437 ) ) ;
#69715=CARTESIAN_POINT ( 'NONE',  ( -0.5118110236220466680, -0.5511811023622047445, 6.969142054262312111E-17 ) ) ;
#69716=CARTESIAN_POINT ( 'NONE',  ( -0.8202099737532801971, -0.6692913385826771977, 0.1292274648535927661 ) ) ;
#69717=CARTESIAN_POINT ( 'NONE',  ( 1.489501312335958172, -0.3162353388693405765, 0.4822834645669290543 ) ) ;
#69718=CARTESIAN_POINT ( 'NONE',  ( 0.9448818897637802916, -0.1870078740157480879, -0.4822834645669291653 ) ) ;
#69719=CARTESIAN_POINT ( 'NONE',  ( 1.489501312335958172, -0.05778040916215560624, -0.4822834645669293319 ) ) ;
#69720=CARTESIAN_POINT ( 'NONE',  ( -0.9908136482939626788, -0.5511811023622048555, -0.09757992244046775898 ) ) ;
#69725=CARTESIAN_POINT ( 'NONE',  ( 1.358267716535433323, 0.07958543189024085140, 0.2665933059059887866 ) ) ;
#69726=CARTESIAN_POINT ( 'NONE',  ( 0.6758530183727039509, 0.1771653543307087075, -0.09757992244046823083 ) ) ;
#69727=CARTESIAN_POINT ( 'NONE',  ( 0.4790026246719167324, -0.05778040916215522460, 0.4822834645669289988 ) ) ;
#69730=CARTESIAN_POINT ( 'NONE',  ( 0.8989501312335964611, 0.1771653543307087630, 0.09757992244046791164 ) ) ;
#69732=CARTESIAN_POINT ( 'NONE',  ( -0.4265091863517051496, -0.6692913385826771977, 0.1292274648535927661 ) ) ;
#69733=CARTESIAN_POINT ( 'NONE',  ( -1.187664041994749731, -0.3162353388693405765, 0.4822834645669290543 ) ) ;
#69734=CARTESIAN_POINT ( 'NONE',  ( 1.200787401574803681, 0.1660481256975885056, 0.3530559997133364547 ) ) ;
#69737=CARTESIAN_POINT ( 'NONE',  ( -0.1443569553805768291, -0.004921259842519576551, 0.3153832671262227771 ) ) ;
#69738=VERTEX_POINT ( 'NONE', #28877 ) ;
#69740=CARTESIAN_POINT ( 'NONE',  ( -0.8727034120734901146, -0.05778040916215560624, -0.4822834645669293319 ) ) ;
#69741=CARTESIAN_POINT ( 'NONE',  ( -0.5118110236220466680, 0.2952755905511811885, 0.000000000000000000 ) ) ;
#69742=CARTESIAN_POINT ( 'NONE',  ( -0.7545931758530176614, -0.6692913385826773087, -0.1292274648535924053 ) ) ;
#69743=CARTESIAN_POINT ( 'NONE',  ( 0.3674540682414705883, -0.6046776061558807314, 0.2411417322834647770 ) ) ;
#69744=CARTESIAN_POINT ( 'NONE',  ( -0.4133858267716528645, -0.5400638737290844871, 0.3530559997133364547 ) ) ;
#69745=CARTESIAN_POINT ( 'NONE',  ( -1.541994750656167090, -0.6692913385826773087, -0.1292274648535924053 ) ) ;
#69746=CARTESIAN_POINT ( 'NONE',  ( -1.010498687664041384, -0.4281496062992127816, -0.4176697321401328100 ) ) ;
#69747=CARTESIAN_POINT ( 'NONE',  ( 0.7020997375328090762, -0.05778040916215560624, -0.4822834645669293319 ) ) ;
#69749=CARTESIAN_POINT ( 'NONE',  ( -0.5118110236220466680, 0.1771653543307087630, 0.000000000000000000 ) ) ;
#69750=EDGE_LOOP ( 'NONE', ( #49250, #47162, #30835, #15299, #44253, #5867, #56963 ) ) ;
#69752=VERTEX_POINT ( 'NONE', #80255 ) ;
#69753=CARTESIAN_POINT ( 'NONE',  ( -1.437007874015747477, -0.4536011799217367080, 0.2665933059059888421 ) ) ;
#69754=CARTESIAN_POINT ( 'NONE',  ( -0.9514435695538050464, -0.05778040916215560624, -0.4822834645669293319 ) ) ;
#69755=CARTESIAN_POINT ( 'NONE',  ( -1.003937007874014853, 0.1660481256975885056, 0.3530559997133364547 ) ) ;
#69757=CARTESIAN_POINT ( 'NONE',  ( -1.305774278215222184, -0.6692913385826773087, -0.1292274648535924053 ) ) ;
#69758=CARTESIAN_POINT ( 'NONE',  ( -0.7808398950131225646, -0.05778040916215522460, 0.4822834645669289988 ) ) ;
#69760=EDGE_CURVE ( 'NONE', #35306, #69836, #57339, .T. ) ;
#69762=CARTESIAN_POINT ( 'NONE',  ( 0.5249343832021005074, -0.5023911411419708095, 0.1820866141732285504 ) ) ;
#69763=CARTESIAN_POINT ( 'NONE',  ( -0.4843739873036757571, -1.316179764993976518E-15, -0.3627985898453525149 ) ) ;
#69765=CARTESIAN_POINT ( 'NONE',  ( 0.1312335958005255154, -0.5023911411419708095, 0.1820866141732285504 ) ) ;
#69766=CARTESIAN_POINT ( 'NONE',  ( -0.4986876640419939388, 0.2306618581243847221, -0.2411417322834647770 ) ) ;
#69768=CARTESIAN_POINT ( 'NONE',  ( 1.240157480314961314, -0.5400638737290844871, 0.3530559997133364547 ) ) ;
#69769=CARTESIAN_POINT ( 'NONE',  ( -0.6561679790026240244, 0.2306618581243847221, -0.2411417322834647770 ) ) ;
#69770=VERTEX_POINT ( 'NONE', #3628 ) ;
#69772=CARTESIAN_POINT ( 'NONE',  ( 0.2486400153428833526, 3.421639014772782816E-16, 0.3464511005275203726 ) ) ;
#69775=CARTESIAN_POINT ( 'NONE',  ( -0.4002624671916004129, -0.3162353388693405765, 0.4822834645669290543 ) ) ;
#69776=CARTESIAN_POINT ( 'NONE',  ( 1.417322834645670104, -0.1870078740157479769, 0.4822834645669291653 ) ) ;
#69777=CARTESIAN_POINT ( 'NONE',  ( -0.9711286089238838626, -0.5023911411419708095, 0.1820866141732285504 ) ) ;
#69778=CARTESIAN_POINT ( 'NONE',  ( -1.233595800524933894, 0.2306618581243848609, 0.2411417322834645549 ) ) ;
#69782=CARTESIAN_POINT ( 'NONE',  ( 1.384514435695538559, 0.2952755905511810774, -0.1292274648535930714 ) ) ;
#69784=CARTESIAN_POINT ( 'NONE',  ( 0.09842519685039434474, 0.1660481256975885056, 0.3530559997133364547 ) ) ;
#69785=CARTESIAN_POINT ( 'NONE',  ( -0.9908136482939626788, 0.1771653543307087630, 0.09757992244046791164 ) ) ;
#69786=CARTESIAN_POINT ( 'NONE',  ( -0.1706036745406816491, -0.4281496062992124485, 0.4176697321401328655 ) ) ;
#69788=CARTESIAN_POINT ( 'NONE',  ( -0.8267716535433065062, -0.6692913385826771977, 8.415575281601705876E-17 ) ) ;
#69790=CARTESIAN_POINT ( 'NONE',  ( 0.7283464566929140904, -0.4536011799217368745, -0.2665933059059886201 ) ) ;
#69791=CARTESIAN_POINT ( 'NONE',  ( -0.1771653543307080136, -0.4536011799217367080, 0.2665933059059888421 ) ) ;
#69792=CARTESIAN_POINT ( 'NONE',  ( 0.9448818897637802916, -0.1870078740157480601, -0.3641732283464567677 ) ) ;
#69793=CARTESIAN_POINT ( 'NONE',  ( -1.364829396325458521, 0.2306618581243847221, -0.2411417322834647770 ) ) ;
#69795=CARTESIAN_POINT ( 'NONE',  ( 0.7349081364829403995, 0.1283753931104748280, 0.1820866141732283561 ) ) ;
#69796=CARTESIAN_POINT ( 'NONE',  ( -1.043307086614172041, -0.5400638737290844871, 0.3530559997133364547 ) ) ;
#69798=CARTESIAN_POINT ( 'NONE',  ( -0.03937007874015669567, 0.1771653543307087630, 0.000000000000000000 ) ) ;
#69799=CARTESIAN_POINT ( 'NONE',  ( -1.541994750656167090, 0.1771653543307087630, 0.09757992244046791164 ) ) ;
#69800=CARTESIAN_POINT ( 'NONE',  ( 0.5708661417322842269, 0.1660481256975885056, 0.3530559997133364547 ) ) ;
#69801=CARTESIAN_POINT ( 'NONE',  ( 0.6986524979670498681, 8.471767977567108961E-16, -0.4445507791589058955 ) ) ;
#69802=CARTESIAN_POINT ( 'NONE',  ( 1.305774278215223960, 0.1771653543307087075, -0.09757992244046823083 ) ) ;
#69803=CARTESIAN_POINT ( 'NONE',  ( -1.240157480314959759, 0.1660481256975885056, 0.3530559997133364547 ) ) ;
#69804=CARTESIAN_POINT ( 'NONE',  ( -0.1771653543307080136, 0.07958543189024071263, -0.2665933059059888421 ) ) ;
#69805=CARTESIAN_POINT ( 'NONE',  ( -0.7137454485294959516, 2.001539355558159983, 0.4917280318828578523 ) ) ;
#69806=CARTESIAN_POINT ( 'NONE',  ( 0.2362204724409456558, -0.1870078740157480601, -0.3641732283464567677 ) ) ;
#69807=CARTESIAN_POINT ( 'NONE',  ( -1.279527559055116948, -0.5400638737290844871, 0.3530559997133364547 ) ) ;
#69808=CARTESIAN_POINT ( 'NONE',  ( -0.5839895013123351797, -0.6692913385826771977, 0.1292274648535927661 ) ) ;
#69811=CARTESIAN_POINT ( 'NONE',  ( 0.6692913385826777528, 0.1771653543307087630, 0.000000000000000000 ) ) ;
#69812=CARTESIAN_POINT ( 'NONE',  ( -0.2296587926509179312, -0.05778040916215522460, 0.4822834645669289988 ) ) ;
#69813=CARTESIAN_POINT ( 'NONE',  ( -0.6102362204724400829, -0.5400638737290845981, -0.3530559997133363437 ) ) ;
#69814=CARTESIAN_POINT ( 'NONE',  ( -1.010498687664041384, -0.004921259842519576551, 0.3153832671262227771 ) ) ;
#69816=CARTESIAN_POINT ( 'NONE',  ( -0.04593175853018302557, 0.2952755905511811885, 0.1292274648535926551 ) ) ;
#69817=CARTESIAN_POINT ( 'NONE',  ( -1.686351706036744558, 0.1771653543307087075, -0.09757992244046823083 ) ) ;
#69818=CARTESIAN_POINT ( 'NONE',  ( 1.266404199475066328, -0.05778040916215522460, 0.4822834645669289988 ) ) ;
#69823=CARTESIAN_POINT ( 'NONE',  ( -1.502624671916009680, -0.05778040916215560624, -0.4822834645669293319 ) ) ;
#69824=CARTESIAN_POINT ( 'NONE',  ( -1.062992125984250968, 0.2952755905511811885, 0.000000000000000000 ) ) ;
#69825=CARTESIAN_POINT ( 'NONE',  ( 1.489501312335958172, -0.05778040916215560624, -0.4822834645669293319 ) ) ;
#69828=CARTESIAN_POINT ( 'NONE',  ( 0.7414698162729663755, 0.2952755905511811885, 0.1292274648535926551 ) ) ;
#69829=CARTESIAN_POINT ( 'NONE',  ( 0.03937007874015833325, -0.6692913385826771977, 8.415575281601705876E-17 ) ) ;
#69831=DIRECTION ( 'NONE',  ( -3.114085624724525612E-16, 1.000000000000000000, 5.270319453084425600E-32 ) ) ;
#69832=CARTESIAN_POINT ( 'NONE',  ( 1.351706036745407458, -0.3690944881889765550, -0.3153832671262227771 ) ) ;
#69836=VERTEX_POINT ( 'NONE', #43144 ) ;
#69837=CARTESIAN_POINT ( 'NONE',  ( 0.2230971128608929543, 0.05413385826771626580, -0.4176697321401330321 ) ) ;
#69838=CARTESIAN_POINT ( 'NONE',  ( -0.8595800524934373854, -0.3162353388693409650, -0.4822834645669289433 ) ) ;
#69839=CARTESIAN_POINT ( 'NONE',  ( -1.417322834645668772, -0.1870078740157480879, -0.4822834645669291653 ) ) ;
#69840=CARTESIAN_POINT ( 'NONE',  ( 0.5118110236220480003, -0.6692913385826771977, 8.415575281601705876E-17 ) ) ;
#69841=CARTESIAN_POINT ( 'NONE',  ( 1.456692913385827515, -0.6692913385826771977, 8.415575281601705876E-17 ) ) ;
#69842=CARTESIAN_POINT ( 'NONE',  ( 1.266404199475066328, -0.05778040916215522460, 0.4822834645669289988 ) ) ;
#69843=CARTESIAN_POINT ( 'NONE',  ( -0.1377952755905504645, -0.5400638737290845981, -0.3530559997133363437 ) ) ;
#69844=CARTESIAN_POINT ( 'NONE',  ( -1.325459317585300889, 0.05413385826771666132, 0.4176697321401328100 ) ) ;
#69845=CYLINDRICAL_SURFACE ( 'NONE', #3076, 0.3937007874015748254 ) ;
#69846=CARTESIAN_POINT ( 'NONE',  ( 1.528871391076116026, 0.2952755905511811885, 0.1292274648535926551 ) ) ;
#69848=CARTESIAN_POINT ( 'NONE',  ( 0.8398950131233602345, -0.5023911411419708095, 0.1820866141732285504 ) ) ;
#69851=VERTEX_POINT ( 'NONE', #29296 ) ;
#69852=CARTESIAN_POINT ( 'NONE',  ( 0.05249343832021075018, 0.1283753931104746893, -0.1820866141732285504 ) ) ;
#69854=CARTESIAN_POINT ( 'NONE',  ( 0.5183727034120741983, 0.2952755905511810774, -0.1292274648535930714 ) ) ;
#69855=CARTESIAN_POINT ( 'NONE',  ( 0.5708661417322841158, -0.5400638737290845981, -0.3530559997133363437 ) ) ;
#69857=CARTESIAN_POINT ( 'NONE',  ( -0.4986876640419942164, -0.6046776061558807314, 0.2411417322834647770 ) ) ;
#69859=CARTESIAN_POINT ( 'NONE',  ( -1.200787401574802349, -0.5400638737290844871, 0.3530559997133364547 ) ) ;
#69861=CARTESIAN_POINT ( 'NONE',  ( 1.279527559055118724, 0.07958543189024085140, 0.2665933059059887866 ) ) ;
#69862=CARTESIAN_POINT ( 'NONE',  ( -1.574803149606298192, -0.1870078740157480879, -0.4822834645669291653 ) ) ;
#69863=CARTESIAN_POINT ( 'NONE',  ( 0.8070866141732289112, -0.5400638737290845981, -0.3530559997133363437 ) ) ;
#69864=CARTESIAN_POINT ( 'NONE',  ( 1.292650918635171564, -0.6692913385826773087, -0.1292274648535924053 ) ) ;
#69866=CARTESIAN_POINT ( 'NONE',  ( -1.423884514435694859, -0.3162353388693405765, 0.4822834645669290543 ) ) ;
#69869=CARTESIAN_POINT ( 'NONE',  ( 0.04593175853018440641, 0.2952755905511810774, -0.1292274648535930714 ) ) ;
#69872=CARTESIAN_POINT ( 'NONE',  ( 1.286089238845145033, -0.6046776061558809534, -0.2411417322834644161 ) ) ;
#69873=CARTESIAN_POINT ( 'NONE',  ( 0.2165354330708668673, -0.4536011799217367080, 0.2665933059059888421 ) ) ;
#69874=CARTESIAN_POINT ( 'NONE',  ( 0.7217847769028878924, -0.4281496062992127816, -0.4176697321401328100 ) ) ;
#69876=CARTESIAN_POINT ( 'NONE',  ( 0.4330708661417329575, 0.1771653543307087630, 0.000000000000000000 ) ) ;
#69877=CARTESIAN_POINT ( 'NONE',  ( 0.4002624671916016896, -0.3162353388693409650, -0.4822834645669289433 ) ) ;
#69879=CARTESIAN_POINT ( 'NONE',  ( -0.6824146981627291497, -0.6046776061558809534, -0.2411417322834644161 ) ) ;
#69880=CARTESIAN_POINT ( 'NONE',  ( 0.9580052493438326877, -0.004921259842519576551, 0.3153832671262227771 ) ) ;
#69881=CARTESIAN_POINT ( 'NONE',  ( -1.128608923884513837, 0.2306618581243847221, -0.2411417322834647770 ) ) ;
#69882=CARTESIAN_POINT ( 'NONE',  ( -0.1837270341207343505, -0.6046776061558807314, 0.2411417322834647770 ) ) ;
#69883=CARTESIAN_POINT ( 'NONE',  ( 0.1968503937007881344, -0.5511811023622047445, 6.969142054262312111E-17 ) ) ;
#69885=CARTESIAN_POINT ( 'NONE',  ( -0.2559055118110230564, 0.1660481256975883668, -0.3530559997133364547 ) ) ;
#69886=CARTESIAN_POINT ( 'NONE',  ( 0.2755905511811031494, -0.5511811023622047445, 6.969142054262312111E-17 ) ) ;
#69888=CARTESIAN_POINT ( 'NONE',  ( 0.4199475065616805614, 0.2306618581243848609, 0.2411417322834645549 ) ) ;
#69889=CARTESIAN_POINT ( 'NONE',  ( 1.325459317585302665, -0.3690944881889763329, 0.3153832671262228327 ) ) ;
#69891=CARTESIAN_POINT ( 'NONE',  ( -0.5314960629921254842, -0.4536011799217368745, -0.2665933059059886201 ) ) ;
#69892=CARTESIAN_POINT ( 'NONE',  ( -0.5643044619422565855, -0.004921259842519870586, -0.3153832671262229437 ) ) ;
#69893=CARTESIAN_POINT ( 'NONE',  ( -0.1837270341207340729, 0.2306618581243847221, -0.2411417322834647770 ) ) ;
#69894=CARTESIAN_POINT ( 'NONE',  ( 0.3346456692913390985, 0.1660481256975885056, 0.3530559997133364547 ) ) ;
#69895=CARTESIAN_POINT ( 'NONE',  ( 0.8727034120734913358, -0.08942795157527998196, 0.3641732283464567121 ) ) ;
#69896=CARTESIAN_POINT ( 'NONE',  ( -1.620734908136482577, -0.5511811023622048555, -0.09757992244046775898 ) ) ;
#69897=CARTESIAN_POINT ( 'NONE',  ( -1.692913385826770645, 0.2952755905511811885, 0.000000000000000000 ) ) ;
#69898=CARTESIAN_POINT ( 'NONE',  ( 0.5774278215223104249, 0.2306618581243848609, 0.2411417322834645549 ) ) ;
#69900=CARTESIAN_POINT ( 'NONE',  ( -0.08530183727034056085, -0.05778040916215560624, -0.4822834645669293319 ) ) ;
#69902=CARTESIAN_POINT ( 'NONE',  ( 1.095800524934383846, -0.05778040916215560624, -0.4822834645669293319 ) ) ;
#69903=CARTESIAN_POINT ( 'NONE',  ( 0.6430446194225729606, -0.4281496062992127816, -0.4176697321401328100 ) ) ;
#69905=CARTESIAN_POINT ( 'NONE',  ( 0.3083989501312343062, -0.08942795157528024563, -0.3641732283464568787 ) ) ;
#69906=CARTESIAN_POINT ( 'NONE',  ( 1.213910761154856299, 0.2952755905511811885, 0.1292274648535926551 ) ) ;
#69907=CARTESIAN_POINT ( 'NONE',  ( -0.3346456692913377662, -0.4536011799217367080, 0.2665933059059888421 ) ) ;
#69908=CARTESIAN_POINT ( 'NONE',  ( -0.2099737532808391705, 0.2306618581243848609, 0.2411417322834645549 ) ) ;
#69910=CARTESIAN_POINT ( 'NONE',  ( 0.2034120734908142214, 0.2952755905511810774, -0.1292274648535930714 ) ) ;
#69911=CARTESIAN_POINT ( 'NONE',  ( -0.8923884514435688198, -0.6046776061558807314, 0.2411417322834647770 ) ) ;
#69912=CARTESIAN_POINT ( 'NONE',  ( -0.5643044619422565855, -0.004921259842519870586, -0.3153832671262229437 ) ) ;
#69913=CARTESIAN_POINT ( 'NONE',  ( 0.3608923884514443348, 0.2952755905511810774, -0.1292274648535930714 ) ) ;
#69914=CARTESIAN_POINT ( 'NONE',  ( -1.305774278215222184, -0.6692913385826773087, -0.1292274648535924053 ) ) ;
#69915=CARTESIAN_POINT ( 'NONE',  ( -0.3608923884514428360, 0.2952755905511811885, 0.1292274648535926551 ) ) ;
#69918=CARTESIAN_POINT ( 'NONE',  ( 1.325459317585302665, 0.05413385826771626580, -0.4176697321401330321 ) ) ;
#69919=CARTESIAN_POINT ( 'NONE',  ( 1.102362204724410155, -0.1870078740157480879, -0.4822834645669291653 ) ) ;
#69921=CARTESIAN_POINT ( 'NONE',  ( -1.620734908136482577, 0.2952755905511811885, 0.1292274648535926551 ) ) ;
#69922=CARTESIAN_POINT ( 'NONE',  ( -1.049868766404198794, 0.2306618581243847221, -0.2411417322834647770 ) ) ;
#69926=CARTESIAN_POINT ( 'NONE',  ( -0.03937007874015669567, 0.1771653543307087630, 0.000000000000000000 ) ) ;
#69928=CARTESIAN_POINT ( 'NONE',  ( 0.7545931758530188826, -0.6692913385826771977, 0.1292274648535927661 ) ) ;
#69931=CARTESIAN_POINT ( 'NONE',  ( -0.5774278215223089816, -0.5023911411419708095, 0.1820866141732285504 ) ) ;
#69933=CARTESIAN_POINT ( 'NONE',  ( 1.062992125984252745, 0.2952755905511811885, 0.000000000000000000 ) ) ;
#69934=CARTESIAN_POINT ( 'NONE',  ( 1.062992125984252745, -0.5511811023622047445, 6.969142054262312111E-17 ) ) ;
#69935=CARTESIAN_POINT ( 'NONE',  ( -0.1902887139107604098, 0.2952755905511810774, -0.1292274648535930714 ) ) ;
#69937=CARTESIAN_POINT ( 'NONE',  ( -0.2427821522309703550, -0.3162353388693405765, 0.4822834645669290543 ) ) ;
#69938=CARTESIAN_POINT ( 'NONE',  ( -1.371391076115484831, 0.1771653543307087075, -0.09757992244046823083 ) ) ;
#69939=EDGE_CURVE ( 'NONE', #79831, #46664, #55367, .T. ) ;
#69940=CARTESIAN_POINT ( 'NONE',  ( -0.3346456692913377662, -0.5400638737290844871, 0.3530559997133364547 ) ) ;
#69941=DIRECTION ( 'NONE',  ( -3.096699300667737957E-16, 1.000000000000000000, -0.000000000000000000 ) ) ;
#69945=CARTESIAN_POINT ( 'NONE',  ( 0.2887139107611556010, 0.2306618581243847221, -0.2411417322834647770 ) ) ;
#69946=VERTEX_POINT ( 'NONE', #80665 ) ;
#69947=CARTESIAN_POINT ( 'NONE',  ( -0.9120734908136475250, 0.2952755905511811885, 0.1292274648535926551 ) ) ;
#69948=CARTESIAN_POINT ( 'NONE',  ( -1.364829396325458521, -0.6046776061558807314, 0.2411417322834647770 ) ) ;
#69949=CARTESIAN_POINT ( 'NONE',  ( 0.8267716535433077274, 0.2952755905511811885, 0.000000000000000000 ) ) ;
#69950=EDGE_CURVE ( 'NONE', #10845, #4446, #49880, .T. ) ;
#69951=CARTESIAN_POINT ( 'NONE',  ( -0.1246719160104980823, -0.6692913385826773087, -0.1292274648535924053 ) ) ;
#69953=CARTESIAN_POINT ( 'NONE',  ( -0.5839895013123351797, 0.2952755905511810774, -0.1292274648535930714 ) ) ;
#69954=CARTESIAN_POINT ( 'NONE',  ( -0.2887139107611542133, -0.6046776061558809534, -0.2411417322834644161 ) ) ;
#69955=CARTESIAN_POINT ( 'NONE',  ( -0.8989501312335946848, -0.6692913385826771977, 0.1292274648535927661 ) ) ;
#69956=CARTESIAN_POINT ( 'NONE',  ( 0.4265091863517067594, 0.1771653543307087630, 0.09757992244046791164 ) ) ;
#69958=CARTESIAN_POINT ( 'NONE',  ( -0.01968503937007793844, -0.5400638737290844871, 0.3530559997133364547 ) ) ;
#69959=DIRECTION ( 'NONE',  ( -0.000000000000000000, 1.000000000000000000, -0.000000000000000000 ) ) ;
#69960=CARTESIAN_POINT ( 'NONE',  ( 1.089238845144357537, -0.4281496062992124485, 0.4176697321401328655 ) ) ;
#69964=CARTESIAN_POINT ( 'NONE',  ( 0.1837270341207357105, -0.6046776061558809534, -0.2411417322834644161 ) ) ;
#69965=CARTESIAN_POINT ( 'NONE',  ( -0.04593175853018302557, -0.5511811023622048555, -0.09757992244046775898 ) ) ;
#69966=CARTESIAN_POINT ( 'NONE',  ( 1.437007874015748810, -0.4536011799217368745, -0.2665933059059886201 ) ) ;
#69971=CARTESIAN_POINT ( 'NONE',  ( -1.456692913385826182, 0.2952755905511811885, 0.000000000000000000 ) ) ;
#69973=CARTESIAN_POINT ( 'NONE',  ( 0.3805774278215230400, 0.05413385826771626580, -0.4176697321401330321 ) ) ;
#69974=CARTESIAN_POINT ( 'NONE',  ( -1.108923884514435132, -0.05778040916215560624, -0.4822834645669293319 ) ) ;
#69975=CARTESIAN_POINT ( 'NONE',  ( -1.148293963254592542, -0.6692913385826773087, -0.1292274648535924053 ) ) ;
#69976=CARTESIAN_POINT ( 'NONE',  ( 0.1771653543307093182, 0.1660481256975885056, 0.3530559997133364547 ) ) ;
#69977=CARTESIAN_POINT ( 'NONE',  ( 0.9776902887139113929, 0.2952755905511811885, 0.1292274648535926551 ) ) ;
#69978=CARTESIAN_POINT ( 'NONE',  ( 1.548556430446194954, 0.1283753931104746893, -0.1820866141732285504 ) ) ;
#69980=CARTESIAN_POINT ( 'NONE',  ( 0.6955380577427828781, -0.3690944881889763329, 0.3153832671262228327 ) ) ;
#69981=CARTESIAN_POINT ( 'NONE',  ( -0.8202099737532799750, 0.2952755905511810774, -0.1292274648535930714 ) ) ;
#69983=CARTESIAN_POINT ( 'NONE',  ( 1.450131233595801428, -0.6692913385826773087, -0.1292274648535924053 ) ) ;
#69985=CARTESIAN_POINT ( 'NONE',  ( 0.6496062992125991586, -0.5400638737290845981, -0.3530559997133363437 ) ) ;
#69987=CARTESIAN_POINT ( 'NONE',  ( -1.614173228346456268, -0.5511811023622047445, 6.969142054262312111E-17 ) ) ;
#69988=CARTESIAN_POINT ( 'NONE',  ( -0.03280839895013062252, 0.2952755905511810774, -0.1292274648535930714 ) ) ;
#69989=CARTESIAN_POINT ( 'NONE',  ( 1.056430446194226436, -0.5511811023622048555, -0.09757992244046775898 ) ) ;
#69990=CARTESIAN_POINT ( 'NONE',  ( -1.476377952755905110, -0.4536011799217368745, -0.2665933059059886201 ) ) ;
#69991=CARTESIAN_POINT ( 'NONE',  ( 1.154855643044620184, -0.6046776061558807314, 0.2411417322834647770 ) ) ;
#69992=CARTESIAN_POINT ( 'NONE',  ( -0.5380577427821514602, 0.05413385826771666132, 0.4176697321401328100 ) ) ;
#69993=CARTESIAN_POINT ( 'NONE',  ( -0.3412073490813641308, -0.5023911411419708095, 0.1820866141732285504 ) ) ;
#69994=CARTESIAN_POINT ( 'NONE',  ( -0.3937007874015740483, -0.1870078740157480879, -0.4822834645669291653 ) ) ;
#69995=CARTESIAN_POINT ( 'NONE',  ( 1.377952755905512472, 0.2952755905511811885, 0.000000000000000000 ) ) ;
#69996=CARTESIAN_POINT ( 'NONE',  ( -1.108923884514435132, -0.3162353388693405765, 0.4822834645669290543 ) ) ;
#69997=CARTESIAN_POINT ( 'NONE',  ( 1.253280839895013710, -0.05778040916215560624, -0.4822834645669293319 ) ) ;
#69999=CARTESIAN_POINT ( 'NONE',  ( -1.227034120734907141, -0.5511811023622048555, -0.09757992244046775898 ) ) ;
#70001=CARTESIAN_POINT ( 'NONE',  ( 0.8792650918635177559, -0.4281496062992127816, -0.4176697321401328100 ) ) ;
#70003=CARTESIAN_POINT ( 'NONE',  ( -1.686351706036744558, 0.2952755905511810774, -0.1292274648535930714 ) ) ;
#70004=CARTESIAN_POINT ( 'NONE',  ( -1.601049868766403650, 0.1283753931104746893, -0.1820866141732285504 ) ) ;
#70005=CARTESIAN_POINT ( 'NONE',  ( -1.128608923884513837, -0.5023911411419708095, 0.1820866141732285504 ) ) ;
#70006=CARTESIAN_POINT ( 'NONE',  ( 1.430446194225722500, -0.3690944881889765550, -0.3153832671262227771 ) ) ;
#70007=CARTESIAN_POINT ( 'NONE',  ( -0.5839895013123351797, -0.6692913385826771977, 0.1292274648535927661 ) ) ;
#70008=CARTESIAN_POINT ( 'NONE',  ( -0.1377952755905504645, -0.4536011799217368745, -0.2665933059059886201 ) ) ;
#70009=CARTESIAN_POINT ( 'NONE',  ( -1.679790026246718693, 0.1283753931104746893, -0.1820866141732285504 ) ) ;
#70010=CARTESIAN_POINT ( 'NONE',  ( 0.9055118110236227702, -0.5511811023622047445, 6.969142054262312111E-17 ) ) ;
#70011=CARTESIAN_POINT ( 'NONE',  ( 1.076115485564305141, 0.2306618581243847221, -0.2411417322834647770 ) ) ;
#70012=CARTESIAN_POINT ( 'NONE',  ( 1.384514435695538337, -0.6692913385826771977, 0.1292274648535927661 ) ) ;
#70013=CARTESIAN_POINT ( 'NONE',  ( 0.2165354330708668673, -0.4536011799217367080, 0.2665933059059888421 ) ) ;
#70015=CARTESIAN_POINT ( 'NONE',  ( 0.6364829396325465405, -0.3162353388693409650, -0.4822834645669289433 ) ) ;
#70017=CARTESIAN_POINT ( 'NONE',  ( 0.4002624671916016896, -0.2845877964562161244, -0.3641732283464567121 ) ) ;
#70019=CARTESIAN_POINT ( 'NONE',  ( -1.601049868766403650, 0.2306618581243847221, -0.2411417322834647770 ) ) ;
#70020=CARTESIAN_POINT ( 'NONE',  ( -1.233595800524933894, -0.6046776061558809534, -0.2411417322834644161 ) ) ;
#70021=CARTESIAN_POINT ( 'NONE',  ( -0.6364829396325453192, -0.3162353388693405765, 0.4822834645669290543 ) ) ;
#70024=CARTESIAN_POINT ( 'NONE',  ( 0.3477690288713918276, 0.2952755905511811885, 0.1292274648535926551 ) ) ;
#70025=CARTESIAN_POINT ( 'NONE',  ( 0.9842519685039375910, 0.1771653543307087630, 0.000000000000000000 ) ) ;
#70026=CARTESIAN_POINT ( 'NONE',  ( -0.3346456692913377662, 0.1660481256975883668, -0.3530559997133364547 ) ) ;
#70027=CARTESIAN_POINT ( 'NONE',  ( 0.3083989501312343062, -0.3162353388693405765, 0.4822834645669290543 ) ) ;
#70033=CARTESIAN_POINT ( 'NONE',  ( -0.7086614173228339419, -0.1870078740157480601, -0.3641732283464567677 ) ) ;
#70034=CARTESIAN_POINT ( 'NONE',  ( -1.220472440944881054, 0.2952755905511811885, 0.000000000000000000 ) ) ;
#70036=CARTESIAN_POINT ( 'NONE',  ( 0.8464566929133866546, -0.5400638737290844871, 0.3530559997133364547 ) ) ;
#70037=CARTESIAN_POINT ( 'NONE',  ( 1.482939632545932307, 0.05413385826771626580, -0.4176697321401330321 ) ) ;
#70038=CARTESIAN_POINT ( 'NONE',  ( 0.9842519685039375910, 0.2952755905511811885, 0.000000000000000000 ) ) ;
#70042=CARTESIAN_POINT ( 'NONE',  ( 0.9383202099737536495, -0.3162353388693405765, 0.4822834645669290543 ) ) ;
#70043=CARTESIAN_POINT ( 'NONE',  ( 0.7742782152230978099, -0.4281496062992124485, 0.4176697321401328655 ) ) ;
#70044=CARTESIAN_POINT ( 'NONE',  ( 0.8464566929133865436, 0.07958543189024071263, -0.2665933059059888421 ) ) ;
#70045=CARTESIAN_POINT ( 'NONE',  ( 1.332020997375329197, -0.3162353388693405765, 0.4822834645669290543 ) ) ;
#70047=CARTESIAN_POINT ( 'NONE',  ( 1.043307086614173818, 0.1660481256975885056, 0.3530559997133364547 ) ) ;
#70048=CARTESIAN_POINT ( 'NONE',  ( 0.4396325459317593221, 0.2952755905511810774, -0.1292274648535930714 ) ) ;
#70049=CARTESIAN_POINT ( 'NONE',  ( 1.430446194225722500, -0.3690944881889765550, -0.3153832671262227771 ) ) ;
#70050=CARTESIAN_POINT ( 'NONE',  ( -0.7152230971128602510, -0.05778040916215560624, -0.4822834645669293319 ) ) ;
#70051=CARTESIAN_POINT ( 'NONE',  ( -1.167979002624671470, -0.4281496062992127816, -0.4176697321401328100 ) ) ;
#70052=AXIS2_PLACEMENT_3D ( 'NONE', #51202, #36942, #70579 ) ;
#70053=CARTESIAN_POINT ( 'NONE',  ( 1.174540682414699111, -0.05778040916215560624, -0.4822834645669293319 ) ) ;
#70059=ORIENTED_EDGE ( 'NONE', *, *, #24157, .T. ) ;
#70061=CARTESIAN_POINT ( 'NONE',  ( 1.351706036745407458, -0.3690944881889765550, -0.3153832671262227771 ) ) ;
#70063=CARTESIAN_POINT ( 'NONE',  ( 1.345144356955381593, -0.08942795157527998196, 0.3641732283464567121 ) ) ;
#70064=CARTESIAN_POINT ( 'NONE',  ( 0.4581548277944226255, 1.539554514980418620, -0.5309055118110237448 ) ) ;
#70068=CARTESIAN_POINT ( 'NONE',  ( -0.9383202099737524282, -0.2845877964562161244, -0.3641732283464567121 ) ) ;
#70069=CARTESIAN_POINT ( 'NONE',  ( -1.646981627296586703, -0.2845877964562161244, -0.3641732283464567121 ) ) ;
#70070=CARTESIAN_POINT ( 'NONE',  ( -1.194225721784776262, -0.4281496062992124485, 0.4176697321401328655 ) ) ;
#70071=CARTESIAN_POINT ( 'NONE',  ( 0.1706036745406830368, 0.05413385826771666132, 0.4176697321401328100 ) ) ;
#70072=CARTESIAN_POINT ( 'NONE',  ( -1.587926509186350810, 0.05413385826771626580, -0.4176697321401330321 ) ) ;
#70076=( LENGTH_UNIT ( ) NAMED_UNIT ( * ) SI_UNIT ( $, .METRE. ) );
#70079=CARTESIAN_POINT ( 'NONE',  ( -0.5643044619422565855, -0.3690944881889763329, 0.3153832671262228327 ) ) ;
#70080=CARTESIAN_POINT ( 'NONE',  ( -1.036745406824146176, -0.4281496062992124485, 0.4176697321401328655 ) ) ;
#70081=CARTESIAN_POINT ( 'NONE',  ( 1.122047244094488860, -0.5400638737290845981, -0.3530559997133363437 ) ) ;
#70084=CARTESIAN_POINT ( 'NONE',  ( -1.586052503253848611, 0.7480314960629931287, 0.1653254495020559378 ) ) ;
#70085=CARTESIAN_POINT ( 'NONE',  ( 1.207349081364829990, 0.2306618581243848609, 0.2411417322834645549 ) ) ;
#70086=CARTESIAN_POINT ( 'NONE',  ( -1.266404199475064773, -0.3162353388693405765, 0.4822834645669290543 ) ) ;
#70088=CARTESIAN_POINT ( 'NONE',  ( -0.4790026246719154557, -0.2845877964562159024, 0.3641732283464567677 ) ) ;
#70090=CARTESIAN_POINT ( 'NONE',  ( -0.4658792650918627265, -0.2845877964562161244, -0.3641732283464567121 ) ) ;
#70091=CARTESIAN_POINT ( 'NONE',  ( 0.3149606299212603933, -0.1870078740157479769, 0.3641732283464567677 ) ) ;
#70092=CARTESIAN_POINT ( 'NONE',  ( 0.2821522309711292364, -0.6692913385826771977, 0.1292274648535927661 ) ) ;
#70093=CARTESIAN_POINT ( 'NONE',  ( -0.7874015748031489847, -0.1870078740157480601, -0.3641732283464567677 ) ) ;
#70095=CARTESIAN_POINT ( 'NONE',  ( 0.9908136482939640111, 0.2952755905511810774, -0.1292274648535930714 ) ) ;
#70096=ADVANCED_FACE ( 'NONE', ( #17103 ), #51958, .F. ) ;
#70097=ADVANCED_FACE ( 'NONE', ( #26321 ), #68696, .F. ) ;
#70098=CARTESIAN_POINT ( 'NONE',  ( -1.384514435695537005, -0.6692913385826773087, -0.1292274648535924053 ) ) ;
#70100=CARTESIAN_POINT ( 'NONE',  ( -0.5774278215223089816, 0.2306618581243847221, -0.2411417322834647770 ) ) ;
#70101=CARTESIAN_POINT ( 'NONE',  ( -1.102362204724408601, -0.1870078740157480879, -0.4822834645669291653 ) ) ;
#70102=CARTESIAN_POINT ( 'NONE',  ( 1.115485564304462551, -0.3690944881889765550, -0.3153832671262227771 ) ) ;
#70103=CARTESIAN_POINT ( 'NONE',  ( -0.2493438320209966919, -0.004921259842519870586, -0.3153832671262229437 ) ) ;
#70104=CARTESIAN_POINT ( 'NONE',  ( -0.8070866141732276899, -0.5400638737290844871, 0.3530559997133364547 ) ) ;
#70105=CARTESIAN_POINT ( 'NONE',  ( -1.266404199475064773, -0.05778040916215560624, -0.4822834645669293319 ) ) ;
#70106=DIRECTION ( 'NONE',  ( -1.000000000000000000, 0.000000000000000000, 0.000000000000000000 ) ) ;
#70107=CARTESIAN_POINT ( 'NONE',  ( 1.279527559055118724, -0.4536011799217368745, -0.2665933059059886201 ) ) ;
#70108=CARTESIAN_POINT ( 'NONE',  ( -0.2559055118110227234, -0.5400638737290844871, 0.3530559997133364547 ) ) ;
#70110=CARTESIAN_POINT ( 'NONE',  ( -1.213910761154854745, 0.2952755905511810774, -0.1292274648535930714 ) ) ;
#70113=CARTESIAN_POINT ( 'NONE',  ( -0.7086614173228339419, -0.1870078740157479769, 0.3641732283464567677 ) ) ;
#70114=CARTESIAN_POINT ( 'NONE',  ( 1.207349081364829990, -0.6046776061558809534, -0.2411417322834644161 ) ) ;
#70115=CARTESIAN_POINT ( 'NONE',  ( -1.122047244094487306, -0.4536011799217367080, 0.2665933059059888421 ) ) ;
#70117=CARTESIAN_POINT ( 'NONE',  ( -0.8989501312335946848, 0.2952755905511810774, -0.1292274648535930714 ) ) ;
#70118=CARTESIAN_POINT ( 'NONE',  ( 0.8661417322834653598, -0.1870078740157479769, 0.4822834645669291653 ) ) ;
#70119=CARTESIAN_POINT ( 'NONE',  ( 0.9711286089238851948, -0.6046776061558809534, -0.2411417322834644161 ) ) ;
#70120=CARTESIAN_POINT ( 'NONE',  ( 1.541994750656168645, -0.6692913385826771977, 0.1292274648535927661 ) ) ;
#70121=CARTESIAN_POINT ( 'NONE',  ( -1.371391076115484831, 0.1771653543307087075, -0.09757992244046823083 ) ) ;
#70126=CARTESIAN_POINT ( 'NONE',  ( 1.174540682414699111, -0.2845877964562159024, 0.3641732283464567677 ) ) ;
#70127=CARTESIAN_POINT ( 'NONE',  ( 0.8858267716535438430, -0.4536011799217368745, -0.2665933059059886201 ) ) ;
#70128=CARTESIAN_POINT ( 'NONE',  ( 0.4068241469816279987, -0.4281496062992127816, -0.4176697321401328100 ) ) ;
#70129=CARTESIAN_POINT ( 'NONE',  ( 1.614173228346457378, 0.2952755905511811885, 0.000000000000000000 ) ) ;
#70131=CARTESIAN_POINT ( 'NONE',  ( 0.6692913385826778638, -0.5511811023622047445, 6.969142054262312111E-17 ) ) ;
#70132=CARTESIAN_POINT ( 'NONE',  ( -0.2099737532808391705, 0.2306618581243848609, 0.2411417322834645549 ) ) ;
#70133=CARTESIAN_POINT ( 'NONE',  ( -1.272965879265091305, 0.05413385826771626580, -0.4176697321401330321 ) ) ;
#70134=CARTESIAN_POINT ( 'NONE',  ( 0.8333333333333340365, -0.6692913385826771977, 0.1292274648535927661 ) ) ;
#70137=ORIENTED_EDGE ( 'NONE', *, *, #31689, .F. ) ;
#70138=ORIENTED_EDGE ( 'NONE', *, *, #73756, .T. ) ;
#70139=CARTESIAN_POINT ( 'NONE',  ( -1.135170603674539924, -0.6692913385826771977, 0.1292274648535927661 ) ) ;
#70140=CARTESIAN_POINT ( 'NONE',  ( -0.4986876640419939388, 0.2306618581243847221, -0.2411417322834647770 ) ) ;
#70141=CARTESIAN_POINT ( 'NONE',  ( -0.7480314960629914633, -0.5511811023622047445, 6.969142054262312111E-17 ) ) ;
#70142=CARTESIAN_POINT ( 'NONE',  ( -0.6364829396325453192, -0.05778040916215560624, -0.4822834645669293319 ) ) ;
#70144=CARTESIAN_POINT ( 'NONE',  ( 0.5643044619422579178, 0.05413385826771666132, 0.4176697321401328100 ) ) ;
#70145=CARTESIAN_POINT ( 'NONE',  ( -0.2493438320209966919, -0.4281496062992124485, 0.4176697321401328655 ) ) ;
#70146=CARTESIAN_POINT ( 'NONE',  ( -1.620734908136482577, 0.2952755905511811885, 0.1292274648535926551 ) ) ;
#70147=CARTESIAN_POINT ( 'NONE',  ( -0.7874015748031489847, -0.1870078740157479769, 0.4822834645669291653 ) ) ;
#70148=CARTESIAN_POINT ( 'NONE',  ( 0.4002624671916016896, -0.3162353388693409650, -0.4822834645669289433 ) ) ;
#70149=ADVANCED_FACE ( 'NONE', ( #8608 ), #2593, .F. ) ;
#70151=CARTESIAN_POINT ( 'NONE',  ( -0.9776902887139098386, 0.1771653543307087075, -0.09757992244046823083 ) ) ;
#70155=CARTESIAN_POINT ( 'NONE',  ( -1.443569553805773564, -0.5023911411419708095, 0.1820866141732285504 ) ) ;
#70156=CARTESIAN_POINT ( 'NONE',  ( -1.036745406824146176, -0.4281496062992124485, 0.4176697321401328655 ) ) ;
#70157=CARTESIAN_POINT ( 'NONE',  ( -0.6824146981627288167, 0.2306618581243848609, 0.2411417322834645549 ) ) ;
#70159=CARTESIAN_POINT ( 'NONE',  ( -1.030183727034119867, -0.05778040916215560624, -0.4822834645669293319 ) ) ;
#70160=CARTESIAN_POINT ( 'NONE',  ( -1.095800524934382292, -0.05778040916215522460, 0.4822834645669289988 ) ) ;
#70161=CARTESIAN_POINT ( 'NONE',  ( -1.220472440944881054, 2.362204724409448620, 0.5309055118110237448 ) ) ;
#70163=CARTESIAN_POINT ( 'NONE',  ( 0.6889763779527566800, -0.4536011799217367080, 0.2665933059059888421 ) ) ;
#70166=CARTESIAN_POINT ( 'NONE',  ( -0.5577427821522301654, -0.08942795157528024563, -0.3641732283464568787 ) ) ;
#70167=CARTESIAN_POINT ( 'NONE',  ( -0.2493438320209966919, -0.4281496062992124485, 0.4176697321401328655 ) ) ;
#70168=CARTESIAN_POINT ( 'NONE',  ( 1.548556430446194954, -0.6046776061558807314, 0.2411417322834647770 ) ) ;
#70169=CARTESIAN_POINT ( 'NONE',  ( -0.4527559055118102749, -0.5400638737290845981, -0.3530559997133363437 ) ) ;
#70173=CARTESIAN_POINT ( 'NONE',  ( -0.5314960629921250401, 0.1660481256975885056, 0.3530559997133364547 ) ) ;
#70175=CARTESIAN_POINT ( 'NONE',  ( 1.095800524934383846, -0.3162353388693405765, 0.4822834645669290543 ) ) ;
#70176=CARTESIAN_POINT ( 'NONE',  ( -1.089238845144356427, -0.004921259842519576551, 0.3153832671262227771 ) ) ;
#70177=CARTESIAN_POINT ( 'NONE',  ( -1.292650918635170010, -0.6692913385826771977, 0.1292274648535927661 ) ) ;
#70179=LINE ( 'NONE', #76919, #76120 ) ;
#70181=CARTESIAN_POINT ( 'NONE',  ( 1.587926509186352142, 0.05413385826771666132, 0.4176697321401328100 ) ) ;
#70183=CARTESIAN_POINT ( 'NONE',  ( 0.02624671916010564918, -0.6046776061558809534, -0.2411417322834644161 ) ) ;
#70184=CARTESIAN_POINT ( 'NONE',  ( -1.056430446194224881, -0.5511811023622046335, 0.09757992244046803654 ) ) ;
#70185=CARTESIAN_POINT ( 'NONE',  ( -0.2887139107611542133, 0.2306618581243848609, 0.2411417322834645549 ) ) ;
#70187=CARTESIAN_POINT ( 'NONE',  ( -0.6889763779527552368, -0.5400638737290845981, -0.3530559997133363437 ) ) ;
#70188=CARTESIAN_POINT ( 'NONE',  ( -1.207349081364828880, 0.2306618581243847221, -0.2411417322834647770 ) ) ;
#70190=CARTESIAN_POINT ( 'NONE',  ( 0.9448818897637802916, -0.1870078740157479769, 0.3641732283464567677 ) ) ;
#70191=CARTESIAN_POINT ( 'NONE',  ( -0.6299212598425188991, -0.1870078740157479769, 0.3641732283464567677 ) ) ;
#70192=CARTESIAN_POINT ( 'NONE',  ( 0.9251968503937015864, 0.07958543189024071263, -0.2665933059059888421 ) ) ;
#70193=CARTESIAN_POINT ( 'NONE',  ( -1.568241469816272105, -0.05778040916215522460, 0.4822834645669289988 ) ) ;
#70194=CARTESIAN_POINT ( 'NONE',  ( 1.286089238845145033, 0.2306618581243848609, 0.2411417322834645549 ) ) ;
#70195=CARTESIAN_POINT ( 'NONE',  ( 0.3740157480314966754, -0.4536011799217367080, 0.2665933059059888421 ) ) ;
#70196=CARTESIAN_POINT ( 'NONE',  ( -0.7414698162729651543, -0.6692913385826771977, 0.1292274648535927661 ) ) ;
#70197=CARTESIAN_POINT ( 'NONE',  ( 1.272965879265092637, 0.05413385826771666132, 0.4176697321401328100 ) ) ;
#70199=CARTESIAN_POINT ( 'NONE',  ( -0.2230971128608915943, -0.004921259842519576551, 0.3153832671262227771 ) ) ;
#70201=CARTESIAN_POINT ( 'NONE',  ( 0.4002624671916016896, -0.05778040916215522460, 0.4822834645669289988 ) ) ;
#70202=CARTESIAN_POINT ( 'NONE',  ( 0.9776902887139113929, 0.1771653543307087630, 0.09757992244046791164 ) ) ;
#70203=CARTESIAN_POINT ( 'NONE',  ( 0.03937007874015806264, 0.1771653543307087630, 0.000000000000000000 ) ) ;
#70204=CARTESIAN_POINT ( 'NONE',  ( -1.535433070866141225, 0.2952755905511811885, 0.000000000000000000 ) ) ;
#70206=CARTESIAN_POINT ( 'NONE',  ( -0.8005249343832011588, -0.004921259842519870586, -0.3153832671262229437 ) ) ;
#70207=DIRECTION ( 'NONE',  ( -0.000000000000000000, -1.000000000000000000, -0.000000000000000000 ) ) ;
#70208=CARTESIAN_POINT ( 'NONE',  ( -1.187664041994750175, -0.05778040916215560624, -0.4822834645669293319 ) ) ;
#70209=CARTESIAN_POINT ( 'NONE',  ( -0.6364829396325453192, -0.05778040916215560624, -0.4822834645669293319 ) ) ;
#70212=CARTESIAN_POINT ( 'NONE',  ( 0.2165354330708668673, 0.07958543189024071263, -0.2665933059059888421 ) ) ;
#70213=CARTESIAN_POINT ( 'NONE',  ( -0.4330708661417315697, -0.6692913385826771977, 8.415575281601705876E-17 ) ) ;
#70214=CARTESIAN_POINT ( 'NONE',  ( -0.7808398950131222316, -0.3162353388693409650, -0.4822834645669289433 ) ) ;
#70215=CARTESIAN_POINT ( 'NONE',  ( -0.6889763779527552368, 0.07958543189024085140, 0.2665933059059887866 ) ) ;
#70217=CARTESIAN_POINT ( 'NONE',  ( 0.01968503937007957949, -0.5400638737290845981, -0.3530559997133363437 ) ) ;
#70219=CARTESIAN_POINT ( 'NONE',  ( -1.489501312335957062, -0.2845877964562161244, -0.3641732283464567121 ) ) ;
#70220=CARTESIAN_POINT ( 'NONE',  ( 1.259842519685040019, -0.1870078740157479769, 0.4822834645669291653 ) ) ;
#70225=EDGE_CURVE ( 'NONE', #4976, #11614, #60594, .T. ) ;
#70227=CARTESIAN_POINT ( 'NONE',  ( -1.476377952755905110, -0.5400638737290845981, -0.3530559997133363437 ) ) ;
#70228=CARTESIAN_POINT ( 'NONE',  ( -0.8464566929133852113, -0.5400638737290845981, -0.3530559997133363437 ) ) ;
#70229=CARTESIAN_POINT ( 'NONE',  ( -1.515748031496062076, -0.5400638737290844871, 0.3530559997133364547 ) ) ;
#70231=DIRECTION ( 'NONE',  ( 0.000000000000000000, -1.000000000000000000, 0.000000000000000000 ) ) ;
#70232=CARTESIAN_POINT ( 'NONE',  ( 0.8727034120734913358, -0.05778040916215522460, 0.4822834645669289988 ) ) ;
#70233=CARTESIAN_POINT ( 'NONE',  ( 0.2034120734908144990, -0.6692913385826771977, 0.1292274648535927661 ) ) ;
#70234=CARTESIAN_POINT ( 'NONE',  ( -0.3252997568826541674, -5.134928753749862370E-15, -0.4281989832122467532 ) ) ;
#70236=CARTESIAN_POINT ( 'NONE',  ( 1.312335958005249825, 0.1283753931104746893, -0.1820866141732285504 ) ) ;
#70238=VERTEX_POINT ( 'NONE', #82438 ) ;
#70241=CARTESIAN_POINT ( 'NONE',  ( -0.1312335958005241554, 0.2306618581243848609, 0.2411417322834645549 ) ) ;
#70242=CARTESIAN_POINT ( 'NONE',  ( -0.7283464566929126471, 0.1660481256975883668, -0.3530559997133364547 ) ) ;
#70243=CARTESIAN_POINT ( 'NONE',  ( -1.489501312335957062, -0.05778040916215522460, 0.4822834645669289988 ) ) ;
#70244=CARTESIAN_POINT ( 'NONE',  ( 0.6167979002624679463, 0.05413385826771626580, -0.4176697321401330321 ) ) ;
#70245=CARTESIAN_POINT ( 'NONE',  ( 1.489501312335958172, -0.3162353388693405765, 0.4822834645669290543 ) ) ;
#70247=CARTESIAN_POINT ( 'NONE',  ( 0.006561679790026889343, -0.3162353388693409650, -0.4822834645669289433 ) ) ;
#70248=CARTESIAN_POINT ( 'NONE',  ( -1.102362204724408601, -0.1870078740157480879, -0.4822834645669291653 ) ) ;
#70249=CARTESIAN_POINT ( 'NONE',  ( 1.522309711286089939, -0.6046776061558809534, -0.2411417322834644161 ) ) ;
#70251=CARTESIAN_POINT ( 'NONE',  ( 1.502624671916010790, -0.05778040916215522460, 0.4822834645669289988 ) ) ;
#70252=CARTESIAN_POINT ( 'NONE',  ( 0.006561679790026889343, -0.05778040916215522460, 0.4822834645669289988 ) ) ;
#70254=CARTESIAN_POINT ( 'NONE',  ( 0.3083989501312343062, -0.08942795157528024563, -0.3641732283464568787 ) ) ;
#70255=ORIENTED_EDGE ( 'NONE', *, *, #14652, .F. ) ;
#70257=ORIENTED_EDGE ( 'NONE', *, *, #40280, .F. ) ;
#70258=CARTESIAN_POINT ( 'NONE',  ( 0.08530183727034192087, -0.2845877964562161244, -0.3641732283464567121 ) ) ;
#70260=CARTESIAN_POINT ( 'NONE',  ( -0.006561679790025524116, -0.3162353388693405765, 0.4822834645669290543 ) ) ;
#70261=CARTESIAN_POINT ( 'NONE',  ( -0.1115485564304456306, 0.2952755905511810774, -0.1292274648535930714 ) ) ;
#70262=CARTESIAN_POINT ( 'NONE',  ( -0.4593175853018366950, 0.05413385826771666132, 0.4176697321401328100 ) ) ;
#70265=CARTESIAN_POINT ( 'NONE',  ( -1.010498687664041384, 0.05413385826771666132, 0.4176697321401328100 ) ) ;
#70267=CARTESIAN_POINT ( 'NONE',  ( 1.141732283464567566, 0.1771653543307087630, 0.000000000000000000 ) ) ;
#70269=CARTESIAN_POINT ( 'NONE',  ( 0.9776902887139113929, -0.6692913385826773087, -0.1292274648535924053 ) ) ;
#70270=CARTESIAN_POINT ( 'NONE',  ( 0.7217847769028878924, 0.05413385826771666132, 0.4176697321401328100 ) ) ;
#70272=CARTESIAN_POINT ( 'NONE',  ( -1.279527559055116948, -0.5400638737290844871, 0.3530559997133364547 ) ) ;
#70275=CARTESIAN_POINT ( 'NONE',  ( 0.03937007874015806264, 0.2952755905511811885, 0.000000000000000000 ) ) ;
#70279=CARTESIAN_POINT ( 'NONE',  ( 1.377952755905512472, -0.6692913385826771977, 8.415575281601705876E-17 ) ) ;
#70280=CARTESIAN_POINT ( 'NONE',  ( 1.364829396325460076, 0.2306618581243848609, 0.2411417322834645549 ) ) ;
#70281=CARTESIAN_POINT ( 'NONE',  ( 0.3674540682414705883, -0.5023911411419708095, 0.1820866141732285504 ) ) ;
#70282=CARTESIAN_POINT ( 'NONE',  ( 1.049868766404200127, -0.6046776061558809534, -0.2411417322834644161 ) ) ;
#70284=CARTESIAN_POINT ( 'NONE',  ( 0.5380577427821529035, -0.3690944881889763329, 0.3153832671262228327 ) ) ;
#70285=CARTESIAN_POINT ( 'NONE',  ( 0.1837270341207354329, 0.2306618581243848609, 0.2411417322834645549 ) ) ;
#70288=CARTESIAN_POINT ( 'NONE',  ( -1.377952755905511140, 0.2952755905511811885, 0.000000000000000000 ) ) ;
#70289=CARTESIAN_POINT ( 'NONE',  ( 1.076115485564305141, -0.5023911411419708095, 0.1820866141732285504 ) ) ;
#70291=CARTESIAN_POINT ( 'NONE',  ( -0.4199475065616791736, 0.2306618581243847221, -0.2411417322834647770 ) ) ;
#70292=CARTESIAN_POINT ( 'NONE',  ( -0.1115485564304453947, -0.5511811023622046335, 0.09757992244046803654 ) ) ;
#70293=CARTESIAN_POINT ( 'NONE',  ( 0.4556365106396694786, 1.773775493036639617, 0.5309055118110234117 ) ) ;
#70294=CARTESIAN_POINT ( 'NONE',  ( -0.1640419947506555343, -0.3162353388693405765, 0.4822834645669290543 ) ) ;
#70295=CARTESIAN_POINT ( 'NONE',  ( 0.1377952755905518800, -0.4536011799217367080, 0.2665933059059888421 ) ) ;
#70297=CARTESIAN_POINT ( 'NONE',  ( -0.006561679790025524116, -0.05778040916215560624, -0.4822834645669293319 ) ) ;
#70298=( BOUNDED_CURVE ( )  B_SPLINE_CURVE ( 2, ( #53046, #27808, #77494, #13945, #79178, #39602, #19830, #7630, #40850, #40028, #58962, #71176, #32868 ),
 .UNSPECIFIED., .F., .F. ) 
 B_SPLINE_CURVE_WITH_KNOTS ( ( 3, 2, 2, 2, 2, 2, 3 ),
 ( 0.7187856400893463116, 0.7196969696969697239, 0.7234848484848485084, 0.7272727272727272929, 0.7310606060606060774, 0.7348484848484848619, 0.7357598144561083853 ),
 .UNSPECIFIED. ) 
 CURVE ( )  GEOMETRIC_REPRESENTATION_ITEM ( )  RATIONAL_B_SPLINE_CURVE ( ( 0.9875488213027523443, 0.9918020599134680371, 1.000000000000000000, 0.9659258262890683122, 1.000000000000000000, 0.9659258262890683122, 1.000000000000000000, 0.9659258262890683122, 1.000000000000000000, 0.9659258262890683122, 1.000000000000000000, 0.9918020599134671489, 0.9875488213027514561 ) ) 
 REPRESENTATION_ITEM ( '' )  );
#70300=CARTESIAN_POINT ( 'NONE',  ( 1.286089238845145033, -0.5023911411419708095, -0.1820866141732282451 ) ) ;
#70301=CARTESIAN_POINT ( 'NONE',  ( -1.112371124080194340, -2.567464376874931580E-15, -0.4445507791589072832 ) ) ;
#70302=CARTESIAN_POINT ( 'NONE',  ( -0.9448818897637790704, -0.1870078740157479769, 0.3641732283464567677 ) ) ;
#70303=CARTESIAN_POINT ( 'NONE',  ( -0.6955380577427815458, -0.3690944881889765550, -0.3153832671262227771 ) ) ;
#70304=CARTESIAN_POINT ( 'NONE',  ( -0.2296587926509179312, -0.05778040916215522460, 0.4822834645669289988 ) ) ;
#70305=CARTESIAN_POINT ( 'NONE',  ( -0.2559055118110230564, 0.1660481256975883668, -0.3530559997133364547 ) ) ;
#70306=CARTESIAN_POINT ( 'NONE',  ( 0.5839895013123367340, 0.1771653543307087630, 0.09757992244046791164 ) ) ;
#70308=CARTESIAN_POINT ( 'NONE',  ( 1.397637795275591177, -0.4536011799217367080, 0.2665933059059888421 ) ) ;
#70309=CARTESIAN_POINT ( 'NONE',  ( 0.6955380577427828781, -0.4281496062992124485, 0.4176697321401328655 ) ) ;
#70311=CARTESIAN_POINT ( 'NONE',  ( -0.3412073490813641308, -0.6046776061558807314, 0.2411417322834647770 ) ) ;
#70313=CARTESIAN_POINT ( 'NONE',  ( -1.377952755905511140, 0.2952755905511811885, 0.000000000000000000 ) ) ;
#70314=CARTESIAN_POINT ( 'NONE',  ( 0.9645669291338591078, -0.5400638737290845981, -0.3530559997133363437 ) ) ;
#70315=CARTESIAN_POINT ( 'NONE',  ( 0.3871391076115493490, -0.3162353388693405765, 0.4822834645669290543 ) ) ;
#70317=CARTESIAN_POINT ( 'NONE',  ( 0.2099737532808405305, -0.5023911411419708095, 0.1820866141732285504 ) ) ;
#70318=CARTESIAN_POINT ( 'NONE',  ( 1.318897637795276356, -0.5400638737290844871, 0.3530559997133364547 ) ) ;
#70319=EDGE_CURVE ( 'NONE', #22642, #44890, #30674, .T. ) ;
#70320=CARTESIAN_POINT ( 'NONE',  ( -0.5052493438320203589, -0.5511811023622046335, 0.09757992244046803654 ) ) ;
#70321=CARTESIAN_POINT ( 'NONE',  ( -0.8267716535433065062, 0.2952755905511811885, 0.000000000000000000 ) ) ;
#70323=CARTESIAN_POINT ( 'NONE',  ( 0.3805774278215230400, 0.05413385826771626580, -0.4176697321401330321 ) ) ;
#70324=CARTESIAN_POINT ( 'NONE',  ( -0.8792650918635160906, -0.4281496062992124485, 0.4176697321401328655 ) ) ;
#70325=CARTESIAN_POINT ( 'NONE',  ( -0.7349081364829390672, 0.1283753931104746893, -0.1820866141732285504 ) ) ;
#70326=CARTESIAN_POINT ( 'NONE',  ( 0.2165354330708668673, 0.1660481256975883668, -0.3530559997133364547 ) ) ;
#70327=CARTESIAN_POINT ( 'NONE',  ( -1.240157480314959759, 0.1660481256975885056, 0.3530559997133364547 ) ) ;
#70328=CARTESIAN_POINT ( 'NONE',  ( -0.1443569553805765515, -0.4281496062992127816, -0.4176697321401328100 ) ) ;
#70329=CARTESIAN_POINT ( 'NONE',  ( 1.141732283464567788, 0.2066929133858268208, 0.000000000000000000 ) ) ;
#70331=CARTESIAN_POINT ( 'NONE',  ( 1.167979002624672580, 0.05413385826771626580, -0.4176697321401330321 ) ) ;
#70332=CARTESIAN_POINT ( 'NONE',  ( 1.148293963254593875, -0.6692913385826771977, 0.1292274648535927661 ) ) ;
#70334=CARTESIAN_POINT ( 'NONE',  ( -1.220472440944878834, 2.362204724409448620, -0.5309055118110234117 ) ) ;
#70335=CARTESIAN_POINT ( 'NONE',  ( -0.9645669291338575535, -0.5400638737290844871, 0.3530559997133364547 ) ) ;
#70336=B_SPLINE_CURVE_WITH_KNOTS ( 'NONE', 3,
 ( #67143, #67971, #3577, #67555 ),
 .UNSPECIFIED., .F., .F.,
 ( 4, 4 ),
 ( 3.593986969192262371E-07, 0.001287825409103155903 ),
 .UNSPECIFIED. ) ;
#70340=CARTESIAN_POINT ( 'NONE',  ( -0.006561679790025524116, -0.08942795157528024563, -0.3641732283464568787 ) ) ;
#70343=CARTESIAN_POINT ( 'NONE',  ( 0.8005249343832027131, 0.05413385826771666132, 0.4176697321401328100 ) ) ;
#70346=CARTESIAN_POINT ( 'NONE',  ( -0.5511811023622038563, -0.1870078740157479769, 0.3641732283464567677 ) ) ;
#70347=CARTESIAN_POINT ( 'NONE',  ( 1.377952755905512472, 0.2952755905511811885, 0.000000000000000000 ) ) ;
#70348=CARTESIAN_POINT ( 'NONE',  ( 0.8070866141732288002, 0.07958543189024085140, 0.2665933059059887866 ) ) ;
#70349=CARTESIAN_POINT ( 'NONE',  ( -0.1509186351706028884, -0.3162353388693409650, -0.4822834645669289433 ) ) ;
#70351=CARTESIAN_POINT ( 'NONE',  ( -0.9908136482939626788, 0.2952755905511811885, 0.1292274648535926551 ) ) ;
#70352=CARTESIAN_POINT ( 'NONE',  ( -1.246719160104986512, -0.004921259842519576551, 0.3153832671262227771 ) ) ;
#70353=CARTESIAN_POINT ( 'NONE',  ( -0.3740157480314953431, -0.5400638737290845981, -0.3530559997133363437 ) ) ;
#70354=CARTESIAN_POINT ( 'NONE',  ( -1.614173228346456712, 2.401574803149606474, -0.1372047244094478091 ) ) ;
#70355=CARTESIAN_POINT ( 'NONE',  ( 0.6414174258557936437, -2.592014407703319119E-15, 0.3791475997938231202 ) ) ;
#70358=CARTESIAN_POINT ( 'NONE',  ( 0.4986876640419954376, -0.6046776061558809534, -0.2411417322834644161 ) ) ;
#70360=CARTESIAN_POINT ( 'NONE',  ( -0.8464566929133852113, -0.5400638737290845981, -0.3530559997133363437 ) ) ;
#70361=CARTESIAN_POINT ( 'NONE',  ( 1.463254593175853824, 0.2952755905511810774, -0.1292274648535930714 ) ) ;
#70362=CARTESIAN_POINT ( 'NONE',  ( 0.8530183727034126306, 0.05413385826771626580, -0.4176697321401330321 ) ) ;
#70363=CARTESIAN_POINT ( 'NONE',  ( 0.07217847769028949700, -0.3162353388693405765, 0.4822834645669290543 ) ) ;
#70365=CARTESIAN_POINT ( 'NONE',  ( -0.7742782152230965886, 0.05413385826771666132, 0.4176697321401328100 ) ) ;
#70366=CARTESIAN_POINT ( 'NONE',  ( -0.3280839895013117347, 0.05413385826771626580, -0.4176697321401330321 ) ) ;
#70367=CARTESIAN_POINT ( 'NONE',  ( -0.8267716535433065062, 0.2952755905511811885, 0.000000000000000000 ) ) ;
#70368=CARTESIAN_POINT ( 'NONE',  ( -0.1049868766404193215, -0.5023911411419708095, 0.1820866141732285504 ) ) ;
#70370=CARTESIAN_POINT ( 'NONE',  ( -0.2493438320209966919, 0.05413385826771626580, -0.4176697321401330321 ) ) ;
#70372=CARTESIAN_POINT ( 'NONE',  ( 1.220472440944882386, -0.6692913385826771977, 8.415575281601705876E-17 ) ) ;
#70373=CARTESIAN_POINT ( 'NONE',  ( 0.4848604877838280647, 0.000000000000000000, 0.3464511005275205946 ) ) ;
#70376=CARTESIAN_POINT ( 'NONE',  ( 0.1312335958005257930, 0.2306618581243847221, -0.2411417322834647770 ) ) ;
#70377=CARTESIAN_POINT ( 'NONE',  ( -0.4330708661417315697, 0.1771653543307087630, 0.000000000000000000 ) ) ;
#70378=CARTESIAN_POINT ( 'NONE',  ( 1.305774278215223960, -0.5511811023622046335, 0.09757992244046803654 ) ) ;
#70382=CARTESIAN_POINT ( 'NONE',  ( 1.456692913385827515, -0.5511811023622047445, 6.969142054262312111E-17 ) ) ;
#70383=CARTESIAN_POINT ( 'NONE',  ( 1.482939632545932307, 0.05413385826771626580, -0.4176697321401330321 ) ) ;
#70385=CARTESIAN_POINT ( 'NONE',  ( -0.08530183727034056085, -0.05778040916215560624, -0.4822834645669293319 ) ) ;
#70386=CARTESIAN_POINT ( 'NONE',  ( -1.266404199475064773, -0.05778040916215560624, -0.4822834645669293319 ) ) ;
#70387=AXIS2_PLACEMENT_3D ( 'NONE', #79884, #34001, #73972 ) ;
#70388=CARTESIAN_POINT ( 'NONE',  ( -1.122047244094487306, -0.5400638737290844871, 0.3530559997133364547 ) ) ;
#70389=CARTESIAN_POINT ( 'NONE',  ( 0.1115485564304467270, -0.6692913385826773087, -0.1292274648535924053 ) ) ;
#70391=CARTESIAN_POINT ( 'NONE',  ( 1.673228346456693494, 0.1660481256975885056, 0.3530559997133364547 ) ) ;
#70392=CARTESIAN_POINT ( 'NONE',  ( 0.8267716535433077274, 0.2952755905511811885, 0.000000000000000000 ) ) ;
#70393=CARTESIAN_POINT ( 'NONE',  ( 1.266404199475066328, -0.2845877964562161244, -0.3641732283464567121 ) ) ;
#70394=CARTESIAN_POINT ( 'NONE',  ( 0.4606732211678798428, 1.541615089183433485, -0.5309055118110237448 ) ) ;
#70395=CARTESIAN_POINT ( 'NONE',  ( 0.7677165354330716118, 0.07958543189024071263, -0.2665933059059888421 ) ) ;
#70396=CARTESIAN_POINT ( 'NONE',  ( -1.423884514435694859, -0.05778040916215560624, -0.4822834645669293319 ) ) ;
#70398=CARTESIAN_POINT ( 'NONE',  ( 1.089238845144357759, 0.05413385826771626580, -0.4176697321401330321 ) ) ;
#70400=CARTESIAN_POINT ( 'NONE',  ( 0.6102362204724416372, 0.1660481256975883668, -0.3530559997133364547 ) ) ;
#70401=DIRECTION ( 'NONE',  ( 2.956072690630991733E-16, -1.000000000000000000, -5.002896285981958034E-32 ) ) ;
#70402=CARTESIAN_POINT ( 'NONE',  ( -1.496062992125983815, -0.1870078740157480601, -0.3641732283464567677 ) ) ;
#70403=CARTESIAN_POINT ( 'NONE',  ( -0.1181102362204717315, -0.6692913385826771977, 8.415575281601705876E-17 ) ) ;
#70404=CARTESIAN_POINT ( 'NONE',  ( 0.8202099737532813073, 0.1771653543307087630, 0.09757992244046791164 ) ) ;
#70406=CARTESIAN_POINT ( 'NONE',  ( 0.7874015748031503170, -0.1870078740157480879, -0.4822834645669291653 ) ) ;
#70407=CARTESIAN_POINT ( 'NONE',  ( -0.5395952360118024815, 0.02791078216816064370, 0.4328096321851915285 ) ) ;
#70408=CARTESIAN_POINT ( 'NONE',  ( -0.4593175853018366950, -0.004921259842519576551, 0.3153832671262227771 ) ) ;
#70409=CARTESIAN_POINT ( 'NONE',  ( -0.4068241469816267775, 0.05413385826771626580, -0.4176697321401330321 ) ) ;
#70410=CARTESIAN_POINT ( 'NONE',  ( 1.686351706036745890, 0.2952755905511811885, 0.1292274648535926551 ) ) ;
#70411=CARTESIAN_POINT ( 'NONE',  ( -1.332020997375327642, -0.3162353388693409650, -0.4822834645669289433 ) ) ;
#70412=CARTESIAN_POINT ( 'NONE',  ( 0.9711286089238851948, -0.6046776061558809534, -0.2411417322834644161 ) ) ;
#70414=CARTESIAN_POINT ( 'NONE',  ( -1.450131233595799651, 0.1771653543307087075, -0.09757992244046823083 ) ) ;
#70417=CARTESIAN_POINT ( 'NONE',  ( 0.9645669291338588858, 0.1660481256975885056, 0.3530559997133364547 ) ) ;
#70419=CARTESIAN_POINT ( 'NONE',  ( -1.541994750656167090, 0.2952755905511811885, 0.1292274648535926551 ) ) ;
#70420=CARTESIAN_POINT ( 'NONE',  ( -1.430446194225720724, -0.004921259842519870586, -0.3153832671262229437 ) ) ;
#70421=CARTESIAN_POINT ( 'NONE',  ( -1.036745406824146176, -0.004921259842519870586, -0.3153832671262229437 ) ) ;
#70422=CARTESIAN_POINT ( 'NONE',  ( -0.2952755905511803003, -0.5400638737290845981, -0.3530559997133363437 ) ) ;
#70423=CARTESIAN_POINT ( 'NONE',  ( -0.3018372703412066094, -0.3690944881889765550, -0.3153832671262227771 ) ) ;
#70424=CARTESIAN_POINT ( 'NONE',  ( -1.673228346456691717, 0.07958543189024071263, -0.2665933059059888421 ) ) ;
#70425=CARTESIAN_POINT ( 'NONE',  ( 0.9973753280839902091, 0.1283753931104746893, -0.1820866141732285504 ) ) ;
#70426=CARTESIAN_POINT ( 'NONE',  ( 0.6102362204724416372, 0.1660481256975883668, -0.3530559997133364547 ) ) ;
#70427=CARTESIAN_POINT ( 'NONE',  ( 1.377952755905512472, -0.6692913385826771977, 8.415575281601705876E-17 ) ) ;
#70428=CARTESIAN_POINT ( 'NONE',  ( -0.1377952755905504645, -0.4536011799217368745, -0.2665933059059886201 ) ) ;
#70429=CARTESIAN_POINT ( 'NONE',  ( 0.3805774278215230400, -0.4281496062992124485, 0.4176697321401328655 ) ) ;
#70430=CARTESIAN_POINT ( 'NONE',  ( 0.4265091863517067039, -0.5511811023622048555, -0.09757992244046775898 ) ) ;
#70431=CARTESIAN_POINT ( 'NONE',  ( -1.633858267716534529, 0.1660481256975885056, 0.3530559997133364547 ) ) ;
#70432=CARTESIAN_POINT ( 'NONE',  ( -1.135170603674539924, 0.2952755905511810774, -0.1292274648535930714 ) ) ;
#70433=CARTESIAN_POINT ( 'NONE',  ( -0.5446194225721777693, -0.3162353388693409650, -0.4822834645669289433 ) ) ;
#70436=CARTESIAN_POINT ( 'NONE',  ( 0.5708661417322841158, -0.5400638737290845981, -0.3530559997133363437 ) ) ;
#70437=CARTESIAN_POINT ( 'NONE',  ( 1.128608923884514947, 0.1283753931104748280, 0.1820866141732283561 ) ) ;
#70438=CARTESIAN_POINT ( 'NONE',  ( -0.5839895013123351797, -0.6692913385826771977, 0.1292274648535927661 ) ) ;
#70439=CARTESIAN_POINT ( 'NONE',  ( 0.5577427821522314977, -0.3162353388693409650, -0.4822834645669289433 ) ) ;
#70446=CARTESIAN_POINT ( 'NONE',  ( -1.069553805774277722, 0.1771653543307087630, 0.09757992244046791164 ) ) ;
#70447=CARTESIAN_POINT ( 'NONE',  ( -1.207349081364828880, 0.2306618581243847221, -0.2411417322834647770 ) ) ;
#70449=CARTESIAN_POINT ( 'NONE',  ( 0.8661417322834653598, -0.1870078740157479769, 0.4822834645669291653 ) ) ;
#70450=CARTESIAN_POINT ( 'NONE',  ( 1.332020997375328974, -0.05778040916215560624, -0.4822834645669293319 ) ) ;
#70451=CARTESIAN_POINT ( 'NONE',  ( 0.6167979002624678353, -0.4281496062992124485, 0.4176697321401328655 ) ) ;
#70456=CARTESIAN_POINT ( 'NONE',  ( 0.6692913385826777528, 0.2952755905511811885, 0.000000000000000000 ) ) ;
#70457=CARTESIAN_POINT ( 'NONE',  ( 0.4790026246719167324, -0.05778040916215522460, 0.4822834645669289988 ) ) ;
#70459=CARTESIAN_POINT ( 'NONE',  ( 0.9317585301837276734, -0.3690944881889763329, 0.3153832671262228327 ) ) ;
#70460=CARTESIAN_POINT ( 'NONE',  ( 1.220472440944882608, 0.2952755905511811885, 0.000000000000000000 ) ) ;
#70462=CARTESIAN_POINT ( 'NONE',  ( 0.4855643044619428750, 0.05413385826771666132, 0.4176697321401328100 ) ) ;
#70463=CARTESIAN_POINT ( 'NONE',  ( 0.9776902887139113929, -0.6692913385826773087, -0.1292274648535924053 ) ) ;
#70464=CARTESIAN_POINT ( 'NONE',  ( 0.4593175853018380828, 0.05413385826771626580, -0.4176697321401330321 ) ) ;
#70465=CARTESIAN_POINT ( 'NONE',  ( 1.108923884514436686, -0.2845877964562161244, -0.3641732283464567121 ) ) ;
#70466=CARTESIAN_POINT ( 'NONE',  ( -0.7414698162729651543, 0.2952755905511810774, -0.1292274648535930714 ) ) ;
#70467=CARTESIAN_POINT ( 'NONE',  ( -0.8727034120734901146, -0.05778040916215560624, -0.4822834645669293319 ) ) ;
#70468=CARTESIAN_POINT ( 'NONE',  ( 1.272965879265092637, 0.05413385826771666132, 0.4176697321401328100 ) ) ;
#70475=CARTESIAN_POINT ( 'NONE',  ( 1.476377952755906442, -0.5400638737290844871, 0.3530559997133364547 ) ) ;
#70476=CARTESIAN_POINT ( 'NONE',  ( 1.358267716535433323, -0.4536011799217368745, -0.2665933059059886201 ) ) ;
#70478=CARTESIAN_POINT ( 'NONE',  ( 1.364829396325460076, 0.1283753931104748280, 0.1820866141732283561 ) ) ;
#70479=CARTESIAN_POINT ( 'NONE',  ( 0.6184250938292470412, 2.084810923686589862E-15, -0.3791475997938226761 ) ) ;
#70483=CARTESIAN_POINT ( 'NONE',  ( -0.5971128608923877978, -0.5511811023622048555, -0.09757992244046775898 ) ) ;
#70484=CARTESIAN_POINT ( 'NONE',  ( -1.443569553805773564, -0.5023911411419708095, 0.1820866141732285504 ) ) ;
#70485=CARTESIAN_POINT ( 'NONE',  ( -1.469816272965878357, 0.2306618581243848609, 0.2411417322834645549 ) ) ;
#70486=CARTESIAN_POINT ( 'NONE',  ( 0.08530183727034192087, -0.3162353388693409650, -0.4822834645669289433 ) ) ;
#70487=CARTESIAN_POINT ( 'NONE',  ( -1.594488188976377119, 0.1660481256975883668, -0.3530559997133364547 ) ) ;
#70489=CARTESIAN_POINT ( 'NONE',  ( -1.193521905106661674, 2.660739321503277841E-15, -0.3464511005275191513 ) ) ;
#70492=CARTESIAN_POINT ( 'NONE',  ( -1.586052503253847057, 1.574803149606300412, 0.1653254495020574921 ) ) ;
#70493=CARTESIAN_POINT ( 'NONE',  ( -0.6758530183727028406, 0.1771653543307087630, 0.09757992244046791164 ) ) ;
#70494=CARTESIAN_POINT ( 'NONE',  ( -1.017060367454067249, -0.05778040916215522460, 0.4822834645669289988 ) ) ;
#70495=CARTESIAN_POINT ( 'NONE',  ( 1.076115485564305141, 0.2306618581243847221, -0.2411417322834647770 ) ) ;
#70498=DIRECTION ( 'NONE',  ( 0.000000000000000000, 0.000000000000000000, 1.000000000000000000 ) ) ;
#70499=CARTESIAN_POINT ( 'NONE',  ( 1.036745406824147731, 0.05413385826771666132, 0.4176697321401328100 ) ) ;
#70500=CARTESIAN_POINT ( 'NONE',  ( -1.141732283464566011, -0.6692913385826771977, 8.415575281601705876E-17 ) ) ;
#70502=CARTESIAN_POINT ( 'NONE',  ( -0.3805774278215216522, -0.3690944881889765550, -0.3153832671262227771 ) ) ;
#70505=CARTESIAN_POINT ( 'NONE',  ( -0.6036745406824141069, -0.5023911411419708095, -0.1820866141732282451 ) ) ;
#70506=CARTESIAN_POINT ( 'NONE',  ( 0.1771653543307093182, 0.07958543189024085140, 0.2665933059059887866 ) ) ;
#70507=CARTESIAN_POINT ( 'NONE',  ( 0.1706036745406830368, 0.05413385826771666132, 0.4176697321401328100 ) ) ;
#70508=CARTESIAN_POINT ( 'NONE',  ( -1.332020997375327642, -0.08942795157527998196, 0.3641732283464567121 ) ) ;
#70510=CARTESIAN_POINT ( 'NONE',  ( 1.056430446194226436, -0.6692913385826773087, -0.1292274648535924053 ) ) ;
#70512=CARTESIAN_POINT ( 'NONE',  ( -1.332020997375327642, -0.05778040916215522460, 0.4822834645669289988 ) ) ;
#70514=CARTESIAN_POINT ( 'NONE',  ( -0.2493438320209966919, 0.05413385826771626580, -0.4176697321401330321 ) ) ;
#70515=CARTESIAN_POINT ( 'NONE',  ( -0.9514435695538050464, -0.05778040916215560624, -0.4822834645669293319 ) ) ;
#70516=CARTESIAN_POINT ( 'NONE',  ( 0.8858267716535438430, 0.07958543189024085140, 0.2665933059059887866 ) ) ;
#70518=CARTESIAN_POINT ( 'NONE',  ( -0.4790026246719154557, -0.2845877964562159024, 0.3641732283464567677 ) ) ;
#70519=CARTESIAN_POINT ( 'NONE',  ( -0.6167979002624665030, 0.05413385826771666132, 0.4176697321401328100 ) ) ;
#70520=CARTESIAN_POINT ( 'NONE',  ( -1.332020997375327642, -0.05778040916215522460, 0.4822834645669289988 ) ) ;
#70522=CARTESIAN_POINT ( 'NONE',  ( 1.259842519685040019, -0.1870078740157480601, -0.3641732283464567677 ) ) ;
#70523=CARTESIAN_POINT ( 'NONE',  ( -0.1902887139107604098, 0.2952755905511810774, -0.1292274648535930714 ) ) ;
#70524=CARTESIAN_POINT ( 'NONE',  ( -1.450131233595799651, -0.6692913385826771977, 0.1292274648535927661 ) ) ;
#70527=( BOUNDED_CURVE ( )  B_SPLINE_CURVE ( 1, ( #54480, #41853 ),
 .UNSPECIFIED., .F., .F. ) 
 B_SPLINE_CURVE_WITH_KNOTS ( ( 2, 2 ),
 ( 0.0007457734483630566735, 0.002000000000000005246 ),
 .UNSPECIFIED. ) 
 CURVE ( )  GEOMETRIC_REPRESENTATION_ITEM ( )  RATIONAL_B_SPLINE_CURVE ( ( 0.9875488213027530104, 0.9875488213027530104 ) ) 
 REPRESENTATION_ITEM ( '' )  );
#70528=CARTESIAN_POINT ( 'NONE',  ( -0.7283464566929126471, -0.4536011799217367080, 0.2665933059059888421 ) ) ;
#70529=CARTESIAN_POINT ( 'NONE',  ( 0.5314960629921264834, 0.1660481256975883668, -0.3530559997133364547 ) ) ;
#70530=CARTESIAN_POINT ( 'NONE',  ( -1.076115485564303809, 0.1283753931104748280, 0.1820866141732283561 ) ) ;
#70532=CARTESIAN_POINT ( 'NONE',  ( -1.161417322834644716, -0.5400638737290845981, -0.3530559997133363437 ) ) ;
#70533=CARTESIAN_POINT ( 'NONE',  ( 0.7414698162729663755, 0.2952755905511811885, 0.1292274648535926551 ) ) ;
#70534=CARTESIAN_POINT ( 'NONE',  ( 0.2887139107611556010, 0.2306618581243847221, -0.2411417322834647770 ) ) ;
#70536=CARTESIAN_POINT ( 'NONE',  ( -1.633858267716534529, -0.4536011799217368745, -0.2665933059059886201 ) ) ;
#70541=CARTESIAN_POINT ( 'NONE',  ( 1.089238845144357759, -0.004921259842519870586, -0.3153832671262229437 ) ) ;
#70543=CARTESIAN_POINT ( 'NONE',  ( 0.1443569553805781891, -0.3690944881889763329, 0.3153832671262228327 ) ) ;
#70544=CARTESIAN_POINT ( 'NONE',  ( 0.1771653543307093182, 0.1660481256975885056, 0.3530559997133364547 ) ) ;
#70547=CARTESIAN_POINT ( 'NONE',  ( 0.2296587926509192634, -0.2845877964562159024, 0.3641732283464567677 ) ) ;
#70548=CARTESIAN_POINT ( 'NONE',  ( -0.6233595800524928121, -0.3162353388693409650, -0.4822834645669289433 ) ) ;
#70549=CARTESIAN_POINT ( 'NONE',  ( -1.292650918635170010, 0.2952755905511810774, -0.1292274648535930714 ) ) ;
#70550=CARTESIAN_POINT ( 'NONE',  ( 0.6824146981627303710, -0.6046776061558807314, 0.2411417322834647770 ) ) ;
#70553=B_SPLINE_CURVE_WITH_KNOTS ( 'NONE', 3,
 ( #49573, #73310, #9332, #8915 ),
 .UNSPECIFIED., .F., .F.,
 ( 4, 4 ),
 ( 0.05883702829161106124, 0.06031386722719112026 ),
 .UNSPECIFIED. ) ;
#70554=ORIENTED_EDGE ( 'NONE', *, *, #27043, .F. ) ;
#70555=ORIENTED_EDGE ( 'NONE', *, *, #30143, .F. ) ;
#70556=CARTESIAN_POINT ( 'NONE',  ( -1.482939632545930975, -0.4281496062992127816, -0.4176697321401328100 ) ) ;
#70557=CARTESIAN_POINT ( 'NONE',  ( -0.5774278215223089816, -0.6046776061558807314, 0.2411417322834647770 ) ) ;
#70558=CARTESIAN_POINT ( 'NONE',  ( -0.5774278215223089816, -0.5023911411419708095, 0.1820866141732285504 ) ) ;
#70559=CARTESIAN_POINT ( 'NONE',  ( -0.7480314960629914633, -0.6692913385826771977, 8.415575281601705876E-17 ) ) ;
#70561=CARTESIAN_POINT ( 'NONE',  ( 0.1377952755905518800, -0.4536011799217367080, 0.2665933059059888421 ) ) ;
#70563=CARTESIAN_POINT ( 'NONE',  ( -1.640419947506561060, -0.004921259842519576551, 0.3153832671262227771 ) ) ;
#70564=CARTESIAN_POINT ( 'NONE',  ( -1.194225721784776262, 0.05413385826771626580, -0.4176697321401330321 ) ) ;
#70565=CARTESIAN_POINT ( 'NONE',  ( 0.3018372703412079971, -0.4281496062992124485, 0.4176697321401328655 ) ) ;
#70566=CARTESIAN_POINT ( 'NONE',  ( -0.8661417322834640276, -0.1870078740157479769, 0.4822834645669291653 ) ) ;
#70569=CARTESIAN_POINT ( 'NONE',  ( -0.9186351706036736120, -0.5023911411419708095, -0.1820866141732282451 ) ) ;
#70573=CARTESIAN_POINT ( 'NONE',  ( -1.594488188976377563, -0.4536011799217367080, 0.2665933059059888421 ) ) ;
#70574=CARTESIAN_POINT ( 'NONE',  ( -1.213910761154854745, -0.6692913385826771977, 0.1292274648535927661 ) ) ;
#70575=CARTESIAN_POINT ( 'NONE',  ( -0.7480314960629914633, -0.6692913385826771977, 8.415575281601705876E-17 ) ) ;
#70577=CARTESIAN_POINT ( 'NONE',  ( -1.240157480314959759, 0.1660481256975885056, 0.3530559997133364547 ) ) ;
#70578=CARTESIAN_POINT ( 'NONE',  ( -1.325459317585300889, -0.4281496062992127816, -0.4176697321401328100 ) ) ;
#70579=DIRECTION ( 'NONE',  ( -3.096699300667737957E-16, 1.000000000000000000, -0.000000000000000000 ) ) ;
#70582=CARTESIAN_POINT ( 'NONE',  ( 0.3149606299212606708, -0.1870078740157480601, -0.3641732283464567677 ) ) ;
#70583=CARTESIAN_POINT ( 'NONE',  ( -0.4831401376419939830, -3.153061149046662969E-15, -0.4118477457933005237 ) ) ;
#70585=CARTESIAN_POINT ( 'NONE',  ( -0.2362204724409442680, -0.1870078740157480601, -0.3641732283464567677 ) ) ;
#70586=CARTESIAN_POINT ( 'NONE',  ( -0.6627296587926501115, 0.2952755905511810774, -0.1292274648535930714 ) ) ;
#70587=CARTESIAN_POINT ( 'NONE',  ( 1.325459317585302665, 0.05413385826771626580, -0.4176697321401330321 ) ) ;
#70588=CARTESIAN_POINT ( 'NONE',  ( -0.5839895013123351797, -0.6692913385826771977, 0.1292274648535927661 ) ) ;
#70592=CARTESIAN_POINT ( 'NONE',  ( -0.9186351706036736120, -0.6046776061558809534, -0.2411417322834644161 ) ) ;
#70593=CARTESIAN_POINT ( 'NONE',  ( 1.482939632545932307, 0.05413385826771626580, -0.4176697321401330321 ) ) ;
#70594=CARTESIAN_POINT ( 'NONE',  ( -1.200787401574802349, 0.07958543189024071263, -0.2665933059059888421 ) ) ;
#70595=CARTESIAN_POINT ( 'NONE',  ( -1.502624671916009680, -0.05778040916215560624, -0.4822834645669293319 ) ) ;
#70600=CARTESIAN_POINT ( 'NONE',  ( 0.1049868766404206816, 0.2306618581243848609, 0.2411417322834645549 ) ) ;
#70601=CARTESIAN_POINT ( 'NONE',  ( -1.069553805774277722, -0.5511811023622048555, -0.09757992244046775898 ) ) ;
#70602=CARTESIAN_POINT ( 'NONE',  ( -0.7414698162729651543, 0.2952755905511810774, -0.1292274648535930714 ) ) ;
#70604=CARTESIAN_POINT ( 'NONE',  ( -1.345144356955379816, -0.05778040916215560624, -0.4822834645669293319 ) ) ;
#70605=CARTESIAN_POINT ( 'NONE',  ( -1.023622047244094002, -0.1870078740157480879, -0.4822834645669291653 ) ) ;
#70606=CARTESIAN_POINT ( 'NONE',  ( -0.1574803149606292529, -0.1870078740157479769, 0.4822834645669291653 ) ) ;
#70608=CARTESIAN_POINT ( 'NONE',  ( 0.9908136482939640111, 0.1771653543307087075, -0.09757992244046823083 ) ) ;
#70609=CARTESIAN_POINT ( 'NONE',  ( -0.6167979002624665030, -0.004921259842519576551, 0.3153832671262227771 ) ) ;
#70611=CARTESIAN_POINT ( 'NONE',  ( 0.8202099737532814183, -0.5511811023622048555, -0.09757992244046775898 ) ) ;
#70612=CARTESIAN_POINT ( 'NONE',  ( 1.194225721784777594, -0.3690944881889765550, -0.3153832671262227771 ) ) ;
#70613=CARTESIAN_POINT ( 'NONE',  ( 1.246719160104987623, -0.4281496062992124485, 0.4176697321401328655 ) ) ;
#70614=CARTESIAN_POINT ( 'NONE',  ( 0.5052493438320218022, -0.5511811023622048555, -0.09757992244046775898 ) ) ;
#70616=CARTESIAN_POINT ( 'NONE',  ( -0.8333333333333323711, 0.2952755905511811885, 0.1292274648535926551 ) ) ;
#70617=CARTESIAN_POINT ( 'NONE',  ( 1.345144356955381593, -0.3162353388693409650, -0.4822834645669289433 ) ) ;
#70619=CARTESIAN_POINT ( 'NONE',  ( -0.5052493438320203589, 0.1771653543307087075, -0.09757992244046823083 ) ) ;
#70620=CARTESIAN_POINT ( 'NONE',  ( 0.03937007874015806264, 0.2952755905511811885, 0.000000000000000000 ) ) ;
#70621=CARTESIAN_POINT ( 'NONE',  ( 0.4265091863517067594, 0.2952755905511811885, 0.1292274648535926551 ) ) ;
#70623=CARTESIAN_POINT ( 'NONE',  ( 0.8530183727034126306, -0.004921259842519870586, -0.3153832671262229437 ) ) ;
#70624=CARTESIAN_POINT ( 'NONE',  ( 0.04593175853018440641, 0.1771653543307087075, -0.09757992244046823083 ) ) ;
#70625=CARTESIAN_POINT ( 'NONE',  ( 0.06561679790026316017, -0.4281496062992124485, 0.4176697321401328655 ) ) ;
#70626=CARTESIAN_POINT ( 'NONE',  ( -1.450131233595799651, -0.6692913385826771977, 0.1292274648535927661 ) ) ;
#70627=CARTESIAN_POINT ( 'NONE',  ( -0.5708661417322825615, -0.4536011799217367080, 0.2665933059059888421 ) ) ;
#70629=CARTESIAN_POINT ( 'NONE',  ( -0.3018372703412066094, -0.4281496062992127816, -0.4176697321401328100 ) ) ;
#70632=CARTESIAN_POINT ( 'NONE',  ( 0.2296587926509192634, -0.08942795157528024563, -0.3641732283464568787 ) ) ;
#70633=CARTESIAN_POINT ( 'NONE',  ( -0.7480314960629914633, -0.6692913385826771977, 8.415575281601705876E-17 ) ) ;
#70635=CARTESIAN_POINT ( 'NONE',  ( -0.9448818897637790704, -0.1870078740157480879, -0.4822834645669291653 ) ) ;
#70636=CARTESIAN_POINT ( 'NONE',  ( -1.318897637795274802, 0.07958543189024085140, 0.2665933059059887866 ) ) ;
#70638=CARTESIAN_POINT ( 'NONE',  ( -0.3412073490813641308, 0.2306618581243847221, -0.2411417322834647770 ) ) ;
#70639=CARTESIAN_POINT ( 'NONE',  ( -0.8923884514435688198, -0.5023911411419708095, 0.1820866141732285504 ) ) ;
#70640=CARTESIAN_POINT ( 'NONE',  ( -1.679790026246718693, 0.1283753931104746893, -0.1820866141732285504 ) ) ;
#70641=CARTESIAN_POINT ( 'NONE',  ( 1.272965879265092637, 0.05413385826771666132, 0.4176697321401328100 ) ) ;
#70644=ORIENTED_EDGE ( 'NONE', *, *, #5930, .T. ) ;
#70646=EDGE_CURVE ( 'NONE', #76146, #25432, #37402, .T. ) ;
#70647=CARTESIAN_POINT ( 'NONE',  ( -1.259842519685038686, -0.1870078740157479769, 0.4822834645669291653 ) ) ;
#70648=CARTESIAN_POINT ( 'NONE',  ( -0.8202099737532801971, -0.6692913385826771977, 0.1292274648535927661 ) ) ;
#70649=CARTESIAN_POINT ( 'NONE',  ( -1.476377952755905110, 0.1660481256975885056, 0.3530559997133364547 ) ) ;
#70651=CARTESIAN_POINT ( 'NONE',  ( 1.463254593175853824, -0.5511811023622046335, 0.09757992244046803654 ) ) ;
#70652=CARTESIAN_POINT ( 'NONE',  ( 0.4265091863517067594, 0.2952755905511811885, 0.1292274648535926551 ) ) ;
#70653=CARTESIAN_POINT ( 'NONE',  ( 0.1509186351706045259, -0.05778040916215560624, -0.4822834645669293319 ) ) ;
#70654=CARTESIAN_POINT ( 'NONE',  ( -0.3249695492770445782, -2.567464376874931580E-15, -0.4445507791589072832 ) ) ;
#70655=DIRECTION ( 'NONE',  ( -3.096699300667737957E-16, 1.000000000000000000, -0.000000000000000000 ) ) ;
#70656=CARTESIAN_POINT ( 'NONE',  ( 0.9514435695538062676, -0.08942795157527998196, 0.3641732283464567121 ) ) ;
#70662=CARTESIAN_POINT ( 'NONE',  ( -0.2099737532808391705, -0.6046776061558809534, -0.2411417322834644161 ) ) ;
#70663=CARTESIAN_POINT ( 'NONE',  ( -0.8923884514435688198, 0.2306618581243847221, -0.2411417322834647770 ) ) ;
#70664=CARTESIAN_POINT ( 'NONE',  ( -1.528871391076114250, -0.6692913385826771977, 0.1292274648535927661 ) ) ;
#70665=CARTESIAN_POINT ( 'NONE',  ( 0.5971128608923891301, 0.2952755905511810774, -0.1292274648535930714 ) ) ;
#70666=CARTESIAN_POINT ( 'NONE',  ( -1.587926509186350810, -0.004921259842519870586, -0.3153832671262229437 ) ) ;
#70667=CARTESIAN_POINT ( 'NONE',  ( 1.437007874015748810, 0.1660481256975885056, 0.3530559997133364547 ) ) ;
#70668=CARTESIAN_POINT ( 'NONE',  ( -0.3937007874015740483, -0.1870078740157479769, 0.4822834645669291653 ) ) ;
#70669=CARTESIAN_POINT ( 'NONE',  ( 0.5708661417322841158, -0.5400638737290845981, -0.3530559997133363437 ) ) ;
#70670=CARTESIAN_POINT ( 'NONE',  ( -1.614173228346455824, 0.2952755905511811885, 0.000000000000000000 ) ) ;
#70671=CARTESIAN_POINT ( 'NONE',  ( 1.299212598425197429, 0.2952755905511811885, 0.000000000000000000 ) ) ;
#70672=CARTESIAN_POINT ( 'NONE',  ( 1.679790026246720025, 0.2306618581243848609, 0.2411417322834645549 ) ) ;
#70673=CARTESIAN_POINT ( 'NONE',  ( -0.2427821522309703550, -0.05778040916215560624, -0.4822834645669293319 ) ) ;
#70674=ADVANCED_FACE ( 'NONE', ( #4581 ), #30252, .F. ) ;
#70676=CARTESIAN_POINT ( 'NONE',  ( 0.4265091863517067594, 0.1771653543307087630, 0.09757992244046791164 ) ) ;
#70680=CARTESIAN_POINT ( 'NONE',  ( -0.3805774278215216522, -0.3690944881889765550, -0.3153832671262227771 ) ) ;
#70684=CARTESIAN_POINT ( 'NONE',  ( 0.2165354330708668673, 0.1660481256975883668, -0.3530559997133364547 ) ) ;
#70685=CARTESIAN_POINT ( 'NONE',  ( -0.02624671916010428221, -0.6046776061558807314, 0.2411417322834647770 ) ) ;
#70687=CARTESIAN_POINT ( 'NONE',  ( -0.8858267716535425107, 0.1660481256975883668, -0.3530559997133364547 ) ) ;
#70689=CARTESIAN_POINT ( 'NONE',  ( -1.095800524934382292, -0.3162353388693409650, -0.4822834645669289433 ) ) ;
#70691=CARTESIAN_POINT ( 'NONE',  ( 0.8661417322834652488, -0.1870078740157480601, -0.3641732283464567677 ) ) ;
#70692=CARTESIAN_POINT ( 'NONE',  ( 0.4133858267716541968, 0.1660481256975885056, 0.3530559997133364547 ) ) ;
#70693=CARTESIAN_POINT ( 'NONE',  ( 0.9580052493438327987, -0.4281496062992127816, -0.4176697321401328100 ) ) ;
#70695=CARTESIAN_POINT ( 'NONE',  ( 0.3268936723430476143, 1.795490347638496118E-16, 0.3627985898453511271 ) ) ;
#70698=CARTESIAN_POINT ( 'NONE',  ( -0.02624671916010428221, -0.6046776061558807314, 0.2411417322834647770 ) ) ;
#70701=CARTESIAN_POINT ( 'NONE',  ( -1.272965879265091305, -0.004921259842519870586, -0.3153832671262229437 ) ) ;
#70702=CARTESIAN_POINT ( 'NONE',  ( 1.338582677165355062, -0.1870078740157480879, -0.4822834645669291653 ) ) ;
#70703=CONICAL_SURFACE ( 'NONE', #76058, 2.362204724409449508, 0.8726646259971734265 ) ;
#70704=CARTESIAN_POINT ( 'NONE',  ( 1.181102362204725198, -0.1870078740157479769, 0.4822834645669291653 ) ) ;
#70705=CARTESIAN_POINT ( 'NONE',  ( 8.195543980992789655E-16, -0.1870078740157480601, -0.3641732283464567677 ) ) ;
#70706=CARTESIAN_POINT ( 'NONE',  ( 0.4724409448818904789, -0.1870078740157479769, 0.4822834645669291653 ) ) ;
#70708=CARTESIAN_POINT ( 'NONE',  ( 0.5052493438320218022, -0.5511811023622048555, -0.09757992244046775898 ) ) ;
#70709=CARTESIAN_POINT ( 'NONE',  ( 0.1968503937007881344, 0.2952755905511811885, 0.000000000000000000 ) ) ;
#70711=CARTESIAN_POINT ( 'NONE',  ( -1.200787401574802349, 0.1660481256975883668, -0.3530559997133364547 ) ) ;
#70712=CARTESIAN_POINT ( 'NONE',  ( 0.6627296587926515548, 0.1771653543307087630, 0.09757992244046791164 ) ) ;
#70715=CARTESIAN_POINT ( 'NONE',  ( -0.1377952755905504645, 0.1660481256975885056, 0.3530559997133364547 ) ) ;
#70716=CARTESIAN_POINT ( 'NONE',  ( -0.4265091863517051496, -0.5511811023622046335, 0.09757992244046803654 ) ) ;
#70718=CARTESIAN_POINT ( 'NONE',  ( -0.3412073490813641308, -0.6046776061558807314, 0.2411417322834647770 ) ) ;
#70719=CARTESIAN_POINT ( 'NONE',  ( 0.1181102362204730916, -0.5511811023622047445, 6.969142054262312111E-17 ) ) ;
#70721=CARTESIAN_POINT ( 'NONE',  ( -0.07217847769028787330, -0.05778040916215522460, 0.4822834645669289988 ) ) ;
#70724=CARTESIAN_POINT ( 'NONE',  ( 1.351706036745407680, -0.004921259842519576551, 0.3153832671262227771 ) ) ;
#70725=CARTESIAN_POINT ( 'NONE',  ( 0.4835386291766070044, 2.606013654608237919E-15, 0.3954974714151456849 ) ) ;
#70726=CARTESIAN_POINT ( 'NONE',  ( -0.9973753280839886548, -0.5023911411419708095, -0.1820866141732282451 ) ) ;
#70727=CARTESIAN_POINT ( 'NONE',  ( -0.7808398950131225646, -0.08942795157527998196, 0.3641732283464567121 ) ) ;
#70728=CARTESIAN_POINT ( 'NONE',  ( -0.6036745406824141069, -0.6046776061558809534, -0.2411417322834644161 ) ) ;
#70729=CARTESIAN_POINT ( 'NONE',  ( 0.05905511811023681640, 0.1660481256975883668, -0.3530559997133364547 ) ) ;
#70730=CARTESIAN_POINT ( 'NONE',  ( 0.6758530183727039509, -0.5511811023622046335, 0.09757992244046803654 ) ) ;
#70731=LINE ( 'NONE', #64415, #63600 ) ;
#70732=CARTESIAN_POINT ( 'NONE',  ( 0.8989501312335963501, -0.5511811023622048555, -0.09757992244046775898 ) ) ;
#70733=ADVANCED_FACE ( 'NONE', ( #39047 ), #65160, .F. ) ;
#70734=CARTESIAN_POINT ( 'NONE',  ( 0.7677165354330716118, 0.1660481256975883668, -0.3530559997133364547 ) ) ;
#70735=CARTESIAN_POINT ( 'NONE',  ( -1.646051170424378096, -0.1870078740157480046, 1.254653134982923898E-17 ) ) ;
#70736=CARTESIAN_POINT ( 'NONE',  ( -0.05905511811023545637, -0.5400638737290845981, -0.3530559997133363437 ) ) ;
#70739=CARTESIAN_POINT ( 'NONE',  ( 1.423884514435696191, -0.08942795157527998196, 0.3641732283464567121 ) ) ;
#70740=CARTESIAN_POINT ( 'NONE',  ( 0.7545931758530189937, 0.2952755905511810774, -0.1292274648535930714 ) ) ;
#70742=CARTESIAN_POINT ( 'NONE',  ( -0.03280839895013062252, 0.2952755905511810774, -0.1292274648535930714 ) ) ;
#70744=CARTESIAN_POINT ( 'NONE',  ( 0.5446194225721792126, -0.2845877964562159024, 0.3641732283464567677 ) ) ;
#70745=CARTESIAN_POINT ( 'NONE',  ( 0.7414698162729663755, 0.2952755905511811885, 0.1292274648535926551 ) ) ;
#70746=CARTESIAN_POINT ( 'NONE',  ( -0.4199475065616791736, 0.1283753931104746893, -0.1820866141732285504 ) ) ;
#70747=CARTESIAN_POINT ( 'NONE',  ( -0.7414698162729651543, -0.6692913385826771977, 0.1292274648535927661 ) ) ;
#70749=CARTESIAN_POINT ( 'NONE',  ( 0.1706036745406830368, 0.05413385826771666132, 0.4176697321401328100 ) ) ;
#70750=CARTESIAN_POINT ( 'NONE',  ( -1.384514435695537005, -0.6692913385826773087, -0.1292274648535924053 ) ) ;
#70751=CARTESIAN_POINT ( 'NONE',  ( -0.8398950131233589023, -0.5023911411419708095, -0.1820866141732282451 ) ) ;
#70752=CARTESIAN_POINT ( 'NONE',  ( 0.2427821522309716595, -0.3162353388693409650, -0.4822834645669289433 ) ) ;
#70753=CARTESIAN_POINT ( 'NONE',  ( -1.312335958005248715, -0.6046776061558809534, -0.2411417322834644161 ) ) ;
#70754=CARTESIAN_POINT ( 'NONE',  ( -0.4986876640419939388, 0.2306618581243847221, -0.2411417322834647770 ) ) ;
#70755=EDGE_CURVE ( 'NONE', #30707, #820, #14655, .T. ) ;
#70757=CARTESIAN_POINT ( 'NONE',  ( 1.535433070866142335, -0.6692913385826771977, 8.415575281601705876E-17 ) ) ;
#70758=CARTESIAN_POINT ( 'NONE',  ( 1.351706036745407680, 0.05413385826771666132, 0.4176697321401328100 ) ) ;
#70761=CARTESIAN_POINT ( 'NONE',  ( -1.601049868766403650, 0.2306618581243847221, -0.2411417322834647770 ) ) ;
#70763=CARTESIAN_POINT ( 'NONE',  ( -0.9055118110236215490, 0.2952755905511811885, 0.000000000000000000 ) ) ;
#70767=CARTESIAN_POINT ( 'NONE',  ( 0.1049868766404206816, 0.1283753931104748280, 0.1820866141732283561 ) ) ;
#70769=ORIENTED_EDGE ( 'NONE', *, *, #41785, .T. ) ;
#70770=CARTESIAN_POINT ( 'NONE',  ( 0.1640419947506569498, -0.05778040916215522460, 0.4822834645669289988 ) ) ;
#70771=CARTESIAN_POINT ( 'NONE',  ( 0.4658792650918640033, -0.3162353388693405765, 0.4822834645669290543 ) ) ;
#70773=DIRECTION ( 'NONE',  ( -1.000000000000000000, -3.469446951953613696E-16, 0.000000000000000000 ) ) ;
#70774=CARTESIAN_POINT ( 'NONE',  ( -0.5314960629921250401, 0.07958543189024085140, 0.2665933059059887866 ) ) ;
#70776=CARTESIAN_POINT ( 'NONE',  ( 0.7939632545931766261, -0.3162353388693409650, -0.4822834645669289433 ) ) ;
#70777=CARTESIAN_POINT ( 'NONE',  ( 0.9251968503937015864, -0.4536011799217367080, 0.2665933059059888421 ) ) ;
#70778=CARTESIAN_POINT ( 'NONE',  ( -0.5839895013123351797, -0.6692913385826771977, 0.1292274648535927661 ) ) ;
#70780=CARTESIAN_POINT ( 'NONE',  ( -0.8070866141732276899, 0.1660481256975883668, -0.3530559997133364547 ) ) ;
#70781=CARTESIAN_POINT ( 'NONE',  ( -1.391076115485563758, 0.1283753931104748280, 0.1820866141732283561 ) ) ;
#70782=CARTESIAN_POINT ( 'NONE',  ( -0.7939632545931754048, -0.3162353388693405765, 0.4822834645669290543 ) ) ;
#70783=CARTESIAN_POINT ( 'NONE',  ( 1.686351706036745890, 0.2952755905511811885, 0.1292274648535926551 ) ) ;
#70785=EDGE_LOOP ( 'NONE', ( #7424, #14590, #25903, #13864 ) ) ;
#70787=CARTESIAN_POINT ( 'NONE',  ( 0.1443569553805781891, 0.05413385826771626580, -0.4176697321401330321 ) ) ;
#70789=CARTESIAN_POINT ( 'NONE',  ( -0.7283464566929126471, 0.1660481256975883668, -0.3530559997133364547 ) ) ;
#70790=CARTESIAN_POINT ( 'NONE',  ( 1.266404199475066328, -0.05778040916215522460, 0.4822834645669289988 ) ) ;
#70791=CARTESIAN_POINT ( 'NONE',  ( 1.266404199475066328, -0.05778040916215522460, 0.4822834645669289988 ) ) ;
#70792=CARTESIAN_POINT ( 'NONE',  ( 0.6430446194225728496, 0.05413385826771666132, 0.4176697321401328100 ) ) ;
#70793=CARTESIAN_POINT ( 'NONE',  ( 0.2427821522309719648, -0.05778040916215522460, 0.4822834645669289988 ) ) ;
#70795=CARTESIAN_POINT ( 'NONE',  ( -1.115485564304461219, -0.4281496062992124485, 0.4176697321401328655 ) ) ;
#70796=CARTESIAN_POINT ( 'NONE',  ( -0.2165354330708654795, 0.1660481256975885056, 0.3530559997133364547 ) ) ;
#70797=CARTESIAN_POINT ( 'NONE',  ( -0.1574803149606292529, -0.1870078740157480601, -0.3641732283464567677 ) ) ;
#70799=CARTESIAN_POINT ( 'NONE',  ( 0.03280839895013198948, 0.2952755905511811885, 0.1292274648535926551 ) ) ;
#70801=CARTESIAN_POINT ( 'NONE',  ( 0.9711286089238851948, 0.2306618581243848609, 0.2411417322834645549 ) ) ;
#70803=ORIENTED_EDGE ( 'NONE', *, *, #24986, .F. ) ;
#70806=CARTESIAN_POINT ( 'NONE',  ( 0.4593175853018380828, 0.05413385826771626580, -0.4176697321401330321 ) ) ;
#70807=CARTESIAN_POINT ( 'NONE',  ( -0.1968503937007867743, -0.5511811023622047445, 6.969142054262312111E-17 ) ) ;
#70808=VECTOR ( 'NONE', #54740, 39.37007874015748854 ) ;
#70810=CARTESIAN_POINT ( 'NONE',  ( 1.522309711286089939, 0.1283753931104748280, 0.1820866141732283561 ) ) ;
#70811=CARTESIAN_POINT ( 'NONE',  ( -0.06632061457837669372, -2.294479370626195693E-15, 0.3464511005275217603 ) ) ;
#70813=CARTESIAN_POINT ( 'NONE',  ( 1.601049868766404982, -0.5023911411419708095, -0.1820866141732282451 ) ) ;
#70815=CARTESIAN_POINT ( 'NONE',  ( -1.496062992125983815, -0.1870078740157479769, 0.4822834645669291653 ) ) ;
#70818=CARTESIAN_POINT ( 'NONE',  ( -0.09186351706036689768, 0.05413385826771626580, -0.4176697321401330321 ) ) ;
#70819=CARTESIAN_POINT ( 'NONE',  ( -1.069553805774277722, -0.6692913385826773087, -0.1292274648535924053 ) ) ;
#70820=CARTESIAN_POINT ( 'NONE',  ( -1.541994750656167090, 0.2952755905511811885, 0.1292274648535926551 ) ) ;
#70821=CARTESIAN_POINT ( 'NONE',  ( 0.2755905511811031494, -0.6692913385826771977, 8.415575281601705876E-17 ) ) ;
#70824=CARTESIAN_POINT ( 'NONE',  ( 1.568241469816273659, -0.05778040916215560624, -0.4822834645669293319 ) ) ;
#70825=CARTESIAN_POINT ( 'NONE',  ( 0.9514435695538062676, -0.05778040916215522460, 0.4822834645669289988 ) ) ;
#70826=CARTESIAN_POINT ( 'NONE',  ( 1.141732283464567788, -0.5511811023622047445, 6.969142054262312111E-17 ) ) ;
#70828=CARTESIAN_POINT ( 'NONE',  ( 0.8792650918635177559, -0.004921259842519576551, 0.3153832671262227771 ) ) ;
#70829=CARTESIAN_POINT ( 'NONE',  ( -1.345144356955379816, -0.3162353388693405765, 0.4822834645669290543 ) ) ;
#70831=CARTESIAN_POINT ( 'NONE',  ( 1.010498687664042716, -0.4281496062992124485, 0.4176697321401328655 ) ) ;
#70833=CARTESIAN_POINT ( 'NONE',  ( 0.5249343832021005074, -0.6046776061558807314, 0.2411417322834647770 ) ) ;
#70835=CARTESIAN_POINT ( 'NONE',  ( -1.692913385826770645, 0.1771653543307087630, 0.000000000000000000 ) ) ;
#70836=CARTESIAN_POINT ( 'NONE',  ( 0.5643044619422579178, -0.3690944881889765550, -0.3153832671262227771 ) ) ;
#70837=CARTESIAN_POINT ( 'NONE',  ( 0.6167979002624679463, 0.05413385826771626580, -0.4176697321401330321 ) ) ;
#70838=CARTESIAN_POINT ( 'NONE',  ( 1.614173228346457378, -0.5511811023622047445, 6.969142054262312111E-17 ) ) ;
#70839=CARTESIAN_POINT ( 'NONE',  ( -0.7283464566929126471, 0.07958543189024071263, -0.2665933059059888421 ) ) ;
#70840=CARTESIAN_POINT ( 'NONE',  ( -0.4265091863517051496, 0.2952755905511810774, -0.1292274648535930714 ) ) ;
#70841=CARTESIAN_POINT ( 'NONE',  ( -1.633858267716534529, 0.07958543189024085140, 0.2665933059059887866 ) ) ;
#70842=CARTESIAN_POINT ( 'NONE',  ( -0.9973753280839886548, -0.6046776061558809534, -0.2411417322834644161 ) ) ;
#70843=CARTESIAN_POINT ( 'NONE',  ( 0.8530183727034128527, -0.4281496062992124485, 0.4176697321401328655 ) ) ;
#70844=CARTESIAN_POINT ( 'NONE',  ( -1.423884514435694859, -0.08942795157528024563, -0.3641732283464568787 ) ) ;
#70846=CARTESIAN_POINT ( 'NONE',  ( 0.9580052493438326877, 0.05413385826771666132, 0.4176697321401328100 ) ) ;
#70848=CARTESIAN_POINT ( 'NONE',  ( -1.692913385826770645, 0.2952755905511811885, 0.000000000000000000 ) ) ;
#70849=CARTESIAN_POINT ( 'NONE',  ( 1.240157480314961314, 0.1660481256975883668, -0.3530559997133364547 ) ) ;
#70850=CARTESIAN_POINT ( 'NONE',  ( -1.082677165354329896, 0.07958543189024085140, 0.2665933059059887866 ) ) ;
#70852=CARTESIAN_POINT ( 'NONE',  ( -0.2755905511811015396, -0.6692913385826771977, 8.415575281601705876E-17 ) ) ;
#70853=CARTESIAN_POINT ( 'NONE',  ( -0.4068241469816264999, -0.3690944881889763329, 0.3153832671262228327 ) ) ;
#70854=CARTESIAN_POINT ( 'NONE',  ( -1.653543307086613234, -0.1870078740157480601, -0.3641732283464567677 ) ) ;
#70855=CARTESIAN_POINT ( 'NONE',  ( 0.8858267716535438430, -0.4536011799217368745, -0.2665933059059886201 ) ) ;
#70856=CARTESIAN_POINT ( 'NONE',  ( 0.6233595800524942554, -0.05778040916215560624, -0.4822834645669293319 ) ) ;
#70857=CARTESIAN_POINT ( 'NONE',  ( 1.430446194225722500, 0.05413385826771666132, 0.4176697321401328100 ) ) ;
#70858=CARTESIAN_POINT ( 'NONE',  ( 0.3215223097112867578, -0.3162353388693409650, -0.4822834645669289433 ) ) ;
#70859=CARTESIAN_POINT ( 'NONE',  ( 0.3740157480314966754, 0.07958543189024071263, -0.2665933059059888421 ) ) ;
#70861=CARTESIAN_POINT ( 'NONE',  ( -1.555118110236219930, -0.5400638737290845981, -0.3530559997133363437 ) ) ;
#70862=CARTESIAN_POINT ( 'NONE',  ( -1.371391076115484609, -0.6692913385826771977, 0.1292274648535927661 ) ) ;
#70863=CARTESIAN_POINT ( 'NONE',  ( -0.6430446194225716283, -0.4281496062992124485, 0.4176697321401328655 ) ) ;
#70867=CARTESIAN_POINT ( 'NONE',  ( -0.07217847769028813698, -0.3162353388693409650, -0.4822834645669289433 ) ) ;
#70868=CARTESIAN_POINT ( 'NONE',  ( 1.279527559055118724, 0.07958543189024085140, 0.2665933059059887866 ) ) ;
#70870=CARTESIAN_POINT ( 'NONE',  ( -0.6036745406824141069, -0.6046776061558809534, -0.2411417322834644161 ) ) ;
#70871=CARTESIAN_POINT ( 'NONE',  ( 0.4855643044619428750, 0.05413385826771666132, 0.4176697321401328100 ) ) ;
#70877=CARTESIAN_POINT ( 'NONE',  ( -0.9251968503937002541, 0.07958543189024085140, 0.2665933059059887866 ) ) ;
#70878=CARTESIAN_POINT ( 'NONE',  ( -1.043307086614172707, 0.1660481256975883668, -0.3530559997133364547 ) ) ;
#70880=CARTESIAN_POINT ( 'NONE',  ( 0.2559055118110243332, 0.1660481256975885056, 0.3530559997133364547 ) ) ;
#70881=CARTESIAN_POINT ( 'NONE',  ( 1.253280839895013710, -0.3162353388693405765, 0.4822834645669290543 ) ) ;
#70882=CARTESIAN_POINT ( 'NONE',  ( 0.9251968503937015864, -0.5400638737290844871, 0.3530559997133364547 ) ) ;
#70886=CARTESIAN_POINT ( 'NONE',  ( 1.640419947506562393, -0.4281496062992124485, 0.4176697321401328655 ) ) ;
#70887=CARTESIAN_POINT ( 'NONE',  ( 0.4658792650918640033, -0.3162353388693405765, 0.4822834645669290543 ) ) ;
#70888=CARTESIAN_POINT ( 'NONE',  ( 0.3674540682414705883, 0.2306618581243847221, -0.2411417322834647770 ) ) ;
#70889=CARTESIAN_POINT ( 'NONE',  ( 0.6496062992125991586, 0.07958543189024085140, 0.2665933059059887866 ) ) ;
#70890=CARTESIAN_POINT ( 'NONE',  ( 1.430446194225722500, -0.4281496062992127816, -0.4176697321401328100 ) ) ;
#70892=CARTESIAN_POINT ( 'NONE',  ( 0.4265091863517067039, -0.6692913385826773087, -0.1292274648535924053 ) ) ;
#70893=CARTESIAN_POINT ( 'NONE',  ( 1.036745406824147731, 0.05413385826771666132, 0.4176697321401328100 ) ) ;
#70894=CARTESIAN_POINT ( 'NONE',  ( 0.4330708661417329575, 0.2952755905511811885, 0.000000000000000000 ) ) ;
#70895=CARTESIAN_POINT ( 'NONE',  ( 1.148293963254593875, -0.5511811023622046335, 0.09757992244046803654 ) ) ;
#70896=CARTESIAN_POINT ( 'NONE',  ( -1.049868766404198794, 0.2306618581243847221, -0.2411417322834647770 ) ) ;
#70897=CARTESIAN_POINT ( 'NONE',  ( -1.056430446194224881, 0.2952755905511810774, -0.1292274648535930714 ) ) ;
#70898=CARTESIAN_POINT ( 'NONE',  ( 1.286089238845145033, 0.2306618581243848609, 0.2411417322834645549 ) ) ;
#70905=CARTESIAN_POINT ( 'NONE',  ( 0.8595800524934390507, -0.08942795157528024563, -0.3641732283464568787 ) ) ;
#70907=CARTESIAN_POINT ( 'NONE',  ( 1.181102362204725198, -0.1870078740157479769, 0.3641732283464567677 ) ) ;
#70908=CARTESIAN_POINT ( 'NONE',  ( 0.4531182788721080934, 1.535433070866141447, -0.5309055118110237448 ) ) ;
#70913=CARTESIAN_POINT ( 'NONE',  ( -1.194225721784776262, -0.3690944881889763329, 0.3153832671262228327 ) ) ;
#70914=CARTESIAN_POINT ( 'NONE',  ( -1.699475065616797398, 0.1771653543307087630, 0.09757992244046791164 ) ) ;
#70915=CARTESIAN_POINT ( 'NONE',  ( -1.233595800524933894, -0.6046776061558809534, -0.2411417322834644161 ) ) ;
#70916=CARTESIAN_POINT ( 'NONE',  ( 0.2755905511811031494, -0.6692913385826771977, 8.415575281601705876E-17 ) ) ;
#70917=CARTESIAN_POINT ( 'NONE',  ( 1.364829396325459854, -0.6046776061558809534, -0.2411417322834644161 ) ) ;
#70923=CARTESIAN_POINT ( 'NONE',  ( -1.614173228346456712, 2.401574803149606474, -0.1372047244094478091 ) ) ;
#70924=CARTESIAN_POINT ( 'NONE',  ( -0.8989501312335946848, -0.5511811023622046335, 0.09757992244046803654 ) ) ;
#70926=CARTESIAN_POINT ( 'NONE',  ( 0.7677165354330716118, 0.1660481256975883668, -0.3530559997133364547 ) ) ;
#70931=CARTESIAN_POINT ( 'NONE',  ( 1.049868766404200349, 0.2306618581243848609, 0.2411417322834645549 ) ) ;
#70932=CARTESIAN_POINT ( 'NONE',  ( 1.535433070866142335, -0.5511811023622047445, 6.969142054262312111E-17 ) ) ;
#70934=CARTESIAN_POINT ( 'NONE',  ( -0.5446194225721777693, -0.2845877964562161244, -0.3641732283464567121 ) ) ;
#70935=CARTESIAN_POINT ( 'NONE',  ( -1.286089238845143479, 0.1283753931104746893, -0.1820866141732285504 ) ) ;
#70937=CARTESIAN_POINT ( 'NONE',  ( -0.3543307086614165824, 0.1771653543307087630, 0.000000000000000000 ) ) ;
#70938=CARTESIAN_POINT ( 'NONE',  ( 0.2821522309711292364, -0.5511811023622046335, 0.09757992244046803654 ) ) ;
#70939=CARTESIAN_POINT ( 'NONE',  ( -0.03937007874015669567, -0.6692913385826771977, 8.415575281601705876E-17 ) ) ;
#70940=CARTESIAN_POINT ( 'NONE',  ( -1.115485564304461219, -0.004921259842519870586, -0.3153832671262229437 ) ) ;
#70942=CARTESIAN_POINT ( 'NONE',  ( 1.010498687664042716, 0.05413385826771626580, -0.4176697321401330321 ) ) ;
#70943=CARTESIAN_POINT ( 'NONE',  ( -1.601049868766403650, 0.2306618581243847221, -0.2411417322834647770 ) ) ;
#70945=CARTESIAN_POINT ( 'NONE',  ( -0.4396325459317579898, 0.2952755905511811885, 0.1292274648535926551 ) ) ;
#70946=CARTESIAN_POINT ( 'NONE',  ( -1.030183727034119867, -0.3162353388693405765, 0.4822834645669290543 ) ) ;
#70947=CARTESIAN_POINT ( 'NONE',  ( 0.9186351706036752773, 0.1283753931104746893, -0.1820866141732285504 ) ) ;
#70948=CARTESIAN_POINT ( 'NONE',  ( -0.2887139107611542133, 0.1283753931104748280, 0.1820866141732283561 ) ) ;
#70949=CARTESIAN_POINT ( 'NONE',  ( -0.7742782152230965886, 0.05413385826771666132, 0.4176697321401328100 ) ) ;
#70950=CARTESIAN_POINT ( 'NONE',  ( -1.417322834645668772, -0.1870078740157480879, -0.4822834645669291653 ) ) ;
#70952=CARTESIAN_POINT ( 'NONE',  ( 1.246719160104987623, -0.004921259842519870586, -0.3153832671262229437 ) ) ;
#70953=CARTESIAN_POINT ( 'NONE',  ( -1.450131233595799651, 0.2952755905511810774, -0.1292274648535930714 ) ) ;
#70954=CARTESIAN_POINT ( 'NONE',  ( -1.377952755905511140, 0.2952755905511811885, 0.000000000000000000 ) ) ;
#70957=CARTESIAN_POINT ( 'NONE',  ( -0.7349081364829387342, -0.5023911411419708095, 0.1820866141732285504 ) ) ;
#70958=CARTESIAN_POINT ( 'NONE',  ( 0.6364829396325465405, -0.05778040916215522460, 0.4822834645669289988 ) ) ;
#70959=CARTESIAN_POINT ( 'NONE',  ( -1.148293963254592542, -0.5511811023622048555, -0.09757992244046775898 ) ) ;
#70961=CARTESIAN_POINT ( 'NONE',  ( -1.122047244094487306, -0.5400638737290844871, 0.3530559997133364547 ) ) ;
#70962=CARTESIAN_POINT ( 'NONE',  ( 0.6758530183727039509, -0.6692913385826771977, 0.1292274648535927661 ) ) ;
#70963=CARTESIAN_POINT ( 'NONE',  ( 0.4921259842519691285, -0.5400638737290845981, -0.3530559997133363437 ) ) ;
#70965=CARTESIAN_POINT ( 'NONE',  ( -1.318897637795274802, -0.4536011799217368745, -0.2665933059059886201 ) ) ;
#70969=CARTESIAN_POINT ( 'NONE',  ( 2.795275590551181466, 2.793565526369266916, 0.000000000000000000 ) ) ;
#70970=CARTESIAN_POINT ( 'NONE',  ( 1.377952755905512472, 0.1771653543307087630, 0.000000000000000000 ) ) ;
#70971=CARTESIAN_POINT ( 'NONE',  ( 0.2624671916010504757, -0.5023911411419708095, -0.1820866141732282451 ) ) ;
#70972=CARTESIAN_POINT ( 'NONE',  ( 0.2821522309711292364, -0.6692913385826771977, 0.1292274648535927661 ) ) ;
#70973=CARTESIAN_POINT ( 'NONE',  ( 1.410761154855643795, -0.3162353388693405765, 0.4822834645669290543 ) ) ;
#70975=CARTESIAN_POINT ( 'NONE',  ( 0.5511811023622055217, -0.1870078740157479769, 0.3641732283464567677 ) ) ;
#70976=CARTESIAN_POINT ( 'NONE',  ( -0.6364829396325453192, -0.05778040916215560624, -0.4822834645669293319 ) ) ;
#70977=CARTESIAN_POINT ( 'NONE',  ( -1.233595800524933894, -0.6046776061558809534, -0.2411417322834644161 ) ) ;
#70978=CARTESIAN_POINT ( 'NONE',  ( 0.8530183727034128527, -0.4281496062992124485, 0.4176697321401328655 ) ) ;
#70981=CARTESIAN_POINT ( 'NONE',  ( -0.7217847769028863381, 0.05413385826771626580, -0.4176697321401330321 ) ) ;
#70983=ORIENTED_EDGE ( 'NONE', *, *, #51624, .F. ) ;
#70984=CARTESIAN_POINT ( 'NONE',  ( -1.141732283464566011, -0.6692913385826771977, 8.415575281601705876E-17 ) ) ;
#70985=CARTESIAN_POINT ( 'NONE',  ( -0.5446194225721777693, -0.05778040916215522460, 0.4822834645669289988 ) ) ;
#70986=CARTESIAN_POINT ( 'NONE',  ( -0.7217847769028863381, -0.3690944881889763329, 0.3153832671262228327 ) ) ;
#70987=CARTESIAN_POINT ( 'NONE',  ( -0.9055118110236215490, -0.6692913385826771977, 8.415575281601705876E-17 ) ) ;
#70989=CARTESIAN_POINT ( 'NONE',  ( -0.4617417521217842546, -1.429000049448402363E-15, 0.4118477457933010233 ) ) ;
#70990=CARTESIAN_POINT ( 'NONE',  ( -1.528871391076114250, -0.5511811023622046335, 0.09757992244046803654 ) ) ;
#70991=CARTESIAN_POINT ( 'NONE',  ( -1.292650918635170010, -0.6692913385826771977, 0.1292274648535927661 ) ) ;
#70992=CARTESIAN_POINT ( 'NONE',  ( 0.1902887139107617975, 0.2952755905511811885, 0.1292274648535926551 ) ) ;
#70993=CARTESIAN_POINT ( 'NONE',  ( -0.7020997375328074108, -0.05778040916215522460, 0.4822834645669289988 ) ) ;
#70996=CARTESIAN_POINT ( 'NONE',  ( -1.017060367454067249, -0.08942795157527998196, 0.3641732283464567121 ) ) ;
#70997=ORIENTED_EDGE ( 'NONE', *, *, #28086, .F. ) ;
#70999=EDGE_LOOP ( 'NONE', ( #29272, #52102, #76811, #57831 ) ) ;
#71001=CARTESIAN_POINT ( 'NONE',  ( -1.286089238845143479, -0.6046776061558807314, 0.2411417322834647770 ) ) ;
#71002=CARTESIAN_POINT ( 'NONE',  ( -1.266404199475064773, -0.05778040916215560624, -0.4822834645669293319 ) ) ;
#71004=CARTESIAN_POINT ( 'NONE',  ( -1.122047244094487306, -0.5400638737290844871, 0.3530559997133364547 ) ) ;
#71005=CARTESIAN_POINT ( 'NONE',  ( -1.102362204724408601, -0.1870078740157479769, 0.4822834645669291653 ) ) ;
#71006=CARTESIAN_POINT ( 'NONE',  ( -0.3822046412494086165, -4.992347309556208597E-15, 0.3791483426435189319 ) ) ;
#71008=CARTESIAN_POINT ( 'NONE',  ( -0.09842519685039295696, -0.4536011799217367080, 0.2665933059059888421 ) ) ;
#71011=CARTESIAN_POINT ( 'NONE',  ( -0.1837270341207343505, -0.5023911411419708095, 0.1820866141732285504 ) ) ;
#71012=CARTESIAN_POINT ( 'NONE',  ( -0.7677165354330699465, -0.5400638737290845981, -0.3530559997133363437 ) ) ;
#71013=CARTESIAN_POINT ( 'NONE',  ( 1.246719160104987623, -0.4281496062992124485, 0.4176697321401328655 ) ) ;
#71014=CARTESIAN_POINT ( 'NONE',  ( -0.6889763779527552368, 0.1660481256975885056, 0.3530559997133364547 ) ) ;
#71015=ORIENTED_EDGE ( 'NONE', *, *, #17807, .F. ) ;
#71018=CARTESIAN_POINT ( 'NONE',  ( -0.8005249343832011588, 0.05413385826771626580, -0.4176697321401330321 ) ) ;
#71019=CARTESIAN_POINT ( 'NONE',  ( 1.233595800524935227, -0.6046776061558807314, 0.2411417322834647770 ) ) ;
#71020=CARTESIAN_POINT ( 'NONE',  ( -1.279527559055116948, -0.4536011799217367080, 0.2665933059059888421 ) ) ;
#71021=CARTESIAN_POINT ( 'NONE',  ( -1.469816272965878357, -0.6046776061558809534, -0.2411417322834644161 ) ) ;
#71026=CARTESIAN_POINT ( 'NONE',  ( 0.2296587926509192634, -0.3162353388693405765, 0.4822834645669290543 ) ) ;
#71027=CARTESIAN_POINT ( 'NONE',  ( -1.443569553805773564, 0.1283753931104746893, -0.1820866141732285504 ) ) ;
#71028=CARTESIAN_POINT ( 'NONE',  ( -0.5905511811023615998, 0.2952755905511811885, 0.000000000000000000 ) ) ;
#71030=CARTESIAN_POINT ( 'NONE',  ( -1.128608923884513837, -0.6046776061558807314, 0.2411417322834647770 ) ) ;
#71032=CARTESIAN_POINT ( 'NONE',  ( -0.8202099737532801971, -0.6692913385826771977, 0.1292274648535927661 ) ) ;
#71033=CARTESIAN_POINT ( 'NONE',  ( 0.1246719160104994284, -0.6692913385826771977, 0.1292274648535927661 ) ) ;
#71035=CARTESIAN_POINT ( 'NONE',  ( 0.7020997375328090762, -0.08942795157528024563, -0.3641732283464568787 ) ) ;
#71036=CARTESIAN_POINT ( 'NONE',  ( -0.7545931758530177724, 0.1771653543307087630, 0.09757992244046791164 ) ) ;
#71038=CARTESIAN_POINT ( 'NONE',  ( 0.7349081364829403995, 0.1283753931104748280, 0.1820866141732283561 ) ) ;
#71039=CARTESIAN_POINT ( 'NONE',  ( 1.463254593175853824, 0.1771653543307087075, -0.09757992244046823083 ) ) ;
#71040=CARTESIAN_POINT ( 'NONE',  ( 1.200787401574803681, -0.5400638737290845981, -0.3530559997133363437 ) ) ;
#71041=CARTESIAN_POINT ( 'NONE',  ( 0.3083989501312343062, -0.08942795157528024563, -0.3641732283464568787 ) ) ;
#71043=CARTESIAN_POINT ( 'NONE',  ( -0.7677165354330699465, -0.5400638737290845981, -0.3530559997133363437 ) ) ;
#71044=CARTESIAN_POINT ( 'NONE',  ( 1.279527559055118724, 0.1660481256975885056, 0.3530559997133364547 ) ) ;
#71045=( BOUNDED_CURVE ( )  B_SPLINE_CURVE ( 2, ( #11125, #67545, #54898, #22914, #42264, #48581, #4387, #16622, #30471, #30055, #81840, #67961, #68379 ),
 .UNSPECIFIED., .F., .F. ) 
 B_SPLINE_CURVE_WITH_KNOTS ( ( 3, 2, 2, 2, 2, 2, 3 ),
 ( 0.6285787205705962721, 0.6287878787878787845, 0.6325757575757575690, 0.6363636363636363535, 0.6401515151515151381, 0.6439393939393939226, 0.6441485521566764350 ),
 .UNSPECIFIED. ) 
 CURVE ( )  GEOMETRIC_REPRESENTATION_ITEM ( )  RATIONAL_B_SPLINE_CURVE ( ( 0.9964447847208419695, 0.9981185001348091834, 1.000000000000000000, 0.9659258262890683122, 1.000000000000000000, 0.9659258262890683122, 1.000000000000000000, 0.9659258262890683122, 1.000000000000000000, 0.9659258262890683122, 1.000000000000000000, 0.9981185001348091834, 0.9964447847208420805 ) ) 
 REPRESENTATION_ITEM ( '' )  );
#71047=CARTESIAN_POINT ( 'NONE',  ( -0.4921259842519677963, 0.07958543189024071263, -0.2665933059059888421 ) ) ;
#71048=CARTESIAN_POINT ( 'NONE',  ( -0.4199475065616791736, 0.2306618581243847221, -0.2411417322834647770 ) ) ;
#71049=CARTESIAN_POINT ( 'NONE',  ( 0.2690288713910767848, 0.2952755905511811885, 0.1292274648535926551 ) ) ;
#71051=CARTESIAN_POINT ( 'NONE',  ( 0.9645669291338588858, 0.07958543189024085140, 0.2665933059059887866 ) ) ;
#71052=CARTESIAN_POINT ( 'NONE',  ( 0.1574803149606306130, -0.1870078740157479769, 0.3641732283464567677 ) ) ;
#71053=CARTESIAN_POINT ( 'NONE',  ( -0.1509186351706028884, -0.3162353388693409650, -0.4822834645669289433 ) ) ;
#71054=CARTESIAN_POINT ( 'NONE',  ( -1.469816272965878357, -0.6046776061558809534, -0.2411417322834644161 ) ) ;
#71055=CARTESIAN_POINT ( 'NONE',  ( -0.8202099737532799750, 0.1771653543307087075, -0.09757992244046823083 ) ) ;
#71056=CARTESIAN_POINT ( 'NONE',  ( -1.646051170424378096, -0.1870078740157480046, 1.254653134982923898E-17 ) ) ;
#71057=CARTESIAN_POINT ( 'NONE',  ( -0.7545931758530176614, -0.6692913385826773087, -0.1292274648535924053 ) ) ;
#71060=CARTESIAN_POINT ( 'NONE',  ( 0.09186351706036799403, -0.3690944881889765550, -0.3153832671262227771 ) ) ;
#71061=CARTESIAN_POINT ( 'NONE',  ( -0.8398950131233585692, 0.2306618581243848609, 0.2411417322834645549 ) ) ;
#71062=CARTESIAN_POINT ( 'NONE',  ( -1.069553805774277722, -0.6692913385826773087, -0.1292274648535924053 ) ) ;
#71063=CARTESIAN_POINT ( 'NONE',  ( -1.279527559055116948, 0.07958543189024071263, -0.2665933059059888421 ) ) ;
#71065=CARTESIAN_POINT ( 'NONE',  ( -0.8136482939632537770, 0.1283753931104746893, -0.1820866141732285504 ) ) ;
#71066=CARTESIAN_POINT ( 'NONE',  ( 0.4330708661417321248, 2.793565526369266028, 0.000000000000000000 ) ) ;
#71067=CARTESIAN_POINT ( 'NONE',  ( 1.233595800524935227, -0.6046776061558807314, 0.2411417322834647770 ) ) ;
#71072=VERTEX_POINT ( 'NONE', #7497 ) ;
#71074=CARTESIAN_POINT ( 'NONE',  ( 1.391076115485564868, -0.5023911411419708095, 0.1820866141732285504 ) ) ;
#71075=CARTESIAN_POINT ( 'NONE',  ( -1.463254593175852492, -0.6692913385826773087, -0.1292274648535924053 ) ) ;
#71076=CARTESIAN_POINT ( 'NONE',  ( 1.233595800524935227, -0.6046776061558807314, 0.2411417322834647770 ) ) ;
#71078=CARTESIAN_POINT ( 'NONE',  ( 1.469816272965879911, -0.5023911411419708095, 0.1820866141732285504 ) ) ;
#71079=CARTESIAN_POINT ( 'NONE',  ( 0.5511811023622055217, -0.1870078740157479769, 0.4822834645669291653 ) ) ;
#71080=CARTESIAN_POINT ( 'NONE',  ( -0.006561679790025524116, -0.05778040916215560624, -0.4822834645669293319 ) ) ;
#71082=CARTESIAN_POINT ( 'NONE',  ( -0.7137454485294953965, 2.165354330708661124, -0.4917280318828585184 ) ) ;
#71083=CARTESIAN_POINT ( 'NONE',  ( 0.8398950131233602345, 0.1283753931104746893, -0.1820866141732285504 ) ) ;
#71088=CARTESIAN_POINT ( 'NONE',  ( -0.1706036745406816491, -0.4281496062992124485, 0.4176697321401328655 ) ) ;
#71089=CARTESIAN_POINT ( 'NONE',  ( -1.614173228346455824, 0.2952755905511811885, 0.000000000000000000 ) ) ;
#71090=CARTESIAN_POINT ( 'NONE',  ( 0.4790026246719168435, -0.3162353388693409650, -0.4822834645669289433 ) ) ;
#71091=CARTESIAN_POINT ( 'NONE',  ( 1.338582677165355062, -0.1870078740157479769, 0.4822834645669291653 ) ) ;
#71092=CARTESIAN_POINT ( 'NONE',  ( 1.233595800524935227, -0.6046776061558807314, 0.2411417322834647770 ) ) ;
#71093=CARTESIAN_POINT ( 'NONE',  ( -0.5708661417322825615, -0.5400638737290844871, 0.3530559997133364547 ) ) ;
#71094=CARTESIAN_POINT ( 'NONE',  ( 0.1574803149606306130, -0.1870078740157479769, 0.4822834645669291653 ) ) ;
#71095=CARTESIAN_POINT ( 'NONE',  ( 1.417322834645670104, -0.1870078740157479769, 0.4822834645669291653 ) ) ;
#71096=CARTESIAN_POINT ( 'NONE',  ( 1.476377952755906220, 0.1660481256975883668, -0.3530559997133364547 ) ) ;
#71097=CARTESIAN_POINT ( 'NONE',  ( 1.148293963254593875, -0.6692913385826771977, 0.1292274648535927661 ) ) ;
#71098=CARTESIAN_POINT ( 'NONE',  ( -0.2755905511811018171, 0.2952755905511811885, 0.000000000000000000 ) ) ;
#71100=CARTESIAN_POINT ( 'NONE',  ( 0.2821522309711292364, 0.1771653543307087075, -0.09757992244046823083 ) ) ;
#71101=ORIENTED_EDGE ( 'NONE', *, *, #77172, .F. ) ;
#71104=CARTESIAN_POINT ( 'NONE',  ( -0.6102362204724400829, 0.07958543189024085140, 0.2665933059059887866 ) ) ;
#71106=CARTESIAN_POINT ( 'NONE',  ( 0.2887139107611556010, -0.6046776061558807314, 0.2411417322834647770 ) ) ;
#71107=CARTESIAN_POINT ( 'NONE',  ( -0.1968503937007867743, -0.6692913385826771977, 8.415575281601705876E-17 ) ) ;
#71108=CARTESIAN_POINT ( 'NONE',  ( -1.069553805774277722, 0.2952755905511811885, 0.1292274648535926551 ) ) ;
#71110=CARTESIAN_POINT ( 'NONE',  ( -1.509186351706035767, -0.4281496062992124485, 0.4176697321401328655 ) ) ;
#71112=CARTESIAN_POINT ( 'NONE',  ( 0.9711286089238851948, 0.1283753931104748280, 0.1820866141732283561 ) ) ;
#71113=CARTESIAN_POINT ( 'NONE',  ( 0.6758530183727039509, -0.6692913385826771977, 0.1292274648535927661 ) ) ;
#71114=CARTESIAN_POINT ( 'NONE',  ( 0.9055118110236227702, 0.2952755905511811885, 0.000000000000000000 ) ) ;
#71116=CARTESIAN_POINT ( 'NONE',  ( 0.3252997568826557773, 2.459406111854941508E-15, 0.4281989832122450323 ) ) ;
#71119=CARTESIAN_POINT ( 'NONE',  ( -0.1706036745406816491, -0.4281496062992124485, 0.4176697321401328655 ) ) ;
#71122=CARTESIAN_POINT ( 'NONE',  ( -1.181102362204723644, -0.1870078740157479769, 0.3641732283464567677 ) ) ;
#71123=CARTESIAN_POINT ( 'NONE',  ( 1.240157480314961314, -0.5400638737290844871, 0.3530559997133364547 ) ) ;
#71124=CARTESIAN_POINT ( 'NONE',  ( 1.384514435695538559, 0.2952755905511810774, -0.1292274648535930714 ) ) ;
#71125=CARTESIAN_POINT ( 'NONE',  ( 0.2296587926509192634, -0.2845877964562159024, 0.3641732283464567677 ) ) ;
#71126=CARTESIAN_POINT ( 'NONE',  ( 0.4461942257217855201, -0.6046776061558807314, 0.2411417322834647770 ) ) ;
#71128=CARTESIAN_POINT ( 'NONE',  ( 0.3280839895013130669, -0.3690944881889765550, -0.3153832671262227771 ) ) ;
#71129=CARTESIAN_POINT ( 'NONE',  ( -0.1049868766404193215, 0.2306618581243847221, -0.2411417322834647770 ) ) ;
#71131=CARTESIAN_POINT ( 'NONE',  ( -1.404199475065615932, 0.05413385826771666132, 0.4176697321401328100 ) ) ;
#71132=CARTESIAN_POINT ( 'NONE',  ( 0.4986876640419954376, 0.1283753931104748280, 0.1820866141732283561 ) ) ;
#71133=DIRECTION ( 'NONE',  ( 0.000000000000000000, 0.000000000000000000, -1.000000000000000000 ) ) ;
#71134=CARTESIAN_POINT ( 'NONE',  ( -0.5380577427821514602, -0.4281496062992127816, -0.4176697321401328100 ) ) ;
#71136=CARTESIAN_POINT ( 'NONE',  ( -0.3477690288713902178, 0.1771653543307087075, -0.09757992244046823083 ) ) ;
#71138=CARTESIAN_POINT ( 'NONE',  ( -0.9186351706036736120, 0.2306618581243848609, 0.2411417322834645549 ) ) ;
#71139=CARTESIAN_POINT ( 'NONE',  ( -0.09186351706036663400, -0.4281496062992124485, 0.4176697321401328655 ) ) ;
#71140=CARTESIAN_POINT ( 'NONE',  ( 0.1837270341207354329, 0.1283753931104748280, 0.1820866141732283561 ) ) ;
#71142=CARTESIAN_POINT ( 'NONE',  ( -0.07874015748031421014, -0.1870078740157479769, 0.4822834645669291653 ) ) ;
#71145=CARTESIAN_POINT ( 'NONE',  ( 0.8530183727034128527, -0.3690944881889763329, 0.3153832671262228327 ) ) ;
#71146=CARTESIAN_POINT ( 'NONE',  ( 1.213910761154856299, -0.6692913385826773087, -0.1292274648535924053 ) ) ;
#71148=CARTESIAN_POINT ( 'NONE',  ( -1.023622047244094002, -0.1870078740157480601, -0.3641732283464567677 ) ) ;
#71149=CARTESIAN_POINT ( 'NONE',  ( -1.246719160104986512, -0.004921259842519576551, 0.3153832671262227771 ) ) ;
#71150=CARTESIAN_POINT ( 'NONE',  ( -0.5839895013123351797, -0.6692913385826771977, 0.1292274648535927661 ) ) ;
#71151=CARTESIAN_POINT ( 'NONE',  ( 0.09842519685039434474, -0.5400638737290845981, -0.3530559997133363437 ) ) ;
#71152=CARTESIAN_POINT ( 'NONE',  ( 0.3805774278215230400, -0.3690944881889763329, 0.3153832671262228327 ) ) ;
#71154=CARTESIAN_POINT ( 'NONE',  ( 1.023622047244095112, -0.1870078740157480601, -0.3641732283464567677 ) ) ;
#71155=CARTESIAN_POINT ( 'NONE',  ( 0.1771653543307093182, -0.5400638737290845981, -0.3530559997133363437 ) ) ;
#71157=CARTESIAN_POINT ( 'NONE',  ( -1.614173228346456712, 2.362204724409448620, 0.1372047244094477536 ) ) ;
#71158=CARTESIAN_POINT ( 'NONE',  ( -0.07874015748031421014, -0.1870078740157480879, -0.4822834645669291653 ) ) ;
#71160=CARTESIAN_POINT ( 'NONE',  ( 1.515748031496063186, -0.4536011799217368745, -0.2665933059059886201 ) ) ;
#71161=CARTESIAN_POINT ( 'NONE',  ( 0.2624671916010504757, 0.2306618581243848609, 0.2411417322834645549 ) ) ;
#71162=CARTESIAN_POINT ( 'NONE',  ( 0.2952755905511819101, 0.1660481256975883668, -0.3530559997133364547 ) ) ;
#71163=CARTESIAN_POINT ( 'NONE',  ( 0.5708661417322841158, 0.1012011053420777407, 0.2882089793578256898 ) ) ;
#71164=CARTESIAN_POINT ( 'NONE',  ( 0.01968503937007957949, -0.4536011799217368745, -0.2665933059059886201 ) ) ;
#71165=CARTESIAN_POINT ( 'NONE',  ( 0.8923884514435703741, 0.2306618581243848609, 0.2411417322834645549 ) ) ;
#71166=CARTESIAN_POINT ( 'NONE',  ( -0.3215223097112853146, -0.2845877964562159024, 0.3641732283464567677 ) ) ;
#71167=CARTESIAN_POINT ( 'NONE',  ( -0.7611548556430438595, -0.6046776061558809534, -0.2411417322834644161 ) ) ;
#71169=CARTESIAN_POINT ( 'NONE',  ( -0.2690288713910754526, 0.2952755905511810774, -0.1292274648535930714 ) ) ;
#71170=CARTESIAN_POINT ( 'NONE',  ( -1.246719160104985846, -0.4281496062992127816, -0.4176697321401328100 ) ) ;
#71171=CARTESIAN_POINT ( 'NONE',  ( -0.4855643044619415427, -0.3690944881889763329, 0.3153832671262228327 ) ) ;
#71172=CARTESIAN_POINT ( 'NONE',  ( 0.1574803149606306130, -0.1870078740157479769, 0.4822834645669291653 ) ) ;
#71173=CARTESIAN_POINT ( 'NONE',  ( -1.430446194225721390, -0.4281496062992124485, 0.4176697321401328655 ) ) ;
#71174=CARTESIAN_POINT ( 'NONE',  ( -0.1968503937007867743, 0.2952755905511811885, 0.000000000000000000 ) ) ;
#71176=CARTESIAN_POINT ( 'NONE',  ( -0.9332960234133773625, 0.02791078216816064370, 0.4328096321851915285 ) ) ;
#71177=CARTESIAN_POINT ( 'NONE',  ( 1.148293963254593653, 0.2952755905511810774, -0.1292274648535930714 ) ) ;
#71178=CARTESIAN_POINT ( 'NONE',  ( 1.213910761154856299, 0.2952755905511811885, 0.1292274648535926551 ) ) ;
#71181=CARTESIAN_POINT ( 'NONE',  ( -1.371391076115484831, 0.2952755905511810774, -0.1292274648535930714 ) ) ;
#71184=ORIENTED_EDGE ( 'NONE', *, *, #23107, .F. ) ;
#71185=CARTESIAN_POINT ( 'NONE',  ( 0.01312335958005323398, -0.3690944881889765550, -0.3153832671262227771 ) ) ;
#71188=CARTESIAN_POINT ( 'NONE',  ( 0.3608923884514443348, 0.2952755905511810774, -0.1292274648535930714 ) ) ;
#71189=CARTESIAN_POINT ( 'NONE',  ( 0.4265091863517067039, -0.6692913385826773087, -0.1292274648535924053 ) ) ;
#71191=CARTESIAN_POINT ( 'NONE',  ( -1.586052503253849499, 0.4724409448818907564, 0.1653254495020552439 ) ) ;
#71192=CARTESIAN_POINT ( 'NONE',  ( -0.8661417322834640276, -0.1870078740157479769, 0.3641732283464567677 ) ) ;
#71194=CARTESIAN_POINT ( 'NONE',  ( 0.8530183727034128527, -0.4281496062992124485, 0.4176697321401328655 ) ) ;
#71195=CARTESIAN_POINT ( 'NONE',  ( 0.8595800524934390507, -0.08942795157528024563, -0.3641732283464568787 ) ) ;
#71196=CARTESIAN_POINT ( 'NONE',  ( -0.2099737532808391705, 0.2306618581243848609, 0.2411417322834645549 ) ) ;
#71198=CARTESIAN_POINT ( 'NONE',  ( -0.8727034120734901146, -0.3162353388693405765, 0.4822834645669290543 ) ) ;
#71199=CARTESIAN_POINT ( 'NONE',  ( -1.725721784776902190, -0.08942795157527998196, 0.3641732283464567121 ) ) ;
#71200=CARTESIAN_POINT ( 'NONE',  ( -0.8398950131233589023, -0.6046776061558809534, -0.2411417322834644161 ) ) ;
#71201=CARTESIAN_POINT ( 'NONE',  ( 1.391076115485564868, 0.2306618581243847221, -0.2411417322834647770 ) ) ;
#71202=CARTESIAN_POINT ( 'NONE',  ( 1.614173228346457378, -0.5511811023622047445, 6.969142054262312111E-17 ) ) ;
#71205=CARTESIAN_POINT ( 'NONE',  ( -0.1837270341207340729, 0.2306618581243847221, -0.2411417322834647770 ) ) ;
#71206=VERTEX_POINT ( 'NONE', #20955 ) ;
#71207=CARTESIAN_POINT ( 'NONE',  ( -0.6496062992125976043, -0.5400638737290844871, 0.3530559997133364547 ) ) ;
#71208=CARTESIAN_POINT ( 'NONE',  ( 1.535433070866142335, -0.6692913385826771977, 8.415575281601705876E-17 ) ) ;
#71209=CARTESIAN_POINT ( 'NONE',  ( 1.364829396325459854, -0.6046776061558809534, -0.2411417322834644161 ) ) ;
#71210=CARTESIAN_POINT ( 'NONE',  ( 0.1837270341207354329, 0.2306618581243848609, 0.2411417322834645549 ) ) ;
#71211=CARTESIAN_POINT ( 'NONE',  ( -0.03280839895013062252, 0.2952755905511810774, -0.1292274648535930714 ) ) ;
#71213=CARTESIAN_POINT ( 'NONE',  ( -1.043307086614172707, 0.1660481256975883668, -0.3530559997133364547 ) ) ;
#71214=CARTESIAN_POINT ( 'NONE',  ( -0.3871391076115476282, -0.05778040916215522460, 0.4822834645669289988 ) ) ;
#71215=CARTESIAN_POINT ( 'NONE',  ( -0.1968503937007867743, 0.1771653543307087630, 0.000000000000000000 ) ) ;
#71217=CARTESIAN_POINT ( 'NONE',  ( 1.286089238845145033, -0.6046776061558809534, -0.2411417322834644161 ) ) ;
#71218=CARTESIAN_POINT ( 'NONE',  ( -0.5905511811023615998, 0.2952755905511811885, 0.000000000000000000 ) ) ;
#71219=B_SPLINE_CURVE_WITH_KNOTS ( 'NONE', 3,
 ( #77876, #20630, #45857, #65251 ),
 .UNSPECIFIED., .F., .F.,
 ( 4, 4 ),
 ( 3.210432057730626195E-07, 0.001287787053611958712 ),
 .UNSPECIFIED. ) ;
#71220=CARTESIAN_POINT ( 'NONE',  ( -1.194225721784776262, 0.05413385826771626580, -0.4176697321401330321 ) ) ;
#71222=CARTESIAN_POINT ( 'NONE',  ( 0.9842519685039375910, 0.2952755905511811885, 0.000000000000000000 ) ) ;
#71226=CARTESIAN_POINT ( 'NONE',  ( 0.3543307086614181922, -0.6692913385826771977, 8.415575281601705876E-17 ) ) ;
#71227=CARTESIAN_POINT ( 'NONE',  ( -0.1049868766404193215, 0.1283753931104746893, -0.1820866141732285504 ) ) ;
#71228=CARTESIAN_POINT ( 'NONE',  ( 1.397637795275591177, 0.07958543189024071263, -0.2665933059059888421 ) ) ;
#71231=CARTESIAN_POINT ( 'NONE',  ( 1.607611548556431069, -0.5511811023622048555, -0.09757992244046775898 ) ) ;
#71232=CARTESIAN_POINT ( 'NONE',  ( 1.358267716535433323, -0.5400638737290845981, -0.3530559997133363437 ) ) ;
#71234=CARTESIAN_POINT ( 'NONE',  ( 0.04593175853018440641, 0.2952755905511810774, -0.1292274648535930714 ) ) ;
#71236=CARTESIAN_POINT ( 'NONE',  ( -1.666666666666665853, 0.05413385826771626580, -0.4176697321401330321 ) ) ;
#71237=CARTESIAN_POINT ( 'NONE',  ( -0.3346456692913377662, -0.5400638737290844871, 0.3530559997133364547 ) ) ;
#71239=CARTESIAN_POINT ( 'NONE',  ( -1.489501312335957062, -0.08942795157527998196, 0.3641732283464567121 ) ) ;
#71240=CARTESIAN_POINT ( 'NONE',  ( 0.3280839895013130669, 0.05413385826771666132, 0.4176697321401328100 ) ) ;
#71241=CARTESIAN_POINT ( 'NONE',  ( 1.023622047244095334, -0.1870078740157479769, 0.3641732283464567677 ) ) ;
#71243=CARTESIAN_POINT ( 'NONE',  ( 0.9186351706036752773, 0.1283753931104746893, -0.1820866141732285504 ) ) ;
#71244=CARTESIAN_POINT ( 'NONE',  ( -1.089238845144356427, -0.4281496062992127816, -0.4176697321401328100 ) ) ;
#71246=CARTESIAN_POINT ( 'NONE',  ( 1.115485564304462551, -0.4281496062992127816, -0.4176697321401328100 ) ) ;
#71248=CARTESIAN_POINT ( 'NONE',  ( 0.7020997375328090762, -0.3162353388693405765, 0.4822834645669290543 ) ) ;
#71249=CARTESIAN_POINT ( 'NONE',  ( 0.9317585301837276734, 0.05413385826771626580, -0.4176697321401330321 ) ) ;
#71250=LINE ( 'NONE', #77990, #26798 ) ;
#71251=CARTESIAN_POINT ( 'NONE',  ( 0.2821522309711292364, -0.5511811023622046335, 0.09757992244046803654 ) ) ;
#71252=CARTESIAN_POINT ( 'NONE',  ( 0.4265091863517067594, 0.2952755905511811885, 0.1292274648535926551 ) ) ;
#71254=CARTESIAN_POINT ( 'NONE',  ( -1.115485564304461219, -0.3690944881889763329, 0.3153832671262228327 ) ) ;
#71255=CARTESIAN_POINT ( 'NONE',  ( -0.9908136482939626788, -0.6692913385826773087, -0.1292274648535924053 ) ) ;
#71256=CARTESIAN_POINT ( 'NONE',  ( 1.017060367454068803, -0.3162353388693405765, 0.4822834645669290543 ) ) ;
#71257=CARTESIAN_POINT ( 'NONE',  ( -1.023622047244094002, -0.1870078740157480879, -0.4822834645669291653 ) ) ;
#71258=CARTESIAN_POINT ( 'NONE',  ( 0.7742782152230979209, 0.05413385826771626580, -0.4176697321401330321 ) ) ;
#71259=CARTESIAN_POINT ( 'NONE',  ( -1.489501312335957062, -0.08942795157527998196, 0.3641732283464567121 ) ) ;
#71261=CARTESIAN_POINT ( 'NONE',  ( 1.167979002624672580, 0.05413385826771626580, -0.4176697321401330321 ) ) ;
#71263=CARTESIAN_POINT ( 'NONE',  ( 1.358267716535433323, 0.1660481256975885056, 0.3530559997133364547 ) ) ;
#71264=CARTESIAN_POINT ( 'NONE',  ( -1.522309711286088607, 0.1283753931104746893, -0.1820866141732285504 ) ) ;
#71265=CARTESIAN_POINT ( 'NONE',  ( 1.561679790026247350, -0.004921259842519870586, -0.3153832671262229437 ) ) ;
#71266=CARTESIAN_POINT ( 'NONE',  ( -1.489501312335957062, -0.08942795157527998196, 0.3641732283464567121 ) ) ;
#71267=CARTESIAN_POINT ( 'NONE',  ( -0.4265091863517051496, -0.5511811023622046335, 0.09757992244046803654 ) ) ;
#71269=CARTESIAN_POINT ( 'NONE',  ( 0.9383202099737536495, -0.2845877964562159024, 0.3641732283464567677 ) ) ;
#71270=CARTESIAN_POINT ( 'NONE',  ( 0.5905511811023629321, 0.2952755905511811885, 0.000000000000000000 ) ) ;
#71271=CARTESIAN_POINT ( 'NONE',  ( 1.187664041994751285, -0.3162353388693409650, -0.4822834645669289433 ) ) ;
#71272=CARTESIAN_POINT ( 'NONE',  ( -0.02624671916010428221, 0.2306618581243847221, -0.2411417322834647770 ) ) ;
#71273=CARTESIAN_POINT ( 'NONE',  ( 0.7611548556430451917, -0.5023911411419708095, 0.1820866141732285504 ) ) ;
#71274=CARTESIAN_POINT ( 'NONE',  ( -1.482939632545930975, 0.05413385826771666132, 0.4176697321401328100 ) ) ;
#71275=CARTESIAN_POINT ( 'NONE',  ( -1.614173228346455824, 0.2952755905511811885, 0.000000000000000000 ) ) ;
#71276=CARTESIAN_POINT ( 'NONE',  ( -0.4068241469816267775, 0.05413385826771626580, -0.4176697321401330321 ) ) ;
#71279=CARTESIAN_POINT ( 'NONE',  ( 0.1771653543307093182, 0.1660481256975885056, 0.3530559997133364547 ) ) ;
#71280=CARTESIAN_POINT ( 'NONE',  ( -0.5446194225721777693, -0.05778040916215522460, 0.4822834645669289988 ) ) ;
#71281=CARTESIAN_POINT ( 'NONE',  ( -0.006561679790025524116, -0.3162353388693405765, 0.4822834645669290543 ) ) ;
#71289=CARTESIAN_POINT ( 'NONE',  ( -1.108923884514435132, -0.2845877964562159024, 0.3641732283464567677 ) ) ;
#71291=CARTESIAN_POINT ( 'NONE',  ( -1.030183727034119867, -0.05778040916215560624, -0.4822834645669293319 ) ) ;
#71293=CARTESIAN_POINT ( 'NONE',  ( 0.2493438320209980519, 0.05413385826771666132, 0.4176697321401328100 ) ) ;
#71294=CARTESIAN_POINT ( 'NONE',  ( -0.1640419947506555343, -0.2845877964562159024, 0.3641732283464567677 ) ) ;
#71295=CARTESIAN_POINT ( 'NONE',  ( 1.272965879265092637, 0.05413385826771666132, 0.4176697321401328100 ) ) ;
#71296=CARTESIAN_POINT ( 'NONE',  ( 0.2624671916010504757, -0.6046776061558809534, -0.2411417322834644161 ) ) ;
#71300=CARTESIAN_POINT ( 'NONE',  ( 1.305774278215223960, -0.6692913385826771977, 0.1292274648535927661 ) ) ;
#71301=CARTESIAN_POINT ( 'NONE',  ( 0.4133858267716541968, -0.5400638737290845981, -0.3530559997133363437 ) ) ;
#71302=CARTESIAN_POINT ( 'NONE',  ( 0.2362204724409456558, -0.1870078740157480879, -0.4822834645669291653 ) ) ;
#71303=CARTESIAN_POINT ( 'NONE',  ( 1.345144356955381593, -0.05778040916215522460, 0.4822834645669289988 ) ) ;
#71306=CARTESIAN_POINT ( 'NONE',  ( 0.03280839895013198948, 0.2952755905511811885, 0.1292274648535926551 ) ) ;
#71307=CARTESIAN_POINT ( 'NONE',  ( 1.017060367454068803, -0.3162353388693405765, 0.4822834645669290543 ) ) ;
#71308=CARTESIAN_POINT ( 'NONE',  ( 0.3543307086614181922, -0.6692913385826771977, 8.415575281601705876E-17 ) ) ;
#71309=CARTESIAN_POINT ( 'NONE',  ( 1.003937007874016407, -0.4536011799217367080, 0.2665933059059888421 ) ) ;
#71310=CARTESIAN_POINT ( 'NONE',  ( -1.023622047244094002, -0.1870078740157480879, -0.4822834645669291653 ) ) ;
#71311=CARTESIAN_POINT ( 'NONE',  ( -1.312335958005248715, -0.6046776061558809534, -0.2411417322834644161 ) ) ;
#71312=CARTESIAN_POINT ( 'NONE',  ( 0.8398950131233602345, 0.2306618581243847221, -0.2411417322834647770 ) ) ;
#71315=CARTESIAN_POINT ( 'NONE',  ( 1.509186351706037543, 0.05413385826771666132, 0.4176697321401328100 ) ) ;
#71319=CARTESIAN_POINT ( 'NONE',  ( 1.653543307086614789, -0.1870078740157479769, 0.4822834645669291653 ) ) ;
#71320=CARTESIAN_POINT ( 'NONE',  ( 0.9251968503937015864, -0.4536011799217367080, 0.2665933059059888421 ) ) ;
#71322=CARTESIAN_POINT ( 'NONE',  ( -0.1443569553805768291, 0.05413385826771666132, 0.4176697321401328100 ) ) ;
#71326=CARTESIAN_POINT ( 'NONE',  ( -1.292650918635170010, 0.1771653543307087075, -0.09757992244046823083 ) ) ;
#71327=CARTESIAN_POINT ( 'NONE',  ( 1.587926509186352142, 0.05413385826771666132, 0.4176697321401328100 ) ) ;
#71328=CARTESIAN_POINT ( 'NONE',  ( -1.640419947506561060, 0.05413385826771666132, 0.4176697321401328100 ) ) ;
#71329=CARTESIAN_POINT ( 'NONE',  ( -0.1312335958005241554, 0.2306618581243848609, 0.2411417322834645549 ) ) ;
#71330=CARTESIAN_POINT ( 'NONE',  ( 1.430446194225722500, 0.05413385826771666132, 0.4176697321401328100 ) ) ;
#71333=CARTESIAN_POINT ( 'NONE',  ( -0.7210809602247715278, -2.613618158232546091E-15, -0.3464511005275220379 ) ) ;
#71336=CARTESIAN_POINT ( 'NONE',  ( -0.7283464566929126471, -0.4536011799217367080, 0.2665933059059888421 ) ) ;
#71337=CARTESIAN_POINT ( 'NONE',  ( -1.489501312335957062, -0.05778040916215522460, 0.4822834645669289988 ) ) ;
#71338=CARTESIAN_POINT ( 'NONE',  ( 0.7020997375328090762, -0.3162353388693405765, 0.4822834645669290543 ) ) ;
#71339=VERTEX_POINT ( 'NONE', #35653 ) ;
#71342=CARTESIAN_POINT ( 'NONE',  ( 1.167979002624672580, -0.4281496062992124485, 0.4176697321401328655 ) ) ;
#71343=CARTESIAN_POINT ( 'NONE',  ( -1.574803149606298636, -0.1870078740157479769, 0.4822834645669291653 ) ) ;
#71345=CARTESIAN_POINT ( 'NONE',  ( -0.2952755905511804668, 0.07958543189024085140, 0.2665933059059887866 ) ) ;
#71346=CARTESIAN_POINT ( 'NONE',  ( -1.587926509186350810, -0.004921259842519870586, -0.3153832671262229437 ) ) ;
#71348=CARTESIAN_POINT ( 'NONE',  ( 0.4396325459317590445, -0.6692913385826771977, 0.1292274648535927661 ) ) ;
#71349=CARTESIAN_POINT ( 'NONE',  ( -0.4461942257217840213, -0.5023911411419708095, -0.1820866141732282451 ) ) ;
#71350=CARTESIAN_POINT ( 'NONE',  ( 0.04593175853018440641, 0.1771653543307087075, -0.09757992244046823083 ) ) ;
#71352=CARTESIAN_POINT ( 'NONE',  ( 0.1115485564304467270, -0.6692913385826773087, -0.1292274648535924053 ) ) ;
#71353=CARTESIAN_POINT ( 'NONE',  ( -1.043307086614172041, -0.4536011799217367080, 0.2665933059059888421 ) ) ;
#71355=CARTESIAN_POINT ( 'NONE',  ( 0.8398950131233602345, 0.2306618581243847221, -0.2411417322834647770 ) ) ;
#71356=CARTESIAN_POINT ( 'NONE',  ( -1.581364829396324945, -0.05778040916215560624, -0.4822834645669293319 ) ) ;
#71358=CARTESIAN_POINT ( 'NONE',  ( -0.4658792650918627265, -0.05778040916215522460, 0.4822834645669289988 ) ) ;
#71359=CARTESIAN_POINT ( 'NONE',  ( 0.2624671916010504757, -0.5023911411419708095, -0.1820866141732282451 ) ) ;
#71360=CARTESIAN_POINT ( 'NONE',  ( -0.8595800524934373854, -0.05778040916215522460, 0.4822834645669289988 ) ) ;
#71361=CARTESIAN_POINT ( 'NONE',  ( 0.7152230971128616943, -0.08942795157527998196, 0.3641732283464567121 ) ) ;
#71362=CARTESIAN_POINT ( 'NONE',  ( -0.3018372703412066094, -0.004921259842519576551, 0.3153832671262227771 ) ) ;
#71363=CARTESIAN_POINT ( 'NONE',  ( -0.8398950131233589023, -0.6046776061558809534, -0.2411417322834644161 ) ) ;
#71364=CARTESIAN_POINT ( 'NONE',  ( -1.502624671916009680, -0.3162353388693405765, 0.4822834645669290543 ) ) ;
#71366=CARTESIAN_POINT ( 'NONE',  ( 1.377952755905512472, 0.1771653543307087630, 0.000000000000000000 ) ) ;
#71367=CARTESIAN_POINT ( 'NONE',  ( 0.5380577427821529035, -0.4281496062992124485, 0.4176697321401328655 ) ) ;
#71368=CARTESIAN_POINT ( 'NONE',  ( -1.410761154855641575, -0.3162353388693409650, -0.4822834645669289433 ) ) ;
#71369=CARTESIAN_POINT ( 'NONE',  ( -1.541994750656167090, 0.2952755905511811885, 0.1292274648535926551 ) ) ;
#71372=CARTESIAN_POINT ( 'NONE',  ( -1.043307086614172041, -0.4536011799217367080, 0.2665933059059888421 ) ) ;
#71373=CARTESIAN_POINT ( 'NONE',  ( 0.8727034120734912248, -0.3162353388693409650, -0.4822834645669289433 ) ) ;
#71374=CARTESIAN_POINT ( 'NONE',  ( -1.167979002624671470, -0.3690944881889765550, -0.3153832671262227771 ) ) ;
#71376=CARTESIAN_POINT ( 'NONE',  ( -1.102362204724408601, -0.1870078740157479769, 0.4822834645669291653 ) ) ;
#71377=CARTESIAN_POINT ( 'NONE',  ( 0.9448818897637802916, -0.1870078740157480879, -0.4822834645669291653 ) ) ;
#71378=CARTESIAN_POINT ( 'NONE',  ( 0.4265091863517067594, 0.2952755905511811885, 0.1292274648535926551 ) ) ;
#71379=CARTESIAN_POINT ( 'NONE',  ( 1.614173228346457378, 0.2753471884572478157, 0.1372047244094478646 ) ) ;
#71380=CARTESIAN_POINT ( 'NONE',  ( -1.699475065616797398, 0.1771653543307087630, 0.09757992244046791164 ) ) ;
#71386=CARTESIAN_POINT ( 'NONE',  ( 0.7414698162729663755, 0.1771653543307087630, 0.09757992244046791164 ) ) ;
#71387=CARTESIAN_POINT ( 'NONE',  ( 0.3149606299212603933, -0.1870078740157479769, 0.3641732283464567677 ) ) ;
#71388=CARTESIAN_POINT ( 'NONE',  ( 0.1640419947506569498, -0.05778040916215522460, 0.4822834645669289988 ) ) ;
#71389=CARTESIAN_POINT ( 'NONE',  ( 1.141732283464567566, 0.2952755905511811885, 0.000000000000000000 ) ) ;
#71391=CARTESIAN_POINT ( 'NONE',  ( 0.2427821522309719648, -0.08942795157527998196, 0.3641732283464567121 ) ) ;
#71392=CARTESIAN_POINT ( 'NONE',  ( -0.8333333333333323711, 0.2952755905511811885, 0.1292274648535926551 ) ) ;
#71393=CARTESIAN_POINT ( 'NONE',  ( -1.646981627296586703, -0.05778040916215522460, 0.4822834645669289988 ) ) ;
#71394=CARTESIAN_POINT ( 'NONE',  ( 0.6561679790026253567, -0.6046776061558809534, -0.2411417322834644161 ) ) ;
#71397=( BOUNDED_CURVE ( )  B_SPLINE_CURVE ( 2, ( #35614, #73930, #35202, #9124, #15023, #54125, #41514, #15866, #61277, #79839, #3630, #28050, #60453 ),
 .UNSPECIFIED., .F., .F. ) 
 B_SPLINE_CURVE_WITH_KNOTS ( ( 3, 2, 2, 2, 2, 2, 3 ),
 ( 0.7642401855438917258, 0.7651515151515151381, 0.7689393939393939226, 0.7727272727272727071, 0.7765151515151514916, 0.7803030303030302761, 0.7812143599106537994 ),
 .UNSPECIFIED. ) 
 CURVE ( )  GEOMETRIC_REPRESENTATION_ITEM ( )  RATIONAL_B_SPLINE_CURVE ( ( 0.9875488213027523443, 0.9918020599134680371, 1.000000000000000000, 0.9659258262890683122, 1.000000000000000000, 0.9659258262890683122, 1.000000000000000000, 0.9659258262890683122, 1.000000000000000000, 0.9659258262890683122, 1.000000000000000000, 0.9918020599134671489, 0.9875488213027514561 ) ) 
 REPRESENTATION_ITEM ( '' )  );
#71398=VERTEX_POINT ( 'NONE', #60493 ) ;
#71400=CARTESIAN_POINT ( 'NONE',  ( -1.338582677165353729, -0.1870078740157480879, -0.4822834645669291653 ) ) ;
#71401=CARTESIAN_POINT ( 'NONE',  ( -0.9973753280839886548, 0.2306618581243848609, 0.2411417322834645549 ) ) ;
#71402=CARTESIAN_POINT ( 'NONE',  ( -0.7677165354330699465, -0.4536011799217368745, -0.2665933059059886201 ) ) ;
#71403=CARTESIAN_POINT ( 'NONE',  ( -0.8464566929133852113, 0.1660481256975885056, 0.3530559997133364547 ) ) ;
#71406=CARTESIAN_POINT ( 'NONE',  ( -1.574803149606298192, -0.1870078740157480601, -0.3641732283464567677 ) ) ;
#71408=CARTESIAN_POINT ( 'NONE',  ( -1.423884514435694859, -0.3162353388693405765, 0.4822834645669290543 ) ) ;
#71409=CARTESIAN_POINT ( 'NONE',  ( 0.1443569553805781891, -0.4281496062992124485, 0.4176697321401328655 ) ) ;
#71410=CARTESIAN_POINT ( 'NONE',  ( -0.9514435695538050464, -0.05778040916215560624, -0.4822834645669293319 ) ) ;
#71412=CARTESIAN_POINT ( 'NONE',  ( 0.7677165354330716118, -0.5400638737290844871, 0.3530559997133364547 ) ) ;
#71414=CARTESIAN_POINT ( 'NONE',  ( -0.6430446194225712953, -0.004921259842519870586, -0.3153832671262229437 ) ) ;
#71418=CARTESIAN_POINT ( 'NONE',  ( -1.712598425196849572, 0.07958543189024085140, 0.2665933059059887866 ) ) ;
#71419=CARTESIAN_POINT ( 'NONE',  ( -1.128608923884513837, -0.6046776061558807314, 0.2411417322834647770 ) ) ;
#71420=CARTESIAN_POINT ( 'NONE',  ( -1.174540682414697335, -0.05778040916215522460, 0.4822834645669289988 ) ) ;
#71422=CARTESIAN_POINT ( 'NONE',  ( -0.9514435695538050464, -0.3162353388693405765, 0.4822834645669290543 ) ) ;
#71423=CARTESIAN_POINT ( 'NONE',  ( -1.207349081364828880, 0.2306618581243847221, -0.2411417322834647770 ) ) ;
#71424=CARTESIAN_POINT ( 'NONE',  ( -1.515748031496062076, -0.5400638737290844871, 0.3530559997133364547 ) ) ;
#71426=CARTESIAN_POINT ( 'NONE',  ( 0.2755905511811031494, 0.1771653543307087630, 0.000000000000000000 ) ) ;
#71429=CARTESIAN_POINT ( 'NONE',  ( -0.1640419947506555343, -0.2845877964562159024, 0.3641732283464567677 ) ) ;
#71430=CARTESIAN_POINT ( 'NONE',  ( -0.9842519685039360366, 0.2952755905511811885, 0.000000000000000000 ) ) ;
#71431=CARTESIAN_POINT ( 'NONE',  ( 0.8267716535433077274, 0.2952755905511811885, 0.000000000000000000 ) ) ;
#71432=CARTESIAN_POINT ( 'NONE',  ( -0.4199475065616791736, -0.6046776061558807314, 0.2411417322834647770 ) ) ;
#71436=CARTESIAN_POINT ( 'NONE',  ( -0.8595800524934373854, -0.05778040916215522460, 0.4822834645669289988 ) ) ;
#71437=CARTESIAN_POINT ( 'NONE',  ( 1.259842519685040019, -0.1870078740157479769, 0.4822834645669291653 ) ) ;
#71438=CARTESIAN_POINT ( 'NONE',  ( -1.397637795275589623, 0.07958543189024085140, 0.2665933059059887866 ) ) ;
#71443=CARTESIAN_POINT ( 'NONE',  ( -0.4265091863517051496, -0.6692913385826771977, 0.1292274648535927661 ) ) ;
#71444=CARTESIAN_POINT ( 'NONE',  ( -1.627296587926508442, 0.1283753931104748280, 0.1820866141732283561 ) ) ;
#71445=CARTESIAN_POINT ( 'NONE',  ( -0.7939632545931754048, -0.3162353388693405765, 0.4822834645669290543 ) ) ;
#71447=CARTESIAN_POINT ( 'NONE',  ( -1.482939632545930975, -0.4281496062992127816, -0.4176697321401328100 ) ) ;
#71449=CARTESIAN_POINT ( 'NONE',  ( -0.9317585301837263412, 0.05413385826771666132, 0.4176697321401328100 ) ) ;
#71450=CARTESIAN_POINT ( 'NONE',  ( -0.4658792650918627265, -0.05778040916215522460, 0.4822834645669289988 ) ) ;
#71452=CARTESIAN_POINT ( 'NONE',  ( 0.9120734908136489683, -0.5511811023622046335, 0.09757992244046803654 ) ) ;
#71454=CARTESIAN_POINT ( 'NONE',  ( 0.5643044619422579178, -0.004921259842519576551, 0.3153832671262227771 ) ) ;
#71455=CARTESIAN_POINT ( 'NONE',  ( 1.240157480314961314, -0.4536011799217367080, 0.2665933059059888421 ) ) ;
#71457=CARTESIAN_POINT ( 'NONE',  ( 1.574803149606299746, -0.1870078740157479769, 0.4822834645669291653 ) ) ;
#71459=CARTESIAN_POINT ( 'NONE',  ( 0.1706036745406830368, -0.3690944881889765550, -0.3153832671262227771 ) ) ;
#71461=CARTESIAN_POINT ( 'NONE',  ( -1.325459317585300889, 0.05413385826771666132, 0.4176697321401328100 ) ) ;
#71462=CARTESIAN_POINT ( 'NONE',  ( 1.253280839895013710, -0.3162353388693405765, 0.4822834645669290543 ) ) ;
#71464=CARTESIAN_POINT ( 'NONE',  ( -0.5971128608923877978, -0.5511811023622048555, -0.09757992244046775898 ) ) ;
#71465=CARTESIAN_POINT ( 'NONE',  ( -0.4133858267716528090, 0.1660481256975883391, -0.3530559997133364547 ) ) ;
#71466=CARTESIAN_POINT ( 'NONE',  ( 0.3543307086614181922, -0.6692913385826771977, 8.415575281601705876E-17 ) ) ;
#71467=DIRECTION ( 'NONE',  ( 0.000000000000000000, 1.000000000000000000, 0.000000000000000000 ) ) ;
#71468=CARTESIAN_POINT ( 'NONE',  ( 0.9317585301837276734, -0.3690944881889763329, 0.3153832671262228327 ) ) ;
#71469=CARTESIAN_POINT ( 'NONE',  ( 0.1443569553805781891, -0.3690944881889763329, 0.3153832671262228327 ) ) ;
#71470=CARTESIAN_POINT ( 'NONE',  ( -0.2624671916010490880, -0.6046776061558807314, 0.2411417322834647770 ) ) ;
#71471=CARTESIAN_POINT ( 'NONE',  ( -1.443569553805773564, -0.6046776061558807314, 0.2411417322834647770 ) ) ;
#71472=CARTESIAN_POINT ( 'NONE',  ( -0.7217847769028863381, -0.3690944881889763329, 0.3153832671262228327 ) ) ;
#71474=CARTESIAN_POINT ( 'NONE',  ( 0.4724409448818904789, -0.1870078740157480879, -0.4822834645669291653 ) ) ;
#71475=CARTESIAN_POINT ( 'NONE',  ( -0.9842519685039360366, 0.2952755905511811885, 0.000000000000000000 ) ) ;
#71477=ADVANCED_FACE ( 'NONE', ( #68064 ), #16418, .F. ) ;
#71479=CARTESIAN_POINT ( 'NONE',  ( 0.3674540682414705883, 0.1283753931104746893, -0.1820866141732285504 ) ) ;
#71480=CARTESIAN_POINT ( 'NONE',  ( -0.9251968503937002541, -0.5400638737290845981, -0.3530559997133363437 ) ) ;
#71481=CARTESIAN_POINT ( 'NONE',  ( -1.240157480314959759, -0.5400638737290845981, -0.3530559997133363437 ) ) ;
#71482=CARTESIAN_POINT ( 'NONE',  ( -1.272965879265091305, -0.004921259842519870586, -0.3153832671262229437 ) ) ;
#71483=CARTESIAN_POINT ( 'NONE',  ( 1.607611548556431069, -0.6692913385826773087, -0.1292274648535924053 ) ) ;
#71484=CARTESIAN_POINT ( 'NONE',  ( -0.6824146981627288167, 0.1283753931104748280, 0.1820866141732283561 ) ) ;
#71485=CARTESIAN_POINT ( 'NONE',  ( -0.7545931758530176614, 0.2066929133858267931, 0.1054918080437490802 ) ) ;
#71486=CARTESIAN_POINT ( 'NONE',  ( 1.502624671916010790, -0.3162353388693409650, -0.4822834645669289433 ) ) ;
#71491=CARTESIAN_POINT ( 'NONE',  ( 1.371391076115485719, -0.5511811023622048555, -0.09757992244046775898 ) ) ;
#71492=CARTESIAN_POINT ( 'NONE',  ( -1.496062992125983815, -0.1870078740157480879, -0.4822834645669291653 ) ) ;
#71493=CARTESIAN_POINT ( 'NONE',  ( 1.135170603674541256, 0.2952755905511811885, 0.1292274648535926551 ) ) ;
#71496=CARTESIAN_POINT ( 'NONE',  ( 0.6036745406824154392, 0.2306618581243847221, -0.2411417322834647770 ) ) ;
#71497=CARTESIAN_POINT ( 'NONE',  ( 0.1968503937007881344, -0.6692913385826771977, 8.415575281601705876E-17 ) ) ;
#71500=CARTESIAN_POINT ( 'NONE',  ( 0.6364829396325465405, -0.08942795157527998196, 0.3641732283464567121 ) ) ;
#71505=CARTESIAN_POINT ( 'NONE',  ( 0.05905511811023681640, 0.1660481256975883668, -0.3530559997133364547 ) ) ;
#71507=CARTESIAN_POINT ( 'NONE',  ( 1.128608923884514947, 0.2306618581243848609, 0.2411417322834645549 ) ) ;
#71508=CARTESIAN_POINT ( 'NONE',  ( 0.5380577427821529035, -0.4281496062992124485, 0.4176697321401328655 ) ) ;
#71509=CARTESIAN_POINT ( 'NONE',  ( 1.266404199475066328, -0.3162353388693409650, -0.4822834645669289433 ) ) ;
#71510=CARTESIAN_POINT ( 'NONE',  ( -0.4396325459317577122, -0.6692913385826773087, -0.1292274648535924053 ) ) ;
#71511=CARTESIAN_POINT ( 'NONE',  ( 0.2230971128608929543, 0.05413385826771626580, -0.4176697321401330321 ) ) ;
#71512=CARTESIAN_POINT ( 'NONE',  ( -1.607611548556429737, 0.2952755905511810774, -0.1292274648535930714 ) ) ;
#71514=CARTESIAN_POINT ( 'NONE',  ( 1.207349081364829990, -0.6046776061558809534, -0.2411417322834644161 ) ) ;
#71515=CARTESIAN_POINT ( 'NONE',  ( 1.115485564304462551, -0.4281496062992127816, -0.4176697321401328100 ) ) ;
#71517=CARTESIAN_POINT ( 'NONE',  ( 0.2887139107611556010, 0.1283753931104746893, -0.1820866141732285504 ) ) ;
#71520=ORIENTED_EDGE ( 'NONE', *, *, #44498, .F. ) ;
#71521=CARTESIAN_POINT ( 'NONE',  ( -0.4461942257217840213, 0.1283753931104748280, 0.1820866141732283561 ) ) ;
#71522=CARTESIAN_POINT ( 'NONE',  ( -0.08530183727034056085, -0.3162353388693405765, 0.4822834645669290543 ) ) ;
#71524=CARTESIAN_POINT ( 'NONE',  ( 0.1837270341207354329, 0.2306618581243848609, 0.2411417322834645549 ) ) ;
#71525=CARTESIAN_POINT ( 'NONE',  ( 0.1443569553805781891, -0.4281496062992124485, 0.4176697321401328655 ) ) ;
#71526=CARTESIAN_POINT ( 'NONE',  ( -0.8333333333333323711, -0.6692913385826773087, -0.1292274648535924053 ) ) ;
#71527=CARTESIAN_POINT ( 'NONE',  ( 1.522309711286089939, 0.1283753931104748280, 0.1820866141732283561 ) ) ;
#71530=CARTESIAN_POINT ( 'NONE',  ( 0.9120734908136489683, -0.5511811023622046335, 0.09757992244046803654 ) ) ;
#71531=CARTESIAN_POINT ( 'NONE',  ( 0.3740157480314966754, -0.5400638737290844871, 0.3530559997133364547 ) ) ;
#71532=CARTESIAN_POINT ( 'NONE',  ( 0.9514435695538062676, -0.3162353388693409650, -0.4822834645669289433 ) ) ;
#71537=CARTESIAN_POINT ( 'NONE',  ( -0.6561679790026240244, -0.6046776061558807314, 0.2411417322834647770 ) ) ;
#71539=( BOUNDED_CURVE ( )  B_SPLINE_CURVE ( 1, ( #63481, #82845 ),
 .UNSPECIFIED., .F., .F. ) 
 B_SPLINE_CURVE_WITH_KNOTS ( ( 2, 2 ),
 ( 0.000000000000000000, 0.002000000000000001776 ),
 .UNSPECIFIED. ) 
 CURVE ( )  GEOMETRIC_REPRESENTATION_ITEM ( )  RATIONAL_B_SPLINE_CURVE ( ( 0.9875488213027530104, 0.9875488213027530104 ) ) 
 REPRESENTATION_ITEM ( '' )  );
#71541=CARTESIAN_POINT ( 'NONE',  ( -1.174540682414697335, -0.08942795157527998196, 0.3641732283464567121 ) ) ;
#71542=CARTESIAN_POINT ( 'NONE',  ( 1.115485564304462551, 0.05413385826771666132, 0.4176697321401328100 ) ) ;
#71543=CARTESIAN_POINT ( 'NONE',  ( 0.9120734908136490793, 0.2952755905511810774, -0.1292274648535930714 ) ) ;
#71544=CARTESIAN_POINT ( 'NONE',  ( -0.4396325459317577122, -0.5511811023622048555, -0.09757992244046775898 ) ) ;
#71545=CARTESIAN_POINT ( 'NONE',  ( 0.2952755905511816326, -0.5400638737290844871, 0.3530559997133364547 ) ) ;
#71547=CARTESIAN_POINT ( 'NONE',  ( 0.2230971128608932319, -0.3690944881889763329, 0.3153832671262228327 ) ) ;
#71548=CARTESIAN_POINT ( 'NONE',  ( 0.03937007874015806264, 0.2952755905511811885, 0.000000000000000000 ) ) ;
#71550=CARTESIAN_POINT ( 'NONE',  ( -1.174540682414697335, -0.3162353388693409650, -0.4822834645669289433 ) ) ;
#71551=CARTESIAN_POINT ( 'NONE',  ( 0.4396325459317590445, -0.5511811023622046335, 0.09757992244046803654 ) ) ;
#71553=CARTESIAN_POINT ( 'NONE',  ( -0.6430446194225716283, -0.4281496062992124485, 0.4176697321401328655 ) ) ;
#71554=CARTESIAN_POINT ( 'NONE',  ( -0.5052493438320203589, 0.1771653543307087075, -0.09757992244046823083 ) ) ;
#71556=CARTESIAN_POINT ( 'NONE',  ( -0.5380577427821514602, -0.4281496062992127816, -0.4176697321401328100 ) ) ;
#71557=CARTESIAN_POINT ( 'NONE',  ( -0.5446194225721777693, -0.05778040916215522460, 0.4822834645669289988 ) ) ;
#71558=CARTESIAN_POINT ( 'NONE',  ( 0.4724409448818904789, -0.1870078740157479769, 0.3641732283464567677 ) ) ;
#71560=CARTESIAN_POINT ( 'NONE',  ( -0.1509186351706028884, -0.3162353388693409650, -0.4822834645669289433 ) ) ;
#71563=CARTESIAN_POINT ( 'NONE',  ( 0.9580052493438327987, -0.3690944881889765550, -0.3153832671262227771 ) ) ;
#71564=CARTESIAN_POINT ( 'NONE',  ( 1.594488188976378673, 0.1660481256975885056, 0.3530559997133364547 ) ) ;
#71565=CARTESIAN_POINT ( 'NONE',  ( -1.017060367454067249, -0.2845877964562161244, -0.3641732283464567121 ) ) ;
#71566=CARTESIAN_POINT ( 'NONE',  ( -1.253280839895012377, -0.08942795157527998196, 0.3641732283464567121 ) ) ;
#71567=CARTESIAN_POINT ( 'NONE',  ( -0.7939632545931750718, -0.05778040916215560624, -0.4822834645669293319 ) ) ;
#71568=CARTESIAN_POINT ( 'NONE',  ( 0.03280839895013198948, 0.2952755905511811885, 0.1292274648535926551 ) ) ;
#71569=CARTESIAN_POINT ( 'NONE',  ( 0.3674540682414705883, -0.5023911411419708095, 0.1820866141732285504 ) ) ;
#71571=CARTESIAN_POINT ( 'NONE',  ( 0.8792650918635177559, -0.3690944881889765550, -0.3153832671262227771 ) ) ;
#71572=CARTESIAN_POINT ( 'NONE',  ( 0.1706036745406830368, -0.4281496062992127816, -0.4176697321401328100 ) ) ;
#71574=CARTESIAN_POINT ( 'NONE',  ( -0.5183727034120726440, -0.6692913385826773087, -0.1292274648535924053 ) ) ;
#71576=CARTESIAN_POINT ( 'NONE',  ( 1.338582677165355062, -0.1870078740157480601, -0.3641732283464567677 ) ) ;
#71577=CARTESIAN_POINT ( 'NONE',  ( 0.3871391076115493490, -0.3162353388693405765, 0.4822834645669290543 ) ) ;
#71578=CARTESIAN_POINT ( 'NONE',  ( 0.1115485564304470323, 0.2952755905511811885, 0.1292274648535926551 ) ) ;
#71579=DIRECTION ( 'NONE',  ( -0.000000000000000000, 1.000000000000000000, -0.000000000000000000 ) ) ;
#71580=CARTESIAN_POINT ( 'NONE',  ( 0.04593175853018440641, -0.5511811023622046335, 0.09757992244046803654 ) ) ;
#71581=CARTESIAN_POINT ( 'NONE',  ( 0.9251968503937015864, 0.1660481256975883668, -0.3530559997133364547 ) ) ;
#71582=CARTESIAN_POINT ( 'NONE',  ( -0.2230971128608915943, -0.3690944881889765550, -0.3153832671262227771 ) ) ;
#71583=CARTESIAN_POINT ( 'NONE',  ( -0.8530183727034112984, 0.05413385826771666132, 0.4176697321401328100 ) ) ;
#71585=CARTESIAN_POINT ( 'NONE',  ( -0.3412073490813641308, -0.6046776061558807314, 0.2411417322834647770 ) ) ;
#71587=CARTESIAN_POINT ( 'NONE',  ( -1.049868766404198794, -0.6046776061558807314, 0.2411417322834647770 ) ) ;
#71588=CARTESIAN_POINT ( 'NONE',  ( -0.6102362204724400829, 0.07958543189024085140, 0.2665933059059887866 ) ) ;
#71589=CARTESIAN_POINT ( 'NONE',  ( -0.03280839895013062252, -0.6692913385826771977, 0.1292274648535927661 ) ) ;
#71590=CARTESIAN_POINT ( 'NONE',  ( -1.286089238845143479, -0.6046776061558807314, 0.2411417322834647770 ) ) ;
#71591=CARTESIAN_POINT ( 'NONE',  ( -0.5643044619422565855, -0.4281496062992124485, 0.4176697321401328655 ) ) ;
#71592=CARTESIAN_POINT ( 'NONE',  ( 2.795275590551181910, 1.535433070866142335, 0.000000000000000000 ) ) ;
#71593=CARTESIAN_POINT ( 'NONE',  ( 1.646981627296588035, -0.3162353388693405765, 0.4822834645669290543 ) ) ;
#71594=CARTESIAN_POINT ( 'NONE',  ( 0.8595800524934390507, -0.05778040916215560624, -0.4822834645669293319 ) ) ;
#71595=CARTESIAN_POINT ( 'NONE',  ( 1.082677165354331228, 0.1660481256975883668, -0.3530559997133364547 ) ) ;
#71598=CARTESIAN_POINT ( 'NONE',  ( -1.253280839895012377, -0.05778040916215522460, 0.4822834645669289988 ) ) ;
#71601=ORIENTED_EDGE ( 'NONE', *, *, #72820, .T. ) ;
#71602=CARTESIAN_POINT ( 'NONE',  ( 0.07874015748031558404, -0.1870078740157479769, 0.3641732283464567677 ) ) ;
#71605=CARTESIAN_POINT ( 'NONE',  ( 0.4199475065616803948, -0.6046776061558809534, -0.2411417322834644161 ) ) ;
#71606=CARTESIAN_POINT ( 'NONE',  ( -0.09842519685039295696, 0.1660481256975883668, -0.3530559997133364547 ) ) ;
#71607=CARTESIAN_POINT ( 'NONE',  ( -0.7349081364829387342, -0.6046776061558807314, 0.2411417322834647770 ) ) ;
#71609=CARTESIAN_POINT ( 'NONE',  ( -0.7217847769028863381, -0.3690944881889763329, 0.3153832671262228327 ) ) ;
#71610=CARTESIAN_POINT ( 'NONE',  ( 0.3608923884514443348, 0.2952755905511810219, -0.1292274648535930437 ) ) ;
#71611=CARTESIAN_POINT ( 'NONE',  ( 0.7414698162729663755, 0.2952755905511811885, 0.1292274648535926551 ) ) ;
#71613=CARTESIAN_POINT ( 'NONE',  ( 0.8267716535433077274, 0.1771653543307087630, 0.000000000000000000 ) ) ;
#71614=CARTESIAN_POINT ( 'NONE',  ( -0.4461942257217840213, -0.6046776061558809534, -0.2411417322834644161 ) ) ;
#71616=CARTESIAN_POINT ( 'NONE',  ( -0.9317585301837263412, -0.4281496062992127816, -0.4176697321401328100 ) ) ;
#71618=CARTESIAN_POINT ( 'NONE',  ( 1.528871391076116026, 0.2952755905511811885, 0.1292274648535926551 ) ) ;
#71622=CARTESIAN_POINT ( 'NONE',  ( 0.06561679790026316017, -0.4281496062992124485, 0.4176697321401328655 ) ) ;
#71623=ORIENTED_EDGE ( 'NONE', *, *, #46286, .T. ) ;
#71624=CARTESIAN_POINT ( 'NONE',  ( -0.6758530183727028406, -0.6692913385826773087, -0.1292274648535924053 ) ) ;
#71625=CARTESIAN_POINT ( 'NONE',  ( 1.194225721784777594, -0.4281496062992127816, -0.4176697321401328100 ) ) ;
#71626=CARTESIAN_POINT ( 'NONE',  ( 1.443569553805774897, 0.2306618581243848609, 0.2411417322834645549 ) ) ;
#71627=CARTESIAN_POINT ( 'NONE',  ( 0.1706036745406830368, 0.05413385826771666132, 0.4176697321401328100 ) ) ;
#71629=CARTESIAN_POINT ( 'NONE',  ( -0.4068241469816264999, -0.4281496062992124485, 0.4176697321401328655 ) ) ;
#71631=CARTESIAN_POINT ( 'NONE',  ( -1.056430446194224881, 0.2952755905511810774, -0.1292274648535930714 ) ) ;
#71632=CARTESIAN_POINT ( 'NONE',  ( -0.1706036745406816491, 0.05413385826771626580, -0.4176697321401330321 ) ) ;
#71633=CARTESIAN_POINT ( 'NONE',  ( -0.03937007874015669567, 0.1771653543307087630, 0.000000000000000000 ) ) ;
#71634=CARTESIAN_POINT ( 'NONE',  ( 1.561679790026247350, 0.05413385826771626580, -0.4176697321401330321 ) ) ;
#71635=CARTESIAN_POINT ( 'NONE',  ( 1.456692913385827515, -0.6692913385826771977, 8.415575281601705876E-17 ) ) ;
#71636=CARTESIAN_POINT ( 'NONE',  ( -0.6561679790026240244, -0.6046776061558807314, 0.2411417322834647770 ) ) ;
#71638=CARTESIAN_POINT ( 'NONE',  ( 1.023622047244095112, -0.1870078740157480879, -0.4822834645669291653 ) ) ;
#71641=VERTEX_POINT ( 'NONE', #62160 ) ;
#71642=CARTESIAN_POINT ( 'NONE',  ( 0.3674540682414705883, -0.6046776061558807314, 0.2411417322834647770 ) ) ;
#71643=CARTESIAN_POINT ( 'NONE',  ( -0.1706036745406816491, -0.3690944881889763329, 0.3153832671262228327 ) ) ;
#71644=CARTESIAN_POINT ( 'NONE',  ( 0.9055118110236227702, 0.1771653543307087630, 0.000000000000000000 ) ) ;
#71645=CARTESIAN_POINT ( 'NONE',  ( -0.8989501312335947958, 0.2066929133858267098, -0.1054918080437494132 ) ) ;
#71648=CARTESIAN_POINT ( 'NONE',  ( 1.351706036745407458, -0.4281496062992127816, -0.4176697321401328100 ) ) ;
#71650=CARTESIAN_POINT ( 'NONE',  ( 0.03937007874015806264, 0.2952755905511811885, 0.000000000000000000 ) ) ;
#71651=CARTESIAN_POINT ( 'NONE',  ( -1.653543307086613234, -0.1870078740157479769, 0.4822834645669291653 ) ) ;
#71652=CARTESIAN_POINT ( 'NONE',  ( -1.633858267716534529, -0.5400638737290845981, -0.3530559997133363437 ) ) ;
#71653=CARTESIAN_POINT ( 'NONE',  ( -0.2559055118110230564, 0.1660481256975883668, -0.3530559997133364547 ) ) ;
#71655=CARTESIAN_POINT ( 'NONE',  ( -1.614173228346455824, 0.1771653543307087630, 0.000000000000000000 ) ) ;
#71656=CARTESIAN_POINT ( 'NONE',  ( 0.4330708661417329575, -0.6692913385826771977, 8.415575281601705876E-17 ) ) ;
#71657=CARTESIAN_POINT ( 'NONE',  ( 0.9776902887139113929, -0.5511811023622048555, -0.09757992244046775898 ) ) ;
#71658=CARTESIAN_POINT ( 'NONE',  ( -0.01158586635040114929, 0.02791078216816508459, -0.4328096321851889194 ) ) ;
#71660=CARTESIAN_POINT ( 'NONE',  ( 0.3412073490813655186, -0.5023911411419708095, -0.1820866141732282451 ) ) ;
#71661=CARTESIAN_POINT ( 'NONE',  ( -1.305774278215222184, 0.2952755905511811885, 0.1292274648535926551 ) ) ;
#71663=CARTESIAN_POINT ( 'NONE',  ( 1.351706036745407680, 0.05413385826771666132, 0.4176697321401328100 ) ) ;
#71665=CARTESIAN_POINT ( 'NONE',  ( 0.8858267716535438430, 0.1660481256975885056, 0.3530559997133364547 ) ) ;
#71668=CARTESIAN_POINT ( 'NONE',  ( 0.6036745406824153282, -0.5023911411419708095, 0.1820866141732285504 ) ) ;
#71669=CARTESIAN_POINT ( 'NONE',  ( 0.6496062992125991586, -0.5400638737290845981, -0.3530559997133363437 ) ) ;
#71671=CARTESIAN_POINT ( 'NONE',  ( -0.7545931758530177724, 0.1771653543307087630, 0.09757992244046791164 ) ) ;
#71672=CARTESIAN_POINT ( 'NONE',  ( -0.8661417322834640276, -0.1870078740157480879, -0.4822834645669291653 ) ) ;
#71674=CARTESIAN_POINT ( 'NONE',  ( -1.541994750656167090, 0.2952755905511811885, 0.1292274648535926551 ) ) ;
#71675=CARTESIAN_POINT ( 'NONE',  ( 0.8858267716535438430, 0.1660481256975885056, 0.3530559997133364547 ) ) ;
#71676=CARTESIAN_POINT ( 'NONE',  ( 1.496062992125985147, -0.1870078740157479769, 0.4822834645669291653 ) ) ;
#71678=CARTESIAN_POINT ( 'NONE',  ( 0.9842519685039375910, 0.2952755905511811885, 0.000000000000000000 ) ) ;
#71680=CARTESIAN_POINT ( 'NONE',  ( 1.679790026246720025, 0.2306618581243848609, 0.2411417322834645549 ) ) ;
#71681=CARTESIAN_POINT ( 'NONE',  ( 1.450131233595801428, -0.6692913385826773087, -0.1292274648535924053 ) ) ;
#71682=CARTESIAN_POINT ( 'NONE',  ( -1.489501312335957062, -0.2845877964562161244, -0.3641732283464567121 ) ) ;
#71683=CARTESIAN_POINT ( 'NONE',  ( 1.345144356955381593, -0.08942795157527998196, 0.3641732283464567121 ) ) ;
#71684=CARTESIAN_POINT ( 'NONE',  ( -1.240157480314959759, -0.4536011799217368745, -0.2665933059059886201 ) ) ;
#71685=CARTESIAN_POINT ( 'NONE',  ( -0.6233595800524928121, -0.2845877964562161244, -0.3641732283464567121 ) ) ;
#71687=CARTESIAN_POINT ( 'NONE',  ( 0.7349081364829402885, -0.5023911411419708095, -0.1820866141732282451 ) ) ;
#71689=CARTESIAN_POINT ( 'NONE',  ( 0.7283464566929143125, 0.1660481256975885056, 0.3530559997133364547 ) ) ;
#71690=CARTESIAN_POINT ( 'NONE',  ( 0.9711286089238851948, 0.2306618581243848609, 0.2411417322834645549 ) ) ;
#71691=CARTESIAN_POINT ( 'NONE',  ( -0.1312335958005241554, -0.6046776061558809534, -0.2411417322834644161 ) ) ;
#71692=CARTESIAN_POINT ( 'NONE',  ( 0.7545931758530188826, -0.5511811023622046335, 0.09757992244046803654 ) ) ;
#71693=CARTESIAN_POINT ( 'NONE',  ( 1.194225721784777594, -0.4281496062992127816, -0.4176697321401328100 ) ) ;
#71694=CARTESIAN_POINT ( 'NONE',  ( -0.2234477481026881651, 0.004960608223778821026, 0.3437734562760189072 ) ) ;
#71695=CARTESIAN_POINT ( 'NONE',  ( -0.5380577427821514602, -0.4281496062992127816, -0.4176697321401328100 ) ) ;
#71697=CYLINDRICAL_SURFACE ( 'NONE', #552, 1.181102362204724310 ) ;
#71698=CARTESIAN_POINT ( 'NONE',  ( 0.2034120734908142214, 0.2952755905511810774, -0.1292274648535930714 ) ) ;
#71699=CARTESIAN_POINT ( 'NONE',  ( -0.4002624671916004129, -0.3162353388693405765, 0.4822834645669290543 ) ) ;
#71700=CARTESIAN_POINT ( 'NONE',  ( -0.1968503937007867743, -0.6692913385826771977, 8.415575281601705876E-17 ) ) ;
#71706=CARTESIAN_POINT ( 'NONE',  ( -0.9055118110236215490, 0.1771653543307087630, 0.000000000000000000 ) ) ;
#71708=CARTESIAN_POINT ( 'NONE',  ( -0.9973753280839886548, -0.6046776061558809534, -0.2411417322834644161 ) ) ;
#71710=CARTESIAN_POINT ( 'NONE',  ( 0.3346456692913393205, -0.5400638737290845981, -0.3530559997133363437 ) ) ;
#71711=CARTESIAN_POINT ( 'NONE',  ( -0.6233595800524928121, -0.08942795157527998196, 0.3641732283464567121 ) ) ;
#71712=CARTESIAN_POINT ( 'NONE',  ( 1.089238845144357537, -0.4281496062992124485, 0.4176697321401328655 ) ) ;
#71713=CARTESIAN_POINT ( 'NONE',  ( 0.2034120734908142214, 0.2952755905511810774, -0.1292274648535930714 ) ) ;
#71717=CARTESIAN_POINT ( 'NONE',  ( 1.391076115485564868, 0.2306618581243847221, -0.2411417322834647770 ) ) ;
#71718=CARTESIAN_POINT ( 'NONE',  ( 0.5052493438320215802, 0.2952755905511811885, 0.1292274648535926551 ) ) ;
#71719=CARTESIAN_POINT ( 'NONE',  ( 0.03280839895013198948, 0.2952755905511811885, 0.1292274648535926551 ) ) ;
#71720=CARTESIAN_POINT ( 'NONE',  ( 1.463254593175853824, 0.2952755905511810774, -0.1292274648535930714 ) ) ;
#71721=CARTESIAN_POINT ( 'NONE',  ( 0.7545931758530189937, 0.2952755905511810774, -0.1292274648535930714 ) ) ;
#71723=CARTESIAN_POINT ( 'NONE',  ( 0.2034120734908142214, 0.2952755905511810774, -0.1292274648535930714 ) ) ;
#71724=CARTESIAN_POINT ( 'NONE',  ( 1.076115485564305141, 0.2306618581243847221, -0.2411417322834647770 ) ) ;
#71725=CARTESIAN_POINT ( 'NONE',  ( 0.3412073490813655186, -0.6046776061558809534, -0.2411417322834644161 ) ) ;
#71726=CIRCLE ( 'NONE', #34058, 1.220472440944881942 ) ;
#71727=CARTESIAN_POINT ( 'NONE',  ( 0.9514435695538062676, -0.2845877964562161244, -0.3641732283464567121 ) ) ;
#71728=CARTESIAN_POINT ( 'NONE',  ( -0.8070866141732276899, -0.5400638737290844871, 0.3530559997133364547 ) ) ;
#71729=CARTESIAN_POINT ( 'NONE',  ( -1.240157480314959759, 0.1660481256975885056, 0.3530559997133364547 ) ) ;
#71730=CARTESIAN_POINT ( 'NONE',  ( 0.6430446194225728496, 0.05413385826771666132, 0.4176697321401328100 ) ) ;
#71736=CARTESIAN_POINT ( 'NONE',  ( 1.607611548556431069, -0.6692913385826773087, -0.1292274648535924053 ) ) ;
#71737=CARTESIAN_POINT ( 'NONE',  ( 0.8136482939632553313, 0.1283753931104748280, 0.1820866141732283561 ) ) ;
#71742=AXIS2_PLACEMENT_3D ( 'NONE', #15732, #68316, #55650 ) ;
#71743=CARTESIAN_POINT ( 'NONE',  ( -1.227034120734907141, -0.5511811023622048555, -0.09757992244046775898 ) ) ;
#71744=CARTESIAN_POINT ( 'NONE',  ( 1.535433070866142335, -0.6692913385826771977, 8.415575281601705876E-17 ) ) ;
#71746=CARTESIAN_POINT ( 'NONE',  ( -0.1509186351706028884, -0.05778040916215522460, 0.4822834645669289988 ) ) ;
#71747=CARTESIAN_POINT ( 'NONE',  ( 1.108923884514436242, -0.05778040916215522460, 0.4822834645669289988 ) ) ;
#71749=CARTESIAN_POINT ( 'NONE',  ( -1.653543307086613234, -0.1870078740157480879, -0.4822834645669291653 ) ) ;
#71750=CARTESIAN_POINT ( 'NONE',  ( 0.5157744752565104340, 1.509207849855103811, 0.5177606540819029712 ) ) ;
#71751=LINE ( 'NONE', #18742, #17019 ) ;
#71753=CARTESIAN_POINT ( 'NONE',  ( -0.9055118110236215490, -0.5511811023622047445, 6.969142054262312111E-17 ) ) ;
#71754=CARTESIAN_POINT ( 'NONE',  ( -1.502624671916009680, -0.3162353388693405765, 0.4822834645669290543 ) ) ;
#71755=CARTESIAN_POINT ( 'NONE',  ( 0.4461942257217856311, 0.2306618581243847221, -0.2411417322834647770 ) ) ;
#71758=LINE ( 'NONE', #62436, #27787 ) ;
#71760=CARTESIAN_POINT ( 'NONE',  ( 0.7283464566929143125, 0.1660481256975885056, 0.3530559997133364547 ) ) ;
#71761=CARTESIAN_POINT ( 'NONE',  ( -1.541994750656167090, 0.2952755905511811885, 0.1292274648535926551 ) ) ;
#71763=CARTESIAN_POINT ( 'NONE',  ( -1.010498687664041384, -0.3690944881889765550, -0.3153832671262227771 ) ) ;
#71764=CARTESIAN_POINT ( 'NONE',  ( 1.679790026246720025, 0.2306618581243848609, 0.2411417322834645549 ) ) ;
#71765=CARTESIAN_POINT ( 'NONE',  ( 0.4849061582275019378, 2.793565526369266028, -0.4921425059946357705 ) ) ;
#71766=CARTESIAN_POINT ( 'NONE',  ( 0.5249343832021003964, 0.2306618581243847221, -0.2411417322834647770 ) ) ;
#71768=CARTESIAN_POINT ( 'NONE',  ( -1.043307086614172041, -0.4536011799217367080, 0.2665933059059888421 ) ) ;
#71769=CARTESIAN_POINT ( 'NONE',  ( 0.006561679790026889343, -0.08942795157527998196, 0.3641732283464567121 ) ) ;
#71770=CARTESIAN_POINT ( 'NONE',  ( -0.4461942257217840213, 0.2306618581243848609, 0.2411417322834645549 ) ) ;
#71771=CARTESIAN_POINT ( 'NONE',  ( -1.174540682414697335, -0.08942795157527998196, 0.3641732283464567121 ) ) ;
#71773=CARTESIAN_POINT ( 'NONE',  ( 0.8661417322834652488, -0.1870078740157480879, -0.4822834645669291653 ) ) ;
#71774=CARTESIAN_POINT ( 'NONE',  ( -1.358267716535432434, -0.5400638737290844871, 0.3530559997133364547 ) ) ;
#71776=CARTESIAN_POINT ( 'NONE',  ( -0.9120734908136475250, 0.2952755905511811885, 0.1292274648535926551 ) ) ;
#71777=CARTESIAN_POINT ( 'NONE',  ( -0.2624671916010490880, 0.1283753931104746893, -0.1820866141732285504 ) ) ;
#71778=CARTESIAN_POINT ( 'NONE',  ( -1.305774278215222184, 0.2952755905511811885, 0.1292274648535926551 ) ) ;
#71779=CARTESIAN_POINT ( 'NONE',  ( 0.7611548556430454138, 0.1283753931104746893, -0.1820866141732285504 ) ) ;
#71780=CARTESIAN_POINT ( 'NONE',  ( -0.3543307086614165824, -0.5511811023622047445, 6.969142054262312111E-17 ) ) ;
#71781=CARTESIAN_POINT ( 'NONE',  ( -1.062992125984250968, 0.2952755905511811885, 0.000000000000000000 ) ) ;
#71782=CARTESIAN_POINT ( 'NONE',  ( -0.9973753280839886548, -0.6046776061558809534, -0.2411417322834644161 ) ) ;
#71783=CARTESIAN_POINT ( 'NONE',  ( -1.476377952755905110, 0.1660481256975885056, 0.3530559997133364547 ) ) ;
#71785=CARTESIAN_POINT ( 'NONE',  ( 1.161417322834646493, -0.4536011799217367080, 0.2665933059059888421 ) ) ;
#71787=CARTESIAN_POINT ( 'NONE',  ( 0.5314960629921267055, -0.5400638737290844871, 0.3530559997133364547 ) ) ;
#71788=CARTESIAN_POINT ( 'NONE',  ( -1.548556430446193399, -0.6046776061558809534, -0.2411417322834644161 ) ) ;
#71789=CARTESIAN_POINT ( 'NONE',  ( -1.515748031496062076, 0.1660481256975883668, -0.3530559997133364547 ) ) ;
#71793=CARTESIAN_POINT ( 'NONE',  ( -1.049868766404198794, -0.5023911411419708095, 0.1820866141732285504 ) ) ;
#71794=CARTESIAN_POINT ( 'NONE',  ( 0.9251968503937015864, -0.5400638737290844871, 0.3530559997133364547 ) ) ;
#71795=CARTESIAN_POINT ( 'NONE',  ( -1.240157480314959759, 0.07958543189024085140, 0.2665933059059887866 ) ) ;
#71797=CARTESIAN_POINT ( 'NONE',  ( -1.548556430446193399, 0.2306618581243848609, 0.2411417322834645549 ) ) ;
#71798=CARTESIAN_POINT ( 'NONE',  ( 0.9776902887139113929, -0.6692913385826773087, -0.1292274648535924053 ) ) ;
#71799=CARTESIAN_POINT ( 'NONE',  ( 0.5052493438320218022, -0.6692913385826773087, -0.1292274648535924053 ) ) ;
#71800=CARTESIAN_POINT ( 'NONE',  ( 1.141732283464567566, 0.2952755905511811885, 0.000000000000000000 ) ) ;
#71801=CARTESIAN_POINT ( 'NONE',  ( -1.332020997375327642, -0.2845877964562161244, -0.3641732283464567121 ) ) ;
#71804=ADVANCED_FACE ( 'NONE', ( #49935 ), #81520, .F. ) ;
#71807=DIRECTION ( 'NONE',  ( -1.000000000000000000, -3.083952846180990774E-16, 0.000000000000000000 ) ) ;
#71808=CARTESIAN_POINT ( 'NONE',  ( 0.6627296587926517768, -0.5511811023622048555, -0.09757992244046775898 ) ) ;
#71809=CARTESIAN_POINT ( 'NONE',  ( 0.2690288713910767848, -0.5511811023622048555, -0.09757992244046775898 ) ) ;
#71810=CARTESIAN_POINT ( 'NONE',  ( 0.1837270341207354329, 0.2306618581243848609, 0.2411417322834645549 ) ) ;
#71811=CARTESIAN_POINT ( 'NONE',  ( 1.463254593175853824, 0.2952755905511810774, -0.1292274648535930714 ) ) ;
#71813=CARTESIAN_POINT ( 'NONE',  ( 0.5905511811023629321, 0.1771653543307087630, 0.000000000000000000 ) ) ;
#71815=CARTESIAN_POINT ( 'NONE',  ( -0.8595800524934373854, -0.05778040916215522460, 0.4822834645669289988 ) ) ;
#71816=CARTESIAN_POINT ( 'NONE',  ( -1.515748031496062076, -0.5400638737290844871, 0.3530559997133364547 ) ) ;
#71817=CARTESIAN_POINT ( 'NONE',  ( 0.9580052493438327987, -0.4281496062992127816, -0.4176697321401328100 ) ) ;
#71821=EDGE_LOOP ( 'NONE', ( #25733, #52372, #3826, #74654 ) ) ;
#71822=CARTESIAN_POINT ( 'NONE',  ( -1.292650918635170010, -0.6692913385826771977, 0.1292274648535927661 ) ) ;
#71823=CARTESIAN_POINT ( 'NONE',  ( -0.9186351706036736120, -0.5023911411419708095, -0.1820866141732282451 ) ) ;
#71824=CARTESIAN_POINT ( 'NONE',  ( -1.292650918635170010, 0.2952755905511810774, -0.1292274648535930714 ) ) ;
#71826=DIRECTION ( 'NONE',  ( 0.000000000000000000, 0.000000000000000000, 1.000000000000000000 ) ) ;
#71827=CARTESIAN_POINT ( 'NONE',  ( 1.469816272965879911, -0.6046776061558807314, 0.2411417322834647770 ) ) ;
#71828=CARTESIAN_POINT ( 'NONE',  ( -1.043307086614172707, 0.1660481256975883668, -0.3530559997133364547 ) ) ;
#71829=CARTESIAN_POINT ( 'NONE',  ( 0.1968503937007881344, 0.2952755905511811885, 0.000000000000000000 ) ) ;
#71830=CARTESIAN_POINT ( 'NONE',  ( -1.259842519685038686, -0.1870078740157480879, -0.4822834645669291653 ) ) ;
#71833=CARTESIAN_POINT ( 'NONE',  ( 0.6167979002624678353, -0.4281496062992124485, 0.4176697321401328655 ) ) ;
#71835=CARTESIAN_POINT ( 'NONE',  ( -0.7545931758530176614, -0.5511811023622048555, -0.09757992244046775898 ) ) ;
#71838=ORIENTED_EDGE ( 'NONE', *, *, #51676, .T. ) ;
#71839=CARTESIAN_POINT ( 'NONE',  ( -0.6414174258557919783, -3.721645946415733147E-15, -0.3791475997938235643 ) ) ;
#71840=CARTESIAN_POINT ( 'NONE',  ( -1.154855643044618851, -0.6046776061558809534, -0.2411417322834644161 ) ) ;
#71841=CARTESIAN_POINT ( 'NONE',  ( -1.476377952755905110, 0.1660481256975885056, 0.3530559997133364547 ) ) ;
#71843=CARTESIAN_POINT ( 'NONE',  ( -1.666666666666665853, 0.05413385826771626580, -0.4176697321401330321 ) ) ;
#71844=CARTESIAN_POINT ( 'NONE',  ( -1.161417322834644716, -0.5400638737290845981, -0.3530559997133363437 ) ) ;
#71845=CARTESIAN_POINT ( 'NONE',  ( -1.607611548556429737, 0.2952755905511810774, -0.1292274648535930714 ) ) ;
#71848=CARTESIAN_POINT ( 'NONE',  ( 0.1246719160104994284, 0.1771653543307087075, -0.09757992244046823083 ) ) ;
#71851=CARTESIAN_POINT ( 'NONE',  ( -0.4396325459317579898, 0.1771653543307087630, 0.09757992244046791164 ) ) ;
#71853=CARTESIAN_POINT ( 'NONE',  ( -0.7545931758530176614, -0.6692913385826773087, -0.1292274648535924053 ) ) ;
#71854=CARTESIAN_POINT ( 'NONE',  ( 1.102362204724410155, -0.1870078740157479769, 0.4822834645669291653 ) ) ;
#71855=CARTESIAN_POINT ( 'NONE',  ( -0.7545931758530176614, -0.6692913385826773087, -0.1292274648535924053 ) ) ;
#71856=VERTEX_POINT ( 'NONE', #71379 ) ;
#71858=CARTESIAN_POINT ( 'NONE',  ( -1.082677165354329896, -0.5400638737290845981, -0.3530559997133363437 ) ) ;
#71859=CARTESIAN_POINT ( 'NONE',  ( 0.9776902887139113929, 0.2952755905511811885, 0.1292274648535926551 ) ) ;
#71860=CARTESIAN_POINT ( 'NONE',  ( -1.443569553805773564, -0.5023911411419708095, 0.1820866141732285504 ) ) ;
#71865=CARTESIAN_POINT ( 'NONE',  ( -0.1968503937007867743, 0.2952755905511811885, 0.000000000000000000 ) ) ;
#71866=CARTESIAN_POINT ( 'NONE',  ( 1.673228346456693494, 0.1660481256975885056, 0.3530559997133364547 ) ) ;
#71867=CARTESIAN_POINT ( 'NONE',  ( -0.7480314960629914633, 0.2952755905511811885, 0.000000000000000000 ) ) ;
#71869=CARTESIAN_POINT ( 'NONE',  ( -1.456692913385826182, -0.6692913385826771977, 8.415575281601705876E-17 ) ) ;
#71871=CARTESIAN_POINT ( 'NONE',  ( -0.9973753280839886548, -0.6046776061558809534, -0.2411417322834644161 ) ) ;
#71872=CARTESIAN_POINT ( 'NONE',  ( -0.1902887139107604098, -0.6692913385826771977, 0.1292274648535927661 ) ) ;
#71875=CARTESIAN_POINT ( 'NONE',  ( 0.4921259842519691285, 0.07958543189024085140, 0.2665933059059887866 ) ) ;
#71877=CARTESIAN_POINT ( 'NONE',  ( 0.2755905511811031494, 0.1771653543307087630, 0.000000000000000000 ) ) ;
#71878=CARTESIAN_POINT ( 'NONE',  ( 1.325459317585302665, -0.004921259842519870586, -0.3153832671262229437 ) ) ;
#71879=CARTESIAN_POINT ( 'NONE',  ( 1.292650918635171564, 0.2952755905511811885, 0.1292274648535926551 ) ) ;
#71880=CARTESIAN_POINT ( 'NONE',  ( 0.01312335958005323398, -0.3690944881889765550, -0.3153832671262227771 ) ) ;
#71882=CARTESIAN_POINT ( 'NONE',  ( -1.443569553805773564, 0.2306618581243847221, -0.2411417322834647770 ) ) ;
#71883=CARTESIAN_POINT ( 'NONE',  ( 1.338582677165355062, -0.1870078740157480879, -0.4822834645669291653 ) ) ;
#71885=CARTESIAN_POINT ( 'NONE',  ( -0.6561679790026240244, 0.1283753931104746893, -0.1820866141732285504 ) ) ;
#71886=CARTESIAN_POINT ( 'NONE',  ( 0.01158586635040232717, 0.02791078216816225699, 0.4328096321851905293 ) ) ;
#71887=CARTESIAN_POINT ( 'NONE',  ( 0.1837270341207357105, -0.6046776061558809534, -0.2411417322834644161 ) ) ;
#71889=CARTESIAN_POINT ( 'NONE',  ( 1.108923884514436242, -0.08942795157527998196, 0.3641732283464567121 ) ) ;
#71890=CARTESIAN_POINT ( 'NONE',  ( 0.2952755905511816326, -0.4536011799217367080, 0.2665933059059888421 ) ) ;
#71891=CARTESIAN_POINT ( 'NONE',  ( -0.09842519685039295696, -0.5400638737290844871, 0.3530559997133364547 ) ) ;
#71893=CARTESIAN_POINT ( 'NONE',  ( -0.6758530183727028406, 0.1771653543307087630, 0.09757992244046791164 ) ) ;
#71895=CARTESIAN_POINT ( 'NONE',  ( 0.3871391076115493490, -0.3162353388693405765, 0.4822834645669290543 ) ) ;
#71896=CARTESIAN_POINT ( 'NONE',  ( -0.9055118110236215490, -0.6692913385826771977, 8.415575281601705876E-17 ) ) ;
#71899=CARTESIAN_POINT ( 'NONE',  ( 0.1377952755905518800, -0.4536011799217367080, 0.2665933059059888421 ) ) ;
#71900=CARTESIAN_POINT ( 'NONE',  ( -0.8202099737532799750, 0.2952755905511810774, -0.1292274648535930714 ) ) ;
#71901=CARTESIAN_POINT ( 'NONE',  ( -1.095800524934382292, -0.3162353388693409650, -0.4822834645669289433 ) ) ;
#71902=CARTESIAN_POINT ( 'NONE',  ( -1.128608923884513837, 0.1283753931104746893, -0.1820866141732285504 ) ) ;
#71904=( BOUNDED_CURVE ( )  B_SPLINE_CURVE ( 2, ( #68494, #41979, #23039, #55016, #67261, #35674, #48705, #10834, #67673, #10009, #9594, #28116, #3277 ),
 .UNSPECIFIED., .F., .F. ) 
 B_SPLINE_CURVE_WITH_KNOTS ( ( 3, 2, 2, 2, 2, 2, 3 ),
 ( 0.3558514478433236206, 0.3560606060606060774, 0.3598484848484848619, 0.3636363636363636465, 0.3674242424242424310, 0.3712121212121212155, 0.3714212794294036724 ),
 .UNSPECIFIED. ) 
 CURVE ( )  GEOMETRIC_REPRESENTATION_ITEM ( )  RATIONAL_B_SPLINE_CURVE ( ( 0.9964447847208428577, 0.9981185001348096275, 1.000000000000000000, 0.9659258262890683122, 1.000000000000000000, 0.9659258262890683122, 1.000000000000000000, 0.9659258262890683122, 1.000000000000000000, 0.9659258262890683122, 1.000000000000000000, 0.9981185001348097385, 0.9964447847208430797 ) ) 
 REPRESENTATION_ITEM ( '' )  );
#71905=CARTESIAN_POINT ( 'NONE',  ( -1.023622047244093558, -0.1870078740157479769, 0.3641732283464567677 ) ) ;
#71906=FACE_OUTER_BOUND ( 'NONE', #22231, .T. ) ;
#71907=CARTESIAN_POINT ( 'NONE',  ( 0.6889763779527563470, 0.1660481256975883668, -0.3530559997133364547 ) ) ;
#71912=CARTESIAN_POINT ( 'NONE',  ( -0.9348729704079935532, -2.191421614605370878E-15, 0.4445507791589071167 ) ) ;
#71913=CARTESIAN_POINT ( 'NONE',  ( 1.450131233595801428, 0.1771653543307087630, 0.09757992244046791164 ) ) ;
#71914=CARTESIAN_POINT ( 'NONE',  ( -1.404199475065615932, 0.05413385826771666132, 0.4176697321401328100 ) ) ;
#71915=CARTESIAN_POINT ( 'NONE',  ( 1.056430446194226436, -0.6692913385826773087, -0.1292274648535924053 ) ) ;
#71917=CARTESIAN_POINT ( 'NONE',  ( 1.528871391076116026, 0.1771653543307087630, 0.09757992244046791164 ) ) ;
#71918=CARTESIAN_POINT ( 'NONE',  ( 0.4658792650918641698, -0.05778040916215560624, -0.4822834645669293319 ) ) ;
#71919=CARTESIAN_POINT ( 'NONE',  ( -0.2230971128608915943, 0.05413385826771666132, 0.4176697321401328100 ) ) ;
#71922=CARTESIAN_POINT ( 'NONE',  ( 0.6955380577427828781, -0.004921259842519870586, -0.3153832671262229437 ) ) ;
#71928=CARTESIAN_POINT ( 'NONE',  ( -0.09842519685039295696, 0.1660481256975883668, -0.3530559997133364547 ) ) ;
#71929=CARTESIAN_POINT ( 'NONE',  ( 1.345144356955381593, -0.3162353388693409650, -0.4822834645669289433 ) ) ;
#71930=CARTESIAN_POINT ( 'NONE',  ( 0.3280839895013130669, -0.4281496062992127816, -0.4176697321401328100 ) ) ;
#71931=CARTESIAN_POINT ( 'NONE',  ( 1.423884514435696413, -0.3162353388693409650, -0.4822834645669289433 ) ) ;
#71932=CARTESIAN_POINT ( 'NONE',  ( -0.5774278215223089816, -0.6046776061558807314, 0.2411417322834647770 ) ) ;
#71933=CARTESIAN_POINT ( 'NONE',  ( 0.01968503937007930540, 0.1660481256975885056, 0.3530559997133364547 ) ) ;
#71934=CARTESIAN_POINT ( 'NONE',  ( 1.437007874015748810, 0.1660481256975885056, 0.3530559997133364547 ) ) ;
#71935=CARTESIAN_POINT ( 'NONE',  ( 1.213910761154856299, -0.6692913385826773087, -0.1292274648535924053 ) ) ;
#71936=CARTESIAN_POINT ( 'NONE',  ( 0.9776902887139113929, -0.6692913385826773087, -0.1292274648535924053 ) ) ;
#71938=CARTESIAN_POINT ( 'NONE',  ( 0.3346456692913393205, -0.4536011799217368745, -0.2665933059059886201 ) ) ;
#71942=CARTESIAN_POINT ( 'NONE',  ( -0.5905511811023615998, 0.1771653543307087630, 0.000000000000000000 ) ) ;
#71943=CARTESIAN_POINT ( 'NONE',  ( -0.1706036745406816491, 0.05413385826771626580, -0.4176697321401330321 ) ) ;
#71945=CARTESIAN_POINT ( 'NONE',  ( -0.3937007874015740483, -0.1870078740157480879, -0.4822834645669291653 ) ) ;
#71946=CARTESIAN_POINT ( 'NONE',  ( 0.03937007874015806264, 0.2952755905511811885, 0.000000000000000000 ) ) ;
#71947=CARTESIAN_POINT ( 'NONE',  ( -0.8530183727034112984, 0.05413385826771666132, 0.4176697321401328100 ) ) ;
#71948=CARTESIAN_POINT ( 'NONE',  ( -1.187664041994750175, -0.05778040916215560624, -0.4822834645669293319 ) ) ;
#71949=CARTESIAN_POINT ( 'NONE',  ( 1.174540682414699111, -0.2845877964562159024, 0.3641732283464567677 ) ) ;
#71950=CARTESIAN_POINT ( 'NONE',  ( -1.620734908136482577, 0.2952755905511811885, 0.1292274648535926551 ) ) ;
#71952=CARTESIAN_POINT ( 'NONE',  ( 1.076115485564305141, -0.5023911411419708095, 0.1820866141732285504 ) ) ;
#71953=CARTESIAN_POINT ( 'NONE',  ( 0.4724409448818904789, -0.1870078740157480879, -0.4822834645669291653 ) ) ;
#71954=CARTESIAN_POINT ( 'NONE',  ( 0.6233595800524942554, -0.05778040916215560624, -0.4822834645669293319 ) ) ;
#71959=CARTESIAN_POINT ( 'NONE',  ( -0.7086614173228339419, -0.1870078740157480879, -0.4822834645669291653 ) ) ;
#71962=CARTESIAN_POINT ( 'NONE',  ( -1.102362204724408601, -0.1870078740157480601, -0.3641732283464567677 ) ) ;
#71963=CARTESIAN_POINT ( 'NONE',  ( 1.003937007874016185, 0.1660481256975883668, -0.3530559997133364547 ) ) ;
#71964=CARTESIAN_POINT ( 'NONE',  ( 1.128608923884515169, -0.6046776061558809534, -0.2411417322834644161 ) ) ;
#71965=CARTESIAN_POINT ( 'NONE',  ( -0.03937007874015669567, 0.1771653543307087630, 0.000000000000000000 ) ) ;
#71966=CARTESIAN_POINT ( 'NONE',  ( 0.5643044619422579178, -0.4281496062992127816, -0.4176697321401328100 ) ) ;
#71968=CARTESIAN_POINT ( 'NONE',  ( -0.09842519685039295696, -0.4536011799217367080, 0.2665933059059888421 ) ) ;
#71969=CARTESIAN_POINT ( 'NONE',  ( 0.04593175853018440641, 0.2952755905511810774, -0.1292274648535930714 ) ) ;
#71972=CARTESIAN_POINT ( 'NONE',  ( -1.272965879265091305, -0.4281496062992124485, 0.4176697321401328655 ) ) ;
#71973=CARTESIAN_POINT ( 'NONE',  ( 0.5249343832021003964, 0.1283753931104746893, -0.1820866141732285504 ) ) ;
#71974=CARTESIAN_POINT ( 'NONE',  ( -0.7233796917120549619, 1.992010844874188447, -0.5048038503170217961 ) ) ;
#71975=CARTESIAN_POINT ( 'NONE',  ( -0.5971128608923877978, 0.2952755905511811885, 0.1292274648535926551 ) ) ;
#71976=CARTESIAN_POINT ( 'NONE',  ( -0.1771653543307080136, 0.07958543189024071263, -0.2665933059059888421 ) ) ;
#71978=CARTESIAN_POINT ( 'NONE',  ( -0.5446194225721777693, -0.3162353388693409650, -0.4822834645669289433 ) ) ;
#71979=CARTESIAN_POINT ( 'NONE',  ( -0.5249343832020990641, 0.2306618581243848609, 0.2411417322834645549 ) ) ;
#71980=CARTESIAN_POINT ( 'NONE',  ( -0.02624671916010428221, 0.2306618581243847221, -0.2411417322834647770 ) ) ;
#71983=VECTOR ( 'NONE', #13606, 39.37007874015748143 ) ;
#71984=CARTESIAN_POINT ( 'NONE',  ( -1.646981627296586703, -0.2845877964562161244, -0.3641732283464567121 ) ) ;
#71985=CARTESIAN_POINT ( 'NONE',  ( 0.5774278215223104249, 0.1283753931104748280, 0.1820866141732283561 ) ) ;
#71986=CARTESIAN_POINT ( 'NONE',  ( 1.233595800524935227, -0.6046776061558807314, 0.2411417322834647770 ) ) ;
#71987=CARTESIAN_POINT ( 'NONE',  ( -0.7742782152230965886, -0.004921259842519576551, 0.3153832671262227771 ) ) ;
#71988=CARTESIAN_POINT ( 'NONE',  ( -1.076115485564303809, 0.1283753931104748280, 0.1820866141732283561 ) ) ;
#71989=CARTESIAN_POINT ( 'NONE',  ( -0.5971128608923877978, -0.6692913385826773087, -0.1292274648535924053 ) ) ;
#71990=CARTESIAN_POINT ( 'NONE',  ( -0.6299212598425188991, -0.1870078740157479769, 0.4822834645669291653 ) ) ;
#71991=CARTESIAN_POINT ( 'NONE',  ( 0.6627296587926517768, -0.5511811023622048555, -0.09757992244046775898 ) ) ;
#71993=CARTESIAN_POINT ( 'NONE',  ( 1.181102362204724976, -0.1870078740157480601, -0.3641732283464567677 ) ) ;
#71994=CARTESIAN_POINT ( 'NONE',  ( 0.3280839895013130669, -0.4281496062992127816, -0.4176697321401328100 ) ) ;
#71996=CARTESIAN_POINT ( 'NONE',  ( -0.5708661417322828946, 0.1660481256975883668, -0.3530559997133364547 ) ) ;
#71998=CARTESIAN_POINT ( 'NONE',  ( 1.253280839895013710, -0.2845877964562159024, 0.3641732283464567677 ) ) ;
#71999=CARTESIAN_POINT ( 'NONE',  ( 0.5118110236220480003, -0.6692913385826771977, 8.415575281601705876E-17 ) ) ;
#72000=CARTESIAN_POINT ( 'NONE',  ( 0.2099737532808405305, -0.6046776061558807314, 0.2411417322834647770 ) ) ;
#72001=CARTESIAN_POINT ( 'NONE',  ( -0.1181102362204717315, -0.5511811023622047445, 6.969142054262312111E-17 ) ) ;
#72003=CARTESIAN_POINT ( 'NONE',  ( -0.1837270341207340729, 0.1283753931104746893, -0.1820866141732285504 ) ) ;
#72004=CARTESIAN_POINT ( 'NONE',  ( 0.5971128608923891301, 0.2952755905511810774, -0.1292274648535930714 ) ) ;
#72005=CARTESIAN_POINT ( 'NONE',  ( -0.5446194225721777693, -0.2845877964562161244, -0.3641732283464567121 ) ) ;
#72006=CARTESIAN_POINT ( 'NONE',  ( -0.8858267716535425107, -0.5400638737290844871, 0.3530559997133364547 ) ) ;
#72007=CARTESIAN_POINT ( 'NONE',  ( -1.220472440944878834, 0.000000000000000000, -0.5309055118110234117 ) ) ;
#72009=CARTESIAN_POINT ( 'NONE',  ( -1.253280839895012377, -0.3162353388693409650, -0.4822834645669289433 ) ) ;
#72010=CARTESIAN_POINT ( 'NONE',  ( -0.9383202099737524282, -0.08942795157527998196, 0.3641732283464567121 ) ) ;
#72011=CARTESIAN_POINT ( 'NONE',  ( -0.1771653543307080136, -0.5400638737290844871, 0.3530559997133364547 ) ) ;
#72012=CARTESIAN_POINT ( 'NONE',  ( -1.633858267716534529, -0.5400638737290845981, -0.3530559997133363437 ) ) ;
#72013=CARTESIAN_POINT ( 'NONE',  ( -0.7217847769028863381, -0.4281496062992124485, 0.4176697321401328655 ) ) ;
#72016=CARTESIAN_POINT ( 'NONE',  ( 0.8923884514435701520, -0.6046776061558809534, -0.2411417322834644161 ) ) ;
#72017=CARTESIAN_POINT ( 'NONE',  ( 0.8136482939632553313, -0.6046776061558809534, -0.2411417322834644161 ) ) ;
#72019=CARTESIAN_POINT ( 'NONE',  ( 1.607611548556431069, 0.2952755905511811885, 0.1292274648535926551 ) ) ;
#72020=CARTESIAN_POINT ( 'NONE',  ( -1.450131233595799651, -0.6692913385826771977, 0.1292274648535927661 ) ) ;
#72023=CARTESIAN_POINT ( 'NONE',  ( -0.3871391076115476282, -0.08942795157527998196, 0.3641732283464567121 ) ) ;
#72025=ORIENTED_EDGE ( 'NONE', *, *, #28086, .T. ) ;
#72026=CARTESIAN_POINT ( 'NONE',  ( 0.05905511811023681640, 0.1660481256975883668, -0.3530559997133364547 ) ) ;
#72027=CARTESIAN_POINT ( 'NONE',  ( 0.05905511811023681640, 0.1660481256975883668, -0.3530559997133364547 ) ) ;
#72028=CARTESIAN_POINT ( 'NONE',  ( -0.7545931758530176614, -0.6692913385826773087, -0.1292274648535924053 ) ) ;
#72029=CARTESIAN_POINT ( 'NONE',  ( 1.581364829396326277, -0.3162353388693409650, -0.4822834645669289433 ) ) ;
#72030=CARTESIAN_POINT ( 'NONE',  ( -0.9383202099737524282, -0.2845877964562161244, -0.3641732283464567121 ) ) ;
#72032=CARTESIAN_POINT ( 'NONE',  ( 0.9645669291338591078, -0.5400638737290845981, -0.3530559997133363437 ) ) ;
#72033=CARTESIAN_POINT ( 'NONE',  ( 0.6692913385826777528, 0.1771653543307087630, 0.000000000000000000 ) ) ;
#72034=CARTESIAN_POINT ( 'NONE',  ( -0.3018372703412066094, -0.4281496062992127816, -0.4176697321401328100 ) ) ;
#72036=CARTESIAN_POINT ( 'NONE',  ( -0.7939632545931750718, -0.05778040916215560624, -0.4822834645669293319 ) ) ;
#72037=CARTESIAN_POINT ( 'NONE',  ( -1.555118110236219930, 0.07958543189024085140, 0.2665933059059887866 ) ) ;
#72038=( BOUNDED_CURVE ( )  B_SPLINE_CURVE ( 2, ( #76944, #31485, #39045, #14236, #13812, #77362, #70620, #57146, #12976, #77786, #6644, #71886, #65158 ),
 .UNSPECIFIED., .F., .F. ) 
 B_SPLINE_CURVE_WITH_KNOTS ( ( 3, 2, 2, 2, 2, 2, 3 ),
 ( 0.4460583673620736045, 0.4469696969696969613, 0.4507575757575757458, 0.4545454545454545303, 0.4583333333333333148, 0.4621212121212120993, 0.4630325417288355672 ),
 .UNSPECIFIED. ) 
 CURVE ( )  GEOMETRIC_REPRESENTATION_ITEM ( )  RATIONAL_B_SPLINE_CURVE ( ( 0.9875488213027530104, 0.9918020599134685922, 1.000000000000000000, 0.9659258262890683122, 1.000000000000000000, 0.9659258262890683122, 1.000000000000000000, 0.9659258262890683122, 1.000000000000000000, 0.9659258262890683122, 1.000000000000000000, 0.9918020599134675930, 0.9875488213027519002 ) ) 
 REPRESENTATION_ITEM ( '' )  );
#72039=CARTESIAN_POINT ( 'NONE',  ( 1.502624671916010790, -0.05778040916215522460, 0.4822834645669289988 ) ) ;
#72040=CARTESIAN_POINT ( 'NONE',  ( 1.528871391076116026, 0.1771653543307087630, 0.09757992244046791164 ) ) ;
#72043=CARTESIAN_POINT ( 'NONE',  ( 0.1246719160104994284, 0.2952755905511810774, -0.1292274648535930714 ) ) ;
#72045=CONICAL_SURFACE ( 'NONE', #46479, 1.181102362204724310, 0.7853981633974621568 ) ;
#72046=CARTESIAN_POINT ( 'NONE',  ( -1.345144356955379816, -0.05778040916215560624, -0.4822834645669293319 ) ) ;
#72047=CARTESIAN_POINT ( 'NONE',  ( 1.391076115485564868, -0.6046776061558807314, 0.2411417322834647770 ) ) ;
#72048=CARTESIAN_POINT ( 'NONE',  ( 1.358267716535433323, -0.5400638737290845981, -0.3530559997133363437 ) ) ;
#72049=CARTESIAN_POINT ( 'NONE',  ( 0.3018372703412079971, -0.4281496062992124485, 0.4176697321401328655 ) ) ;
#72050=CARTESIAN_POINT ( 'NONE',  ( -0.4461942257217840213, -0.6046776061558809534, -0.2411417322834644161 ) ) ;
#72052=CARTESIAN_POINT ( 'NONE',  ( -1.141732283464566011, -0.6692913385826771977, 8.415575281601705876E-17 ) ) ;
#72053=CARTESIAN_POINT ( 'NONE',  ( -0.7611548556430438595, -0.6046776061558809534, -0.2411417322834644161 ) ) ;
#72054=CARTESIAN_POINT ( 'NONE',  ( -0.5314960629921250401, 0.07958543189024085140, 0.2665933059059887866 ) ) ;
#72055=CARTESIAN_POINT ( 'NONE',  ( 1.522309711286089939, 0.2306618581243848609, 0.2411417322834645549 ) ) ;
#72056=CARTESIAN_POINT ( 'NONE',  ( -0.3871391076115479057, -0.3162353388693409650, -0.4822834645669289433 ) ) ;
#72058=CARTESIAN_POINT ( 'NONE',  ( 0.6167979002624678353, -0.4281496062992124485, 0.4176697321401328655 ) ) ;
#72059=CARTESIAN_POINT ( 'NONE',  ( 0.5384083780239495853, 0.004960608223778644084, -0.3437734562760191293 ) ) ;
#72060=EDGE_CURVE ( 'NONE', #43230, #8650, #39383, .T. ) ;
#72061=CARTESIAN_POINT ( 'NONE',  ( -0.2362204724409440182, -0.1870078740157479769, 0.4822834645669291653 ) ) ;
#72062=CARTESIAN_POINT ( 'NONE',  ( -0.2887139107611542133, 0.1283753931104748280, 0.1820866141732283561 ) ) ;
#72063=CARTESIAN_POINT ( 'NONE',  ( 0.8727034120734913358, -0.08942795157527998196, 0.3641732283464567121 ) ) ;
#72064=CARTESIAN_POINT ( 'NONE',  ( 0.6971652711706697314, -4.135162568743707313E-16, -0.3791483426435169335 ) ) ;
#72066=LINE ( 'NONE', #33351, #39169 ) ;
#72067=CARTESIAN_POINT ( 'NONE',  ( 1.187664041994751285, -0.3162353388693409650, -0.4822834645669289433 ) ) ;
#72069=CARTESIAN_POINT ( 'NONE',  ( 0.1771653543307093182, 0.1660481256975885056, 0.3530559997133364547 ) ) ;
#72070=LINE ( 'NONE', #27441, #24354 ) ;
#72071=CARTESIAN_POINT ( 'NONE',  ( 1.574803149606299746, -0.1870078740157479769, 0.3641732283464567677 ) ) ;
#72072=CARTESIAN_POINT ( 'NONE',  ( -0.3608923884514428360, -0.6692913385826773087, -0.1292274648535924053 ) ) ;
#72074=CARTESIAN_POINT ( 'NONE',  ( -1.594488188976377119, 0.07958543189024071263, -0.2665933059059888421 ) ) ;
#72075=CARTESIAN_POINT ( 'NONE',  ( 0.6364829396325465405, -0.05778040916215522460, 0.4822834645669289988 ) ) ;
#72076=CARTESIAN_POINT ( 'NONE',  ( 0.8727034120734913358, -0.08942795157527998196, 0.3641732283464567121 ) ) ;
#72077=CYLINDRICAL_SURFACE ( 'NONE', #33139, 1.181102362204724310 ) ;
#72078=CARTESIAN_POINT ( 'NONE',  ( 0.3018372703412079971, -0.004921259842519870586, -0.3153832671262229437 ) ) ;
#72079=CARTESIAN_POINT ( 'NONE',  ( -1.082677165354329896, -0.5400638737290845981, -0.3530559997133363437 ) ) ;
#72081=CARTESIAN_POINT ( 'NONE',  ( 1.345144356955381593, -0.05778040916215522460, 0.4822834645669289988 ) ) ;
#72085=CARTESIAN_POINT ( 'NONE',  ( 0.3608923884514443348, -0.6692913385826771977, 0.1292274648535927661 ) ) ;
#72087=CARTESIAN_POINT ( 'NONE',  ( 0.3346456692913390985, 0.07958543189024085140, 0.2665933059059887866 ) ) ;
#72088=CARTESIAN_POINT ( 'NONE',  ( 0.4658792650918641698, -0.05778040916215560624, -0.4822834645669293319 ) ) ;
#72089=CARTESIAN_POINT ( 'NONE',  ( -0.8661417322834640276, -0.1870078740157480601, -0.3641732283464567677 ) ) ;
#72090=CARTESIAN_POINT ( 'NONE',  ( -0.9645669291338575535, -0.5400638737290844871, 0.3530559997133364547 ) ) ;
#72091=CARTESIAN_POINT ( 'NONE',  ( -1.712598425196849572, 0.1660481256975885056, 0.3530559997133364547 ) ) ;
#72092=CARTESIAN_POINT ( 'NONE',  ( 1.036745406824147731, 0.05413385826771666132, 0.4176697321401328100 ) ) ;
#72093=CARTESIAN_POINT ( 'NONE',  ( 1.489501312335958172, -0.3162353388693405765, 0.4822834645669290543 ) ) ;
#72095=CARTESIAN_POINT ( 'NONE',  ( 0.7152230971128614723, -0.3162353388693409650, -0.4822834645669289433 ) ) ;
#72098=CARTESIAN_POINT ( 'NONE',  ( 1.601049868766404982, -0.6046776061558809534, -0.2411417322834644161 ) ) ;
#72099=CARTESIAN_POINT ( 'NONE',  ( 1.286089238845145033, -0.6046776061558809534, -0.2411417322834644161 ) ) ;
#72100=CARTESIAN_POINT ( 'NONE',  ( -1.646981627296586703, -0.2845877964562161244, -0.3641732283464567121 ) ) ;
#72101=CARTESIAN_POINT ( 'NONE',  ( 1.181102362204725198, -0.1870078740157479769, 0.3641732283464567677 ) ) ;
#72102=CARTESIAN_POINT ( 'NONE',  ( -1.299212598425196097, 0.1771653543307087630, 0.000000000000000000 ) ) ;
#72103=CARTESIAN_POINT ( 'NONE',  ( -0.4461942257217840213, -0.5023911411419708095, -0.1820866141732282451 ) ) ;
#72105=CARTESIAN_POINT ( 'NONE',  ( 0.3280839895013130669, -0.004921259842519576551, 0.3153832671262227771 ) ) ;
#72106=CARTESIAN_POINT ( 'NONE',  ( 0.5774278215223104249, 0.2306618581243848609, 0.2411417322834645549 ) ) ;
#72107=CARTESIAN_POINT ( 'NONE',  ( 0.9120734908136489683, -0.6692913385826771977, 0.1292274648535927661 ) ) ;
#72108=CARTESIAN_POINT ( 'NONE',  ( 0.03937007874015833325, -0.6692913385826771977, 8.415575281601705876E-17 ) ) ;
#72109=CARTESIAN_POINT ( 'NONE',  ( -0.03937007874015669567, -0.5511811023622047445, 6.969142054262312111E-17 ) ) ;
#72110=CARTESIAN_POINT ( 'NONE',  ( 1.213910761154856299, -0.6692913385826773087, -0.1292274648535924053 ) ) ;
#72112=CARTESIAN_POINT ( 'NONE',  ( -1.141732283464566011, -0.6692913385826771977, 8.415575281601705876E-17 ) ) ;
#72114=CARTESIAN_POINT ( 'NONE',  ( 0.01312335958005323398, 0.009842519685039463617, 0.3409548833797002576 ) ) ;
#72115=CARTESIAN_POINT ( 'NONE',  ( 0.06561679790026316017, 0.05413385826771626580, -0.4176697321401330321 ) ) ;
#72116=CARTESIAN_POINT ( 'NONE',  ( -0.8727034120734901146, -0.3162353388693405765, 0.4822834645669290543 ) ) ;
#72117=CARTESIAN_POINT ( 'NONE',  ( -0.2624671916010490880, 0.2306618581243847221, -0.2411417322834647770 ) ) ;
#72120=B_SPLINE_CURVE_WITH_KNOTS ( 'NONE', 3,
 ( #43457, #17824, #74661, #49783, #81387, #68342, #42645 ),
 .UNSPECIFIED., .F., .F.,
 ( 4, 3, 4 ),
 ( 1.734723475976807094E-18, 0.001246230184515569571, 0.002492489877932635954 ),
 .UNSPECIFIED. ) ;
#72123=CARTESIAN_POINT ( 'NONE',  ( -0.8333333333333323711, -0.5511811023622048555, -0.09757992244046775898 ) ) ;
#72125=CARTESIAN_POINT ( 'NONE',  ( -1.732283464566928277, -0.1870078740157479769, 0.4822834645669291653 ) ) ;
#72127=CARTESIAN_POINT ( 'NONE',  ( 0.2624671916010504757, 0.2306618581243848609, 0.2411417322834645549 ) ) ;
#72128=CARTESIAN_POINT ( 'NONE',  ( -0.6102362204724400829, 0.07958543189024085140, 0.2665933059059887866 ) ) ;
#72129=CARTESIAN_POINT ( 'NONE',  ( 0.7611548556430451917, -0.6046776061558807314, 0.2411417322834647770 ) ) ;
#72130=CARTESIAN_POINT ( 'NONE',  ( 0.3740157480314966754, 0.1660481256975883668, -0.3530559997133364547 ) ) ;
#72135=CARTESIAN_POINT ( 'NONE',  ( 1.253280839895013710, -0.05778040916215560624, -0.4822834645669293319 ) ) ;
#72136=VECTOR ( 'NONE', #38961, 39.37007874015748854 ) ;
#72138=CARTESIAN_POINT ( 'NONE',  ( 0.4724409448818904789, -0.1870078740157479769, 0.4822834645669291653 ) ) ;
#72139=CARTESIAN_POINT ( 'NONE',  ( 0.2099737532808405305, 0.2306618581243847221, -0.2411417322834647770 ) ) ;
#72140=CARTESIAN_POINT ( 'NONE',  ( 1.325459317585302665, 0.05413385826771626580, -0.4176697321401330321 ) ) ;
#72141=CARTESIAN_POINT ( 'NONE',  ( 0.7152230971128616943, -0.05778040916215522460, 0.4822834645669289988 ) ) ;
#72143=CARTESIAN_POINT ( 'NONE',  ( 0.05249343832021075018, 0.2306618581243847221, -0.2411417322834647770 ) ) ;
#72144=CARTESIAN_POINT ( 'NONE',  ( 0.6430446194225729606, -0.4281496062992127816, -0.4176697321401328100 ) ) ;
#72145=CARTESIAN_POINT ( 'NONE',  ( -0.06561679790026180015, 0.05413385826771666132, 0.4176697321401328100 ) ) ;
#72146=CARTESIAN_POINT ( 'NONE',  ( 1.220472440944882608, 0.1771653543307087630, 0.000000000000000000 ) ) ;
#72147=CARTESIAN_POINT ( 'NONE',  ( -1.502624671916009680, -0.05778040916215560624, -0.4822834645669293319 ) ) ;
#72148=CARTESIAN_POINT ( 'NONE',  ( -1.325459317585300889, -0.4281496062992127816, -0.4176697321401328100 ) ) ;
#72149=CARTESIAN_POINT ( 'NONE',  ( 0.6102362204724416372, -0.5400638737290844871, 0.3530559997133364547 ) ) ;
#72151=B_SPLINE_CURVE_WITH_KNOTS ( 'NONE', 3,
 ( #67659, #2445, #79469, #61324 ),
 .UNSPECIFIED., .F., .F.,
 ( 4, 4 ),
 ( 3.593986969204291827E-07, 0.001287825409103209679 ),
 .UNSPECIFIED. ) ;
#72156=CARTESIAN_POINT ( 'NONE',  ( 1.049868766404200349, 0.2306618581243848609, 0.2411417322834645549 ) ) ;
#72157=CARTESIAN_POINT ( 'NONE',  ( 1.148293963254593653, 0.1771653543307087075, -0.09757992244046823083 ) ) ;
#72158=CARTESIAN_POINT ( 'NONE',  ( 0.6036745406824154392, 0.2306618581243847221, -0.2411417322834647770 ) ) ;
#72162=CARTESIAN_POINT ( 'NONE',  ( 1.128608923884514947, 0.2306618581243848609, 0.2411417322834645549 ) ) ;
#72163=CARTESIAN_POINT ( 'NONE',  ( -1.594488188976377119, 0.1660481256975883668, -0.3530559997133364547 ) ) ;
#72164=CARTESIAN_POINT ( 'NONE',  ( -0.2624671916010490880, 0.2306618581243847221, -0.2411417322834647770 ) ) ;
#72165=CARTESIAN_POINT ( 'NONE',  ( 0.9383202099737536495, -0.3162353388693405765, 0.4822834645669290543 ) ) ;
#72166=VERTEX_POINT ( 'NONE', #57480 ) ;
#72167=CARTESIAN_POINT ( 'NONE',  ( -1.581364829396324945, -0.3162353388693405765, 0.4822834645669290543 ) ) ;
#72168=CARTESIAN_POINT ( 'NONE',  ( 0.4824498642376759960, 1.223219560026271499E-15, 0.4445507791589056734 ) ) ;
#72170=CARTESIAN_POINT ( 'NONE',  ( 1.555118110236221041, 0.07958543189024071263, -0.2665933059059888421 ) ) ;
#72172=CARTESIAN_POINT ( 'NONE',  ( -1.062992125984250968, -0.5511811023622047445, 6.969142054262312111E-17 ) ) ;
#72173=CARTESIAN_POINT ( 'NONE',  ( -1.614173228346455824, 0.2952755905511811885, 0.000000000000000000 ) ) ;
#72174=CARTESIAN_POINT ( 'NONE',  ( 0.4790026246719168435, -0.3162353388693409650, -0.4822834645669289433 ) ) ;
#72176=CARTESIAN_POINT ( 'NONE',  ( -0.7426113562969628434, 2.209901789876557832, 0.5309055118110236338 ) ) ;
#72178=CARTESIAN_POINT ( 'NONE',  ( 0.7217847769028878924, 0.05413385826771666132, 0.4176697321401328100 ) ) ;
#72179=CARTESIAN_POINT ( 'NONE',  ( -1.548556430446193399, 0.2306618581243848609, 0.2411417322834645549 ) ) ;
#72181=CARTESIAN_POINT ( 'NONE',  ( -0.8464566929133852113, -0.4536011799217368745, -0.2665933059059886201 ) ) ;
#72182=CARTESIAN_POINT ( 'NONE',  ( 1.627296587926509996, -0.6046776061558807314, 0.2411417322834647770 ) ) ;
#72184=CARTESIAN_POINT ( 'NONE',  ( 0.5052493438320215802, 0.2952755905511811885, 0.1292274648535926551 ) ) ;
#72185=CARTESIAN_POINT ( 'NONE',  ( -0.9055118110236215490, -0.5511811023622047445, 6.969142054262312111E-17 ) ) ;
#72186=CARTESIAN_POINT ( 'NONE',  ( -0.03937007874015669567, -0.5511811023622047445, 6.969142054262312111E-17 ) ) ;
#72188=CARTESIAN_POINT ( 'NONE',  ( -0.4986876640419942164, -0.6046776061558807314, 0.2411417322834647770 ) ) ;
#72189=CARTESIAN_POINT ( 'NONE',  ( -1.200787401574802349, -0.4536011799217367080, 0.2665933059059888421 ) ) ;
#72191=CARTESIAN_POINT ( 'NONE',  ( 0.8333333333333340365, 0.2952755905511810774, -0.1292274648535930714 ) ) ;
#72192=VECTOR ( 'NONE', #39390, 39.37007874015748143 ) ;
#72193=ADVANCED_FACE ( 'NONE', ( #6982 ), #79854, .F. ) ;
#72196=STYLED_ITEM ( 'NONE', ( #29187 ), #59541 ) ;
#72199=CARTESIAN_POINT ( 'NONE',  ( -0.6496062992125976043, -0.5400638737290844871, 0.3530559997133364547 ) ) ;
#72200=CARTESIAN_POINT ( 'NONE',  ( -0.3608923884514428360, -0.5511811023622048555, -0.09757992244046775898 ) ) ;
#72201=CARTESIAN_POINT ( 'NONE',  ( -1.351706036745406347, -0.4281496062992124485, 0.4176697321401328655 ) ) ;
#72202=CARTESIAN_POINT ( 'NONE',  ( 0.7020997375328090762, -0.2845877964562159024, 0.3641732283464567677 ) ) ;
#72203=CARTESIAN_POINT ( 'NONE',  ( -0.6758530183727028406, -0.5511811023622048555, -0.09757992244046775898 ) ) ;
#72204=CARTESIAN_POINT ( 'NONE',  ( -1.102362204724408601, -0.1870078740157479769, 0.4822834645669291653 ) ) ;
#72205=CARTESIAN_POINT ( 'NONE',  ( -1.082677165354329896, 0.1660481256975885056, 0.3530559997133364547 ) ) ;
#72206=CARTESIAN_POINT ( 'NONE',  ( 1.627296587926509996, -0.6046776061558807314, 0.2411417322834647770 ) ) ;
#72208=CARTESIAN_POINT ( 'NONE',  ( 1.062992125984252745, 0.1771653543307087630, 0.000000000000000000 ) ) ;
#72210=CARTESIAN_POINT ( 'NONE',  ( 0.3674540682414705883, -0.6046776061558807314, 0.2411417322834647770 ) ) ;
#72211=CARTESIAN_POINT ( 'NONE',  ( -1.646981627296586703, -0.05778040916215522460, 0.4822834645669289988 ) ) ;
#72212=CARTESIAN_POINT ( 'NONE',  ( -1.719160104986876103, 0.05413385826771666132, 0.4176697321401328100 ) ) ;
#72216=CARTESIAN_POINT ( 'NONE',  ( -1.220472440944881054, -0.5511811023622047445, 6.969142054262312111E-17 ) ) ;
#72217=CARTESIAN_POINT ( 'NONE',  ( -0.6627296587926501115, 0.2952755905511810774, -0.1292274648535930714 ) ) ;
#72218=CARTESIAN_POINT ( 'NONE',  ( 0.8333333333333340365, 0.2952755905511810774, -0.1292274648535930714 ) ) ;
#72219=CARTESIAN_POINT ( 'NONE',  ( -1.535433070866141225, 0.1771653543307087630, 0.000000000000000000 ) ) ;
#72221=CARTESIAN_POINT ( 'NONE',  ( -1.601049868766403650, -0.6046776061558807314, 0.2411417322834647770 ) ) ;
#72222=CARTESIAN_POINT ( 'NONE',  ( 0.6430446194225729606, -0.4281496062992127816, -0.4176697321401328100 ) ) ;
#72223=CARTESIAN_POINT ( 'NONE',  ( 0.6430446194225729606, -0.4281496062992127816, -0.4176697321401328100 ) ) ;
#72224=EDGE_CURVE ( 'NONE', #16885, #48718, #60233, .T. ) ;
#72225=CARTESIAN_POINT ( 'NONE',  ( 1.207349081364829990, -0.6046776061558809534, -0.2411417322834644161 ) ) ;
#72226=DIRECTION ( 'NONE',  ( -0.4999999999999987788, -0.7071067811865503483, 0.4999999999999972244 ) ) ;
#72230=CARTESIAN_POINT ( 'NONE',  ( 0.2165354330708668673, 0.07958543189024071263, -0.2665933059059888421 ) ) ;
#72231=CARTESIAN_POINT ( 'NONE',  ( 0.05249343832021075018, 0.2306618581243847221, -0.2411417322834647770 ) ) ;
#72232=CARTESIAN_POINT ( 'NONE',  ( 1.450131233595801428, 0.2952755905511811885, 0.1292274648535926551 ) ) ;
#72234=CARTESIAN_POINT ( 'NONE',  ( 0.4133858267716541968, 0.07958543189024085140, 0.2665933059059887866 ) ) ;
#72235=CARTESIAN_POINT ( 'NONE',  ( -0.6299212598425188991, -0.1870078740157480879, -0.4822834645669291653 ) ) ;
#72236=CARTESIAN_POINT ( 'NONE',  ( 1.469816272965879911, 0.2306618581243847221, -0.2411417322834647770 ) ) ;
#72237=CARTESIAN_POINT ( 'NONE',  ( 0.3215223097112867578, -0.3162353388693409650, -0.4822834645669289433 ) ) ;
#72239=DIRECTION ( 'NONE',  ( 0.7071067811865462405, 2.189697074797793648E-16, 0.7071067811865486830 ) ) ;
#72242=CARTESIAN_POINT ( 'NONE',  ( 1.463254593175853824, 0.1771653543307087075, -0.09757992244046823083 ) ) ;
#72243=CARTESIAN_POINT ( 'NONE',  ( -1.194225721784776262, -0.3690944881889763329, 0.3153832671262228327 ) ) ;
#72244=CARTESIAN_POINT ( 'NONE',  ( -1.115485564304461219, 0.05413385826771626580, -0.4176697321401330321 ) ) ;
#72247=CARTESIAN_POINT ( 'NONE',  ( -1.522309711286088607, -0.5023911411419708095, 0.1820866141732285504 ) ) ;
#72248=CARTESIAN_POINT ( 'NONE',  ( -1.371391076115484831, 0.2952755905511810774, -0.1292274648535930714 ) ) ;
#72249=CARTESIAN_POINT ( 'NONE',  ( 0.05905511811023681640, 0.1660481256975883668, -0.3530559997133364547 ) ) ;
#72250=CARTESIAN_POINT ( 'NONE',  ( -1.364829396325458521, -0.6046776061558807314, 0.2411417322834647770 ) ) ;
#72252=CARTESIAN_POINT ( 'NONE',  ( 0.6824146981627303710, 0.2306618581243847221, -0.2411417322834647770 ) ) ;
#72254=CARTESIAN_POINT ( 'NONE',  ( -1.122047244094487306, 0.07958543189024071263, -0.2665933059059888421 ) ) ;
#72258=CARTESIAN_POINT ( 'NONE',  ( -1.653543307086613234, -0.1870078740157480601, -0.3641732283464567677 ) ) ;
#72259=AXIS2_PLACEMENT_3D ( 'NONE', #49239, #18099, #75757 ) ;
#72260=CARTESIAN_POINT ( 'NONE',  ( -1.003937007874015297, -0.5400638737290845981, -0.3530559997133363437 ) ) ;
#72261=CARTESIAN_POINT ( 'NONE',  ( -1.423884514435694859, -0.05778040916215560624, -0.4822834645669293319 ) ) ;
#72264=CARTESIAN_POINT ( 'NONE',  ( -1.660104986876639543, -0.05778040916215560624, -0.4822834645669293319 ) ) ;
#72265=CARTESIAN_POINT ( 'NONE',  ( -1.292650918635170010, 0.2952755905511810774, -0.1292274648535930714 ) ) ;
#72267=CARTESIAN_POINT ( 'NONE',  ( -1.614173228346456712, 0.7166040191147899918, -0.1372047244094478091 ) ) ;
#72268=CARTESIAN_POINT ( 'NONE',  ( 0.05905511811023709395, -0.4536011799217367080, 0.2665933059059888421 ) ) ;
#72270=CARTESIAN_POINT ( 'NONE',  ( -0.7020997375328076329, -0.2845877964562161244, -0.3641732283464567121 ) ) ;
#72271=CARTESIAN_POINT ( 'NONE',  ( -0.7283464566929126471, -0.5400638737290844871, 0.3530559997133364547 ) ) ;
#72272=CARTESIAN_POINT ( 'NONE',  ( 0.7414698162729663755, -0.6692913385826773087, -0.1292274648535924053 ) ) ;
#72273=CARTESIAN_POINT ( 'NONE',  ( -1.108923884514435132, -0.05778040916215560624, -0.4822834645669293319 ) ) ;
#72275=ORIENTED_EDGE ( 'NONE', *, *, #62163, .T. ) ;
#72276=B_SPLINE_CURVE_WITH_KNOTS ( 'NONE', 3,
 ( #21456, #47114, #72803, #15990, #67328, #15152, #66918 ),
 .UNSPECIFIED., .F., .F.,
 ( 4, 3, 4 ),
 ( 1.232595164407830946E-32, 0.001246232571205310594, 0.002492492258783241162 ),
 .UNSPECIFIED. ) ;
#72277=CARTESIAN_POINT ( 'NONE',  ( -0.9055118110236215490, -0.6692913385826771977, 8.415575281601705876E-17 ) ) ;
#72278=CARTESIAN_POINT ( 'NONE',  ( 0.9317585301837276734, -0.4281496062992124485, 0.4176697321401328655 ) ) ;
#72279=CARTESIAN_POINT ( 'NONE',  ( -1.640419947506561060, -0.3690944881889765550, -0.3153832671262227771 ) ) ;
#72280=CARTESIAN_POINT ( 'NONE',  ( -1.719160104986876103, 0.05413385826771666132, 0.4176697321401328100 ) ) ;
#72286=CARTESIAN_POINT ( 'NONE',  ( -0.4855643044619415427, 0.05413385826771626580, -0.4176697321401330321 ) ) ;
#72287=CARTESIAN_POINT ( 'NONE',  ( -1.391076115485563314, -0.5023911411419708095, -0.1820866141732282451 ) ) ;
#72289=CARTESIAN_POINT ( 'NONE',  ( -1.207349081364828880, 0.2306618581243847221, -0.2411417322834647770 ) ) ;
#72290=CARTESIAN_POINT ( 'NONE',  ( 2.795275590551181466, 1.023622047244095556, -2.156651478620225655E-16 ) ) ;
#72291=CARTESIAN_POINT ( 'NONE',  ( -1.345144356955379816, -0.05778040916215560624, -0.4822834645669293319 ) ) ;
#72292=CARTESIAN_POINT ( 'NONE',  ( -0.2362204724409442680, -0.1870078740157480879, -0.4822834645669291653 ) ) ;
#72294=CARTESIAN_POINT ( 'NONE',  ( 0.5118110236220478892, 0.1771653543307087630, 0.000000000000000000 ) ) ;
#72296=CARTESIAN_POINT ( 'NONE',  ( 0.4133858267716541968, 0.07958543189024085140, 0.2665933059059887866 ) ) ;
#72297=CARTESIAN_POINT ( 'NONE',  ( 1.548556430446194954, -0.5023911411419708095, 0.1820866141732285504 ) ) ;
#72298=CARTESIAN_POINT ( 'NONE',  ( 0.7742782152230978099, -0.4281496062992124485, 0.4176697321401328655 ) ) ;
#72299=CARTESIAN_POINT ( 'NONE',  ( -0.01968503937007793844, 0.07958543189024071263, -0.2665933059059888421 ) ) ;
#72301=CARTESIAN_POINT ( 'NONE',  ( -1.482939632545930975, 0.05413385826771666132, 0.4176697321401328100 ) ) ;
#72302=CARTESIAN_POINT ( 'NONE',  ( -0.07874015748031421014, -0.1870078740157480601, -0.3641732283464567677 ) ) ;
#72303=CARTESIAN_POINT ( 'NONE',  ( -1.476377952755905110, 0.07958543189024085140, 0.2665933059059887866 ) ) ;
#72305=CARTESIAN_POINT ( 'NONE',  ( -0.5905511811023613777, -0.5511811023622047445, 6.969142054262312111E-17 ) ) ;
#72307=CARTESIAN_POINT ( 'NONE',  ( -0.09842519685039295696, -0.5400638737290844871, 0.3530559997133364547 ) ) ;
#72309=CARTESIAN_POINT ( 'NONE',  ( 0.4396325459317590445, -0.5511811023622046335, 0.09757992244046803654 ) ) ;
#72310=CARTESIAN_POINT ( 'NONE',  ( -0.1771653543307080136, -0.4536011799217367080, 0.2665933059059888421 ) ) ;
#72311=CARTESIAN_POINT ( 'NONE',  ( -0.3937007874015740483, -0.1870078740157479769, 0.4822834645669291653 ) ) ;
#72313=CARTESIAN_POINT ( 'NONE',  ( -0.9186351706036736120, -0.5023911411419708095, -0.1820866141732282451 ) ) ;
#72315=CARTESIAN_POINT ( 'NONE',  ( 0.7677165354330716118, 0.1660481256975883668, -0.3530559997133364547 ) ) ;
#72316=CARTESIAN_POINT ( 'NONE',  ( -0.8136482939632537770, 0.2306618581243847221, -0.2411417322834647770 ) ) ;
#72320=CARTESIAN_POINT ( 'NONE',  ( -0.3412073490813641308, -0.5023911411419708095, 0.1820866141732285504 ) ) ;
#72321=CARTESIAN_POINT ( 'NONE',  ( -1.417322834645668772, -0.1870078740157480879, -0.4822834645669291653 ) ) ;
#72322=CARTESIAN_POINT ( 'NONE',  ( -1.036745406824146176, -0.3690944881889763329, 0.3153832671262228327 ) ) ;
#72323=FACE_OUTER_BOUND ( 'NONE', #67719, .T. ) ;
#72324=CARTESIAN_POINT ( 'NONE',  ( -0.9842519685039360366, 0.1771653543307087630, 0.000000000000000000 ) ) ;
#72326=CARTESIAN_POINT ( 'NONE',  ( 0.9580052493438326877, 0.05413385826771666132, 0.4176697321401328100 ) ) ;
#72330=CARTESIAN_POINT ( 'NONE',  ( 1.443569553805774897, 0.1283753931104748280, 0.1820866141732283561 ) ) ;
#72331=CARTESIAN_POINT ( 'NONE',  ( -1.148293963254592542, -0.6692913385826773087, -0.1292274648535924053 ) ) ;
#72332=CARTESIAN_POINT ( 'NONE',  ( 1.318897637795276356, 0.1660481256975883668, -0.3530559997133364547 ) ) ;
#72334=CARTESIAN_POINT ( 'NONE',  ( 1.509186351706037543, -0.004921259842519576551, 0.3153832671262227771 ) ) ;
#72335=CARTESIAN_POINT ( 'NONE',  ( 0.3280839895013130669, -0.4281496062992127816, -0.4176697321401328100 ) ) ;
#72336=CARTESIAN_POINT ( 'NONE',  ( -0.5708661417322825615, -0.5400638737290844871, 0.3530559997133364547 ) ) ;
#72337=CARTESIAN_POINT ( 'NONE',  ( 1.541994750656168645, 0.2952755905511810774, -0.1292274648535930714 ) ) ;
#72339=CARTESIAN_POINT ( 'NONE',  ( 0.8333333333333340365, 0.1771653543307087075, -0.09757992244046823083 ) ) ;
#72340=EDGE_CURVE ( 'NONE', #24792, #19878, #67362, .T. ) ;
#72345=CARTESIAN_POINT ( 'NONE',  ( -0.3805774278215216522, -0.4281496062992127816, -0.4176697321401328100 ) ) ;
#72346=CARTESIAN_POINT ( 'NONE',  ( 1.522309711286089939, -0.6046776061558809534, -0.2411417322834644161 ) ) ;
#72347=CARTESIAN_POINT ( 'NONE',  ( 0.2427821522309719648, -0.05778040916215522460, 0.4822834645669289988 ) ) ;
#72348=CARTESIAN_POINT ( 'NONE',  ( -0.4068241469816264999, -0.3690944881889763329, 0.3153832671262228327 ) ) ;
#72349=CARTESIAN_POINT ( 'NONE',  ( 1.122047244094488860, -0.5400638737290845981, -0.3530559997133363437 ) ) ;
#72350=EDGE_CURVE ( 'NONE', #32475, #22642, #2264, .T. ) ;
#72351=CARTESIAN_POINT ( 'NONE',  ( -0.6233595800524928121, -0.3162353388693409650, -0.4822834645669289433 ) ) ;
#72352=CARTESIAN_POINT ( 'NONE',  ( 0.2296587926509192634, -0.05778040916215560624, -0.4822834645669293319 ) ) ;
#72353=CARTESIAN_POINT ( 'NONE',  ( -1.561679790026246017, -0.4281496062992127816, -0.4176697321401328100 ) ) ;
#72354=CARTESIAN_POINT ( 'NONE',  ( 0.8661417322834652488, -0.1870078740157480879, -0.4822834645669291653 ) ) ;
#72355=CARTESIAN_POINT ( 'NONE',  ( 1.049868766404200349, 0.2306618581243848609, 0.2411417322834645549 ) ) ;
#72357=CARTESIAN_POINT ( 'NONE',  ( 0.1574803149606306130, -0.1870078740157480601, -0.3641732283464567677 ) ) ;
#72361=CARTESIAN_POINT ( 'NONE',  ( -0.2624671916010490880, 0.1283753931104746893, -0.1820866141732285504 ) ) ;
#72362=CARTESIAN_POINT ( 'NONE',  ( 0.1574803149606306130, -0.1870078740157480879, -0.4822834645669291653 ) ) ;
#72364=CARTESIAN_POINT ( 'NONE',  ( -0.2755905511811018171, 0.2952755905511811885, 0.000000000000000000 ) ) ;
#72365=CARTESIAN_POINT ( 'NONE',  ( -0.4330708661417315697, 0.2952755905511811885, 0.000000000000000000 ) ) ;
#72366=CARTESIAN_POINT ( 'NONE',  ( -0.8333333333333323711, 0.2952755905511811885, 0.1292274648535926551 ) ) ;
#72367=CARTESIAN_POINT ( 'NONE',  ( -1.207349081364828880, 0.2306618581243847221, -0.2411417322834647770 ) ) ;
#72368=CARTESIAN_POINT ( 'NONE',  ( 1.391076115485564868, 0.1283753931104746893, -0.1820866141732285504 ) ) ;
#72370=CARTESIAN_POINT ( 'NONE',  ( 1.614173228346457378, 0.7166040191147859950, -0.1372047244094476148 ) ) ;
#72371=CARTESIAN_POINT ( 'NONE',  ( 1.082677165354331228, -0.4536011799217367080, 0.2665933059059888421 ) ) ;
#72372=CARTESIAN_POINT ( 'NONE',  ( 0.5774278215223104249, 0.2306618581243848609, 0.2411417322834645549 ) ) ;
#72373=CARTESIAN_POINT ( 'NONE',  ( 0.2034120734908144990, -0.6692913385826771977, 0.1292274648535927661 ) ) ;
#72378=CARTESIAN_POINT ( 'NONE',  ( -0.6364829396325453192, -0.3162353388693405765, 0.4822834645669290543 ) ) ;
#72381=CARTESIAN_POINT ( 'NONE',  ( -1.187664041994749731, -0.2845877964562159024, 0.3641732283464567677 ) ) ;
#72382=CARTESIAN_POINT ( 'NONE',  ( 0.8661417322834652488, -0.1870078740157480879, -0.4822834645669291653 ) ) ;
#72383=CARTESIAN_POINT ( 'NONE',  ( 0.9317585301837276734, 0.05413385826771626580, -0.4176697321401330321 ) ) ;
#72384=CARTESIAN_POINT ( 'NONE',  ( -0.3805774278215216522, -0.004921259842519576551, 0.3153832671262227771 ) ) ;
#72385=CARTESIAN_POINT ( 'NONE',  ( 0.5577427821522314977, -0.3162353388693409650, -0.4822834645669289433 ) ) ;
#72387=CARTESIAN_POINT ( 'NONE',  ( 0.06561679790026316017, -0.3690944881889763329, 0.3153832671262228327 ) ) ;
#72388=CARTESIAN_POINT ( 'NONE',  ( -0.2427821522309703550, -0.05778040916215560624, -0.4822834645669293319 ) ) ;
#72390=CARTESIAN_POINT ( 'NONE',  ( -1.732283464566928277, -0.1870078740157479769, 0.4822834645669291653 ) ) ;
#72391=CARTESIAN_POINT ( 'NONE',  ( 0.5446194225721792126, -0.08942795157528024563, -0.3641732283464568787 ) ) ;
#72392=CARTESIAN_POINT ( 'NONE',  ( 1.391076115485564868, 0.1283753931104746893, -0.1820866141732285504 ) ) ;
#72393=CARTESIAN_POINT ( 'NONE',  ( -0.5774278215223089816, 0.2306618581243847221, -0.2411417322834647770 ) ) ;
#72394=CARTESIAN_POINT ( 'NONE',  ( -0.5380577427821514602, -0.004921259842519576551, 0.3153832671262227771 ) ) ;
#72396=CARTESIAN_POINT ( 'NONE',  ( -0.7283464566929126471, 0.1660481256975883668, -0.3530559997133364547 ) ) ;
#72397=CARTESIAN_POINT ( 'NONE',  ( -0.5118110236220466680, 0.2952755905511811885, 0.000000000000000000 ) ) ;
#72398=B_SPLINE_CURVE_WITH_KNOTS ( 'NONE', 3,
 ( #18033, #76513, #62220, #12125 ),
 .UNSPECIFIED., .F., .F.,
 ( 4, 4 ),
 ( 0.000000000000000000, 0.001510660848375622615 ),
 .UNSPECIFIED. ) ;
#72399=CARTESIAN_POINT ( 'NONE',  ( -0.1706036745406816491, 0.05413385826771626580, -0.4176697321401330321 ) ) ;
#72403=CARTESIAN_POINT ( 'NONE',  ( 0.7349081364829403995, 0.1283753931104748280, 0.1820866141732283561 ) ) ;
#72404=CARTESIAN_POINT ( 'NONE',  ( 1.194225721784777594, -0.4281496062992127816, -0.4176697321401328100 ) ) ;
#72405=CARTESIAN_POINT ( 'NONE',  ( -1.410761154855642463, -0.08942795157527998196, 0.3641732283464567121 ) ) ;
#72406=CARTESIAN_POINT ( 'NONE',  ( -1.141732283464566011, -0.5511811023622047445, 6.969142054262312111E-17 ) ) ;
#72407=CARTESIAN_POINT ( 'NONE',  ( -0.7086614173228339419, -0.1870078740157480879, -0.4822834645669291653 ) ) ;
#72408=CARTESIAN_POINT ( 'NONE',  ( -0.03280839895013062252, 0.1771653543307087075, -0.09757992244046823083 ) ) ;
#72410=CARTESIAN_POINT ( 'NONE',  ( 1.240157480314961314, -0.4536011799217367080, 0.2665933059059888421 ) ) ;
#72411=CARTESIAN_POINT ( 'NONE',  ( 0.2821522309711292364, 0.2952755905511810774, -0.1292274648535930714 ) ) ;
#72413=CARTESIAN_POINT ( 'NONE',  ( -0.6036745406824141069, 0.2306618581243848609, 0.2411417322834645549 ) ) ;
#72415=CARTESIAN_POINT ( 'NONE',  ( 1.607611548556431069, 0.1771653543307087630, 0.09757992244046791164 ) ) ;
#72416=CARTESIAN_POINT ( 'NONE',  ( 0.6692913385826778638, -0.6692913385826771977, 8.415575281601705876E-17 ) ) ;
#72417=CARTESIAN_POINT ( 'NONE',  ( -0.006561679790025524116, -0.05778040916215560624, -0.4822834645669293319 ) ) ;
#72418=CARTESIAN_POINT ( 'NONE',  ( 0.01312335958005323398, -0.3690944881889765550, -0.3153832671262227771 ) ) ;
#72419=CARTESIAN_POINT ( 'NONE',  ( 1.586052503253845503, 1.023622047244095556, 0.1653254495020588799 ) ) ;
#72420=CARTESIAN_POINT ( 'NONE',  ( -0.2362204724409440182, -0.1870078740157479769, 0.3641732283464567677 ) ) ;
#72421=CARTESIAN_POINT ( 'NONE',  ( 0.7808398950131241190, -0.05778040916215560624, -0.4822834645669293319 ) ) ;
#72422=CARTESIAN_POINT ( 'NONE',  ( -0.6102362204724400829, 0.07958543189024085140, 0.2665933059059887866 ) ) ;
#72424=CARTESIAN_POINT ( 'NONE',  ( -0.9711286089238838626, 0.2306618581243847221, -0.2411417322834647770 ) ) ;
#72425=CARTESIAN_POINT ( 'NONE',  ( 0.1968503937007881344, 0.2066929133858268208, 0.000000000000000000 ) ) ;
#72426=ORIENTED_EDGE ( 'NONE', *, *, #58379, .F. ) ;
#72427=CARTESIAN_POINT ( 'NONE',  ( -1.017060367454067249, -0.05778040916215522460, 0.4822834645669289988 ) ) ;
#72428=CARTESIAN_POINT ( 'NONE',  ( -1.023622047244094002, -0.1870078740157480601, -0.3641732283464567677 ) ) ;
#72429=CARTESIAN_POINT ( 'NONE',  ( 0.1706036745406830368, 0.05413385826771666132, 0.4176697321401328100 ) ) ;
#72430=CARTESIAN_POINT ( 'NONE',  ( -1.581364829396324945, -0.3162353388693405765, 0.4822834645669290543 ) ) ;
#72431=CARTESIAN_POINT ( 'NONE',  ( -0.6364829396325453192, -0.05778040916215560624, -0.4822834645669293319 ) ) ;
#72434=CARTESIAN_POINT ( 'NONE',  ( 0.7283464566929140904, -0.5400638737290845981, -0.3530559997133363437 ) ) ;
#72435=CARTESIAN_POINT ( 'NONE',  ( 1.069553805774278832, 0.2952755905511810774, -0.1292274648535930714 ) ) ;
#72437=CARTESIAN_POINT ( 'NONE',  ( 1.614173228346457378, 0.2952755905511811885, 0.000000000000000000 ) ) ;
#72438=CARTESIAN_POINT ( 'NONE',  ( -1.220472440944881054, 0.2952755905511811885, 0.000000000000000000 ) ) ;
#72442=CARTESIAN_POINT ( 'NONE',  ( -0.3543307086614165824, 0.1771653543307087630, 0.000000000000000000 ) ) ;
#72445=CARTESIAN_POINT ( 'NONE',  ( 0.2493438320209980519, -0.4281496062992127816, -0.4176697321401328100 ) ) ;
#72446=CARTESIAN_POINT ( 'NONE',  ( 0.1771653543307093182, 0.1660481256975885056, 0.3530559997133364547 ) ) ;
#72447=CARTESIAN_POINT ( 'NONE',  ( -0.8070866141732276899, 0.1660481256975883668, -0.3530559997133364547 ) ) ;
#72448=CARTESIAN_POINT ( 'NONE',  ( 1.469816272965879911, -0.6046776061558807314, 0.2411417322834647770 ) ) ;
#72449=CARTESIAN_POINT ( 'NONE',  ( -1.043307086614172041, -0.4536011799217367080, 0.2665933059059888421 ) ) ;
#72451=CARTESIAN_POINT ( 'NONE',  ( 0.7283464566929143125, 0.1660481256975885056, 0.3530559997133364547 ) ) ;
#72452=CARTESIAN_POINT ( 'NONE',  ( 0.4396325459317590445, -0.5511811023622046335, 0.09757992244046803654 ) ) ;
#72453=CARTESIAN_POINT ( 'NONE',  ( -0.4790026246719152336, -0.05778040916215560624, -0.4822834645669293319 ) ) ;
#72455=CARTESIAN_POINT ( 'NONE',  ( -1.358267716535432434, -0.5400638737290844871, 0.3530559997133364547 ) ) ;
#72456=CARTESIAN_POINT ( 'NONE',  ( -1.548556430446193399, 0.1283753931104748280, 0.1820866141732283561 ) ) ;
#72457=CARTESIAN_POINT ( 'NONE',  ( 1.305774278215223960, -0.6692913385826771977, 0.1292274648535927661 ) ) ;
#72459=ORIENTED_EDGE ( 'NONE', *, *, #1460, .T. ) ;
#72461=CARTESIAN_POINT ( 'NONE',  ( -0.05905511811023545637, 0.1660481256975885056, 0.3530559997133364547 ) ) ;
#72462=VERTEX_POINT ( 'NONE', #21516 ) ;
#72463=CARTESIAN_POINT ( 'NONE',  ( 0.7349081364829402885, -0.5023911411419708095, -0.1820866141732282451 ) ) ;
#72464=CARTESIAN_POINT ( 'NONE',  ( -1.384514435695537005, 0.2952755905511811885, 0.1292274648535926551 ) ) ;
#72465=CARTESIAN_POINT ( 'NONE',  ( 1.148293963254593653, 0.2952755905511810774, -0.1292274648535930714 ) ) ;
#72466=CARTESIAN_POINT ( 'NONE',  ( 1.207349081364829990, -0.6046776061558809534, -0.2411417322834644161 ) ) ;
#72467=CARTESIAN_POINT ( 'NONE',  ( 0.1771653543307093182, 0.1660481256975885056, 0.3530559997133364547 ) ) ;
#72468=CARTESIAN_POINT ( 'NONE',  ( -0.4330708661417315697, -0.6692913385826771977, 8.415575281601705876E-17 ) ) ;
#72470=CARTESIAN_POINT ( 'NONE',  ( -1.351706036745406347, 0.05413385826771626580, -0.4176697321401330321 ) ) ;
#72471=CARTESIAN_POINT ( 'NONE',  ( -0.7742782152230962556, -0.4281496062992127816, -0.4176697321401328100 ) ) ;
#72472=CARTESIAN_POINT ( 'NONE',  ( -0.4724409448818890911, -0.1870078740157480601, -0.3641732283464567677 ) ) ;
#72474=CARTESIAN_POINT ( 'NONE',  ( -0.4724409448818890911, -0.1870078740157479769, 0.4822834645669291653 ) ) ;
#72475=CARTESIAN_POINT ( 'NONE',  ( -1.191111281560509383, -2.567464376874931580E-15, -0.4445507791589072832 ) ) ;
#72476=CARTESIAN_POINT ( 'NONE',  ( 0.5971128608923890191, -0.6692913385826771977, 0.1292274648535927661 ) ) ;
#72479=CARTESIAN_POINT ( 'NONE',  ( -0.1049868766404193215, -0.6046776061558807314, 0.2411417322834647770 ) ) ;
#72480=CARTESIAN_POINT ( 'NONE',  ( 0.8267716535433078384, -0.5511811023622047445, 6.969142054262312111E-17 ) ) ;
#72481=CARTESIAN_POINT ( 'NONE',  ( -0.9120734908136473029, 0.2066929133858267931, 0.1054918080437490802 ) ) ;
#72483=CARTESIAN_POINT ( 'NONE',  ( 1.312335958005250269, -0.5023911411419708095, 0.1820866141732285504 ) ) ;
#72484=CARTESIAN_POINT ( 'NONE',  ( 1.115485564304462551, 0.05413385826771666132, 0.4176697321401328100 ) ) ;
#72486=CARTESIAN_POINT ( 'NONE',  ( -0.2362204724409442680, -0.1870078740157480879, -0.4822834645669291653 ) ) ;
#72488=CARTESIAN_POINT ( 'NONE',  ( -1.706036745406823485, 0.2306618581243848609, 0.2411417322834645549 ) ) ;
#72489=CARTESIAN_POINT ( 'NONE',  ( -0.2952755905511804668, 0.1660481256975885056, 0.3530559997133364547 ) ) ;
#72491=CARTESIAN_POINT ( 'NONE',  ( 1.161417322834646493, -0.5400638737290844871, 0.3530559997133364547 ) ) ;
#72492=CARTESIAN_POINT ( 'NONE',  ( 0.6036745406824153282, -0.6046776061558807314, 0.2411417322834647770 ) ) ;
#72493=CARTESIAN_POINT ( 'NONE',  ( 0.8005249343832028242, -0.3690944881889765550, -0.3153832671262227771 ) ) ;
#72495=CARTESIAN_POINT ( 'NONE',  ( 0.5118110236220480003, -0.5511811023622047445, 6.969142054262312111E-17 ) ) ;
#72496=CARTESIAN_POINT ( 'NONE',  ( -1.089942661822471459, 0.000000000000000000, 0.3464511005275205946 ) ) ;
#72498=CARTESIAN_POINT ( 'NONE',  ( 0.6036745406824154392, 0.2306618581243847221, -0.2411417322834647770 ) ) ;
#72500=CARTESIAN_POINT ( 'NONE',  ( 0.2034120734908144990, -0.6692913385826771977, 0.1292274648535927661 ) ) ;
#72503=CARTESIAN_POINT ( 'NONE',  ( 0.6167979002624678353, -0.3690944881889763329, 0.3153832671262228327 ) ) ;
#72504=CARTESIAN_POINT ( 'NONE',  ( 0.3608923884514443348, -0.6692913385826771977, 0.1292274648535927661 ) ) ;
#72506=CARTESIAN_POINT ( 'NONE',  ( -0.9383202099737524282, -0.08942795157527998196, 0.3641732283464567121 ) ) ;
#72507=CARTESIAN_POINT ( 'NONE',  ( -1.115485564304461219, -0.4281496062992124485, 0.4176697321401328655 ) ) ;
#72508=CARTESIAN_POINT ( 'NONE',  ( -1.443569553805773564, -0.6046776061558807314, 0.2411417322834647770 ) ) ;
#72509=CARTESIAN_POINT ( 'NONE',  ( 0.4461942257217856311, 0.2306618581243847221, -0.2411417322834647770 ) ) ;
#72510=CARTESIAN_POINT ( 'NONE',  ( -1.568241469816272105, -0.2845877964562161244, -0.3641732283464567121 ) ) ;
#72512=CARTESIAN_POINT ( 'NONE',  ( 0.6364829396325465405, -0.05778040916215522460, 0.4822834645669289988 ) ) ;
#72515=CARTESIAN_POINT ( 'NONE',  ( 1.469816272965879911, -0.6046776061558807314, 0.2411417322834647770 ) ) ;
#72516=B_SPLINE_CURVE_WITH_KNOTS ( 'NONE', 3,
 ( #78167, #46569, #13351, #13772 ),
 .UNSPECIFIED., .F., .F.,
 ( 4, 4 ),
 ( 3.593986969189856797E-07, 0.001287825409103297717 ),
 .UNSPECIFIED. ) ;
#72517=CARTESIAN_POINT ( 'NONE',  ( -1.404199475065615932, -0.004921259842519576551, 0.3153832671262227771 ) ) ;
#72518=CARTESIAN_POINT ( 'NONE',  ( 1.240157480314961314, 0.07958543189024071263, -0.2665933059059888421 ) ) ;
#72519=CARTESIAN_POINT ( 'NONE',  ( -1.358267716535432434, -0.4536011799217367080, 0.2665933059059888421 ) ) ;
#72520=CARTESIAN_POINT ( 'NONE',  ( -0.6824146981627288167, 0.1283753931104748280, 0.1820866141732283561 ) ) ;
#72521=CARTESIAN_POINT ( 'NONE',  ( 1.607611548556431069, 0.2952755905511811885, 0.1292274648535926551 ) ) ;
#72522=CARTESIAN_POINT ( 'NONE',  ( 0.5183727034120741983, 0.1771653543307087075, -0.09757992244046823083 ) ) ;
#72523=CARTESIAN_POINT ( 'NONE',  ( 0.03937007874015833325, -0.6692913385826771977, 8.415575281601705876E-17 ) ) ;
#72524=CARTESIAN_POINT ( 'NONE',  ( 1.279527559055118724, 0.1660481256975885056, 0.3530559997133364547 ) ) ;
#72525=CARTESIAN_POINT ( 'NONE',  ( 0.1574803149606306130, -0.1870078740157480879, -0.4822834645669291653 ) ) ;
#72526=CARTESIAN_POINT ( 'NONE',  ( 0.2690288713910767848, -0.5511811023622048555, -0.09757992244046775898 ) ) ;
#72527=CARTESIAN_POINT ( 'NONE',  ( 1.410761154855643795, -0.3162353388693405765, 0.4822834645669290543 ) ) ;
#72529=( BOUNDED_CURVE ( )  B_SPLINE_CURVE ( 2, ( #19469, #40088, #6425, #65775, #32094, #51433, #77136, #6840, #45119, #58173, #80891, #74157, #67843 ),
 .UNSPECIFIED., .F., .F. ) 
 B_SPLINE_CURVE_WITH_KNOTS ( ( 3, 2, 2, 2, 2, 2, 3 ),
 ( 0.7308514478433235650, 0.7310606060606060774, 0.7348484848484848619, 0.7386363636363636465, 0.7424242424242424310, 0.7462121212121212155, 0.7464212794294037279 ),
 .UNSPECIFIED. ) 
 CURVE ( )  GEOMETRIC_REPRESENTATION_ITEM ( )  RATIONAL_B_SPLINE_CURVE ( ( 0.9964447847208419695, 0.9981185001348091834, 1.000000000000000000, 0.9659258262890683122, 1.000000000000000000, 0.9659258262890683122, 1.000000000000000000, 0.9659258262890683122, 1.000000000000000000, 0.9659258262890683122, 1.000000000000000000, 0.9981185001348091834, 0.9964447847208420805 ) ) 
 REPRESENTATION_ITEM ( '' )  );
#72530=CARTESIAN_POINT ( 'NONE',  ( -0.2165354330708654795, 0.1012011053420777407, 0.2882089793578256898 ) ) ;
#72531=CARTESIAN_POINT ( 'NONE',  ( -0.9317585301837263412, 0.05413385826771666132, 0.4176697321401328100 ) ) ;
#72534=CARTESIAN_POINT ( 'NONE',  ( -0.9383202099737524282, -0.3162353388693409650, -0.4822834645669289433 ) ) ;
#72535=CARTESIAN_POINT ( 'NONE',  ( -0.07217847769028813698, -0.3162353388693409650, -0.4822834645669289433 ) ) ;
#72540=DIRECTION ( 'NONE',  ( 0.000000000000000000, 0.000000000000000000, -1.000000000000000000 ) ) ;
#72541=CARTESIAN_POINT ( 'NONE',  ( -1.456692913385826182, -0.5511811023622047445, 6.969142054262312111E-17 ) ) ;
#72543=CARTESIAN_POINT ( 'NONE',  ( -1.699475065616797398, 0.2952755905511811885, 0.1292274648535926551 ) ) ;
#72545=CARTESIAN_POINT ( 'NONE',  ( 0.3871391076115493490, -0.3162353388693405765, 0.4822834645669290543 ) ) ;
#72546=CARTESIAN_POINT ( 'NONE',  ( -0.6430446194225716283, -0.3690944881889763329, 0.3153832671262228327 ) ) ;
#72547=CARTESIAN_POINT ( 'NONE',  ( 0.9383202099737536495, -0.3162353388693405765, 0.4822834645669290543 ) ) ;
#72548=CARTESIAN_POINT ( 'NONE',  ( 0.2821522309711292364, -0.6692913385826771977, 0.1292274648535927661 ) ) ;
#72552=CARTESIAN_POINT ( 'NONE',  ( 1.286089238845145033, -0.6046776061558809534, -0.2411417322834644161 ) ) ;
#72553=CARTESIAN_POINT ( 'NONE',  ( 0.02624671916010564918, 0.2306618581243848609, 0.2411417322834645549 ) ) ;
#72554=CARTESIAN_POINT ( 'NONE',  ( 1.482939632545932307, 0.05413385826771626580, -0.4176697321401330321 ) ) ;
#72555=CARTESIAN_POINT ( 'NONE',  ( 0.7742782152230979209, 0.05413385826771626580, -0.4176697321401330321 ) ) ;
#72557=CARTESIAN_POINT ( 'NONE',  ( 0.1181102362204730916, -0.6692913385826771977, 8.415575281601705876E-17 ) ) ;
#72558=CARTESIAN_POINT ( 'NONE',  ( 0.6758530183727039509, -0.6692913385826771977, 0.1292274648535927661 ) ) ;
#72559=CARTESIAN_POINT ( 'NONE',  ( 0.01968503937007957949, -0.5400638737290845981, -0.3530559997133363437 ) ) ;
#72560=CARTESIAN_POINT ( 'NONE',  ( 0.8989501312335964611, 0.1771653543307087630, 0.09757992244046791164 ) ) ;
#72561=CARTESIAN_POINT ( 'NONE',  ( -1.325459317585300889, -0.4281496062992127816, -0.4176697321401328100 ) ) ;
#72562=CARTESIAN_POINT ( 'NONE',  ( -1.601049868766403650, -0.6046776061558807314, 0.2411417322834647770 ) ) ;
#72563=CARTESIAN_POINT ( 'NONE',  ( 0.8136482939632553313, 0.2306618581243848609, 0.2411417322834645549 ) ) ;
#72566=ORIENTED_EDGE ( 'NONE', *, *, #15170, .F. ) ;
#72568=ORIENTED_EDGE ( 'NONE', *, *, #61281, .T. ) ;
#72569=CARTESIAN_POINT ( 'NONE',  ( 1.115485564304462551, -0.4281496062992127816, -0.4176697321401328100 ) ) ;
#72570=CARTESIAN_POINT ( 'NONE',  ( 0.3740157480314966754, 0.07958543189024071263, -0.2665933059059888421 ) ) ;
#72575=CARTESIAN_POINT ( 'NONE',  ( 1.482939632545932307, 0.05413385826771626580, -0.4176697321401330321 ) ) ;
#72577=CARTESIAN_POINT ( 'NONE',  ( -0.2034120734908131112, -0.6692913385826773087, -0.1292274648535924053 ) ) ;
#72578=CARTESIAN_POINT ( 'NONE',  ( 1.181102362204724976, -0.1870078740157480879, -0.4822834645669291653 ) ) ;
#72580=CARTESIAN_POINT ( 'NONE',  ( -1.489501312335957062, -0.3162353388693409650, -0.4822834645669289433 ) ) ;
#72583=CARTESIAN_POINT ( 'NONE',  ( 1.541994750656168645, 0.1771653543307087075, -0.09757992244046823083 ) ) ;
#72585=B_SPLINE_CURVE_WITH_KNOTS ( 'NONE', 3,
 ( #53086, #65333, #33749, #51831 ),
 .UNSPECIFIED., .F., .F.,
 ( 4, 4 ),
 ( 1.999999999897049408E-07, 0.006970199999999935128 ),
 .UNSPECIFIED. ) ;
#72586=CARTESIAN_POINT ( 'NONE',  ( -1.076115485564303809, -0.5023911411419708095, -0.1820866141732282451 ) ) ;
#72587=CARTESIAN_POINT ( 'NONE',  ( -1.496062992125983815, -0.1870078740157479769, 0.4822834645669291653 ) ) ;
#72588=CARTESIAN_POINT ( 'NONE',  ( 0.6692913385826778638, -0.6692913385826771977, 8.415575281601705876E-17 ) ) ;
#72589=ORIENTED_EDGE ( 'NONE', *, *, #44487, .F. ) ;
#72590=CARTESIAN_POINT ( 'NONE',  ( 1.437007874015748810, -0.5400638737290845981, -0.3530559997133363437 ) ) ;
#72591=CARTESIAN_POINT ( 'NONE',  ( -0.4330708661417315697, 0.2066929133858268208, 0.000000000000000000 ) ) ;
#72592=CARTESIAN_POINT ( 'NONE',  ( -0.7283464566929126471, 0.07958543189024071263, -0.2665933059059888421 ) ) ;
#72593=CARTESIAN_POINT ( 'NONE',  ( 0.7414698162729663755, 0.2952755905511811885, 0.1292274648535926551 ) ) ;
#72594=CARTESIAN_POINT ( 'NONE',  ( -1.712598425196849572, 0.1660481256975885056, 0.3530559997133364547 ) ) ;
#72596=CARTESIAN_POINT ( 'NONE',  ( -0.9383202099737524282, -0.08942795157527998196, 0.3641732283464567121 ) ) ;
#72598=CARTESIAN_POINT ( 'NONE',  ( -1.410761154855641575, -0.2845877964562161244, -0.3641732283464567121 ) ) ;
#72600=CARTESIAN_POINT ( 'NONE',  ( 0.4790026246719167324, -0.05778040916215522460, 0.4822834645669289988 ) ) ;
#72601=CARTESIAN_POINT ( 'NONE',  ( -1.010498687664041384, -0.004921259842519576551, 0.3153832671262227771 ) ) ;
#72602=CARTESIAN_POINT ( 'NONE',  ( -0.1968503937007867743, -0.5511811023622047445, 6.969142054262312111E-17 ) ) ;
#72603=CARTESIAN_POINT ( 'NONE',  ( -0.3740157480314953431, -0.5400638737290845981, -0.3530559997133363437 ) ) ;
#72604=CARTESIAN_POINT ( 'NONE',  ( 1.620734908136483465, -0.6692913385826771977, 0.1292274648535927661 ) ) ;
#72606=CARTESIAN_POINT ( 'NONE',  ( 0.5643044619422579178, -0.4281496062992127816, -0.4176697321401328100 ) ) ;
#72607=CARTESIAN_POINT ( 'NONE',  ( 2.795275590551181466, 2.165354330708662012, 0.000000000000000000 ) ) ;
#72609=CARTESIAN_POINT ( 'NONE',  ( -0.6430446194225716283, -0.4281496062992124485, 0.4176697321401328655 ) ) ;
#72610=CARTESIAN_POINT ( 'NONE',  ( -0.2755905511811018171, 0.1771653543307087630, 0.000000000000000000 ) ) ;
#72611=CARTESIAN_POINT ( 'NONE',  ( -1.312335958005248715, 0.2306618581243848609, 0.2411417322834645549 ) ) ;
#72612=CARTESIAN_POINT ( 'NONE',  ( 0.5511811023622055217, -0.1870078740157479769, 0.3641732283464567677 ) ) ;
#72613=CARTESIAN_POINT ( 'NONE',  ( -0.8333333333333323711, -0.5511811023622048555, -0.09757992244046775898 ) ) ;
#72614=CARTESIAN_POINT ( 'NONE',  ( -1.240157480314959759, 0.1660481256975885056, 0.3530559997133364547 ) ) ;
#72615=CARTESIAN_POINT ( 'NONE',  ( -1.555118110236219930, 0.1660481256975885056, 0.3530559997133364547 ) ) ;
#72616=CARTESIAN_POINT ( 'NONE',  ( -1.450131233595799651, 0.2952755905511810774, -0.1292274648535930714 ) ) ;
#72618=CARTESIAN_POINT ( 'NONE',  ( 0.9055118110236227702, 0.1771653543307087630, 0.000000000000000000 ) ) ;
#72619=CARTESIAN_POINT ( 'NONE',  ( 0.4133858267716541968, 0.1660481256975885056, 0.3530559997133364547 ) ) ;
#72621=CARTESIAN_POINT ( 'NONE',  ( 1.476377952755906220, 0.07958543189024071263, -0.2665933059059888421 ) ) ;
#72624=CARTESIAN_POINT ( 'NONE',  ( -1.286089238845143479, 0.1283753931104746893, -0.1820866141732285504 ) ) ;
#72625=CARTESIAN_POINT ( 'NONE',  ( -0.5118110236220466680, 0.2952755905511811885, 0.000000000000000000 ) ) ;
#72626=CARTESIAN_POINT ( 'NONE',  ( 0.2952755905511816326, -0.5400638737290844871, 0.3530559997133364547 ) ) ;
#72627=CARTESIAN_POINT ( 'NONE',  ( -1.404199475065615932, -0.004921259842519576551, 0.3153832671262227771 ) ) ;
#72629=CARTESIAN_POINT ( 'NONE',  ( -1.476377952755905110, -0.5400638737290845981, -0.3530559997133363437 ) ) ;
#72630=CARTESIAN_POINT ( 'NONE',  ( 0.6233595800524942554, -0.05778040916215560624, -0.4822834645669293319 ) ) ;
#72631=CARTESIAN_POINT ( 'NONE',  ( 0.07874015748031558404, -0.1870078740157479769, 0.4822834645669291653 ) ) ;
#72632=CARTESIAN_POINT ( 'NONE',  ( 1.227034120734908917, -0.6692913385826771977, 0.1292274648535927661 ) ) ;
#72637=CARTESIAN_POINT ( 'NONE',  ( -0.3018372703412066094, -0.004921259842519576551, 0.3153832671262227771 ) ) ;
#72638=CARTESIAN_POINT ( 'NONE',  ( -0.4396325459317579898, 0.2952755905511811885, 0.1292274648535926551 ) ) ;
#72639=CARTESIAN_POINT ( 'NONE',  ( 0.9580052493438326877, 0.05413385826771666132, 0.4176697321401328100 ) ) ;
#72641=CARTESIAN_POINT ( 'NONE',  ( -0.05905511811023545637, 0.07958543189024085140, 0.2665933059059887866 ) ) ;
#72642=CARTESIAN_POINT ( 'NONE',  ( -1.279527559055116948, 0.1660481256975883668, -0.3530559997133364547 ) ) ;
#72643=CARTESIAN_POINT ( 'NONE',  ( -1.456692913385826182, 0.2952755905511811885, 0.000000000000000000 ) ) ;
#72647=ORIENTED_EDGE ( 'NONE', *, *, #48636, .T. ) ;
#72648=CARTESIAN_POINT ( 'NONE',  ( 1.338582677165355062, -0.1870078740157480879, -0.4822834645669291653 ) ) ;
#72649=CARTESIAN_POINT ( 'NONE',  ( -1.607611548556429737, -0.6692913385826771977, 0.1292274648535927661 ) ) ;
#72650=CARTESIAN_POINT ( 'NONE',  ( -1.220472440944881054, -0.5511811023622047445, 6.969142054262312111E-17 ) ) ;
#72651=CARTESIAN_POINT ( 'NONE',  ( -1.286089238845143479, 0.2306618581243847221, -0.2411417322834647770 ) ) ;
#72653=CARTESIAN_POINT ( 'NONE',  ( 0.2486400153428833526, 3.421639014772782816E-16, 0.3464511005275203726 ) ) ;
#72654=CARTESIAN_POINT ( 'NONE',  ( 1.049868766404200349, 0.2306618581243848609, 0.2411417322834645549 ) ) ;
#72655=CARTESIAN_POINT ( 'NONE',  ( -1.653543307086613234, -0.1870078740157480879, -0.4822834645669291653 ) ) ;
#72656=CARTESIAN_POINT ( 'NONE',  ( -0.2230971128608915943, -0.4281496062992127816, -0.4176697321401328100 ) ) ;
#72657=CARTESIAN_POINT ( 'NONE',  ( -0.02624671916010428221, -0.6046776061558807314, 0.2411417322834647770 ) ) ;
#72659=VECTOR ( 'NONE', #9631, 39.37007874015748854 ) ;
#72660=CARTESIAN_POINT ( 'NONE',  ( -1.423884514435694859, -0.05778040916215560624, -0.4822834645669293319 ) ) ;
#72662=CARTESIAN_POINT ( 'NONE',  ( 0.6955380577427828781, 0.05413385826771626580, -0.4176697321401330321 ) ) ;
#72664=CARTESIAN_POINT ( 'NONE',  ( -1.286089238845143479, 0.1283753931104746893, -0.1820866141732285504 ) ) ;
#72667=ORIENTED_EDGE ( 'NONE', *, *, #8579, .F. ) ;
#72669=CARTESIAN_POINT ( 'NONE',  ( -0.9973753280839886548, -0.6046776061558809534, -0.2411417322834644161 ) ) ;
#72670=CARTESIAN_POINT ( 'NONE',  ( -1.404199475065615932, -0.4281496062992127816, -0.4176697321401328100 ) ) ;
#72672=CARTESIAN_POINT ( 'NONE',  ( -1.587926509186350810, -0.4281496062992124485, 0.4176697321401328655 ) ) ;
#72673=CARTESIAN_POINT ( 'NONE',  ( -1.496062992125983815, -0.1870078740157480879, -0.4822834645669291653 ) ) ;
#72674=DIRECTION ( 'NONE',  ( -1.000000000000000000, -3.083952846180990281E-16, 0.000000000000000000 ) ) ;
#72675=CARTESIAN_POINT ( 'NONE',  ( -0.3249695492770445782, -2.567464376874931580E-15, -0.4445507791589072832 ) ) ;
#72677=CARTESIAN_POINT ( 'NONE',  ( -0.04593175853018302557, 0.1771653543307087630, 0.09757992244046791164 ) ) ;
#72679=CARTESIAN_POINT ( 'NONE',  ( -0.9514435695538050464, -0.2845877964562159024, 0.3641732283464567677 ) ) ;
#72680=CARTESIAN_POINT ( 'NONE',  ( -1.312335958005248715, 0.2306618581243848609, 0.2411417322834645549 ) ) ;
#72681=CARTESIAN_POINT ( 'NONE',  ( 0.9383202099737536495, -0.3162353388693405765, 0.4822834645669290543 ) ) ;
#72682=CARTESIAN_POINT ( 'NONE',  ( -0.7152230971128602510, -0.3162353388693405765, 0.4822834645669290543 ) ) ;
#72684=ORIENTED_EDGE ( 'NONE', *, *, #66179, .F. ) ;
#72685=CARTESIAN_POINT ( 'NONE',  ( -1.437007874015747477, 0.1660481256975883668, -0.3530559997133364547 ) ) ;
#72686=CARTESIAN_POINT ( 'NONE',  ( 0.8464566929133865436, 0.1660481256975883668, -0.3530559997133364547 ) ) ;
#72687=CARTESIAN_POINT ( 'NONE',  ( -1.450131233595799651, -0.5511811023622046335, 0.09757992244046803654 ) ) ;
#72694=CARTESIAN_POINT ( 'NONE',  ( -0.4133858267716528645, -0.5400638737290844871, 0.3530559997133364547 ) ) ;
#72695=CARTESIAN_POINT ( 'NONE',  ( -1.325459317585300889, -0.004921259842519576551, 0.3153832671262227771 ) ) ;
#72697=CARTESIAN_POINT ( 'NONE',  ( -1.706036745406823485, 0.2306618581243848609, 0.2411417322834645549 ) ) ;
#72699=CARTESIAN_POINT ( 'NONE',  ( -1.266404199475064773, -0.3162353388693405765, 0.4822834645669290543 ) ) ;
#72700=CARTESIAN_POINT ( 'NONE',  ( -0.4068241469816267775, 0.05413385826771626580, -0.4176697321401330321 ) ) ;
#72702=CARTESIAN_POINT ( 'NONE',  ( 0.4133858267716541968, -0.4536011799217368745, -0.2665933059059886201 ) ) ;
#72704=CARTESIAN_POINT ( 'NONE',  ( 0.4527559055118117182, 0.07958543189024071263, -0.2665933059059888421 ) ) ;
#72705=CARTESIAN_POINT ( 'NONE',  ( 0.9055118110236227702, -0.5511811023622047445, 6.969142054262312111E-17 ) ) ;
#72706=CARTESIAN_POINT ( 'NONE',  ( 0.9186351706036751663, -0.6046776061558807314, 0.2411417322834647770 ) ) ;
#72707=CARTESIAN_POINT ( 'NONE',  ( 0.1771653543307093182, -0.4536011799217368745, -0.2665933059059886201 ) ) ;
#72709=CARTESIAN_POINT ( 'NONE',  ( -1.351706036745406347, -0.4281496062992124485, 0.4176697321401328655 ) ) ;
#72710=CARTESIAN_POINT ( 'NONE',  ( 0.06561679790026316017, -0.004921259842519870586, -0.3153832671262229437 ) ) ;
#72711=CARTESIAN_POINT ( 'NONE',  ( -1.404199475065615932, -0.3690944881889765550, -0.3153832671262227771 ) ) ;
#72713=CARTESIAN_POINT ( 'NONE',  ( -1.010498687664041384, -0.004921259842519576551, 0.3153832671262227771 ) ) ;
#72715=CARTESIAN_POINT ( 'NONE',  ( -0.1574803149606292529, -0.1870078740157480879, -0.4822834645669291653 ) ) ;
#72717=CARTESIAN_POINT ( 'NONE',  ( 0.4330708661417329575, -0.5511811023622047445, 6.969142054262312111E-17 ) ) ;
#72718=CARTESIAN_POINT ( 'NONE',  ( -0.4068241469816267775, -0.004921259842519870586, -0.3153832671262229437 ) ) ;
#72719=CARTESIAN_POINT ( 'NONE',  ( -0.2887139107611542133, -0.6046776061558809534, -0.2411417322834644161 ) ) ;
#72720=CARTESIAN_POINT ( 'NONE',  ( -1.679790026246718693, 0.2306618581243847221, -0.2411417322834647770 ) ) ;
#72721=CARTESIAN_POINT ( 'NONE',  ( -1.187664041994749731, -0.2845877964562159024, 0.3641732283464567677 ) ) ;
#72723=CARTESIAN_POINT ( 'NONE',  ( 0.6824146981627303710, -0.6046776061558807314, 0.2411417322834647770 ) ) ;
#72725=ORIENTED_EDGE ( 'NONE', *, *, #40855, .T. ) ;
#72727=FACE_OUTER_BOUND ( 'NONE', #16696, .T. ) ;
#72728=CARTESIAN_POINT ( 'NONE',  ( -0.05249343832020938322, -0.5023911411419708095, -0.1820866141732282451 ) ) ;
#72729=CARTESIAN_POINT ( 'NONE',  ( -1.358267716535432434, -0.5400638737290844871, 0.3530559997133364547 ) ) ;
#72730=CARTESIAN_POINT ( 'NONE',  ( 1.607611548556431069, -0.6692913385826773087, -0.1292274648535924053 ) ) ;
#72731=CARTESIAN_POINT ( 'NONE',  ( 1.272965879265092637, -0.4281496062992127816, -0.4176697321401328100 ) ) ;
#72732=CARTESIAN_POINT ( 'NONE',  ( -0.7217847769028863381, -0.004921259842519870586, -0.3153832671262229437 ) ) ;
#72734=CARTESIAN_POINT ( 'NONE',  ( 0.7349081364829402885, -0.6046776061558809534, -0.2411417322834644161 ) ) ;
#72738=CARTESIAN_POINT ( 'NONE',  ( 1.496062992125984703, -0.1870078740157480601, -0.3641732283464567677 ) ) ;
#72739=CARTESIAN_POINT ( 'NONE',  ( -1.141732283464566011, -0.6692913385826771977, 8.415575281601705876E-17 ) ) ;
#72740=CARTESIAN_POINT ( 'NONE',  ( 1.332020997375328974, -0.05778040916215560624, -0.4822834645669293319 ) ) ;
#72742=CARTESIAN_POINT ( 'NONE',  ( 1.410761154855643795, -0.08942795157528024563, -0.3641732283464568787 ) ) ;
#72743=CARTESIAN_POINT ( 'NONE',  ( 0.006561679790026889343, -0.3162353388693409650, -0.4822834645669289433 ) ) ;
#72744=CARTESIAN_POINT ( 'NONE',  ( -0.3805774278215216522, 0.05413385826771666132, 0.4176697321401328100 ) ) ;
#72745=CARTESIAN_POINT ( 'NONE',  ( 1.666666666666667185, 0.05413385826771666132, 0.4176697321401328100 ) ) ;
#72747=CARTESIAN_POINT ( 'NONE',  ( 0.4527559055118117182, -0.4536011799217367080, 0.2665933059059888421 ) ) ;
#72751=CARTESIAN_POINT ( 'NONE',  ( -0.2887139107611542133, 0.2306618581243848609, 0.2411417322834645549 ) ) ;
#72752=CARTESIAN_POINT ( 'NONE',  ( 1.397637795275591177, -0.5400638737290844871, 0.3530559997133364547 ) ) ;
#72753=CARTESIAN_POINT ( 'NONE',  ( 0.2690288713910767848, 0.2952755905511811885, 0.1292274648535926551 ) ) ;
#72754=CARTESIAN_POINT ( 'NONE',  ( -0.2165354330708654795, 0.07958543189024085140, 0.2665933059059887866 ) ) ;
#72755=CARTESIAN_POINT ( 'NONE',  ( 1.364829396325460076, 0.2306618581243848609, 0.2411417322834645549 ) ) ;
#72756=CARTESIAN_POINT ( 'NONE',  ( -1.115485564304461219, 0.05413385826771626580, -0.4176697321401330321 ) ) ;
#72757=CARTESIAN_POINT ( 'NONE',  ( -0.03937007874015669567, -0.6692913385826771977, 8.415575281601705876E-17 ) ) ;
#72758=CARTESIAN_POINT ( 'NONE',  ( -0.9842519685039365918, -0.6692913385826771977, 8.415575281601705876E-17 ) ) ;
#72759=CARTESIAN_POINT ( 'NONE',  ( 0.9711286089238851948, 0.2306618581243848609, 0.2411417322834645549 ) ) ;
#72760=CARTESIAN_POINT ( 'NONE',  ( 1.049868766404200127, -0.6046776061558809534, -0.2411417322834644161 ) ) ;
#72761=CARTESIAN_POINT ( 'NONE',  ( 1.062992125984252745, 0.2952755905511811885, 0.000000000000000000 ) ) ;
#72763=CARTESIAN_POINT ( 'NONE',  ( -0.06561679790026180015, -0.004921259842519576551, 0.3153832671262227771 ) ) ;
#72767=CARTESIAN_POINT ( 'NONE',  ( -0.7217847769028863381, -0.004921259842519870586, -0.3153832671262229437 ) ) ;
#72768=CARTESIAN_POINT ( 'NONE',  ( -0.1181102362204717315, -0.6692913385826771977, 8.415575281601705876E-17 ) ) ;
#72770=CARTESIAN_POINT ( 'NONE',  ( -0.3608923884514428360, -0.6692913385826773087, -0.1292274648535924053 ) ) ;
#72771=CARTESIAN_POINT ( 'NONE',  ( -0.2230971128608915943, -0.4281496062992127816, -0.4176697321401328100 ) ) ;
#72772=CARTESIAN_POINT ( 'NONE',  ( -0.8792650918635160906, -0.4281496062992124485, 0.4176697321401328655 ) ) ;
#72773=CARTESIAN_POINT ( 'NONE',  ( -1.607611548556429737, -0.6692913385826771977, 0.1292274648535927661 ) ) ;
#72774=CARTESIAN_POINT ( 'NONE',  ( 1.437007874015748810, -0.4536011799217368745, -0.2665933059059886201 ) ) ;
#72775=CARTESIAN_POINT ( 'NONE',  ( -1.614173228346455824, 0.2952755905511811885, 0.000000000000000000 ) ) ;
#72777=CARTESIAN_POINT ( 'NONE',  ( 0.4461942257217855201, -0.5023911411419708095, 0.1820866141732285504 ) ) ;
#72778=CARTESIAN_POINT ( 'NONE',  ( 0.1049868766404206816, 0.2306618581243848609, 0.2411417322834645549 ) ) ;
#72779=CARTESIAN_POINT ( 'NONE',  ( 0.2493438320209980519, 0.05413385826771666132, 0.4176697321401328100 ) ) ;
#72782=CARTESIAN_POINT ( 'NONE',  ( -0.6167979002624665030, 0.009842519685039463617, 0.3409548833797002576 ) ) ;
#72785=CARTESIAN_POINT ( 'NONE',  ( -0.7349081364829390672, 0.2306618581243847221, -0.2411417322834647770 ) ) ;
#72788=CARTESIAN_POINT ( 'NONE',  ( -1.423884514435694859, -0.08942795157528024563, -0.3641732283464568787 ) ) ;
#72789=CARTESIAN_POINT ( 'NONE',  ( 0.8989501312335963501, -0.6692913385826773087, -0.1292274648535924053 ) ) ;
#72790=CARTESIAN_POINT ( 'NONE',  ( 0.9580052493438327987, -0.4281496062992127816, -0.4176697321401328100 ) ) ;
#72791=CARTESIAN_POINT ( 'NONE',  ( -0.02624671916010428221, 0.1283753931104746893, -0.1820866141732285504 ) ) ;
#72792=CARTESIAN_POINT ( 'NONE',  ( 0.1312335958005255154, -0.6046776061558807314, 0.2411417322834647770 ) ) ;
#72794=CARTESIAN_POINT ( 'NONE',  ( 0.09842519685039434474, 0.07958543189024085140, 0.2665933059059887866 ) ) ;
#72795=CARTESIAN_POINT ( 'NONE',  ( 0.006561679790026889343, -0.05778040916215522460, 0.4822834645669289988 ) ) ;
#72798=CARTESIAN_POINT ( 'NONE',  ( 1.561679790026247350, -0.3690944881889763329, 0.3153832671262228327 ) ) ;
#72799=CARTESIAN_POINT ( 'NONE',  ( 0.1246719160104994284, -0.5511811023622046335, 0.09757992244046803654 ) ) ;
#72800=CARTESIAN_POINT ( 'NONE',  ( 1.437007874015748810, -0.4536011799217368745, -0.2665933059059886201 ) ) ;
#72801=CARTESIAN_POINT ( 'NONE',  ( -1.305774278215222184, -0.6692913385826773087, -0.1292274648535924053 ) ) ;
#72802=CARTESIAN_POINT ( 'NONE',  ( -0.5839895013123351797, -0.5511811023622046335, 0.09757992244046803654 ) ) ;
#72803=CARTESIAN_POINT ( 'NONE',  ( -1.034321223653607236, 5.987370802660155681E-15, -0.4118484887281962936 ) ) ;
#72804=CARTESIAN_POINT ( 'NONE',  ( -0.8989501312335946848, 0.2952755905511810774, -0.1292274648535930714 ) ) ;
#72805=CARTESIAN_POINT ( 'NONE',  ( -0.7349081364829387342, -0.6046776061558807314, 0.2411417322834647770 ) ) ;
#72806=CARTESIAN_POINT ( 'NONE',  ( 0.1706036745406830368, -0.4281496062992127816, -0.4176697321401328100 ) ) ;
#72809=LINE ( 'NONE', #47951, #26063 ) ;
#72810=CARTESIAN_POINT ( 'NONE',  ( 0.8070866141732289112, -0.4536011799217368745, -0.2665933059059886201 ) ) ;
#72811=CARTESIAN_POINT ( 'NONE',  ( 0.8333333333333340365, 0.2952755905511810774, -0.1292274648535930714 ) ) ;
#72812=CARTESIAN_POINT ( 'NONE',  ( -1.299212598425196097, -0.5511811023622047445, 6.969142054262312111E-17 ) ) ;
#72813=EDGE_CURVE ( 'NONE', #25966, #23493, #42106, .T. ) ;
#72814=CARTESIAN_POINT ( 'NONE',  ( 0.9973753280839902091, -0.6046776061558807314, 0.2411417322834647770 ) ) ;
#72815=CARTESIAN_POINT ( 'NONE',  ( -1.102362204724408601, -0.1870078740157479769, 0.3641732283464567677 ) ) ;
#72816=CARTESIAN_POINT ( 'NONE',  ( -0.6561679790026240244, -0.6046776061558807314, 0.2411417322834647770 ) ) ;
#72817=CARTESIAN_POINT ( 'NONE',  ( 0.07217847769028949700, -0.2845877964562159024, 0.3641732283464567677 ) ) ;
#72818=CARTESIAN_POINT ( 'NONE',  ( -0.8768409086929770391, 5.410171027439680070E-15, -0.4118484887281949058 ) ) ;
#72819=CARTESIAN_POINT ( 'NONE',  ( 0.8202099737532813073, 0.1771653543307087630, 0.09757992244046791164 ) ) ;
#72820=EDGE_CURVE ( 'NONE', #36098, #7338, #29886, .T. ) ;
#72821=CARTESIAN_POINT ( 'NONE',  ( 0.1640419947506569498, -0.3162353388693409650, -0.4822834645669289433 ) ) ;
#72823=CARTESIAN_POINT ( 'NONE',  ( -0.8202099737532801971, -0.6692913385826771977, 0.1292274648535927661 ) ) ;
#72825=CARTESIAN_POINT ( 'NONE',  ( 1.069553805774278610, -0.5511811023622046335, 0.09757992244046803654 ) ) ;
#72826=CARTESIAN_POINT ( 'NONE',  ( 0.5774278215223104249, 0.2306618581243848609, 0.2411417322834645549 ) ) ;
#72827=CARTESIAN_POINT ( 'NONE',  ( -0.4199475065616791736, -0.6046776061558807314, 0.2411417322834647770 ) ) ;
#72828=CARTESIAN_POINT ( 'NONE',  ( -0.4265091863517051496, -0.5511811023622046335, 0.09757992244046803654 ) ) ;
#72830=CARTESIAN_POINT ( 'NONE',  ( 0.1443569553805781891, -0.004921259842519870586, -0.3153832671262229437 ) ) ;
#72831=CARTESIAN_POINT ( 'NONE',  ( 0.2427821522309719648, -0.05778040916215522460, 0.4822834645669289988 ) ) ;
#72832=CARTESIAN_POINT ( 'NONE',  ( -0.9251968503937002541, 0.07958543189024085140, 0.2665933059059887866 ) ) ;
#72834=CARTESIAN_POINT ( 'NONE',  ( -0.9580052493438311334, 0.05413385826771626580, -0.4176697321401330321 ) ) ;
#72835=CARTESIAN_POINT ( 'NONE',  ( 0.8558026128237107288, -1.283732188437465593E-15, -0.4281993546915538462 ) ) ;
#72837=CARTESIAN_POINT ( 'NONE',  ( -0.9514435695538050464, -0.2845877964562159024, 0.3641732283464567677 ) ) ;
#72838=CARTESIAN_POINT ( 'NONE',  ( -0.02624671916010428221, -0.6046776061558807314, 0.2411417322834647770 ) ) ;
#72839=ADVANCED_FACE ( 'NONE', ( #42515 ), #2993, .T. ) ;
#72841=CARTESIAN_POINT ( 'NONE',  ( -0.7414698162729651543, -0.6692913385826771977, 0.1292274648535927661 ) ) ;
#72842=CARTESIAN_POINT ( 'NONE',  ( -2.795275590551181910, 1.850393700787402729, -6.635626899597537341E-17 ) ) ;
#72843=CARTESIAN_POINT ( 'NONE',  ( 1.033630966599880630, -4.927456884911482678E-16, 0.4445507791589062840 ) ) ;
#72844=CARTESIAN_POINT ( 'NONE',  ( 1.102362204724410155, -0.1870078740157479769, 0.4822834645669291653 ) ) ;
#72845=CARTESIAN_POINT ( 'NONE',  ( 0.6889763779527566800, -0.5400638737290844871, 0.3530559997133364547 ) ) ;
#72847=CARTESIAN_POINT ( 'NONE',  ( 1.463254593175853824, 0.2952755905511810774, -0.1292274648535930714 ) ) ;
#72848=CARTESIAN_POINT ( 'NONE',  ( -1.509186351706035767, 0.05413385826771626580, -0.4176697321401330321 ) ) ;
#72851=ADVANCED_FACE ( 'NONE', ( #54318 ), #17292, .F. ) ;
#72852=CARTESIAN_POINT ( 'NONE',  ( -0.5643044619422565855, -0.3690944881889763329, 0.3153832671262228327 ) ) ;
#72855=CARTESIAN_POINT ( 'NONE',  ( 0.6496062992125991586, 0.1660481256975885056, 0.3530559997133364547 ) ) ;
#72856=CARTESIAN_POINT ( 'NONE',  ( -0.02624671916010428221, -0.6046776061558807314, 0.2411417322834647770 ) ) ;
#72857=CARTESIAN_POINT ( 'NONE',  ( -0.8595800524934373854, -0.05778040916215522460, 0.4822834645669289988 ) ) ;
#72858=CARTESIAN_POINT ( 'NONE',  ( 1.666666666666667185, 0.05413385826771666132, 0.4176697321401328100 ) ) ;
#72859=CARTESIAN_POINT ( 'NONE',  ( -1.082677165354329896, -0.4536011799217368745, -0.2665933059059886201 ) ) ;
#72861=CARTESIAN_POINT ( 'NONE',  ( 0.5511811023622055217, -0.1870078740157479769, 0.4822834645669291653 ) ) ;
#72862=CARTESIAN_POINT ( 'NONE',  ( 0.5118110236220478892, 0.1771653543307087630, 0.000000000000000000 ) ) ;
#72863=CARTESIAN_POINT ( 'NONE',  ( -1.010498687664041384, 0.05413385826771666132, 0.4176697321401328100 ) ) ;
#72865=CARTESIAN_POINT ( 'NONE',  ( -1.391076115485563314, -0.6046776061558809534, -0.2411417322834644161 ) ) ;
#72866=CARTESIAN_POINT ( 'NONE',  ( -1.587926509186350810, -0.3690944881889763329, 0.3153832671262228327 ) ) ;
#72868=CARTESIAN_POINT ( 'NONE',  ( 1.207349081364829990, 0.2306618581243848609, 0.2411417322834645549 ) ) ;
#72869=CARTESIAN_POINT ( 'NONE',  ( 1.469816272965879911, -0.5023911411419708095, 0.1820866141732285504 ) ) ;
#72872=CARTESIAN_POINT ( 'NONE',  ( -0.4790026246719152336, -0.05778040916215560624, -0.4822834645669293319 ) ) ;
#72874=CARTESIAN_POINT ( 'NONE',  ( 0.5643044619422579178, -0.3690944881889765550, -0.3153832671262227771 ) ) ;
#72875=CARTESIAN_POINT ( 'NONE',  ( -1.233595800524933894, 0.2306618581243848609, 0.2411417322834645549 ) ) ;
#72876=CARTESIAN_POINT ( 'NONE',  ( 0.8661417322834652488, -0.1870078740157480879, -0.4822834645669291653 ) ) ;
#72877=CARTESIAN_POINT ( 'NONE',  ( 0.8202099737532813073, 0.2952755905511811885, 0.1292274648535926551 ) ) ;
#72878=CARTESIAN_POINT ( 'NONE',  ( 0.3674540682414705883, 0.2306618581243847221, -0.2411417322834647770 ) ) ;
#72879=CARTESIAN_POINT ( 'NONE',  ( -0.5643044619422565855, -0.4281496062992124485, 0.4176697321401328655 ) ) ;
#72881=CARTESIAN_POINT ( 'NONE',  ( -1.706036745406823485, 0.2306618581243848609, 0.2411417322834645549 ) ) ;
#72882=CARTESIAN_POINT ( 'NONE',  ( -0.7939632545931750718, -0.05778040916215560624, -0.4822834645669293319 ) ) ;
#72883=CARTESIAN_POINT ( 'NONE',  ( -0.4068241469816264999, -0.3690944881889763329, 0.3153832671262228327 ) ) ;
#72884=CARTESIAN_POINT ( 'NONE',  ( 1.305774278215223960, -0.6692913385826771977, 0.1292274648535927661 ) ) ;
#72885=CARTESIAN_POINT ( 'NONE',  ( 1.502624671916010790, -0.05778040916215522460, 0.4822834645669289988 ) ) ;
#72886=CARTESIAN_POINT ( 'NONE',  ( -0.3083989501312330295, -0.05778040916215522460, 0.4822834645669289988 ) ) ;
#72888=CARTESIAN_POINT ( 'NONE',  ( 0.7939632545931766261, -0.05778040916215522460, 0.4822834645669289988 ) ) ;
#72890=CARTESIAN_POINT ( 'NONE',  ( -1.436417322834643739, 2.401574803149606474, -0.3149606299212598381 ) ) ;
#72891=CARTESIAN_POINT ( 'NONE',  ( -0.1706036745406816491, 0.05413385826771626580, -0.4176697321401330321 ) ) ;
#72892=CARTESIAN_POINT ( 'NONE',  ( 1.023622047244095334, -0.1870078740157479769, 0.3641732283464567677 ) ) ;
#72893=CARTESIAN_POINT ( 'NONE',  ( 0.4848630542936502308, 1.968099216065431811, -0.4919401540133077622 ) ) ;
#72895=CARTESIAN_POINT ( 'NONE',  ( 1.391076115485564868, 0.1283753931104746893, -0.1820866141732285504 ) ) ;
#72896=CARTESIAN_POINT ( 'NONE',  ( 1.286089238845145033, 0.2306618581243848609, 0.2411417322834645549 ) ) ;
#72898=CARTESIAN_POINT ( 'NONE',  ( -0.4265091863517051496, 0.2952755905511810774, -0.1292274648535930714 ) ) ;
#72900=CARTESIAN_POINT ( 'NONE',  ( 1.253280839895013710, -0.2845877964562159024, 0.3641732283464567677 ) ) ;
#72901=CARTESIAN_POINT ( 'NONE',  ( -0.03937007874015669567, -0.6692913385826771977, 8.415575281601705876E-17 ) ) ;
#72903=CARTESIAN_POINT ( 'NONE',  ( 1.200787401574803681, 0.1660481256975885056, 0.3530559997133364547 ) ) ;
#72904=CARTESIAN_POINT ( 'NONE',  ( 0.7086614173228352742, -0.1870078740157480879, -0.4822834645669291653 ) ) ;
#72905=CARTESIAN_POINT ( 'NONE',  ( 0.4658792650918641698, -0.08942795157528024563, -0.3641732283464568787 ) ) ;
#72907=CARTESIAN_POINT ( 'NONE',  ( 0.3346456692913393205, -0.4536011799217368745, -0.2665933059059886201 ) ) ;
#72910=CARTESIAN_POINT ( 'NONE',  ( 0.8727034120734913358, -0.05778040916215522460, 0.4822834645669289988 ) ) ;
#72912=CARTESIAN_POINT ( 'NONE',  ( 0.9348729704079946634, -8.644661201599092366E-16, -0.4445507791589066171 ) ) ;
#72914=CARTESIAN_POINT ( 'NONE',  ( 5.463695987328526437E-16, -0.1870078740157479769, 0.3641732283464567677 ) ) ;
#72916=CARTESIAN_POINT ( 'NONE',  ( -0.07874015748031421014, -0.1870078740157479769, 0.4822834645669291653 ) ) ;
#72917=CARTESIAN_POINT ( 'NONE',  ( 1.574803149606299746, -0.1870078740157480601, -0.3641732283464567677 ) ) ;
#72918=CARTESIAN_POINT ( 'NONE',  ( -1.404199475065615932, -0.004921259842519576551, 0.3153832671262227771 ) ) ;
#72919=CARTESIAN_POINT ( 'NONE',  ( -1.049868766404198794, 0.2306618581243847221, -0.2411417322834647770 ) ) ;
#72920=CARTESIAN_POINT ( 'NONE',  ( 0.7086614173228353852, -0.1870078740157479769, 0.4822834645669291653 ) ) ;
#72921=CARTESIAN_POINT ( 'NONE',  ( 1.515748031496063408, 0.1660481256975885056, 0.3530559997133364547 ) ) ;
#72922=CARTESIAN_POINT ( 'NONE',  ( 0.3049517105654749871, 8.471767977567108961E-16, -0.4445507791589058955 ) ) ;
#72923=CARTESIAN_POINT ( 'NONE',  ( 0.6955380577427828781, 0.05413385826771626580, -0.4176697321401330321 ) ) ;
#72925=CARTESIAN_POINT ( 'NONE',  ( 1.594488188976378673, -0.5400638737290845981, -0.3530559997133363437 ) ) ;
#72926=CARTESIAN_POINT ( 'NONE',  ( 0.8530183727034128527, -0.4281496062992124485, 0.4176697321401328655 ) ) ;
#72928=CARTESIAN_POINT ( 'NONE',  ( -1.443569553805773564, -0.5023911411419708095, 0.1820866141732285504 ) ) ;
#72929=CARTESIAN_POINT ( 'NONE',  ( 1.397637795275591177, 0.07958543189024071263, -0.2665933059059888421 ) ) ;
#72930=CARTESIAN_POINT ( 'NONE',  ( -1.384514435695537005, -0.5511811023622048555, -0.09757992244046775898 ) ) ;
#72931=CARTESIAN_POINT ( 'NONE',  ( -0.8989501312335946848, -0.5511811023622046335, 0.09757992244046803654 ) ) ;
#72932=CARTESIAN_POINT ( 'NONE',  ( 1.522309711286089939, -0.6046776061558809534, -0.2411417322834644161 ) ) ;
#72933=CARTESIAN_POINT ( 'NONE',  ( 0.5446194225721792126, -0.08942795157528024563, -0.3641732283464568787 ) ) ;
#72934=CARTESIAN_POINT ( 'NONE',  ( 0.2099737532808405305, -0.6046776061558807314, 0.2411417322834647770 ) ) ;
#72935=CARTESIAN_POINT ( 'NONE',  ( 1.062992125984252745, -0.6692913385826771977, 8.415575281601705876E-17 ) ) ;
#72936=CARTESIAN_POINT ( 'NONE',  ( 0.08530183727034192087, -0.05778040916215522460, 0.4822834645669289988 ) ) ;
#72937=CARTESIAN_POINT ( 'NONE',  ( -0.05249343832020938322, -0.5023911411419708095, -0.1820866141732282451 ) ) ;
#72938=CARTESIAN_POINT ( 'NONE',  ( 1.292650918635171564, 0.2952755905511811885, 0.1292274648535926551 ) ) ;
#72939=CARTESIAN_POINT ( 'NONE',  ( -1.574803149606298192, -0.1870078740157480879, -0.4822834645669291653 ) ) ;
#72940=CARTESIAN_POINT ( 'NONE',  ( -0.9973753280839886548, -0.6046776061558809534, -0.2411417322834644161 ) ) ;
#72943=CARTESIAN_POINT ( 'NONE',  ( -0.6627296587926501115, 0.2952755905511810774, -0.1292274648535930714 ) ) ;
#72944=CARTESIAN_POINT ( 'NONE',  ( 0.01968503937007930540, 0.1660481256975885056, 0.3530559997133364547 ) ) ;
#72947=VERTEX_POINT ( 'NONE', #42920 ) ;
#72950=CARTESIAN_POINT ( 'NONE',  ( 0.9776902887139113929, 0.2952755905511811885, 0.1292274648535926551 ) ) ;
#72952=CARTESIAN_POINT ( 'NONE',  ( -1.161417322834644716, -0.4536011799217368745, -0.2665933059059886201 ) ) ;
#72954=CARTESIAN_POINT ( 'NONE',  ( 1.568241469816273437, -0.2845877964562159024, 0.3641732283464567677 ) ) ;
#72956=CARTESIAN_POINT ( 'NONE',  ( -0.02624671916010428221, 0.2306618581243847221, -0.2411417322834647770 ) ) ;
#72957=CARTESIAN_POINT ( 'NONE',  ( -0.5971128608923877978, 0.1771653543307087630, 0.09757992244046791164 ) ) ;
#72958=CARTESIAN_POINT ( 'NONE',  ( 0.6758530183727039509, 0.2952755905511810774, -0.1292274648535930714 ) ) ;
#72959=CARTESIAN_POINT ( 'NONE',  ( 0.4068241469816279987, -0.4281496062992127816, -0.4176697321401328100 ) ) ;
#72963=CARTESIAN_POINT ( 'NONE',  ( 1.148293963254593875, -0.6692913385826771977, 0.1292274648535927661 ) ) ;
#72964=CARTESIAN_POINT ( 'NONE',  ( 0.1968503937007881344, 0.2952755905511811885, 0.000000000000000000 ) ) ;
#72965=CARTESIAN_POINT ( 'NONE',  ( -0.9251968503937002541, -0.5400638737290845981, -0.3530559997133363437 ) ) ;
#72966=CARTESIAN_POINT ( 'NONE',  ( -1.581364829396324945, -0.05778040916215560624, -0.4822834645669293319 ) ) ;
#72967=CARTESIAN_POINT ( 'NONE',  ( 0.9383202099737538715, -0.05778040916215560624, -0.4822834645669293319 ) ) ;
#72969=CARTESIAN_POINT ( 'NONE',  ( -0.4396325459317579898, 0.2952755905511811885, 0.1292274648535926551 ) ) ;
#72970=CARTESIAN_POINT ( 'NONE',  ( 0.4855643044619430415, -0.4281496062992127816, -0.4176697321401328100 ) ) ;
#72971=CARTESIAN_POINT ( 'NONE',  ( -0.03937007874015669567, 0.2952755905511811885, 0.000000000000000000 ) ) ;
#72972=CARTESIAN_POINT ( 'NONE',  ( 0.8398950131233602345, -0.5023911411419708095, 0.1820866141732285504 ) ) ;
#72973=CARTESIAN_POINT ( 'NONE',  ( -1.528871391076114250, 0.2952755905511810774, -0.1292274648535930714 ) ) ;
#72974=CARTESIAN_POINT ( 'NONE',  ( -1.535433070866141225, 0.2952755905511811885, 0.000000000000000000 ) ) ;
#72975=CARTESIAN_POINT ( 'NONE',  ( 0.6955380577427828781, 0.05413385826771626580, -0.4176697321401330321 ) ) ;
#72981=CARTESIAN_POINT ( 'NONE',  ( 1.220472440944882608, 0.2952755905511811885, 0.000000000000000000 ) ) ;
#72982=CARTESIAN_POINT ( 'NONE',  ( 0.7414698162729663755, -0.5511811023622048555, -0.09757992244046775898 ) ) ;
#72988=CARTESIAN_POINT ( 'NONE',  ( -1.620734908136482577, 0.2952755905511811885, 0.1292274648535926551 ) ) ;
#72990=CARTESIAN_POINT ( 'NONE',  ( -0.2493438320209966919, 0.05413385826771626580, -0.4176697321401330321 ) ) ;
#72991=CARTESIAN_POINT ( 'NONE',  ( 1.305774278215223960, 0.2952755905511810774, -0.1292274648535930714 ) ) ;
#72992=VERTEX_POINT ( 'NONE', #62291 ) ;
#72993=CARTESIAN_POINT ( 'NONE',  ( -1.686351706036744558, 0.2952755905511810774, -0.1292274648535930714 ) ) ;
#72994=CARTESIAN_POINT ( 'NONE',  ( 1.614173228346457378, -0.5511811023622047445, 6.969142054262312111E-17 ) ) ;
#72996=CARTESIAN_POINT ( 'NONE',  ( 1.574803149606299746, -0.1870078740157480601, -0.3641732283464567677 ) ) ;
#72998=CARTESIAN_POINT ( 'NONE',  ( -1.391076115485563314, -0.5023911411419708095, -0.1820866141732282451 ) ) ;
#73000=CARTESIAN_POINT ( 'NONE',  ( 0.3740157480314966754, -0.5400638737290844871, 0.3530559997133364547 ) ) ;
#73002=CARTESIAN_POINT ( 'NONE',  ( 1.561679790026247350, 0.05413385826771626580, -0.4176697321401330321 ) ) ;
#73004=CARTESIAN_POINT ( 'NONE',  ( -0.9383202099737524282, -0.08942795157527998196, 0.3641732283464567121 ) ) ;
#73005=CARTESIAN_POINT ( 'NONE',  ( 0.6824146981627303710, -0.6046776061558807314, 0.2411417322834647770 ) ) ;
#73006=CARTESIAN_POINT ( 'NONE',  ( 1.430446194225722500, -0.004921259842519576551, 0.3153832671262227771 ) ) ;
#73009=CARTESIAN_POINT ( 'NONE',  ( -0.8070866141732276899, -0.4536011799217367080, 0.2665933059059888421 ) ) ;
#73010=CARTESIAN_POINT ( 'NONE',  ( -1.437007874015747477, 0.07958543189024071263, -0.2665933059059888421 ) ) ;
#73011=CARTESIAN_POINT ( 'NONE',  ( -1.220472440944882386, 0.000000000000000000, -0.4445507791589061175 ) ) ;
#73012=CARTESIAN_POINT ( 'NONE',  ( 0.4461942257217855201, -0.6046776061558807314, 0.2411417322834647770 ) ) ;
#73013=CARTESIAN_POINT ( 'NONE',  ( -1.036745406824146176, -0.3690944881889763329, 0.3153832671262228327 ) ) ;
#73014=CARTESIAN_POINT ( 'NONE',  ( -0.2952755905511804668, 0.07958543189024085140, 0.2665933059059887866 ) ) ;
#73015=CARTESIAN_POINT ( 'NONE',  ( -0.3083989501312330295, -0.05778040916215522460, 0.4822834645669289988 ) ) ;
#73016=CARTESIAN_POINT ( 'NONE',  ( -1.555118110236219930, -0.4536011799217368745, -0.2665933059059886201 ) ) ;
#73018=CARTESIAN_POINT ( 'NONE',  ( 0.8595800524934390507, -0.05778040916215560624, -0.4822834645669293319 ) ) ;
#73019=( BOUNDED_CURVE ( )  B_SPLINE_CURVE ( 2, ( #70373, #12728, #64064, #30005, #32916, #57734, #6820, #19448, #26175, #45941, #32490, #72059, #522 ),
 .UNSPECIFIED., .F., .F. ) 
 B_SPLINE_CURVE_WITH_KNOTS ( ( 3, 2, 2, 2, 2, 2, 3 ),
 ( 0.6399423569342326257, 0.6401515151515151381, 0.6439393939393940336, 0.6477272727272727071, 0.6515151515151516026, 0.6553030303030302761, 0.6555121885203127885 ),
 .UNSPECIFIED. ) 
 CURVE ( )  GEOMETRIC_REPRESENTATION_ITEM ( )  RATIONAL_B_SPLINE_CURVE ( ( 0.9964447847208418585, 0.9981185001348090724, 1.000000000000000000, 0.9659258262890683122, 1.000000000000000000, 0.9659258262890683122, 1.000000000000000000, 0.9659258262890683122, 1.000000000000000000, 0.9659258262890683122, 1.000000000000000000, 0.9981185001348091834, 0.9964447847208420805 ) ) 
 REPRESENTATION_ITEM ( '' )  );
#73020=CARTESIAN_POINT ( 'NONE',  ( 0.8764808517432199908, -2.398893483443748302E-16, 0.4281993546915529580 ) ) ;
#73022=CARTESIAN_POINT ( 'NONE',  ( -0.7414698162729651543, 0.2952755905511810774, -0.1292274648535930714 ) ) ;
#73023=CARTESIAN_POINT ( 'NONE',  ( -0.2099737532808391705, -0.5023911411419708095, -0.1820866141732282451 ) ) ;
#73024=CARTESIAN_POINT ( 'NONE',  ( -1.332020997375327642, -0.05778040916215522460, 0.4822834645669289988 ) ) ;
#73025=CARTESIAN_POINT ( 'NONE',  ( 0.3543307086614181922, -0.5511811023622047445, 6.969142054262312111E-17 ) ) ;
#73026=CARTESIAN_POINT ( 'NONE',  ( -0.8070866141732276899, -0.4536011799217367080, 0.2665933059059888421 ) ) ;
#73027=CARTESIAN_POINT ( 'NONE',  ( -1.076115485564303809, 0.2306618581243848609, 0.2411417322834645549 ) ) ;
#73028=CARTESIAN_POINT ( 'NONE',  ( 1.581364829396326277, -0.08942795157527998196, 0.3641732283464567121 ) ) ;
#73029=CARTESIAN_POINT ( 'NONE',  ( 1.272965879265092637, -0.4281496062992127816, -0.4176697321401328100 ) ) ;
#73030=CARTESIAN_POINT ( 'NONE',  ( 1.089589480386154330, 0.004960608223779187052, -0.3437734562760187962 ) ) ;
#73031=CARTESIAN_POINT ( 'NONE',  ( 0.9645669291338591078, -0.4536011799217368745, -0.2665933059059886201 ) ) ;
#73032=CARTESIAN_POINT ( 'NONE',  ( 0.4658792650918641698, -0.05778040916215560624, -0.4822834645669293319 ) ) ;
#73034=CARTESIAN_POINT ( 'NONE',  ( 1.443569553805774897, 0.1283753931104748280, 0.1820866141732283561 ) ) ;
#73036=B_SPLINE_CURVE_WITH_KNOTS ( 'NONE', 3,
 ( #59387, #8473, #40456, #9304 ),
 .UNSPECIFIED., .F., .F.,
 ( 4, 4 ),
 ( 0.07436403195037320779, 0.07455104739251885992 ),
 .UNSPECIFIED. ) ;
#73038=CARTESIAN_POINT ( 'NONE',  ( -1.141732283464566011, 0.1771653543307087630, 0.000000000000000000 ) ) ;
#73039=CARTESIAN_POINT ( 'NONE',  ( -0.4002624671916004129, -0.3162353388693405765, 0.4822834645669290543 ) ) ;
#73040=CARTESIAN_POINT ( 'NONE',  ( 0.4527559055118117182, -0.5400638737290844871, 0.3530559997133364547 ) ) ;
#73041=CARTESIAN_POINT ( 'NONE',  ( -1.581364829396324945, -0.2845877964562159024, 0.3641732283464567677 ) ) ;
#73043=CARTESIAN_POINT ( 'NONE',  ( -1.430446194225721390, -0.4281496062992124485, 0.4176697321401328655 ) ) ;
#73044=CARTESIAN_POINT ( 'NONE',  ( 0.2755905511811031494, 0.2952755905511811885, 0.000000000000000000 ) ) ;
#73045=CARTESIAN_POINT ( 'NONE',  ( -0.08530183727034056085, -0.3162353388693405765, 0.4822834645669290543 ) ) ;
#73046=CARTESIAN_POINT ( 'NONE',  ( 1.351706036745407458, -0.4281496062992127816, -0.4176697321401328100 ) ) ;
#73054=CARTESIAN_POINT ( 'NONE',  ( -0.07874015748031421014, -0.1870078740157480601, -0.3641732283464567677 ) ) ;
#73055=CARTESIAN_POINT ( 'NONE',  ( -0.4199475065616791736, 0.2306618581243847221, -0.2411417322834647770 ) ) ;
#73056=CARTESIAN_POINT ( 'NONE',  ( 0.9776902887139113929, 0.2952755905511811885, 0.1292274648535926551 ) ) ;
#73058=CARTESIAN_POINT ( 'NONE',  ( 0.03280839895013198948, -0.5511811023622048555, -0.09757992244046775898 ) ) ;
#73059=CARTESIAN_POINT ( 'NONE',  ( -1.128608923884513837, 0.2306618581243847221, -0.2411417322834647770 ) ) ;
#73060=CARTESIAN_POINT ( 'NONE',  ( 1.522309711286089939, -0.6046776061558809534, -0.2411417322834644161 ) ) ;
#73063=ORIENTED_EDGE ( 'NONE', *, *, #11002, .T. ) ;
#73064=VERTEX_POINT ( 'NONE', #66976 ) ;
#73065=CARTESIAN_POINT ( 'NONE',  ( 1.108923884514436242, -0.05778040916215522460, 0.4822834645669289988 ) ) ;
#73067=CARTESIAN_POINT ( 'NONE',  ( -1.548556430446193399, 0.2306618581243848609, 0.2411417322834645549 ) ) ;
#73068=CARTESIAN_POINT ( 'NONE',  ( -1.259842519685038686, -0.1870078740157480601, -0.3641732283464567677 ) ) ;
#73069=CARTESIAN_POINT ( 'NONE',  ( -1.161417322834644716, 0.1660481256975885056, 0.3530559997133364547 ) ) ;
#73072=CARTESIAN_POINT ( 'NONE',  ( 1.167979002624672580, -0.4281496062992124485, 0.4176697321401328655 ) ) ;
#73073=CARTESIAN_POINT ( 'NONE',  ( -1.469816272965878357, -0.6046776061558809534, -0.2411417322834644161 ) ) ;
#73074=CARTESIAN_POINT ( 'NONE',  ( -0.09842519685039295696, 0.1660481256975883668, -0.3530559997133364547 ) ) ;
#73075=CARTESIAN_POINT ( 'NONE',  ( -0.006561679790025524116, -0.3162353388693405765, 0.4822834645669290543 ) ) ;
#73076=CARTESIAN_POINT ( 'NONE',  ( -1.292650918635170010, 0.2952755905511810774, -0.1292274648535930714 ) ) ;
#73078=CARTESIAN_POINT ( 'NONE',  ( 0.8202099737532813073, 0.2952755905511811885, 0.1292274648535926551 ) ) ;
#73080=CARTESIAN_POINT ( 'NONE',  ( -1.194225721784776262, -0.3690944881889763329, 0.3153832671262228327 ) ) ;
#73081=ORIENTED_EDGE ( 'NONE', *, *, #11466, .F. ) ;
#73085=CARTESIAN_POINT ( 'NONE',  ( -1.548556430446193399, 0.2306618581243848609, 0.2411417322834645549 ) ) ;
#73086=CARTESIAN_POINT ( 'NONE',  ( 1.574803149606299746, -0.1870078740157479769, 0.4822834645669291653 ) ) ;
#73089=LINE ( 'NONE', #40266, #4732 ) ;
#73091=FACE_OUTER_BOUND ( 'NONE', #77825, .T. ) ;
#73093=CARTESIAN_POINT ( 'NONE',  ( -0.3937007874015740483, -0.1870078740157479769, 0.3641732283464567677 ) ) ;
#73094=CARTESIAN_POINT ( 'NONE',  ( -0.9251968503937002541, 0.07958543189024085140, 0.2665933059059887866 ) ) ;
#73095=CARTESIAN_POINT ( 'NONE',  ( -1.095800524934382292, -0.3162353388693409650, -0.4822834645669289433 ) ) ;
#73096=CARTESIAN_POINT ( 'NONE',  ( 0.7611548556430451917, -0.6046776061558807314, 0.2411417322834647770 ) ) ;
#73097=CARTESIAN_POINT ( 'NONE',  ( -0.9055118110236215490, -0.6692913385826771977, 8.415575281601705876E-17 ) ) ;
#73100=CARTESIAN_POINT ( 'NONE',  ( -1.541994750656167090, -0.6692913385826773087, -0.1292274648535924053 ) ) ;
#73101=CARTESIAN_POINT ( 'NONE',  ( -1.574803149606298636, -0.1870078740157479769, 0.3641732283464567677 ) ) ;
#73108=CARTESIAN_POINT ( 'NONE',  ( -0.3018372703412066094, -0.4281496062992127816, -0.4176697321401328100 ) ) ;
#73109=CARTESIAN_POINT ( 'NONE',  ( 1.437007874015748810, -0.5400638737290845981, -0.3530559997133363437 ) ) ;
#73111=FACE_OUTER_BOUND ( 'NONE', #66454, .T. ) ;
#73113=CARTESIAN_POINT ( 'NONE',  ( -1.364829396325458521, 0.2306618581243847221, -0.2411417322834647770 ) ) ;
#73114=CARTESIAN_POINT ( 'NONE',  ( -0.7414698162729651543, 0.2952755905511810774, -0.1292274648535930714 ) ) ;
#73116=CARTESIAN_POINT ( 'NONE',  ( 0.5839895013123367340, -0.5511811023622048555, -0.09757992244046775898 ) ) ;
#73119=CARTESIAN_POINT ( 'NONE',  ( 0.4658792650918641698, -0.08942795157528024563, -0.3641732283464568787 ) ) ;
#73120=CARTESIAN_POINT ( 'NONE',  ( 0.7742782152230978099, -0.3690944881889763329, 0.3153832671262228327 ) ) ;
#73121=CARTESIAN_POINT ( 'NONE',  ( 1.089238845144357537, -0.4281496062992124485, 0.4176697321401328655 ) ) ;
#73123=CARTESIAN_POINT ( 'NONE',  ( -0.2034120734908128059, 0.1771653543307087630, 0.09757992244046791164 ) ) ;
#73125=CARTESIAN_POINT ( 'NONE',  ( -1.384514435695537005, -0.6692913385826773087, -0.1292274648535924053 ) ) ;
#73126=CARTESIAN_POINT ( 'NONE',  ( -0.08530183727034056085, -0.08942795157528024563, -0.3641732283464568787 ) ) ;
#73127=CARTESIAN_POINT ( 'NONE',  ( -1.194225721784776262, -0.3690944881889763329, 0.3153832671262228327 ) ) ;
#73129=CARTESIAN_POINT ( 'NONE',  ( -0.8005249343832011588, -0.004921259842519870586, -0.3153832671262229437 ) ) ;
#73130=CARTESIAN_POINT ( 'NONE',  ( -0.1509186351706028884, -0.3162353388693409650, -0.4822834645669289433 ) ) ;
#73133=CARTESIAN_POINT ( 'NONE',  ( 0.3412073490813655186, 0.1283753931104748280, 0.1820866141732283561 ) ) ;
#73134=CARTESIAN_POINT ( 'NONE',  ( -0.4396325459317579898, 0.1771653543307087630, 0.09757992244046791164 ) ) ;
#73135=CARTESIAN_POINT ( 'NONE',  ( -0.5183727034120726440, 0.2952755905511811885, 0.1292274648535926551 ) ) ;
#73136=CARTESIAN_POINT ( 'NONE',  ( -1.614173228346456268, -0.6692913385826771977, 8.415575281601705876E-17 ) ) ;
#73137=CARTESIAN_POINT ( 'NONE',  ( -1.082677165354329896, -0.4536011799217368745, -0.2665933059059886201 ) ) ;
#73139=ADVANCED_FACE ( 'NONE', ( #18511 ), #65339, .F. ) ;
#73140=CARTESIAN_POINT ( 'NONE',  ( 0.5971128608923891301, 0.2952755905511810774, -0.1292274648535930714 ) ) ;
#73142=FACE_OUTER_BOUND ( 'NONE', #26961, .T. ) ;
#73143=CARTESIAN_POINT ( 'NONE',  ( -0.2887139107611542133, 0.1283753931104748280, 0.1820866141732283561 ) ) ;
#73144=CARTESIAN_POINT ( 'NONE',  ( -0.1377952755905504645, 0.1660481256975885056, 0.3530559997133364547 ) ) ;
#73145=CARTESIAN_POINT ( 'NONE',  ( -1.646981627296586703, -0.05778040916215522460, 0.4822834645669289988 ) ) ;
#73146=CARTESIAN_POINT ( 'NONE',  ( -1.574803149606298192, -0.1870078740157480601, -0.3641732283464567677 ) ) ;
#73147=CARTESIAN_POINT ( 'NONE',  ( 1.227034120734908917, 0.2952755905511810774, -0.1292274648535930714 ) ) ;
#73148=CARTESIAN_POINT ( 'NONE',  ( -0.8530183727034112984, -0.3690944881889765550, -0.3153832671262227771 ) ) ;
#73149=CARTESIAN_POINT ( 'NONE',  ( -1.091663011964304042, -2.570477104772672414E-15, 0.4118477457933002461 ) ) ;
#73152=CARTESIAN_POINT ( 'NONE',  ( -1.614173228346457378, 0.2753471884572480932, 0.1372047244094471985 ) ) ;
#73153=CARTESIAN_POINT ( 'NONE',  ( 1.161417322834646271, 0.07958543189024071263, -0.2665933059059888421 ) ) ;
#73154=CARTESIAN_POINT ( 'NONE',  ( 0.7020997375328090762, -0.05778040916215560624, -0.4822834645669293319 ) ) ;
#73156=CARTESIAN_POINT ( 'NONE',  ( 1.227034120734908917, 0.1771653543307087075, -0.09757992244046823083 ) ) ;
#73157=EDGE_CURVE ( 'NONE', #55671, #3211, #47905, .T. ) ;
#73158=CARTESIAN_POINT ( 'NONE',  ( 0.07217847769028949700, -0.3162353388693405765, 0.4822834645669290543 ) ) ;
#73159=CARTESIAN_POINT ( 'NONE',  ( -0.6036745406824141069, -0.6046776061558809534, -0.2411417322834644161 ) ) ;
#73160=CARTESIAN_POINT ( 'NONE',  ( 1.515748031496063408, 0.1660481256975885056, 0.3530559997133364547 ) ) ;
#73163=CARTESIAN_POINT ( 'NONE',  ( 0.1771653543307093182, 0.07958543189024085140, 0.2665933059059887866 ) ) ;
#73164=VERTEX_POINT ( 'NONE', #15067 ) ;
#73167=CARTESIAN_POINT ( 'NONE',  ( -0.6036745406824141069, 0.2306618581243848609, 0.2411417322834645549 ) ) ;
#73168=CARTESIAN_POINT ( 'NONE',  ( 1.469816272965879911, 0.2306618581243847221, -0.2411417322834647770 ) ) ;
#73169=CARTESIAN_POINT ( 'NONE',  ( 0.4330708661417329575, 0.2952755905511811885, 0.000000000000000000 ) ) ;
#73170=CARTESIAN_POINT ( 'NONE',  ( -0.2887139107611542133, -0.5023911411419708095, -0.1820866141732282451 ) ) ;
#73172=CARTESIAN_POINT ( 'NONE',  ( 0.9514435695538062676, -0.3162353388693409650, -0.4822834645669289433 ) ) ;
#73173=CARTESIAN_POINT ( 'NONE',  ( -1.049868766404198794, -0.6046776061558807314, 0.2411417322834647770 ) ) ;
#73174=CARTESIAN_POINT ( 'NONE',  ( -0.2230971128608915943, -0.4281496062992127816, -0.4176697321401328100 ) ) ;
#73175=CARTESIAN_POINT ( 'NONE',  ( -0.9711286089238838626, -0.6046776061558807314, 0.2411417322834647770 ) ) ;
#73176=CARTESIAN_POINT ( 'NONE',  ( 1.089238845144357537, -0.4281496062992124485, 0.4176697321401328655 ) ) ;
#73177=CARTESIAN_POINT ( 'NONE',  ( 1.095800524934383846, -0.3162353388693405765, 0.4822834645669290543 ) ) ;
#73178=CARTESIAN_POINT ( 'NONE',  ( 0.8464566929133866546, -0.5400638737290844871, 0.3530559997133364547 ) ) ;
#73180=CARTESIAN_POINT ( 'NONE',  ( -0.09186351706036663400, -0.3690944881889763329, 0.3153832671262228327 ) ) ;
#73183=ORIENTED_EDGE ( 'NONE', *, *, #42934, .F. ) ;
#73184=CARTESIAN_POINT ( 'NONE',  ( -0.8530183727034112984, -0.3690944881889765550, -0.3153832671262227771 ) ) ;
#73185=CARTESIAN_POINT ( 'NONE',  ( 0.07874015748031558404, -0.1870078740157479769, 0.4822834645669291653 ) ) ;
#73187=CARTESIAN_POINT ( 'NONE',  ( -0.1115485564304456306, 0.2952755905511810774, -0.1292274648535930714 ) ) ;
#73188=CARTESIAN_POINT ( 'NONE',  ( -0.3346456692913377662, -0.5400638737290844871, 0.3530559997133364547 ) ) ;
#73189=CARTESIAN_POINT ( 'NONE',  ( -1.272965879265091305, 0.05413385826771626580, -0.4176697321401330321 ) ) ;
#73190=CARTESIAN_POINT ( 'NONE',  ( -1.364829396325458521, 0.2306618581243847221, -0.2411417322834647770 ) ) ;
#73192=CARTESIAN_POINT ( 'NONE',  ( 1.220472440944882608, 0.1771653543307087630, 0.000000000000000000 ) ) ;
#73195=CARTESIAN_POINT ( 'NONE',  ( 0.5249343832021003964, 0.1283753931104746893, -0.1820866141732285504 ) ) ;
#73196=CARTESIAN_POINT ( 'NONE',  ( 8.195543980992789655E-16, -0.1870078740157480879, -0.4822834645669291653 ) ) ;
#73197=CARTESIAN_POINT ( 'NONE',  ( 0.1574803149606306130, -0.1870078740157480879, -0.4822834645669291653 ) ) ;
#73198=ORIENTED_EDGE ( 'NONE', *, *, #21598, .T. ) ;
#73200=CARTESIAN_POINT ( 'NONE',  ( -0.5905511811023615998, 0.2952755905511811885, 0.000000000000000000 ) ) ;
#73204=CARTESIAN_POINT ( 'NONE',  ( -0.4527559055118102749, 0.1660481256975885056, 0.3530559997133364547 ) ) ;
#73207=CARTESIAN_POINT ( 'NONE',  ( -1.456692913385826182, 0.1771653543307087630, 0.000000000000000000 ) ) ;
#73208=CARTESIAN_POINT ( 'NONE',  ( 0.9842519685039375910, 0.2952755905511811885, 0.000000000000000000 ) ) ;
#73209=CARTESIAN_POINT ( 'NONE',  ( 0.7283464566929143125, 0.1660481256975885056, 0.3530559997133364547 ) ) ;
#73210=CARTESIAN_POINT ( 'NONE',  ( -0.3083989501312330295, -0.2845877964562161244, -0.3641732283464567121 ) ) ;
#73211=CARTESIAN_POINT ( 'NONE',  ( 0.2296587926509192634, -0.05778040916215560624, -0.4822834645669293319 ) ) ;
#73213=CARTESIAN_POINT ( 'NONE',  ( 0.09186351706036827158, -0.004921259842519576551, 0.3153832671262227771 ) ) ;
#73214=CARTESIAN_POINT ( 'NONE',  ( -0.5577427821522301654, -0.05778040916215560624, -0.4822834645669293319 ) ) ;
#73216=CARTESIAN_POINT ( 'NONE',  ( -1.620734908136482577, -0.6692913385826773087, -0.1292274648535924053 ) ) ;
#73217=CARTESIAN_POINT ( 'NONE',  ( 0.09842519685039434474, -0.4536011799217368745, -0.2665933059059886201 ) ) ;
#73218=CARTESIAN_POINT ( 'NONE',  ( 1.541994750656168645, 0.1771653543307087075, -0.09757992244046823083 ) ) ;
#73219=CARTESIAN_POINT ( 'NONE',  ( -1.187664041994750175, -0.05778040916215560624, -0.4822834645669293319 ) ) ;
#73220=CARTESIAN_POINT ( 'NONE',  ( -0.8858267716535425107, -0.4536011799217367080, 0.2665933059059888421 ) ) ;
#73222=CARTESIAN_POINT ( 'NONE',  ( -1.351706036745406347, 0.05413385826771626580, -0.4176697321401330321 ) ) ;
#73223=CARTESIAN_POINT ( 'NONE',  ( -0.7086614173228339419, -0.1870078740157479769, 0.4822834645669291653 ) ) ;
#73224=CARTESIAN_POINT ( 'NONE',  ( 0.02624671916010564918, -0.6046776061558809534, -0.2411417322834644161 ) ) ;
#73228=CARTESIAN_POINT ( 'NONE',  ( 0.3083989501312343062, -0.08942795157528024563, -0.3641732283464568787 ) ) ;
#73229=CARTESIAN_POINT ( 'NONE',  ( 1.141732283464567566, 0.2952755905511811885, 0.000000000000000000 ) ) ;
#73230=CARTESIAN_POINT ( 'NONE',  ( -1.174540682414697335, -0.2845877964562161244, -0.3641732283464567121 ) ) ;
#73231=CARTESIAN_POINT ( 'NONE',  ( 1.279527559055118724, -0.5400638737290845981, -0.3530559997133363437 ) ) ;
#73232=CARTESIAN_POINT ( 'NONE',  ( -1.391076115485563758, 0.1283753931104748280, 0.1820866141732283561 ) ) ;
#73233=CARTESIAN_POINT ( 'NONE',  ( -0.4461942257217840213, 0.2306618581243848609, 0.2411417322834645549 ) ) ;
#73234=CARTESIAN_POINT ( 'NONE',  ( 0.1246719160104994284, 0.1771653543307087075, -0.09757992244046823083 ) ) ;
#73236=CARTESIAN_POINT ( 'NONE',  ( 0.5380577427821529035, -0.004921259842519870586, -0.3153832671262229437 ) ) ;
#73237=PRODUCT_DEFINITION_FORMATION_WITH_SPECIFIED_SOURCE ( 'ANY', '', #3024, .NOT_KNOWN. ) ;
#73239=CARTESIAN_POINT ( 'NONE',  ( 0.07874015748031558404, -0.1870078740157479769, 0.4822834645669291653 ) ) ;
#73242=CARTESIAN_POINT ( 'NONE',  ( -0.8070866141732276899, -0.5400638737290844871, 0.3530559997133364547 ) ) ;
#73244=CARTESIAN_POINT ( 'NONE',  ( 1.108923884514436242, -0.08942795157527998196, 0.3641732283464567121 ) ) ;
#73245=CARTESIAN_POINT ( 'NONE',  ( 0.1377952755905518800, 0.1660481256975883668, -0.3530559997133364547 ) ) ;
#73246=CARTESIAN_POINT ( 'NONE',  ( -0.3412073490813641308, 0.2306618581243847221, -0.2411417322834647770 ) ) ;
#73247=CARTESIAN_POINT ( 'NONE',  ( -0.2493438320209966919, -0.3690944881889763329, 0.3153832671262228327 ) ) ;
#73248=CARTESIAN_POINT ( 'NONE',  ( 1.010849322905839287, 0.004960608223778500969, -0.3437734562760191848 ) ) ;
#73249=CARTESIAN_POINT ( 'NONE',  ( -0.2690288713910754526, -0.5511811023622046335, 0.09757992244046803654 ) ) ;
#73250=CARTESIAN_POINT ( 'NONE',  ( 0.3083989501312343062, -0.05778040916215560624, -0.4822834645669293319 ) ) ;
#73251=CARTESIAN_POINT ( 'NONE',  ( -0.8530183727034112984, -0.3690944881889765550, -0.3153832671262227771 ) ) ;
#73254=CARTESIAN_POINT ( 'NONE',  ( -1.082677165354329896, -0.5400638737290845981, -0.3530559997133363437 ) ) ;
#73255=CARTESIAN_POINT ( 'NONE',  ( 0.1702530392988864383, 0.004960608223778963273, 0.3437734562760189072 ) ) ;
#73257=CARTESIAN_POINT ( 'NONE',  ( -1.030183727034119867, -0.08942795157528024563, -0.3641732283464568787 ) ) ;
#73258=CARTESIAN_POINT ( 'NONE',  ( -0.5183727034120726440, -0.6692913385826773087, -0.1292274648535924053 ) ) ;
#73259=CARTESIAN_POINT ( 'NONE',  ( -1.561679790026246017, 0.05413385826771666132, 0.4176697321401328100 ) ) ;
#73260=CARTESIAN_POINT ( 'NONE',  ( -1.141732283464566011, 0.2952755905511811885, 0.000000000000000000 ) ) ;
#73262=ADVANCED_FACE ( 'NONE', ( #2847 ), #55946, .F. ) ;
#73263=CARTESIAN_POINT ( 'NONE',  ( 1.410761154855643795, -0.05778040916215560624, -0.4822834645669293319 ) ) ;
#73264=CARTESIAN_POINT ( 'NONE',  ( 0.8333333333333340365, -0.6692913385826771977, 0.1292274648535927661 ) ) ;
#73265=CARTESIAN_POINT ( 'NONE',  ( 1.568241469816273437, -0.3162353388693405765, 0.4822834645669290543 ) ) ;
#73267=EDGE_CURVE ( 'NONE', #58699, #8650, #67243, .T. ) ;
#73268=CARTESIAN_POINT ( 'NONE',  ( -1.725721784776902190, -0.05778040916215522460, 0.4822834645669289988 ) ) ;
#73271=CARTESIAN_POINT ( 'NONE',  ( -0.5052493438320203589, 0.1771653543307087075, -0.09757992244046823083 ) ) ;
#73273=EDGE_LOOP ( 'NONE', ( #46346, #60316, #36100, #17598 ) ) ;
#73274=CARTESIAN_POINT ( 'NONE',  ( 0.9973753280839902091, 0.2306618581243847221, -0.2411417322834647770 ) ) ;
#73276=CARTESIAN_POINT ( 'NONE',  ( 5.463695987328526437E-16, -0.1870078740157479769, 0.4822834645669291653 ) ) ;
#73277=CARTESIAN_POINT ( 'NONE',  ( -0.6889763779527552368, 0.1660481256975885056, 0.3530559997133364547 ) ) ;
#73278=CARTESIAN_POINT ( 'NONE',  ( 1.377952755905512472, 0.2952755905511811885, 0.000000000000000000 ) ) ;
#73279=CARTESIAN_POINT ( 'NONE',  ( -1.489501312335957062, -0.08942795157527998196, 0.3641732283464567121 ) ) ;
#73281=CARTESIAN_POINT ( 'NONE',  ( 0.5446194225721792126, -0.3162353388693405765, 0.4822834645669290543 ) ) ;
#73282=CARTESIAN_POINT ( 'NONE',  ( 0.6627296587926515548, 0.1771653543307087630, 0.09757992244046791164 ) ) ;
#73283=CARTESIAN_POINT ( 'NONE',  ( -0.6496062992125976043, 0.1660481256975883668, -0.3530559997133364547 ) ) ;
#73285=CARTESIAN_POINT ( 'NONE',  ( -1.299212598425196097, 0.2952755905511811885, 0.000000000000000000 ) ) ;
#73286=CARTESIAN_POINT ( 'NONE',  ( 8.318810292902001717E-17, 2.401574803149606474, 0.4915354330708643360 ) ) ;
#73287=CARTESIAN_POINT ( 'NONE',  ( 0.8595800524934390507, -0.3162353388693405765, 0.4822834645669290543 ) ) ;
#73288=CARTESIAN_POINT ( 'NONE',  ( 1.135170603674541256, -0.5511811023622048555, -0.09757992244046775898 ) ) ;
#73291=CARTESIAN_POINT ( 'NONE',  ( -0.5643044619422565855, -0.4281496062992124485, 0.4176697321401328655 ) ) ;
#73292=EDGE_LOOP ( 'NONE', ( #73836, #49247, #34786, #50805 ) ) ;
#73293=CARTESIAN_POINT ( 'NONE',  ( 0.2821522309711292364, -0.5511811023622046335, 0.09757992244046803654 ) ) ;
#73294=CARTESIAN_POINT ( 'NONE',  ( -1.089238845144356427, 0.05413385826771666132, 0.4176697321401328100 ) ) ;
#73295=CARTESIAN_POINT ( 'NONE',  ( 0.8267716535433077274, 0.2952755905511811885, 0.000000000000000000 ) ) ;
#73296=CARTESIAN_POINT ( 'NONE',  ( 0.9055118110236227702, -0.6692913385826771977, 8.415575281601705876E-17 ) ) ;
#73297=CARTESIAN_POINT ( 'NONE',  ( 0.02624671916010564918, 0.2306618581243848609, 0.2411417322834645549 ) ) ;
#73298=CARTESIAN_POINT ( 'NONE',  ( -0.5511811023622038563, -0.1870078740157479769, 0.4822834645669291653 ) ) ;
#73300=CARTESIAN_POINT ( 'NONE',  ( -1.587926509186350810, -0.4281496062992124485, 0.4176697321401328655 ) ) ;
#73301=CARTESIAN_POINT ( 'NONE',  ( -0.5118110236220466680, 0.2952755905511811885, 0.000000000000000000 ) ) ;
#73303=CARTESIAN_POINT ( 'NONE',  ( -0.4461942257217840213, -0.5023911411419708095, -0.1820866141732282451 ) ) ;
#73304=CARTESIAN_POINT ( 'NONE',  ( 1.213910761154856299, 0.2952755905511811885, 0.1292274648535926551 ) ) ;
#73305=CARTESIAN_POINT ( 'NONE',  ( 1.620734908136483465, -0.6692913385826771977, 0.1292274648535927661 ) ) ;
#73306=CARTESIAN_POINT ( 'NONE',  ( -0.8923884514435688198, 0.2306618581243847221, -0.2411417322834647770 ) ) ;
#73308=CARTESIAN_POINT ( 'NONE',  ( 0.6364829396325465405, -0.05778040916215522460, 0.4822834645669289988 ) ) ;
#73310=CARTESIAN_POINT ( 'NONE',  ( -0.6912002312465808096, 1.909921115055098095, -0.5309055118110235227 ) ) ;
#73311=CARTESIAN_POINT ( 'NONE',  ( -0.2296587926509179312, -0.05778040916215522460, 0.4822834645669289988 ) ) ;
#73313=CARTESIAN_POINT ( 'NONE',  ( -1.358267716535432434, -0.4536011799217367080, 0.2665933059059888421 ) ) ;
#73314=CARTESIAN_POINT ( 'NONE',  ( 0.9908136482939640111, -0.5511811023622046335, 0.09757992244046803654 ) ) ;
#73316=CARTESIAN_POINT ( 'NONE',  ( 1.253280839895013710, -0.08942795157528024563, -0.3641732283464568787 ) ) ;
#73317=CARTESIAN_POINT ( 'NONE',  ( 0.7677165354330716118, -0.5400638737290844871, 0.3530559997133364547 ) ) ;
#73318=AXIS2_PLACEMENT_3D ( 'NONE', #60019, #48216, #60845 ) ;
#73320=CARTESIAN_POINT ( 'NONE',  ( -0.4461942257217840213, 0.2306618581243848609, 0.2411417322834645549 ) ) ;
#73321=DIRECTION ( 'NONE',  ( -0.7071067811865489050, -0.000000000000000000, 0.7071067811865460184 ) ) ;
#73322=CARTESIAN_POINT ( 'NONE',  ( 1.443569553805774897, 0.1283753931104748280, 0.1820866141732283561 ) ) ;
#73323=CARTESIAN_POINT ( 'NONE',  ( -0.5118110236220466680, -0.6692913385826771977, 8.415575281601705876E-17 ) ) ;
#73325=CARTESIAN_POINT ( 'NONE',  ( 1.332020997375329197, -0.3162353388693405765, 0.4822834645669290543 ) ) ;
#73326=CARTESIAN_POINT ( 'NONE',  ( 0.02624671916010564918, 0.2306618581243848609, 0.2411417322834645549 ) ) ;
#73327=CARTESIAN_POINT ( 'NONE',  ( 0.6561679790026253567, -0.5023911411419708095, -0.1820866141732282451 ) ) ;
#73329=CARTESIAN_POINT ( 'NONE',  ( 0.3477690288713918276, -0.5511811023622048555, -0.09757992244046775898 ) ) ;
#73330=CARTESIAN_POINT ( 'NONE',  ( -1.069553805774277722, 0.2066929133858267931, 0.1054918080437490802 ) ) ;
#73333=CARTESIAN_POINT ( 'NONE',  ( 0.9580052493438327987, -0.4281496062992127816, -0.4176697321401328100 ) ) ;
#73335=CARTESIAN_POINT ( 'NONE',  ( 1.673228346456693494, 0.07958543189024085140, 0.2665933059059887866 ) ) ;
#73336=FACE_OUTER_BOUND ( 'NONE', #42005, .T. ) ;
#73337=CARTESIAN_POINT ( 'NONE',  ( -0.03937007874015669567, -0.5511811023622047445, 6.969142054262312111E-17 ) ) ;
#73339=CARTESIAN_POINT ( 'NONE',  ( 0.2034120734908144990, -0.6692913385826771977, 0.1292274648535927661 ) ) ;
#73340=CARTESIAN_POINT ( 'NONE',  ( 1.515748031496063408, 0.07958543189024085140, 0.2665933059059887866 ) ) ;
#73341=CARTESIAN_POINT ( 'NONE',  ( -1.535433070866141225, 0.1771653543307087630, 0.000000000000000000 ) ) ;
#73342=CARTESIAN_POINT ( 'NONE',  ( -1.332020997375327642, -0.3162353388693409650, -0.4822834645669289433 ) ) ;
#73343=CARTESIAN_POINT ( 'NONE',  ( 0.6364829396325465405, -0.3162353388693409650, -0.4822834645669289433 ) ) ;
#73344=CARTESIAN_POINT ( 'NONE',  ( 1.581364829396326277, -0.3162353388693409650, -0.4822834645669289433 ) ) ;
#73347=CARTESIAN_POINT ( 'NONE',  ( 0.7742782152230978099, -0.4281496062992124485, 0.4176697321401328655 ) ) ;
#73348=CARTESIAN_POINT ( 'NONE',  ( 1.167979002624672580, -0.4281496062992124485, 0.4176697321401328655 ) ) ;
#73349=CARTESIAN_POINT ( 'NONE',  ( 0.8464566929133866546, -0.5400638737290844871, 0.3530559997133364547 ) ) ;
#73350=CARTESIAN_POINT ( 'NONE',  ( -1.660104986876639543, -0.08942795157528024563, -0.3641732283464568787 ) ) ;
#73351=CARTESIAN_POINT ( 'NONE',  ( 1.108923884514436686, -0.2845877964562161244, -0.3641732283464567121 ) ) ;
#73352=CARTESIAN_POINT ( 'NONE',  ( 1.640419947506562393, -0.4281496062992124485, 0.4176697321401328655 ) ) ;
#73353=CARTESIAN_POINT ( 'NONE',  ( -0.7152230971128602510, -0.2845877964562159024, 0.3641732283464567677 ) ) ;
#73354=CARTESIAN_POINT ( 'NONE',  ( 0.4133858267716541968, -0.4536011799217368745, -0.2665933059059886201 ) ) ;
#73355=CARTESIAN_POINT ( 'NONE',  ( 0.006561679790026889343, -0.3162353388693409650, -0.4822834645669289433 ) ) ;
#73356=CARTESIAN_POINT ( 'NONE',  ( 0.7611548556430451917, -0.6046776061558807314, 0.2411417322834647770 ) ) ;
#73357=CARTESIAN_POINT ( 'NONE',  ( -0.1706036745406816491, 0.05413385826771626580, -0.4176697321401330321 ) ) ;
#73358=CARTESIAN_POINT ( 'NONE',  ( 0.2755905511811031494, -0.5511811023622047445, 6.969142054262312111E-17 ) ) ;
#73359=CARTESIAN_POINT ( 'NONE',  ( 1.318897637795276356, 0.1660481256975883668, -0.3530559997133364547 ) ) ;
#73361=CARTESIAN_POINT ( 'NONE',  ( -1.010498687664041384, -0.4281496062992127816, -0.4176697321401328100 ) ) ;
#73364=CARTESIAN_POINT ( 'NONE',  ( -0.7874015748031489847, -0.1870078740157480879, -0.4822834645669291653 ) ) ;
#73366=CARTESIAN_POINT ( 'NONE',  ( -0.5511811023622041894, -0.1870078740157480879, -0.4822834645669291653 ) ) ;
#73369=ORIENTED_EDGE ( 'NONE', *, *, #30564, .F. ) ;
#73370=CARTESIAN_POINT ( 'NONE',  ( 0.8070866141732289112, -0.4536011799217368745, -0.2665933059059886201 ) ) ;
#73372=CARTESIAN_POINT ( 'NONE',  ( 1.279527559055118724, 0.1660481256975885056, 0.3530559997133364547 ) ) ;
#73374=CARTESIAN_POINT ( 'NONE',  ( -1.404199475065615932, -0.004921259842519576551, 0.3153832671262227771 ) ) ;
#73375=CARTESIAN_POINT ( 'NONE',  ( 1.620734908136483465, -0.6692913385826771977, 0.1292274648535927661 ) ) ;
#73376=CARTESIAN_POINT ( 'NONE',  ( -1.437007874015747477, -0.5400638737290844871, 0.3530559997133364547 ) ) ;
#73378=CARTESIAN_POINT ( 'NONE',  ( -0.1443569553805765515, -0.4281496062992127816, -0.4176697321401328100 ) ) ;
#73379=CARTESIAN_POINT ( 'NONE',  ( -0.3018372703412066094, -0.004921259842519576551, 0.3153832671262227771 ) ) ;
#73380=CARTESIAN_POINT ( 'NONE',  ( 0.8530183727034126306, 0.05413385826771626580, -0.4176697321401330321 ) ) ;
#73381=CARTESIAN_POINT ( 'NONE',  ( -0.1837270341207343505, -0.6046776061558807314, 0.2411417322834647770 ) ) ;
#73382=CARTESIAN_POINT ( 'NONE',  ( 0.4840268112322921312, 0.02791078216816386681, 0.4328096321851896966 ) ) ;
#73383=CARTESIAN_POINT ( 'NONE',  ( 2.795275590551181910, 1.771653543307087242, 0.000000000000000000 ) ) ;
#73385=CARTESIAN_POINT ( 'NONE',  ( 0.7480314960629927956, 0.2952755905511811885, 0.000000000000000000 ) ) ;
#73386=CARTESIAN_POINT ( 'NONE',  ( 0.2230971128608929543, 0.05413385826771626580, -0.4176697321401330321 ) ) ;
#73387=CARTESIAN_POINT ( 'NONE',  ( -1.062992125984250968, -0.6692913385826771977, 8.415575281601705876E-17 ) ) ;
#73389=CARTESIAN_POINT ( 'NONE',  ( 1.036745406824147508, -0.4281496062992127816, -0.4176697321401328100 ) ) ;
#73390=CARTESIAN_POINT ( 'NONE',  ( 0.8398950131233602345, -0.6046776061558807314, 0.2411417322834647770 ) ) ;
#73392=CARTESIAN_POINT ( 'NONE',  ( -0.3937007874015740483, -0.1870078740157480879, -0.4822834645669291653 ) ) ;
#73393=CARTESIAN_POINT ( 'NONE',  ( 0.4593175853018380828, 0.05413385826771626580, -0.4176697321401330321 ) ) ;
#73394=CARTESIAN_POINT ( 'NONE',  ( 0.1115485564304470323, 0.2952755905511811885, 0.1292274648535926551 ) ) ;
#73396=CARTESIAN_POINT ( 'NONE',  ( 0.8005249343832028242, -0.3690944881889765550, -0.3153832671262227771 ) ) ;
#73397=CARTESIAN_POINT ( 'NONE',  ( -1.299212598425196097, -0.6692913385826771977, 8.415575281601705876E-17 ) ) ;
#73398=CARTESIAN_POINT ( 'NONE',  ( -1.627296587926508442, -0.6046776061558809534, -0.2411417322834644161 ) ) ;
#73399=CARTESIAN_POINT ( 'NONE',  ( 0.3412073490813655186, 0.2306618581243848609, 0.2411417322834645549 ) ) ;
#73404=CARTESIAN_POINT ( 'NONE',  ( 0.9776902887139113929, -0.6692913385826773087, -0.1292274648535924053 ) ) ;
#73405=CARTESIAN_POINT ( 'NONE',  ( 0.5905511811023629321, -0.5511811023622047445, 6.969142054262312111E-17 ) ) ;
#73409=CARTESIAN_POINT ( 'NONE',  ( -0.7767023820430439818, -3.623651218081290895E-15, 0.4118477457932994690 ) ) ;
#73410=B_SPLINE_CURVE_WITH_KNOTS ( 'NONE', 3,
 ( #48909, #55627, #48081, #81336 ),
 .UNSPECIFIED., .F., .F.,
 ( 4, 4 ),
 ( 0.000000000000000000, 0.001493228121701133636 ),
 .UNSPECIFIED. ) ;
#73415=CARTESIAN_POINT ( 'NONE',  ( -0.7349081364829387342, -0.6046776061558807314, 0.2411417322834647770 ) ) ;
#73416=CARTESIAN_POINT ( 'NONE',  ( -0.5971128608923877978, 0.2952755905511811885, 0.1292274648535926551 ) ) ;
#73417=CARTESIAN_POINT ( 'NONE',  ( 1.135170603674541256, 0.2952755905511811885, 0.1292274648535926551 ) ) ;
#73419=CARTESIAN_POINT ( 'NONE',  ( 1.240157480314961314, -0.5400638737290844871, 0.3530559997133364547 ) ) ;
#73420=CARTESIAN_POINT ( 'NONE',  ( -1.169606216052558434, -4.983732387537991731E-15, 0.3791483426435189874 ) ) ;
#73421=DIRECTION ( 'NONE',  ( 1.000000000000000000, -0.000000000000000000, -0.000000000000000000 ) ) ;
#73423=CARTESIAN_POINT ( 'NONE',  ( -1.522309711286088607, -0.5023911411419708095, 0.1820866141732285504 ) ) ;
#73424=CARTESIAN_POINT ( 'NONE',  ( 1.614173228346456712, 0.000000000000000000, 0.1372047244094478646 ) ) ;
#73425=CARTESIAN_POINT ( 'NONE',  ( 0.1049868766404206816, 0.2306618581243848609, 0.2411417322834645549 ) ) ;
#73427=CARTESIAN_POINT ( 'NONE',  ( 1.469816272965879911, -0.6046776061558807314, 0.2411417322834647770 ) ) ;
#73428=CARTESIAN_POINT ( 'NONE',  ( -1.102362204724408601, -0.1870078740157479769, 0.3641732283464567677 ) ) ;
#73429=CARTESIAN_POINT ( 'NONE',  ( 0.5971128608923891301, 0.2952755905511810774, -0.1292274648535930714 ) ) ;
#73430=CARTESIAN_POINT ( 'NONE',  ( 1.332020997375328974, -0.08942795157528024563, -0.3641732283464568787 ) ) ;
#73432=CARTESIAN_POINT ( 'NONE',  ( -0.9055118110236215490, 0.1771653543307087630, 0.000000000000000000 ) ) ;
#73433=CARTESIAN_POINT ( 'NONE',  ( 1.482939632545932307, -0.4281496062992124485, 0.4176697321401328655 ) ) ;
#73435=CARTESIAN_POINT ( 'NONE',  ( -0.09842519685039295696, 0.1660481256975883668, -0.3530559997133364547 ) ) ;
#73436=CARTESIAN_POINT ( 'NONE',  ( -1.476377952755905110, 0.07958543189024085140, 0.2665933059059887866 ) ) ;
#73437=CARTESIAN_POINT ( 'NONE',  ( -0.1574803149606292529, -0.1870078740157479769, 0.3641732283464567677 ) ) ;
#73438=CARTESIAN_POINT ( 'NONE',  ( -0.4593175853018366950, 0.05413385826771666132, 0.4176697321401328100 ) ) ;
#73439=CARTESIAN_POINT ( 'NONE',  ( 1.692913385826772421, 0.2952755905511811885, 0.000000000000000000 ) ) ;
#73441=CARTESIAN_POINT ( 'NONE',  ( 0.3871391076115492380, -0.05778040916215560624, -0.4822834645669293319 ) ) ;
#73443=( BOUNDED_SURFACE ( )  B_SPLINE_SURFACE ( 1, 2, ( 
 ( #79751, #35529, #48150, #9442, #27966, #73845, #16185, #14937, #34288, #79332, #61191, #21652, #3547, #3130, #59950, #35113, #2305, #8203, #47312, #53624, #73002, #41832, #47728, #15354, #59532, #29213, #54880, #9034, #33868, #1889, #28795, #41015, #2717, #46896, #73427, #27549, #53207, #78919, #21241, #72590, #66701, #34708, #40596, #66278, #60369, #67111, #28377, #54458, #54038, #80172, #22486, #43887, #5599, #48975, #17838, #50208, #36759, #37585, #24942, #56112, #4772, #81818, #76320, #30448, #10696, #24128, #82628, #67939, #50615, #56932, #36351, #75499, #42244, #10281, #49390, #61617, #62027, #11103, #31266, #35947, #82224, #11930, #49797, #3959, #43473, #68759, #55694, #29622, #55282, #80992, #23305, #69169, #4363, #75906, #11520, #37177, #23719, #74674, #17020, #62856, #30031, #42659, #63258, #75084, #56522, #68357, #5192, #81402, #17431, #43062, #62435, #30857, #24544, #18245, #69584, #27039, #37996, #39673, #6847, #52700, #548, #20317, #63672, #71665, #19903, #64931, #38831, #18650, #45551, #58179, #59031, #14016, #51439, #44294, #77569, #1386, #12340, #31684, #44704, #6013, #77142, #45127, #51864, #39248, #77988, #83039, #975, #57343, #13181, #65366, #26201, #71248, #58607, #13594, #25778, #7269, #7701, #32517, #32941, #69985, #57761, #51025, #25362, #64095, #76724, #70400, #123, #33368, #45970, #26629, #19056, #64510, #12756, #38414, #52283, #6431, #32102, #19475, #70833, #40094, #42457, #35743, #1795, #78410, #48359, #16404, #33779, #55495, #61411, #68157, #74474, #60998, #10501, #23520, #55083, #54677, #80792, #46390, #61828, #21154, #36155, #4168, #16821, #72085, #27457, #74058, #14849, #3346, #23109, #80388, #14442, #40509, #81205, #65781, #8113, #59442, #42050, #46809, #29832, #67746, #22700, #9665, #53116, #20739, #78827, #10080, #35334, #72500, #48775, #67332, #3760, #29011, #29425, #59711, #72362, #40773, #27312, #28146, #15535, #46668, #78685, #14710, #66883, #21008, #1247, #40365, #73185, #58464, #41195, #47493, #26896, #66045, #32795, #65215, #827, #53802, #65642, #26486, #8383, #52137, #77844, #45823, #58888, #20173, #7972, #59298, #34048, #53397, #8794, #13868, #15119, #71522, #52971, #79515, #2066, #27732, #72768, #79104, #39956, #21423, #2487, #47077, #66458, #39527, #71943, #7554, #33225, #78264, #52555, #20595, #14295, #46247, #34470, #60136, #21830, #33635, #1655, #75257, #16779, #47907, #68117, #74017, #55867, #79934, #36522, #36116, #9623, #34886, #23067, #48735, #73612, #49563, #10462, #10862, #17195, #67703, #62198, #17601, #55454, #3722, #81163, #60547, #30205, #3306, #4535, #81580, #42828, #2898, #67290, #74432, #80348, #10039, #23479, #29386, #28562, #54218, #61788, #35703, #4128, #43233, #22249, #15954, #35294, #41600, #61372, #55046, #42417, #29793, #68521, #60956, #74853, #28971, #80753, #23897, #49146, #9213, #54638, #22661, #16364, #48320, #42009, #57102, #70157, #77316, #24712, #18010, #19646, #31027, #24302, #37355, #50380, #297, #70575, #12510, #6601, #63434, #68930, #51611, #76492, #49972, #44466, #76078, #32273, #56291, #12929, #38171, #69347, #11279, #82797, #25121, #75670, #25953, #63845, #38589, #76896, #44063, #64267, #36938, #31861, #5770, #57520, #62616, #57933, #63028, #4958, #30626, #19226, #81988, #43644, #50791, #56695, #69755, #83211, #31439, #11701, #5366, #6183, #12101, #82394, #18422, #37759, #18819, #25533, #51198, #44876, #53292, #59197, #7870, #26794, #718, #79413, #27210, #39424, #7021, #66360, #52451, #59612, #71420, #26376, #33948, #8282, #15019, #58786, #65108, #40675, #20071, #45307, #53704, #64682, #8698, #33534, #71002, #52873, #46976, #32689, #34369, #46562, #1967, #78583, #2390, #27630, #77740, #28046, #60034, #78161, #13345, #38999, #58356, #52036, #1556, #45723, #20909, #72670, #13767, #7446, #72261, #79004, #14609, #33116, #21323, #1144, #20492, #46146, #71841, #14191, #40263, #39848, #65539, #65946, #48950, #66785, #81377, #49364, #56088, #43447, #82199, #3937, #5168, #9120, #17408, #43856, #4747, #81793, #62834, #30420, #30004, #17814, #75880, #11076, #24104, #31241 ),
 ( #49773, #30832, #56907, #18221, #69559, #63235, #73086, #68332, #36327, #36733, #24517, #56497, #75473, #10671, #50183, #11907, #55257, #74651, #62002, #37561, #4338, #5575, #69145, #16992, #11495, #42635, #21732, #55668, #23690, #75060, #47395, #62408, #43038, #15436, #41097, #35924, #68734, #61591, #29596, #37149, #80966, #23280, #63647, #38805, #32915, #33344, #44269, #18626, #12314, #19029, #25334, #26604, #20292, #44677, #521, #96, #26174, #5986, #64904, #31657, #70372, #7241, #51836, #64481, #58581, #77114, #77962, #65337, #39646, #13565, #57315, #7672, #45940, #32073, #82603, #58152, #24921, #76296, #37972, #50997, #69960, #57733, #25749, #32489, #19875, #947, #83012, #52256, #76695, #19447, #71638, #6819, #77540, #39219, #45524, #6403, #71222, #13990, #70801, #50588, #12727, #38386, #64063, #51412, #45098, #13154, #27428, #40485, #73732, #60666, #2604, #80052, #53513, #59006, #41715, #66578, #14416, #34589, #66163, #22371, #46365, #3014, #28262, #59414, #1361, #72888, #15237, #40069, #16069, #60256, #28681, #66998, #34169, #54342, #67407, #21954, #79221, #47612, #27013, #48030, #53089, #9742, #52675, #9330, #78382, #33753, #40897, #46785, #59832, #73308, #21537, #20713, #72058, #53924, #2185, #72476, #65756, #8089, #1771, #78801, #47197, #21126, #35000, #8913, #79636, #8503, #14825, #27853, #15656, #41315, #80467, #56405, #42540, #49679, #61495, #74139, #24011, #81700, #5073, #48855, #29503, #30742, #10163, #69463, #43757, #54761, #82104, #23596, #35413, #17315, #37053, #22778, #24417, #36637, #75371, #68638, #55163, #62313, #36234, #4650, #16483, #17717, #42130, #80873, #43345, #30321, #74969, #69047, #29908, #50087, #18125, #49267, #81280, #42943, #61078, #10977, #3843, #55989, #75783, #3428, #29091, #48439, #23185, #67825, #4246, #11396, #61904, #35829, #74556, #55572, #16901, #68242, #62736, #10577, #25652, #64383, #76603, #63964, #32812, #69869, #70275, #843, #76195, #19770, #39119, #37468, #7139, #51733, #418, #3359, #70698, #77859, #18533, #31977, #26501, #50903, #18934, #51314, #20188, #52153, #13462, #44582, #77435, #6301, #32389, #50492, #77017, #44999, #19349, #45423, #63141, #13051, #71119, #45839, #64800, #58479, #11813, #5482, #57216, #25238, #38704, #31142, #56809, #6719, #82918, #82508, #24824, #44176, #37878, #12629, #12221, #38288, #63552, #58052, #5886, #26074, #31559, #57637, #52988, #59315, #27328, #21848, #27749, #78701, #65233, #9231, #66901, #14727, #47512, #79534, #8811, #46685, #8399, #52572, #53413, #73204, #22268, #33242, #7570, #1264, #7988, #14312, #15554, #34904, #2918, #39972, #58904, #40380, #40791, #66063, #26912, #65659, #34066, #60567, #79955, #28164, #41213, #2084, #66476, #21024, #59729, #28581, #46264, #72378, #54238, #78280, #71537, #13885, #39544, #20612, #53820, #60153, #79122, #47095, #71959, #33652, #21439, #1671, #72785, #15135, #34487, #2505, #62636, #49582, #3741, #4556, #16799, #68541, #3326, #36134, #81183, #61807, #81600, #15973, #49166, #30226, #82008, #17621, #68950, #4980, #41620, #10059, #61392, #4147, #75278, #55889, #74872, #35722, #23917, #43253, #80367, #74036, #29405, #11300, #55064, #36959, #42848, #16383, #17215, #42029, #47926, #80772, #23087, #48754, #30646, #29812, #74453, #67309, #56311, #73631, #42436, #9644, #35313, #10881, #68136, #10481, #28990, #55473, #60975, #54656, #22680, #48339, #67723, #23500, #36542, #62218, #45326, #44084, #25552, #25141, #51219, #5386, #6620, #31047, #69778, #32291, #76916, #63865, #57951, #18840, #19664, #7042, #38190, #70177, #6202, #58377, #12529, #76098, #31880, #64702, #49993, #32711, #56717, #50401, #37780, #51631, #63456, #25972, #19245, #18442, #44896, #12122, #24323, #5791, #31461, #57123, #319, #57540, #82817, #18031, #71021, #13365, #50810, #77335, #39018, #70595, #76511, #44485, #82414, #83231, #75690, #43665, #69367, #11721, #37377, #12949, #38607, #63047, #24733, #64285, #1985, #1576, #27648, #65131, #66377, #7466, #20512, #8714, #53310, #40282, #34385, #78603, #79429, #66801, #14627, #46582, #65964, #34807, #72280, #52473, #8300 ) ),
 .UNSPECIFIED., .F., .F., .F. ) 
 B_SPLINE_SURFACE_WITH_KNOTS ( ( 2, 2 ),
 ( 3, 2, 2, 2, 2, 2, 2, 2, 2, 2, 2, 2, 2, 2, 2, 2, 2, 2, 2, 2, 2, 2, 2, 2, 2, 2, 2, 2, 2, 2, 2, 2, 2, 2, 2, 2, 2, 2, 2, 2, 2, 2, 2, 2, 2, 2, 2, 2, 2, 2, 2, 2, 2, 2, 2, 2, 2, 2, 2, 2, 2, 2, 2, 2, 2, 2, 2, 2, 2, 2, 2, 2, 2, 2, 2, 2, 2, 2, 2, 2, 2, 2, 2, 2, 2, 2, 2, 2, 2, 2, 2, 2, 2, 2, 2, 2, 2, 2, 2, 2, 2, 2, 2, 2, 2, 2, 2, 2, 2, 2, 2, 2, 2, 2, 2, 2, 2, 2, 2, 2, 2, 2, 2, 2, 2, 2, 2, 2, 2, 2, 2, 2, 2, 2, 2, 2, 2, 2, 2, 2, 2, 2, 2, 2, 2, 2, 2, 2, 2, 2, 2, 2, 2, 2, 2, 2, 2, 2, 2, 2, 2, 2, 2, 2, 2, 2, 2, 2, 2, 2, 2, 2, 2, 2, 2, 2, 2, 2, 2, 2, 2, 2, 2, 2, 2, 2, 2, 2, 2, 2, 2, 2, 2, 2, 2, 2, 2, 2, 2, 2, 2, 2, 2, 2, 2, 2, 2, 2, 2, 2, 2, 2, 2, 2, 2, 2, 2, 2, 2, 2, 2, 2, 2, 2, 2, 2, 2, 2, 2, 2, 2, 2, 2, 2, 2, 2, 2, 2, 2, 2, 2, 2, 2, 2, 2, 2, 2, 2, 2, 2, 2, 2, 2, 2, 2, 3 ),
 ( 0.000000000000000000, 1.000000000000000000 ),
 ( 0.000000000000000000, 0.003787878787878787984, 0.007575757575757575968, 0.01136363636363636395, 0.01515151515151515194, 0.01893939393939393992, 0.02272727272727272790, 0.02651515151515151589, 0.03030303030303030387, 0.03409090909090908839, 0.03787878787878787984, 0.04166666666666666435, 0.04545454545454545581, 0.04924242424242424032, 0.05303030303030303177, 0.05681818181818181629, 0.06060606060606060774, 0.06439393939393939226, 0.06818181818181817677, 0.07196969696969697516, 0.07575757575757575968, 0.07954545454545454419, 0.08333333333333332871, 0.08712121212121212710, 0.09090909090909091161, 0.09469696969696969613, 0.09848484848484848064, 0.1022727272727272790, 0.1060606060606060635, 0.1098484848484848481, 0.1136363636363636326, 0.1174242424242424310, 0.1212121212121212155, 0.1250000000000000000, 0.1287878787878787845, 0.1325757575757575690, 0.1363636363636363535, 0.1401515151515151381, 0.1439393939393939503, 0.1477272727272727348, 0.1515151515151515194, 0.1553030303030303039, 0.1590909090909090884, 0.1628787878787878729, 0.1666666666666666574, 0.1704545454545454419, 0.1742424242424242542, 0.1780303030303030387, 0.1818181818181818232, 0.1856060606060606077, 0.1893939393939393923, 0.1931818181818181768, 0.1969696969696969613, 0.2007575757575757458, 0.2045454545454545581, 0.2083333333333333426, 0.2121212121212121271, 0.2159090909090909116, 0.2196969696969696961, 0.2234848484848484806, 0.2272727272727272652, 0.2310606060606060497, 0.2348484848484848619, 0.2386363636363636465, 0.2424242424242424310, 0.2462121212121212155, 0.2500000000000000000, 0.2537878787878787845, 0.2575757575757575690, 0.2613636363636363535, 0.2651515151515151381, 0.2689393939393939226, 0.2727272727272727071, 0.2765151515151514916, 0.2803030303030302761, 0.2840909090909091161, 0.2878787878787879007, 0.2916666666666666852, 0.2954545454545454697, 0.2992424242424242542, 0.3030303030303030387, 0.3068181818181818232, 0.3106060606060606077, 0.3143939393939393923, 0.3181818181818181768, 0.3219696969696969613, 0.3257575757575757458, 0.3295454545454545303, 0.3333333333333333148, 0.3371212121212120993, 0.3409090909090908839, 0.3446969696969697239, 0.3484848484848485084, 0.3522727272727272929, 0.3560606060606060774, 0.3598484848484848619, 0.3636363636363636465, 0.3674242424242424310, 0.3712121212121212155, 0.3750000000000000000, 0.3787878787878787845, 0.3825757575757575690, 0.3863636363636363535, 0.3901515151515151381, 0.3939393939393939226, 0.3977272727272727071, 0.4015151515151514916, 0.4053030303030302761, 0.4090909090909091161, 0.4128787878787879007, 0.4166666666666666852, 0.4204545454545454697, 0.4242424242424242542, 0.4280303030303030387, 0.4318181818181818232, 0.4356060606060606077, 0.4393939393939393923, 0.4431818181818181768, 0.4469696969696969613, 0.4507575757575757458, 0.4545454545454545303, 0.4583333333333333148, 0.4621212121212120993, 0.4659090909090908839, 0.4696969696969697239, 0.4734848484848485084, 0.4772727272727272929, 0.4810606060606060774, 0.4848484848484848619, 0.4886363636363636465, 0.4924242424242424310, 0.4962121212121212155, 0.5000000000000000000, 0.5037878787878787845, 0.5075757575757575690, 0.5113636363636363535, 0.5151515151515151381, 0.5189393939393939226, 0.5227272727272727071, 0.5265151515151514916, 0.5303030303030302761, 0.5340909090909090606, 0.5378787878787878451, 0.5416666666666666297, 0.5454545454545454142, 0.5492424242424241987, 0.5530303030303029832, 0.5568181818181817677, 0.5606060606060605522, 0.5643939393939394478, 0.5681818181818182323, 0.5719696969696970168, 0.5757575757575758013, 0.5795454545454545858, 0.5833333333333333703, 0.5871212121212121549, 0.5909090909090909394, 0.5946969696969697239, 0.5984848484848485084, 0.6022727272727272929, 0.6060606060606060774, 0.6098484848484848619, 0.6136363636363636465, 0.6174242424242424310, 0.6212121212121212155, 0.6250000000000000000, 0.6287878787878787845, 0.6325757575757575690, 0.6363636363636363535, 0.6401515151515151381, 0.6439393939393939226, 0.6477272727272727071, 0.6515151515151514916, 0.6553030303030302761, 0.6590909090909090606, 0.6628787878787878451, 0.6666666666666666297, 0.6704545454545454142, 0.6742424242424241987, 0.6780303030303029832, 0.6818181818181817677, 0.6856060606060605522, 0.6893939393939394478, 0.6931818181818182323, 0.6969696969696970168, 0.7007575757575758013, 0.7045454545454545858, 0.7083333333333333703, 0.7121212121212121549, 0.7159090909090909394, 0.7196969696969697239, 0.7234848484848485084, 0.7272727272727272929, 0.7310606060606060774, 0.7348484848484848619, 0.7386363636363636465, 0.7424242424242424310, 0.7462121212121212155, 0.7500000000000000000, 0.7537878787878787845, 0.7575757575757575690, 0.7613636363636363535, 0.7651515151515151381, 0.7689393939393939226, 0.7727272727272727071, 0.7765151515151514916, 0.7803030303030302761, 0.7840909090909090606, 0.7878787878787878451, 0.7916666666666666297, 0.7954545454545454142, 0.7992424242424241987, 0.8030303030303029832, 0.8068181818181817677, 0.8106060606060605522, 0.8143939393939394478, 0.8181818181818182323, 0.8219696969696970168, 0.8257575757575758013, 0.8295454545454545858, 0.8333333333333333703, 0.8371212121212121549, 0.8409090909090909394, 0.8446969696969697239, 0.8484848484848485084, 0.8522727272727272929, 0.8560606060606060774, 0.8598484848484848619, 0.8636363636363636465, 0.8674242424242424310, 0.8712121212121212155, 0.8750000000000000000, 0.8787878787878787845, 0.8825757575757575690, 0.8863636363636363535, 0.8901515151515151381, 0.8939393939393939226, 0.8977272727272727071, 0.9015151515151514916, 0.9053030303030302761, 0.9090909090909090606, 0.9128787878787878451, 0.9166666666666666297, 0.9204545454545454142, 0.9242424242424241987, 0.9280303030303029832, 0.9318181818181817677, 0.9356060606060605522, 0.9393939393939394478, 0.9431818181818182323, 0.9469696969696970168, 0.9507575757575758013, 0.9545454545454545858, 0.9583333333333333703, 0.9621212121212121549, 0.9659090909090909394 ),
 .UNSPECIFIED. ) 
 GEOMETRIC_REPRESENTATION_ITEM ( )  RATIONAL_B_SPLINE_SURFACE ( (
 ( 1.000000000000000000, 0.9659258262890683122, 1.000000000000000000, 0.9659258262890683122, 1.000000000000000000, 0.9659258262890683122, 1.000000000000000000, 0.9659258262890683122, 1.000000000000000000, 0.9659258262890683122, 1.000000000000000000, 0.9659258262890683122, 1.000000000000000000, 0.9659258262890683122, 1.000000000000000000, 0.9659258262890683122, 1.000000000000000000, 0.9659258262890683122, 1.000000000000000000, 0.9659258262890683122, 1.000000000000000000, 0.9659258262890683122, 1.000000000000000000, 0.9659258262890683122, 1.000000000000000000, 0.9659258262890683122, 1.000000000000000000, 0.9659258262890683122, 1.000000000000000000, 0.9659258262890683122, 1.000000000000000000, 0.9659258262890683122, 1.000000000000000000, 0.9659258262890683122, 1.000000000000000000, 0.9659258262890683122, 1.000000000000000000, 0.9659258262890683122, 1.000000000000000000, 0.9659258262890683122, 1.000000000000000000, 0.9659258262890683122, 1.000000000000000000, 0.9659258262890683122, 1.000000000000000000, 0.9659258262890683122, 1.000000000000000000, 0.9659258262890683122, 1.000000000000000000, 0.9659258262890683122, 1.000000000000000000, 0.9659258262890683122, 1.000000000000000000, 0.9659258262890683122, 1.000000000000000000, 0.9659258262890683122, 1.000000000000000000, 0.9659258262890683122, 1.000000000000000000, 0.9659258262890683122, 1.000000000000000000, 0.9659258262890683122, 1.000000000000000000, 0.9659258262890683122, 1.000000000000000000, 0.9659258262890683122, 1.000000000000000000, 0.9659258262890683122, 1.000000000000000000, 0.9659258262890683122, 1.000000000000000000, 0.9659258262890683122, 1.000000000000000000, 0.9659258262890683122, 1.000000000000000000, 0.9659258262890683122, 1.000000000000000000, 0.9659258262890683122, 1.000000000000000000, 0.9659258262890683122, 1.000000000000000000, 0.9659258262890683122, 1.000000000000000000, 0.9659258262890683122, 1.000000000000000000, 0.9659258262890683122, 1.000000000000000000, 0.9659258262890683122, 1.000000000000000000, 0.9659258262890683122, 1.000000000000000000, 0.9659258262890683122, 1.000000000000000000, 0.9659258262890683122, 1.000000000000000000, 0.9659258262890683122, 1.000000000000000000, 0.9659258262890683122, 1.000000000000000000, 0.9659258262890683122, 1.000000000000000000, 0.9659258262890683122, 1.000000000000000000, 0.9659258262890683122, 1.000000000000000000, 0.9659258262890683122, 1.000000000000000000, 0.9659258262890683122, 1.000000000000000000, 0.9659258262890683122, 1.000000000000000000, 0.9659258262890683122, 1.000000000000000000, 0.9659258262890683122, 1.000000000000000000, 0.9659258262890683122, 1.000000000000000000, 0.9659258262890683122, 1.000000000000000000, 0.9659258262890683122, 1.000000000000000000, 0.9659258262890683122, 1.000000000000000000, 0.9659258262890683122, 1.000000000000000000, 0.9659258262890683122, 1.000000000000000000, 0.9659258262890683122, 1.000000000000000000, 0.9659258262890683122, 1.000000000000000000, 0.9659258262890683122, 1.000000000000000000, 0.9659258262890683122, 1.000000000000000000, 0.9659258262890683122, 1.000000000000000000, 0.9659258262890683122, 1.000000000000000000, 0.9659258262890683122, 1.000000000000000000, 0.9659258262890683122, 1.000000000000000000, 0.9659258262890683122, 1.000000000000000000, 0.9659258262890683122, 1.000000000000000000, 0.9659258262890683122, 1.000000000000000000, 0.9659258262890683122, 1.000000000000000000, 0.9659258262890683122, 1.000000000000000000, 0.9659258262890683122, 1.000000000000000000, 0.9659258262890683122, 1.000000000000000000, 0.9659258262890683122, 1.000000000000000000, 0.9659258262890683122, 1.000000000000000000, 0.9659258262890683122, 1.000000000000000000, 0.9659258262890683122, 1.000000000000000000, 0.9659258262890683122, 1.000000000000000000, 0.9659258262890683122, 1.000000000000000000, 0.9659258262890683122, 1.000000000000000000, 0.9659258262890683122, 1.000000000000000000, 0.9659258262890683122, 1.000000000000000000, 0.9659258262890683122, 1.000000000000000000, 0.9659258262890683122, 1.000000000000000000, 0.9659258262890683122, 1.000000000000000000, 0.9659258262890683122, 1.000000000000000000, 0.9659258262890683122, 1.000000000000000000, 0.9659258262890683122, 1.000000000000000000, 0.9659258262890683122, 1.000000000000000000, 0.9659258262890683122, 1.000000000000000000, 0.9659258262890683122, 1.000000000000000000, 0.9659258262890683122, 1.000000000000000000, 0.9659258262890683122, 1.000000000000000000, 0.9659258262890683122, 1.000000000000000000, 0.9659258262890683122, 1.000000000000000000, 0.9659258262890683122, 1.000000000000000000, 0.9659258262890683122, 1.000000000000000000, 0.9659258262890683122, 1.000000000000000000, 0.9659258262890683122, 1.000000000000000000, 0.9659258262890683122, 1.000000000000000000, 0.9659258262890683122, 1.000000000000000000, 0.9659258262890683122, 1.000000000000000000, 0.9659258262890683122, 1.000000000000000000, 0.9659258262890683122, 1.000000000000000000, 0.9659258262890683122, 1.000000000000000000, 0.9659258262890683122, 1.000000000000000000, 0.9659258262890683122, 1.000000000000000000, 0.9659258262890683122, 1.000000000000000000, 0.9659258262890683122, 1.000000000000000000, 0.9659258262890683122, 1.000000000000000000, 0.9659258262890683122, 1.000000000000000000, 0.9659258262890683122, 1.000000000000000000, 0.9659258262890683122, 1.000000000000000000, 0.9659258262890683122, 1.000000000000000000, 0.9659258262890683122, 1.000000000000000000, 0.9659258262890683122, 1.000000000000000000, 0.9659258262890683122, 1.000000000000000000, 0.9659258262890683122, 1.000000000000000000, 0.9659258262890683122, 1.000000000000000000, 0.9659258262890683122, 1.000000000000000000, 0.9659258262890683122, 1.000000000000000000, 0.9659258262890683122, 1.000000000000000000, 0.9659258262890683122, 1.000000000000000000, 0.9659258262890683122, 1.000000000000000000, 0.9659258262890683122, 1.000000000000000000, 0.9659258262890683122, 1.000000000000000000, 0.9659258262890683122, 1.000000000000000000, 0.9659258262890683122, 1.000000000000000000, 0.9659258262890683122, 1.000000000000000000, 0.9659258262890683122, 1.000000000000000000, 0.9659258262890683122, 1.000000000000000000, 0.9659258262890683122, 1.000000000000000000, 0.9659258262890683122, 1.000000000000000000, 0.9659258262890683122, 1.000000000000000000, 0.9659258262890683122, 1.000000000000000000, 0.9659258262890683122, 1.000000000000000000, 0.9659258262890683122, 1.000000000000000000, 0.9659258262890683122, 1.000000000000000000, 0.9659258262890683122, 1.000000000000000000, 0.9659258262890683122, 1.000000000000000000, 0.9659258262890683122, 1.000000000000000000, 0.9659258262890683122, 1.000000000000000000, 0.9659258262890683122, 1.000000000000000000, 0.9659258262890683122, 1.000000000000000000, 0.9659258262890683122, 1.000000000000000000, 0.9659258262890683122, 1.000000000000000000, 0.9659258262890683122, 1.000000000000000000, 0.9659258262890683122, 1.000000000000000000, 0.9659258262890683122, 1.000000000000000000, 0.9659258262890683122, 1.000000000000000000, 0.9659258262890683122, 1.000000000000000000, 0.9659258262890683122, 1.000000000000000000, 0.9659258262890683122, 1.000000000000000000, 0.9659258262890683122, 1.000000000000000000, 0.9659258262890683122, 1.000000000000000000, 0.9659258262890683122, 1.000000000000000000, 0.9659258262890683122, 1.000000000000000000, 0.9659258262890683122, 1.000000000000000000, 0.9659258262890683122, 1.000000000000000000, 0.9659258262890683122, 1.000000000000000000, 0.9659258262890683122, 1.000000000000000000, 0.9659258262890683122, 1.000000000000000000, 0.9659258262890683122, 1.000000000000000000, 0.9659258262890683122, 1.000000000000000000, 0.9659258262890683122, 1.000000000000000000, 0.9659258262890683122, 1.000000000000000000, 0.9659258262890683122, 1.000000000000000000, 0.9659258262890683122, 1.000000000000000000, 0.9659258262890683122, 1.000000000000000000, 0.9659258262890683122, 1.000000000000000000, 0.9659258262890683122, 1.000000000000000000, 0.9659258262890683122, 1.000000000000000000, 0.9659258262890683122, 1.000000000000000000, 0.9659258262890683122, 1.000000000000000000, 0.9659258262890683122, 1.000000000000000000, 0.9659258262890683122, 1.000000000000000000, 0.9659258262890683122, 1.000000000000000000, 0.9659258262890683122, 1.000000000000000000, 0.9659258262890683122, 1.000000000000000000, 0.9659258262890683122, 1.000000000000000000, 0.9659258262890683122, 1.000000000000000000, 0.9659258262890683122, 1.000000000000000000, 0.9659258262890683122, 1.000000000000000000, 0.9659258262890683122, 1.000000000000000000, 0.9659258262890683122, 1.000000000000000000, 0.9659258262890683122, 1.000000000000000000, 0.9659258262890683122, 1.000000000000000000, 0.9659258262890683122, 1.000000000000000000, 0.9659258262890683122, 1.000000000000000000, 0.9659258262890683122, 1.000000000000000000, 0.9659258262890683122, 1.000000000000000000, 0.9659258262890683122, 1.000000000000000000, 0.9659258262890683122, 1.000000000000000000, 0.9659258262890683122, 1.000000000000000000, 0.9659258262890683122, 1.000000000000000000, 0.9659258262890683122, 1.000000000000000000, 0.9659258262890683122, 1.000000000000000000, 0.9659258262890683122, 1.000000000000000000, 0.9659258262890683122, 1.000000000000000000, 0.9659258262890683122, 1.000000000000000000, 0.9659258262890683122, 1.000000000000000000, 0.9659258262890683122, 1.000000000000000000, 0.9659258262890683122, 1.000000000000000000, 0.9659258262890683122, 1.000000000000000000, 0.9659258262890683122, 1.000000000000000000, 0.9659258262890683122, 1.000000000000000000, 0.9659258262890683122, 1.000000000000000000, 0.9659258262890683122, 1.000000000000000000, 0.9659258262890683122, 1.000000000000000000, 0.9659258262890683122, 1.000000000000000000, 0.9659258262890683122, 1.000000000000000000, 0.9659258262890683122, 1.000000000000000000, 0.9659258262890683122, 1.000000000000000000, 0.9659258262890683122, 1.000000000000000000, 0.9659258262890683122, 1.000000000000000000, 0.9659258262890683122, 1.000000000000000000, 0.9659258262890683122, 1.000000000000000000, 0.9659258262890683122, 1.000000000000000000, 0.9659258262890683122, 1.000000000000000000, 0.9659258262890683122, 1.000000000000000000, 0.9659258262890683122, 1.000000000000000000, 0.9659258262890683122, 1.000000000000000000, 0.9659258262890683122, 1.000000000000000000, 0.9659258262890683122, 1.000000000000000000, 0.9659258262890683122, 1.000000000000000000, 0.9659258262890683122, 1.000000000000000000, 0.9659258262890683122, 1.000000000000000000, 0.9659258262890683122, 1.000000000000000000, 0.9659258262890683122, 1.000000000000000000, 0.9659258262890683122, 1.000000000000000000, 0.9659258262890683122, 1.000000000000000000, 0.9659258262890683122, 1.000000000000000000, 0.9659258262890683122, 1.000000000000000000, 0.9659258262890683122, 1.000000000000000000, 0.9659258262890683122, 1.000000000000000000, 0.9659258262890683122, 1.000000000000000000, 0.9659258262890683122, 1.000000000000000000, 0.9659258262890683122, 1.000000000000000000, 0.9659258262890683122, 1.000000000000000000, 0.9659258262890683122, 1.000000000000000000, 0.9659258262890683122, 1.000000000000000000, 0.9659258262890683122, 1.000000000000000000, 0.9659258262890683122, 1.000000000000000000, 0.9659258262890683122, 1.000000000000000000, 0.9659258262890683122, 1.000000000000000000, 0.9659258262890683122, 1.000000000000000000, 0.9659258262890683122, 1.000000000000000000, 0.9659258262890683122, 1.000000000000000000, 0.9659258262890683122, 1.000000000000000000, 0.9659258262890683122, 1.000000000000000000),
 ( 1.000000000000000000, 0.9659258262890683122, 1.000000000000000000, 0.9659258262890683122, 1.000000000000000000, 0.9659258262890683122, 1.000000000000000000, 0.9659258262890683122, 1.000000000000000000, 0.9659258262890683122, 1.000000000000000000, 0.9659258262890683122, 1.000000000000000000, 0.9659258262890683122, 1.000000000000000000, 0.9659258262890683122, 1.000000000000000000, 0.9659258262890683122, 1.000000000000000000, 0.9659258262890683122, 1.000000000000000000, 0.9659258262890683122, 1.000000000000000000, 0.9659258262890683122, 1.000000000000000000, 0.9659258262890683122, 1.000000000000000000, 0.9659258262890683122, 1.000000000000000000, 0.9659258262890683122, 1.000000000000000000, 0.9659258262890683122, 1.000000000000000000, 0.9659258262890683122, 1.000000000000000000, 0.9659258262890683122, 1.000000000000000000, 0.9659258262890683122, 1.000000000000000000, 0.9659258262890683122, 1.000000000000000000, 0.9659258262890683122, 1.000000000000000000, 0.9659258262890683122, 1.000000000000000000, 0.9659258262890683122, 1.000000000000000000, 0.9659258262890683122, 1.000000000000000000, 0.9659258262890683122, 1.000000000000000000, 0.9659258262890683122, 1.000000000000000000, 0.9659258262890683122, 1.000000000000000000, 0.9659258262890683122, 1.000000000000000000, 0.9659258262890683122, 1.000000000000000000, 0.9659258262890683122, 1.000000000000000000, 0.9659258262890683122, 1.000000000000000000, 0.9659258262890683122, 1.000000000000000000, 0.9659258262890683122, 1.000000000000000000, 0.9659258262890683122, 1.000000000000000000, 0.9659258262890683122, 1.000000000000000000, 0.9659258262890683122, 1.000000000000000000, 0.9659258262890683122, 1.000000000000000000, 0.9659258262890683122, 1.000000000000000000, 0.9659258262890683122, 1.000000000000000000, 0.9659258262890683122, 1.000000000000000000, 0.9659258262890683122, 1.000000000000000000, 0.9659258262890683122, 1.000000000000000000, 0.9659258262890683122, 1.000000000000000000, 0.9659258262890683122, 1.000000000000000000, 0.9659258262890683122, 1.000000000000000000, 0.9659258262890683122, 1.000000000000000000, 0.9659258262890683122, 1.000000000000000000, 0.9659258262890683122, 1.000000000000000000, 0.9659258262890683122, 1.000000000000000000, 0.9659258262890683122, 1.000000000000000000, 0.9659258262890683122, 1.000000000000000000, 0.9659258262890683122, 1.000000000000000000, 0.9659258262890683122, 1.000000000000000000, 0.9659258262890683122, 1.000000000000000000, 0.9659258262890683122, 1.000000000000000000, 0.9659258262890683122, 1.000000000000000000, 0.9659258262890683122, 1.000000000000000000, 0.9659258262890683122, 1.000000000000000000, 0.9659258262890683122, 1.000000000000000000, 0.9659258262890683122, 1.000000000000000000, 0.9659258262890683122, 1.000000000000000000, 0.9659258262890683122, 1.000000000000000000, 0.9659258262890683122, 1.000000000000000000, 0.9659258262890683122, 1.000000000000000000, 0.9659258262890683122, 1.000000000000000000, 0.9659258262890683122, 1.000000000000000000, 0.9659258262890683122, 1.000000000000000000, 0.9659258262890683122, 1.000000000000000000, 0.9659258262890683122, 1.000000000000000000, 0.9659258262890683122, 1.000000000000000000, 0.9659258262890683122, 1.000000000000000000, 0.9659258262890683122, 1.000000000000000000, 0.9659258262890683122, 1.000000000000000000, 0.9659258262890683122, 1.000000000000000000, 0.9659258262890683122, 1.000000000000000000, 0.9659258262890683122, 1.000000000000000000, 0.9659258262890683122, 1.000000000000000000, 0.9659258262890683122, 1.000000000000000000, 0.9659258262890683122, 1.000000000000000000, 0.9659258262890683122, 1.000000000000000000, 0.9659258262890683122, 1.000000000000000000, 0.9659258262890683122, 1.000000000000000000, 0.9659258262890683122, 1.000000000000000000, 0.9659258262890683122, 1.000000000000000000, 0.9659258262890683122, 1.000000000000000000, 0.9659258262890683122, 1.000000000000000000, 0.9659258262890683122, 1.000000000000000000, 0.9659258262890683122, 1.000000000000000000, 0.9659258262890683122, 1.000000000000000000, 0.9659258262890683122, 1.000000000000000000, 0.9659258262890683122, 1.000000000000000000, 0.9659258262890683122, 1.000000000000000000, 0.9659258262890683122, 1.000000000000000000, 0.9659258262890683122, 1.000000000000000000, 0.9659258262890683122, 1.000000000000000000, 0.9659258262890683122, 1.000000000000000000, 0.9659258262890683122, 1.000000000000000000, 0.9659258262890683122, 1.000000000000000000, 0.9659258262890683122, 1.000000000000000000, 0.9659258262890683122, 1.000000000000000000, 0.9659258262890683122, 1.000000000000000000, 0.9659258262890683122, 1.000000000000000000, 0.9659258262890683122, 1.000000000000000000, 0.9659258262890683122, 1.000000000000000000, 0.9659258262890683122, 1.000000000000000000, 0.9659258262890683122, 1.000000000000000000, 0.9659258262890683122, 1.000000000000000000, 0.9659258262890683122, 1.000000000000000000, 0.9659258262890683122, 1.000000000000000000, 0.9659258262890683122, 1.000000000000000000, 0.9659258262890683122, 1.000000000000000000, 0.9659258262890683122, 1.000000000000000000, 0.9659258262890683122, 1.000000000000000000, 0.9659258262890683122, 1.000000000000000000, 0.9659258262890683122, 1.000000000000000000, 0.9659258262890683122, 1.000000000000000000, 0.9659258262890683122, 1.000000000000000000, 0.9659258262890683122, 1.000000000000000000, 0.9659258262890683122, 1.000000000000000000, 0.9659258262890683122, 1.000000000000000000, 0.9659258262890683122, 1.000000000000000000, 0.9659258262890683122, 1.000000000000000000, 0.9659258262890683122, 1.000000000000000000, 0.9659258262890683122, 1.000000000000000000, 0.9659258262890683122, 1.000000000000000000, 0.9659258262890683122, 1.000000000000000000, 0.9659258262890683122, 1.000000000000000000, 0.9659258262890683122, 1.000000000000000000, 0.9659258262890683122, 1.000000000000000000, 0.9659258262890683122, 1.000000000000000000, 0.9659258262890683122, 1.000000000000000000, 0.9659258262890683122, 1.000000000000000000, 0.9659258262890683122, 1.000000000000000000, 0.9659258262890683122, 1.000000000000000000, 0.9659258262890683122, 1.000000000000000000, 0.9659258262890683122, 1.000000000000000000, 0.9659258262890683122, 1.000000000000000000, 0.9659258262890683122, 1.000000000000000000, 0.9659258262890683122, 1.000000000000000000, 0.9659258262890683122, 1.000000000000000000, 0.9659258262890683122, 1.000000000000000000, 0.9659258262890683122, 1.000000000000000000, 0.9659258262890683122, 1.000000000000000000, 0.9659258262890683122, 1.000000000000000000, 0.9659258262890683122, 1.000000000000000000, 0.9659258262890683122, 1.000000000000000000, 0.9659258262890683122, 1.000000000000000000, 0.9659258262890683122, 1.000000000000000000, 0.9659258262890683122, 1.000000000000000000, 0.9659258262890683122, 1.000000000000000000, 0.9659258262890683122, 1.000000000000000000, 0.9659258262890683122, 1.000000000000000000, 0.9659258262890683122, 1.000000000000000000, 0.9659258262890683122, 1.000000000000000000, 0.9659258262890683122, 1.000000000000000000, 0.9659258262890683122, 1.000000000000000000, 0.9659258262890683122, 1.000000000000000000, 0.9659258262890683122, 1.000000000000000000, 0.9659258262890683122, 1.000000000000000000, 0.9659258262890683122, 1.000000000000000000, 0.9659258262890683122, 1.000000000000000000, 0.9659258262890683122, 1.000000000000000000, 0.9659258262890683122, 1.000000000000000000, 0.9659258262890683122, 1.000000000000000000, 0.9659258262890683122, 1.000000000000000000, 0.9659258262890683122, 1.000000000000000000, 0.9659258262890683122, 1.000000000000000000, 0.9659258262890683122, 1.000000000000000000, 0.9659258262890683122, 1.000000000000000000, 0.9659258262890683122, 1.000000000000000000, 0.9659258262890683122, 1.000000000000000000, 0.9659258262890683122, 1.000000000000000000, 0.9659258262890683122, 1.000000000000000000, 0.9659258262890683122, 1.000000000000000000, 0.9659258262890683122, 1.000000000000000000, 0.9659258262890683122, 1.000000000000000000, 0.9659258262890683122, 1.000000000000000000, 0.9659258262890683122, 1.000000000000000000, 0.9659258262890683122, 1.000000000000000000, 0.9659258262890683122, 1.000000000000000000, 0.9659258262890683122, 1.000000000000000000, 0.9659258262890683122, 1.000000000000000000, 0.9659258262890683122, 1.000000000000000000, 0.9659258262890683122, 1.000000000000000000, 0.9659258262890683122, 1.000000000000000000, 0.9659258262890683122, 1.000000000000000000, 0.9659258262890683122, 1.000000000000000000, 0.9659258262890683122, 1.000000000000000000, 0.9659258262890683122, 1.000000000000000000, 0.9659258262890683122, 1.000000000000000000, 0.9659258262890683122, 1.000000000000000000, 0.9659258262890683122, 1.000000000000000000, 0.9659258262890683122, 1.000000000000000000, 0.9659258262890683122, 1.000000000000000000, 0.9659258262890683122, 1.000000000000000000, 0.9659258262890683122, 1.000000000000000000, 0.9659258262890683122, 1.000000000000000000, 0.9659258262890683122, 1.000000000000000000, 0.9659258262890683122, 1.000000000000000000, 0.9659258262890683122, 1.000000000000000000, 0.9659258262890683122, 1.000000000000000000, 0.9659258262890683122, 1.000000000000000000, 0.9659258262890683122, 1.000000000000000000, 0.9659258262890683122, 1.000000000000000000, 0.9659258262890683122, 1.000000000000000000, 0.9659258262890683122, 1.000000000000000000, 0.9659258262890683122, 1.000000000000000000, 0.9659258262890683122, 1.000000000000000000, 0.9659258262890683122, 1.000000000000000000, 0.9659258262890683122, 1.000000000000000000, 0.9659258262890683122, 1.000000000000000000, 0.9659258262890683122, 1.000000000000000000, 0.9659258262890683122, 1.000000000000000000, 0.9659258262890683122, 1.000000000000000000, 0.9659258262890683122, 1.000000000000000000, 0.9659258262890683122, 1.000000000000000000, 0.9659258262890683122, 1.000000000000000000, 0.9659258262890683122, 1.000000000000000000, 0.9659258262890683122, 1.000000000000000000, 0.9659258262890683122, 1.000000000000000000, 0.9659258262890683122, 1.000000000000000000, 0.9659258262890683122, 1.000000000000000000, 0.9659258262890683122, 1.000000000000000000, 0.9659258262890683122, 1.000000000000000000, 0.9659258262890683122, 1.000000000000000000, 0.9659258262890683122, 1.000000000000000000, 0.9659258262890683122, 1.000000000000000000, 0.9659258262890683122, 1.000000000000000000, 0.9659258262890683122, 1.000000000000000000, 0.9659258262890683122, 1.000000000000000000, 0.9659258262890683122, 1.000000000000000000, 0.9659258262890683122, 1.000000000000000000, 0.9659258262890683122, 1.000000000000000000, 0.9659258262890683122, 1.000000000000000000, 0.9659258262890683122, 1.000000000000000000, 0.9659258262890683122, 1.000000000000000000, 0.9659258262890683122, 1.000000000000000000, 0.9659258262890683122, 1.000000000000000000, 0.9659258262890683122, 1.000000000000000000, 0.9659258262890683122, 1.000000000000000000, 0.9659258262890683122, 1.000000000000000000, 0.9659258262890683122, 1.000000000000000000, 0.9659258262890683122, 1.000000000000000000, 0.9659258262890683122, 1.000000000000000000, 0.9659258262890683122, 1.000000000000000000, 0.9659258262890683122, 1.000000000000000000, 0.9659258262890683122, 1.000000000000000000, 0.9659258262890683122, 1.000000000000000000, 0.9659258262890683122, 1.000000000000000000, 0.9659258262890683122, 1.000000000000000000, 0.9659258262890683122, 1.000000000000000000, 0.9659258262890683122, 1.000000000000000000, 0.9659258262890683122, 1.000000000000000000, 0.9659258262890683122, 1.000000000000000000, 0.9659258262890683122, 1.000000000000000000) ) ) 
 REPRESENTATION_ITEM ( '' )  SURFACE ( )  );
#73446=CARTESIAN_POINT ( 'NONE',  ( -0.7874015748031489847, -0.1870078740157479769, 0.4822834645669291653 ) ) ;
#73447=CARTESIAN_POINT ( 'NONE',  ( -0.1246719160104980823, 0.1771653543307087630, 0.09757992244046791164 ) ) ;
#73448=CARTESIAN_POINT ( 'NONE',  ( -1.541994750656167090, -0.6692913385826773087, -0.1292274648535924053 ) ) ;
#73449=CARTESIAN_POINT ( 'NONE',  ( 0.03280839895013198948, -0.6692913385826773087, -0.1292274648535924053 ) ) ;
#73450=CARTESIAN_POINT ( 'NONE',  ( 0.4986876640419954376, -0.5023911411419708095, -0.1820866141732282451 ) ) ;
#73451=CARTESIAN_POINT ( 'NONE',  ( -0.7611548556430438595, 0.1283753931104748280, 0.1820866141732283561 ) ) ;
#73452=CARTESIAN_POINT ( 'NONE',  ( -1.220472440944881054, 0.2952755905511811885, 0.000000000000000000 ) ) ;
#73453=CARTESIAN_POINT ( 'NONE',  ( 1.574803149606299746, -0.1870078740157479769, 0.3641732283464567677 ) ) ;
#73454=CARTESIAN_POINT ( 'NONE',  ( 1.502624671916010790, -0.05778040916215522460, 0.4822834645669289988 ) ) ;
#73456=CARTESIAN_POINT ( 'NONE',  ( 0.6824146981627303710, -0.5023911411419708095, 0.1820866141732285504 ) ) ;
#73457=CARTESIAN_POINT ( 'NONE',  ( 0.7020997375328090762, -0.3162353388693405765, 0.4822834645669290543 ) ) ;
#73459=CARTESIAN_POINT ( 'NONE',  ( 1.522309711286089939, -0.5023911411419708095, -0.1820866141732282451 ) ) ;
#73461=CARTESIAN_POINT ( 'NONE',  ( -0.7939632545931750718, -0.05778040916215560624, -0.4822834645669293319 ) ) ;
#73463=CARTESIAN_POINT ( 'NONE',  ( -1.371391076115484609, -0.5511811023622046335, 0.09757992244046803654 ) ) ;
#73464=CARTESIAN_POINT ( 'NONE',  ( -0.6167979002624665030, -0.4281496062992127816, -0.4176697321401328100 ) ) ;
#73465=CARTESIAN_POINT ( 'NONE',  ( 0.3215223097112867578, -0.05778040916215522460, 0.4822834645669289988 ) ) ;
#73467=CARTESIAN_POINT ( 'NONE',  ( -1.692913385826770645, 0.1771653543307087630, 0.000000000000000000 ) ) ;
#73469=CARTESIAN_POINT ( 'NONE',  ( -1.377952755905511140, 0.2952755905511811885, 0.000000000000000000 ) ) ;
#73470=VECTOR ( 'NONE', #2164, 39.37007874015748143 ) ;
#73472=CARTESIAN_POINT ( 'NONE',  ( 0.3477690288713918276, -0.6692913385826773087, -0.1292274648535924053 ) ) ;
#73473=CARTESIAN_POINT ( 'NONE',  ( -0.1377952755905504645, -0.5400638737290845981, -0.3530559997133363437 ) ) ;
#73474=CARTESIAN_POINT ( 'NONE',  ( 1.049868766404200127, -0.6046776061558809534, -0.2411417322834644161 ) ) ;
#73475=CARTESIAN_POINT ( 'NONE',  ( 1.646981627296588035, -0.3162353388693405765, 0.4822834645669290543 ) ) ;
#73481=CARTESIAN_POINT ( 'NONE',  ( -0.2034120734908131112, -0.5511811023622048555, -0.09757992244046775898 ) ) ;
#73482=CARTESIAN_POINT ( 'NONE',  ( -0.1706036745406816491, -0.4281496062992124485, 0.4176697321401328655 ) ) ;
#73483=CARTESIAN_POINT ( 'NONE',  ( 0.9908136482939640111, 0.2952755905511810774, -0.1292274648535930714 ) ) ;
#73485=CARTESIAN_POINT ( 'NONE',  ( -0.09186351706036663400, -0.3690944881889763329, 0.3153832671262228327 ) ) ;
#73486=CARTESIAN_POINT ( 'NONE',  ( -1.030183727034119867, -0.3162353388693405765, 0.4822834645669290543 ) ) ;
#73487=CARTESIAN_POINT ( 'NONE',  ( 1.089238845144357537, -0.4281496062992124485, 0.4176697321401328655 ) ) ;
#73489=CARTESIAN_POINT ( 'NONE',  ( -0.06873123812452887338, -2.191421614605370878E-15, 0.4445507791589071167 ) ) ;
#73492=EDGE_CURVE ( 'NONE', #41772, #76682, #28921, .T. ) ;
#73494=CARTESIAN_POINT ( 'NONE',  ( 0.9251968503937015864, -0.5400638737290844871, 0.3530559997133364547 ) ) ;
#73495=CARTESIAN_POINT ( 'NONE',  ( 1.469816272965879911, 0.1283753931104746893, -0.1820866141732285504 ) ) ;
#73496=CARTESIAN_POINT ( 'NONE',  ( -1.023622047244093558, -0.1870078740157479769, 0.3641732283464567677 ) ) ;
#73497=CARTESIAN_POINT ( 'NONE',  ( -1.017060367454067249, -0.05778040916215522460, 0.4822834645669289988 ) ) ;
#73499=DIRECTION ( 'NONE',  ( -1.000000000000000000, -0.000000000000000000, -0.000000000000000000 ) ) ;
#73500=CARTESIAN_POINT ( 'NONE',  ( 1.299212598425197429, -0.6692913385826771977, 8.415575281601705876E-17 ) ) ;
#73502=CARTESIAN_POINT ( 'NONE',  ( -0.2034120734908131112, -0.6692913385826773087, -0.1292274648535924053 ) ) ;
#73503=CARTESIAN_POINT ( 'NONE',  ( -0.5774278215223089816, 0.2306618581243847221, -0.2411417322834647770 ) ) ;
#73504=CARTESIAN_POINT ( 'NONE',  ( -1.345144356955379816, -0.3162353388693405765, 0.4822834645669290543 ) ) ;
#73506=CARTESIAN_POINT ( 'NONE',  ( 0.1640419947506569498, -0.05778040916215522460, 0.4822834645669289988 ) ) ;
#73508=CARTESIAN_POINT ( 'NONE',  ( -1.181102362204723644, -0.1870078740157479769, 0.3641732283464567677 ) ) ;
#73511=ORIENTED_EDGE ( 'NONE', *, *, #11002, .F. ) ;
#73513=CARTESIAN_POINT ( 'NONE',  ( -1.686351706036744558, 0.2952755905511810774, -0.1292274648535930714 ) ) ;
#73515=CARTESIAN_POINT ( 'NONE',  ( -1.614173228346456268, -0.6692913385826771977, 8.415575281601705876E-17 ) ) ;
#73517=DIRECTION ( 'NONE',  ( 0.000000000000000000, 0.000000000000000000, 1.000000000000000000 ) ) ;
#73518=CARTESIAN_POINT ( 'NONE',  ( -0.3412073490813641308, 0.2306618581243847221, -0.2411417322834647770 ) ) ;
#73520=CARTESIAN_POINT ( 'NONE',  ( -0.4461942257217840213, -0.5023911411419708095, -0.1820866141732282451 ) ) ;
#73521=CARTESIAN_POINT ( 'NONE',  ( -0.9317585301837263412, -0.004921259842519576551, 0.3153832671262227771 ) ) ;
#73522=CARTESIAN_POINT ( 'NONE',  ( -1.056430446194224881, -0.6692913385826771977, 0.1292274648535927661 ) ) ;
#73523=CARTESIAN_POINT ( 'NONE',  ( 0.4330708661417329575, -0.6692913385826771977, 8.415575281601705876E-17 ) ) ;
#73524=CARTESIAN_POINT ( 'NONE',  ( -0.7217847769028863381, -0.4281496062992124485, 0.4176697321401328655 ) ) ;
#73526=VERTEX_POINT ( 'NONE', #81940 ) ;
#73527=CARTESIAN_POINT ( 'NONE',  ( -1.489501312335957062, -0.05778040916215522460, 0.4822834645669289988 ) ) ;
#73528=FACE_OUTER_BOUND ( 'NONE', #29484, .T. ) ;
#73530=AXIS2_PLACEMENT_3D ( 'NONE', #20873, #72226, #46941 ) ;
#73534=( BOUNDED_CURVE ( )  B_SPLINE_CURVE ( 2, ( #33781, #59444, #34195, #13596, #79247, #20319, #77571, #21155, #14851, #39675, #39250, #977, #58609 ),
 .UNSPECIFIED., .F., .F. ) 
 B_SPLINE_CURVE_WITH_KNOTS ( ( 3, 2, 2, 2, 2, 2, 3 ),
 ( 0.5831241751160508580, 0.5833333333333333703, 0.5871212121212121549, 0.5909090909090909394, 0.5946969696969697239, 0.5984848484848485084, 0.5986940067021310208 ),
 .UNSPECIFIED. ) 
 CURVE ( )  GEOMETRIC_REPRESENTATION_ITEM ( )  RATIONAL_B_SPLINE_CURVE ( ( 0.9964447847208419695, 0.9981185001348091834, 1.000000000000000000, 0.9659258262890683122, 1.000000000000000000, 0.9659258262890683122, 1.000000000000000000, 0.9659258262890683122, 1.000000000000000000, 0.9659258262890683122, 1.000000000000000000, 0.9981185001348091834, 0.9964447847208420805 ) ) 
 REPRESENTATION_ITEM ( '' )  );
#73537=CARTESIAN_POINT ( 'NONE',  ( -0.5446194225721777693, -0.05778040916215522460, 0.4822834645669289988 ) ) ;
#73538=CARTESIAN_POINT ( 'NONE',  ( 1.548556430446194954, 0.2306618581243847221, -0.2411417322834647770 ) ) ;
#73539=CIRCLE ( 'NONE', #60059, 1.220472440944881942 ) ;
#73541=CARTESIAN_POINT ( 'NONE',  ( -0.7478466213799872531, 2.204724409448818978, -0.5309055118110235227 ) ) ;
#73543=CARTESIAN_POINT ( 'NONE',  ( -1.227034120734907585, 0.2952755905511811885, 0.1292274648535926551 ) ) ;
#73544=CARTESIAN_POINT ( 'NONE',  ( -0.8202099737532801971, -0.6692913385826771977, 0.1292274648535927661 ) ) ;
#73546=CARTESIAN_POINT ( 'NONE',  ( 0.3280839895013130669, -0.004921259842519576551, 0.3153832671262227771 ) ) ;
#73548=CARTESIAN_POINT ( 'NONE',  ( 0.2230971128608932319, -0.3690944881889763329, 0.3153832671262228327 ) ) ;
#73549=CARTESIAN_POINT ( 'NONE',  ( 0.9448818897637802916, -0.1870078740157479769, 0.3641732283464567677 ) ) ;
#73550=CARTESIAN_POINT ( 'NONE',  ( 0.8202099737532813073, 0.2952755905511811885, 0.1292274648535926551 ) ) ;
#73551=CARTESIAN_POINT ( 'NONE',  ( -0.1771653543307080136, 0.07958543189024071263, -0.2665933059059888421 ) ) ;
#73553=CARTESIAN_POINT ( 'NONE',  ( 1.404199475065617264, -0.4281496062992124485, 0.4176697321401328655 ) ) ;
#73554=CARTESIAN_POINT ( 'NONE',  ( -1.207349081364828436, -0.5023911411419708095, 0.1820866141732285504 ) ) ;
#73556=CARTESIAN_POINT ( 'NONE',  ( -0.7677165354330699465, -0.4536011799217368745, -0.2665933059059886201 ) ) ;
#73557=CARTESIAN_POINT ( 'NONE',  ( 0.08530183727034192087, -0.05778040916215522460, 0.4822834645669289988 ) ) ;
#73558=CARTESIAN_POINT ( 'NONE',  ( 1.692913385826772421, 0.1771653543307087630, 0.000000000000000000 ) ) ;
#73559=CARTESIAN_POINT ( 'NONE',  ( 0.6692913385826777528, 0.1771653543307087630, 0.000000000000000000 ) ) ;
#73560=CARTESIAN_POINT ( 'NONE',  ( -0.1837270341207343505, -0.5023911411419708095, 0.1820866141732285504 ) ) ;
#73561=CARTESIAN_POINT ( 'NONE',  ( -0.6561679790026240244, 0.2306618581243847221, -0.2411417322834647770 ) ) ;
#73563=CARTESIAN_POINT ( 'NONE',  ( -1.614173228346456712, 2.401574803149606474, 0.1372047244094477536 ) ) ;
#73564=CARTESIAN_POINT ( 'NONE',  ( 0.3608923884514443348, -0.6692913385826771977, 0.1292274648535927661 ) ) ;
#73566=CARTESIAN_POINT ( 'NONE',  ( 1.607611548556431069, 0.2952755905511811885, 0.1292274648535926551 ) ) ;
#73567=CARTESIAN_POINT ( 'NONE',  ( -0.2362204724409442680, -0.1870078740157480601, -0.3641732283464567677 ) ) ;
#73568=CARTESIAN_POINT ( 'NONE',  ( 0.01312335958005323398, 0.05413385826771666132, 0.4176697321401328100 ) ) ;
#73569=CARTESIAN_POINT ( 'NONE',  ( -1.384514435695537005, -0.6692913385826773087, -0.1292274648535924053 ) ) ;
#73570=CARTESIAN_POINT ( 'NONE',  ( 1.679790026246720025, 0.2306618581243848609, 0.2411417322834645549 ) ) ;
#73571=CARTESIAN_POINT ( 'NONE',  ( 1.482939632545932307, -0.4281496062992124485, 0.4176697321401328655 ) ) ;
#73572=CARTESIAN_POINT ( 'NONE',  ( -0.5643044619422565855, -0.004921259842519870586, -0.3153832671262229437 ) ) ;
#73576=CARTESIAN_POINT ( 'NONE',  ( 1.502624671916010790, -0.08942795157527998196, 0.3641732283464567121 ) ) ;
#73577=CARTESIAN_POINT ( 'NONE',  ( 1.213910761154856299, -0.5511811023622048555, -0.09757992244046775898 ) ) ;
#73579=CARTESIAN_POINT ( 'NONE',  ( 0.9842519685039375910, 0.2952755905511811885, 0.000000000000000000 ) ) ;
#73581=CARTESIAN_POINT ( 'NONE',  ( 1.207349081364829990, 0.1283753931104748280, 0.1820866141732283561 ) ) ;
#73582=ADVANCED_FACE ( 'NONE', ( #68068 ), #74385, .F. ) ;
#73583=CARTESIAN_POINT ( 'NONE',  ( -0.07217847769028787330, -0.05778040916215522460, 0.4822834645669289988 ) ) ;
#73584=CARTESIAN_POINT ( 'NONE',  ( -0.2952755905511803003, -0.5400638737290845981, -0.3530559997133363437 ) ) ;
#73590=CARTESIAN_POINT ( 'NONE',  ( 0.5511811023622054106, -0.1870078740157480601, -0.3641732283464567677 ) ) ;
#73591=ORIENTED_EDGE ( 'NONE', *, *, #4963, .T. ) ;
#73593=ORIENTED_EDGE ( 'NONE', *, *, #79585, .T. ) ;
#73595=CARTESIAN_POINT ( 'NONE',  ( -0.3280839895013117347, -0.4281496062992124485, 0.4176697321401328655 ) ) ;
#73596=CARTESIAN_POINT ( 'NONE',  ( 0.8661417322834652488, -0.1870078740157480879, -0.4822834645669291653 ) ) ;
#73597=CARTESIAN_POINT ( 'NONE',  ( 0.2952755905511819101, 0.1660481256975883668, -0.3530559997133364547 ) ) ;
#73598=CARTESIAN_POINT ( 'NONE',  ( -0.4265091863517051496, -0.5511811023622046335, 0.09757992244046803654 ) ) ;
#73599=CARTESIAN_POINT ( 'NONE',  ( 0.9186351706036752773, 0.2306618581243847221, -0.2411417322834647770 ) ) ;
#73600=CARTESIAN_POINT ( 'NONE',  ( -0.9580052493438311334, 0.05413385826771626580, -0.4176697321401330321 ) ) ;
#73601=CARTESIAN_POINT ( 'NONE',  ( -0.3543307086614165824, -0.6692913385826771977, 8.415575281601705876E-17 ) ) ;
#73602=CARTESIAN_POINT ( 'NONE',  ( -0.7217847769028863381, 0.05413385826771626580, -0.4176697321401330321 ) ) ;
#73603=CARTESIAN_POINT ( 'NONE',  ( 1.384514435695538337, -0.6692913385826771977, 0.1292274648535927661 ) ) ;
#73604=CARTESIAN_POINT ( 'NONE',  ( 0.8398950131233602345, 0.2306618581243847221, -0.2411417322834647770 ) ) ;
#73605=CARTESIAN_POINT ( 'NONE',  ( 0.7283464566929143125, 0.1660481256975885056, 0.3530559997133364547 ) ) ;
#73607=CARTESIAN_POINT ( 'NONE',  ( 0.2165354330708668673, -0.4536011799217367080, 0.2665933059059888421 ) ) ;
#73611=CARTESIAN_POINT ( 'NONE',  ( -1.049868766404198794, 0.1283753931104746893, -0.1820866141732285504 ) ) ;
#73612=CARTESIAN_POINT ( 'NONE',  ( -0.3412073490813641308, 0.2306618581243847221, -0.2411417322834647770 ) ) ;
#73614=CARTESIAN_POINT ( 'NONE',  ( -0.3215223097112853146, -0.3162353388693405765, 0.4822834645669290543 ) ) ;
#73615=CARTESIAN_POINT ( 'NONE',  ( -0.5971128608923877978, 0.2952755905511811885, 0.1292274648535926551 ) ) ;
#73616=CARTESIAN_POINT ( 'NONE',  ( -1.423884514435694859, -0.05778040916215560624, -0.4822834645669293319 ) ) ;
#73617=CARTESIAN_POINT ( 'NONE',  ( -1.574803149606298636, -0.1870078740157479769, 0.4822834645669291653 ) ) ;
#73618=CARTESIAN_POINT ( 'NONE',  ( 1.010498687664042716, -0.3690944881889763329, 0.3153832671262228327 ) ) ;
#73621=CARTESIAN_POINT ( 'NONE',  ( 0.5839895013123367340, -0.5511811023622048555, -0.09757992244046775898 ) ) ;
#73622=CARTESIAN_POINT ( 'NONE',  ( 0.1312335958005257930, 0.2306618581243847221, -0.2411417322834647770 ) ) ;
#73623=CARTESIAN_POINT ( 'NONE',  ( 0.5380577427821529035, -0.4281496062992124485, 0.4176697321401328655 ) ) ;
#73630=CARTESIAN_POINT ( 'NONE',  ( -0.5380577427821514602, -0.3690944881889765550, -0.3153832671262227771 ) ) ;
#73631=CARTESIAN_POINT ( 'NONE',  ( -1.069553805774277722, 0.2952755905511811885, 0.1292274648535926551 ) ) ;
#73634=CARTESIAN_POINT ( 'NONE',  ( -1.581364829396324945, -0.08942795157528024563, -0.3641732283464568787 ) ) ;
#73635=CARTESIAN_POINT ( 'NONE',  ( 0.8858267716535438430, -0.5400638737290845981, -0.3530559997133363437 ) ) ;
#73636=CARTESIAN_POINT ( 'NONE',  ( 0.3412073490813655186, -0.6046776061558809534, -0.2411417322834644161 ) ) ;
#73637=CARTESIAN_POINT ( 'NONE',  ( -0.4921259842519677963, 0.07958543189024071263, -0.2665933059059888421 ) ) ;
#73638=CARTESIAN_POINT ( 'NONE',  ( 0.03937007874015806264, 0.2952755905511811885, 0.000000000000000000 ) ) ;
#73640=CARTESIAN_POINT ( 'NONE',  ( -0.1574803149606292529, -0.1870078740157480601, -0.3641732283464567677 ) ) ;
#73641=CARTESIAN_POINT ( 'NONE',  ( -0.5708661417322828946, 0.1660481256975883668, -0.3530559997133364547 ) ) ;
#73643=CARTESIAN_POINT ( 'NONE',  ( -1.706036745406823485, 0.2306618581243848609, 0.2411417322834645549 ) ) ;
#73644=CARTESIAN_POINT ( 'NONE',  ( 0.2296587926509192634, -0.08942795157528024563, -0.3641732283464568787 ) ) ;
#73645=CARTESIAN_POINT ( 'NONE',  ( 1.450131233595801428, -0.5511811023622048555, -0.09757992244046775898 ) ) ;
#73646=CARTESIAN_POINT ( 'NONE',  ( -1.259842519685038686, -0.1870078740157479769, 0.4822834645669291653 ) ) ;
#73647=CARTESIAN_POINT ( 'NONE',  ( -0.9055118110236215490, -0.5511811023622047445, 6.969142054262312111E-17 ) ) ;
#73648=DIRECTION ( 'NONE',  ( 1.000000000000000000, -0.000000000000000000, -0.000000000000000000 ) ) ;
#73649=CARTESIAN_POINT ( 'NONE',  ( -1.266404199475064773, -0.3162353388693405765, 0.4822834645669290543 ) ) ;
#73650=CARTESIAN_POINT ( 'NONE',  ( -0.1115485564304453947, -0.6692913385826771977, 0.1292274648535927661 ) ) ;
#73655=CARTESIAN_POINT ( 'NONE',  ( 0.4068241469816281097, -0.004921259842519576551, 0.3153832671262227771 ) ) ;
#73656=CARTESIAN_POINT ( 'NONE',  ( 1.069553805774278610, -0.6692913385826771977, 0.1292274648535927661 ) ) ;
#73657=CARTESIAN_POINT ( 'NONE',  ( -1.351706036745406347, -0.004921259842519870586, -0.3153832671262229437 ) ) ;
#73658=CARTESIAN_POINT ( 'NONE',  ( 1.095800524934383846, -0.05778040916215560624, -0.4822834645669293319 ) ) ;
#73659=CARTESIAN_POINT ( 'NONE',  ( -1.633858267716534529, -0.4536011799217368745, -0.2665933059059886201 ) ) ;
#73660=EDGE_CURVE ( 'NONE', #73693, #22261, #10999, .T. ) ;
#73661=CARTESIAN_POINT ( 'NONE',  ( -0.6036745406824141069, 0.2306618581243848609, 0.2411417322834645549 ) ) ;
#73662=CARTESIAN_POINT ( 'NONE',  ( 0.1902887139107617975, -0.5511811023622048555, -0.09757992244046775898 ) ) ;
#73664=CARTESIAN_POINT ( 'NONE',  ( 0.4658792650918640033, -0.2845877964562159024, 0.3641732283464567677 ) ) ;
#73665=CARTESIAN_POINT ( 'NONE',  ( 0.03280839895013198948, -0.6692913385826773087, -0.1292274648535924053 ) ) ;
#73667=CARTESIAN_POINT ( 'NONE',  ( -1.240157480314959759, 0.1660481256975885056, 0.3530559997133364547 ) ) ;
#73669=CARTESIAN_POINT ( 'NONE',  ( 1.187664041994751285, -0.2845877964562161244, -0.3641732283464567121 ) ) ;
#73670=CARTESIAN_POINT ( 'NONE',  ( -0.1246719160104980823, -0.6692913385826773087, -0.1292274648535924053 ) ) ;
#73671=CARTESIAN_POINT ( 'NONE',  ( -0.2952755905511803003, -0.5400638737290845981, -0.3530559997133363437 ) ) ;
#73672=CARTESIAN_POINT ( 'NONE',  ( -0.5708661417322825615, -0.4536011799217367080, 0.2665933059059888421 ) ) ;
#73673=CARTESIAN_POINT ( 'NONE',  ( 1.194225721784777594, 0.05413385826771666132, 0.4176697321401328100 ) ) ;
#73674=CARTESIAN_POINT ( 'NONE',  ( -0.4461942257217840213, -0.5023911411419708095, -0.1820866141732282451 ) ) ;
#73675=CARTESIAN_POINT ( 'NONE',  ( 0.2362204724409456558, -0.1870078740157479769, 0.4822834645669291653 ) ) ;
#73676=B_SPLINE_CURVE_WITH_KNOTS ( 'NONE', 3,
 ( #10863, #54639, #61373, #62199, #3723, #23898, #42829 ),
 .UNSPECIFIED., .F., .F.,
 ( 4, 3, 4 ),
 ( 1.734723475976807094E-18, 0.001246230184515564584, 0.002492489877932635520 ),
 .UNSPECIFIED. ) ;
#73677=CARTESIAN_POINT ( 'NONE',  ( -0.6758530183727028406, -0.5511811023622048555, -0.09757992244046775898 ) ) ;
#73679=CARTESIAN_POINT ( 'NONE',  ( -1.338582677165353729, -0.1870078740157479769, 0.4822834645669291653 ) ) ;
#73681=EDGE_LOOP ( 'NONE', ( #56307, #5323, #7674, #41581 ) ) ;
#73682=CARTESIAN_POINT ( 'NONE',  ( -1.174540682414697335, -0.2845877964562161244, -0.3641732283464567121 ) ) ;
#73683=CARTESIAN_POINT ( 'NONE',  ( -0.2493438320209966919, 0.05413385826771626580, -0.4176697321401330321 ) ) ;
#73685=CARTESIAN_POINT ( 'NONE',  ( -1.220472440944881054, -0.6692913385826771977, 8.415575281601705876E-17 ) ) ;
#73687=CARTESIAN_POINT ( 'NONE',  ( 1.200787401574803681, 0.1660481256975885056, 0.3530559997133364547 ) ) ;
#73688=CARTESIAN_POINT ( 'NONE',  ( 0.8661417322834653598, -0.1870078740157479769, 0.4822834645669291653 ) ) ;
#73691=CARTESIAN_POINT ( 'NONE',  ( -1.587926509186350810, -0.4281496062992124485, 0.4176697321401328655 ) ) ;
#73693=VERTEX_POINT ( 'NONE', #24251 ) ;
#73694=CARTESIAN_POINT ( 'NONE',  ( -0.4790026246719152336, -0.08942795157528024563, -0.3641732283464568787 ) ) ;
#73697=CARTESIAN_POINT ( 'NONE',  ( 0.9842519685039375910, 0.2952755905511811885, 0.000000000000000000 ) ) ;
#73698=CARTESIAN_POINT ( 'NONE',  ( -0.4921259842519677963, -0.5400638737290844871, 0.3530559997133364547 ) ) ;
#73699=CARTESIAN_POINT ( 'NONE',  ( -1.089238845144356427, -0.4281496062992127816, -0.4176697321401328100 ) ) ;
#73700=CARTESIAN_POINT ( 'NONE',  ( 1.679790026246720025, 0.2306618581243848609, 0.2411417322834645549 ) ) ;
#73701=CARTESIAN_POINT ( 'NONE',  ( -1.377952755905511140, -0.5511811023622047445, 6.969142054262312111E-17 ) ) ;
#73703=CARTESIAN_POINT ( 'NONE',  ( 0.5183727034120741983, -0.6692913385826771977, 0.1292274648535927661 ) ) ;
#73704=CARTESIAN_POINT ( 'NONE',  ( -0.8005249343832011588, 0.05413385826771626580, -0.4176697321401330321 ) ) ;
#73706=CARTESIAN_POINT ( 'NONE',  ( -1.246719160104985846, -0.4281496062992127816, -0.4176697321401328100 ) ) ;
#73708=CARTESIAN_POINT ( 'NONE',  ( 0.8202099737532814183, -0.6692913385826773087, -0.1292274648535924053 ) ) ;
#73709=CARTESIAN_POINT ( 'NONE',  ( 1.174540682414699111, -0.2845877964562159024, 0.3641732283464567677 ) ) ;
#73712=CARTESIAN_POINT ( 'NONE',  ( -0.2427821522309703550, -0.3162353388693405765, 0.4822834645669290543 ) ) ;
#73713=ORIENTED_EDGE ( 'NONE', *, *, #16758, .T. ) ;
#73715=CARTESIAN_POINT ( 'NONE',  ( 0.1968503937007881344, 0.1771653543307087630, 0.000000000000000000 ) ) ;
#73716=CARTESIAN_POINT ( 'NONE',  ( -1.187664041994750175, -0.05778040916215560624, -0.4822834645669293319 ) ) ;
#73717=CARTESIAN_POINT ( 'NONE',  ( 0.7939632545931766261, -0.05778040916215522460, 0.4822834645669289988 ) ) ;
#73718=CARTESIAN_POINT ( 'NONE',  ( 0.9973753280839902091, 0.2306618581243847221, -0.2411417322834647770 ) ) ;
#73719=CARTESIAN_POINT ( 'NONE',  ( -0.1115485564304456306, 0.2952755905511810774, -0.1292274648535930714 ) ) ;
#73721=CARTESIAN_POINT ( 'NONE',  ( -0.8727034120734901146, -0.3162353388693405765, 0.4822834645669290543 ) ) ;
#73723=CARTESIAN_POINT ( 'NONE',  ( -1.509186351706035767, 0.05413385826771626580, -0.4176697321401330321 ) ) ;
#73724=CARTESIAN_POINT ( 'NONE',  ( -0.6233595800524928121, -0.3162353388693409650, -0.4822834645669289433 ) ) ;
#73725=CARTESIAN_POINT ( 'NONE',  ( -0.4921259842519677963, 0.07958543189024071263, -0.2665933059059888421 ) ) ;
#73726=CARTESIAN_POINT ( 'NONE',  ( 1.253280839895013710, -0.05778040916215560624, -0.4822834645669293319 ) ) ;
#73727=CARTESIAN_POINT ( 'NONE',  ( 1.430446194225722500, -0.4281496062992127816, -0.4176697321401328100 ) ) ;
#73729=CARTESIAN_POINT ( 'NONE',  ( -0.7808398950131225646, -0.05778040916215522460, 0.4822834645669289988 ) ) ;
#73732=CARTESIAN_POINT ( 'NONE',  ( 0.9055118110236227702, -0.6692913385826771977, 8.415575281601705876E-17 ) ) ;
#73735=EDGE_CURVE ( 'NONE', #11499, #4976, #56686, .T. ) ;
#73736=CARTESIAN_POINT ( 'NONE',  ( 0.01312335958005323398, -0.4281496062992127816, -0.4176697321401328100 ) ) ;
#73737=CARTESIAN_POINT ( 'NONE',  ( -1.167979002624671470, -0.004921259842519576551, 0.3153832671262227771 ) ) ;
#73738=CARTESIAN_POINT ( 'NONE',  ( 0.7020997375328090762, -0.2845877964562159024, 0.3641732283464567677 ) ) ;
#73740=CARTESIAN_POINT ( 'NONE',  ( 1.069553805774278832, 0.1771653543307087075, -0.09757992244046823083 ) ) ;
#73741=CARTESIAN_POINT ( 'NONE',  ( 0.6233595800524939223, -0.3162353388693405765, 0.4822834645669290543 ) ) ;
#73743=CARTESIAN_POINT ( 'NONE',  ( -0.1771653543307080136, -0.5400638737290844871, 0.3530559997133364547 ) ) ;
#73745=CARTESIAN_POINT ( 'NONE',  ( 1.181102362204724976, -0.1870078740157480601, -0.3641732283464567677 ) ) ;
#73746=CARTESIAN_POINT ( 'NONE',  ( -0.5839895013123351797, 0.2952755905511810774, -0.1292274648535930714 ) ) ;
#73748=CARTESIAN_POINT ( 'NONE',  ( 1.128608923884515169, -0.6046776061558809534, -0.2411417322834644161 ) ) ;
#73749=CARTESIAN_POINT ( 'NONE',  ( 0.1968503937007881344, 0.2952755905511811885, 0.000000000000000000 ) ) ;
#73750=CARTESIAN_POINT ( 'NONE',  ( 0.6627296587926517768, -0.5511811023622048555, -0.09757992244046775898 ) ) ;
#73752=CARTESIAN_POINT ( 'NONE',  ( 0.1771653543307093182, -0.4536011799217368745, -0.2665933059059886201 ) ) ;
#73755=CARTESIAN_POINT ( 'NONE',  ( 0.6364829396325465405, -0.3162353388693409650, -0.4822834645669289433 ) ) ;
#73756=EDGE_CURVE ( 'NONE', #46664, #73939, #75208, .T. ) ;
#73758=CARTESIAN_POINT ( 'NONE',  ( 1.640419947506562393, -0.3690944881889763329, 0.3153832671262228327 ) ) ;
#73759=CARTESIAN_POINT ( 'NONE',  ( 0.1246719160104994284, 0.2952755905511810219, -0.1292274648535930437 ) ) ;
#73760=CARTESIAN_POINT ( 'NONE',  ( -0.05905511811023545637, -0.4536011799217368745, -0.2665933059059886201 ) ) ;
#73761=CARTESIAN_POINT ( 'NONE',  ( -0.006561679790025524116, -0.05778040916215560624, -0.4822834645669293319 ) ) ;
#73762=CARTESIAN_POINT ( 'NONE',  ( 1.417322834645670104, -0.1870078740157480601, -0.3641732283464567677 ) ) ;
#73763=CARTESIAN_POINT ( 'NONE',  ( -1.548556430446193399, 0.1283753931104748280, 0.1820866141732283561 ) ) ;
#73764=CARTESIAN_POINT ( 'NONE',  ( -1.404199475065615932, 0.05413385826771666132, 0.4176697321401328100 ) ) ;
#73765=CARTESIAN_POINT ( 'NONE',  ( 0.6036745406824154392, 0.2306618581243847221, -0.2411417322834647770 ) ) ;
#73766=CARTESIAN_POINT ( 'NONE',  ( 1.220472440944882608, 0.2952755905511811885, 0.000000000000000000 ) ) ;
#73767=( BOUNDED_CURVE ( )  B_SPLINE_CURVE ( 1, ( #48180, #74288 ),
 .UNSPECIFIED., .F., .F. ) 
 B_SPLINE_CURVE_WITH_KNOTS ( ( 2, 2 ),
 ( 4.933119884809045175E-18, 0.002000000000000006981 ),
 .UNSPECIFIED. ) 
 CURVE ( )  GEOMETRIC_REPRESENTATION_ITEM ( )  RATIONAL_B_SPLINE_CURVE ( ( 0.9875488213027523443, 0.9875488213027523443 ) ) 
 REPRESENTATION_ITEM ( '' )  );
#73769=CARTESIAN_POINT ( 'NONE',  ( 0.3477690288713918276, 0.2952755905511811885, 0.1292274648535926551 ) ) ;
#73770=CARTESIAN_POINT ( 'NONE',  ( 1.227034120734908917, 0.2952755905511810774, -0.1292274648535930714 ) ) ;
#73771=CARTESIAN_POINT ( 'NONE',  ( 0.9580052493438327987, -0.4281496062992127816, -0.4176697321401328100 ) ) ;
#73772=CARTESIAN_POINT ( 'NONE',  ( 0.6561679790026253567, -0.5023911411419708095, -0.1820866141732282451 ) ) ;
#73773=CARTESIAN_POINT ( 'NONE',  ( 1.463254593175853824, -0.6692913385826771977, 0.1292274648535927661 ) ) ;
#73774=CARTESIAN_POINT ( 'NONE',  ( -0.6496062992125976043, 0.07958543189024071263, -0.2665933059059888421 ) ) ;
#73775=CARTESIAN_POINT ( 'NONE',  ( 0.5314960629921264834, 0.07958543189024071263, -0.2665933059059888421 ) ) ;
#73776=CARTESIAN_POINT ( 'NONE',  ( 0.1837270341207357105, -0.6046776061558809534, -0.2411417322834644161 ) ) ;
#73777=CARTESIAN_POINT ( 'NONE',  ( 0.8661417322834652488, -0.1870078740157480879, -0.4822834645669291653 ) ) ;
#73778=CARTESIAN_POINT ( 'NONE',  ( -0.5052493438320203589, 0.2952755905511810774, -0.1292274648535930714 ) ) ;
#73779=CARTESIAN_POINT ( 'NONE',  ( 0.2887139107611556010, -0.5023911411419708095, 0.1820866141732285504 ) ) ;
#73780=CARTESIAN_POINT ( 'NONE',  ( 0.6364829396325465405, -0.05778040916215522460, 0.4822834645669289988 ) ) ;
#73782=CARTESIAN_POINT ( 'NONE',  ( -0.8595800524934373854, -0.3162353388693409650, -0.4822834645669289433 ) ) ;
#73786=CARTESIAN_POINT ( 'NONE',  ( -0.9120734908136475250, -0.6692913385826773087, -0.1292274648535924053 ) ) ;
#73787=CARTESIAN_POINT ( 'NONE',  ( -0.2755905511811018171, 0.2952755905511811885, 0.000000000000000000 ) ) ;
#73790=EDGE_LOOP ( 'NONE', ( #44326, #17993, #79697, #75239 ) ) ;
#73791=CARTESIAN_POINT ( 'NONE',  ( 0.6561679790026253567, -0.5023911411419708095, -0.1820866141732282451 ) ) ;
#73793=CARTESIAN_POINT ( 'NONE',  ( 0.9645669291338588858, 0.1660481256975885056, 0.3530559997133364547 ) ) ;
#73795=CARTESIAN_POINT ( 'NONE',  ( -1.535433070866141225, 0.1771653543307087630, 0.000000000000000000 ) ) ;
#73796=CARTESIAN_POINT ( 'NONE',  ( 1.450131233595801428, -0.6692913385826773087, -0.1292274648535924053 ) ) ;
#73797=CARTESIAN_POINT ( 'NONE',  ( -1.502624671916009680, -0.05778040916215560624, -0.4822834645669293319 ) ) ;
#73798=CARTESIAN_POINT ( 'NONE',  ( 0.2755905511811031494, 0.2952755905511811885, 0.000000000000000000 ) ) ;
#73800=EDGE_CURVE ( 'NONE', #29072, #20803, #25143, .T. ) ;
#73801=CARTESIAN_POINT ( 'NONE',  ( 0.01312335958005323398, -0.4281496062992127816, -0.4176697321401328100 ) ) ;
#73802=CARTESIAN_POINT ( 'NONE',  ( -0.7349081364829390672, 0.1283753931104746893, -0.1820866141732285504 ) ) ;
#73803=CARTESIAN_POINT ( 'NONE',  ( 0.9251968503937015864, -0.5400638737290844871, 0.3530559997133364547 ) ) ;
#73804=CARTESIAN_POINT ( 'NONE',  ( -0.05249343832020938322, -0.6046776061558809534, -0.2411417322834644161 ) ) ;
#73808=CARTESIAN_POINT ( 'NONE',  ( 0.9383202099737538715, -0.05778040916215560624, -0.4822834645669293319 ) ) ;
#73809=CARTESIAN_POINT ( 'NONE',  ( 0.2427821522309716595, -0.3162353388693409650, -0.4822834645669289433 ) ) ;
#73810=CARTESIAN_POINT ( 'NONE',  ( -0.8792650918635160906, -0.4281496062992124485, 0.4176697321401328655 ) ) ;
#73811=CARTESIAN_POINT ( 'NONE',  ( 1.286089238845145033, 0.2306618581243848609, 0.2411417322834645549 ) ) ;
#73812=CARTESIAN_POINT ( 'NONE',  ( 0.6102362204724416372, 0.1660481256975883668, -0.3530559997133364547 ) ) ;
#73814=CARTESIAN_POINT ( 'NONE',  ( -0.3871391076115479057, -0.3162353388693409650, -0.4822834645669289433 ) ) ;
#73815=CARTESIAN_POINT ( 'NONE',  ( 0.7217847769028878924, 0.05413385826771666132, 0.4176697321401328100 ) ) ;
#73816=CARTESIAN_POINT ( 'NONE',  ( -0.01312335958005186876, 0.05413385826771626580, -0.4176697321401330321 ) ) ;
#73817=CARTESIAN_POINT ( 'NONE',  ( 0.7349081364829403995, 0.1283753931104748280, 0.1820866141732283561 ) ) ;
#73818=CARTESIAN_POINT ( 'NONE',  ( -1.377952755905511140, 0.2952755905511811885, 0.000000000000000000 ) ) ;
#73820=CARTESIAN_POINT ( 'NONE',  ( 0.2755905511811031494, -0.6692913385826771977, 8.415575281601705876E-17 ) ) ;
#73824=EDGE_LOOP ( 'NONE', ( #1981, #67884, #6598, #31421 ) ) ;
#73825=CARTESIAN_POINT ( 'NONE',  ( 1.272965879265092637, -0.4281496062992127816, -0.4176697321401328100 ) ) ;
#73826=CARTESIAN_POINT ( 'NONE',  ( 0.7086614173228352742, -0.1870078740157480601, -0.3641732283464567677 ) ) ;
#73833=CARTESIAN_POINT ( 'NONE',  ( -0.9973753280839886548, 0.2306618581243848609, 0.2411417322834645549 ) ) ;
#73834=CARTESIAN_POINT ( 'NONE',  ( -0.7874015748031489847, -0.1870078740157479769, 0.4822834645669291653 ) ) ;
#73835=CARTESIAN_POINT ( 'NONE',  ( 0.6561679790026253567, 0.2306618581243848609, 0.2411417322834645549 ) ) ;
#73836=ORIENTED_EDGE ( 'NONE', *, *, #82527, .F. ) ;
#73837=CARTESIAN_POINT ( 'NONE',  ( 1.463254593175853824, 0.2952755905511810774, -0.1292274648535930714 ) ) ;
#73842=CARTESIAN_POINT ( 'NONE',  ( -1.358267716535432434, -0.4536011799217367080, 0.2665933059059888421 ) ) ;
#73843=CARTESIAN_POINT ( 'NONE',  ( 1.614173228346457378, 0.7794589730111999293, 0.1372047244094478369 ) ) ;
#73844=CARTESIAN_POINT ( 'NONE',  ( 0.1312335958005257930, 0.2306618581243847221, -0.2411417322834647770 ) ) ;
#73845=CARTESIAN_POINT ( 'NONE',  ( 1.660104986876641320, -0.05778040916215522460, 0.4822834645669289988 ) ) ;
#73847=CARTESIAN_POINT ( 'NONE',  ( -1.266404199475064773, -0.2845877964562159024, 0.3641732283464567677 ) ) ;
#73848=CARTESIAN_POINT ( 'NONE',  ( 0.2362204724409456558, -0.1870078740157479769, 0.4822834645669291653 ) ) ;
#73849=CARTESIAN_POINT ( 'NONE',  ( 1.476377952755906220, 0.07958543189024071263, -0.2665933059059888421 ) ) ;
#73851=CARTESIAN_POINT ( 'NONE',  ( -1.108923884514435132, -0.2845877964562159024, 0.3641732283464567677 ) ) ;
#73852=CARTESIAN_POINT ( 'NONE',  ( 1.548556430446194954, 0.2306618581243847221, -0.2411417322834647770 ) ) ;
#73854=CARTESIAN_POINT ( 'NONE',  ( -0.2952755905511804668, 0.1660481256975885056, 0.3530559997133364547 ) ) ;
#73855=CARTESIAN_POINT ( 'NONE',  ( -1.220472440944881054, -0.5511811023622047445, 6.969142054262312111E-17 ) ) ;
#73856=CARTESIAN_POINT ( 'NONE',  ( -0.4330708661417315697, 0.1771653543307087630, 0.000000000000000000 ) ) ;
#73857=CARTESIAN_POINT ( 'NONE',  ( -0.6102362204724400829, 0.1660481256975885056, 0.3530559997133364547 ) ) ;
#73858=CARTESIAN_POINT ( 'NONE',  ( -1.437007874015747477, 0.07958543189024071263, -0.2665933059059888421 ) ) ;
#73860=CARTESIAN_POINT ( 'NONE',  ( 0.2165354330708668673, 0.1660481256975883668, -0.3530559997133364547 ) ) ;
#73861=CARTESIAN_POINT ( 'NONE',  ( 0.8785612751854029456, 3.421639014772782816E-16, 0.3464511005275203726 ) ) ;
#73863=CARTESIAN_POINT ( 'NONE',  ( -1.023622047244094002, -0.1870078740157480879, -0.4822834645669291653 ) ) ;
#73864=CARTESIAN_POINT ( 'NONE',  ( -0.6299212598425188991, -0.1870078740157479769, 0.3641732283464567677 ) ) ;
#73866=CARTESIAN_POINT ( 'NONE',  ( 0.7984992590978667870, -1.206088964116209378E-16, 0.3954974714151466841 ) ) ;
#73867=CARTESIAN_POINT ( 'NONE',  ( -0.1246719160104980823, -0.6692913385826773087, -0.1292274648535924053 ) ) ;
#73868=CARTESIAN_POINT ( 'NONE',  ( 0.5118110236220480003, -0.5511811023622047445, 6.969142054262312111E-17 ) ) ;
#73869=CARTESIAN_POINT ( 'NONE',  ( -0.8792650918635160906, -0.004921259842519870586, -0.3153832671262229437 ) ) ;
#73870=CARTESIAN_POINT ( 'NONE',  ( -1.633858267716534529, -0.5400638737290845981, -0.3530559997133363437 ) ) ;
#73871=CARTESIAN_POINT ( 'NONE',  ( -1.528871391076114250, 0.2952755905511810774, -0.1292274648535930714 ) ) ;
#73872=CARTESIAN_POINT ( 'NONE',  ( 1.364829396325460076, 0.2306618581243848609, 0.2411417322834645549 ) ) ;
#73874=CARTESIAN_POINT ( 'NONE',  ( 0.9186351706036752773, 0.1283753931104746893, -0.1820866141732285504 ) ) ;
#73875=CARTESIAN_POINT ( 'NONE',  ( 0.7217847769028878924, 0.05413385826771666132, 0.4176697321401328100 ) ) ;
#73878=CARTESIAN_POINT ( 'NONE',  ( 1.502624671916010790, -0.2845877964562161244, -0.3641732283464567121 ) ) ;
#73879=ORIENTED_EDGE ( 'NONE', *, *, #9980, .T. ) ;
#73880=CARTESIAN_POINT ( 'NONE',  ( -1.325459317585300889, 0.05413385826771666132, 0.4176697321401328100 ) ) ;
#73881=CARTESIAN_POINT ( 'NONE',  ( -0.9514435695538050464, -0.05778040916215560624, -0.4822834645669293319 ) ) ;
#73882=CARTESIAN_POINT ( 'NONE',  ( 0.2624671916010504757, -0.6046776061558809534, -0.2411417322834644161 ) ) ;
#73883=CARTESIAN_POINT ( 'NONE',  ( -1.299212598425196097, -0.5511811023622047445, 6.969142054262312111E-17 ) ) ;
#73885=CARTESIAN_POINT ( 'NONE',  ( 1.548556430446194954, -0.5023911411419708095, 0.1820866141732285504 ) ) ;
#73886=CARTESIAN_POINT ( 'NONE',  ( 0.4199475065616805614, 0.2306618581243848609, 0.2411417322834645549 ) ) ;
#73887=CARTESIAN_POINT ( 'NONE',  ( 0.7677165354330716118, -0.5400638737290844871, 0.3530559997133364547 ) ) ;
#73888=CARTESIAN_POINT ( 'NONE',  ( 1.653543307086614789, -0.1870078740157479769, 0.4822834645669291653 ) ) ;
#73894=CARTESIAN_POINT ( 'NONE',  ( 0.01312335958005323398, -0.004921259842519576551, 0.3153832671262227771 ) ) ;
#73895=CARTESIAN_POINT ( 'NONE',  ( -0.2034120734908131112, -0.6692913385826773087, -0.1292274648535924053 ) ) ;
#73896=CARTESIAN_POINT ( 'NONE',  ( 0.9120734908136489683, -0.6692913385826771977, 0.1292274648535927661 ) ) ;
#73898=CARTESIAN_POINT ( 'NONE',  ( -0.006561679790025524116, -0.08942795157528024563, -0.3641732283464568787 ) ) ;
#73899=CARTESIAN_POINT ( 'NONE',  ( -0.9842519685039360366, 0.2952755905511811885, 0.000000000000000000 ) ) ;
#73900=CARTESIAN_POINT ( 'NONE',  ( 1.128608923884514947, 0.2306618581243848609, 0.2411417322834645549 ) ) ;
#73903=PLANE ( 'NONE',  #57256 ) ;
#73906=CARTESIAN_POINT ( 'NONE',  ( 1.187664041994751285, -0.3162353388693409650, -0.4822834645669289433 ) ) ;
#73907=EDGE_CURVE ( 'NONE', #19973, #38184, #35150, .T. ) ;
#73908=CARTESIAN_POINT ( 'NONE',  ( -1.719160104986876103, 0.05413385826771666132, 0.4176697321401328100 ) ) ;
#73909=CARTESIAN_POINT ( 'NONE',  ( -1.017060367454067249, -0.08942795157527998196, 0.3641732283464567121 ) ) ;
#73910=CARTESIAN_POINT ( 'NONE',  ( -1.450131233595799651, 0.2952755905511810774, -0.1292274648535930714 ) ) ;
#73912=CARTESIAN_POINT ( 'NONE',  ( 1.192598508356890630, 4.598214627222820490E-16, 0.3791483426435169335 ) ) ;
#73913=CARTESIAN_POINT ( 'NONE',  ( 1.213910761154856299, 0.2952755905511811885, 0.1292274648535926551 ) ) ;
#73914=CARTESIAN_POINT ( 'NONE',  ( -1.450131233595799651, -0.6692913385826771977, 0.1292274648535927661 ) ) ;
#73915=CARTESIAN_POINT ( 'NONE',  ( -0.05249343832020938322, -0.6046776061558809534, -0.2411417322834644161 ) ) ;
#73916=CARTESIAN_POINT ( 'NONE',  ( -0.5052493438320203589, -0.6692913385826771977, 0.1292274648535927661 ) ) ;
#73917=CARTESIAN_POINT ( 'NONE',  ( 1.496062992125984703, -0.1870078740157480879, -0.4822834645669291653 ) ) ;
#73919=CARTESIAN_POINT ( 'NONE',  ( 0.07217847769028949700, -0.05778040916215560624, -0.4822834645669293319 ) ) ;
#73921=CARTESIAN_POINT ( 'NONE',  ( -1.443569553805773564, 0.1283753931104746893, -0.1820866141732285504 ) ) ;
#73925=CARTESIAN_POINT ( 'NONE',  ( -1.220472440944881054, 2.362204724409448620, 0.5309055118110237448 ) ) ;
#73926=CARTESIAN_POINT ( 'NONE',  ( -1.391076115485563758, 0.2306618581243848609, 0.2411417322834645549 ) ) ;
#73930=CARTESIAN_POINT ( 'NONE',  ( -0.9564677561141805562, 0.02791078216816347476, -0.4328096321851898631 ) ) ;
#73931=DIRECTION ( 'NONE',  ( 1.000000000000000000, 0.000000000000000000, 0.000000000000000000 ) ) ;
#73933=CARTESIAN_POINT ( 'NONE',  ( -0.2165354330708654795, 0.07958543189024085140, 0.2665933059059887866 ) ) ;
#73934=CARTESIAN_POINT ( 'NONE',  ( -0.7611548556430438595, 0.1283753931104748280, 0.1820866141732283561 ) ) ;
#73935=CARTESIAN_POINT ( 'NONE',  ( -1.122047244094487306, 0.1660481256975883668, -0.3530559997133364547 ) ) ;
#73936=CARTESIAN_POINT ( 'NONE',  ( 0.4461942257217855201, -0.6046776061558807314, 0.2411417322834647770 ) ) ;
#73937=CARTESIAN_POINT ( 'NONE',  ( -1.463254593175852492, 0.2952755905511811885, 0.1292274648535926551 ) ) ;
#73939=VERTEX_POINT ( 'NONE', #54999 ) ;
#73940=CARTESIAN_POINT ( 'NONE',  ( -1.476377952755905110, 0.1660481256975885056, 0.3530559997133364547 ) ) ;
#73941=CARTESIAN_POINT ( 'NONE',  ( -1.614173228346456712, 2.094556775020298467, -0.1372047244094478091 ) ) ;
#73943=CARTESIAN_POINT ( 'NONE',  ( 2.795275590551181910, 1.488513638086842006, 0.000000000000000000 ) ) ;
#73945=CARTESIAN_POINT ( 'NONE',  ( 1.614173228346456712, 2.401574803149606474, -0.5309055118110239668 ) ) ;
#73946=CARTESIAN_POINT ( 'NONE',  ( -0.5905511811023613777, -0.6692913385826771977, 8.415575281601705876E-17 ) ) ;
#73947=CARTESIAN_POINT ( 'NONE',  ( 1.351706036745407680, 0.05413385826771666132, 0.4176697321401328100 ) ) ;
#73948=DIRECTION ( 'NONE',  ( -0.000000000000000000, 1.000000000000000000, -0.000000000000000000 ) ) ;
#73950=CARTESIAN_POINT ( 'NONE',  ( -1.541994750656167090, 0.2952755905511811885, 0.1292274648535926551 ) ) ;
#73951=CARTESIAN_POINT ( 'NONE',  ( -0.8267716535433065062, -0.6692913385826771977, 8.415575281601705876E-17 ) ) ;
#73953=CARTESIAN_POINT ( 'NONE',  ( -0.03937007874015669567, -0.5511811023622047445, 6.969142054262312111E-17 ) ) ;
#73955=CARTESIAN_POINT ( 'NONE',  ( -0.2821522309711278487, -0.5511811023622048555, -0.09757992244046775898 ) ) ;
#73956=CARTESIAN_POINT ( 'NONE',  ( 1.003937007874016185, 0.07958543189024071263, -0.2665933059059888421 ) ) ;
#73957=CARTESIAN_POINT ( 'NONE',  ( 0.8267716535433077274, 0.2952755905511811885, 0.000000000000000000 ) ) ;
#73958=UNCERTAINTY_MEASURE_WITH_UNIT (LENGTH_MEASURE( 1.000000000000000082E-05 ), #215, 'distance_accuracy_value', 'NONE');
#73959=CARTESIAN_POINT ( 'NONE',  ( -0.3280839895013117347, -0.004921259842519870586, -0.3153832671262229437 ) ) ;
#73961=CARTESIAN_POINT ( 'NONE',  ( -1.535433070866141225, -0.6692913385826771977, 8.415575281601705876E-17 ) ) ;
#73962=CARTESIAN_POINT ( 'NONE',  ( -1.410761154855641575, -0.2845877964562161244, -0.3641732283464567121 ) ) ;
#73964=CARTESIAN_POINT ( 'NONE',  ( 0.2559055118110243332, -0.5400638737290845981, -0.3530559997133363437 ) ) ;
#73966=CARTESIAN_POINT ( 'NONE',  ( -0.08530183727034056085, -0.3162353388693405765, 0.4822834645669290543 ) ) ;
#73967=CARTESIAN_POINT ( 'NONE',  ( 1.476377952755906442, -0.4536011799217367080, 0.2665933059059888421 ) ) ;
#73968=CARTESIAN_POINT ( 'NONE',  ( 0.6561679790026253567, 0.1283753931104748280, 0.1820866141732283561 ) ) ;
#73969=CARTESIAN_POINT ( 'NONE',  ( -0.2559055118110230564, 0.07958543189024071263, -0.2665933059059888421 ) ) ;
#73970=CARTESIAN_POINT ( 'NONE',  ( -0.7874015748031489847, -0.1870078740157480879, -0.4822834645669291653 ) ) ;
#73971=CARTESIAN_POINT ( 'NONE',  ( -1.586052503253845503, 2.125984251968505045, 0.1653254495020588799 ) ) ;
#73972=DIRECTION ( 'NONE',  ( 0.000000000000000000, 0.000000000000000000, 1.000000000000000000 ) ) ;
#73973=CARTESIAN_POINT ( 'NONE',  ( 0.2559055118110243332, 0.1660481256975885056, 0.3530559997133364547 ) ) ;
#73976=CARTESIAN_POINT ( 'NONE',  ( -0.08530183727034056085, -0.08942795157528024563, -0.3641732283464568787 ) ) ;
#73977=CARTESIAN_POINT ( 'NONE',  ( -0.1771653543307080136, -0.5400638737290844871, 0.3530559997133364547 ) ) ;
#73978=LINE ( 'NONE', #16324, #20951 ) ;
#73979=CARTESIAN_POINT ( 'NONE',  ( 1.528871391076116026, 0.2952755905511811885, 0.1292274648535926551 ) ) ;
#73980=CARTESIAN_POINT ( 'NONE',  ( 1.410761154855643795, -0.05778040916215560624, -0.4822834645669293319 ) ) ;
#73982=CARTESIAN_POINT ( 'NONE',  ( -0.7086614173228339419, -0.1870078740157480601, -0.3641732283464567677 ) ) ;
#73987=FACE_OUTER_BOUND ( 'NONE', #81908, .T. ) ;
#73988=CARTESIAN_POINT ( 'NONE',  ( 1.227034120734908917, -0.5511811023622046335, 0.09757992244046803654 ) ) ;
#73989=CARTESIAN_POINT ( 'NONE',  ( -1.509186351706035767, 0.05413385826771626580, -0.4176697321401330321 ) ) ;
#73990=CARTESIAN_POINT ( 'NONE',  ( 0.9448818897637802916, -0.1870078740157479769, 0.4822834645669291653 ) ) ;
#73992=CARTESIAN_POINT ( 'NONE',  ( 1.030183727034121421, -0.08942795157527998196, 0.3641732283464567121 ) ) ;
#73993=CARTESIAN_POINT ( 'NONE',  ( 0.1640419947506569498, -0.3162353388693409650, -0.4822834645669289433 ) ) ;
#73994=CARTESIAN_POINT ( 'NONE',  ( -1.017060367454067249, -0.05778040916215522460, 0.4822834645669289988 ) ) ;
#73995=CARTESIAN_POINT ( 'NONE',  ( 1.633858267716535639, -0.5400638737290844871, 0.3530559997133364547 ) ) ;
#73998=CARTESIAN_POINT ( 'NONE',  ( 0.2755905511811031494, -0.5511811023622047445, 6.969142054262312111E-17 ) ) ;
#74002=CARTESIAN_POINT ( 'NONE',  ( -0.2952755905511804668, 0.1660481256975885056, 0.3530559997133364547 ) ) ;
#74003=CARTESIAN_POINT ( 'NONE',  ( 0.01312335958005323398, -0.4281496062992127816, -0.4176697321401328100 ) ) ;
#74004=CARTESIAN_POINT ( 'NONE',  ( -0.2821522309711278487, -0.5511811023622048555, -0.09757992244046775898 ) ) ;
#74005=CARTESIAN_POINT ( 'NONE',  ( 0.6955380577427828781, -0.4281496062992124485, 0.4176697321401328655 ) ) ;
#74006=CARTESIAN_POINT ( 'NONE',  ( -0.7808398950131222316, -0.3162353388693409650, -0.4822834645669289433 ) ) ;
#74007=CARTESIAN_POINT ( 'NONE',  ( -0.3412073490813641308, -0.6046776061558807314, 0.2411417322834647770 ) ) ;
#74008=CARTESIAN_POINT ( 'NONE',  ( 0.9973753280839902091, 0.2306618581243847221, -0.2411417322834647770 ) ) ;
#74009=CARTESIAN_POINT ( 'NONE',  ( 0.9186351706036751663, -0.6046776061558807314, 0.2411417322834647770 ) ) ;
#74010=CARTESIAN_POINT ( 'NONE',  ( 0.9317585301837276734, 0.05413385826771626580, -0.4176697321401330321 ) ) ;
#74012=CARTESIAN_POINT ( 'NONE',  ( 0.01312335958005323398, -0.3690944881889765550, -0.3153832671262227771 ) ) ;
#74013=ORIENTED_EDGE ( 'NONE', *, *, #27995, .T. ) ;
#74016=CARTESIAN_POINT ( 'NONE',  ( -1.023622047244094002, -0.1870078740157480601, -0.3641732283464567677 ) ) ;
#74017=CARTESIAN_POINT ( 'NONE',  ( -0.2821522309711278487, -0.6692913385826773087, -0.1292274648535924053 ) ) ;
#74019=CARTESIAN_POINT ( 'NONE',  ( -0.5774278215223089816, 0.2306618581243847221, -0.2411417322834647770 ) ) ;
#74020=CARTESIAN_POINT ( 'NONE',  ( -0.4593175853018366950, 0.05413385826771666132, 0.4176697321401328100 ) ) ;
#74021=CARTESIAN_POINT ( 'NONE',  ( -1.266404199475064773, -0.05778040916215560624, -0.4822834645669293319 ) ) ;
#74022=CARTESIAN_POINT ( 'NONE',  ( -1.620734908136482577, -0.6692913385826773087, -0.1292274648535924053 ) ) ;
#74023=CARTESIAN_POINT ( 'NONE',  ( 1.003937007874016407, -0.4536011799217367080, 0.2665933059059888421 ) ) ;
#74026=CARTESIAN_POINT ( 'NONE',  ( 0.4986876640419954376, 0.1283753931104748280, 0.1820866141732283561 ) ) ;
#74027=CARTESIAN_POINT ( 'NONE',  ( -0.09842519685039295696, -0.5400638737290844871, 0.3530559997133364547 ) ) ;
#74028=CARTESIAN_POINT ( 'NONE',  ( 0.2755905511811031494, 0.2952755905511811885, 0.000000000000000000 ) ) ;
#74032=ORIENTED_EDGE ( 'NONE', *, *, #79270, .F. ) ;
#74034=CARTESIAN_POINT ( 'NONE',  ( 1.535433070866142335, -0.6692913385826771977, 8.415575281601705876E-17 ) ) ;
#74035=CARTESIAN_POINT ( 'NONE',  ( -0.8202099737532801971, -0.5511811023622046335, 0.09757992244046803654 ) ) ;
#74036=CARTESIAN_POINT ( 'NONE',  ( -0.9514435695538050464, -0.3162353388693405765, 0.4822834645669290543 ) ) ;
#74039=CARTESIAN_POINT ( 'NONE',  ( 1.522309711286089939, 0.2306618581243848609, 0.2411417322834645549 ) ) ;
#74040=CARTESIAN_POINT ( 'NONE',  ( 0.5905511811023629321, -0.6692913385826771977, 8.415575281601705876E-17 ) ) ;
#74041=CARTESIAN_POINT ( 'NONE',  ( 0.6824146981627303710, -0.6046776061558807314, 0.2411417322834647770 ) ) ;
#74042=CARTESIAN_POINT ( 'NONE',  ( -0.5971128608923877978, -0.5511811023622048555, -0.09757992244046775898 ) ) ;
#74043=CARTESIAN_POINT ( 'NONE',  ( 0.09186351706036799403, -0.4281496062992127816, -0.4176697321401328100 ) ) ;
#74045=CARTESIAN_POINT ( 'NONE',  ( -0.4593175853018364174, -0.3690944881889765550, -0.3153832671262227771 ) ) ;
#74046=CARTESIAN_POINT ( 'NONE',  ( -0.3543307086614165824, -0.6692913385826771977, 8.415575281601705876E-17 ) ) ;
#74048=CARTESIAN_POINT ( 'NONE',  ( -1.541994750656167090, 0.2952755905511811885, 0.1292274648535926551 ) ) ;
#74049=CARTESIAN_POINT ( 'NONE',  ( 0.05249343832021075018, 0.1283753931104746893, -0.1820866141732285504 ) ) ;
#74050=CARTESIAN_POINT ( 'NONE',  ( 1.358267716535433323, 0.07958543189024085140, 0.2665933059059887866 ) ) ;
#74051=CARTESIAN_POINT ( 'NONE',  ( -1.023622047244094002, -0.1870078740157480879, -0.4822834645669291653 ) ) ;
#74053=CARTESIAN_POINT ( 'NONE',  ( -0.8530183727034112984, -0.004921259842519576551, 0.3153832671262227771 ) ) ;
#74055=CARTESIAN_POINT ( 'NONE',  ( -1.135170603674539924, -0.6692913385826771977, 0.1292274648535927661 ) ) ;
#74056=CARTESIAN_POINT ( 'NONE',  ( -0.2887139107611542133, -0.6046776061558809534, -0.2411417322834644161 ) ) ;
#74058=CARTESIAN_POINT ( 'NONE',  ( 0.3477690288713918276, -0.6692913385826773087, -0.1292274648535924053 ) ) ;
#74061=CARTESIAN_POINT ( 'NONE',  ( 0.4396325459317593221, 0.1771653543307087075, -0.09757992244046823083 ) ) ;
#74062=CARTESIAN_POINT ( 'NONE',  ( 1.115485564304462551, 0.05413385826771666132, 0.4176697321401328100 ) ) ;
#74063=CARTESIAN_POINT ( 'NONE',  ( -1.089238845144356427, -0.004921259842519576551, 0.3153832671262227771 ) ) ;
#74064=CARTESIAN_POINT ( 'NONE',  ( 1.240157480314961314, 0.1660481256975883668, -0.3530559997133364547 ) ) ;
#74065=CARTESIAN_POINT ( 'NONE',  ( -1.646981627296586703, -0.2845877964562161244, -0.3641732283464567121 ) ) ;
#74066=CARTESIAN_POINT ( 'NONE',  ( -1.515748031496062076, 0.1660481256975883668, -0.3530559997133364547 ) ) ;
#74067=CARTESIAN_POINT ( 'NONE',  ( -0.8858267716535425107, 0.1660481256975883668, -0.3530559997133364547 ) ) ;
#74068=CARTESIAN_POINT ( 'NONE',  ( 0.08530183727034192087, -0.08942795157527998196, 0.3641732283464567121 ) ) ;
#74069=CARTESIAN_POINT ( 'NONE',  ( -0.8776378784356294593, 5.410171027439680070E-15, -0.3791483426435165449 ) ) ;
#74070=CARTESIAN_POINT ( 'NONE',  ( 0.6299212598425204535, -0.1870078740157479769, 0.3641732283464567677 ) ) ;
#74072=CARTESIAN_POINT ( 'NONE',  ( -0.1377952755905504645, -0.5400638737290845981, -0.3530559997133363437 ) ) ;
#74074=CARTESIAN_POINT ( 'NONE',  ( -1.003937007874015297, -0.5400638737290845981, -0.3530559997133363437 ) ) ;
#74076=CARTESIAN_POINT ( 'NONE',  ( 1.102362204724410155, -0.1870078740157479769, 0.3641732283464567677 ) ) ;
#74077=CARTESIAN_POINT ( 'NONE',  ( 0.1640419947506569498, -0.3162353388693409650, -0.4822834645669289433 ) ) ;
#74078=CARTESIAN_POINT ( 'NONE',  ( -0.4461942257217840213, -0.6046776061558809534, -0.2411417322834644161 ) ) ;
#74079=CARTESIAN_POINT ( 'NONE',  ( -0.5249343832020990641, 0.1283753931104748280, 0.1820866141732283561 ) ) ;
#74081=CARTESIAN_POINT ( 'NONE',  ( -0.3608923884514428360, 0.1771653543307087630, 0.09757992244046791164 ) ) ;
#74082=CARTESIAN_POINT ( 'NONE',  ( 0.4199475065616805614, 0.2306618581243848609, 0.2411417322834645549 ) ) ;
#74083=CARTESIAN_POINT ( 'NONE',  ( -1.056430446194224881, 0.1771653543307087075, -0.09757992244046823083 ) ) ;
#74085=CARTESIAN_POINT ( 'NONE',  ( -1.299212598425196097, 0.2952755905511811885, 0.000000000000000000 ) ) ;
#74086=CARTESIAN_POINT ( 'NONE',  ( 0.2238009295390077091, 2.409604939980833412E-17, -0.3464511005275205946 ) ) ;
#74087=VERTEX_POINT ( 'NONE', #69708 ) ;
#74088=CARTESIAN_POINT ( 'NONE',  ( -1.607611548556429737, -0.5511811023622046335, 0.09757992244046803654 ) ) ;
#74089=CARTESIAN_POINT ( 'NONE',  ( -0.6102362204724400829, 0.1660481256975885056, 0.3530559997133364547 ) ) ;
#74092=CARTESIAN_POINT ( 'NONE',  ( -1.043307086614172041, -0.5400638737290844871, 0.3530559997133364547 ) ) ;
#74095=CARTESIAN_POINT ( 'NONE',  ( 1.417322834645670104, -0.1870078740157480879, -0.4822834645669291653 ) ) ;
#74096=CARTESIAN_POINT ( 'NONE',  ( 0.3740157480314966754, -0.5400638737290844871, 0.3530559997133364547 ) ) ;
#74099=CARTESIAN_POINT ( 'NONE',  ( -1.679790026246718693, 0.2306618581243847221, -0.2411417322834647770 ) ) ;
#74102=CARTESIAN_POINT ( 'NONE',  ( -0.9842519685039360366, 0.1771653543307087630, 0.000000000000000000 ) ) ;
#74105=CARTESIAN_POINT ( 'NONE',  ( 0.6167979002624678353, -0.4281496062992124485, 0.4176697321401328655 ) ) ;
#74106=CARTESIAN_POINT ( 'NONE',  ( -0.4658792650918627265, -0.05778040916215522460, 0.4822834645669289988 ) ) ;
#74107=CARTESIAN_POINT ( 'NONE',  ( -0.9580052493438311334, 0.05413385826771626580, -0.4176697321401330321 ) ) ;
#74108=CARTESIAN_POINT ( 'NONE',  ( 1.220472440944882608, 0.2952755905511811885, 0.000000000000000000 ) ) ;
#74109=CARTESIAN_POINT ( 'NONE',  ( -1.233595800524933894, -0.5023911411419708095, -0.1820866141732282451 ) ) ;
#74111=CARTESIAN_POINT ( 'NONE',  ( 0.4790026246719168435, -0.3162353388693409650, -0.4822834645669289433 ) ) ;
#74112=CARTESIAN_POINT ( 'NONE',  ( -0.8136482939632537770, 0.2306618581243847221, -0.2411417322834647770 ) ) ;
#74114=CARTESIAN_POINT ( 'NONE',  ( -1.430446194225720724, 0.05413385826771626580, -0.4176697321401330321 ) ) ;
#74116=CARTESIAN_POINT ( 'NONE',  ( 0.8005249343832028242, -0.4281496062992127816, -0.4176697321401328100 ) ) ;
#74118=CARTESIAN_POINT ( 'NONE',  ( 1.476377952755906442, -0.4536011799217367080, 0.2665933059059888421 ) ) ;
#74119=ORIENTED_EDGE ( 'NONE', *, *, #54784, .T. ) ;
#74121=CARTESIAN_POINT ( 'NONE',  ( -0.6036745406824141069, -0.6046776061558809534, -0.2411417322834644161 ) ) ;
#74122=ORIENTED_EDGE ( 'NONE', *, *, #12573, .T. ) ;
#74123=CARTESIAN_POINT ( 'NONE',  ( 0.5314960629921264834, 0.07958543189024071263, -0.2665933059059888421 ) ) ;
#74124=CARTESIAN_POINT ( 'NONE',  ( -1.450131233595799651, -0.6692913385826771977, 0.1292274648535927661 ) ) ;
#74125=CARTESIAN_POINT ( 'NONE',  ( 1.174540682414699111, -0.05778040916215560624, -0.4822834645669293319 ) ) ;
#74126=CARTESIAN_POINT ( 'NONE',  ( 0.8070866141732288002, 0.1660481256975885056, 0.3530559997133364547 ) ) ;
#74127=( BOUNDED_CURVE ( )  B_SPLINE_CURVE ( 2, ( #79576, #66943, #68182, #17258, #54281, #16015, #61437, #67352, #49208, #55106, #34946, #73248, #80410 ),
 .UNSPECIFIED., .F., .F. ) 
 B_SPLINE_CURVE_WITH_KNOTS ( ( 3, 2, 2, 2, 2, 2, 3 ),
 ( 0.7763059932978690902, 0.7765151515151516026, 0.7803030303030302761, 0.7840909090909091717, 0.7878787878787878451, 0.7916666666666667407, 0.7918758248839492531 ),
 .UNSPECIFIED. ) 
 CURVE ( )  GEOMETRIC_REPRESENTATION_ITEM ( )  RATIONAL_B_SPLINE_CURVE ( ( 0.9964447847208420805, 0.9981185001348091834, 1.000000000000000000, 0.9659258262890683122, 1.000000000000000000, 0.9659258262890683122, 1.000000000000000000, 0.9659258262890683122, 1.000000000000000000, 0.9659258262890683122, 1.000000000000000000, 0.9981185001348091834, 0.9964447847208420805 ) ) 
 REPRESENTATION_ITEM ( '' )  );
#74128=CARTESIAN_POINT ( 'NONE',  ( 0.01968503937007930540, 0.1660481256975885056, 0.3530559997133364547 ) ) ;
#74130=CARTESIAN_POINT ( 'NONE',  ( -0.8792650918635160906, -0.4281496062992124485, 0.4176697321401328655 ) ) ;
#74132=CARTESIAN_POINT ( 'NONE',  ( -1.594488188976377563, -0.5400638737290844871, 0.3530559997133364547 ) ) ;
#74133=CARTESIAN_POINT ( 'NONE',  ( -0.9908136482939626788, 0.2952755905511811885, 0.1292274648535926551 ) ) ;
#74134=CARTESIAN_POINT ( 'NONE',  ( 1.502624671916010790, -0.05778040916215522460, 0.4822834645669289988 ) ) ;
#74136=CARTESIAN_POINT ( 'NONE',  ( 1.686351706036745890, 0.2952755905511811885, 0.1292274648535926551 ) ) ;
#74137=CARTESIAN_POINT ( 'NONE',  ( -0.7545931758530177724, 0.2952755905511811885, 0.1292274648535926551 ) ) ;
#74139=CARTESIAN_POINT ( 'NONE',  ( 0.4658792650918640033, -0.3162353388693405765, 0.4822834645669290543 ) ) ;
#74141=CARTESIAN_POINT ( 'NONE',  ( -0.6299212598425188991, -0.1870078740157480879, -0.4822834645669291653 ) ) ;
#74142=CARTESIAN_POINT ( 'NONE',  ( -1.404199475065615932, -0.3690944881889765550, -0.3153832671262227771 ) ) ;
#74143=CARTESIAN_POINT ( 'NONE',  ( 0.6561679790026253567, -0.5023911411419708095, -0.1820866141732282451 ) ) ;
#74144=CARTESIAN_POINT ( 'NONE',  ( 1.489501312335958172, -0.05778040916215560624, -0.4822834645669293319 ) ) ;
#74146=CARTESIAN_POINT ( 'NONE',  ( 0.7414698162729663755, 0.1771653543307087630, 0.09757992244046791164 ) ) ;
#74147=CARTESIAN_POINT ( 'NONE',  ( 0.6036745406824153282, -0.6046776061558807314, 0.2411417322834647770 ) ) ;
#74149=CARTESIAN_POINT ( 'NONE',  ( -0.3805774278215216522, -0.4281496062992127816, -0.4176697321401328100 ) ) ;
#74151=CARTESIAN_POINT ( 'NONE',  ( 1.404199475065617264, -0.3690944881889763329, 0.3153832671262228327 ) ) ;
#74152=CARTESIAN_POINT ( 'NONE',  ( -0.6955380577427815458, -0.4281496062992127816, -0.4176697321401328100 ) ) ;
#74154=CARTESIAN_POINT ( 'NONE',  ( 1.246719160104987623, 0.05413385826771626580, -0.4176697321401330321 ) ) ;
#74155=CARTESIAN_POINT ( 'NONE',  ( 0.1574803149606306130, -0.1870078740157479769, 0.4822834645669291653 ) ) ;
#74156=CARTESIAN_POINT ( 'NONE',  ( 0.7349081364829403995, 0.1283753931104748280, 0.1820866141732283561 ) ) ;
#74157=CARTESIAN_POINT ( 'NONE',  ( 0.8533690079452093125, 0.004960608223778500969, -0.3437734562760191848 ) ) ;
#74158=CARTESIAN_POINT ( 'NONE',  ( -0.1312335958005241554, -0.5023911411419708095, -0.1820866141732282451 ) ) ;
#74159=CARTESIAN_POINT ( 'NONE',  ( 0.7349081364829402885, -0.5023911411419708095, -0.1820866141732282451 ) ) ;
#74160=CARTESIAN_POINT ( 'NONE',  ( -1.535433070866141225, -0.6692913385826771977, 8.415575281601705876E-17 ) ) ;
#74162=CARTESIAN_POINT ( 'NONE',  ( 0.8136482939632553313, -0.6046776061558809534, -0.2411417322834644161 ) ) ;
#74163=EDGE_CURVE ( 'NONE', #62837, #52448, #38109, .T. ) ;
#74165=CARTESIAN_POINT ( 'NONE',  ( 1.568241469816273659, -0.08942795157528024563, -0.3641732283464568787 ) ) ;
#74166=CARTESIAN_POINT ( 'NONE',  ( 0.1458944486102289051, 0.02791078216816508459, -0.4328096321851889194 ) ) ;
#74167=CARTESIAN_POINT ( 'NONE',  ( -0.1837270341207343505, -0.5023911411419708095, 0.1820866141732285504 ) ) ;
#74168=CARTESIAN_POINT ( 'NONE',  ( 0.05905511811023709395, -0.5400638737290844871, 0.3530559997133364547 ) ) ;
#74169=CARTESIAN_POINT ( 'NONE',  ( 1.568241469816273659, -0.08942795157528024563, -0.3641732283464568787 ) ) ;
#74170=CARTESIAN_POINT ( 'NONE',  ( -1.200787401574802349, 0.07958543189024071263, -0.2665933059059888421 ) ) ;
#74171=CARTESIAN_POINT ( 'NONE',  ( -1.561679790026246017, 0.05413385826771666132, 0.4176697321401328100 ) ) ;
#74173=CARTESIAN_POINT ( 'NONE',  ( 0.4133858267716541968, 0.1660481256975885056, 0.3530559997133364547 ) ) ;
#74174=CARTESIAN_POINT ( 'NONE',  ( 1.187664041994751285, -0.05778040916215522460, 0.4822834645669289988 ) ) ;
#74176=CARTESIAN_POINT ( 'NONE',  ( -0.006561679790025524116, -0.3162353388693405765, 0.4822834645669290543 ) ) ;
#74177=CARTESIAN_POINT ( 'NONE',  ( 1.456692913385827515, -0.6692913385826771977, 8.415575281601705876E-17 ) ) ;
#74178=CARTESIAN_POINT ( 'NONE',  ( 0.9711286089238851948, -0.6046776061558809534, -0.2411417322834644161 ) ) ;
#74180=CARTESIAN_POINT ( 'NONE',  ( 0.9776902887139113929, -0.5511811023622048555, -0.09757992244046775898 ) ) ;
#74181=CARTESIAN_POINT ( 'NONE',  ( 1.646981627296588035, -0.3162353388693405765, 0.4822834645669290543 ) ) ;
#74182=CARTESIAN_POINT ( 'NONE',  ( 0.03937007874015806264, 0.1771653543307087630, 0.000000000000000000 ) ) ;
#74183=CARTESIAN_POINT ( 'NONE',  ( 0.1509186351706045259, -0.05778040916215560624, -0.4822834645669293319 ) ) ;
#74184=CARTESIAN_POINT ( 'NONE',  ( 0.8267716535433077274, 0.2952755905511811885, 0.000000000000000000 ) ) ;
#74185=CARTESIAN_POINT ( 'NONE',  ( -0.4133858267716528645, -0.5400638737290844871, 0.3530559997133364547 ) ) ;
#74187=CARTESIAN_POINT ( 'NONE',  ( -0.1902887139107604098, -0.5511811023622046335, 0.09757992244046803654 ) ) ;
#74188=CARTESIAN_POINT ( 'NONE',  ( 0.6561679790026253567, 0.2306618581243848609, 0.2411417322834645549 ) ) ;
#74189=CARTESIAN_POINT ( 'NONE',  ( 0.7677165354330716118, 0.07958543189024071263, -0.2665933059059888421 ) ) ;
#74191=CARTESIAN_POINT ( 'NONE',  ( -1.056430446194224881, 0.2952755905511810219, -0.1292274648535930437 ) ) ;
#74194=CARTESIAN_POINT ( 'NONE',  ( -1.318897637795274802, 0.1660481256975885056, 0.3530559997133364547 ) ) ;
#74195=CARTESIAN_POINT ( 'NONE',  ( -0.3346456692913377662, -0.5400638737290844871, 0.3530559997133364547 ) ) ;
#74199=CARTESIAN_POINT ( 'NONE',  ( 0.5905511811023629321, 0.1771653543307087630, 0.000000000000000000 ) ) ;
#74201=CARTESIAN_POINT ( 'NONE',  ( 1.286089238845145033, 0.2306618581243848609, 0.2411417322834645549 ) ) ;
#74203=CARTESIAN_POINT ( 'NONE',  ( 0.4935044252197980930, 1.488513638086841118, 0.5309055118110234117 ) ) ;
#74204=CARTESIAN_POINT ( 'NONE',  ( -1.482939632545930975, -0.3690944881889765550, -0.3153832671262227771 ) ) ;
#74205=CARTESIAN_POINT ( 'NONE',  ( 1.633858267716535639, -0.5400638737290844871, 0.3530559997133364547 ) ) ;
#74206=CARTESIAN_POINT ( 'NONE',  ( 1.443569553805774897, 0.1283753931104748280, 0.1820866141732283561 ) ) ;
#74207=CARTESIAN_POINT ( 'NONE',  ( 0.5708661417322842269, 0.1660481256975885056, 0.3530559997133364547 ) ) ;
#74210=CARTESIAN_POINT ( 'NONE',  ( 0.09186351706036827158, 0.05413385826771666132, 0.4176697321401328100 ) ) ;
#74211=CARTESIAN_POINT ( 'NONE',  ( -1.003937007874015297, -0.4536011799217368745, -0.2665933059059886201 ) ) ;
#74213=CARTESIAN_POINT ( 'NONE',  ( 0.3280839895013130669, 0.05413385826771666132, 0.4176697321401328100 ) ) ;
#74214=CARTESIAN_POINT ( 'NONE',  ( -0.1640419947506555343, -0.3162353388693405765, 0.4822834645669290543 ) ) ;
#74215=CARTESIAN_POINT ( 'NONE',  ( 0.5380577427821529035, 0.05413385826771626580, -0.4176697321401330321 ) ) ;
#74216=CARTESIAN_POINT ( 'NONE',  ( -0.01000891935578489267, 8.471767977567108961E-16, -0.4445507791589058955 ) ) ;
#74218=CARTESIAN_POINT ( 'NONE',  ( 0.9448818897637802916, -0.1870078740157480879, -0.4822834645669291653 ) ) ;
#74219=CARTESIAN_POINT ( 'NONE',  ( -0.3018372703412066094, 0.05413385826771666132, 0.4176697321401328100 ) ) ;
#74220=CARTESIAN_POINT ( 'NONE',  ( -1.056430446194224881, -0.6692913385826771977, 0.1292274648535927661 ) ) ;
#74221=CARTESIAN_POINT ( 'NONE',  ( 1.227034120734908917, -0.6692913385826771977, 0.1292274648535927661 ) ) ;
#74222=CARTESIAN_POINT ( 'NONE',  ( 0.5577427821522316087, -0.05778040916215522460, 0.4822834645669289988 ) ) ;
#74224=CARTESIAN_POINT ( 'NONE',  ( -0.1902887139107604098, -0.6692913385826771977, 0.1292274648535927661 ) ) ;
#74225=CARTESIAN_POINT ( 'NONE',  ( 0.2821522309711292364, 0.2952755905511810774, -0.1292274648535930714 ) ) ;
#74226=CARTESIAN_POINT ( 'NONE',  ( -0.6561679790026240244, 0.2306618581243847221, -0.2411417322834647770 ) ) ;
#74227=CARTESIAN_POINT ( 'NONE',  ( 0.8858267716535438430, 0.07958543189024085140, 0.2665933059059887866 ) ) ;
#74228=CARTESIAN_POINT ( 'NONE',  ( -1.614173228346456268, -0.6692913385826771977, 8.415575281601705876E-17 ) ) ;
#74230=CARTESIAN_POINT ( 'NONE',  ( 0.3805774278215230400, 0.05413385826771626580, -0.4176697321401330321 ) ) ;
#74234=VERTEX_POINT ( 'NONE', #44014 ) ;
#74235=ORIENTED_EDGE ( 'NONE', *, *, #14670, .T. ) ;
#74236=CARTESIAN_POINT ( 'NONE',  ( 0.7808398950131241190, -0.05778040916215560624, -0.4822834645669293319 ) ) ;
#74237=CARTESIAN_POINT ( 'NONE',  ( 0.5118110236220478892, 0.1771653543307087630, 0.000000000000000000 ) ) ;
#74245=CARTESIAN_POINT ( 'NONE',  ( 1.017060367454068581, -0.05778040916215560624, -0.4822834645669293319 ) ) ;
#74246=CARTESIAN_POINT ( 'NONE',  ( -0.6955380577427815458, 0.05413385826771666132, 0.4176697321401328100 ) ) ;
#74247=CARTESIAN_POINT ( 'NONE',  ( -0.6692913385826764205, -0.6692913385826771977, 8.415575281601705876E-17 ) ) ;
#74248=CARTESIAN_POINT ( 'NONE',  ( 0.8070866141732288002, 0.1660481256975885056, 0.3530559997133364547 ) ) ;
#74249=CARTESIAN_POINT ( 'NONE',  ( 1.377952755905512472, -0.6692913385826771977, 8.415575281601705876E-17 ) ) ;
#74252=CARTESIAN_POINT ( 'NONE',  ( 1.312335958005250269, -0.5023911411419708095, 0.1820866141732285504 ) ) ;
#74254=CARTESIAN_POINT ( 'NONE',  ( -1.207349081364828436, -0.5023911411419708095, 0.1820866141732285504 ) ) ;
#74255=( BOUNDED_CURVE ( )  B_SPLINE_CURVE ( 1, ( #35165, #35994 ),
 .UNSPECIFIED., .F., .F. ) 
 B_SPLINE_CURVE_WITH_KNOTS ( ( 2, 2 ),
 ( 3.469446951953614189E-18, 0.002000000000000005246 ),
 .UNSPECIFIED. ) 
 CURVE ( )  GEOMETRIC_REPRESENTATION_ITEM ( )  RATIONAL_B_SPLINE_CURVE ( ( 0.9875488213027523443, 0.9875488213027523443 ) ) 
 REPRESENTATION_ITEM ( '' )  );
#74257=CARTESIAN_POINT ( 'NONE',  ( -0.01312335958005186876, 0.05413385826771626580, -0.4176697321401330321 ) ) ;
#74259=PLANE ( 'NONE',  #38526 ) ;
#74260=CARTESIAN_POINT ( 'NONE',  ( -0.9842519685039365918, -0.5511811023622047445, 6.969142054262312111E-17 ) ) ;
#74261=CARTESIAN_POINT ( 'NONE',  ( 0.2099737532808405305, -0.6046776061558807314, 0.2411417322834647770 ) ) ;
#74262=CARTESIAN_POINT ( 'NONE',  ( 1.115485564304462551, -0.004921259842519576551, 0.3153832671262227771 ) ) ;
#74264=CARTESIAN_POINT ( 'NONE',  ( -1.128608923884513837, -0.5023911411419708095, 0.1820866141732285504 ) ) ;
#74265=CARTESIAN_POINT ( 'NONE',  ( 1.371391076115485941, 0.2952755905511811885, 0.1292274648535926551 ) ) ;
#74267=CARTESIAN_POINT ( 'NONE',  ( -0.3215223097112853146, -0.3162353388693405765, 0.4822834645669290543 ) ) ;
#74268=CARTESIAN_POINT ( 'NONE',  ( -1.384514435695537005, -0.5511811023622048555, -0.09757992244046775898 ) ) ;
#74269=CARTESIAN_POINT ( 'NONE',  ( -0.5577427821522301654, -0.05778040916215560624, -0.4822834645669293319 ) ) ;
#74270=CARTESIAN_POINT ( 'NONE',  ( 1.666666666666667185, 0.05413385826771666132, 0.4176697321401328100 ) ) ;
#74272=CARTESIAN_POINT ( 'NONE',  ( 0.4724409448818904789, -0.1870078740157479769, 0.4822834645669291653 ) ) ;
#74274=CARTESIAN_POINT ( 'NONE',  ( 1.227034120734908917, -0.6692913385826771977, 0.1292274648535927661 ) ) ;
#74276=CARTESIAN_POINT ( 'NONE',  ( -1.148293963254592542, -0.6692913385826773087, -0.1292274648535924053 ) ) ;
#74277=CARTESIAN_POINT ( 'NONE',  ( -0.7480314960629914633, 0.1771653543307087630, 0.000000000000000000 ) ) ;
#74278=CARTESIAN_POINT ( 'NONE',  ( 0.7974104941589355011, -4.927456884911482678E-16, 0.4445507791589062840 ) ) ;
#74279=CARTESIAN_POINT ( 'NONE',  ( -0.1771653543307080136, 0.1660481256975883668, -0.3530559997133364547 ) ) ;
#74280=CARTESIAN_POINT ( 'NONE',  ( 0.2230971128608932319, -0.3690944881889763329, 0.3153832671262228327 ) ) ;
#74281=CARTESIAN_POINT ( 'NONE',  ( -1.023622047244094002, -0.1870078740157480601, -0.3641732283464567677 ) ) ;
#74282=CARTESIAN_POINT ( 'NONE',  ( -1.450131233595799651, -0.6692913385826771977, 0.1292274648535927661 ) ) ;
#74283=CARTESIAN_POINT ( 'NONE',  ( -1.574803149606298636, -0.1870078740157479769, 0.4822834645669291653 ) ) ;
#74284=CARTESIAN_POINT ( 'NONE',  ( 1.574803149606299746, -0.1870078740157480879, -0.4822834645669291653 ) ) ;
#74286=CARTESIAN_POINT ( 'NONE',  ( 0.6036745406824154392, 0.1283753931104746893, -0.1820866141732285504 ) ) ;
#74287=CARTESIAN_POINT ( 'NONE',  ( 0.8530183727034128527, -0.4281496062992124485, 0.4176697321401328655 ) ) ;
#74288=CARTESIAN_POINT ( 'NONE',  ( -0.08874907683609993547, 8.471767977567108961E-16, -0.4445507791589058955 ) ) ;
#74289=CARTESIAN_POINT ( 'NONE',  ( 1.279527559055118724, 0.07958543189024085140, 0.2665933059059887866 ) ) ;
#74291=CARTESIAN_POINT ( 'NONE',  ( -1.259842519685038686, -0.1870078740157480879, -0.4822834645669291653 ) ) ;
#74292=CARTESIAN_POINT ( 'NONE',  ( -0.8070866141732276899, 0.1660481256975883668, -0.3530559997133364547 ) ) ;
#74293=CARTESIAN_POINT ( 'NONE',  ( 0.1771653543307093182, 0.1660481256975885056, 0.3530559997133364547 ) ) ;
#74294=CARTESIAN_POINT ( 'NONE',  ( -1.732283464566928277, -0.1870078740157479769, 0.3641732283464567677 ) ) ;
#74296=CARTESIAN_POINT ( 'NONE',  ( 0.8661417322834652488, -0.1870078740157480879, -0.4822834645669291653 ) ) ;
#74297=CARTESIAN_POINT ( 'NONE',  ( -1.640419947506561060, -0.4281496062992127816, -0.4176697321401328100 ) ) ;
#74298=CARTESIAN_POINT ( 'NONE',  ( 0.01968503937007957949, -0.5400638737290845981, -0.3530559997133363437 ) ) ;
#74299=CARTESIAN_POINT ( 'NONE',  ( 0.5839895013123367340, -0.6692913385826773087, -0.1292274648535924053 ) ) ;
#74303=CARTESIAN_POINT ( 'NONE',  ( -1.595398199321656829, 1.013096522517431097, -0.1559797534342478031 ) ) ;
#74305=CARTESIAN_POINT ( 'NONE',  ( -0.1574803149606292529, -0.1870078740157479769, 0.3641732283464567677 ) ) ;
#74306=CARTESIAN_POINT ( 'NONE',  ( -0.6561679790026240244, -0.6046776061558807314, 0.2411417322834647770 ) ) ;
#74307=CARTESIAN_POINT ( 'NONE',  ( 0.9448818897637802916, -0.1870078740157479769, 0.4822834645669291653 ) ) ;
#74309=CARTESIAN_POINT ( 'NONE',  ( 0.08530183727034192087, -0.08942795157527998196, 0.3641732283464567121 ) ) ;
#74310=CARTESIAN_POINT ( 'NONE',  ( -1.194225721784776262, -0.4281496062992124485, 0.4176697321401328655 ) ) ;
#74311=CARTESIAN_POINT ( 'NONE',  ( 1.194225721784777594, -0.4281496062992127816, -0.4176697321401328100 ) ) ;
#74317=CARTESIAN_POINT ( 'NONE',  ( 0.8005249343832027131, 0.05413385826771666132, 0.4176697321401328100 ) ) ;
#74318=CARTESIAN_POINT ( 'NONE',  ( 1.213910761154856299, -0.5511811023622048555, -0.09757992244046775898 ) ) ;
#74319=CARTESIAN_POINT ( 'NONE',  ( -1.482939632545930975, -0.004921259842519576551, 0.3153832671262227771 ) ) ;
#74320=CARTESIAN_POINT ( 'NONE',  ( -1.502624671916009680, -0.3162353388693405765, 0.4822834645669290543 ) ) ;
#74323=CARTESIAN_POINT ( 'NONE',  ( 1.200787401574803681, 0.1660481256975885056, 0.3530559997133364547 ) ) ;
#74325=CARTESIAN_POINT ( 'NONE',  ( -0.6036745406824141069, 0.2306618581243848609, 0.2411417322834645549 ) ) ;
#74326=CARTESIAN_POINT ( 'NONE',  ( -0.5249343832020990641, -0.6046776061558809534, -0.2411417322834644161 ) ) ;
#74327=CARTESIAN_POINT ( 'NONE',  ( 1.555118110236221041, -0.5400638737290844871, 0.3530559997133364547 ) ) ;
#74329=CARTESIAN_POINT ( 'NONE',  ( 0.08530183727034192087, -0.3162353388693409650, -0.4822834645669289433 ) ) ;
#74331=CARTESIAN_POINT ( 'NONE',  ( -1.568241469816272105, -0.2845877964562161244, -0.3641732283464567121 ) ) ;
#74335=CARTESIAN_POINT ( 'NONE',  ( -0.01241954290193713825, 2.784432375088962958E-17, -0.3464511005275205946 ) ) ;
#74336=CARTESIAN_POINT ( 'NONE',  ( -1.732283464566928277, -0.1870078740157479769, 0.4822834645669291653 ) ) ;
#74338=CARTESIAN_POINT ( 'NONE',  ( 1.666666666666667185, -0.004921259842519576551, 0.3153832671262227771 ) ) ;
#74340=DIRECTION ( 'NONE',  ( 0.000000000000000000, 1.000000000000000000, 0.000000000000000000 ) ) ;
#74341=CARTESIAN_POINT ( 'NONE',  ( -0.3477690288713902178, 0.2952755905511810219, -0.1292274648535930437 ) ) ;
#74345=CARTESIAN_POINT ( 'NONE',  ( -0.5052493438320203589, 0.1771653543307087075, -0.09757992244046823083 ) ) ;
#74346=CARTESIAN_POINT ( 'NONE',  ( -1.010498687664041384, -0.3690944881889765550, -0.3153832671262227771 ) ) ;
#74347=CARTESIAN_POINT ( 'NONE',  ( 1.489501312335958172, -0.05778040916215560624, -0.4822834645669293319 ) ) ;
#74349=CARTESIAN_POINT ( 'NONE',  ( 0.4724409448818904789, -0.1870078740157479769, 0.4822834645669291653 ) ) ;
#74350=CARTESIAN_POINT ( 'NONE',  ( -1.187664041994749731, -0.3162353388693405765, 0.4822834645669290543 ) ) ;
#74352=ORIENTED_EDGE ( 'NONE', *, *, #3797, .F. ) ;
#74353=CARTESIAN_POINT ( 'NONE',  ( -1.246719160104985846, -0.4281496062992127816, -0.4176697321401328100 ) ) ;
#74359=DIRECTION ( 'NONE',  ( 1.000000000000000000, -0.000000000000000000, -1.692413147294445970E-16 ) ) ;
#74360=CARTESIAN_POINT ( 'NONE',  ( -0.5839895013123351797, -0.6692913385826771977, 0.1292274648535927661 ) ) ;
#74361=CARTESIAN_POINT ( 'NONE',  ( 1.541994750656168645, 0.2952755905511810774, -0.1292274648535930714 ) ) ;
#74362=CARTESIAN_POINT ( 'NONE',  ( -1.587926509186350810, -0.4281496062992124485, 0.4176697321401328655 ) ) ;
#74365=CARTESIAN_POINT ( 'NONE',  ( -0.9514435695538050464, -0.3162353388693405765, 0.4822834645669290543 ) ) ;
#74367=CARTESIAN_POINT ( 'NONE',  ( -0.1049868766404193215, 0.1283753931104746893, -0.1820866141732285504 ) ) ;
#74369=CARTESIAN_POINT ( 'NONE',  ( -0.2887139107611542133, -0.5023911411419708095, -0.1820866141732282451 ) ) ;
#74370=CARTESIAN_POINT ( 'NONE',  ( 1.023622047244095112, -0.1870078740157480601, -0.3641732283464567677 ) ) ;
#74371=CARTESIAN_POINT ( 'NONE',  ( 0.7217847769028878924, -0.4281496062992127816, -0.4176697321401328100 ) ) ;
#74372=CARTESIAN_POINT ( 'NONE',  ( -0.4133858267716528645, -0.4536011799217367080, 0.2665933059059888421 ) ) ;
#74374=CARTESIAN_POINT ( 'NONE',  ( 1.548556430446194954, -0.6046776061558807314, 0.2411417322834647770 ) ) ;
#74375=EDGE_CURVE ( 'NONE', #59008, #80968, #66311, .T. ) ;
#74376=CARTESIAN_POINT ( 'NONE',  ( -0.9776902887139098386, 0.2952755905511810774, -0.1292274648535930714 ) ) ;
#74378=CARTESIAN_POINT ( 'NONE',  ( 0.1509186351706042484, -0.3162353388693405765, 0.4822834645669290543 ) ) ;
#74379=CARTESIAN_POINT ( 'NONE',  ( -0.6233595800524928121, -0.3162353388693409650, -0.4822834645669289433 ) ) ;
#74381=EDGE_CURVE ( 'NONE', #69946, #2588, #77688, .T. ) ;
#74382=CARTESIAN_POINT ( 'NONE',  ( -0.01312335958005186876, -0.3690944881889763329, 0.3153832671262228327 ) ) ;
#74383=CARTESIAN_POINT ( 'NONE',  ( -0.3805774278215216522, -0.4281496062992127816, -0.4176697321401328100 ) ) ;
#74384=CARTESIAN_POINT ( 'NONE',  ( -0.6430446194225712953, 0.05413385826771626580, -0.4176697321401330321 ) ) ;
#74385=PLANE ( 'NONE',  #54636 ) ;
#74386=AXIS2_PLACEMENT_3D ( 'NONE', #26743, #66727, #40622 ) ;
#74387=CARTESIAN_POINT ( 'NONE',  ( 0.1706036745406830368, -0.4281496062992127816, -0.4176697321401328100 ) ) ;
#74390=CARTESIAN_POINT ( 'NONE',  ( 1.456692913385827515, 0.2952755905511811885, 0.000000000000000000 ) ) ;
#74391=CARTESIAN_POINT ( 'NONE',  ( -0.6430446194225716283, -0.3690944881889763329, 0.3153832671262228327 ) ) ;
#74392=CARTESIAN_POINT ( 'NONE',  ( -0.5774278215223089816, 0.2306618581243847221, -0.2411417322834647770 ) ) ;
#74393=CARTESIAN_POINT ( 'NONE',  ( 1.594488188976378673, -0.5400638737290845981, -0.3530559997133363437 ) ) ;
#74394=CARTESIAN_POINT ( 'NONE',  ( 1.437007874015748810, -0.5400638737290845981, -0.3530559997133363437 ) ) ;
#74395=CARTESIAN_POINT ( 'NONE',  ( -1.555118110236219930, -0.5400638737290845981, -0.3530559997133363437 ) ) ;
#74396=CARTESIAN_POINT ( 'NONE',  ( -0.8792650918635160906, -0.004921259842519870586, -0.3153832671262229437 ) ) ;
#74399=AXIS2_PLACEMENT_3D ( 'NONE', #56478, #69941, #82181 ) ;
#74402=CARTESIAN_POINT ( 'NONE',  ( 1.233595800524935227, -0.5023911411419708095, 0.1820866141732285504 ) ) ;
#74403=CARTESIAN_POINT ( 'NONE',  ( 0.9711286089238851948, 0.2306618581243848609, 0.2411417322834645549 ) ) ;
#74405=CARTESIAN_POINT ( 'NONE',  ( 0.7611548556430451917, -0.6046776061558807314, 0.2411417322834647770 ) ) ;
#74407=CARTESIAN_POINT ( 'NONE',  ( 1.312335958005250269, -0.5023911411419708095, 0.1820866141732285504 ) ) ;
#74408=CARTESIAN_POINT ( 'NONE',  ( 0.08530183727034192087, -0.05778040916215522460, 0.4822834645669289988 ) ) ;
#74409=CARTESIAN_POINT ( 'NONE',  ( -0.9973753280839886548, 0.2306618581243848609, 0.2411417322834645549 ) ) ;
#74410=CARTESIAN_POINT ( 'NONE',  ( 1.391076115485564868, 0.2306618581243847221, -0.2411417322834647770 ) ) ;
#74413=CARTESIAN_POINT ( 'NONE',  ( 0.3083989501312343062, -0.2845877964562159024, 0.3641732283464567677 ) ) ;
#74414=ORIENTED_EDGE ( 'NONE', *, *, #16758, .F. ) ;
#74416=ORIENTED_EDGE ( 'NONE', *, *, #18267, .T. ) ;
#74417=CARTESIAN_POINT ( 'NONE',  ( -0.7677165354330699465, 0.1660481256975885056, 0.3530559997133364547 ) ) ;
#74418=CARTESIAN_POINT ( 'NONE',  ( -0.1246719160104980823, -0.6692913385826773087, -0.1292274648535924053 ) ) ;
#74419=CARTESIAN_POINT ( 'NONE',  ( -0.3018372703412066094, -0.4281496062992127816, -0.4176697321401328100 ) ) ;
#74420=CARTESIAN_POINT ( 'NONE',  ( 0.7217847769028878924, 0.05413385826771666132, 0.4176697321401328100 ) ) ;
#74421=CARTESIAN_POINT ( 'NONE',  ( -0.9776902887139098386, 0.2952755905511810774, -0.1292274648535930714 ) ) ;
#74422=CARTESIAN_POINT ( 'NONE',  ( -0.1902887139107604098, -0.6692913385826771977, 0.1292274648535927661 ) ) ;
#74423=CARTESIAN_POINT ( 'NONE',  ( 1.364829396325459854, -0.6046776061558809534, -0.2411417322834644161 ) ) ;
#74424=CARTESIAN_POINT ( 'NONE',  ( 0.6430446194225728496, 0.05413385826771666132, 0.4176697321401328100 ) ) ;
#74425=CARTESIAN_POINT ( 'NONE',  ( 0.7414698162729663755, 0.2952755905511811885, 0.1292274648535926551 ) ) ;
#74427=CARTESIAN_POINT ( 'NONE',  ( -0.3215223097112853146, -0.08942795157528024563, -0.3641732283464568787 ) ) ;
#74430=VERTEX_POINT ( 'NONE', #13296 ) ;
#74431=CARTESIAN_POINT ( 'NONE',  ( -0.8923884514435688198, 0.1283753931104746893, -0.1820866141732285504 ) ) ;
#74432=CARTESIAN_POINT ( 'NONE',  ( -0.4658792650918627265, -0.3162353388693409650, -0.4822834645669289433 ) ) ;
#74434=CARTESIAN_POINT ( 'NONE',  ( -0.7217847769028863381, 0.05413385826771626580, -0.4176697321401330321 ) ) ;
#74435=CARTESIAN_POINT ( 'NONE',  ( -1.036745406824146176, 0.05413385826771626580, -0.4176697321401330321 ) ) ;
#74436=CARTESIAN_POINT ( 'NONE',  ( -1.351706036745406347, -0.4281496062992124485, 0.4176697321401328655 ) ) ;
#74437=ADVANCED_FACE ( 'NONE', ( #57467 ), #12877, .T. ) ;
#74438=CARTESIAN_POINT ( 'NONE',  ( -1.489501312335957062, -0.3162353388693409650, -0.4822834645669289433 ) ) ;
#74439=CARTESIAN_POINT ( 'NONE',  ( 0.9711286089238851948, -0.5023911411419708095, -0.1820866141732282451 ) ) ;
#74442=CARTESIAN_POINT ( 'NONE',  ( 0.2493438320209980519, -0.3690944881889765550, -0.3153832671262227771 ) ) ;
#74443=AXIS2_PLACEMENT_3D ( 'NONE', #29842, #36570, #61838 ) ;
#74444=CARTESIAN_POINT ( 'NONE',  ( 0.04593175853018440641, -0.6692913385826771977, 0.1292274648535927661 ) ) ;
#74445=CARTESIAN_POINT ( 'NONE',  ( -0.1706036745406816491, 0.05413385826771626580, -0.4176697321401330321 ) ) ;
#74449=VERTEX_POINT ( 'NONE', #76029 ) ;
#74451=CARTESIAN_POINT ( 'NONE',  ( 1.601049868766404982, 0.2306618581243848609, 0.2411417322834645549 ) ) ;
#74452=CARTESIAN_POINT ( 'NONE',  ( -0.6824146981627291497, -0.5023911411419708095, -0.1820866141732282451 ) ) ;
#74453=CARTESIAN_POINT ( 'NONE',  ( -1.049868766404198794, 0.2306618581243847221, -0.2411417322834647770 ) ) ;
#74457=CARTESIAN_POINT ( 'NONE',  ( -1.607611548556429737, 0.1771653543307087075, -0.09757992244046823083 ) ) ;
#74458=CARTESIAN_POINT ( 'NONE',  ( 0.5971128608923890191, -0.6692913385826771977, 0.1292274648535927661 ) ) ;
#74459=CARTESIAN_POINT ( 'NONE',  ( 0.5314960629921267055, -0.5400638737290844871, 0.3530559997133364547 ) ) ;
#74460=CARTESIAN_POINT ( 'NONE',  ( -0.6167979002624665030, -0.3690944881889765550, -0.3153832671262227771 ) ) ;
#74461=CARTESIAN_POINT ( 'NONE',  ( -0.06561679790026180015, -0.4281496062992127816, -0.4176697321401328100 ) ) ;
#74463=CARTESIAN_POINT ( 'NONE',  ( -0.6102362204724400829, 0.1660481256975885056, 0.3530559997133364547 ) ) ;
#74464=AXIS2_PLACEMENT_3D ( 'NONE', #39188, #5955, #64451 ) ;
#74466=CARTESIAN_POINT ( 'NONE',  ( 1.292650918635171564, 0.1771653543307087630, 0.09757992244046791164 ) ) ;
#74467=CARTESIAN_POINT ( 'NONE',  ( 0.2952755905511816326, -0.4536011799217367080, 0.2665933059059888421 ) ) ;
#74468=CARTESIAN_POINT ( 'NONE',  ( 1.227034120734908917, 0.1771653543307087075, -0.09757992244046823083 ) ) ;
#74469=CARTESIAN_POINT ( 'NONE',  ( -1.220472440944881054, 0.2952755905511811885, 0.000000000000000000 ) ) ;
#74470=CARTESIAN_POINT ( 'NONE',  ( -1.167979002624671470, -0.004921259842519576551, 0.3153832671262227771 ) ) ;
#74472=CARTESIAN_POINT ( 'NONE',  ( -1.030183727034119867, -0.05778040916215560624, -0.4822834645669293319 ) ) ;
#74473=CARTESIAN_POINT ( 'NONE',  ( -0.2493438320209966919, -0.4281496062992124485, 0.4176697321401328655 ) ) ;
#74474=CARTESIAN_POINT ( 'NONE',  ( 0.4461942257217856311, 0.2306618581243847221, -0.2411417322834647770 ) ) ;
#74477=CARTESIAN_POINT ( 'NONE',  ( 0.5118110236220480003, -0.5511811023622047445, 6.969142054262312111E-17 ) ) ;
#74478=CARTESIAN_POINT ( 'NONE',  ( 1.102362204724410155, -0.1870078740157479769, 0.4822834645669291653 ) ) ;
#74479=CARTESIAN_POINT ( 'NONE',  ( -1.686351706036744558, 0.1771653543307087075, -0.09757992244046823083 ) ) ;
#74480=CARTESIAN_POINT ( 'NONE',  ( 0.9120734908136490793, 0.2952755905511810774, -0.1292274648535930714 ) ) ;
#74481=CARTESIAN_POINT ( 'NONE',  ( -1.725721784776902190, -0.08942795157527998196, 0.3641732283464567121 ) ) ;
#74482=CARTESIAN_POINT ( 'NONE',  ( -1.502624671916009680, -0.05778040916215560624, -0.4822834645669293319 ) ) ;
#74483=CARTESIAN_POINT ( 'NONE',  ( -0.7939632545931754048, -0.3162353388693405765, 0.4822834645669290543 ) ) ;
#74484=CARTESIAN_POINT ( 'NONE',  ( -0.3018372703412066094, -0.3690944881889765550, -0.3153832671262227771 ) ) ;
#74486=CARTESIAN_POINT ( 'NONE',  ( 0.6364829396325465405, -0.08942795157527998196, 0.3641732283464567121 ) ) ;
#74488=CARTESIAN_POINT ( 'NONE',  ( -0.09186351706036663400, -0.4281496062992124485, 0.4176697321401328655 ) ) ;
#74490=CARTESIAN_POINT ( 'NONE',  ( -1.036745406824146176, 0.05413385826771626580, -0.4176697321401330321 ) ) ;
#74492=CARTESIAN_POINT ( 'NONE',  ( 0.8727034120734912248, -0.2845877964562161244, -0.3641732283464567121 ) ) ;
#74493=CARTESIAN_POINT ( 'NONE',  ( -0.1574803149606292529, -0.1870078740157480879, -0.4822834645669291653 ) ) ;
#74494=CARTESIAN_POINT ( 'NONE',  ( -0.4658792650918627265, -0.3162353388693409650, -0.4822834645669289433 ) ) ;
#74495=CARTESIAN_POINT ( 'NONE',  ( -0.4527559055118102749, -0.4536011799217368745, -0.2665933059059886201 ) ) ;
#74497=CARTESIAN_POINT ( 'NONE',  ( -0.3083989501312330295, -0.2845877964562161244, -0.3641732283464567121 ) ) ;
#74498=CARTESIAN_POINT ( 'NONE',  ( 0.5446194225721792126, -0.3162353388693405765, 0.4822834645669290543 ) ) ;
#74499=CARTESIAN_POINT ( 'NONE',  ( -1.030183727034119867, -0.08942795157528024563, -0.3641732283464568787 ) ) ;
#74501=CARTESIAN_POINT ( 'NONE',  ( 1.528871391076116026, -0.6692913385826773087, -0.1292274648535924053 ) ) ;
#74502=DIRECTION ( 'NONE',  ( -3.096699300667737957E-16, 1.000000000000000000, -0.000000000000000000 ) ) ;
#74503=VERTEX_POINT ( 'NONE', #30977 ) ;
#74505=CARTESIAN_POINT ( 'NONE',  ( -1.417322834645668772, -0.1870078740157479769, 0.3641732283464567677 ) ) ;
#74506=CARTESIAN_POINT ( 'NONE',  ( -0.3805774278215216522, -0.4281496062992127816, -0.4176697321401328100 ) ) ;
#74507=CARTESIAN_POINT ( 'NONE',  ( -1.167979002624671470, 0.05413385826771666132, 0.4176697321401328100 ) ) ;
#74510=CARTESIAN_POINT ( 'NONE',  ( 1.345144356955381593, -0.05778040916215522460, 0.4822834645669289988 ) ) ;
#74511=CARTESIAN_POINT ( 'NONE',  ( 0.5052493438320218022, -0.6692913385826773087, -0.1292274648535924053 ) ) ;
#74514=CARTESIAN_POINT ( 'NONE',  ( 1.607611548556431069, 0.1771653543307087630, 0.09757992244046791164 ) ) ;
#74517=CARTESIAN_POINT ( 'NONE',  ( -0.8398950131233585692, 0.1283753931104748280, 0.1820866141732283561 ) ) ;
#74521=CARTESIAN_POINT ( 'NONE',  ( 0.6955380577427828781, 0.05413385826771626580, -0.4176697321401330321 ) ) ;
#74522=CARTESIAN_POINT ( 'NONE',  ( -0.2559055118110230564, 0.1660481256975883668, -0.3530559997133364547 ) ) ;
#74524=CARTESIAN_POINT ( 'NONE',  ( -1.128608923884513837, 0.2306618581243847221, -0.2411417322834647770 ) ) ;
#74525=CARTESIAN_POINT ( 'NONE',  ( 1.043307086614173818, 0.1660481256975885056, 0.3530559997133364547 ) ) ;
#74526=CARTESIAN_POINT ( 'NONE',  ( -1.397637795275589623, -0.4536011799217368745, -0.2665933059059886201 ) ) ;
#74527=PLANE ( 'NONE',  #72259 ) ;
#74528=CARTESIAN_POINT ( 'NONE',  ( 0.1574803149606306130, -0.1870078740157480879, -0.4822834645669291653 ) ) ;
#74529=CARTESIAN_POINT ( 'NONE',  ( -0.9317585301837263412, -0.4281496062992127816, -0.4176697321401328100 ) ) ;
#74531=CARTESIAN_POINT ( 'NONE',  ( 1.555118110236221041, -0.5400638737290844871, 0.3530559997133364547 ) ) ;
#74533=CARTESIAN_POINT ( 'NONE',  ( 0.9317585301837276734, 0.05413385826771626580, -0.4176697321401330321 ) ) ;
#74535=CARTESIAN_POINT ( 'NONE',  ( 1.351706036745407680, -0.004921259842519576551, 0.3153832671262227771 ) ) ;
#74538=CARTESIAN_POINT ( 'NONE',  ( -0.2230971128608915943, 0.05413385826771666132, 0.4176697321401328100 ) ) ;
#74540=CARTESIAN_POINT ( 'NONE',  ( 0.5511811023622054106, -0.1870078740157480601, -0.3641732283464567677 ) ) ;
#74541=CARTESIAN_POINT ( 'NONE',  ( -1.502624671916009680, -0.05778040916215560624, -0.4822834645669293319 ) ) ;
#74542=CARTESIAN_POINT ( 'NONE',  ( 0.5314960629921264834, 0.1660481256975883668, -0.3530559997133364547 ) ) ;
#74543=CARTESIAN_POINT ( 'NONE',  ( 0.7086614173228352742, -0.1870078740157480879, -0.4822834645669291653 ) ) ;
#74545=CARTESIAN_POINT ( 'NONE',  ( -0.1181102362204717315, 0.2952755905511811885, 0.000000000000000000 ) ) ;
#74547=CARTESIAN_POINT ( 'NONE',  ( -0.6233595800524928121, -0.3162353388693409650, -0.4822834645669289433 ) ) ;
#74549=CARTESIAN_POINT ( 'NONE',  ( -1.640419947506561060, -0.4281496062992127816, -0.4176697321401328100 ) ) ;
#74550=CARTESIAN_POINT ( 'NONE',  ( -1.128608923884513837, 0.2306618581243847221, -0.2411417322834647770 ) ) ;
#74551=CARTESIAN_POINT ( 'NONE',  ( 1.463254593175853824, -0.6692913385826771977, 0.1292274648535927661 ) ) ;
#74552=CARTESIAN_POINT ( 'NONE',  ( 1.246719160104987623, 0.05413385826771626580, -0.4176697321401330321 ) ) ;
#74554=CARTESIAN_POINT ( 'NONE',  ( -1.135170603674539924, -0.6692913385826771977, 0.1292274648535927661 ) ) ;
#74556=CARTESIAN_POINT ( 'NONE',  ( 0.1181102362204730916, -0.6692913385826771977, 8.415575281601705876E-17 ) ) ;
#74558=CARTESIAN_POINT ( 'NONE',  ( -0.5052493438320203589, 0.2952755905511810774, -0.1292274648535930714 ) ) ;
#74559=CARTESIAN_POINT ( 'NONE',  ( 1.633858267716535639, -0.5400638737290844871, 0.3530559997133364547 ) ) ;
#74560=CARTESIAN_POINT ( 'NONE',  ( 0.7677165354330716118, 0.07958543189024071263, -0.2665933059059888421 ) ) ;
#74561=CARTESIAN_POINT ( 'NONE',  ( 1.259842519685040019, -0.1870078740157479769, 0.4822834645669291653 ) ) ;
#74563=CARTESIAN_POINT ( 'NONE',  ( 0.6758530183727039509, -0.5511811023622046335, 0.09757992244046803654 ) ) ;
#74564=CARTESIAN_POINT ( 'NONE',  ( 0.9908136482939640111, 0.2952755905511810774, -0.1292274648535930714 ) ) ;
#74566=CARTESIAN_POINT ( 'NONE',  ( -0.7283464566929126471, 0.1660481256975883668, -0.3530559997133364547 ) ) ;
#74568=VECTOR ( 'NONE', #79438, 39.37007874015748143 ) ;
#74569=CARTESIAN_POINT ( 'NONE',  ( 1.161417322834646271, 0.07958543189024071263, -0.2665933059059888421 ) ) ;
#74570=CARTESIAN_POINT ( 'NONE',  ( -0.3740157480314953431, -0.5400638737290845981, -0.3530559997133363437 ) ) ;
#74571=CARTESIAN_POINT ( 'NONE',  ( 0.09842519685039434474, -0.5400638737290845981, -0.3530559997133363437 ) ) ;
#74572=CARTESIAN_POINT ( 'NONE',  ( 0.09115970038225353067, 3.421639014772782816E-16, 0.3464511005275203726 ) ) ;
#74573=CARTESIAN_POINT ( 'NONE',  ( -0.09186351706036689768, 0.05413385826771626580, -0.4176697321401330321 ) ) ;
#74574=CARTESIAN_POINT ( 'NONE',  ( 0.7283464566929143125, 0.07958543189024085140, 0.2665933059059887866 ) ) ;
#74576=CARTESIAN_POINT ( 'NONE',  ( -0.01968503937007793844, 0.07958543189024071263, -0.2665933059059888421 ) ) ;
#74577=CARTESIAN_POINT ( 'NONE',  ( 0.9120734908136489683, -0.5511811023622046335, 0.09757992244046803654 ) ) ;
#74578=DIRECTION ( 'NONE',  ( -3.096699300667737957E-16, 1.000000000000000000, -0.000000000000000000 ) ) ;
#74580=CARTESIAN_POINT ( 'NONE',  ( 0.4396325459317593221, 0.2952755905511810774, -0.1292274648535930714 ) ) ;
#74582=CARTESIAN_POINT ( 'NONE',  ( 1.423884514435696413, -0.2845877964562161244, -0.3641732283464567121 ) ) ;
#74584=CARTESIAN_POINT ( 'NONE',  ( -0.3871391076115479057, -0.2845877964562161244, -0.3641732283464567121 ) ) ;
#74586=CARTESIAN_POINT ( 'NONE',  ( -0.01312335958005186876, 0.05413385826771626580, -0.4176697321401330321 ) ) ;
#74587=CARTESIAN_POINT ( 'NONE',  ( 1.240157480314961314, 0.07958543189024071263, -0.2665933059059888421 ) ) ;
#74588=CARTESIAN_POINT ( 'NONE',  ( -1.423884514435694859, -0.2845877964562159024, 0.3641732283464567677 ) ) ;
#74589=CARTESIAN_POINT ( 'NONE',  ( -1.338582677165353729, -0.1870078740157480879, -0.4822834645669291653 ) ) ;
#74590=CARTESIAN_POINT ( 'NONE',  ( 0.2559055118110243332, 0.1660481256975885056, 0.3530559997133364547 ) ) ;
#74591=CARTESIAN_POINT ( 'NONE',  ( 1.023622047244095334, -0.1870078740157479769, 0.4822834645669291653 ) ) ;
#74593=CARTESIAN_POINT ( 'NONE',  ( 0.3280839895013130669, 0.05413385826771666132, 0.4176697321401328100 ) ) ;
#74594=CARTESIAN_POINT ( 'NONE',  ( 1.154855643044620184, -0.6046776061558807314, 0.2411417322834647770 ) ) ;
#74595=B_SPLINE_CURVE_WITH_KNOTS ( 'NONE', 3,
 ( #64441, #38349, #6364, #26132 ),
 .UNSPECIFIED., .F., .F.,
 ( 4, 4 ),
 ( 9.341771812940338307E-18, 0.001494448006632299744 ),
 .UNSPECIFIED. ) ;
#74596=CARTESIAN_POINT ( 'NONE',  ( 0.7939632545931766261, -0.3162353388693409650, -0.4822834645669289433 ) ) ;
#74598=CARTESIAN_POINT ( 'NONE',  ( 0.8792650918635177559, -0.004921259842519576551, 0.3153832671262227771 ) ) ;
#74599=CARTESIAN_POINT ( 'NONE',  ( -1.587926509186350810, -0.004921259842519870586, -0.3153832671262229437 ) ) ;
#74600=CARTESIAN_POINT ( 'NONE',  ( -0.05905511811023545637, -0.4536011799217368745, -0.2665933059059886201 ) ) ;
#74601=CARTESIAN_POINT ( 'NONE',  ( -0.1312335958005241554, -0.6046776061558809534, -0.2411417322834644161 ) ) ;
#74602=CARTESIAN_POINT ( 'NONE',  ( 0.5971128608923890191, -0.6692913385826771977, 0.1292274648535927661 ) ) ;
#74603=CARTESIAN_POINT ( 'NONE',  ( -0.2887139107611542133, -0.6046776061558809534, -0.2411417322834644161 ) ) ;
#74605=CARTESIAN_POINT ( 'NONE',  ( -0.1377952755905504645, 0.07958543189024085140, 0.2665933059059887866 ) ) ;
#74606=CARTESIAN_POINT ( 'NONE',  ( 0.8792650918635177559, -0.4281496062992127816, -0.4176697321401328100 ) ) ;
#74607=CARTESIAN_POINT ( 'NONE',  ( 0.9186351706036752773, 0.1283753931104746893, -0.1820866141732285504 ) ) ;
#74610=CARTESIAN_POINT ( 'NONE',  ( 1.011202504342157527, 9.477779430591278127E-17, -0.3464511005275205946 ) ) ;
#74612=CARTESIAN_POINT ( 'NONE',  ( -1.233595800524933894, -0.6046776061558809534, -0.2411417322834644161 ) ) ;
#74613=CARTESIAN_POINT ( 'NONE',  ( -0.3871391076115479057, -0.3162353388693409650, -0.4822834645669289433 ) ) ;
#74614=( BOUNDED_CURVE ( )  B_SPLINE_CURVE ( 2, ( #12701, #38777, #6375, #57706, #77088, #71610, #64454, #26985, #13963, #69, #25723, #51383, #58124 ),
 .UNSPECIFIED., .F., .F. ) 
 B_SPLINE_CURVE_WITH_KNOTS ( ( 3, 2, 2, 2, 2, 2, 3 ),
 ( 0.3551492764529827206, 0.3560606060606060774, 0.3598484848484848619, 0.3636363636363636465, 0.3674242424242424310, 0.3712121212121212155, 0.3721234508197446278 ),
 .UNSPECIFIED. ) 
 CURVE ( )  GEOMETRIC_REPRESENTATION_ITEM ( )  RATIONAL_B_SPLINE_CURVE ( ( 0.9875488213027530104, 0.9918020599134685922, 1.000000000000000000, 0.9659258262890683122, 1.000000000000000000, 0.9659258262890683122, 1.000000000000000000, 0.9659258262890683122, 1.000000000000000000, 0.9659258262890683122, 1.000000000000000000, 0.9918020599134680371, 0.9875488213027523443 ) ) 
 REPRESENTATION_ITEM ( '' )  );
#74618=CARTESIAN_POINT ( 'NONE',  ( 0.3937007874015754361, -0.1870078740157479769, 0.3641732283464567677 ) ) ;
#74620=CARTESIAN_POINT ( 'NONE',  ( 1.108923884514436242, -0.05778040916215522460, 0.4822834645669289988 ) ) ;
#74623=CARTESIAN_POINT ( 'NONE',  ( -1.692913385826770645, 0.1771653543307087630, 0.000000000000000000 ) ) ;
#74624=CARTESIAN_POINT ( 'NONE',  ( 1.666666666666667185, 0.05413385826771666132, 0.4176697321401328100 ) ) ;
#74625=CARTESIAN_POINT ( 'NONE',  ( 1.482939632545932307, -0.004921259842519870586, -0.3153832671262229437 ) ) ;
#74626=CARTESIAN_POINT ( 'NONE',  ( 0.5905511811023629321, 0.2952755905511811885, 0.000000000000000000 ) ) ;
#74628=CARTESIAN_POINT ( 'NONE',  ( -0.03937007874015669567, 0.2952755905511811885, 0.000000000000000000 ) ) ;
#74629=CARTESIAN_POINT ( 'NONE',  ( -0.8136482939632537770, -0.5023911411419708095, 0.1820866141732285504 ) ) ;
#74630=CARTESIAN_POINT ( 'NONE',  ( 0.4133858267716541968, -0.5400638737290845981, -0.3530559997133363437 ) ) ;
#74632=CARTESIAN_POINT ( 'NONE',  ( -0.006561679790025524116, -0.3162353388693405765, 0.4822834645669290543 ) ) ;
#74633=CARTESIAN_POINT ( 'NONE',  ( -1.603475055217291612, 2.094628720676861011, 0.04573490813648255215 ) ) ;
#74636=CARTESIAN_POINT ( 'NONE',  ( 1.017060367454068803, -0.3162353388693405765, 0.4822834645669290543 ) ) ;
#74637=CARTESIAN_POINT ( 'NONE',  ( -0.3346456692913377662, -0.5400638737290844871, 0.3530559997133364547 ) ) ;
#74638=CARTESIAN_POINT ( 'NONE',  ( -1.502624671916009680, -0.3162353388693405765, 0.4822834645669290543 ) ) ;
#74640=CARTESIAN_POINT ( 'NONE',  ( 1.003937007874016185, 0.1660481256975883668, -0.3530559997133364547 ) ) ;
#74641=CARTESIAN_POINT ( 'NONE',  ( 0.5249343832021005074, -0.6046776061558807314, 0.2411417322834647770 ) ) ;
#74643=CARTESIAN_POINT ( 'NONE',  ( -0.3740157480314953431, -0.5400638737290845981, -0.3530559997133363437 ) ) ;
#74644=CARTESIAN_POINT ( 'NONE',  ( 0.1377952755905518800, 0.1660481256975883668, -0.3530559997133364547 ) ) ;
#74645=CARTESIAN_POINT ( 'NONE',  ( -0.6233595800524928121, -0.3162353388693409650, -0.4822834645669289433 ) ) ;
#74646=CARTESIAN_POINT ( 'NONE',  ( 0.1443569553805781891, -0.004921259842519870586, -0.3153832671262229437 ) ) ;
#74647=CARTESIAN_POINT ( 'NONE',  ( -1.640419947506561060, -0.4281496062992127816, -0.4176697321401328100 ) ) ;
#74649=CARTESIAN_POINT ( 'NONE',  ( 0.1902887139107617975, 0.2952755905511811885, 0.1292274648535926551 ) ) ;
#74651=CARTESIAN_POINT ( 'NONE',  ( 1.502624671916010790, -0.3162353388693409650, -0.4822834645669289433 ) ) ;
#74654=ORIENTED_EDGE ( 'NONE', *, *, #29199, .F. ) ;
#74655=CARTESIAN_POINT ( 'NONE',  ( 0.6496062992125991586, -0.5400638737290845981, -0.3530559997133363437 ) ) ;
#74656=CARTESIAN_POINT ( 'NONE',  ( 0.03937007874015806264, 0.1771653543307087630, 0.000000000000000000 ) ) ;
#74657=CARTESIAN_POINT ( 'NONE',  ( 1.666666666666667185, -0.004921259842519576551, 0.3153832671262227771 ) ) ;
#74661=CARTESIAN_POINT ( 'NONE',  ( 0.3034644639079869255, -3.790565315793794774E-16, -0.3791475997938105191 ) ) ;
#74663=CARTESIAN_POINT ( 'NONE',  ( 1.043307086614173818, -0.5400638737290845981, -0.3530559997133363437 ) ) ;
#74664=CARTESIAN_POINT ( 'NONE',  ( -0.7874015748031489847, -0.1870078740157480879, -0.4822834645669291653 ) ) ;
#74665=CARTESIAN_POINT ( 'NONE',  ( -0.6824146981627291497, -0.6046776061558809534, -0.2411417322834644161 ) ) ;
#74666=CARTESIAN_POINT ( 'NONE',  ( 0.7217847769028878924, -0.4281496062992127816, -0.4176697321401328100 ) ) ;
#74667=CARTESIAN_POINT ( 'NONE',  ( 1.200787401574803681, -0.5400638737290845981, -0.3530559997133363437 ) ) ;
#74668=CARTESIAN_POINT ( 'NONE',  ( 1.640419947506562393, -0.3690944881889763329, 0.3153832671262228327 ) ) ;
#74670=CARTESIAN_POINT ( 'NONE',  ( 1.200787401574803681, 0.07958543189024085140, 0.2665933059059887866 ) ) ;
#74672=CARTESIAN_POINT ( 'NONE',  ( -1.200787401574802349, -0.4536011799217367080, 0.2665933059059888421 ) ) ;
#74673=CARTESIAN_POINT ( 'NONE',  ( 0.3083989501312343062, -0.05778040916215560624, -0.4822834645669293319 ) ) ;
#74674=CARTESIAN_POINT ( 'NONE',  ( 1.056430446194226658, 0.2952755905511811885, 0.1292274648535926551 ) ) ;
#74675=DIRECTION ( 'NONE',  ( 0.000000000000000000, -1.000000000000000000, 0.000000000000000000 ) ) ;
#74676=CARTESIAN_POINT ( 'NONE',  ( -1.364829396325458521, 0.1283753931104746893, -0.1820866141732285504 ) ) ;
#74677=CARTESIAN_POINT ( 'NONE',  ( 0.2559055118110243332, 0.1660481256975885056, 0.3530559997133364547 ) ) ;
#74678=CARTESIAN_POINT ( 'NONE',  ( 1.443569553805774897, 0.1283753931104748280, 0.1820866141732283561 ) ) ;
#74680=CARTESIAN_POINT ( 'NONE',  ( -1.318897637795274802, -0.4536011799217368745, -0.2665933059059886201 ) ) ;
#74681=CARTESIAN_POINT ( 'NONE',  ( 1.541994750656168645, 0.2952755905511810774, -0.1292274648535930714 ) ) ;
#74683=CARTESIAN_POINT ( 'NONE',  ( 0.08530183727034192087, -0.2845877964562161244, -0.3641732283464567121 ) ) ;
#74684=CARTESIAN_POINT ( 'NONE',  ( -0.1640419947506555343, -0.3162353388693405765, 0.4822834645669290543 ) ) ;
#74685=CARTESIAN_POINT ( 'NONE',  ( -1.266404199475064773, -0.08942795157528024563, -0.3641732283464568787 ) ) ;
#74686=CARTESIAN_POINT ( 'NONE',  ( -0.8005249343832013809, -0.4281496062992124485, 0.4176697321401328655 ) ) ;
#74687=CARTESIAN_POINT ( 'NONE',  ( 1.515748031496063408, 0.1660481256975885056, 0.3530559997133364547 ) ) ;
#74690=CARTESIAN_POINT ( 'NONE',  ( 1.272965879265092637, 0.05413385826771666132, 0.4176697321401328100 ) ) ;
#74693=CARTESIAN_POINT ( 'NONE',  ( -1.128608923884513837, -0.6046776061558807314, 0.2411417322834647770 ) ) ;
#74694=CARTESIAN_POINT ( 'NONE',  ( -1.174540682414697335, -0.08942795157527998196, 0.3641732283464567121 ) ) ;
#74695=CARTESIAN_POINT ( 'NONE',  ( -0.6824146981627291497, -0.5023911411419708095, -0.1820866141732282451 ) ) ;
#74696=CARTESIAN_POINT ( 'NONE',  ( -1.220472440944882386, -0.1870078740157480046, 1.254653134982923898E-17 ) ) ;
#74697=CARTESIAN_POINT ( 'NONE',  ( -0.09186351706036663400, -0.4281496062992124485, 0.4176697321401328655 ) ) ;
#74698=CARTESIAN_POINT ( 'NONE',  ( 0.1771653543307093182, -0.4536011799217368745, -0.2665933059059886201 ) ) ;
#74699=CARTESIAN_POINT ( 'NONE',  ( -0.9383202099737524282, -0.08942795157527998196, 0.3641732283464567121 ) ) ;
#74700=CARTESIAN_POINT ( 'NONE',  ( -1.646981627296586703, -0.3162353388693409650, -0.4822834645669289433 ) ) ;
#74701=CARTESIAN_POINT ( 'NONE',  ( 1.535433070866142335, -0.5511811023622047445, 6.969142054262312111E-17 ) ) ;
#74702=CARTESIAN_POINT ( 'NONE',  ( 1.443569553805774897, -0.6046776061558809534, -0.2411417322834644161 ) ) ;
#74704=CARTESIAN_POINT ( 'NONE',  ( 0.4986876640419954376, -0.5023911411419708095, -0.1820866141732282451 ) ) ;
#74705=CARTESIAN_POINT ( 'NONE',  ( 0.9580052493438327987, -0.4281496062992127816, -0.4176697321401328100 ) ) ;
#74706=CARTESIAN_POINT ( 'NONE',  ( 1.154855643044620184, 0.1283753931104746893, -0.1820866141732285504 ) ) ;
#74708=CARTESIAN_POINT ( 'NONE',  ( -1.384514435695537005, -0.6692913385826773087, -0.1292274648535924053 ) ) ;
#74709=CARTESIAN_POINT ( 'NONE',  ( -1.030183727034119867, -0.3162353388693405765, 0.4822834645669290543 ) ) ;
#74710=CARTESIAN_POINT ( 'NONE',  ( -0.04593175853018302557, -0.6692913385826773087, -0.1292274648535924053 ) ) ;
#74711=CARTESIAN_POINT ( 'NONE',  ( 0.5392480709929744487, -4.069555009745408348E-17, -0.3627989612356148363 ) ) ;
#74713=CARTESIAN_POINT ( 'NONE',  ( 0.7611548556430451917, -0.6046776061558807314, 0.2411417322834647770 ) ) ;
#74714=CARTESIAN_POINT ( 'NONE',  ( 1.397637795275591177, -0.4536011799217367080, 0.2665933059059888421 ) ) ;
#74715=CARTESIAN_POINT ( 'NONE',  ( 0.2034120734908144990, -0.6692913385826771977, 0.1292274648535927661 ) ) ;
#74716=CARTESIAN_POINT ( 'NONE',  ( 0.6824146981627303710, 0.2306618581243847221, -0.2411417322834647770 ) ) ;
#74720=CARTESIAN_POINT ( 'NONE',  ( -0.7478466213799872531, 1.968503937007873850, -0.5309055118110235227 ) ) ;
#74722=CARTESIAN_POINT ( 'NONE',  ( -0.5708661417322828946, 0.07958543189024071263, -0.2665933059059888421 ) ) ;
#74723=CARTESIAN_POINT ( 'NONE',  ( -0.5708661417322828946, 0.1660481256975883668, -0.3530559997133364547 ) ) ;
#74724=CARTESIAN_POINT ( 'NONE',  ( 0.2624671916010504757, -0.6046776061558809534, -0.2411417322834644161 ) ) ;
#74726=CARTESIAN_POINT ( 'NONE',  ( -1.555118110236219930, -0.5400638737290845981, -0.3530559997133363437 ) ) ;
#74727=CARTESIAN_POINT ( 'NONE',  ( 0.9908136482939640111, 0.2952755905511810774, -0.1292274648535930714 ) ) ;
#74730=CARTESIAN_POINT ( 'NONE',  ( 1.135170603674541256, 0.2952755905511811885, 0.1292274648535926551 ) ) ;
#74732=CARTESIAN_POINT ( 'NONE',  ( 1.030183727034121421, -0.3162353388693409650, -0.4822834645669289433 ) ) ;
#74733=CARTESIAN_POINT ( 'NONE',  ( 1.154855643044620184, 0.1283753931104746893, -0.1820866141732285504 ) ) ;
#74734=CARTESIAN_POINT ( 'NONE',  ( -1.640419947506561060, -0.004921259842519576551, 0.3153832671262227771 ) ) ;
#74735=CARTESIAN_POINT ( 'NONE',  ( -1.535433070866141225, -0.6692913385826771977, 8.415575281601705876E-17 ) ) ;
#74738=CARTESIAN_POINT ( 'NONE',  ( 0.8792650918635177559, 0.05413385826771666132, 0.4176697321401328100 ) ) ;
#74739=CARTESIAN_POINT ( 'NONE',  ( 1.358267716535433323, 0.07958543189024085140, 0.2665933059059887866 ) ) ;
#74740=CARTESIAN_POINT ( 'NONE',  ( -0.6627296587926503335, -0.6692913385826771977, 0.1292274648535927661 ) ) ;
#74741=CARTESIAN_POINT ( 'NONE',  ( -0.4396325459317579898, 0.2952755905511811885, 0.1292274648535926551 ) ) ;
#74742=CARTESIAN_POINT ( 'NONE',  ( -1.587926509186350810, 0.05413385826771626580, -0.4176697321401330321 ) ) ;
#74744=CARTESIAN_POINT ( 'NONE',  ( 0.2755905511811031494, -0.6692913385826771977, 8.415575281601705876E-17 ) ) ;
#74747=CARTESIAN_POINT ( 'NONE',  ( 1.620734908136483465, -0.6692913385826771977, 0.1292274648535927661 ) ) ;
#74748=VERTEX_POINT ( 'NONE', #21679 ) ;
#74753=CARTESIAN_POINT ( 'NONE',  ( 1.614173228346457378, 0.1771653543307087630, 0.000000000000000000 ) ) ;
#74755=CARTESIAN_POINT ( 'NONE',  ( 1.581364829396326277, -0.2845877964562161244, -0.3641732283464567121 ) ) ;
#74756=CARTESIAN_POINT ( 'NONE',  ( -0.1447075906223733999, 0.004960608223778823628, 0.3437734562760190182 ) ) ;
#74760=CARTESIAN_POINT ( 'NONE',  ( -0.2559055118110227234, -0.4536011799217367080, 0.2665933059059888421 ) ) ;
#74761=CARTESIAN_POINT ( 'NONE',  ( -1.292650918635170010, -0.5511811023622046335, 0.09757992244046803654 ) ) ;
#74762=CARTESIAN_POINT ( 'NONE',  ( 1.502624671916010790, -0.3162353388693409650, -0.4822834645669289433 ) ) ;
#74763=CARTESIAN_POINT ( 'NONE',  ( 0.3740157480314966754, 0.1660481256975883668, -0.3530559997133364547 ) ) ;
#74764=CARTESIAN_POINT ( 'NONE',  ( -1.456692913385826182, 0.2952755905511811885, 0.000000000000000000 ) ) ;
#74768=CARTESIAN_POINT ( 'NONE',  ( 1.423884514435696191, -0.05778040916215522460, 0.4822834645669289988 ) ) ;
#74771=CARTESIAN_POINT ( 'NONE',  ( -1.646051170424378096, 0.4405861044731112508, -0.5309055118110234117 ) ) ;
#74773=PLANE ( 'NONE',  #11695 ) ;
#74774=CARTESIAN_POINT ( 'NONE',  ( -0.6036745406824141069, -0.6046776061558809534, -0.2411417322834644161 ) ) ;
#74775=CARTESIAN_POINT ( 'NONE',  ( 1.568241469816273659, -0.05778040916215560624, -0.4822834645669293319 ) ) ;
#74777=CARTESIAN_POINT ( 'NONE',  ( 0.6426939841807760567, 0.004960608223778823628, 0.3437734562760190182 ) ) ;
#74778=CARTESIAN_POINT ( 'NONE',  ( 1.541994750656168645, 0.2952755905511810774, -0.1292274648535930714 ) ) ;
#74779=CARTESIAN_POINT ( 'NONE',  ( -0.7808398950131225646, -0.05778040916215522460, 0.4822834645669289988 ) ) ;
#74781=CARTESIAN_POINT ( 'NONE',  ( -0.05249343832020938322, -0.5023911411419708095, -0.1820866141732282451 ) ) ;
#74783=CARTESIAN_POINT ( 'NONE',  ( 0.03937007874015833325, -0.5511811023622047445, 6.969142054262312111E-17 ) ) ;
#74784=CARTESIAN_POINT ( 'NONE',  ( 0.5511811023622054106, -0.1870078740157480601, -0.3641732283464567677 ) ) ;
#74785=CARTESIAN_POINT ( 'NONE',  ( 0.7152230971128614723, -0.3162353388693409650, -0.4822834645669289433 ) ) ;
#74786=CARTESIAN_POINT ( 'NONE',  ( -0.2887139107611542133, -0.5023911411419708095, -0.1820866141732282451 ) ) ;
#74788=CARTESIAN_POINT ( 'NONE',  ( 1.456692913385827515, 0.2952755905511811885, 0.000000000000000000 ) ) ;
#74790=CARTESIAN_POINT ( 'NONE',  ( -1.213910761154854745, -0.6692913385826771977, 0.1292274648535927661 ) ) ;
#74794=CARTESIAN_POINT ( 'NONE',  ( 5.463695987328526437E-16, -0.1870078740157479769, 0.4822834645669291653 ) ) ;
#74796=CARTESIAN_POINT ( 'NONE',  ( -0.3083989501312330295, -0.3162353388693409650, -0.4822834645669289433 ) ) ;
#74797=CARTESIAN_POINT ( 'NONE',  ( 1.646981627296588035, -0.2845877964562159024, 0.3641732283464567677 ) ) ;
#74798=CARTESIAN_POINT ( 'NONE',  ( 0.1509186351706042484, -0.2845877964562159024, 0.3641732283464567677 ) ) ;
#74799=CARTESIAN_POINT ( 'NONE',  ( -0.3674540682414692561, -0.6046776061558809534, -0.2411417322834644161 ) ) ;
#74800=CARTESIAN_POINT ( 'NONE',  ( -0.8202099737532799750, 0.2952755905511810774, -0.1292274648535930714 ) ) ;
#74802=CARTESIAN_POINT ( 'NONE',  ( 1.509186351706037543, -0.004921259842519576551, 0.3153832671262227771 ) ) ;
#74803=CARTESIAN_POINT ( 'NONE',  ( 0.3412073490813655186, -0.6046776061558809534, -0.2411417322834644161 ) ) ;
#74804=ORIENTED_EDGE ( 'NONE', *, *, #40435, .F. ) ;
#74806=CARTESIAN_POINT ( 'NONE',  ( 1.148293963254593653, 0.2952755905511810774, -0.1292274648535930714 ) ) ;
#74808=CARTESIAN_POINT ( 'NONE',  ( -0.6824146981627291497, -0.5023911411419708095, -0.1820866141732282451 ) ) ;
#74809=CONICAL_SURFACE ( 'NONE', #54595, 3.543307086614174484, 0.7853981633974447263 ) ;
#74810=CARTESIAN_POINT ( 'NONE',  ( -0.4265091863517051496, 0.2952755905511810774, -0.1292274648535930714 ) ) ;
#74811=CARTESIAN_POINT ( 'NONE',  ( 1.476377952755906442, -0.5400638737290844871, 0.3530559997133364547 ) ) ;
#74812=CARTESIAN_POINT ( 'NONE',  ( 0.9186351706036752773, 0.2306618581243847221, -0.2411417322834647770 ) ) ;
#74814=CARTESIAN_POINT ( 'NONE',  ( -1.102362204724408601, -0.1870078740157479769, 0.3641732283464567677 ) ) ;
#74818=CARTESIAN_POINT ( 'NONE',  ( 1.640419947506562393, -0.3690944881889763329, 0.3153832671262228327 ) ) ;
#74819=CARTESIAN_POINT ( 'NONE',  ( 1.023622047244095112, -0.1870078740157480601, -0.3641732283464567677 ) ) ;
#74820=CARTESIAN_POINT ( 'NONE',  ( 0.6430446194225728496, 0.05413385826771666132, 0.4176697321401328100 ) ) ;
#74821=CARTESIAN_POINT ( 'NONE',  ( -1.561679790026246017, 0.05413385826771666132, 0.4176697321401328100 ) ) ;
#74824=CARTESIAN_POINT ( 'NONE',  ( 0.9120734908136490793, 0.1771653543307087075, -0.09757992244046823083 ) ) ;
#74825=CARTESIAN_POINT ( 'NONE',  ( -0.2427821522309703550, -0.3162353388693405765, 0.4822834645669290543 ) ) ;
#74826=CARTESIAN_POINT ( 'NONE',  ( -0.6430446194225712953, 0.05413385826771626580, -0.4176697321401330321 ) ) ;
#74827=CARTESIAN_POINT ( 'NONE',  ( 1.299212598425197429, -0.6692913385826771977, 8.415575281601705876E-17 ) ) ;
#74830=CARTESIAN_POINT ( 'NONE',  ( -0.09842519685039295696, 0.07958543189024071263, -0.2665933059059888421 ) ) ;
#74835=CARTESIAN_POINT ( 'NONE',  ( -0.7217847769028863381, 0.05413385826771626580, -0.4176697321401330321 ) ) ;
#74836=CARTESIAN_POINT ( 'NONE',  ( -0.01312335958005186876, 0.05413385826771626580, -0.4176697321401330321 ) ) ;
#74837=CARTESIAN_POINT ( 'NONE',  ( -0.3083989501312330295, -0.3162353388693409650, -0.4822834645669289433 ) ) ;
#74838=CARTESIAN_POINT ( 'NONE',  ( 0.9448818897637802916, -0.1870078740157480879, -0.4822834645669291653 ) ) ;
#74839=CARTESIAN_POINT ( 'NONE',  ( -0.4921259842519677963, 0.1660481256975883668, -0.3530559997133364547 ) ) ;
#74840=CARTESIAN_POINT ( 'NONE',  ( -1.286089238845143479, 0.2306618581243847221, -0.2411417322834647770 ) ) ;
#74841=CARTESIAN_POINT ( 'NONE',  ( -0.5118110236220466680, -0.6692913385826771977, 8.415575281601705876E-17 ) ) ;
#74842=CARTESIAN_POINT ( 'NONE',  ( 0.8070866141732288002, 0.1660481256975885056, 0.3530559997133364547 ) ) ;
#74843=CARTESIAN_POINT ( 'NONE',  ( 0.6364829396325465405, -0.05778040916215522460, 0.4822834645669289988 ) ) ;
#74846=CARTESIAN_POINT ( 'NONE',  ( -0.3149606299212590610, -0.1870078740157480601, -0.3641732283464567677 ) ) ;
#74850=CARTESIAN_POINT ( 'NONE',  ( -1.469816272965878357, -0.5023911411419708095, -0.1820866141732282451 ) ) ;
#74853=CARTESIAN_POINT ( 'NONE',  ( -0.6036745406824141069, -0.6046776061558809534, -0.2411417322834644161 ) ) ;
#74855=CARTESIAN_POINT ( 'NONE',  ( -0.7283464566929126471, 0.1660481256975883668, -0.3530559997133364547 ) ) ;
#74856=CARTESIAN_POINT ( 'NONE',  ( -0.6692913385826764205, -0.6692913385826771977, 8.415575281601705876E-17 ) ) ;
#74857=CARTESIAN_POINT ( 'NONE',  ( -1.213910761154854745, -0.6692913385826771977, 0.1292274648535927661 ) ) ;
#74858=CARTESIAN_POINT ( 'NONE',  ( -1.732283464566928277, -0.1870078740157479769, 0.4822834645669291653 ) ) ;
#74859=CARTESIAN_POINT ( 'NONE',  ( 1.023622047244095334, -0.1870078740157479769, 0.3641732283464567677 ) ) ;
#74862=CARTESIAN_POINT ( 'NONE',  ( 0.02624671916010564918, 0.1283753931104748280, 0.1820866141732283561 ) ) ;
#74863=CARTESIAN_POINT ( 'NONE',  ( -0.3871391076115476282, -0.05778040916215522460, 0.4822834645669289988 ) ) ;
#74864=CARTESIAN_POINT ( 'NONE',  ( -0.1509186351706028884, -0.3162353388693409650, -0.4822834645669289433 ) ) ;
#74867=CARTESIAN_POINT ( 'NONE',  ( 0.2465595919007004533, 6.148515279637353769E-16, 0.4281993546915524584 ) ) ;
#74871=CARTESIAN_POINT ( 'NONE',  ( -0.5839895013123351797, 0.1771653543307087075, -0.09757992244046823083 ) ) ;
#74872=CARTESIAN_POINT ( 'NONE',  ( -0.9186351706036736120, 0.2306618581243848609, 0.2411417322834645549 ) ) ;
#74874=FACE_OUTER_BOUND ( 'NONE', #12612, .T. ) ;
#74876=CARTESIAN_POINT ( 'NONE',  ( 1.246719160104987623, 0.05413385826771626580, -0.4176697321401330321 ) ) ;
#74877=CARTESIAN_POINT ( 'NONE',  ( 0.6430446194225728496, 0.05413385826771666132, 0.4176697321401328100 ) ) ;
#74878=CARTESIAN_POINT ( 'NONE',  ( 0.5183727034120741983, -0.6692913385826771977, 0.1292274648535927661 ) ) ;
#74879=CARTESIAN_POINT ( 'NONE',  ( -0.4527559055118102749, -0.4536011799217368745, -0.2665933059059886201 ) ) ;
#74880=CARTESIAN_POINT ( 'NONE',  ( -0.5052493438320203589, -0.6692913385826771977, 0.1292274648535927661 ) ) ;
#74882=CARTESIAN_POINT ( 'NONE',  ( -0.2952755905511804668, 0.1660481256975885056, 0.3530559997133364547 ) ) ;
#74884=CARTESIAN_POINT ( 'NONE',  ( 1.443569553805774897, 0.1283753931104748280, 0.1820866141732283561 ) ) ;
#74885=CARTESIAN_POINT ( 'NONE',  ( -0.3215223097112853146, -0.2845877964562159024, 0.3641732283464567677 ) ) ;
#74886=CARTESIAN_POINT ( 'NONE',  ( 1.259842519685040019, -0.1870078740157480601, -0.3641732283464567677 ) ) ;
#74887=CARTESIAN_POINT ( 'NONE',  ( -1.528871391076114250, 0.2952755905511810774, -0.1292274648535930714 ) ) ;
#74888=CARTESIAN_POINT ( 'NONE',  ( -1.003937007874014853, 0.07958543189024085140, 0.2665933059059887866 ) ) ;
#74889=CARTESIAN_POINT ( 'NONE',  ( 1.614173228346457378, 0.2952755905511811885, 0.000000000000000000 ) ) ;
#74890=CARTESIAN_POINT ( 'NONE',  ( -1.305774278215222184, -0.6692913385826773087, -0.1292274648535924053 ) ) ;
#74891=CARTESIAN_POINT ( 'NONE',  ( -0.4002624671916004129, -0.3162353388693405765, 0.4822834645669290543 ) ) ;
#74893=CARTESIAN_POINT ( 'NONE',  ( 0.3871391076115493490, -0.2845877964562159024, 0.3641732283464567677 ) ) ;
#74894=CARTESIAN_POINT ( 'NONE',  ( -1.502624671916009680, -0.08942795157528024563, -0.3641732283464568787 ) ) ;
#74895=CARTESIAN_POINT ( 'NONE',  ( 0.6233595800524942554, -0.05778040916215560624, -0.4822834645669293319 ) ) ;
#74896=CARTESIAN_POINT ( 'NONE',  ( -1.699475065616797398, 0.1771653543307087630, 0.09757992244046791164 ) ) ;
#74897=CARTESIAN_POINT ( 'NONE',  ( 1.377952755905512472, -0.5511811023622047445, 6.969142054262312111E-17 ) ) ;
#74898=CARTESIAN_POINT ( 'NONE',  ( -1.082677165354329896, 0.1660481256975885056, 0.3530559997133364547 ) ) ;
#74899=CARTESIAN_POINT ( 'NONE',  ( -0.4790026246719152336, -0.08942795157528024563, -0.3641732283464568787 ) ) ;
#74901=CARTESIAN_POINT ( 'NONE',  ( 0.2887139107611556010, -0.5023911411419708095, 0.1820866141732285504 ) ) ;
#74902=CARTESIAN_POINT ( 'NONE',  ( -0.09842519685039295696, -0.5400638737290844871, 0.3530559997133364547 ) ) ;
#74906=CARTESIAN_POINT ( 'NONE',  ( 0.7414698162729663755, -0.5511811023622048555, -0.09757992244046775898 ) ) ;
#74907=CARTESIAN_POINT ( 'NONE',  ( 0.08530183727034192087, -0.05778040916215522460, 0.4822834645669289988 ) ) ;
#74908=VECTOR ( 'NONE', #41312, 39.37007874015748143 ) ;
#74910=CARTESIAN_POINT ( 'NONE',  ( -0.7742782152230962556, -0.4281496062992127816, -0.4176697321401328100 ) ) ;
#74911=CARTESIAN_POINT ( 'NONE',  ( -0.8005249343832011588, -0.004921259842519870586, -0.3153832671262229437 ) ) ;
#74913=CARTESIAN_POINT ( 'NONE',  ( -0.4658792650918627265, -0.2845877964562161244, -0.3641732283464567121 ) ) ;
#74914=CARTESIAN_POINT ( 'NONE',  ( -0.1574803149606292529, -0.1870078740157480879, -0.4822834645669291653 ) ) ;
#74915=EDGE_CURVE ( 'NONE', #44566, #13764, #5097, .T. ) ;
#74916=CARTESIAN_POINT ( 'NONE',  ( -1.174540682414697335, -0.2845877964562161244, -0.3641732283464567121 ) ) ;
#74918=CARTESIAN_POINT ( 'NONE',  ( -1.601049868766403650, 0.2306618581243847221, -0.2411417322834647770 ) ) ;
#74919=CARTESIAN_POINT ( 'NONE',  ( 0.4621018179204952614, 1.702998256715020864E-15, -0.4281989832122452544 ) ) ;
#74920=ORIENTED_EDGE ( 'NONE', *, *, #69249, .T. ) ;
#74921=ADVANCED_FACE ( 'NONE', ( #27992 ), #28407, .F. ) ;
#74922=CARTESIAN_POINT ( 'NONE',  ( -1.489501312335957062, -0.2845877964562161244, -0.3641732283464567121 ) ) ;
#74923=CARTESIAN_POINT ( 'NONE',  ( -0.3280839895013117347, -0.4281496062992124485, 0.4176697321401328655 ) ) ;
#74924=CARTESIAN_POINT ( 'NONE',  ( -1.023622047244093558, -0.1870078740157479769, 0.4822834645669291653 ) ) ;
#74927=CARTESIAN_POINT ( 'NONE',  ( 1.194225721784777594, 0.05413385826771666132, 0.4176697321401328100 ) ) ;
#74928=CARTESIAN_POINT ( 'NONE',  ( 0.4133858267716541968, 0.1660481256975885056, 0.3530559997133364547 ) ) ;
#74931=CARTESIAN_POINT ( 'NONE',  ( 1.515748031496063186, -0.4536011799217368745, -0.2665933059059886201 ) ) ;
#74933=ORIENTED_EDGE ( 'NONE', *, *, #32543, .T. ) ;
#74934=CARTESIAN_POINT ( 'NONE',  ( -0.7545931758530176614, -0.5511811023622048555, -0.09757992244046775898 ) ) ;
#74937=CARTESIAN_POINT ( 'NONE',  ( 0.5380577427821529035, 0.05413385826771626580, -0.4176697321401330321 ) ) ;
#74938=CARTESIAN_POINT ( 'NONE',  ( -0.5708661417322828946, 0.1660481256975883668, -0.3530559997133364547 ) ) ;
#74939=CARTESIAN_POINT ( 'NONE',  ( -1.200787401574802349, -0.5400638737290844871, 0.3530559997133364547 ) ) ;
#74940=CARTESIAN_POINT ( 'NONE',  ( 0.8595800524934390507, -0.3162353388693405765, 0.4822834645669290543 ) ) ;
#74941=CARTESIAN_POINT ( 'NONE',  ( -1.423884514435694859, -0.08942795157528024563, -0.3641732283464568787 ) ) ;
#74943=CARTESIAN_POINT ( 'NONE',  ( -0.04593175853018302557, 0.2952755905511811885, 0.1292274648535926551 ) ) ;
#74944=CARTESIAN_POINT ( 'NONE',  ( -1.286089238845143479, 0.2306618581243847221, -0.2411417322834647770 ) ) ;
#74946=CARTESIAN_POINT ( 'NONE',  ( -1.620734908136482577, 0.2952755905511811885, 0.1292274648535926551 ) ) ;
#74949=CARTESIAN_POINT ( 'NONE',  ( 0.9186351706036752773, 0.1283753931104746893, -0.1820866141732285504 ) ) ;
#74950=ORIENTED_EDGE ( 'NONE', *, *, #16635, .F. ) ;
#74952=CARTESIAN_POINT ( 'NONE',  ( -0.9908136482939626788, 0.2952755905511811885, 0.1292274648535926551 ) ) ;
#74954=CARTESIAN_POINT ( 'NONE',  ( -0.1115485564304456306, 0.1771653543307087075, -0.09757992244046823083 ) ) ;
#74955=CARTESIAN_POINT ( 'NONE',  ( -1.594488188976377563, -0.5400638737290844871, 0.3530559997133364547 ) ) ;
#74956=CARTESIAN_POINT ( 'NONE',  ( 0.4724409448818904789, -0.1870078740157479769, 0.4822834645669291653 ) ) ;
#74957=CARTESIAN_POINT ( 'NONE',  ( 0.3018372703412079971, -0.4281496062992124485, 0.4176697321401328655 ) ) ;
#74958=CARTESIAN_POINT ( 'NONE',  ( -0.2821522309711278487, 0.2952755905511811885, 0.1292274648535926551 ) ) ;
#74960=CARTESIAN_POINT ( 'NONE',  ( -0.6364829396325453192, -0.05778040916215560624, -0.4822834645669293319 ) ) ;
#74962=CARTESIAN_POINT ( 'NONE',  ( 1.522309711286089939, -0.5023911411419708095, -0.1820866141732282451 ) ) ;
#74963=CARTESIAN_POINT ( 'NONE',  ( -1.062992125984250968, -0.6692913385826771977, 8.415575281601705876E-17 ) ) ;
#74964=CARTESIAN_POINT ( 'NONE',  ( 0.8727034120734913358, -0.05778040916215522460, 0.4822834645669289988 ) ) ;
#74965=CARTESIAN_POINT ( 'NONE',  ( 1.299212598425197429, -0.6692913385826771977, 8.415575281601705876E-17 ) ) ;
#74967=CARTESIAN_POINT ( 'NONE',  ( -0.8989501312335946848, 0.2952755905511810774, -0.1292274648535930714 ) ) ;
#74969=CARTESIAN_POINT ( 'NONE',  ( 0.2624671916010504757, -0.6046776061558809534, -0.2411417322834644161 ) ) ;
#74971=CARTESIAN_POINT ( 'NONE',  ( -0.6561679790026240244, 0.2306618581243847221, -0.2411417322834647770 ) ) ;
#74973=CARTESIAN_POINT ( 'NONE',  ( -1.535433070866141225, -0.5511811023622047445, 6.969142054262312111E-17 ) ) ;
#74974=CARTESIAN_POINT ( 'NONE',  ( 0.5446194225721792126, -0.2845877964562159024, 0.3641732283464567677 ) ) ;
#74975=CARTESIAN_POINT ( 'NONE',  ( 1.266404199475066328, -0.05778040916215522460, 0.4822834645669289988 ) ) ;
#74977=CARTESIAN_POINT ( 'NONE',  ( 0.9055118110236227702, 0.1771653543307087630, 0.000000000000000000 ) ) ;
#74978=CARTESIAN_POINT ( 'NONE',  ( 0.8464566929133865436, 0.1660481256975883668, -0.3530559997133364547 ) ) ;
#74980=CARTESIAN_POINT ( 'NONE',  ( -0.6627296587926503335, -0.6692913385826771977, 0.1292274648535927661 ) ) ;
#74982=CARTESIAN_POINT ( 'NONE',  ( 0.8267716535433077274, 0.1771653543307087630, 0.000000000000000000 ) ) ;
#74983=CARTESIAN_POINT ( 'NONE',  ( -0.6102362204724400829, 0.1660481256975885056, 0.3530559997133364547 ) ) ;
#74984=CARTESIAN_POINT ( 'NONE',  ( -0.07217847769028813698, -0.3162353388693409650, -0.4822834645669289433 ) ) ;
#74986=CARTESIAN_POINT ( 'NONE',  ( 0.03937007874015806264, 0.2952755905511811885, 0.000000000000000000 ) ) ;
#74987=CARTESIAN_POINT ( 'NONE',  ( 0.1443569553805781891, -0.004921259842519870586, -0.3153832671262229437 ) ) ;
#74989=CARTESIAN_POINT ( 'NONE',  ( 0.1902887139107617975, -0.5511811023622048555, -0.09757992244046775898 ) ) ;
#74990=CARTESIAN_POINT ( 'NONE',  ( 0.5446194225721792126, -0.08942795157528024563, -0.3641732283464568787 ) ) ;
#74993=CARTESIAN_POINT ( 'NONE',  ( 0.3871391076115493490, -0.3162353388693405765, 0.4822834645669290543 ) ) ;
#74995=CARTESIAN_POINT ( 'NONE',  ( 0.2247243262887798632, -4.135162568743707313E-16, -0.3791483426435169890 ) ) ;
#74997=CARTESIAN_POINT ( 'NONE',  ( -0.3477690288713905509, -0.5511811023622046335, 0.09757992244046803654 ) ) ;
#74998=CARTESIAN_POINT ( 'NONE',  ( -0.2559055118110227234, -0.5400638737290844871, 0.3530559997133364547 ) ) ;
#74999=CARTESIAN_POINT ( 'NONE',  ( 1.030183727034121421, -0.08942795157527998196, 0.3641732283464567121 ) ) ;
#75001=CARTESIAN_POINT ( 'NONE',  ( -1.397637795275589623, 0.1660481256975885056, 0.3530559997133364547 ) ) ;
#75002=CARTESIAN_POINT ( 'NONE',  ( 0.2230971128608932319, -0.4281496062992124485, 0.4176697321401328655 ) ) ;
#75003=CARTESIAN_POINT ( 'NONE',  ( 1.364829396325460076, 0.2306618581243848609, 0.2411417322834645549 ) ) ;
#75005=CARTESIAN_POINT ( 'NONE',  ( 0.2230971128608929543, 0.05413385826771626580, -0.4176697321401330321 ) ) ;
#75006=CARTESIAN_POINT ( 'NONE',  ( 1.515748031496063408, 0.1660481256975885056, 0.3530559997133364547 ) ) ;
#75007=CARTESIAN_POINT ( 'NONE',  ( 0.3477690288713918276, -0.6692913385826773087, -0.1292274648535924053 ) ) ;
#75008=CARTESIAN_POINT ( 'NONE',  ( -1.603475055217291612, 1.330568129716839909, 0.04573490813648253134 ) ) ;
#75009=CARTESIAN_POINT ( 'NONE',  ( 0.8333333333333340365, -0.5511811023622046335, 0.09757992244046803654 ) ) ;
#75010=CARTESIAN_POINT ( 'NONE',  ( 1.404199475065617708, 0.05413385826771626580, -0.4176697321401330321 ) ) ;
#75011=EDGE_CURVE ( 'NONE', #3706, #36535, #80340, .T. ) ;
#75012=CARTESIAN_POINT ( 'NONE',  ( 0.1640419947506569498, -0.08942795157527998196, 0.3641732283464567121 ) ) ;
#75013=CARTESIAN_POINT ( 'NONE',  ( -0.4133858267716528645, -0.5400638737290844871, 0.3530559997133364547 ) ) ;
#75014=CARTESIAN_POINT ( 'NONE',  ( 0.4921259842519691285, 0.1660481256975885056, 0.3530559997133364547 ) ) ;
#75015=CARTESIAN_POINT ( 'NONE',  ( -0.2165354330708654795, 0.1660481256975885056, 0.3530559997133364547 ) ) ;
#75017=CARTESIAN_POINT ( 'NONE',  ( -0.4068241469816267775, -0.004921259842519870586, -0.3153832671262229437 ) ) ;
#75018=CARTESIAN_POINT ( 'NONE',  ( 0.8923884514435701520, -0.6046776061558809534, -0.2411417322834644161 ) ) ;
#75019=CARTESIAN_POINT ( 'NONE',  ( 0.9908136482939640111, -0.5511811023622046335, 0.09757992244046803654 ) ) ;
#75020=CARTESIAN_POINT ( 'NONE',  ( 0.04593175853018440641, -0.6692913385826771977, 0.1292274648535927661 ) ) ;
#75023=CARTESIAN_POINT ( 'NONE',  ( 1.594488188976378673, 0.1660481256975885056, 0.3530559997133364547 ) ) ;
#75026=CARTESIAN_POINT ( 'NONE',  ( -1.325459317585300889, 0.05413385826771666132, 0.4176697321401328100 ) ) ;
#75027=CARTESIAN_POINT ( 'NONE',  ( -0.5774278215223089816, 0.2306618581243847221, -0.2411417322834647770 ) ) ;
#75030=ORIENTED_EDGE ( 'NONE', *, *, #12573, .F. ) ;
#75031=CARTESIAN_POINT ( 'NONE',  ( 0.4790026246719168435, -0.2845877964562161244, -0.3641732283464567121 ) ) ;
#75033=CARTESIAN_POINT ( 'NONE',  ( 0.7677165354330716118, -0.5400638737290844871, 0.3530559997133364547 ) ) ;
#75036=CARTESIAN_POINT ( 'NONE',  ( 1.174540682414699111, -0.3162353388693405765, 0.4822834645669290543 ) ) ;
#75037=CARTESIAN_POINT ( 'NONE',  ( 1.167979002624672580, -0.004921259842519870586, -0.3153832671262229437 ) ) ;
#75038=CARTESIAN_POINT ( 'NONE',  ( 0.4396325459317593221, 0.2952755905511810774, -0.1292274648535930714 ) ) ;
#75040=CARTESIAN_POINT ( 'NONE',  ( -0.3280839895013117347, 0.05413385826771626580, -0.4176697321401330321 ) ) ;
#75041=CARTESIAN_POINT ( 'NONE',  ( -0.9383202099737524282, -0.08942795157527998196, 0.3641732283464567121 ) ) ;
#75042=CARTESIAN_POINT ( 'NONE',  ( 0.2624671916010504757, -0.6046776061558809534, -0.2411417322834644161 ) ) ;
#75043=CARTESIAN_POINT ( 'NONE',  ( 0.05905511811023681640, 0.1660481256975883668, -0.3530559997133364547 ) ) ;
#75045=PLANE ( 'NONE',  #58391 ) ;
#75047=CARTESIAN_POINT ( 'NONE',  ( 1.010498687664042716, -0.4281496062992124485, 0.4176697321401328655 ) ) ;
#75048=CARTESIAN_POINT ( 'NONE',  ( -0.2821522309711278487, 0.2952755905511811885, 0.1292274648535926551 ) ) ;
#75049=CARTESIAN_POINT ( 'NONE',  ( -1.397637795275589623, -0.5400638737290845981, -0.3530559997133363437 ) ) ;
#75050=CARTESIAN_POINT ( 'NONE',  ( 1.299212598425197429, 0.2952755905511811885, 0.000000000000000000 ) ) ;
#75051=CARTESIAN_POINT ( 'NONE',  ( 0.3280839895013130669, -0.4281496062992127816, -0.4176697321401328100 ) ) ;
#75053=CARTESIAN_POINT ( 'NONE',  ( -0.8727034120734901146, -0.05778040916215560624, -0.4822834645669293319 ) ) ;
#75054=CARTESIAN_POINT ( 'NONE',  ( 0.05905511811023709395, -0.5400638737290844871, 0.3530559997133364547 ) ) ;
#75055=CARTESIAN_POINT ( 'NONE',  ( -0.5183727034120726440, 0.2952755905511811885, 0.1292274648535926551 ) ) ;
#75056=CARTESIAN_POINT ( 'NONE',  ( 0.3412073490813655186, -0.5023911411419708095, -0.1820866141732282451 ) ) ;
#75057=CARTESIAN_POINT ( 'NONE',  ( -1.725721784776902190, -0.05778040916215522460, 0.4822834645669289988 ) ) ;
#75058=CARTESIAN_POINT ( 'NONE',  ( -1.692913385826770645, 0.2952755905511811885, 0.000000000000000000 ) ) ;
#75059=CARTESIAN_POINT ( 'NONE',  ( 0.3018372703412079971, -0.4281496062992124485, 0.4176697321401328655 ) ) ;
#75060=CARTESIAN_POINT ( 'NONE',  ( 1.423884514435696191, -0.05778040916215522460, 0.4822834645669289988 ) ) ;
#75062=ORIENTED_EDGE ( 'NONE', *, *, #51779, .F. ) ;
#75064=CARTESIAN_POINT ( 'NONE',  ( 0.8661417322834653598, -0.1870078740157479769, 0.4822834645669291653 ) ) ;
#75065=CARTESIAN_POINT ( 'NONE',  ( 0.01968503937007930540, 0.07958543189024085140, 0.2665933059059887866 ) ) ;
#75072=CARTESIAN_POINT ( 'NONE',  ( 0.6299212598425204535, -0.1870078740157479769, 0.4822834645669291653 ) ) ;
#75073=CARTESIAN_POINT ( 'NONE',  ( -0.6102362204724400829, -0.5400638737290845981, -0.3530559997133363437 ) ) ;
#75074=CARTESIAN_POINT ( 'NONE',  ( -0.9251968503937002541, 0.1660481256975885056, 0.3530559997133364547 ) ) ;
#75075=CARTESIAN_POINT ( 'NONE',  ( 0.6430446194225728496, 0.05413385826771666132, 0.4176697321401328100 ) ) ;
#75076=CARTESIAN_POINT ( 'NONE',  ( 1.496062992125984703, -0.1870078740157480879, -0.4822834645669291653 ) ) ;
#75077=CARTESIAN_POINT ( 'NONE',  ( 1.181102362204725198, -0.1870078740157479769, 0.3641732283464567677 ) ) ;
#75078=CARTESIAN_POINT ( 'NONE',  ( 1.227034120734908917, 0.1771653543307087075, -0.09757992244046823083 ) ) ;
#75079=CARTESIAN_POINT ( 'NONE',  ( -0.8989501312335946848, -0.6692913385826771977, 0.1292274648535927661 ) ) ;
#75081=CARTESIAN_POINT ( 'NONE',  ( -1.561679790026246017, -0.3690944881889765550, -0.3153832671262227771 ) ) ;
#75083=CARTESIAN_POINT ( 'NONE',  ( -0.3477690288713902178, 0.2952755905511810774, -0.1292274648535930714 ) ) ;
#75084=CARTESIAN_POINT ( 'NONE',  ( 1.017060367454068803, -0.3162353388693405765, 0.4822834645669290543 ) ) ;
#75085=CARTESIAN_POINT ( 'NONE',  ( -0.7080320533160967544, 1.900312960331933976, 0.5309055118110236338 ) ) ;
#75086=CARTESIAN_POINT ( 'NONE',  ( -1.253280839895012377, -0.08942795157527998196, 0.3641732283464567121 ) ) ;
#75087=CARTESIAN_POINT ( 'NONE',  ( 0.4855643044619430415, -0.4281496062992127816, -0.4176697321401328100 ) ) ;
#75088=CARTESIAN_POINT ( 'NONE',  ( 0.9514435695538062676, -0.08942795157527998196, 0.3641732283464567121 ) ) ;
#75090=CARTESIAN_POINT ( 'NONE',  ( -1.404199475065615932, -0.004921259842519576551, 0.3153832671262227771 ) ) ;
#75091=CARTESIAN_POINT ( 'NONE',  ( 1.286089238845145033, -0.6046776061558809534, -0.2411417322834644161 ) ) ;
#75093=CARTESIAN_POINT ( 'NONE',  ( -0.6627296587926503335, -0.5511811023622046335, 0.09757992244046803654 ) ) ;
#75094=CARTESIAN_POINT ( 'NONE',  ( -0.1246719160104980823, 0.2952755905511811885, 0.1292274648535926551 ) ) ;
#75095=CARTESIAN_POINT ( 'NONE',  ( -1.463254593175852492, 0.1771653543307087630, 0.09757992244046791164 ) ) ;
#75096=CARTESIAN_POINT ( 'NONE',  ( -0.6233595800524928121, -0.05778040916215522460, 0.4822834645669289988 ) ) ;
#75097=CARTESIAN_POINT ( 'NONE',  ( 1.233595800524935227, 0.2306618581243847221, -0.2411417322834647770 ) ) ;
#75099=CARTESIAN_POINT ( 'NONE',  ( -0.8464566929133852113, 0.07958543189024085140, 0.2665933059059887866 ) ) ;
#75102=CARTESIAN_POINT ( 'NONE',  ( 1.548556430446194954, -0.6046776061558807314, 0.2411417322834647770 ) ) ;
#75104=CARTESIAN_POINT ( 'NONE',  ( -1.227034120734907585, 0.2952755905511811885, 0.1292274648535926551 ) ) ;
#75105=CARTESIAN_POINT ( 'NONE',  ( -1.286089238845143479, 0.1283753931104746893, -0.1820866141732285504 ) ) ;
#75106=CARTESIAN_POINT ( 'NONE',  ( -0.7152230971128602510, -0.08942795157528024563, -0.3641732283464568787 ) ) ;
#75108=CARTESIAN_POINT ( 'NONE',  ( -1.594488188976377119, 0.1660481256975883668, -0.3530559997133364547 ) ) ;
#75109=CARTESIAN_POINT ( 'NONE',  ( 0.05249343832021075018, -0.6046776061558807314, 0.2411417322834647770 ) ) ;
#75110=CARTESIAN_POINT ( 'NONE',  ( -0.2099737532808391705, 0.1283753931104748280, 0.1820866141732283561 ) ) ;
#75111=CARTESIAN_POINT ( 'NONE',  ( -1.345144356955379816, -0.08942795157528024563, -0.3641732283464568787 ) ) ;
#75112=CARTESIAN_POINT ( 'NONE',  ( -1.535433070866141225, 0.2952755905511811885, 0.000000000000000000 ) ) ;
#75113=CARTESIAN_POINT ( 'NONE',  ( 1.528871391076116026, -0.5511811023622048555, -0.09757992244046775898 ) ) ;
#75115=CARTESIAN_POINT ( 'NONE',  ( 1.062992125984252745, 0.2952755905511811885, 0.000000000000000000 ) ) ;
#75117=CARTESIAN_POINT ( 'NONE',  ( 0.5183727034120741983, -0.5511811023622046335, 0.09757992244046803654 ) ) ;
#75118=CARTESIAN_POINT ( 'NONE',  ( 0.7414698162729663755, 0.2952755905511811885, 0.1292274648535926551 ) ) ;
#75119=CARTESIAN_POINT ( 'NONE',  ( 1.115485564304462551, -0.004921259842519576551, 0.3153832671262227771 ) ) ;
#75121=CARTESIAN_POINT ( 'NONE',  ( -1.299212598425196097, 0.2952755905511811885, 0.000000000000000000 ) ) ;
#75122=CARTESIAN_POINT ( 'NONE',  ( -0.9383202099737524282, -0.3162353388693409650, -0.4822834645669289433 ) ) ;
#75123=CARTESIAN_POINT ( 'NONE',  ( 0.06561679790026316017, 0.05413385826771626580, -0.4176697321401330321 ) ) ;
#75126=CARTESIAN_POINT ( 'NONE',  ( 0.3674540682414705883, 0.2306618581243847221, -0.2411417322834647770 ) ) ;
#75127=CARTESIAN_POINT ( 'NONE',  ( -1.673228346456691717, 0.1660481256975883668, -0.3530559997133364547 ) ) ;
#75128=CARTESIAN_POINT ( 'NONE',  ( 0.1049868766404206816, 0.2306618581243848609, 0.2411417322834645549 ) ) ;
#75129=CARTESIAN_POINT ( 'NONE',  ( 0.7086614173228352742, -0.1870078740157480879, -0.4822834645669291653 ) ) ;
#75133=CARTESIAN_POINT ( 'NONE',  ( -1.586052503253849055, 0.4724409448818907564, -0.1653254495020551051 ) ) ;
#75135=CARTESIAN_POINT ( 'NONE',  ( -0.6233595800524928121, -0.08942795157527998196, 0.3641732283464567121 ) ) ;
#75136=CARTESIAN_POINT ( 'NONE',  ( -0.8661417322834640276, -0.1870078740157480879, -0.4822834645669291653 ) ) ;
#75137=CARTESIAN_POINT ( 'NONE',  ( 0.6102362204724416372, -0.5400638737290844871, 0.3530559997133364547 ) ) ;
#75139=CARTESIAN_POINT ( 'NONE',  ( 1.030183727034121421, -0.05778040916215522460, 0.4822834645669289988 ) ) ;
#75140=CARTESIAN_POINT ( 'NONE',  ( 1.528871391076116026, -0.6692913385826773087, -0.1292274648535924053 ) ) ;
#75141=CARTESIAN_POINT ( 'NONE',  ( 1.272965879265092637, 0.05413385826771666132, 0.4176697321401328100 ) ) ;
#75145=CARTESIAN_POINT ( 'NONE',  ( 1.095800524934383846, -0.3162353388693405765, 0.4822834645669290543 ) ) ;
#75146=CARTESIAN_POINT ( 'NONE',  ( 0.5971128608923890191, -0.6692913385826771977, 0.1292274648535927661 ) ) ;
#75147=CARTESIAN_POINT ( 'NONE',  ( 1.338582677165355062, -0.1870078740157480601, -0.3641732283464567677 ) ) ;
#75148=CARTESIAN_POINT ( 'NONE',  ( 1.686351706036745890, 0.2952755905511811885, 0.1292274648535926551 ) ) ;
#75149=CARTESIAN_POINT ( 'NONE',  ( 1.568241469816273437, -0.3162353388693405765, 0.4822834645669290543 ) ) ;
#75151=CARTESIAN_POINT ( 'NONE',  ( -1.595398199321656607, 1.288687073698533414, 0.1559797534342480252 ) ) ;
#75152=CARTESIAN_POINT ( 'NONE',  ( 0.8136482939632553313, -0.6046776061558809534, -0.2411417322834644161 ) ) ;
#75153=FACE_OUTER_BOUND ( 'NONE', #22973, .T. ) ;
#75154=CARTESIAN_POINT ( 'NONE',  ( -0.4133858267716528645, 0.1660481256975883668, -0.3530559997133364547 ) ) ;
#75155=CARTESIAN_POINT ( 'NONE',  ( -0.7020997375328076329, -0.3162353388693409650, -0.4822834645669289433 ) ) ;
#75156=CARTESIAN_POINT ( 'NONE',  ( 1.594488188976378673, 0.1660481256975885056, 0.3530559997133364547 ) ) ;
#75158=CARTESIAN_POINT ( 'NONE',  ( 5.463695987328526437E-16, -0.1870078740157479769, 0.4822834645669291653 ) ) ;
#75160=CARTESIAN_POINT ( 'NONE',  ( -1.646981627296586703, -0.08942795157527998196, 0.3641732283464567121 ) ) ;
#75163=VERTEX_POINT ( 'NONE', #42271 ) ;
#75165=CARTESIAN_POINT ( 'NONE',  ( 1.496062992125984703, -0.1870078740157480601, -0.3641732283464567677 ) ) ;
#75172=CARTESIAN_POINT ( 'NONE',  ( -0.7939632545931750718, -0.08942795157528024563, -0.3641732283464568787 ) ) ;
#75173=CARTESIAN_POINT ( 'NONE',  ( -1.154855643044618851, -0.5023911411419708095, -0.1820866141732282451 ) ) ;
#75174=CARTESIAN_POINT ( 'NONE',  ( -1.535433070866141225, -0.6692913385826771977, 8.415575281601705876E-17 ) ) ;
#75175=CARTESIAN_POINT ( 'NONE',  ( 0.5905511811023629321, -0.6692913385826771977, 8.415575281601705876E-17 ) ) ;
#75176=CARTESIAN_POINT ( 'NONE',  ( -1.233595800524933894, -0.6046776061558809534, -0.2411417322834644161 ) ) ;
#75178=ORIENTED_EDGE ( 'NONE', *, *, #37233, .T. ) ;
#75179=CARTESIAN_POINT ( 'NONE',  ( 1.496062992125984703, -0.1870078740157480879, -0.4822834645669291653 ) ) ;
#75184=CARTESIAN_POINT ( 'NONE',  ( -0.7874015748031489847, -0.1870078740157480879, -0.4822834645669291653 ) ) ;
#75185=CARTESIAN_POINT ( 'NONE',  ( 1.030183727034121421, -0.05778040916215522460, 0.4822834645669289988 ) ) ;
#75186=DIRECTION ( 'NONE',  ( 0.000000000000000000, 1.000000000000000000, 0.000000000000000000 ) ) ;
#75189=CARTESIAN_POINT ( 'NONE',  ( 1.476377952755906442, -0.5400638737290844871, 0.3530559997133364547 ) ) ;
#75190=CARTESIAN_POINT ( 'NONE',  ( -1.318897637795274802, -0.5400638737290845981, -0.3530559997133363437 ) ) ;
#75192=CARTESIAN_POINT ( 'NONE',  ( 0.09842519685039434474, -0.4536011799217368745, -0.2665933059059886201 ) ) ;
#75194=CARTESIAN_POINT ( 'NONE',  ( -0.2427821522309703550, -0.2845877964562159024, 0.3641732283464567677 ) ) ;
#75195=CARTESIAN_POINT ( 'NONE',  ( 0.6627296587926515548, 0.1771653543307087630, 0.09757992244046791164 ) ) ;
#75196=CARTESIAN_POINT ( 'NONE',  ( 0.4133858267716541968, -0.5400638737290845981, -0.3530559997133363437 ) ) ;
#75197=CARTESIAN_POINT ( 'NONE',  ( -0.5183727034120726440, 0.1771653543307087630, 0.09757992244046791164 ) ) ;
#75199=CARTESIAN_POINT ( 'NONE',  ( -1.548556430446193399, -0.6046776061558809534, -0.2411417322834644161 ) ) ;
#75200=CARTESIAN_POINT ( 'NONE',  ( -1.154855643044618851, 0.2306618581243848609, 0.2411417322834645549 ) ) ;
#75202=CARTESIAN_POINT ( 'NONE',  ( 0.1181102362204730916, -0.6692913385826771977, 8.415575281601705876E-17 ) ) ;
#75203=CARTESIAN_POINT ( 'NONE',  ( -0.6889763779527552368, 0.1660481256975885056, 0.3530559997133364547 ) ) ;
#75204=CARTESIAN_POINT ( 'NONE',  ( 1.187664041994751285, -0.08942795157527998196, 0.3641732283464567121 ) ) ;
#75205=CARTESIAN_POINT ( 'NONE',  ( 0.3018372703412079971, -0.3690944881889763329, 0.3153832671262228327 ) ) ;
#75206=CARTESIAN_POINT ( 'NONE',  ( -0.2099737532808391705, -0.6046776061558809534, -0.2411417322834644161 ) ) ;
#75207=CARTESIAN_POINT ( 'NONE',  ( -0.9448818897637790704, -0.1870078740157480879, -0.4822834645669291653 ) ) ;
#75208=LINE ( 'NONE', #43184, #76157 ) ;
#75210=CARTESIAN_POINT ( 'NONE',  ( 0.02624671916010564918, -0.6046776061558809534, -0.2411417322834644161 ) ) ;
#75213=CARTESIAN_POINT ( 'NONE',  ( 0.9973753280839902091, 0.2306618581243847221, -0.2411417322834647770 ) ) ;
#75214=CARTESIAN_POINT ( 'NONE',  ( -0.7874015748031489847, -0.1870078740157479769, 0.3641732283464567677 ) ) ;
#75215=CARTESIAN_POINT ( 'NONE',  ( -0.5577427821522301654, -0.05778040916215560624, -0.4822834645669293319 ) ) ;
#75216=CARTESIAN_POINT ( 'NONE',  ( 1.338582677165355062, -0.1870078740157479769, 0.4822834645669291653 ) ) ;
#75217=CARTESIAN_POINT ( 'NONE',  ( 0.9383202099737538715, -0.05778040916215560624, -0.4822834645669293319 ) ) ;
#75218=CARTESIAN_POINT ( 'NONE',  ( -1.502624671916009680, -0.3162353388693405765, 0.4822834645669290543 ) ) ;
#75219=CARTESIAN_POINT ( 'NONE',  ( -1.266404199475064773, -0.2845877964562159024, 0.3641732283464567677 ) ) ;
#75223=CARTESIAN_POINT ( 'NONE',  ( 1.653543307086614789, -0.1870078740157479769, 0.3641732283464567677 ) ) ;
#75224=EDGE_CURVE ( 'NONE', #33617, #41461, #54210, .T. ) ;
#75225=CARTESIAN_POINT ( 'NONE',  ( 0.8989501312335963501, -0.5511811023622048555, -0.09757992244046775898 ) ) ;
#75226=CARTESIAN_POINT ( 'NONE',  ( 0.4265091863517067039, -0.6692913385826773087, -0.1292274648535924053 ) ) ;
#75227=CARTESIAN_POINT ( 'NONE',  ( 1.535433070866142335, -0.6692913385826771977, 8.415575281601705876E-17 ) ) ;
#75229=CARTESIAN_POINT ( 'NONE',  ( 0.7808398950131241190, -0.08942795157528024563, -0.3641732283464568787 ) ) ;
#75231=CARTESIAN_POINT ( 'NONE',  ( -0.2624671916010490880, -0.6046776061558807314, 0.2411417322834647770 ) ) ;
#75232=CARTESIAN_POINT ( 'NONE',  ( -0.6692913385826764205, 0.2952755905511811885, 0.000000000000000000 ) ) ;
#75233=CARTESIAN_POINT ( 'NONE',  ( 1.108923884514436686, -0.3162353388693409650, -0.4822834645669289433 ) ) ;
#75236=CARTESIAN_POINT ( 'NONE',  ( -0.2296587926509179312, -0.2845877964562161244, -0.3641732283464567121 ) ) ;
#75239=ORIENTED_EDGE ( 'NONE', *, *, #14066, .T. ) ;
#75240=CARTESIAN_POINT ( 'NONE',  ( -1.043307086614172707, 0.1660481256975883668, -0.3530559997133364547 ) ) ;
#75241=CARTESIAN_POINT ( 'NONE',  ( -0.04593175853018302557, 0.2952755905511811885, 0.1292274648535926551 ) ) ;
#75242=CARTESIAN_POINT ( 'NONE',  ( -0.2755905511811015396, -0.6692913385826771977, 8.415575281601705876E-17 ) ) ;
#75243=CARTESIAN_POINT ( 'NONE',  ( 0.3412073490813655186, -0.6046776061558809534, -0.2411417322834644161 ) ) ;
#75244=CARTESIAN_POINT ( 'NONE',  ( -0.6430446194225712953, 0.05413385826771626580, -0.4176697321401330321 ) ) ;
#75245=CARTESIAN_POINT ( 'NONE',  ( -1.463254593175852492, 0.2952755905511811885, 0.1292274648535926551 ) ) ;
#75246=CARTESIAN_POINT ( 'NONE',  ( -0.8727034120734901146, -0.05778040916215560624, -0.4822834645669293319 ) ) ;
#75247=CARTESIAN_POINT ( 'NONE',  ( 0.9645669291338588858, 0.1660481256975885056, 0.3530559997133364547 ) ) ;
#75248=CARTESIAN_POINT ( 'NONE',  ( 0.6758530183727039509, 0.2952755905511810774, -0.1292274648535930714 ) ) ;
#75251=CARTESIAN_POINT ( 'NONE',  ( -0.4199475065616791736, -0.5023911411419708095, 0.1820866141732285504 ) ) ;
#75255=CARTESIAN_POINT ( 'NONE',  ( -1.305774278215222184, -0.5511811023622048555, -0.09757992244046775898 ) ) ;
#75256=CARTESIAN_POINT ( 'NONE',  ( -0.9120734908136475250, -0.6692913385826773087, -0.1292274648535924053 ) ) ;
#75257=CARTESIAN_POINT ( 'NONE',  ( -0.2559055118110227234, -0.5400638737290844871, 0.3530559997133364547 ) ) ;
#75259=CARTESIAN_POINT ( 'NONE',  ( -0.7939632545931754048, -0.3162353388693405765, 0.4822834645669290543 ) ) ;
#75260=CARTESIAN_POINT ( 'NONE',  ( -0.8792650918635160906, 0.05413385826771626580, -0.4176697321401330321 ) ) ;
#75263=B_SPLINE_CURVE_WITH_KNOTS ( 'NONE', 3,
 ( #19298, #50858, #18886, #26450 ),
 .UNSPECIFIED., .F., .F.,
 ( 4, 4 ),
 ( 0.06769753431378609798, 0.06787032835250683682 ),
 .UNSPECIFIED. ) ;
#75264=CARTESIAN_POINT ( 'NONE',  ( 0.9973753280839902091, -0.5023911411419708095, 0.1820866141732285504 ) ) ;
#75267=CARTESIAN_POINT ( 'NONE',  ( 0.03280839895013198948, 0.1771653543307087630, 0.09757992244046791164 ) ) ;
#75268=CARTESIAN_POINT ( 'NONE',  ( -0.5708661417322825615, -0.5400638737290844871, 0.3530559997133364547 ) ) ;
#75269=CARTESIAN_POINT ( 'NONE',  ( 1.614173228346457156, 1.496062992125984037, -0.5309055118110239668 ) ) ;
#75270=CARTESIAN_POINT ( 'NONE',  ( 0.09186351706036827158, 0.05413385826771666132, 0.4176697321401328100 ) ) ;
#75274=ORIENTED_EDGE ( 'NONE', *, *, #76979, .T. ) ;
#75276=FACE_OUTER_BOUND ( 'NONE', #59724, .T. ) ;
#75277=CARTESIAN_POINT ( 'NONE',  ( -0.6299212598425188991, -0.1870078740157479769, 0.3641732283464567677 ) ) ;
#75278=CARTESIAN_POINT ( 'NONE',  ( -0.9055118110236215490, 0.2952755905511811885, 0.000000000000000000 ) ) ;
#75282=CARTESIAN_POINT ( 'NONE',  ( 1.358267716535433323, 0.1660481256975885056, 0.3530559997133364547 ) ) ;
#75283=CARTESIAN_POINT ( 'NONE',  ( 0.2690288713910767848, -0.6692913385826773087, -0.1292274648535924053 ) ) ;
#75284=CARTESIAN_POINT ( 'NONE',  ( 0.4068241469816281097, 0.05413385826771666132, 0.4176697321401328100 ) ) ;
#75285=CARTESIAN_POINT ( 'NONE',  ( -0.7939632545931750718, -0.08942795157528024563, -0.3641732283464568787 ) ) ;
#75286=CARTESIAN_POINT ( 'NONE',  ( -0.2230971128608915943, -0.4281496062992127816, -0.4176697321401328100 ) ) ;
#75288=CARTESIAN_POINT ( 'NONE',  ( -0.9711286089238838626, -0.6046776061558807314, 0.2411417322834647770 ) ) ;
#75290=CARTESIAN_POINT ( 'NONE',  ( 1.345144356955381593, -0.2845877964562161244, -0.3641732283464567121 ) ) ;
#75291=CARTESIAN_POINT ( 'NONE',  ( -0.4527559055118102749, 0.07958543189024085140, 0.2665933059059887866 ) ) ;
#75292=CARTESIAN_POINT ( 'NONE',  ( 1.253280839895013710, -0.08942795157528024563, -0.3641732283464568787 ) ) ;
#75293=CARTESIAN_POINT ( 'NONE',  ( -1.515748031496062076, 0.1660481256975883668, -0.3530559997133364547 ) ) ;
#75294=CARTESIAN_POINT ( 'NONE',  ( -0.9711286089238838626, 0.1283753931104746893, -0.1820866141732285504 ) ) ;
#75296=CARTESIAN_POINT ( 'NONE',  ( 0.6036745406824154392, 0.1283753931104746893, -0.1820866141732285504 ) ) ;
#75297=CARTESIAN_POINT ( 'NONE',  ( -0.4790026246719152336, -0.05778040916215560624, -0.4822834645669293319 ) ) ;
#75298=CARTESIAN_POINT ( 'NONE',  ( 0.2478063387913472249, 0.02791078216816225699, 0.4328096321851905293 ) ) ;
#75299=CARTESIAN_POINT ( 'NONE',  ( 0.1181102362204730916, 0.1771653543307087630, 0.000000000000000000 ) ) ;
#75300=CARTESIAN_POINT ( 'NONE',  ( -1.640419947506561060, -0.3690944881889765550, -0.3153832671262227771 ) ) ;
#75301=CARTESIAN_POINT ( 'NONE',  ( 0.7677165354330716118, 0.1660481256975883668, -0.3530559997133364547 ) ) ;
#75303=CARTESIAN_POINT ( 'NONE',  ( 1.272965879265092637, -0.004921259842519576551, 0.3153832671262227771 ) ) ;
#75304=CARTESIAN_POINT ( 'NONE',  ( -0.9514435695538050464, -0.3162353388693405765, 0.4822834645669290543 ) ) ;
#75305=CARTESIAN_POINT ( 'NONE',  ( -0.2887139107611542133, -0.5023911411419708095, -0.1820866141732282451 ) ) ;
#75306=CARTESIAN_POINT ( 'NONE',  ( -1.603475055217291612, 0.9922665159524542977, 0.04573490813648251746 ) ) ;
#75307=CARTESIAN_POINT ( 'NONE',  ( 0.3412073490813655186, 0.1283753931104748280, 0.1820866141732283561 ) ) ;
#75308=CARTESIAN_POINT ( 'NONE',  ( -0.7086614173228339419, -0.1870078740157479769, 0.4822834645669291653 ) ) ;
#75311=CARTESIAN_POINT ( 'NONE',  ( 0.4724409448818904789, -0.1870078740157479769, 0.3641732283464567677 ) ) ;
#75312=CARTESIAN_POINT ( 'NONE',  ( -0.3608923884514428360, 0.2952755905511811885, 0.1292274648535926551 ) ) ;
#75313=CARTESIAN_POINT ( 'NONE',  ( -0.8989501312335946848, -0.6692913385826771977, 0.1292274648535927661 ) ) ;
#75314=CARTESIAN_POINT ( 'NONE',  ( -0.8661417322834640276, -0.1870078740157479769, 0.3641732283464567677 ) ) ;
#75316=CARTESIAN_POINT ( 'NONE',  ( -0.07217847769028787330, -0.05778040916215522460, 0.4822834645669289988 ) ) ;
#75317=CARTESIAN_POINT ( 'NONE',  ( -1.167979002624671470, -0.3690944881889765550, -0.3153832671262227771 ) ) ;
#75318=CARTESIAN_POINT ( 'NONE',  ( -1.391076115485563314, -0.6046776061558809534, -0.2411417322834644161 ) ) ;
#75319=CARTESIAN_POINT ( 'NONE',  ( 0.2165354330708668951, 0.1012011053420775880, -0.2882089793578257453 ) ) ;
#75322=CARTESIAN_POINT ( 'NONE',  ( -1.627296587926508442, -0.5023911411419708095, -0.1820866141732282451 ) ) ;
#75323=CARTESIAN_POINT ( 'NONE',  ( -1.167979002624671470, -0.4281496062992127816, -0.4176697321401328100 ) ) ;
#75324=CARTESIAN_POINT ( 'NONE',  ( -0.8727034120734901146, -0.05778040916215560624, -0.4822834645669293319 ) ) ;
#75325=CARTESIAN_POINT ( 'NONE',  ( 1.581364829396326277, -0.05778040916215522460, 0.4822834645669289988 ) ) ;
#75328=CARTESIAN_POINT ( 'NONE',  ( 1.010498687664042716, -0.4281496062992124485, 0.4176697321401328655 ) ) ;
#75329=CARTESIAN_POINT ( 'NONE',  ( 0.6167979002624679463, 0.05413385826771626580, -0.4176697321401330321 ) ) ;
#75332=CARTESIAN_POINT ( 'NONE',  ( 1.364829396325459854, -0.5023911411419708095, -0.1820866141732282451 ) ) ;
#75334=ORIENTED_EDGE ( 'NONE', *, *, #66845, .T. ) ;
#75335=CARTESIAN_POINT ( 'NONE',  ( -0.8005249343832011588, -0.004921259842519870586, -0.3153832671262229437 ) ) ;
#75337=ORIENTED_EDGE ( 'NONE', *, *, #79988, .F. ) ;
#75338=CARTESIAN_POINT ( 'NONE',  ( 0.5774278215223103139, -0.6046776061558809534, -0.2411417322834644161 ) ) ;
#75339=CARTESIAN_POINT ( 'NONE',  ( -0.2165354330708654795, -0.5400638737290845981, -0.3530559997133363437 ) ) ;
#75340=CARTESIAN_POINT ( 'NONE',  ( -1.292650918635170010, 0.2952755905511810774, -0.1292274648535930714 ) ) ;
#75341=CARTESIAN_POINT ( 'NONE',  ( 1.017060367454068803, -0.3162353388693405765, 0.4822834645669290543 ) ) ;
#75342=CARTESIAN_POINT ( 'NONE',  ( 1.528871391076116026, 0.2952755905511811885, 0.1292274648535926551 ) ) ;
#75344=CARTESIAN_POINT ( 'NONE',  ( -0.1443569553805765515, -0.4281496062992127816, -0.4176697321401328100 ) ) ;
#75345=CARTESIAN_POINT ( 'NONE',  ( -1.299212598425196097, 0.2952755905511811885, 0.000000000000000000 ) ) ;
#75346=CARTESIAN_POINT ( 'NONE',  ( -1.640419947506561060, 0.05413385826771666132, 0.4176697321401328100 ) ) ;
#75349=CARTESIAN_POINT ( 'NONE',  ( 0.6955380577427828781, -0.3690944881889763329, 0.3153832671262228327 ) ) ;
#75350=ORIENTED_EDGE ( 'NONE', *, *, #14488, .F. ) ;
#75352=CARTESIAN_POINT ( 'NONE',  ( -0.7545931758530176614, -0.6692913385826773087, -0.1292274648535924053 ) ) ;
#75353=ORIENTED_EDGE ( 'NONE', *, *, #56823, .T. ) ;
#75354=CARTESIAN_POINT ( 'NONE',  ( 0.1574803149606306130, -0.1870078740157479769, 0.3641732283464567677 ) ) ;
#75355=CARTESIAN_POINT ( 'NONE',  ( -1.640419947506561060, -0.4281496062992127816, -0.4176697321401328100 ) ) ;
#75356=CARTESIAN_POINT ( 'NONE',  ( 0.6758530183727039509, 0.2952755905511810774, -0.1292274648535930714 ) ) ;
#75357=CARTESIAN_POINT ( 'NONE',  ( 0.4921259842519691285, 0.1660481256975885056, 0.3530559997133364547 ) ) ;
#75358=CARTESIAN_POINT ( 'NONE',  ( -0.6889763779527552368, -0.5400638737290845981, -0.3530559997133363437 ) ) ;
#75360=CARTESIAN_POINT ( 'NONE',  ( -0.9186351706036736120, -0.6046776061558809534, -0.2411417322834644161 ) ) ;
#75362=CARTESIAN_POINT ( 'NONE',  ( 1.115485564304462551, -0.004921259842519576551, 0.3153832671262227771 ) ) ;
#75363=CARTESIAN_POINT ( 'NONE',  ( -0.8202099737532799750, 0.2952755905511810774, -0.1292274648535930714 ) ) ;
#75364=CARTESIAN_POINT ( 'NONE',  ( 0.7349081364829403995, 0.2306618581243848609, 0.2411417322834645549 ) ) ;
#75365=CARTESIAN_POINT ( 'NONE',  ( 1.122047244094488860, -0.5400638737290845981, -0.3530559997133363437 ) ) ;
#75366=VECTOR ( 'NONE', #42017, 39.37007874015748143 ) ;
#75368=CARTESIAN_POINT ( 'NONE',  ( -1.515748031496062076, 0.1660481256975883668, -0.3530559997133364547 ) ) ;
#75371=CARTESIAN_POINT ( 'NONE',  ( 0.3412073490813655186, 0.2306618581243848609, 0.2411417322834645549 ) ) ;
#75373=CARTESIAN_POINT ( 'NONE',  ( -1.489501312335957062, -0.08942795157527998196, 0.3641732283464567121 ) ) ;
#75374=CARTESIAN_POINT ( 'NONE',  ( 0.4330708661417329575, 0.1771653543307087630, 0.000000000000000000 ) ) ;
#75375=CARTESIAN_POINT ( 'NONE',  ( 0.9448818897637802916, -0.1870078740157479769, 0.4822834645669291653 ) ) ;
#75377=CARTESIAN_POINT ( 'NONE',  ( 0.6364829396325465405, -0.2845877964562161244, -0.3641732283464567121 ) ) ;
#75379=CARTESIAN_POINT ( 'NONE',  ( 0.4658792650918640033, -0.3162353388693405765, 0.4822834645669290543 ) ) ;
#75381=CARTESIAN_POINT ( 'NONE',  ( -0.9448818897637790704, -0.1870078740157479769, 0.4822834645669291653 ) ) ;
#75383=CARTESIAN_POINT ( 'NONE',  ( 1.095800524934383846, -0.2845877964562159024, 0.3641732283464567677 ) ) ;
#75385=CARTESIAN_POINT ( 'NONE',  ( -0.1443569553805768291, 0.05413385826771666132, 0.4176697321401328100 ) ) ;
#75388=CARTESIAN_POINT ( 'NONE',  ( -0.5183727034120726440, -0.6692913385826773087, -0.1292274648535924053 ) ) ;
#75389=CARTESIAN_POINT ( 'NONE',  ( 8.195543980992789655E-16, -0.1870078740157480601, -0.3641732283464567677 ) ) ;
#75391=CARTESIAN_POINT ( 'NONE',  ( -0.4527559055118102749, 0.1660481256975885056, 0.3530559997133364547 ) ) ;
#75392=CARTESIAN_POINT ( 'NONE',  ( -0.08530183727034056085, -0.2845877964562159024, 0.3641732283464567677 ) ) ;
#75393=CARTESIAN_POINT ( 'NONE',  ( 0.5839895013123367340, -0.5511811023622048555, -0.09757992244046775898 ) ) ;
#75396=CARTESIAN_POINT ( 'NONE',  ( 0.3280839895013130669, -0.4281496062992127816, -0.4176697321401328100 ) ) ;
#75398=CARTESIAN_POINT ( 'NONE',  ( 1.076115485564305141, 0.1283753931104746893, -0.1820866141732285504 ) ) ;
#75400=CARTESIAN_POINT ( 'NONE',  ( -0.4658792650918627265, -0.08942795157527998196, 0.3641732283464567121 ) ) ;
#75401=CARTESIAN_POINT ( 'NONE',  ( -0.7677165354330699465, 0.07958543189024085140, 0.2665933059059887866 ) ) ;
#75402=CARTESIAN_POINT ( 'NONE',  ( -0.4527559055118102749, -0.5400638737290845981, -0.3530559997133363437 ) ) ;
#75403=CARTESIAN_POINT ( 'NONE',  ( 1.154855643044620184, -0.5023911411419708095, 0.1820866141732285504 ) ) ;
#75404=CARTESIAN_POINT ( 'NONE',  ( -1.633858267716534529, -0.4536011799217368745, -0.2665933059059886201 ) ) ;
#75405=CARTESIAN_POINT ( 'NONE',  ( 1.594488188976378673, 0.07958543189024085140, 0.2665933059059887866 ) ) ;
#75406=CARTESIAN_POINT ( 'NONE',  ( 0.2493438320209980519, 0.05413385826771666132, 0.4176697321401328100 ) ) ;
#75407=EDGE_CURVE ( 'NONE', #35363, #74087, #75704, .T. ) ;
#75409=CARTESIAN_POINT ( 'NONE',  ( 0.9645669291338591078, -0.5400638737290845981, -0.3530559997133363437 ) ) ;
#75411=CARTESIAN_POINT ( 'NONE',  ( 0.1771653543307093182, 0.1660481256975885056, 0.3530559997133364547 ) ) ;
#75413=CARTESIAN_POINT ( 'NONE',  ( 0.7086614173228353852, -0.1870078740157479769, 0.4822834645669291653 ) ) ;
#75414=CARTESIAN_POINT ( 'NONE',  ( 0.5511811023622055217, -0.1870078740157479769, 0.4822834645669291653 ) ) ;
#75416=CARTESIAN_POINT ( 'NONE',  ( 0.7611548556430454138, 0.1283753931104746893, -0.1820866141732285504 ) ) ;
#75417=CARTESIAN_POINT ( 'NONE',  ( 1.384514435695538559, 0.2952755905511810774, -0.1292274648535930714 ) ) ;
#75419=CARTESIAN_POINT ( 'NONE',  ( 0.1246719160104994284, -0.5511811023622046335, 0.09757992244046803654 ) ) ;
#75420=CARTESIAN_POINT ( 'NONE',  ( -0.4461942257217840213, -0.6046776061558809534, -0.2411417322834644161 ) ) ;
#75421=CARTESIAN_POINT ( 'NONE',  ( 0.4396325459317590445, -0.6692913385826771977, 0.1292274648535927661 ) ) ;
#75422=CARTESIAN_POINT ( 'NONE',  ( -0.6955380577427815458, 0.05413385826771666132, 0.4176697321401328100 ) ) ;
#75423=CARTESIAN_POINT ( 'NONE',  ( -0.3871391076115479057, -0.2845877964562161244, -0.3641732283464567121 ) ) ;
#75425=CARTESIAN_POINT ( 'NONE',  ( 0.9448818897637802916, -0.1870078740157479769, 0.4822834645669291653 ) ) ;
#75426=CARTESIAN_POINT ( 'NONE',  ( 1.095800524934383846, -0.08942795157528024563, -0.3641732283464568787 ) ) ;
#75427=CARTESIAN_POINT ( 'NONE',  ( 0.2230971128608932319, -0.4281496062992124485, 0.4176697321401328655 ) ) ;
#75430=CARTESIAN_POINT ( 'NONE',  ( -1.646051170424378096, -0.1870078740157480046, 1.254653134982923898E-17 ) ) ;
#75432=CARTESIAN_POINT ( 'NONE',  ( -0.1474713956048439301, -2.191421614605370878E-15, 0.4445507791589071167 ) ) ;
#75434=CARTESIAN_POINT ( 'NONE',  ( -1.115485564304461219, 0.05413385826771626580, -0.4176697321401330321 ) ) ;
#75435=CARTESIAN_POINT ( 'NONE',  ( -0.7742782152230965886, 0.05413385826771666132, 0.4176697321401328100 ) ) ;
#75436=B_SPLINE_CURVE_WITH_KNOTS ( 'NONE', 3,
 ( #23403, #48657, #61289, #73941 ),
 .UNSPECIFIED., .F., .F.,
 ( 4, 4 ),
 ( 3.210432057660995322E-07, 0.001287787053612127848 ),
 .UNSPECIFIED. ) ;
#75440=CARTESIAN_POINT ( 'NONE',  ( 0.4199475065616805614, 0.1283753931104748280, 0.1820866141732283561 ) ) ;
#75442=CARTESIAN_POINT ( 'NONE',  ( 0.8858267716535438430, -0.5400638737290845981, -0.3530559997133363437 ) ) ;
#75445=CARTESIAN_POINT ( 'NONE',  ( -1.627296587926508442, -0.5023911411419708095, -0.1820866141732282451 ) ) ;
#75447=CARTESIAN_POINT ( 'NONE',  ( 1.364829396325460076, 0.2306618581243848609, 0.2411417322834645549 ) ) ;
#75448=CARTESIAN_POINT ( 'NONE',  ( 1.207349081364829990, -0.5023911411419708095, -0.1820866141732282451 ) ) ;
#75449=CARTESIAN_POINT ( 'NONE',  ( -0.07217847769028787330, -0.05778040916215522460, 0.4822834645669289988 ) ) ;
#75451=CARTESIAN_POINT ( 'NONE',  ( -0.2165354330708654795, 0.1660481256975885056, 0.3530559997133364547 ) ) ;
#75452=CARTESIAN_POINT ( 'NONE',  ( -0.7152230971128602510, -0.08942795157528024563, -0.3641732283464568787 ) ) ;
#75453=CARTESIAN_POINT ( 'NONE',  ( 0.5052493438320215802, 0.2952755905511811885, 0.1292274648535926551 ) ) ;
#75454=CARTESIAN_POINT ( 'NONE',  ( -0.5380577427821514602, -0.4281496062992127816, -0.4176697321401328100 ) ) ;
#75457=ORIENTED_EDGE ( 'NONE', *, *, #69293, .T. ) ;
#75459=CARTESIAN_POINT ( 'NONE',  ( 0.5971128608923891301, 0.2952755905511810774, -0.1292274648535930714 ) ) ;
#75460=CARTESIAN_POINT ( 'NONE',  ( -0.4724409448818890911, -0.1870078740157479769, 0.4822834645669291653 ) ) ;
#75461=CARTESIAN_POINT ( 'NONE',  ( -1.620734908136482577, 0.2952755905511811885, 0.1292274648535926551 ) ) ;
#75462=CARTESIAN_POINT ( 'NONE',  ( 0.7020997375328090762, -0.05778040916215560624, -0.4822834645669293319 ) ) ;
#75463=CARTESIAN_POINT ( 'NONE',  ( 0.3215223097112867578, -0.3162353388693409650, -0.4822834645669289433 ) ) ;
#75465=CARTESIAN_POINT ( 'NONE',  ( -0.6299212598425188991, -0.1870078740157479769, 0.4822834645669291653 ) ) ;
#75466=CARTESIAN_POINT ( 'NONE',  ( 0.3871391076115493490, -0.3162353388693405765, 0.4822834645669290543 ) ) ;
#75467=CARTESIAN_POINT ( 'NONE',  ( -0.4330708661417315697, -0.6692913385826771977, 8.415575281601705876E-17 ) ) ;
#75468=CARTESIAN_POINT ( 'NONE',  ( 0.3674540682414705883, -0.5023911411419708095, 0.1820866141732285504 ) ) ;
#75469=CARTESIAN_POINT ( 'NONE',  ( -1.706036745406823485, 0.2306618581243848609, 0.2411417322834645549 ) ) ;
#75471=CARTESIAN_POINT ( 'NONE',  ( -0.2427821522309703550, -0.05778040916215560624, -0.4822834645669293319 ) ) ;
#75472=CYLINDRICAL_SURFACE ( 'NONE', #46643, 1.181102362204724310 ) ;
#75473=CARTESIAN_POINT ( 'NONE',  ( 1.535433070866142335, -0.6692913385826771977, 8.415575281601705876E-17 ) ) ;
#75477=CARTESIAN_POINT ( 'NONE',  ( 0.5643044619422579178, 0.05413385826771666132, 0.4176697321401328100 ) ) ;
#75478=CARTESIAN_POINT ( 'NONE',  ( 0.1443569553805781891, -0.3690944881889763329, 0.3153832671262228327 ) ) ;
#75480=CARTESIAN_POINT ( 'NONE',  ( -1.036041590146031366, -2.613618158232546091E-15, -0.3464511005275220379 ) ) ;
#75486=CARTESIAN_POINT ( 'NONE',  ( 0.4593175853018379162, -0.4281496062992124485, 0.4176697321401328655 ) ) ;
#75487=CARTESIAN_POINT ( 'NONE',  ( -1.410761154855641575, -0.3162353388693409650, -0.4822834645669289433 ) ) ;
#75488=CARTESIAN_POINT ( 'NONE',  ( -1.194225721784776262, 0.05413385826771626580, -0.4176697321401330321 ) ) ;
#75489=CARTESIAN_POINT ( 'NONE',  ( 0.7939632545931766261, -0.05778040916215522460, 0.4822834645669289988 ) ) ;
#75491=CARTESIAN_POINT ( 'NONE',  ( 0.7480314960629927956, -0.6692913385826771977, 8.415575281601705876E-17 ) ) ;
#75492=CARTESIAN_POINT ( 'NONE',  ( 1.292650918635171564, -0.5511811023622048555, -0.09757992244046775898 ) ) ;
#75493=CARTESIAN_POINT ( 'NONE',  ( 1.043307086614173818, 0.07958543189024085140, 0.2665933059059887866 ) ) ;
#75494=CARTESIAN_POINT ( 'NONE',  ( -0.7545931758530176614, -0.6692913385826773087, -0.1292274648535924053 ) ) ;
#75496=CARTESIAN_POINT ( 'NONE',  ( -1.607611548556429737, 0.1771653543307087075, -0.09757992244046823083 ) ) ;
#75498=CARTESIAN_POINT ( 'NONE',  ( -0.4396325459317577122, -0.6692913385826773087, -0.1292274648535924053 ) ) ;
#75499=CARTESIAN_POINT ( 'NONE',  ( 1.227034120734908917, 0.2952755905511810774, -0.1292274648535930714 ) ) ;
#75501=CARTESIAN_POINT ( 'NONE',  ( -1.417322834645668772, -0.1870078740157479769, 0.3641732283464567677 ) ) ;
#75502=CARTESIAN_POINT ( 'NONE',  ( 0.4658792650918641698, -0.05778040916215560624, -0.4822834645669293319 ) ) ;
#75503=CARTESIAN_POINT ( 'NONE',  ( 0.8464566929133865436, 0.07958543189024071263, -0.2665933059059888421 ) ) ;
#75505=CARTESIAN_POINT ( 'NONE',  ( -1.213910761154854745, 0.1771653543307087075, -0.09757992244046823083 ) ) ;
#75506=CARTESIAN_POINT ( 'NONE',  ( 0.9251968503937015864, 0.1660481256975883668, -0.3530559997133364547 ) ) ;
#75507=CARTESIAN_POINT ( 'NONE',  ( -0.5183727034120726440, 0.2952755905511811885, 0.1292274648535926551 ) ) ;
#75508=CARTESIAN_POINT ( 'NONE',  ( -0.4461942257217840213, 0.1283753931104748280, 0.1820866141732283561 ) ) ;
#75509=CARTESIAN_POINT ( 'NONE',  ( -0.4527559055118102749, 0.1660481256975885056, 0.3530559997133364547 ) ) ;
#75510=CARTESIAN_POINT ( 'NONE',  ( 1.496062992125985147, -0.1870078740157479769, 0.4822834645669291653 ) ) ;
#75511=CARTESIAN_POINT ( 'NONE',  ( -0.6824146981627291497, -0.6046776061558809534, -0.2411417322834644161 ) ) ;
#75512=CARTESIAN_POINT ( 'NONE',  ( 1.581364829396326277, -0.3162353388693409650, -0.4822834645669289433 ) ) ;
#75514=CARTESIAN_POINT ( 'NONE',  ( -0.8530183727034112984, -0.004921259842519576551, 0.3153832671262227771 ) ) ;
#75516=CARTESIAN_POINT ( 'NONE',  ( 1.253280839895013710, -0.3162353388693405765, 0.4822834645669290543 ) ) ;
#75518=CARTESIAN_POINT ( 'NONE',  ( -1.318897637795274802, -0.5400638737290845981, -0.3530559997133363437 ) ) ;
#75519=CARTESIAN_POINT ( 'NONE',  ( -1.515748031496062076, -0.4536011799217367080, 0.2665933059059888421 ) ) ;
#75520=CARTESIAN_POINT ( 'NONE',  ( -0.4658792650918627265, -0.08942795157527998196, 0.3641732283464567121 ) ) ;
#75522=CARTESIAN_POINT ( 'NONE',  ( -0.4921259842519677963, 0.1660481256975883668, -0.3530559997133364547 ) ) ;
#75523=CARTESIAN_POINT ( 'NONE',  ( -0.006561679790025524116, -0.08942795157528024563, -0.3641732283464568787 ) ) ;
#75524=CARTESIAN_POINT ( 'NONE',  ( -1.043307086614172707, 0.07958543189024071263, -0.2665933059059888421 ) ) ;
#75525=CARTESIAN_POINT ( 'NONE',  ( 1.397637795275591177, -0.4536011799217367080, 0.2665933059059888421 ) ) ;
#75526=CARTESIAN_POINT ( 'NONE',  ( 0.9251968503937015864, 0.1660481256975883668, -0.3530559997133364547 ) ) ;
#75527=DIRECTION ( 'NONE',  ( 1.000000000000000000, -0.000000000000000000, -0.000000000000000000 ) ) ;
#75528=CARTESIAN_POINT ( 'NONE',  ( 0.5839895013123367340, 0.1771653543307087630, 0.09757992244046791164 ) ) ;
#75529=CARTESIAN_POINT ( 'NONE',  ( 0.2755905511811031494, 0.2952755905511811885, 0.000000000000000000 ) ) ;
#75530=CARTESIAN_POINT ( 'NONE',  ( 0.8202099737532813073, 0.1771653543307087630, 0.09757992244046791164 ) ) ;
#75532=CARTESIAN_POINT ( 'NONE',  ( -1.030183727034119867, -0.3162353388693405765, 0.4822834645669290543 ) ) ;
#75533=CARTESIAN_POINT ( 'NONE',  ( -0.9776902887139098386, 0.2952755905511810774, -0.1292274648535930714 ) ) ;
#75534=CARTESIAN_POINT ( 'NONE',  ( -0.2887139107611542133, 0.2306618581243848609, 0.2411417322834645549 ) ) ;
#75537=CARTESIAN_POINT ( 'NONE',  ( 0.5380577427821529035, 0.05413385826771626580, -0.4176697321401330321 ) ) ;
#75538=CARTESIAN_POINT ( 'NONE',  ( 1.509186351706037543, -0.3690944881889765550, -0.3153832671262227771 ) ) ;
#75539=CARTESIAN_POINT ( 'NONE',  ( -0.1312335958005241554, -0.6046776061558809534, -0.2411417322834644161 ) ) ;
#75540=CARTESIAN_POINT ( 'NONE',  ( 0.9776902887139113929, 0.2952755905511811885, 0.1292274648535926551 ) ) ;
#75546=CARTESIAN_POINT ( 'NONE',  ( -0.7217847769028863381, -0.004921259842519870586, -0.3153832671262229437 ) ) ;
#75547=CARTESIAN_POINT ( 'NONE',  ( -0.7020997375328076329, -0.3162353388693409650, -0.4822834645669289433 ) ) ;
#75548=CARTESIAN_POINT ( 'NONE',  ( 0.3215223097112867578, -0.05778040916215522460, 0.4822834645669289988 ) ) ;
#75551=CARTESIAN_POINT ( 'NONE',  ( 1.003937007874016407, -0.5400638737290844871, 0.3530559997133364547 ) ) ;
#75552=CARTESIAN_POINT ( 'NONE',  ( 1.574803149606299746, -0.1870078740157479769, 0.4822834645669291653 ) ) ;
#75553=CARTESIAN_POINT ( 'NONE',  ( 0.8398950131233602345, 0.2306618581243847221, -0.2411417322834647770 ) ) ;
#75556=CARTESIAN_POINT ( 'NONE',  ( 1.489501312335958172, -0.3162353388693405765, 0.4822834645669290543 ) ) ;
#75557=CARTESIAN_POINT ( 'NONE',  ( 0.7480314960629927956, -0.6692913385826771977, 8.415575281601705876E-17 ) ) ;
#75558=CARTESIAN_POINT ( 'NONE',  ( 0.7217847769028878924, -0.4281496062992127816, -0.4176697321401328100 ) ) ;
#75559=CARTESIAN_POINT ( 'NONE',  ( 1.371391076115485719, -0.5511811023622048555, -0.09757992244046775898 ) ) ;
#75560=CARTESIAN_POINT ( 'NONE',  ( -1.476377952755905110, 0.07958543189024085140, 0.2665933059059887866 ) ) ;
#75561=CARTESIAN_POINT ( 'NONE',  ( 1.561679790026247350, -0.4281496062992124485, 0.4176697321401328655 ) ) ;
#75564=CARTESIAN_POINT ( 'NONE',  ( 0.9973753280839902091, -0.6046776061558807314, 0.2411417322834647770 ) ) ;
#75565=CARTESIAN_POINT ( 'NONE',  ( 1.391076115485564868, 0.1283753931104746893, -0.1820866141732285504 ) ) ;
#75566=CARTESIAN_POINT ( 'NONE',  ( -0.4855643044619415427, -0.4281496062992124485, 0.4176697321401328655 ) ) ;
#75567=CARTESIAN_POINT ( 'NONE',  ( -0.7939632545931754048, -0.3162353388693405765, 0.4822834645669290543 ) ) ;
#75568=CARTESIAN_POINT ( 'NONE',  ( 1.587926509186352142, 0.05413385826771666132, 0.4176697321401328100 ) ) ;
#75570=B_SPLINE_CURVE_WITH_KNOTS ( 'NONE', 3,
 ( #73541, #60061, #28072, #16293 ),
 .UNSPECIFIED., .F., .F.,
 ( 4, 4 ),
 ( 0.07239528109754654606, 0.07258229963060973400 ),
 .UNSPECIFIED. ) ;
#75573=CARTESIAN_POINT ( 'NONE',  ( 1.673228346456693494, 0.1660481256975885056, 0.3530559997133364547 ) ) ;
#75577=CARTESIAN_POINT ( 'NONE',  ( -1.604771003085130099, 1.595806277125122241, -0.1466069496707745334 ) ) ;
#75578=CARTESIAN_POINT ( 'NONE',  ( 1.299212598425197429, 0.1771653543307087630, 0.000000000000000000 ) ) ;
#75586=CARTESIAN_POINT ( 'NONE',  ( -0.8333333333333323711, 0.1771653543307087630, 0.09757992244046791164 ) ) ;
#75587=CARTESIAN_POINT ( 'NONE',  ( -1.056430446194224881, 0.1771653543307087075, -0.09757992244046823083 ) ) ;
#75588=CARTESIAN_POINT ( 'NONE',  ( -1.207349081364828436, -0.6046776061558807314, 0.2411417322834647770 ) ) ;
#75589=CARTESIAN_POINT ( 'NONE',  ( -0.01312335958005186876, -0.4281496062992124485, 0.4176697321401328655 ) ) ;
#75590=CARTESIAN_POINT ( 'NONE',  ( -1.338582677165353729, -0.1870078740157479769, 0.4822834645669291653 ) ) ;
#75591=ORIENTED_EDGE ( 'NONE', *, *, #65602, .F. ) ;
#75592=CARTESIAN_POINT ( 'NONE',  ( 1.522309711286089939, -0.6046776061558809534, -0.2411417322834644161 ) ) ;
#75593=CARTESIAN_POINT ( 'NONE',  ( -1.611562765098779382, 0.2819705615091875339, 0.1148851572488242823 ) ) ;
#75595=DIRECTION ( 'NONE',  ( 1.000000000000000000, -0.000000000000000000, -0.000000000000000000 ) ) ;
#75596=CARTESIAN_POINT ( 'NONE',  ( -0.3477690288713902178, 0.1771653543307087075, -0.09757992244046823083 ) ) ;
#75597=CARTESIAN_POINT ( 'NONE',  ( -1.023622047244093558, -0.1870078740157479769, 0.4822834645669291653 ) ) ;
#75598=CARTESIAN_POINT ( 'NONE',  ( 0.9514435695538062676, -0.3162353388693409650, -0.4822834645669289433 ) ) ;
#75600=CARTESIAN_POINT ( 'NONE',  ( 0.7480314960629927956, 0.2952755905511811885, 0.000000000000000000 ) ) ;
#75602=CARTESIAN_POINT ( 'NONE',  ( 1.692913385826772421, 0.2952755905511811885, 0.000000000000000000 ) ) ;
#75603=CARTESIAN_POINT ( 'NONE',  ( -1.384514435695537005, 0.2952755905511811885, 0.1292274648535926551 ) ) ;
#75605=CARTESIAN_POINT ( 'NONE',  ( 0.1509186351706042484, -0.2845877964562159024, 0.3641732283464567677 ) ) ;
#75607=CARTESIAN_POINT ( 'NONE',  ( -0.2099737532808391705, 0.1283753931104748280, 0.1820866141732283561 ) ) ;
#75608=CARTESIAN_POINT ( 'NONE',  ( 0.3740157480314966754, 0.07958543189024071263, -0.2665933059059888421 ) ) ;
#75609=CARTESIAN_POINT ( 'NONE',  ( 0.7349081364829402885, -0.6046776061558809534, -0.2411417322834644161 ) ) ;
#75611=CARTESIAN_POINT ( 'NONE',  ( -0.7283464566929126471, -0.4536011799217367080, 0.2665933059059888421 ) ) ;
#75613=CARTESIAN_POINT ( 'NONE',  ( 1.076115485564305141, -0.6046776061558807314, 0.2411417322834647770 ) ) ;
#75614=CARTESIAN_POINT ( 'NONE',  ( -0.9317585301837263412, -0.4281496062992127816, -0.4176697321401328100 ) ) ;
#75616=CARTESIAN_POINT ( 'NONE',  ( -0.01312335958005186876, -0.4281496062992124485, 0.4176697321401328655 ) ) ;
#75617=CARTESIAN_POINT ( 'NONE',  ( -0.4002624671916004129, -0.3162353388693405765, 0.4822834645669290543 ) ) ;
#75618=CARTESIAN_POINT ( 'NONE',  ( 1.345144356955381593, -0.08942795157527998196, 0.3641732283464567121 ) ) ;
#75619=CARTESIAN_POINT ( 'NONE',  ( 0.1640419947506569498, -0.08942795157527998196, 0.3641732283464567121 ) ) ;
#75620=CARTESIAN_POINT ( 'NONE',  ( -0.07874015748031421014, -0.1870078740157480879, -0.4822834645669291653 ) ) ;
#75621=CARTESIAN_POINT ( 'NONE',  ( -0.9580052493438311334, 0.05413385826771626580, -0.4176697321401330321 ) ) ;
#75623=CARTESIAN_POINT ( 'NONE',  ( 1.587926509186352586, -0.3690944881889765550, -0.3153832671262227771 ) ) ;
#75625=CARTESIAN_POINT ( 'NONE',  ( -0.2690288713910754526, -0.6692913385826771977, 0.1292274648535927661 ) ) ;
#75626=ORIENTED_EDGE ( 'NONE', *, *, #34718, .F. ) ;
#75628=CARTESIAN_POINT ( 'NONE',  ( 1.095800524934383846, -0.3162353388693405765, 0.4822834645669290543 ) ) ;
#75629=CARTESIAN_POINT ( 'NONE',  ( -0.6561679790026240244, -0.5023911411419708095, 0.1820866141732285504 ) ) ;
#75630=CARTESIAN_POINT ( 'NONE',  ( -0.4068241469816267775, 0.05413385826771626580, -0.4176697321401330321 ) ) ;
#75631=CARTESIAN_POINT ( 'NONE',  ( 1.397637795275591177, 0.1660481256975883668, -0.3530559997133364547 ) ) ;
#75632=CARTESIAN_POINT ( 'NONE',  ( 1.003937007874016407, -0.5400638737290844871, 0.3530559997133364547 ) ) ;
#75634=CARTESIAN_POINT ( 'NONE',  ( -1.253280839895012377, -0.08942795157527998196, 0.3641732283464567121 ) ) ;
#75639=CARTESIAN_POINT ( 'NONE',  ( 1.240157480314961314, 0.07958543189024071263, -0.2665933059059888421 ) ) ;
#75640=CARTESIAN_POINT ( 'NONE',  ( 0.8267716535433077274, 0.1771653543307087630, 0.000000000000000000 ) ) ;
#75641=CARTESIAN_POINT ( 'NONE',  ( 0.6627296587926515548, 0.2952755905511811885, 0.1292274648535926551 ) ) ;
#75644=CARTESIAN_POINT ( 'NONE',  ( 0.7939632545931766261, -0.2845877964562161244, -0.3641732283464567121 ) ) ;
#75645=CARTESIAN_POINT ( 'NONE',  ( -0.2296587926509179312, -0.05778040916215522460, 0.4822834645669289988 ) ) ;
#75646=CARTESIAN_POINT ( 'NONE',  ( -0.8989501312335946848, -0.6692913385826771977, 0.1292274648535927661 ) ) ;
#75647=CARTESIAN_POINT ( 'NONE',  ( 1.305774278215223960, -0.6692913385826771977, 0.1292274648535927661 ) ) ;
#75650=CARTESIAN_POINT ( 'NONE',  ( -0.1706036745406816491, -0.3690944881889763329, 0.3153832671262228327 ) ) ;
#75653=ORIENTED_EDGE ( 'NONE', *, *, #82446, .T. ) ;
#75654=CARTESIAN_POINT ( 'NONE',  ( -0.8595800524934373854, -0.3162353388693409650, -0.4822834645669289433 ) ) ;
#75655=CARTESIAN_POINT ( 'NONE',  ( -0.1771653543307080136, 0.1660481256975883668, -0.3530559997133364547 ) ) ;
#75656=CARTESIAN_POINT ( 'NONE',  ( -0.2952755905511803003, -0.5400638737290845981, -0.3530559997133363437 ) ) ;
#75657=CARTESIAN_POINT ( 'NONE',  ( 0.2952755905511819101, 0.1660481256975883668, -0.3530559997133364547 ) ) ;
#75658=CARTESIAN_POINT ( 'NONE',  ( -0.4790026246719152336, -0.05778040916215560624, -0.4822834645669293319 ) ) ;
#75659=CARTESIAN_POINT ( 'NONE',  ( -1.482939632545930975, 0.05413385826771666132, 0.4176697321401328100 ) ) ;
#75660=CARTESIAN_POINT ( 'NONE',  ( -0.7152230971128602510, -0.05778040916215560624, -0.4822834645669293319 ) ) ;
#75661=CARTESIAN_POINT ( 'NONE',  ( 0.5774278215223103139, -0.6046776061558809534, -0.2411417322834644161 ) ) ;
#75662=ADVANCED_FACE ( 'NONE', ( #18274 ), #31712, .F. ) ;
#75664=CARTESIAN_POINT ( 'NONE',  ( -0.3018372703412066094, -0.3690944881889765550, -0.3153832671262227771 ) ) ;
#75665=VERTEX_POINT ( 'NONE', #82656 ) ;
#75668=CARTESIAN_POINT ( 'NONE',  ( -1.115485564304461219, -0.3690944881889763329, 0.3153832671262228327 ) ) ;
#75669=CARTESIAN_POINT ( 'NONE',  ( -1.108923884514435132, -0.05778040916215560624, -0.4822834645669293319 ) ) ;
#75670=CARTESIAN_POINT ( 'NONE',  ( -0.8661417322834640276, -0.1870078740157479769, 0.4822834645669291653 ) ) ;
#75672=CARTESIAN_POINT ( 'NONE',  ( -0.6758530183727028406, -0.6692913385826773087, -0.1292274648535924053 ) ) ;
#75673=CARTESIAN_POINT ( 'NONE',  ( -0.8661417322834640276, -0.1870078740157480879, -0.4822834645669291653 ) ) ;
#75676=CARTESIAN_POINT ( 'NONE',  ( 0.4921259842519691285, -0.4536011799217368745, -0.2665933059059886201 ) ) ;
#75679=CARTESIAN_POINT ( 'NONE',  ( -0.09842519685039295696, 0.07958543189024071263, -0.2665933059059888421 ) ) ;
#75680=CARTESIAN_POINT ( 'NONE',  ( -0.1640419947506553400, -0.05778040916215560624, -0.4822834645669293319 ) ) ;
#75681=CARTESIAN_POINT ( 'NONE',  ( 1.604771003085129433, 1.044625174762918496, 0.1466069496707750885 ) ) ;
#75682=CARTESIAN_POINT ( 'NONE',  ( -0.03280839895013062252, 0.2952755905511810774, -0.1292274648535930714 ) ) ;
#75683=ORIENTED_EDGE ( 'NONE', *, *, #58402, .F. ) ;
#75685=CARTESIAN_POINT ( 'NONE',  ( 0.2477166185931112263, 2.056812631849083806E-16, 0.3791483426435167670 ) ) ;
#75689=CARTESIAN_POINT ( 'NONE',  ( -1.299212598425196097, -0.5511811023622047445, 6.969142054262312111E-17 ) ) ;
#75690=CARTESIAN_POINT ( 'NONE',  ( -1.535433070866141225, 0.2952755905511811885, 0.000000000000000000 ) ) ;
#75694=CARTESIAN_POINT ( 'NONE',  ( 1.286089238845145033, -0.6046776061558809534, -0.2411417322834644161 ) ) ;
#75695=CARTESIAN_POINT ( 'NONE',  ( 0.4724409448818904789, -0.1870078740157479769, 0.4822834645669291653 ) ) ;
#75696=CARTESIAN_POINT ( 'NONE',  ( -0.1049868766404193215, -0.6046776061558807314, 0.2411417322834647770 ) ) ;
#75697=CARTESIAN_POINT ( 'NONE',  ( -1.030183727034119867, -0.2845877964562159024, 0.3641732283464567677 ) ) ;
#75698=CARTESIAN_POINT ( 'NONE',  ( -0.5643044619422565855, 0.05413385826771626580, -0.4176697321401330321 ) ) ;
#75700=CARTESIAN_POINT ( 'NONE',  ( -0.9317585301837263412, 0.05413385826771666132, 0.4176697321401328100 ) ) ;
#75702=CARTESIAN_POINT ( 'NONE',  ( 1.253280839895013710, -0.2845877964562159024, 0.3641732283464567677 ) ) ;
#75703=CARTESIAN_POINT ( 'NONE',  ( -0.5314960629921254842, -0.4536011799217368745, -0.2665933059059886201 ) ) ;
#75704=CIRCLE ( 'NONE', #8471, 2.401574803149606474 ) ;
#75705=CARTESIAN_POINT ( 'NONE',  ( 1.181102362204725198, -0.1870078740157479769, 0.3641732283464567677 ) ) ;
#75706=CARTESIAN_POINT ( 'NONE',  ( -1.548556430446193399, 0.2306618581243848609, 0.2411417322834645549 ) ) ;
#75707=CARTESIAN_POINT ( 'NONE',  ( -0.9776902887139098386, 0.1771653543307087075, -0.09757992244046823083 ) ) ;
#75709=CARTESIAN_POINT ( 'NONE',  ( 0.5118110236220480003, -0.5511811023622047445, 6.969142054262312111E-17 ) ) ;
#75710=CARTESIAN_POINT ( 'NONE',  ( -0.5052493438320203589, 0.2952755905511810774, -0.1292274648535930714 ) ) ;
#75711=CARTESIAN_POINT ( 'NONE',  ( 0.3033747635708586854, 0.02791078216816508459, -0.4328096321851889194 ) ) ;
#75712=CARTESIAN_POINT ( 'NONE',  ( 0.07217847769028949700, -0.2845877964562159024, 0.3641732283464567677 ) ) ;
#75714=CARTESIAN_POINT ( 'NONE',  ( 0.8661417322834653598, -0.1870078740157479769, 0.4822834645669291653 ) ) ;
#75717=CARTESIAN_POINT ( 'NONE',  ( 1.371391076115485719, -0.5511811023622048555, -0.09757992244046775898 ) ) ;
#75718=CARTESIAN_POINT ( 'NONE',  ( -0.8005249343832013809, -0.4281496062992124485, 0.4176697321401328655 ) ) ;
#75719=CARTESIAN_POINT ( 'NONE',  ( -0.3149606299212590610, -0.1870078740157480601, -0.3641732283464567677 ) ) ;
#75721=CARTESIAN_POINT ( 'NONE',  ( 0.2034120734908142214, 0.1771653543307087075, -0.09757992244046823083 ) ) ;
#75722=CARTESIAN_POINT ( 'NONE',  ( -1.207349081364828880, 0.2306618581243847221, -0.2411417322834647770 ) ) ;
#75723=CARTESIAN_POINT ( 'NONE',  ( -0.5314960629921250401, 0.1660481256975885056, 0.3530559997133364547 ) ) ;
#75726=CARTESIAN_POINT ( 'NONE',  ( 0.5839895013123367340, -0.5511811023622048555, -0.09757992244046775898 ) ) ;
#75727=CARTESIAN_POINT ( 'NONE',  ( -0.3083989501312330295, -0.3162353388693409650, -0.4822834645669289433 ) ) ;
#75728=CARTESIAN_POINT ( 'NONE',  ( -0.5577427821522301654, -0.3162353388693405765, 0.4822834645669290543 ) ) ;
#75729=CARTESIAN_POINT ( 'NONE',  ( -0.9711286089238838626, 0.1283753931104746893, -0.1820866141732285504 ) ) ;
#75731=CARTESIAN_POINT ( 'NONE',  ( -0.1706036745406816491, 0.05413385826771626580, -0.4176697321401330321 ) ) ;
#75732=CARTESIAN_POINT ( 'NONE',  ( -1.246719160104986512, -0.004921259842519576551, 0.3153832671262227771 ) ) ;
#75733=CARTESIAN_POINT ( 'NONE',  ( -1.371391076115484609, -0.6692913385826771977, 0.1292274648535927661 ) ) ;
#75735=ORIENTED_EDGE ( 'NONE', *, *, #69293, .F. ) ;
#75736=CARTESIAN_POINT ( 'NONE',  ( -1.482939632545930975, -0.3690944881889765550, -0.3153832671262227771 ) ) ;
#75737=CARTESIAN_POINT ( 'NONE',  ( -1.174540682414697335, -0.3162353388693409650, -0.4822834645669289433 ) ) ;
#75738=CARTESIAN_POINT ( 'NONE',  ( -0.7283464566929126471, 0.1660481256975883668, -0.3530559997133364547 ) ) ;
#75739=CARTESIAN_POINT ( 'NONE',  ( -1.423884514435694859, -0.05778040916215560624, -0.4822834645669293319 ) ) ;
#75742=CARTESIAN_POINT ( 'NONE',  ( 1.089238845144357759, 0.05413385826771626580, -0.4176697321401330321 ) ) ;
#75743=CARTESIAN_POINT ( 'NONE',  ( 0.5971128608923891301, 0.2952755905511810774, -0.1292274648535930714 ) ) ;
#75746=CARTESIAN_POINT ( 'NONE',  ( 1.259842519685040019, -0.1870078740157479769, 0.3641732283464567677 ) ) ;
#75747=B_SPLINE_CURVE_WITH_KNOTS ( 'NONE', 3,
 ( #18461, #5813, #48777, #16823, #68159, #10503, #55912 ),
 .UNSPECIFIED., .F., .F.,
 ( 4, 3, 4 ),
 ( 3.469446951953614189E-18, 0.001246230184515571522, 0.002492489877932649398 ),
 .UNSPECIFIED. ) ;
#75752=CARTESIAN_POINT ( 'NONE',  ( 0.4330708661417329575, -0.6692913385826771977, 8.415575281601705876E-17 ) ) ;
#75753=CARTESIAN_POINT ( 'NONE',  ( -0.6627296587926503335, -0.6692913385826771977, 0.1292274648535927661 ) ) ;
#75754=CARTESIAN_POINT ( 'NONE',  ( 1.561679790026247350, -0.4281496062992124485, 0.4176697321401328655 ) ) ;
#75755=CARTESIAN_POINT ( 'NONE',  ( 0.9973753280839902091, -0.6046776061558807314, 0.2411417322834647770 ) ) ;
#75756=CARTESIAN_POINT ( 'NONE',  ( -1.653543307086613234, -0.1870078740157479769, 0.3641732283464567677 ) ) ;
#75757=DIRECTION ( 'NONE',  ( 0.7071067811865489050, 2.189697074797801291E-16, -0.7071067811865460184 ) ) ;
#75758=CARTESIAN_POINT ( 'NONE',  ( -0.1706036745406816491, 0.05413385826771626580, -0.4176697321401330321 ) ) ;
#75759=CARTESIAN_POINT ( 'NONE',  ( -1.423884514435694859, -0.05778040916215560624, -0.4822834645669293319 ) ) ;
#75760=CARTESIAN_POINT ( 'NONE',  ( -1.502624671916009680, -0.3162353388693405765, 0.4822834645669290543 ) ) ;
#75761=CARTESIAN_POINT ( 'NONE',  ( 1.417322834645670104, -0.1870078740157480879, -0.4822834645669291653 ) ) ;
#75763=CARTESIAN_POINT ( 'NONE',  ( 0.6496062992125991586, -0.4536011799217368745, -0.2665933059059886201 ) ) ;
#75767=CARTESIAN_POINT ( 'NONE',  ( 0.07217847769028949700, -0.08942795157528024563, -0.3641732283464568787 ) ) ;
#75768=CARTESIAN_POINT ( 'NONE',  ( -1.541994750656167090, 0.2952755905511811885, 0.1292274648535926551 ) ) ;
#75769=CARTESIAN_POINT ( 'NONE',  ( 0.3674540682414705883, 0.2306618581243847221, -0.2411417322834647770 ) ) ;
#75770=CARTESIAN_POINT ( 'NONE',  ( 0.3149606299212603933, -0.1870078740157479769, 0.4822834645669291653 ) ) ;
#75771=CARTESIAN_POINT ( 'NONE',  ( -0.6955380577427815458, -0.4281496062992127816, -0.4176697321401328100 ) ) ;
#75772=AXIS2_PLACEMENT_3D ( 'NONE', #4536, #55455, #61789 ) ;
#75774=CARTESIAN_POINT ( 'NONE',  ( -1.108923884514435132, -0.05778040916215560624, -0.4822834645669293319 ) ) ;
#75776=CARTESIAN_POINT ( 'NONE',  ( 1.502624671916010790, -0.2845877964562161244, -0.3641732283464567121 ) ) ;
#75777=CARTESIAN_POINT ( 'NONE',  ( -0.8398950131233585692, 0.2306618581243848609, 0.2411417322834645549 ) ) ;
#75778=CARTESIAN_POINT ( 'NONE',  ( 0.6955380577427828781, -0.4281496062992124485, 0.4176697321401328655 ) ) ;
#75779=CARTESIAN_POINT ( 'NONE',  ( 1.233595800524935227, 0.2306618581243847221, -0.2411417322834647770 ) ) ;
#75781=CARTESIAN_POINT ( 'NONE',  ( -1.555118110236219930, 0.1660481256975885056, 0.3530559997133364547 ) ) ;
#75783=CARTESIAN_POINT ( 'NONE',  ( 0.1837270341207354329, 0.2306618581243848609, 0.2411417322834645549 ) ) ;
#75786=CARTESIAN_POINT ( 'NONE',  ( 1.627296587926509996, -0.6046776061558807314, 0.2411417322834647770 ) ) ;
#75787=CARTESIAN_POINT ( 'NONE',  ( 0.1115485564304470323, 0.1771653543307087630, 0.09757992244046791164 ) ) ;
#75788=CARTESIAN_POINT ( 'NONE',  ( 0.8333333333333340365, 0.2952755905511810774, -0.1292274648535930714 ) ) ;
#75790=CARTESIAN_POINT ( 'NONE',  ( 0.8267716535433078384, -0.5511811023622047445, 6.969142054262312111E-17 ) ) ;
#75791=CARTESIAN_POINT ( 'NONE',  ( 0.5380577427821529035, 0.05413385826771626580, -0.4176697321401330321 ) ) ;
#75793=CARTESIAN_POINT ( 'NONE',  ( -0.7480314960629914633, 0.2952755905511811885, 0.000000000000000000 ) ) ;
#75795=CARTESIAN_POINT ( 'NONE',  ( 0.7939632545931766261, -0.08942795157527998196, 0.3641732283464567121 ) ) ;
#75797=CARTESIAN_POINT ( 'NONE',  ( -0.3412073490813641308, -0.6046776061558807314, 0.2411417322834647770 ) ) ;
#75798=ADVANCED_FACE ( 'NONE', ( #43915 ), #44385, .F. ) ;
#75799=CARTESIAN_POINT ( 'NONE',  ( 0.3215223097112867578, -0.2845877964562161244, -0.3641732283464567121 ) ) ;
#75801=CARTESIAN_POINT ( 'NONE',  ( -0.2427821522309703550, -0.05778040916215560624, -0.4822834645669293319 ) ) ;
#75802=CARTESIAN_POINT ( 'NONE',  ( 0.7086614173228352742, -0.1870078740157480601, -0.3641732283464567677 ) ) ;
#75803=CARTESIAN_POINT ( 'NONE',  ( -1.114295247146195988, 1.305470409705170549E-15, -0.3627985898453510161 ) ) ;
#75805=CARTESIAN_POINT ( 'NONE',  ( 0.2427821522309719648, -0.05778040916215522460, 0.4822834645669289988 ) ) ;
#75807=CARTESIAN_POINT ( 'NONE',  ( 1.259842519685040019, -0.1870078740157480601, -0.3641732283464567677 ) ) ;
#75809=CARTESIAN_POINT ( 'NONE',  ( -0.4724409448818890911, -0.1870078740157479769, 0.3641732283464567677 ) ) ;
#75810=CARTESIAN_POINT ( 'NONE',  ( -0.6233595800524928121, -0.08942795157527998196, 0.3641732283464567121 ) ) ;
#75811=CARTESIAN_POINT ( 'NONE',  ( -0.5118110236220466680, 0.2952755905511811885, 0.000000000000000000 ) ) ;
#75812=CARTESIAN_POINT ( 'NONE',  ( 0.4461942257217855201, -0.6046776061558807314, 0.2411417322834647770 ) ) ;
#75813=CARTESIAN_POINT ( 'NONE',  ( 0.9645669291338591078, -0.4536011799217368745, -0.2665933059059886201 ) ) ;
#75815=CARTESIAN_POINT ( 'NONE',  ( 1.496062992125984703, -0.1870078740157480601, -0.3641732283464567677 ) ) ;
#75817=CARTESIAN_POINT ( 'NONE',  ( 0.9055118110236227702, 0.2952755905511811885, 0.000000000000000000 ) ) ;
#75820=CARTESIAN_POINT ( 'NONE',  ( -0.2296587926509179312, -0.3162353388693409650, -0.4822834645669289433 ) ) ;
#75822=CARTESIAN_POINT ( 'NONE',  ( 0.9383202099737538715, -0.05778040916215560624, -0.4822834645669293319 ) ) ;
#75823=CARTESIAN_POINT ( 'NONE',  ( 0.4724409448818904789, -0.1870078740157480879, -0.4822834645669291653 ) ) ;
#75826=CARTESIAN_POINT ( 'NONE',  ( 0.2493438320209980519, -0.004921259842519576551, 0.3153832671262227771 ) ) ;
#75827=CARTESIAN_POINT ( 'NONE',  ( 1.017060367454068803, -0.3162353388693405765, 0.4822834645669290543 ) ) ;
#75828=CARTESIAN_POINT ( 'NONE',  ( 0.1377952755905518800, -0.4536011799217367080, 0.2665933059059888421 ) ) ;
#75829=CARTESIAN_POINT ( 'NONE',  ( -0.3937007874015740483, -0.1870078740157479769, 0.4822834645669291653 ) ) ;
#75831=CARTESIAN_POINT ( 'NONE',  ( 0.1181102362204730916, -0.6692913385826771977, 8.415575281601705876E-17 ) ) ;
#75832=CARTESIAN_POINT ( 'NONE',  ( -0.8005249343832011588, 0.05413385826771626580, -0.4176697321401330321 ) ) ;
#75833=CARTESIAN_POINT ( 'NONE',  ( -0.1640419947506555343, -0.2845877964562159024, 0.3641732283464567677 ) ) ;
#75834=CARTESIAN_POINT ( 'NONE',  ( 0.3543307086614179147, 0.2952755905511811885, 0.000000000000000000 ) ) ;
#75835=CARTESIAN_POINT ( 'NONE',  ( 0.8136482939632553313, -0.5023911411419708095, -0.1820866141732282451 ) ) ;
#75836=CARTESIAN_POINT ( 'NONE',  ( -0.3937007874015740483, -0.1870078740157479769, 0.4822834645669291653 ) ) ;
#75838=CARTESIAN_POINT ( 'NONE',  ( 1.286089238845145033, 0.2306618581243848609, 0.2411417322834645549 ) ) ;
#75839=CARTESIAN_POINT ( 'NONE',  ( 1.574803149606299746, -0.1870078740157480879, -0.4822834645669291653 ) ) ;
#75841=CARTESIAN_POINT ( 'NONE',  ( -1.286089238845143479, 0.2306618581243847221, -0.2411417322834647770 ) ) ;
#75842=CARTESIAN_POINT ( 'NONE',  ( -0.8792650918635160906, 0.05413385826771626580, -0.4176697321401330321 ) ) ;
#75846=CARTESIAN_POINT ( 'NONE',  ( 0.3740157480314966754, -0.4536011799217367080, 0.2665933059059888421 ) ) ;
#75848=CARTESIAN_POINT ( 'NONE',  ( 0.8267716535433077274, 0.2952755905511811885, 0.000000000000000000 ) ) ;
#75850=CARTESIAN_POINT ( 'NONE',  ( 0.9908136482939640111, 0.2952755905511810219, -0.1292274648535930437 ) ) ;
#75851=CARTESIAN_POINT ( 'NONE',  ( -0.3871391076115476282, -0.08942795157527998196, 0.3641732283464567121 ) ) ;
#75852=CARTESIAN_POINT ( 'NONE',  ( 0.4849061582275024929, 1.805669738366188382, -0.4921425059946357150 ) ) ;
#75853=CARTESIAN_POINT ( 'NONE',  ( 1.017060367454068803, -0.3162353388693405765, 0.4822834645669290543 ) ) ;
#75854=CARTESIAN_POINT ( 'NONE',  ( 1.364829396325459854, -0.5023911411419708095, -0.1820866141732282451 ) ) ;
#75855=CARTESIAN_POINT ( 'NONE',  ( -0.1181102362204717315, -0.6692913385826771977, 8.415575281601705876E-17 ) ) ;
#75857=CARTESIAN_POINT ( 'NONE',  ( -0.4527559055118102749, -0.5400638737290845981, -0.3530559997133363437 ) ) ;
#75858=CARTESIAN_POINT ( 'NONE',  ( -1.469816272965878357, -0.5023911411419708095, -0.1820866141732282451 ) ) ;
#75859=CARTESIAN_POINT ( 'NONE',  ( -0.3805774278215216522, -0.4281496062992127816, -0.4176697321401328100 ) ) ;
#75860=CARTESIAN_POINT ( 'NONE',  ( 1.646981627296588035, -0.3162353388693405765, 0.4822834645669290543 ) ) ;
#75862=ORIENTED_EDGE ( 'NONE', *, *, #50024, .F. ) ;
#75864=CARTESIAN_POINT ( 'NONE',  ( 0.4724409448818904789, -0.1870078740157480879, -0.4822834645669291653 ) ) ;
#75866=CARTESIAN_POINT ( 'NONE',  ( -0.2099737532808391705, -0.6046776061558809534, -0.2411417322834644161 ) ) ;
#75867=CARTESIAN_POINT ( 'NONE',  ( -1.423884514435694859, -0.05778040916215560624, -0.4822834645669293319 ) ) ;
#75868=CARTESIAN_POINT ( 'NONE',  ( 0.6036745406824153282, -0.6046776061558807314, 0.2411417322834647770 ) ) ;
#75869=CARTESIAN_POINT ( 'NONE',  ( -0.1115485564304453947, -0.6692913385826771977, 0.1292274648535927661 ) ) ;
#75871=CARTESIAN_POINT ( 'NONE',  ( -0.8923884514435688198, 0.2306618581243847221, -0.2411417322834647770 ) ) ;
#75872=CARTESIAN_POINT ( 'NONE',  ( 0.4265091863517067594, 0.2952755905511811885, 0.1292274648535926551 ) ) ;
#75873=CARTESIAN_POINT ( 'NONE',  ( -0.6036745406824141069, -0.6046776061558809534, -0.2411417322834644161 ) ) ;
#75875=CARTESIAN_POINT ( 'NONE',  ( 0.2821522309711292364, 0.1771653543307087075, -0.09757992244046823083 ) ) ;
#75877=CARTESIAN_POINT ( 'NONE',  ( 0.07874015748031558404, -0.1870078740157480879, -0.4822834645669291653 ) ) ;
#75878=CARTESIAN_POINT ( 'NONE',  ( 0.3025410870193226964, 2.784432375088962958E-17, -0.3464511005275205946 ) ) ;
#75880=CARTESIAN_POINT ( 'NONE',  ( -1.633858267716534529, 0.1660481256975885056, 0.3530559997133364547 ) ) ;
#75882=ORIENTED_EDGE ( 'NONE', *, *, #15723, .F. ) ;
#75884=CARTESIAN_POINT ( 'NONE',  ( 0.6955380577427828781, -0.4281496062992124485, 0.4176697321401328655 ) ) ;
#75885=CARTESIAN_POINT ( 'NONE',  ( 0.1837270341207354329, 0.1283753931104748280, 0.1820866141732283561 ) ) ;
#75886=CARTESIAN_POINT ( 'NONE',  ( 0.9559795740584967616, -8.614921172258640174E-17, 0.3954974714151467396 ) ) ;
#75891=CIRCLE ( 'NONE', #39591, 3.543307086614173596 ) ;
#75893=CARTESIAN_POINT ( 'NONE',  ( 0.2755905511811031494, -0.6692913385826771977, 8.415575281601705876E-17 ) ) ;
#75894=CARTESIAN_POINT ( 'NONE',  ( -1.305774278215222184, 0.2952755905511811885, 0.1292274648535926551 ) ) ;
#75895=CARTESIAN_POINT ( 'NONE',  ( -1.259842519685038686, -0.1870078740157479769, 0.4822834645669291653 ) ) ;
#75896=CARTESIAN_POINT ( 'NONE',  ( 0.4396325459317590445, -0.6692913385826771977, 0.1292274648535927661 ) ) ;
#75897=CARTESIAN_POINT ( 'NONE',  ( 0.9186351706036751663, -0.6046776061558807314, 0.2411417322834647770 ) ) ;
#75898=CARTESIAN_POINT ( 'NONE',  ( 1.541994750656168645, 0.1771653543307087075, -0.09757992244046823083 ) ) ;
#75899=CARTESIAN_POINT ( 'NONE',  ( 1.167979002624672580, -0.3690944881889763329, 0.3153832671262228327 ) ) ;
#75900=CARTESIAN_POINT ( 'NONE',  ( -0.8333333333333323711, 0.2952755905511811885, 0.1292274648535926551 ) ) ;
#75902=CARTESIAN_POINT ( 'NONE',  ( 1.535433070866142558, 0.2952755905511811885, 0.000000000000000000 ) ) ;
#75905=CARTESIAN_POINT ( 'NONE',  ( -0.07874015748031421014, -0.1870078740157479769, 0.4822834645669291653 ) ) ;
#75906=CARTESIAN_POINT ( 'NONE',  ( 1.082677165354331228, 0.1660481256975883668, -0.3530559997133364547 ) ) ;
#75908=CARTESIAN_POINT ( 'NONE',  ( -1.489501312335957062, -0.2845877964562161244, -0.3641732283464567121 ) ) ;
#75909=CARTESIAN_POINT ( 'NONE',  ( 0.1377952755905518800, 0.1660481256975883668, -0.3530559997133364547 ) ) ;
#75910=CARTESIAN_POINT ( 'NONE',  ( 0.7611548556430451917, -0.5023911411419708095, 0.1820866141732285504 ) ) ;
#75911=CARTESIAN_POINT ( 'NONE',  ( -1.568241469816272105, -0.08942795157527998196, 0.3641732283464567121 ) ) ;
#75912=CARTESIAN_POINT ( 'NONE',  ( 1.095800524934383846, -0.05778040916215560624, -0.4822834645669293319 ) ) ;
#75914=CARTESIAN_POINT ( 'NONE',  ( -0.6036745406824141069, 0.1283753931104748280, 0.1820866141732283561 ) ) ;
#75915=CARTESIAN_POINT ( 'NONE',  ( -0.7086614173228339419, -0.1870078740157480879, -0.4822834645669291653 ) ) ;
#75916=CARTESIAN_POINT ( 'NONE',  ( 1.581364829396326277, -0.3162353388693409650, -0.4822834645669289433 ) ) ;
#75917=CARTESIAN_POINT ( 'NONE',  ( -1.017060367454067249, -0.3162353388693409650, -0.4822834645669289433 ) ) ;
#75918=CARTESIAN_POINT ( 'NONE',  ( 1.227034120734908917, 0.2952755905511810774, -0.1292274648535930714 ) ) ;
#75920=CARTESIAN_POINT ( 'NONE',  ( -1.371391076115484609, -0.5511811023622046335, 0.09757992244046803654 ) ) ;
#75922=CARTESIAN_POINT ( 'NONE',  ( 1.332020997375328974, -0.05778040916215560624, -0.4822834645669293319 ) ) ;
#75924=CARTESIAN_POINT ( 'NONE',  ( -1.463254593175852492, -0.6692913385826773087, -0.1292274648535924053 ) ) ;
#75925=CARTESIAN_POINT ( 'NONE',  ( -1.404199475065615932, -0.3690944881889765550, -0.3153832671262227771 ) ) ;
#75926=CARTESIAN_POINT ( 'NONE',  ( -0.9514435695538050464, -0.2845877964562159024, 0.3641732283464567677 ) ) ;
#75928=CARTESIAN_POINT ( 'NONE',  ( -0.2034120734908128059, 0.2952755905511811885, 0.1292274648535926551 ) ) ;
#75929=CARTESIAN_POINT ( 'NONE',  ( 8.195543980992789655E-16, -0.1870078740157480601, -0.3641732283464567677 ) ) ;
#75930=CARTESIAN_POINT ( 'NONE',  ( -1.102362204724408601, -0.1870078740157479769, 0.3641732283464567677 ) ) ;
#75931=CARTESIAN_POINT ( 'NONE',  ( 1.358267716535433323, -0.4536011799217368745, -0.2665933059059886201 ) ) ;
#75932=CARTESIAN_POINT ( 'NONE',  ( 0.8070866141732289112, -0.5400638737290845981, -0.3530559997133363437 ) ) ;
#75933=CARTESIAN_POINT ( 'NONE',  ( 1.437007874015748810, 0.1660481256975885056, 0.3530559997133364547 ) ) ;
#75934=CARTESIAN_POINT ( 'NONE',  ( 0.5774278215223104249, 0.1283753931104748280, 0.1820866141732283561 ) ) ;
#75936=CARTESIAN_POINT ( 'NONE',  ( 0.4002624671916016896, -0.05778040916215522460, 0.4822834645669289988 ) ) ;
#75937=CARTESIAN_POINT ( 'NONE',  ( 1.003937007874016185, 0.07958543189024071263, -0.2665933059059888421 ) ) ;
#75938=EDGE_LOOP ( 'NONE', ( #58678, #20904, #54116, #67091 ) ) ;
#75939=CARTESIAN_POINT ( 'NONE',  ( 1.496062992125984703, -0.1870078740157480879, -0.4822834645669291653 ) ) ;
#75940=CARTESIAN_POINT ( 'NONE',  ( -1.213910761154854745, -0.6692913385826771977, 0.1292274648535927661 ) ) ;
#75941=CARTESIAN_POINT ( 'NONE',  ( -0.05249343832020938322, -0.6046776061558809534, -0.2411417322834644161 ) ) ;
#75944=CARTESIAN_POINT ( 'NONE',  ( 0.3346456692913390985, 0.1660481256975885056, 0.3530559997133364547 ) ) ;
#75945=CARTESIAN_POINT ( 'NONE',  ( 1.200787401574803681, -0.4536011799217368745, -0.2665933059059886201 ) ) ;
#75946=CARTESIAN_POINT ( 'NONE',  ( 0.2165354330708668673, -0.5400638737290844871, 0.3530559997133364547 ) ) ;
#75947=CARTESIAN_POINT ( 'NONE',  ( 0.1902887139107617975, 0.2952755905511811885, 0.1292274648535926551 ) ) ;
#75950=VECTOR ( 'NONE', #205, 39.37007874015748143 ) ;
#75955=EDGE_CURVE ( 'NONE', #22261, #47474, #70731, .T. ) ;
#75956=CARTESIAN_POINT ( 'NONE',  ( -0.4396325459317579898, 0.1771653543307087630, 0.09757992244046791164 ) ) ;
#75957=CARTESIAN_POINT ( 'NONE',  ( -0.8923884514435688198, 0.2306618581243847221, -0.2411417322834647770 ) ) ;
#75958=CARTESIAN_POINT ( 'NONE',  ( 0.5839895013123367340, -0.6692913385826773087, -0.1292274648535924053 ) ) ;
#75960=CARTESIAN_POINT ( 'NONE',  ( 0.7414698162729663755, 0.2952755905511811885, 0.1292274648535926551 ) ) ;
#75961=CARTESIAN_POINT ( 'NONE',  ( -1.377952755905511140, -0.6692913385826771977, 8.415575281601705876E-17 ) ) ;
#75962=CARTESIAN_POINT ( 'NONE',  ( 0.6299212598425204535, -0.1870078740157479769, 0.4822834645669291653 ) ) ;
#75963=CARTESIAN_POINT ( 'NONE',  ( -0.6184250938292459310, -3.724876541855331158E-15, 0.3791475997938233422 ) ) ;
#75965=CARTESIAN_POINT ( 'NONE',  ( 1.561679790026247350, 0.05413385826771626580, -0.4176697321401330321 ) ) ;
#75966=CARTESIAN_POINT ( 'NONE',  ( 0.7677165354330716118, -0.5400638737290844871, 0.3530559997133364547 ) ) ;
#75967=CARTESIAN_POINT ( 'NONE',  ( 0.3871391076115492380, -0.05778040916215560624, -0.4822834645669293319 ) ) ;
#75968=CARTESIAN_POINT ( 'NONE',  ( 1.423884514435696191, -0.08942795157527998196, 0.3641732283464567121 ) ) ;
#75969=CARTESIAN_POINT ( 'NONE',  ( 1.410761154855643795, -0.05778040916215560624, -0.4822834645669293319 ) ) ;
#75972=CARTESIAN_POINT ( 'NONE',  ( 0.9580052493438327987, -0.4281496062992127816, -0.4176697321401328100 ) ) ;
#75973=CARTESIAN_POINT ( 'NONE',  ( 1.594488188976378673, -0.4536011799217368745, -0.2665933059059886201 ) ) ;
#75974=CARTESIAN_POINT ( 'NONE',  ( -0.3477690288713905509, -0.6692913385826771977, 0.1292274648535927661 ) ) ;
#75975=CARTESIAN_POINT ( 'NONE',  ( -1.095800524934382292, -0.05778040916215522460, 0.4822834645669289988 ) ) ;
#75976=CARTESIAN_POINT ( 'NONE',  ( 0.9842519685039375910, 0.2952755905511811885, 0.000000000000000000 ) ) ;
#75980=CARTESIAN_POINT ( 'NONE',  ( 1.522309711286089939, 0.2306618581243848609, 0.2411417322834645549 ) ) ;
#75981=ORIENTED_EDGE ( 'NONE', *, *, #16494, .F. ) ;
#75985=CARTESIAN_POINT ( 'NONE',  ( 1.561679790026247350, -0.3690944881889763329, 0.3153832671262228327 ) ) ;
#75987=CARTESIAN_POINT ( 'NONE',  ( 1.450131233595801428, -0.5511811023622048555, -0.09757992244046775898 ) ) ;
#75990=CARTESIAN_POINT ( 'NONE',  ( 0.8537221893815273299, 2.409604939980833412E-17, -0.3464511005275205946 ) ) ;
#75992=CARTESIAN_POINT ( 'NONE',  ( -0.5380577427821514602, -0.004921259842519576551, 0.3153832671262227771 ) ) ;
#75993=CARTESIAN_POINT ( 'NONE',  ( -1.102362204724408601, -0.1870078740157479769, 0.3641732283464567677 ) ) ;
#75994=CARTESIAN_POINT ( 'NONE',  ( -1.430446194225720724, 0.05413385826771626580, -0.4176697321401330321 ) ) ;
#75995=CARTESIAN_POINT ( 'NONE',  ( 0.1115485564304467270, -0.6692913385826773087, -0.1292274648535924053 ) ) ;
#75996=CARTESIAN_POINT ( 'NONE',  ( -1.620734908136482577, 0.2952755905511811885, 0.1292274648535926551 ) ) ;
#75997=ORIENTED_EDGE ( 'NONE', *, *, #66513, .T. ) ;
#75998=CARTESIAN_POINT ( 'NONE',  ( -1.614173228346455824, 0.2952755905511811885, 0.000000000000000000 ) ) ;
#75999=CARTESIAN_POINT ( 'NONE',  ( -1.013613127888308485, -2.191421614605370878E-15, 0.4445507791589071167 ) ) ;
#76002=CARTESIAN_POINT ( 'NONE',  ( 2.795275590551181466, 2.793565526369266916, 0.000000000000000000 ) ) ;
#76003=CARTESIAN_POINT ( 'NONE',  ( -0.4265091863517051496, -0.5511811023622046335, 0.09757992244046803654 ) ) ;
#76004=CARTESIAN_POINT ( 'NONE',  ( -1.351706036745406347, -0.4281496062992124485, 0.4176697321401328655 ) ) ;
#76005=CARTESIAN_POINT ( 'NONE',  ( 1.095800524934383846, -0.05778040916215560624, -0.4822834645669293319 ) ) ;
#76009=CARTESIAN_POINT ( 'NONE',  ( 1.555118110236221041, 0.1660481256975883668, -0.3530559997133364547 ) ) ;
#76010=CARTESIAN_POINT ( 'NONE',  ( -1.286089238845143479, -0.6046776061558807314, 0.2411417322834647770 ) ) ;
#76012=CARTESIAN_POINT ( 'NONE',  ( -0.1968503937007867743, -0.5511811023622047445, 6.969142054262312111E-17 ) ) ;
#76014=CARTESIAN_POINT ( 'NONE',  ( -0.4396325459317577122, -0.5511811023622048555, -0.09757992244046775898 ) ) ;
#76015=CARTESIAN_POINT ( 'NONE',  ( 0.6758530183727039509, 0.1771653543307087075, -0.09757992244046823083 ) ) ;
#76016=CARTESIAN_POINT ( 'NONE',  ( 0.09186351706036799403, -0.4281496062992127816, -0.4176697321401328100 ) ) ;
#76017=CARTESIAN_POINT ( 'NONE',  ( -0.5971128608923877978, -0.5511811023622048555, -0.09757992244046775898 ) ) ;
#76019=CARTESIAN_POINT ( 'NONE',  ( 1.246719160104987623, -0.4281496062992124485, 0.4176697321401328655 ) ) ;
#76021=CARTESIAN_POINT ( 'NONE',  ( -1.207349081364828436, -0.6046776061558807314, 0.2411417322834647770 ) ) ;
#76023=CARTESIAN_POINT ( 'NONE',  ( -0.5249343832020990641, -0.6046776061558809534, -0.2411417322834644161 ) ) ;
#76024=CARTESIAN_POINT ( 'NONE',  ( -0.7677165354330699465, -0.5400638737290845981, -0.3530559997133363437 ) ) ;
#76025=CARTESIAN_POINT ( 'NONE',  ( 1.417322834645670104, -0.1870078740157480601, -0.3641732283464567677 ) ) ;
#76026=CARTESIAN_POINT ( 'NONE',  ( 0.2362204724409456558, -0.1870078740157480601, -0.3641732283464567677 ) ) ;
#76027=CARTESIAN_POINT ( 'NONE',  ( -0.3740157480314953431, -0.5400638737290845981, -0.3530559997133363437 ) ) ;
#76028=CARTESIAN_POINT ( 'NONE',  ( -1.023622047244093558, -0.1870078740157479769, 0.4822834645669291653 ) ) ;
#76029=CARTESIAN_POINT ( 'NONE',  ( -0.8785612751854012803, -2.613618158232546091E-15, -0.3464511005275220379 ) ) ;
#76031=CARTESIAN_POINT ( 'NONE',  ( -0.3477690288713902178, 0.2952755905511810774, -0.1292274648535930714 ) ) ;
#76032=CARTESIAN_POINT ( 'NONE',  ( -0.9973753280839886548, -0.6046776061558809534, -0.2411417322834644161 ) ) ;
#76033=ORIENTED_EDGE ( 'NONE', *, *, #10993, .T. ) ;
#76035=CARTESIAN_POINT ( 'NONE',  ( 1.253280839895013710, -0.3162353388693405765, 0.4822834645669290543 ) ) ;
#76036=CARTESIAN_POINT ( 'NONE',  ( -0.7611548556430438595, 0.1283753931104748280, 0.1820866141732283561 ) ) ;
#76037=CARTESIAN_POINT ( 'NONE',  ( -0.9776902887139098386, -0.6692913385826771977, 0.1292274648535927661 ) ) ;
#76038=CARTESIAN_POINT ( 'NONE',  ( 1.122047244094488860, -0.5400638737290845981, -0.3530559997133363437 ) ) ;
#76039=CARTESIAN_POINT ( 'NONE',  ( 0.7545931758530189937, 0.2952755905511810774, -0.1292274648535930714 ) ) ;
#76041=CARTESIAN_POINT ( 'NONE',  ( -1.161417322834644716, -0.4536011799217368745, -0.2665933059059886201 ) ) ;
#76047=CARTESIAN_POINT ( 'NONE',  ( 1.371391076115485941, 0.1771653543307087630, 0.09757992244046791164 ) ) ;
#76048=CARTESIAN_POINT ( 'NONE',  ( 0.8333333333333340365, 0.1771653543307087075, -0.09757992244046823083 ) ) ;
#76049=CARTESIAN_POINT ( 'NONE',  ( 0.4461942257217855201, -0.6046776061558807314, 0.2411417322834647770 ) ) ;
#76052=CARTESIAN_POINT ( 'NONE',  ( 0.9645669291338591078, -0.4536011799217368745, -0.2665933059059886201 ) ) ;
#76053=CARTESIAN_POINT ( 'NONE',  ( -0.1377952755905504645, -0.5400638737290845981, -0.3530559997133363437 ) ) ;
#76054=CARTESIAN_POINT ( 'NONE',  ( -1.154855643044618851, 0.2306618581243848609, 0.2411417322834645549 ) ) ;
#76055=CARTESIAN_POINT ( 'NONE',  ( 1.069553805774278832, 0.2952755905511810774, -0.1292274648535930714 ) ) ;
#76058=AXIS2_PLACEMENT_3D ( 'NONE', #5175, #3528, #35931 ) ;
#76059=CARTESIAN_POINT ( 'NONE',  ( -0.1377952755905504645, 0.07958543189024085140, 0.2665933059059887866 ) ) ;
#76062=CARTESIAN_POINT ( 'NONE',  ( -0.9645669291338575535, -0.5400638737290844871, 0.3530559997133364547 ) ) ;
#76063=CARTESIAN_POINT ( 'NONE',  ( -0.5577427821522301654, -0.3162353388693405765, 0.4822834645669290543 ) ) ;
#76064=CARTESIAN_POINT ( 'NONE',  ( -0.5577427821522301654, -0.3162353388693405765, 0.4822834645669290543 ) ) ;
#76065=DIMENSIONAL_EXPONENTS ( 1.000000000000000000, 0.000000000000000000, 0.000000000000000000, 0.000000000000000000, 0.000000000000000000, 0.000000000000000000, 0.000000000000000000 ) ;
#76066=CARTESIAN_POINT ( 'NONE',  ( 0.4396325459317593221, 0.2952755905511810774, -0.1292274648535930714 ) ) ;
#76067=CARTESIAN_POINT ( 'NONE',  ( -0.4658792650918627265, -0.3162353388693409650, -0.4822834645669289433 ) ) ;
#76068=CARTESIAN_POINT ( 'NONE',  ( -1.528871391076114250, -0.6692913385826771977, 0.1292274648535927661 ) ) ;
#76069=CARTESIAN_POINT ( 'NONE',  ( -1.003937007874015297, -0.5400638737290845981, -0.3530559997133363437 ) ) ;
#76070=CARTESIAN_POINT ( 'NONE',  ( 0.7217847769028878924, -0.4281496062992127816, -0.4176697321401328100 ) ) ;
#76072=CARTESIAN_POINT ( 'NONE',  ( -0.4396325459317577122, -0.5511811023622048555, -0.09757992244046775898 ) ) ;
#76073=ORIENTED_EDGE ( 'NONE', *, *, #80383, .F. ) ;
#76076=CARTESIAN_POINT ( 'NONE',  ( -1.391076115485563758, 0.1283753931104748280, 0.1820866141732283561 ) ) ;
#76077=CARTESIAN_POINT ( 'NONE',  ( -1.161417322834644716, 0.1660481256975885056, 0.3530559997133364547 ) ) ;
#76078=CARTESIAN_POINT ( 'NONE',  ( -0.8070866141732276899, 0.1660481256975883668, -0.3530559997133364547 ) ) ;
#76080=CARTESIAN_POINT ( 'NONE',  ( -1.154855643044618851, -0.6046776061558809534, -0.2411417322834644161 ) ) ;
#76081=CARTESIAN_POINT ( 'NONE',  ( -0.8530183727034112984, -0.4281496062992127816, -0.4176697321401328100 ) ) ;
#76082=CARTESIAN_POINT ( 'NONE',  ( -1.535433070866141225, -0.6692913385826771977, 8.415575281601705876E-17 ) ) ;
#76084=CARTESIAN_POINT ( 'NONE',  ( 0.5774278215223104249, 0.1283753931104748280, 0.1820866141732283561 ) ) ;
#76085=DIRECTION ( 'NONE',  ( -1.000000000000000000, 0.000000000000000000, 0.000000000000000000 ) ) ;
#76087=CARTESIAN_POINT ( 'NONE',  ( 0.01312335958005323398, -0.004921259842519576551, 0.3153832671262227771 ) ) ;
#76088=CARTESIAN_POINT ( 'NONE',  ( -0.5249343832020990641, 0.2306618581243848609, 0.2411417322834645549 ) ) ;
#76089=CARTESIAN_POINT ( 'NONE',  ( 1.450131233595801428, 0.2952755905511811885, 0.1292274648535926551 ) ) ;
#76090=CARTESIAN_POINT ( 'NONE',  ( -0.02624671916010428221, 0.2306618581243847221, -0.2411417322834647770 ) ) ;
#76094=ORIENTED_EDGE ( 'NONE', *, *, #82940, .T. ) ;
#76096=CARTESIAN_POINT ( 'NONE',  ( 1.115485564304462551, 0.05413385826771666132, 0.4176697321401328100 ) ) ;
#76097=CARTESIAN_POINT ( 'NONE',  ( -1.135170603674539924, -0.5511811023622046335, 0.09757992244046803654 ) ) ;
#76098=CARTESIAN_POINT ( 'NONE',  ( -1.318897637795274802, -0.5400638737290845981, -0.3530559997133363437 ) ) ;
#76102=CARTESIAN_POINT ( 'NONE',  ( 1.141732283464567788, -0.6692913385826771977, 8.415575281601705876E-17 ) ) ;
#76105=CARTESIAN_POINT ( 'NONE',  ( 0.1509186351706045259, -0.05778040916215560624, -0.4822834645669293319 ) ) ;
#76106=CARTESIAN_POINT ( 'NONE',  ( -1.108923884514435132, -0.08942795157528024563, -0.3641732283464568787 ) ) ;
#76109=CARTESIAN_POINT ( 'NONE',  ( -0.5446194225721777693, -0.3162353388693409650, -0.4822834645669289433 ) ) ;
#76111=CARTESIAN_POINT ( 'NONE',  ( -1.082677165354329896, 0.1660481256975885056, 0.3530559997133364547 ) ) ;
#76113=CARTESIAN_POINT ( 'NONE',  ( 1.115485564304462551, -0.004921259842519576551, 0.3153832671262227771 ) ) ;
#76114=CARTESIAN_POINT ( 'NONE',  ( -0.1968503937007867743, -0.5511811023622047445, 6.969142054262312111E-17 ) ) ;
#76115=CARTESIAN_POINT ( 'NONE',  ( 0.8595800524934390507, -0.2845877964562159024, 0.3641732283464567677 ) ) ;
#76116=CARTESIAN_POINT ( 'NONE',  ( -1.410761154855642463, -0.05778040916215522460, 0.4822834645669289988 ) ) ;
#76118=CARTESIAN_POINT ( 'NONE',  ( 0.6758530183727039509, -0.5511811023622046335, 0.09757992244046803654 ) ) ;
#76119=CARTESIAN_POINT ( 'NONE',  ( -0.7939632545931750718, -0.05778040916215560624, -0.4822834645669293319 ) ) ;
#76120=VECTOR ( 'NONE', #59216, 39.37007874015748143 ) ;
#76121=CARTESIAN_POINT ( 'NONE',  ( 0.02624671916010564918, -0.5023911411419708095, -0.1820866141732282451 ) ) ;
#76122=CARTESIAN_POINT ( 'NONE',  ( -1.607611548556429737, -0.5511811023622046335, 0.09757992244046803654 ) ) ;
#76123=CARTESIAN_POINT ( 'NONE',  ( 0.8202099737532814183, -0.6692913385826773087, -0.1292274648535924053 ) ) ;
#76124=CARTESIAN_POINT ( 'NONE',  ( 0.6561679790026253567, 0.2306618581243848609, 0.2411417322834645549 ) ) ;
#76125=CARTESIAN_POINT ( 'NONE',  ( 1.351706036745407458, -0.3690944881889765550, -0.3153832671262227771 ) ) ;
#76126=CARTESIAN_POINT ( 'NONE',  ( -1.391076115485563758, 0.2306618581243848609, 0.2411417322834645549 ) ) ;
#76127=CARTESIAN_POINT ( 'NONE',  ( -0.2755905511811015396, -0.5511811023622047445, 6.969142054262312111E-17 ) ) ;
#76128=CARTESIAN_POINT ( 'NONE',  ( 2.795275590551181910, 1.900312960331935086, 0.000000000000000000 ) ) ;
#76129=CARTESIAN_POINT ( 'NONE',  ( 0.04593175853018440641, 0.1771653543307087075, -0.09757992244046823083 ) ) ;
#76130=CARTESIAN_POINT ( 'NONE',  ( -1.358267716535432434, 0.1660481256975883668, -0.3530559997133364547 ) ) ;
#76131=CARTESIAN_POINT ( 'NONE',  ( -0.5118110236220466680, 0.2952755905511811885, 0.000000000000000000 ) ) ;
#76136=CARTESIAN_POINT ( 'NONE',  ( 0.4265091863517067039, -0.5511811023622048555, -0.09757992244046775898 ) ) ;
#76137=CARTESIAN_POINT ( 'NONE',  ( -0.5052493438320203589, 0.2952755905511810774, -0.1292274648535930714 ) ) ;
#76138=CARTESIAN_POINT ( 'NONE',  ( -0.7480314960629914633, -0.6692913385826771977, 8.415575281601705876E-17 ) ) ;
#76139=CARTESIAN_POINT ( 'NONE',  ( -0.9120734908136475250, -0.5511811023622048555, -0.09757992244046775898 ) ) ;
#76141=CARTESIAN_POINT ( 'NONE',  ( -0.2559055118110227234, -0.5400638737290844871, 0.3530559997133364547 ) ) ;
#76142=CARTESIAN_POINT ( 'NONE',  ( -1.404199475065615932, -0.004921259842519576551, 0.3153832671262227771 ) ) ;
#76143=CARTESIAN_POINT ( 'NONE',  ( 1.594488188976378673, 0.1660481256975885056, 0.3530559997133364547 ) ) ;
#76146=VERTEX_POINT ( 'NONE', #34098 ) ;
#76148=CARTESIAN_POINT ( 'NONE',  ( -1.318897637795274802, -0.5400638737290845981, -0.3530559997133363437 ) ) ;
#76149=CARTESIAN_POINT ( 'NONE',  ( -0.7874015748031489847, -0.1870078740157479769, 0.4822834645669291653 ) ) ;
#76150=CARTESIAN_POINT ( 'NONE',  ( 1.601049868766404982, 0.2306618581243848609, 0.2411417322834645549 ) ) ;
#76153=CARTESIAN_POINT ( 'NONE',  ( 0.9317585301837276734, 0.05413385826771626580, -0.4176697321401330321 ) ) ;
#76154=CARTESIAN_POINT ( 'NONE',  ( 0.2296587926509192634, -0.3162353388693405765, 0.4822834645669290543 ) ) ;
#76157=VECTOR ( 'NONE', #29338, 39.37007874015748854 ) ;
#76159=AXIS2_PLACEMENT_3D ( 'NONE', #33453, #1472, #65863 ) ;
#76160=CARTESIAN_POINT ( 'NONE',  ( 1.391076115485564868, -0.5023911411419708095, 0.1820866141732285504 ) ) ;
#76165=CARTESIAN_POINT ( 'NONE',  ( 0.5052493438320215802, 0.2952755905511811885, 0.1292274648535926551 ) ) ;
#76166=CARTESIAN_POINT ( 'NONE',  ( -0.7742782152230965886, 0.05413385826771666132, 0.4176697321401328100 ) ) ;
#76167=CARTESIAN_POINT ( 'NONE',  ( 1.614173228346457378, 0.2952755905511811885, 0.000000000000000000 ) ) ;
#76168=CARTESIAN_POINT ( 'NONE',  ( 0.8070866141732289112, -0.5400638737290845981, -0.3530559997133363437 ) ) ;
#76169=CARTESIAN_POINT ( 'NONE',  ( 1.476377952755906442, -0.5400638737290844871, 0.3530559997133364547 ) ) ;
#76170=CARTESIAN_POINT ( 'NONE',  ( 1.246719160104987623, -0.4281496062992124485, 0.4176697321401328655 ) ) ;
#76171=CARTESIAN_POINT ( 'NONE',  ( 0.03937007874015833325, -0.6692913385826771977, 8.415575281601705876E-17 ) ) ;
#76172=CARTESIAN_POINT ( 'NONE',  ( -1.148293963254592542, 0.2952755905511811885, 0.1292274648535926551 ) ) ;
#76173=DIRECTION ( 'NONE',  ( 0.7071067811865472397, -0.000000000000000000, 0.7071067811865476838 ) ) ;
#76174=CARTESIAN_POINT ( 'NONE',  ( 1.686351706036745890, 0.2952755905511811885, 0.1292274648535926551 ) ) ;
#76176=CARTESIAN_POINT ( 'NONE',  ( 1.036745406824147731, -0.004921259842519576551, 0.3153832671262227771 ) ) ;
#76180=CARTESIAN_POINT ( 'NONE',  ( -0.05905511811023545637, -0.4536011799217368745, -0.2665933059059886201 ) ) ;
#76182=CARTESIAN_POINT ( 'NONE',  ( 0.4593175853018379162, -0.4281496062992124485, 0.4176697321401328655 ) ) ;
#76183=CARTESIAN_POINT ( 'NONE',  ( 0.2296587926509192634, -0.05778040916215560624, -0.4822834645669293319 ) ) ;
#76184=CARTESIAN_POINT ( 'NONE',  ( -0.5380577427821514602, -0.4281496062992127816, -0.4176697321401328100 ) ) ;
#76186=CARTESIAN_POINT ( 'NONE',  ( -1.102362204724408601, -0.1870078740157480879, -0.4822834645669291653 ) ) ;
#76188=CARTESIAN_POINT ( 'NONE',  ( 1.135170603674541256, 0.1771653543307087630, 0.09757992244046791164 ) ) ;
#76189=CARTESIAN_POINT ( 'NONE',  ( -1.568241469816272105, -0.3162353388693409650, -0.4822834645669289433 ) ) ;
#76190=CARTESIAN_POINT ( 'NONE',  ( 0.7808398950131241190, -0.05778040916215560624, -0.4822834645669293319 ) ) ;
#76191=CARTESIAN_POINT ( 'NONE',  ( 1.272965879265092637, -0.4281496062992127816, -0.4176697321401328100 ) ) ;
#76193=CARTESIAN_POINT ( 'NONE',  ( -1.364829396325458521, 0.2306618581243847221, -0.2411417322834647770 ) ) ;
#76195=CARTESIAN_POINT ( 'NONE',  ( 0.02624671916010564918, 0.2306618581243848609, 0.2411417322834645549 ) ) ;
#76199=CARTESIAN_POINT ( 'NONE',  ( 1.272965879265092637, -0.4281496062992127816, -0.4176697321401328100 ) ) ;
#76200=CARTESIAN_POINT ( 'NONE',  ( 0.04593175853018440641, -0.5511811023622046335, 0.09757992244046803654 ) ) ;
#76201=CARTESIAN_POINT ( 'NONE',  ( 0.7414698162729663755, -0.6692913385826773087, -0.1292274648535924053 ) ) ;
#76203=CARTESIAN_POINT ( 'NONE',  ( 0.1706036745406830368, -0.3690944881889765550, -0.3153832671262227771 ) ) ;
#76204=CARTESIAN_POINT ( 'NONE',  ( 0.4527559055118117182, -0.5400638737290844871, 0.3530559997133364547 ) ) ;
#76207=CARTESIAN_POINT ( 'NONE',  ( -0.7742782152230965886, 0.05413385826771666132, 0.4176697321401328100 ) ) ;
#76209=CARTESIAN_POINT ( 'NONE',  ( 0.7480314960629927956, -0.5511811023622047445, 6.969142054262312111E-17 ) ) ;
#76210=CARTESIAN_POINT ( 'NONE',  ( 0.1450607720586929161, 2.784432375088962958E-17, -0.3464511005275205946 ) ) ;
#76211=CARTESIAN_POINT ( 'NONE',  ( -0.2690288713910754526, 0.2952755905511810774, -0.1292274648535930714 ) ) ;
#76212=CARTESIAN_POINT ( 'NONE',  ( 0.2887139107611556010, 0.1283753931104746893, -0.1820866141732285504 ) ) ;
#76214=CARTESIAN_POINT ( 'NONE',  ( -0.1443569553805768291, 0.05413385826771666132, 0.4176697321401328100 ) ) ;
#76215=CARTESIAN_POINT ( 'NONE',  ( 0.3412073490813655186, 0.1283753931104748280, 0.1820866141732283561 ) ) ;
#76218=CARTESIAN_POINT ( 'NONE',  ( 0.3608923884514443348, -0.6692913385826771977, 0.1292274648535927661 ) ) ;
#76219=( BOUNDED_CURVE ( )  B_SPLINE_CURVE ( 2, ( #20498, #57526, #39004, #7452, #1150, #27216, #12934, #46152, #52878, #64271, #45312, #51616, #77746 ),
 .UNSPECIFIED., .F., .F. ) 
 B_SPLINE_CURVE_WITH_KNOTS ( ( 3, 2, 2, 2, 2, 2, 3 ),
 ( 0.7187856400893463116, 0.7196969696969697239, 0.7234848484848485084, 0.7272727272727272929, 0.7310606060606060774, 0.7348484848484848619, 0.7357598144561083853 ),
 .UNSPECIFIED. ) 
 CURVE ( )  GEOMETRIC_REPRESENTATION_ITEM ( )  RATIONAL_B_SPLINE_CURVE ( ( 0.9875488213027523443, 0.9918020599134680371, 1.000000000000000000, 0.9659258262890683122, 1.000000000000000000, 0.9659258262890683122, 1.000000000000000000, 0.9659258262890683122, 1.000000000000000000, 0.9659258262890683122, 1.000000000000000000, 0.9918020599134671489, 0.9875488213027514561 ) ) 
 REPRESENTATION_ITEM ( '' )  );
#76221=AXIS2_PLACEMENT_3D ( 'NONE', #63234, #69959, #31240 ) ;
#76223=CARTESIAN_POINT ( 'NONE',  ( 0.9908136482939640111, -0.5511811023622046335, 0.09757992244046803654 ) ) ;
#76224=CARTESIAN_POINT ( 'NONE',  ( -0.4199475065616791736, 0.1283753931104746893, -0.1820866141732285504 ) ) ;
#76225=CARTESIAN_POINT ( 'NONE',  ( -0.5511811023622041894, -0.1870078740157480601, -0.3641732283464567677 ) ) ;
#76226=CARTESIAN_POINT ( 'NONE',  ( -0.4724409448818890911, -0.1870078740157480879, -0.4822834645669291653 ) ) ;
#76227=CARTESIAN_POINT ( 'NONE',  ( 0.3083989501312343062, -0.3162353388693405765, 0.4822834645669290543 ) ) ;
#76228=CARTESIAN_POINT ( 'NONE',  ( 1.167979002624672580, -0.3690944881889763329, 0.3153832671262228327 ) ) ;
#76229=CARTESIAN_POINT ( 'NONE',  ( -1.607611548556429737, -0.5511811023622046335, 0.09757992244046803654 ) ) ;
#76230=CARTESIAN_POINT ( 'NONE',  ( 1.410761154855643795, -0.2845877964562159024, 0.3641732283464567677 ) ) ;
#76231=CARTESIAN_POINT ( 'NONE',  ( 0.9120734908136490793, 0.2952755905511810774, -0.1292274648535930714 ) ) ;
#76233=CARTESIAN_POINT ( 'NONE',  ( -0.1443569553805768291, 0.05413385826771666132, 0.4176697321401328100 ) ) ;
#76235=CARTESIAN_POINT ( 'NONE',  ( 0.7020997375328090762, -0.3162353388693405765, 0.4822834645669290543 ) ) ;
#76236=CARTESIAN_POINT ( 'NONE',  ( 0.6364829396325465405, -0.3162353388693409650, -0.4822834645669289433 ) ) ;
#76238=CARTESIAN_POINT ( 'NONE',  ( 0.3280839895013130669, -0.3690944881889765550, -0.3153832671262227771 ) ) ;
#76239=CARTESIAN_POINT ( 'NONE',  ( 1.043307086614173818, 0.1660481256975885056, 0.3530559997133364547 ) ) ;
#76240=CARTESIAN_POINT ( 'NONE',  ( -0.3674540682414692561, -0.5023911411419708095, -0.1820866141732282451 ) ) ;
#76241=CARTESIAN_POINT ( 'NONE',  ( -0.4986876640419939388, 0.2306618581243847221, -0.2411417322834647770 ) ) ;
#76243=CARTESIAN_POINT ( 'NONE',  ( 0.2296587926509192634, -0.05778040916215560624, -0.4822834645669293319 ) ) ;
#76244=CARTESIAN_POINT ( 'NONE',  ( -0.6692913385826764205, 0.2952755905511811885, 0.000000000000000000 ) ) ;
#76245=CARTESIAN_POINT ( 'NONE',  ( -0.5511811023622041894, -0.1870078740157480601, -0.3641732283464567677 ) ) ;
#76246=CARTESIAN_POINT ( 'NONE',  ( 0.4658792650918640033, -0.3162353388693405765, 0.4822834645669290543 ) ) ;
#76247=CARTESIAN_POINT ( 'NONE',  ( -1.259842519685038686, -0.1870078740157479769, 0.4822834645669291653 ) ) ;
#76248=CARTESIAN_POINT ( 'NONE',  ( -0.5249343832020990641, 0.2306618581243848609, 0.2411417322834645549 ) ) ;
#76250=CARTESIAN_POINT ( 'NONE',  ( -0.9348729704079935532, -2.191421614605370878E-15, 0.4445507791589071167 ) ) ;
#76251=CARTESIAN_POINT ( 'NONE',  ( 1.332020997375328974, -0.05778040916215560624, -0.4822834645669293319 ) ) ;
#76252=CARTESIAN_POINT ( 'NONE',  ( 1.522309711286089939, 0.2306618581243848609, 0.2411417322834645549 ) ) ;
#76254=CARTESIAN_POINT ( 'NONE',  ( -1.450131233595799651, 0.2952755905511810774, -0.1292274648535930714 ) ) ;
#76255=CARTESIAN_POINT ( 'NONE',  ( -0.8267716535433065062, -0.6692913385826771977, 8.415575281601705876E-17 ) ) ;
#76258=ORIENTED_EDGE ( 'NONE', *, *, #8336, .F. ) ;
#76259=CARTESIAN_POINT ( 'NONE',  ( 0.1574803149606306130, -0.1870078740157480601, -0.3641732283464567677 ) ) ;
#76261=CARTESIAN_POINT ( 'NONE',  ( 0.5446194225721792126, -0.05778040916215560624, -0.4822834645669293319 ) ) ;
#76264=CARTESIAN_POINT ( 'NONE',  ( -0.6299212598425188991, -0.1870078740157480601, -0.3641732283464567677 ) ) ;
#76265=CARTESIAN_POINT ( 'NONE',  ( -0.2493438320209966919, 0.05413385826771626580, -0.4176697321401330321 ) ) ;
#76266=CARTESIAN_POINT ( 'NONE',  ( 1.128608923884515169, -0.6046776061558809534, -0.2411417322834644161 ) ) ;
#76268=CARTESIAN_POINT ( 'NONE',  ( 1.095800524934383846, -0.2845877964562159024, 0.3641732283464567677 ) ) ;
#76269=CARTESIAN_POINT ( 'NONE',  ( -0.1640419947506553400, -0.05778040916215560624, -0.4822834645669293319 ) ) ;
#76271=CARTESIAN_POINT ( 'NONE',  ( -0.6102362204724400829, -0.5400638737290845981, -0.3530559997133363437 ) ) ;
#76272=CARTESIAN_POINT ( 'NONE',  ( -1.364829396325458521, 0.1283753931104746893, -0.1820866141732285504 ) ) ;
#76273=CARTESIAN_POINT ( 'NONE',  ( -0.2755905511811018171, 0.2952755905511811885, 0.000000000000000000 ) ) ;
#76274=EDGE_CURVE ( 'NONE', #23151, #59949, #30397, .T. ) ;
#76280=CARTESIAN_POINT ( 'NONE',  ( 0.3280839895013130669, -0.4281496062992127816, -0.4176697321401328100 ) ) ;
#76282=AXIS2_PLACEMENT_3D ( 'NONE', #47447, #3679, #54593 ) ;
#76283=CARTESIAN_POINT ( 'NONE',  ( -0.9317585301837263412, 0.05413385826771666132, 0.4176697321401328100 ) ) ;
#76284=CARTESIAN_POINT ( 'NONE',  ( -1.456692913385826182, 0.2952755905511811885, 0.000000000000000000 ) ) ;
#76285=CARTESIAN_POINT ( 'NONE',  ( 0.5577427821522314977, -0.3162353388693409650, -0.4822834645669289433 ) ) ;
#76286=CARTESIAN_POINT ( 'NONE',  ( -0.01312335958005186876, 0.05413385826771626580, -0.4176697321401330321 ) ) ;
#76288=CARTESIAN_POINT ( 'NONE',  ( -0.8333333333333323711, -0.6692913385826773087, -0.1292274648535924053 ) ) ;
#76289=CARTESIAN_POINT ( 'NONE',  ( -0.2559055118110227234, -0.5400638737290844871, 0.3530559997133364547 ) ) ;
#76290=CARTESIAN_POINT ( 'NONE',  ( -1.010498687664041384, 0.05413385826771666132, 0.4176697321401328100 ) ) ;
#76291=CARTESIAN_POINT ( 'NONE',  ( 0.4790026246719168435, -0.2845877964562161244, -0.3641732283464567121 ) ) ;
#76293=CARTESIAN_POINT ( 'NONE',  ( 0.09842519685039434474, -0.5400638737290845981, -0.3530559997133363437 ) ) ;
#76296=CARTESIAN_POINT ( 'NONE',  ( 1.108923884514436242, -0.05778040916215522460, 0.4822834645669289988 ) ) ;
#76299=EDGE_CURVE ( 'NONE', #71856, #59949, #47219, .T. ) ;
#76301=CARTESIAN_POINT ( 'NONE',  ( 0.2230971128608932319, -0.4281496062992124485, 0.4176697321401328655 ) ) ;
#76302=CARTESIAN_POINT ( 'NONE',  ( -0.07874015748031421014, -0.1870078740157480601, -0.3641732283464567677 ) ) ;
#76303=CARTESIAN_POINT ( 'NONE',  ( 1.548556430446194954, 0.1283753931104746893, -0.1820866141732285504 ) ) ;
#76308=CARTESIAN_POINT ( 'NONE',  ( 0.6102362204724416372, -0.5400638737290844871, 0.3530559997133364547 ) ) ;
#76309=CARTESIAN_POINT ( 'NONE',  ( -1.240157480314959759, -0.5400638737290845981, -0.3530559997133363437 ) ) ;
#76310=CARTESIAN_POINT ( 'NONE',  ( -0.9842519685039365918, -0.6692913385826771977, 8.415575281601705876E-17 ) ) ;
#76311=CARTESIAN_POINT ( 'NONE',  ( 0.4265091863517067039, -0.6692913385826773087, -0.1292274648535924053 ) ) ;
#76312=CARTESIAN_POINT ( 'NONE',  ( 0.8070866141732288002, 0.1660481256975885056, 0.3530559997133364547 ) ) ;
#76313=CARTESIAN_POINT ( 'NONE',  ( 1.364829396325460076, 0.1283753931104748280, 0.1820866141732283561 ) ) ;
#76315=CARTESIAN_POINT ( 'NONE',  ( 0.9120734908136490793, 0.1771653543307087075, -0.09757992244046823083 ) ) ;
#76316=CARTESIAN_POINT ( 'NONE',  ( -0.8136482939632537770, 0.2306618581243847221, -0.2411417322834647770 ) ) ;
#76318=CARTESIAN_POINT ( 'NONE',  ( 1.679790026246720025, 0.2306618581243848609, 0.2411417322834645549 ) ) ;
#76320=CARTESIAN_POINT ( 'NONE',  ( 1.286089238845145033, -0.6046776061558809534, -0.2411417322834644161 ) ) ;
#76321=CARTESIAN_POINT ( 'NONE',  ( 1.595398199321655275, 0.7585570207896586981, -0.1559797534342493852 ) ) ;
#76322=CARTESIAN_POINT ( 'NONE',  ( -1.535433070866141225, 0.1771653543307087630, 0.000000000000000000 ) ) ;
#76323=CARTESIAN_POINT ( 'NONE',  ( -0.02624671916010428221, 0.2306618581243847221, -0.2411417322834647770 ) ) ;
#76324=CARTESIAN_POINT ( 'NONE',  ( 0.6889763779527563470, 0.07958543189024071263, -0.2665933059059888421 ) ) ;
#76325=CARTESIAN_POINT ( 'NONE',  ( -1.712598425196849572, 0.07958543189024085140, 0.2665933059059887866 ) ) ;
#76326=CARTESIAN_POINT ( 'NONE',  ( 0.9383202099737538715, -0.05778040916215560624, -0.4822834645669293319 ) ) ;
#76328=CARTESIAN_POINT ( 'NONE',  ( -0.4790026246719154557, -0.2845877964562159024, 0.3641732283464567677 ) ) ;
#76329=CARTESIAN_POINT ( 'NONE',  ( -0.4461942257217840213, 0.2306618581243848609, 0.2411417322834645549 ) ) ;
#76330=CARTESIAN_POINT ( 'NONE',  ( 1.391076115485564868, 0.2306618581243847221, -0.2411417322834647770 ) ) ;
#76331=CARTESIAN_POINT ( 'NONE',  ( -0.9776902887139098386, -0.6692913385826771977, 0.1292274648535927661 ) ) ;
#76332=CARTESIAN_POINT ( 'NONE',  ( 1.259842519685040019, -0.1870078740157480879, -0.4822834645669291653 ) ) ;
#76334=CARTESIAN_POINT ( 'NONE',  ( -1.318897637795274802, 0.07958543189024085140, 0.2665933059059887866 ) ) ;
#76335=CARTESIAN_POINT ( 'NONE',  ( -0.7426113562969628434, 2.209901789876557832, 0.5309055118110236338 ) ) ;
#76336=CARTESIAN_POINT ( 'NONE',  ( 0.9908136482939640111, 0.2952755905511810774, -0.1292274648535930714 ) ) ;
#76338=CARTESIAN_POINT ( 'NONE',  ( -1.679790026246718693, 0.2306618581243847221, -0.2411417322834647770 ) ) ;
#76339=CARTESIAN_POINT ( 'NONE',  ( -1.377952755905511140, -0.5511811023622047445, 6.969142054262312111E-17 ) ) ;
#76340=CARTESIAN_POINT ( 'NONE',  ( -0.8530183727034112984, -0.3690944881889765550, -0.3153832671262227771 ) ) ;
#76341=CARTESIAN_POINT ( 'NONE',  ( 1.437007874015748810, -0.4536011799217368745, -0.2665933059059886201 ) ) ;
#76342=CARTESIAN_POINT ( 'NONE',  ( -0.4133858267716528645, -0.5400638737290844871, 0.3530559997133364547 ) ) ;
#76343=CARTESIAN_POINT ( 'NONE',  ( -0.1181102362204717315, -0.5511811023622047445, 6.969142054262312111E-17 ) ) ;
#76344=CARTESIAN_POINT ( 'NONE',  ( -1.509186351706035767, -0.004921259842519870586, -0.3153832671262229437 ) ) ;
#76345=CARTESIAN_POINT ( 'NONE',  ( 1.062992125984252745, -0.5511811023622047445, 6.969142054262312111E-17 ) ) ;
#76346=CARTESIAN_POINT ( 'NONE',  ( 0.8858267716535438430, 0.1660481256975885056, 0.3530559997133364547 ) ) ;
#76348=CARTESIAN_POINT ( 'NONE',  ( -0.07217847769028787330, -0.08942795157527998196, 0.3641732283464567121 ) ) ;
#76349=CARTESIAN_POINT ( 'NONE',  ( 0.3740157480314966754, -0.5400638737290844871, 0.3530559997133364547 ) ) ;
#76350=CARTESIAN_POINT ( 'NONE',  ( 0.4068241469816279987, -0.3690944881889765550, -0.3153832671262227771 ) ) ;
#76352=CARTESIAN_POINT ( 'NONE',  ( -1.528871391076114250, -0.6692913385826771977, 0.1292274648535927661 ) ) ;
#76353=ADVANCED_FACE ( 'NONE', ( #42062 ), #35346, .T. ) ;
#76354=CARTESIAN_POINT ( 'NONE',  ( -1.108923884514435132, -0.05778040916215560624, -0.4822834645669293319 ) ) ;
#76355=CARTESIAN_POINT ( 'NONE',  ( 0.09186351706036799403, -0.4281496062992127816, -0.4176697321401328100 ) ) ;
#76358=CARTESIAN_POINT ( 'NONE',  ( 0.5118110236220478892, 0.2952755905511811885, 0.000000000000000000 ) ) ;
#76359=CARTESIAN_POINT ( 'NONE',  ( 1.305774278215223960, 0.1771653543307087075, -0.09757992244046823083 ) ) ;
#76360=CARTESIAN_POINT ( 'NONE',  ( -0.1968503937007867743, 0.2952755905511811885, 0.000000000000000000 ) ) ;
#76361=CARTESIAN_POINT ( 'NONE',  ( 0.1968503937007881344, 0.2952755905511811885, 0.000000000000000000 ) ) ;
#76367=CARTESIAN_POINT ( 'NONE',  ( -0.7152230971128602510, -0.08942795157528024563, -0.3641732283464568787 ) ) ;
#76368=CARTESIAN_POINT ( 'NONE',  ( -1.023622047244094002, -0.1870078740157480879, -0.4822834645669291653 ) ) ;
#76370=CARTESIAN_POINT ( 'NONE',  ( 0.6758530183727039509, -0.6692913385826771977, 0.1292274648535927661 ) ) ;
#76371=CARTESIAN_POINT ( 'NONE',  ( -1.620734908136482577, 0.2952755905511811885, 0.1292274648535926551 ) ) ;
#76372=CARTESIAN_POINT ( 'NONE',  ( 0.5905511811023629321, -0.6692913385826771977, 8.415575281601705876E-17 ) ) ;
#76373=CARTESIAN_POINT ( 'NONE',  ( -0.6199123404867337150, -2.191421614605370878E-15, 0.4445507791589071167 ) ) ;
#76375=CARTESIAN_POINT ( 'NONE',  ( 1.679790026246720025, 0.2306618581243848609, 0.2411417322834645549 ) ) ;
#76376=CARTESIAN_POINT ( 'NONE',  ( 0.9908136482939640111, 0.2952755905511810774, -0.1292274648535930714 ) ) ;
#76377=CARTESIAN_POINT ( 'NONE',  ( 0.5577427821522314977, -0.3162353388693409650, -0.4822834645669289433 ) ) ;
#76378=CARTESIAN_POINT ( 'NONE',  ( 0.7677165354330716118, -0.4536011799217367080, 0.2665933059059888421 ) ) ;
#76379=CARTESIAN_POINT ( 'NONE',  ( 1.305774278215223960, -0.6692913385826771977, 0.1292274648535927661 ) ) ;
#76381=CARTESIAN_POINT ( 'NONE',  ( -1.595398199321655275, 2.115458727241839476, 0.1559797534342494407 ) ) ;
#76382=CARTESIAN_POINT ( 'NONE',  ( 0.6692913385826778638, -0.6692913385826771977, 8.415575281601705876E-17 ) ) ;
#76383=CARTESIAN_POINT ( 'NONE',  ( 1.423884514435696413, -0.2845877964562161244, -0.3641732283464567121 ) ) ;
#76384=CARTESIAN_POINT ( 'NONE',  ( -0.8530183727034112984, -0.4281496062992127816, -0.4176697321401328100 ) ) ;
#76385=CARTESIAN_POINT ( 'NONE',  ( -1.141732283464566011, -0.6692913385826771977, 8.415575281601705876E-17 ) ) ;
#76386=CARTESIAN_POINT ( 'NONE',  ( 1.299212598425197429, 0.2952755905511811885, 0.000000000000000000 ) ) ;
#76390=ORIENTED_EDGE ( 'NONE', *, *, #25562, .F. ) ;
#76393=CARTESIAN_POINT ( 'NONE',  ( 1.620734908136483465, -0.6692913385826771977, 0.1292274648535927661 ) ) ;
#76394=AXIS2_PLACEMENT_3D ( 'NONE', #14257, #39915, #65604 ) ;
#76395=CARTESIAN_POINT ( 'NONE',  ( 1.384514435695538337, -0.5511811023622046335, 0.09757992244046803654 ) ) ;
#76397=CARTESIAN_POINT ( 'NONE',  ( 1.292650918635171564, -0.5511811023622048555, -0.09757992244046775898 ) ) ;
#76402=CARTESIAN_POINT ( 'NONE',  ( -0.5643044619422565855, -0.3690944881889763329, 0.3153832671262228327 ) ) ;
#76403=CARTESIAN_POINT ( 'NONE',  ( -1.614173228346456268, -0.5511811023622047445, 6.969142054262312111E-17 ) ) ;
#76405=CARTESIAN_POINT ( 'NONE',  ( -1.345144356955379816, -0.3162353388693405765, 0.4822834645669290543 ) ) ;
#76406=CARTESIAN_POINT ( 'NONE',  ( -0.07874015748031421014, -0.1870078740157480879, -0.4822834645669291653 ) ) ;
#76407=CARTESIAN_POINT ( 'NONE',  ( 1.377952755905512472, -0.6692913385826771977, 8.415575281601705876E-17 ) ) ;
#76413=CARTESIAN_POINT ( 'NONE',  ( -0.3280839895013117347, -0.004921259842519870586, -0.3153832671262229437 ) ) ;
#76414=CARTESIAN_POINT ( 'NONE',  ( -1.154855643044618851, 0.2306618581243848609, 0.2411417322834645549 ) ) ;
#76415=CARTESIAN_POINT ( 'NONE',  ( 1.154855643044620184, -0.6046776061558807314, 0.2411417322834647770 ) ) ;
#76420=CARTESIAN_POINT ( 'NONE',  ( 1.299212598425197429, -0.6692913385826771977, 8.415575281601705876E-17 ) ) ;
#76421=CARTESIAN_POINT ( 'NONE',  ( -1.364829396325458521, 0.2306618581243847221, -0.2411417322834647770 ) ) ;
#76423=CARTESIAN_POINT ( 'NONE',  ( -0.3543307086614165824, -0.5511811023622047445, 6.969142054262312111E-17 ) ) ;
#76426=CARTESIAN_POINT ( 'NONE',  ( -0.5577427821522301654, -0.2845877964562159024, 0.3641732283464567677 ) ) ;
#76427=CARTESIAN_POINT ( 'NONE',  ( 0.5774278215223103139, -0.5023911411419708095, -0.1820866141732282451 ) ) ;
#76428=CARTESIAN_POINT ( 'NONE',  ( 0.2559055118110243332, -0.5400638737290845981, -0.3530559997133363437 ) ) ;
#76429=CARTESIAN_POINT ( 'NONE',  ( -0.6364829396325453192, -0.08942795157528024563, -0.3641732283464568787 ) ) ;
#76431=CARTESIAN_POINT ( 'NONE',  ( 1.200787401574803681, -0.5400638737290845981, -0.3530559997133363437 ) ) ;
#76432=CARTESIAN_POINT ( 'NONE',  ( -1.443569553805773564, 0.2306618581243847221, -0.2411417322834647770 ) ) ;
#76434=CARTESIAN_POINT ( 'NONE',  ( -0.5577427821522301654, -0.05778040916215560624, -0.4822834645669293319 ) ) ;
#76435=CARTESIAN_POINT ( 'NONE',  ( -0.9448818897637790704, -0.1870078740157480879, -0.4822834645669291653 ) ) ;
#76436=CARTESIAN_POINT ( 'NONE',  ( 1.318897637795276356, -0.4536011799217367080, 0.2665933059059888421 ) ) ;
#76437=CARTESIAN_POINT ( 'NONE',  ( -0.4724409448818890911, -0.1870078740157479769, 0.3641732283464567677 ) ) ;
#76438=CARTESIAN_POINT ( 'NONE',  ( -0.7086614173228339419, -0.1870078740157480879, -0.4822834645669291653 ) ) ;
#76439=CARTESIAN_POINT ( 'NONE',  ( -1.286089238845143479, 0.2306618581243847221, -0.2411417322834647770 ) ) ;
#76441=CARTESIAN_POINT ( 'NONE',  ( 1.397637795275591177, 0.07958543189024071263, -0.2665933059059888421 ) ) ;
#76442=CARTESIAN_POINT ( 'NONE',  ( -0.4396325459317577122, -0.6692913385826773087, -0.1292274648535924053 ) ) ;
#76443=CARTESIAN_POINT ( 'NONE',  ( -1.049868766404198794, 0.2306618581243847221, -0.2411417322834647770 ) ) ;
#76444=EDGE_LOOP ( 'NONE', ( #24519, #11497, #26057, #1964 ) ) ;
#76448=CARTESIAN_POINT ( 'NONE',  ( -0.7611548556430438595, -0.5023911411419708095, -0.1820866141732282451 ) ) ;
#76449=CARTESIAN_POINT ( 'NONE',  ( 1.292650918635171564, 0.2952755905511811885, 0.1292274648535926551 ) ) ;
#76450=CARTESIAN_POINT ( 'NONE',  ( -0.9186351706036736120, 0.1283753931104748280, 0.1820866141732283561 ) ) ;
#76452=CARTESIAN_POINT ( 'NONE',  ( -0.9580052493438311334, -0.4281496062992124485, 0.4176697321401328655 ) ) ;
#76453=CARTESIAN_POINT ( 'NONE',  ( 1.351706036745407680, 0.05413385826771666132, 0.4176697321401328100 ) ) ;
#76454=CARTESIAN_POINT ( 'NONE',  ( 0.7020997375328090762, -0.3162353388693405765, 0.4822834645669290543 ) ) ;
#76455=CARTESIAN_POINT ( 'NONE',  ( 1.548556430446194954, -0.6046776061558807314, 0.2411417322834647770 ) ) ;
#76456=CARTESIAN_POINT ( 'NONE',  ( -1.587926509186350810, -0.3690944881889763329, 0.3153832671262228327 ) ) ;
#76459=EDGE_CURVE ( 'NONE', #1651, #74449, #9071, .T. ) ;
#76462=CARTESIAN_POINT ( 'NONE',  ( 1.338582677165355062, -0.1870078740157479769, 0.3641732283464567677 ) ) ;
#76463=CARTESIAN_POINT ( 'NONE',  ( 0.7480314960629927956, -0.5511811023622047445, 6.969142054262312111E-17 ) ) ;
#76464=CARTESIAN_POINT ( 'NONE',  ( 0.6496062992125991586, 0.1660481256975885056, 0.3530559997133364547 ) ) ;
#76465=CARTESIAN_POINT ( 'NONE',  ( 1.515748031496063186, -0.5400638737290845981, -0.3530559997133363437 ) ) ;
#76467=CARTESIAN_POINT ( 'NONE',  ( 0.7874015748031503170, -0.1870078740157480601, -0.3641732283464567677 ) ) ;
#76468=CARTESIAN_POINT ( 'NONE',  ( -0.3740157480314953431, 0.1660481256975885056, 0.3530559997133364547 ) ) ;
#76469=CARTESIAN_POINT ( 'NONE',  ( -1.259842519685038686, -0.1870078740157480879, -0.4822834645669291653 ) ) ;
#76470=CARTESIAN_POINT ( 'NONE',  ( 1.003937007874016407, -0.5400638737290844871, 0.3530559997133364547 ) ) ;
#76475=CARTESIAN_POINT ( 'NONE',  ( -1.122047244094487306, -0.5400638737290844871, 0.3530559997133364547 ) ) ;
#76476=CARTESIAN_POINT ( 'NONE',  ( -0.6955380577427815458, 0.05413385826771666132, 0.4176697321401328100 ) ) ;
#76477=CARTESIAN_POINT ( 'NONE',  ( -0.9711286089238838626, 0.1283753931104746893, -0.1820866141732285504 ) ) ;
#76478=CARTESIAN_POINT ( 'NONE',  ( -0.6627296587926501115, 0.2952755905511810774, -0.1292274648535930714 ) ) ;
#76480=CARTESIAN_POINT ( 'NONE',  ( 0.2427821522309719648, -0.05778040916215522460, 0.4822834645669289988 ) ) ;
#76481=CARTESIAN_POINT ( 'NONE',  ( -0.5643044619422565855, -0.4281496062992124485, 0.4176697321401328655 ) ) ;
#76482=CARTESIAN_POINT ( 'NONE',  ( 1.502624671916010790, -0.3162353388693409650, -0.4822834645669289433 ) ) ;
#76483=CARTESIAN_POINT ( 'NONE',  ( -0.8858267716535425107, 0.1660481256975883668, -0.3530559997133364547 ) ) ;
#76484=CARTESIAN_POINT ( 'NONE',  ( 0.6102362204724416372, -0.5400638737290844871, 0.3530559997133364547 ) ) ;
#76486=CARTESIAN_POINT ( 'NONE',  ( -0.9055118110236215490, -0.5511811023622047445, 6.969142054262312111E-17 ) ) ;
#76487=ORIENTED_EDGE ( 'NONE', *, *, #58647, .F. ) ;
#76490=CARTESIAN_POINT ( 'NONE',  ( -1.417322834645668772, -0.1870078740157479769, 0.3641732283464567677 ) ) ;
#76491=CARTESIAN_POINT ( 'NONE',  ( -1.259842519685038686, -0.1870078740157480879, -0.4822834645669291653 ) ) ;
#76492=CARTESIAN_POINT ( 'NONE',  ( -0.7874015748031489847, -0.1870078740157480879, -0.4822834645669291653 ) ) ;
#76494=CARTESIAN_POINT ( 'NONE',  ( -0.9973753280839886548, -0.6046776061558809534, -0.2411417322834644161 ) ) ;
#76495=CARTESIAN_POINT ( 'NONE',  ( -1.371391076115484831, 0.2952755905511810774, -0.1292274648535930714 ) ) ;
#76497=CARTESIAN_POINT ( 'NONE',  ( -1.699475065616797398, 0.2952755905511811885, 0.1292274648535926551 ) ) ;
#76498=CARTESIAN_POINT ( 'NONE',  ( 0.4330708661417329575, 0.1771653543307087630, 0.000000000000000000 ) ) ;
#76499=CARTESIAN_POINT ( 'NONE',  ( -1.646051170424378096, 0.000000000000000000, -0.3464511005275205946 ) ) ;
#76501=CARTESIAN_POINT ( 'NONE',  ( -0.2230971128608915943, -0.3690944881889765550, -0.3153832671262227771 ) ) ;
#76502=CARTESIAN_POINT ( 'NONE',  ( -0.2296587926509179312, -0.05778040916215522460, 0.4822834645669289988 ) ) ;
#76503=CARTESIAN_POINT ( 'NONE',  ( 1.272965879265092637, 0.05413385826771666132, 0.4176697321401328100 ) ) ;
#76504=CARTESIAN_POINT ( 'NONE',  ( -0.4002624671916004129, -0.3162353388693405765, 0.4822834645669290543 ) ) ;
#76508=CARTESIAN_POINT ( 'NONE',  ( -0.4855643044619415427, 0.05413385826771626580, -0.4176697321401330321 ) ) ;
#76509=CARTESIAN_POINT ( 'NONE',  ( 1.496062992125984703, -0.1870078740157480879, -0.4822834645669291653 ) ) ;
#76510=CARTESIAN_POINT ( 'NONE',  ( -0.9973753280839886548, -0.5023911411419708095, -0.1820866141732282451 ) ) ;
#76511=CARTESIAN_POINT ( 'NONE',  ( -1.509186351706035767, 0.05413385826771626580, -0.4176697321401330321 ) ) ;
#76513=CARTESIAN_POINT ( 'NONE',  ( -0.7330049731600565277, 2.188112158501061444, 0.5178675056770625229 ) ) ;
#76515=CARTESIAN_POINT ( 'NONE',  ( 1.200787401574803681, 0.1660481256975885056, 0.3530559997133364547 ) ) ;
#76517=CARTESIAN_POINT ( 'NONE',  ( 8.195543980992789655E-16, -0.1870078740157480879, -0.4822834645669291653 ) ) ;
#76518=CARTESIAN_POINT ( 'NONE',  ( -1.200787401574802349, -0.4536011799217367080, 0.2665933059059888421 ) ) ;
#76519=CARTESIAN_POINT ( 'NONE',  ( -0.2821522309711278487, 0.2952755905511811885, 0.1292274648535926551 ) ) ;
#76521=CARTESIAN_POINT ( 'NONE',  ( -0.9120734908136475250, 0.2952755905511811885, 0.1292274648535926551 ) ) ;
#76522=ADVANCED_FACE ( 'NONE', ( #5416 ), #44113, .F. ) ;
#76523=CARTESIAN_POINT ( 'NONE',  ( -1.194225721784776262, 0.05413385826771626580, -0.4176697321401330321 ) ) ;
#76525=CARTESIAN_POINT ( 'NONE',  ( 1.056430446194226436, -0.5511811023622048555, -0.09757992244046775898 ) ) ;
#76526=CARTESIAN_POINT ( 'NONE',  ( -0.4199475065616791736, 0.1283753931104746893, -0.1820866141732285504 ) ) ;
#76527=CARTESIAN_POINT ( 'NONE',  ( 0.6627296587926517768, -0.5511811023622048555, -0.09757992244046775898 ) ) ;
#76528=CARTESIAN_POINT ( 'NONE',  ( -1.561679790026246017, 0.05413385826771666132, 0.4176697321401328100 ) ) ;
#76529=CARTESIAN_POINT ( 'NONE',  ( 1.581364829396326277, -0.05778040916215522460, 0.4822834645669289988 ) ) ;
#76530=CARTESIAN_POINT ( 'NONE',  ( 0.4330708661417329575, 0.1771653543307087630, 0.000000000000000000 ) ) ;
#76531=CARTESIAN_POINT ( 'NONE',  ( -0.8595800524934373854, -0.05778040916215522460, 0.4822834645669289988 ) ) ;
#76532=CARTESIAN_POINT ( 'NONE',  ( 1.200787401574803681, -0.5400638737290845981, -0.3530559997133363437 ) ) ;
#76534=CARTESIAN_POINT ( 'NONE',  ( -0.1181102362204717315, -0.5511811023622047445, 6.969142054262312111E-17 ) ) ;
#76536=CARTESIAN_POINT ( 'NONE',  ( 0.1443569553805781891, 0.05413385826771626580, -0.4176697321401330321 ) ) ;
#76538=CARTESIAN_POINT ( 'NONE',  ( 1.450131233595801428, 0.1771653543307087630, 0.09757992244046791164 ) ) ;
#76539=CARTESIAN_POINT ( 'NONE',  ( 0.01968503937007930540, 0.07958543189024085140, 0.2665933059059887866 ) ) ;
#76540=CARTESIAN_POINT ( 'NONE',  ( -1.345144356955379816, -0.05778040916215560624, -0.4822834645669293319 ) ) ;
#76541=CARTESIAN_POINT ( 'NONE',  ( -0.7020997375328074108, -0.08942795157527998196, 0.3641732283464567121 ) ) ;
#76542=PLANE ( 'NONE',  #43461 ) ;
#76543=CARTESIAN_POINT ( 'NONE',  ( -1.266404199475064773, -0.3162353388693405765, 0.4822834645669290543 ) ) ;
#76544=CARTESIAN_POINT ( 'NONE',  ( -0.4002624671916004129, -0.3162353388693405765, 0.4822834645669290543 ) ) ;
#76547=CARTESIAN_POINT ( 'NONE',  ( 0.7480314960629927956, -0.5511811023622047445, 6.969142054262312111E-17 ) ) ;
#76548=CARTESIAN_POINT ( 'NONE',  ( -0.2887139107611542133, -0.6046776061558809534, -0.2411417322834644161 ) ) ;
#76549=CARTESIAN_POINT ( 'NONE',  ( -0.5839895013123351797, -0.6692913385826771977, 0.1292274648535927661 ) ) ;
#76550=CARTESIAN_POINT ( 'NONE',  ( -0.7086614173228339419, -0.1870078740157479769, 0.3641732283464567677 ) ) ;
#76552=CARTESIAN_POINT ( 'NONE',  ( -0.01312335958005186876, 0.05413385826771626580, -0.4176697321401330321 ) ) ;
#76553=CARTESIAN_POINT ( 'NONE',  ( -1.561679790026246017, -0.004921259842519576551, 0.3153832671262227771 ) ) ;
#76554=CARTESIAN_POINT ( 'NONE',  ( 1.345144356955381593, -0.3162353388693409650, -0.4822834645669289433 ) ) ;
#76559=CARTESIAN_POINT ( 'NONE',  ( -1.266404199475064773, -0.3162353388693405765, 0.4822834645669290543 ) ) ;
#76560=CARTESIAN_POINT ( 'NONE',  ( -0.9317585301837263412, 0.05413385826771666132, 0.4176697321401328100 ) ) ;
#76561=CARTESIAN_POINT ( 'NONE',  ( 1.574803149606299746, -0.1870078740157479769, 0.4822834645669291653 ) ) ;
#76564=CARTESIAN_POINT ( 'NONE',  ( 1.023622047244095334, -0.1870078740157479769, 0.4822834645669291653 ) ) ;
#76565=CARTESIAN_POINT ( 'NONE',  ( -0.01312335958005186876, 0.05413385826771626580, -0.4176697321401330321 ) ) ;
#76567=CARTESIAN_POINT ( 'NONE',  ( -0.7480314960629916854, 2.793565526369265584, 0.000000000000000000 ) ) ;
#76568=CARTESIAN_POINT ( 'NONE',  ( 1.200787401574803681, -0.4536011799217368745, -0.2665933059059886201 ) ) ;
#76570=ORIENTED_EDGE ( 'NONE', *, *, #66179, .T. ) ;
#76573=CARTESIAN_POINT ( 'NONE',  ( 0.3740157480314966754, 0.1660481256975883668, -0.3530559997133364547 ) ) ;
#76574=CARTESIAN_POINT ( 'NONE',  ( -0.6430446194225716283, -0.4281496062992124485, 0.4176697321401328655 ) ) ;
#76575=CARTESIAN_POINT ( 'NONE',  ( -1.561679790026246017, -0.4281496062992127816, -0.4176697321401328100 ) ) ;
#76576=CARTESIAN_POINT ( 'NONE',  ( 0.8530183727034128527, -0.4281496062992124485, 0.4176697321401328655 ) ) ;
#76577=CARTESIAN_POINT ( 'NONE',  ( -1.561679790026246017, -0.3690944881889765550, -0.3153832671262227771 ) ) ;
#76578=CARTESIAN_POINT ( 'NONE',  ( 1.377952755905512472, -0.6692913385826771977, 8.415575281601705876E-17 ) ) ;
#76579=CARTESIAN_POINT ( 'NONE',  ( -0.07217847769028787330, -0.05778040916215522460, 0.4822834645669289988 ) ) ;
#76580=CARTESIAN_POINT ( 'NONE',  ( -1.200787401574802349, -0.5400638737290844871, 0.3530559997133364547 ) ) ;
#76581=CARTESIAN_POINT ( 'NONE',  ( 1.456692913385827515, 0.2952755905511811885, 0.000000000000000000 ) ) ;
#76582=CARTESIAN_POINT ( 'NONE',  ( 1.646981627296588035, -0.3162353388693405765, 0.4822834645669290543 ) ) ;
#76584=CARTESIAN_POINT ( 'NONE',  ( 0.8989501312335964611, 0.1771653543307087630, 0.09757992244046791164 ) ) ;
#76588=CARTESIAN_POINT ( 'NONE',  ( 0.1837270341207354329, 0.1283753931104748280, 0.1820866141732283561 ) ) ;
#76590=CARTESIAN_POINT ( 'NONE',  ( 0.09186351706036799403, -0.4281496062992127816, -0.4176697321401328100 ) ) ;
#76591=CARTESIAN_POINT ( 'NONE',  ( 0.3346456692913390985, 0.1660481256975885056, 0.3530559997133364547 ) ) ;
#76592=CARTESIAN_POINT ( 'NONE',  ( -0.7020997375328076329, -0.3162353388693409650, -0.4822834645669289433 ) ) ;
#76594=CARTESIAN_POINT ( 'NONE',  ( -1.076115485564303809, -0.6046776061558809534, -0.2411417322834644161 ) ) ;
#76596=CARTESIAN_POINT ( 'NONE',  ( 1.161417322834646271, 0.07958543189024071263, -0.2665933059059888421 ) ) ;
#76597=CARTESIAN_POINT ( 'NONE',  ( 0.7086614173228353852, -0.1870078740157479769, 0.4822834645669291653 ) ) ;
#76598=CARTESIAN_POINT ( 'NONE',  ( 0.8398950131233602345, -0.6046776061558807314, 0.2411417322834647770 ) ) ;
#76600=CARTESIAN_POINT ( 'NONE',  ( -1.338582677165353729, -0.1870078740157480879, -0.4822834645669291653 ) ) ;
#76603=CARTESIAN_POINT ( 'NONE',  ( 0.06561679790026316017, 0.05413385826771626580, -0.4176697321401330321 ) ) ;
#76607=CARTESIAN_POINT ( 'NONE',  ( 1.410761154855643795, -0.3162353388693405765, 0.4822834645669290543 ) ) ;
#76608=CARTESIAN_POINT ( 'NONE',  ( 1.417322834645670104, -0.1870078740157480879, -0.4822834645669291653 ) ) ;
#76609=CARTESIAN_POINT ( 'NONE',  ( 0.2559055118110243332, 0.07958543189024085140, 0.2665933059059887866 ) ) ;
#76610=CARTESIAN_POINT ( 'NONE',  ( 1.056430446194226436, -0.6692913385826773087, -0.1292274648535924053 ) ) ;
#76612=CARTESIAN_POINT ( 'NONE',  ( 0.2099737532808405305, -0.5023911411419708095, 0.1820866141732285504 ) ) ;
#76613=CARTESIAN_POINT ( 'NONE',  ( 0.1902887139107617975, 0.2952755905511811885, 0.1292274648535926551 ) ) ;
#76615=CARTESIAN_POINT ( 'NONE',  ( -1.312335958005248715, -0.6046776061558809534, -0.2411417322834644161 ) ) ;
#76616=CARTESIAN_POINT ( 'NONE',  ( 0.9514435695538062676, -0.08942795157527998196, 0.3641732283464567121 ) ) ;
#76617=CARTESIAN_POINT ( 'NONE',  ( 0.3412073490813655186, 0.1539470093639523085, 0.1968503937007873850 ) ) ;
#76618=CARTESIAN_POINT ( 'NONE',  ( -0.1115485564304456306, 0.2952755905511810774, -0.1292274648535930714 ) ) ;
#76619=CARTESIAN_POINT ( 'NONE',  ( -0.3280839895013117347, -0.004921259842519870586, -0.3153832671262229437 ) ) ;
#76621=CARTESIAN_POINT ( 'NONE',  ( -0.3674540682414692561, -0.6046776061558809534, -0.2411417322834644161 ) ) ;
#76622=CARTESIAN_POINT ( 'NONE',  ( 0.1509186351706042484, -0.2845877964562159024, 0.3641732283464567677 ) ) ;
#76624=CARTESIAN_POINT ( 'NONE',  ( -0.2230971128608915943, 0.05413385826771666132, 0.4176697321401328100 ) ) ;
#76625=CARTESIAN_POINT ( 'NONE',  ( 1.003937007874016407, -0.4536011799217367080, 0.2665933059059888421 ) ) ;
#76627=CARTESIAN_POINT ( 'NONE',  ( -0.8136482939632537770, -0.5023911411419708095, 0.1820866141732285504 ) ) ;
#76628=CARTESIAN_POINT ( 'NONE',  ( -0.5446194225721777693, -0.2845877964562161244, -0.3641732283464567121 ) ) ;
#76629=CARTESIAN_POINT ( 'NONE',  ( -0.3083989501312330295, -0.3162353388693409650, -0.4822834645669289433 ) ) ;
#76630=CARTESIAN_POINT ( 'NONE',  ( 0.02624671916010564918, 0.2306618581243848609, 0.2411417322834645549 ) ) ;
#76631=CARTESIAN_POINT ( 'NONE',  ( 0.9448818897637802916, -0.1870078740157480601, -0.3641732283464567677 ) ) ;
#76633=CARTESIAN_POINT ( 'NONE',  ( 1.423884514435696191, -0.08942795157527998196, 0.3641732283464567121 ) ) ;
#76634=CARTESIAN_POINT ( 'NONE',  ( 0.8595800524934390507, -0.3162353388693405765, 0.4822834645669290543 ) ) ;
#76636=CARTESIAN_POINT ( 'NONE',  ( -0.3215223097112853146, -0.3162353388693405765, 0.4822834645669290543 ) ) ;
#76638=CARTESIAN_POINT ( 'NONE',  ( -1.528871391076114250, 0.2952755905511810774, -0.1292274648535930714 ) ) ;
#76639=CARTESIAN_POINT ( 'NONE',  ( 1.089238845144357759, 0.05413385826771626580, -0.4176697321401330321 ) ) ;
#76640=CARTESIAN_POINT ( 'NONE',  ( 0.4790026246719168435, -0.3162353388693409650, -0.4822834645669289433 ) ) ;
#76642=CARTESIAN_POINT ( 'NONE',  ( 0.2165354330708668673, -0.4536011799217367080, 0.2665933059059888421 ) ) ;
#76643=CARTESIAN_POINT ( 'NONE',  ( 1.325459317585302665, -0.4281496062992124485, 0.4176697321401328655 ) ) ;
#76644=CARTESIAN_POINT ( 'NONE',  ( -0.4658792650918627265, -0.08942795157527998196, 0.3641732283464567121 ) ) ;
#76645=CARTESIAN_POINT ( 'NONE',  ( -0.5511811023622038563, -0.1870078740157479769, 0.4822834645669291653 ) ) ;
#76647=CARTESIAN_POINT ( 'NONE',  ( 0.07874015748031558404, -0.1870078740157480879, -0.4822834645669291653 ) ) ;
#76648=CARTESIAN_POINT ( 'NONE',  ( -0.7349081364829387342, -0.6046776061558807314, 0.2411417322834647770 ) ) ;
#76649=CARTESIAN_POINT ( 'NONE',  ( -0.8202099737532801971, -0.5511811023622046335, 0.09757992244046803654 ) ) ;
#76650=CARTESIAN_POINT ( 'NONE',  ( 0.3674540682414705883, 0.2306618581243847221, -0.2411417322834647770 ) ) ;
#76651=CARTESIAN_POINT ( 'NONE',  ( -1.463254593175852492, -0.6692913385826773087, -0.1292274648535924053 ) ) ;
#76652=CARTESIAN_POINT ( 'NONE',  ( -0.2493438320209966919, -0.4281496062992124485, 0.4176697321401328655 ) ) ;
#76653=DIRECTION ( 'NONE',  ( 0.000000000000000000, 0.000000000000000000, -1.000000000000000000 ) ) ;
#76654=CARTESIAN_POINT ( 'NONE',  ( 1.187664041994751285, -0.3162353388693409650, -0.4822834645669289433 ) ) ;
#76655=CARTESIAN_POINT ( 'NONE',  ( 1.167979002624672580, -0.4281496062992124485, 0.4176697321401328655 ) ) ;
#76657=CARTESIAN_POINT ( 'NONE',  ( -1.581364829396324945, -0.05778040916215560624, -0.4822834645669293319 ) ) ;
#76658=CARTESIAN_POINT ( 'NONE',  ( -0.7152230971128602510, -0.05778040916215560624, -0.4822834645669293319 ) ) ;
#76662=CARTESIAN_POINT ( 'NONE',  ( -0.1181102362204717315, -0.5511811023622047445, 6.969142054262312111E-17 ) ) ;
#76664=CARTESIAN_POINT ( 'NONE',  ( 0.7808398950131240079, -0.3162353388693405765, 0.4822834645669290543 ) ) ;
#76667=CARTESIAN_POINT ( 'NONE',  ( -0.3018372703412066094, -0.3690944881889765550, -0.3153832671262227771 ) ) ;
#76669=CARTESIAN_POINT ( 'NONE',  ( 1.154855643044620184, -0.6046776061558807314, 0.2411417322834647770 ) ) ;
#76670=CARTESIAN_POINT ( 'NONE',  ( 0.8792650918635177559, -0.3690944881889765550, -0.3153832671262227771 ) ) ;
#76671=CIRCLE ( 'NONE', #40397, 3.543307086614173151 ) ;
#76672=CARTESIAN_POINT ( 'NONE',  ( -0.1968503937007867743, 0.2952755905511811885, 0.000000000000000000 ) ) ;
#76674=CARTESIAN_POINT ( 'NONE',  ( -0.2952755905511803003, -0.5400638737290845981, -0.3530559997133363437 ) ) ;
#76675=CARTESIAN_POINT ( 'NONE',  ( -1.404199475065615932, -0.004921259842519576551, 0.3153832671262227771 ) ) ;
#76676=CARTESIAN_POINT ( 'NONE',  ( -0.3018372703412066094, 0.05413385826771666132, 0.4176697321401328100 ) ) ;
#76678=CARTESIAN_POINT ( 'NONE',  ( 0.4581547953330915024, 1.765968763644078399, -0.5309055118110237448 ) ) ;
#76681=CARTESIAN_POINT ( 'NONE',  ( 0.4461942257217856311, 0.2306618581243847221, -0.2411417322834647770 ) ) ;
#76682=VERTEX_POINT ( 'NONE', #62668 ) ;
#76683=CARTESIAN_POINT ( 'NONE',  ( -0.5643044619422565855, 0.05413385826771626580, -0.4176697321401330321 ) ) ;
#76684=CARTESIAN_POINT ( 'NONE',  ( 1.502624671916010790, -0.3162353388693409650, -0.4822834645669289433 ) ) ;
#76685=CARTESIAN_POINT ( 'NONE',  ( 0.7939632545931766261, -0.05778040916215522460, 0.4822834645669289988 ) ) ;
#76686=CARTESIAN_POINT ( 'NONE',  ( -0.1312335958005241554, -0.6046776061558809534, -0.2411417322834644161 ) ) ;
#76688=CARTESIAN_POINT ( 'NONE',  ( -0.8661417322834640276, -0.1870078740157480879, -0.4822834645669291653 ) ) ;
#76689=CARTESIAN_POINT ( 'NONE',  ( -0.3215223097112853146, -0.05778040916215560624, -0.4822834645669293319 ) ) ;
#76690=CARTESIAN_POINT ( 'NONE',  ( -1.069553805774277722, -0.6692913385826773087, -0.1292274648535924053 ) ) ;
#76691=CARTESIAN_POINT ( 'NONE',  ( 0.03280839895013198948, -0.5511811023622048555, -0.09757992244046775898 ) ) ;
#76693=CARTESIAN_POINT ( 'NONE',  ( -0.04593175853018302557, -0.6692913385826773087, -0.1292274648535924053 ) ) ;
#76695=CARTESIAN_POINT ( 'NONE',  ( 1.036745406824147508, -0.4281496062992127816, -0.4176697321401328100 ) ) ;
#76697=ORIENTED_EDGE ( 'NONE', *, *, #68362, .F. ) ;
#76698=EDGE_CURVE ( 'NONE', #21487, #36098, #82258, .T. ) ;
#76699=ORIENTED_EDGE ( 'NONE', *, *, #21875, .T. ) ;
#76700=CARTESIAN_POINT ( 'NONE',  ( 0.1968503937007881344, -0.6692913385826771977, 8.415575281601705876E-17 ) ) ;
#76701=CARTESIAN_POINT ( 'NONE',  ( -0.4593175853018366950, -0.004921259842519576551, 0.3153832671262227771 ) ) ;
#76702=CARTESIAN_POINT ( 'NONE',  ( 1.404199475065617708, -0.004921259842519870586, -0.3153832671262229437 ) ) ;
#76703=CARTESIAN_POINT ( 'NONE',  ( -0.06840103802055999549, -4.511432564584533345E-15, 0.4281993546915565108 ) ) ;
#76706=CARTESIAN_POINT ( 'NONE',  ( 1.450131233595801428, -0.5511811023622048555, -0.09757992244046775898 ) ) ;
#76707=CARTESIAN_POINT ( 'NONE',  ( -1.568241469816272105, -0.3162353388693409650, -0.4822834645669289433 ) ) ;
#76709=CARTESIAN_POINT ( 'NONE',  ( 0.5905511811023629321, -0.6692913385826771977, 8.415575281601705876E-17 ) ) ;
#76710=CARTESIAN_POINT ( 'NONE',  ( -1.312335958005248715, 0.2306618581243848609, 0.2411417322834645549 ) ) ;
#76711=CARTESIAN_POINT ( 'NONE',  ( -1.062992125984250968, 0.2952755905511811885, 0.000000000000000000 ) ) ;
#76712=CARTESIAN_POINT ( 'NONE',  ( 0.2559055118110243332, -0.5400638737290845981, -0.3530559997133363437 ) ) ;
#76714=CARTESIAN_POINT ( 'NONE',  ( -1.482939632545930975, -0.004921259842519576551, 0.3153832671262227771 ) ) ;
#76715=CARTESIAN_POINT ( 'NONE',  ( 0.8923884514435701520, -0.6046776061558809534, -0.2411417322834644161 ) ) ;
#76716=CARTESIAN_POINT ( 'NONE',  ( 1.371391076115485941, 0.1771653543307087630, 0.09757992244046791164 ) ) ;
#76719=CARTESIAN_POINT ( 'NONE',  ( 0.6627296587926517768, -0.5511811023622048555, -0.09757992244046775898 ) ) ;
#76720=CARTESIAN_POINT ( 'NONE',  ( -1.102362204724408601, -0.1870078740157480879, -0.4822834645669291653 ) ) ;
#76722=CARTESIAN_POINT ( 'NONE',  ( 1.384514435695538559, 0.2952755905511810774, -0.1292274648535930714 ) ) ;
#76724=CARTESIAN_POINT ( 'NONE',  ( 0.6167979002624679463, 0.05413385826771626580, -0.4176697321401330321 ) ) ;
#76726=CARTESIAN_POINT ( 'NONE',  ( -1.660104986876639543, -0.08942795157528024563, -0.3641732283464568787 ) ) ;
#76727=CARTESIAN_POINT ( 'NONE',  ( -0.1049868766404193215, -0.6046776061558807314, 0.2411417322834647770 ) ) ;
#76728=CARTESIAN_POINT ( 'NONE',  ( 0.8661417322834652488, -0.1870078740157480601, -0.3641732283464567677 ) ) ;
#76729=CARTESIAN_POINT ( 'NONE',  ( 0.9055118110236227702, 0.2952755905511811885, 0.000000000000000000 ) ) ;
#76731=CARTESIAN_POINT ( 'NONE',  ( -0.7020997375328076329, -0.2845877964562161244, -0.3641732283464567121 ) ) ;
#76732=CARTESIAN_POINT ( 'NONE',  ( -0.6561679790026240244, -0.6046776061558807314, 0.2411417322834647770 ) ) ;
#76733=CARTESIAN_POINT ( 'NONE',  ( 1.587926509186352586, -0.4281496062992127816, -0.4176697321401328100 ) ) ;
#76735=CARTESIAN_POINT ( 'NONE',  ( -1.082677165354329896, 0.1660481256975885056, 0.3530559997133364547 ) ) ;
#76737=CARTESIAN_POINT ( 'NONE',  ( 1.003937007874016407, -0.5400638737290844871, 0.3530559997133364547 ) ) ;
#76739=CARTESIAN_POINT ( 'NONE',  ( -1.496062992125983815, -0.1870078740157479769, 0.3641732283464567677 ) ) ;
#76741=CARTESIAN_POINT ( 'NONE',  ( 1.017060367454068581, -0.05778040916215560624, -0.4822834645669293319 ) ) ;
#76744=CARTESIAN_POINT ( 'NONE',  ( -1.338582677165353729, -0.1870078740157479769, 0.3641732283464567677 ) ) ;
#76745=CARTESIAN_POINT ( 'NONE',  ( -1.213910761154854745, 0.1771653543307087075, -0.09757992244046823083 ) ) ;
#76746=CARTESIAN_POINT ( 'NONE',  ( 1.568241469816273659, -0.08942795157528024563, -0.3641732283464568787 ) ) ;
#76747=CARTESIAN_POINT ( 'NONE',  ( -0.1968503937007867743, 0.2952755905511811885, 0.000000000000000000 ) ) ;
#76748=CARTESIAN_POINT ( 'NONE',  ( -0.3543307086614165824, 0.1771653543307087630, 0.000000000000000000 ) ) ;
#76750=CARTESIAN_POINT ( 'NONE',  ( 1.082677165354331228, -0.4536011799217367080, 0.2665933059059888421 ) ) ;
#76751=CARTESIAN_POINT ( 'NONE',  ( 0.9317585301837276734, 0.05413385826771626580, -0.4176697321401330321 ) ) ;
#76753=CARTESIAN_POINT ( 'NONE',  ( -0.006561679790025524116, -0.08942795157528024563, -0.3641732283464568787 ) ) ;
#76754=CARTESIAN_POINT ( 'NONE',  ( 0.4658792650918641698, -0.05778040916215560624, -0.4822834645669293319 ) ) ;
#76755=CARTESIAN_POINT ( 'NONE',  ( 0.5314960629921264834, 0.07958543189024071263, -0.2665933059059888421 ) ) ;
#76756=CARTESIAN_POINT ( 'NONE',  ( 1.450131233595801428, 0.2952755905511811885, 0.1292274648535926551 ) ) ;
#76758=CARTESIAN_POINT ( 'NONE',  ( -1.463254593175852492, 0.2952755905511811885, 0.1292274648535926551 ) ) ;
#76759=CARTESIAN_POINT ( 'NONE',  ( -0.4330708661417315697, 0.2952755905511811885, 0.000000000000000000 ) ) ;
#76762=CARTESIAN_POINT ( 'NONE',  ( 0.4790026246719167324, -0.05778040916215522460, 0.4822834645669289988 ) ) ;
#76763=CARTESIAN_POINT ( 'NONE',  ( 1.253280839895013710, -0.2845877964562159024, 0.3641732283464567677 ) ) ;
#76764=CARTESIAN_POINT ( 'NONE',  ( -0.5314960629921250401, 0.1660481256975885056, 0.3530559997133364547 ) ) ;
#76765=CARTESIAN_POINT ( 'NONE',  ( 0.4265091863517067039, -0.6692913385826773087, -0.1292274648535924053 ) ) ;
#76770=CARTESIAN_POINT ( 'NONE',  ( -1.135170603674539924, -0.5511811023622046335, 0.09757992244046803654 ) ) ;
#76771=CARTESIAN_POINT ( 'NONE',  ( -1.056430446194224881, 0.2952755905511810774, -0.1292274648535930714 ) ) ;
#76773=CARTESIAN_POINT ( 'NONE',  ( 1.043307086614173818, 0.1660481256975885056, 0.3530559997133364547 ) ) ;
#76774=CARTESIAN_POINT ( 'NONE',  ( 1.443569553805774897, 0.2306618581243848609, 0.2411417322834645549 ) ) ;
#76775=CARTESIAN_POINT ( 'NONE',  ( 0.6496062992125991586, 0.1660481256975885056, 0.3530559997133364547 ) ) ;
#76778=CARTESIAN_POINT ( 'NONE',  ( 1.528871391076116026, 0.2952755905511811885, 0.1292274648535926551 ) ) ;
#76779=CARTESIAN_POINT ( 'NONE',  ( 0.4068241469816279987, -0.4281496062992127816, -0.4176697321401328100 ) ) ;
#76780=CARTESIAN_POINT ( 'NONE',  ( 0.6233595800524939223, -0.3162353388693405765, 0.4822834645669290543 ) ) ;
#76781=CARTESIAN_POINT ( 'NONE',  ( 1.023622047244095112, -0.1870078740157480601, -0.3641732283464567677 ) ) ;
#76782=CARTESIAN_POINT ( 'NONE',  ( 1.299212598425197429, -0.6692913385826771977, 8.415575281601705876E-17 ) ) ;
#76784=CARTESIAN_POINT ( 'NONE',  ( 0.3083989501312343062, -0.3162353388693405765, 0.4822834645669290543 ) ) ;
#76785=CARTESIAN_POINT ( 'NONE',  ( 1.213910761154856299, 0.2952755905511811885, 0.1292274648535926551 ) ) ;
#76786=CARTESIAN_POINT ( 'NONE',  ( 0.3805774278215230400, -0.4281496062992124485, 0.4176697321401328655 ) ) ;
#76787=CARTESIAN_POINT ( 'NONE',  ( 1.299212598425197429, -0.5511811023622047445, 6.969142054262312111E-17 ) ) ;
#76788=CARTESIAN_POINT ( 'NONE',  ( -0.7874015748031489847, -0.1870078740157479769, 0.4822834645669291653 ) ) ;
#76789=CARTESIAN_POINT ( 'NONE',  ( -1.076115485564303809, 0.2306618581243848609, 0.2411417322834645549 ) ) ;
#76791=CARTESIAN_POINT ( 'NONE',  ( 1.345144356955381593, -0.3162353388693409650, -0.4822834645669289433 ) ) ;
#76798=CARTESIAN_POINT ( 'NONE',  ( 1.686351706036745890, 0.2952755905511811885, 0.1292274648535926551 ) ) ;
#76799=CARTESIAN_POINT ( 'NONE',  ( 1.266404199475066328, -0.08942795157527998196, 0.3641732283464567121 ) ) ;
#76801=CARTESIAN_POINT ( 'NONE',  ( 1.332020997375329197, -0.2845877964562159024, 0.3641732283464567677 ) ) ;
#76802=CARTESIAN_POINT ( 'NONE',  ( 0.6175017169405826456, 2.784432375088962958E-17, -0.3464511005275205946 ) ) ;
#76803=CARTESIAN_POINT ( 'NONE',  ( -0.1181102362204717315, 0.2952755905511811885, 0.000000000000000000 ) ) ;
#76806=CARTESIAN_POINT ( 'NONE',  ( -0.7283464566929126471, -0.4536011799217367080, 0.2665933059059888421 ) ) ;
#76807=FACE_OUTER_BOUND ( 'NONE', #32684, .T. ) ;
#76808=CARTESIAN_POINT ( 'NONE',  ( -1.377952755905511140, -0.6692913385826771977, 8.415575281601705876E-17 ) ) ;
#76809=CARTESIAN_POINT ( 'NONE',  ( 0.2559055118110243332, -0.5400638737290845981, -0.3530559997133363437 ) ) ;
#76810=CARTESIAN_POINT ( 'NONE',  ( 1.397637795275591177, -0.5400638737290844871, 0.3530559997133364547 ) ) ;
#76811=ORIENTED_EDGE ( 'NONE', *, *, #17436, .T. ) ;
#76815=CARTESIAN_POINT ( 'NONE',  ( -0.4986876640419939388, 0.1283753931104746893, -0.1820866141732285504 ) ) ;
#76816=CARTESIAN_POINT ( 'NONE',  ( -1.108923884514435132, -0.05778040916215560624, -0.4822834645669293319 ) ) ;
#76817=CARTESIAN_POINT ( 'NONE',  ( 0.8792650918635177559, 0.05413385826771666132, 0.4176697321401328100 ) ) ;
#76818=ORIENTED_EDGE ( 'NONE', *, *, #2159, .T. ) ;
#76820=CARTESIAN_POINT ( 'NONE',  ( 0.6958886929845793379, 0.004960608223781096116, -0.3437734562760177970 ) ) ;
#76821=CARTESIAN_POINT ( 'NONE',  ( 1.043307086614173818, 0.1660481256975885056, 0.3530559997133364547 ) ) ;
#76822=CARTESIAN_POINT ( 'NONE',  ( -1.174540682414697335, -0.3162353388693409650, -0.4822834645669289433 ) ) ;
#76824=CARTESIAN_POINT ( 'NONE',  ( -0.5577427821522301654, -0.08942795157528024563, -0.3641732283464568787 ) ) ;
#76826=CARTESIAN_POINT ( 'NONE',  ( -0.4593175853018364174, -0.3690944881889765550, -0.3153832671262227771 ) ) ;
#76827=CARTESIAN_POINT ( 'NONE',  ( 0.2427821522309716595, -0.2845877964562161244, -0.3641732283464567121 ) ) ;
#76829=CARTESIAN_POINT ( 'NONE',  ( -0.01312335958005186876, -0.4281496062992124485, 0.4176697321401328655 ) ) ;
#76830=CARTESIAN_POINT ( 'NONE',  ( -1.135170603674539924, 0.1771653543307087075, -0.09757992244046823083 ) ) ;
#76832=CARTESIAN_POINT ( 'NONE',  ( 1.115485564304462551, 0.05413385826771666132, 0.4176697321401328100 ) ) ;
#76833=CARTESIAN_POINT ( 'NONE',  ( -1.246719160104985846, -0.4281496062992127816, -0.4176697321401328100 ) ) ;
#76835=CARTESIAN_POINT ( 'NONE',  ( -0.2034120734908131112, -0.6692913385826773087, -0.1292274648535924053 ) ) ;
#76836=CARTESIAN_POINT ( 'NONE',  ( -0.8333333333333323711, 0.2952755905511811885, 0.1292274648535926551 ) ) ;
#76837=CARTESIAN_POINT ( 'NONE',  ( 0.6496062992125991586, -0.4536011799217368745, -0.2665933059059886201 ) ) ;
#76838=CARTESIAN_POINT ( 'NONE',  ( -0.1443569553805768291, -0.004921259842519576551, 0.3153832671262227771 ) ) ;
#76839=CARTESIAN_POINT ( 'NONE',  ( -0.6364829396325453192, -0.3162353388693405765, 0.4822834645669290543 ) ) ;
#76840=CARTESIAN_POINT ( 'NONE',  ( -1.312335958005248715, 0.2306618581243848609, 0.2411417322834645549 ) ) ;
#76842=CARTESIAN_POINT ( 'NONE',  ( 1.266404199475066328, -0.2845877964562161244, -0.3641732283464567121 ) ) ;
#76843=CARTESIAN_POINT ( 'NONE',  ( -0.06561679790026180015, 0.05413385826771666132, 0.4176697321401328100 ) ) ;
#76844=CARTESIAN_POINT ( 'NONE',  ( -1.587926509186350810, -0.4281496062992124485, 0.4176697321401328655 ) ) ;
#76847=ADVANCED_FACE ( 'NONE', ( #82443 ), #31390, .T. ) ;
#76848=CARTESIAN_POINT ( 'NONE',  ( -0.8070866141732276899, 0.07958543189024071263, -0.2665933059059888421 ) ) ;
#76849=CARTESIAN_POINT ( 'NONE',  ( 0.6496062992125991586, 0.1660481256975885056, 0.3530559997133364547 ) ) ;
#76850=CARTESIAN_POINT ( 'NONE',  ( -0.9120734908136475250, 0.1771653543307087630, 0.09757992244046791164 ) ) ;
#76852=CARTESIAN_POINT ( 'NONE',  ( -1.148293963254592542, -0.6692913385826773087, -0.1292274648535924053 ) ) ;
#76853=CARTESIAN_POINT ( 'NONE',  ( 0.7742782152230979209, 0.05413385826771626580, -0.4176697321401330321 ) ) ;
#76854=CARTESIAN_POINT ( 'NONE',  ( 0.6692913385826778638, -0.6692913385826771977, 8.415575281601705876E-17 ) ) ;
#76855=EDGE_CURVE ( 'NONE', #36505, #62181, #63162, .T. ) ;
#76856=CARTESIAN_POINT ( 'NONE',  ( 1.450131233595801428, 0.2952755905511811885, 0.1292274648535926551 ) ) ;
#76857=CARTESIAN_POINT ( 'NONE',  ( -1.437007874015747477, -0.4536011799217367080, 0.2665933059059888421 ) ) ;
#76863=CARTESIAN_POINT ( 'NONE',  ( 1.108923884514436686, -0.2845877964562161244, -0.3641732283464567121 ) ) ;
#76864=CARTESIAN_POINT ( 'NONE',  ( 0.5839895013123367340, -0.5511811023622048555, -0.09757992244046775898 ) ) ;
#76865=CARTESIAN_POINT ( 'NONE',  ( 0.04593175853018440641, 0.2952755905511810774, -0.1292274648535930714 ) ) ;
#76868=CARTESIAN_POINT ( 'NONE',  ( 0.2493438320209980519, -0.004921259842519576551, 0.3153832671262227771 ) ) ;
#76869=CARTESIAN_POINT ( 'NONE',  ( -0.5511811023622038563, -0.1870078740157479769, 0.4822834645669291653 ) ) ;
#76870=CARTESIAN_POINT ( 'NONE',  ( -1.384514435695537005, -0.6692913385826773087, -0.1292274648535924053 ) ) ;
#76871=CARTESIAN_POINT ( 'NONE',  ( 0.7020997375328090762, -0.3162353388693405765, 0.4822834645669290543 ) ) ;
#76873=B_SPLINE_CURVE_WITH_KNOTS ( 'NONE', 3,
 ( #70084, #63771, #12437, #5696 ),
 .UNSPECIFIED., .F., .F.,
 ( 4, 4 ),
 ( 3.210432057725814518E-07, 0.001287787053612007718 ),
 .UNSPECIFIED. ) ;
#76875=ADVANCED_FACE ( 'NONE', ( #23944 ), #8535, .F. ) ;
#76877=VERTEX_POINT ( 'NONE', #12153 ) ;
#76878=CARTESIAN_POINT ( 'NONE',  ( -1.200787401574802349, 0.1660481256975883668, -0.3530559997133364547 ) ) ;
#76879=CARTESIAN_POINT ( 'NONE',  ( -0.7611548556430438595, -0.6046776061558809534, -0.2411417322834644161 ) ) ;
#76880=CARTESIAN_POINT ( 'NONE',  ( -0.6102362204724400829, -0.4536011799217368745, -0.2665933059059886201 ) ) ;
#76881=CARTESIAN_POINT ( 'NONE',  ( -0.7808398950131222316, -0.3162353388693409650, -0.4822834645669289433 ) ) ;
#76885=CARTESIAN_POINT ( 'NONE',  ( 1.450131233595801428, -0.6692913385826773087, -0.1292274648535924053 ) ) ;
#76886=CARTESIAN_POINT ( 'NONE',  ( -0.6430446194225716283, -0.4281496062992124485, 0.4176697321401328655 ) ) ;
#76887=CARTESIAN_POINT ( 'NONE',  ( 0.3674540682414705883, 0.2306618581243847221, -0.2411417322834647770 ) ) ;
#76888=CARTESIAN_POINT ( 'NONE',  ( -0.7217847769028863381, -0.4281496062992124485, 0.4176697321401328655 ) ) ;
#76890=CARTESIAN_POINT ( 'NONE',  ( -0.9973753280839886548, 0.1283753931104748280, 0.1820866141732283561 ) ) ;
#76893=ORIENTED_EDGE ( 'NONE', *, *, #19084, .T. ) ;
#76894=PLANE ( 'NONE',  #5919 ) ;
#76895=CARTESIAN_POINT ( 'NONE',  ( -1.056430446194224881, -0.6692913385826771977, 0.1292274648535927661 ) ) ;
#76896=CARTESIAN_POINT ( 'NONE',  ( -0.8923884514435688198, -0.6046776061558807314, 0.2411417322834647770 ) ) ;
#76898=CARTESIAN_POINT ( 'NONE',  ( -1.227034120734907585, 0.2952755905511811885, 0.1292274648535926551 ) ) ;
#76899=CARTESIAN_POINT ( 'NONE',  ( -1.154855643044618851, -0.6046776061558809534, -0.2411417322834644161 ) ) ;
#76900=CARTESIAN_POINT ( 'NONE',  ( -1.633858267716534529, 0.1660481256975885056, 0.3530559997133364547 ) ) ;
#76902=CARTESIAN_POINT ( 'NONE',  ( 0.7086614173228353852, -0.1870078740157479769, 0.3641732283464567677 ) ) ;
#76905=CARTESIAN_POINT ( 'NONE',  ( -0.2952755905511804668, 0.07958543189024085140, 0.2665933059059887866 ) ) ;
#76906=CARTESIAN_POINT ( 'NONE',  ( -0.9711286089238838626, 0.2306618581243847221, -0.2411417322834647770 ) ) ;
#76907=CARTESIAN_POINT ( 'NONE',  ( 1.423884514435696191, -0.05778040916215522460, 0.4822834645669289988 ) ) ;
#76908=CARTESIAN_POINT ( 'NONE',  ( -0.3543307086614165824, 0.2952755905511811885, 0.000000000000000000 ) ) ;
#76912=CARTESIAN_POINT ( 'NONE',  ( -0.9973753280839886548, 0.2306618581243848609, 0.2411417322834645549 ) ) ;
#76914=CARTESIAN_POINT ( 'NONE',  ( 1.476377952755906220, 0.1660481256975883668, -0.3530559997133364547 ) ) ;
#76915=CARTESIAN_POINT ( 'NONE',  ( -1.325459317585300889, -0.3690944881889765550, -0.3153832671262227771 ) ) ;
#76916=CARTESIAN_POINT ( 'NONE',  ( -1.246719160104986512, 0.05413385826771666132, 0.4176697321401328100 ) ) ;
#76919=CARTESIAN_POINT ( 'NONE',  ( -0.7480314960629916854, 2.793565526369265584, 0.000000000000000000 ) ) ;
#76922=CARTESIAN_POINT ( 'NONE',  ( 0.06561679790026316017, -0.4281496062992124485, 0.4176697321401328655 ) ) ;
#76923=CARTESIAN_POINT ( 'NONE',  ( -1.148293963254592542, 0.1771653543307087630, 0.09757992244046791164 ) ) ;
#76924=CARTESIAN_POINT ( 'NONE',  ( -0.7020997375328076329, -0.3162353388693409650, -0.4822834645669289433 ) ) ;
#76926=CARTESIAN_POINT ( 'NONE',  ( -1.220472440944881054, 0.2952755905511811885, 0.000000000000000000 ) ) ;
#76927=CARTESIAN_POINT ( 'NONE',  ( -0.9776902887139098386, -0.6692913385826771977, 0.1292274648535927661 ) ) ;
#76929=CARTESIAN_POINT ( 'NONE',  ( -0.1049868766404193215, 0.2306618581243847221, -0.2411417322834647770 ) ) ;
#76931=CARTESIAN_POINT ( 'NONE',  ( 0.9776902887139113929, 0.1771653543307087630, 0.09757992244046791164 ) ) ;
#76932=CARTESIAN_POINT ( 'NONE',  ( -0.5643044619422565855, -0.004921259842519870586, -0.3153832671262229437 ) ) ;
#76933=CARTESIAN_POINT ( 'NONE',  ( 0.6102362204724416372, 0.07958543189024071263, -0.2665933059059888421 ) ) ;
#76934=CARTESIAN_POINT ( 'NONE',  ( 1.345144356955381593, -0.2845877964562161244, -0.3641732283464567121 ) ) ;
#76935=CARTESIAN_POINT ( 'NONE',  ( 1.259842519685040019, -0.1870078740157479769, 0.4822834645669291653 ) ) ;
#76936=CARTESIAN_POINT ( 'NONE',  ( 0.5314960629921267055, -0.4536011799217367080, 0.2665933059059888421 ) ) ;
#76938=CARTESIAN_POINT ( 'NONE',  ( -0.7611548556430438595, -0.6046776061558809534, -0.2411417322834644161 ) ) ;
#76939=CARTESIAN_POINT ( 'NONE',  ( 1.043307086614173818, -0.5400638737290845981, -0.3530559997133363437 ) ) ;
#76940=( BOUNDED_CURVE ( )  B_SPLINE_CURVE ( 1, ( #49893, #75999 ),
 .UNSPECIFIED., .F., .F. ) 
 B_SPLINE_CURVE_WITH_KNOTS ( ( 2, 2 ),
 ( 2.081668171172168513E-17, 0.001999999999999987899 ),
 .UNSPECIFIED. ) 
 CURVE ( )  GEOMETRIC_REPRESENTATION_ITEM ( )  RATIONAL_B_SPLINE_CURVE ( ( 0.9875488213027535656, 0.9875488213027535656 ) ) 
 REPRESENTATION_ITEM ( '' )  );
#76941=EDGE_CURVE ( 'NONE', #58371, #13764, #78234, .T. ) ;
#76943=CARTESIAN_POINT ( 'NONE',  ( -0.6364829396325453192, -0.08942795157528024563, -0.3641732283464568787 ) ) ;
#76944=CARTESIAN_POINT ( 'NONE',  ( 0.06873123812453012238, 8.471767977567108961E-16, -0.4445507791589058955 ) ) ;
#76945=CARTESIAN_POINT ( 'NONE',  ( 0.1902887139107617975, -0.6692913385826773087, -0.1292274648535924053 ) ) ;
#76947=CARTESIAN_POINT ( 'NONE',  ( 0.9120734908136489683, -0.5511811023622046335, 0.09757992244046803654 ) ) ;
#76948=CARTESIAN_POINT ( 'NONE',  ( 0.07217847769028949700, -0.08942795157528024563, -0.3641732283464568787 ) ) ;
#76949=CARTESIAN_POINT ( 'NONE',  ( 0.04593175853018440641, -0.6692913385826771977, 0.1292274648535927661 ) ) ;
#76950=CARTESIAN_POINT ( 'NONE',  ( -1.292650918635170010, -0.6692913385826771977, 0.1292274648535927661 ) ) ;
#76951=CARTESIAN_POINT ( 'NONE',  ( -0.7480314960629914633, -0.5511811023622047445, 6.969142054262312111E-17 ) ) ;
#76953=CARTESIAN_POINT ( 'NONE',  ( -0.5774278215223089816, -0.6046776061558807314, 0.2411417322834647770 ) ) ;
#76956=CARTESIAN_POINT ( 'NONE',  ( 0.2821522309711292364, -0.5511811023622046335, 0.09757992244046803654 ) ) ;
#76957=CARTESIAN_POINT ( 'NONE',  ( -0.5511811023622038563, -0.1870078740157479769, 0.4822834645669291653 ) ) ;
#76958=CARTESIAN_POINT ( 'NONE',  ( -1.036745406824146176, -0.4281496062992124485, 0.4176697321401328655 ) ) ;
#76959=CARTESIAN_POINT ( 'NONE',  ( -1.259842519685038686, -0.1870078740157480601, -0.3641732283464567677 ) ) ;
#76961=CARTESIAN_POINT ( 'NONE',  ( -0.5971128608923877978, -0.6692913385826773087, -0.1292274648535924053 ) ) ;
#76962=CARTESIAN_POINT ( 'NONE',  ( -0.7480314960629914633, -0.5511811023622047445, 6.969142054262312111E-17 ) ) ;
#76963=CARTESIAN_POINT ( 'NONE',  ( -1.384514435695537005, 0.1771653543307087630, 0.09757992244046791164 ) ) ;
#76964=CARTESIAN_POINT ( 'NONE',  ( 1.141732283464567566, 0.2952755905511811885, 0.000000000000000000 ) ) ;
#76968=CARTESIAN_POINT ( 'NONE',  ( -0.7480314960629922405, 1.900312960331933976, 0.000000000000000000 ) ) ;
#76969=CARTESIAN_POINT ( 'NONE',  ( -1.541994750656167090, 0.2952755905511811885, 0.1292274648535926551 ) ) ;
#76970=CARTESIAN_POINT ( 'NONE',  ( -1.082677165354329896, 0.1660481256975885056, 0.3530559997133364547 ) ) ;
#76971=CARTESIAN_POINT ( 'NONE',  ( -1.469816272965878357, 0.2306618581243848609, 0.2411417322834645549 ) ) ;
#76974=CARTESIAN_POINT ( 'NONE',  ( 0.9711286089238851948, -0.6046776061558809534, -0.2411417322834644161 ) ) ;
#76975=CARTESIAN_POINT ( 'NONE',  ( -0.05905511811023545637, 0.1660481256975885056, 0.3530559997133364547 ) ) ;
#76977=CARTESIAN_POINT ( 'NONE',  ( -0.9548908091195642545, -2.567464376874931580E-15, -0.4445507791589072832 ) ) ;
#76978=CARTESIAN_POINT ( 'NONE',  ( 1.003937007874016185, 0.07958543189024071263, -0.2665933059059888421 ) ) ;
#76979=EDGE_CURVE ( 'NONE', #34321, #65845, #42468, .T. ) ;
#76981=ORIENTED_EDGE ( 'NONE', *, *, #75011, .F. ) ;
#76984=CARTESIAN_POINT ( 'NONE',  ( -0.04593175853018302557, -0.6692913385826773087, -0.1292274648535924053 ) ) ;
#76985=CARTESIAN_POINT ( 'NONE',  ( -0.9383202099737524282, -0.05778040916215522460, 0.4822834645669289988 ) ) ;
#76986=CARTESIAN_POINT ( 'NONE',  ( -1.463254593175852492, 0.2952755905511811885, 0.1292274648535926551 ) ) ;
#76987=CARTESIAN_POINT ( 'NONE',  ( 0.8333333333333340365, -0.6692913385826771977, 0.1292274648535927661 ) ) ;
#76988=CARTESIAN_POINT ( 'NONE',  ( -1.640419947506561060, -0.004921259842519576551, 0.3153832671262227771 ) ) ;
#76989=CARTESIAN_POINT ( 'NONE',  ( 1.292650918635171564, 0.2952755905511811885, 0.1292274648535926551 ) ) ;
#76990=CARTESIAN_POINT ( 'NONE',  ( -0.6430446194225712953, 0.05413385826771626580, -0.4176697321401330321 ) ) ;
#76991=CARTESIAN_POINT ( 'NONE',  ( 0.4265091863517067039, -0.6692913385826773087, -0.1292274648535924053 ) ) ;
#76992=CARTESIAN_POINT ( 'NONE',  ( 1.535433070866142335, -0.6692913385826771977, 8.415575281601705876E-17 ) ) ;
#76993=CARTESIAN_POINT ( 'NONE',  ( 1.174540682414699111, -0.05778040916215560624, -0.4822834645669293319 ) ) ;
#76994=CARTESIAN_POINT ( 'NONE',  ( 1.660104986876641320, -0.05778040916215522460, 0.4822834645669289988 ) ) ;
#76995=CARTESIAN_POINT ( 'NONE',  ( -0.1902887139107604098, -0.6692913385826771977, 0.1292274648535927661 ) ) ;
#76997=CARTESIAN_POINT ( 'NONE',  ( 0.4527559055118117182, 0.07958543189024071263, -0.2665933059059888421 ) ) ;
#77001=CARTESIAN_POINT ( 'NONE',  ( -0.4068241469816267775, -0.004921259842519870586, -0.3153832671262229437 ) ) ;
#77003=CARTESIAN_POINT ( 'NONE',  ( 0.1574803149606306130, -0.1870078740157479769, 0.4822834645669291653 ) ) ;
#77004=CARTESIAN_POINT ( 'NONE',  ( 0.05905511811023681640, 0.1660481256975883668, -0.3530559997133364547 ) ) ;
#77005=CARTESIAN_POINT ( 'NONE',  ( -0.7283464566929126471, 0.1660481256975883668, -0.3530559997133364547 ) ) ;
#77007=CARTESIAN_POINT ( 'NONE',  ( -1.036745406824146176, -0.4281496062992124485, 0.4176697321401328655 ) ) ;
#77008=CARTESIAN_POINT ( 'NONE',  ( -1.604771003085129655, 1.553800022087478805, -0.1466069496707747277 ) ) ;
#77009=CARTESIAN_POINT ( 'NONE',  ( 1.089238845144357537, -0.3690944881889763329, 0.3153832671262228327 ) ) ;
#77011=CARTESIAN_POINT ( 'NONE',  ( 0.5511811023622055217, -0.1870078740157479769, 0.4822834645669291653 ) ) ;
#77012=CARTESIAN_POINT ( 'NONE',  ( 0.6824146981627303710, -0.6046776061558807314, 0.2411417322834647770 ) ) ;
#77014=CARTESIAN_POINT ( 'NONE',  ( -1.476377952755905110, -0.5400638737290845981, -0.3530559997133363437 ) ) ;
#77017=CARTESIAN_POINT ( 'NONE',  ( -0.1312335958005241554, 0.2306618581243848609, 0.2411417322834645549 ) ) ;
#77020=CARTESIAN_POINT ( 'NONE',  ( -1.154855643044618851, 0.1283753931104748280, 0.1820866141732283561 ) ) ;
#77021=CARTESIAN_POINT ( 'NONE',  ( 1.279527559055118724, 0.1660481256975885056, 0.3530559997133364547 ) ) ;
#77022=CARTESIAN_POINT ( 'NONE',  ( 1.187664041994751285, -0.05778040916215522460, 0.4822834645669289988 ) ) ;
#77023=CARTESIAN_POINT ( 'NONE',  ( 0.1574803149606306130, -0.1870078740157480601, -0.3641732283464567677 ) ) ;
#77024=CARTESIAN_POINT ( 'NONE',  ( 0.5971128608923890191, -0.6692913385826771977, 0.1292274648535927661 ) ) ;
#77026=CARTESIAN_POINT ( 'NONE',  ( 0.4461942257217856311, 0.1283753931104746893, -0.1820866141732285504 ) ) ;
#77027=CARTESIAN_POINT ( 'NONE',  ( 0.2821522309711292364, -0.6692913385826771977, 0.1292274648535927661 ) ) ;
#77030=CARTESIAN_POINT ( 'NONE',  ( -1.266404199475064773, -0.3162353388693405765, 0.4822834645669290543 ) ) ;
#77031=CARTESIAN_POINT ( 'NONE',  ( 0.6364829396325465405, -0.08942795157527998196, 0.3641732283464567121 ) ) ;
#77033=CARTESIAN_POINT ( 'NONE',  ( -0.2034120734908131112, -0.6692913385826773087, -0.1292274648535924053 ) ) ;
#77034=CARTESIAN_POINT ( 'NONE',  ( -0.2821522309711278487, -0.5511811023622048555, -0.09757992244046775898 ) ) ;
#77036=CARTESIAN_POINT ( 'NONE',  ( -0.1181102362204717315, 0.2952755905511811885, 0.000000000000000000 ) ) ;
#77037=CARTESIAN_POINT ( 'NONE',  ( 0.3477690288713918276, 0.1771653543307087630, 0.09757992244046791164 ) ) ;
#77039=CARTESIAN_POINT ( 'NONE',  ( 0.09842519685039434474, 0.1660481256975885056, 0.3530559997133364547 ) ) ;
#77041=CARTESIAN_POINT ( 'NONE',  ( 1.154855643044620184, -0.5023911411419708095, 0.1820866141732285504 ) ) ;
#77042=CARTESIAN_POINT ( 'NONE',  ( 0.1902887139107617975, 0.2952755905511811885, 0.1292274648535926551 ) ) ;
#77043=CARTESIAN_POINT ( 'NONE',  ( -0.8595800524934373854, -0.2845877964562161244, -0.3641732283464567121 ) ) ;
#77044=CARTESIAN_POINT ( 'NONE',  ( -0.5839895013123351797, 0.1771653543307087075, -0.09757992244046823083 ) ) ;
#77045=CARTESIAN_POINT ( 'NONE',  ( -0.7545931758530176614, -0.6692913385826773087, -0.1292274648535924053 ) ) ;
#77046=CARTESIAN_POINT ( 'NONE',  ( -0.07217847769028813698, -0.3162353388693409650, -0.4822834645669289433 ) ) ;
#77047=CARTESIAN_POINT ( 'NONE',  ( 0.4199475065616805614, 0.1283753931104748280, 0.1820866141732283561 ) ) ;
#77048=DIRECTION ( 'NONE',  ( 1.000000000000000000, 3.096699300667737464E-16, -1.692413147294446216E-16 ) ) ;
#77049=CARTESIAN_POINT ( 'NONE',  ( 1.332020997375328974, -0.08942795157528024563, -0.3641732283464568787 ) ) ;
#77050=CARTESIAN_POINT ( 'NONE',  ( 0.9251968503937015864, 0.1660481256975883668, -0.3530559997133364547 ) ) ;
#77052=CARTESIAN_POINT ( 'NONE',  ( -0.1312335958005241554, 0.2306618581243848609, 0.2411417322834645549 ) ) ;
#77054=CARTESIAN_POINT ( 'NONE',  ( 1.463254593175853824, 0.1771653543307087075, -0.09757992244046823083 ) ) ;
#77055=CARTESIAN_POINT ( 'NONE',  ( 0.7808398950131241190, -0.05778040916215560624, -0.4822834645669293319 ) ) ;
#77056=CARTESIAN_POINT ( 'NONE',  ( 0.05249343832021075018, -0.6046776061558807314, 0.2411417322834647770 ) ) ;
#77058=CARTESIAN_POINT ( 'NONE',  ( 0.5511811023622055217, -0.1870078740157479769, 0.3641732283464567677 ) ) ;
#77059=CARTESIAN_POINT ( 'NONE',  ( 0.7874015748031503170, -0.1870078740157480879, -0.4822834645669291653 ) ) ;
#77060=CARTESIAN_POINT ( 'NONE',  ( -0.5118110236220466680, -0.5511811023622047445, 6.969142054262312111E-17 ) ) ;
#77061=CARTESIAN_POINT ( 'NONE',  ( -0.5971128608923877978, -0.6692913385826773087, -0.1292274648535924053 ) ) ;
#77063=CARTESIAN_POINT ( 'NONE',  ( 0.1640419947506569498, -0.05778040916215522460, 0.4822834645669289988 ) ) ;
#77064=CARTESIAN_POINT ( 'NONE',  ( -1.371391076115484609, -0.6692913385826771977, 0.1292274648535927661 ) ) ;
#77066=CARTESIAN_POINT ( 'NONE',  ( -0.7611548556430438595, 0.1283753931104748280, 0.1820866141732283561 ) ) ;
#77067=CARTESIAN_POINT ( 'NONE',  ( 0.1771653543307093182, 0.1660481256975885056, 0.3530559997133364547 ) ) ;
#77068=CARTESIAN_POINT ( 'NONE',  ( -1.227034120734907585, 0.2952755905511811885, 0.1292274648535926551 ) ) ;
#77069=CARTESIAN_POINT ( 'NONE',  ( -0.2034120734908128059, 0.2952755905511811885, 0.1292274648535926551 ) ) ;
#77071=CARTESIAN_POINT ( 'NONE',  ( 1.272965879265092637, 0.05413385826771666132, 0.4176697321401328100 ) ) ;
#77072=CARTESIAN_POINT ( 'NONE',  ( 1.456692913385827515, -0.6692913385826771977, 8.415575281601705876E-17 ) ) ;
#77074=CARTESIAN_POINT ( 'NONE',  ( -1.528871391076114250, -0.6692913385826771977, 0.1292274648535927661 ) ) ;
#77075=CARTESIAN_POINT ( 'NONE',  ( -0.9908136482939626788, -0.6692913385826773087, -0.1292274648535924053 ) ) ;
#77080=CARTESIAN_POINT ( 'NONE',  ( -0.2099737532808391705, 0.1283753931104748280, 0.1820866141732283561 ) ) ;
#77084=CARTESIAN_POINT ( 'NONE',  ( 0.1706036745406830368, 0.05413385826771666132, 0.4176697321401328100 ) ) ;
#77087=CARTESIAN_POINT ( 'NONE',  ( -0.3608923884514428360, 0.1771653543307087630, 0.09757992244046791164 ) ) ;
#77088=CARTESIAN_POINT ( 'NONE',  ( 0.3674540682414705883, 0.2306618581243847221, -0.2411417322834647770 ) ) ;
#77089=CARTESIAN_POINT ( 'NONE',  ( 0.7349081364829403995, 0.2306618581243848609, 0.2411417322834645549 ) ) ;
#77090=CARTESIAN_POINT ( 'NONE',  ( 1.115485564304462551, -0.004921259842519576551, 0.3153832671262227771 ) ) ;
#77091=CARTESIAN_POINT ( 'NONE',  ( 0.1181102362204730916, 0.2952755905511811885, 0.000000000000000000 ) ) ;
#77093=CARTESIAN_POINT ( 'NONE',  ( -0.6955380577427815458, 0.05413385826771666132, 0.4176697321401328100 ) ) ;
#77094=CARTESIAN_POINT ( 'NONE',  ( -1.476377952755905110, -0.4536011799217368745, -0.2665933059059886201 ) ) ;
#77095=CARTESIAN_POINT ( 'NONE',  ( -0.6233595800524928121, -0.05778040916215522460, 0.4822834645669289988 ) ) ;
#77100=CARTESIAN_POINT ( 'NONE',  ( 0.1509186351706045259, -0.05778040916215560624, -0.4822834645669293319 ) ) ;
#77102=CARTESIAN_POINT ( 'NONE',  ( -0.7020997375328076329, -0.3162353388693409650, -0.4822834645669289433 ) ) ;
#77103=CARTESIAN_POINT ( 'NONE',  ( 1.312335958005249825, 0.2306618581243847221, -0.2411417322834647770 ) ) ;
#77104=CARTESIAN_POINT ( 'NONE',  ( 1.377952755905512472, -0.6692913385826771977, 8.415575281601705876E-17 ) ) ;
#77105=CARTESIAN_POINT ( 'NONE',  ( 0.7349081364829402885, -0.6046776061558809534, -0.2411417322834644161 ) ) ;
#77106=CARTESIAN_POINT ( 'NONE',  ( 0.1312335958005257930, 0.2306618581243847221, -0.2411417322834647770 ) ) ;
#77108=CARTESIAN_POINT ( 'NONE',  ( -1.017060367454067249, -0.3162353388693409650, -0.4822834645669289433 ) ) ;
#77109=CARTESIAN_POINT ( 'NONE',  ( -0.3608923884514428360, 0.2952755905511811885, 0.1292274648535926551 ) ) ;
#77110=CARTESIAN_POINT ( 'NONE',  ( -0.1706036745406816491, -0.004921259842519870586, -0.3153832671262229437 ) ) ;
#77112=CARTESIAN_POINT ( 'NONE',  ( -0.1312335958005241554, 0.2306618581243848609, 0.2411417322834645549 ) ) ;
#77114=CARTESIAN_POINT ( 'NONE',  ( 1.187664041994751285, -0.3162353388693409650, -0.4822834645669289433 ) ) ;
#77118=CARTESIAN_POINT ( 'NONE',  ( 0.1443569553805781891, 0.05413385826771626580, -0.4176697321401330321 ) ) ;
#77119=CARTESIAN_POINT ( 'NONE',  ( -0.2230971128608915943, -0.3690944881889765550, -0.3153832671262227771 ) ) ;
#77120=CARTESIAN_POINT ( 'NONE',  ( 1.482939632545932307, -0.3690944881889763329, 0.3153832671262228327 ) ) ;
#77124=CARTESIAN_POINT ( 'NONE',  ( 1.404199475065617708, -0.004921259842519870586, -0.3153832671262229437 ) ) ;
#77125=CARTESIAN_POINT ( 'NONE',  ( 1.515748031496063186, -0.5400638737290845981, -0.3530559997133363437 ) ) ;
#77127=CARTESIAN_POINT ( 'NONE',  ( -0.07217847769028813698, -0.3162353388693409650, -0.4822834645669289433 ) ) ;
#77128=CARTESIAN_POINT ( 'NONE',  ( -1.135170603674539924, 0.2952755905511810774, -0.1292274648535930714 ) ) ;
#77130=CARTESIAN_POINT ( 'NONE',  ( -1.108923884514435132, -0.3162353388693405765, 0.4822834645669290543 ) ) ;
#77131=CARTESIAN_POINT ( 'NONE',  ( 0.1181102362204730916, -0.6692913385826771977, 8.415575281601705876E-17 ) ) ;
#77133=CARTESIAN_POINT ( 'NONE',  ( -1.456692913385826182, 0.1771653543307087630, 0.000000000000000000 ) ) ;
#77134=CARTESIAN_POINT ( 'NONE',  ( 0.8595800524934390507, -0.05778040916215560624, -0.4822834645669293319 ) ) ;
#77135=CARTESIAN_POINT ( 'NONE',  ( 0.7480314960629927956, 0.1771653543307087630, 0.000000000000000000 ) ) ;
#77136=CARTESIAN_POINT ( 'NONE',  ( 0.8267716535433077274, 0.2066929133858268208, 0.000000000000000000 ) ) ;
#77137=CARTESIAN_POINT ( 'NONE',  ( 0.9973753280839902091, -0.5023911411419708095, 0.1820866141732285504 ) ) ;
#77138=CARTESIAN_POINT ( 'NONE',  ( -1.220472440944881054, -0.6692913385826771977, 8.415575281601705876E-17 ) ) ;
#77140=CARTESIAN_POINT ( 'NONE',  ( 1.279527559055118724, -0.5400638737290845981, -0.3530559997133363437 ) ) ;
#77142=CARTESIAN_POINT ( 'NONE',  ( 0.7742782152230979209, 0.05413385826771626580, -0.4176697321401330321 ) ) ;
#77144=CARTESIAN_POINT ( 'NONE',  ( -1.603475055217291612, 1.054977578535736926, -0.04573490813648262154 ) ) ;
#77145=CARTESIAN_POINT ( 'NONE',  ( -0.04593175853018302557, 0.2952755905511811885, 0.1292274648535926551 ) ) ;
#77146=CARTESIAN_POINT ( 'NONE',  ( 0.5577427821522314977, -0.2845877964562161244, -0.3641732283464567121 ) ) ;
#77148=CARTESIAN_POINT ( 'NONE',  ( 0.8530183727034128527, -0.4281496062992124485, 0.4176697321401328655 ) ) ;
#77149=CARTESIAN_POINT ( 'NONE',  ( -1.614173228346456712, 0.9921945702958917535, -0.1372047244094478091 ) ) ;
#77150=CARTESIAN_POINT ( 'NONE',  ( -0.9055118110236215490, 0.1771653543307087630, 0.000000000000000000 ) ) ;
#77151=CARTESIAN_POINT ( 'NONE',  ( -0.5708661417322828946, 0.1660481256975883668, -0.3530559997133364547 ) ) ;
#77152=CARTESIAN_POINT ( 'NONE',  ( 1.627296587926509996, -0.6046776061558807314, 0.2411417322834647770 ) ) ;
#77153=CARTESIAN_POINT ( 'NONE',  ( -1.115485564304461219, -0.4281496062992124485, 0.4176697321401328655 ) ) ;
#77154=CARTESIAN_POINT ( 'NONE',  ( 0.8792650918635177559, 0.05413385826771666132, 0.4176697321401328100 ) ) ;
#77155=CARTESIAN_POINT ( 'NONE',  ( -1.325459317585300889, -0.004921259842519576551, 0.3153832671262227771 ) ) ;
#77156=CARTESIAN_POINT ( 'NONE',  ( 0.9548908091195654757, -4.927456884911482678E-16, 0.4445507791589062840 ) ) ;
#77157=CARTESIAN_POINT ( 'NONE',  ( 1.200787401574803681, -0.5400638737290845981, -0.3530559997133363437 ) ) ;
#77159=CARTESIAN_POINT ( 'NONE',  ( -1.568241469816272105, -0.05778040916215522460, 0.4822834645669289988 ) ) ;
#77160=CARTESIAN_POINT ( 'NONE',  ( -1.522309711286088607, -0.5023911411419708095, 0.1820866141732285504 ) ) ;
#77161=CARTESIAN_POINT ( 'NONE',  ( -0.9383202099737524282, -0.08942795157527998196, 0.3641732283464567121 ) ) ;
#77162=CARTESIAN_POINT ( 'NONE',  ( 1.686351706036745890, 0.1771653543307087630, 0.09757992244046791164 ) ) ;
#77163=CARTESIAN_POINT ( 'NONE',  ( -0.3083989501312330295, -0.3162353388693409650, -0.4822834645669289433 ) ) ;
#77164=CARTESIAN_POINT ( 'NONE',  ( -0.2427821522309703550, -0.2845877964562159024, 0.3641732283464567677 ) ) ;
#77165=CARTESIAN_POINT ( 'NONE',  ( -1.463254593175852492, -0.5511811023622048555, -0.09757992244046775898 ) ) ;
#77166=CARTESIAN_POINT ( 'NONE',  ( 1.095800524934383846, -0.2845877964562159024, 0.3641732283464567677 ) ) ;
#77167=CARTESIAN_POINT ( 'NONE',  ( 0.5643044619422579178, 0.05413385826771666132, 0.4176697321401328100 ) ) ;
#77169=CARTESIAN_POINT ( 'NONE',  ( 0.4461942257217856311, 0.2306618581243847221, -0.2411417322834647770 ) ) ;
#77170=CARTESIAN_POINT ( 'NONE',  ( 0.4724409448818904789, -0.1870078740157479769, 0.3641732283464567677 ) ) ;
#77171=CARTESIAN_POINT ( 'NONE',  ( 1.561679790026247350, -0.4281496062992124485, 0.4176697321401328655 ) ) ;
#77172=EDGE_CURVE ( 'NONE', #38994, #77522, #71726, .T. ) ;
#77173=CARTESIAN_POINT ( 'NONE',  ( -1.437007874015747477, 0.1660481256975883668, -0.3530559997133364547 ) ) ;
#77174=CARTESIAN_POINT ( 'NONE',  ( -0.4133858267716528645, 0.1660481256975883668, -0.3530559997133364547 ) ) ;
#77177=CARTESIAN_POINT ( 'NONE',  ( -0.03937007874015669567, -0.6692913385826771977, 8.415575281601705876E-17 ) ) ;
#77178=CARTESIAN_POINT ( 'NONE',  ( 1.161417322834646271, 0.07958543189024071263, -0.2665933059059888421 ) ) ;
#77179=CARTESIAN_POINT ( 'NONE',  ( -0.2624671916010490880, -0.6046776061558807314, 0.2411417322834647770 ) ) ;
#77180=CARTESIAN_POINT ( 'NONE',  ( 0.3412073490813655186, 0.2306618581243848609, 0.2411417322834645549 ) ) ;
#77186=CARTESIAN_POINT ( 'NONE',  ( -0.8792650918635160906, -0.004921259842519870586, -0.3153832671262229437 ) ) ;
#77187=CARTESIAN_POINT ( 'NONE',  ( -1.135170603674539924, -0.6692913385826771977, 0.1292274648535927661 ) ) ;
#77189=CARTESIAN_POINT ( 'NONE',  ( 0.3083989501312343062, -0.05778040916215560624, -0.4822834645669293319 ) ) ;
#77190=CARTESIAN_POINT ( 'NONE',  ( 1.377952755905512472, -0.6692913385826771977, 8.415575281601705876E-17 ) ) ;
#77191=CARTESIAN_POINT ( 'NONE',  ( 0.6561679790026253567, 0.2306618581243848609, 0.2411417322834645549 ) ) ;
#77196=CARTESIAN_POINT ( 'NONE',  ( 0.3346456692913390985, 0.1660481256975885056, 0.3530559997133364547 ) ) ;
#77197=CARTESIAN_POINT ( 'NONE',  ( 0.06561679790026316017, 0.05413385826771626580, -0.4176697321401330321 ) ) ;
#77198=AXIS2_PLACEMENT_3D ( 'NONE', #51692, #18894, #19727 ) ;
#77199=CARTESIAN_POINT ( 'NONE',  ( 0.8398950131233602345, 0.1283753931104746893, -0.1820866141732285504 ) ) ;
#77200=CARTESIAN_POINT ( 'NONE',  ( 1.181102362204725198, -0.1870078740157479769, 0.4822834645669291653 ) ) ;
#77203=CARTESIAN_POINT ( 'NONE',  ( 0.5511811023622054106, -0.1870078740157480879, -0.4822834645669291653 ) ) ;
#77204=CARTESIAN_POINT ( 'NONE',  ( 1.207349081364829990, 0.2306618581243848609, 0.2411417322834645549 ) ) ;
#77205=CARTESIAN_POINT ( 'NONE',  ( 0.2165354330708668673, -0.5400638737290844871, 0.3530559997133364547 ) ) ;
#77206=CARTESIAN_POINT ( 'NONE',  ( 1.227034120734908917, 0.1771653543307087075, -0.09757992244046823083 ) ) ;
#77207=CARTESIAN_POINT ( 'NONE',  ( -1.076115485564303809, 0.2306618581243848609, 0.2411417322834645549 ) ) ;
#77208=CARTESIAN_POINT ( 'NONE',  ( -0.9120734908136475250, 0.2952755905511811885, 0.1292274648535926551 ) ) ;
#77209=CARTESIAN_POINT ( 'NONE',  ( 1.371391076115485719, -0.6692913385826773087, -0.1292274648535924053 ) ) ;
#77213=ORIENTED_EDGE ( 'NONE', *, *, #3251, .T. ) ;
#77217=CARTESIAN_POINT ( 'NONE',  ( 1.062992125984252745, -0.5511811023622047445, 6.969142054262312111E-17 ) ) ;
#77219=CARTESIAN_POINT ( 'NONE',  ( 1.194225721784777594, -0.004921259842519576551, 0.3153832671262227771 ) ) ;
#77222=CARTESIAN_POINT ( 'NONE',  ( -1.306827173596996738, 0.000000000000000000, -0.4445507791589060620 ) ) ;
#77224=CARTESIAN_POINT ( 'NONE',  ( -1.043307086614172041, -0.4536011799217367080, 0.2665933059059888421 ) ) ;
#77225=CARTESIAN_POINT ( 'NONE',  ( -1.469816272965878357, -0.5023911411419708095, -0.1820866141732282451 ) ) ;
#77226=CARTESIAN_POINT ( 'NONE',  ( -1.135170603674539924, 0.2952755905511810774, -0.1292274648535930714 ) ) ;
#77227=CARTESIAN_POINT ( 'NONE',  ( 0.01968503937007930540, 0.1660481256975885056, 0.3530559997133364547 ) ) ;
#77228=CARTESIAN_POINT ( 'NONE',  ( 1.601049868766404982, 0.2306618581243848609, 0.2411417322834645549 ) ) ;
#77230=CARTESIAN_POINT ( 'NONE',  ( 0.5611900217179910388, 1.223219560026271499E-15, 0.4445507791589056734 ) ) ;
#77234=CARTESIAN_POINT ( 'NONE',  ( 1.603475055217291612, 1.267857067133554061, 0.04573490813648273950 ) ) ;
#77235=CARTESIAN_POINT ( 'NONE',  ( -1.089238845144356427, -0.3690944881889765550, -0.3153832671262227771 ) ) ;
#77236=CARTESIAN_POINT ( 'NONE',  ( -0.9580052493438311334, 0.05413385826771626580, -0.4176697321401330321 ) ) ;
#77237=CARTESIAN_POINT ( 'NONE',  ( 0.5708661417322842269, 0.1660481256975885056, 0.3530559997133364547 ) ) ;
#77241=CARTESIAN_POINT ( 'NONE',  ( 1.332020997375329197, -0.3162353388693405765, 0.4822834645669290543 ) ) ;
#77242=CARTESIAN_POINT ( 'NONE',  ( 1.568241469816273437, -0.2845877964562159024, 0.3641732283464567677 ) ) ;
#77244=CARTESIAN_POINT ( 'NONE',  ( -0.2165354330708654795, -0.4536011799217368745, -0.2665933059059886201 ) ) ;
#77245=CARTESIAN_POINT ( 'NONE',  ( -1.266404199475064773, -0.08942795157528024563, -0.3641732283464568787 ) ) ;
#77248=CARTESIAN_POINT ( 'NONE',  ( -0.4199475065616791736, -0.5023911411419708095, 0.1820866141732285504 ) ) ;
#77249=CARTESIAN_POINT ( 'NONE',  ( 0.3083989501312343062, -0.2845877964562159024, 0.3641732283464567677 ) ) ;
#77250=CARTESIAN_POINT ( 'NONE',  ( 0.07217847769028949700, -0.05778040916215560624, -0.4822834645669293319 ) ) ;
#77251=CARTESIAN_POINT ( 'NONE',  ( -1.030183727034119867, -0.2845877964562159024, 0.3641732283464567677 ) ) ;
#77253=CARTESIAN_POINT ( 'NONE',  ( 1.259842519685040019, -0.1870078740157479769, 0.4822834645669291653 ) ) ;
#77254=CARTESIAN_POINT ( 'NONE',  ( -1.555118110236219930, -0.5400638737290845981, -0.3530559997133363437 ) ) ;
#77256=CARTESIAN_POINT ( 'NONE',  ( -0.2099737532808391705, -0.6046776061558809534, -0.2411417322834644161 ) ) ;
#77257=CARTESIAN_POINT ( 'NONE',  ( -1.049868766404198794, -0.6046776061558807314, 0.2411417322834647770 ) ) ;
#77258=CARTESIAN_POINT ( 'NONE',  ( 0.9514435695538062676, -0.2845877964562161244, -0.3641732283464567121 ) ) ;
#77260=CARTESIAN_POINT ( 'NONE',  ( -0.1115485564304456306, 0.1771653543307087075, -0.09757992244046823083 ) ) ;
#77261=CARTESIAN_POINT ( 'NONE',  ( -0.4855643044619415427, -0.4281496062992124485, 0.4176697321401328655 ) ) ;
#77262=CARTESIAN_POINT ( 'NONE',  ( -1.509186351706035767, -0.4281496062992124485, 0.4176697321401328655 ) ) ;
#77264=CARTESIAN_POINT ( 'NONE',  ( 1.482939632545932307, -0.3690944881889763329, 0.3153832671262228327 ) ) ;
#77265=CARTESIAN_POINT ( 'NONE',  ( -0.2493438320209966919, -0.4281496062992124485, 0.4176697321401328655 ) ) ;
#77266=CARTESIAN_POINT ( 'NONE',  ( -1.627296587926508442, -0.6046776061558809534, -0.2411417322834644161 ) ) ;
#77269=CARTESIAN_POINT ( 'NONE',  ( -0.8858267716535425107, -0.4536011799217367080, 0.2665933059059888421 ) ) ;
#77270=CARTESIAN_POINT ( 'NONE',  ( 0.6955380577427828781, 0.05413385826771626580, -0.4176697321401330321 ) ) ;
#77271=CARTESIAN_POINT ( 'NONE',  ( -1.023622047244094002, -0.1870078740157480601, -0.3641732283464567677 ) ) ;
#77273=CARTESIAN_POINT ( 'NONE',  ( -0.7939632545931754048, -0.3162353388693405765, 0.4822834645669290543 ) ) ;
#77274=CARTESIAN_POINT ( 'NONE',  ( 0.6824146981627303710, -0.6046776061558807314, 0.2411417322834647770 ) ) ;
#77275=CARTESIAN_POINT ( 'NONE',  ( 0.5511811023622055217, -0.1870078740157479769, 0.4822834645669291653 ) ) ;
#77276=CARTESIAN_POINT ( 'NONE',  ( 1.417322834645670104, -0.1870078740157479769, 0.4822834645669291653 ) ) ;
#77277=CARTESIAN_POINT ( 'NONE',  ( -1.522309711286088607, 0.1283753931104746893, -0.1820866141732285504 ) ) ;
#77282=CARTESIAN_POINT ( 'NONE',  ( 1.135170603674541256, -0.5511811023622048555, -0.09757992244046775898 ) ) ;
#77283=CARTESIAN_POINT ( 'NONE',  ( 0.3543307086614179147, 0.1771653543307087630, 0.000000000000000000 ) ) ;
#77284=CARTESIAN_POINT ( 'NONE',  ( 0.02624671916010564918, 0.2306618581243848609, 0.2411417322834645549 ) ) ;
#77285=CARTESIAN_POINT ( 'NONE',  ( 1.443569553805774897, 0.2306618581243848609, 0.2411417322834645549 ) ) ;
#77287=CARTESIAN_POINT ( 'NONE',  ( 0.3346456692913393205, -0.4536011799217368745, -0.2665933059059886201 ) ) ;
#77288=CARTESIAN_POINT ( 'NONE',  ( -0.5249343832020990641, 0.2306618581243848609, 0.2411417322834645549 ) ) ;
#77289=CARTESIAN_POINT ( 'NONE',  ( -1.082677165354329896, -0.5400638737290845981, -0.3530559997133363437 ) ) ;
#77290=CARTESIAN_POINT ( 'NONE',  ( 0.6364829396325465405, -0.3162353388693409650, -0.4822834645669289433 ) ) ;
#77295=VERTEX_POINT ( 'NONE', #7076 ) ;
#77296=CARTESIAN_POINT ( 'NONE',  ( -1.076115485564303809, 0.2306618581243848609, 0.2411417322834645549 ) ) ;
#77297=CARTESIAN_POINT ( 'NONE',  ( -0.7349081364829387342, -0.6046776061558807314, 0.2411417322834647770 ) ) ;
#77298=CARTESIAN_POINT ( 'NONE',  ( -0.6561679790026240244, 0.1283753931104746893, -0.1820866141732285504 ) ) ;
#77299=CARTESIAN_POINT ( 'NONE',  ( -0.7874015748031489847, -0.1870078740157480879, -0.4822834645669291653 ) ) ;
#77302=CARTESIAN_POINT ( 'NONE',  ( 0.4849061582275024929, 1.568468489416427580, -0.4921425059946356040 ) ) ;
#77303=CARTESIAN_POINT ( 'NONE',  ( -1.614173228346455824, 0.1771653543307087630, 0.000000000000000000 ) ) ;
#77304=CARTESIAN_POINT ( 'NONE',  ( -1.240157480314959759, 0.1660481256975885056, 0.3530559997133364547 ) ) ;
#77305=CARTESIAN_POINT ( 'NONE',  ( 0.2230971128608929543, 0.05413385826771626580, -0.4176697321401330321 ) ) ;
#77306=ADVANCED_FACE ( 'NONE', ( #26847 ), #76542, .T. ) ;
#77307=CARTESIAN_POINT ( 'NONE',  ( -0.7283464566929126471, -0.5400638737290844871, 0.3530559997133364547 ) ) ;
#77310=CARTESIAN_POINT ( 'NONE',  ( -0.9711286089238838626, 0.1283753931104746893, -0.1820866141732285504 ) ) ;
#77315=CARTESIAN_POINT ( 'NONE',  ( -1.272965879265091305, -0.4281496062992124485, 0.4176697321401328655 ) ) ;
#77316=CARTESIAN_POINT ( 'NONE',  ( -0.6889763779527552368, 0.1660481256975885056, 0.3530559997133364547 ) ) ;
#77318=CARTESIAN_POINT ( 'NONE',  ( -1.010498687664041384, -0.4281496062992127816, -0.4176697321401328100 ) ) ;
#77319=CARTESIAN_POINT ( 'NONE',  ( -1.437007874015747477, -0.5400638737290844871, 0.3530559997133364547 ) ) ;
#77322=CARTESIAN_POINT ( 'NONE',  ( 0.6496062992125991586, -0.4536011799217368745, -0.2665933059059886201 ) ) ;
#77323=CARTESIAN_POINT ( 'NONE',  ( 1.604771003085129433, 0.4934440724007135848, 0.1466069496707750885 ) ) ;
#77325=CARTESIAN_POINT ( 'NONE',  ( -0.4265091863517051496, 0.1771653543307087075, -0.09757992244046823083 ) ) ;
#77326=CARTESIAN_POINT ( 'NONE',  ( -0.6889763779527552368, 0.1660481256975885056, 0.3530559997133364547 ) ) ;
#77327=CARTESIAN_POINT ( 'NONE',  ( 1.430446194225722500, 0.05413385826771666132, 0.4176697321401328100 ) ) ;
#77328=CARTESIAN_POINT ( 'NONE',  ( -0.4921259842519677963, 0.1660481256975883668, -0.3530559997133364547 ) ) ;
#77332=CARTESIAN_POINT ( 'NONE',  ( -1.135170603674539924, 0.2952755905511810774, -0.1292274648535930714 ) ) ;
#77333=CARTESIAN_POINT ( 'NONE',  ( 1.489501312335958172, -0.05778040916215560624, -0.4822834645669293319 ) ) ;
#77334=CARTESIAN_POINT ( 'NONE',  ( -1.286089238845143479, -0.5023911411419708095, 0.1820866141732285504 ) ) ;
#77335=CARTESIAN_POINT ( 'NONE',  ( -1.489501312335957062, -0.3162353388693409650, -0.4822834645669289433 ) ) ;
#77341=CARTESIAN_POINT ( 'NONE',  ( -0.04593175853018302557, 0.2952755905511811885, 0.1292274648535926551 ) ) ;
#77342=CARTESIAN_POINT ( 'NONE',  ( -1.207349081364828436, -0.5023911411419708095, 0.1820866141732285504 ) ) ;
#77343=CARTESIAN_POINT ( 'NONE',  ( -0.8464566929133852113, -0.5400638737290845981, -0.3530559997133363437 ) ) ;
#77345=CARTESIAN_POINT ( 'NONE',  ( -1.187664041994750175, -0.05778040916215560624, -0.4822834645669293319 ) ) ;
#77346=CARTESIAN_POINT ( 'NONE',  ( -0.8923884514435688198, 0.2306618581243847221, -0.2411417322834647770 ) ) ;
#77347=CARTESIAN_POINT ( 'NONE',  ( -0.1115485564304456306, 0.2952755905511810774, -0.1292274648535930714 ) ) ;
#77349=CARTESIAN_POINT ( 'NONE',  ( 0.7086614173228352742, -0.1870078740157480601, -0.3641732283464567677 ) ) ;
#77350=CARTESIAN_POINT ( 'NONE',  ( -0.8202099737532801971, -0.5511811023622046335, 0.09757992244046803654 ) ) ;
#77352=CARTESIAN_POINT ( 'NONE',  ( 0.5708661417322842269, 0.07958543189024085140, 0.2665933059059887866 ) ) ;
#77353=CARTESIAN_POINT ( 'NONE',  ( 1.469816272965879911, 0.1283753931104746893, -0.1820866141732285504 ) ) ;
#77354=CARTESIAN_POINT ( 'NONE',  ( 1.456692913385827515, 0.2952755905511811885, 0.000000000000000000 ) ) ;
#77356=CARTESIAN_POINT ( 'NONE',  ( -0.07874015748031421014, -0.1870078740157479769, 0.3641732283464567677 ) ) ;
#77358=CARTESIAN_POINT ( 'NONE',  ( -0.7283464566929126471, -0.5400638737290844871, 0.3530559997133364547 ) ) ;
#77359=CARTESIAN_POINT ( 'NONE',  ( 1.364829396325459854, -0.6046776061558809534, -0.2411417322834644161 ) ) ;
#77361=CARTESIAN_POINT ( 'NONE',  ( -0.4068241469816264999, -0.3690944881889763329, 0.3153832671262228327 ) ) ;
#77362=CARTESIAN_POINT ( 'NONE',  ( 0.04593175853018440641, 0.2952755905511810219, -0.1292274648535930437 ) ) ;
#77363=CARTESIAN_POINT ( 'NONE',  ( 0.4527559055118117182, 0.1660481256975883668, -0.3530559997133364547 ) ) ;
#77365=CARTESIAN_POINT ( 'NONE',  ( 0.8661417322834652488, -0.1870078740157480601, -0.3641732283464567677 ) ) ;
#77366=CARTESIAN_POINT ( 'NONE',  ( 5.463695987328526437E-16, -0.1870078740157479769, 0.3641732283464567677 ) ) ;
#77367=CARTESIAN_POINT ( 'NONE',  ( 0.1771653543307093182, -0.5400638737290845981, -0.3530559997133363437 ) ) ;
#77368=CARTESIAN_POINT ( 'NONE',  ( -1.364829396325458521, 0.2306618581243847221, -0.2411417322834647770 ) ) ;
#77369=CARTESIAN_POINT ( 'NONE',  ( -0.5183727034120726440, 0.1771653543307087630, 0.09757992244046791164 ) ) ;
#77370=DIRECTION ( 'NONE',  ( 0.000000000000000000, 0.000000000000000000, -1.000000000000000000 ) ) ;
#77371=CARTESIAN_POINT ( 'NONE',  ( -1.017060367454067249, -0.05778040916215522460, 0.4822834645669289988 ) ) ;
#77374=CARTESIAN_POINT ( 'NONE',  ( 0.09842519685039434474, -0.4536011799217368745, -0.2665933059059886201 ) ) ;
#77375=CARTESIAN_POINT ( 'NONE',  ( -0.6889763779527552368, 0.1660481256975885056, 0.3530559997133364547 ) ) ;
#77377=CARTESIAN_POINT ( 'NONE',  ( -0.9580052493438311334, 0.05413385826771626580, -0.4176697321401330321 ) ) ;
#77378=CARTESIAN_POINT ( 'NONE',  ( -1.404199475065615932, -0.3690944881889765550, -0.3153832671262227771 ) ) ;
#77379=ADVANCED_FACE ( 'NONE', ( #31911 ), #38222, .F. ) ;
#77380=CARTESIAN_POINT ( 'NONE',  ( -0.7414698162729651543, -0.5511811023622046335, 0.09757992244046803654 ) ) ;
#77381=CARTESIAN_POINT ( 'NONE',  ( -1.581364829396324945, -0.2845877964562159024, 0.3641732283464567677 ) ) ;
#77382=CARTESIAN_POINT ( 'NONE',  ( 1.410761154855643795, -0.3162353388693405765, 0.4822834645669290543 ) ) ;
#77385=ORIENTED_EDGE ( 'NONE', *, *, #19613, .T. ) ;
#77387=CARTESIAN_POINT ( 'NONE',  ( 1.614173228346457378, 0.1771653543307087630, 0.000000000000000000 ) ) ;
#77388=CARTESIAN_POINT ( 'NONE',  ( -1.437007874015747477, -0.5400638737290844871, 0.3530559997133364547 ) ) ;
#77390=CARTESIAN_POINT ( 'NONE',  ( 1.082677165354331228, -0.5400638737290844871, 0.3530559997133364547 ) ) ;
#77392=CARTESIAN_POINT ( 'NONE',  ( 1.581364829396326277, -0.2845877964562161244, -0.3641732283464567121 ) ) ;
#77393=CARTESIAN_POINT ( 'NONE',  ( 0.6889763779527566800, -0.5400638737290844871, 0.3530559997133364547 ) ) ;
#77394=CARTESIAN_POINT ( 'NONE',  ( 0.09186351706036827158, 0.05413385826771666132, 0.4176697321401328100 ) ) ;
#77397=CARTESIAN_POINT ( 'NONE',  ( 0.7414698162729663755, -0.5511811023622048555, -0.09757992244046775898 ) ) ;
#77399=ORIENTED_EDGE ( 'NONE', *, *, #45400, .F. ) ;
#77402=CARTESIAN_POINT ( 'NONE',  ( 0.1377952755905518800, -0.5400638737290844871, 0.3530559997133364547 ) ) ;
#77403=CARTESIAN_POINT ( 'NONE',  ( -1.496062992125983815, -0.1870078740157479769, 0.4822834645669291653 ) ) ;
#77404=CARTESIAN_POINT ( 'NONE',  ( 0.4593175853018380828, 0.05413385826771626580, -0.4176697321401330321 ) ) ;
#77405=CARTESIAN_POINT ( 'NONE',  ( 1.187664041994751285, -0.05778040916215522460, 0.4822834645669289988 ) ) ;
#77406=CARTESIAN_POINT ( 'NONE',  ( 1.286089238845145033, 0.2306618581243848609, 0.2411417322834645549 ) ) ;
#77407=CARTESIAN_POINT ( 'NONE',  ( -0.6496062992125976043, 0.1660481256975883668, -0.3530559997133364547 ) ) ;
#77408=CARTESIAN_POINT ( 'NONE',  ( 0.1771653543307093182, 0.1660481256975885056, 0.3530559997133364547 ) ) ;
#77409=CARTESIAN_POINT ( 'NONE',  ( -1.476377952755905110, 0.1660481256975885056, 0.3530559997133364547 ) ) ;
#77410=CARTESIAN_POINT ( 'NONE',  ( 1.325459317585302665, 0.05413385826771626580, -0.4176697321401330321 ) ) ;
#77411=CARTESIAN_POINT ( 'NONE',  ( 1.089238845144357759, 0.05413385826771626580, -0.4176697321401330321 ) ) ;
#77412=CARTESIAN_POINT ( 'NONE',  ( -0.2296587926509179312, -0.3162353388693409650, -0.4822834645669289433 ) ) ;
#77414=CARTESIAN_POINT ( 'NONE',  ( 0.6102362204724416372, 0.07958543189024071263, -0.2665933059059888421 ) ) ;
#77417=ORIENTED_EDGE ( 'NONE', *, *, #82130, .T. ) ;
#77418=CARTESIAN_POINT ( 'NONE',  ( -0.3477690288713905509, -0.5511811023622046335, 0.09757992244046803654 ) ) ;
#77422=CARTESIAN_POINT ( 'NONE',  ( 0.2230971128608929543, 0.05413385826771626580, -0.4176697321401330321 ) ) ;
#77423=CARTESIAN_POINT ( 'NONE',  ( 0.2099737532808405305, 0.2306618581243847221, -0.2411417322834647770 ) ) ;
#77424=CARTESIAN_POINT ( 'NONE',  ( -1.049868766404198794, 0.2306618581243847221, -0.2411417322834647770 ) ) ;
#77426=CARTESIAN_POINT ( 'NONE',  ( -1.574803149606298192, -0.1870078740157480879, -0.4822834645669291653 ) ) ;
#77428=CARTESIAN_POINT ( 'NONE',  ( 0.7545931758530188826, -0.5511811023622046335, 0.09757992244046803654 ) ) ;
#77429=CARTESIAN_POINT ( 'NONE',  ( 0.6627296587926517768, -0.6692913385826773087, -0.1292274648535924053 ) ) ;
#77430=CARTESIAN_POINT ( 'NONE',  ( 0.5643044619422579178, 0.05413385826771666132, 0.4176697321401328100 ) ) ;
#77435=CARTESIAN_POINT ( 'NONE',  ( -0.1049868766404193215, 0.2306618581243847221, -0.2411417322834647770 ) ) ;
#77437=( BOUNDED_CURVE ( )  B_SPLINE_CURVE ( 1, ( #38214, #44923 ),
 .UNSPECIFIED., .F., .F. ) 
 B_SPLINE_CURVE_WITH_KNOTS ( ( 2, 2 ),
 ( 0.000000000000000000, 0.001999999999999998307 ),
 .UNSPECIFIED. ) 
 CURVE ( )  GEOMETRIC_REPRESENTATION_ITEM ( )  RATIONAL_B_SPLINE_CURVE ( ( 0.9875488213027527884, 0.9875488213027527884 ) ) 
 REPRESENTATION_ITEM ( '' )  );
#77439=CARTESIAN_POINT ( 'NONE',  ( -0.9973753280839886548, 0.1283753931104748280, 0.1820866141732283561 ) ) ;
#77440=CARTESIAN_POINT ( 'NONE',  ( 1.469816272965879911, 0.2306618581243847221, -0.2411417322834647770 ) ) ;
#77442=CARTESIAN_POINT ( 'NONE',  ( 1.161417322834646493, -0.5400638737290844871, 0.3530559997133364547 ) ) ;
#77443=CARTESIAN_POINT ( 'NONE',  ( 0.3215223097112867578, -0.2845877964562161244, -0.3641732283464567121 ) ) ;
#77444=CARTESIAN_POINT ( 'NONE',  ( 0.6496062992125991586, 0.1660481256975885056, 0.3530559997133364547 ) ) ;
#77446=CARTESIAN_POINT ( 'NONE',  ( 0.4724409448818904789, -0.1870078740157480601, -0.3641732283464567677 ) ) ;
#77447=CARTESIAN_POINT ( 'NONE',  ( 0.1509186351706042484, -0.3162353388693405765, 0.4822834645669290543 ) ) ;
#77449=CARTESIAN_POINT ( 'NONE',  ( -1.384514435695537005, 0.2952755905511811885, 0.1292274648535926551 ) ) ;
#77450=CARTESIAN_POINT ( 'NONE',  ( 0.4461942257217855201, -0.5023911411419708095, 0.1820866141732285504 ) ) ;
#77452=CARTESIAN_POINT ( 'NONE',  ( -0.5839895013123351797, 0.2952755905511810774, -0.1292274648535930714 ) ) ;
#77453=CARTESIAN_POINT ( 'NONE',  ( -0.2755905511811015396, -0.5511811023622047445, 6.969142054262312111E-17 ) ) ;
#77455=CARTESIAN_POINT ( 'NONE',  ( -0.8727034120734901146, -0.05778040916215560624, -0.4822834645669293319 ) ) ;
#77456=CARTESIAN_POINT ( 'NONE',  ( -0.03280839895013062252, 0.2952755905511810774, -0.1292274648535930714 ) ) ;
#77457=CARTESIAN_POINT ( 'NONE',  ( 0.2296587926509192634, -0.08942795157528024563, -0.3641732283464568787 ) ) ;
#77459=CARTESIAN_POINT ( 'NONE',  ( -0.1968503937007867743, 0.2952755905511811885, 0.000000000000000000 ) ) ;
#77461=CARTESIAN_POINT ( 'NONE',  ( 0.6364829396325465405, -0.2845877964562161244, -0.3641732283464567121 ) ) ;
#77462=CARTESIAN_POINT ( 'NONE',  ( 1.312335958005249825, 0.2306618581243847221, -0.2411417322834647770 ) ) ;
#77463=CARTESIAN_POINT ( 'NONE',  ( -0.9776902887139098386, -0.5511811023622046335, 0.09757992244046803654 ) ) ;
#77465=CARTESIAN_POINT ( 'NONE',  ( -1.062992125984250968, 0.1771653543307087630, 0.000000000000000000 ) ) ;
#77466=CARTESIAN_POINT ( 'NONE',  ( -0.5249343832020990641, 0.2306618581243848609, 0.2411417322834645549 ) ) ;
#77467=CARTESIAN_POINT ( 'NONE',  ( -0.006561679790025524116, -0.3162353388693405765, 0.4822834645669290543 ) ) ;
#77468=CARTESIAN_POINT ( 'NONE',  ( 0.7677165354330716118, 0.07958543189024071263, -0.2665933059059888421 ) ) ;
#77470=CARTESIAN_POINT ( 'NONE',  ( 1.062992125984252745, -0.5511811023622047445, 6.969142054262312111E-17 ) ) ;
#77472=CARTESIAN_POINT ( 'NONE',  ( 0.6430446194225729606, -0.4281496062992127816, -0.4176697321401328100 ) ) ;
#77474=CARTESIAN_POINT ( 'NONE',  ( -0.1771653543307080136, -0.5400638737290844871, 0.3530559997133364547 ) ) ;
#77477=CARTESIAN_POINT ( 'NONE',  ( 1.410761154855643795, -0.2845877964562159024, 0.3641732283464567677 ) ) ;
#77478=CARTESIAN_POINT ( 'NONE',  ( 0.2821522309711292364, 0.2952755905511810774, -0.1292274648535930714 ) ) ;
#77480=CARTESIAN_POINT ( 'NONE',  ( -0.06561679790026180015, 0.05413385826771666132, 0.4176697321401328100 ) ) ;
#77481=CARTESIAN_POINT ( 'NONE',  ( 0.5839895013123366230, 0.2066929133858267931, 0.1054918080437490802 ) ) ;
#77482=CARTESIAN_POINT ( 'NONE',  ( -0.05905511811023545637, 0.07958543189024085140, 0.2665933059059887866 ) ) ;
#77483=CARTESIAN_POINT ( 'NONE',  ( 0.6627296587926517768, -0.6692913385826773087, -0.1292274648535924053 ) ) ;
#77484=CARTESIAN_POINT ( 'NONE',  ( -0.3937007874015740483, -0.1870078740157480601, -0.3641732283464567677 ) ) ;
#77485=CARTESIAN_POINT ( 'NONE',  ( -0.5249343832020990641, 0.2306618581243848609, 0.2411417322834645549 ) ) ;
#77486=CARTESIAN_POINT ( 'NONE',  ( 0.7989874411535518028, 0.02791078216816225699, 0.4328096321851905293 ) ) ;
#77487=CARTESIAN_POINT ( 'NONE',  ( -0.1246719160104980823, 0.2952755905511811885, 0.1292274648535926551 ) ) ;
#77488=CARTESIAN_POINT ( 'NONE',  ( -1.227034120734907141, -0.6692913385826773087, -0.1292274648535924053 ) ) ;
#77489=CARTESIAN_POINT ( 'NONE',  ( -0.8858267716535425107, 0.07958543189024071263, -0.2665933059059888421 ) ) ;
#77490=CARTESIAN_POINT ( 'NONE',  ( 0.4199475065616803948, -0.6046776061558809534, -0.2411417322834644161 ) ) ;
#77491=CARTESIAN_POINT ( 'NONE',  ( -1.417322834645668772, -0.1870078740157479769, 0.4822834645669291653 ) ) ;
#77492=CARTESIAN_POINT ( 'NONE',  ( -0.1509186351706028884, -0.3162353388693409650, -0.4822834645669289433 ) ) ;
#77494=CARTESIAN_POINT ( 'NONE',  ( -0.8792650918635160906, 0.05413385826771626580, -0.4176697321401330321 ) ) ;
#77495=CARTESIAN_POINT ( 'NONE',  ( 1.154855643044620184, 0.2306618581243847221, -0.2411417322834647770 ) ) ;
#77496=CARTESIAN_POINT ( 'NONE',  ( 1.443569553805774897, -0.6046776061558809534, -0.2411417322834644161 ) ) ;
#77500=CARTESIAN_POINT ( 'NONE',  ( -1.135170603674539924, -0.6692913385826771977, 0.1292274648535927661 ) ) ;
#77504=CARTESIAN_POINT ( 'NONE',  ( -0.01968503937007793844, 0.07958543189024071263, -0.2665933059059888421 ) ) ;
#77506=ORIENTED_EDGE ( 'NONE', *, *, #54690, .F. ) ;
#77507=CARTESIAN_POINT ( 'NONE',  ( 0.1574803149606306130, -0.1870078740157479769, 0.4822834645669291653 ) ) ;
#77508=CARTESIAN_POINT ( 'NONE',  ( 0.4330708661417329575, -0.6692913385826771977, 8.415575281601705876E-17 ) ) ;
#77510=CARTESIAN_POINT ( 'NONE',  ( -0.5408419829024493364, -1.094630224652485432E-15, 0.4281993546915541238 ) ) ;
#77511=CARTESIAN_POINT ( 'NONE',  ( -0.4790026246719152336, -0.08942795157528024563, -0.3641732283464568787 ) ) ;
#77513=CARTESIAN_POINT ( 'NONE',  ( 0.7480314960629927956, 0.2952755905511811885, 0.000000000000000000 ) ) ;
#77514=CARTESIAN_POINT ( 'NONE',  ( 0.8923884514435701520, -0.5023911411419708095, -0.1820866141732282451 ) ) ;
#77515=CARTESIAN_POINT ( 'NONE',  ( -0.2230971128608915943, 0.05413385826771666132, 0.4176697321401328100 ) ) ;
#77517=CARTESIAN_POINT ( 'NONE',  ( -0.7020997375328074108, -0.05778040916215522460, 0.4822834645669289988 ) ) ;
#77518=CARTESIAN_POINT ( 'NONE',  ( -1.227034120734907585, 0.1771653543307087630, 0.09757992244046791164 ) ) ;
#77519=CARTESIAN_POINT ( 'NONE',  ( -1.043307086614172707, 0.1660481256975883668, -0.3530559997133364547 ) ) ;
#77520=CARTESIAN_POINT ( 'NONE',  ( 1.318897637795276356, -0.5400638737290844871, 0.3530559997133364547 ) ) ;
#77522=VERTEX_POINT ( 'NONE', #52085 ) ;
#77524=CARTESIAN_POINT ( 'NONE',  ( -0.07217847769028787330, -0.05778040916215522460, 0.4822834645669289988 ) ) ;
#77526=CARTESIAN_POINT ( 'NONE',  ( -0.5971128608923877978, 0.2952755905511811885, 0.1292274648535926551 ) ) ;
#77527=CARTESIAN_POINT ( 'NONE',  ( 1.489501312335958172, -0.05778040916215560624, -0.4822834645669293319 ) ) ;
#77528=CARTESIAN_POINT ( 'NONE',  ( 1.062992125984252745, -0.6692913385826771977, 8.415575281601705876E-17 ) ) ;
#77530=CARTESIAN_POINT ( 'NONE',  ( 0.2427821522309716595, -0.3162353388693409650, -0.4822834645669289433 ) ) ;
#77531=CARTESIAN_POINT ( 'NONE',  ( 0.01312335958005323398, -0.4281496062992127816, -0.4176697321401328100 ) ) ;
#77533=CARTESIAN_POINT ( 'NONE',  ( -1.213910761154854745, 0.2952755905511810774, -0.1292274648535930714 ) ) ;
#77534=CARTESIAN_POINT ( 'NONE',  ( -0.3740157480314953431, 0.1660481256975885056, 0.3530559997133364547 ) ) ;
#77535=CARTESIAN_POINT ( 'NONE',  ( -0.3018372703412066094, -0.3690944881889765550, -0.3153832671262227771 ) ) ;
#77537=CARTESIAN_POINT ( 'NONE',  ( 1.332020997375329197, -0.3162353388693405765, 0.4822834645669290543 ) ) ;
#77538=CARTESIAN_POINT ( 'NONE',  ( -0.6955380577427815458, -0.4281496062992127816, -0.4176697321401328100 ) ) ;
#77539=CARTESIAN_POINT ( 'NONE',  ( 0.2559055118110243887, 0.1012011053420777407, 0.2882089793578256898 ) ) ;
#77540=CARTESIAN_POINT ( 'NONE',  ( 1.010498687664042716, 0.05413385826771626580, -0.4176697321401330321 ) ) ;
#77545=CARTESIAN_POINT ( 'NONE',  ( 0.3149606299212606708, -0.1870078740157480879, -0.4822834645669291653 ) ) ;
#77546=CARTESIAN_POINT ( 'NONE',  ( -0.4986876640419942164, -0.5023911411419708095, 0.1820866141732285504 ) ) ;
#77549=CARTESIAN_POINT ( 'NONE',  ( 1.463254593175853824, -0.5511811023622046335, 0.09757992244046803654 ) ) ;
#77553=CARTESIAN_POINT ( 'NONE',  ( 1.410761154855643795, -0.3162353388693405765, 0.4822834645669290543 ) ) ;
#77555=CARTESIAN_POINT ( 'NONE',  ( 0.05249343832021075018, 0.2306618581243847221, -0.2411417322834647770 ) ) ;
#77556=CARTESIAN_POINT ( 'NONE',  ( -1.568241469816272105, -0.3162353388693409650, -0.4822834645669289433 ) ) ;
#77557=CARTESIAN_POINT ( 'NONE',  ( -1.587926509186350810, -0.4281496062992124485, 0.4176697321401328655 ) ) ;
#77558=CARTESIAN_POINT ( 'NONE',  ( 0.3608923884514443348, 0.2952755905511810774, -0.1292274648535930714 ) ) ;
#77560=CARTESIAN_POINT ( 'NONE',  ( 1.528871391076116026, 0.2952755905511811885, 0.1292274648535926551 ) ) ;
#77561=CARTESIAN_POINT ( 'NONE',  ( 0.6299212598425204535, -0.1870078740157479769, 0.4822834645669291653 ) ) ;
#77562=CARTESIAN_POINT ( 'NONE',  ( 0.8464566929133866546, -0.4536011799217367080, 0.2665933059059888421 ) ) ;
#77563=CARTESIAN_POINT ( 'NONE',  ( -0.01968503937007793844, 0.1660481256975883391, -0.3530559997133364547 ) ) ;
#77564=CARTESIAN_POINT ( 'NONE',  ( 0.8267716535433078384, -0.5511811023622047445, 6.969142054262312111E-17 ) ) ;
#77565=CARTESIAN_POINT ( 'NONE',  ( -1.246719160104985846, -0.4281496062992127816, -0.4176697321401328100 ) ) ;
#77567=CARTESIAN_POINT ( 'NONE',  ( 1.174540682414699111, -0.3162353388693405765, 0.4822834645669290543 ) ) ;
#77569=CARTESIAN_POINT ( 'NONE',  ( 0.8136482939632553313, -0.6046776061558809534, -0.2411417322834644161 ) ) ;
#77571=CARTESIAN_POINT ( 'NONE',  ( -0.3543307086614165824, 0.2066929133858268208, 0.000000000000000000 ) ) ;
#77572=CARTESIAN_POINT ( 'NONE',  ( 0.2952755905511816326, -0.4536011799217367080, 0.2665933059059888421 ) ) ;
#77573=ADVANCED_FACE ( 'NONE', ( #18870 ), #35444, .F. ) ;
#77574=CARTESIAN_POINT ( 'NONE',  ( 0.4396325459317593221, 0.2952755905511810774, -0.1292274648535930714 ) ) ;
#77576=CARTESIAN_POINT ( 'NONE',  ( -0.8333333333333323711, -0.5511811023622048555, -0.09757992244046775898 ) ) ;
#77577=CARTESIAN_POINT ( 'NONE',  ( -1.089238845144356427, 0.05413385826771666132, 0.4176697321401328100 ) ) ;
#77578=CARTESIAN_POINT ( 'NONE',  ( 0.9711286089238851948, -0.6046776061558809534, -0.2411417322834644161 ) ) ;
#77579=CARTESIAN_POINT ( 'NONE',  ( -1.056430446194224881, 0.2952755905511810774, -0.1292274648535930714 ) ) ;
#77580=CARTESIAN_POINT ( 'NONE',  ( 0.8202099737532814183, -0.6692913385826773087, -0.1292274648535924053 ) ) ;
#77581=CARTESIAN_POINT ( 'NONE',  ( -1.233595800524933894, -0.5023911411419708095, -0.1820866141732282451 ) ) ;
#77583=CARTESIAN_POINT ( 'NONE',  ( 1.010498687664042716, 0.05413385826771626580, -0.4176697321401330321 ) ) ;
#77586=CARTESIAN_POINT ( 'NONE',  ( 1.515748031496063408, 0.1660481256975885056, 0.3530559997133364547 ) ) ;
#77587=CARTESIAN_POINT ( 'NONE',  ( -1.102362204724408601, -0.1870078740157479769, 0.3641732283464567677 ) ) ;
#77588=CARTESIAN_POINT ( 'NONE',  ( 1.169606216052559544, -4.479759449472349425E-16, -0.3791483426435169335 ) ) ;
#77589=CARTESIAN_POINT ( 'NONE',  ( -1.174540682414697335, -0.08942795157527998196, 0.3641732283464567121 ) ) ;
#77590=CARTESIAN_POINT ( 'NONE',  ( -0.3740157480314953431, 0.07958543189024085140, 0.2665933059059887866 ) ) ;
#77591=CARTESIAN_POINT ( 'NONE',  ( -1.732283464566928277, -0.1870078740157479769, 0.3641732283464567677 ) ) ;
#77592=CARTESIAN_POINT ( 'NONE',  ( 1.017060367454068581, -0.08942795157528024563, -0.3641732283464568787 ) ) ;
#77593=CARTESIAN_POINT ( 'NONE',  ( 0.6692913385826778638, -0.6692913385826771977, 8.415575281601705876E-17 ) ) ;
#77594=CARTESIAN_POINT ( 'NONE',  ( 1.095800524934383846, -0.3162353388693405765, 0.4822834645669290543 ) ) ;
#77595=CARTESIAN_POINT ( 'NONE',  ( -0.05249343832020911260, 0.2306618581243848609, 0.2411417322834645549 ) ) ;
#77596=CARTESIAN_POINT ( 'NONE',  ( 0.6364829396325465405, -0.08942795157527998196, 0.3641732283464567121 ) ) ;
#77598=CARTESIAN_POINT ( 'NONE',  ( 1.541994750656168645, -0.6692913385826771977, 0.1292274648535927661 ) ) ;
#77599=DIRECTION ( 'NONE',  ( -0.000000000000000000, -1.000000000000000000, -0.000000000000000000 ) ) ;
#77600=CARTESIAN_POINT ( 'NONE',  ( -0.6692913385826764205, -0.6692913385826771977, 8.415575281601705876E-17 ) ) ;
#77602=DIRECTION ( 'NONE',  ( -3.096699300667737957E-16, 1.000000000000000000, -0.000000000000000000 ) ) ;
#77603=CARTESIAN_POINT ( 'NONE',  ( -0.1049868766404193215, 0.2306618581243847221, -0.2411417322834647770 ) ) ;
#77605=CARTESIAN_POINT ( 'NONE',  ( -0.3740157480314953431, 0.1660481256975885056, 0.3530559997133364547 ) ) ;
#77606=CARTESIAN_POINT ( 'NONE',  ( 0.4002624671916016896, -0.3162353388693409650, -0.4822834645669289433 ) ) ;
#77612=CARTESIAN_POINT ( 'NONE',  ( -0.7480314960629914633, 0.1771653543307087630, 0.000000000000000000 ) ) ;
#77614=CARTESIAN_POINT ( 'NONE',  ( -1.115485564304461219, -0.4281496062992124485, 0.4176697321401328655 ) ) ;
#77616=CARTESIAN_POINT ( 'NONE',  ( 0.5118110236220480003, -0.6692913385826771977, 8.415575281601705876E-17 ) ) ;
#77617=CARTESIAN_POINT ( 'NONE',  ( -0.06561679790026180015, -0.3690944881889765550, -0.3153832671262227771 ) ) ;
#77618=CARTESIAN_POINT ( 'NONE',  ( 1.351706036745407458, -0.4281496062992127816, -0.4176697321401328100 ) ) ;
#77619=CARTESIAN_POINT ( 'NONE',  ( 0.3083989501312343062, -0.3162353388693405765, 0.4822834645669290543 ) ) ;
#77620=CARTESIAN_POINT ( 'NONE',  ( -1.614173228346457378, 1.881821177735609085, 0.1372047244094476981 ) ) ;
#77623=CARTESIAN_POINT ( 'NONE',  ( 1.135170603674541256, -0.6692913385826773087, -0.1292274648535924053 ) ) ;
#77624=CARTESIAN_POINT ( 'NONE',  ( 0.4527559055118117182, -0.5400638737290844871, 0.3530559997133364547 ) ) ;
#77625=CARTESIAN_POINT ( 'NONE',  ( 0.1771653543307093182, 0.1660481256975885056, 0.3530559997133364547 ) ) ;
#77626=CARTESIAN_POINT ( 'NONE',  ( 0.9645669291338588858, 0.07958543189024085140, 0.2665933059059887866 ) ) ;
#77627=CARTESIAN_POINT ( 'NONE',  ( 1.496062992125985147, -0.1870078740157479769, 0.4822834645669291653 ) ) ;
#77629=CARTESIAN_POINT ( 'NONE',  ( 0.1509186351706042484, -0.3162353388693405765, 0.4822834645669290543 ) ) ;
#77630=CARTESIAN_POINT ( 'NONE',  ( 0.8661417322834653598, -0.1870078740157479769, 0.4822834645669291653 ) ) ;
#77631=CARTESIAN_POINT ( 'NONE',  ( 0.2887139107611556010, 0.2306618581243847221, -0.2411417322834647770 ) ) ;
#77632=CARTESIAN_POINT ( 'NONE',  ( 1.351706036745407680, -0.004921259842519576551, 0.3153832671262227771 ) ) ;
#77633=CARTESIAN_POINT ( 'NONE',  ( -0.8136482939632537770, -0.6046776061558807314, 0.2411417322834647770 ) ) ;
#77634=CARTESIAN_POINT ( 'NONE',  ( -1.272965879265091305, -0.4281496062992124485, 0.4176697321401328655 ) ) ;
#77635=CARTESIAN_POINT ( 'NONE',  ( 1.141732283464567566, 0.2952755905511811885, 0.000000000000000000 ) ) ;
#77636=CARTESIAN_POINT ( 'NONE',  ( -0.7137454485294950635, 2.362204724409448620, -0.4917280318828581298 ) ) ;
#77638=CARTESIAN_POINT ( 'NONE',  ( 1.548556430446194954, 0.2306618581243847221, -0.2411417322834647770 ) ) ;
#77642=CARTESIAN_POINT ( 'NONE',  ( 1.535433070866142558, 0.2952755905511811885, 0.000000000000000000 ) ) ;
#77643=CARTESIAN_POINT ( 'NONE',  ( 0.7545931758530188826, -0.5511811023622046335, 0.09757992244046803654 ) ) ;
#77646=CARTESIAN_POINT ( 'NONE',  ( 0.7749820319012125092, 2.784432375088962958E-17, -0.3464511005275205946 ) ) ;
#77648=CARTESIAN_POINT ( 'NONE',  ( -1.095800524934382292, -0.2845877964562161244, -0.3641732283464567121 ) ) ;
#77649=CARTESIAN_POINT ( 'NONE',  ( -1.627296587926508442, -0.5023911411419708095, -0.1820866141732282451 ) ) ;
#77650=CARTESIAN_POINT ( 'NONE',  ( -1.522309711286088607, -0.6046776061558807314, 0.2411417322834647770 ) ) ;
#77651=CARTESIAN_POINT ( 'NONE',  ( -0.2427821522309703550, -0.05778040916215560624, -0.4822834645669293319 ) ) ;
#77652=CARTESIAN_POINT ( 'NONE',  ( 1.541994750656168645, -0.6692913385826771977, 0.1292274648535927661 ) ) ;
#77653=ORIENTED_EDGE ( 'NONE', *, *, #72813, .F. ) ;
#77656=CARTESIAN_POINT ( 'NONE',  ( -1.614173228346457378, 0.7794589730111965986, 0.1372047244094476981 ) ) ;
#77658=CARTESIAN_POINT ( 'NONE',  ( -1.115485564304461219, -0.004921259842519870586, -0.3153832671262229437 ) ) ;
#77659=ADVANCED_FACE ( 'NONE', ( #12984 ), #38640, .F. ) ;
#77660=CARTESIAN_POINT ( 'NONE',  ( -1.535433070866141225, -0.6692913385826771977, 8.415575281601705876E-17 ) ) ;
#77661=CARTESIAN_POINT ( 'NONE',  ( 0.4658792650918641698, -0.05778040916215560624, -0.4822834645669293319 ) ) ;
#77664=CYLINDRICAL_SURFACE ( 'NONE', #31738, 1.181102362204724310 ) ;
#77665=CARTESIAN_POINT ( 'NONE',  ( 1.292650918635171564, -0.6692913385826773087, -0.1292274648535924053 ) ) ;
#77666=CARTESIAN_POINT ( 'NONE',  ( -1.673228346456691717, 0.1660481256975883668, -0.3530559997133364547 ) ) ;
#77669=CARTESIAN_POINT ( 'NONE',  ( -0.2427821522309703550, -0.08942795157528024563, -0.3641732283464568787 ) ) ;
#77670=CARTESIAN_POINT ( 'NONE',  ( -1.430446194225720724, -0.004921259842519870586, -0.3153832671262229437 ) ) ;
#77672=CARTESIAN_POINT ( 'NONE',  ( 0.3280839895013130669, 0.05413385826771666132, 0.4176697321401328100 ) ) ;
#77673=CARTESIAN_POINT ( 'NONE',  ( -0.3740157480314953431, 0.07958543189024085140, 0.2665933059059887866 ) ) ;
#77674=CARTESIAN_POINT ( 'NONE',  ( 0.07874015748031558404, -0.1870078740157480601, -0.3641732283464567677 ) ) ;
#77675=CARTESIAN_POINT ( 'NONE',  ( -0.02624671916010428221, -0.6046776061558807314, 0.2411417322834647770 ) ) ;
#77676=CARTESIAN_POINT ( 'NONE',  ( -1.017060367454067249, -0.08942795157527998196, 0.3641732283464567121 ) ) ;
#77678=CARTESIAN_POINT ( 'NONE',  ( 0.8923884514435701520, -0.6046776061558809534, -0.2411417322834644161 ) ) ;
#77679=CARTESIAN_POINT ( 'NONE',  ( -1.561679790026246017, -0.4281496062992127816, -0.4176697321401328100 ) ) ;
#77681=CARTESIAN_POINT ( 'NONE',  ( -0.4265091863517051496, 0.2952755905511810774, -0.1292274648535930714 ) ) ;
#77682=CARTESIAN_POINT ( 'NONE',  ( 0.2690288713910767848, -0.5511811023622048555, -0.09757992244046775898 ) ) ;
#77683=CARTESIAN_POINT ( 'NONE',  ( -0.7349081364829387342, -0.6046776061558807314, 0.2411417322834647770 ) ) ;
#77684=CARTESIAN_POINT ( 'NONE',  ( 0.7808398950131241190, -0.08942795157528024563, -0.3641732283464568787 ) ) ;
#77685=CARTESIAN_POINT ( 'NONE',  ( -0.1181102362204717315, 0.1771653543307087630, 0.000000000000000000 ) ) ;
#77686=CARTESIAN_POINT ( 'NONE',  ( -0.7217847769028863381, 0.05413385826771626580, -0.4176697321401330321 ) ) ;
#77687=CARTESIAN_POINT ( 'NONE',  ( -1.482939632545930975, 0.05413385826771666132, 0.4176697321401328100 ) ) ;
#77688=LINE ( 'NONE', #56644, #36684 ) ;
#77689=CARTESIAN_POINT ( 'NONE',  ( 1.286089238845145033, -0.5023911411419708095, -0.1820866141732282451 ) ) ;
#77690=CARTESIAN_POINT ( 'NONE',  ( 0.5905511811023629321, 0.2952755905511811885, 0.000000000000000000 ) ) ;
#77691=CARTESIAN_POINT ( 'NONE',  ( -1.423884514435694859, -0.05778040916215560624, -0.4822834645669293319 ) ) ;
#77692=CARTESIAN_POINT ( 'NONE',  ( -1.463254593175852492, -0.6692913385826773087, -0.1292274648535924053 ) ) ;
#77695=CARTESIAN_POINT ( 'NONE',  ( -0.9711286089238838626, 0.1283753931104746893, -0.1820866141732285504 ) ) ;
#77696=CARTESIAN_POINT ( 'NONE',  ( 0.5905511811023629321, -0.6692913385826771977, 8.415575281601705876E-17 ) ) ;
#77697=CARTESIAN_POINT ( 'NONE',  ( -1.089238845144356427, -0.004921259842519576551, 0.3153832671262227771 ) ) ;
#77699=CARTESIAN_POINT ( 'NONE',  ( -1.036745406824146176, 0.05413385826771626580, -0.4176697321401330321 ) ) ;
#77700=CARTESIAN_POINT ( 'NONE',  ( 1.069553805774278832, 0.2952755905511810774, -0.1292274648535930714 ) ) ;
#77701=CARTESIAN_POINT ( 'NONE',  ( 0.3608923884514443348, -0.6692913385826771977, 0.1292274648535927661 ) ) ;
#77702=CARTESIAN_POINT ( 'NONE',  ( 1.496062992125984703, -0.1870078740157480879, -0.4822834645669291653 ) ) ;
#77703=CARTESIAN_POINT ( 'NONE',  ( -1.673228346456691717, 0.07958543189024071263, -0.2665933059059888421 ) ) ;
#77708=CARTESIAN_POINT ( 'NONE',  ( 0.9120734908136490793, 0.1771653543307087075, -0.09757992244046823083 ) ) ;
#77709=CARTESIAN_POINT ( 'NONE',  ( 0.4986876640419954376, 0.1283753931104748280, 0.1820866141732283561 ) ) ;
#77710=CARTESIAN_POINT ( 'NONE',  ( -0.07217847769028813698, -0.3162353388693409650, -0.4822834645669289433 ) ) ;
#77711=CARTESIAN_POINT ( 'NONE',  ( 1.154855643044620184, 0.2306618581243847221, -0.2411417322834647770 ) ) ;
#77713=CARTESIAN_POINT ( 'NONE',  ( 0.5183727034120741983, -0.5511811023622046335, 0.09757992244046803654 ) ) ;
#77714=CARTESIAN_POINT ( 'NONE',  ( -0.7020997375328074108, -0.05778040916215522460, 0.4822834645669289988 ) ) ;
#77715=CARTESIAN_POINT ( 'NONE',  ( -1.345144356955379816, -0.3162353388693405765, 0.4822834645669290543 ) ) ;
#77716=CARTESIAN_POINT ( 'NONE',  ( 0.8202099737532814183, -0.6692913385826773087, -0.1292274648535924053 ) ) ;
#77722=CARTESIAN_POINT ( 'NONE',  ( -1.397637795275589623, 0.1660481256975885056, 0.3530559997133364547 ) ) ;
#77723=CARTESIAN_POINT ( 'NONE',  ( -0.6824146981627288167, 0.2306618581243848609, 0.2411417322834645549 ) ) ;
#77724=CARTESIAN_POINT ( 'NONE',  ( -0.8202099737532799750, 0.1771653543307087075, -0.09757992244046823083 ) ) ;
#77725=CARTESIAN_POINT ( 'NONE',  ( -0.7349081364829387342, -0.6046776061558807314, 0.2411417322834647770 ) ) ;
#77728=CARTESIAN_POINT ( 'NONE',  ( 1.548556430446194954, 0.2306618581243847221, -0.2411417322834647770 ) ) ;
#77729=CARTESIAN_POINT ( 'NONE',  ( -1.312335958005248715, -0.6046776061558809534, -0.2411417322834644161 ) ) ;
#77730=CARTESIAN_POINT ( 'NONE',  ( 0.3215223097112867578, -0.05778040916215522460, 0.4822834645669289988 ) ) ;
#77731=CARTESIAN_POINT ( 'NONE',  ( -0.8923884514435688198, -0.6046776061558807314, 0.2411417322834647770 ) ) ;
#77732=CARTESIAN_POINT ( 'NONE',  ( 0.8005249343832027131, 0.05413385826771666132, 0.4176697321401328100 ) ) ;
#77734=CARTESIAN_POINT ( 'NONE',  ( -0.7349081364829387342, -0.5023911411419708095, 0.1820866141732285504 ) ) ;
#77735=ORIENTED_EDGE ( 'NONE', *, *, #63775, .T. ) ;
#77737=ORIENTED_EDGE ( 'NONE', *, *, #49126, .T. ) ;
#77738=CARTESIAN_POINT ( 'NONE',  ( -1.646981627296586703, -0.2845877964562161244, -0.3641732283464567121 ) ) ;
#77739=CARTESIAN_POINT ( 'NONE',  ( -1.305774278215222184, -0.6692913385826773087, -0.1292274648535924053 ) ) ;
#77740=CARTESIAN_POINT ( 'NONE',  ( -1.332020997375327642, -0.05778040916215522460, 0.4822834645669289988 ) ) ;
#77742=CARTESIAN_POINT ( 'NONE',  ( -1.043307086614172707, 0.1660481256975883668, -0.3530559997133364547 ) ) ;
#77743=CARTESIAN_POINT ( 'NONE',  ( -1.404199475065615932, 0.05413385826771666132, 0.4176697321401328100 ) ) ;
#77744=CARTESIAN_POINT ( 'NONE',  ( -1.377952755905511140, -0.6692913385826771977, 8.415575281601705876E-17 ) ) ;
#77745=CARTESIAN_POINT ( 'NONE',  ( -0.3826031302655962807, -4.992347309556208597E-15, 0.3954985857520076920 ) ) ;
#77746=CARTESIAN_POINT ( 'NONE',  ( -0.8561328129276786214, -2.191421614605370878E-15, 0.4445507791589071167 ) ) ;
#77747=CARTESIAN_POINT ( 'NONE',  ( 0.2887139107611556010, 0.1283753931104746893, -0.1820866141732285504 ) ) ;
#77750=CARTESIAN_POINT ( 'NONE',  ( -0.2821522309711278487, 0.1771653543307087630, 0.09757992244046791164 ) ) ;
#77751=CARTESIAN_POINT ( 'NONE',  ( -0.7611548556430438595, -0.6046776061558809534, -0.2411417322834644161 ) ) ;
#77752=CARTESIAN_POINT ( 'NONE',  ( 1.187664041994751285, -0.3162353388693409650, -0.4822834645669289433 ) ) ;
#77753=CARTESIAN_POINT ( 'NONE',  ( -0.3937007874015740483, -0.1870078740157479769, 0.4822834645669291653 ) ) ;
#77757=CARTESIAN_POINT ( 'NONE',  ( -1.017060367454067249, -0.05778040916215522460, 0.4822834645669289988 ) ) ;
#77758=CARTESIAN_POINT ( 'NONE',  ( 1.272965879265092637, 0.05413385826771666132, 0.4176697321401328100 ) ) ;
#77765=CARTESIAN_POINT ( 'NONE',  ( -0.3280839895013117347, 0.05413385826771626580, -0.4176697321401330321 ) ) ;
#77766=CARTESIAN_POINT ( 'NONE',  ( -1.594488188976377119, 0.07958543189024071263, -0.2665933059059888421 ) ) ;
#77767=CARTESIAN_POINT ( 'NONE',  ( -0.6364829396325453192, -0.3162353388693405765, 0.4822834645669290543 ) ) ;
#77769=CARTESIAN_POINT ( 'NONE',  ( -1.430446194225721390, -0.4281496062992124485, 0.4176697321401328655 ) ) ;
#77771=CARTESIAN_POINT ( 'NONE',  ( -0.8727034120734901146, -0.05778040916215560624, -0.4822834645669293319 ) ) ;
#77772=CARTESIAN_POINT ( 'NONE',  ( -0.4002624671916004129, -0.05778040916215560624, -0.4822834645669293319 ) ) ;
#77774=CARTESIAN_POINT ( 'NONE',  ( 0.9383202099737536495, -0.2845877964562159024, 0.3641732283464567677 ) ) ;
#77775=DIRECTION ( 'NONE',  ( 0.000000000000000000, 1.000000000000000000, 0.000000000000000000 ) ) ;
#77776=CARTESIAN_POINT ( 'NONE',  ( 0.7152230971128616943, -0.08942795157527998196, 0.3641732283464567121 ) ) ;
#77777=CARTESIAN_POINT ( 'NONE',  ( 1.246719160104987623, -0.3690944881889763329, 0.3153832671262228327 ) ) ;
#77778=CARTESIAN_POINT ( 'NONE',  ( 1.318897637795276356, 0.1660481256975883668, -0.3530559997133364547 ) ) ;
#77779=CARTESIAN_POINT ( 'NONE',  ( 0.09842519685039434474, 0.07958543189024085140, 0.2665933059059887866 ) ) ;
#77781=CARTESIAN_POINT ( 'NONE',  ( -1.010498687664041384, 0.05413385826771666132, 0.4176697321401328100 ) ) ;
#77782=CARTESIAN_POINT ( 'NONE',  ( 1.089238845144357537, -0.4281496062992124485, 0.4176697321401328655 ) ) ;
#77785=CARTESIAN_POINT ( 'NONE',  ( -0.6627296587926501115, 0.1771653543307087075, -0.09757992244046823083 ) ) ;
#77786=CARTESIAN_POINT ( 'NONE',  ( 0.01968503937007930540, 0.1660481256975885056, 0.3530559997133364547 ) ) ;
#77787=CARTESIAN_POINT ( 'NONE',  ( 0.2034120734908144990, -0.6692913385826771977, 0.1292274648535927661 ) ) ;
#77789=CARTESIAN_POINT ( 'NONE',  ( 0.9711286089238851948, 0.1283753931104748280, 0.1820866141732283561 ) ) ;
#77790=CARTESIAN_POINT ( 'NONE',  ( -0.006561679790025524116, -0.2845877964562159024, 0.3641732283464567677 ) ) ;
#77791=CARTESIAN_POINT ( 'NONE',  ( -0.4265091863517051496, -0.6692913385826771977, 0.1292274648535927661 ) ) ;
#77792=CARTESIAN_POINT ( 'NONE',  ( -1.548556430446193399, 0.2306618581243848609, 0.2411417322834645549 ) ) ;
#77793=CARTESIAN_POINT ( 'NONE',  ( -0.7283464566929126471, -0.4536011799217367080, 0.2665933059059888421 ) ) ;
#77796=CARTESIAN_POINT ( 'NONE',  ( 0.4921259842519691285, -0.5400638737290845981, -0.3530559997133363437 ) ) ;
#77797=CARTESIAN_POINT ( 'NONE',  ( -1.043307086614172041, -0.5400638737290844871, 0.3530559997133364547 ) ) ;
#77800=CARTESIAN_POINT ( 'NONE',  ( 0.1443569553805781891, -0.3690944881889763329, 0.3153832671262228327 ) ) ;
#77801=CARTESIAN_POINT ( 'NONE',  ( -0.6364829396325453192, -0.05778040916215560624, -0.4822834645669293319 ) ) ;
#77802=CARTESIAN_POINT ( 'NONE',  ( -0.9317585301837263412, -0.4281496062992127816, -0.4176697321401328100 ) ) ;
#77803=CARTESIAN_POINT ( 'NONE',  ( -1.200787401574802349, -0.4536011799217367080, 0.2665933059059888421 ) ) ;
#77806=CARTESIAN_POINT ( 'NONE',  ( -1.010498687664041384, -0.004921259842519576551, 0.3153832671262227771 ) ) ;
#77807=CARTESIAN_POINT ( 'NONE',  ( -0.7746288504648931594, 0.004960608223778823628, 0.3437734562760190182 ) ) ;
#77808=CARTESIAN_POINT ( 'NONE',  ( 1.371391076115485719, -0.6692913385826773087, -0.1292274648535924053 ) ) ;
#77811=ORIENTED_EDGE ( 'NONE', *, *, #22324, .T. ) ;
#77813=CARTESIAN_POINT ( 'NONE',  ( 1.568241469816273437, -0.2845877964562159024, 0.3641732283464567677 ) ) ;
#77814=CARTESIAN_POINT ( 'NONE',  ( -1.364829396325458521, 0.2306618581243847221, -0.2411417322834647770 ) ) ;
#77815=CARTESIAN_POINT ( 'NONE',  ( 1.213910761154856299, -0.6692913385826773087, -0.1292274648535924053 ) ) ;
#77817=CARTESIAN_POINT ( 'NONE',  ( 1.627296587926509996, -0.5023911411419708095, 0.1820866141732285504 ) ) ;
#77819=CARTESIAN_POINT ( 'NONE',  ( 0.3805774278215230400, -0.4281496062992124485, 0.4176697321401328655 ) ) ;
#77820=CARTESIAN_POINT ( 'NONE',  ( -0.1771653543307080136, 0.1660481256975883668, -0.3530559997133364547 ) ) ;
#77822=DIRECTION ( 'NONE',  ( 0.000000000000000000, -1.000000000000000000, 0.000000000000000000 ) ) ;
#77823=CARTESIAN_POINT ( 'NONE',  ( 0.6889763779527563470, 0.07958543189024071263, -0.2665933059059888421 ) ) ;
#77825=EDGE_LOOP ( 'NONE', ( #20890, #65554, #58974, #31775 ) ) ;
#77828=CARTESIAN_POINT ( 'NONE',  ( 0.1115485564304467270, -0.6692913385826773087, -0.1292274648535924053 ) ) ;
#77829=CARTESIAN_POINT ( 'NONE',  ( 1.135170603674541256, 0.2952755905511811885, 0.1292274648535926551 ) ) ;
#77830=CARTESIAN_POINT ( 'NONE',  ( 0.7283464566929143125, 0.1660481256975885056, 0.3530559997133364547 ) ) ;
#77831=CARTESIAN_POINT ( 'NONE',  ( 1.312335958005250269, -0.6046776061558807314, 0.2411417322834647770 ) ) ;
#77832=CARTESIAN_POINT ( 'NONE',  ( -0.3346456692913377662, 0.1660481256975883668, -0.3530559997133364547 ) ) ;
#77833=CARTESIAN_POINT ( 'NONE',  ( 0.09842519685039434474, -0.5400638737290845981, -0.3530559997133363437 ) ) ;
#77834=CARTESIAN_POINT ( 'NONE',  ( -1.502624671916009680, -0.3162353388693405765, 0.4822834645669290543 ) ) ;
#77835=CARTESIAN_POINT ( 'NONE',  ( 1.246719160104987623, -0.4281496062992124485, 0.4176697321401328655 ) ) ;
#77837=CARTESIAN_POINT ( 'NONE',  ( 1.299212598425197429, -0.6692913385826771977, 8.415575281601705876E-17 ) ) ;
#77839=CARTESIAN_POINT ( 'NONE',  ( 0.2690288713910767848, 0.1771653543307087630, 0.09757992244046791164 ) ) ;
#77842=ORIENTED_EDGE ( 'NONE', *, *, #80522, .F. ) ;
#77843=CARTESIAN_POINT ( 'NONE',  ( -0.2559055118110230564, 0.07958543189024071263, -0.2665933059059888421 ) ) ;
#77844=CARTESIAN_POINT ( 'NONE',  ( -0.01312335958005186876, 0.05413385826771626580, -0.4176697321401330321 ) ) ;
#77846=CARTESIAN_POINT ( 'NONE',  ( -0.02624671916010428221, -0.6046776061558807314, 0.2411417322834647770 ) ) ;
#77847=CARTESIAN_POINT ( 'NONE',  ( 0.05249343832021075018, 0.2306618581243847221, -0.2411417322834647770 ) ) ;
#77848=CARTESIAN_POINT ( 'NONE',  ( -1.062992125984250968, 0.2952755905511811885, 0.000000000000000000 ) ) ;
#77849=CARTESIAN_POINT ( 'NONE',  ( 1.207349081364829990, 0.1283753931104748280, 0.1820866141732283561 ) ) ;
#77851=LINE ( 'NONE', #51306, #8834 ) ;
#77852=CARTESIAN_POINT ( 'NONE',  ( 1.049868766404200127, -0.5023911411419708095, -0.1820866141732282451 ) ) ;
#77853=CARTESIAN_POINT ( 'NONE',  ( 0.2690288713910767848, 0.2952755905511811885, 0.1292274648535926551 ) ) ;
#77854=CARTESIAN_POINT ( 'NONE',  ( 0.7152230971128616943, -0.05778040916215522460, 0.4822834645669289988 ) ) ;
#77856=CARTESIAN_POINT ( 'NONE',  ( -1.686351706036744558, 0.2952755905511810774, -0.1292274648535930714 ) ) ;
#77859=CARTESIAN_POINT ( 'NONE',  ( -0.03280839895013062252, -0.6692913385826771977, 0.1292274648535927661 ) ) ;
#77862=CARTESIAN_POINT ( 'NONE',  ( -1.056430446194224881, -0.5511811023622046335, 0.09757992244046803654 ) ) ;
#77863=CARTESIAN_POINT ( 'NONE',  ( 1.122047244094488860, 0.1660481256975885056, 0.3530559997133364547 ) ) ;
#77864=CARTESIAN_POINT ( 'NONE',  ( 1.404199475065617708, 0.05413385826771626580, -0.4176697321401330321 ) ) ;
#77865=CARTESIAN_POINT ( 'NONE',  ( -0.09186351706036663400, -0.3690944881889763329, 0.3153832671262228327 ) ) ;
#77866=CARTESIAN_POINT ( 'NONE',  ( 0.6102362204724416372, -0.5400638737290844871, 0.3530559997133364547 ) ) ;
#77868=CARTESIAN_POINT ( 'NONE',  ( 0.2427821522309719648, -0.08942795157527998196, 0.3641732283464567121 ) ) ;
#77869=CARTESIAN_POINT ( 'NONE',  ( -0.1771653543307080136, -0.5400638737290844871, 0.3530559997133364547 ) ) ;
#77871=CARTESIAN_POINT ( 'NONE',  ( -1.069553805774277722, 0.2952755905511811885, 0.1292274648535926551 ) ) ;
#77872=CARTESIAN_POINT ( 'NONE',  ( 0.6102362204724416372, -0.4536011799217367080, 0.2665933059059888421 ) ) ;
#77874=CARTESIAN_POINT ( 'NONE',  ( -0.8530183727034112984, -0.4281496062992127816, -0.4176697321401328100 ) ) ;
#77875=CARTESIAN_POINT ( 'NONE',  ( -0.4790026246719152336, -0.08942795157528024563, -0.3641732283464568787 ) ) ;
#77876=CARTESIAN_POINT ( 'NONE',  ( -1.586052503253849055, 0.4724409448818907564, -0.1653254495020551051 ) ) ;
#77877=CARTESIAN_POINT ( 'NONE',  ( -0.6036745406824141069, 0.2306618581243848609, 0.2411417322834645549 ) ) ;
#77878=CARTESIAN_POINT ( 'NONE',  ( -0.3674540682414689785, 0.2306618581243848609, 0.2411417322834645549 ) ) ;
#77879=CARTESIAN_POINT ( 'NONE',  ( 0.4527559055118117182, -0.4536011799217367080, 0.2665933059059888421 ) ) ;
#77881=CARTESIAN_POINT ( 'NONE',  ( -0.1049868766404193215, -0.6046776061558807314, 0.2411417322834647770 ) ) ;
#77883=CARTESIAN_POINT ( 'NONE',  ( -1.515748031496062076, 0.07958543189024071263, -0.2665933059059888421 ) ) ;
#77884=CARTESIAN_POINT ( 'NONE',  ( 0.5971128608923891301, 0.1771653543307087075, -0.09757992244046823083 ) ) ;
#77885=CARTESIAN_POINT ( 'NONE',  ( 1.469816272965879911, 0.2306618581243847221, -0.2411417322834647770 ) ) ;
#77886=VECTOR ( 'NONE', #21128, 39.37007874015748143 ) ;
#77887=CARTESIAN_POINT ( 'NONE',  ( -0.8464566929133852113, -0.4536011799217368745, -0.2665933059059886201 ) ) ;
#77888=CARTESIAN_POINT ( 'NONE',  ( -1.049868766404198794, 0.1283753931104746893, -0.1820866141732285504 ) ) ;
#77889=CARTESIAN_POINT ( 'NONE',  ( -0.7349081364829387342, -0.6046776061558807314, 0.2411417322834647770 ) ) ;
#77890=CARTESIAN_POINT ( 'NONE',  ( -0.2099737532808391705, -0.6046776061558809534, -0.2411417322834644161 ) ) ;
#77891=CARTESIAN_POINT ( 'NONE',  ( 0.7020997375328090762, -0.2845877964562159024, 0.3641732283464567677 ) ) ;
#77893=CARTESIAN_POINT ( 'NONE',  ( 1.167979002624672580, -0.004921259842519870586, -0.3153832671262229437 ) ) ;
#77894=EDGE_CURVE ( 'NONE', #16662, #12926, #28512, .T. ) ;
#77895=CARTESIAN_POINT ( 'NONE',  ( 0.3740157480314966754, -0.5400638737290844871, 0.3530559997133364547 ) ) ;
#77897=CARTESIAN_POINT ( 'NONE',  ( -0.8858267716535425107, 0.1660481256975883668, -0.3530559997133364547 ) ) ;
#77899=CARTESIAN_POINT ( 'NONE',  ( 1.299212598425197429, 0.1771653543307087630, 0.000000000000000000 ) ) ;
#77900=CARTESIAN_POINT ( 'NONE',  ( 0.4396325459317593221, 0.2952755905511810774, -0.1292274648535930714 ) ) ;
#77901=CARTESIAN_POINT ( 'NONE',  ( 0.04593175853018440641, -0.6692913385826771977, 0.1292274648535927661 ) ) ;
#77902=CARTESIAN_POINT ( 'NONE',  ( 1.595398199321655275, 1.013096522517430209, 0.1559797534342494407 ) ) ;
#77903=CARTESIAN_POINT ( 'NONE',  ( -0.07874015748031421014, -0.1870078740157479769, 0.3641732283464567677 ) ) ;
#77904=CARTESIAN_POINT ( 'NONE',  ( 0.9842519685039378130, -0.6692913385826771977, 8.415575281601705876E-17 ) ) ;
#77905=CARTESIAN_POINT ( 'NONE',  ( -0.2362204724409442680, -0.1870078740157480601, -0.3641732283464567677 ) ) ;
#77906=CARTESIAN_POINT ( 'NONE',  ( -0.8333333333333323711, 0.2952755905511811885, 0.1292274648535926551 ) ) ;
#77907=CARTESIAN_POINT ( 'NONE',  ( 0.7974104941589355011, -4.927456884911482678E-16, 0.4445507791589062840 ) ) ;
#77908=CARTESIAN_POINT ( 'NONE',  ( -0.05905511811023545637, -0.5400638737290845981, -0.3530559997133363437 ) ) ;
#77910=CARTESIAN_POINT ( 'NONE',  ( -1.154855643044618851, 0.2306618581243848609, 0.2411417322834645549 ) ) ;
#77911=CARTESIAN_POINT ( 'NONE',  ( -0.5314960629921254842, -0.4536011799217368745, -0.2665933059059886201 ) ) ;
#77912=CARTESIAN_POINT ( 'NONE',  ( 0.1246719160104994284, -0.6692913385826771977, 0.1292274648535927661 ) ) ;
#77913=CARTESIAN_POINT ( 'NONE',  ( -1.141732283464566011, -0.6692913385826771977, 8.415575281601705876E-17 ) ) ;
#77914=CARTESIAN_POINT ( 'NONE',  ( -0.5774278215223089816, -0.6046776061558807314, 0.2411417322834647770 ) ) ;
#77915=CARTESIAN_POINT ( 'NONE',  ( -0.7426113562971994320, 2.199547029021313715, 0.5309055118110236338 ) ) ;
#77917=CARTESIAN_POINT ( 'NONE',  ( 0.7742782152230978099, -0.4281496062992124485, 0.4176697321401328655 ) ) ;
#77918=CARTESIAN_POINT ( 'NONE',  ( 1.358267716535433323, 0.1660481256975885056, 0.3530559997133364547 ) ) ;
#77920=CARTESIAN_POINT ( 'NONE',  ( -1.574803149606298192, -0.1870078740157480879, -0.4822834645669291653 ) ) ;
#77921=CARTESIAN_POINT ( 'NONE',  ( -1.437007874015747477, -0.5400638737290844871, 0.3530559997133364547 ) ) ;
#77925=CARTESIAN_POINT ( 'NONE',  ( 0.05249343832021075018, -0.5023911411419708095, 0.1820866141732285504 ) ) ;
#77927=ORIENTED_EDGE ( 'NONE', *, *, #44328, .T. ) ;
#77928=CARTESIAN_POINT ( 'NONE',  ( 0.2099737532808405305, 0.2306618581243847221, -0.2411417322834647770 ) ) ;
#77929=CARTESIAN_POINT ( 'NONE',  ( -0.05249343832020938322, -0.6046776061558809534, -0.2411417322834644161 ) ) ;
#77932=CARTESIAN_POINT ( 'NONE',  ( -0.8202099737532799750, 0.1771653543307087075, -0.09757992244046823083 ) ) ;
#77934=CARTESIAN_POINT ( 'NONE',  ( 0.9317585301837276734, 0.05413385826771626580, -0.4176697321401330321 ) ) ;
#77935=CARTESIAN_POINT ( 'NONE',  ( 1.102362204724410155, -0.1870078740157479769, 0.3641732283464567677 ) ) ;
#77936=CARTESIAN_POINT ( 'NONE',  ( -0.4199475065616791736, -0.6046776061558807314, 0.2411417322834647770 ) ) ;
#77938=CARTESIAN_POINT ( 'NONE',  ( -0.6627296587926501115, 0.2952755905511810774, -0.1292274648535930714 ) ) ;
#77939=CARTESIAN_POINT ( 'NONE',  ( -1.601049868766403650, -0.5023911411419708095, 0.1820866141732285504 ) ) ;
#77940=( BOUNDED_CURVE ( )  B_SPLINE_CURVE ( 2, ( #49689, #18136, #17326, #82115, #18545, #24835, #58388, #11408, #11827, #10987, #13375, #39028, #64712 ),
 .UNSPECIFIED., .F., .F. ) 
 B_SPLINE_CURVE_WITH_KNOTS ( ( 3, 2, 2, 2, 2, 2, 3 ),
 ( 0.5369674582711644328, 0.5378787878787878451, 0.5416666666666666297, 0.5454545454545454142, 0.5492424242424241987, 0.5530303030303029832, 0.5539416326379265065 ),
 .UNSPECIFIED. ) 
 CURVE ( )  GEOMETRIC_REPRESENTATION_ITEM ( )  RATIONAL_B_SPLINE_CURVE ( ( 0.9875488213027523443, 0.9918020599134680371, 1.000000000000000000, 0.9659258262890683122, 1.000000000000000000, 0.9659258262890683122, 1.000000000000000000, 0.9659258262890683122, 1.000000000000000000, 0.9659258262890683122, 1.000000000000000000, 0.9918020599134671489, 0.9875488213027514561 ) ) 
 REPRESENTATION_ITEM ( '' )  );
#77941=CARTESIAN_POINT ( 'NONE',  ( 1.161417322834646493, -0.5400638737290844871, 0.3530559997133364547 ) ) ;
#77942=CARTESIAN_POINT ( 'NONE',  ( 1.574803149606299746, -0.1870078740157480601, -0.3641732283464567677 ) ) ;
#77945=CARTESIAN_POINT ( 'NONE',  ( 0.07217847769028949700, -0.3162353388693405765, 0.4822834645669290543 ) ) ;
#77947=CARTESIAN_POINT ( 'NONE',  ( -0.7874015748031489847, -0.1870078740157479769, 0.4822834645669291653 ) ) ;
#77948=CARTESIAN_POINT ( 'NONE',  ( 1.207349081364829990, -0.6046776061558809534, -0.2411417322834644161 ) ) ;
#77949=CARTESIAN_POINT ( 'NONE',  ( 1.161417322834646271, 0.1660481256975883668, -0.3530559997133364547 ) ) ;
#77950=ADVANCED_FACE ( 'NONE', ( #2848 ), #8335, .F. ) ;
#77951=CARTESIAN_POINT ( 'NONE',  ( 0.2493438320209980519, -0.4281496062992127816, -0.4176697321401328100 ) ) ;
#77952=CARTESIAN_POINT ( 'NONE',  ( -0.3018372703412066094, -0.4281496062992127816, -0.4176697321401328100 ) ) ;
#77954=CARTESIAN_POINT ( 'NONE',  ( -1.266404199475064773, -0.3162353388693405765, 0.4822834645669290543 ) ) ;
#77955=CARTESIAN_POINT ( 'NONE',  ( -0.1049868766404193215, -0.6046776061558807314, 0.2411417322834647770 ) ) ;
#77957=CARTESIAN_POINT ( 'NONE',  ( -0.2887139107611542133, -0.5023911411419708095, -0.1820866141732282451 ) ) ;
#77958=DIRECTION ( 'NONE',  ( -0.000000000000000000, -1.000000000000000000, -0.000000000000000000 ) ) ;
#77959=CARTESIAN_POINT ( 'NONE',  ( 1.417322834645670104, -0.1870078740157480879, -0.4822834645669291653 ) ) ;
#77960=CARTESIAN_POINT ( 'NONE',  ( -0.4461942257217840213, 0.2306618581243848609, 0.2411417322834645549 ) ) ;
#77961=CARTESIAN_POINT ( 'NONE',  ( 0.3021879055830045124, 0.004960608223779807216, -0.3437734562760184631 ) ) ;
#77962=CARTESIAN_POINT ( 'NONE',  ( 1.181102362204724976, -0.1870078740157480879, -0.4822834645669291653 ) ) ;
#77965=CARTESIAN_POINT ( 'NONE',  ( 0.2821522309711292364, 0.2952755905511810774, -0.1292274648535930714 ) ) ;
#77966=CARTESIAN_POINT ( 'NONE',  ( -0.1771653543307080136, -0.4536011799217367080, 0.2665933059059888421 ) ) ;
#77967=CARTESIAN_POINT ( 'NONE',  ( 1.286089238845145033, -0.5023911411419708095, -0.1820866141732282451 ) ) ;
#77970=CARTESIAN_POINT ( 'NONE',  ( 1.515748031496063408, 0.07958543189024085140, 0.2665933059059887866 ) ) ;
#77971=CARTESIAN_POINT ( 'NONE',  ( 1.056430446194226436, -0.6692913385826773087, -0.1292274648535924053 ) ) ;
#77973=CARTESIAN_POINT ( 'NONE',  ( 0.2165354330708668673, 0.1660481256975883668, -0.3530559997133364547 ) ) ;
#77974=CARTESIAN_POINT ( 'NONE',  ( -0.3249695492770445782, -2.567464376874931580E-15, -0.4445507791589072832 ) ) ;
#77975=CARTESIAN_POINT ( 'NONE',  ( 1.587926509186352142, -0.004921259842519576551, 0.3153832671262227771 ) ) ;
#77976=CARTESIAN_POINT ( 'NONE',  ( -0.2034120734908131112, -0.6692913385826773087, -0.1292274648535924053 ) ) ;
#77978=CARTESIAN_POINT ( 'NONE',  ( 1.496062992125985147, -0.1870078740157479769, 0.4822834645669291653 ) ) ;
#77979=CARTESIAN_POINT ( 'NONE',  ( 0.6627296587926515548, 0.2952755905511811885, 0.1292274648535926551 ) ) ;
#77980=CARTESIAN_POINT ( 'NONE',  ( 0.9973753280839902091, -0.5023911411419708095, 0.1820866141732285504 ) ) ;
#77981=CARTESIAN_POINT ( 'NONE',  ( -2.787279214012418738, 0.000000000000000000, 0.000000000000000000 ) ) ;
#77982=CARTESIAN_POINT ( 'NONE',  ( 0.8202099737532814183, -0.5511811023622048555, -0.09757992244046775898 ) ) ;
#77983=CARTESIAN_POINT ( 'NONE',  ( -1.325459317585300889, 0.05413385826771666132, 0.4176697321401328100 ) ) ;
#77986=CARTESIAN_POINT ( 'NONE',  ( 1.227034120734908917, 0.2952755905511810774, -0.1292274648535930714 ) ) ;
#77988=CARTESIAN_POINT ( 'NONE',  ( 0.7480314960629927956, 0.2952755905511811885, 0.000000000000000000 ) ) ;
#77989=FACE_OUTER_BOUND ( 'NONE', #20473, .T. ) ;
#77990=CARTESIAN_POINT ( 'NONE',  ( -0.7137454485294948414, 2.793565526369265584, -0.4917280318828580743 ) ) ;
#77991=CARTESIAN_POINT ( 'NONE',  ( 0.4855643044619428750, -0.004921259842519576551, 0.3153832671262227771 ) ) ;
#77993=CARTESIAN_POINT ( 'NONE',  ( 0.7152230971128616943, -0.05778040916215522460, 0.4822834645669289988 ) ) ;
#77994=CARTESIAN_POINT ( 'NONE',  ( 0.7677165354330716118, 0.1012011053420775880, -0.2882089793578256898 ) ) ;
#77995=CARTESIAN_POINT ( 'NONE',  ( -0.8530183727034112984, -0.3690944881889765550, -0.3153832671262227771 ) ) ;
#77996=CARTESIAN_POINT ( 'NONE',  ( -1.135170603674539924, -0.6692913385826771977, 0.1292274648535927661 ) ) ;
#77997=CARTESIAN_POINT ( 'NONE',  ( -1.535433070866141225, 0.2952755905511811885, 0.000000000000000000 ) ) ;
#77998=CARTESIAN_POINT ( 'NONE',  ( 0.8267716535433078384, -0.6692913385826771977, 8.415575281601705876E-17 ) ) ;
#77999=CARTESIAN_POINT ( 'NONE',  ( 1.679790026246720025, 0.2306618581243848609, 0.2411417322834645549 ) ) ;
#78002=CARTESIAN_POINT ( 'NONE',  ( 0.8530183727034126306, 0.05413385826771626580, -0.4176697321401330321 ) ) ;
#78005=CARTESIAN_POINT ( 'NONE',  ( 1.463254593175853824, -0.6692913385826771977, 0.1292274648535927661 ) ) ;
#78006=CARTESIAN_POINT ( 'NONE',  ( -1.338582677165353729, -0.1870078740157480601, -0.3641732283464567677 ) ) ;
#78007=CARTESIAN_POINT ( 'NONE',  ( 1.036745406824147731, -0.004921259842519576551, 0.3153832671262227771 ) ) ;
#78008=CARTESIAN_POINT ( 'NONE',  ( -1.122047244094487306, 0.07958543189024071263, -0.2665933059059888421 ) ) ;
#78009=CARTESIAN_POINT ( 'NONE',  ( -0.6167979002624665030, -0.3690944881889765550, -0.3153832671262227771 ) ) ;
#78010=CARTESIAN_POINT ( 'NONE',  ( -1.391076115485563758, 0.1283753931104748280, 0.1820866141732283561 ) ) ;
#78011=CARTESIAN_POINT ( 'NONE',  ( 1.049868766404200127, -0.5023911411419708095, -0.1820866141732282451 ) ) ;
#78012=CARTESIAN_POINT ( 'NONE',  ( 0.4855643044619430415, -0.4281496062992127816, -0.4176697321401328100 ) ) ;
#78013=CARTESIAN_POINT ( 'NONE',  ( 1.161417322834646271, 0.1660481256975883668, -0.3530559997133364547 ) ) ;
#78015=CARTESIAN_POINT ( 'NONE',  ( 0.1181102362204730916, 0.2952755905511811885, 0.000000000000000000 ) ) ;
#78016=CARTESIAN_POINT ( 'NONE',  ( 0.6167979002624678353, -0.3690944881889763329, 0.3153832671262228327 ) ) ;
#78017=CARTESIAN_POINT ( 'NONE',  ( 1.345144356955381593, -0.3162353388693409650, -0.4822834645669289433 ) ) ;
#78019=CARTESIAN_POINT ( 'NONE',  ( -0.4986876640419942164, -0.6046776061558807314, 0.2411417322834647770 ) ) ;
#78022=CARTESIAN_POINT ( 'NONE',  ( 0.03280839895013198948, 0.2952755905511811885, 0.1292274648535926551 ) ) ;
#78023=CARTESIAN_POINT ( 'NONE',  ( -0.2034120734908128059, 0.2952755905511811885, 0.1292274648535926551 ) ) ;
#78024=CARTESIAN_POINT ( 'NONE',  ( -0.2165354330708654795, -0.5400638737290845981, -0.3530559997133363437 ) ) ;
#78030=CARTESIAN_POINT ( 'NONE',  ( -0.9776902887139098386, -0.5511811023622046335, 0.09757992244046803654 ) ) ;
#78032=CARTESIAN_POINT ( 'NONE',  ( -1.017060367454067249, -0.3162353388693409650, -0.4822834645669289433 ) ) ;
#78034=CARTESIAN_POINT ( 'NONE',  ( 0.5971128608923891301, 0.2952755905511810774, -0.1292274648535930714 ) ) ;
#78035=CARTESIAN_POINT ( 'NONE',  ( -0.5839895013123351797, 0.1771653543307087075, -0.09757992244046823083 ) ) ;
#78036=CARTESIAN_POINT ( 'NONE',  ( 1.128608923884514947, 0.2306618581243848609, 0.2411417322834645549 ) ) ;
#78037=CARTESIAN_POINT ( 'NONE',  ( 0.5380577427821529035, 0.05413385826771626580, -0.4176697321401330321 ) ) ;
#78041=CARTESIAN_POINT ( 'NONE',  ( 1.443569553805774897, -0.6046776061558809534, -0.2411417322834644161 ) ) ;
#78042=CARTESIAN_POINT ( 'NONE',  ( 0.3674540682414705883, 0.2306618581243847221, -0.2411417322834647770 ) ) ;
#78044=CARTESIAN_POINT ( 'NONE',  ( 0.09842519685039434474, -0.5400638737290845981, -0.3530559997133363437 ) ) ;
#78045=CARTESIAN_POINT ( 'NONE',  ( 1.371391076115485719, -0.6692913385826773087, -0.1292274648535924053 ) ) ;
#78046=CARTESIAN_POINT ( 'NONE',  ( 0.8989501312335964611, 0.2952755905511811885, 0.1292274648535926551 ) ) ;
#78048=CARTESIAN_POINT ( 'NONE',  ( -0.1115485564304456306, 0.2952755905511810774, -0.1292274648535930714 ) ) ;
#78049=CARTESIAN_POINT ( 'NONE',  ( 1.227034120734908917, 0.2952755905511810774, -0.1292274648535930714 ) ) ;
#78050=CARTESIAN_POINT ( 'NONE',  ( 0.3083989501312343062, -0.05778040916215560624, -0.4822834645669293319 ) ) ;
#78051=CARTESIAN_POINT ( 'NONE',  ( 1.082677165354331228, 0.07958543189024071263, -0.2665933059059888421 ) ) ;
#78052=CARTESIAN_POINT ( 'NONE',  ( -0.8989501312335946848, 0.2952755905511810774, -0.1292274648535930714 ) ) ;
#78053=CARTESIAN_POINT ( 'NONE',  ( -1.384514435695537005, 0.2952755905511811885, 0.1292274648535926551 ) ) ;
#78054=CARTESIAN_POINT ( 'NONE',  ( 0.8858267716535438430, -0.5400638737290845981, -0.3530559997133363437 ) ) ;
#78057=ORIENTED_EDGE ( 'NONE', *, *, #73157, .T. ) ;
#78060=CARTESIAN_POINT ( 'NONE',  ( 1.345144356955381593, -0.05778040916215522460, 0.4822834645669289988 ) ) ;
#78061=CARTESIAN_POINT ( 'NONE',  ( 0.9383202099737536495, -0.2845877964562159024, 0.3641732283464567677 ) ) ;
#78066=CARTESIAN_POINT ( 'NONE',  ( -1.122047244094487306, 0.07958543189024071263, -0.2665933059059888421 ) ) ;
#78067=CARTESIAN_POINT ( 'NONE',  ( -1.712598425196849572, 0.07958543189024085140, 0.2665933059059887866 ) ) ;
#78069=CARTESIAN_POINT ( 'NONE',  ( -0.2755905511811018171, 0.2952755905511811885, 0.000000000000000000 ) ) ;
#78070=CARTESIAN_POINT ( 'NONE',  ( 1.194225721784777594, -0.4281496062992127816, -0.4176697321401328100 ) ) ;
#78073=CARTESIAN_POINT ( 'NONE',  ( -1.627296587926508442, -0.6046776061558809534, -0.2411417322834644161 ) ) ;
#78077=CARTESIAN_POINT ( 'NONE',  ( -0.7808398950131222316, -0.2845877964562161244, -0.3641732283464567121 ) ) ;
#78078=CARTESIAN_POINT ( 'NONE',  ( -1.528871391076114250, -0.6692913385826771977, 0.1292274648535927661 ) ) ;
#78079=CARTESIAN_POINT ( 'NONE',  ( 0.7414698162729663755, 0.2952755905511811885, 0.1292274648535926551 ) ) ;
#78080=ORIENTED_EDGE ( 'NONE', *, *, #75407, .T. ) ;
#78081=CARTESIAN_POINT ( 'NONE',  ( -0.7443564586554828333, 2.208176010637902031, 0.5309055118110236338 ) ) ;
#78083=CARTESIAN_POINT ( 'NONE',  ( 1.181102362204725198, -0.1870078740157479769, 0.4822834645669291653 ) ) ;
#78084=CARTESIAN_POINT ( 'NONE',  ( 1.555118110236221041, -0.4536011799217367080, 0.2665933059059888421 ) ) ;
#78086=B_SPLINE_CURVE_WITH_KNOTS ( 'NONE', 3,
 ( #7026, #7451, #23391, #22980, #3218, #79840, #54543 ),
 .UNSPECIFIED., .F., .F.,
 ( 4, 3, 4 ),
 ( 1.734723475976807094E-18, 0.001246230184515576727, 0.002492489877932654602 ),
 .UNSPECIFIED. ) ;
#78087=CARTESIAN_POINT ( 'NONE',  ( -0.9776902887139098386, -0.5511811023622046335, 0.09757992244046803654 ) ) ;
#78088=CARTESIAN_POINT ( 'NONE',  ( -1.541994750656167090, -0.5511811023622048555, -0.09757992244046775898 ) ) ;
#78090=CARTESIAN_POINT ( 'NONE',  ( 0.5971128608923890191, -0.6692913385826771977, 0.1292274648535927661 ) ) ;
#78091=CARTESIAN_POINT ( 'NONE',  ( -0.7414698162729651543, -0.5511811023622046335, 0.09757992244046803654 ) ) ;
#78092=CARTESIAN_POINT ( 'NONE',  ( -0.09842519685039295696, 0.07958543189024071263, -0.2665933059059888421 ) ) ;
#78093=CARTESIAN_POINT ( 'NONE',  ( -0.2099737532808391705, -0.6046776061558809534, -0.2411417322834644161 ) ) ;
#78094=CARTESIAN_POINT ( 'NONE',  ( -1.095800524934382292, -0.2845877964562161244, -0.3641732283464567121 ) ) ;
#78096=CARTESIAN_POINT ( 'NONE',  ( 0.6692913385826777528, 0.2952755905511811885, 0.000000000000000000 ) ) ;
#78097=CARTESIAN_POINT ( 'NONE',  ( -1.318897637795274802, 0.1660481256975885056, 0.3530559997133364547 ) ) ;
#78099=CARTESIAN_POINT ( 'NONE',  ( -0.6233595800524928121, -0.05778040916215522460, 0.4822834645669289988 ) ) ;
#78100=CARTESIAN_POINT ( 'NONE',  ( -0.1706036745406816491, -0.3690944881889763329, 0.3153832671262228327 ) ) ;
#78101=CARTESIAN_POINT ( 'NONE',  ( -1.463254593175852492, 0.2952755905511811885, 0.1292274648535926551 ) ) ;
#78102=CARTESIAN_POINT ( 'NONE',  ( 0.6824146981627303710, -0.5023911411419708095, 0.1820866141732285504 ) ) ;
#78103=CARTESIAN_POINT ( 'NONE',  ( -0.3280839895013117347, -0.3690944881889763329, 0.3153832671262228327 ) ) ;
#78104=CARTESIAN_POINT ( 'NONE',  ( -0.7349081364829390672, 0.2306618581243847221, -0.2411417322834647770 ) ) ;
#78105=CARTESIAN_POINT ( 'NONE',  ( -1.161417322834644716, -0.5400638737290845981, -0.3530559997133363437 ) ) ;
#78106=CARTESIAN_POINT ( 'NONE',  ( -1.404199475065615932, -0.4281496062992127816, -0.4176697321401328100 ) ) ;
#78108=CARTESIAN_POINT ( 'NONE',  ( 1.240157480314961314, 0.07958543189024071263, -0.2665933059059888421 ) ) ;
#78109=CARTESIAN_POINT ( 'NONE',  ( 0.2296587926509192634, -0.3162353388693405765, 0.4822834645669290543 ) ) ;
#78110=CARTESIAN_POINT ( 'NONE',  ( -1.469816272965878357, 0.2306618581243848609, 0.2411417322834645549 ) ) ;
#78111=CARTESIAN_POINT ( 'NONE',  ( -1.692913385826770645, 0.2952755905511811885, 0.000000000000000000 ) ) ;
#78114=CARTESIAN_POINT ( 'NONE',  ( -1.082677165354329896, -0.4536011799217368745, -0.2665933059059886201 ) ) ;
#78115=CARTESIAN_POINT ( 'NONE',  ( 0.6627296587926515548, 0.2952755905511811885, 0.1292274648535926551 ) ) ;
#78116=CARTESIAN_POINT ( 'NONE',  ( -1.095800524934382292, -0.08942795157527998196, 0.3641732283464567121 ) ) ;
#78118=CARTESIAN_POINT ( 'NONE',  ( -1.305774278215222184, -0.6692913385826773087, -0.1292274648535924053 ) ) ;
#78119=CARTESIAN_POINT ( 'NONE',  ( 1.056430446194226658, 0.2952755905511811885, 0.1292274648535926551 ) ) ;
#78120=CARTESIAN_POINT ( 'NONE',  ( 0.3871391076115493490, -0.3162353388693405765, 0.4822834645669290543 ) ) ;
#78121=CARTESIAN_POINT ( 'NONE',  ( 1.397637795275591177, -0.5400638737290844871, 0.3530559997133364547 ) ) ;
#78122=CARTESIAN_POINT ( 'NONE',  ( -1.430446194225721390, -0.3690944881889763329, 0.3153832671262228327 ) ) ;
#78127=CARTESIAN_POINT ( 'NONE',  ( 0.9383202099737538715, -0.08942795157528024563, -0.3641732283464568787 ) ) ;
#78128=CARTESIAN_POINT ( 'NONE',  ( 0.1312335958005255154, -0.5023911411419708095, 0.1820866141732285504 ) ) ;
#78130=CARTESIAN_POINT ( 'NONE',  ( 0.2099737532808405305, 0.2306618581243847221, -0.2411417322834647770 ) ) ;
#78131=CARTESIAN_POINT ( 'NONE',  ( 1.233595800524935227, -0.6046776061558807314, 0.2411417322834647770 ) ) ;
#78133=CARTESIAN_POINT ( 'NONE',  ( 0.2034120734908144990, -0.5511811023622046335, 0.09757992244046803654 ) ) ;
#78134=CARTESIAN_POINT ( 'NONE',  ( -0.7545931758530176614, -0.6692913385826773087, -0.1292274648535924053 ) ) ;
#78135=CARTESIAN_POINT ( 'NONE',  ( -1.489501312335957062, -0.05778040916215522460, 0.4822834645669289988 ) ) ;
#78136=CARTESIAN_POINT ( 'NONE',  ( 0.7086614173228353852, -0.1870078740157479769, 0.4822834645669291653 ) ) ;
#78138=CARTESIAN_POINT ( 'NONE',  ( 1.603475055217291612, 1.330568129716842130, 0.04573490813648269093 ) ) ;
#78140=EDGE_CURVE ( 'NONE', #80835, #48838, #39460, .T. ) ;
#78142=CARTESIAN_POINT ( 'NONE',  ( -1.312335958005248715, -0.6046776061558809534, -0.2411417322834644161 ) ) ;
#78143=CARTESIAN_POINT ( 'NONE',  ( -0.6036745406824141069, -0.5023911411419708095, -0.1820866141732282451 ) ) ;
#78144=CARTESIAN_POINT ( 'NONE',  ( -1.253280839895012377, -0.3162353388693409650, -0.4822834645669289433 ) ) ;
#78147=CARTESIAN_POINT ( 'NONE',  ( 1.502624671916010790, -0.05778040916215522460, 0.4822834645669289988 ) ) ;
#78149=CARTESIAN_POINT ( 'NONE',  ( -1.062992125984250968, 0.2952755905511811885, 0.000000000000000000 ) ) ;
#78150=CARTESIAN_POINT ( 'NONE',  ( 0.2821522309711292364, -0.6692913385826771977, 0.1292274648535927661 ) ) ;
#78151=CARTESIAN_POINT ( 'NONE',  ( -1.456692913385826182, 0.2952755905511811885, 0.000000000000000000 ) ) ;
#78153=CARTESIAN_POINT ( 'NONE',  ( 0.4461942257217855201, -0.6046776061558807314, 0.2411417322834647770 ) ) ;
#78155=CARTESIAN_POINT ( 'NONE',  ( -0.6692913385826764205, 0.1771653543307087630, 0.000000000000000000 ) ) ;
#78160=CARTESIAN_POINT ( 'NONE',  ( -1.318897637795274802, -0.5400638737290845981, -0.3530559997133363437 ) ) ;
#78161=CARTESIAN_POINT ( 'NONE',  ( -1.351706036745406347, -0.4281496062992124485, 0.4176697321401328655 ) ) ;
#78163=CARTESIAN_POINT ( 'NONE',  ( -1.627296587926508442, -0.6046776061558809534, -0.2411417322834644161 ) ) ;
#78164=CARTESIAN_POINT ( 'NONE',  ( -1.181102362204723644, -0.1870078740157480879, -0.4822834645669291653 ) ) ;
#78165=CARTESIAN_POINT ( 'NONE',  ( -1.502624671916009680, -0.3162353388693405765, 0.4822834645669290543 ) ) ;
#78167=CARTESIAN_POINT ( 'NONE',  ( 1.614173228346457378, 1.267785121476991073, -0.1372047244094476148 ) ) ;
#78168=CARTESIAN_POINT ( 'NONE',  ( 0.3083989501312343062, -0.08942795157528024563, -0.3641732283464568787 ) ) ;
#78171=CARTESIAN_POINT ( 'NONE',  ( -0.4330708661417315697, 0.1771653543307087630, 0.000000000000000000 ) ) ;
#78172=CARTESIAN_POINT ( 'NONE',  ( -0.6299212598425188991, -0.1870078740157480879, -0.4822834645669291653 ) ) ;
#78173=CARTESIAN_POINT ( 'NONE',  ( 0.7480314960629927956, -0.6692913385826771977, 8.415575281601705876E-17 ) ) ;
#78174=CARTESIAN_POINT ( 'NONE',  ( -0.8727034120734901146, -0.3162353388693405765, 0.4822834645669290543 ) ) ;
#78178=CARTESIAN_POINT ( 'NONE',  ( -1.062992125984250968, -0.6692913385826771977, 8.415575281601705876E-17 ) ) ;
#78179=CARTESIAN_POINT ( 'NONE',  ( 0.7480314960629927956, -0.6692913385826771977, 8.415575281601705876E-17 ) ) ;
#78186=CARTESIAN_POINT ( 'NONE',  ( -0.4199475065616791736, -0.6046776061558807314, 0.2411417322834647770 ) ) ;
#78187=CARTESIAN_POINT ( 'NONE',  ( -1.614173228346455824, 0.1771653543307087630, 0.000000000000000000 ) ) ;
#78188=CARTESIAN_POINT ( 'NONE',  ( -0.8858267716535425107, 0.1660481256975883668, -0.3530559997133364547 ) ) ;
#78190=CARTESIAN_POINT ( 'NONE',  ( -1.286089238845143479, -0.6046776061558807314, 0.2411417322834647770 ) ) ;
#78192=CARTESIAN_POINT ( 'NONE',  ( -0.8267716535433065062, -0.6692913385826771977, 8.415575281601705876E-17 ) ) ;
#78193=CARTESIAN_POINT ( 'NONE',  ( -0.3871391076115479057, -0.3162353388693409650, -0.4822834645669289433 ) ) ;
#78195=CARTESIAN_POINT ( 'NONE',  ( 0.7611548556430451917, -0.5023911411419708095, 0.1820866141732285504 ) ) ;
#78196=LINE ( 'NONE', #46179, #33074 ) ;
#78197=CARTESIAN_POINT ( 'NONE',  ( 0.3346456692913393205, -0.4536011799217368745, -0.2665933059059886201 ) ) ;
#78198=CARTESIAN_POINT ( 'NONE',  ( 1.489501312335958172, -0.08942795157528024563, -0.3641732283464568787 ) ) ;
#78200=CARTESIAN_POINT ( 'NONE',  ( 1.496062992125984703, -0.1870078740157480879, -0.4822834645669291653 ) ) ;
#78201=CARTESIAN_POINT ( 'NONE',  ( 0.1509186351706045259, -0.08942795157528024563, -0.3641732283464568787 ) ) ;
#78203=CARTESIAN_POINT ( 'NONE',  ( -1.423884514435694859, -0.05778040916215560624, -0.4822834645669293319 ) ) ;
#78204=CARTESIAN_POINT ( 'NONE',  ( 1.358267716535433323, -0.5400638737290845981, -0.3530559997133363437 ) ) ;
#78206=CARTESIAN_POINT ( 'NONE',  ( -0.4855643044619415427, -0.004921259842519870586, -0.3153832671262229437 ) ) ;
#78207=CARTESIAN_POINT ( 'NONE',  ( -0.4461942257217840213, 0.2306618581243848609, 0.2411417322834645549 ) ) ;
#78208=CARTESIAN_POINT ( 'NONE',  ( 0.2296587926509192634, -0.3162353388693405765, 0.4822834645669290543 ) ) ;
#78210=CARTESIAN_POINT ( 'NONE',  ( 0.8858267716535438430, -0.4536011799217368745, -0.2665933059059886201 ) ) ;
#78211=CARTESIAN_POINT ( 'NONE',  ( 0.3083989501312343062, -0.2845877964562159024, 0.3641732283464567677 ) ) ;
#78212=CARTESIAN_POINT ( 'NONE',  ( -0.1246719160104980823, -0.6692913385826773087, -0.1292274648535924053 ) ) ;
#78213=CARTESIAN_POINT ( 'NONE',  ( -1.660104986876639543, -0.05778040916215560624, -0.4822834645669293319 ) ) ;
#78214=CARTESIAN_POINT ( 'NONE',  ( -0.6233595800524928121, -0.2845877964562161244, -0.3641732283464567121 ) ) ;
#78216=CARTESIAN_POINT ( 'NONE',  ( 0.4133858267716541968, 0.1660481256975885056, 0.3530559997133364547 ) ) ;
#78217=CARTESIAN_POINT ( 'NONE',  ( -0.7611548556430438595, -0.6046776061558809534, -0.2411417322834644161 ) ) ;
#78220=CARTESIAN_POINT ( 'NONE',  ( 0.1049868766404206816, -0.5023911411419708095, -0.1820866141732282451 ) ) ;
#78221=CARTESIAN_POINT ( 'NONE',  ( -0.5971128608923877978, -0.6692913385826773087, -0.1292274648535924053 ) ) ;
#78222=CARTESIAN_POINT ( 'NONE',  ( -0.9645669291338575535, 0.1660481256975883668, -0.3530559997133364547 ) ) ;
#78223=CARTESIAN_POINT ( 'NONE',  ( -1.351706036745406347, -0.3690944881889763329, 0.3153832671262228327 ) ) ;
#78224=CARTESIAN_POINT ( 'NONE',  ( 1.673228346456693494, 0.1660481256975885056, 0.3530559997133364547 ) ) ;
#78225=CARTESIAN_POINT ( 'NONE',  ( -0.7349081364829387342, -0.5023911411419708095, 0.1820866141732285504 ) ) ;
#78227=CARTESIAN_POINT ( 'NONE',  ( 1.456692913385827515, 0.2952755905511811885, 0.000000000000000000 ) ) ;
#78232=CARTESIAN_POINT ( 'NONE',  ( 1.463254593175853824, 0.1771653543307087075, -0.09757992244046823083 ) ) ;
#78233=CARTESIAN_POINT ( 'NONE',  ( -1.312335958005248715, -0.6046776061558809534, -0.2411417322834644161 ) ) ;
#78234=B_SPLINE_CURVE_WITH_KNOTS ( 'NONE', 3,
 ( #50021, #55920, #4179, #31492, #49611, #57153, #17650 ),
 .UNSPECIFIED., .F., .F.,
 ( 4, 3, 4 ),
 ( 0.000000000000000000, 0.001246232571205256601, 0.002492492258783257208 ),
 .UNSPECIFIED. ) ;
#78235=CARTESIAN_POINT ( 'NONE',  ( 1.062992125984252745, -0.6692913385826771977, 8.415575281601705876E-17 ) ) ;
#78237=CARTESIAN_POINT ( 'NONE',  ( 1.601049868766404982, -0.5023911411419708095, -0.1820866141732282451 ) ) ;
#78238=EDGE_CURVE ( 'NONE', #69738, #11377, #13939, .T. ) ;
#78239=CARTESIAN_POINT ( 'NONE',  ( 0.3412073490813655186, -0.6046776061558809534, -0.2411417322834644161 ) ) ;
#78240=CARTESIAN_POINT ( 'NONE',  ( -0.5052493438320203589, 0.2952755905511810774, -0.1292274648535930714 ) ) ;
#78243=CARTESIAN_POINT ( 'NONE',  ( 0.9251968503937015864, -0.4536011799217367080, 0.2665933059059888421 ) ) ;
#78245=ORIENTED_EDGE ( 'NONE', *, *, #15589, .F. ) ;
#78248=CARTESIAN_POINT ( 'NONE',  ( -0.1181102362204717315, 0.2952755905511811885, 0.000000000000000000 ) ) ;
#78250=CARTESIAN_POINT ( 'NONE',  ( 1.423884514435696191, -0.05778040916215522460, 0.4822834645669289988 ) ) ;
#78251=CARTESIAN_POINT ( 'NONE',  ( 0.3805774278215230400, -0.4281496062992124485, 0.4176697321401328655 ) ) ;
#78252=CARTESIAN_POINT ( 'NONE',  ( 1.345144356955381593, -0.05778040916215522460, 0.4822834645669289988 ) ) ;
#78253=CARTESIAN_POINT ( 'NONE',  ( -0.5511811023622038563, -0.1870078740157479769, 0.4822834645669291653 ) ) ;
#78254=CARTESIAN_POINT ( 'NONE',  ( -0.08530183727034056085, -0.05778040916215560624, -0.4822834645669293319 ) ) ;
#78255=CARTESIAN_POINT ( 'NONE',  ( -1.528871391076114250, -0.6692913385826771977, 0.1292274648535927661 ) ) ;
#78256=CARTESIAN_POINT ( 'NONE',  ( 1.417322834645670104, -0.1870078740157479769, 0.4822834645669291653 ) ) ;
#78257=CARTESIAN_POINT ( 'NONE',  ( 1.200787401574803681, 0.1660481256975885056, 0.3530559997133364547 ) ) ;
#78259=CARTESIAN_POINT ( 'NONE',  ( 0.5839895013123367340, 0.1771653543307087630, 0.09757992244046791164 ) ) ;
#78260=ORIENTED_EDGE ( 'NONE', *, *, #31580, .T. ) ;
#78263=CARTESIAN_POINT ( 'NONE',  ( -0.2952755905511804668, 0.07958543189024085140, 0.2665933059059887866 ) ) ;
#78264=CARTESIAN_POINT ( 'NONE',  ( -0.1902887139107604098, 0.2952755905511810774, -0.1292274648535930714 ) ) ;
#78266=CARTESIAN_POINT ( 'NONE',  ( 0.02624671916010564918, 0.2306618581243848609, 0.2411417322834645549 ) ) ;
#78267=CARTESIAN_POINT ( 'NONE',  ( 0.1115485564304467270, -0.6692913385826773087, -0.1292274648535924053 ) ) ;
#78268=CARTESIAN_POINT ( 'NONE',  ( -0.9776902887139098386, 0.2952755905511810774, -0.1292274648535930714 ) ) ;
#78269=CARTESIAN_POINT ( 'NONE',  ( -1.010498687664041384, -0.4281496062992127816, -0.4176697321401328100 ) ) ;
#78270=CARTESIAN_POINT ( 'NONE',  ( 1.253280839895013710, -0.08942795157528024563, -0.3641732283464568787 ) ) ;
#78271=CARTESIAN_POINT ( 'NONE',  ( -1.568241469816272105, -0.3162353388693409650, -0.4822834645669289433 ) ) ;
#78273=CARTESIAN_POINT ( 'NONE',  ( 0.9055118110236227702, -0.5511811023622047445, 6.969142054262312111E-17 ) ) ;
#78274=CARTESIAN_POINT ( 'NONE',  ( 0.5577427821522316087, -0.05778040916215522460, 0.4822834645669289988 ) ) ;
#78275=CARTESIAN_POINT ( 'NONE',  ( 0.7349081364829403995, 0.2306618581243848609, 0.2411417322834645549 ) ) ;
#78277=CARTESIAN_POINT ( 'NONE',  ( -1.679790026246718693, 0.2306618581243847221, -0.2411417322834647770 ) ) ;
#78280=CARTESIAN_POINT ( 'NONE',  ( -0.6496062992125976043, -0.5400638737290844871, 0.3530559997133364547 ) ) ;
#78281=B_SPLINE_CURVE_WITH_KNOTS ( 'NONE', 3,
 ( #43456, #30014, #43047, #42644, #55677, #81386, #12323 ),
 .UNSPECIFIED., .F., .F.,
 ( 4, 3, 4 ),
 ( 5.551115123125782702E-17, 0.001246230184515611855, 0.002492489877932689731 ),
 .UNSPECIFIED. ) ;
#78284=CARTESIAN_POINT ( 'NONE',  ( -1.292650918635170010, 0.1771653543307087075, -0.09757992244046823083 ) ) ;
#78285=CARTESIAN_POINT ( 'NONE',  ( 1.417322834645670104, -0.1870078740157479769, 0.4822834645669291653 ) ) ;
#78286=CARTESIAN_POINT ( 'NONE',  ( 1.062992125984252745, 0.2952755905511811885, 0.000000000000000000 ) ) ;
#78287=CARTESIAN_POINT ( 'NONE',  ( -0.1837270341207340729, 0.1283753931104746893, -0.1820866141732285504 ) ) ;
#78288=CARTESIAN_POINT ( 'NONE',  ( 0.6167979002624678353, -0.4281496062992124485, 0.4176697321401328655 ) ) ;
#78290=CARTESIAN_POINT ( 'NONE',  ( -0.2296587926509179312, -0.08942795157527998196, 0.3641732283464567121 ) ) ;
#78291=CARTESIAN_POINT ( 'NONE',  ( -0.2362204724409442680, -0.1870078740157480879, -0.4822834645669291653 ) ) ;
#78293=CARTESIAN_POINT ( 'NONE',  ( -1.095800524934382292, -0.05778040916215522460, 0.4822834645669289988 ) ) ;
#78294=CARTESIAN_POINT ( 'NONE',  ( 0.6233595800524939223, -0.2845877964562159024, 0.3641732283464567677 ) ) ;
#78296=CARTESIAN_POINT ( 'NONE',  ( -0.7874015748031489847, -0.1870078740157479769, 0.4822834645669291653 ) ) ;
#78297=CARTESIAN_POINT ( 'NONE',  ( -0.2624671916010490880, -0.5023911411419708095, 0.1820866141732285504 ) ) ;
#78298=CARTESIAN_POINT ( 'NONE',  ( 1.614173228346456712, 2.401574803149606474, 0.5309055118110233007 ) ) ;
#78299=CARTESIAN_POINT ( 'NONE',  ( -0.8333333333333323711, -0.6692913385826773087, -0.1292274648535924053 ) ) ;
#78300=CARTESIAN_POINT ( 'NONE',  ( -0.6036745406824141069, -0.6046776061558809534, -0.2411417322834644161 ) ) ;
#78301=CARTESIAN_POINT ( 'NONE',  ( 0.01968503937007957949, -0.5400638737290845981, -0.3530559997133363437 ) ) ;
#78304=CARTESIAN_POINT ( 'NONE',  ( -1.653543307086613234, -0.1870078740157480601, -0.3641732283464567677 ) ) ;
#78305=CARTESIAN_POINT ( 'NONE',  ( 0.9383202099737538715, -0.08942795157528024563, -0.3641732283464568787 ) ) ;
#78306=CARTESIAN_POINT ( 'NONE',  ( 1.240157480314961314, -0.5400638737290844871, 0.3530559997133364547 ) ) ;
#78307=CARTESIAN_POINT ( 'NONE',  ( -0.9514435695538050464, -0.2845877964562159024, 0.3641732283464567677 ) ) ;
#78308=CARTESIAN_POINT ( 'NONE',  ( -1.082677165354329896, 0.07958543189024085140, 0.2665933059059887866 ) ) ;
#78310=CARTESIAN_POINT ( 'NONE',  ( -0.5905511811023613777, -0.6692913385826771977, 8.415575281601705876E-17 ) ) ;
#78311=CARTESIAN_POINT ( 'NONE',  ( 0.09186351706036799403, -0.4281496062992127816, -0.4176697321401328100 ) ) ;
#78312=CARTESIAN_POINT ( 'NONE',  ( 0.6430446194225729606, -0.3690944881889765550, -0.3153832671262227771 ) ) ;
#78314=CARTESIAN_POINT ( 'NONE',  ( 0.9186351706036751663, -0.5023911411419708095, 0.1820866141732285504 ) ) ;
#78316=CARTESIAN_POINT ( 'NONE',  ( 0.5249343832021005074, -0.6046776061558807314, 0.2411417322834647770 ) ) ;
#78318=CARTESIAN_POINT ( 'NONE',  ( -0.8923884514435688198, 0.2306618581243847221, -0.2411417322834647770 ) ) ;
#78320=CARTESIAN_POINT ( 'NONE',  ( 1.351706036745407458, -0.3690944881889765550, -0.3153832671262227771 ) ) ;
#78321=CARTESIAN_POINT ( 'NONE',  ( 0.3674540682414705883, -0.6046776061558807314, 0.2411417322834647770 ) ) ;
#78322=CARTESIAN_POINT ( 'NONE',  ( 0.1574803149606306130, -0.1870078740157480879, -0.4822834645669291653 ) ) ;
#78323=CARTESIAN_POINT ( 'NONE',  ( 0.006561679790026889343, -0.2845877964562161244, -0.3641732283464567121 ) ) ;
#78324=CARTESIAN_POINT ( 'NONE',  ( 0.6171485355042644061, 0.004960608223779807216, -0.3437734562760184631 ) ) ;
#78325=CARTESIAN_POINT ( 'NONE',  ( -0.1443569553805765515, -0.3690944881889765550, -0.3153832671262227771 ) ) ;
#78326=CARTESIAN_POINT ( 'NONE',  ( 0.6955380577427828781, -0.4281496062992124485, 0.4176697321401328655 ) ) ;
#78327=CARTESIAN_POINT ( 'NONE',  ( -0.9448818897637790704, -0.1870078740157479769, 0.3641732283464567677 ) ) ;
#78328=CARTESIAN_POINT ( 'NONE',  ( -0.7808398950131222316, -0.3162353388693409650, -0.4822834645669289433 ) ) ;
#78329=CARTESIAN_POINT ( 'NONE',  ( 0.8537221893815273299, 2.409604939980833412E-17, -0.3464511005275205946 ) ) ;
#78332=CARTESIAN_POINT ( 'NONE',  ( -1.148293963254592542, 0.2952755905511811885, 0.1292274648535926551 ) ) ;
#78333=CARTESIAN_POINT ( 'NONE',  ( -1.312335958005248715, -0.5023911411419708095, -0.1820866141732282451 ) ) ;
#78334=CARTESIAN_POINT ( 'NONE',  ( -0.1443569553805768291, 0.05413385826771666132, 0.4176697321401328100 ) ) ;
#78335=CARTESIAN_POINT ( 'NONE',  ( -1.679790026246718693, 0.2306618581243847221, -0.2411417322834647770 ) ) ;
#78336=CARTESIAN_POINT ( 'NONE',  ( -0.5708661417322825615, -0.5400638737290844871, 0.3530559997133364547 ) ) ;
#78337=DIRECTION ( 'NONE',  ( 0.000000000000000000, 1.000000000000000000, 0.000000000000000000 ) ) ;
#78338=CARTESIAN_POINT ( 'NONE',  ( 1.640419947506562393, -0.4281496062992124485, 0.4176697321401328655 ) ) ;
#78339=CARTESIAN_POINT ( 'NONE',  ( 1.036745406824147508, -0.4281496062992127816, -0.4176697321401328100 ) ) ;
#78340=CARTESIAN_POINT ( 'NONE',  ( 1.194225721784777594, 0.05413385826771666132, 0.4176697321401328100 ) ) ;
#78343=CARTESIAN_POINT ( 'NONE',  ( -1.476377952755905110, -0.5400638737290845981, -0.3530559997133363437 ) ) ;
#78346=CARTESIAN_POINT ( 'NONE',  ( 0.05905511811023709395, -0.4536011799217367080, 0.2665933059059888421 ) ) ;
#78348=ORIENTED_EDGE ( 'NONE', *, *, #11980, .F. ) ;
#78349=CARTESIAN_POINT ( 'NONE',  ( 0.2230971128608929543, 0.05413385826771626580, -0.4176697321401330321 ) ) ;
#78350=CARTESIAN_POINT ( 'NONE',  ( 0.09186351706036799403, -0.4281496062992127816, -0.4176697321401328100 ) ) ;
#78351=CARTESIAN_POINT ( 'NONE',  ( -0.5380577427821514602, 0.05413385826771666132, 0.4176697321401328100 ) ) ;
#78353=CARTESIAN_POINT ( 'NONE',  ( -0.7152230971128602510, -0.2845877964562159024, 0.3641732283464567677 ) ) ;
#78355=CARTESIAN_POINT ( 'NONE',  ( 0.5774278215223104249, 0.2306618581243848609, 0.2411417322834645549 ) ) ;
#78356=CARTESIAN_POINT ( 'NONE',  ( 0.4002624671916016896, -0.2845877964562161244, -0.3641732283464567121 ) ) ;
#78357=CARTESIAN_POINT ( 'NONE',  ( -0.5052493438320203589, 0.2952755905511810774, -0.1292274648535930714 ) ) ;
#78358=B_SPLINE_CURVE_WITH_KNOTS ( 'NONE', 3,
 ( #31034, #19233, #36946, #37363 ),
 .UNSPECIFIED., .F., .F.,
 ( 4, 4 ),
 ( 3.593986969197074047E-07, 0.001287825409103299885 ),
 .UNSPECIFIED. ) ;
#78360=CARTESIAN_POINT ( 'NONE',  ( -0.7086614173228339419, -0.1870078740157479769, 0.4822834645669291653 ) ) ;
#78362=CARTESIAN_POINT ( 'NONE',  ( 1.443569553805774897, -0.6046776061558809534, -0.2411417322834644161 ) ) ;
#78363=CARTESIAN_POINT ( 'NONE',  ( 1.555118110236221041, 0.07958543189024071263, -0.2665933059059888421 ) ) ;
#78364=ORIENTED_EDGE ( 'NONE', *, *, #82011, .F. ) ;
#78366=CARTESIAN_POINT ( 'NONE',  ( -0.1968503937007867743, 0.2952755905511811885, 0.000000000000000000 ) ) ;
#78368=CARTESIAN_POINT ( 'NONE',  ( -0.9908136482939626788, -0.6692913385826773087, -0.1292274648535924053 ) ) ;
#78369=CARTESIAN_POINT ( 'NONE',  ( 1.594488188976378673, 0.1660481256975885056, 0.3530559997133364547 ) ) ;
#78370=CARTESIAN_POINT ( 'NONE',  ( 1.181102362204724976, -0.1870078740157480879, -0.4822834645669291653 ) ) ;
#78371=CARTESIAN_POINT ( 'NONE',  ( 0.07874015748031558404, -0.1870078740157480879, -0.4822834645669291653 ) ) ;
#78372=AXIS2_PLACEMENT_3D ( 'NONE', #74696, #16206, #23741 ) ;
#78373=CARTESIAN_POINT ( 'NONE',  ( -0.3674540682414689785, 0.2306618581243848609, 0.2411417322834645549 ) ) ;
#78375=CARTESIAN_POINT ( 'NONE',  ( -1.305774278215222184, -0.6692913385826773087, -0.1292274648535924053 ) ) ;
#78376=CARTESIAN_POINT ( 'NONE',  ( -0.7480314960629914633, -0.6692913385826771977, 8.415575281601705876E-17 ) ) ;
#78377=CARTESIAN_POINT ( 'NONE',  ( 0.03937007874015833325, -0.5511811023622047445, 6.969142054262312111E-17 ) ) ;
#78378=CARTESIAN_POINT ( 'NONE',  ( 1.653543307086614789, -0.1870078740157479769, 0.4822834645669291653 ) ) ;
#78380=CARTESIAN_POINT ( 'NONE',  ( -0.4921259842519677963, -0.5400638737290844871, 0.3530559997133364547 ) ) ;
#78381=CARTESIAN_POINT ( 'NONE',  ( -0.2486400153428821869, 2.660739321503277841E-15, -0.3464511005275191513 ) ) ;
#78382=CARTESIAN_POINT ( 'NONE',  ( 0.6692913385826777528, 0.2952755905511811885, 0.000000000000000000 ) ) ;
#78385=CARTESIAN_POINT ( 'NONE',  ( -0.1509186351706028884, -0.3162353388693409650, -0.4822834645669289433 ) ) ;
#78386=CARTESIAN_POINT ( 'NONE',  ( -0.3280839895013117347, -0.3690944881889763329, 0.3153832671262228327 ) ) ;
#78387=CARTESIAN_POINT ( 'NONE',  ( 1.076115485564305141, 0.1283753931104746893, -0.1820866141732285504 ) ) ;
#78388=CARTESIAN_POINT ( 'NONE',  ( 0.6979622409133220406, -4.135162568743707313E-16, -0.4118484887281965157 ) ) ;
#78391=CARTESIAN_POINT ( 'NONE',  ( 1.030183727034121421, -0.3162353388693409650, -0.4822834645669289433 ) ) ;
#78393=CARTESIAN_POINT ( 'NONE',  ( 0.09186351706036799403, -0.4281496062992127816, -0.4176697321401328100 ) ) ;
#78394=CARTESIAN_POINT ( 'NONE',  ( -1.456692913385826182, 0.2952755905511811885, 0.000000000000000000 ) ) ;
#78395=CARTESIAN_POINT ( 'NONE',  ( -1.469816272965878357, -0.6046776061558809534, -0.2411417322834644161 ) ) ;
#78396=CARTESIAN_POINT ( 'NONE',  ( 0.04593175853018440641, 0.2952755905511810774, -0.1292274648535930714 ) ) ;
#78398=CARTESIAN_POINT ( 'NONE',  ( -1.548556430446193399, -0.5023911411419708095, -0.1820866141732282451 ) ) ;
#78399=CARTESIAN_POINT ( 'NONE',  ( 0.4593175853018379162, -0.4281496062992124485, 0.4176697321401328655 ) ) ;
#78400=CARTESIAN_POINT ( 'NONE',  ( 1.082677165354331228, 0.07958543189024071263, -0.2665933059059888421 ) ) ;
#78401=CARTESIAN_POINT ( 'NONE',  ( -0.01000891935578489267, 8.471767977567108961E-16, -0.4445507791589058955 ) ) ;
#78402=CARTESIAN_POINT ( 'NONE',  ( 0.4724409448818904789, -0.1870078740157480601, -0.3641732283464567677 ) ) ;
#78403=CARTESIAN_POINT ( 'NONE',  ( -1.338582677165353729, -0.1870078740157479769, 0.4822834645669291653 ) ) ;
#78406=CARTESIAN_POINT ( 'NONE',  ( 1.272965879265092637, -0.4281496062992127816, -0.4176697321401328100 ) ) ;
#78410=CARTESIAN_POINT ( 'NONE',  ( 0.4921259842519691285, -0.5400638737290845981, -0.3530559997133363437 ) ) ;
#78411=DIRECTION ( 'NONE',  ( -0.8479387356305989609, -2.625811289636361676E-16, -0.5300942374872427143 ) ) ;
#78412=DIRECTION ( 'NONE',  ( -0.4999999999999902855, 0.7071067811865615615, 0.4999999999999899525 ) ) ;
#78413=CARTESIAN_POINT ( 'NONE',  ( 0.3740157480314966754, 0.07958543189024071263, -0.2665933059059888421 ) ) ;
#78414=B_SPLINE_CURVE_WITH_KNOTS ( 'NONE', 3,
 ( #24599, #32157, #38468, #5249 ),
 .UNSPECIFIED., .F., .F.,
 ( 4, 4 ),
 ( 0.07436403195037287472, 0.07455104739251855461 ),
 .UNSPECIFIED. ) ;
#78415=CARTESIAN_POINT ( 'NONE',  ( 0.5314960629921267055, -0.5400638737290844871, 0.3530559997133364547 ) ) ;
#78416=CARTESIAN_POINT ( 'NONE',  ( 0.7217847769028878924, 0.009842519685039467087, 0.3409548833797002021 ) ) ;
#78417=CARTESIAN_POINT ( 'NONE',  ( -0.7677165354330699465, 0.07958543189024085140, 0.2665933059059887866 ) ) ;
#78418=CARTESIAN_POINT ( 'NONE',  ( -1.220472440944881054, 0.2952755905511811885, 0.000000000000000000 ) ) ;
#78420=CARTESIAN_POINT ( 'NONE',  ( -1.430446194225721390, -0.4281496062992124485, 0.4176697321401328655 ) ) ;
#78421=CARTESIAN_POINT ( 'NONE',  ( 1.154855643044620184, -0.6046776061558807314, 0.2411417322834647770 ) ) ;
#78422=CARTESIAN_POINT ( 'NONE',  ( 1.522309711286089939, 0.2306618581243848609, 0.2411417322834645549 ) ) ;
#78424=CARTESIAN_POINT ( 'NONE',  ( 0.5577427821522314977, -0.3162353388693409650, -0.4822834645669289433 ) ) ;
#78427=CARTESIAN_POINT ( 'NONE',  ( 1.345144356955381593, -0.05778040916215522460, 0.4822834645669289988 ) ) ;
#78428=CARTESIAN_POINT ( 'NONE',  ( -1.286089238845143479, -0.5023911411419708095, 0.1820866141732285504 ) ) ;
#78429=CARTESIAN_POINT ( 'NONE',  ( 1.135170603674541256, -0.5511811023622048555, -0.09757992244046775898 ) ) ;
#78430=CARTESIAN_POINT ( 'NONE',  ( -1.292650918635170010, 0.1771653543307087075, -0.09757992244046823083 ) ) ;
#78431=CARTESIAN_POINT ( 'NONE',  ( -0.3346456692913377662, 0.07958543189024071263, -0.2665933059059888421 ) ) ;
#78433=CARTESIAN_POINT ( 'NONE',  ( 0.3412073490813655186, 0.1283753931104748280, 0.1820866141732283561 ) ) ;
#78434=VECTOR ( 'NONE', #34117, 39.37007874015748143 ) ;
#78435=CARTESIAN_POINT ( 'NONE',  ( 0.7020997375328090762, -0.3162353388693405765, 0.4822834645669290543 ) ) ;
#78436=CARTESIAN_POINT ( 'NONE',  ( 0.9251968503937015864, -0.5400638737290844871, 0.3530559997133364547 ) ) ;
#78437=CARTESIAN_POINT ( 'NONE',  ( 0.07874015748031558404, -0.1870078740157479769, 0.4822834645669291653 ) ) ;
#78438=CARTESIAN_POINT ( 'NONE',  ( 0.09842519685039434474, -0.4536011799217368745, -0.2665933059059886201 ) ) ;
#78439=CARTESIAN_POINT ( 'NONE',  ( 1.397637795275591177, -0.5400638737290844871, 0.3530559997133364547 ) ) ;
#78440=CARTESIAN_POINT ( 'NONE',  ( -0.1902887139107604098, 0.2066929133858267098, -0.1054918080437494132 ) ) ;
#78441=CARTESIAN_POINT ( 'NONE',  ( -0.6233595800524928121, -0.05778040916215522460, 0.4822834645669289988 ) ) ;
#78444=CARTESIAN_POINT ( 'NONE',  ( 0.1902887139107617975, 0.2952755905511811885, 0.1292274648535926551 ) ) ;
#78445=CARTESIAN_POINT ( 'NONE',  ( -0.7545931758530176614, -0.6692913385826773087, -0.1292274648535924053 ) ) ;
#78446=CARTESIAN_POINT ( 'NONE',  ( -0.2493438320209966919, 0.05413385826771626580, -0.4176697321401330321 ) ) ;
#78451=CARTESIAN_POINT ( 'NONE',  ( -0.9842519685039365918, -0.5511811023622047445, 6.969142054262312111E-17 ) ) ;
#78453=CARTESIAN_POINT ( 'NONE',  ( -1.673228346456691717, 0.1660481256975883668, -0.3530559997133364547 ) ) ;
#78456=CARTESIAN_POINT ( 'NONE',  ( 0.6167979002624679463, 0.05413385826771626580, -0.4176697321401330321 ) ) ;
#78457=CARTESIAN_POINT ( 'NONE',  ( -0.4002624671916004129, -0.08942795157528024563, -0.3641732283464568787 ) ) ;
#78458=CARTESIAN_POINT ( 'NONE',  ( 1.358267716535433323, -0.5400638737290845981, -0.3530559997133363437 ) ) ;
#78459=CARTESIAN_POINT ( 'NONE',  ( 0.2296587926509192634, -0.05778040916215560624, -0.4822834645669293319 ) ) ;
#78463=CARTESIAN_POINT ( 'NONE',  ( 1.397637795275591177, 0.1660481256975883668, -0.3530559997133364547 ) ) ;
#78464=CARTESIAN_POINT ( 'NONE',  ( 0.5314960629921264834, 0.1660481256975883668, -0.3530559997133364547 ) ) ;
#78465=CARTESIAN_POINT ( 'NONE',  ( 0.2165354330708668673, 0.1660481256975883668, -0.3530559997133364547 ) ) ;
#78466=CARTESIAN_POINT ( 'NONE',  ( 1.397637795275591177, -0.5400638737290844871, 0.3530559997133364547 ) ) ;
#78467=CARTESIAN_POINT ( 'NONE',  ( 0.7414698162729663755, 0.2952755905511811885, 0.1292274648535926551 ) ) ;
#78469=CARTESIAN_POINT ( 'NONE',  ( 0.2493438320209980519, -0.4281496062992127816, -0.4176697321401328100 ) ) ;
#78470=CARTESIAN_POINT ( 'NONE',  ( 1.200787401574803681, 0.1660481256975885056, 0.3530559997133364547 ) ) ;
#78471=CARTESIAN_POINT ( 'NONE',  ( 0.2755905511811031494, 0.2952755905511811885, 0.000000000000000000 ) ) ;
#78472=AXIS2_PLACEMENT_3D ( 'NONE', #76128, #56339, #25173 ) ;
#78473=CARTESIAN_POINT ( 'NONE',  ( 1.338582677165355062, -0.1870078740157479769, 0.3641732283464567677 ) ) ;
#78474=CARTESIAN_POINT ( 'NONE',  ( -1.417322834645668772, -0.1870078740157479769, 0.4822834645669291653 ) ) ;
#78475=CARTESIAN_POINT ( 'NONE',  ( -1.259842519685038686, -0.1870078740157479769, 0.4822834645669291653 ) ) ;
#78476=CARTESIAN_POINT ( 'NONE',  ( 0.7939632545931766261, -0.05778040916215522460, 0.4822834645669289988 ) ) ;
#78481=ORIENTED_EDGE ( 'NONE', *, *, #3931, .T. ) ;
#78482=CARTESIAN_POINT ( 'NONE',  ( 1.174540682414699111, -0.3162353388693405765, 0.4822834645669290543 ) ) ;
#78483=CARTESIAN_POINT ( 'NONE',  ( 0.8005249343832027131, -0.004921259842519576551, 0.3153832671262227771 ) ) ;
#78485=B_SPLINE_CURVE_WITH_KNOTS ( 'NONE', 3,
 ( #63606, #62791, #11450, #56864 ),
 .UNSPECIFIED., .F., .F.,
 ( 4, 4 ),
 ( 2.687447247556935660E-15, 0.002136818956430557546 ),
 .UNSPECIFIED. ) ;
#78490=CARTESIAN_POINT ( 'NONE',  ( 1.410761154855643795, -0.3162353388693405765, 0.4822834645669290543 ) ) ;
#78492=CARTESIAN_POINT ( 'NONE',  ( -0.3346456692913377662, -0.5400638737290844871, 0.3530559997133364547 ) ) ;
#78493=CARTESIAN_POINT ( 'NONE',  ( 0.9514435695538062676, -0.05778040916215522460, 0.4822834645669289988 ) ) ;
#78494=VERTEX_POINT ( 'NONE', #2441 ) ;
#78495=CARTESIAN_POINT ( 'NONE',  ( -1.568241469816272105, -0.05778040916215522460, 0.4822834645669289988 ) ) ;
#78498=CARTESIAN_POINT ( 'NONE',  ( -1.614173228346457378, 0.7794589730111968207, -0.1372047244094477536 ) ) ;
#78499=CARTESIAN_POINT ( 'NONE',  ( -0.3038629456265427575, -2.551093532135090261E-15, 0.3954974714151479609 ) ) ;
#78500=CARTESIAN_POINT ( 'NONE',  ( -1.017060367454067249, -0.08942795157527998196, 0.3641732283464567121 ) ) ;
#78501=EDGE_CURVE ( 'NONE', #56774, #10845, #81609, .T. ) ;
#78502=CARTESIAN_POINT ( 'NONE',  ( 0.8785612751854029456, 3.421639014772782816E-16, 0.3464511005275203726 ) ) ;
#78503=CARTESIAN_POINT ( 'NONE',  ( 0.7480314960629927956, 0.2952755905511811885, 0.000000000000000000 ) ) ;
#78504=EDGE_LOOP ( 'NONE', ( #57030, #78481, #62211, #50166, #28324 ) ) ;
#78505=LINE ( 'NONE', #13687, #1976 ) ;
#78506=CARTESIAN_POINT ( 'NONE',  ( -0.4064735117398301512, 0.004960608223778500969, -0.3437734562760191848 ) ) ;
#78507=CARTESIAN_POINT ( 'NONE',  ( 0.7349081364829403995, 0.2306618581243848609, 0.2411417322834645549 ) ) ;
#78508=CARTESIAN_POINT ( 'NONE',  ( 1.496062992125984703, -0.1870078740157480601, -0.3641732283464567677 ) ) ;
#78510=CARTESIAN_POINT ( 'NONE',  ( -0.7545931758530177724, 0.1771653543307087630, 0.09757992244046791164 ) ) ;
#78511=CARTESIAN_POINT ( 'NONE',  ( -1.522309711286088607, -0.5023911411419708095, 0.1820866141732285504 ) ) ;
#78513=CARTESIAN_POINT ( 'NONE',  ( 0.4986876640419954376, 0.2306618581243848609, 0.2411417322834645549 ) ) ;
#78514=CARTESIAN_POINT ( 'NONE',  ( -1.122047244094487306, 0.07958543189024071263, -0.2665933059059888421 ) ) ;
#78515=CARTESIAN_POINT ( 'NONE',  ( -0.03280839895013062252, -0.5511811023622046335, 0.09757992244046803654 ) ) ;
#78516=CARTESIAN_POINT ( 'NONE',  ( -0.3149606299212590610, -0.1870078740157479769, 0.4822834645669291653 ) ) ;
#78517=CARTESIAN_POINT ( 'NONE',  ( -1.062992125984250968, -0.5511811023622047445, 6.969142054262312111E-17 ) ) ;
#78519=CARTESIAN_POINT ( 'NONE',  ( 0.5839895013123367340, -0.6692913385826773087, -0.1292274648535924053 ) ) ;
#78522=CARTESIAN_POINT ( 'NONE',  ( -0.9317585301837263412, 0.05413385826771666132, 0.4176697321401328100 ) ) ;
#78523=CARTESIAN_POINT ( 'NONE',  ( -0.3018372703412066094, -0.004921259842519576551, 0.3153832671262227771 ) ) ;
#78524=EDGE_CURVE ( 'NONE', #32475, #33739, #17149, .T. ) ;
#78525=CARTESIAN_POINT ( 'NONE',  ( -1.437007874015747477, 0.1660481256975883668, -0.3530559997133364547 ) ) ;
#78526=CARTESIAN_POINT ( 'NONE',  ( 0.8070866141732289112, -0.4536011799217368745, -0.2665933059059886201 ) ) ;
#78527=CARTESIAN_POINT ( 'NONE',  ( -0.8727034120734901146, -0.08942795157528024563, -0.3641732283464568787 ) ) ;
#78528=CARTESIAN_POINT ( 'NONE',  ( -1.227034120734907585, 0.2952755905511811885, 0.1292274648535926551 ) ) ;
#78529=CARTESIAN_POINT ( 'NONE',  ( -1.062992125984250968, 0.2952755905511811885, 0.000000000000000000 ) ) ;
#78530=CARTESIAN_POINT ( 'NONE',  ( 1.640419947506562393, -0.4281496062992124485, 0.4176697321401328655 ) ) ;
#78531=CARTESIAN_POINT ( 'NONE',  ( 0.7874015748031503170, -0.1870078740157480601, -0.3641732283464567677 ) ) ;
#78533=CARTESIAN_POINT ( 'NONE',  ( 0.1968503937007881344, -0.6692913385826771977, 8.415575281601705876E-17 ) ) ;
#78535=CARTESIAN_POINT ( 'NONE',  ( -1.574803149606298192, -0.1870078740157480879, -0.4822834645669291653 ) ) ;
#78536=CARTESIAN_POINT ( 'NONE',  ( -1.574803149606298636, -0.1870078740157479769, 0.4822834645669291653 ) ) ;
#78537=VERTEX_POINT ( 'NONE', #49516 ) ;
#78539=CARTESIAN_POINT ( 'NONE',  ( -1.443569553805773564, 0.1283753931104746893, -0.1820866141732285504 ) ) ;
#78540=CARTESIAN_POINT ( 'NONE',  ( -0.6233595800524928121, -0.3162353388693409650, -0.4822834645669289433 ) ) ;
#78541=CARTESIAN_POINT ( 'NONE',  ( 0.8464566929133865436, 0.1660481256975883668, -0.3530559997133364547 ) ) ;
#78542=CARTESIAN_POINT ( 'NONE',  ( -1.456692913385826182, -0.5511811023622047445, 6.969142054262312111E-17 ) ) ;
#78544=CARTESIAN_POINT ( 'NONE',  ( -1.594488188976377563, -0.5400638737290844871, 0.3530559997133364547 ) ) ;
#78545=CARTESIAN_POINT ( 'NONE',  ( 1.030183727034121421, -0.05778040916215522460, 0.4822834645669289988 ) ) ;
#78546=CARTESIAN_POINT ( 'NONE',  ( 0.3543307086614181922, -0.6692913385826771977, 8.415575281601705876E-17 ) ) ;
#78547=CARTESIAN_POINT ( 'NONE',  ( 1.364829396325459854, -0.6046776061558809534, -0.2411417322834644161 ) ) ;
#78548=PLANE ( 'NONE',  #73530 ) ;
#78553=CARTESIAN_POINT ( 'NONE',  ( 0.3674540682414705883, 0.1283753931104746893, -0.1820866141732285504 ) ) ;
#78554=CARTESIAN_POINT ( 'NONE',  ( 0.2165354330708668673, 0.1660481256975883668, -0.3530559997133364547 ) ) ;
#78555=CARTESIAN_POINT ( 'NONE',  ( 1.358267716535433323, -0.5400638737290845981, -0.3530559997133363437 ) ) ;
#78557=CARTESIAN_POINT ( 'NONE',  ( 0.3937007874015754361, -0.1870078740157479769, 0.3641732283464567677 ) ) ;
#78558=CARTESIAN_POINT ( 'NONE',  ( -0.5446194225721777693, -0.05778040916215522460, 0.4822834645669289988 ) ) ;
#78559=CARTESIAN_POINT ( 'NONE',  ( 1.496062992125984703, -0.1870078740157480879, -0.4822834645669291653 ) ) ;
#78560=CARTESIAN_POINT ( 'NONE',  ( 0.4527559055118117182, 0.1660481256975883668, -0.3530559997133364547 ) ) ;
#78563=ORIENTED_EDGE ( 'NONE', *, *, #18464, .T. ) ;
#78564=VERTEX_POINT ( 'NONE', #55000 ) ;
#78565=CARTESIAN_POINT ( 'NONE',  ( 1.535433070866142335, -0.5511811023622047445, 6.969142054262312111E-17 ) ) ;
#78566=CARTESIAN_POINT ( 'NONE',  ( -1.010498687664041384, -0.004921259842519576551, 0.3153832671262227771 ) ) ;
#78567=CARTESIAN_POINT ( 'NONE',  ( -1.174540682414697335, -0.05778040916215522460, 0.4822834645669289988 ) ) ;
#78570=CARTESIAN_POINT ( 'NONE',  ( 1.482939632545932307, -0.4281496062992124485, 0.4176697321401328655 ) ) ;
#78571=CARTESIAN_POINT ( 'NONE',  ( -1.272965879265091305, -0.4281496062992124485, 0.4176697321401328655 ) ) ;
#78572=CARTESIAN_POINT ( 'NONE',  ( 0.5118110236220478892, 0.2952755905511811885, 0.000000000000000000 ) ) ;
#78573=CARTESIAN_POINT ( 'NONE',  ( -1.167979002624671470, 0.05413385826771666132, 0.4176697321401328100 ) ) ;
#78575=CARTESIAN_POINT ( 'NONE',  ( 0.6758530183727039509, 0.2952755905511810774, -0.1292274648535930714 ) ) ;
#78577=CARTESIAN_POINT ( 'NONE',  ( -1.082677165354329896, -0.4536011799217368745, -0.2665933059059886201 ) ) ;
#78580=EDGE_LOOP ( 'NONE', ( #32075, #5686, #2467, #16021 ) ) ;
#78581=CARTESIAN_POINT ( 'NONE',  ( -1.679790026246718693, 0.1283753931104746893, -0.1820866141732285504 ) ) ;
#78582=CARTESIAN_POINT ( 'NONE',  ( -0.9645669291338575535, -0.5400638737290844871, 0.3530559997133364547 ) ) ;
#78583=CARTESIAN_POINT ( 'NONE',  ( -1.312335958005248715, 0.2306618581243848609, 0.2411417322834645549 ) ) ;
#78585=CARTESIAN_POINT ( 'NONE',  ( -1.712598425196849572, 0.1660481256975885056, 0.3530559997133364547 ) ) ;
#78586=CARTESIAN_POINT ( 'NONE',  ( -1.561679790026246017, 0.05413385826771666132, 0.4176697321401328100 ) ) ;
#78587=CARTESIAN_POINT ( 'NONE',  ( -1.653543307086613234, -0.1870078740157479769, 0.4822834645669291653 ) ) ;
#78588=DIRECTION ( 'NONE',  ( -1.000000000000000000, 0.000000000000000000, 0.000000000000000000 ) ) ;
#78590=CARTESIAN_POINT ( 'NONE',  ( 0.09186351706036827158, -0.004921259842519576551, 0.3153832671262227771 ) ) ;
#78593=CARTESIAN_POINT ( 'NONE',  ( -0.9776902887139098386, -0.5511811023622046335, 0.09757992244046803654 ) ) ;
#78595=CARTESIAN_POINT ( 'NONE',  ( -0.5905511811023613777, -0.6692913385826771977, 8.415575281601705876E-17 ) ) ;
#78596=CARTESIAN_POINT ( 'NONE',  ( 0.9711286089238851948, 0.2306618581243848609, 0.2411417322834645549 ) ) ;
#78597=CARTESIAN_POINT ( 'NONE',  ( -0.8202099737532799750, 0.2952755905511810774, -0.1292274648535930714 ) ) ;
#78598=EDGE_LOOP ( 'NONE', ( #49215, #49233, #41279, #9723 ) ) ;
#78600=CARTESIAN_POINT ( 'NONE',  ( -1.010498687664041384, 0.05413385826771666132, 0.4176697321401328100 ) ) ;
#78601=CARTESIAN_POINT ( 'NONE',  ( 0.7086614173228352742, -0.1870078740157480879, -0.4822834645669291653 ) ) ;
#78602=CARTESIAN_POINT ( 'NONE',  ( -1.456692913385826182, -0.5511811023622047445, 6.969142054262312111E-17 ) ) ;
#78603=CARTESIAN_POINT ( 'NONE',  ( -1.673228346456691717, 0.1660481256975883668, -0.3530559997133364547 ) ) ;
#78608=CARTESIAN_POINT ( 'NONE',  ( -0.4527559055118102749, -0.5400638737290845981, -0.3530559997133363437 ) ) ;
#78609=CARTESIAN_POINT ( 'NONE',  ( -1.541994750656167090, -0.5511811023622048555, -0.09757992244046775898 ) ) ;
#78611=CARTESIAN_POINT ( 'NONE',  ( -1.266404199475064773, -0.3162353388693405765, 0.4822834645669290543 ) ) ;
#78613=CARTESIAN_POINT ( 'NONE',  ( -1.489501312335957062, -0.3162353388693409650, -0.4822834645669289433 ) ) ;
#78614=CARTESIAN_POINT ( 'NONE',  ( -0.3215223097112853146, -0.3162353388693405765, 0.4822834645669290543 ) ) ;
#78615=CIRCLE ( 'NONE', #61105, 2.401574803149606474 ) ;
#78617=CARTESIAN_POINT ( 'NONE',  ( 0.4265091863517067039, -0.5511811023622048555, -0.09757992244046775898 ) ) ;
#78618=FACE_OUTER_BOUND ( 'NONE', #79019, .T. ) ;
#78619=CARTESIAN_POINT ( 'NONE',  ( 0.3608923884514443348, -0.5511811023622046335, 0.09757992244046803654 ) ) ;
#78620=CARTESIAN_POINT ( 'NONE',  ( 1.456692913385827515, 0.1771653543307087630, 0.000000000000000000 ) ) ;
#78621=CARTESIAN_POINT ( 'NONE',  ( 0.8595800524934390507, -0.05778040916215560624, -0.4822834645669293319 ) ) ;
#78622=CARTESIAN_POINT ( 'NONE',  ( 0.01968503937007957949, -0.4536011799217368745, -0.2665933059059886201 ) ) ;
#78624=CARTESIAN_POINT ( 'NONE',  ( -1.286089238845143479, 0.2306618581243847221, -0.2411417322834647770 ) ) ;
#78625=CARTESIAN_POINT ( 'NONE',  ( 0.05249343832021075018, 0.1283753931104746893, -0.1820866141732285504 ) ) ;
#78627=CARTESIAN_POINT ( 'NONE',  ( -0.4593175853018364174, -0.3690944881889765550, -0.3153832671262227771 ) ) ;
#78630=CARTESIAN_POINT ( 'NONE',  ( -0.03937007874015669567, 0.2952755905511811885, 0.000000000000000000 ) ) ;
#78632=CARTESIAN_POINT ( 'NONE',  ( 0.6364829396325465405, -0.08942795157527998196, 0.3641732283464567121 ) ) ;
#78633=CARTESIAN_POINT ( 'NONE',  ( -0.1640419947506555343, -0.2845877964562159024, 0.3641732283464567677 ) ) ;
#78634=CARTESIAN_POINT ( 'NONE',  ( -0.3083989501312330295, -0.3162353388693409650, -0.4822834645669289433 ) ) ;
#78636=CARTESIAN_POINT ( 'NONE',  ( -1.318897637795274802, 0.07958543189024085140, 0.2665933059059887866 ) ) ;
#78638=CARTESIAN_POINT ( 'NONE',  ( 0.5314960629921267055, -0.5400638737290844871, 0.3530559997133364547 ) ) ;
#78639=CARTESIAN_POINT ( 'NONE',  ( -0.9973753280839886548, 0.2306618581243848609, 0.2411417322834645549 ) ) ;
#78642=CARTESIAN_POINT ( 'NONE',  ( 0.3805774278215230400, -0.004921259842519870586, -0.3153832671262229437 ) ) ;
#78643=CARTESIAN_POINT ( 'NONE',  ( -1.312335958005248715, 0.2306618581243848609, 0.2411417322834645549 ) ) ;
#78644=CARTESIAN_POINT ( 'NONE',  ( -1.115485564304461219, -0.004921259842519870586, -0.3153832671262229437 ) ) ;
#78645=CARTESIAN_POINT ( 'NONE',  ( 1.692913385826772421, 0.2952755905511811885, 0.000000000000000000 ) ) ;
#78647=CARTESIAN_POINT ( 'NONE',  ( -0.9251968503937002541, -0.4536011799217368745, -0.2665933059059886201 ) ) ;
#78649=CARTESIAN_POINT ( 'NONE',  ( 0.9448818897637802916, -0.1870078740157479769, 0.4822834645669291653 ) ) ;
#78654=CARTESIAN_POINT ( 'NONE',  ( -1.712598425196849572, 0.1660481256975885056, 0.3530559997133364547 ) ) ;
#78655=CARTESIAN_POINT ( 'NONE',  ( -1.108923884514435132, -0.3162353388693405765, 0.4822834645669290543 ) ) ;
#78656=CARTESIAN_POINT ( 'NONE',  ( 1.207349081364829990, -0.6046776061558809534, -0.2411417322834644161 ) ) ;
#78658=CARTESIAN_POINT ( 'NONE',  ( 1.561679790026247350, -0.004921259842519870586, -0.3153832671262229437 ) ) ;
#78659=CARTESIAN_POINT ( 'NONE',  ( 0.3608923884514443348, -0.6692913385826771977, 0.1292274648535927661 ) ) ;
#78660=CARTESIAN_POINT ( 'NONE',  ( -0.2624671916010490880, -0.6046776061558807314, 0.2411417322834647770 ) ) ;
#78661=CARTESIAN_POINT ( 'NONE',  ( 1.555118110236221041, 0.1660481256975883668, -0.3530559997133364547 ) ) ;
#78663=CARTESIAN_POINT ( 'NONE',  ( 0.5839895013123367340, -0.5511811023622048555, -0.09757992244046775898 ) ) ;
#78669=CARTESIAN_POINT ( 'NONE',  ( 0.1246719160104994284, -0.6692913385826771977, 0.1292274648535927661 ) ) ;
#78670=CARTESIAN_POINT ( 'NONE',  ( 1.220472440944882386, -0.6692913385826771977, 8.415575281601705876E-17 ) ) ;
#78671=CARTESIAN_POINT ( 'NONE',  ( 0.2624671916010504757, 0.2306618581243848609, 0.2411417322834645549 ) ) ;
#78672=CARTESIAN_POINT ( 'NONE',  ( -0.5708661417322825615, -0.4536011799217367080, 0.2665933059059888421 ) ) ;
#78673=CARTESIAN_POINT ( 'NONE',  ( 1.200787401574803681, 0.1660481256975885056, 0.3530559997133364547 ) ) ;
#78674=CARTESIAN_POINT ( 'NONE',  ( -0.3018372703412066094, -0.4281496062992127816, -0.4176697321401328100 ) ) ;
#78675=CARTESIAN_POINT ( 'NONE',  ( 0.1049868766404206816, -0.6046776061558809534, -0.2411417322834644161 ) ) ;
#78676=CARTESIAN_POINT ( 'NONE',  ( -1.640419947506561060, 0.05413385826771666132, 0.4176697321401328100 ) ) ;
#78677=CARTESIAN_POINT ( 'NONE',  ( 1.030183727034121421, -0.3162353388693409650, -0.4822834645669289433 ) ) ;
#78678=CARTESIAN_POINT ( 'NONE',  ( 1.135170603674541256, -0.6692913385826773087, -0.1292274648535924053 ) ) ;
#78680=CARTESIAN_POINT ( 'NONE',  ( 0.5905511811023629321, 0.1771653543307087630, 0.000000000000000000 ) ) ;
#78681=ORIENTED_EDGE ( 'NONE', *, *, #1687, .T. ) ;
#78683=ORIENTED_EDGE ( 'NONE', *, *, #41951, .F. ) ;
#78684=CARTESIAN_POINT ( 'NONE',  ( -0.2821522309711278487, 0.1771653543307087630, 0.09757992244046791164 ) ) ;
#78685=CARTESIAN_POINT ( 'NONE',  ( 0.1181102362204730916, 0.2952755905511811885, 0.000000000000000000 ) ) ;
#78687=CARTESIAN_POINT ( 'NONE',  ( -0.2427821522309703550, -0.05778040916215560624, -0.4822834645669293319 ) ) ;
#78688=CARTESIAN_POINT ( 'NONE',  ( -0.2887139107611542133, 0.2306618581243848609, 0.2411417322834645549 ) ) ;
#78689=CARTESIAN_POINT ( 'NONE',  ( -0.8070866141732276899, 0.1660481256975883668, -0.3530559997133364547 ) ) ;
#78690=CARTESIAN_POINT ( 'NONE',  ( -1.167979002624671470, -0.4281496062992127816, -0.4176697321401328100 ) ) ;
#78691=CARTESIAN_POINT ( 'NONE',  ( 1.154855643044620184, -0.5023911411419708095, 0.1820866141732285504 ) ) ;
#78692=LINE ( 'NONE', #21015, #907 ) ;
#78694=CARTESIAN_POINT ( 'NONE',  ( 0.7808398950131240079, -0.2845877964562159024, 0.3641732283464567677 ) ) ;
#78695=CARTESIAN_POINT ( 'NONE',  ( 0.4855643044619430415, -0.4281496062992127816, -0.4176697321401328100 ) ) ;
#78696=CARTESIAN_POINT ( 'NONE',  ( 0.3871391076115493490, -0.3162353388693405765, 0.4822834645669290543 ) ) ;
#78698=CARTESIAN_POINT ( 'NONE',  ( -1.607611548556429737, -0.6692913385826771977, 0.1292274648535927661 ) ) ;
#78701=CARTESIAN_POINT ( 'NONE',  ( -0.3740157480314953431, -0.5400638737290845981, -0.3530559997133363437 ) ) ;
#78704=CARTESIAN_POINT ( 'NONE',  ( -1.345144356955379816, -0.2845877964562159024, 0.3641732283464567677 ) ) ;
#78705=CARTESIAN_POINT ( 'NONE',  ( 0.9776902887139113929, 0.2952755905511811885, 0.1292274648535926551 ) ) ;
#78706=CARTESIAN_POINT ( 'NONE',  ( 0.9842519685039378130, -0.6692913385826771977, 8.415575281601705876E-17 ) ) ;
#78707=CARTESIAN_POINT ( 'NONE',  ( -0.1574803149606292529, -0.1870078740157480601, -0.3641732283464567677 ) ) ;
#78708=CARTESIAN_POINT ( 'NONE',  ( 0.4330708661417329575, -0.6692913385826771977, 8.415575281601705876E-17 ) ) ;
#78710=CARTESIAN_POINT ( 'NONE',  ( -0.2755905511811015396, -0.5511811023622047445, 6.969142054262312111E-17 ) ) ;
#78711=CARTESIAN_POINT ( 'NONE',  ( -0.1968503937007867743, -0.6692913385826771977, 8.415575281601705876E-17 ) ) ;
#78713=CARTESIAN_POINT ( 'NONE',  ( -1.653543307086613234, -0.1870078740157480879, -0.4822834645669291653 ) ) ;
#78714=CARTESIAN_POINT ( 'NONE',  ( 0.6692913385826777528, 0.1771653543307087630, 0.000000000000000000 ) ) ;
#78715=CARTESIAN_POINT ( 'NONE',  ( 1.601049868766404982, -0.5023911411419708095, -0.1820866141732282451 ) ) ;
#78716=CARTESIAN_POINT ( 'NONE',  ( -0.6692913385826764205, -0.6692913385826771977, 8.415575281601705876E-17 ) ) ;
#78717=CARTESIAN_POINT ( 'NONE',  ( -0.7677165354330699465, -0.4536011799217368745, -0.2665933059059886201 ) ) ;
#78719=CARTESIAN_POINT ( 'NONE',  ( -0.6824146981627291497, -0.6046776061558809534, -0.2411417322834644161 ) ) ;
#78720=CARTESIAN_POINT ( 'NONE',  ( -0.5839895013123351797, -0.6692913385826771977, 0.1292274648535927661 ) ) ;
#78721=CARTESIAN_POINT ( 'NONE',  ( -0.1443569553805765515, -0.4281496062992127816, -0.4176697321401328100 ) ) ;
#78727=CARTESIAN_POINT ( 'NONE',  ( 0.8202099737532814183, -0.5511811023622048555, -0.09757992244046775898 ) ) ;
#78728=CARTESIAN_POINT ( 'NONE',  ( 1.227034120734908917, -0.6692913385826771977, 0.1292274648535927661 ) ) ;
#78729=CARTESIAN_POINT ( 'NONE',  ( -1.358267716535432434, 0.07958543189024071263, -0.2665933059059888421 ) ) ;
#78730=CARTESIAN_POINT ( 'NONE',  ( -1.023622047244094002, -0.1870078740157480601, -0.3641732283464567677 ) ) ;
#78731=ADVANCED_FACE ( 'NONE', ( #56244 ), #62608, .F. ) ;
#78732=CARTESIAN_POINT ( 'NONE',  ( -0.5511811023622041894, -0.1870078740157480879, -0.4822834645669291653 ) ) ;
#78733=CARTESIAN_POINT ( 'NONE',  ( 0.6889763779527566800, -0.4536011799217367080, 0.2665933059059888421 ) ) ;
#78735=CARTESIAN_POINT ( 'NONE',  ( 1.141732283464567566, 0.1771653543307087630, 0.000000000000000000 ) ) ;
#78736=CARTESIAN_POINT ( 'NONE',  ( 0.3871391076115493490, -0.3162353388693405765, 0.4822834645669290543 ) ) ;
#78737=DIRECTION ( 'NONE',  ( 0.000000000000000000, 0.000000000000000000, -1.000000000000000000 ) ) ;
#78738=CARTESIAN_POINT ( 'NONE',  ( -0.6824146981627291497, -0.6046776061558809534, -0.2411417322834644161 ) ) ;
#78740=CARTESIAN_POINT ( 'NONE',  ( -1.725721784776902190, -0.05778040916215522460, 0.4822834645669289988 ) ) ;
#78741=CARTESIAN_POINT ( 'NONE',  ( 0.3608923884514443348, -0.6692913385826771977, 0.1292274648535927661 ) ) ;
#78742=CARTESIAN_POINT ( 'NONE',  ( 0.1443569553805781891, 0.05413385826771626580, -0.4176697321401330321 ) ) ;
#78743=CARTESIAN_POINT ( 'NONE',  ( -0.07874015748031421014, -0.1870078740157479769, 0.3641732283464567677 ) ) ;
#78745=CARTESIAN_POINT ( 'NONE',  ( 0.05249343832021075018, -0.5023911411419708095, 0.1820866141732285504 ) ) ;
#78746=CARTESIAN_POINT ( 'NONE',  ( 0.6824146981627303710, -0.6046776061558807314, 0.2411417322834647770 ) ) ;
#78747=CARTESIAN_POINT ( 'NONE',  ( -0.8136482939632537770, -0.5023911411419708095, 0.1820866141732285504 ) ) ;
#78749=CARTESIAN_POINT ( 'NONE',  ( -1.089238845144356427, -0.4281496062992127816, -0.4176697321401328100 ) ) ;
#78750=CARTESIAN_POINT ( 'NONE',  ( 0.1837270341207354329, 0.1539470093639523085, 0.1968503937007873850 ) ) ;
#78752=CARTESIAN_POINT ( 'NONE',  ( -1.187664041994749731, -0.3162353388693405765, 0.4822834645669290543 ) ) ;
#78753=CARTESIAN_POINT ( 'NONE',  ( -1.154855643044618851, -0.5023911411419708095, -0.1820866141732282451 ) ) ;
#78754=CARTESIAN_POINT ( 'NONE',  ( -0.1640419947506555343, -0.3162353388693405765, 0.4822834645669290543 ) ) ;
#78755=CARTESIAN_POINT ( 'NONE',  ( -1.515748031496062076, 0.1660481256975883668, -0.3530559997133364547 ) ) ;
#78756=CARTESIAN_POINT ( 'NONE',  ( -0.8923884514435688198, -0.6046776061558807314, 0.2411417322834647770 ) ) ;
#78757=CARTESIAN_POINT ( 'NONE',  ( -0.1674892343164145203, -2.567464376874931580E-15, -0.4445507791589072832 ) ) ;
#78758=CARTESIAN_POINT ( 'NONE',  ( 0.7611548556430451917, -0.6046776061558807314, 0.2411417322834647770 ) ) ;
#78759=CARTESIAN_POINT ( 'NONE',  ( 0.8070866141732289112, -0.5400638737290845981, -0.3530559997133363437 ) ) ;
#78761=CARTESIAN_POINT ( 'NONE',  ( 1.502624671916010790, -0.3162353388693409650, -0.4822834645669289433 ) ) ;
#78763=CARTESIAN_POINT ( 'NONE',  ( -1.410761154855642463, -0.05778040916215522460, 0.4822834645669289988 ) ) ;
#78766=CARTESIAN_POINT ( 'NONE',  ( -0.4068241469816264999, -0.3690944881889763329, 0.3153832671262228327 ) ) ;
#78769=CARTESIAN_POINT ( 'NONE',  ( 0.4527559055118117182, -0.5400638737290844871, 0.3530559997133364547 ) ) ;
#78770=CARTESIAN_POINT ( 'NONE',  ( 0.03280839895013198948, 0.2952755905511811885, 0.1292274648535926551 ) ) ;
#78771=CARTESIAN_POINT ( 'NONE',  ( -0.7086614173228339419, -0.1870078740157479769, 0.4822834645669291653 ) ) ;
#78772=CARTESIAN_POINT ( 'NONE',  ( 1.384514435695538559, 0.2952755905511810774, -0.1292274648535930714 ) ) ;
#78773=CARTESIAN_POINT ( 'NONE',  ( -0.8333333333333323711, 0.1771653543307087630, 0.09757992244046791164 ) ) ;
#78775=CARTESIAN_POINT ( 'NONE',  ( 0.6299212598425204535, -0.1870078740157480879, -0.4822834645669291653 ) ) ;
#78776=CARTESIAN_POINT ( 'NONE',  ( 0.4724409448818904789, -0.1870078740157479769, 0.3641732283464567677 ) ) ;
#78777=CARTESIAN_POINT ( 'NONE',  ( -0.4330708661417315697, -0.6692913385826771977, 8.415575281601705876E-17 ) ) ;
#78779=CARTESIAN_POINT ( 'NONE',  ( -0.9776902887139098386, 0.2952755905511810774, -0.1292274648535930714 ) ) ;
#78780=CARTESIAN_POINT ( 'NONE',  ( 1.220472440944881942, 2.401574803149606474, -0.5309055118110238558 ) ) ;
#78781=CARTESIAN_POINT ( 'NONE',  ( 1.404199475065617708, 0.05413385826771626580, -0.4176697321401330321 ) ) ;
#78782=CARTESIAN_POINT ( 'NONE',  ( 1.620734908136483465, -0.5511811023622046335, 0.09757992244046803654 ) ) ;
#78785=CARTESIAN_POINT ( 'NONE',  ( -0.03280839895013062252, 0.2952755905511810774, -0.1292274648535930714 ) ) ;
#78787=AXIS2_PLACEMENT_3D ( 'NONE', #55675, #43045, #42228 ) ;
#78788=CARTESIAN_POINT ( 'NONE',  ( -1.062992125984250968, 0.2952755905511811885, 0.000000000000000000 ) ) ;
#78789=CARTESIAN_POINT ( 'NONE',  ( 1.135170603674541256, 0.2952755905511811885, 0.1292274648535926551 ) ) ;
#78790=CARTESIAN_POINT ( 'NONE',  ( 1.246719160104987623, -0.4281496062992124485, 0.4176697321401328655 ) ) ;
#78791=CARTESIAN_POINT ( 'NONE',  ( 0.2887139107611556010, -0.6046776061558807314, 0.2411417322834647770 ) ) ;
#78792=ADVANCED_FACE ( 'NONE', ( #56868 ), #5537, .F. ) ;
#78793=CARTESIAN_POINT ( 'NONE',  ( -0.3215223097112853146, -0.05778040916215560624, -0.4822834645669293319 ) ) ;
#78795=CARTESIAN_POINT ( 'NONE',  ( -1.161417322834644716, -0.5400638737290845981, -0.3530559997133363437 ) ) ;
#78796=CARTESIAN_POINT ( 'NONE',  ( -0.7086614173228339419, -0.1870078740157479769, 0.4822834645669291653 ) ) ;
#78797=CARTESIAN_POINT ( 'NONE',  ( -0.6430446194225712953, -0.004921259842519870586, -0.3153832671262229437 ) ) ;
#78799=CARTESIAN_POINT ( 'NONE',  ( -0.6824146981627291497, -0.6046776061558809534, -0.2411417322834644161 ) ) ;
#78801=CARTESIAN_POINT ( 'NONE',  ( 0.5708661417322841158, -0.5400638737290845981, -0.3530559997133363437 ) ) ;
#78804=CARTESIAN_POINT ( 'NONE',  ( -0.2952755905511803003, -0.5400638737290845981, -0.3530559997133363437 ) ) ;
#78805=CARTESIAN_POINT ( 'NONE',  ( 1.049868766404200349, 0.1283753931104748280, 0.1820866141732283561 ) ) ;
#78806=CARTESIAN_POINT ( 'NONE',  ( -0.8789144566217194088, 0.004960608223777852183, -0.3437734562760195733 ) ) ;
#78808=CARTESIAN_POINT ( 'NONE',  ( 1.161417322834646493, -0.4536011799217367080, 0.2665933059059888421 ) ) ;
#78809=CARTESIAN_POINT ( 'NONE',  ( 1.095800524934383846, -0.3162353388693405765, 0.4822834645669290543 ) ) ;
#78811=CARTESIAN_POINT ( 'NONE',  ( 0.09842519685039434474, -0.5400638737290845981, -0.3530559997133363437 ) ) ;
#78812=CARTESIAN_POINT ( 'NONE',  ( -1.574803149606298192, -0.1870078740157480879, -0.4822834645669291653 ) ) ;
#78813=CARTESIAN_POINT ( 'NONE',  ( -1.515748031496062076, 0.1660481256975883668, -0.3530559997133364547 ) ) ;
#78814=CARTESIAN_POINT ( 'NONE',  ( -0.2887139107611542133, 0.2306618581243848609, 0.2411417322834645549 ) ) ;
#78816=CARTESIAN_POINT ( 'NONE',  ( 1.266404199475066328, -0.3162353388693409650, -0.4822834645669289433 ) ) ;
#78817=CARTESIAN_POINT ( 'NONE',  ( 0.5052493438320215802, 0.2952755905511811885, 0.1292274648535926551 ) ) ;
#78818=CARTESIAN_POINT ( 'NONE',  ( 0.8070866141732289112, -0.4536011799217368745, -0.2665933059059886201 ) ) ;
#78820=CARTESIAN_POINT ( 'NONE',  ( 0.3740157480314966754, -0.4536011799217367080, 0.2665933059059888421 ) ) ;
#78823=CARTESIAN_POINT ( 'NONE',  ( 0.8923884514435703741, 0.2306618581243848609, 0.2411417322834645549 ) ) ;
#78827=CARTESIAN_POINT ( 'NONE',  ( 0.2230971128608932319, -0.4281496062992124485, 0.4176697321401328655 ) ) ;
#78830=CARTESIAN_POINT ( 'NONE',  ( 0.4527559055118117182, -0.4536011799217367080, 0.2665933059059888421 ) ) ;
#78831=CARTESIAN_POINT ( 'NONE',  ( 0.3674540682414705883, -0.6046776061558807314, 0.2411417322834647770 ) ) ;
#78833=CARTESIAN_POINT ( 'NONE',  ( -1.108923884514435132, -0.2845877964562159024, 0.3641732283464567677 ) ) ;
#78834=CARTESIAN_POINT ( 'NONE',  ( -0.9973753280839886548, -0.6046776061558809534, -0.2411417322834644161 ) ) ;
#78835=CARTESIAN_POINT ( 'NONE',  ( -1.377952755905511140, 0.2952755905511811885, 0.000000000000000000 ) ) ;
#78836=CARTESIAN_POINT ( 'NONE',  ( 0.3477690288713918276, -0.6692913385826773087, -0.1292274648535924053 ) ) ;
#78837=CARTESIAN_POINT ( 'NONE',  ( -1.581364829396324945, -0.08942795157528024563, -0.3641732283464568787 ) ) ;
#78839=CARTESIAN_POINT ( 'NONE',  ( 0.7217847769028878924, -0.4281496062992127816, -0.4176697321401328100 ) ) ;
#78842=CARTESIAN_POINT ( 'NONE',  ( 1.437007874015748810, -0.5400638737290845981, -0.3530559997133363437 ) ) ;
#78843=CARTESIAN_POINT ( 'NONE',  ( -1.246719160104986512, -0.004921259842519576551, 0.3153832671262227771 ) ) ;
#78844=CARTESIAN_POINT ( 'NONE',  ( 1.187664041994751285, -0.08942795157527998196, 0.3641732283464567121 ) ) ;
#78845=CARTESIAN_POINT ( 'NONE',  ( -1.135170603674539924, 0.1771653543307087075, -0.09757992244046823083 ) ) ;
#78846=CARTESIAN_POINT ( 'NONE',  ( -0.7677165354330699465, -0.4536011799217368745, -0.2665933059059886201 ) ) ;
#78847=CARTESIAN_POINT ( 'NONE',  ( 1.555118110236221041, -0.5400638737290844871, 0.3530559997133364547 ) ) ;
#78848=CARTESIAN_POINT ( 'NONE',  ( 0.6430446194225728496, -0.004921259842519576551, 0.3153832671262227771 ) ) ;
#78849=CARTESIAN_POINT ( 'NONE',  ( 0.4790026246719168435, -0.3162353388693409650, -0.4822834645669289433 ) ) ;
#78850=CARTESIAN_POINT ( 'NONE',  ( 1.141732283464567566, 0.2952755905511811885, 0.000000000000000000 ) ) ;
#78851=CARTESIAN_POINT ( 'NONE',  ( -0.1377952755905504645, -0.5400638737290845981, -0.3530559997133363437 ) ) ;
#78853=CARTESIAN_POINT ( 'NONE',  ( 0.1312335958005255154, -0.5023911411419708095, 0.1820866141732285504 ) ) ;
#78854=CARTESIAN_POINT ( 'NONE',  ( 1.259842519685040019, -0.1870078740157479769, 0.4822834645669291653 ) ) ;
#78855=( BOUNDED_CURVE ( )  B_SPLINE_CURVE ( 1, ( #41533, #23409 ),
 .UNSPECIFIED., .F., .F. ) 
 B_SPLINE_CURVE_WITH_KNOTS ( ( 2, 2 ),
 ( 0.000000000000000000, 0.002000000000000005246 ),
 .UNSPECIFIED. ) 
 CURVE ( )  GEOMETRIC_REPRESENTATION_ITEM ( )  RATIONAL_B_SPLINE_CURVE ( ( 0.9875488213027523443, 0.9875488213027523443 ) ) 
 REPRESENTATION_ITEM ( '' )  );
#78856=CARTESIAN_POINT ( 'NONE',  ( -0.2034120734908128059, 0.2066929133858267931, 0.1054918080437490802 ) ) ;
#78857=CARTESIAN_POINT ( 'NONE',  ( -0.7349081364829390672, 0.2306618581243847221, -0.2411417322834647770 ) ) ;
#78859=FACE_OUTER_BOUND ( 'NONE', #70785, .T. ) ;
#78860=CARTESIAN_POINT ( 'NONE',  ( -1.003937007874014853, 0.1660481256975885056, 0.3530559997133364547 ) ) ;
#78861=CARTESIAN_POINT ( 'NONE',  ( -0.05249343832020938322, -0.6046776061558809534, -0.2411417322834644161 ) ) ;
#78866=CARTESIAN_POINT ( 'NONE',  ( -1.325459317585300889, -0.3690944881889765550, -0.3153832671262227771 ) ) ;
#78868=CARTESIAN_POINT ( 'NONE',  ( -1.601049868766403650, -0.6046776061558807314, 0.2411417322834647770 ) ) ;
#78871=CARTESIAN_POINT ( 'NONE',  ( 0.4199475065616805614, 0.2306618581243848609, 0.2411417322834645549 ) ) ;
#78872=CARTESIAN_POINT ( 'NONE',  ( -0.4855643044619415427, -0.3690944881889763329, 0.3153832671262228327 ) ) ;
#78874=CARTESIAN_POINT ( 'NONE',  ( 0.6824146981627303710, 0.2306618581243847221, -0.2411417322834647770 ) ) ;
#78875=CARTESIAN_POINT ( 'NONE',  ( 0.1771653543307093182, 0.1660481256975885056, 0.3530559997133364547 ) ) ;
#78880=CARTESIAN_POINT ( 'NONE',  ( 1.082677165354331228, 0.1660481256975883668, -0.3530559997133364547 ) ) ;
#78883=CARTESIAN_POINT ( 'NONE',  ( 0.2362204724409456558, -0.1870078740157480879, -0.4822834645669291653 ) ) ;
#78884=CARTESIAN_POINT ( 'NONE',  ( 1.535433070866142335, -0.6692913385826771977, 8.415575281601705876E-17 ) ) ;
#78885=CARTESIAN_POINT ( 'NONE',  ( 1.095800524934383846, -0.05778040916215560624, -0.4822834645669293319 ) ) ;
#78887=CARTESIAN_POINT ( 'NONE',  ( 0.1115485564304467270, -0.6692913385826773087, -0.1292274648535924053 ) ) ;
#78888=CARTESIAN_POINT ( 'NONE',  ( 0.8267716535433078384, -0.6692913385826771977, 8.415575281601705876E-17 ) ) ;
#78889=CARTESIAN_POINT ( 'NONE',  ( 0.02624671916010564918, -0.6046776061558809534, -0.2411417322834644161 ) ) ;
#78890=CARTESIAN_POINT ( 'NONE',  ( 0.5708661417322842269, 0.07958543189024085140, 0.2665933059059887866 ) ) ;
#78891=CARTESIAN_POINT ( 'NONE',  ( -1.351706036745406347, 0.05413385826771626580, -0.4176697321401330321 ) ) ;
#78892=CARTESIAN_POINT ( 'NONE',  ( -1.574803149606298636, -0.1870078740157479769, 0.4822834645669291653 ) ) ;
#78893=CARTESIAN_POINT ( 'NONE',  ( 0.8267716535433077274, 0.2952755905511811885, 0.000000000000000000 ) ) ;
#78899=CARTESIAN_POINT ( 'NONE',  ( 1.194225721784777594, 0.05413385826771666132, 0.4176697321401328100 ) ) ;
#78900=CARTESIAN_POINT ( 'NONE',  ( 1.095800524934383846, -0.2845877964562159024, 0.3641732283464567677 ) ) ;
#78905=CARTESIAN_POINT ( 'NONE',  ( 1.437007874015748810, 0.1660481256975885056, 0.3530559997133364547 ) ) ;
#78906=CARTESIAN_POINT ( 'NONE',  ( -1.555118110236219930, -0.5400638737290845981, -0.3530559997133363437 ) ) ;
#78907=CARTESIAN_POINT ( 'NONE',  ( -0.3740157480314953431, -0.5400638737290845981, -0.3530559997133363437 ) ) ;
#78908=CARTESIAN_POINT ( 'NONE',  ( 0.9448818897637802916, -0.1870078740157479769, 0.4822834645669291653 ) ) ;
#78909=VERTEX_POINT ( 'NONE', #70334 ) ;
#78910=CARTESIAN_POINT ( 'NONE',  ( -1.633858267716534529, -0.5400638737290845981, -0.3530559997133363437 ) ) ;
#78913=CARTESIAN_POINT ( 'NONE',  ( 1.660104986876641320, -0.08942795157527998196, 0.3641732283464567121 ) ) ;
#78915=CARTESIAN_POINT ( 'NONE',  ( -0.8923884514435688198, -0.5023911411419708095, 0.1820866141732285504 ) ) ;
#78916=CARTESIAN_POINT ( 'NONE',  ( -1.391076115485563314, -0.6046776061558809534, -0.2411417322834644161 ) ) ;
#78917=CARTESIAN_POINT ( 'NONE',  ( 0.8070866141732289112, -0.5400638737290845981, -0.3530559997133363437 ) ) ;
#78919=CARTESIAN_POINT ( 'NONE',  ( 1.450131233595801428, -0.6692913385826773087, -0.1292274648535924053 ) ) ;
#78921=CARTESIAN_POINT ( 'NONE',  ( -0.7217847769028863381, -0.004921259842519870586, -0.3153832671262229437 ) ) ;
#78922=CARTESIAN_POINT ( 'NONE',  ( 0.7545931758530189937, 0.2952755905511810774, -0.1292274648535930714 ) ) ;
#78923=CARTESIAN_POINT ( 'NONE',  ( -1.607611548556429737, -0.6692913385826771977, 0.1292274648535927661 ) ) ;
#78925=CARTESIAN_POINT ( 'NONE',  ( -0.8595800524934373854, -0.2845877964562161244, -0.3641732283464567121 ) ) ;
#78926=CARTESIAN_POINT ( 'NONE',  ( -1.646981627296586703, -0.08942795157527998196, 0.3641732283464567121 ) ) ;
#78927=DIRECTION ( 'NONE',  ( -1.000000000000000000, -3.096699300667737464E-16, 1.692413147294446216E-16 ) ) ;
#78928=CARTESIAN_POINT ( 'NONE',  ( 0.6167979002624678353, -0.4281496062992124485, 0.4176697321401328655 ) ) ;
#78929=CARTESIAN_POINT ( 'NONE',  ( -0.8267716535433065062, 0.1771653543307087630, 0.000000000000000000 ) ) ;
#78930=CARTESIAN_POINT ( 'NONE',  ( -0.3937007874015740483, -0.1870078740157480601, -0.3641732283464567677 ) ) ;
#78931=CARTESIAN_POINT ( 'NONE',  ( -0.2690288713910754526, 0.2952755905511810774, -0.1292274648535930714 ) ) ;
#78932=CARTESIAN_POINT ( 'NONE',  ( 1.627296587926509996, -0.6046776061558807314, 0.2411417322834647770 ) ) ;
#78934=CARTESIAN_POINT ( 'NONE',  ( 0.7086614173228352742, -0.1870078740157480879, -0.4822834645669291653 ) ) ;
#78936=EDGE_CURVE ( 'NONE', #79833, #66112, #74595, .T. ) ;
#78937=( BOUNDED_CURVE ( )  B_SPLINE_CURVE ( 2, ( #59786, #6773, #902, #65291, #33301, #1319, #58536, #26559, #53468, #21493, #26968, #13518, #72843 ),
 .UNSPECIFIED., .F., .F. ) 
 B_SPLINE_CURVE_WITH_KNOTS ( ( 3, 2, 2, 2, 2, 2, 3 ),
 ( 0.1733310946348008696, 0.1742424242424242542, 0.1780303030303030387, 0.1818181818181818232, 0.1856060606060606077, 0.1893939393939393923, 0.1903052690015628601 ),
 .UNSPECIFIED. ) 
 CURVE ( )  GEOMETRIC_REPRESENTATION_ITEM ( )  RATIONAL_B_SPLINE_CURVE ( ( 0.9875488213027527884, 0.9918020599134683701, 1.000000000000000000, 0.9659258262890683122, 1.000000000000000000, 0.9659258262890683122, 1.000000000000000000, 0.9659258262890683122, 1.000000000000000000, 0.9659258262890683122, 1.000000000000000000, 0.9918020599134675930, 0.9875488213027519002 ) ) 
 REPRESENTATION_ITEM ( '' )  );
#78943=CARTESIAN_POINT ( 'NONE',  ( -0.9776902887139098386, -0.6692913385826771977, 0.1292274648535927661 ) ) ;
#78944=CARTESIAN_POINT ( 'NONE',  ( -0.2362204724409442680, -0.1870078740157480601, -0.3641732283464567677 ) ) ;
#78945=CARTESIAN_POINT ( 'NONE',  ( -1.430446194225720724, 0.05413385826771626580, -0.4176697321401330321 ) ) ;
#78946=CARTESIAN_POINT ( 'NONE',  ( 0.2952755905511819101, 0.07958543189024071263, -0.2665933059059888421 ) ) ;
#78947=CARTESIAN_POINT ( 'NONE',  ( -0.7677165354330699465, 0.07958543189024085140, 0.2665933059059887866 ) ) ;
#78948=CARTESIAN_POINT ( 'NONE',  ( -1.167979002624671470, -0.4281496062992127816, -0.4176697321401328100 ) ) ;
#78949=CARTESIAN_POINT ( 'NONE',  ( -1.587926509186350810, -0.4281496062992124485, 0.4176697321401328655 ) ) ;
#78950=CARTESIAN_POINT ( 'NONE',  ( -1.443569553805773564, 0.2306618581243847221, -0.2411417322834647770 ) ) ;
#78951=CARTESIAN_POINT ( 'NONE',  ( 1.056430446194226436, 0.2066929133858267931, 0.1054918080437490802 ) ) ;
#78952=CARTESIAN_POINT ( 'NONE',  ( 0.7480314960629927956, 0.1771653543307087630, 0.000000000000000000 ) ) ;
#78953=CARTESIAN_POINT ( 'NONE',  ( 0.3018372703412079971, 0.05413385826771626580, -0.4176697321401330321 ) ) ;
#78954=CARTESIAN_POINT ( 'NONE',  ( -1.430446194225720724, 0.05413385826771626580, -0.4176697321401330321 ) ) ;
#78955=CARTESIAN_POINT ( 'NONE',  ( 1.227034120734908917, -0.5511811023622046335, 0.09757992244046803654 ) ) ;
#78958=CARTESIAN_POINT ( 'NONE',  ( -1.115485564304461219, -0.004921259842519870586, -0.3153832671262229437 ) ) ;
#78959=CARTESIAN_POINT ( 'NONE',  ( -0.2821522309711278487, -0.6692913385826773087, -0.1292274648535924053 ) ) ;
#78960=CARTESIAN_POINT ( 'NONE',  ( 0.1968503937007881344, 0.2952755905511811885, 0.000000000000000000 ) ) ;
#78961=CARTESIAN_POINT ( 'NONE',  ( -1.509186351706035767, -0.004921259842519870586, -0.3153832671262229437 ) ) ;
#78963=CARTESIAN_POINT ( 'NONE',  ( -1.207349081364828880, 0.2306618581243847221, -0.2411417322834647770 ) ) ;
#78964=CARTESIAN_POINT ( 'NONE',  ( 0.3543307086614181922, -0.6692913385826771977, 8.415575281601705876E-17 ) ) ;
#78965=CARTESIAN_POINT ( 'NONE',  ( 0.1640419947506569498, -0.3162353388693409650, -0.4822834645669289433 ) ) ;
#78966=CARTESIAN_POINT ( 'NONE',  ( 1.220472440944882386, -0.6692913385826771977, 8.415575281601705876E-17 ) ) ;
#78971=CARTESIAN_POINT ( 'NONE',  ( 0.3412073490813655186, 0.1283753931104748280, 0.1820866141732283561 ) ) ;
#78972=CARTESIAN_POINT ( 'NONE',  ( -0.3346456692913377662, -0.5400638737290844871, 0.3530559997133364547 ) ) ;
#78973=CARTESIAN_POINT ( 'NONE',  ( 1.194225721784777594, -0.4281496062992127816, -0.4176697321401328100 ) ) ;
#78975=CARTESIAN_POINT ( 'NONE',  ( -0.2034120734908128059, 0.1771653543307087630, 0.09757992244046791164 ) ) ;
#78976=CARTESIAN_POINT ( 'NONE',  ( -1.167979002624671470, 0.05413385826771666132, 0.4176697321401328100 ) ) ;
#78977=CARTESIAN_POINT ( 'NONE',  ( -1.581364829396324945, -0.05778040916215560624, -0.4822834645669293319 ) ) ;
#78982=CARTESIAN_POINT ( 'NONE',  ( 1.430446194225722500, 0.05413385826771666132, 0.4176697321401328100 ) ) ;
#78983=CARTESIAN_POINT ( 'NONE',  ( 1.607611548556431069, 0.1771653543307087630, 0.09757992244046791164 ) ) ;
#78985=CARTESIAN_POINT ( 'NONE',  ( -1.318897637795274802, 0.07958543189024085140, 0.2665933059059887866 ) ) ;
#78986=CARTESIAN_POINT ( 'NONE',  ( -1.345144356955379816, -0.3162353388693405765, 0.4822834645669290543 ) ) ;
#78989=CARTESIAN_POINT ( 'NONE',  ( 1.246719160104987623, 0.05413385826771626580, -0.4176697321401330321 ) ) ;
#78990=CARTESIAN_POINT ( 'NONE',  ( -1.141732283464566011, -0.6692913385826771977, 8.415575281601705876E-17 ) ) ;
#78991=CARTESIAN_POINT ( 'NONE',  ( 0.08530183727034192087, -0.3162353388693409650, -0.4822834645669289433 ) ) ;
#78992=CARTESIAN_POINT ( 'NONE',  ( -0.2165354330708654795, -0.5400638737290845981, -0.3530559997133363437 ) ) ;
#78993=CARTESIAN_POINT ( 'NONE',  ( -1.299212598425196097, 0.2952755905511811885, 0.000000000000000000 ) ) ;
#78995=CARTESIAN_POINT ( 'NONE',  ( 0.5839895013123367340, -0.6692913385826773087, -0.1292274648535924053 ) ) ;
#78997=CARTESIAN_POINT ( 'NONE',  ( -1.266404199475064773, -0.08942795157528024563, -0.3641732283464568787 ) ) ;
#79003=CARTESIAN_POINT ( 'NONE',  ( -0.9711286089238838626, -0.6046776061558807314, 0.2411417322834647770 ) ) ;
#79004=CARTESIAN_POINT ( 'NONE',  ( -1.430446194225720724, 0.05413385826771626580, -0.4176697321401330321 ) ) ;
#79006=CARTESIAN_POINT ( 'NONE',  ( -1.548556430446193399, 0.2306618581243848609, 0.2411417322834645549 ) ) ;
#79007=CARTESIAN_POINT ( 'NONE',  ( -1.614173228346456268, -0.6692913385826771977, 8.415575281601705876E-17 ) ) ;
#79008=CARTESIAN_POINT ( 'NONE',  ( -1.345144356955379816, -0.3162353388693405765, 0.4822834645669290543 ) ) ;
#79011=CARTESIAN_POINT ( 'NONE',  ( 0.1377952755905518800, 0.07958543189024071263, -0.2665933059059888421 ) ) ;
#79013=CARTESIAN_POINT ( 'NONE',  ( -0.9448818897637790704, -0.1870078740157479769, 0.3641732283464567677 ) ) ;
#79014=CARTESIAN_POINT ( 'NONE',  ( -1.128608923884513837, 0.2306618581243847221, -0.2411417322834647770 ) ) ;
#79015=EDGE_CURVE ( 'NONE', #41807, #21784, #8586, .T. ) ;
#79016=CARTESIAN_POINT ( 'NONE',  ( 0.8464566929133865436, 0.1660481256975883668, -0.3530559997133364547 ) ) ;
#79017=CARTESIAN_POINT ( 'NONE',  ( -0.9908136482939626788, 0.2952755905511811885, 0.1292274648535926551 ) ) ;
#79019=EDGE_LOOP ( 'NONE', ( #57182, #55146, #57717, #64885, #78057 ) ) ;
#79020=CARTESIAN_POINT ( 'NONE',  ( -1.515748031496062076, -0.5400638737290844871, 0.3530559997133364547 ) ) ;
#79021=CARTESIAN_POINT ( 'NONE',  ( 1.056430446194226436, -0.6692913385826773087, -0.1292274648535924053 ) ) ;
#79022=CARTESIAN_POINT ( 'NONE',  ( -1.541994750656167090, 0.1771653543307087630, 0.09757992244046791164 ) ) ;
#79028=CARTESIAN_POINT ( 'NONE',  ( -0.1574803149606292529, -0.1870078740157480879, -0.4822834645669291653 ) ) ;
#79029=CARTESIAN_POINT ( 'NONE',  ( -1.351706036745406347, -0.3690944881889763329, 0.3153832671262228327 ) ) ;
#79031=CARTESIAN_POINT ( 'NONE',  ( -1.673228346456691717, 0.1660481256975883668, -0.3530559997133364547 ) ) ;
#79033=CARTESIAN_POINT ( 'NONE',  ( -1.292650918635170010, -0.6692913385826771977, 0.1292274648535927661 ) ) ;
#79034=CARTESIAN_POINT ( 'NONE',  ( -0.3608923884514428360, -0.6692913385826773087, -0.1292274648535924053 ) ) ;
#79036=CARTESIAN_POINT ( 'NONE',  ( 0.6102362204724416372, -0.4536011799217367080, 0.2665933059059888421 ) ) ;
#79038=CARTESIAN_POINT ( 'NONE',  ( 0.1443569553805781891, -0.004921259842519870586, -0.3153832671262229437 ) ) ;
#79039=CARTESIAN_POINT ( 'NONE',  ( 0.9973753280839902091, 0.1283753931104746893, -0.1820866141732285504 ) ) ;
#79040=CARTESIAN_POINT ( 'NONE',  ( 1.056430446194226436, -0.6692913385826773087, -0.1292274648535924053 ) ) ;
#79041=CARTESIAN_POINT ( 'NONE',  ( 0.1968503937007881344, -0.5511811023622047445, 6.969142054262312111E-17 ) ) ;
#79043=CARTESIAN_POINT ( 'NONE',  ( -1.069553805774277722, -0.6692913385826773087, -0.1292274648535924053 ) ) ;
#79044=CARTESIAN_POINT ( 'NONE',  ( -0.2821522309711278487, 0.1771653543307087630, 0.09757992244046791164 ) ) ;
#79046=CARTESIAN_POINT ( 'NONE',  ( -1.246719160104985846, -0.3690944881889765550, -0.3153832671262227771 ) ) ;
#79048=CARTESIAN_POINT ( 'NONE',  ( -0.9711286089238838626, 0.1283753931104746893, -0.1820866141732285504 ) ) ;
#79049=CARTESIAN_POINT ( 'NONE',  ( 1.614173228346456712, 2.401574803149606474, -0.5309055118110239668 ) ) ;
#79050=CARTESIAN_POINT ( 'NONE',  ( -0.05905511811023545637, 0.1660481256975885056, 0.3530559997133364547 ) ) ;
#79053=CARTESIAN_POINT ( 'NONE',  ( 0.5577427821522314977, -0.2845877964562161244, -0.3641732283464567121 ) ) ;
#79054=CARTESIAN_POINT ( 'NONE',  ( -0.3215223097112853146, -0.2845877964562159024, 0.3641732283464567677 ) ) ;
#79055=CARTESIAN_POINT ( 'NONE',  ( -0.4330708661417315697, -0.6692913385826771977, 8.415575281601705876E-17 ) ) ;
#79056=CARTESIAN_POINT ( 'NONE',  ( -1.607611548556429737, -0.6692913385826771977, 0.1292274648535927661 ) ) ;
#79057=CARTESIAN_POINT ( 'NONE',  ( -1.102362204724408601, -0.1870078740157480601, -0.3641732283464567677 ) ) ;
#79059=CARTESIAN_POINT ( 'NONE',  ( 0.4461942257217856311, 0.2306618581243847221, -0.2411417322834647770 ) ) ;
#79062=CARTESIAN_POINT ( 'NONE',  ( 1.555118110236221041, -0.5400638737290844871, 0.3530559997133364547 ) ) ;
#79063=CARTESIAN_POINT ( 'NONE',  ( -0.09186351706036689768, -0.004921259842519870586, -0.3153832671262229437 ) ) ;
#79065=CARTESIAN_POINT ( 'NONE',  ( -1.450131233595799651, 0.2952755905511810774, -0.1292274648535930714 ) ) ;
#79066=CARTESIAN_POINT ( 'NONE',  ( 1.581364829396326277, -0.3162353388693409650, -0.4822834645669289433 ) ) ;
#79068=CARTESIAN_POINT ( 'NONE',  ( -0.6496062992125976043, -0.4536011799217367080, 0.2665933059059888421 ) ) ;
#79069=CARTESIAN_POINT ( 'NONE',  ( -0.7677165354330700575, 0.1012011053420777407, 0.2882089793578257453 ) ) ;
#79070=CARTESIAN_POINT ( 'NONE',  ( 0.8267716535433077274, 0.2952755905511811885, 0.000000000000000000 ) ) ;
#79074=CARTESIAN_POINT ( 'NONE',  ( -1.673228346456691717, 0.1660481256975883668, -0.3530559997133364547 ) ) ;
#79075=CARTESIAN_POINT ( 'NONE',  ( -1.128608923884513837, -0.6046776061558807314, 0.2411417322834647770 ) ) ;
#79076=CARTESIAN_POINT ( 'NONE',  ( 1.430446194225722500, 0.05413385826771666132, 0.4176697321401328100 ) ) ;
#79078=CARTESIAN_POINT ( 'NONE',  ( 1.174540682414699111, -0.2845877964562159024, 0.3641732283464567677 ) ) ;
#79079=CARTESIAN_POINT ( 'NONE',  ( 0.3149606299212606708, -0.1870078740157480879, -0.4822834645669291653 ) ) ;
#79080=CARTESIAN_POINT ( 'NONE',  ( -0.3346456692913377662, 0.1660481256975883668, -0.3530559997133364547 ) ) ;
#79081=CARTESIAN_POINT ( 'NONE',  ( 1.686351706036745890, 0.2952755905511811885, 0.1292274648535926551 ) ) ;
#79083=CARTESIAN_POINT ( 'NONE',  ( 0.9120734908136489683, -0.5511811023622046335, 0.09757992244046803654 ) ) ;
#79087=CARTESIAN_POINT ( 'NONE',  ( -0.3477690288713905509, -0.6692913385826771977, 0.1292274648535927661 ) ) ;
#79088=CARTESIAN_POINT ( 'NONE',  ( 1.266404199475066328, -0.05778040916215522460, 0.4822834645669289988 ) ) ;
#79089=CARTESIAN_POINT ( 'NONE',  ( 0.3412073490813655186, -0.6046776061558809534, -0.2411417322834644161 ) ) ;
#79090=CARTESIAN_POINT ( 'NONE',  ( -0.1902887139107604098, 0.1771653543307087075, -0.09757992244046823083 ) ) ;
#79091=CARTESIAN_POINT ( 'NONE',  ( 1.167979002624672580, -0.4281496062992124485, 0.4176697321401328655 ) ) ;
#79092=CARTESIAN_POINT ( 'NONE',  ( -0.9448818897637790704, -0.1870078740157480879, -0.4822834645669291653 ) ) ;
#79093=CARTESIAN_POINT ( 'NONE',  ( 0.1640419947506569498, -0.05778040916215522460, 0.4822834645669289988 ) ) ;
#79094=CARTESIAN_POINT ( 'NONE',  ( -0.8202099737532801971, -0.6692913385826771977, 0.1292274648535927661 ) ) ;
#79095=CARTESIAN_POINT ( 'NONE',  ( 1.266404199475066328, -0.05778040916215522460, 0.4822834645669289988 ) ) ;
#79096=CARTESIAN_POINT ( 'NONE',  ( 0.8530183727034126306, 0.05413385826771626580, -0.4176697321401330321 ) ) ;
#79097=CARTESIAN_POINT ( 'NONE',  ( 1.312335958005250269, -0.6046776061558807314, 0.2411417322834647770 ) ) ;
#79099=CARTESIAN_POINT ( 'NONE',  ( -0.08530183727034056085, -0.2845877964562159024, 0.3641732283464567677 ) ) ;
#79103=CARTESIAN_POINT ( 'NONE',  ( -0.7086614173228339419, -0.1870078740157480601, -0.3641732283464567677 ) ) ;
#79104=CARTESIAN_POINT ( 'NONE',  ( -0.1246719160104980823, -0.6692913385826773087, -0.1292274648535924053 ) ) ;
#79106=CARTESIAN_POINT ( 'NONE',  ( -0.1902887139107604098, -0.6692913385826771977, 0.1292274648535927661 ) ) ;
#79107=CARTESIAN_POINT ( 'NONE',  ( -0.2493438320209966919, 0.05413385826771626580, -0.4176697321401330321 ) ) ;
#79108=CARTESIAN_POINT ( 'NONE',  ( -0.7217847769028863381, -0.4281496062992124485, 0.4176697321401328655 ) ) ;
#79110=CARTESIAN_POINT ( 'NONE',  ( -1.555118110236219930, 0.1660481256975885056, 0.3530559997133364547 ) ) ;
#79111=CARTESIAN_POINT ( 'NONE',  ( 1.377952755905512472, 0.1771653543307087630, 0.000000000000000000 ) ) ;
#79112=CARTESIAN_POINT ( 'NONE',  ( -1.541994750656167090, -0.6692913385826773087, -0.1292274648535924053 ) ) ;
#79114=CARTESIAN_POINT ( 'NONE',  ( 0.6561679790026253567, 0.1283753931104748280, 0.1820866141732283561 ) ) ;
#79115=CARTESIAN_POINT ( 'NONE',  ( 0.01312335958005323398, -0.4281496062992127816, -0.4176697321401328100 ) ) ;
#79116=CARTESIAN_POINT ( 'NONE',  ( 0.1968503937007881344, -0.6692913385826771977, 8.415575281601705876E-17 ) ) ;
#79119=CARTESIAN_POINT ( 'NONE',  ( -1.614173228346456268, -0.6692913385826771977, 8.415575281601705876E-17 ) ) ;
#79122=CARTESIAN_POINT ( 'NONE',  ( -0.6955380577427815458, -0.4281496062992127816, -0.4176697321401328100 ) ) ;
#79125=CARTESIAN_POINT ( 'NONE',  ( -1.587926509186350810, -0.004921259842519870586, -0.3153832671262229437 ) ) ;
#79126=CARTESIAN_POINT ( 'NONE',  ( 0.7217847769028878924, -0.4281496062992127816, -0.4176697321401328100 ) ) ;
#79127=CARTESIAN_POINT ( 'NONE',  ( 0.8398950131233602345, -0.6046776061558807314, 0.2411417322834647770 ) ) ;
#79128=CARTESIAN_POINT ( 'NONE',  ( -0.3543307086614165824, 0.1771653543307087630, 0.000000000000000000 ) ) ;
#79129=CARTESIAN_POINT ( 'NONE',  ( -0.02624671916010428221, -0.6046776061558807314, 0.2411417322834647770 ) ) ;
#79131=CARTESIAN_POINT ( 'NONE',  ( 0.01968503937007957949, -0.4536011799217368745, -0.2665933059059886201 ) ) ;
#79132=CARTESIAN_POINT ( 'NONE',  ( 0.08530183727034192087, -0.3162353388693409650, -0.4822834645669289433 ) ) ;
#79134=CARTESIAN_POINT ( 'NONE',  ( 1.587926509186352142, -0.004921259842519576551, 0.3153832671262227771 ) ) ;
#79135=CARTESIAN_POINT ( 'NONE',  ( 0.2821522309711292364, -0.5511811023622046335, 0.09757992244046803654 ) ) ;
#79136=CARTESIAN_POINT ( 'NONE',  ( 1.686351706036745890, 0.1771653543307087630, 0.09757992244046791164 ) ) ;
#79137=CARTESIAN_POINT ( 'NONE',  ( -0.9317585301837263412, 0.05413385826771666132, 0.4176697321401328100 ) ) ;
#79138=CARTESIAN_POINT ( 'NONE',  ( -0.8005249343832011588, -0.004921259842519870586, -0.3153832671262229437 ) ) ;
#79140=CARTESIAN_POINT ( 'NONE',  ( -0.9120734908136475250, 0.2952755905511811885, 0.1292274648535926551 ) ) ;
#79141=CARTESIAN_POINT ( 'NONE',  ( -0.4921259842519677963, 0.1660481256975883668, -0.3530559997133364547 ) ) ;
#79142=CARTESIAN_POINT ( 'NONE',  ( -0.06561679790026180015, 0.05413385826771666132, 0.4176697321401328100 ) ) ;
#79146=CARTESIAN_POINT ( 'NONE',  ( 0.7874015748031503170, -0.1870078740157480601, -0.3641732283464567677 ) ) ;
#79147=CARTESIAN_POINT ( 'NONE',  ( 1.541994750656168645, -0.6692913385826771977, 0.1292274648535927661 ) ) ;
#79148=CARTESIAN_POINT ( 'NONE',  ( -1.430446194225721390, -0.3690944881889763329, 0.3153832671262228327 ) ) ;
#79149=CARTESIAN_POINT ( 'NONE',  ( 0.9776902887139113929, -0.6692913385826773087, -0.1292274648535924053 ) ) ;
#79150=CARTESIAN_POINT ( 'NONE',  ( -1.095800524934382292, -0.08942795157527998196, 0.3641732283464567121 ) ) ;
#79152=CARTESIAN_POINT ( 'NONE',  ( -0.3674540682414692561, -0.6046776061558809534, -0.2411417322834644161 ) ) ;
#79153=CARTESIAN_POINT ( 'NONE',  ( 0.3149606299212606708, -0.1870078740157480601, -0.3641732283464567677 ) ) ;
#79154=CARTESIAN_POINT ( 'NONE',  ( 0.7283464566929140904, -0.4536011799217368745, -0.2665933059059886201 ) ) ;
#79155=CARTESIAN_POINT ( 'NONE',  ( 0.1902887139107617975, -0.6692913385826773087, -0.1292274648535924053 ) ) ;
#79157=CARTESIAN_POINT ( 'NONE',  ( -0.6299212598425188991, -0.1870078740157479769, 0.4822834645669291653 ) ) ;
#79159=CARTESIAN_POINT ( 'NONE',  ( 1.023622047244095112, -0.1870078740157480601, -0.3641732283464567677 ) ) ;
#79160=CARTESIAN_POINT ( 'NONE',  ( 0.5905511811023629321, 0.2952755905511811885, 0.000000000000000000 ) ) ;
#79161=CARTESIAN_POINT ( 'NONE',  ( -0.1574803149606292529, -0.1870078740157480879, -0.4822834645669291653 ) ) ;
#79162=CARTESIAN_POINT ( 'NONE',  ( -0.3280839895013117347, -0.004921259842519870586, -0.3153832671262229437 ) ) ;
#79164=CARTESIAN_POINT ( 'NONE',  ( -0.08530183727034056085, -0.2845877964562159024, 0.3641732283464567677 ) ) ;
#79165=CARTESIAN_POINT ( 'NONE',  ( 0.1574803149606306130, -0.1870078740157480879, -0.4822834645669291653 ) ) ;
#79166=CARTESIAN_POINT ( 'NONE',  ( -0.7020997375328076329, -0.2845877964562161244, -0.3641732283464567121 ) ) ;
#79168=CARTESIAN_POINT ( 'NONE',  ( -0.9383202099737524282, -0.3162353388693409650, -0.4822834645669289433 ) ) ;
#79171=CARTESIAN_POINT ( 'NONE',  ( -0.9711286089238838626, -0.5023911411419708095, 0.1820866141732285504 ) ) ;
#79172=CARTESIAN_POINT ( 'NONE',  ( 0.06561679790026316017, 0.05413385826771626580, -0.4176697321401330321 ) ) ;
#79174=CARTESIAN_POINT ( 'NONE',  ( -1.568241469816272105, -0.05778040916215522460, 0.4822834645669289988 ) ) ;
#79175=CARTESIAN_POINT ( 'NONE',  ( -0.7939632545931750718, -0.05778040916215560624, -0.4822834645669293319 ) ) ;
#79176=( BOUNDED_CURVE ( )  B_SPLINE_CURVE ( 2, ( #14724, #59726, #2081, #16378, #2502, #3321, #73200, #36129, #67718, #35308, #80767, #79950, #15968 ),
 .UNSPECIFIED., .F., .F. ) 
 B_SPLINE_CURVE_WITH_KNOTS ( ( 3, 2, 2, 2, 2, 2, 3 ),
 ( 0.6278765491802553722, 0.6287878787878787845, 0.6325757575757575690, 0.6363636363636363535, 0.6401515151515151381, 0.6439393939393939226, 0.6448507235470174459 ),
 .UNSPECIFIED. ) 
 CURVE ( )  GEOMETRIC_REPRESENTATION_ITEM ( )  RATIONAL_B_SPLINE_CURVE ( ( 0.9875488213027523443, 0.9918020599134680371, 1.000000000000000000, 0.9659258262890683122, 1.000000000000000000, 0.9659258262890683122, 1.000000000000000000, 0.9659258262890683122, 1.000000000000000000, 0.9659258262890683122, 1.000000000000000000, 0.9918020599134671489, 0.9875488213027514561 ) ) 
 REPRESENTATION_ITEM ( '' )  );
#79178=CARTESIAN_POINT ( 'NONE',  ( -0.8923884514435688198, 0.2306618581243847221, -0.2411417322834647770 ) ) ;
#79179=CARTESIAN_POINT ( 'NONE',  ( 0.9580052493438326877, 0.05413385826771666132, 0.4176697321401328100 ) ) ;
#79180=CARTESIAN_POINT ( 'NONE',  ( 1.030183727034121421, -0.05778040916215522460, 0.4822834645669289988 ) ) ;
#79183=CARTESIAN_POINT ( 'NONE',  ( -1.391076115485563758, 0.2306618581243848609, 0.2411417322834645549 ) ) ;
#79186=CARTESIAN_POINT ( 'NONE',  ( -0.4461942257217840213, -0.5023911411419708095, -0.1820866141732282451 ) ) ;
#79189=CARTESIAN_POINT ( 'NONE',  ( 0.8858267716535438430, -0.5400638737290845981, -0.3530559997133363437 ) ) ;
#79190=CARTESIAN_POINT ( 'NONE',  ( -0.1181102362204717315, 0.2952755905511811885, 0.000000000000000000 ) ) ;
#79191=CARTESIAN_POINT ( 'NONE',  ( -0.8267716535433065062, 0.2952755905511811885, 0.000000000000000000 ) ) ;
#79192=CARTESIAN_POINT ( 'NONE',  ( 1.607611548556431069, -0.6692913385826773087, -0.1292274648535924053 ) ) ;
#79193=CARTESIAN_POINT ( 'NONE',  ( -0.8136482939632537770, 0.1283753931104746893, -0.1820866141732285504 ) ) ;
#79195=CARTESIAN_POINT ( 'NONE',  ( 0.4199475065616805614, 0.2306618581243848609, 0.2411417322834645549 ) ) ;
#79196=CARTESIAN_POINT ( 'NONE',  ( 0.6889763779527563470, 0.07958543189024071263, -0.2665933059059888421 ) ) ;
#79197=CARTESIAN_POINT ( 'NONE',  ( -0.5708661417322825615, -0.5400638737290844871, 0.3530559997133364547 ) ) ;
#79199=CARTESIAN_POINT ( 'NONE',  ( -1.345144356955379816, -0.3162353388693405765, 0.4822834645669290543 ) ) ;
#79201=CARTESIAN_POINT ( 'NONE',  ( 1.233595800524935227, 0.2306618581243847221, -0.2411417322834647770 ) ) ;
#79202=CARTESIAN_POINT ( 'NONE',  ( 1.463254593175853824, -0.5511811023622046335, 0.09757992244046803654 ) ) ;
#79203=ORIENTED_EDGE ( 'NONE', *, *, #2022, .F. ) ;
#79205=CARTESIAN_POINT ( 'NONE',  ( -0.3937007874015740483, -0.1870078740157479769, 0.4822834645669291653 ) ) ;
#79207=CARTESIAN_POINT ( 'NONE',  ( 0.6102362204724416372, -0.4536011799217367080, 0.2665933059059888421 ) ) ;
#79208=CARTESIAN_POINT ( 'NONE',  ( -1.023622047244094002, -0.1870078740157480879, -0.4822834645669291653 ) ) ;
#79209=CARTESIAN_POINT ( 'NONE',  ( 1.003937007874016185, 0.1660481256975883668, -0.3530559997133364547 ) ) ;
#79210=CARTESIAN_POINT ( 'NONE',  ( 0.6364829396325465405, -0.05778040916215522460, 0.4822834645669289988 ) ) ;
#79211=CARTESIAN_POINT ( 'NONE',  ( 0.1509186351706042484, -0.3162353388693405765, 0.4822834645669290543 ) ) ;
#79212=CARTESIAN_POINT ( 'NONE',  ( -0.5380577427821514602, 0.05413385826771666132, 0.4176697321401328100 ) ) ;
#79214=CARTESIAN_POINT ( 'NONE',  ( 1.548556430446194954, -0.5023911411419708095, 0.1820866141732285504 ) ) ;
#79215=CARTESIAN_POINT ( 'NONE',  ( -0.7283464566929126471, -0.5400638737290844871, 0.3530559997133364547 ) ) ;
#79216=CARTESIAN_POINT ( 'NONE',  ( -0.6233595800524928121, -0.2845877964562161244, -0.3641732283464567121 ) ) ;
#79217=CARTESIAN_POINT ( 'NONE',  ( 1.646981627296588035, -0.3162353388693405765, 0.4822834645669290543 ) ) ;
#79219=CARTESIAN_POINT ( 'NONE',  ( -0.3674540682414692561, -0.6046776061558809534, -0.2411417322834644161 ) ) ;
#79220=CARTESIAN_POINT ( 'NONE',  ( 0.2624671916010504757, 0.1539470093639523085, 0.1968503937007873850 ) ) ;
#79221=CARTESIAN_POINT ( 'NONE',  ( 0.7217847769028878924, -0.4281496062992127816, -0.4176697321401328100 ) ) ;
#79224=CARTESIAN_POINT ( 'NONE',  ( -0.08530183727034056085, -0.3162353388693405765, 0.4822834645669290543 ) ) ;
#79225=CARTESIAN_POINT ( 'NONE',  ( 0.9186351706036752773, 0.1283753931104746893, -0.1820866141732285504 ) ) ;
#79228=CARTESIAN_POINT ( 'NONE',  ( 1.286089238845145033, -0.5023911411419708095, -0.1820866141732282451 ) ) ;
#79230=CARTESIAN_POINT ( 'NONE',  ( 1.017060367454068581, -0.05778040916215560624, -0.4822834645669293319 ) ) ;
#79232=CARTESIAN_POINT ( 'NONE',  ( -0.1902887139107604098, -0.6692913385826771977, 0.1292274648535927661 ) ) ;
#79233=CARTESIAN_POINT ( 'NONE',  ( -1.640419947506561060, 0.05413385826771666132, 0.4176697321401328100 ) ) ;
#79234=CARTESIAN_POINT ( 'NONE',  ( -1.719160104986876103, 0.05413385826771666132, 0.4176697321401328100 ) ) ;
#79235=CARTESIAN_POINT ( 'NONE',  ( -0.07874015748031421014, -0.1870078740157480879, -0.4822834645669291653 ) ) ;
#79237=CARTESIAN_POINT ( 'NONE',  ( 1.089238845144357759, 0.05413385826771626580, -0.4176697321401330321 ) ) ;
#79238=CARTESIAN_POINT ( 'NONE',  ( 0.3937007874015754361, -0.1870078740157480879, -0.4822834645669291653 ) ) ;
#79239=CARTESIAN_POINT ( 'NONE',  ( 0.5839895013123367340, 0.1771653543307087630, 0.09757992244046791164 ) ) ;
#79241=CARTESIAN_POINT ( 'NONE',  ( 0.4461942257217856311, 0.1283753931104746893, -0.1820866141732285504 ) ) ;
#79242=CARTESIAN_POINT ( 'NONE',  ( -1.036394771582349383, 0.004960608223777852183, -0.3437734562760195733 ) ) ;
#79244=CARTESIAN_POINT ( 'NONE',  ( 0.7874015748031503170, -0.1870078740157480879, -0.4822834645669291653 ) ) ;
#79246=CARTESIAN_POINT ( 'NONE',  ( 0.8923884514435703741, 0.2306618581243848609, 0.2411417322834645549 ) ) ;
#79247=CARTESIAN_POINT ( 'NONE',  ( -0.3412073490813641308, 0.1539470093639521697, -0.1968503937007875793 ) ) ;
#79248=CARTESIAN_POINT ( 'NONE',  ( 0.1377952755905518800, -0.4536011799217367080, 0.2665933059059888421 ) ) ;
#79249=CARTESIAN_POINT ( 'NONE',  ( -0.06561679790026180015, 0.05413385826771666132, 0.4176697321401328100 ) ) ;
#79250=CARTESIAN_POINT ( 'NONE',  ( 1.207349081364829990, 0.1283753931104748280, 0.1820866141732283561 ) ) ;
#79251=CARTESIAN_POINT ( 'NONE',  ( -1.220472440944881054, 0.1771653543307087630, 0.000000000000000000 ) ) ;
#79252=CARTESIAN_POINT ( 'NONE',  ( -1.043307086614172707, 0.1660481256975883668, -0.3530559997133364547 ) ) ;
#79253=CARTESIAN_POINT ( 'NONE',  ( -1.692913385826770645, 0.2952755905511811885, 0.000000000000000000 ) ) ;
#79254=CARTESIAN_POINT ( 'NONE',  ( 0.7349081364829403995, 0.2306618581243848609, 0.2411417322834645549 ) ) ;
#79255=CARTESIAN_POINT ( 'NONE',  ( 1.404199475065617708, 0.05413385826771626580, -0.4176697321401330321 ) ) ;
#79257=CARTESIAN_POINT ( 'NONE',  ( 0.7020997375328090762, -0.05778040916215560624, -0.4822834645669293319 ) ) ;
#79260=CARTESIAN_POINT ( 'NONE',  ( 1.233595800524935227, 0.2306618581243847221, -0.2411417322834647770 ) ) ;
#79261=CARTESIAN_POINT ( 'NONE',  ( -1.450131233595799651, -0.5511811023622046335, 0.09757992244046803654 ) ) ;
#79262=CARTESIAN_POINT ( 'NONE',  ( 1.056430446194226658, 0.1771653543307087630, 0.09757992244046791164 ) ) ;
#79263=CARTESIAN_POINT ( 'NONE',  ( -1.371391076115484609, -0.5511811023622046335, 0.09757992244046803654 ) ) ;
#79264=CARTESIAN_POINT ( 'NONE',  ( -0.7349081364829387342, -0.5023911411419708095, 0.1820866141732285504 ) ) ;
#79266=CARTESIAN_POINT ( 'NONE',  ( 0.5774278215223103139, -0.5023911411419708095, -0.1820866141732282451 ) ) ;
#79267=CARTESIAN_POINT ( 'NONE',  ( 0.1902887139107617975, -0.6692913385826773087, -0.1292274648535924053 ) ) ;
#79268=CARTESIAN_POINT ( 'NONE',  ( 1.292650918635171564, 0.2952755905511811885, 0.1292274648535926551 ) ) ;
#79269=CARTESIAN_POINT ( 'NONE',  ( -0.03937007874015669567, 0.2952755905511811885, 0.000000000000000000 ) ) ;
#79270=EDGE_CURVE ( 'NONE', #48838, #22548, #54439, .T. ) ;
#79271=CARTESIAN_POINT ( 'NONE',  ( 0.006561679790026889343, -0.08942795157527998196, 0.3641732283464567121 ) ) ;
#79272=CARTESIAN_POINT ( 'NONE',  ( 1.062992125984252745, -0.6692913385826771977, 8.415575281601705876E-17 ) ) ;
#79273=DIRECTION ( 'NONE',  ( 3.096699300667737957E-16, -1.000000000000000000, 0.000000000000000000 ) ) ;
#79274=CARTESIAN_POINT ( 'NONE',  ( -1.023622047244094002, -0.1870078740157480879, -0.4822834645669291653 ) ) ;
#79277=CARTESIAN_POINT ( 'NONE',  ( -0.8595800524934373854, -0.05778040916215522460, 0.4822834645669289988 ) ) ;
#79278=CARTESIAN_POINT ( 'NONE',  ( -0.2690288713910754526, 0.2952755905511810774, -0.1292274648535930714 ) ) ;
#79283=CARTESIAN_POINT ( 'NONE',  ( -1.614173228346456712, 2.401574803149606474, 0.1372047244094477536 ) ) ;
#79284=CARTESIAN_POINT ( 'NONE',  ( -1.469816272965878357, -0.5023911411419708095, -0.1820866141732282451 ) ) ;
#79286=CARTESIAN_POINT ( 'NONE',  ( 1.587926509186352142, -0.004921259842519576551, 0.3153832671262227771 ) ) ;
#79288=CARTESIAN_POINT ( 'NONE',  ( -0.1509186351706028884, -0.3162353388693409650, -0.4822834645669289433 ) ) ;
#79289=CARTESIAN_POINT ( 'NONE',  ( -0.5183727034120726440, -0.5511811023622048555, -0.09757992244046775898 ) ) ;
#79290=CARTESIAN_POINT ( 'NONE',  ( 0.6955380577427828781, 0.05413385826771626580, -0.4176697321401330321 ) ) ;
#79292=CARTESIAN_POINT ( 'NONE',  ( 0.3543307086614179147, 0.2952755905511811885, 0.000000000000000000 ) ) ;
#79295=CARTESIAN_POINT ( 'NONE',  ( 1.450131233595801428, -0.6692913385826773087, -0.1292274648535924053 ) ) ;
#79296=CARTESIAN_POINT ( 'NONE',  ( 0.1902887139107617975, 0.2952755905511811885, 0.1292274648535926551 ) ) ;
#79297=CARTESIAN_POINT ( 'NONE',  ( -0.8267716535433065062, 0.2952755905511811885, 0.000000000000000000 ) ) ;
#79298=CARTESIAN_POINT ( 'NONE',  ( 1.364829396325459854, -0.6046776061558809534, -0.2411417322834644161 ) ) ;
#79299=CARTESIAN_POINT ( 'NONE',  ( 0.8202099737532814183, -0.6692913385826773087, -0.1292274648535924053 ) ) ;
#79301=CARTESIAN_POINT ( 'NONE',  ( -0.04593175853018302557, -0.6692913385826773087, -0.1292274648535924053 ) ) ;
#79302=CARTESIAN_POINT ( 'NONE',  ( 0.6627296587926517768, -0.6692913385826773087, -0.1292274648535924053 ) ) ;
#79303=CARTESIAN_POINT ( 'NONE',  ( -0.006561679790025524116, -0.05778040916215560624, -0.4822834645669293319 ) ) ;
#79304=CARTESIAN_POINT ( 'NONE',  ( 0.6430446194225729606, -0.3690944881889765550, -0.3153832671262227771 ) ) ;
#79305=CARTESIAN_POINT ( 'NONE',  ( -1.509186351706035767, 0.05413385826771626580, -0.4176697321401330321 ) ) ;
#79306=CARTESIAN_POINT ( 'NONE',  ( -1.463254593175852492, -0.6692913385826773087, -0.1292274648535924053 ) ) ;
#79307=CARTESIAN_POINT ( 'NONE',  ( 0.6167979002624678353, -0.4281496062992124485, 0.4176697321401328655 ) ) ;
#79310=ORIENTED_EDGE ( 'NONE', *, *, #8336, .T. ) ;
#79313=CARTESIAN_POINT ( 'NONE',  ( 1.108923884514436686, -0.3162353388693409650, -0.4822834645669289433 ) ) ;
#79314=CARTESIAN_POINT ( 'NONE',  ( 0.6627296587926515548, 0.1771653543307087630, 0.09757992244046791164 ) ) ;
#79316=CARTESIAN_POINT ( 'NONE',  ( -0.8561328129276786214, -2.191421614605370878E-15, 0.4445507791589071167 ) ) ;
#79317=CARTESIAN_POINT ( 'NONE',  ( 1.614173228346457378, 1.330640075373405118, 0.1372047244094478369 ) ) ;
#79319=CARTESIAN_POINT ( 'NONE',  ( -1.561679790026246017, -0.4281496062992127816, -0.4176697321401328100 ) ) ;
#79320=CARTESIAN_POINT ( 'NONE',  ( -0.2559055118110230564, 0.1660481256975883668, -0.3530559997133364547 ) ) ;
#79321=CARTESIAN_POINT ( 'NONE',  ( 0.9120734908136489683, -0.6692913385826771977, 0.1292274648535927661 ) ) ;
#79323=ADVANCED_FACE ( 'NONE', ( #7634 ), #24495, .F. ) ;
#79324=CARTESIAN_POINT ( 'NONE',  ( -1.417322834645668772, -0.1870078740157479769, 0.4822834645669291653 ) ) ;
#79325=CARTESIAN_POINT ( 'NONE',  ( -1.171093442848938793, -2.191421614605370878E-15, 0.4445507791589071167 ) ) ;
#79328=CARTESIAN_POINT ( 'NONE',  ( -1.194225721784776262, -0.3690944881889763329, 0.3153832671262228327 ) ) ;
#79329=CARTESIAN_POINT ( 'NONE',  ( -1.607611548556429737, 0.2952755905511810774, -0.1292274648535930714 ) ) ;
#79330=CARTESIAN_POINT ( 'NONE',  ( 0.2624671916010504757, 0.2306618581243848609, 0.2411417322834645549 ) ) ;
#79331=ORIENTED_EDGE ( 'NONE', *, *, #61119, .T. ) ;
#79332=CARTESIAN_POINT ( 'NONE',  ( 1.633858267716535639, -0.5400638737290844871, 0.3530559997133364547 ) ) ;
#79333=CARTESIAN_POINT ( 'NONE',  ( -0.4396325459317579343, 0.2066929133858267931, 0.1054918080437490802 ) ) ;
#79334=CARTESIAN_POINT ( 'NONE',  ( -0.8792650918635160906, -0.004921259842519870586, -0.3153832671262229437 ) ) ;
#79335=CARTESIAN_POINT ( 'NONE',  ( 0.7152230971128616943, -0.05778040916215522460, 0.4822834645669289988 ) ) ;
#79336=CARTESIAN_POINT ( 'NONE',  ( 1.351706036745407458, -0.3690944881889765550, -0.3153832671262227771 ) ) ;
#79338=CARTESIAN_POINT ( 'NONE',  ( -0.7152230971128602510, -0.08942795157528024563, -0.3641732283464568787 ) ) ;
#79339=CARTESIAN_POINT ( 'NONE',  ( -1.482939632545930975, -0.004921259842519576551, 0.3153832671262227771 ) ) ;
#79341=CARTESIAN_POINT ( 'NONE',  ( 0.5446194225721792126, -0.05778040916215560624, -0.4822834645669293319 ) ) ;
#79342=CARTESIAN_POINT ( 'NONE',  ( -1.003937007874014853, 0.07958543189024085140, 0.2665933059059887866 ) ) ;
#79343=CARTESIAN_POINT ( 'NONE',  ( -0.4002624671916004129, -0.08942795157528024563, -0.3641732283464568787 ) ) ;
#79344=CARTESIAN_POINT ( 'NONE',  ( -0.3018372703412066094, 0.05413385826771666132, 0.4176697321401328100 ) ) ;
#79345=CARTESIAN_POINT ( 'NONE',  ( -1.522309711286088607, -0.5023911411419708095, 0.1820866141732285504 ) ) ;
#79347=CARTESIAN_POINT ( 'NONE',  ( 0.5380577427821529035, 0.05413385826771626580, -0.4176697321401330321 ) ) ;
#79352=CARTESIAN_POINT ( 'NONE',  ( -0.6364829396325453192, -0.3162353388693405765, 0.4822834645669290543 ) ) ;
#79353=CARTESIAN_POINT ( 'NONE',  ( -0.1443569553805768291, -0.004921259842519576551, 0.3153832671262227771 ) ) ;
#79354=CARTESIAN_POINT ( 'NONE',  ( -1.253280839895012377, -0.3162353388693409650, -0.4822834645669289433 ) ) ;
#79355=CARTESIAN_POINT ( 'NONE',  ( 0.6167979002624679463, -0.004921259842519870586, -0.3153832671262229437 ) ) ;
#79356=CARTESIAN_POINT ( 'NONE',  ( -0.7349081364829390672, 0.1283753931104746893, -0.1820866141732285504 ) ) ;
#79357=CARTESIAN_POINT ( 'NONE',  ( -1.266404199475064773, -0.3162353388693405765, 0.4822834645669290543 ) ) ;
#79358=CARTESIAN_POINT ( 'NONE',  ( -1.732283464566928277, -0.1870078740157479769, 0.4822834645669291653 ) ) ;
#79359=CARTESIAN_POINT ( 'NONE',  ( 1.240157480314961314, 0.1660481256975883668, -0.3530559997133364547 ) ) ;
#79360=CARTESIAN_POINT ( 'NONE',  ( -0.6575345472713096662, 1.929133858267489954, 0.5309055118110236338 ) ) ;
#79361=CARTESIAN_POINT ( 'NONE',  ( 1.003937007874016407, -0.4536011799217367080, 0.2665933059059888421 ) ) ;
#79362=CARTESIAN_POINT ( 'NONE',  ( 0.2624671916010504757, 0.2306618581243848609, 0.2411417322834645549 ) ) ;
#79363=CARTESIAN_POINT ( 'NONE',  ( -1.581364829396324945, -0.05778040916215560624, -0.4822834645669293319 ) ) ;
#79364=CARTESIAN_POINT ( 'NONE',  ( 1.220472440944882386, -0.5511811023622047445, 6.969142054262312111E-17 ) ) ;
#79367=CARTESIAN_POINT ( 'NONE',  ( -1.345144356955379816, -0.2845877964562159024, 0.3641732283464567677 ) ) ;
#79368=CARTESIAN_POINT ( 'NONE',  ( -0.3346456692913377662, 0.1660481256975883668, -0.3530559997133364547 ) ) ;
#79369=CARTESIAN_POINT ( 'NONE',  ( 0.1837270341207354329, 0.2306618581243848609, 0.2411417322834645549 ) ) ;
#79370=CARTESIAN_POINT ( 'NONE',  ( -1.601049868766403650, -0.5023911411419708095, 0.1820866141732285504 ) ) ;
#79372=CARTESIAN_POINT ( 'NONE',  ( -1.456692913385826182, -0.6692913385826771977, 8.415575281601705876E-17 ) ) ;
#79373=CARTESIAN_POINT ( 'NONE',  ( 0.3149606299212606708, -0.1870078740157480879, -0.4822834645669291653 ) ) ;
#79374=CARTESIAN_POINT ( 'NONE',  ( -0.05249343832020911260, 0.2306618581243848609, 0.2411417322834645549 ) ) ;
#79375=CARTESIAN_POINT ( 'NONE',  ( 1.286089238845145033, 0.2306618581243848609, 0.2411417322834645549 ) ) ;
#79381=CARTESIAN_POINT ( 'NONE',  ( -0.03280839895013062252, -0.5511811023622046335, 0.09757992244046803654 ) ) ;
#79382=CARTESIAN_POINT ( 'NONE',  ( -0.4790026246719154557, -0.3162353388693405765, 0.4822834645669290543 ) ) ;
#79383=CARTESIAN_POINT ( 'NONE',  ( 0.9317585301837276734, -0.4281496062992124485, 0.4176697321401328655 ) ) ;
#79385=CARTESIAN_POINT ( 'NONE',  ( 0.1640419947506569498, -0.2845877964562161244, -0.3641732283464567121 ) ) ;
#79386=CARTESIAN_POINT ( 'NONE',  ( -1.253280839895012377, -0.3162353388693409650, -0.4822834645669289433 ) ) ;
#79387=CARTESIAN_POINT ( 'NONE',  ( 1.541994750656168645, -0.6692913385826771977, 0.1292274648535927661 ) ) ;
#79392=CARTESIAN_POINT ( 'NONE',  ( 1.161417322834646271, 0.1660481256975883668, -0.3530559997133364547 ) ) ;
#79393=CARTESIAN_POINT ( 'NONE',  ( 1.450131233595801428, 0.1771653543307087630, 0.09757992244046791164 ) ) ;
#79394=CARTESIAN_POINT ( 'NONE',  ( -1.056430446194224881, -0.5511811023622046335, 0.09757992244046803654 ) ) ;
#79395=CARTESIAN_POINT ( 'NONE',  ( -1.082677165354329896, -0.5400638737290845981, -0.3530559997133363437 ) ) ;
#79398=CARTESIAN_POINT ( 'NONE',  ( 1.410761154855643795, -0.05778040916215560624, -0.4822834645669293319 ) ) ;
#79399=CARTESIAN_POINT ( 'NONE',  ( -1.620734908136482577, -0.6692913385826773087, -0.1292274648535924053 ) ) ;
#79400=CARTESIAN_POINT ( 'NONE',  ( 0.1115485564304467270, -0.6692913385826773087, -0.1292274648535924053 ) ) ;
#79401=CARTESIAN_POINT ( 'NONE',  ( -0.2099737532808391705, -0.6046776061558809534, -0.2411417322834644161 ) ) ;
#79403=CARTESIAN_POINT ( 'NONE',  ( -1.148293963254592542, 0.2952755905511811885, 0.1292274648535926551 ) ) ;
#79405=CARTESIAN_POINT ( 'NONE',  ( 0.5511811023622054106, -0.1870078740157480879, -0.4822834645669291653 ) ) ;
#79407=CARTESIAN_POINT ( 'NONE',  ( -1.338582677165353729, -0.1870078740157479769, 0.3641732283464567677 ) ) ;
#79410=VERTEX_POINT ( 'NONE', #38587 ) ;
#79412=CARTESIAN_POINT ( 'NONE',  ( -1.384514435695537005, 0.2952755905511811885, 0.1292274648535926551 ) ) ;
#79413=CARTESIAN_POINT ( 'NONE',  ( -1.128608923884513837, 0.2306618581243847221, -0.2411417322834647770 ) ) ;
#79415=CARTESIAN_POINT ( 'NONE',  ( -1.397637795275589623, 0.1660481256975885056, 0.3530559997133364547 ) ) ;
#79416=CARTESIAN_POINT ( 'NONE',  ( -1.476377952755905110, -0.5400638737290845981, -0.3530559997133363437 ) ) ;
#79419=CARTESIAN_POINT ( 'NONE',  ( -0.3674540682414689785, 0.1283753931104748280, 0.1820866141732283561 ) ) ;
#79420=CARTESIAN_POINT ( 'NONE',  ( -0.8661417322834640276, -0.1870078740157480601, -0.3641732283464567677 ) ) ;
#79421=CARTESIAN_POINT ( 'NONE',  ( -1.135170603674539924, 0.2952755905511810774, -0.1292274648535930714 ) ) ;
#79422=CARTESIAN_POINT ( 'NONE',  ( 0.7677165354330716118, -0.5400638737290844871, 0.3530559997133364547 ) ) ;
#79423=CARTESIAN_POINT ( 'NONE',  ( -0.9251968503937002541, -0.5400638737290845981, -0.3530559997133363437 ) ) ;
#79426=ADVANCED_FACE ( 'NONE', ( #58783 ), #76894, .F. ) ;
#79427=CARTESIAN_POINT ( 'NONE',  ( -1.332020997375327642, -0.05778040916215522460, 0.4822834645669289988 ) ) ;
#79428=CARTESIAN_POINT ( 'NONE',  ( -1.377952755905511140, 0.1771653543307087630, 0.000000000000000000 ) ) ;
#79429=CARTESIAN_POINT ( 'NONE',  ( -1.679790026246718693, 0.2306618581243847221, -0.2411417322834647770 ) ) ;
#79435=CARTESIAN_POINT ( 'NONE',  ( -0.4002624671916004129, -0.3162353388693405765, 0.4822834645669290543 ) ) ;
#79436=CARTESIAN_POINT ( 'NONE',  ( -1.345144356955379816, -0.2845877964562159024, 0.3641732283464567677 ) ) ;
#79438=DIRECTION ( 'NONE',  ( 2.956072690630991733E-16, -1.000000000000000000, -5.002896285981958034E-32 ) ) ;
#79440=CARTESIAN_POINT ( 'NONE',  ( -1.627296587926508442, -0.6046776061558809534, -0.2411417322834644161 ) ) ;
#79441=CARTESIAN_POINT ( 'NONE',  ( -0.2952755905511804668, 0.1660481256975885056, 0.3530559997133364547 ) ) ;
#79443=CARTESIAN_POINT ( 'NONE',  ( 0.6167979002624678353, -0.3690944881889763329, 0.3153832671262228327 ) ) ;
#79445=CARTESIAN_POINT ( 'NONE',  ( 0.2821522309711292364, 0.1771653543307087075, -0.09757992244046823083 ) ) ;
#79446=CARTESIAN_POINT ( 'NONE',  ( 0.7939632545931766261, -0.08942795157527998196, 0.3641732283464567121 ) ) ;
#79447=CARTESIAN_POINT ( 'NONE',  ( 0.8136482939632553313, 0.2306618581243848609, 0.2411417322834645549 ) ) ;
#79448=CARTESIAN_POINT ( 'NONE',  ( -0.1377952755905504645, -0.4536011799217368745, -0.2665933059059886201 ) ) ;
#79450=CARTESIAN_POINT ( 'NONE',  ( -1.207349081364828436, -0.6046776061558807314, 0.2411417322834647770 ) ) ;
#79451=CARTESIAN_POINT ( 'NONE',  ( 0.1115485564304467270, -0.5511811023622048555, -0.09757992244046775898 ) ) ;
#79453=CARTESIAN_POINT ( 'NONE',  ( -1.332020997375327642, -0.08942795157527998196, 0.3641732283464567121 ) ) ;
#79455=CARTESIAN_POINT ( 'NONE',  ( -1.049868766404198794, -0.5023911411419708095, 0.1820866141732285504 ) ) ;
#79458=CARTESIAN_POINT ( 'NONE',  ( -0.06561679790026180015, 0.05413385826771666132, 0.4176697321401328100 ) ) ;
#79460=CARTESIAN_POINT ( 'NONE',  ( 0.5511811023622054106, -0.1870078740157480601, -0.3641732283464567677 ) ) ;
#79461=CARTESIAN_POINT ( 'NONE',  ( -0.4330708661417315697, 0.1771653543307087630, 0.000000000000000000 ) ) ;
#79462=CARTESIAN_POINT ( 'NONE',  ( -0.8727034120734901146, -0.3162353388693405765, 0.4822834645669290543 ) ) ;
#79464=CARTESIAN_POINT ( 'NONE',  ( -0.9448818897637790704, -0.1870078740157480601, -0.3641732283464567677 ) ) ;
#79466=CARTESIAN_POINT ( 'NONE',  ( 0.3805774278215230400, -0.4281496062992124485, 0.4176697321401328655 ) ) ;
#79467=AXIS2_PLACEMENT_3D ( 'NONE', #54126, #73931, #16274 ) ;
#79469=CARTESIAN_POINT ( 'NONE',  ( -1.595398199321656607, 1.309738123151862998, -0.1559797534342480529 ) ) ;
#79470=CARTESIAN_POINT ( 'NONE',  ( -0.2952755905511804668, 0.07958543189024085140, 0.2665933059059887866 ) ) ;
#79471=CARTESIAN_POINT ( 'NONE',  ( -0.07217847769028813698, -0.3162353388693409650, -0.4822834645669289433 ) ) ;
#79472=CARTESIAN_POINT ( 'NONE',  ( -1.515748031496062076, -0.5400638737290844871, 0.3530559997133364547 ) ) ;
#79473=CARTESIAN_POINT ( 'NONE',  ( -1.568241469816272105, -0.2845877964562161244, -0.3641732283464567121 ) ) ;
#79474=CARTESIAN_POINT ( 'NONE',  ( 1.240157480314961314, 0.1660481256975883668, -0.3530559997133364547 ) ) ;
#79475=CARTESIAN_POINT ( 'NONE',  ( -0.6102362204724400829, 0.07958543189024085140, 0.2665933059059887866 ) ) ;
#79476=CARTESIAN_POINT ( 'NONE',  ( -0.7749820319012115100, 0.000000000000000000, 0.3464511005275205946 ) ) ;
#79479=EDGE_CURVE ( 'NONE', #11346, #47146, #25531, .T. ) ;
#79480=VECTOR ( 'NONE', #4660, 39.37007874015748143 ) ;
#79482=CARTESIAN_POINT ( 'NONE',  ( 0.9580052493438326877, -0.004921259842519576551, 0.3153832671262227771 ) ) ;
#79483=CARTESIAN_POINT ( 'NONE',  ( -1.620734908136482577, -0.6692913385826773087, -0.1292274648535924053 ) ) ;
#79484=CARTESIAN_POINT ( 'NONE',  ( 0.8464566929133865436, 0.1660481256975883668, -0.3530559997133364547 ) ) ;
#79486=CARTESIAN_POINT ( 'NONE',  ( 1.371391076115485941, 0.1771653543307087630, 0.09757992244046791164 ) ) ;
#79487=CARTESIAN_POINT ( 'NONE',  ( 0.2952755905511819101, 0.1660481256975883668, -0.3530559997133364547 ) ) ;
#79488=CARTESIAN_POINT ( 'NONE',  ( -0.5380577427821514602, 0.05413385826771666132, 0.4176697321401328100 ) ) ;
#79489=CARTESIAN_POINT ( 'NONE',  ( 1.601049868766404982, -0.6046776061558809534, -0.2411417322834644161 ) ) ;
#79492=CARTESIAN_POINT ( 'NONE',  ( 0.5380577427821529035, -0.004921259842519870586, -0.3153832671262229437 ) ) ;
#79493=ORIENTED_EDGE ( 'NONE', *, *, #45942, .T. ) ;
#79496=CARTESIAN_POINT ( 'NONE',  ( -0.5708661417322828946, 0.1660481256975883668, -0.3530559997133364547 ) ) ;
#79497=CARTESIAN_POINT ( 'NONE',  ( 1.181102362204724976, -0.1870078740157480879, -0.4822834645669291653 ) ) ;
#79498=CARTESIAN_POINT ( 'NONE',  ( 0.05249343832021075018, -0.6046776061558807314, 0.2411417322834647770 ) ) ;
#79499=CARTESIAN_POINT ( 'NONE',  ( -0.5446194225721777693, -0.08942795157527998196, 0.3641732283464567121 ) ) ;
#79500=CARTESIAN_POINT ( 'NONE',  ( 0.7677165354330716118, 0.1660481256975883668, -0.3530559997133364547 ) ) ;
#79501=CARTESIAN_POINT ( 'NONE',  ( -0.8136482939632537770, 0.2306618581243847221, -0.2411417322834647770 ) ) ;
#79502=CARTESIAN_POINT ( 'NONE',  ( -0.4396325459317579898, 0.2952755905511811885, 0.1292274648535926551 ) ) ;
#79503=CARTESIAN_POINT ( 'NONE',  ( -0.7545931758530177724, 0.2952755905511811885, 0.1292274648535926551 ) ) ;
#79504=CARTESIAN_POINT ( 'NONE',  ( 1.227034120734908917, -0.6692913385826771977, 0.1292274648535927661 ) ) ;
#79505=CARTESIAN_POINT ( 'NONE',  ( 0.8595800524934390507, -0.05778040916215560624, -0.4822834645669293319 ) ) ;
#79506=EDGE_CURVE ( 'NONE', #71072, #75665, #9292, .T. ) ;
#79507=CARTESIAN_POINT ( 'NONE',  ( 0.9055118110236227702, 0.2952755905511811885, 0.000000000000000000 ) ) ;
#79509=CARTESIAN_POINT ( 'NONE',  ( 0.1246719160104994284, 0.1771653543307087075, -0.09757992244046823083 ) ) ;
#79512=ORIENTED_EDGE ( 'NONE', *, *, #37312, .T. ) ;
#79513=CARTESIAN_POINT ( 'NONE',  ( -0.8333333333333323711, -0.5511811023622048555, -0.09757992244046775898 ) ) ;
#79515=CARTESIAN_POINT ( 'NONE',  ( -0.09842519685039295696, -0.5400638737290844871, 0.3530559997133364547 ) ) ;
#79516=CARTESIAN_POINT ( 'NONE',  ( -1.614173228346456712, 0.000000000000000000, -0.1372047244094478091 ) ) ;
#79517=CARTESIAN_POINT ( 'NONE',  ( -0.4068241469816267775, 0.05413385826771626580, -0.4176697321401330321 ) ) ;
#79518=CARTESIAN_POINT ( 'NONE',  ( -0.5446194225721777693, -0.3162353388693409650, -0.4822834645669289433 ) ) ;
#79519=CARTESIAN_POINT ( 'NONE',  ( -1.404199475065615932, -0.4281496062992127816, -0.4176697321401328100 ) ) ;
#79520=CARTESIAN_POINT ( 'NONE',  ( -1.227034120734907585, 0.2952755905511811885, 0.1292274648535926551 ) ) ;
#79521=CARTESIAN_POINT ( 'NONE',  ( 1.384514435695538559, 0.1771653543307087075, -0.09757992244046823083 ) ) ;
#79524=CARTESIAN_POINT ( 'NONE',  ( 0.4658792650918640033, -0.2845877964562159024, 0.3641732283464567677 ) ) ;
#79525=CARTESIAN_POINT ( 'NONE',  ( 0.2493438320209980519, 0.05413385826771666132, 0.4176697321401328100 ) ) ;
#79526=CARTESIAN_POINT ( 'NONE',  ( 0.3937007874015754361, -0.1870078740157479769, 0.4822834645669291653 ) ) ;
#79527=ORIENTED_EDGE ( 'NONE', *, *, #76941, .T. ) ;
#79528=AXIS2_PLACEMENT_3D ( 'NONE', #15441, #66790, #2806 ) ;
#79530=CARTESIAN_POINT ( 'NONE',  ( -0.9348729704079935532, -2.191421614605370878E-15, 0.4445507791589071167 ) ) ;
#79534=CARTESIAN_POINT ( 'NONE',  ( -0.4133858267716528645, 0.1660481256975883668, -0.3530559997133364547 ) ) ;
#79538=CARTESIAN_POINT ( 'NONE',  ( -1.437007874015747477, 0.07958543189024071263, -0.2665933059059888421 ) ) ;
#79539=CARTESIAN_POINT ( 'NONE',  ( 0.9186351706036751663, -0.6046776061558807314, 0.2411417322834647770 ) ) ;
#79540=CARTESIAN_POINT ( 'NONE',  ( 0.7414698162729663755, 0.2952755905511811885, 0.1292274648535926551 ) ) ;
#79541=CARTESIAN_POINT ( 'NONE',  ( -0.1968503937007867743, 0.1771653543307087630, 0.000000000000000000 ) ) ;
#79542=CARTESIAN_POINT ( 'NONE',  ( 0.1181102362204730916, -0.6692913385826771977, 8.415575281601705876E-17 ) ) ;
#79544=CARTESIAN_POINT ( 'NONE',  ( 0.006561679790026889343, -0.2845877964562161244, -0.3641732283464567121 ) ) ;
#79545=CARTESIAN_POINT ( 'NONE',  ( -0.5380577427821514602, -0.4281496062992127816, -0.4176697321401328100 ) ) ;
#79547=CARTESIAN_POINT ( 'NONE',  ( -1.555118110236219930, 0.1660481256975885056, 0.3530559997133364547 ) ) ;
#79548=CARTESIAN_POINT ( 'NONE',  ( 0.01312335958005323398, -0.004921259842519576551, 0.3153832671262227771 ) ) ;
#79549=CARTESIAN_POINT ( 'NONE',  ( 0.9548908091195654757, -4.927456884911482678E-16, 0.4445507791589062840 ) ) ;
#79550=CARTESIAN_POINT ( 'NONE',  ( -1.161417322834644716, -0.5400638737290845981, -0.3530559997133363437 ) ) ;
#79551=CARTESIAN_POINT ( 'NONE',  ( -0.7480314960629914633, -0.5511811023622047445, 6.969142054262312111E-17 ) ) ;
#79553=CARTESIAN_POINT ( 'NONE',  ( -1.010498687664041384, -0.4281496062992127816, -0.4176697321401328100 ) ) ;
#79554=CARTESIAN_POINT ( 'NONE',  ( -0.6167979002624665030, -0.4281496062992127816, -0.4176697321401328100 ) ) ;
#79555=CARTESIAN_POINT ( 'NONE',  ( 0.1246719160104994284, 0.2952755905511810774, -0.1292274648535930714 ) ) ;
#79559=CARTESIAN_POINT ( 'NONE',  ( 0.3608923884514443348, -0.5511811023622046335, 0.09757992244046803654 ) ) ;
#79560=CARTESIAN_POINT ( 'NONE',  ( 1.174540682414699111, -0.05778040916215560624, -0.4822834645669293319 ) ) ;
#79561=CARTESIAN_POINT ( 'NONE',  ( -1.377952755905511140, 0.1771653543307087630, 0.000000000000000000 ) ) ;
#79562=CARTESIAN_POINT ( 'NONE',  ( 1.338582677165355062, -0.1870078740157479769, 0.4822834645669291653 ) ) ;
#79563=CARTESIAN_POINT ( 'NONE',  ( -1.541994750656167090, 0.1771653543307087630, 0.09757992244046791164 ) ) ;
#79564=CARTESIAN_POINT ( 'NONE',  ( -0.3937007874015740483, -0.1870078740157480879, -0.4822834645669291653 ) ) ;
#79565=CARTESIAN_POINT ( 'NONE',  ( 0.3280839895013130669, -0.3690944881889765550, -0.3153832671262227771 ) ) ;
#79567=CARTESIAN_POINT ( 'NONE',  ( 0.5643044619422579178, -0.3690944881889765550, -0.3153832671262227771 ) ) ;
#79568=CARTESIAN_POINT ( 'NONE',  ( 0.08530183727034192087, -0.05778040916215522460, 0.4822834645669289988 ) ) ;
#79570=CARTESIAN_POINT ( 'NONE',  ( -0.6561679790026240244, -0.6046776061558807314, 0.2411417322834647770 ) ) ;
#79572=CARTESIAN_POINT ( 'NONE',  ( 1.089238845144357537, -0.3690944881889763329, 0.3153832671262228327 ) ) ;
#79573=CARTESIAN_POINT ( 'NONE',  ( 0.03937007874015833325, -0.6692913385826771977, 8.415575281601705876E-17 ) ) ;
#79574=CARTESIAN_POINT ( 'NONE',  ( -0.2034120734908128059, 0.2952755905511811885, 0.1292274648535926551 ) ) ;
#79575=CARTESIAN_POINT ( 'NONE',  ( -0.3083989501312330295, -0.2845877964562161244, -0.3641732283464567121 ) ) ;
#79576=CARTESIAN_POINT ( 'NONE',  ( 0.9573014326657177664, 0.000000000000000000, 0.3464511005275205946 ) ) ;
#79577=CARTESIAN_POINT ( 'NONE',  ( -0.6036745406824141069, -0.5023911411419708095, -0.1820866141732282451 ) ) ;
#79578=CARTESIAN_POINT ( 'NONE',  ( 0.5511811023622055217, -0.1870078740157479769, 0.4822834645669291653 ) ) ;
#79580=CARTESIAN_POINT ( 'NONE',  ( -0.8333333333333323711, -0.5511811023622048555, -0.09757992244046775898 ) ) ;
#79582=CARTESIAN_POINT ( 'NONE',  ( -0.9317585301837263412, -0.4281496062992127816, -0.4176697321401328100 ) ) ;
#79584=EDGE_LOOP ( 'NONE', ( #2879, #34382, #26589, #67392 ) ) ;
#79585=EDGE_CURVE ( 'NONE', #7120, #34463, #60032, .T. ) ;
#79586=CARTESIAN_POINT ( 'NONE',  ( -1.089238845144356427, -0.004921259842519576551, 0.3153832671262227771 ) ) ;
#79588=CARTESIAN_POINT ( 'NONE',  ( -0.2099737532808391705, -0.6046776061558809534, -0.2411417322834644161 ) ) ;
#79589=CARTESIAN_POINT ( 'NONE',  ( -1.725721784776902190, -0.05778040916215522460, 0.4822834645669289988 ) ) ;
#79590=CARTESIAN_POINT ( 'NONE',  ( -0.7874015748031489847, -0.1870078740157480879, -0.4822834645669291653 ) ) ;
#79592=CARTESIAN_POINT ( 'NONE',  ( 1.364829396325460076, 0.2306618581243848609, 0.2411417322834645549 ) ) ;
#79593=CARTESIAN_POINT ( 'NONE',  ( 0.7939632545931766261, -0.3162353388693409650, -0.4822834645669289433 ) ) ;
#79595=CARTESIAN_POINT ( 'NONE',  ( -1.586052503253847501, 1.299212598425198095, 0.1653254495020568260 ) ) ;
#79597=CARTESIAN_POINT ( 'NONE',  ( -1.646981627296586703, -0.3162353388693409650, -0.4822834645669289433 ) ) ;
#79599=ORIENTED_EDGE ( 'NONE', *, *, #38721, .F. ) ;
#79600=CARTESIAN_POINT ( 'NONE',  ( -0.5839895013123351797, -0.5511811023622046335, 0.09757992244046803654 ) ) ;
#79603=CARTESIAN_POINT ( 'NONE',  ( 0.8398950131233602345, 0.2306618581243847221, -0.2411417322834647770 ) ) ;
#79604=CARTESIAN_POINT ( 'NONE',  ( 0.1706036745406830368, 0.05413385826771666132, 0.4176697321401328100 ) ) ;
#79605=CARTESIAN_POINT ( 'NONE',  ( -0.5577427821522301654, -0.3162353388693405765, 0.4822834645669290543 ) ) ;
#79606=CARTESIAN_POINT ( 'NONE',  ( 1.430446194225722500, -0.4281496062992127816, -0.4176697321401328100 ) ) ;
#79607=CARTESIAN_POINT ( 'NONE',  ( -0.6889763779527552368, 0.07958543189024085140, 0.2665933059059887866 ) ) ;
#79609=CARTESIAN_POINT ( 'NONE',  ( 0.4855643044619430415, -0.4281496062992127816, -0.4176697321401328100 ) ) ;
#79610=CARTESIAN_POINT ( 'NONE',  ( 0.4133858267716541968, -0.4536011799217368745, -0.2665933059059886201 ) ) ;
#79611=CARTESIAN_POINT ( 'NONE',  ( -0.6364829396325453192, -0.05778040916215560624, -0.4822834645669293319 ) ) ;
#79613=CARTESIAN_POINT ( 'NONE',  ( -1.253280839895012377, -0.3162353388693409650, -0.4822834645669289433 ) ) ;
#79615=CARTESIAN_POINT ( 'NONE',  ( -1.646981627296586703, -0.2845877964562161244, -0.3641732283464567121 ) ) ;
#79616=CARTESIAN_POINT ( 'NONE',  ( 1.043307086614173818, 0.1660481256975885056, 0.3530559997133364547 ) ) ;
#79617=CARTESIAN_POINT ( 'NONE',  ( 1.102362204724410155, -0.1870078740157480601, -0.3641732283464567677 ) ) ;
#79618=ORIENTED_EDGE ( 'NONE', *, *, #48636, .F. ) ;
#79620=CARTESIAN_POINT ( 'NONE',  ( -0.5380577427821514602, 0.05413385826771666132, 0.4176697321401328100 ) ) ;
#79622=CARTESIAN_POINT ( 'NONE',  ( 0.2952755905511816326, -0.4536011799217367080, 0.2665933059059888421 ) ) ;
#79623=CARTESIAN_POINT ( 'NONE',  ( -1.036745406824146176, 0.05413385826771626580, -0.4176697321401330321 ) ) ;
#79624=CARTESIAN_POINT ( 'NONE',  ( 1.076115485564305141, -0.6046776061558807314, 0.2411417322834647770 ) ) ;
#79625=CARTESIAN_POINT ( 'NONE',  ( 1.030183727034121421, -0.3162353388693409650, -0.4822834645669289433 ) ) ;
#79626=CARTESIAN_POINT ( 'NONE',  ( -0.04593175853018302557, -0.6692913385826773087, -0.1292274648535924053 ) ) ;
#79627=CARTESIAN_POINT ( 'NONE',  ( -0.4396325459317577122, -0.6692913385826773087, -0.1292274648535924053 ) ) ;
#79629=CARTESIAN_POINT ( 'NONE',  ( 1.614173228346457378, 0.1771653543307087630, 0.000000000000000000 ) ) ;
#79630=CARTESIAN_POINT ( 'NONE',  ( -0.4133858267716528645, -0.5400638737290844871, 0.3530559997133364547 ) ) ;
#79631=CARTESIAN_POINT ( 'NONE',  ( -0.4593175853018364174, -0.3690944881889765550, -0.3153832671262227771 ) ) ;
#79632=CARTESIAN_POINT ( 'NONE',  ( 1.515748031496063408, 0.1660481256975885056, 0.3530559997133364547 ) ) ;
#79633=CARTESIAN_POINT ( 'NONE',  ( 1.489501312335958172, -0.3162353388693405765, 0.4822834645669290543 ) ) ;
#79634=CARTESIAN_POINT ( 'NONE',  ( -0.8792650918635160906, 0.05413385826771626580, -0.4176697321401330321 ) ) ;
#79636=CARTESIAN_POINT ( 'NONE',  ( 0.5380577427821529035, 0.05413385826771626580, -0.4176697321401330321 ) ) ;
#79639=CARTESIAN_POINT ( 'NONE',  ( -0.2493438320209966919, -0.4281496062992124485, 0.4176697321401328655 ) ) ;
#79640=CARTESIAN_POINT ( 'NONE',  ( -1.351706036745406347, -0.3690944881889763329, 0.3153832671262228327 ) ) ;
#79641=CARTESIAN_POINT ( 'NONE',  ( 1.030183727034121421, -0.08942795157527998196, 0.3641732283464567121 ) ) ;
#79644=CARTESIAN_POINT ( 'NONE',  ( 1.181102362204725198, -0.1870078740157479769, 0.3641732283464567677 ) ) ;
#79645=CARTESIAN_POINT ( 'NONE',  ( 0.6955380577427828781, 0.05413385826771626580, -0.4176697321401330321 ) ) ;
#79647=CARTESIAN_POINT ( 'NONE',  ( -0.2821522309711278487, 0.2952755905511811885, 0.1292274648535926551 ) ) ;
#79649=CARTESIAN_POINT ( 'NONE',  ( 1.187664041994751285, -0.2845877964562161244, -0.3641732283464567121 ) ) ;
#79650=CARTESIAN_POINT ( 'NONE',  ( -0.7283464566929126471, 0.1660481256975883668, -0.3530559997133364547 ) ) ;
#79652=CARTESIAN_POINT ( 'NONE',  ( 1.154855643044620184, -0.6046776061558807314, 0.2411417322834647770 ) ) ;
#79653=CARTESIAN_POINT ( 'NONE',  ( 0.1115485564304467270, -0.6692913385826773087, -0.1292274648535924053 ) ) ;
#79655=CARTESIAN_POINT ( 'NONE',  ( 0.6102362204724416372, 0.07958543189024071263, -0.2665933059059888421 ) ) ;
#79657=CARTESIAN_POINT ( 'NONE',  ( 0.3674540682414705883, -0.5023911411419708095, 0.1820866141732285504 ) ) ;
#79660=CARTESIAN_POINT ( 'NONE',  ( 0.7742782152230979209, 0.05413385826771626580, -0.4176697321401330321 ) ) ;
#79662=CARTESIAN_POINT ( 'NONE',  ( 1.679790026246720025, 0.1283753931104748280, 0.1820866141732283561 ) ) ;
#79664=CARTESIAN_POINT ( 'NONE',  ( -0.09842519685039295696, 0.07958543189024071263, -0.2665933059059888421 ) ) ;
#79665=CARTESIAN_POINT ( 'NONE',  ( 0.1640419947506569498, -0.3162353388693409650, -0.4822834645669289433 ) ) ;
#79666=CARTESIAN_POINT ( 'NONE',  ( 1.607611548556431069, -0.5511811023622048555, -0.09757992244046775898 ) ) ;
#79667=CARTESIAN_POINT ( 'NONE',  ( -1.338582677165353729, -0.1870078740157480601, -0.3641732283464567677 ) ) ;
#79668=CARTESIAN_POINT ( 'NONE',  ( -1.482939632545930975, -0.4281496062992127816, -0.4176697321401328100 ) ) ;
#79669=CARTESIAN_POINT ( 'NONE',  ( 0.7152230971128616943, -0.05778040916215522460, 0.4822834645669289988 ) ) ;
#79670=CARTESIAN_POINT ( 'NONE',  ( 1.384514435695538559, 0.2952755905511810774, -0.1292274648535930714 ) ) ;
#79673=CARTESIAN_POINT ( 'NONE',  ( 0.3674540682414705883, 0.2306618581243847221, -0.2411417322834647770 ) ) ;
#79674=CARTESIAN_POINT ( 'NONE',  ( 1.279527559055118724, -0.5400638737290845981, -0.3530559997133363437 ) ) ;
#79675=CARTESIAN_POINT ( 'NONE',  ( 0.8661417322834653598, -0.1870078740157479769, 0.4822834645669291653 ) ) ;
#79676=CARTESIAN_POINT ( 'NONE',  ( -1.332020997375327642, -0.2845877964562161244, -0.3641732283464567121 ) ) ;
#79677=CARTESIAN_POINT ( 'NONE',  ( 1.128608923884515169, -0.5023911411419708095, -0.1820866141732282451 ) ) ;
#79678=CARTESIAN_POINT ( 'NONE',  ( 1.686351706036745890, 0.2952755905511811885, 0.1292274648535926551 ) ) ;
#79679=CARTESIAN_POINT ( 'NONE',  ( -0.7414698162729651543, -0.5511811023622046335, 0.09757992244046803654 ) ) ;
#79680=EDGE_CURVE ( 'NONE', #33309, #43739, #34366, .T. ) ;
#79682=CARTESIAN_POINT ( 'NONE',  ( 0.6889763779527563470, 0.07958543189024071263, -0.2665933059059888421 ) ) ;
#79683=CARTESIAN_POINT ( 'NONE',  ( 0.09186351706036827158, 0.05413385826771666132, 0.4176697321401328100 ) ) ;
#79684=CARTESIAN_POINT ( 'NONE',  ( 0.8464566929133865436, 0.1660481256975883668, -0.3530559997133364547 ) ) ;
#79685=CARTESIAN_POINT ( 'NONE',  ( -0.4265091863517051496, -0.6692913385826771977, 0.1292274648535927661 ) ) ;
#79686=CARTESIAN_POINT ( 'NONE',  ( 0.1574803149606306130, -0.1870078740157479769, 0.3641732283464567677 ) ) ;
#79687=CARTESIAN_POINT ( 'NONE',  ( 1.325459317585302665, 0.05413385826771626580, -0.4176697321401330321 ) ) ;
#79689=CARTESIAN_POINT ( 'NONE',  ( -0.8923884514435688198, 0.2306618581243847221, -0.2411417322834647770 ) ) ;
#79693=CARTESIAN_POINT ( 'NONE',  ( -0.7086614173228339419, -0.1870078740157479769, 0.4822834645669291653 ) ) ;
#79694=CARTESIAN_POINT ( 'NONE',  ( -0.5708661417322828946, 0.1660481256975883668, -0.3530559997133364547 ) ) ;
#79697=ORIENTED_EDGE ( 'NONE', *, *, #46085, .T. ) ;
#79698=CARTESIAN_POINT ( 'NONE',  ( 0.8202099737532814183, -0.5511811023622048555, -0.09757992244046775898 ) ) ;
#79701=CARTESIAN_POINT ( 'NONE',  ( 1.036745406824147508, -0.4281496062992127816, -0.4176697321401328100 ) ) ;
#79703=CARTESIAN_POINT ( 'NONE',  ( -1.528871391076114250, 0.1771653543307087075, -0.09757992244046823083 ) ) ;
#79704=CARTESIAN_POINT ( 'NONE',  ( 1.469816272965879911, -0.6046776061558807314, 0.2411417322834647770 ) ) ;
#79705=CARTESIAN_POINT ( 'NONE',  ( -1.653543307086613234, -0.1870078740157480879, -0.4822834645669291653 ) ) ;
#79707=CARTESIAN_POINT ( 'NONE',  ( -0.09186351706036663400, -0.4281496062992124485, 0.4176697321401328655 ) ) ;
#79708=CARTESIAN_POINT ( 'NONE',  ( -0.3215223097112853146, -0.2845877964562159024, 0.3641732283464567677 ) ) ;
#79709=CARTESIAN_POINT ( 'NONE',  ( 1.010498687664042716, 0.05413385826771626580, -0.4176697321401330321 ) ) ;
#79710=CARTESIAN_POINT ( 'NONE',  ( 0.1312335958005255154, -0.6046776061558807314, 0.2411417322834647770 ) ) ;
#79712=CARTESIAN_POINT ( 'NONE',  ( -1.614173228346457378, 0.5038684218300931716, 0.1372047244094476981 ) ) ;
#79714=CARTESIAN_POINT ( 'NONE',  ( 0.8661417322834653598, -0.1870078740157479769, 0.4822834645669291653 ) ) ;
#79715=CARTESIAN_POINT ( 'NONE',  ( 0.1049868766404206816, -0.6046776061558809534, -0.2411417322834644161 ) ) ;
#79716=CARTESIAN_POINT ( 'NONE',  ( -1.017060367454067249, -0.05778040916215522460, 0.4822834645669289988 ) ) ;
#79717=CARTESIAN_POINT ( 'NONE',  ( 0.8923884514435701520, -0.6046776061558809534, -0.2411417322834644161 ) ) ;
#79718=CARTESIAN_POINT ( 'NONE',  ( 1.056430446194226658, 0.2952755905511811885, 0.1292274648535926551 ) ) ;
#79720=CARTESIAN_POINT ( 'NONE',  ( -0.2690288713910754526, 0.2952755905511810774, -0.1292274648535930714 ) ) ;
#79721=CARTESIAN_POINT ( 'NONE',  ( 0.7611548556430454138, 0.2306618581243847221, -0.2411417322834647770 ) ) ;
#79722=CARTESIAN_POINT ( 'NONE',  ( 0.07217847769028949700, -0.3162353388693405765, 0.4822834645669290543 ) ) ;
#79723=CARTESIAN_POINT ( 'NONE',  ( 0.5183727034120741983, -0.5511811023622046335, 0.09757992244046803654 ) ) ;
#79724=CARTESIAN_POINT ( 'NONE',  ( -1.194225721784776262, 0.05413385826771626580, -0.4176697321401330321 ) ) ;
#79726=CARTESIAN_POINT ( 'NONE',  ( 0.3937007874015754361, -0.1870078740157480879, -0.4822834645669291653 ) ) ;
#79731=CARTESIAN_POINT ( 'NONE',  ( 1.076115485564305141, 0.2306618581243847221, -0.2411417322834647770 ) ) ;
#79732=CARTESIAN_POINT ( 'NONE',  ( 0.5774278215223103139, -0.5023911411419708095, -0.1820866141732282451 ) ) ;
#79734=CARTESIAN_POINT ( 'NONE',  ( -0.7426113562972000981, 2.793565526369265584, -0.5309055118110234117 ) ) ;
#79738=CARTESIAN_POINT ( 'NONE',  ( -0.8464566929133852113, 0.1660481256975885056, 0.3530559997133364547 ) ) ;
#79740=CARTESIAN_POINT ( 'NONE',  ( -0.8333333333333323711, -0.6692913385826773087, -0.1292274648535924053 ) ) ;
#79741=CARTESIAN_POINT ( 'NONE',  ( 1.148293963254593653, 0.2952755905511810774, -0.1292274648535930714 ) ) ;
#79743=CARTESIAN_POINT ( 'NONE',  ( 1.601049868766404982, 0.2306618581243848609, 0.2411417322834645549 ) ) ;
#79748=CARTESIAN_POINT ( 'NONE',  ( -1.345144356955379816, -0.2845877964562159024, 0.3641732283464567677 ) ) ;
#79750=CARTESIAN_POINT ( 'NONE',  ( 0.3149606299212606708, -0.1870078740157480879, -0.4822834645669291653 ) ) ;
#79751=CARTESIAN_POINT ( 'NONE',  ( 1.692913385826772421, 0.2952755905511811885, 0.000000000000000000 ) ) ;
#79753=CARTESIAN_POINT ( 'NONE',  ( -0.6955380577427815458, -0.3690944881889765550, -0.3153832671262227771 ) ) ;
#79754=CARTESIAN_POINT ( 'NONE',  ( 0.8989501312335964611, 0.2952755905511811885, 0.1292274648535926551 ) ) ;
#79755=CARTESIAN_POINT ( 'NONE',  ( 1.377952755905512472, -0.5511811023622047445, 6.969142054262312111E-17 ) ) ;
#79758=CARTESIAN_POINT ( 'NONE',  ( -0.7414698162729651543, 0.1771653543307087075, -0.09757992244046823083 ) ) ;
#79759=CARTESIAN_POINT ( 'NONE',  ( 1.167979002624672580, -0.4281496062992124485, 0.4176697321401328655 ) ) ;
#79761=CARTESIAN_POINT ( 'NONE',  ( -0.3083989501312330295, -0.05778040916215522460, 0.4822834645669289988 ) ) ;
#79762=CARTESIAN_POINT ( 'NONE',  ( -0.9251968503937002541, -0.4536011799217368745, -0.2665933059059886201 ) ) ;
#79763=CARTESIAN_POINT ( 'NONE',  ( -0.3543307086614165824, -0.5511811023622047445, 6.969142054262312111E-17 ) ) ;
#79764=CARTESIAN_POINT ( 'NONE',  ( -0.4133858267716528645, 0.1660481256975883668, -0.3530559997133364547 ) ) ;
#79765=CARTESIAN_POINT ( 'NONE',  ( 1.679790026246720025, 0.2306618581243848609, 0.2411417322834645549 ) ) ;
#79767=CARTESIAN_POINT ( 'NONE',  ( 0.4330708661417329575, -0.6692913385826771977, 8.415575281601705876E-17 ) ) ;
#79771=CARTESIAN_POINT ( 'NONE',  ( -0.8005249343832013809, -0.4281496062992124485, 0.4176697321401328655 ) ) ;
#79772=CARTESIAN_POINT ( 'NONE',  ( -0.1181102362204717315, 0.1771653543307087630, 0.000000000000000000 ) ) ;
#79773=CARTESIAN_POINT ( 'NONE',  ( -1.148293963254592542, 0.2952755905511811885, 0.1292274648535926551 ) ) ;
#79774=CARTESIAN_POINT ( 'NONE',  ( -0.1115485564304453947, -0.6692913385826771977, 0.1292274648535927661 ) ) ;
#79775=CARTESIAN_POINT ( 'NONE',  ( 0.5314960629921267055, -0.4536011799217367080, 0.2665933059059888421 ) ) ;
#79776=CARTESIAN_POINT ( 'NONE',  ( -0.8005249343832013809, -0.3690944881889763329, 0.3153832671262228327 ) ) ;
#79777=CARTESIAN_POINT ( 'NONE',  ( -0.9186351706036736120, 0.2306618581243848609, 0.2411417322834645549 ) ) ;
#79778=CARTESIAN_POINT ( 'NONE',  ( -1.489501312335957062, -0.3162353388693409650, -0.4822834645669289433 ) ) ;
#79780=CARTESIAN_POINT ( 'NONE',  ( 1.181102362204725198, -0.1870078740157479769, 0.4822834645669291653 ) ) ;
#79782=CARTESIAN_POINT ( 'NONE',  ( 0.7217847769028878924, -0.004921259842519576551, 0.3153832671262227771 ) ) ;
#79783=CARTESIAN_POINT ( 'NONE',  ( 0.9776902887139113929, -0.6692913385826773087, -0.1292274648535924053 ) ) ;
#79785=CARTESIAN_POINT ( 'NONE',  ( 1.358267716535433323, -0.4536011799217368745, -0.2665933059059886201 ) ) ;
#79787=CARTESIAN_POINT ( 'NONE',  ( -0.8005249343832011588, 0.05413385826771626580, -0.4176697321401330321 ) ) ;
#79789=CARTESIAN_POINT ( 'NONE',  ( -1.305774278215222184, 0.1771653543307087630, 0.09757992244046791164 ) ) ;
#79790=CARTESIAN_POINT ( 'NONE',  ( -0.5249343832020990641, 0.2306618581243848609, 0.2411417322834645549 ) ) ;
#79791=CARTESIAN_POINT ( 'NONE',  ( 0.4724409448818904789, -0.1870078740157479769, 0.4822834645669291653 ) ) ;
#79792=CARTESIAN_POINT ( 'NONE',  ( -1.568241469816272105, -0.08942795157527998196, 0.3641732283464567121 ) ) ;
#79794=CARTESIAN_POINT ( 'NONE',  ( -1.541994750656167090, 0.2952755905511811885, 0.1292274648535926551 ) ) ;
#79795=CARTESIAN_POINT ( 'NONE',  ( 0.3805774278215230400, -0.4281496062992124485, 0.4176697321401328655 ) ) ;
#79796=CARTESIAN_POINT ( 'NONE',  ( 0.1115485564304470323, 0.2952755905511811885, 0.1292274648535926551 ) ) ;
#79797=CARTESIAN_POINT ( 'NONE',  ( 0.9908136482939640111, 0.2952755905511810774, -0.1292274648535930714 ) ) ;
#79798=CARTESIAN_POINT ( 'NONE',  ( 1.673228346456693494, 0.1660481256975885056, 0.3530559997133364547 ) ) ;
#79804=CARTESIAN_POINT ( 'NONE',  ( 0.01968503937007930540, 0.07958543189024085140, 0.2665933059059887866 ) ) ;
#79805=CARTESIAN_POINT ( 'NONE',  ( -0.2230971128608915943, -0.4281496062992127816, -0.4176697321401328100 ) ) ;
#79806=CARTESIAN_POINT ( 'NONE',  ( 0.8661417322834652488, -0.1870078740157480879, -0.4822834645669291653 ) ) ;
#79808=CARTESIAN_POINT ( 'NONE',  ( 0.05905511811023709395, -0.4536011799217367080, 0.2665933059059888421 ) ) ;
#79809=CARTESIAN_POINT ( 'NONE',  ( -1.076115485564303809, -0.6046776061558809534, -0.2411417322834644161 ) ) ;
#79810=CARTESIAN_POINT ( 'NONE',  ( -1.535433070866141225, -0.6692913385826771977, 8.415575281601705876E-17 ) ) ;
#79815=CARTESIAN_POINT ( 'NONE',  ( 0.9055118110236227702, -0.6692913385826771977, 8.415575281601705876E-17 ) ) ;
#79817=CARTESIAN_POINT ( 'NONE',  ( 1.601049868766404982, 0.1283753931104748280, 0.1820866141732283561 ) ) ;
#79818=CARTESIAN_POINT ( 'NONE',  ( -1.410761154855641575, -0.2845877964562161244, -0.3641732283464567121 ) ) ;
#79819=CARTESIAN_POINT ( 'NONE',  ( -1.200787401574802349, -0.5400638737290844871, 0.3530559997133364547 ) ) ;
#79821=DIRECTION ( 'NONE',  ( 0.000000000000000000, 8.673617379884035472E-16, -1.000000000000000000 ) ) ;
#79822=CARTESIAN_POINT ( 'NONE',  ( 1.305774278215223960, -0.6692913385826771977, 0.1292274648535927661 ) ) ;
#79823=CARTESIAN_POINT ( 'NONE',  ( -1.568241469816272105, -0.05778040916215522460, 0.4822834645669289988 ) ) ;
#79824=CARTESIAN_POINT ( 'NONE',  ( -0.1706036745406816491, -0.4281496062992124485, 0.4176697321401328655 ) ) ;
#79825=CARTESIAN_POINT ( 'NONE',  ( 0.03280839895013198948, 0.2952755905511811885, 0.1292274648535926551 ) ) ;
#79826=CARTESIAN_POINT ( 'NONE',  ( -1.102362204724408601, -0.1870078740157480879, -0.4822834645669291653 ) ) ;
#79828=CARTESIAN_POINT ( 'NONE',  ( 0.1902887139107617975, 0.2952755905511811885, 0.1292274648535926551 ) ) ;
#79830=CARTESIAN_POINT ( 'NONE',  ( -1.345144356955379816, -0.2845877964562159024, 0.3641732283464567677 ) ) ;
#79831=VERTEX_POINT ( 'NONE', #9525 ) ;
#79833=VERTEX_POINT ( 'NONE', #29292 ) ;
#79835=CARTESIAN_POINT ( 'NONE',  ( -1.561679790026246017, 0.05413385826771666132, 0.4176697321401328100 ) ) ;
#79837=CARTESIAN_POINT ( 'NONE',  ( -1.581364829396324945, -0.3162353388693405765, 0.4822834645669290543 ) ) ;
#79839=CARTESIAN_POINT ( 'NONE',  ( -1.003937007874014853, 0.1660481256975885056, 0.3530559997133364547 ) ) ;
#79840=CARTESIAN_POINT ( 'NONE',  ( 0.9345427628023850186, -1.711642917916620527E-15, -0.4281989832122460871 ) ) ;
#79842=CARTESIAN_POINT ( 'NONE',  ( -0.1574803149606292529, -0.1870078740157480601, -0.3641732283464567677 ) ) ;
#79843=EDGE_CURVE ( 'NONE', #12831, #19838, #33946, .T. ) ;
#79844=CARTESIAN_POINT ( 'NONE',  ( -0.8595800524934373854, -0.2845877964562161244, -0.3641732283464567121 ) ) ;
#79845=CARTESIAN_POINT ( 'NONE',  ( -1.161417322834644716, 0.1660481256975885056, 0.3530559997133364547 ) ) ;
#79846=CARTESIAN_POINT ( 'NONE',  ( 0.4921259842519691285, 0.1660481256975885056, 0.3530559997133364547 ) ) ;
#79847=CARTESIAN_POINT ( 'NONE',  ( -0.7742782152230962556, -0.4281496062992127816, -0.4176697321401328100 ) ) ;
#79849=VERTEX_POINT ( 'NONE', #80662 ) ;
#79850=CARTESIAN_POINT ( 'NONE',  ( -1.456692913385826182, 0.2952755905511811885, 0.000000000000000000 ) ) ;
#79854=( BOUNDED_SURFACE ( )  B_SPLINE_SURFACE ( 1, 2, ( 
 ( #32651, #83174, #31820, #30988, #12891, #32236, #13309, #38550, #26336, #82760, #76455, #70120, #57894, #56656, #38133, #5730, #24675, #25494, #77702, #69719, #63807, #45683, #20032, #261, #18782, #76856, #44426, #44837, #64230, #25914, #77276, #45268, #54082, #78121, #34752, #34331, #27173, #7832, #78547, #33499, #73046, #46940, #15823, #14980, #15395, #65909, #60412, #41472, #53668, #1931, #79375, #58744, #66321, #2763, #28008, #40639, #41057, #1106, #65500, #72632, #78966, #33911, #72225, #47357, #26757, #52412, #8660, #59575, #20872, #22113, #20454, #46107, #71800, #21286, #59161, #66745, #59996, #53254, #14575, #14153, #7407, #2352, #1519, #39810, #47773, #46525, #73474, #52835, #21694, #40227, #8246, #27594, #9081, #28422, #33077, #79797, #17880, #75540, #3172, #4816, #55327, #67157, #49019, #68801, #28836, #36805, #68399, #30076, #4001, #9486, #10738, #23348, #24172, #62481, #16645, #35161, #42702, #49841, #60821, #80213, #9900, #54500, #42285, #10328, #17065, #4408, #43105, #22528, #48190, #73887, #35572, #16227, #67983, #35990, #36395, #55739, #11146, #41874, #75129, #61660, #29665, #67568, #74716, #62069, #23764, #81447, #30494, #61235, #3590, #22937, #49435, #29255, #48603, #54919, #80625, #81036, #17474, #74299, #56157, #81860, #45165, #70439, #64547, #38038, #43514, #26238, #51065, #82266, #19095, #24985, #6884, #30898, #70871, #12796, #63303, #43933, #31308, #69627, #25817, #83080, #51899, #76765, #51477, #18693, #13220, #77606, #6470, #63713, #32140, #11563, #44744, #38866, #64138, #38452, #77180, #37222, #18288, #25401, #31725, #70027, #50661, #164, #62899, #5234, #57797, #12380, #56972, #58217, #56565, #24584, #50251, #57388, #11972, #19511, #32554, #6053, #76361, #75947, #69214, #583, #37627, #5641, #82670, #44336, #34649, #58642, #65815, #65400, #46004, #20352, #40543, #1010, #19939, #66223, #53982, #28321, #39282, #40957, #8148, #45588, #1831, #21593, #64969, #72944, #21187, #8561, #40129, #71281, #46841, #59478, #60313, #15296, #52735, #13630, #78861, #66638, #39709, #72535, #20772, #7737, #14476, #33403, #33813, #47255, #8975, #26663, #14883, #7305, #52317, #59065, #27492, #53149, #34229, #59892, #32975, #2244, #71700, #27910, #2662, #78024, #14054, #1420, #27076, #53569, #78446, #46426, #72117, #79278, #73787, #48494, #43002, #4708, #36290, #49325, #10219, #48913, #61132, #74195, #17372, #54397, #54819, #68695, #60721, #68299, #29966, #74613, #16958, #61963, #10635, #67881, #55221, #11037, #47671, #16541, #42186, #35468, #3484, #35886, #30382, #61556, #3899, #36695, #62370, #29558, #42597, #35055, #80928, #23243, #4303, #55631, #73366, #81340, #23655, #79694, #75027, #22011, #15714, #41371, #41769, #67052, #9385, #3070, #16123, #28737, #80110, #22428, #48086, #67462, #9796, #29150, #80520, #22835, #57696, #50961, #82163, #76658, #58, #69521, #31203, #43817, #11871, #6365, #12277, #37934, #75435, #17775, #43408, #82564, #32037, #64025, #18991, #56869, #76255, #37113, #63611, #25712, #6778, #69107, #11455, #62796, #75842, #24479, #51372, #37523, #70763, #5131, #18590, #18184, #50145, #56461, #44639, #30795, #56048, #70335, #81757, #64442, #63197, #77075, #44232, #24067, #5948, #19409, #5538, #45060, #57279, #12691, #69922, #49736, #82976, #31617, #13112, #38765, #24883, #50552, #25295, #38350, #26133, #45484, #58541, #77500, #7635, #58967, #65720, #53051, #8461, #13523, #40444, #1324, #33306, #32450, #14376, #8052, #72438, #40033, #27813, #908, #26564, #71598, #33714, #40856, #13950, #64863, #58112, #26973, #66124, #66540, #39608, #47157, #34130, #59376, #53473, #52638, #478, #15197, #1734, #71181, #27390, #65296, #79183, #19835, #59791, #78763, #52218, #32873, #20252, #77921, #14788, #72020, #51795, #21087, #2146, #78343, #21498, #39179, #46746, #20674, #72848, #7202, #45901, #46327, #29465, #42090, #16861, #60215, #66960, #48399, #80429, #35374, #73691, #48815, #28224, #2565, #10123, #61039, #22331, #23557, #53882, #79597, #21912, #22739, #60626, #42499, #74099, #54724, #16031, #47574, #42904, #16445, #2976, #73268, #49227 ),
 ( #3803, #74514, #80832, #67785, #35787, #29870, #15617, #3389, #29053, #47992, #41677, #61455, #17276, #55123, #23146, #74931, #81241, #68200, #10538, #41274, #36195, #61865, #4206, #55532, #9293, #8873, #34549, #34963, #28642, #54300, #80013, #67370, #9704, #44140, #76160, #55949, #62697, #31523, #75332, #6263, #69832, #17679, #11358, #82067, #12591, #24380, #70236, #63517, #37016, #5847, #38249, #50052, #43722, #56368, #75746, #18896, #24787, #50456, #4611, #30283, #81661, #11779, #44545, #76568, #57180, #69426, #5444, #49639, #18497, #63927, #19308, #23972, #43309, #69007, #5036, #30704, #31939, #57600, #18087, #12181, #37432, #63105, #31105, #56772, #82472, #83290, #25613, #37839, #82882, #10939, #25202, #50868, #51276, #76978, #68599, #36596, #62274, #33203, #13426, #26875, #2044, #70656, #27709, #59689, #39082, #78243, #53375, #79083, #52115, #64345, #64763, #13848, #8361, #44960, #6681, #32353, #58014, #7102, #71083, #72339, #66024, #32772, #46226, #45803, #58439, #39506, #801, #65194, #46646, #34028, #51694, #20575, #13013, #77397, #26464, #58868, #1226, #7530, #52535, #38667, #71922, #77823, #14272, #379, #26034, #19731, #45386, #20153, #39933, #71500, #65620, #7951, #33613, #59276, #1632, #27291, #52949, #78663, #14687, #20984, #40344, #2875, #73590, #42397, #79492, #79911, #10441, #2466, #10018, #55026, #16345, #41988, #61349, #35684, #9603, #80327, #68095, #72747, #15933, #41580, #60526, #28538, #60936, #29774, #3286, #28951, #61768, #36097, #67270, #67682, #60115, #35271, #54616, #22641, #80734, #15095, #48301, #3703, #55435, #74413, #4108, #21400, #40752, #66862, #73998, #29366, #8772, #15513, #23048, #28124, #47055, #48715, #53779, #47471, #34864, #16757, #54195, #66436, #34446, #73163, #21807, #41171, #22228, #47883, #9192, #36918, #31419, #37336, #63008, #17175, #42808, #68502, #24281, #58228, #5748, #18402, #56270, #17990, #62178, #5347, #595, #10842, #19950, #69329, #7317, #31006, #26251, #36502, #51910, #82374, #44045, #43625, #81144, #24693, #56674, #39295, #77617, #30605, #32986, #50361, #64981, #74830, #4516, #23875, #30185, #81966, #49952, #76059, #69737, #45600, #55848, #71294, #75650, #11678, #23459, #12081, #37739, #63413, #13642, #49125, #49541, #75236, #62595, #81556, #17579, #4937, #43212, #68908, #11260, #8990, #67066, #40140, #73379, #60326, #2256, #79708, #53161, #58654, #41385, #66234, #14065, #34242, #65825, #22024, #46017, #2675, #27921, #78457, #59075, #46437, #1430, #40971, #14893, #9398, #8572, #66653, #33823, #28334, #1021, #21607, #78872, #47267, #26674, #59904, #53996, #79289, #53580, #34663, #52329, #33413, #40553, #46851, #1843, #8158, #15308, #78035, #20365, #72957, #27504, #72128, #15729, #71711, #39719, #65410, #72546, #27086, #47684, #7748, #21197, #59489, #52749, #20782, #14486, #29165, #80124, #75452, #22851, #49752, #73802, #80944, #80539, #61147, #35483, #55646, #16138, #35069, #81357, #69122, #43425, #23259, #74629, #60735, #48929, #3499, #16973, #17790, #3087, #28751, #54413, #54834, #68313, #22443, #48104, #42201, #41784, #48511, #3914, #81772, #67477, #75041, #4723, #42613, #4318, #16557, #29575, #56063, #9811, #10235, #24082, #74211, #23669, #68712, #29983, #49341, #17387, #43018, #10650, #36305, #67897, #35902, #55238, #61981, #61571, #11053, #36711, #62386, #30398, #19007, #51813, #497, #63627, #32053, #50162, #82992, #44656, #25313, #45078, #62812, #12707, #51389, #45502, #64460, #32468, #77518, #5146, #56887, #70352, #38366, #82179, #5555, #57713, #18200, #58130, #64042, #43835, #37539, #24899, #38783, #50568, #13132, #6381, #63215, #76, #6797, #76272, #69938, #82580, #18606, #70781, #50977, #76675, #30811, #56476, #24496, #37950, #26152, #19426, #25729, #12294, #31634, #75858, #77094, #19853, #11471, #69537, #11887, #31219, #44249, #5964, #37128, #57294, #7654, #72456, #72037, #58986, #65737, #33324, #8070, #72866, #34567, #77939, #46763, #13542, #20269, #1341, #59393, #1751, #79615, #7220, #8890, #27408, #21931, #53069, #15215, #32891, #40875, #14805, #34148, #33732, #71199, #40463 ) ),
 .UNSPECIFIED., .F., .F., .F. ) 
 B_SPLINE_SURFACE_WITH_KNOTS ( ( 2, 2 ),
 ( 3, 2, 2, 2, 2, 2, 2, 2, 2, 2, 2, 2, 2, 2, 2, 2, 2, 2, 2, 2, 2, 2, 2, 2, 2, 2, 2, 2, 2, 2, 2, 2, 2, 2, 2, 2, 2, 2, 2, 2, 2, 2, 2, 2, 2, 2, 2, 2, 2, 2, 2, 2, 2, 2, 2, 2, 2, 2, 2, 2, 2, 2, 2, 2, 2, 2, 2, 2, 2, 2, 2, 2, 2, 2, 2, 2, 2, 2, 2, 2, 2, 2, 2, 2, 2, 2, 2, 2, 2, 2, 2, 2, 2, 2, 2, 2, 2, 2, 2, 2, 2, 2, 2, 2, 2, 2, 2, 2, 2, 2, 2, 2, 2, 2, 2, 2, 2, 2, 2, 2, 2, 2, 2, 2, 2, 2, 2, 2, 2, 2, 2, 2, 2, 2, 2, 2, 2, 2, 2, 2, 2, 2, 2, 2, 2, 2, 2, 2, 2, 2, 2, 2, 2, 2, 2, 2, 2, 2, 2, 2, 2, 2, 2, 2, 2, 2, 2, 2, 2, 2, 2, 2, 2, 2, 2, 2, 2, 2, 2, 2, 2, 2, 2, 2, 2, 2, 2, 2, 2, 2, 2, 2, 2, 2, 2, 2, 2, 2, 2, 2, 2, 2, 2, 2, 2, 2, 2, 2, 2, 2, 2, 2, 2, 2, 2, 2, 2, 2, 2, 2, 2, 2, 2, 2, 2, 2, 2, 2, 2, 2, 2, 2, 2, 2, 2, 2, 2, 2, 2, 2, 2, 2, 2, 2, 2, 2, 2, 2, 2, 2, 2, 2, 2, 2, 2, 3 ),
 ( 0.000000000000000000, 1.000000000000000000 ),
 ( 0.000000000000000000, 0.003787878787878787984, 0.007575757575757575968, 0.01136363636363636395, 0.01515151515151515194, 0.01893939393939393992, 0.02272727272727272790, 0.02651515151515151589, 0.03030303030303030387, 0.03409090909090908839, 0.03787878787878787984, 0.04166666666666666435, 0.04545454545454545581, 0.04924242424242424032, 0.05303030303030303177, 0.05681818181818181629, 0.06060606060606060774, 0.06439393939393939226, 0.06818181818181817677, 0.07196969696969697516, 0.07575757575757575968, 0.07954545454545454419, 0.08333333333333332871, 0.08712121212121212710, 0.09090909090909091161, 0.09469696969696969613, 0.09848484848484848064, 0.1022727272727272790, 0.1060606060606060635, 0.1098484848484848481, 0.1136363636363636326, 0.1174242424242424310, 0.1212121212121212155, 0.1250000000000000000, 0.1287878787878787845, 0.1325757575757575690, 0.1363636363636363535, 0.1401515151515151381, 0.1439393939393939503, 0.1477272727272727348, 0.1515151515151515194, 0.1553030303030303039, 0.1590909090909090884, 0.1628787878787878729, 0.1666666666666666574, 0.1704545454545454419, 0.1742424242424242542, 0.1780303030303030387, 0.1818181818181818232, 0.1856060606060606077, 0.1893939393939393923, 0.1931818181818181768, 0.1969696969696969613, 0.2007575757575757458, 0.2045454545454545581, 0.2083333333333333426, 0.2121212121212121271, 0.2159090909090909116, 0.2196969696969696961, 0.2234848484848484806, 0.2272727272727272652, 0.2310606060606060497, 0.2348484848484848619, 0.2386363636363636465, 0.2424242424242424310, 0.2462121212121212155, 0.2500000000000000000, 0.2537878787878787845, 0.2575757575757575690, 0.2613636363636363535, 0.2651515151515151381, 0.2689393939393939226, 0.2727272727272727071, 0.2765151515151514916, 0.2803030303030302761, 0.2840909090909091161, 0.2878787878787879007, 0.2916666666666666852, 0.2954545454545454697, 0.2992424242424242542, 0.3030303030303030387, 0.3068181818181818232, 0.3106060606060606077, 0.3143939393939393923, 0.3181818181818181768, 0.3219696969696969613, 0.3257575757575757458, 0.3295454545454545303, 0.3333333333333333148, 0.3371212121212120993, 0.3409090909090908839, 0.3446969696969697239, 0.3484848484848485084, 0.3522727272727272929, 0.3560606060606060774, 0.3598484848484848619, 0.3636363636363636465, 0.3674242424242424310, 0.3712121212121212155, 0.3750000000000000000, 0.3787878787878787845, 0.3825757575757575690, 0.3863636363636363535, 0.3901515151515151381, 0.3939393939393939226, 0.3977272727272727071, 0.4015151515151514916, 0.4053030303030302761, 0.4090909090909091161, 0.4128787878787879007, 0.4166666666666666852, 0.4204545454545454697, 0.4242424242424242542, 0.4280303030303030387, 0.4318181818181818232, 0.4356060606060606077, 0.4393939393939393923, 0.4431818181818181768, 0.4469696969696969613, 0.4507575757575757458, 0.4545454545454545303, 0.4583333333333333148, 0.4621212121212120993, 0.4659090909090908839, 0.4696969696969697239, 0.4734848484848485084, 0.4772727272727272929, 0.4810606060606060774, 0.4848484848484848619, 0.4886363636363636465, 0.4924242424242424310, 0.4962121212121212155, 0.5000000000000000000, 0.5037878787878787845, 0.5075757575757575690, 0.5113636363636363535, 0.5151515151515151381, 0.5189393939393939226, 0.5227272727272727071, 0.5265151515151514916, 0.5303030303030302761, 0.5340909090909090606, 0.5378787878787878451, 0.5416666666666666297, 0.5454545454545454142, 0.5492424242424241987, 0.5530303030303029832, 0.5568181818181817677, 0.5606060606060605522, 0.5643939393939394478, 0.5681818181818182323, 0.5719696969696970168, 0.5757575757575758013, 0.5795454545454545858, 0.5833333333333333703, 0.5871212121212121549, 0.5909090909090909394, 0.5946969696969697239, 0.5984848484848485084, 0.6022727272727272929, 0.6060606060606060774, 0.6098484848484848619, 0.6136363636363636465, 0.6174242424242424310, 0.6212121212121212155, 0.6250000000000000000, 0.6287878787878787845, 0.6325757575757575690, 0.6363636363636363535, 0.6401515151515151381, 0.6439393939393939226, 0.6477272727272727071, 0.6515151515151514916, 0.6553030303030302761, 0.6590909090909090606, 0.6628787878787878451, 0.6666666666666666297, 0.6704545454545454142, 0.6742424242424241987, 0.6780303030303029832, 0.6818181818181817677, 0.6856060606060605522, 0.6893939393939394478, 0.6931818181818182323, 0.6969696969696970168, 0.7007575757575758013, 0.7045454545454545858, 0.7083333333333333703, 0.7121212121212121549, 0.7159090909090909394, 0.7196969696969697239, 0.7234848484848485084, 0.7272727272727272929, 0.7310606060606060774, 0.7348484848484848619, 0.7386363636363636465, 0.7424242424242424310, 0.7462121212121212155, 0.7500000000000000000, 0.7537878787878787845, 0.7575757575757575690, 0.7613636363636363535, 0.7651515151515151381, 0.7689393939393939226, 0.7727272727272727071, 0.7765151515151514916, 0.7803030303030302761, 0.7840909090909090606, 0.7878787878787878451, 0.7916666666666666297, 0.7954545454545454142, 0.7992424242424241987, 0.8030303030303029832, 0.8068181818181817677, 0.8106060606060605522, 0.8143939393939394478, 0.8181818181818182323, 0.8219696969696970168, 0.8257575757575758013, 0.8295454545454545858, 0.8333333333333333703, 0.8371212121212121549, 0.8409090909090909394, 0.8446969696969697239, 0.8484848484848485084, 0.8522727272727272929, 0.8560606060606060774, 0.8598484848484848619, 0.8636363636363636465, 0.8674242424242424310, 0.8712121212121212155, 0.8750000000000000000, 0.8787878787878787845, 0.8825757575757575690, 0.8863636363636363535, 0.8901515151515151381, 0.8939393939393939226, 0.8977272727272727071, 0.9015151515151514916, 0.9053030303030302761, 0.9090909090909090606, 0.9128787878787878451, 0.9166666666666666297, 0.9204545454545454142, 0.9242424242424241987, 0.9280303030303029832, 0.9318181818181817677, 0.9356060606060605522, 0.9393939393939394478, 0.9431818181818182323, 0.9469696969696970168, 0.9507575757575758013, 0.9545454545454545858, 0.9583333333333333703, 0.9621212121212121549, 0.9659090909090909394 ),
 .UNSPECIFIED. ) 
 GEOMETRIC_REPRESENTATION_ITEM ( )  RATIONAL_B_SPLINE_SURFACE ( (
 ( 1.000000000000000000, 0.9659258262890683122, 1.000000000000000000, 0.9659258262890683122, 1.000000000000000000, 0.9659258262890683122, 1.000000000000000000, 0.9659258262890683122, 1.000000000000000000, 0.9659258262890683122, 1.000000000000000000, 0.9659258262890683122, 1.000000000000000000, 0.9659258262890683122, 1.000000000000000000, 0.9659258262890683122, 1.000000000000000000, 0.9659258262890683122, 1.000000000000000000, 0.9659258262890683122, 1.000000000000000000, 0.9659258262890683122, 1.000000000000000000, 0.9659258262890683122, 1.000000000000000000, 0.9659258262890683122, 1.000000000000000000, 0.9659258262890683122, 1.000000000000000000, 0.9659258262890683122, 1.000000000000000000, 0.9659258262890683122, 1.000000000000000000, 0.9659258262890683122, 1.000000000000000000, 0.9659258262890683122, 1.000000000000000000, 0.9659258262890683122, 1.000000000000000000, 0.9659258262890683122, 1.000000000000000000, 0.9659258262890683122, 1.000000000000000000, 0.9659258262890683122, 1.000000000000000000, 0.9659258262890683122, 1.000000000000000000, 0.9659258262890683122, 1.000000000000000000, 0.9659258262890683122, 1.000000000000000000, 0.9659258262890683122, 1.000000000000000000, 0.9659258262890683122, 1.000000000000000000, 0.9659258262890683122, 1.000000000000000000, 0.9659258262890683122, 1.000000000000000000, 0.9659258262890683122, 1.000000000000000000, 0.9659258262890683122, 1.000000000000000000, 0.9659258262890683122, 1.000000000000000000, 0.9659258262890683122, 1.000000000000000000, 0.9659258262890683122, 1.000000000000000000, 0.9659258262890683122, 1.000000000000000000, 0.9659258262890683122, 1.000000000000000000, 0.9659258262890683122, 1.000000000000000000, 0.9659258262890683122, 1.000000000000000000, 0.9659258262890683122, 1.000000000000000000, 0.9659258262890683122, 1.000000000000000000, 0.9659258262890683122, 1.000000000000000000, 0.9659258262890683122, 1.000000000000000000, 0.9659258262890683122, 1.000000000000000000, 0.9659258262890683122, 1.000000000000000000, 0.9659258262890683122, 1.000000000000000000, 0.9659258262890683122, 1.000000000000000000, 0.9659258262890683122, 1.000000000000000000, 0.9659258262890683122, 1.000000000000000000, 0.9659258262890683122, 1.000000000000000000, 0.9659258262890683122, 1.000000000000000000, 0.9659258262890683122, 1.000000000000000000, 0.9659258262890683122, 1.000000000000000000, 0.9659258262890683122, 1.000000000000000000, 0.9659258262890683122, 1.000000000000000000, 0.9659258262890683122, 1.000000000000000000, 0.9659258262890683122, 1.000000000000000000, 0.9659258262890683122, 1.000000000000000000, 0.9659258262890683122, 1.000000000000000000, 0.9659258262890683122, 1.000000000000000000, 0.9659258262890683122, 1.000000000000000000, 0.9659258262890683122, 1.000000000000000000, 0.9659258262890683122, 1.000000000000000000, 0.9659258262890683122, 1.000000000000000000, 0.9659258262890683122, 1.000000000000000000, 0.9659258262890683122, 1.000000000000000000, 0.9659258262890683122, 1.000000000000000000, 0.9659258262890683122, 1.000000000000000000, 0.9659258262890683122, 1.000000000000000000, 0.9659258262890683122, 1.000000000000000000, 0.9659258262890683122, 1.000000000000000000, 0.9659258262890683122, 1.000000000000000000, 0.9659258262890683122, 1.000000000000000000, 0.9659258262890683122, 1.000000000000000000, 0.9659258262890683122, 1.000000000000000000, 0.9659258262890683122, 1.000000000000000000, 0.9659258262890683122, 1.000000000000000000, 0.9659258262890683122, 1.000000000000000000, 0.9659258262890683122, 1.000000000000000000, 0.9659258262890683122, 1.000000000000000000, 0.9659258262890683122, 1.000000000000000000, 0.9659258262890683122, 1.000000000000000000, 0.9659258262890683122, 1.000000000000000000, 0.9659258262890683122, 1.000000000000000000, 0.9659258262890683122, 1.000000000000000000, 0.9659258262890683122, 1.000000000000000000, 0.9659258262890683122, 1.000000000000000000, 0.9659258262890683122, 1.000000000000000000, 0.9659258262890683122, 1.000000000000000000, 0.9659258262890683122, 1.000000000000000000, 0.9659258262890683122, 1.000000000000000000, 0.9659258262890683122, 1.000000000000000000, 0.9659258262890683122, 1.000000000000000000, 0.9659258262890683122, 1.000000000000000000, 0.9659258262890683122, 1.000000000000000000, 0.9659258262890683122, 1.000000000000000000, 0.9659258262890683122, 1.000000000000000000, 0.9659258262890683122, 1.000000000000000000, 0.9659258262890683122, 1.000000000000000000, 0.9659258262890683122, 1.000000000000000000, 0.9659258262890683122, 1.000000000000000000, 0.9659258262890683122, 1.000000000000000000, 0.9659258262890683122, 1.000000000000000000, 0.9659258262890683122, 1.000000000000000000, 0.9659258262890683122, 1.000000000000000000, 0.9659258262890683122, 1.000000000000000000, 0.9659258262890683122, 1.000000000000000000, 0.9659258262890683122, 1.000000000000000000, 0.9659258262890683122, 1.000000000000000000, 0.9659258262890683122, 1.000000000000000000, 0.9659258262890683122, 1.000000000000000000, 0.9659258262890683122, 1.000000000000000000, 0.9659258262890683122, 1.000000000000000000, 0.9659258262890683122, 1.000000000000000000, 0.9659258262890683122, 1.000000000000000000, 0.9659258262890683122, 1.000000000000000000, 0.9659258262890683122, 1.000000000000000000, 0.9659258262890683122, 1.000000000000000000, 0.9659258262890683122, 1.000000000000000000, 0.9659258262890683122, 1.000000000000000000, 0.9659258262890683122, 1.000000000000000000, 0.9659258262890683122, 1.000000000000000000, 0.9659258262890683122, 1.000000000000000000, 0.9659258262890683122, 1.000000000000000000, 0.9659258262890683122, 1.000000000000000000, 0.9659258262890683122, 1.000000000000000000, 0.9659258262890683122, 1.000000000000000000, 0.9659258262890683122, 1.000000000000000000, 0.9659258262890683122, 1.000000000000000000, 0.9659258262890683122, 1.000000000000000000, 0.9659258262890683122, 1.000000000000000000, 0.9659258262890683122, 1.000000000000000000, 0.9659258262890683122, 1.000000000000000000, 0.9659258262890683122, 1.000000000000000000, 0.9659258262890683122, 1.000000000000000000, 0.9659258262890683122, 1.000000000000000000, 0.9659258262890683122, 1.000000000000000000, 0.9659258262890683122, 1.000000000000000000, 0.9659258262890683122, 1.000000000000000000, 0.9659258262890683122, 1.000000000000000000, 0.9659258262890683122, 1.000000000000000000, 0.9659258262890683122, 1.000000000000000000, 0.9659258262890683122, 1.000000000000000000, 0.9659258262890683122, 1.000000000000000000, 0.9659258262890683122, 1.000000000000000000, 0.9659258262890683122, 1.000000000000000000, 0.9659258262890683122, 1.000000000000000000, 0.9659258262890683122, 1.000000000000000000, 0.9659258262890683122, 1.000000000000000000, 0.9659258262890683122, 1.000000000000000000, 0.9659258262890683122, 1.000000000000000000, 0.9659258262890683122, 1.000000000000000000, 0.9659258262890683122, 1.000000000000000000, 0.9659258262890683122, 1.000000000000000000, 0.9659258262890683122, 1.000000000000000000, 0.9659258262890683122, 1.000000000000000000, 0.9659258262890683122, 1.000000000000000000, 0.9659258262890683122, 1.000000000000000000, 0.9659258262890683122, 1.000000000000000000, 0.9659258262890683122, 1.000000000000000000, 0.9659258262890683122, 1.000000000000000000, 0.9659258262890683122, 1.000000000000000000, 0.9659258262890683122, 1.000000000000000000, 0.9659258262890683122, 1.000000000000000000, 0.9659258262890683122, 1.000000000000000000, 0.9659258262890683122, 1.000000000000000000, 0.9659258262890683122, 1.000000000000000000, 0.9659258262890683122, 1.000000000000000000, 0.9659258262890683122, 1.000000000000000000, 0.9659258262890683122, 1.000000000000000000, 0.9659258262890683122, 1.000000000000000000, 0.9659258262890683122, 1.000000000000000000, 0.9659258262890683122, 1.000000000000000000, 0.9659258262890683122, 1.000000000000000000, 0.9659258262890683122, 1.000000000000000000, 0.9659258262890683122, 1.000000000000000000, 0.9659258262890683122, 1.000000000000000000, 0.9659258262890683122, 1.000000000000000000, 0.9659258262890683122, 1.000000000000000000, 0.9659258262890683122, 1.000000000000000000, 0.9659258262890683122, 1.000000000000000000, 0.9659258262890683122, 1.000000000000000000, 0.9659258262890683122, 1.000000000000000000, 0.9659258262890683122, 1.000000000000000000, 0.9659258262890683122, 1.000000000000000000, 0.9659258262890683122, 1.000000000000000000, 0.9659258262890683122, 1.000000000000000000, 0.9659258262890683122, 1.000000000000000000, 0.9659258262890683122, 1.000000000000000000, 0.9659258262890683122, 1.000000000000000000, 0.9659258262890683122, 1.000000000000000000, 0.9659258262890683122, 1.000000000000000000, 0.9659258262890683122, 1.000000000000000000, 0.9659258262890683122, 1.000000000000000000, 0.9659258262890683122, 1.000000000000000000, 0.9659258262890683122, 1.000000000000000000, 0.9659258262890683122, 1.000000000000000000, 0.9659258262890683122, 1.000000000000000000, 0.9659258262890683122, 1.000000000000000000, 0.9659258262890683122, 1.000000000000000000, 0.9659258262890683122, 1.000000000000000000, 0.9659258262890683122, 1.000000000000000000, 0.9659258262890683122, 1.000000000000000000, 0.9659258262890683122, 1.000000000000000000, 0.9659258262890683122, 1.000000000000000000, 0.9659258262890683122, 1.000000000000000000, 0.9659258262890683122, 1.000000000000000000, 0.9659258262890683122, 1.000000000000000000, 0.9659258262890683122, 1.000000000000000000, 0.9659258262890683122, 1.000000000000000000, 0.9659258262890683122, 1.000000000000000000, 0.9659258262890683122, 1.000000000000000000, 0.9659258262890683122, 1.000000000000000000, 0.9659258262890683122, 1.000000000000000000, 0.9659258262890683122, 1.000000000000000000, 0.9659258262890683122, 1.000000000000000000, 0.9659258262890683122, 1.000000000000000000, 0.9659258262890683122, 1.000000000000000000, 0.9659258262890683122, 1.000000000000000000, 0.9659258262890683122, 1.000000000000000000, 0.9659258262890683122, 1.000000000000000000, 0.9659258262890683122, 1.000000000000000000, 0.9659258262890683122, 1.000000000000000000, 0.9659258262890683122, 1.000000000000000000, 0.9659258262890683122, 1.000000000000000000, 0.9659258262890683122, 1.000000000000000000, 0.9659258262890683122, 1.000000000000000000, 0.9659258262890683122, 1.000000000000000000, 0.9659258262890683122, 1.000000000000000000, 0.9659258262890683122, 1.000000000000000000, 0.9659258262890683122, 1.000000000000000000, 0.9659258262890683122, 1.000000000000000000, 0.9659258262890683122, 1.000000000000000000, 0.9659258262890683122, 1.000000000000000000, 0.9659258262890683122, 1.000000000000000000, 0.9659258262890683122, 1.000000000000000000, 0.9659258262890683122, 1.000000000000000000, 0.9659258262890683122, 1.000000000000000000, 0.9659258262890683122, 1.000000000000000000, 0.9659258262890683122, 1.000000000000000000, 0.9659258262890683122, 1.000000000000000000, 0.9659258262890683122, 1.000000000000000000, 0.9659258262890683122, 1.000000000000000000, 0.9659258262890683122, 1.000000000000000000, 0.9659258262890683122, 1.000000000000000000, 0.9659258262890683122, 1.000000000000000000, 0.9659258262890683122, 1.000000000000000000, 0.9659258262890683122, 1.000000000000000000, 0.9659258262890683122, 1.000000000000000000, 0.9659258262890683122, 1.000000000000000000, 0.9659258262890683122, 1.000000000000000000, 0.9659258262890683122, 1.000000000000000000, 0.9659258262890683122, 1.000000000000000000, 0.9659258262890683122, 1.000000000000000000, 0.9659258262890683122, 1.000000000000000000, 0.9659258262890683122, 1.000000000000000000),
 ( 1.000000000000000000, 0.9659258262890683122, 1.000000000000000000, 0.9659258262890683122, 1.000000000000000000, 0.9659258262890683122, 1.000000000000000000, 0.9659258262890683122, 1.000000000000000000, 0.9659258262890683122, 1.000000000000000000, 0.9659258262890683122, 1.000000000000000000, 0.9659258262890683122, 1.000000000000000000, 0.9659258262890683122, 1.000000000000000000, 0.9659258262890683122, 1.000000000000000000, 0.9659258262890683122, 1.000000000000000000, 0.9659258262890683122, 1.000000000000000000, 0.9659258262890683122, 1.000000000000000000, 0.9659258262890683122, 1.000000000000000000, 0.9659258262890683122, 1.000000000000000000, 0.9659258262890683122, 1.000000000000000000, 0.9659258262890683122, 1.000000000000000000, 0.9659258262890683122, 1.000000000000000000, 0.9659258262890683122, 1.000000000000000000, 0.9659258262890683122, 1.000000000000000000, 0.9659258262890683122, 1.000000000000000000, 0.9659258262890683122, 1.000000000000000000, 0.9659258262890683122, 1.000000000000000000, 0.9659258262890683122, 1.000000000000000000, 0.9659258262890683122, 1.000000000000000000, 0.9659258262890683122, 1.000000000000000000, 0.9659258262890683122, 1.000000000000000000, 0.9659258262890683122, 1.000000000000000000, 0.9659258262890683122, 1.000000000000000000, 0.9659258262890683122, 1.000000000000000000, 0.9659258262890683122, 1.000000000000000000, 0.9659258262890683122, 1.000000000000000000, 0.9659258262890683122, 1.000000000000000000, 0.9659258262890683122, 1.000000000000000000, 0.9659258262890683122, 1.000000000000000000, 0.9659258262890683122, 1.000000000000000000, 0.9659258262890683122, 1.000000000000000000, 0.9659258262890683122, 1.000000000000000000, 0.9659258262890683122, 1.000000000000000000, 0.9659258262890683122, 1.000000000000000000, 0.9659258262890683122, 1.000000000000000000, 0.9659258262890683122, 1.000000000000000000, 0.9659258262890683122, 1.000000000000000000, 0.9659258262890683122, 1.000000000000000000, 0.9659258262890683122, 1.000000000000000000, 0.9659258262890683122, 1.000000000000000000, 0.9659258262890683122, 1.000000000000000000, 0.9659258262890683122, 1.000000000000000000, 0.9659258262890683122, 1.000000000000000000, 0.9659258262890683122, 1.000000000000000000, 0.9659258262890683122, 1.000000000000000000, 0.9659258262890683122, 1.000000000000000000, 0.9659258262890683122, 1.000000000000000000, 0.9659258262890683122, 1.000000000000000000, 0.9659258262890683122, 1.000000000000000000, 0.9659258262890683122, 1.000000000000000000, 0.9659258262890683122, 1.000000000000000000, 0.9659258262890683122, 1.000000000000000000, 0.9659258262890683122, 1.000000000000000000, 0.9659258262890683122, 1.000000000000000000, 0.9659258262890683122, 1.000000000000000000, 0.9659258262890683122, 1.000000000000000000, 0.9659258262890683122, 1.000000000000000000, 0.9659258262890683122, 1.000000000000000000, 0.9659258262890683122, 1.000000000000000000, 0.9659258262890683122, 1.000000000000000000, 0.9659258262890683122, 1.000000000000000000, 0.9659258262890683122, 1.000000000000000000, 0.9659258262890683122, 1.000000000000000000, 0.9659258262890683122, 1.000000000000000000, 0.9659258262890683122, 1.000000000000000000, 0.9659258262890683122, 1.000000000000000000, 0.9659258262890683122, 1.000000000000000000, 0.9659258262890683122, 1.000000000000000000, 0.9659258262890683122, 1.000000000000000000, 0.9659258262890683122, 1.000000000000000000, 0.9659258262890683122, 1.000000000000000000, 0.9659258262890683122, 1.000000000000000000, 0.9659258262890683122, 1.000000000000000000, 0.9659258262890683122, 1.000000000000000000, 0.9659258262890683122, 1.000000000000000000, 0.9659258262890683122, 1.000000000000000000, 0.9659258262890683122, 1.000000000000000000, 0.9659258262890683122, 1.000000000000000000, 0.9659258262890683122, 1.000000000000000000, 0.9659258262890683122, 1.000000000000000000, 0.9659258262890683122, 1.000000000000000000, 0.9659258262890683122, 1.000000000000000000, 0.9659258262890683122, 1.000000000000000000, 0.9659258262890683122, 1.000000000000000000, 0.9659258262890683122, 1.000000000000000000, 0.9659258262890683122, 1.000000000000000000, 0.9659258262890683122, 1.000000000000000000, 0.9659258262890683122, 1.000000000000000000, 0.9659258262890683122, 1.000000000000000000, 0.9659258262890683122, 1.000000000000000000, 0.9659258262890683122, 1.000000000000000000, 0.9659258262890683122, 1.000000000000000000, 0.9659258262890683122, 1.000000000000000000, 0.9659258262890683122, 1.000000000000000000, 0.9659258262890683122, 1.000000000000000000, 0.9659258262890683122, 1.000000000000000000, 0.9659258262890683122, 1.000000000000000000, 0.9659258262890683122, 1.000000000000000000, 0.9659258262890683122, 1.000000000000000000, 0.9659258262890683122, 1.000000000000000000, 0.9659258262890683122, 1.000000000000000000, 0.9659258262890683122, 1.000000000000000000, 0.9659258262890683122, 1.000000000000000000, 0.9659258262890683122, 1.000000000000000000, 0.9659258262890683122, 1.000000000000000000, 0.9659258262890683122, 1.000000000000000000, 0.9659258262890683122, 1.000000000000000000, 0.9659258262890683122, 1.000000000000000000, 0.9659258262890683122, 1.000000000000000000, 0.9659258262890683122, 1.000000000000000000, 0.9659258262890683122, 1.000000000000000000, 0.9659258262890683122, 1.000000000000000000, 0.9659258262890683122, 1.000000000000000000, 0.9659258262890683122, 1.000000000000000000, 0.9659258262890683122, 1.000000000000000000, 0.9659258262890683122, 1.000000000000000000, 0.9659258262890683122, 1.000000000000000000, 0.9659258262890683122, 1.000000000000000000, 0.9659258262890683122, 1.000000000000000000, 0.9659258262890683122, 1.000000000000000000, 0.9659258262890683122, 1.000000000000000000, 0.9659258262890683122, 1.000000000000000000, 0.9659258262890683122, 1.000000000000000000, 0.9659258262890683122, 1.000000000000000000, 0.9659258262890683122, 1.000000000000000000, 0.9659258262890683122, 1.000000000000000000, 0.9659258262890683122, 1.000000000000000000, 0.9659258262890683122, 1.000000000000000000, 0.9659258262890683122, 1.000000000000000000, 0.9659258262890683122, 1.000000000000000000, 0.9659258262890683122, 1.000000000000000000, 0.9659258262890683122, 1.000000000000000000, 0.9659258262890683122, 1.000000000000000000, 0.9659258262890683122, 1.000000000000000000, 0.9659258262890683122, 1.000000000000000000, 0.9659258262890683122, 1.000000000000000000, 0.9659258262890683122, 1.000000000000000000, 0.9659258262890683122, 1.000000000000000000, 0.9659258262890683122, 1.000000000000000000, 0.9659258262890683122, 1.000000000000000000, 0.9659258262890683122, 1.000000000000000000, 0.9659258262890683122, 1.000000000000000000, 0.9659258262890683122, 1.000000000000000000, 0.9659258262890683122, 1.000000000000000000, 0.9659258262890683122, 1.000000000000000000, 0.9659258262890683122, 1.000000000000000000, 0.9659258262890683122, 1.000000000000000000, 0.9659258262890683122, 1.000000000000000000, 0.9659258262890683122, 1.000000000000000000, 0.9659258262890683122, 1.000000000000000000, 0.9659258262890683122, 1.000000000000000000, 0.9659258262890683122, 1.000000000000000000, 0.9659258262890683122, 1.000000000000000000, 0.9659258262890683122, 1.000000000000000000, 0.9659258262890683122, 1.000000000000000000, 0.9659258262890683122, 1.000000000000000000, 0.9659258262890683122, 1.000000000000000000, 0.9659258262890683122, 1.000000000000000000, 0.9659258262890683122, 1.000000000000000000, 0.9659258262890683122, 1.000000000000000000, 0.9659258262890683122, 1.000000000000000000, 0.9659258262890683122, 1.000000000000000000, 0.9659258262890683122, 1.000000000000000000, 0.9659258262890683122, 1.000000000000000000, 0.9659258262890683122, 1.000000000000000000, 0.9659258262890683122, 1.000000000000000000, 0.9659258262890683122, 1.000000000000000000, 0.9659258262890683122, 1.000000000000000000, 0.9659258262890683122, 1.000000000000000000, 0.9659258262890683122, 1.000000000000000000, 0.9659258262890683122, 1.000000000000000000, 0.9659258262890683122, 1.000000000000000000, 0.9659258262890683122, 1.000000000000000000, 0.9659258262890683122, 1.000000000000000000, 0.9659258262890683122, 1.000000000000000000, 0.9659258262890683122, 1.000000000000000000, 0.9659258262890683122, 1.000000000000000000, 0.9659258262890683122, 1.000000000000000000, 0.9659258262890683122, 1.000000000000000000, 0.9659258262890683122, 1.000000000000000000, 0.9659258262890683122, 1.000000000000000000, 0.9659258262890683122, 1.000000000000000000, 0.9659258262890683122, 1.000000000000000000, 0.9659258262890683122, 1.000000000000000000, 0.9659258262890683122, 1.000000000000000000, 0.9659258262890683122, 1.000000000000000000, 0.9659258262890683122, 1.000000000000000000, 0.9659258262890683122, 1.000000000000000000, 0.9659258262890683122, 1.000000000000000000, 0.9659258262890683122, 1.000000000000000000, 0.9659258262890683122, 1.000000000000000000, 0.9659258262890683122, 1.000000000000000000, 0.9659258262890683122, 1.000000000000000000, 0.9659258262890683122, 1.000000000000000000, 0.9659258262890683122, 1.000000000000000000, 0.9659258262890683122, 1.000000000000000000, 0.9659258262890683122, 1.000000000000000000, 0.9659258262890683122, 1.000000000000000000, 0.9659258262890683122, 1.000000000000000000, 0.9659258262890683122, 1.000000000000000000, 0.9659258262890683122, 1.000000000000000000, 0.9659258262890683122, 1.000000000000000000, 0.9659258262890683122, 1.000000000000000000, 0.9659258262890683122, 1.000000000000000000, 0.9659258262890683122, 1.000000000000000000, 0.9659258262890683122, 1.000000000000000000, 0.9659258262890683122, 1.000000000000000000, 0.9659258262890683122, 1.000000000000000000, 0.9659258262890683122, 1.000000000000000000, 0.9659258262890683122, 1.000000000000000000, 0.9659258262890683122, 1.000000000000000000, 0.9659258262890683122, 1.000000000000000000, 0.9659258262890683122, 1.000000000000000000, 0.9659258262890683122, 1.000000000000000000, 0.9659258262890683122, 1.000000000000000000, 0.9659258262890683122, 1.000000000000000000, 0.9659258262890683122, 1.000000000000000000, 0.9659258262890683122, 1.000000000000000000, 0.9659258262890683122, 1.000000000000000000, 0.9659258262890683122, 1.000000000000000000, 0.9659258262890683122, 1.000000000000000000, 0.9659258262890683122, 1.000000000000000000, 0.9659258262890683122, 1.000000000000000000, 0.9659258262890683122, 1.000000000000000000, 0.9659258262890683122, 1.000000000000000000, 0.9659258262890683122, 1.000000000000000000, 0.9659258262890683122, 1.000000000000000000, 0.9659258262890683122, 1.000000000000000000, 0.9659258262890683122, 1.000000000000000000, 0.9659258262890683122, 1.000000000000000000, 0.9659258262890683122, 1.000000000000000000, 0.9659258262890683122, 1.000000000000000000, 0.9659258262890683122, 1.000000000000000000, 0.9659258262890683122, 1.000000000000000000, 0.9659258262890683122, 1.000000000000000000, 0.9659258262890683122, 1.000000000000000000, 0.9659258262890683122, 1.000000000000000000, 0.9659258262890683122, 1.000000000000000000, 0.9659258262890683122, 1.000000000000000000, 0.9659258262890683122, 1.000000000000000000, 0.9659258262890683122, 1.000000000000000000, 0.9659258262890683122, 1.000000000000000000, 0.9659258262890683122, 1.000000000000000000, 0.9659258262890683122, 1.000000000000000000, 0.9659258262890683122, 1.000000000000000000, 0.9659258262890683122, 1.000000000000000000, 0.9659258262890683122, 1.000000000000000000, 0.9659258262890683122, 1.000000000000000000, 0.9659258262890683122, 1.000000000000000000, 0.9659258262890683122, 1.000000000000000000) ) ) 
 REPRESENTATION_ITEM ( '' )  SURFACE ( )  );
#79857=CARTESIAN_POINT ( 'NONE',  ( -0.6627296587926501115, 0.2952755905511810774, -0.1292274648535930714 ) ) ;
#79858=CARTESIAN_POINT ( 'NONE',  ( 1.640419947506562393, -0.4281496062992124485, 0.4176697321401328655 ) ) ;
#79860=CARTESIAN_POINT ( 'NONE',  ( -1.614173228346456712, 2.401574803149606474, -0.1372047244094478091 ) ) ;
#79862=CARTESIAN_POINT ( 'NONE',  ( -1.430446194225721390, -0.4281496062992124485, 0.4176697321401328655 ) ) ;
#79863=CARTESIAN_POINT ( 'NONE',  ( -0.6364829396325453192, -0.3162353388693405765, 0.4822834645669290543 ) ) ;
#79865=CARTESIAN_POINT ( 'NONE',  ( 0.3412073490813655186, 0.1283753931104748280, 0.1820866141732283561 ) ) ;
#79868=CARTESIAN_POINT ( 'NONE',  ( 0.2690288713910767848, 0.1771653543307087630, 0.09757992244046791164 ) ) ;
#79869=CARTESIAN_POINT ( 'NONE',  ( 1.030183727034121421, -0.2845877964562161244, -0.3641732283464567121 ) ) ;
#79870=CARTESIAN_POINT ( 'NONE',  ( 1.095800524934383846, -0.3162353388693405765, 0.4822834645669290543 ) ) ;
#79871=CARTESIAN_POINT ( 'NONE',  ( -0.5052493438320203589, 0.1771653543307087075, -0.09757992244046823083 ) ) ;
#79873=CARTESIAN_POINT ( 'NONE',  ( -1.122047244094487306, 0.1660481256975883668, -0.3530559997133364547 ) ) ;
#79874=CARTESIAN_POINT ( 'NONE',  ( -1.259842519685038686, -0.1870078740157480601, -0.3641732283464567677 ) ) ;
#79876=CARTESIAN_POINT ( 'NONE',  ( -0.9317585301837263412, -0.3690944881889765550, -0.3153832671262227771 ) ) ;
#79877=CARTESIAN_POINT ( 'NONE',  ( -0.2821522309711278487, -0.6692913385826773087, -0.1292274648535924053 ) ) ;
#79878=CARTESIAN_POINT ( 'NONE',  ( 1.601049868766404982, -0.5023911411419708095, -0.1820866141732282451 ) ) ;
#79880=CARTESIAN_POINT ( 'NONE',  ( 0.4265091863517067039, -0.5511811023622048555, -0.09757992244046775898 ) ) ;
#79881=CARTESIAN_POINT ( 'NONE',  ( -0.4527559055118102749, 0.07958543189024085140, 0.2665933059059887866 ) ) ;
#79882=CARTESIAN_POINT ( 'NONE',  ( -0.7217847769028863381, -0.4281496062992124485, 0.4176697321401328655 ) ) ;
#79883=DIRECTION ( 'NONE',  ( 0.000000000000000000, 0.000000000000000000, -1.000000000000000000 ) ) ;
#79884=CARTESIAN_POINT ( 'NONE',  ( -2.795275590551183686, 1.299212598425198095, -1.990688069879260956E-16 ) ) ;
#79885=CARTESIAN_POINT ( 'NONE',  ( 0.2755905511811031494, 0.2952755905511811885, 0.000000000000000000 ) ) ;
#79887=CARTESIAN_POINT ( 'NONE',  ( 1.614173228346457378, 0.2952755905511811885, 0.000000000000000000 ) ) ;
#79888=CARTESIAN_POINT ( 'NONE',  ( -0.1312335958005241554, 0.1283753931104748280, 0.1820866141732283561 ) ) ;
#79889=CARTESIAN_POINT ( 'NONE',  ( -0.006561679790025524116, -0.3162353388693405765, 0.4822834645669290543 ) ) ;
#79890=CARTESIAN_POINT ( 'NONE',  ( -1.443569553805773564, 0.2306618581243847221, -0.2411417322834647770 ) ) ;
#79891=CARTESIAN_POINT ( 'NONE',  ( 1.522309711286089939, 0.2306618581243848609, 0.2411417322834645549 ) ) ;
#79892=CARTESIAN_POINT ( 'NONE',  ( 1.292650918635171564, -0.6692913385826773087, -0.1292274648535924053 ) ) ;
#79893=CARTESIAN_POINT ( 'NONE',  ( -0.5314960629921254842, -0.4536011799217368745, -0.2665933059059886201 ) ) ;
#79897=CARTESIAN_POINT ( 'NONE',  ( 1.574803149606299746, -0.1870078740157480601, -0.3641732283464567677 ) ) ;
#79899=CARTESIAN_POINT ( 'NONE',  ( 1.253280839895013710, -0.2845877964562159024, 0.3641732283464567677 ) ) ;
#79902=CARTESIAN_POINT ( 'NONE',  ( 0.8005249343832027131, 0.05413385826771666132, 0.4176697321401328100 ) ) ;
#79904=CARTESIAN_POINT ( 'NONE',  ( 1.272965879265092637, -0.3690944881889765550, -0.3153832671262227771 ) ) ;
#79906=CARTESIAN_POINT ( 'NONE',  ( 0.1902887139107617975, -0.6692913385826773087, -0.1292274648535924053 ) ) ;
#79907=CARTESIAN_POINT ( 'NONE',  ( -0.5118110236220466680, 0.2952755905511811885, 0.000000000000000000 ) ) ;
#79911=CARTESIAN_POINT ( 'NONE',  ( 0.5314960629921264834, 0.07958543189024071263, -0.2665933059059888421 ) ) ;
#79912=ORIENTED_EDGE ( 'NONE', *, *, #37828, .T. ) ;
#79915=CARTESIAN_POINT ( 'NONE',  ( -0.6233595800524928121, -0.05778040916215522460, 0.4822834645669289988 ) ) ;
#79916=CARTESIAN_POINT ( 'NONE',  ( 0.9645669291338588858, 0.1660481256975885056, 0.3530559997133364547 ) ) ;
#79917=CARTESIAN_POINT ( 'NONE',  ( 0.3018372703412079971, 0.05413385826771626580, -0.4176697321401330321 ) ) ;
#79918=CARTESIAN_POINT ( 'NONE',  ( -0.1771653543307080136, 0.07958543189024071263, -0.2665933059059888421 ) ) ;
#79919=VECTOR ( 'NONE', #7670, 39.37007874015748143 ) ;
#79920=CARTESIAN_POINT ( 'NONE',  ( 0.6364829396325465405, -0.3162353388693409650, -0.4822834645669289433 ) ) ;
#79921=CARTESIAN_POINT ( 'NONE',  ( -0.8333333333333323711, 0.2952755905511811885, 0.1292274648535926551 ) ) ;
#79922=CARTESIAN_POINT ( 'NONE',  ( -0.5314960629921254842, -0.5400638737290845981, -0.3530559997133363437 ) ) ;
#79923=CARTESIAN_POINT ( 'NONE',  ( -0.9908136482939626788, -0.6692913385826773087, -0.1292274648535924053 ) ) ;
#79924=CARTESIAN_POINT ( 'NONE',  ( 1.036745406824147508, -0.4281496062992127816, -0.4176697321401328100 ) ) ;
#79925=CARTESIAN_POINT ( 'NONE',  ( 0.7283464566929140904, -0.5400638737290845981, -0.3530559997133363437 ) ) ;
#79926=CARTESIAN_POINT ( 'NONE',  ( 0.8070866141732289112, -0.5400638737290845981, -0.3530559997133363437 ) ) ;
#79929=CARTESIAN_POINT ( 'NONE',  ( -0.1312335958005241554, -0.5023911411419708095, -0.1820866141732282451 ) ) ;
#79933=CARTESIAN_POINT ( 'NONE',  ( -1.030183727034119867, -0.08942795157528024563, -0.3641732283464568787 ) ) ;
#79934=CARTESIAN_POINT ( 'NONE',  ( -0.2952755905511803003, -0.5400638737290845981, -0.3530559997133363437 ) ) ;
#79936=CARTESIAN_POINT ( 'NONE',  ( -0.1706036745406816491, -0.4281496062992124485, 0.4176697321401328655 ) ) ;
#79937=CARTESIAN_POINT ( 'NONE',  ( -0.5118110236220466680, -0.6692913385826771977, 8.415575281601705876E-17 ) ) ;
#79938=CARTESIAN_POINT ( 'NONE',  ( -1.194225721784776262, -0.4281496062992124485, 0.4176697321401328655 ) ) ;
#79939=CARTESIAN_POINT ( 'NONE',  ( -1.332020997375327642, -0.3162353388693409650, -0.4822834645669289433 ) ) ;
#79940=VECTOR ( 'NONE', #38923, 39.37007874015748143 ) ;
#79941=CARTESIAN_POINT ( 'NONE',  ( 0.7742782152230979209, -0.004921259842519870586, -0.3153832671262229437 ) ) ;
#79944=CARTESIAN_POINT ( 'NONE',  ( 0.3280839895013130669, -0.004921259842519576551, 0.3153832671262227771 ) ) ;
#79946=CARTESIAN_POINT ( 'NONE',  ( -0.1443569553805765515, -0.4281496062992127816, -0.4176697321401328100 ) ) ;
#79947=CARTESIAN_POINT ( 'NONE',  ( 0.2296587926509192634, -0.3162353388693405765, 0.4822834645669290543 ) ) ;
#79950=CARTESIAN_POINT ( 'NONE',  ( -0.6183353934921174133, 0.02791078216816064370, 0.4328096321851915285 ) ) ;
#79954=CARTESIAN_POINT ( 'NONE',  ( -0.6758530183727028406, -0.5511811023622048555, -0.09757992244046775898 ) ) ;
#79955=CARTESIAN_POINT ( 'NONE',  ( -0.5774278215223089816, 0.2306618581243847221, -0.2411417322834647770 ) ) ;
#79958=CARTESIAN_POINT ( 'NONE',  ( -1.430446194225720724, -0.004921259842519870586, -0.3153832671262229437 ) ) ;
#79959=CARTESIAN_POINT ( 'NONE',  ( 0.6889763779527563470, 0.1660481256975883668, -0.3530559997133364547 ) ) ;
#79960=CARTESIAN_POINT ( 'NONE',  ( 0.9251968503937015864, 0.1660481256975883668, -0.3530559997133364547 ) ) ;
#79961=CARTESIAN_POINT ( 'NONE',  ( -0.6627296587926501115, 0.1771653543307087075, -0.09757992244046823083 ) ) ;
#79962=CARTESIAN_POINT ( 'NONE',  ( 0.1968503937007881344, 0.2952755905511811885, 0.000000000000000000 ) ) ;
#79964=CARTESIAN_POINT ( 'NONE',  ( -0.1312335958005241554, -0.5023911411419708095, -0.1820866141732282451 ) ) ;
#79965=CARTESIAN_POINT ( 'NONE',  ( -0.5643044619422565855, 0.05413385826771626580, -0.4176697321401330321 ) ) ;
#79967=CARTESIAN_POINT ( 'NONE',  ( 1.509186351706037543, -0.3690944881889765550, -0.3153832671262227771 ) ) ;
#79968=CARTESIAN_POINT ( 'NONE',  ( 0.07217847769028949700, -0.08942795157528024563, -0.3641732283464568787 ) ) ;
#79969=CARTESIAN_POINT ( 'NONE',  ( 1.581364829396326277, -0.2845877964562161244, -0.3641732283464567121 ) ) ;
#79970=CARTESIAN_POINT ( 'NONE',  ( -1.102362204724408601, -0.1870078740157479769, 0.4822834645669291653 ) ) ;
#79971=CARTESIAN_POINT ( 'NONE',  ( -0.6233595800524928121, -0.2845877964562161244, -0.3641732283464567121 ) ) ;
#79973=CARTESIAN_POINT ( 'NONE',  ( -1.076115485564303809, 0.2306618581243848609, 0.2411417322834645549 ) ) ;
#79974=CARTESIAN_POINT ( 'NONE',  ( -0.2099737532808391705, 0.2306618581243848609, 0.2411417322834645549 ) ) ;
#79978=CARTESIAN_POINT ( 'NONE',  ( 0.1968503937007881344, -0.5511811023622047445, 6.969142054262312111E-17 ) ) ;
#79979=CARTESIAN_POINT ( 'NONE',  ( 1.148293963254593653, 0.2952755905511810774, -0.1292274648535930714 ) ) ;
#79980=CARTESIAN_POINT ( 'NONE',  ( -1.062992125984250968, 0.1771653543307087630, 0.000000000000000000 ) ) ;
#79981=CARTESIAN_POINT ( 'NONE',  ( 1.062992125984252745, 0.2952755905511811885, 0.000000000000000000 ) ) ;
#79982=CARTESIAN_POINT ( 'NONE',  ( -1.568241469816272105, -0.08942795157527998196, 0.3641732283464567121 ) ) ;
#79983=CARTESIAN_POINT ( 'NONE',  ( -0.6233595800524928121, -0.05778040916215522460, 0.4822834645669289988 ) ) ;
#79984=CARTESIAN_POINT ( 'NONE',  ( 0.05905511811023709395, -0.4536011799217367080, 0.2665933059059888421 ) ) ;
#79986=CARTESIAN_POINT ( 'NONE',  ( 0.7611548556430451917, -0.5023911411419708095, 0.1820866141732285504 ) ) ;
#79988=EDGE_CURVE ( 'NONE', #9295, #3606, #48476, .T. ) ;
#79989=CARTESIAN_POINT ( 'NONE',  ( -0.08530183727034056085, -0.3162353388693405765, 0.4822834645669290543 ) ) ;
#79991=CARTESIAN_POINT ( 'NONE',  ( -0.9055118110236215490, 0.2952755905511811885, 0.000000000000000000 ) ) ;
#79993=CARTESIAN_POINT ( 'NONE',  ( 1.017060367454068581, -0.08942795157528024563, -0.3641732283464568787 ) ) ;
#79994=CARTESIAN_POINT ( 'NONE',  ( -0.1049868766404193215, -0.6046776061558807314, 0.2411417322834647770 ) ) ;
#79995=CARTESIAN_POINT ( 'NONE',  ( -0.1640419947506553400, -0.05778040916215560624, -0.4822834645669293319 ) ) ;
#79996=CARTESIAN_POINT ( 'NONE',  ( -0.5511811023622038563, -0.1870078740157479769, 0.3641732283464567677 ) ) ;
#79997=CARTESIAN_POINT ( 'NONE',  ( 1.213910761154856299, 0.2952755905511811885, 0.1292274648535926551 ) ) ;
#79998=CARTESIAN_POINT ( 'NONE',  ( -0.2821522309711278487, -0.5511811023622048555, -0.09757992244046775898 ) ) ;
#79999=CARTESIAN_POINT ( 'NONE',  ( 0.2165354330708668673, -0.5400638737290844871, 0.3530559997133364547 ) ) ;
#80000=CARTESIAN_POINT ( 'NONE',  ( -0.6561679790026240244, -0.5023911411419708095, 0.1820866141732285504 ) ) ;
#80003=CARTESIAN_POINT ( 'NONE',  ( -1.318897637795274802, 0.1660481256975885056, 0.3530559997133364547 ) ) ;
#80004=DIRECTION ( 'NONE',  ( 0.000000000000000000, -1.000000000000000000, 0.000000000000000000 ) ) ;
#80006=CARTESIAN_POINT ( 'NONE',  ( -1.200787401574802349, 0.07958543189024071263, -0.2665933059059888421 ) ) ;
#80007=CARTESIAN_POINT ( 'NONE',  ( -0.5314960629921254842, -0.5400638737290845981, -0.3530559997133363437 ) ) ;
#80008=CARTESIAN_POINT ( 'NONE',  ( -1.522309711286088607, 0.2306618581243847221, -0.2411417322834647770 ) ) ;
#80009=CARTESIAN_POINT ( 'NONE',  ( -1.246719160104985846, -0.4281496062992127816, -0.4176697321401328100 ) ) ;
#80010=CARTESIAN_POINT ( 'NONE',  ( 1.161417322834646493, -0.5400638737290844871, 0.3530559997133364547 ) ) ;
#80011=CARTESIAN_POINT ( 'NONE',  ( 0.9186351706036752773, 0.2306618581243847221, -0.2411417322834647770 ) ) ;
#80013=CARTESIAN_POINT ( 'NONE',  ( 1.417322834645670104, -0.1870078740157479769, 0.3641732283464567677 ) ) ;
#80015=ORIENTED_EDGE ( 'NONE', *, *, #41924, .F. ) ;
#80016=CARTESIAN_POINT ( 'NONE',  ( -0.4002624671916004129, -0.2845877964562159024, 0.3641732283464567677 ) ) ;
#80019=CARTESIAN_POINT ( 'NONE',  ( 0.7349081364829402885, -0.6046776061558809534, -0.2411417322834644161 ) ) ;
#80020=CARTESIAN_POINT ( 'NONE',  ( -0.3018372703412066094, 0.05413385826771666132, 0.4176697321401328100 ) ) ;
#80021=CARTESIAN_POINT ( 'NONE',  ( -0.6955380577427815458, 0.05413385826771666132, 0.4176697321401328100 ) ) ;
#80022=CARTESIAN_POINT ( 'NONE',  ( 1.463254593175853824, -0.6692913385826771977, 0.1292274648535927661 ) ) ;
#80023=CARTESIAN_POINT ( 'NONE',  ( -1.207349081364828436, -0.5023911411419708095, 0.1820866141732285504 ) ) ;
#80025=CARTESIAN_POINT ( 'NONE',  ( 0.3018372703412079971, 0.05413385826771626580, -0.4176697321401330321 ) ) ;
#80026=CARTESIAN_POINT ( 'NONE',  ( -0.8530183727034112984, 0.05413385826771666132, 0.4176697321401328100 ) ) ;
#80028=CARTESIAN_POINT ( 'NONE',  ( -1.095800524934382292, -0.3162353388693409650, -0.4822834645669289433 ) ) ;
#80029=CARTESIAN_POINT ( 'NONE',  ( 2.787279214012418738, 0.000000000000000000, 0.000000000000000000 ) ) ;
#80030=CARTESIAN_POINT ( 'NONE',  ( 0.8727034120734913358, -0.05778040916215522460, 0.4822834645669289988 ) ) ;
#80031=CARTESIAN_POINT ( 'NONE',  ( 1.377952755905512472, 0.1771653543307087630, 0.000000000000000000 ) ) ;
#80034=CARTESIAN_POINT ( 'NONE',  ( -0.2559055118110227234, -0.5400638737290844871, 0.3530559997133364547 ) ) ;
#80036=CARTESIAN_POINT ( 'NONE',  ( 0.4068241469816279987, -0.3690944881889765550, -0.3153832671262227771 ) ) ;
#80037=CARTESIAN_POINT ( 'NONE',  ( -1.240157480314959759, 0.1660481256975885056, 0.3530559997133364547 ) ) ;
#80038=CARTESIAN_POINT ( 'NONE',  ( 1.108923884514436242, -0.05778040916215522460, 0.4822834645669289988 ) ) ;
#80039=CARTESIAN_POINT ( 'NONE',  ( 0.9908136482939640111, 0.2952755905511810774, -0.1292274648535930714 ) ) ;
#80040=( BOUNDED_CURVE ( )  B_SPLINE_CURVE ( 2, ( #16669, #27615, #46961, #28031, #3197, #68006, #35184, #9511, #16252, #9924, #15003, #66770, #28861 ),
 .UNSPECIFIED., .F., .F. ) 
 B_SPLINE_CURVE_WITH_KNOTS ( ( 3, 2, 2, 2, 2, 2, 3 ),
 ( 0.7649423569342326257, 0.7651515151515151381, 0.7689393939393939226, 0.7727272727272727071, 0.7765151515151514916, 0.7803030303030302761, 0.7805121885203127885 ),
 .UNSPECIFIED. ) 
 CURVE ( )  GEOMETRIC_REPRESENTATION_ITEM ( )  RATIONAL_B_SPLINE_CURVE ( ( 0.9964447847208419695, 0.9981185001348091834, 1.000000000000000000, 0.9659258262890683122, 1.000000000000000000, 0.9659258262890683122, 1.000000000000000000, 0.9659258262890683122, 1.000000000000000000, 0.9659258262890683122, 1.000000000000000000, 0.9981185001348091834, 0.9964447847208420805 ) ) 
 REPRESENTATION_ITEM ( '' )  );
#80041=CARTESIAN_POINT ( 'NONE',  ( -0.03937007874015669567, -0.6692913385826771977, 8.415575281601705876E-17 ) ) ;
#80043=CARTESIAN_POINT ( 'NONE',  ( -0.7217847769028863381, -0.4281496062992124485, 0.4176697321401328655 ) ) ;
#80045=CARTESIAN_POINT ( 'NONE',  ( -1.581364829396324945, -0.3162353388693405765, 0.4822834645669290543 ) ) ;
#80046=CARTESIAN_POINT ( 'NONE',  ( -0.5380577427821514602, 0.05413385826771666132, 0.4176697321401328100 ) ) ;
#80047=CARTESIAN_POINT ( 'NONE',  ( -0.3871391076115476282, -0.08942795157527998196, 0.3641732283464567121 ) ) ;
#80048=CARTESIAN_POINT ( 'NONE',  ( 1.410761154855643795, -0.05778040916215560624, -0.4822834645669293319 ) ) ;
#80049=CARTESIAN_POINT ( 'NONE',  ( 1.666666666666667185, 0.05413385826771666132, 0.4176697321401328100 ) ) ;
#80050=CARTESIAN_POINT ( 'NONE',  ( -1.089238845144356427, 0.05413385826771666132, 0.4176697321401328100 ) ) ;
#80052=CARTESIAN_POINT ( 'NONE',  ( 0.8858267716535438430, -0.5400638737290845981, -0.3530559997133363437 ) ) ;
#80054=CARTESIAN_POINT ( 'NONE',  ( 1.614173228346457378, 1.055049524192302357, 0.1372047244094478369 ) ) ;
#80055=CARTESIAN_POINT ( 'NONE',  ( -0.09186351706036663400, -0.4281496062992124485, 0.4176697321401328655 ) ) ;
#80057=CARTESIAN_POINT ( 'NONE',  ( -0.9973753280839886548, 0.1283753931104748280, 0.1820866141732283561 ) ) ;
#80058=CARTESIAN_POINT ( 'NONE',  ( 0.5839895013123367340, 0.1771653543307087630, 0.09757992244046791164 ) ) ;
#80060=CARTESIAN_POINT ( 'NONE',  ( 1.102362204724410155, -0.1870078740157480601, -0.3641732283464567677 ) ) ;
#80062=CARTESIAN_POINT ( 'NONE',  ( 0.9186351706036751663, -0.6046776061558807314, 0.2411417322834647770 ) ) ;
#80064=CARTESIAN_POINT ( 'NONE',  ( -0.2690288713910754526, 0.2952755905511810774, -0.1292274648535930714 ) ) ;
#80066=CARTESIAN_POINT ( 'NONE',  ( 1.246719160104987623, -0.3690944881889763329, 0.3153832671262228327 ) ) ;
#80067=CARTESIAN_POINT ( 'NONE',  ( -0.3805774278215216522, -0.4281496062992127816, -0.4176697321401328100 ) ) ;
#80070=CARTESIAN_POINT ( 'NONE',  ( 1.305774278215223960, -0.6692913385826771977, 0.1292274648535927661 ) ) ;
#80071=CARTESIAN_POINT ( 'NONE',  ( 0.006561679790026889343, -0.05778040916215522460, 0.4822834645669289988 ) ) ;
#80072=CARTESIAN_POINT ( 'NONE',  ( 0.4330708661417329575, 0.1771653543307087630, 0.000000000000000000 ) ) ;
#80074=CARTESIAN_POINT ( 'NONE',  ( 0.4593175853018380828, -0.004921259842519870586, -0.3153832671262229437 ) ) ;
#80075=CARTESIAN_POINT ( 'NONE',  ( -1.062992125984250968, 0.2066929133858268208, 0.000000000000000000 ) ) ;
#80077=CARTESIAN_POINT ( 'NONE',  ( 0.6758530183727039509, -0.6692913385826771977, 0.1292274648535927661 ) ) ;
#80079=CARTESIAN_POINT ( 'NONE',  ( 1.450131233595801428, -0.5511811023622048555, -0.09757992244046775898 ) ) ;
#80081=CARTESIAN_POINT ( 'NONE',  ( 0.09186351706036799403, -0.3690944881889765550, -0.3153832671262227771 ) ) ;
#80082=CARTESIAN_POINT ( 'NONE',  ( 0.06561679790026316017, -0.4281496062992124485, 0.4176697321401328655 ) ) ;
#80083=CARTESIAN_POINT ( 'NONE',  ( 1.423884514435696413, -0.2845877964562161244, -0.3641732283464567121 ) ) ;
#80084=CARTESIAN_POINT ( 'NONE',  ( -1.391076115485563758, 0.1283753931104748280, 0.1820866141732283561 ) ) ;
#80085=CARTESIAN_POINT ( 'NONE',  ( -1.535433070866141225, 0.2952755905511811885, 0.000000000000000000 ) ) ;
#80086=CARTESIAN_POINT ( 'NONE',  ( 0.5971128608923891301, 0.2952755905511810774, -0.1292274648535930714 ) ) ;
#80087=CARTESIAN_POINT ( 'NONE',  ( 1.200787401574803681, 0.1660481256975885056, 0.3530559997133364547 ) ) ;
#80089=CARTESIAN_POINT ( 'NONE',  ( 0.4461942257217855201, -0.6046776061558807314, 0.2411417322834647770 ) ) ;
#80090=CARTESIAN_POINT ( 'NONE',  ( 1.253280839895013710, -0.05778040916215560624, -0.4822834645669293319 ) ) ;
#80091=CARTESIAN_POINT ( 'NONE',  ( 1.023622047244095334, -0.1870078740157479769, 0.4822834645669291653 ) ) ;
#80093=CARTESIAN_POINT ( 'NONE',  ( 0.7677165354330716118, 0.07958543189024071263, -0.2665933059059888421 ) ) ;
#80094=CARTESIAN_POINT ( 'NONE',  ( 1.581364829396326277, -0.3162353388693409650, -0.4822834645669289433 ) ) ;
#80095=CARTESIAN_POINT ( 'NONE',  ( -0.9842519685039360366, 0.1771653543307087630, 0.000000000000000000 ) ) ;
#80097=CARTESIAN_POINT ( 'NONE',  ( 0.3871391076115492380, -0.08942795157528024563, -0.3641732283464568787 ) ) ;
#80098=CARTESIAN_POINT ( 'NONE',  ( 0.2296587926509192634, -0.3162353388693405765, 0.4822834645669290543 ) ) ;
#80099=CARTESIAN_POINT ( 'NONE',  ( 0.6824146981627303710, 0.2306618581243847221, -0.2411417322834647770 ) ) ;
#80100=CARTESIAN_POINT ( 'NONE',  ( -0.4986876640419939388, 0.2306618581243847221, -0.2411417322834647770 ) ) ;
#80101=CARTESIAN_POINT ( 'NONE',  ( 0.2165354330708668673, 0.07958543189024071263, -0.2665933059059888421 ) ) ;
#80102=CARTESIAN_POINT ( 'NONE',  ( 0.7677165354330716118, -0.5400638737290844871, 0.3530559997133364547 ) ) ;
#80104=CARTESIAN_POINT ( 'NONE',  ( -0.7677165354330699465, 0.1660481256975885056, 0.3530559997133364547 ) ) ;
#80107=CARTESIAN_POINT ( 'NONE',  ( 1.011202504342157527, 9.477779430591278127E-17, -0.3464511005275205946 ) ) ;
#80108=CARTESIAN_POINT ( 'NONE',  ( -0.7742782152230962556, -0.4281496062992127816, -0.4176697321401328100 ) ) ;
#80110=CARTESIAN_POINT ( 'NONE',  ( -0.6430446194225716283, -0.4281496062992124485, 0.4176697321401328655 ) ) ;
#80113=ORIENTED_EDGE ( 'NONE', *, *, #55755, .F. ) ;
#80114=CARTESIAN_POINT ( 'NONE',  ( 0.7545931758530189937, 0.1771653543307087075, -0.09757992244046823083 ) ) ;
#80116=CARTESIAN_POINT ( 'NONE',  ( 1.181102362204724976, -0.1870078740157480879, -0.4822834645669291653 ) ) ;
#80117=CARTESIAN_POINT ( 'NONE',  ( 1.191111281560510715, -4.927456884911482678E-16, 0.4445507791589062840 ) ) ;
#80118=CARTESIAN_POINT ( 'NONE',  ( -1.345144356955379816, -0.08942795157528024563, -0.3641732283464568787 ) ) ;
#80119=CARTESIAN_POINT ( 'NONE',  ( 1.456692913385827515, -0.6692913385826771977, 8.415575281601705876E-17 ) ) ;
#80120=CARTESIAN_POINT ( 'NONE',  ( -1.463254593175852492, -0.6692913385826773087, -0.1292274648535924053 ) ) ;
#80121=CARTESIAN_POINT ( 'NONE',  ( 0.3543307086614181922, -0.6692913385826771977, 8.415575281601705876E-17 ) ) ;
#80123=CARTESIAN_POINT ( 'NONE',  ( 0.05905511811023709395, -0.5400638737290844871, 0.3530559997133364547 ) ) ;
#80124=CARTESIAN_POINT ( 'NONE',  ( -0.7086614173228339419, -0.1870078740157480601, -0.3641732283464567677 ) ) ;
#80125=CARTESIAN_POINT ( 'NONE',  ( 1.043307086614173818, -0.5400638737290845981, -0.3530559997133363437 ) ) ;
#80126=CARTESIAN_POINT ( 'NONE',  ( -0.01968503937007793844, -0.5400638737290844871, 0.3530559997133364547 ) ) ;
#80128=CARTESIAN_POINT ( 'NONE',  ( -0.01033912696139454093, 1.702998256715020864E-15, -0.4281989832122450323 ) ) ;
#80130=CARTESIAN_POINT ( 'NONE',  ( 1.036745406824147731, 0.05413385826771666132, 0.4176697321401328100 ) ) ;
#80131=CARTESIAN_POINT ( 'NONE',  ( 0.2755905511811031494, -0.6692913385826771977, 8.415575281601705876E-17 ) ) ;
#80132=CARTESIAN_POINT ( 'NONE',  ( -1.135170603674539924, 0.2952755905511810774, -0.1292274648535930714 ) ) ;
#80133=CARTESIAN_POINT ( 'NONE',  ( 1.240157480314961314, -0.5400638737290844871, 0.3530559997133364547 ) ) ;
#80134=CARTESIAN_POINT ( 'NONE',  ( 0.2755905511811031494, 0.2952755905511811885, 0.000000000000000000 ) ) ;
#80136=CARTESIAN_POINT ( 'NONE',  ( -0.2755905511811018171, 0.2952755905511811885, 0.000000000000000000 ) ) ;
#80137=CARTESIAN_POINT ( 'NONE',  ( 0.7020997375328090762, -0.3162353388693405765, 0.4822834645669290543 ) ) ;
#80138=CARTESIAN_POINT ( 'NONE',  ( 0.05249343832021075018, -0.6046776061558807314, 0.2411417322834647770 ) ) ;
#80139=CARTESIAN_POINT ( 'NONE',  ( 0.8661417322834653598, -0.1870078740157479769, 0.3641732283464567677 ) ) ;
#80140=CARTESIAN_POINT ( 'NONE',  ( -1.220472440944881054, 0.2952755905511811885, 0.000000000000000000 ) ) ;
#80142=CARTESIAN_POINT ( 'NONE',  ( 0.2165354330708668673, 0.1660481256975883668, -0.3530559997133364547 ) ) ;
#80143=( NAMED_UNIT ( * ) SI_UNIT ( $, .STERADIAN. ) SOLID_ANGLE_UNIT ( ) );
#80145=EDGE_LOOP ( 'NONE', ( #9422, #24299, #23559, #55057 ) ) ;
#80148=CARTESIAN_POINT ( 'NONE',  ( 1.082677165354331228, 0.1660481256975883668, -0.3530559997133364547 ) ) ;
#80149=CARTESIAN_POINT ( 'NONE',  ( 0.4855643044619428750, -0.004921259842519576551, 0.3153832671262227771 ) ) ;
#80150=VECTOR ( 'NONE', #22572, 39.37007874015748143 ) ;
#80152=LINE ( 'NONE', #15757, #1466 ) ;
#80156=EDGE_CURVE ( 'NONE', #25851, #34321, #38991, .T. ) ;
#80158=CARTESIAN_POINT ( 'NONE',  ( -0.9514435695538050464, -0.05778040916215560624, -0.4822834645669293319 ) ) ;
#80159=CARTESIAN_POINT ( 'NONE',  ( -0.6889763779527552368, -0.5400638737290845981, -0.3530559997133363437 ) ) ;
#80160=CARTESIAN_POINT ( 'NONE',  ( 0.6889763779527563470, 0.1660481256975883668, -0.3530559997133364547 ) ) ;
#80162=CARTESIAN_POINT ( 'NONE',  ( 1.535433070866142335, -0.6692913385826771977, 8.415575281601705876E-17 ) ) ;
#80163=CARTESIAN_POINT ( 'NONE',  ( 1.660104986876641320, -0.08942795157527998196, 0.3641732283464567121 ) ) ;
#80167=CARTESIAN_POINT ( 'NONE',  ( -1.240157480314959759, -0.4536011799217368745, -0.2665933059059886201 ) ) ;
#80169=CARTESIAN_POINT ( 'NONE',  ( 0.4849061582275016602, 2.793565526369266028, -0.4921425059946356595 ) ) ;
#80170=CARTESIAN_POINT ( 'NONE',  ( 0.04593175853018440641, -0.6692913385826771977, 0.1292274648535927661 ) ) ;
#80172=CARTESIAN_POINT ( 'NONE',  ( 1.371391076115485941, 0.2952755905511811885, 0.1292274648535926551 ) ) ;
#80174=CARTESIAN_POINT ( 'NONE',  ( -1.299212598425196097, -0.5511811023622047445, 6.969142054262312111E-17 ) ) ;
#80175=CARTESIAN_POINT ( 'NONE',  ( 0.9645669291338591078, -0.5400638737290845981, -0.3530559997133363437 ) ) ;
#80176=CARTESIAN_POINT ( 'NONE',  ( 1.272965879265092637, -0.004921259842519576551, 0.3153832671262227771 ) ) ;
#80178=CARTESIAN_POINT ( 'NONE',  ( -1.154855643044618851, -0.5023911411419708095, -0.1820866141732282451 ) ) ;
#80179=CARTESIAN_POINT ( 'NONE',  ( 1.299212598425197429, -0.6692913385826771977, 8.415575281601705876E-17 ) ) ;
#80181=CARTESIAN_POINT ( 'NONE',  ( -0.1312335958005241554, 0.2306618581243848609, 0.2411417322834645549 ) ) ;
#80182=CARTESIAN_POINT ( 'NONE',  ( -1.141732283464566011, 0.1771653543307087630, 0.000000000000000000 ) ) ;
#80183=CARTESIAN_POINT ( 'NONE',  ( -0.3280839895013117347, -0.3690944881889763329, 0.3153832671262228327 ) ) ;
#80184=CARTESIAN_POINT ( 'NONE',  ( -0.6758530183727028406, -0.6692913385826773087, -0.1292274648535924053 ) ) ;
#80185=CARTESIAN_POINT ( 'NONE',  ( -1.620734908136482577, 0.1771653543307087630, 0.09757992244046791164 ) ) ;
#80187=CARTESIAN_POINT ( 'NONE',  ( 0.2755905511811031494, -0.6692913385826771977, 8.415575281601705876E-17 ) ) ;
#80190=CARTESIAN_POINT ( 'NONE',  ( -1.325459317585300889, -0.4281496062992127816, -0.4176697321401328100 ) ) ;
#80191=CARTESIAN_POINT ( 'NONE',  ( -0.6233595800524928121, -0.08942795157527998196, 0.3641732283464567121 ) ) ;
#80192=CARTESIAN_POINT ( 'NONE',  ( -0.01312335958005186876, 0.05413385826771626580, -0.4176697321401330321 ) ) ;
#80193=CARTESIAN_POINT ( 'NONE',  ( 0.4330708661417329575, 0.1771653543307087630, 0.000000000000000000 ) ) ;
#80194=CARTESIAN_POINT ( 'NONE',  ( -0.9120734908136475250, 0.1771653543307087630, 0.09757992244046791164 ) ) ;
#80195=CARTESIAN_POINT ( 'NONE',  ( -1.292650918635170010, -0.6692913385826771977, 0.1292274648535927661 ) ) ;
#80196=CARTESIAN_POINT ( 'NONE',  ( -1.719160104986876103, 0.05413385826771666132, 0.4176697321401328100 ) ) ;
#80197=CARTESIAN_POINT ( 'NONE',  ( 1.568241469816273659, -0.05778040916215560624, -0.4822834645669293319 ) ) ;
#80199=CARTESIAN_POINT ( 'NONE',  ( 0.9383202099737538715, -0.08942795157528024563, -0.3641732283464568787 ) ) ;
#80200=CARTESIAN_POINT ( 'NONE',  ( 0.9120734908136490793, 0.2952755905511810774, -0.1292274648535930714 ) ) ;
#80201=CARTESIAN_POINT ( 'NONE',  ( -0.5387615594602663815, -2.294479370626195693E-15, 0.3464511005275217603 ) ) ;
#80202=CARTESIAN_POINT ( 'NONE',  ( 1.423884514435696191, -0.08942795157527998196, 0.3641732283464567121 ) ) ;
#80204=CARTESIAN_POINT ( 'NONE',  ( -0.6824146981627288167, 0.2306618581243848609, 0.2411417322834645549 ) ) ;
#80205=CARTESIAN_POINT ( 'NONE',  ( -0.7414698162729651543, -0.6692913385826771977, 0.1292274648535927661 ) ) ;
#80206=CARTESIAN_POINT ( 'NONE',  ( 0.4855643044619428750, 0.05413385826771666132, 0.4176697321401328100 ) ) ;
#80207=VECTOR ( 'NONE', #14436, 39.37007874015748143 ) ;
#80208=CARTESIAN_POINT ( 'NONE',  ( -1.496062992125983815, -0.1870078740157480601, -0.3641732283464567677 ) ) ;
#80210=CARTESIAN_POINT ( 'NONE',  ( -1.633858267716534529, -0.5400638737290845981, -0.3530559997133363437 ) ) ;
#80211=CONICAL_SURFACE ( 'NONE', #15683, 1.181102362204724310, 0.7853981633974552734 ) ;
#80212=CARTESIAN_POINT ( 'NONE',  ( 0.2821522309711292364, 0.2952755905511810774, -0.1292274648535930714 ) ) ;
#80213=CARTESIAN_POINT ( 'NONE',  ( 0.8333333333333340365, 0.2952755905511810774, -0.1292274648535930714 ) ) ;
#80214=CARTESIAN_POINT ( 'NONE',  ( -1.595398199321656385, 1.288687073698533414, -0.1559797534342482195 ) ) ;
#80220=CARTESIAN_POINT ( 'NONE',  ( 0.05905511811023681640, 0.07958543189024071263, -0.2665933059059888421 ) ) ;
#80221=CARTESIAN_POINT ( 'NONE',  ( -0.3412073490813641308, -0.6046776061558807314, 0.2411417322834647770 ) ) ;
#80222=CARTESIAN_POINT ( 'NONE',  ( 0.6889763779527563470, 0.1660481256975883668, -0.3530559997133364547 ) ) ;
#80224=CARTESIAN_POINT ( 'NONE',  ( 0.02624671916010564918, -0.5023911411419708095, -0.1820866141732282451 ) ) ;
#80225=CARTESIAN_POINT ( 'NONE',  ( -1.358267716535432434, -0.5400638737290844871, 0.3530559997133364547 ) ) ;
#80226=CARTESIAN_POINT ( 'NONE',  ( 1.181102362204724976, -0.1870078740157480879, -0.4822834645669291653 ) ) ;
#80229=CARTESIAN_POINT ( 'NONE',  ( 0.08874907683610111508, -2.191421614605370878E-15, 0.4445507791589071167 ) ) ;
#80230=AXIS2_PLACEMENT_3D ( 'NONE', #40178, #73421, #54453 ) ;
#80231=EDGE_LOOP ( 'NONE', ( #37843, #76487, #53817, #18106 ) ) ;
#80232=ORIENTED_EDGE ( 'NONE', *, *, #49009, .T. ) ;
#80233=CARTESIAN_POINT ( 'NONE',  ( 0.8464566929133865436, 0.1660481256975883668, -0.3530559997133364547 ) ) ;
#80234=CARTESIAN_POINT ( 'NONE',  ( -1.515748031496062076, 0.1660481256975883668, -0.3530559997133364547 ) ) ;
#80235=CARTESIAN_POINT ( 'NONE',  ( -1.272965879265091305, -0.004921259842519870586, -0.3153832671262229437 ) ) ;
#80236=CARTESIAN_POINT ( 'NONE',  ( 1.489501312335958172, -0.05778040916215560624, -0.4822834645669293319 ) ) ;
#80238=CARTESIAN_POINT ( 'NONE',  ( 1.220472440944882164, -0.1870078740157480046, 1.254653134982923898E-17 ) ) ;
#80239=CARTESIAN_POINT ( 'NONE',  ( 1.437007874015748810, -0.5400638737290845981, -0.3530559997133363437 ) ) ;
#80240=CARTESIAN_POINT ( 'NONE',  ( -1.679790026246718693, 0.2306618581243847221, -0.2411417322834647770 ) ) ;
#80241=CARTESIAN_POINT ( 'NONE',  ( 0.01312335958005323398, 0.05413385826771666132, 0.4176697321401328100 ) ) ;
#80242=CARTESIAN_POINT ( 'NONE',  ( -0.6561679790026240244, -0.6046776061558807314, 0.2411417322834647770 ) ) ;
#80243=CARTESIAN_POINT ( 'NONE',  ( 1.522309711286089939, -0.6046776061558809534, -0.2411417322834644161 ) ) ;
#80246=CARTESIAN_POINT ( 'NONE',  ( 0.1246719160104994284, -0.6692913385826771977, 0.1292274648535927661 ) ) ;
#80248=CARTESIAN_POINT ( 'NONE',  ( -1.115485564304461219, -0.004921259842519870586, -0.3153832671262229437 ) ) ;
#80253=CARTESIAN_POINT ( 'NONE',  ( -1.463254593175852492, -0.6692913385826773087, -0.1292274648535924053 ) ) ;
#80255=CARTESIAN_POINT ( 'NONE',  ( -1.614173228346457378, 2.094556775020298023, 0.1372047244094476981 ) ) ;
#80256=CARTESIAN_POINT ( 'NONE',  ( -1.548556430446193399, 0.2306618581243848609, 0.2411417322834645549 ) ) ;
#80258=DIRECTION ( 'NONE',  ( 0.000000000000000000, 1.000000000000000000, 0.000000000000000000 ) ) ;
#80260=CARTESIAN_POINT ( 'NONE',  ( -0.4921259842519677963, 0.07958543189024071263, -0.2665933059059888421 ) ) ;
#80261=CARTESIAN_POINT ( 'NONE',  ( -0.8005249343832013809, -0.3690944881889763329, 0.3153832671262228327 ) ) ;
#80262=CARTESIAN_POINT ( 'NONE',  ( -1.364829396325458521, -0.6046776061558807314, 0.2411417322834647770 ) ) ;
#80263=CARTESIAN_POINT ( 'NONE',  ( 0.5774278215223103139, -0.6046776061558809534, -0.2411417322834644161 ) ) ;
#80264=CARTESIAN_POINT ( 'NONE',  ( -1.141732283464566011, 0.2952755905511811885, 0.000000000000000000 ) ) ;
#80267=CARTESIAN_POINT ( 'NONE',  ( -1.318897637795274802, 0.1660481256975885056, 0.3530559997133364547 ) ) ;
#80274=CARTESIAN_POINT ( 'NONE',  ( 0.4687364453271865017, 1.550612376216477184, -0.5180075785470105165 ) ) ;
#80275=CARTESIAN_POINT ( 'NONE',  ( -0.8661417322834640276, -0.1870078740157479769, 0.4822834645669291653 ) ) ;
#80276=CARTESIAN_POINT ( 'NONE',  ( 1.482939632545932307, -0.4281496062992124485, 0.4176697321401328655 ) ) ;
#80278=CARTESIAN_POINT ( 'NONE',  ( -1.581364829396324945, -0.3162353388693405765, 0.4822834645669290543 ) ) ;
#80280=CARTESIAN_POINT ( 'NONE',  ( -1.482939632545930975, -0.4281496062992127816, -0.4176697321401328100 ) ) ;
#80281=CARTESIAN_POINT ( 'NONE',  ( -0.9973753280839886548, -0.6046776061558809534, -0.2411417322834644161 ) ) ;
#80283=CARTESIAN_POINT ( 'NONE',  ( 0.2821522309711292364, -0.5511811023622046335, 0.09757992244046803654 ) ) ;
#80285=CARTESIAN_POINT ( 'NONE',  ( 0.04593175853018440641, -0.5511811023622046335, 0.09757992244046803654 ) ) ;
#80286=CARTESIAN_POINT ( 'NONE',  ( 0.8989501312335963501, -0.5511811023622048555, -0.09757992244046775898 ) ) ;
#80287=CARTESIAN_POINT ( 'NONE',  ( 0.8989501312335963501, -0.6692913385826773087, -0.1292274648535924053 ) ) ;
#80288=CARTESIAN_POINT ( 'NONE',  ( -0.2559055118110227234, -0.4536011799217367080, 0.2665933059059888421 ) ) ;
#80290=CARTESIAN_POINT ( 'NONE',  ( 1.555118110236221041, -0.5400638737290844871, 0.3530559997133364547 ) ) ;
#80291=CARTESIAN_POINT ( 'NONE',  ( -1.338582677165353729, -0.1870078740157479769, 0.3641732283464567677 ) ) ;
#80293=CARTESIAN_POINT ( 'NONE',  ( -0.09186351706036689768, 0.05413385826771626580, -0.4176697321401330321 ) ) ;
#80294=CARTESIAN_POINT ( 'NONE',  ( 0.06561679790026316017, -0.4281496062992124485, 0.4176697321401328655 ) ) ;
#80295=CARTESIAN_POINT ( 'NONE',  ( 1.502624671916010790, -0.08942795157527998196, 0.3641732283464567121 ) ) ;
#80296=CARTESIAN_POINT ( 'NONE',  ( 0.5971128608923890191, -0.5511811023622046335, 0.09757992244046803654 ) ) ;
#80297=CARTESIAN_POINT ( 'NONE',  ( -0.1443569553805768291, -0.004921259842519576551, 0.3153832671262227771 ) ) ;
#80298=CARTESIAN_POINT ( 'NONE',  ( -0.6233595800524928121, -0.3162353388693409650, -0.4822834645669289433 ) ) ;
#80301=CARTESIAN_POINT ( 'NONE',  ( 0.03280839895013198948, -0.6692913385826773087, -0.1292274648535924053 ) ) ;
#80303=CARTESIAN_POINT ( 'NONE',  ( 1.568241469816273437, -0.3162353388693405765, 0.4822834645669290543 ) ) ;
#80304=CARTESIAN_POINT ( 'NONE',  ( -0.3937007874015740483, -0.1870078740157480601, -0.3641732283464567677 ) ) ;
#80305=CARTESIAN_POINT ( 'NONE',  ( -0.09842519685039295696, 0.1660481256975883668, -0.3530559997133364547 ) ) ;
#80306=CARTESIAN_POINT ( 'NONE',  ( -1.377952755905511140, -0.6692913385826771977, 8.415575281601705876E-17 ) ) ;
#80307=CARTESIAN_POINT ( 'NONE',  ( 1.627296587926509996, -0.6046776061558807314, 0.2411417322834647770 ) ) ;
#80308=CARTESIAN_POINT ( 'NONE',  ( 1.332020997375329197, -0.3162353388693405765, 0.4822834645669290543 ) ) ;
#80310=CARTESIAN_POINT ( 'NONE',  ( -0.6167979002624665030, -0.004921259842519576551, 0.3153832671262227771 ) ) ;
#80314=CARTESIAN_POINT ( 'NONE',  ( 1.430446194225722500, -0.3690944881889765550, -0.3153832671262227771 ) ) ;
#80315=CARTESIAN_POINT ( 'NONE',  ( 1.272965879265092637, -0.004921259842519576551, 0.3153832671262227771 ) ) ;
#80316=CARTESIAN_POINT ( 'NONE',  ( -1.686351706036744558, 0.2952755905511810774, -0.1292274648535930714 ) ) ;
#80317=CARTESIAN_POINT ( 'NONE',  ( 0.6955380577427828781, 0.05413385826771626580, -0.4176697321401330321 ) ) ;
#80319=CARTESIAN_POINT ( 'NONE',  ( 1.049868766404200349, 0.1283753931104748280, 0.1820866141732283561 ) ) ;
#80320=CARTESIAN_POINT ( 'NONE',  ( 0.1115485564304470323, 0.2952755905511811885, 0.1292274648535926551 ) ) ;
#80321=CARTESIAN_POINT ( 'NONE',  ( -0.9711286089238838626, 0.2306618581243847221, -0.2411417322834647770 ) ) ;
#80322=CARTESIAN_POINT ( 'NONE',  ( 1.660104986876641320, -0.05778040916215522460, 0.4822834645669289988 ) ) ;
#80327=CARTESIAN_POINT ( 'NONE',  ( 0.4658792650918640033, -0.2845877964562159024, 0.3641732283464567677 ) ) ;
#80331=CARTESIAN_POINT ( 'NONE',  ( -0.2493438320209966919, 0.05413385826771626580, -0.4176697321401330321 ) ) ;
#80332=CARTESIAN_POINT ( 'NONE',  ( -0.3608923884514428360, 0.2952755905511811885, 0.1292274648535926551 ) ) ;
#80333=CARTESIAN_POINT ( 'NONE',  ( -0.4921259842519677963, 0.07958543189024071263, -0.2665933059059888421 ) ) ;
#80334=CARTESIAN_POINT ( 'NONE',  ( 0.8727034120734913358, -0.05778040916215522460, 0.4822834645669289988 ) ) ;
#80335=CARTESIAN_POINT ( 'NONE',  ( -1.043307086614172041, -0.5400638737290844871, 0.3530559997133364547 ) ) ;
#80336=CARTESIAN_POINT ( 'NONE',  ( -0.2755905511811018171, 0.2952755905511811885, 0.000000000000000000 ) ) ;
#80337=CARTESIAN_POINT ( 'NONE',  ( 1.030183727034121421, -0.3162353388693409650, -0.4822834645669289433 ) ) ;
#80339=CARTESIAN_POINT ( 'NONE',  ( 0.9514435695538062676, -0.05778040916215522460, 0.4822834645669289988 ) ) ;
#80340=B_SPLINE_CURVE_WITH_KNOTS ( 'NONE', 3,
 ( #79360, #33894, #7391, #66305 ),
 .UNSPECIFIED., .F., .F.,
 ( 4, 4 ),
 ( 0.1090648859799403791, 0.1105484317322390914 ),
 .UNSPECIFIED. ) ;
#80341=CARTESIAN_POINT ( 'NONE',  ( 0.8333333333333340365, -0.6692913385826771977, 0.1292274648535927661 ) ) ;
#80343=CARTESIAN_POINT ( 'NONE',  ( -0.1706036745406816491, -0.004921259842519870586, -0.3153832671262229437 ) ) ;
#80347=CARTESIAN_POINT ( 'NONE',  ( -0.8136482939632537770, -0.5023911411419708095, 0.1820866141732285504 ) ) ;
#80348=CARTESIAN_POINT ( 'NONE',  ( -0.4724409448818890911, -0.1870078740157480879, -0.4822834645669291653 ) ) ;
#80350=CARTESIAN_POINT ( 'NONE',  ( -0.4330708661417315697, 0.2952755905511811885, 0.000000000000000000 ) ) ;
#80351=CARTESIAN_POINT ( 'NONE',  ( -0.3215223097112853146, -0.3162353388693405765, 0.4822834645669290543 ) ) ;
#80352=CARTESIAN_POINT ( 'NONE',  ( -1.102362204724408601, -0.1870078740157480879, -0.4822834645669291653 ) ) ;
#80353=CARTESIAN_POINT ( 'NONE',  ( -1.581364829396324945, -0.3162353388693405765, 0.4822834645669290543 ) ) ;
#80354=CARTESIAN_POINT ( 'NONE',  ( 0.8398950131233602345, -0.5023911411419708095, 0.1820866141732285504 ) ) ;
#80357=CARTESIAN_POINT ( 'NONE',  ( 0.5708661417322841158, -0.4536011799217368745, -0.2665933059059886201 ) ) ;
#80358=CARTESIAN_POINT ( 'NONE',  ( -0.08530183727034056085, -0.3162353388693405765, 0.4822834645669290543 ) ) ;
#80359=CARTESIAN_POINT ( 'NONE',  ( 0.3543307086614181922, -0.6692913385826771977, 8.415575281601705876E-17 ) ) ;
#80365=CARTESIAN_POINT ( 'NONE',  ( 1.574803149606299746, -0.1870078740157479769, 0.4822834645669291653 ) ) ;
#80366=CARTESIAN_POINT ( 'NONE',  ( -0.6102362204724400829, 0.07958543189024085140, 0.2665933059059887866 ) ) ;
#80367=CARTESIAN_POINT ( 'NONE',  ( -0.9448818897637790704, -0.1870078740157479769, 0.4822834645669291653 ) ) ;
#80370=CARTESIAN_POINT ( 'NONE',  ( 1.535433070866142558, 0.2952755905511811885, 0.000000000000000000 ) ) ;
#80371=CARTESIAN_POINT ( 'NONE',  ( 0.6627296587926515548, 0.2952755905511811885, 0.1292274648535926551 ) ) ;
#80372=CARTESIAN_POINT ( 'NONE',  ( 0.7217847769028878924, 0.05413385826771666132, 0.4176697321401328100 ) ) ;
#80373=CARTESIAN_POINT ( 'NONE',  ( -0.4790026246719152336, -0.08942795157528024563, -0.3641732283464568787 ) ) ;
#80374=CARTESIAN_POINT ( 'NONE',  ( 0.006561679790026889343, -0.05778040916215522460, 0.4822834645669289988 ) ) ;
#80376=CARTESIAN_POINT ( 'NONE',  ( -0.4068241469816264999, -0.3690944881889763329, 0.3153832671262228327 ) ) ;
#80377=CARTESIAN_POINT ( 'NONE',  ( -0.2887139107611542133, 0.2306618581243848609, 0.2411417322834645549 ) ) ;
#80379=CARTESIAN_POINT ( 'NONE',  ( -1.430446194225721390, -0.4281496062992124485, 0.4176697321401328655 ) ) ;
#80380=CARTESIAN_POINT ( 'NONE',  ( 0.2165354330708668673, 0.07958543189024071263, -0.2665933059059888421 ) ) ;
#80381=CARTESIAN_POINT ( 'NONE',  ( 1.502624671916010790, -0.08942795157527998196, 0.3641732283464567121 ) ) ;
#80382=CARTESIAN_POINT ( 'NONE',  ( -1.167979002624671470, -0.4281496062992127816, -0.4176697321401328100 ) ) ;
#80383=EDGE_CURVE ( 'NONE', #74430, #74087, #62517, .T. ) ;
#80384=CARTESIAN_POINT ( 'NONE',  ( -0.9186351706036736120, -0.5023911411419708095, -0.1820866141732282451 ) ) ;
#80386=CARTESIAN_POINT ( 'NONE',  ( -1.227034120734907585, 0.2952755905511811885, 0.1292274648535926551 ) ) ;
#80387=CARTESIAN_POINT ( 'NONE',  ( -0.5314960629921250401, 0.1660481256975885056, 0.3530559997133364547 ) ) ;
#80388=CARTESIAN_POINT ( 'NONE',  ( 0.3215223097112867578, -0.3162353388693409650, -0.4822834645669289433 ) ) ;
#80392=CARTESIAN_POINT ( 'NONE',  ( 0.3937007874015754361, -0.1870078740157479769, 0.3641732283464567677 ) ) ;
#80393=CARTESIAN_POINT ( 'NONE',  ( 1.181102362204724976, -0.1870078740157480879, -0.4822834645669291653 ) ) ;
#80394=CARTESIAN_POINT ( 'NONE',  ( -1.049868766404198794, 0.1283753931104746893, -0.1820866141732285504 ) ) ;
#80395=CARTESIAN_POINT ( 'NONE',  ( 0.9842519685039378130, -0.6692913385826771977, 8.415575281601705876E-17 ) ) ;
#80396=CARTESIAN_POINT ( 'NONE',  ( -1.712598425196849572, 0.07958543189024085140, 0.2665933059059887866 ) ) ;
#80397=CARTESIAN_POINT ( 'NONE',  ( -0.3805774278215216522, -0.4281496062992127816, -0.4176697321401328100 ) ) ;
#80398=CARTESIAN_POINT ( 'NONE',  ( 0.3346456692913393205, -0.4536011799217368745, -0.2665933059059886201 ) ) ;
#80399=CARTESIAN_POINT ( 'NONE',  ( -0.8478501267249328732, 2.401574803149606474, -0.8478501267249377582 ) ) ;
#80400=CARTESIAN_POINT ( 'NONE',  ( 0.7414698162729663755, -0.5511811023622048555, -0.09757992244046775898 ) ) ;
#80401=CARTESIAN_POINT ( 'NONE',  ( -0.01968503937007793844, 0.1660481256975883668, -0.3530559997133364547 ) ) ;
#80402=EDGE_CURVE ( 'NONE', #5694, #38486, #6286, .T. ) ;
#80404=CARTESIAN_POINT ( 'NONE',  ( -1.279527559055116948, -0.5400638737290844871, 0.3530559997133364547 ) ) ;
#80406=CARTESIAN_POINT ( 'NONE',  ( 1.135170603674541256, 0.1771653543307087630, 0.09757992244046791164 ) ) ;
#80407=CARTESIAN_POINT ( 'NONE',  ( -0.08530183727034056085, -0.3162353388693405765, 0.4822834645669290543 ) ) ;
#80408=CARTESIAN_POINT ( 'NONE',  ( -0.1837270341207340729, 0.2306618581243847221, -0.2411417322834647770 ) ) ;
#80409=CARTESIAN_POINT ( 'NONE',  ( -0.4068241469816264999, -0.3690944881889763329, 0.3153832671262228327 ) ) ;
#80410=CARTESIAN_POINT ( 'NONE',  ( 1.011202504342157527, 9.477779430591278127E-17, -0.3464511005275205946 ) ) ;
#80411=CARTESIAN_POINT ( 'NONE',  ( -0.6561679790026240244, 0.1283753931104746893, -0.1820866141732285504 ) ) ;
#80412=CARTESIAN_POINT ( 'NONE',  ( 0.1706036745406830368, -0.4281496062992127816, -0.4176697321401328100 ) ) ;
#80413=CARTESIAN_POINT ( 'NONE',  ( -0.9908136482939626788, -0.5511811023622048555, -0.09757992244046775898 ) ) ;
#80415=CARTESIAN_POINT ( 'NONE',  ( -1.325459317585300889, 0.05413385826771666132, 0.4176697321401328100 ) ) ;
#80417=ORIENTED_EDGE ( 'NONE', *, *, #5930, .F. ) ;
#80418=CARTESIAN_POINT ( 'NONE',  ( -0.8537221893815262197, -2.294479370626195693E-15, 0.3464511005275217603 ) ) ;
#80419=CARTESIAN_POINT ( 'NONE',  ( -0.4986876640419942164, -0.6046776061558807314, 0.2411417322834647770 ) ) ;
#80420=EDGE_CURVE ( 'NONE', #43326, #78909, #81895, .T. ) ;
#80422=CARTESIAN_POINT ( 'NONE',  ( -1.108923884514435132, -0.05778040916215560624, -0.4822834645669293319 ) ) ;
#80425=CARTESIAN_POINT ( 'NONE',  ( 1.450131233595801428, -0.6692913385826773087, -0.1292274648535924053 ) ) ;
#80426=CARTESIAN_POINT ( 'NONE',  ( 0.4790026246719168435, -0.3162353388693409650, -0.4822834645669289433 ) ) ;
#80429=CARTESIAN_POINT ( 'NONE',  ( -1.574803149606298636, -0.1870078740157479769, 0.4822834645669291653 ) ) ;
#80431=ORIENTED_EDGE ( 'NONE', *, *, #21875, .F. ) ;
#80432=CARTESIAN_POINT ( 'NONE',  ( -1.049868766404198794, -0.5023911411419708095, 0.1820866141732285504 ) ) ;
#80435=CARTESIAN_POINT ( 'NONE',  ( 0.6627296587926515548, 0.2952755905511811885, 0.1292274648535926551 ) ) ;
#80436=CARTESIAN_POINT ( 'NONE',  ( -0.4724409448818890911, -0.1870078740157479769, 0.4822834645669291653 ) ) ;
#80437=CARTESIAN_POINT ( 'NONE',  ( -1.062992125984250968, -0.6692913385826771977, 8.415575281601705876E-17 ) ) ;
#80438=CARTESIAN_POINT ( 'NONE',  ( 1.240157480314961314, 0.1660481256975883668, -0.3530559997133364547 ) ) ;
#80439=CARTESIAN_POINT ( 'NONE',  ( -1.286089238845143479, 0.1283753931104746893, -0.1820866141732285504 ) ) ;
#80441=CARTESIAN_POINT ( 'NONE',  ( 0.2034120734908144990, -0.6692913385826771977, 0.1292274648535927661 ) ) ;
#80442=CARTESIAN_POINT ( 'NONE',  ( -0.9383202099737524282, -0.3162353388693409650, -0.4822834645669289433 ) ) ;
#80444=CARTESIAN_POINT ( 'NONE',  ( -1.122047244094487306, 0.1660481256975883668, -0.3530559997133364547 ) ) ;
#80446=CARTESIAN_POINT ( 'NONE',  ( 0.8398950131233602345, -0.6046776061558807314, 0.2411417322834647770 ) ) ;
#80447=CARTESIAN_POINT ( 'NONE',  ( 1.292650918635171564, -0.5511811023622048555, -0.09757992244046775898 ) ) ;
#80450=CARTESIAN_POINT ( 'NONE',  ( -0.5839895013123351797, -0.6692913385826771977, 0.1292274648535927661 ) ) ;
#80453=CARTESIAN_POINT ( 'NONE',  ( 0.3871391076115492380, -0.08942795157528024563, -0.3641732283464568787 ) ) ;
#80454=CARTESIAN_POINT ( 'NONE',  ( -1.587926509186350810, -0.4281496062992124485, 0.4176697321401328655 ) ) ;
#80455=CARTESIAN_POINT ( 'NONE',  ( 0.8464566929133865436, 0.1660481256975883668, -0.3530559997133364547 ) ) ;
#80456=CARTESIAN_POINT ( 'NONE',  ( 0.6824146981627303710, 0.2306618581243847221, -0.2411417322834647770 ) ) ;
#80457=CARTESIAN_POINT ( 'NONE',  ( -0.3543307086614165824, -0.6692913385826771977, 8.415575281601705876E-17 ) ) ;
#80459=CARTESIAN_POINT ( 'NONE',  ( -0.7808398950131222316, -0.3162353388693409650, -0.4822834645669289433 ) ) ;
#80461=CARTESIAN_POINT ( 'NONE',  ( -1.476377952755905110, -0.5400638737290845981, -0.3530559997133363437 ) ) ;
#80462=CARTESIAN_POINT ( 'NONE',  ( -0.9514435695538050464, -0.05778040916215560624, -0.4822834645669293319 ) ) ;
#80463=CARTESIAN_POINT ( 'NONE',  ( 1.141732283464567788, -0.6692913385826771977, 8.415575281601705876E-17 ) ) ;
#80464=CARTESIAN_POINT ( 'NONE',  ( 1.679790026246720025, 0.2306618581243848609, 0.2411417322834645549 ) ) ;
#80465=CARTESIAN_POINT ( 'NONE',  ( -0.7742782152230965886, 0.05413385826771666132, 0.4176697321401328100 ) ) ;
#80467=CARTESIAN_POINT ( 'NONE',  ( 0.4986876640419954376, 0.2306618581243848609, 0.2411417322834645549 ) ) ;
#80469=CARTESIAN_POINT ( 'NONE',  ( -0.5183727034120726440, 0.2952755905511811885, 0.1292274648535926551 ) ) ;
#80470=CARTESIAN_POINT ( 'NONE',  ( 1.574803149606299746, -0.1870078740157480879, -0.4822834645669291653 ) ) ;
#80471=CARTESIAN_POINT ( 'NONE',  ( 0.4790026246719168435, -0.2845877964562161244, -0.3641732283464567121 ) ) ;
#80472=CARTESIAN_POINT ( 'NONE',  ( 1.312335958005249825, 0.2306618581243847221, -0.2411417322834647770 ) ) ;
#80474=CARTESIAN_POINT ( 'NONE',  ( 0.9973753280839902091, -0.5023911411419708095, 0.1820866141732285504 ) ) ;
#80475=CARTESIAN_POINT ( 'NONE',  ( 0.6364829396325465405, -0.05778040916215522460, 0.4822834645669289988 ) ) ;
#80477=CARTESIAN_POINT ( 'NONE',  ( -0.5511811023622041894, -0.1870078740157480879, -0.4822834645669291653 ) ) ;
#80478=CARTESIAN_POINT ( 'NONE',  ( 1.207349081364829990, -0.5023911411419708095, -0.1820866141732282451 ) ) ;
#80479=CARTESIAN_POINT ( 'NONE',  ( -0.6364829396325453192, -0.3162353388693405765, 0.4822834645669290543 ) ) ;
#80481=CARTESIAN_POINT ( 'NONE',  ( 1.364829396325460076, 0.2306618581243848609, 0.2411417322834645549 ) ) ;
#80482=CARTESIAN_POINT ( 'NONE',  ( 0.2821522309711292364, -0.6692913385826771977, 0.1292274648535927661 ) ) ;
#80483=CARTESIAN_POINT ( 'NONE',  ( 0.3740157480314966754, -0.4536011799217367080, 0.2665933059059888421 ) ) ;
#80485=CARTESIAN_POINT ( 'NONE',  ( -0.06561679790026180015, -0.004921259842519576551, 0.3153832671262227771 ) ) ;
#80486=CARTESIAN_POINT ( 'NONE',  ( 0.8333333333333340365, 0.1771653543307087075, -0.09757992244046823083 ) ) ;
#80487=CARTESIAN_POINT ( 'NONE',  ( -1.548556430446193399, -0.6046776061558809534, -0.2411417322834644161 ) ) ;
#80489=CARTESIAN_POINT ( 'NONE',  ( 0.8005249343832028242, -0.4281496062992127816, -0.4176697321401328100 ) ) ;
#80492=DIRECTION ( 'NONE',  ( 0.000000000000000000, 0.000000000000000000, 1.000000000000000000 ) ) ;
#80493=CARTESIAN_POINT ( 'NONE',  ( 0.1312335958005255154, -0.5023911411419708095, 0.1820866141732285504 ) ) ;
#80494=CARTESIAN_POINT ( 'NONE',  ( 0.1837270341207357105, -0.6046776061558809534, -0.2411417322834644161 ) ) ;
#80495=CARTESIAN_POINT ( 'NONE',  ( 1.522309711286089939, 0.1283753931104748280, 0.1820866141732283561 ) ) ;
#80496=CARTESIAN_POINT ( 'NONE',  ( -1.430446194225721390, -0.3690944881889763329, 0.3153832671262228327 ) ) ;
#80497=CARTESIAN_POINT ( 'NONE',  ( -1.423884514435694859, -0.3162353388693405765, 0.4822834645669290543 ) ) ;
#80498=CARTESIAN_POINT ( 'NONE',  ( 0.5249343832021005074, -0.6046776061558807314, 0.2411417322834647770 ) ) ;
#80499=CARTESIAN_POINT ( 'NONE',  ( 1.062992125984252745, 0.2952755905511811885, 0.000000000000000000 ) ) ;
#80501=CARTESIAN_POINT ( 'NONE',  ( 0.2887139107611556010, -0.6046776061558807314, 0.2411417322834647770 ) ) ;
#80502=CARTESIAN_POINT ( 'NONE',  ( 1.128608923884515169, -0.6046776061558809534, -0.2411417322834644161 ) ) ;
#80503=CARTESIAN_POINT ( 'NONE',  ( 1.030183727034121421, -0.05778040916215522460, 0.4822834645669289988 ) ) ;
#80506=CARTESIAN_POINT ( 'NONE',  ( 0.6496062992125991586, -0.4536011799217368745, -0.2665933059059886201 ) ) ;
#80507=CARTESIAN_POINT ( 'NONE',  ( 1.522309711286089939, 0.2306618581243848609, 0.2411417322834645549 ) ) ;
#80508=CARTESIAN_POINT ( 'NONE',  ( -0.09186351706036689768, -0.004921259842519870586, -0.3153832671262229437 ) ) ;
#80509=CARTESIAN_POINT ( 'NONE',  ( -0.05249343832020911260, 0.2306618581243848609, 0.2411417322834645549 ) ) ;
#80510=CARTESIAN_POINT ( 'NONE',  ( 0.5380577427821529035, 0.05413385826771626580, -0.4176697321401330321 ) ) ;
#80511=CARTESIAN_POINT ( 'NONE',  ( -0.3871391076115476282, -0.05778040916215522460, 0.4822834645669289988 ) ) ;
#80512=CARTESIAN_POINT ( 'NONE',  ( -0.2493438320209966919, -0.004921259842519870586, -0.3153832671262229437 ) ) ;
#80513=CARTESIAN_POINT ( 'NONE',  ( 0.7808398950131240079, -0.3162353388693405765, 0.4822834645669290543 ) ) ;
#80514=CARTESIAN_POINT ( 'NONE',  ( 1.115485564304462551, -0.3690944881889765550, -0.3153832671262227771 ) ) ;
#80519=CARTESIAN_POINT ( 'NONE',  ( -1.095800524934382292, -0.3162353388693409650, -0.4822834645669289433 ) ) ;
#80520=CARTESIAN_POINT ( 'NONE',  ( -0.6824146981627291497, -0.6046776061558809534, -0.2411417322834644161 ) ) ;
#80521=B_SPLINE_CURVE_WITH_KNOTS ( 'NONE', 3,
 ( #30128, #15453, #41112, #34806, #60465, #56210, #12021, #38505, #75593, #24635 ),
 .UNSPECIFIED., .F., .F.,
 ( 4, 2, 2, 2, 4 ),
 ( 2.168404344971008868E-18, 0.003519800242347440305, 0.004399750302934300056, 0.005279700363521159373, 0.007039600484694878008 ),
 .UNSPECIFIED. ) ;
#80522=EDGE_CURVE ( 'NONE', #820, #42318, #55481, .T. ) ;
#80527=CARTESIAN_POINT ( 'NONE',  ( 0.7086614173228353852, -0.1870078740157479769, 0.3641732283464567677 ) ) ;
#80529=CARTESIAN_POINT ( 'NONE',  ( 1.030183727034121421, -0.3162353388693409650, -0.4822834645669289433 ) ) ;
#80531=DIRECTION ( 'NONE',  ( 1.000000000000000000, -0.000000000000000000, -0.000000000000000000 ) ) ;
#80532=EDGE_CURVE ( 'NONE', #43739, #82183, #31323, .T. ) ;
#80533=CARTESIAN_POINT ( 'NONE',  ( -1.574803149606298636, -0.1870078740157479769, 0.3641732283464567677 ) ) ;
#80534=CARTESIAN_POINT ( 'NONE',  ( 1.587926509186352586, -0.4281496062992127816, -0.4176697321401328100 ) ) ;
#80535=CARTESIAN_POINT ( 'NONE',  ( 1.279527559055118724, 0.07958543189024085140, 0.2665933059059887866 ) ) ;
#80536=CARTESIAN_POINT ( 'NONE',  ( 0.3018372703412079971, 0.05413385826771626580, -0.4176697321401330321 ) ) ;
#80538=CARTESIAN_POINT ( 'NONE',  ( -0.07217847769028787330, -0.05778040916215522460, 0.4822834645669289988 ) ) ;
#80539=CARTESIAN_POINT ( 'NONE',  ( -0.7480314960629914633, 0.1771653543307087630, 0.000000000000000000 ) ) ;
#80540=CARTESIAN_POINT ( 'NONE',  ( 0.3740157480314966754, 0.1660481256975883668, -0.3530559997133364547 ) ) ;
#80541=CARTESIAN_POINT ( 'NONE',  ( -0.2296587926509179312, -0.3162353388693409650, -0.4822834645669289433 ) ) ;
#80543=DIRECTION ( 'NONE',  ( -3.096699300667737957E-16, 1.000000000000000000, -0.000000000000000000 ) ) ;
#80545=CARTESIAN_POINT ( 'NONE',  ( 1.030183727034121421, -0.05778040916215522460, 0.4822834645669289988 ) ) ;
#80546=CARTESIAN_POINT ( 'NONE',  ( -0.05905511811023545637, -0.5400638737290845981, -0.3530559997133363437 ) ) ;
#80547=CARTESIAN_POINT ( 'NONE',  ( -0.9055118110236215490, -0.6692913385826771977, 8.415575281601705876E-17 ) ) ;
#80548=CARTESIAN_POINT ( 'NONE',  ( 1.095800524934383846, -0.3162353388693405765, 0.4822834645669290543 ) ) ;
#80549=CARTESIAN_POINT ( 'NONE',  ( 0.2624671916010504757, 0.2306618581243848609, 0.2411417322834645549 ) ) ;
#80551=CARTESIAN_POINT ( 'NONE',  ( -0.4724409448818890911, -0.1870078740157479769, 0.4822834645669291653 ) ) ;
#80552=CARTESIAN_POINT ( 'NONE',  ( 0.8333333333333340365, -0.6692913385826771977, 0.1292274648535927661 ) ) ;
#80553=CARTESIAN_POINT ( 'NONE',  ( -0.1706036745406816491, 0.05413385826771626580, -0.4176697321401330321 ) ) ;
#80554=CARTESIAN_POINT ( 'NONE',  ( 0.8070866141732289112, -0.4536011799217368745, -0.2665933059059886201 ) ) ;
#80555=CARTESIAN_POINT ( 'NONE',  ( -1.712598425196849572, 0.1660481256975885056, 0.3530559997133364547 ) ) ;
#80557=CARTESIAN_POINT ( 'NONE',  ( 0.3280839895013130669, 0.05413385826771666132, 0.4176697321401328100 ) ) ;
#80562=VERTEX_POINT ( 'NONE', #50286 ) ;
#80563=CARTESIAN_POINT ( 'NONE',  ( 0.7939632545931766261, -0.3162353388693409650, -0.4822834645669289433 ) ) ;
#80564=CARTESIAN_POINT ( 'NONE',  ( 0.4265091863517067039, -0.5511811023622048555, -0.09757992244046775898 ) ) ;
#80565=CARTESIAN_POINT ( 'NONE',  ( -1.586052503253845503, 2.125984251968505045, 0.1653254495020588799 ) ) ;
#80573=CARTESIAN_POINT ( 'NONE',  ( 0.8530183727034126306, 0.05413385826771626580, -0.4176697321401330321 ) ) ;
#80574=CARTESIAN_POINT ( 'NONE',  ( -0.6036745406824141069, -0.6046776061558809534, -0.2411417322834644161 ) ) ;
#80575=CARTESIAN_POINT ( 'NONE',  ( -0.9120734908136475250, 0.2952755905511811885, 0.1292274648535926551 ) ) ;
#80576=CARTESIAN_POINT ( 'NONE',  ( 0.8005249343832027131, 0.05413385826771666132, 0.4176697321401328100 ) ) ;
#80577=CARTESIAN_POINT ( 'NONE',  ( 1.561679790026247350, -0.4281496062992124485, 0.4176697321401328655 ) ) ;
#80580=CARTESIAN_POINT ( 'NONE',  ( 1.371391076115485941, 0.1771653543307087630, 0.09757992244046791164 ) ) ;
#80582=CARTESIAN_POINT ( 'NONE',  ( -1.174540682414697335, -0.08942795157527998196, 0.3641732283464567121 ) ) ;
#80585=CARTESIAN_POINT ( 'NONE',  ( 0.06561679790026316017, -0.4281496062992124485, 0.4176697321401328655 ) ) ;
#80587=CARTESIAN_POINT ( 'NONE',  ( -1.318897637795274802, -0.4536011799217368745, -0.2665933059059886201 ) ) ;
#80588=CARTESIAN_POINT ( 'NONE',  ( 0.5577427821522316087, -0.05778040916215522460, 0.4822834645669289988 ) ) ;
#80589=CARTESIAN_POINT ( 'NONE',  ( 1.318897637795276356, 0.07958543189024071263, -0.2665933059059888421 ) ) ;
#80591=CARTESIAN_POINT ( 'NONE',  ( -1.017060367454067249, -0.2845877964562161244, -0.3641732283464567121 ) ) ;
#80592=CARTESIAN_POINT ( 'NONE',  ( 1.410761154855643795, -0.05778040916215560624, -0.4822834645669293319 ) ) ;
#80594=CARTESIAN_POINT ( 'NONE',  ( -0.3149606299212590610, -0.1870078740157479769, 0.4822834645669291653 ) ) ;
#80595=CARTESIAN_POINT ( 'NONE',  ( -1.535433070866141225, -0.5511811023622047445, 6.969142054262312111E-17 ) ) ;
#80596=CARTESIAN_POINT ( 'NONE',  ( -0.6036745406824141069, 0.2306618581243848609, 0.2411417322834645549 ) ) ;
#80597=CARTESIAN_POINT ( 'NONE',  ( 1.673228346456693494, 0.1660481256975885056, 0.3530559997133364547 ) ) ;
#80599=CARTESIAN_POINT ( 'NONE',  ( 0.3543307086614179147, 0.2952755905511811885, 0.000000000000000000 ) ) ;
#80600=CARTESIAN_POINT ( 'NONE',  ( 1.568241469816273437, -0.3162353388693405765, 0.4822834645669290543 ) ) ;
#80602=CARTESIAN_POINT ( 'NONE',  ( -1.391076115485563758, 0.2306618581243848609, 0.2411417322834645549 ) ) ;
#80603=CARTESIAN_POINT ( 'NONE',  ( -0.7086614173228339419, -0.1870078740157480601, -0.3641732283464567677 ) ) ;
#80604=CARTESIAN_POINT ( 'NONE',  ( -1.581364829396324945, -0.05778040916215560624, -0.4822834645669293319 ) ) ;
#80605=CARTESIAN_POINT ( 'NONE',  ( -0.06561679790026180015, 0.05413385826771666132, 0.4176697321401328100 ) ) ;
#80606=CARTESIAN_POINT ( 'NONE',  ( 0.3280839895013130669, -0.3690944881889765550, -0.3153832671262227771 ) ) ;
#80607=CARTESIAN_POINT ( 'NONE',  ( -1.148293963254592542, -0.5511811023622048555, -0.09757992244046775898 ) ) ;
#80608=CARTESIAN_POINT ( 'NONE',  ( -1.279527559055116948, -0.5400638737290844871, 0.3530559997133364547 ) ) ;
#80609=CARTESIAN_POINT ( 'NONE',  ( -1.450131233595799651, -0.6692913385826771977, 0.1292274648535927661 ) ) ;
#80610=CARTESIAN_POINT ( 'NONE',  ( 1.535433070866142558, 0.2952755905511811885, 0.000000000000000000 ) ) ;
#80612=CARTESIAN_POINT ( 'NONE',  ( 0.5118110236220480003, -0.5511811023622047445, 6.969142054262312111E-17 ) ) ;
#80613=CARTESIAN_POINT ( 'NONE',  ( 1.076115485564305141, 0.2306618581243847221, -0.2411417322834647770 ) ) ;
#80614=DIRECTION ( 'NONE',  ( 0.000000000000000000, 1.000000000000000000, 0.000000000000000000 ) ) ;
#80615=CARTESIAN_POINT ( 'NONE',  ( 1.318897637795276356, 0.07958543189024071263, -0.2665933059059888421 ) ) ;
#80617=CARTESIAN_POINT ( 'NONE',  ( -1.207349081364828436, -0.6046776061558807314, 0.2411417322834647770 ) ) ;
#80618=CARTESIAN_POINT ( 'NONE',  ( -0.7611548556430438595, -0.6046776061558809534, -0.2411417322834644161 ) ) ;
#80619=CARTESIAN_POINT ( 'NONE',  ( 0.2821522309711292364, -0.6692913385826771977, 0.1292274648535927661 ) ) ;
#80622=CARTESIAN_POINT ( 'NONE',  ( 0.8792650918635177559, -0.4281496062992127816, -0.4176697321401328100 ) ) ;
#80623=CARTESIAN_POINT ( 'NONE',  ( 1.522309711286089939, -0.5023911411419708095, -0.1820866141732282451 ) ) ;
#80624=CARTESIAN_POINT ( 'NONE',  ( 0.08530183727034192087, -0.05778040916215522460, 0.4822834645669289988 ) ) ;
#80625=CARTESIAN_POINT ( 'NONE',  ( 0.6036745406824153282, -0.6046776061558807314, 0.2411417322834647770 ) ) ;
#80632=CARTESIAN_POINT ( 'NONE',  ( -0.08530183727034056085, -0.08942795157528024563, -0.3641732283464568787 ) ) ;
#80633=CARTESIAN_POINT ( 'NONE',  ( -0.1312335958005241554, 0.2306618581243848609, 0.2411417322834645549 ) ) ;
#80634=CARTESIAN_POINT ( 'NONE',  ( 0.7545931758530188826, -0.6692913385826771977, 0.1292274648535927661 ) ) ;
#80636=CARTESIAN_POINT ( 'NONE',  ( -0.1837270341207340729, 0.1283753931104746893, -0.1820866141732285504 ) ) ;
#80637=CARTESIAN_POINT ( 'NONE',  ( -1.161417322834644716, 0.1660481256975885056, 0.3530559997133364547 ) ) ;
#80638=CARTESIAN_POINT ( 'NONE',  ( 1.397637795275591177, -0.5400638737290844871, 0.3530559997133364547 ) ) ;
#80642=ORIENTED_EDGE ( 'NONE', *, *, #31497, .F. ) ;
#80643=CARTESIAN_POINT ( 'NONE',  ( 0.8792650918635177559, -0.4281496062992127816, -0.4176697321401328100 ) ) ;
#80644=CARTESIAN_POINT ( 'NONE',  ( 1.272965879265092637, -0.004921259842519576551, 0.3153832671262227771 ) ) ;
#80645=CARTESIAN_POINT ( 'NONE',  ( -1.614173228346455824, 0.1771653543307087630, 0.000000000000000000 ) ) ;
#80646=CARTESIAN_POINT ( 'NONE',  ( 1.509186351706037543, -0.4281496062992127816, -0.4176697321401328100 ) ) ;
#80649=CARTESIAN_POINT ( 'NONE',  ( 1.187664041994751285, -0.05778040916215522460, 0.4822834645669289988 ) ) ;
#80650=CARTESIAN_POINT ( 'NONE',  ( -1.463254593175852492, -0.6692913385826773087, -0.1292274648535924053 ) ) ;
#80651=CARTESIAN_POINT ( 'NONE',  ( -0.09186351706036689768, 0.05413385826771626580, -0.4176697321401330321 ) ) ;
#80652=CARTESIAN_POINT ( 'NONE',  ( -0.4658792650918627265, -0.05778040916215522460, 0.4822834645669289988 ) ) ;
#80653=CARTESIAN_POINT ( 'NONE',  ( -1.574803149606298192, -0.1870078740157480879, -0.4822834645669291653 ) ) ;
#80655=CARTESIAN_POINT ( 'NONE',  ( 0.2034120734908142214, 0.2952755905511810774, -0.1292274648535930714 ) ) ;
#80658=CARTESIAN_POINT ( 'NONE',  ( 1.509186351706037543, 0.05413385826771666132, 0.4176697321401328100 ) ) ;
#80661=ORIENTED_EDGE ( 'NONE', *, *, #34718, .T. ) ;
#80662=CARTESIAN_POINT ( 'NONE',  ( 0.4531182788721080934, 1.771653543307086354, -0.5309055118110237448 ) ) ;
#80663=CARTESIAN_POINT ( 'NONE',  ( -1.489501312335957062, -0.3162353388693409650, -0.4822834645669289433 ) ) ;
#80665=CARTESIAN_POINT ( 'NONE',  ( 0.3812812444996376282, 2.409604939980833412E-17, -0.3464511005275205946 ) ) ;
#80666=CARTESIAN_POINT ( 'NONE',  ( -0.1246719160104980684, 0.2066929133858267931, 0.1054918080437490802 ) ) ;
#80668=DIRECTION ( 'NONE',  ( -1.000000000000000000, -3.412570772413389987E-16, 0.000000000000000000 ) ) ;
#80670=CARTESIAN_POINT ( 'NONE',  ( -0.2624671916010490880, -0.5023911411419708095, 0.1820866141732285504 ) ) ;
#80671=CARTESIAN_POINT ( 'NONE',  ( -1.148293963254592542, -0.5511811023622048555, -0.09757992244046775898 ) ) ;
#80672=CARTESIAN_POINT ( 'NONE',  ( -1.062992125984250968, -0.6692913385826771977, 8.415575281601705876E-17 ) ) ;
#80673=CARTESIAN_POINT ( 'NONE',  ( 0.3674540682414705883, 0.2306618581243847221, -0.2411417322834647770 ) ) ;
#80674=CARTESIAN_POINT ( 'NONE',  ( -1.246719160104985846, -0.4281496062992127816, -0.4176697321401328100 ) ) ;
#80677=CARTESIAN_POINT ( 'NONE',  ( -1.286089238845143479, 0.2306618581243847221, -0.2411417322834647770 ) ) ;
#80682=CARTESIAN_POINT ( 'NONE',  ( -1.646051170424378096, 0.000000000000000000, 0.3464511005275205946 ) ) ;
#80683=CARTESIAN_POINT ( 'NONE',  ( -0.9317585301837263412, -0.4281496062992127816, -0.4176697321401328100 ) ) ;
#80684=CARTESIAN_POINT ( 'NONE',  ( 1.456692913385827515, -0.6692913385826771977, 8.415575281601705876E-17 ) ) ;
#80685=CARTESIAN_POINT ( 'NONE',  ( -1.653543307086613234, -0.1870078740157480879, -0.4822834645669291653 ) ) ;
#80688=CARTESIAN_POINT ( 'NONE',  ( -1.679790026246718693, 0.2306618581243847221, -0.2411417322834647770 ) ) ;
#80689=CARTESIAN_POINT ( 'NONE',  ( -0.8136482939632537770, -0.6046776061558807314, 0.2411417322834647770 ) ) ;
#80691=CARTESIAN_POINT ( 'NONE',  ( 0.2427821522309716595, -0.2845877964562161244, -0.3641732283464567121 ) ) ;
#80693=CARTESIAN_POINT ( 'NONE',  ( -0.1312335958005241554, -0.5023911411419708095, -0.1820866141732282451 ) ) ;
#80694=CARTESIAN_POINT ( 'NONE',  ( 1.062992125984252745, -0.5511811023622047445, 6.969142054262312111E-17 ) ) ;
#80695=CARTESIAN_POINT ( 'NONE',  ( 0.7020997375328090762, -0.05778040916215560624, -0.4822834645669293319 ) ) ;
#80696=CARTESIAN_POINT ( 'NONE',  ( -0.4002624671916004129, -0.2845877964562159024, 0.3641732283464567677 ) ) ;
#80698=CARTESIAN_POINT ( 'NONE',  ( -1.561679790026246017, -0.4281496062992127816, -0.4176697321401328100 ) ) ;
#80699=CARTESIAN_POINT ( 'NONE',  ( -1.469816272965878357, 0.1283753931104748280, 0.1820866141732283561 ) ) ;
#80701=CARTESIAN_POINT ( 'NONE',  ( 0.08530183727034192087, -0.3162353388693409650, -0.4822834645669289433 ) ) ;
#80702=CARTESIAN_POINT ( 'NONE',  ( -0.6102362204724400829, -0.5400638737290845981, -0.3530559997133363437 ) ) ;
#80703=CARTESIAN_POINT ( 'NONE',  ( 1.548556430446194954, 0.1283753931104746893, -0.1820866141732285504 ) ) ;
#80704=CARTESIAN_POINT ( 'NONE',  ( 0.2624671916010504757, -0.5023911411419708095, -0.1820866141732282451 ) ) ;
#80705=CARTESIAN_POINT ( 'NONE',  ( -0.2559055118110230564, 0.1660481256975883668, -0.3530559997133364547 ) ) ;
#80706=CARTESIAN_POINT ( 'NONE',  ( -0.7939632545931750718, -0.05778040916215560624, -0.4822834645669293319 ) ) ;
#80707=CARTESIAN_POINT ( 'NONE',  ( -1.595398199321655275, 2.136509776695170615, 0.1559797534342493575 ) ) ;
#80708=CARTESIAN_POINT ( 'NONE',  ( -1.012524390108115568, 5.991678263669262536E-15, 0.3954985857520036951 ) ) ;
#80709=CARTESIAN_POINT ( 'NONE',  ( 0.3346456692913393205, -0.5400638737290845981, -0.3530559997133363437 ) ) ;
#80711=CARTESIAN_POINT ( 'NONE',  ( 1.489501312335958172, -0.05778040916215560624, -0.4822834645669293319 ) ) ;
#80712=CARTESIAN_POINT ( 'NONE',  ( -0.3215223097112853146, -0.2845877964562159024, 0.3641732283464567677 ) ) ;
#80713=CARTESIAN_POINT ( 'NONE',  ( -0.4396325459317579898, 0.2952755905511811885, 0.1292274648535926551 ) ) ;
#80714=CARTESIAN_POINT ( 'NONE',  ( 1.653543307086614789, -0.1870078740157479769, 0.4822834645669291653 ) ) ;
#80715=CARTESIAN_POINT ( 'NONE',  ( 1.489501312335958172, -0.3162353388693405765, 0.4822834645669290543 ) ) ;
#80716=CARTESIAN_POINT ( 'NONE',  ( -1.456692913385826182, 0.2952755905511811885, 0.000000000000000000 ) ) ;
#80717=CARTESIAN_POINT ( 'NONE',  ( -0.8595800524934373854, -0.2845877964562161244, -0.3641732283464567121 ) ) ;
#80722=CARTESIAN_POINT ( 'NONE',  ( 1.620734908136483465, -0.5511811023622046335, 0.09757992244046803654 ) ) ;
#80723=CARTESIAN_POINT ( 'NONE',  ( 1.266404199475066328, -0.08942795157527998196, 0.3641732283464567121 ) ) ;
#80724=CARTESIAN_POINT ( 'NONE',  ( 0.8530183727034126306, 0.05413385826771626580, -0.4176697321401330321 ) ) ;
#80725=CARTESIAN_POINT ( 'NONE',  ( -1.568241469816272105, -0.05778040916215522460, 0.4822834645669289988 ) ) ;
#80726=CARTESIAN_POINT ( 'NONE',  ( 0.7152230971128614723, -0.3162353388693409650, -0.4822834645669289433 ) ) ;
#80728=CARTESIAN_POINT ( 'NONE',  ( 1.377952755905512472, 0.1771653543307087630, 0.000000000000000000 ) ) ;
#80729=CARTESIAN_POINT ( 'NONE',  ( 0.2362204724409456558, -0.1870078740157479769, 0.4822834645669291653 ) ) ;
#80730=CARTESIAN_POINT ( 'NONE',  ( -0.8005249343832011588, 0.05413385826771626580, -0.4176697321401330321 ) ) ;
#80731=CARTESIAN_POINT ( 'NONE',  ( 1.259842519685040019, -0.1870078740157480879, -0.4822834645669291653 ) ) ;
#80734=CARTESIAN_POINT ( 'NONE',  ( 0.3412073490813655186, 0.1283753931104748280, 0.1820866141732283561 ) ) ;
#80738=CARTESIAN_POINT ( 'NONE',  ( -0.2559055118110230564, 0.1660481256975883668, -0.3530559997133364547 ) ) ;
#80739=CARTESIAN_POINT ( 'NONE',  ( -0.3871391076115476282, -0.05778040916215522460, 0.4822834645669289988 ) ) ;
#80740=CARTESIAN_POINT ( 'NONE',  ( -0.2165354330708654795, 0.1660481256975885056, 0.3530559997133364547 ) ) ;
#80741=CARTESIAN_POINT ( 'NONE',  ( 0.8202099737532814183, -0.6692913385826773087, -0.1292274648535924053 ) ) ;
#80742=CARTESIAN_POINT ( 'NONE',  ( -0.7874015748031489847, -0.1870078740157480879, -0.4822834645669291653 ) ) ;
#80743=CARTESIAN_POINT ( 'NONE',  ( -0.5905511811023615998, 0.2952755905511811885, 0.000000000000000000 ) ) ;
#80744=CARTESIAN_POINT ( 'NONE',  ( 1.253280839895013710, -0.3162353388693405765, 0.4822834645669290543 ) ) ;
#80745=CARTESIAN_POINT ( 'NONE',  ( 0.6233595800524939223, -0.3162353388693405765, 0.4822834645669290543 ) ) ;
#80746=CARTESIAN_POINT ( 'NONE',  ( 0.6430446194225729606, -0.4281496062992127816, -0.4176697321401328100 ) ) ;
#80748=CARTESIAN_POINT ( 'NONE',  ( -0.5380577427821514602, -0.004921259842519576551, 0.3153832671262227771 ) ) ;
#80749=ORIENTED_EDGE ( 'NONE', *, *, #6655, .F. ) ;
#80752=CARTESIAN_POINT ( 'NONE',  ( -0.7939632545931754048, -0.2845877964562159024, 0.3641732283464567677 ) ) ;
#80753=CARTESIAN_POINT ( 'NONE',  ( -0.6167979002624665030, -0.4281496062992127816, -0.4176697321401328100 ) ) ;
#80755=CARTESIAN_POINT ( 'NONE',  ( -0.6102362204724400829, 0.1660481256975885056, 0.3530559997133364547 ) ) ;
#80756=CARTESIAN_POINT ( 'NONE',  ( -0.9186351706036736120, 0.2306618581243848609, 0.2411417322834645549 ) ) ;
#80757=CARTESIAN_POINT ( 'NONE',  ( -1.332020997375327642, -0.05778040916215522460, 0.4822834645669289988 ) ) ;
#80758=CARTESIAN_POINT ( 'NONE',  ( -1.482939632545930975, -0.4281496062992127816, -0.4176697321401328100 ) ) ;
#80759=CARTESIAN_POINT ( 'NONE',  ( 1.036745406824147731, -0.004921259842519576551, 0.3153832671262227771 ) ) ;
#80761=CARTESIAN_POINT ( 'NONE',  ( -1.572991167713776672, 2.401574803149606474, 0.1227090857360981641 ) ) ;
#80762=CARTESIAN_POINT ( 'NONE',  ( 0.2887139107611556010, -0.5023911411419708095, 0.1820866141732285504 ) ) ;
#80763=CARTESIAN_POINT ( 'NONE',  ( 0.1706036745406830368, -0.4281496062992127816, -0.4176697321401328100 ) ) ;
#80764=CARTESIAN_POINT ( 'NONE',  ( -0.01968503937007793844, 0.1660481256975883668, -0.3530559997133364547 ) ) ;
#80767=CARTESIAN_POINT ( 'NONE',  ( -0.6167979002624665030, 0.05413385826771666132, 0.4176697321401328100 ) ) ;
#80771=CARTESIAN_POINT ( 'NONE',  ( -0.5905511811023615998, 0.1771653543307087630, 0.000000000000000000 ) ) ;
#80772=CARTESIAN_POINT ( 'NONE',  ( -1.017060367454067249, -0.3162353388693409650, -0.4822834645669289433 ) ) ;
#80775=CARTESIAN_POINT ( 'NONE',  ( 1.574803149606299746, -0.1870078740157480879, -0.4822834645669291653 ) ) ;
#80776=CARTESIAN_POINT ( 'NONE',  ( 0.5118110236220478892, 0.2952755905511811885, 0.000000000000000000 ) ) ;
#80777=CARTESIAN_POINT ( 'NONE',  ( 0.7152230971128616943, -0.05778040916215522460, 0.4822834645669289988 ) ) ;
#80778=CARTESIAN_POINT ( 'NONE',  ( -0.5643044619422565855, -0.3690944881889763329, 0.3153832671262228327 ) ) ;
#80779=CARTESIAN_POINT ( 'NONE',  ( -0.07217847769028813698, -0.3162353388693409650, -0.4822834645669289433 ) ) ;
#80781=CARTESIAN_POINT ( 'NONE',  ( -0.4133858267716528645, 0.1660481256975883668, -0.3530559997133364547 ) ) ;
#80783=CARTESIAN_POINT ( 'NONE',  ( 1.325459317585302665, -0.004921259842519870586, -0.3153832671262229437 ) ) ;
#80784=CARTESIAN_POINT ( 'NONE',  ( 0.1509186351706042484, -0.2845877964562159024, 0.3641732283464567677 ) ) ;
#80785=CARTESIAN_POINT ( 'NONE',  ( 1.049868766404200349, 0.1283753931104748280, 0.1820866141732283561 ) ) ;
#80786=CARTESIAN_POINT ( 'NONE',  ( -0.9514435695538050464, -0.3162353388693405765, 0.4822834645669290543 ) ) ;
#80788=CARTESIAN_POINT ( 'NONE',  ( -1.325459317585300889, -0.004921259842519576551, 0.3153832671262227771 ) ) ;
#80790=CARTESIAN_POINT ( 'NONE',  ( -1.240157480314959759, 0.1660481256975885056, 0.3530559997133364547 ) ) ;
#80791=CARTESIAN_POINT ( 'NONE',  ( -0.6299212598425188991, -0.1870078740157480879, -0.4822834645669291653 ) ) ;
#80792=CARTESIAN_POINT ( 'NONE',  ( 0.4068241469816281097, 0.05413385826771666132, 0.4176697321401328100 ) ) ;
#80795=CARTESIAN_POINT ( 'NONE',  ( 0.4199475065616805614, 0.1283753931104748280, 0.1820866141732283561 ) ) ;
#80796=CARTESIAN_POINT ( 'NONE',  ( 0.8858267716535438430, -0.5400638737290845981, -0.3530559997133363437 ) ) ;
#80798=CARTESIAN_POINT ( 'NONE',  ( 0.7742782152230979209, 0.05413385826771626580, -0.4176697321401330321 ) ) ;
#80799=CARTESIAN_POINT ( 'NONE',  ( -1.706036745406823485, 0.1283753931104748280, 0.1820866141732283561 ) ) ;
#80800=CARTESIAN_POINT ( 'NONE',  ( -1.463254593175852492, -0.6692913385826773087, -0.1292274648535924053 ) ) ;
#80801=CARTESIAN_POINT ( 'NONE',  ( -0.8923884514435688198, 0.2306618581243847221, -0.2411417322834647770 ) ) ;
#80802=CARTESIAN_POINT ( 'NONE',  ( -0.1377952755905504645, -0.4536011799217368745, -0.2665933059059886201 ) ) ;
#80804=CARTESIAN_POINT ( 'NONE',  ( 0.7742782152230978099, -0.3690944881889763329, 0.3153832671262228327 ) ) ;
#80805=VECTOR ( 'NONE', #40848, 39.37007874015748143 ) ;
#80806=CARTESIAN_POINT ( 'NONE',  ( 0.06561679790026316017, -0.4281496062992124485, 0.4176697321401328655 ) ) ;
#80808=ADVANCED_FACE ( 'NONE', ( #18726 ), #62123, .F. ) ;
#80809=CARTESIAN_POINT ( 'NONE',  ( -1.312335958005248715, -0.6046776061558809534, -0.2411417322834644161 ) ) ;
#80811=CARTESIAN_POINT ( 'NONE',  ( 0.8858267716535438430, -0.4536011799217368745, -0.2665933059059886201 ) ) ;
#80812=CARTESIAN_POINT ( 'NONE',  ( 0.1181102362204730916, 0.2952755905511811885, 0.000000000000000000 ) ) ;
#80813=CARTESIAN_POINT ( 'NONE',  ( -0.07874015748031421014, -0.1870078740157479769, 0.4822834645669291653 ) ) ;
#80814=CARTESIAN_POINT ( 'NONE',  ( -0.3871391076115476282, -0.08942795157527998196, 0.3641732283464567121 ) ) ;
#80815=CARTESIAN_POINT ( 'NONE',  ( 0.9573014326657177664, 0.000000000000000000, 0.3464511005275205946 ) ) ;
#80816=CARTESIAN_POINT ( 'NONE',  ( -0.5446194225721777693, -0.08942795157527998196, 0.3641732283464567121 ) ) ;
#80817=CARTESIAN_POINT ( 'NONE',  ( 0.2296587926509192634, -0.3162353388693405765, 0.4822834645669290543 ) ) ;
#80818=CARTESIAN_POINT ( 'NONE',  ( -1.358267716535432434, 0.07958543189024071263, -0.2665933059059888421 ) ) ;
#80820=CARTESIAN_POINT ( 'NONE',  ( -1.653543307086613234, -0.1870078740157479769, 0.4822834645669291653 ) ) ;
#80822=ORIENTED_EDGE ( 'NONE', *, *, #38397, .F. ) ;
#80823=CARTESIAN_POINT ( 'NONE',  ( -1.391076115485563758, 0.1283753931104748280, 0.1820866141732283561 ) ) ;
#80824=CARTESIAN_POINT ( 'NONE',  ( -0.4593175853018366950, 0.05413385826771666132, 0.4176697321401328100 ) ) ;
#80825=CARTESIAN_POINT ( 'NONE',  ( -1.351706036745406347, -0.4281496062992124485, 0.4176697321401328655 ) ) ;
#80828=CARTESIAN_POINT ( 'NONE',  ( 1.253280839895013710, -0.05778040916215560624, -0.4822834645669293319 ) ) ;
#80829=CARTESIAN_POINT ( 'NONE',  ( 0.5446194225721792126, -0.3162353388693405765, 0.4822834645669290543 ) ) ;
#80832=CARTESIAN_POINT ( 'NONE',  ( 1.601049868766404982, 0.1283753931104748280, 0.1820866141732283561 ) ) ;
#80835=VERTEX_POINT ( 'NONE', #11071 ) ;
#80836=CARTESIAN_POINT ( 'NONE',  ( -1.010498687664041384, -0.004921259842519576551, 0.3153832671262227771 ) ) ;
#80839=CARTESIAN_POINT ( 'NONE',  ( 0.8464566929133865436, 0.1660481256975883668, -0.3530559997133364547 ) ) ;
#80840=CARTESIAN_POINT ( 'NONE',  ( -0.5446194225721777693, -0.3162353388693409650, -0.4822834645669289433 ) ) ;
#80841=CARTESIAN_POINT ( 'NONE',  ( -0.9383202099737524282, -0.3162353388693409650, -0.4822834645669289433 ) ) ;
#80842=CARTESIAN_POINT ( 'NONE',  ( 1.089238845144357759, 0.05413385826771626580, -0.4176697321401330321 ) ) ;
#80843=CARTESIAN_POINT ( 'NONE',  ( -1.364829396325458521, -0.5023911411419708095, 0.1820866141732285504 ) ) ;
#80845=CARTESIAN_POINT ( 'NONE',  ( 0.1706036745406830368, -0.4281496062992127816, -0.4176697321401328100 ) ) ;
#80847=CARTESIAN_POINT ( 'NONE',  ( -0.7874015748031489847, -0.1870078740157480879, -0.4822834645669291653 ) ) ;
#80849=CARTESIAN_POINT ( 'NONE',  ( -1.181102362204723644, -0.1870078740157479769, 0.4822834645669291653 ) ) ;
#80851=CARTESIAN_POINT ( 'NONE',  ( 0.9908136482939640111, -0.6692913385826771977, 0.1292274648535927661 ) ) ;
#80853=CARTESIAN_POINT ( 'NONE',  ( 1.410761154855643795, -0.08942795157528024563, -0.3641732283464568787 ) ) ;
#80856=CARTESIAN_POINT ( 'NONE',  ( -0.5905511811023613777, -0.6692913385826771977, 8.415575281601705876E-17 ) ) ;
#80858=CARTESIAN_POINT ( 'NONE',  ( 0.2493438320209980519, -0.3690944881889765550, -0.3153832671262227771 ) ) ;
#80859=CARTESIAN_POINT ( 'NONE',  ( -1.522309711286088607, 0.2306618581243847221, -0.2411417322834647770 ) ) ;
#80860=CARTESIAN_POINT ( 'NONE',  ( 0.6102362204724416372, -0.5400638737290844871, 0.3530559997133364547 ) ) ;
#80861=CARTESIAN_POINT ( 'NONE',  ( 0.9645669291338588858, 0.1660481256975885056, 0.3530559997133364547 ) ) ;
#80862=CARTESIAN_POINT ( 'NONE',  ( -0.2296587926509179312, -0.3162353388693409650, -0.4822834645669289433 ) ) ;
#80864=CARTESIAN_POINT ( 'NONE',  ( -0.8661417322834640276, -0.1870078740157479769, 0.4822834645669291653 ) ) ;
#80866=CARTESIAN_POINT ( 'NONE',  ( -1.620734908136482577, -0.6692913385826773087, -0.1292274648535924053 ) ) ;
#80867=CARTESIAN_POINT ( 'NONE',  ( -0.8792650918635160906, -0.4281496062992124485, 0.4176697321401328655 ) ) ;
#80868=CARTESIAN_POINT ( 'NONE',  ( 1.351706036745407680, 0.05413385826771666132, 0.4176697321401328100 ) ) ;
#80869=CARTESIAN_POINT ( 'NONE',  ( 1.181102362204725198, -0.1870078740157479769, 0.4822834645669291653 ) ) ;
#80871=CARTESIAN_POINT ( 'NONE',  ( -1.122047244094487306, -0.5400638737290844871, 0.3530559997133364547 ) ) ;
#80873=CARTESIAN_POINT ( 'NONE',  ( 0.2821522309711292364, -0.6692913385826771977, 0.1292274648535927661 ) ) ;
#80875=CARTESIAN_POINT ( 'NONE',  ( -0.4199475065616791736, -0.6046776061558807314, 0.2411417322834647770 ) ) ;
#80876=CARTESIAN_POINT ( 'NONE',  ( -1.640419947506561060, -0.004921259842519576551, 0.3153832671262227771 ) ) ;
#80877=CARTESIAN_POINT ( 'NONE',  ( 0.5905511811023629321, 0.1771653543307087630, 0.000000000000000000 ) ) ;
#80878=CARTESIAN_POINT ( 'NONE',  ( 1.292650918635171564, 0.2952755905511811885, 0.1292274648535926551 ) ) ;
#80880=CARTESIAN_POINT ( 'NONE',  ( 0.9711286089238851948, -0.5023911411419708095, -0.1820866141732282451 ) ) ;
#80881=CARTESIAN_POINT ( 'NONE',  ( 0.9120734908136489683, -0.6692913385826771977, 0.1292274648535927661 ) ) ;
#80883=CARTESIAN_POINT ( 'NONE',  ( -0.7217847769028863381, 0.05413385826771626580, -0.4176697321401330321 ) ) ;
#80884=CARTESIAN_POINT ( 'NONE',  ( 0.08874907683610111508, -2.191421614605370878E-15, 0.4445507791589071167 ) ) ;
#80885=CARTESIAN_POINT ( 'NONE',  ( 1.548556430446194954, -0.5023911411419708095, 0.1820866141732285504 ) ) ;
#80886=CARTESIAN_POINT ( 'NONE',  ( -0.6627296587926503335, -0.6692913385826771977, 0.1292274648535927661 ) ) ;
#80887=CARTESIAN_POINT ( 'NONE',  ( 0.2099737532808405305, 0.2306618581243847221, -0.2411417322834647770 ) ) ;
#80888=CARTESIAN_POINT ( 'NONE',  ( -1.148293963254592542, 0.2952755905511811885, 0.1292274648535926551 ) ) ;
#80889=CARTESIAN_POINT ( 'NONE',  ( 0.2165354330708668673, 0.1660481256975883668, -0.3530559997133364547 ) ) ;
#80890=CARTESIAN_POINT ( 'NONE',  ( 0.3346456692913393205, -0.4536011799217368745, -0.2665933059059886201 ) ) ;
#80891=CARTESIAN_POINT ( 'NONE',  ( 0.8530183727034126306, 0.009842519685039144428, -0.3409548833797004797 ) ) ;
#80892=CARTESIAN_POINT ( 'NONE',  ( -0.02624671916010428221, 0.1283753931104746893, -0.1820866141732285504 ) ) ;
#80893=CARTESIAN_POINT ( 'NONE',  ( 0.8530183727034126306, -0.004921259842519870586, -0.3153832671262229437 ) ) ;
#80894=PLANE ( 'NONE',  #49175 ) ;
#80896=CARTESIAN_POINT ( 'NONE',  ( 0.4593175853018380828, 0.05413385826771626580, -0.4176697321401330321 ) ) ;
#80898=CARTESIAN_POINT ( 'NONE',  ( 1.476377952755906442, -0.4536011799217367080, 0.2665933059059888421 ) ) ;
#80899=CARTESIAN_POINT ( 'NONE',  ( 0.1377952755905518800, 0.1660481256975883391, -0.3530559997133364547 ) ) ;
#80900=CARTESIAN_POINT ( 'NONE',  ( 0.1640419947506569498, -0.08942795157527998196, 0.3641732283464567121 ) ) ;
#80901=CARTESIAN_POINT ( 'NONE',  ( 0.1115485564304470323, 0.2952755905511811885, 0.1292274648535926551 ) ) ;
#80902=CARTESIAN_POINT ( 'NONE',  ( 1.292650918635171564, -0.5511811023622048555, -0.09757992244046775898 ) ) ;
#80903=CARTESIAN_POINT ( 'NONE',  ( -1.279527559055116948, -0.4536011799217367080, 0.2665933059059888421 ) ) ;
#80904=CARTESIAN_POINT ( 'NONE',  ( -1.555118110236219930, 0.1660481256975885056, 0.3530559997133364547 ) ) ;
#80906=CARTESIAN_POINT ( 'NONE',  ( 0.1902887139107617975, -0.6692913385826773087, -0.1292274648535924053 ) ) ;
#80907=CARTESIAN_POINT ( 'NONE',  ( 1.279527559055118724, -0.5400638737290845981, -0.3530559997133363437 ) ) ;
#80909=CARTESIAN_POINT ( 'NONE',  ( -0.03280839895013062252, -0.6692913385826771977, 0.1292274648535927661 ) ) ;
#80910=CARTESIAN_POINT ( 'NONE',  ( 1.233595800524935227, 0.2306618581243847221, -0.2411417322834647770 ) ) ;
#80911=CARTESIAN_POINT ( 'NONE',  ( 1.154855643044620184, -0.6046776061558807314, 0.2411417322834647770 ) ) ;
#80912=CARTESIAN_POINT ( 'NONE',  ( -1.586052503253845503, 2.125984251968505045, -0.1653254495020588799 ) ) ;
#80913=CARTESIAN_POINT ( 'NONE',  ( 0.8070866141732289112, -0.4536011799217368745, -0.2665933059059886201 ) ) ;
#80914=CARTESIAN_POINT ( 'NONE',  ( 1.496062992125985147, -0.1870078740157479769, 0.4822834645669291653 ) ) ;
#80915=CARTESIAN_POINT ( 'NONE',  ( 0.2427821522309716595, -0.2845877964562161244, -0.3641732283464567121 ) ) ;
#80916=CARTESIAN_POINT ( 'NONE',  ( -0.3871391076115476282, -0.05778040916215522460, 0.4822834645669289988 ) ) ;
#80917=CARTESIAN_POINT ( 'NONE',  ( 0.5249343832021003964, 0.2306618581243847221, -0.2411417322834647770 ) ) ;
#80918=CARTESIAN_POINT ( 'NONE',  ( -0.1902887139107604098, 0.2952755905511810774, -0.1292274648535930714 ) ) ;
#80920=CARTESIAN_POINT ( 'NONE',  ( -0.1706036745406816491, -0.3690944881889763329, 0.3153832671262228327 ) ) ;
#80921=CARTESIAN_POINT ( 'NONE',  ( 0.7283464566929140904, -0.5400638737290845981, -0.3530559997133363437 ) ) ;
#80922=CARTESIAN_POINT ( 'NONE',  ( 1.049868766404200349, 0.1283753931104748280, 0.1820866141732283561 ) ) ;
#80924=CARTESIAN_POINT ( 'NONE',  ( -0.9324623468618411515, 0.000000000000000000, 0.3464511005275205946 ) ) ;
#80927=CARTESIAN_POINT ( 'NONE',  ( -1.227034120734907141, -0.6692913385826773087, -0.1292274648535924053 ) ) ;
#80928=CARTESIAN_POINT ( 'NONE',  ( -0.5249343832020990641, -0.6046776061558809534, -0.2411417322834644161 ) ) ;
#80931=ORIENTED_EDGE ( 'NONE', *, *, #34562, .F. ) ;
#80932=CARTESIAN_POINT ( 'NONE',  ( 0.1246719160104994284, 0.1771653543307087075, -0.09757992244046823083 ) ) ;
#80934=CARTESIAN_POINT ( 'NONE',  ( 1.200787401574803681, -0.5400638737290845981, -0.3530559997133363437 ) ) ;
#80936=CARTESIAN_POINT ( 'NONE',  ( 1.012036180893693293, 0.02791078216816447743, -0.4328096321851892525 ) ) ;
#80937=CARTESIAN_POINT ( 'NONE',  ( -0.2887139107611542133, 0.2306618581243848609, 0.2411417322834645549 ) ) ;
#80940=CARTESIAN_POINT ( 'NONE',  ( 1.430446194225722500, -0.004921259842519576551, 0.3153832671262227771 ) ) ;
#80941=CARTESIAN_POINT ( 'NONE',  ( 0.6299212598425204535, -0.1870078740157480879, -0.4822834645669291653 ) ) ;
#80943=CARTESIAN_POINT ( 'NONE',  ( 0.1968503937007881344, -0.6692913385826771977, 8.415575281601705876E-17 ) ) ;
#80944=CARTESIAN_POINT ( 'NONE',  ( -0.7414698162729651543, 0.1771653543307087075, -0.09757992244046823083 ) ) ;
#80945=CARTESIAN_POINT ( 'NONE',  ( 0.6364829396325465405, -0.05778040916215522460, 0.4822834645669289988 ) ) ;
#80946=CARTESIAN_POINT ( 'NONE',  ( -0.1377952755905504645, 0.1660481256975885056, 0.3530559997133364547 ) ) ;
#80951=CARTESIAN_POINT ( 'NONE',  ( 0.8005249343832028242, -0.4281496062992127816, -0.4176697321401328100 ) ) ;
#80952=CARTESIAN_POINT ( 'NONE',  ( -0.2887139107611542133, 0.2306618581243848609, 0.2411417322834645549 ) ) ;
#80953=CARTESIAN_POINT ( 'NONE',  ( -1.200787401574802349, -0.5400638737290844871, 0.3530559997133364547 ) ) ;
#80954=CARTESIAN_POINT ( 'NONE',  ( 1.141732283464567566, 0.2952755905511811885, 0.000000000000000000 ) ) ;
#80955=CARTESIAN_POINT ( 'NONE',  ( 0.4461942257217856311, 0.2306618581243847221, -0.2411417322834647770 ) ) ;
#80957=CARTESIAN_POINT ( 'NONE',  ( -0.2559055118110230564, 0.1660481256975883668, -0.3530559997133364547 ) ) ;
#80958=CARTESIAN_POINT ( 'NONE',  ( 0.2230971128608932319, -0.4281496062992124485, 0.4176697321401328655 ) ) ;
#80959=CARTESIAN_POINT ( 'NONE',  ( -0.2690288713910754526, -0.6692913385826771977, 0.1292274648535927661 ) ) ;
#80960=CARTESIAN_POINT ( 'NONE',  ( 0.3083989501312343062, -0.08942795157528024563, -0.3641732283464568787 ) ) ;
#80961=FACE_OUTER_BOUND ( 'NONE', #40361, .T. ) ;
#80962=CARTESIAN_POINT ( 'NONE',  ( -1.666666666666665853, 0.05413385826771626580, -0.4176697321401330321 ) ) ;
#80963=CARTESIAN_POINT ( 'NONE',  ( 0.2099737532808405305, 0.2306618581243847221, -0.2411417322834647770 ) ) ;
#80966=CARTESIAN_POINT ( 'NONE',  ( 1.351706036745407458, -0.4281496062992127816, -0.4176697321401328100 ) ) ;
#80968=VERTEX_POINT ( 'NONE', #54013 ) ;
#80971=CARTESIAN_POINT ( 'NONE',  ( 0.6692913385826778638, -0.6692913385826771977, 8.415575281601705876E-17 ) ) ;
#80972=CARTESIAN_POINT ( 'NONE',  ( 0.4068241469816279987, -0.3690944881889765550, -0.3153832671262227771 ) ) ;
#80973=CARTESIAN_POINT ( 'NONE',  ( 0.9548908091195654757, -4.927456884911482678E-16, 0.4445507791589062840 ) ) ;
#80980=CARTESIAN_POINT ( 'NONE',  ( 0.8398950131233602345, 0.2306618581243847221, -0.2411417322834647770 ) ) ;
#80981=CARTESIAN_POINT ( 'NONE',  ( -0.6299212598425188991, -0.1870078740157480879, -0.4822834645669291653 ) ) ;
#80982=CARTESIAN_POINT ( 'NONE',  ( -0.7414698162729651543, 0.2952755905511810774, -0.1292274648535930714 ) ) ;
#80983=CARTESIAN_POINT ( 'NONE',  ( 0.4790026246719167324, -0.05778040916215522460, 0.4822834645669289988 ) ) ;
#80984=CARTESIAN_POINT ( 'NONE',  ( 1.332020997375328974, -0.05778040916215560624, -0.4822834645669293319 ) ) ;
#80987=CARTESIAN_POINT ( 'NONE',  ( 1.397637795275591177, 0.07958543189024071263, -0.2665933059059888421 ) ) ;
#80988=DIRECTION ( 'NONE',  ( 0.000000000000000000, 1.000000000000000000, 0.000000000000000000 ) ) ;
#80989=CARTESIAN_POINT ( 'NONE',  ( -1.476377952755905110, 0.07958543189024085140, 0.2665933059059887866 ) ) ;
#80991=CARTESIAN_POINT ( 'NONE',  ( 0.2887139107611556010, 0.2306618581243847221, -0.2411417322834647770 ) ) ;
#80992=CARTESIAN_POINT ( 'NONE',  ( 1.108923884514436686, -0.3162353388693409650, -0.4822834645669289433 ) ) ;
#80994=CARTESIAN_POINT ( 'NONE',  ( -1.332020997375327642, -0.2845877964562161244, -0.3641732283464567121 ) ) ;
#80995=CARTESIAN_POINT ( 'NONE',  ( 0.5511811023622055217, -0.1870078740157479769, 0.4822834645669291653 ) ) ;
#80996=CARTESIAN_POINT ( 'NONE',  ( 1.312335958005249825, 0.1283753931104746893, -0.1820866141732285504 ) ) ;
#80998=CARTESIAN_POINT ( 'NONE',  ( -1.095800524934382292, -0.08942795157527998196, 0.3641732283464567121 ) ) ;
#80999=CARTESIAN_POINT ( 'NONE',  ( 1.423884514435696413, -0.3162353388693409650, -0.4822834645669289433 ) ) ;
#81001=CARTESIAN_POINT ( 'NONE',  ( -0.05249343832020938322, -0.5023911411419708095, -0.1820866141732282451 ) ) ;
#81002=CARTESIAN_POINT ( 'NONE',  ( -0.03280839895013062252, -0.6692913385826771977, 0.1292274648535927661 ) ) ;
#81003=CARTESIAN_POINT ( 'NONE',  ( -1.246719160104985846, -0.3690944881889765550, -0.3153832671262227771 ) ) ;
#81004=CARTESIAN_POINT ( 'NONE',  ( -0.9120734908136475250, 0.2952755905511811885, 0.1292274648535926551 ) ) ;
#81005=CARTESIAN_POINT ( 'NONE',  ( 1.377952755905512472, 0.2952755905511811885, 0.000000000000000000 ) ) ;
#81008=CARTESIAN_POINT ( 'NONE',  ( 1.391076115485564868, -0.6046776061558807314, 0.2411417322834647770 ) ) ;
#81010=CARTESIAN_POINT ( 'NONE',  ( -1.351706036745406347, 0.05413385826771626580, -0.4176697321401330321 ) ) ;
#81011=CARTESIAN_POINT ( 'NONE',  ( -0.9908136482939626788, 0.1771653543307087630, 0.09757992244046791164 ) ) ;
#81012=EDGE_CURVE ( 'NONE', #53395, #46664, #43035, .T. ) ;
#81013=CARTESIAN_POINT ( 'NONE',  ( -0.7742782152230965886, -0.004921259842519576551, 0.3153832671262227771 ) ) ;
#81015=CARTESIAN_POINT ( 'NONE',  ( 0.07874015748031558404, -0.1870078740157479769, 0.4822834645669291653 ) ) ;
#81016=CARTESIAN_POINT ( 'NONE',  ( 0.09186351706036827158, -0.004921259842519576551, 0.3153832671262227771 ) ) ;
#81017=CARTESIAN_POINT ( 'NONE',  ( -1.253280839895012377, -0.08942795157527998196, 0.3641732283464567121 ) ) ;
#81018=CARTESIAN_POINT ( 'NONE',  ( -1.417322834645668772, -0.1870078740157479769, 0.4822834645669291653 ) ) ;
#81019=CARTESIAN_POINT ( 'NONE',  ( 1.515748031496063186, -0.4536011799217368745, -0.2665933059059886201 ) ) ;
#81021=CARTESIAN_POINT ( 'NONE',  ( 1.279527559055118724, -0.5400638737290845981, -0.3530559997133363437 ) ) ;
#81023=CARTESIAN_POINT ( 'NONE',  ( 0.6299212598425204535, -0.1870078740157480601, -0.3641732283464567677 ) ) ;
#81024=CARTESIAN_POINT ( 'NONE',  ( 0.8267716535433078384, -0.6692913385826771977, 8.415575281601705876E-17 ) ) ;
#81025=CARTESIAN_POINT ( 'NONE',  ( 0.9514435695538062676, -0.08942795157527998196, 0.3641732283464567121 ) ) ;
#81026=VERTEX_POINT ( 'NONE', #42633 ) ;
#81027=CARTESIAN_POINT ( 'NONE',  ( -1.102362204724408601, -0.1870078740157480879, -0.4822834645669291653 ) ) ;
#81029=CARTESIAN_POINT ( 'NONE',  ( -1.043307086614172041, -0.5400638737290844871, 0.3530559997133364547 ) ) ;
#81030=CARTESIAN_POINT ( 'NONE',  ( -0.1902887139107604098, -0.6692913385826771977, 0.1292274648535927661 ) ) ;
#81033=CARTESIAN_POINT ( 'NONE',  ( 0.8464566929133865436, 0.1660481256975883668, -0.3530559997133364547 ) ) ;
#81034=CARTESIAN_POINT ( 'NONE',  ( 1.332020997375328974, -0.08942795157528024563, -0.3641732283464568787 ) ) ;
#81035=CARTESIAN_POINT ( 'NONE',  ( -0.1509186351706028884, -0.3162353388693409650, -0.4822834645669289433 ) ) ;
#81036=CARTESIAN_POINT ( 'NONE',  ( 0.5971128608923890191, -0.6692913385826771977, 0.1292274648535927661 ) ) ;
#81042=CARTESIAN_POINT ( 'NONE',  ( -0.02624671916010428221, -0.5023911411419708095, 0.1820866141732285504 ) ) ;
#81043=CARTESIAN_POINT ( 'NONE',  ( -0.8530183727034112984, -0.4281496062992127816, -0.4176697321401328100 ) ) ;
#81044=CARTESIAN_POINT ( 'NONE',  ( 0.8530183727034126306, 0.05413385826771626580, -0.4176697321401330321 ) ) ;
#81046=CARTESIAN_POINT ( 'NONE',  ( -0.3543307086614165824, 0.1771653543307087630, 0.000000000000000000 ) ) ;
#81047=CARTESIAN_POINT ( 'NONE',  ( 1.555118110236221041, -0.5400638737290844871, 0.3530559997133364547 ) ) ;
#81048=CARTESIAN_POINT ( 'NONE',  ( 1.003937007874016185, 0.1660481256975883668, -0.3530559997133364547 ) ) ;
#81051=CARTESIAN_POINT ( 'NONE',  ( 0.8923884514435701520, -0.6046776061558809534, -0.2411417322834644161 ) ) ;
#81052=CARTESIAN_POINT ( 'NONE',  ( 1.161417322834646271, 0.07958543189024071263, -0.2665933059059888421 ) ) ;
#81053=CARTESIAN_POINT ( 'NONE',  ( 1.614173228346457378, -0.6692913385826771977, 8.415575281601705876E-17 ) ) ;
#81054=CARTESIAN_POINT ( 'NONE',  ( -1.601049868766403650, 0.2306618581243847221, -0.2411417322834647770 ) ) ;
#81057=CARTESIAN_POINT ( 'NONE',  ( 0.7480314960629927956, 0.2952755905511811885, 0.000000000000000000 ) ) ;
#81058=CARTESIAN_POINT ( 'NONE',  ( -1.541994750656167090, 0.2952755905511811885, 0.1292274648535926551 ) ) ;
#81059=CARTESIAN_POINT ( 'NONE',  ( -0.4002624671916004129, -0.05778040916215560624, -0.4822834645669293319 ) ) ;
#81060=CARTESIAN_POINT ( 'NONE',  ( -0.5314960629921254842, -0.5400638737290845981, -0.3530559997133363437 ) ) ;
#81061=CARTESIAN_POINT ( 'NONE',  ( 1.607611548556431069, 0.2952755905511811885, 0.1292274648535926551 ) ) ;
#81063=CARTESIAN_POINT ( 'NONE',  ( 0.05905511811023681640, 0.1660481256975883668, -0.3530559997133364547 ) ) ;
#81065=CARTESIAN_POINT ( 'NONE',  ( 1.679790026246720025, 0.2306618581243848609, 0.2411417322834645549 ) ) ;
#81068=ORIENTED_EDGE ( 'NONE', *, *, #29439, .F. ) ;
#81069=CARTESIAN_POINT ( 'NONE',  ( -1.109025475590603493, 2.631261499653055225, -0.2618487365674062595 ) ) ;
#81070=CARTESIAN_POINT ( 'NONE',  ( -1.509186351706035767, 0.05413385826771626580, -0.4176697321401330321 ) ) ;
#81072=CARTESIAN_POINT ( 'NONE',  ( 1.587926509186352586, -0.3690944881889765550, -0.3153832671262227771 ) ) ;
#81078=CARTESIAN_POINT ( 'NONE',  ( -0.3412073490813641308, 0.1283753931104746893, -0.1820866141732285504 ) ) ;
#81079=CARTESIAN_POINT ( 'NONE',  ( -1.082677165354329896, 0.07958543189024085140, 0.2665933059059887866 ) ) ;
#81080=CARTESIAN_POINT ( 'NONE',  ( 1.535433070866142335, -0.6692913385826771977, 8.415575281601705876E-17 ) ) ;
#81081=CARTESIAN_POINT ( 'NONE',  ( 0.4790026246719167324, -0.05778040916215522460, 0.4822834645669289988 ) ) ;
#81082=CARTESIAN_POINT ( 'NONE',  ( -1.528871391076114250, -0.6692913385826771977, 0.1292274648535927661 ) ) ;
#81084=EDGE_LOOP ( 'NONE', ( #51213, #25101, #30621, #30008, #48316 ) ) ;
#81085=CARTESIAN_POINT ( 'NONE',  ( 1.561679790026247350, -0.4281496062992124485, 0.4176697321401328655 ) ) ;
#81090=CARTESIAN_POINT ( 'NONE',  ( -0.9383202099737524282, -0.3162353388693409650, -0.4822834645669289433 ) ) ;
#81091=CARTESIAN_POINT ( 'NONE',  ( 1.646981627296588035, -0.3162353388693405765, 0.4822834645669290543 ) ) ;
#81094=CARTESIAN_POINT ( 'NONE',  ( 1.653543307086614789, -0.1870078740157479769, 0.4822834645669291653 ) ) ;
#81095=CARTESIAN_POINT ( 'NONE',  ( -0.6889763779527552368, -0.5400638737290845981, -0.3530559997133363437 ) ) ;
#81097=CARTESIAN_POINT ( 'NONE',  ( 0.08530183727034192087, -0.2845877964562161244, -0.3641732283464567121 ) ) ;
#81100=CARTESIAN_POINT ( 'NONE',  ( -0.04593175853018302557, 0.1771653543307087630, 0.09757992244046791164 ) ) ;
#81101=CARTESIAN_POINT ( 'NONE',  ( 0.7217847769028878924, -0.3690944881889765550, -0.3153832671262227771 ) ) ;
#81102=CARTESIAN_POINT ( 'NONE',  ( 0.6561679790026253567, 0.2306618581243848609, 0.2411417322834645549 ) ) ;
#81103=CARTESIAN_POINT ( 'NONE',  ( -0.3608923884514428360, 0.1771653543307087630, 0.09757992244046791164 ) ) ;
#81105=CARTESIAN_POINT ( 'NONE',  ( 1.568241469816273437, -0.3162353388693405765, 0.4822834645669290543 ) ) ;
#81106=B_SPLINE_CURVE_WITH_KNOTS ( 'NONE', 3,
 ( #22820, #75008, #17355, #48895 ),
 .UNSPECIFIED., .F., .F.,
 ( 4, 4 ),
 ( 1.999999999927407068E-07, 0.006970199999999936863 ),
 .UNSPECIFIED. ) ;
#81107=CARTESIAN_POINT ( 'NONE',  ( -1.187664041994749731, -0.3162353388693405765, 0.4822834645669290543 ) ) ;
#81109=CARTESIAN_POINT ( 'NONE',  ( 0.2362204724409456558, -0.1870078740157480879, -0.4822834645669291653 ) ) ;
#81110=CARTESIAN_POINT ( 'NONE',  ( -0.5118110236220466680, 0.2952755905511811885, 0.000000000000000000 ) ) ;
#81112=CARTESIAN_POINT ( 'NONE',  ( -0.05249343832020938322, -0.5023911411419708095, -0.1820866141732282451 ) ) ;
#81113=CARTESIAN_POINT ( 'NONE',  ( -0.03937007874015669567, -0.6692913385826771977, 8.415575281601705876E-17 ) ) ;
#81114=CARTESIAN_POINT ( 'NONE',  ( -0.7020997375328074108, -0.05778040916215522460, 0.4822834645669289988 ) ) ;
#81116=CARTESIAN_POINT ( 'NONE',  ( 1.640419947506562393, -0.3690944881889763329, 0.3153832671262228327 ) ) ;
#81117=AXIS2_PLACEMENT_3D ( 'NONE', #22202, #16317, #65997 ) ;
#81118=CARTESIAN_POINT ( 'NONE',  ( 0.1574803149606306130, -0.1870078740157480879, -0.4822834645669291653 ) ) ;
#81121=CARTESIAN_POINT ( 'NONE',  ( 1.161417322834646271, 0.1660481256975883668, -0.3530559997133364547 ) ) ;
#81122=CARTESIAN_POINT ( 'NONE',  ( -0.8267716535433065062, -0.5511811023622047445, 6.969142054262312111E-17 ) ) ;
#81123=CARTESIAN_POINT ( 'NONE',  ( -0.5643044619422565855, 0.05413385826771626580, -0.4176697321401330321 ) ) ;
#81124=CARTESIAN_POINT ( 'NONE',  ( 1.213910761154856299, 0.2952755905511811885, 0.1292274648535926551 ) ) ;
#81125=CARTESIAN_POINT ( 'NONE',  ( 1.246719160104987623, 0.05413385826771626580, -0.4176697321401330321 ) ) ;
#81126=CARTESIAN_POINT ( 'NONE',  ( -1.633858267716534529, 0.1660481256975885056, 0.3530559997133364547 ) ) ;
#81127=CARTESIAN_POINT ( 'NONE',  ( -1.154855643044618851, -0.5023911411419708095, -0.1820866141732282451 ) ) ;
#81130=AXIS2_PLACEMENT_3D ( 'NONE', #402, #39104, #44161 ) ;
#81132=CARTESIAN_POINT ( 'NONE',  ( 1.633858267716535639, -0.4536011799217367080, 0.2665933059059888421 ) ) ;
#81133=CARTESIAN_POINT ( 'NONE',  ( 1.049868766404200127, -0.5023911411419708095, -0.1820866141732282451 ) ) ;
#81134=CARTESIAN_POINT ( 'NONE',  ( 0.3871391076115492380, -0.05778040916215560624, -0.4822834645669293319 ) ) ;
#81135=CARTESIAN_POINT ( 'NONE',  ( -1.732283464566928277, -0.1870078740157479769, 0.4822834645669291653 ) ) ;
#81137=CARTESIAN_POINT ( 'NONE',  ( 0.6036745406824154392, 0.1283753931104746893, -0.1820866141732285504 ) ) ;
#81138=( BOUNDED_CURVE ( )  B_SPLINE_CURVE ( 1, ( #71912, #27279 ),
 .UNSPECIFIED., .F., .F. ) 
 B_SPLINE_CURVE_WITH_KNOTS ( ( 2, 2 ),
 ( 3.469446951953614189E-18, 0.001999999999999994837 ),
 .UNSPECIFIED. ) 
 CURVE ( )  GEOMETRIC_REPRESENTATION_ITEM ( )  RATIONAL_B_SPLINE_CURVE ( ( 0.9875488213027523443, 0.9875488213027523443 ) ) 
 REPRESENTATION_ITEM ( '' )  );
#81139=CARTESIAN_POINT ( 'NONE',  ( -0.3674540682414689785, 0.2306618581243848609, 0.2411417322834645549 ) ) ;
#81140=CARTESIAN_POINT ( 'NONE',  ( -0.8136482939632537770, 0.2306618581243847221, -0.2411417322834647770 ) ) ;
#81141=CARTESIAN_POINT ( 'NONE',  ( 1.456692913385827515, -0.6692913385826771977, 8.415575281601705876E-17 ) ) ;
#81144=CARTESIAN_POINT ( 'NONE',  ( -0.03937007874015669567, -0.5511811023622047445, 6.969142054262312111E-17 ) ) ;
#81147=ORIENTED_EDGE ( 'NONE', *, *, #35131, .F. ) ;
#81148=CARTESIAN_POINT ( 'NONE',  ( -0.9711286089238838626, -0.6046776061558807314, 0.2411417322834647770 ) ) ;
#81149=CARTESIAN_POINT ( 'NONE',  ( -0.02624671916010428221, 0.2306618581243847221, -0.2411417322834647770 ) ) ;
#81150=CARTESIAN_POINT ( 'NONE',  ( -0.5183727034120726440, 0.2952755905511811885, 0.1292274648535926551 ) ) ;
#81151=CARTESIAN_POINT ( 'NONE',  ( 0.9645669291338591078, -0.5400638737290845981, -0.3530559997133363437 ) ) ;
#81152=CARTESIAN_POINT ( 'NONE',  ( -0.2362204724409440182, -0.1870078740157479769, 0.4822834645669291653 ) ) ;
#81153=CARTESIAN_POINT ( 'NONE',  ( -1.200787401574802349, -0.5400638737290844871, 0.3530559997133364547 ) ) ;
#81154=CARTESIAN_POINT ( 'NONE',  ( -0.4330708661417315697, 0.2952755905511811885, 0.000000000000000000 ) ) ;
#81155=CARTESIAN_POINT ( 'NONE',  ( 0.7086614173228352742, -0.1870078740157480879, -0.4822834645669291653 ) ) ;
#81156=CARTESIAN_POINT ( 'NONE',  ( 0.3740157480314966754, 0.1660481256975883668, -0.3530559997133364547 ) ) ;
#81158=CARTESIAN_POINT ( 'NONE',  ( -0.3805774278215216522, -0.004921259842519576551, 0.3153832671262227771 ) ) ;
#81159=ORIENTED_EDGE ( 'NONE', *, *, #37239, .T. ) ;
#81162=CARTESIAN_POINT ( 'NONE',  ( -1.358267716535432434, 0.07958543189024071263, -0.2665933059059888421 ) ) ;
#81163=CARTESIAN_POINT ( 'NONE',  ( -0.4068241469816264999, -0.4281496062992124485, 0.4176697321401328655 ) ) ;
#81165=CARTESIAN_POINT ( 'NONE',  ( -0.5183727034120726440, -0.6692913385826773087, -0.1292274648535924053 ) ) ;
#81166=CARTESIAN_POINT ( 'NONE',  ( -0.8858267716535425107, 0.1660481256975883668, -0.3530559997133364547 ) ) ;
#81167=CARTESIAN_POINT ( 'NONE',  ( -1.417322834645668772, -0.1870078740157480879, -0.4822834645669291653 ) ) ;
#81169=CARTESIAN_POINT ( 'NONE',  ( 1.082677165354331228, 0.07958543189024071263, -0.2665933059059888421 ) ) ;
#81172=CARTESIAN_POINT ( 'NONE',  ( 0.1509186351706042484, -0.2845877964562159024, 0.3641732283464567677 ) ) ;
#81173=VECTOR ( 'NONE', #55506, 39.37007874015748143 ) ;
#81174=CARTESIAN_POINT ( 'NONE',  ( -0.2690288713910754526, -0.6692913385826771977, 0.1292274648535927661 ) ) ;
#81175=CARTESIAN_POINT ( 'NONE',  ( 0.05905511811023709395, -0.5400638737290844871, 0.3530559997133364547 ) ) ;
#81182=CARTESIAN_POINT ( 'NONE',  ( -0.6955380577427815458, -0.3690944881889765550, -0.3153832671262227771 ) ) ;
#81183=CARTESIAN_POINT ( 'NONE',  ( -0.8136482939632537770, -0.6046776061558807314, 0.2411417322834647770 ) ) ;
#81187=CARTESIAN_POINT ( 'NONE',  ( 1.305774278215223960, -0.6692913385826771977, 0.1292274648535927661 ) ) ;
#81188=CARTESIAN_POINT ( 'NONE',  ( 0.4855643044619428750, 0.05413385826771666132, 0.4176697321401328100 ) ) ;
#81189=CARTESIAN_POINT ( 'NONE',  ( 0.4133858267716541968, 0.1660481256975885056, 0.3530559997133364547 ) ) ;
#81190=CARTESIAN_POINT ( 'NONE',  ( -0.8464566929133852113, 0.07958543189024085140, 0.2665933059059887866 ) ) ;
#81191=CARTESIAN_POINT ( 'NONE',  ( -0.4593175853018366950, 0.05413385826771666132, 0.4176697321401328100 ) ) ;
#81193=CARTESIAN_POINT ( 'NONE',  ( -0.3215223097112853146, -0.3162353388693405765, 0.4822834645669290543 ) ) ;
#81197=CARTESIAN_POINT ( 'NONE',  ( 1.167979002624672580, -0.004921259842519870586, -0.3153832671262229437 ) ) ;
#81198=CARTESIAN_POINT ( 'NONE',  ( -0.1837270341207343505, -0.5023911411419708095, 0.1820866141732285504 ) ) ;
#81199=CARTESIAN_POINT ( 'NONE',  ( 1.272965879265092637, -0.3690944881889765550, -0.3153832671262227771 ) ) ;
#81200=CARTESIAN_POINT ( 'NONE',  ( -1.351706036745406347, 0.05413385826771626580, -0.4176697321401330321 ) ) ;
#81201=CARTESIAN_POINT ( 'NONE',  ( -1.030183727034119867, -0.2845877964562159024, 0.3641732283464567677 ) ) ;
#81203=CARTESIAN_POINT ( 'NONE',  ( -0.9973753280839886548, -0.6046776061558809534, -0.2411417322834644161 ) ) ;
#81204=CARTESIAN_POINT ( 'NONE',  ( -0.3346456692913377662, 0.1660481256975883668, -0.3530559997133364547 ) ) ;
#81205=CARTESIAN_POINT ( 'NONE',  ( 0.3018372703412079971, 0.05413385826771626580, -0.4176697321401330321 ) ) ;
#81207=CARTESIAN_POINT ( 'NONE',  ( 0.1509186351706045259, -0.08942795157528024563, -0.3641732283464568787 ) ) ;
#81208=CARTESIAN_POINT ( 'NONE',  ( -1.653543307086613234, -0.1870078740157480601, -0.3641732283464567677 ) ) ;
#81209=CARTESIAN_POINT ( 'NONE',  ( 0.8398950131233602345, -0.6046776061558807314, 0.2411417322834647770 ) ) ;
#81210=CARTESIAN_POINT ( 'NONE',  ( -1.561679790026246017, -0.004921259842519576551, 0.3153832671262227771 ) ) ;
#81211=CARTESIAN_POINT ( 'NONE',  ( 1.286089238845145033, 0.1283753931104748280, 0.1820866141732283561 ) ) ;
#81212=CARTESIAN_POINT ( 'NONE',  ( -1.062992125984250968, 0.2952755905511811885, 0.000000000000000000 ) ) ;
#81213=CARTESIAN_POINT ( 'NONE',  ( -0.2362204724409440182, -0.1870078740157479769, 0.3641732283464567677 ) ) ;
#81215=CARTESIAN_POINT ( 'NONE',  ( 0.05249343832021075018, 0.1283753931104746893, -0.1820866141732285504 ) ) ;
#81216=CARTESIAN_POINT ( 'NONE',  ( -0.03280839895013062252, 0.2952755905511810774, -0.1292274648535930714 ) ) ;
#81219=CARTESIAN_POINT ( 'NONE',  ( 0.6627296587926515548, 0.1771653543307087630, 0.09757992244046791164 ) ) ;
#81220=CARTESIAN_POINT ( 'NONE',  ( 0.1246719160104994284, 0.2952755905511810774, -0.1292274648535930714 ) ) ;
#81221=CARTESIAN_POINT ( 'NONE',  ( -0.5643044619422565855, -0.4281496062992124485, 0.4176697321401328655 ) ) ;
#81222=CARTESIAN_POINT ( 'NONE',  ( -0.6561679790026240244, 0.1283753931104746893, -0.1820866141732285504 ) ) ;
#81224=CARTESIAN_POINT ( 'NONE',  ( -0.5183727034120726440, 0.1771653543307087630, 0.09757992244046791164 ) ) ;
#81225=CARTESIAN_POINT ( 'NONE',  ( 0.07217847769028949700, -0.3162353388693405765, 0.4822834645669290543 ) ) ;
#81226=CARTESIAN_POINT ( 'NONE',  ( -1.213910761154854745, 0.1771653543307087075, -0.09757992244046823083 ) ) ;
#81228=CARTESIAN_POINT ( 'NONE',  ( 1.509186351706037543, -0.4281496062992127816, -0.4176697321401328100 ) ) ;
#81229=CARTESIAN_POINT ( 'NONE',  ( 0.4605079024601035909, 2.141871057760741033E-18, -0.3627985898453511826 ) ) ;
#81230=EDGE_LOOP ( 'NONE', ( #10128, #19877, #60839, #38389 ) ) ;
#81232=CARTESIAN_POINT ( 'NONE',  ( -1.594488188976377563, -0.4536011799217367080, 0.2665933059059888421 ) ) ;
#81233=CARTESIAN_POINT ( 'NONE',  ( -0.3018372703412066094, 0.05413385826771666132, 0.4176697321401328100 ) ) ;
#81234=CARTESIAN_POINT ( 'NONE',  ( -0.9908136482939626788, 0.2952755905511811885, 0.1292274648535926551 ) ) ;
#81236=CYLINDRICAL_SURFACE ( 'NONE', #22988, 2.362204724409449508 ) ;
#81237=CARTESIAN_POINT ( 'NONE',  ( 1.391076115485564868, 0.2306618581243847221, -0.2411417322834647770 ) ) ;
#81238=CARTESIAN_POINT ( 'NONE',  ( 0.2427821522309719648, -0.05778040916215522460, 0.4822834645669289988 ) ) ;
#81241=CARTESIAN_POINT ( 'NONE',  ( 1.509186351706037543, -0.3690944881889765550, -0.3153832671262227771 ) ) ;
#81243=ORIENTED_EDGE ( 'NONE', *, *, #2315, .F. ) ;
#81244=CARTESIAN_POINT ( 'NONE',  ( -1.036745406824146176, -0.3690944881889763329, 0.3153832671262228327 ) ) ;
#81245=AXIS2_PLACEMENT_3D ( 'NONE', #73383, #34668, #60331 ) ;
#81247=VERTEX_POINT ( 'NONE', #44674 ) ;
#81248=CARTESIAN_POINT ( 'NONE',  ( 0.3083989501312343062, -0.3162353388693405765, 0.4822834645669290543 ) ) ;
#81249=CARTESIAN_POINT ( 'NONE',  ( -0.5643044619422565855, 0.05413385826771626580, -0.4176697321401330321 ) ) ;
#81250=CARTESIAN_POINT ( 'NONE',  ( -1.010498687664041384, 0.05413385826771666132, 0.4176697321401328100 ) ) ;
#81251=CARTESIAN_POINT ( 'NONE',  ( 1.272965879265092637, -0.4281496062992127816, -0.4176697321401328100 ) ) ;
#81252=CARTESIAN_POINT ( 'NONE',  ( -1.410761154855641575, -0.2845877964562161244, -0.3641732283464567121 ) ) ;
#81253=CARTESIAN_POINT ( 'NONE',  ( -0.8761506516392493227, -2.567464376874931580E-15, -0.4445507791589072832 ) ) ;
#81254=CARTESIAN_POINT ( 'NONE',  ( 0.05249343832021075018, -0.6046776061558807314, 0.2411417322834647770 ) ) ;
#81255=CARTESIAN_POINT ( 'NONE',  ( -1.246719160104985846, -0.4281496062992127816, -0.4176697321401328100 ) ) ;
#81258=DIRECTION ( 'NONE',  ( -0.000000000000000000, 1.000000000000000000, -0.000000000000000000 ) ) ;
#81260=CARTESIAN_POINT ( 'NONE',  ( 1.003937007874016407, -0.4536011799217367080, 0.2665933059059888421 ) ) ;
#81263=CARTESIAN_POINT ( 'NONE',  ( -0.9776902887139098386, 0.2952755905511810774, -0.1292274648535930714 ) ) ;
#81264=ORIENTED_EDGE ( 'NONE', *, *, #67683, .F. ) ;
#81265=CARTESIAN_POINT ( 'NONE',  ( 0.5905511811023629321, -0.5511811023622047445, 6.969142054262312111E-17 ) ) ;
#81266=CARTESIAN_POINT ( 'NONE',  ( -1.719160104986876103, 0.05413385826771666132, 0.4176697321401328100 ) ) ;
#81267=CARTESIAN_POINT ( 'NONE',  ( 0.7283464566929140904, -0.5400638737290845981, -0.3530559997133363437 ) ) ;
#81268=CARTESIAN_POINT ( 'NONE',  ( 0.3871391076115492380, -0.05778040916215560624, -0.4822834645669293319 ) ) ;
#81269=CARTESIAN_POINT ( 'NONE',  ( -0.2230971128608915943, -0.4281496062992127816, -0.4176697321401328100 ) ) ;
#81271=CARTESIAN_POINT ( 'NONE',  ( -0.6167979002624665030, -0.4281496062992127816, -0.4176697321401328100 ) ) ;
#81273=CARTESIAN_POINT ( 'NONE',  ( 1.410761154855643795, -0.2845877964562159024, 0.3641732283464567677 ) ) ;
#81274=CARTESIAN_POINT ( 'NONE',  ( -1.187664041994749731, -0.3162353388693405765, 0.4822834645669290543 ) ) ;
#81275=CARTESIAN_POINT ( 'NONE',  ( 1.181102362204725198, -0.1870078740157479769, 0.4822834645669291653 ) ) ;
#81276=CARTESIAN_POINT ( 'NONE',  ( 1.266404199475066328, -0.3162353388693409650, -0.4822834645669289433 ) ) ;
#81278=CARTESIAN_POINT ( 'NONE',  ( -0.9317585301837263412, 0.05413385826771666132, 0.4176697321401328100 ) ) ;
#81280=CARTESIAN_POINT ( 'NONE',  ( 0.2230971128608929543, 0.05413385826771626580, -0.4176697321401330321 ) ) ;
#81283=B_SPLINE_CURVE_WITH_KNOTS ( 'NONE', 3,
 ( #76802, #7343, #70479, #64177, #63342, #43970, #6924 ),
 .UNSPECIFIED., .F., .F.,
 ( 4, 3, 4 ),
 ( 1.734723475976807094E-18, 0.001246230184515552441, 0.002492489877932635087 ),
 .UNSPECIFIED. ) ;
#81284=CARTESIAN_POINT ( 'NONE',  ( -0.5249343832020990641, 0.2306618581243848609, 0.2411417322834645549 ) ) ;
#81285=CARTESIAN_POINT ( 'NONE',  ( -1.607611548556429737, 0.1771653543307087075, -0.09757992244046823083 ) ) ;
#81286=CARTESIAN_POINT ( 'NONE',  ( 0.7283464566929143125, 0.07958543189024085140, 0.2665933059059887866 ) ) ;
#81287=CARTESIAN_POINT ( 'NONE',  ( 1.174540682414699111, -0.05778040916215560624, -0.4822834645669293319 ) ) ;
#81289=CARTESIAN_POINT ( 'NONE',  ( 0.9383202099737538715, -0.08942795157528024563, -0.3641732283464568787 ) ) ;
#81290=CARTESIAN_POINT ( 'NONE',  ( 0.9448818897637802916, -0.1870078740157479769, 0.4822834645669291653 ) ) ;
#81293=CARTESIAN_POINT ( 'NONE',  ( -0.8136482939632537770, -0.6046776061558807314, 0.2411417322834647770 ) ) ;
#81296=CARTESIAN_POINT ( 'NONE',  ( 0.8530183727034126306, -0.004921259842519870586, -0.3153832671262229437 ) ) ;
#81297=CARTESIAN_POINT ( 'NONE',  ( -0.4986876640419942164, -0.6046776061558807314, 0.2411417322834647770 ) ) ;
#81298=CARTESIAN_POINT ( 'NONE',  ( -0.01968503937007793844, -0.5400638737290844871, 0.3530559997133364547 ) ) ;
#81300=CARTESIAN_POINT ( 'NONE',  ( 0.2559055118110243332, -0.5400638737290845981, -0.3530559997133363437 ) ) ;
#81301=CARTESIAN_POINT ( 'NONE',  ( -0.04593175853018302557, 0.1771653543307087630, 0.09757992244046791164 ) ) ;
#81303=CARTESIAN_POINT ( 'NONE',  ( -0.03280839895013062252, 0.1771653543307087075, -0.09757992244046823083 ) ) ;
#81304=CARTESIAN_POINT ( 'NONE',  ( 0.5971128608923890191, -0.5511811023622046335, 0.09757992244046803654 ) ) ;
#81305=CARTESIAN_POINT ( 'NONE',  ( 1.595398199321655275, 1.309738123151863665, 0.1559797534342494407 ) ) ;
#81307=CARTESIAN_POINT ( 'NONE',  ( 0.4724409448818904789, -0.1870078740157480879, -0.4822834645669291653 ) ) ;
#81311=CARTESIAN_POINT ( 'NONE',  ( -0.3149606299212590610, -0.1870078740157479769, 0.3641732283464567677 ) ) ;
#81313=CARTESIAN_POINT ( 'NONE',  ( -0.3805774278215216522, 0.05413385826771666132, 0.4176697321401328100 ) ) ;
#81314=CARTESIAN_POINT ( 'NONE',  ( 0.9317585301837276734, -0.004921259842519870586, -0.3153832671262229437 ) ) ;
#81315=CARTESIAN_POINT ( 'NONE',  ( -1.653543307086613234, -0.1870078740157480601, -0.3641732283464567677 ) ) ;
#81316=CARTESIAN_POINT ( 'NONE',  ( -1.502624671916009680, -0.05778040916215560624, -0.4822834645669293319 ) ) ;
#81317=CARTESIAN_POINT ( 'NONE',  ( -0.006561679790025524116, -0.05778040916215560624, -0.4822834645669293319 ) ) ;
#81318=CARTESIAN_POINT ( 'NONE',  ( 1.227034120734908917, 0.2952755905511810774, -0.1292274648535930714 ) ) ;
#81320=CARTESIAN_POINT ( 'NONE',  ( 0.1509186351706042484, -0.3162353388693405765, 0.4822834645669290543 ) ) ;
#81321=CARTESIAN_POINT ( 'NONE',  ( 1.476377952755906442, -0.5400638737290844871, 0.3530559997133364547 ) ) ;
#81322=CARTESIAN_POINT ( 'NONE',  ( 1.095800524934383846, -0.05778040916215560624, -0.4822834645669293319 ) ) ;
#81323=CARTESIAN_POINT ( 'NONE',  ( -1.719160104986876103, -0.004921259842519576551, 0.3153832671262227771 ) ) ;
#81324=CARTESIAN_POINT ( 'NONE',  ( 0.8858267716535438430, 0.07958543189024085140, 0.2665933059059887866 ) ) ;
#81325=CARTESIAN_POINT ( 'NONE',  ( 1.587926509186352586, -0.4281496062992127816, -0.4176697321401328100 ) ) ;
#81326=CARTESIAN_POINT ( 'NONE',  ( 0.2821522309711292364, -0.5511811023622046335, 0.09757992244046803654 ) ) ;
#81327=CARTESIAN_POINT ( 'NONE',  ( -0.2690288713910754526, -0.6692913385826771977, 0.1292274648535927661 ) ) ;
#81328=CARTESIAN_POINT ( 'NONE',  ( 0.4986876640419954376, 0.2306618581243848609, 0.2411417322834645549 ) ) ;
#81329=CARTESIAN_POINT ( 'NONE',  ( -0.2427821522309703550, -0.3162353388693405765, 0.4822834645669290543 ) ) ;
#81331=CARTESIAN_POINT ( 'NONE',  ( -0.4199475065616791736, 0.1283753931104746893, -0.1820866141732285504 ) ) ;
#81332=CARTESIAN_POINT ( 'NONE',  ( 0.7742782152230978099, -0.4281496062992124485, 0.4176697321401328655 ) ) ;
#81333=CARTESIAN_POINT ( 'NONE',  ( 0.8989501312335964611, 0.1771653543307087630, 0.09757992244046791164 ) ) ;
#81334=CARTESIAN_POINT ( 'NONE',  ( 0.2690288713910767848, 0.2952755905511811885, 0.1292274648535926551 ) ) ;
#81336=CARTESIAN_POINT ( 'NONE',  ( 1.572991167713778227, 1.535433070866141447, 0.1227090857360984416 ) ) ;
#81339=CARTESIAN_POINT ( 'NONE',  ( -1.423884514435694859, -0.05778040916215560624, -0.4822834645669293319 ) ) ;
#81340=CARTESIAN_POINT ( 'NONE',  ( -0.5577427821522301654, -0.05778040916215560624, -0.4822834645669293319 ) ) ;
#81344=CARTESIAN_POINT ( 'NONE',  ( 0.5314960629921267055, -0.4536011799217367080, 0.2665933059059888421 ) ) ;
#81346=CARTESIAN_POINT ( 'NONE',  ( 0.6102362204724416372, -0.5400638737290844871, 0.3530559997133364547 ) ) ;
#81347=EDGE_CURVE ( 'NONE', #72947, #16761, #72585, .T. ) ;
#81349=CARTESIAN_POINT ( 'NONE',  ( 0.5971128608923891301, 0.1771653543307087075, -0.09757992244046823083 ) ) ;
#81350=CARTESIAN_POINT ( 'NONE',  ( 1.603475055217291612, 0.7166759647713490944, 0.04573490813648272563 ) ) ;
#81351=CARTESIAN_POINT ( 'NONE',  ( -1.614173228346456268, -0.5511811023622047445, 6.969142054262312111E-17 ) ) ;
#81352=CARTESIAN_POINT ( 'NONE',  ( 1.653543307086614789, -0.1870078740157479769, 0.4822834645669291653 ) ) ;
#81353=CARTESIAN_POINT ( 'NONE',  ( 1.181102362204724976, -0.1870078740157480601, -0.3641732283464567677 ) ) ;
#81354=CARTESIAN_POINT ( 'NONE',  ( 0.4330708661417329575, 0.2952755905511811885, 0.000000000000000000 ) ) ;
#81356=CARTESIAN_POINT ( 'NONE',  ( -0.4593175853018364174, -0.4281496062992127816, -0.4176697321401328100 ) ) ;
#81357=CARTESIAN_POINT ( 'NONE',  ( -0.7874015748031489847, -0.1870078740157479769, 0.3641732283464567677 ) ) ;
#81358=CARTESIAN_POINT ( 'NONE',  ( 0.5314960629921264834, 0.1660481256975883668, -0.3530559997133364547 ) ) ;
#81359=CARTESIAN_POINT ( 'NONE',  ( 0.03280839895013198948, 0.2952755905511811885, 0.1292274648535926551 ) ) ;
#81363=CARTESIAN_POINT ( 'NONE',  ( 0.7152230971128616943, -0.05778040916215522460, 0.4822834645669289988 ) ) ;
#81364=CARTESIAN_POINT ( 'NONE',  ( -0.4265091863517051496, 0.2952755905511810774, -0.1292274648535930714 ) ) ;
#81365=CARTESIAN_POINT ( 'NONE',  ( -1.332020997375327642, -0.05778040916215522460, 0.4822834645669289988 ) ) ;
#81366=CARTESIAN_POINT ( 'NONE',  ( 1.181102362204724976, -0.1870078740157480879, -0.4822834645669291653 ) ) ;
#81367=CARTESIAN_POINT ( 'NONE',  ( 0.4986876640419954376, -0.6046776061558809534, -0.2411417322834644161 ) ) ;
#81369=CARTESIAN_POINT ( 'NONE',  ( -0.2821522309711278487, 0.2952755905511811885, 0.1292274648535926551 ) ) ;
#81370=CARTESIAN_POINT ( 'NONE',  ( 0.1640419947506569498, -0.3162353388693409650, -0.4822834645669289433 ) ) ;
#81371=CARTESIAN_POINT ( 'NONE',  ( -0.3149606299212590610, -0.1870078740157480879, -0.4822834645669291653 ) ) ;
#81372=CARTESIAN_POINT ( 'NONE',  ( 0.3280839895013130669, -0.3690944881889765550, -0.3153832671262227771 ) ) ;
#81373=CARTESIAN_POINT ( 'NONE',  ( -1.653543307086613234, -0.1870078740157480879, -0.4822834645669291653 ) ) ;
#81375=CARTESIAN_POINT ( 'NONE',  ( 0.4265091863517067039, -0.6692913385826773087, -0.1292274648535924053 ) ) ;
#81377=CARTESIAN_POINT ( 'NONE',  ( -1.528871391076114250, -0.6692913385826771977, 0.1292274648535927661 ) ) ;
#81380=EDGE_LOOP ( 'NONE', ( #60770, #52119, #82779, #8875 ) ) ;
#81381=CARTESIAN_POINT ( 'NONE',  ( 0.5314960629921267055, -0.5400638737290844871, 0.3530559997133364547 ) ) ;
#81382=CARTESIAN_POINT ( 'NONE',  ( 0.05249343832021075018, 0.1283753931104746893, -0.1820866141732285504 ) ) ;
#81386=CARTESIAN_POINT ( 'NONE',  ( -0.9552210167251737882, -5.134928753749862370E-15, -0.4281989832122467532 ) ) ;
#81387=CARTESIAN_POINT ( 'NONE',  ( 0.3042614371611548907, -3.790565315793794774E-16, -0.4118477457932737118 ) ) ;
#81389=CARTESIAN_POINT ( 'NONE',  ( 0.5118110236220478892, 0.2952755905511811885, 0.000000000000000000 ) ) ;
#81390=CARTESIAN_POINT ( 'NONE',  ( -0.6889763779527552368, 0.1660481256975885056, 0.3530559997133364547 ) ) ;
#81391=CARTESIAN_POINT ( 'NONE',  ( -0.6036745406824141069, 0.2306618581243848609, 0.2411417322834645549 ) ) ;
#81392=CARTESIAN_POINT ( 'NONE',  ( 0.5839895013123367340, -0.6692913385826773087, -0.1292274648535924053 ) ) ;
#81393=CARTESIAN_POINT ( 'NONE',  ( 1.364829396325459854, -0.6046776061558809534, -0.2411417322834644161 ) ) ;
#81394=CARTESIAN_POINT ( 'NONE',  ( 1.200787401574803681, 0.07958543189024085140, 0.2665933059059887866 ) ) ;
#81396=CARTESIAN_POINT ( 'NONE',  ( 1.108923884514436686, -0.2845877964562161244, -0.3641732283464567121 ) ) ;
#81397=CARTESIAN_POINT ( 'NONE',  ( -0.8005249343832011588, 0.05413385826771626580, -0.4176697321401330321 ) ) ;
#81399=CARTESIAN_POINT ( 'NONE',  ( 1.660104986876641320, -0.05778040916215522460, 0.4822834645669289988 ) ) ;
#81400=DIRECTION ( 'NONE',  ( -0.000000000000000000, 1.000000000000000000, -0.000000000000000000 ) ) ;
#81401=CARTESIAN_POINT ( 'NONE',  ( -0.1443569553805765515, -0.4281496062992127816, -0.4176697321401328100 ) ) ;
#81402=CARTESIAN_POINT ( 'NONE',  ( 0.9908136482939640111, -0.6692913385826771977, 0.1292274648535927661 ) ) ;
#81404=CARTESIAN_POINT ( 'NONE',  ( -1.181102362204723644, -0.1870078740157480601, -0.3641732283464567677 ) ) ;
#81405=CARTESIAN_POINT ( 'NONE',  ( 0.3937007874015754361, -0.1870078740157479769, 0.4822834645669291653 ) ) ;
#81406=CARTESIAN_POINT ( 'NONE',  ( 0.7086614173228352742, -0.1870078740157480601, -0.3641732283464567677 ) ) ;
#81408=CARTESIAN_POINT ( 'NONE',  ( -1.299212598425196097, -0.5511811023622047445, 6.969142054262312111E-17 ) ) ;
#81409=CARTESIAN_POINT ( 'NONE',  ( 1.345144356955381593, -0.05778040916215522460, 0.4822834645669289988 ) ) ;
#81411=CARTESIAN_POINT ( 'NONE',  ( -0.1771653543307080136, -0.4536011799217367080, 0.2665933059059888421 ) ) ;
#81412=CARTESIAN_POINT ( 'NONE',  ( -0.1181102362204717315, 0.2952755905511811885, 0.000000000000000000 ) ) ;
#81413=CARTESIAN_POINT ( 'NONE',  ( -1.213910761154854745, -0.5511811023622046335, 0.09757992244046803654 ) ) ;
#81415=CARTESIAN_POINT ( 'NONE',  ( -0.5839895013123351797, 0.2952755905511810774, -0.1292274648535930714 ) ) ;
#81416=CARTESIAN_POINT ( 'NONE',  ( 1.318897637795276356, -0.5400638737290844871, 0.3530559997133364547 ) ) ;
#81418=CARTESIAN_POINT ( 'NONE',  ( -0.9776902887139098386, 0.1771653543307087075, -0.09757992244046823083 ) ) ;
#81420=CARTESIAN_POINT ( 'NONE',  ( 1.509186351706037543, -0.4281496062992127816, -0.4176697321401328100 ) ) ;
#81423=CARTESIAN_POINT ( 'NONE',  ( -1.122047244094487306, -0.5400638737290844871, 0.3530559997133364547 ) ) ;
#81424=CARTESIAN_POINT ( 'NONE',  ( -1.279527559055116948, 0.07958543189024071263, -0.2665933059059888421 ) ) ;
#81425=CARTESIAN_POINT ( 'NONE',  ( -0.6955380577427815458, -0.3690944881889765550, -0.3153832671262227771 ) ) ;
#81427=CARTESIAN_POINT ( 'NONE',  ( 8.195543980992789655E-16, -0.1870078740157480879, -0.4822834645669291653 ) ) ;
#81428=CARTESIAN_POINT ( 'NONE',  ( -0.1706036745406816491, -0.004921259842519870586, -0.3153832671262229437 ) ) ;
#81429=CARTESIAN_POINT ( 'NONE',  ( -1.272965879265091305, -0.3690944881889763329, 0.3153832671262228327 ) ) ;
#81430=CARTESIAN_POINT ( 'NONE',  ( -1.391076115485563758, 0.2306618581243848609, 0.2411417322834645549 ) ) ;
#81431=CARTESIAN_POINT ( 'NONE',  ( 1.246719160104987623, -0.3690944881889763329, 0.3153832671262228327 ) ) ;
#81432=CARTESIAN_POINT ( 'NONE',  ( 1.154855643044620184, -0.6046776061558807314, 0.2411417322834647770 ) ) ;
#81433=CARTESIAN_POINT ( 'NONE',  ( -1.614173228346457378, 0.5038684218300933937, -0.1372047244094477536 ) ) ;
#81434=CARTESIAN_POINT ( 'NONE',  ( 0.4330708661417329575, 0.1771653543307087630, 0.000000000000000000 ) ) ;
#81435=CARTESIAN_POINT ( 'NONE',  ( 0.9908136482939640111, -0.6692913385826771977, 0.1292274648535927661 ) ) ;
#81436=CARTESIAN_POINT ( 'NONE',  ( 0.8464566929133865436, 0.07958543189024071263, -0.2665933059059888421 ) ) ;
#81438=CARTESIAN_POINT ( 'NONE',  ( -1.253280839895012377, -0.3162353388693409650, -0.4822834645669289433 ) ) ;
#81439=EDGE_CURVE ( 'NONE', #35380, #76682, #13151, .T. ) ;
#81440=CARTESIAN_POINT ( 'NONE',  ( -0.7020997375328074108, -0.05778040916215522460, 0.4822834645669289988 ) ) ;
#81441=CARTESIAN_POINT ( 'NONE',  ( 0.1049868766404206816, -0.6046776061558809534, -0.2411417322834644161 ) ) ;
#81442=CARTESIAN_POINT ( 'NONE',  ( -1.646051170424378096, 0.000000000000000000, -0.3464511005275205946 ) ) ;
#81444=CARTESIAN_POINT ( 'NONE',  ( 1.043307086614173818, -0.5400638737290845981, -0.3530559997133363437 ) ) ;
#81445=CARTESIAN_POINT ( 'NONE',  ( 1.482939632545932307, -0.004921259842519870586, -0.3153832671262229437 ) ) ;
#81446=CARTESIAN_POINT ( 'NONE',  ( 0.1574803149606306130, -0.1870078740157480879, -0.4822834645669291653 ) ) ;
#81447=CARTESIAN_POINT ( 'NONE',  ( 0.6627296587926515548, 0.2952755905511811885, 0.1292274648535926551 ) ) ;
#81451=CARTESIAN_POINT ( 'NONE',  ( -0.5636006452641416642, -2.613618158232546091E-15, -0.3464511005275220379 ) ) ;
#81453=CARTESIAN_POINT ( 'NONE',  ( -0.5577427821522301654, -0.08942795157528024563, -0.3641732283464568787 ) ) ;
#81454=CARTESIAN_POINT ( 'NONE',  ( -0.6299212598425188991, -0.1870078740157479769, 0.4822834645669291653 ) ) ;
#81455=CARTESIAN_POINT ( 'NONE',  ( 0.6627296587926515548, 0.2952755905511811885, 0.1292274648535926551 ) ) ;
#81457=CARTESIAN_POINT ( 'NONE',  ( 0.8989501312335964611, 0.2952755905511811885, 0.1292274648535926551 ) ) ;
#81458=CARTESIAN_POINT ( 'NONE',  ( -1.417322834645668772, -0.1870078740157480879, -0.4822834645669291653 ) ) ;
#81459=CARTESIAN_POINT ( 'NONE',  ( 1.213910761154856299, -0.6692913385826773087, -0.1292274648535924053 ) ) ;
#81462=CARTESIAN_POINT ( 'NONE',  ( 0.9186351706036751663, -0.6046776061558807314, 0.2411417322834647770 ) ) ;
#81463=CARTESIAN_POINT ( 'NONE',  ( 0.6036745406824153282, -0.6046776061558807314, 0.2411417322834647770 ) ) ;
#81464=CARTESIAN_POINT ( 'NONE',  ( 1.095800524934383846, -0.2845877964562159024, 0.3641732283464567677 ) ) ;
#81465=CARTESIAN_POINT ( 'NONE',  ( -1.528871391076114250, -0.5511811023622046335, 0.09757992244046803654 ) ) ;
#81466=CARTESIAN_POINT ( 'NONE',  ( -1.561679790026246017, -0.4281496062992127816, -0.4176697321401328100 ) ) ;
#81469=CARTESIAN_POINT ( 'NONE',  ( 0.9645669291338591078, -0.5400638737290845981, -0.3530559997133363437 ) ) ;
#81470=CARTESIAN_POINT ( 'NONE',  ( 1.568241469816273659, -0.08942795157528024563, -0.3641732283464568787 ) ) ;
#81471=CARTESIAN_POINT ( 'NONE',  ( -0.5708661417322828946, 0.1660481256975883668, -0.3530559997133364547 ) ) ;
#81472=CARTESIAN_POINT ( 'NONE',  ( -0.7545931758530177724, 0.2952755905511811885, 0.1292274648535926551 ) ) ;
#81473=CARTESIAN_POINT ( 'NONE',  ( 1.397637795275591177, -0.5400638737290844871, 0.3530559997133364547 ) ) ;
#81475=CARTESIAN_POINT ( 'NONE',  ( 0.4068241469816279987, -0.4281496062992127816, -0.4176697321401328100 ) ) ;
#81477=CARTESIAN_POINT ( 'NONE',  ( -1.561679790026246017, -0.3690944881889765550, -0.3153832671262227771 ) ) ;
#81478=ORIENTED_EDGE ( 'NONE', *, *, #78936, .F. ) ;
#81482=CIRCLE ( 'NONE', #78787, 0.4822834645669291653 ) ;
#81483=CARTESIAN_POINT ( 'NONE',  ( 1.181102362204724976, -0.1870078740157480601, -0.3641732283464567677 ) ) ;
#81485=CARTESIAN_POINT ( 'NONE',  ( 1.541994750656168645, 0.1771653543307087075, -0.09757992244046823083 ) ) ;
#81490=CARTESIAN_POINT ( 'NONE',  ( -0.5708661417322825615, -0.4536011799217367080, 0.2665933059059888421 ) ) ;
#81491=CARTESIAN_POINT ( 'NONE',  ( -1.062992125984250968, 0.1771653543307087630, 0.000000000000000000 ) ) ;
#81492=CARTESIAN_POINT ( 'NONE',  ( 1.443569553805774897, 0.2306618581243848609, 0.2411417322834645549 ) ) ;
#81493=CARTESIAN_POINT ( 'NONE',  ( 0.6102362204724416372, -0.5400638737290844871, 0.3530559997133364547 ) ) ;
#81494=CARTESIAN_POINT ( 'NONE',  ( -1.154855643044618851, 0.2306618581243848609, 0.2411417322834645549 ) ) ;
#81497=CARTESIAN_POINT ( 'NONE',  ( 1.377952755905512472, -0.6692913385826771977, 8.415575281601705876E-17 ) ) ;
#81502=CARTESIAN_POINT ( 'NONE',  ( -0.5380577427821514602, 0.05413385826771666132, 0.4176697321401328100 ) ) ;
#81503=CARTESIAN_POINT ( 'NONE',  ( 0.8595800524934390507, -0.3162353388693405765, 0.4822834645669290543 ) ) ;
#81506=CARTESIAN_POINT ( 'NONE',  ( -1.633858267716534529, -0.5400638737290845981, -0.3530559997133363437 ) ) ;
#81507=CARTESIAN_POINT ( 'NONE',  ( -0.9251968503937002541, 0.1660481256975885056, 0.3530559997133364547 ) ) ;
#81509=CARTESIAN_POINT ( 'NONE',  ( 0.1443569553805781891, -0.3690944881889763329, 0.3153832671262228327 ) ) ;
#81511=CARTESIAN_POINT ( 'NONE',  ( 0.006561679790026889343, -0.2845877964562161244, -0.3641732283464567121 ) ) ;
#81512=CARTESIAN_POINT ( 'NONE',  ( 0.6692913385826777528, 0.1771653543307087630, 0.000000000000000000 ) ) ;
#81514=CARTESIAN_POINT ( 'NONE',  ( 0.4330708661417329575, -0.6692913385826771977, 8.415575281601705876E-17 ) ) ;
#81515=CARTESIAN_POINT ( 'NONE',  ( -0.8661417322834640276, -0.1870078740157479769, 0.3641732283464567677 ) ) ;
#81517=CARTESIAN_POINT ( 'NONE',  ( -1.627296587926508442, 0.2306618581243848609, 0.2411417322834645549 ) ) ;
#81519=CARTESIAN_POINT ( 'NONE',  ( -1.128608923884513837, 0.2306618581243847221, -0.2411417322834647770 ) ) ;
#81520=CONICAL_SURFACE ( 'NONE', #62694, 1.181102362204724310, 0.7853981633974621568 ) ;
#81522=CARTESIAN_POINT ( 'NONE',  ( 0.1377952755905518800, -0.5400638737290844871, 0.3530559997133364547 ) ) ;
#81523=CARTESIAN_POINT ( 'NONE',  ( -0.5577427821522301654, -0.3162353388693405765, 0.4822834645669290543 ) ) ;
#81524=CARTESIAN_POINT ( 'NONE',  ( 1.043307086614173818, 0.07958543189024085140, 0.2665933059059887866 ) ) ;
#81525=CARTESIAN_POINT ( 'NONE',  ( -0.06561679790026180015, -0.3690944881889765550, -0.3153832671262227771 ) ) ;
#81526=CARTESIAN_POINT ( 'NONE',  ( -0.1181102362204717315, 0.2952755905511811885, 0.000000000000000000 ) ) ;
#81527=CARTESIAN_POINT ( 'NONE',  ( -1.213910761154854745, -0.6692913385826771977, 0.1292274648535927661 ) ) ;
#81530=CARTESIAN_POINT ( 'NONE',  ( 0.1640419947506569498, -0.3162353388693409650, -0.4822834645669289433 ) ) ;
#81531=ORIENTED_EDGE ( 'NONE', *, *, #76698, .F. ) ;
#81533=CARTESIAN_POINT ( 'NONE',  ( 1.345144356955381593, -0.3162353388693409650, -0.4822834645669289433 ) ) ;
#81534=CARTESIAN_POINT ( 'NONE',  ( -0.7480314960629914633, 0.1771653543307087630, 0.000000000000000000 ) ) ;
#81536=CARTESIAN_POINT ( 'NONE',  ( -0.3740157480314953431, -0.5400638737290845981, -0.3530559997133363437 ) ) ;
#81537=CARTESIAN_POINT ( 'NONE',  ( 1.102362204724410155, -0.1870078740157480879, -0.4822834645669291653 ) ) ;
#81538=CARTESIAN_POINT ( 'NONE',  ( 1.089238845144357759, 0.05413385826771626580, -0.4176697321401330321 ) ) ;
#81539=CARTESIAN_POINT ( 'NONE',  ( -1.548556430446193399, -0.6046776061558809534, -0.2411417322834644161 ) ) ;
#81540=CARTESIAN_POINT ( 'NONE',  ( -1.220472440944881054, 0.1771653543307087630, 0.000000000000000000 ) ) ;
#81545=CARTESIAN_POINT ( 'NONE',  ( 1.437007874015748810, -0.4536011799217368745, -0.2665933059059886201 ) ) ;
#81546=CARTESIAN_POINT ( 'NONE',  ( 0.7742782152230978099, -0.3690944881889763329, 0.3153832671262228327 ) ) ;
#81547=CARTESIAN_POINT ( 'NONE',  ( 0.5249343832021003964, 0.2306618581243847221, -0.2411417322834647770 ) ) ;
#81550=CARTESIAN_POINT ( 'NONE',  ( 0.9776902887139113929, -0.5511811023622048555, -0.09757992244046775898 ) ) ;
#81551=CARTESIAN_POINT ( 'NONE',  ( -0.4396325459317577122, -0.6692913385826773087, -0.1292274648535924053 ) ) ;
#81552=CARTESIAN_POINT ( 'NONE',  ( -0.6561679790026240244, 0.2306618581243847221, -0.2411417322834647770 ) ) ;
#81553=CARTESIAN_POINT ( 'NONE',  ( 1.279527559055118724, -0.5400638737290845981, -0.3530559997133363437 ) ) ;
#81556=CARTESIAN_POINT ( 'NONE',  ( -0.2427821522309703550, -0.08942795157528024563, -0.3641732283464568787 ) ) ;
#81557=EDGE_CURVE ( 'NONE', #41461, #42318, #24776, .T. ) ;
#81558=VERTEX_POINT ( 'NONE', #59003 ) ;
#81561=CARTESIAN_POINT ( 'NONE',  ( -0.8661417322834640276, -0.1870078740157480879, -0.4822834645669291653 ) ) ;
#81562=CARTESIAN_POINT ( 'NONE',  ( -0.08530183727034056085, -0.3162353388693405765, 0.4822834645669290543 ) ) ;
#81563=CARTESIAN_POINT ( 'NONE',  ( -0.1443569553805765515, -0.4281496062992127816, -0.4176697321401328100 ) ) ;
#81564=CARTESIAN_POINT ( 'NONE',  ( 0.4002624671916016896, -0.05778040916215522460, 0.4822834645669289988 ) ) ;
#81566=CARTESIAN_POINT ( 'NONE',  ( -0.4265091863517051496, -0.6692913385826771977, 0.1292274648535927661 ) ) ;
#81567=CARTESIAN_POINT ( 'NONE',  ( -1.305774278215222184, 0.2952755905511811885, 0.1292274648535926551 ) ) ;
#81568=CARTESIAN_POINT ( 'NONE',  ( -0.9055118110236215490, 0.2952755905511811885, 0.000000000000000000 ) ) ;
#81569=CARTESIAN_POINT ( 'NONE',  ( 0.6955380577427828781, 0.05413385826771626580, -0.4176697321401330321 ) ) ;
#81570=CARTESIAN_POINT ( 'NONE',  ( 0.6824146981627303710, 0.2306618581243847221, -0.2411417322834647770 ) ) ;
#81572=CARTESIAN_POINT ( 'NONE',  ( -0.2821522309711278487, -0.5511811023622048555, -0.09757992244046775898 ) ) ;
#81575=VECTOR ( 'NONE', #70401, 39.37007874015748143 ) ;
#81576=ORIENTED_EDGE ( 'NONE', *, *, #3360, .T. ) ;
#81577=CARTESIAN_POINT ( 'NONE',  ( -1.351706036745406347, -0.004921259842519870586, -0.3153832671262229437 ) ) ;
#81580=CARTESIAN_POINT ( 'NONE',  ( -0.4396325459317577122, -0.6692913385826773087, -0.1292274648535924053 ) ) ;
#81582=CARTESIAN_POINT ( 'NONE',  ( -0.4921259842519677963, -0.5400638737290844871, 0.3530559997133364547 ) ) ;
#81583=CARTESIAN_POINT ( 'NONE',  ( -0.9645669291338575535, -0.5400638737290844871, 0.3530559997133364547 ) ) ;
#81584=CARTESIAN_POINT ( 'NONE',  ( -1.587926509186350810, 0.05413385826771626580, -0.4176697321401330321 ) ) ;
#81586=CARTESIAN_POINT ( 'NONE',  ( 0.8727034120734913358, -0.08942795157527998196, 0.3641732283464567121 ) ) ;
#81589=CARTESIAN_POINT ( 'NONE',  ( 0.1443569553805781891, -0.3690944881889763329, 0.3153832671262228327 ) ) ;
#81590=CARTESIAN_POINT ( 'NONE',  ( -0.2755905511811015396, -0.6692913385826771977, 8.415575281601705876E-17 ) ) ;
#81592=CARTESIAN_POINT ( 'NONE',  ( -0.03937007874015669567, 0.2952755905511811885, 0.000000000000000000 ) ) ;
#81595=DIRECTION ( 'NONE',  ( 0.000000000000000000, 1.000000000000000000, 0.000000000000000000 ) ) ;
#81599=CARTESIAN_POINT ( 'NONE',  ( -0.5118110236220466680, -0.5511811023622047445, 6.969142054262312111E-17 ) ) ;
#81600=CARTESIAN_POINT ( 'NONE',  ( -0.8267716535433065062, -0.6692913385826771977, 8.415575281601705876E-17 ) ) ;
#81605=CARTESIAN_POINT ( 'NONE',  ( 1.207349081364829990, 0.2306618581243848609, 0.2411417322834645549 ) ) ;
#81606=CARTESIAN_POINT ( 'NONE',  ( 0.4330708661417329575, -0.6692913385826771977, 8.415575281601705876E-17 ) ) ;
#81607=CARTESIAN_POINT ( 'NONE',  ( 0.5446194225721792126, -0.3162353388693405765, 0.4822834645669290543 ) ) ;
#81608=CARTESIAN_POINT ( 'NONE',  ( -0.6496062992125976043, 0.07958543189024071263, -0.2665933059059888421 ) ) ;
#81609=B_SPLINE_CURVE_WITH_KNOTS ( 'NONE', 3,
 ( #53755, #24664, #48689, #80708, #30578, #55821, #42781 ),
 .UNSPECIFIED., .F., .F.,
 ( 4, 3, 4 ),
 ( 7.459310946700270506E-17, 0.001246232571205254649, 0.002492492258783168303 ),
 .UNSPECIFIED. ) ;
#81610=CARTESIAN_POINT ( 'NONE',  ( -0.3280839895013117347, -0.4281496062992124485, 0.4176697321401328655 ) ) ;
#81612=CARTESIAN_POINT ( 'NONE',  ( -1.049868766404198794, 0.2306618581243847221, -0.2411417322834647770 ) ) ;
#81613=ADVANCED_FACE ( 'NONE', ( #38801 ), #4101, .F. ) ;
#81615=CARTESIAN_POINT ( 'NONE',  ( 1.266404199475066328, -0.08942795157527998196, 0.3641732283464567121 ) ) ;
#81616=CARTESIAN_POINT ( 'NONE',  ( -0.1443569553805768291, -0.004921259842519576551, 0.3153832671262227771 ) ) ;
#81617=CARTESIAN_POINT ( 'NONE',  ( 1.056430446194226658, 0.1771653543307087630, 0.09757992244046791164 ) ) ;
#81618=CARTESIAN_POINT ( 'NONE',  ( -1.574803149606298636, -0.1870078740157479769, 0.4822834645669291653 ) ) ;
#81619=CARTESIAN_POINT ( 'NONE',  ( -1.049868766404198794, -0.5023911411419708095, 0.1820866141732285504 ) ) ;
#81620=DIRECTION ( 'NONE',  ( -0.000000000000000000, -1.000000000000000000, -0.000000000000000000 ) ) ;
#81621=CARTESIAN_POINT ( 'NONE',  ( 0.6430446194225729606, -0.3690944881889765550, -0.3153832671262227771 ) ) ;
#81622=CARTESIAN_POINT ( 'NONE',  ( -0.2952755905511803003, -0.5400638737290845981, -0.3530559997133363437 ) ) ;
#81623=EDGE_CURVE ( 'NONE', #36505, #41893, #15044, .T. ) ;
#81624=CARTESIAN_POINT ( 'NONE',  ( 0.2493438320209980519, 0.05413385826771666132, 0.4176697321401328100 ) ) ;
#81625=CARTESIAN_POINT ( 'NONE',  ( -0.2690288713910754526, -0.5511811023622046335, 0.09757992244046803654 ) ) ;
#81626=B_SPLINE_CURVE_WITH_KNOTS ( 'NONE', 3,
 ( #6849, #51441, #77144, #45129 ),
 .UNSPECIFIED., .F., .F.,
 ( 4, 4 ),
 ( 1.999999999927407068E-07, 0.006970199999999936863 ),
 .UNSPECIFIED. ) ;
#81628=CARTESIAN_POINT ( 'NONE',  ( 0.8595800524934390507, -0.3162353388693405765, 0.4822834645669290543 ) ) ;
#81630=CARTESIAN_POINT ( 'NONE',  ( 1.181102362204724976, -0.1870078740157480601, -0.3641732283464567677 ) ) ;
#81631=CARTESIAN_POINT ( 'NONE',  ( -0.9383202099737524282, -0.05778040916215522460, 0.4822834645669289988 ) ) ;
#81632=CARTESIAN_POINT ( 'NONE',  ( -0.2690288713910754526, -0.5511811023622046335, 0.09757992244046803654 ) ) ;
#81633=CARTESIAN_POINT ( 'NONE',  ( -0.7426113562971994320, 1.972848275015058439, 0.5309055118110236338 ) ) ;
#81634=CARTESIAN_POINT ( 'NONE',  ( 0.3805774278215230400, -0.004921259842519870586, -0.3153832671262229437 ) ) ;
#81636=CARTESIAN_POINT ( 'NONE',  ( -0.3280839895013117347, 0.05413385826771626580, -0.4176697321401330321 ) ) ;
#81640=CARTESIAN_POINT ( 'NONE',  ( 0.7020997375328090762, -0.08942795157528024563, -0.3641732283464568787 ) ) ;
#81641=CARTESIAN_POINT ( 'NONE',  ( -0.2690288713910754526, -0.6692913385826771977, 0.1292274648535927661 ) ) ;
#81643=CARTESIAN_POINT ( 'NONE',  ( -0.8727034120734901146, -0.3162353388693405765, 0.4822834645669290543 ) ) ;
#81644=CARTESIAN_POINT ( 'NONE',  ( -0.8727034120734901146, -0.2845877964562159024, 0.3641732283464567677 ) ) ;
#81645=DIRECTION ( 'NONE',  ( -1.000000000000000000, -3.083952846180990774E-16, 0.000000000000000000 ) ) ;
#81646=CARTESIAN_POINT ( 'NONE',  ( -0.1902887139107604098, 0.2952755905511810774, -0.1292274648535930714 ) ) ;
#81647=CARTESIAN_POINT ( 'NONE',  ( -1.181102362204723644, -0.1870078740157480601, -0.3641732283464567677 ) ) ;
#81648=CARTESIAN_POINT ( 'NONE',  ( -1.581364829396324945, -0.05778040916215560624, -0.4822834645669293319 ) ) ;
#81651=CARTESIAN_POINT ( 'NONE',  ( -1.377952755905511140, 0.1771653543307087630, 0.000000000000000000 ) ) ;
#81652=CARTESIAN_POINT ( 'NONE',  ( -1.338582677165353729, -0.1870078740157480879, -0.4822834645669291653 ) ) ;
#81653=CARTESIAN_POINT ( 'NONE',  ( -0.5446194225721777693, -0.3162353388693409650, -0.4822834645669289433 ) ) ;
#81654=CARTESIAN_POINT ( 'NONE',  ( -1.102362204724408601, -0.1870078740157480879, -0.4822834645669291653 ) ) ;
#81657=CARTESIAN_POINT ( 'NONE',  ( 0.9776902887139113929, -0.6692913385826773087, -0.1292274648535924053 ) ) ;
#81658=CARTESIAN_POINT ( 'NONE',  ( 0.4396325459317593221, 0.2952755905511810774, -0.1292274648535930714 ) ) ;
#81661=CARTESIAN_POINT ( 'NONE',  ( 1.220472440944882386, -0.5511811023622047445, 6.969142054262312111E-17 ) ) ;
#81665=CARTESIAN_POINT ( 'NONE',  ( -0.9514435695538050464, -0.08942795157528024563, -0.3641732283464568787 ) ) ;
#81668=CARTESIAN_POINT ( 'NONE',  ( 0.2165354330708668673, 0.1660481256975883668, -0.3530559997133364547 ) ) ;
#81669=CARTESIAN_POINT ( 'NONE',  ( -0.3740157480314953431, -0.5400638737290845981, -0.3530559997133363437 ) ) ;
#81670=CARTESIAN_POINT ( 'NONE',  ( -1.115485564304461219, 0.05413385826771626580, -0.4176697321401330321 ) ) ;
#81671=CARTESIAN_POINT ( 'NONE',  ( 1.253280839895013710, -0.05778040916215560624, -0.4822834645669293319 ) ) ;
#81672=CARTESIAN_POINT ( 'NONE',  ( 1.561679790026247350, 0.05413385826771626580, -0.4176697321401330321 ) ) ;
#81673=CARTESIAN_POINT ( 'NONE',  ( 0.09023630363248136277, 7.699586553780600482E-16, 0.3791483426435171555 ) ) ;
#81674=CARTESIAN_POINT ( 'NONE',  ( -0.1246719160104980823, -0.6692913385826773087, -0.1292274648535924053 ) ) ;
#81675=CARTESIAN_POINT ( 'NONE',  ( -1.358267716535432434, -0.5400638737290844871, 0.3530559997133364547 ) ) ;
#81677=CARTESIAN_POINT ( 'NONE',  ( -1.456692913385826182, 0.2952755905511811885, 0.000000000000000000 ) ) ;
#81678=DIRECTION ( 'NONE',  ( -3.114085624724525612E-16, 1.000000000000000000, 5.270319453084425600E-32 ) ) ;
#81680=CARTESIAN_POINT ( 'NONE',  ( 0.7545931758530189937, 0.1771653543307087075, -0.09757992244046823083 ) ) ;
#81683=CARTESIAN_POINT ( 'NONE',  ( -1.043307086614172041, -0.5400638737290844871, 0.3530559997133364547 ) ) ;
#81685=CARTESIAN_POINT ( 'NONE',  ( -0.07874015748031421014, -0.1870078740157480601, -0.3641732283464567677 ) ) ;
#81686=CARTESIAN_POINT ( 'NONE',  ( -1.607611548556429737, -0.6692913385826771977, 0.1292274648535927661 ) ) ;
#81687=CARTESIAN_POINT ( 'NONE',  ( 0.5511811023622054106, -0.1870078740157480879, -0.4822834645669291653 ) ) ;
#81688=CARTESIAN_POINT ( 'NONE',  ( 0.4790026246719167324, -0.05778040916215522460, 0.4822834645669289988 ) ) ;
#81689=CARTESIAN_POINT ( 'NONE',  ( -0.4790026246719154557, -0.3162353388693405765, 0.4822834645669290543 ) ) ;
#81691=CARTESIAN_POINT ( 'NONE',  ( -0.7874015748031489847, -0.1870078740157480879, -0.4822834645669291653 ) ) ;
#81693=CARTESIAN_POINT ( 'NONE',  ( 1.509186351706037543, -0.3690944881889765550, -0.3153832671262227771 ) ) ;
#81694=CARTESIAN_POINT ( 'NONE',  ( -1.036745406824146176, -0.4281496062992124485, 0.4176697321401328655 ) ) ;
#81695=CARTESIAN_POINT ( 'NONE',  ( 0.7480314960629927956, 0.2952755905511811885, 0.000000000000000000 ) ) ;
#81696=CARTESIAN_POINT ( 'NONE',  ( 1.010498687664042716, -0.4281496062992124485, 0.4176697321401328655 ) ) ;
#81698=CARTESIAN_POINT ( 'NONE',  ( -1.522309711286088607, 0.2306618581243847221, -0.2411417322834647770 ) ) ;
#81700=CARTESIAN_POINT ( 'NONE',  ( 0.4527559055118117182, -0.5400638737290844871, 0.3530559997133364547 ) ) ;
#81703=CARTESIAN_POINT ( 'NONE',  ( -1.548556430446193399, -0.5023911411419708095, -0.1820866141732282451 ) ) ;
#81704=CARTESIAN_POINT ( 'NONE',  ( 0.7808398950131241190, -0.08942795157528024563, -0.3641732283464568787 ) ) ;
#81705=CARTESIAN_POINT ( 'NONE',  ( 0.9711286089238851948, 0.2306618581243848609, 0.2411417322834645549 ) ) ;
#81707=CARTESIAN_POINT ( 'NONE',  ( 0.7020997375328090762, -0.2845877964562159024, 0.3641732283464567677 ) ) ;
#81708=CARTESIAN_POINT ( 'NONE',  ( 0.5052493438320215802, 0.2952755905511811885, 0.1292274648535926551 ) ) ;
#81710=CARTESIAN_POINT ( 'NONE',  ( -0.7020997375328076329, -0.3162353388693409650, -0.4822834645669289433 ) ) ;
#81712=CARTESIAN_POINT ( 'NONE',  ( 1.135170603674541256, 0.1771653543307087630, 0.09757992244046791164 ) ) ;
#81713=CARTESIAN_POINT ( 'NONE',  ( -0.05905511811023545637, -0.5400638737290845981, -0.3530559997133363437 ) ) ;
#81715=CARTESIAN_POINT ( 'NONE',  ( -0.4986876640419942164, -0.6046776061558807314, 0.2411417322834647770 ) ) ;
#81716=CARTESIAN_POINT ( 'NONE',  ( 0.3083989501312343062, -0.08942795157528024563, -0.3641732283464568787 ) ) ;
#81718=CARTESIAN_POINT ( 'NONE',  ( 0.04593175853018440641, -0.5511811023622046335, 0.09757992244046803654 ) ) ;
#81719=CARTESIAN_POINT ( 'NONE',  ( 0.7545931758530188826, -0.5511811023622046335, 0.09757992244046803654 ) ) ;
#81722=CARTESIAN_POINT ( 'NONE',  ( 0.2362204724409456558, -0.1870078740157479769, 0.4822834645669291653 ) ) ;
#81724=CARTESIAN_POINT ( 'NONE',  ( 1.377952755905512472, 0.1771653543307087630, 0.000000000000000000 ) ) ;
#81726=CARTESIAN_POINT ( 'NONE',  ( -0.4133858267716528645, 0.07958543189024071263, -0.2665933059059888421 ) ) ;
#81727=CARTESIAN_POINT ( 'NONE',  ( -0.3871391076115479057, -0.2845877964562161244, -0.3641732283464567121 ) ) ;
#81728=CARTESIAN_POINT ( 'NONE',  ( -0.4133858267716528645, -0.5400638737290844871, 0.3530559997133364547 ) ) ;
#81729=CARTESIAN_POINT ( 'NONE',  ( 0.7939632545931766261, -0.2845877964562161244, -0.3641732283464567121 ) ) ;
#81731=CARTESIAN_POINT ( 'NONE',  ( -1.712598425196849572, 0.1660481256975885056, 0.3530559997133364547 ) ) ;
#81732=CARTESIAN_POINT ( 'NONE',  ( 0.03280839895013198948, -0.6692913385826773087, -0.1292274648535924053 ) ) ;
#81733=CARTESIAN_POINT ( 'NONE',  ( 1.371391076115485941, 0.2952755905511811885, 0.1292274648535926551 ) ) ;
#81735=CARTESIAN_POINT ( 'NONE',  ( 0.2034120734908142214, 0.2952755905511810774, -0.1292274648535930714 ) ) ;
#81737=CARTESIAN_POINT ( 'NONE',  ( 0.7283464566929143125, 0.1660481256975885056, 0.3530559997133364547 ) ) ;
#81738=CARTESIAN_POINT ( 'NONE',  ( 0.7611548556430454138, 0.2306618581243847221, -0.2411417322834647770 ) ) ;
#81739=CARTESIAN_POINT ( 'NONE',  ( -1.572991167713776672, 2.401574803149606474, -0.1227090857360982196 ) ) ;
#81740=CARTESIAN_POINT ( 'NONE',  ( 0.6889763779527566800, -0.4536011799217367080, 0.2665933059059888421 ) ) ;
#81741=CARTESIAN_POINT ( 'NONE',  ( 1.167979002624672580, -0.4281496062992124485, 0.4176697321401328655 ) ) ;
#81742=CARTESIAN_POINT ( 'NONE',  ( -0.08530183727034056085, -0.08942795157528024563, -0.3641732283464568787 ) ) ;
#81743=CARTESIAN_POINT ( 'NONE',  ( -0.3543307086614165824, 0.2952755905511811885, 0.000000000000000000 ) ) ;
#81744=CARTESIAN_POINT ( 'NONE',  ( 0.1771653543307093182, 0.1660481256975885056, 0.3530559997133364547 ) ) ;
#81745=CARTESIAN_POINT ( 'NONE',  ( -0.7414698162729651543, -0.6692913385826771977, 0.1292274648535927661 ) ) ;
#81746=CARTESIAN_POINT ( 'NONE',  ( -0.3674540682414692561, -0.5023911411419708095, -0.1820866141732282451 ) ) ;
#81747=CARTESIAN_POINT ( 'NONE',  ( 0.9580052493438326877, 0.05413385826771666132, 0.4176697321401328100 ) ) ;
#81748=CARTESIAN_POINT ( 'NONE',  ( 0.9251968503937015864, 0.07958543189024071263, -0.2665933059059888421 ) ) ;
#81749=CARTESIAN_POINT ( 'NONE',  ( 0.2559055118110243332, 0.1660481256975885056, 0.3530559997133364547 ) ) ;
#81750=CARTESIAN_POINT ( 'NONE',  ( 1.148293963254593653, 0.2066929133858267098, -0.1054918080437494132 ) ) ;
#81753=CARTESIAN_POINT ( 'NONE',  ( 1.594488188976378673, -0.5400638737290845981, -0.3530559997133363437 ) ) ;
#81756=CARTESIAN_POINT ( 'NONE',  ( -1.299212598425196097, 0.2952755905511811885, 0.000000000000000000 ) ) ;
#81757=CARTESIAN_POINT ( 'NONE',  ( -0.9711286089238838626, -0.6046776061558807314, 0.2411417322834647770 ) ) ;
#81760=ORIENTED_EDGE ( 'NONE', *, *, #6471, .F. ) ;
#81761=CARTESIAN_POINT ( 'NONE',  ( 0.4855643044619430415, -0.3690944881889765550, -0.3153832671262227771 ) ) ;
#81763=CARTESIAN_POINT ( 'NONE',  ( 0.5183727034120741983, 0.2952755905511810774, -0.1292274648535930714 ) ) ;
#81766=CARTESIAN_POINT ( 'NONE',  ( -1.581364829396324945, -0.2845877964562159024, 0.3641732283464567677 ) ) ;
#81767=CARTESIAN_POINT ( 'NONE',  ( 1.312335958005250269, -0.6046776061558807314, 0.2411417322834647770 ) ) ;
#81768=CARTESIAN_POINT ( 'NONE',  ( 1.417322834645670104, -0.1870078740157479769, 0.3641732283464567677 ) ) ;
#81769=CARTESIAN_POINT ( 'NONE',  ( -0.03280839895013062252, 0.2952755905511810774, -0.1292274648535930714 ) ) ;
#81771=CARTESIAN_POINT ( 'NONE',  ( -0.4921259842519677963, 0.1660481256975883668, -0.3530559997133364547 ) ) ;
#81772=CARTESIAN_POINT ( 'NONE',  ( -0.9251968503937002541, 0.07958543189024085140, 0.2665933059059887866 ) ) ;
#81773=CARTESIAN_POINT ( 'NONE',  ( 0.4527559055118117182, -0.5400638737290844871, 0.3530559997133364547 ) ) ;
#81774=CARTESIAN_POINT ( 'NONE',  ( -0.6824146981627291497, -0.6046776061558809534, -0.2411417322834644161 ) ) ;
#81777=ORIENTED_EDGE ( 'NONE', *, *, #43470, .F. ) ;
#81779=CARTESIAN_POINT ( 'NONE',  ( 0.2493438320209980519, 0.05413385826771666132, 0.4176697321401328100 ) ) ;
#81780=CARTESIAN_POINT ( 'NONE',  ( -0.3412073490813641308, -0.6046776061558807314, 0.2411417322834647770 ) ) ;
#81781=CARTESIAN_POINT ( 'NONE',  ( -1.515748031496062076, -0.5400638737290844871, 0.3530559997133364547 ) ) ;
#81782=CARTESIAN_POINT ( 'NONE',  ( 0.7545931758530188826, -0.6692913385826771977, 0.1292274648535927661 ) ) ;
#81783=CARTESIAN_POINT ( 'NONE',  ( 0.4724409448818904789, -0.1870078740157480879, -0.4822834645669291653 ) ) ;
#81785=CARTESIAN_POINT ( 'NONE',  ( -0.7611548556430438595, 0.2306618581243848609, 0.2411417322834645549 ) ) ;
#81786=CARTESIAN_POINT ( 'NONE',  ( 0.2427821522309719648, -0.05778040916215522460, 0.4822834645669289988 ) ) ;
#81787=CARTESIAN_POINT ( 'NONE',  ( -0.3018372703412066094, -0.4281496062992127816, -0.4176697321401328100 ) ) ;
#81788=CARTESIAN_POINT ( 'NONE',  ( 0.1049868766404206816, 0.1283753931104748280, 0.1820866141732283561 ) ) ;
#81789=CARTESIAN_POINT ( 'NONE',  ( 1.653543307086614789, -0.1870078740157479769, 0.3641732283464567677 ) ) ;
#81791=CARTESIAN_POINT ( 'NONE',  ( -0.1049868766404193215, 0.2306618581243847221, -0.2411417322834647770 ) ) ;
#81793=CARTESIAN_POINT ( 'NONE',  ( -1.601049868766403650, 0.2306618581243847221, -0.2411417322834647770 ) ) ;
#81796=VERTEX_POINT ( 'NONE', #67219 ) ;
#81797=CARTESIAN_POINT ( 'NONE',  ( 0.6889763779527566800, -0.5400638737290844871, 0.3530559997133364547 ) ) ;
#81798=CARTESIAN_POINT ( 'NONE',  ( 0.2099737532808405305, 0.1283753931104746893, -0.1820866141732285504 ) ) ;
#81799=CARTESIAN_POINT ( 'NONE',  ( 0.6175017169405826456, 2.784432375088962958E-17, -0.3464511005275205946 ) ) ;
#81804=CARTESIAN_POINT ( 'NONE',  ( 0.3937007874015754361, -0.1870078740157480879, -0.4822834645669291653 ) ) ;
#81805=CARTESIAN_POINT ( 'NONE',  ( -1.397637795275589623, -0.5400638737290845981, -0.3530559997133363437 ) ) ;
#81806=CARTESIAN_POINT ( 'NONE',  ( -1.240157480314959759, 0.1660481256975885056, 0.3530559997133364547 ) ) ;
#81807=CARTESIAN_POINT ( 'NONE',  ( 0.7480314960629927956, -0.6692913385826771977, 8.415575281601705876E-17 ) ) ;
#81808=CARTESIAN_POINT ( 'NONE',  ( 1.318897637795276356, 0.1660481256975883668, -0.3530559997133364547 ) ) ;
#81809=CARTESIAN_POINT ( 'NONE',  ( 1.299212598425197429, -0.5511811023622047445, 6.969142054262312111E-17 ) ) ;
#81811=CARTESIAN_POINT ( 'NONE',  ( 1.062992125984252745, 0.1771653543307087630, 0.000000000000000000 ) ) ;
#81812=CARTESIAN_POINT ( 'NONE',  ( -0.9973753280839886548, 0.2306618581243848609, 0.2411417322834645549 ) ) ;
#81814=CARTESIAN_POINT ( 'NONE',  ( 1.391076115485564868, 0.2306618581243847221, -0.2411417322834647770 ) ) ;
#81817=CARTESIAN_POINT ( 'NONE',  ( -0.3018372703412066094, -0.4281496062992127816, -0.4176697321401328100 ) ) ;
#81818=CARTESIAN_POINT ( 'NONE',  ( 1.292650918635171564, -0.6692913385826773087, -0.1292274648535924053 ) ) ;
#81819=FACE_OUTER_BOUND ( 'NONE', #13937, .T. ) ;
#81820=CARTESIAN_POINT ( 'NONE',  ( -1.187664041994750175, -0.08942795157528024563, -0.3641732283464568787 ) ) ;
#81821=CARTESIAN_POINT ( 'NONE',  ( 0.5643044619422579178, 0.05413385826771666132, 0.4176697321401328100 ) ) ;
#81822=CARTESIAN_POINT ( 'NONE',  ( 0.8792650918635177559, -0.3690944881889765550, -0.3153832671262227771 ) ) ;
#81824=CARTESIAN_POINT ( 'NONE',  ( -1.200787401574802349, 0.07958543189024071263, -0.2665933059059888421 ) ) ;
#81825=CARTESIAN_POINT ( 'NONE',  ( 1.135170603674541256, -0.6692913385826773087, -0.1292274648535924053 ) ) ;
#81827=CARTESIAN_POINT ( 'NONE',  ( -0.5643044619422565855, -0.004921259842519870586, -0.3153832671262229437 ) ) ;
#81828=CARTESIAN_POINT ( 'NONE',  ( -0.6627296587926503335, -0.6692913385826771977, 0.1292274648535927661 ) ) ;
#81829=CARTESIAN_POINT ( 'NONE',  ( -1.522309711286088607, -0.5023911411419708095, 0.1820866141732285504 ) ) ;
#81830=CARTESIAN_POINT ( 'NONE',  ( -0.5446194225721777693, -0.3162353388693409650, -0.4822834645669289433 ) ) ;
#81831=CARTESIAN_POINT ( 'NONE',  ( 1.404199475065617708, 0.05413385826771626580, -0.4176697321401330321 ) ) ;
#81833=CARTESIAN_POINT ( 'NONE',  ( -1.043307086614172041, -0.4536011799217367080, 0.2665933059059888421 ) ) ;
#81834=CARTESIAN_POINT ( 'NONE',  ( -0.7330049731599687091, 2.221336660396680429, 0.5178675056769429519 ) ) ;
#81835=CARTESIAN_POINT ( 'NONE',  ( 1.587926509186352142, 0.05413385826771666132, 0.4176697321401328100 ) ) ;
#81837=CARTESIAN_POINT ( 'NONE',  ( -1.305774278215222184, -0.6692913385826773087, -0.1292274648535924053 ) ) ;
#81838=CARTESIAN_POINT ( 'NONE',  ( -1.502624671916009680, -0.2845877964562159024, 0.3641732283464567677 ) ) ;
#81839=CARTESIAN_POINT ( 'NONE',  ( -0.4461942257217840213, 0.1283753931104748280, 0.1820866141732283561 ) ) ;
#81840=CARTESIAN_POINT ( 'NONE',  ( -0.5380577427821514602, 0.009842519685039467087, 0.3409548833797002021 ) ) ;
#81841=CARTESIAN_POINT ( 'NONE',  ( -0.2887139107611542133, -0.6046776061558809534, -0.2411417322834644161 ) ) ;
#81842=CARTESIAN_POINT ( 'NONE',  ( 0.02624671916010564918, -0.5023911411419708095, -0.1820866141732282451 ) ) ;
#81843=CARTESIAN_POINT ( 'NONE',  ( -0.9580052493438311334, -0.3690944881889763329, 0.3153832671262228327 ) ) ;
#81844=CARTESIAN_POINT ( 'NONE',  ( -1.371391076115484831, 0.2952755905511810774, -0.1292274648535930714 ) ) ;
#81845=CARTESIAN_POINT ( 'NONE',  ( 1.463254593175853824, 0.1771653543307087075, -0.09757992244046823083 ) ) ;
#81846=CARTESIAN_POINT ( 'NONE',  ( 0.9973753280839902091, -0.6046776061558807314, 0.2411417322834647770 ) ) ;
#81848=CARTESIAN_POINT ( 'NONE',  ( 0.2690288713910767848, 0.1771653543307087630, 0.09757992244046791164 ) ) ;
#81849=CARTESIAN_POINT ( 'NONE',  ( 0.3674540682414705883, -0.6046776061558807314, 0.2411417322834647770 ) ) ;
#81850=CARTESIAN_POINT ( 'NONE',  ( 0.9317585301837276734, -0.3690944881889763329, 0.3153832671262228327 ) ) ;
#81852=CARTESIAN_POINT ( 'NONE',  ( -1.082677165354329896, -0.5400638737290845981, -0.3530559997133363437 ) ) ;
#81853=EDGE_CURVE ( 'NONE', #57471, #71398, #75570, .T. ) ;
#81854=CARTESIAN_POINT ( 'NONE',  ( -0.9055118110236215490, -0.6692913385826771977, 8.415575281601705876E-17 ) ) ;
#81855=CARTESIAN_POINT ( 'NONE',  ( -0.1377952755905504645, 0.1660481256975885056, 0.3530559997133364547 ) ) ;
#81857=CARTESIAN_POINT ( 'NONE',  ( 0.5183727034120741983, 0.2952755905511810774, -0.1292274648535930714 ) ) ;
#81858=CARTESIAN_POINT ( 'NONE',  ( -1.719160104986876103, 0.05413385826771666132, 0.4176697321401328100 ) ) ;
#81859=CARTESIAN_POINT ( 'NONE',  ( 0.1902887139107617975, -0.6692913385826773087, -0.1292274648535924053 ) ) ;
#81860=CARTESIAN_POINT ( 'NONE',  ( 0.5708661417322841158, -0.5400638737290845981, -0.3530559997133363437 ) ) ;
#81866=CARTESIAN_POINT ( 'NONE',  ( -0.3871391076115479057, -0.2845877964562161244, -0.3641732283464567121 ) ) ;
#81867=CARTESIAN_POINT ( 'NONE',  ( -0.7217847769028863381, 0.05413385826771626580, -0.4176697321401330321 ) ) ;
#81868=CARTESIAN_POINT ( 'NONE',  ( 0.4461942257217855201, -0.6046776061558807314, 0.2411417322834647770 ) ) ;
#81870=CARTESIAN_POINT ( 'NONE',  ( 0.8070866141732289112, -0.5400638737290845981, -0.3530559997133363437 ) ) ;
#81871=CARTESIAN_POINT ( 'NONE',  ( -1.496062992125983815, -0.1870078740157479769, 0.4822834645669291653 ) ) ;
#81872=CARTESIAN_POINT ( 'NONE',  ( 0.7480314960629927956, -0.6692913385826771977, 8.415575281601705876E-17 ) ) ;
#81875=CARTESIAN_POINT ( 'NONE',  ( 1.496062992125985147, -0.1870078740157479769, 0.4822834645669291653 ) ) ;
#81876=CARTESIAN_POINT ( 'NONE',  ( 0.7545931758530188826, -0.6692913385826771977, 0.1292274648535927661 ) ) ;
#81877=CARTESIAN_POINT ( 'NONE',  ( 0.4527559055118117182, -0.5400638737290844871, 0.3530559997133364547 ) ) ;
#81878=CARTESIAN_POINT ( 'NONE',  ( 1.364829396325459854, -0.5023911411419708095, -0.1820866141732282451 ) ) ;
#81879=CARTESIAN_POINT ( 'NONE',  ( 1.666666666666667185, 0.05413385826771666132, 0.4176697321401328100 ) ) ;
#81880=CARTESIAN_POINT ( 'NONE',  ( -1.587926509186350810, 0.05413385826771626580, -0.4176697321401330321 ) ) ;
#81883=CARTESIAN_POINT ( 'NONE',  ( 0.8989501312335964611, 0.2952755905511811885, 0.1292274648535926551 ) ) ;
#81884=CARTESIAN_POINT ( 'NONE',  ( 1.489501312335958172, -0.2845877964562159024, 0.3641732283464567677 ) ) ;
#81885=CARTESIAN_POINT ( 'NONE',  ( -0.3805774278215216522, -0.4281496062992127816, -0.4176697321401328100 ) ) ;
#81886=CARTESIAN_POINT ( 'NONE',  ( -0.4724409448818890911, -0.1870078740157479769, 0.4822834645669291653 ) ) ;
#81887=CARTESIAN_POINT ( 'NONE',  ( -1.561679790026246017, -0.4281496062992127816, -0.4176697321401328100 ) ) ;
#81891=CARTESIAN_POINT ( 'NONE',  ( 1.502624671916010790, -0.05778040916215522460, 0.4822834645669289988 ) ) ;
#81895=LINE ( 'NONE', #81069, #1917 ) ;
#81896=CARTESIAN_POINT ( 'NONE',  ( 1.574803149606299746, -0.1870078740157479769, 0.3641732283464567677 ) ) ;
#81898=CARTESIAN_POINT ( 'NONE',  ( 0.5622787594981834003, 7.570362723507360306E-16, 0.3954985857520059711 ) ) ;
#81903=CARTESIAN_POINT ( 'NONE',  ( -0.8727034120734901146, -0.2845877964562159024, 0.3641732283464567677 ) ) ;
#81904=CARTESIAN_POINT ( 'NONE',  ( -1.167979002624671470, -0.3690944881889765550, -0.3153832671262227771 ) ) ;
#81905=CARTESIAN_POINT ( 'NONE',  ( 0.05249343832021075018, 0.2306618581243847221, -0.2411417322834647770 ) ) ;
#81906=CARTESIAN_POINT ( 'NONE',  ( -1.318897637795274802, 0.1660481256975885056, 0.3530559997133364547 ) ) ;
#81908=EDGE_LOOP ( 'NONE', ( #63337, #26976, #77735, #44983 ) ) ;
#81909=CARTESIAN_POINT ( 'NONE',  ( 1.463254593175853824, 0.2952755905511810774, -0.1292274648535930714 ) ) ;
#81910=CARTESIAN_POINT ( 'NONE',  ( -1.115134929062664426, 0.004960608223778509643, -0.3437734562760191848 ) ) ;
#81913=LINE ( 'NONE', #49896, #39827 ) ;
#81914=CARTESIAN_POINT ( 'NONE',  ( -0.4790026246719152336, -0.08942795157528024563, -0.3641732283464568787 ) ) ;
#81916=CARTESIAN_POINT ( 'NONE',  ( -1.332020997375327642, -0.05778040916215522460, 0.4822834645669289988 ) ) ;
#81917=CARTESIAN_POINT ( 'NONE',  ( 0.9908136482939640111, -0.6692913385826771977, 0.1292274648535927661 ) ) ;
#81919=LINE ( 'NONE', #24230, #23466 ) ;
#81920=CARTESIAN_POINT ( 'NONE',  ( -1.646051170424378096, 0.4405861044731112508, 0.5309055118110234117 ) ) ;
#81921=CARTESIAN_POINT ( 'NONE',  ( 1.607611548556431069, -0.6692913385826773087, -0.1292274648535924053 ) ) ;
#81922=CARTESIAN_POINT ( 'NONE',  ( -1.371391076115484831, 0.2952755905511810774, -0.1292274648535930714 ) ) ;
#81924=CARTESIAN_POINT ( 'NONE',  ( 0.05905511811023681640, 0.07958543189024071263, -0.2665933059059888421 ) ) ;
#81926=CARTESIAN_POINT ( 'NONE',  ( -0.1509186351706028884, -0.2845877964562161244, -0.3641732283464567121 ) ) ;
#81927=CARTESIAN_POINT ( 'NONE',  ( 0.6233595800524939223, -0.2845877964562159024, 0.3641732283464567677 ) ) ;
#81928=CARTESIAN_POINT ( 'NONE',  ( 0.6167979002624678353, -0.4281496062992124485, 0.4176697321401328655 ) ) ;
#81929=CARTESIAN_POINT ( 'NONE',  ( -0.6430446194225712953, -0.004921259842519870586, -0.3153832671262229437 ) ) ;
#81931=CARTESIAN_POINT ( 'NONE',  ( 1.292650918635171564, 0.2952755905511811885, 0.1292274648535926551 ) ) ;
#81932=CARTESIAN_POINT ( 'NONE',  ( -0.9448818897637790704, -0.1870078740157480879, -0.4822834645669291653 ) ) ;
#81934=CARTESIAN_POINT ( 'NONE',  ( 0.03280839895013198948, 0.2952755905511811885, 0.1292274648535926551 ) ) ;
#81935=CARTESIAN_POINT ( 'NONE',  ( -0.4461942257217840213, -0.6046776061558809534, -0.2411417322834644161 ) ) ;
#81936=CARTESIAN_POINT ( 'NONE',  ( 1.135170603674541256, -0.5511811023622048555, -0.09757992244046775898 ) ) ;
#81937=CARTESIAN_POINT ( 'NONE',  ( -0.04593175853018302557, -0.5511811023622048555, -0.09757992244046775898 ) ) ;
#81938=CARTESIAN_POINT ( 'NONE',  ( -0.2165354330708654795, -0.5400638737290845981, -0.3530559997133363437 ) ) ;
#81939=CARTESIAN_POINT ( 'NONE',  ( -0.9645669291338575535, 0.1660481256975883668, -0.3530559997133364547 ) ) ;
#81940=CARTESIAN_POINT ( 'NONE',  ( -0.7186703366786194591, -2.567464376874931580E-15, -0.4445507791589072832 ) ) ;
#81941=CARTESIAN_POINT ( 'NONE',  ( -0.1771653543307080136, 0.1660481256975883668, -0.3530559997133364547 ) ) ;
#81944=CARTESIAN_POINT ( 'NONE',  ( 1.167979002624672580, 0.05413385826771626580, -0.4176697321401330321 ) ) ;
#81945=CARTESIAN_POINT ( 'NONE',  ( -0.8530183727034112984, -0.3690944881889765550, -0.3153832671262227771 ) ) ;
#81946=CARTESIAN_POINT ( 'NONE',  ( -0.6233595800524928121, -0.05778040916215522460, 0.4822834645669289988 ) ) ;
#81947=CARTESIAN_POINT ( 'NONE',  ( 1.437007874015748810, -0.5400638737290845981, -0.3530559997133363437 ) ) ;
#81948=CARTESIAN_POINT ( 'NONE',  ( 0.9317585301837276734, 0.05413385826771626580, -0.4176697321401330321 ) ) ;
#81950=CARTESIAN_POINT ( 'NONE',  ( -1.108923884514435132, -0.2845877964562159024, 0.3641732283464567677 ) ) ;
#81955=CARTESIAN_POINT ( 'NONE',  ( 0.9711286089238851948, -0.5023911411419708095, -0.1820866141732282451 ) ) ;
#81956=CARTESIAN_POINT ( 'NONE',  ( 0.5314960629921264834, 0.07958543189024071263, -0.2665933059059888421 ) ) ;
#81957=CARTESIAN_POINT ( 'NONE',  ( 0.3149606299212603933, -0.1870078740157479769, 0.4822834645669291653 ) ) ;
#81958=FACE_OUTER_BOUND ( 'NONE', #36518, .T. ) ;
#81960=CARTESIAN_POINT ( 'NONE',  ( 0.7086614173228353852, -0.1870078740157479769, 0.3641732283464567677 ) ) ;
#81961=CARTESIAN_POINT ( 'NONE',  ( -0.1706036745406816491, 0.05413385826771626580, -0.4176697321401330321 ) ) ;
#81962=CARTESIAN_POINT ( 'NONE',  ( -0.7217847769028863381, -0.4281496062992124485, 0.4176697321401328655 ) ) ;
#81963=CARTESIAN_POINT ( 'NONE',  ( 1.443569553805774897, -0.6046776061558809534, -0.2411417322834644161 ) ) ;
#81966=CARTESIAN_POINT ( 'NONE',  ( -0.1246719160104980823, 0.1771653543307087630, 0.09757992244046791164 ) ) ;
#81970=CARTESIAN_POINT ( 'NONE',  ( -0.6955380577427815458, -0.4281496062992127816, -0.4176697321401328100 ) ) ;
#81971=CARTESIAN_POINT ( 'NONE',  ( -0.2952755905511803003, -0.5400638737290845981, -0.3530559997133363437 ) ) ;
#81972=CARTESIAN_POINT ( 'NONE',  ( -0.3412073490813641308, 0.2306618581243847221, -0.2411417322834647770 ) ) ;
#81973=DIMENSIONAL_EXPONENTS ( 1.000000000000000000, 0.000000000000000000, 0.000000000000000000, 0.000000000000000000, 0.000000000000000000, 0.000000000000000000, 0.000000000000000000 ) ;
#81974=CARTESIAN_POINT ( 'NONE',  ( 0.5839895013123367340, 0.2952755905511811885, 0.1292274648535926551 ) ) ;
#81975=CARTESIAN_POINT ( 'NONE',  ( -0.4593175853018364174, -0.4281496062992127816, -0.4176697321401328100 ) ) ;
#81976=CARTESIAN_POINT ( 'NONE',  ( -1.299212598425196097, 0.2952755905511811885, 0.000000000000000000 ) ) ;
#81977=CARTESIAN_POINT ( 'NONE',  ( -0.6627296587926503335, -0.6692913385826771977, 0.1292274648535927661 ) ) ;
#81978=CARTESIAN_POINT ( 'NONE',  ( 0.6233595800524939223, -0.3162353388693405765, 0.4822834645669290543 ) ) ;
#81979=EDGE_CURVE ( 'NONE', #47474, #46955, #53730, .T. ) ;
#81980=ADVANCED_FACE ( 'NONE', ( #73111 ), #41120, .F. ) ;
#81982=CARTESIAN_POINT ( 'NONE',  ( -0.3280839895013117347, -0.004921259842519870586, -0.3153832671262229437 ) ) ;
#81983=EDGE_LOOP ( 'NONE', ( #37018, #36935, #73183, #79599 ) ) ;
#81986=CARTESIAN_POINT ( 'NONE',  ( -1.456692913385826182, -0.5511811023622047445, 6.969142054262312111E-17 ) ) ;
#81987=CARTESIAN_POINT ( 'NONE',  ( -0.9776902887139098386, 0.2952755905511810774, -0.1292274648535930714 ) ) ;
#81988=CARTESIAN_POINT ( 'NONE',  ( -0.9776902887139098386, 0.2952755905511810774, -0.1292274648535930714 ) ) ;
#81990=CARTESIAN_POINT ( 'NONE',  ( -0.6955380577427815458, -0.4281496062992127816, -0.4176697321401328100 ) ) ;
#81991=CARTESIAN_POINT ( 'NONE',  ( -0.8464566929133852113, -0.5400638737290845981, -0.3530559997133363437 ) ) ;
#81992=LINE ( 'NONE', #70161, #55273 ) ;
#81994=CARTESIAN_POINT ( 'NONE',  ( 0.5839895013123367340, 0.1771653543307087630, 0.09757992244046791164 ) ) ;
#81995=CARTESIAN_POINT ( 'NONE',  ( 0.4606732211681152100, 1.541615089183626441, 0.5309055118110234117 ) ) ;
#81997=CARTESIAN_POINT ( 'NONE',  ( 5.463695987328526437E-16, -0.1870078740157479769, 0.3641732283464567677 ) ) ;
#81998=CARTESIAN_POINT ( 'NONE',  ( -0.4396325459317577122, -0.6692913385826773087, -0.1292274648535924053 ) ) ;
#82000=CARTESIAN_POINT ( 'NONE',  ( 0.09842519685039434474, 0.1660481256975885056, 0.3530559997133364547 ) ) ;
#82001=ORIENTED_EDGE ( 'NONE', *, *, #35805, .T. ) ;
#82007=CARTESIAN_POINT ( 'NONE',  ( -1.154855643044618851, -0.5023911411419708095, -0.1820866141732282451 ) ) ;
#82008=CARTESIAN_POINT ( 'NONE',  ( -0.8530183727034112984, -0.4281496062992127816, -0.4176697321401328100 ) ) ;
#82011=EDGE_CURVE ( 'NONE', #62516, #35589, #2825, .T. ) ;
#82013=CARTESIAN_POINT ( 'NONE',  ( 1.371391076115485941, 0.2952755905511811885, 0.1292274648535926551 ) ) ;
#82014=CARTESIAN_POINT ( 'NONE',  ( 0.5249343832021003964, 0.2306618581243847221, -0.2411417322834647770 ) ) ;
#82015=CARTESIAN_POINT ( 'NONE',  ( -0.08530183727034056085, -0.3162353388693405765, 0.4822834645669290543 ) ) ;
#82016=CARTESIAN_POINT ( 'NONE',  ( -1.259842519685038686, -0.1870078740157480601, -0.3641732283464567677 ) ) ;
#82017=CARTESIAN_POINT ( 'NONE',  ( -0.5511811023622041894, -0.1870078740157480879, -0.4822834645669291653 ) ) ;
#82020=CARTESIAN_POINT ( 'NONE',  ( -0.8464566929133852113, -0.5400638737290845981, -0.3530559997133363437 ) ) ;
#82022=CARTESIAN_POINT ( 'NONE',  ( 1.371391076115485719, -0.5511811023622048555, -0.09757992244046775898 ) ) ;
#82023=CARTESIAN_POINT ( 'NONE',  ( -0.4724409448818890911, -0.1870078740157479769, 0.3641732283464567677 ) ) ;
#82024=CARTESIAN_POINT ( 'NONE',  ( 1.332020997375329197, -0.2845877964562159024, 0.3641732283464567677 ) ) ;
#82025=CARTESIAN_POINT ( 'NONE',  ( -1.469816272965878357, -0.6046776061558809534, -0.2411417322834644161 ) ) ;
#82026=CARTESIAN_POINT ( 'NONE',  ( -1.062992125984250968, -0.5511811023622047445, 6.969142054262312111E-17 ) ) ;
#82028=CARTESIAN_POINT ( 'NONE',  ( 0.4002624671916016896, -0.08942795157527998196, 0.3641732283464567121 ) ) ;
#82029=CARTESIAN_POINT ( 'NONE',  ( -0.2821522309711278487, -0.6692913385826773087, -0.1292274648535924053 ) ) ;
#82031=CARTESIAN_POINT ( 'NONE',  ( 0.05249343832021075018, -0.5023911411419708095, 0.1820866141732285504 ) ) ;
#82033=CARTESIAN_POINT ( 'NONE',  ( 0.7545931758530189937, 0.2952755905511810774, -0.1292274648535930714 ) ) ;
#82035=CARTESIAN_POINT ( 'NONE',  ( 1.456692913385827515, 0.1771653543307087630, 0.000000000000000000 ) ) ;
#82036=CARTESIAN_POINT ( 'NONE',  ( -0.7545931758530177724, 0.2952755905511811885, 0.1292274648535926551 ) ) ;
#82037=CARTESIAN_POINT ( 'NONE',  ( -0.1509186351706028884, -0.2845877964562161244, -0.3641732283464567121 ) ) ;
#82039=CARTESIAN_POINT ( 'NONE',  ( 0.2165354330708668673, 0.07958543189024071263, -0.2665933059059888421 ) ) ;
#82040=EDGE_CURVE ( 'NONE', #75665, #73526, #78855, .T. ) ;
#82041=CARTESIAN_POINT ( 'NONE',  ( -1.122047244094487306, -0.5400638737290844871, 0.3530559997133364547 ) ) ;
#82042=CARTESIAN_POINT ( 'NONE',  ( -0.5052493438320203589, 0.2952755905511810774, -0.1292274648535930714 ) ) ;
#82046=CARTESIAN_POINT ( 'NONE',  ( 0.4133858267716541968, -0.4536011799217368745, -0.2665933059059886201 ) ) ;
#82047=CARTESIAN_POINT ( 'NONE',  ( -0.2427821522309703550, -0.3162353388693405765, 0.4822834645669290543 ) ) ;
#82048=CARTESIAN_POINT ( 'NONE',  ( -0.7349081364829387342, -0.6046776061558807314, 0.2411417322834647770 ) ) ;
#82049=CARTESIAN_POINT ( 'NONE',  ( -0.9055118110236215490, -0.5511811023622047445, 6.969142054262312111E-17 ) ) ;
#82051=CARTESIAN_POINT ( 'NONE',  ( 0.1246719160104994284, 0.2952755905511810774, -0.1292274648535930714 ) ) ;
#82052=CARTESIAN_POINT ( 'NONE',  ( -1.148293963254592542, -0.5511811023622048555, -0.09757992244046775898 ) ) ;
#82053=CARTESIAN_POINT ( 'NONE',  ( -1.633858267716534529, 0.1660481256975885056, 0.3530559997133364547 ) ) ;
#82056=CARTESIAN_POINT ( 'NONE',  ( -1.351706036745406347, -0.004921259842519870586, -0.3153832671262229437 ) ) ;
#82057=CARTESIAN_POINT ( 'NONE',  ( -1.194225721784776262, 0.05413385826771626580, -0.4176697321401330321 ) ) ;
#82058=CARTESIAN_POINT ( 'NONE',  ( -0.7020997375328076329, -0.3162353388693409650, -0.4822834645669289433 ) ) ;
#82060=CARTESIAN_POINT ( 'NONE',  ( -1.482939632545930975, 0.05413385826771666132, 0.4176697321401328100 ) ) ;
#82063=CARTESIAN_POINT ( 'NONE',  ( 0.9645669291338591078, -0.5400638737290845981, -0.3530559997133363437 ) ) ;
#82064=CARTESIAN_POINT ( 'NONE',  ( 0.3346456692913393205, -0.5400638737290845981, -0.3530559997133363437 ) ) ;
#82065=CARTESIAN_POINT ( 'NONE',  ( -1.614173228346456712, 1.267785121476993737, -0.1372047244094478091 ) ) ;
#82067=CARTESIAN_POINT ( 'NONE',  ( 1.332020997375328974, -0.08942795157528024563, -0.3641732283464568787 ) ) ;
#82070=CARTESIAN_POINT ( 'NONE',  ( -1.023622047244093558, -0.1870078740157479769, 0.3641732283464567677 ) ) ;
#82072=ORIENTED_EDGE ( 'NONE', *, *, #2754, .F. ) ;
#82073=CARTESIAN_POINT ( 'NONE',  ( 0.4921259842519691285, 0.1660481256975885056, 0.3530559997133364547 ) ) ;
#82074=CARTESIAN_POINT ( 'NONE',  ( -0.6233595800524928121, -0.05778040916215522460, 0.4822834645669289988 ) ) ;
#82075=CARTESIAN_POINT ( 'NONE',  ( -0.9317585301837263412, -0.4281496062992127816, -0.4176697321401328100 ) ) ;
#82076=CARTESIAN_POINT ( 'NONE',  ( 1.049868766404200349, 0.2306618581243848609, 0.2411417322834645549 ) ) ;
#82077=CARTESIAN_POINT ( 'NONE',  ( -1.528871391076114250, -0.5511811023622046335, 0.09757992244046803654 ) ) ;
#82079=CARTESIAN_POINT ( 'NONE',  ( 0.1115485564304470323, 0.2952755905511811885, 0.1292274648535926551 ) ) ;
#82080=CARTESIAN_POINT ( 'NONE',  ( -1.194225721784776262, -0.4281496062992124485, 0.4176697321401328655 ) ) ;
#82081=CARTESIAN_POINT ( 'NONE',  ( 1.620734908136483465, -0.6692913385826771977, 0.1292274648535927661 ) ) ;
#82084=CARTESIAN_POINT ( 'NONE',  ( 1.010498687664042716, -0.3690944881889763329, 0.3153832671262228327 ) ) ;
#82087=ORIENTED_EDGE ( 'NONE', *, *, #79479, .F. ) ;
#82088=CARTESIAN_POINT ( 'NONE',  ( -0.1246719160104980823, 0.1771653543307087630, 0.09757992244046791164 ) ) ;
#82089=CARTESIAN_POINT ( 'NONE',  ( -1.423884514435694859, -0.3162353388693405765, 0.4822834645669290543 ) ) ;
#82090=CARTESIAN_POINT ( 'NONE',  ( 0.3805774278215230400, 0.05413385826771626580, -0.4176697321401330321 ) ) ;
#82091=CARTESIAN_POINT ( 'NONE',  ( 0.2952755905511816326, -0.5400638737290844871, 0.3530559997133364547 ) ) ;
#82092=CARTESIAN_POINT ( 'NONE',  ( -0.6233595800524928121, -0.05778040916215522460, 0.4822834645669289988 ) ) ;
#82094=CARTESIAN_POINT ( 'NONE',  ( -1.043307086614172041, -0.5400638737290844871, 0.3530559997133364547 ) ) ;
#82096=CARTESIAN_POINT ( 'NONE',  ( 1.318897637795276356, 0.07958543189024071263, -0.2665933059059888421 ) ) ;
#82097=CARTESIAN_POINT ( 'NONE',  ( -0.9842519685039360366, 0.2952755905511811885, 0.000000000000000000 ) ) ;
#82098=CARTESIAN_POINT ( 'NONE',  ( 0.8595800524934390507, -0.3162353388693405765, 0.4822834645669290543 ) ) ;
#82099=CARTESIAN_POINT ( 'NONE',  ( 1.003937007874016407, -0.5400638737290844871, 0.3530559997133364547 ) ) ;
#82102=CARTESIAN_POINT ( 'NONE',  ( -1.496062992125983815, -0.1870078740157480879, -0.4822834645669291653 ) ) ;
#82104=CARTESIAN_POINT ( 'NONE',  ( 0.3937007874015754361, -0.1870078740157480879, -0.4822834645669291653 ) ) ;
#82107=CARTESIAN_POINT ( 'NONE',  ( -1.541994750656167090, -0.5511811023622048555, -0.09757992244046775898 ) ) ;
#82108=CARTESIAN_POINT ( 'NONE',  ( 0.3805774278215230400, -0.3690944881889763329, 0.3153832671262228327 ) ) ;
#82109=CARTESIAN_POINT ( 'NONE',  ( 1.082677165354331228, -0.5400638737290844871, 0.3530559997133364547 ) ) ;
#82111=CARTESIAN_POINT ( 'NONE',  ( 0.8727034120734913358, -0.08942795157527998196, 0.3641732283464567121 ) ) ;
#82112=CARTESIAN_POINT ( 'NONE',  ( 0.5839895013123367340, -0.6692913385826773087, -0.1292274648535924053 ) ) ;
#82114=CARTESIAN_POINT ( 'NONE',  ( -0.8923884514435688198, 0.2306618581243847221, -0.2411417322834647770 ) ) ;
#82115=CARTESIAN_POINT ( 'NONE',  ( -0.1771653543307080136, 0.1660481256975883391, -0.3530559997133364547 ) ) ;
#82116=CARTESIAN_POINT ( 'NONE',  ( 1.128608923884514947, 0.1283753931104748280, 0.1820866141732283561 ) ) ;
#82118=CARTESIAN_POINT ( 'NONE',  ( 0.1049868766404206677, 0.1539470093639523085, 0.1968503937007873850 ) ) ;
#82119=CARTESIAN_POINT ( 'NONE',  ( -0.3280839895013117347, -0.4281496062992124485, 0.4176697321401328655 ) ) ;
#82120=CARTESIAN_POINT ( 'NONE',  ( 0.2230971128608932319, -0.3690944881889763329, 0.3153832671262228327 ) ) ;
#82121=CARTESIAN_POINT ( 'NONE',  ( 0.06632061457837788720, 2.409604939980833412E-17, -0.3464511005275205946 ) ) ;
#82122=CARTESIAN_POINT ( 'NONE',  ( -0.4330708661417315697, 0.2952755905511811885, 0.000000000000000000 ) ) ;
#82123=CARTESIAN_POINT ( 'NONE',  ( 0.7742782152230978099, -0.3690944881889763329, 0.3153832671262228327 ) ) ;
#82126=CARTESIAN_POINT ( 'NONE',  ( 0.2034120734908144990, -0.6692913385826771977, 0.1292274648535927661 ) ) ;
#82127=CARTESIAN_POINT ( 'NONE',  ( 1.108923884514436686, -0.2845877964562161244, -0.3641732283464567121 ) ) ;
#82128=CARTESIAN_POINT ( 'NONE',  ( 0.2034120734908141659, 0.2952755905511810219, -0.1292274648535930437 ) ) ;
#82129=CARTESIAN_POINT ( 'NONE',  ( -0.2493438320209966919, -0.004921259842519870586, -0.3153832671262229437 ) ) ;
#82130=EDGE_CURVE ( 'NONE', #11499, #30580, #59417, .T. ) ;
#82131=CARTESIAN_POINT ( 'NONE',  ( -0.5971128608923877978, 0.1771653543307087630, 0.09757992244046791164 ) ) ;
#82132=CARTESIAN_POINT ( 'NONE',  ( -0.1968503937007867743, 0.2952755905511811885, 0.000000000000000000 ) ) ;
#82133=CARTESIAN_POINT ( 'NONE',  ( 0.2559055118110243332, -0.5400638737290845981, -0.3530559997133363437 ) ) ;
#82134=CARTESIAN_POINT ( 'NONE',  ( 1.003937007874016407, -0.4536011799217367080, 0.2665933059059888421 ) ) ;
#82135=CARTESIAN_POINT ( 'NONE',  ( -1.601049868766403650, -0.5023911411419708095, 0.1820866141732285504 ) ) ;
#82136=CARTESIAN_POINT ( 'NONE',  ( 1.502624671916010790, -0.2845877964562161244, -0.3641732283464567121 ) ) ;
#82138=CARTESIAN_POINT ( 'NONE',  ( 0.9186351706036752773, 0.2306618581243847221, -0.2411417322834647770 ) ) ;
#82140=CARTESIAN_POINT ( 'NONE',  ( -0.01312335958005186876, -0.4281496062992124485, 0.4176697321401328655 ) ) ;
#82142=CARTESIAN_POINT ( 'NONE',  ( 0.9973753280839902091, -0.6046776061558807314, 0.2411417322834647770 ) ) ;
#82143=CARTESIAN_POINT ( 'NONE',  ( 0.7545931758530189937, 0.2952755905511810774, -0.1292274648535930714 ) ) ;
#82145=CARTESIAN_POINT ( 'NONE',  ( 0.4658792650918641698, -0.08942795157528024563, -0.3641732283464568787 ) ) ;
#82146=CARTESIAN_POINT ( 'NONE',  ( 1.030183727034121421, -0.05778040916215522460, 0.4822834645669289988 ) ) ;
#82147=CARTESIAN_POINT ( 'NONE',  ( 0.07874015748031558404, -0.1870078740157480601, -0.3641732283464567677 ) ) ;
#82148=CARTESIAN_POINT ( 'NONE',  ( -0.1049868766404193215, -0.6046776061558807314, 0.2411417322834647770 ) ) ;
#82150=CARTESIAN_POINT ( 'NONE',  ( 0.3280839895013130669, 0.05413385826771666132, 0.4176697321401328100 ) ) ;
#82151=CARTESIAN_POINT ( 'NONE',  ( -0.8595800524934373854, -0.05778040916215522460, 0.4822834645669289988 ) ) ;
#82152=CARTESIAN_POINT ( 'NONE',  ( -0.1246719160104980823, 0.1771653543307087630, 0.09757992244046791164 ) ) ;
#82153=CIRCLE ( 'NONE', #79467, 0.4822834645669291653 ) ;
#82154=CARTESIAN_POINT ( 'NONE',  ( 0.4133858267716541968, -0.5400638737290845981, -0.3530559997133363437 ) ) ;
#82155=CARTESIAN_POINT ( 'NONE',  ( 1.128608923884515169, -0.5023911411419708095, -0.1820866141732282451 ) ) ;
#82156=CARTESIAN_POINT ( 'NONE',  ( -0.4002624671916004129, -0.3162353388693405765, 0.4822834645669290543 ) ) ;
#82159=DIRECTION ( 'NONE',  ( -0.7071067811865429098, 0.7071067811865521247, 0.000000000000000000 ) ) ;
#82160=CARTESIAN_POINT ( 'NONE',  ( 1.601049868766404982, -0.6046776061558809534, -0.2411417322834644161 ) ) ;
#82162=CARTESIAN_POINT ( 'NONE',  ( -1.266404199475064773, -0.05778040916215560624, -0.4822834645669293319 ) ) ;
#82163=CARTESIAN_POINT ( 'NONE',  ( -0.7086614173228339419, -0.1870078740157480879, -0.4822834645669291653 ) ) ;
#82167=CARTESIAN_POINT ( 'NONE',  ( 0.1312335958005257930, 0.1283753931104746893, -0.1820866141732285504 ) ) ;
#82169=CARTESIAN_POINT ( 'NONE',  ( 0.5839895013123367340, -0.6692913385826773087, -0.1292274648535924053 ) ) ;
#82171=CARTESIAN_POINT ( 'NONE',  ( -0.5611900217179893735, -2.567464376874931580E-15, -0.4445507791589072832 ) ) ;
#82172=CARTESIAN_POINT ( 'NONE',  ( -1.587926509186350810, -0.3690944881889763329, 0.3153832671262228327 ) ) ;
#82174=CARTESIAN_POINT ( 'NONE',  ( 1.043307086614173818, 0.1660481256975885056, 0.3530559997133364547 ) ) ;
#82175=CARTESIAN_POINT ( 'NONE',  ( 1.437007874015748810, 0.07958543189024085140, 0.2665933059059887866 ) ) ;
#82176=CARTESIAN_POINT ( 'NONE',  ( 0.1312335958005257930, 0.2306618581243847221, -0.2411417322834647770 ) ) ;
#82178=CARTESIAN_POINT ( 'NONE',  ( -0.2624671916010490880, -0.6046776061558807314, 0.2411417322834647770 ) ) ;
#82179=CARTESIAN_POINT ( 'NONE',  ( -1.259842519685038686, -0.1870078740157479769, 0.3641732283464567677 ) ) ;
#82180=CARTESIAN_POINT ( 'NONE',  ( -0.6167979002624665030, 0.05413385826771666132, 0.4176697321401328100 ) ) ;
#82181=DIRECTION ( 'NONE',  ( -1.000000000000000000, -3.469446951953613696E-16, 0.000000000000000000 ) ) ;
#82183=VERTEX_POINT ( 'NONE', #18349 ) ;
#82185=CARTESIAN_POINT ( 'NONE',  ( 0.5839895013123367340, 0.2952755905511811885, 0.1292274648535926551 ) ) ;
#82187=CARTESIAN_POINT ( 'NONE',  ( -0.4986876640419942164, -0.6046776061558807314, 0.2411417322834647770 ) ) ;
#82188=CARTESIAN_POINT ( 'NONE',  ( -1.377952755905511140, -0.6692913385826771977, 8.415575281601705876E-17 ) ) ;
#82189=CARTESIAN_POINT ( 'NONE',  ( 0.5905511811023629321, -0.6692913385826771977, 8.415575281601705876E-17 ) ) ;
#82190=CARTESIAN_POINT ( 'NONE',  ( -0.08530183727034056085, -0.3162353388693405765, 0.4822834645669290543 ) ) ;
#82192=CARTESIAN_POINT ( 'NONE',  ( -0.6233595800524928121, -0.05778040916215522460, 0.4822834645669289988 ) ) ;
#82193=CARTESIAN_POINT ( 'NONE',  ( 0.4330708661417329575, 0.2952755905511811885, 0.000000000000000000 ) ) ;
#82194=CARTESIAN_POINT ( 'NONE',  ( -0.5905511811023613777, -0.6692913385826771977, 8.415575281601705876E-17 ) ) ;
#82195=CARTESIAN_POINT ( 'NONE',  ( 0.2427821522309719648, -0.08942795157527998196, 0.3641732283464567121 ) ) ;
#82197=CARTESIAN_POINT ( 'NONE',  ( -0.07217847769028813698, -0.3162353388693409650, -0.4822834645669289433 ) ) ;
#82199=CARTESIAN_POINT ( 'NONE',  ( -1.555118110236219930, -0.5400638737290845981, -0.3530559997133363437 ) ) ;
#82201=ORIENTED_EDGE ( 'NONE', *, *, #40849, .F. ) ;
#82203=CARTESIAN_POINT ( 'NONE',  ( 0.7086614173228353852, -0.1870078740157479769, 0.4822834645669291653 ) ) ;
#82204=CARTESIAN_POINT ( 'NONE',  ( 0.2165354330708668673, 0.07958543189024071263, -0.2665933059059888421 ) ) ;
#82211=CARTESIAN_POINT ( 'NONE',  ( 0.4921259842519691285, 0.1660481256975885056, 0.3530559997133364547 ) ) ;
#82212=CARTESIAN_POINT ( 'NONE',  ( -1.181102362204723644, -0.1870078740157479769, 0.4822834645669291653 ) ) ;
#82213=CARTESIAN_POINT ( 'NONE',  ( -1.023622047244094002, -0.1870078740157480879, -0.4822834645669291653 ) ) ;
#82214=CARTESIAN_POINT ( 'NONE',  ( 0.3346456692913390985, 0.1660481256975885056, 0.3530559997133364547 ) ) ;
#82216=CARTESIAN_POINT ( 'NONE',  ( 0.9448818897637802916, -0.1870078740157479769, 0.4822834645669291653 ) ) ;
#82217=CARTESIAN_POINT ( 'NONE',  ( 1.174540682414699111, -0.2845877964562159024, 0.3641732283464567677 ) ) ;
#82218=CARTESIAN_POINT ( 'NONE',  ( 1.377952755905512472, 0.1771653543307087630, 0.000000000000000000 ) ) ;
#82219=CARTESIAN_POINT ( 'NONE',  ( -0.6824146981627288167, 0.2306618581243848609, 0.2411417322834645549 ) ) ;
#82221=CARTESIAN_POINT ( 'NONE',  ( 1.673228346456693494, 0.1660481256975885056, 0.3530559997133364547 ) ) ;
#82223=CARTESIAN_POINT ( 'NONE',  ( -0.1312335958005241554, -0.6046776061558809534, -0.2411417322834644161 ) ) ;
#82224=CARTESIAN_POINT ( 'NONE',  ( 1.167979002624672580, -0.4281496062992124485, 0.4176697321401328655 ) ) ;
#82226=CARTESIAN_POINT ( 'NONE',  ( -1.509186351706035767, -0.004921259842519870586, -0.3153832671262229437 ) ) ;
#82227=CARTESIAN_POINT ( 'NONE',  ( -0.07874015748031421014, -0.1870078740157479769, 0.4822834645669291653 ) ) ;
#82228=CARTESIAN_POINT ( 'NONE',  ( 0.7545931758530188826, -0.5511811023622046335, 0.09757992244046803654 ) ) ;
#82230=CARTESIAN_POINT ( 'NONE',  ( -1.450131233595799651, -0.5511811023622046335, 0.09757992244046803654 ) ) ;
#82231=CARTESIAN_POINT ( 'NONE',  ( 1.062992125984252745, 0.2952755905511811885, 0.000000000000000000 ) ) ;
#82232=CARTESIAN_POINT ( 'NONE',  ( -0.7426113562971994320, 1.972848275015058439, 0.5309055118110236338 ) ) ;
#82233=CARTESIAN_POINT ( 'NONE',  ( -0.4133858267716528645, 0.07958543189024071263, -0.2665933059059888421 ) ) ;
#82234=CARTESIAN_POINT ( 'NONE',  ( -0.5052493438320203589, -0.6692913385826771977, 0.1292274648535927661 ) ) ;
#82235=CARTESIAN_POINT ( 'NONE',  ( 1.443569553805774897, -0.6046776061558809534, -0.2411417322834644161 ) ) ;
#82236=CARTESIAN_POINT ( 'NONE',  ( -1.069553805774277722, 0.2952755905511811885, 0.1292274648535926551 ) ) ;
#82237=CARTESIAN_POINT ( 'NONE',  ( 1.299212598425197429, -0.6692913385826771977, 8.415575281601705876E-17 ) ) ;
#82239=CARTESIAN_POINT ( 'NONE',  ( -1.207349081364828436, -0.5023911411419708095, 0.1820866141732285504 ) ) ;
#82241=CARTESIAN_POINT ( 'NONE',  ( 1.450131233595801428, 0.2952755905511811885, 0.1292274648535926551 ) ) ;
#82243=CARTESIAN_POINT ( 'NONE',  ( -1.640419947506561060, -0.4281496062992127816, -0.4176697321401328100 ) ) ;
#82244=CARTESIAN_POINT ( 'NONE',  ( -1.364829396325458521, -0.5023911411419708095, 0.1820866141732285504 ) ) ;
#82245=CARTESIAN_POINT ( 'NONE',  ( -1.030183727034119867, -0.08942795157528024563, -0.3641732283464568787 ) ) ;
#82246=CARTESIAN_POINT ( 'NONE',  ( 1.555118110236221041, 0.07958543189024071263, -0.2665933059059888421 ) ) ;
#82247=CARTESIAN_POINT ( 'NONE',  ( -0.3412073490813641308, 0.2306618581243847221, -0.2411417322834647770 ) ) ;
#82248=CARTESIAN_POINT ( 'NONE',  ( -0.02624671916010428221, 0.1283753931104746893, -0.1820866141732285504 ) ) ;
#82249=CARTESIAN_POINT ( 'NONE',  ( -0.9908136482939626788, -0.5511811023622048555, -0.09757992244046775898 ) ) ;
#82250=CARTESIAN_POINT ( 'NONE',  ( 1.430446194225722500, -0.004921259842519576551, 0.3153832671262227771 ) ) ;
#82251=CARTESIAN_POINT ( 'NONE',  ( 0.9055118110236227702, 0.2952755905511811885, 0.000000000000000000 ) ) ;
#82252=CARTESIAN_POINT ( 'NONE',  ( 1.509186351706037543, -0.4281496062992127816, -0.4176697321401328100 ) ) ;
#82253=CARTESIAN_POINT ( 'NONE',  ( 0.2887139107611556010, 0.1283753931104746893, -0.1820866141732285504 ) ) ;
#82254=CARTESIAN_POINT ( 'NONE',  ( 0.4265091863517067594, 0.2952755905511811885, 0.1292274648535926551 ) ) ;
#82255=CARTESIAN_POINT ( 'NONE',  ( 1.194225721784777594, -0.3690944881889765550, -0.3153832671262227771 ) ) ;
#82256=EDGE_LOOP ( 'NONE', ( #28514, #42079, #70257, #75591 ) ) ;
#82257=CARTESIAN_POINT ( 'NONE',  ( -1.450131233595799651, 0.2952755905511810774, -0.1292274648535930714 ) ) ;
#82258=B_SPLINE_CURVE_WITH_KNOTS ( 'NONE', 3,
 ( #69805, #30678, #69398, #81633 ),
 .UNSPECIFIED., .F., .F.,
 ( 4, 4 ),
 ( 0.000000000000000000, 0.001434885020664813287 ),
 .UNSPECIFIED. ) ;
#82259=CARTESIAN_POINT ( 'NONE',  ( -1.469816272965878357, 0.2306618581243848609, 0.2411417322834645549 ) ) ;
#82260=CARTESIAN_POINT ( 'NONE',  ( -0.2165354330708654795, -0.5400638737290845981, -0.3530559997133363437 ) ) ;
#82261=CARTESIAN_POINT ( 'NONE',  ( 0.5408419829024507797, -1.283732188437465593E-15, -0.4281993546915538462 ) ) ;
#82263=CARTESIAN_POINT ( 'NONE',  ( 0.4199475065616803948, -0.6046776061558809534, -0.2411417322834644161 ) ) ;
#82264=CARTESIAN_POINT ( 'NONE',  ( 1.141732283464567566, 0.1771653543307087630, 0.000000000000000000 ) ) ;
#82265=CARTESIAN_POINT ( 'NONE',  ( 0.1246719160104994284, 0.2952755905511810774, -0.1292274648535930714 ) ) ;
#82266=CARTESIAN_POINT ( 'NONE',  ( 0.5183727034120741983, 0.2952755905511810774, -0.1292274648535930714 ) ) ;
#82272=CARTESIAN_POINT ( 'NONE',  ( -0.7020997375328076329, -0.2845877964562161244, -0.3641732283464567121 ) ) ;
#82273=CARTESIAN_POINT ( 'NONE',  ( -0.8727034120734901146, -0.05778040916215560624, -0.4822834645669293319 ) ) ;
#82274=CARTESIAN_POINT ( 'NONE',  ( 0.3608923884514443348, 0.2952755905511810774, -0.1292274648535930714 ) ) ;
#82276=CARTESIAN_POINT ( 'NONE',  ( 0.8136482939632553313, -0.6046776061558809534, -0.2411417322834644161 ) ) ;
#82277=CARTESIAN_POINT ( 'NONE',  ( -1.548556430446193399, -0.6046776061558809534, -0.2411417322834644161 ) ) ;
#82278=CARTESIAN_POINT ( 'NONE',  ( 0.8661417322834652488, -0.1870078740157480879, -0.4822834645669291653 ) ) ;
#82282=CARTESIAN_POINT ( 'NONE',  ( 0.8792650918635177559, -0.4281496062992127816, -0.4176697321401328100 ) ) ;
#82283=CARTESIAN_POINT ( 'NONE',  ( 0.6692913385826777528, 0.2952755905511811885, 0.000000000000000000 ) ) ;
#82284=CARTESIAN_POINT ( 'NONE',  ( 1.384514435695538337, -0.5511811023622046335, 0.09757992244046803654 ) ) ;
#82285=CARTESIAN_POINT ( 'NONE',  ( 1.555118110236221041, 0.1660481256975883668, -0.3530559997133364547 ) ) ;
#82288=CARTESIAN_POINT ( 'NONE',  ( 0.6430446194225729606, -0.4281496062992127816, -0.4176697321401328100 ) ) ;
#82289=CARTESIAN_POINT ( 'NONE',  ( 1.417322834645670104, -0.1870078740157480601, -0.3641732283464567677 ) ) ;
#82290=CARTESIAN_POINT ( 'NONE',  ( -0.4986876640419942164, -0.6046776061558807314, 0.2411417322834647770 ) ) ;
#82291=CARTESIAN_POINT ( 'NONE',  ( -0.9383202099737524282, -0.05778040916215522460, 0.4822834645669289988 ) ) ;
#82292=CARTESIAN_POINT ( 'NONE',  ( 0.9908136482939640111, 0.2952755905511810774, -0.1292274648535930714 ) ) ;
#82296=CARTESIAN_POINT ( 'NONE',  ( -1.587926509186350810, -0.004921259842519870586, -0.3153832671262229437 ) ) ;
#82299=ORIENTED_EDGE ( 'NONE', *, *, #80402, .T. ) ;
#82301=CARTESIAN_POINT ( 'NONE',  ( 1.555118110236221041, -0.4536011799217367080, 0.2665933059059888421 ) ) ;
#82303=CARTESIAN_POINT ( 'NONE',  ( 1.463254593175853824, -0.5511811023622046335, 0.09757992244046803654 ) ) ;
#82308=CARTESIAN_POINT ( 'NONE',  ( -0.7217847769028863381, -0.3690944881889763329, 0.3153832671262228327 ) ) ;
#82309=CARTESIAN_POINT ( 'NONE',  ( -1.351706036745406347, -0.004921259842519870586, -0.3153832671262229437 ) ) ;
#82310=CARTESIAN_POINT ( 'NONE',  ( -1.351706036745406347, -0.4281496062992124485, 0.4176697321401328655 ) ) ;
#82311=CARTESIAN_POINT ( 'NONE',  ( 0.2427821522309716595, -0.3162353388693409650, -0.4822834645669289433 ) ) ;
#82312=CARTESIAN_POINT ( 'NONE',  ( 1.548556430446194954, -0.6046776061558807314, 0.2411417322834647770 ) ) ;
#82314=CARTESIAN_POINT ( 'NONE',  ( 1.325459317585302665, 0.05413385826771626580, -0.4176697321401330321 ) ) ;
#82318=CARTESIAN_POINT ( 'NONE',  ( -0.3937007874015740483, -0.1870078740157479769, 0.3641732283464567677 ) ) ;
#82319=ADVANCED_FACE ( 'NONE', ( #68859 ), #44390, .F. ) ;
#82320=CARTESIAN_POINT ( 'NONE',  ( -1.292650918635170010, 0.2952755905511810774, -0.1292274648535930714 ) ) ;
#82321=CARTESIAN_POINT ( 'NONE',  ( 1.200787401574803681, 0.1660481256975885056, 0.3530559997133364547 ) ) ;
#82322=VERTEX_POINT ( 'NONE', #57031 ) ;
#82325=CARTESIAN_POINT ( 'NONE',  ( -1.666666666666665853, 0.05413385826771626580, -0.4176697321401330321 ) ) ;
#82326=CARTESIAN_POINT ( 'NONE',  ( -1.213910761154854745, 0.2952755905511810774, -0.1292274648535930714 ) ) ;
#82329=CARTESIAN_POINT ( 'NONE',  ( -0.1902887139107604098, -0.5511811023622046335, 0.09757992244046803654 ) ) ;
#82331=CARTESIAN_POINT ( 'NONE',  ( -0.5249343832020990641, 0.1283753931104748280, 0.1820866141732283561 ) ) ;
#82332=CARTESIAN_POINT ( 'NONE',  ( 0.5118110236220478892, 0.1771653543307087630, 0.000000000000000000 ) ) ;
#82333=CARTESIAN_POINT ( 'NONE',  ( 0.7414698162729663755, -0.6692913385826773087, -0.1292274648535924053 ) ) ;
#82334=CARTESIAN_POINT ( 'NONE',  ( -0.5314960629921250401, 0.07958543189024085140, 0.2665933059059887866 ) ) ;
#82336=CARTESIAN_POINT ( 'NONE',  ( 0.9842519685039375910, 0.2952755905511811885, 0.000000000000000000 ) ) ;
#82337=CARTESIAN_POINT ( 'NONE',  ( -0.9842519685039360366, 0.2952755905511811885, 0.000000000000000000 ) ) ;
#82339=CARTESIAN_POINT ( 'NONE',  ( -0.5446194225721777693, -0.3162353388693409650, -0.4822834645669289433 ) ) ;
#82340=CARTESIAN_POINT ( 'NONE',  ( -0.3740157480314953431, 0.1660481256975885056, 0.3530559997133364547 ) ) ;
#82341=CARTESIAN_POINT ( 'NONE',  ( 1.351706036745407680, -0.004921259842519576551, 0.3153832671262227771 ) ) ;
#82342=CARTESIAN_POINT ( 'NONE',  ( -0.09186351706036689768, -0.004921259842519870586, -0.3153832671262229437 ) ) ;
#82343=CARTESIAN_POINT ( 'NONE',  ( -0.1574803149606292529, -0.1870078740157479769, 0.4822834645669291653 ) ) ;
#82344=CARTESIAN_POINT ( 'NONE',  ( -1.108923884514435132, -0.05778040916215560624, -0.4822834645669293319 ) ) ;
#82347=CARTESIAN_POINT ( 'NONE',  ( -0.3083989501312330295, -0.3162353388693409650, -0.4822834645669289433 ) ) ;
#82348=CARTESIAN_POINT ( 'NONE',  ( -1.148293963254592542, -0.6692913385826773087, -0.1292274648535924053 ) ) ;
#82349=EDGE_LOOP ( 'NONE', ( #41822, #33514, #45405, #27205 ) ) ;
#82352=CARTESIAN_POINT ( 'NONE',  ( 1.108923884514436242, -0.05778040916215522460, 0.4822834645669289988 ) ) ;
#82353=CARTESIAN_POINT ( 'NONE',  ( -0.4986876640419942164, -0.5023911411419708095, 0.1820866141732285504 ) ) ;
#82354=CARTESIAN_POINT ( 'NONE',  ( -0.5380577427821514602, -0.4281496062992127816, -0.4176697321401328100 ) ) ;
#82355=CARTESIAN_POINT ( 'NONE',  ( 1.135170603674541256, -0.6692913385826773087, -0.1292274648535924053 ) ) ;
#82356=CARTESIAN_POINT ( 'NONE',  ( 1.108923884514436686, -0.3162353388693409650, -0.4822834645669289433 ) ) ;
#82358=CARTESIAN_POINT ( 'NONE',  ( -0.9776902887139098386, -0.5511811023622046335, 0.09757992244046803654 ) ) ;
#82363=CARTESIAN_POINT ( 'NONE',  ( 1.030183727034121421, -0.08942795157527998196, 0.3641732283464567121 ) ) ;
#82364=CARTESIAN_POINT ( 'NONE',  ( 0.8595800524934390507, -0.08942795157528024563, -0.3641732283464568787 ) ) ;
#82365=CARTESIAN_POINT ( 'NONE',  ( 0.4527559055118117182, -0.5400638737290844871, 0.3530559997133364547 ) ) ;
#82366=CARTESIAN_POINT ( 'NONE',  ( 1.568241469816273437, -0.3162353388693405765, 0.4822834645669290543 ) ) ;
#82368=CARTESIAN_POINT ( 'NONE',  ( 0.6299212598425204535, -0.1870078740157480601, -0.3641732283464567677 ) ) ;
#82369=CARTESIAN_POINT ( 'NONE',  ( -0.3543307086614165824, 0.2952755905511811885, 0.000000000000000000 ) ) ;
#82370=CARTESIAN_POINT ( 'NONE',  ( -1.325459317585300889, 0.05413385826771666132, 0.4176697321401328100 ) ) ;
#82371=CARTESIAN_POINT ( 'NONE',  ( 1.056430446194226658, 0.2952755905511811885, 0.1292274648535926551 ) ) ;
#82373=CARTESIAN_POINT ( 'NONE',  ( -0.7349081364829390672, 0.2306618581243847221, -0.2411417322834647770 ) ) ;
#82374=CARTESIAN_POINT ( 'NONE',  ( -0.01968503937007793844, -0.4536011799217367080, 0.2665933059059888421 ) ) ;
#82376=ORIENTED_EDGE ( 'NONE', *, *, #42359, .F. ) ;
#82377=AXIS2_PLACEMENT_3D ( 'NONE', #28476, #22992, #29718 ) ;
#82378=CARTESIAN_POINT ( 'NONE',  ( -0.6496062992125976043, -0.5400638737290844871, 0.3530559997133364547 ) ) ;
#82379=ADVANCED_FACE ( 'NONE', ( #36453 ), #49494, .F. ) ;
#82380=CARTESIAN_POINT ( 'NONE',  ( -0.4658792650918627265, -0.3162353388693409650, -0.4822834645669289433 ) ) ;
#82381=CARTESIAN_POINT ( 'NONE',  ( -0.1377952755905504645, -0.5400638737290845981, -0.3530559997133363437 ) ) ;
#82382=CARTESIAN_POINT ( 'NONE',  ( 0.2821522309711292364, 0.2952755905511810774, -0.1292274648535930714 ) ) ;
#82383=CARTESIAN_POINT ( 'NONE',  ( -0.3412073490813641308, 0.2306618581243847221, -0.2411417322834647770 ) ) ;
#82384=CARTESIAN_POINT ( 'NONE',  ( -1.167979002624671470, 0.05413385826771666132, 0.4176697321401328100 ) ) ;
#82385=CARTESIAN_POINT ( 'NONE',  ( -0.7349081364829390672, 0.2306618581243847221, -0.2411417322834647770 ) ) ;
#82386=CARTESIAN_POINT ( 'NONE',  ( 0.8005249343832027131, 0.05413385826771666132, 0.4176697321401328100 ) ) ;
#82388=CARTESIAN_POINT ( 'NONE',  ( -0.3608923884514428360, 0.1771653543307087630, 0.09757992244046791164 ) ) ;
#82389=ORIENTED_EDGE ( 'NONE', *, *, #73735, .T. ) ;
#82392=CARTESIAN_POINT ( 'NONE',  ( -1.332020997375327642, -0.2845877964562161244, -0.3641732283464567121 ) ) ;
#82393=CARTESIAN_POINT ( 'NONE',  ( -0.9580052493438311334, 0.05413385826771626580, -0.4176697321401330321 ) ) ;
#82394=CARTESIAN_POINT ( 'NONE',  ( -1.049868766404198794, -0.6046776061558807314, 0.2411417322834647770 ) ) ;
#82396=CARTESIAN_POINT ( 'NONE',  ( -0.5643044619422565855, 0.05413385826771626580, -0.4176697321401330321 ) ) ;
#82397=CARTESIAN_POINT ( 'NONE',  ( -0.8005249343832013809, -0.4281496062992124485, 0.4176697321401328655 ) ) ;
#82398=CARTESIAN_POINT ( 'NONE',  ( -1.528871391076114250, -0.6692913385826771977, 0.1292274648535927661 ) ) ;
#82399=CARTESIAN_POINT ( 'NONE',  ( -1.725721784776902190, -0.05778040916215522460, 0.4822834645669289988 ) ) ;
#82400=CARTESIAN_POINT ( 'NONE',  ( 0.6758530183727039509, -0.5511811023622046335, 0.09757992244046803654 ) ) ;
#82401=DIRECTION ( 'NONE',  ( 0.000000000000000000, 0.000000000000000000, -1.000000000000000000 ) ) ;
#82403=CARTESIAN_POINT ( 'NONE',  ( 0.1640419947506569498, -0.08942795157527998196, 0.3641732283464567121 ) ) ;
#82404=CARTESIAN_POINT ( 'NONE',  ( -0.5052493438320203589, 0.2952755905511810774, -0.1292274648535930714 ) ) ;
#82405=CARTESIAN_POINT ( 'NONE',  ( 1.522309711286089939, -0.6046776061558809534, -0.2411417322834644161 ) ) ;
#82406=CARTESIAN_POINT ( 'NONE',  ( -0.1181102362204717315, -0.6692913385826771977, 8.415575281601705876E-17 ) ) ;
#82407=ORIENTED_EDGE ( 'NONE', *, *, #82040, .T. ) ;
#82410=ORIENTED_EDGE ( 'NONE', *, *, #2607, .T. ) ;
#82412=CARTESIAN_POINT ( 'NONE',  ( 1.167979002624672580, 0.05413385826771626580, -0.4176697321401330321 ) ) ;
#82413=CARTESIAN_POINT ( 'NONE',  ( -1.207349081364828880, 0.1283753931104746893, -0.1820866141732285504 ) ) ;
#82414=CARTESIAN_POINT ( 'NONE',  ( -1.522309711286088607, 0.2306618581243847221, -0.2411417322834647770 ) ) ;
#82418=CARTESIAN_POINT ( 'NONE',  ( 1.423884514435696413, -0.3162353388693409650, -0.4822834645669289433 ) ) ;
#82419=CARTESIAN_POINT ( 'NONE',  ( 0.4199475065616803948, -0.6046776061558809534, -0.2411417322834644161 ) ) ;
#82420=CARTESIAN_POINT ( 'NONE',  ( 0.1640419947506569498, -0.3162353388693409650, -0.4822834645669289433 ) ) ;
#82421=CARTESIAN_POINT ( 'NONE',  ( -1.141732283464566011, 0.1771653543307087630, 0.000000000000000000 ) ) ;
#82422=CARTESIAN_POINT ( 'NONE',  ( -0.4921259842519677963, -0.5400638737290844871, 0.3530559997133364547 ) ) ;
#82424=CARTESIAN_POINT ( 'NONE',  ( -0.9776902887139098386, -0.6692913385826771977, 0.1292274648535927661 ) ) ;
#82426=CARTESIAN_POINT ( 'NONE',  ( 1.318897637795276356, 0.07958543189024071263, -0.2665933059059888421 ) ) ;
#82427=CARTESIAN_POINT ( 'NONE',  ( -0.3871391076115479057, -0.2845877964562161244, -0.3641732283464567121 ) ) ;
#82429=CARTESIAN_POINT ( 'NONE',  ( 1.161417322834646493, -0.4536011799217367080, 0.2665933059059888421 ) ) ;
#82430=CARTESIAN_POINT ( 'NONE',  ( -1.666666666666665853, 0.05413385826771626580, -0.4176697321401330321 ) ) ;
#82431=CARTESIAN_POINT ( 'NONE',  ( 0.1474713956048451791, 8.471767977567108961E-16, -0.4445507791589058955 ) ) ;
#82432=CARTESIAN_POINT ( 'NONE',  ( 0.6692913385826778638, -0.5511811023622047445, 6.969142054262312111E-17 ) ) ;
#82433=CARTESIAN_POINT ( 'NONE',  ( -0.7808398950131222316, -0.3162353388693409650, -0.4822834645669289433 ) ) ;
#82434=CARTESIAN_POINT ( 'NONE',  ( 0.2624671916010504757, 0.2306618581243848609, 0.2411417322834645549 ) ) ;
#82435=CARTESIAN_POINT ( 'NONE',  ( 8.195543980992789655E-16, -0.1870078740157480601, -0.3641732283464567677 ) ) ;
#82436=CARTESIAN_POINT ( 'NONE',  ( -1.712598425196849572, 0.07958543189024085140, 0.2665933059059887866 ) ) ;
#82437=CARTESIAN_POINT ( 'NONE',  ( 0.9383202099737538715, -0.05778040916215560624, -0.4822834645669293319 ) ) ;
#82438=CARTESIAN_POINT ( 'NONE',  ( -1.220472440944882830, 0.2066929133858268208, 2.389277853677468338E-14 ) ) ;
#82440=CARTESIAN_POINT ( 'NONE',  ( 1.364829396325459854, -0.5023911411419708095, -0.1820866141732282451 ) ) ;
#82441=CARTESIAN_POINT ( 'NONE',  ( -0.7611548556430438595, 0.2306618581243848609, 0.2411417322834645549 ) ) ;
#82442=CARTESIAN_POINT ( 'NONE',  ( -0.3608923884514428360, 0.1771653543307087630, 0.09757992244046791164 ) ) ;
#82443=FACE_OUTER_BOUND ( 'NONE', #36293, .T. ) ;
#82444=CARTESIAN_POINT ( 'NONE',  ( 0.07217847769028949700, -0.08942795157528024563, -0.3641732283464568787 ) ) ;
#82445=CARTESIAN_POINT ( 'NONE',  ( -1.227034120734907585, 0.2952755905511811885, 0.1292274648535926551 ) ) ;
#82446=EDGE_CURVE ( 'NONE', #23151, #3487, #81919, .T. ) ;
#82447=CARTESIAN_POINT ( 'NONE',  ( -0.6430446194225712953, 0.05413385826771626580, -0.4176697321401330321 ) ) ;
#82451=CARTESIAN_POINT ( 'NONE',  ( 0.4330708661417329575, -0.5511811023622047445, 6.969142054262312111E-17 ) ) ;
#82452=CARTESIAN_POINT ( 'NONE',  ( -0.2755905511811015396, -0.6692913385826771977, 8.415575281601705876E-17 ) ) ;
#82453=CARTESIAN_POINT ( 'NONE',  ( -0.8595800524934373854, -0.05778040916215522460, 0.4822834645669289988 ) ) ;
#82454=CARTESIAN_POINT ( 'NONE',  ( -0.7020997375328074108, -0.08942795157527998196, 0.3641732283464567121 ) ) ;
#82456=CARTESIAN_POINT ( 'NONE',  ( -0.2362204724409440182, -0.1870078740157479769, 0.4822834645669291653 ) ) ;
#82457=CARTESIAN_POINT ( 'NONE',  ( -1.719160104986876103, -0.004921259842519576551, 0.3153832671262227771 ) ) ;
#82458=CARTESIAN_POINT ( 'NONE',  ( -1.502624671916009680, -0.3162353388693405765, 0.4822834645669290543 ) ) ;
#82459=CARTESIAN_POINT ( 'NONE',  ( -0.2462293917967295909, -2.567464376874931580E-15, -0.4445507791589072832 ) ) ;
#82462=CARTESIAN_POINT ( 'NONE',  ( -1.397637795275589623, 0.1660481256975885056, 0.3530559997133364547 ) ) ;
#82463=CARTESIAN_POINT ( 'NONE',  ( -0.8595800524934373854, -0.3162353388693409650, -0.4822834645669289433 ) ) ;
#82464=CARTESIAN_POINT ( 'NONE',  ( -1.456692913385826182, 0.2952755905511811885, 0.000000000000000000 ) ) ;
#82468=CARTESIAN_POINT ( 'NONE',  ( 0.7742782152230979209, 0.05413385826771626580, -0.4176697321401330321 ) ) ;
#82469=CARTESIAN_POINT ( 'NONE',  ( -0.1837270341207340729, 0.2306618581243847221, -0.2411417322834647770 ) ) ;
#82471=CARTESIAN_POINT ( 'NONE',  ( -0.6561679790026240244, 0.2306618581243847221, -0.2411417322834647770 ) ) ;
#82472=CARTESIAN_POINT ( 'NONE',  ( 1.062992125984252745, -0.5511811023622047445, 6.969142054262312111E-17 ) ) ;
#82477=CARTESIAN_POINT ( 'NONE',  ( 0.4986876640419954376, 0.2306618581243848609, 0.2411417322834645549 ) ) ;
#82478=CARTESIAN_POINT ( 'NONE',  ( -0.6758530183727028406, -0.6692913385826773087, -0.1292274648535924053 ) ) ;
#82479=CARTESIAN_POINT ( 'NONE',  ( -1.548556430446193399, -0.6046776061558809534, -0.2411417322834644161 ) ) ;
#82480=CARTESIAN_POINT ( 'NONE',  ( 0.7874015748031503170, -0.1870078740157480879, -0.4822834645669291653 ) ) ;
#82482=CARTESIAN_POINT ( 'NONE',  ( -1.535433070866141225, -0.5511811023622047445, 6.969142054262312111E-17 ) ) ;
#82484=CARTESIAN_POINT ( 'NONE',  ( -0.1312335958005241554, -0.6046776061558809534, -0.2411417322834644161 ) ) ;
#82485=CARTESIAN_POINT ( 'NONE',  ( -1.450131233595799651, 0.2952755905511810774, -0.1292274648535930714 ) ) ;
#82486=CARTESIAN_POINT ( 'NONE',  ( -1.627296587926508442, 0.2306618581243848609, 0.2411417322834645549 ) ) ;
#82487=CARTESIAN_POINT ( 'NONE',  ( 1.614173228346457378, -0.6692913385826771977, 8.415575281601705876E-17 ) ) ;
#82489=CARTESIAN_POINT ( 'NONE',  ( 0.7086614173228353852, -0.1870078740157479769, 0.3641732283464567677 ) ) ;
#82493=CARTESIAN_POINT ( 'NONE',  ( -0.1640419947506555343, -0.2845877964562159024, 0.3641732283464567677 ) ) ;
#82495=CARTESIAN_POINT ( 'NONE',  ( 0.4133858267716541968, -0.5400638737290845981, -0.3530559997133363437 ) ) ;
#82496=CARTESIAN_POINT ( 'NONE',  ( 0.4265091863517067039, -0.6692913385826773087, -0.1292274648535924053 ) ) ;
#82497=CARTESIAN_POINT ( 'NONE',  ( -0.4921259842519677963, -0.5400638737290844871, 0.3530559997133364547 ) ) ;
#82499=CARTESIAN_POINT ( 'NONE',  ( -1.122047244094487306, 0.1660481256975883668, -0.3530559997133364547 ) ) ;
#82501=CARTESIAN_POINT ( 'NONE',  ( 1.371391076115485719, -0.5511811023622048555, -0.09757992244046775898 ) ) ;
#82502=CARTESIAN_POINT ( 'NONE',  ( -1.469816272965878357, 0.2306618581243848609, 0.2411417322834645549 ) ) ;
#82503=CARTESIAN_POINT ( 'NONE',  ( 1.076115485564305141, 0.2306618581243847221, -0.2411417322834647770 ) ) ;
#82504=CARTESIAN_POINT ( 'NONE',  ( 1.312335958005250269, -0.6046776061558807314, 0.2411417322834647770 ) ) ;
#82506=CARTESIAN_POINT ( 'NONE',  ( -1.141732283464566011, -0.6692913385826771977, 8.415575281601705876E-17 ) ) ;
#82508=CARTESIAN_POINT ( 'NONE',  ( -0.2559055118110230564, 0.1660481256975883668, -0.3530559997133364547 ) ) ;
#82511=CARTESIAN_POINT ( 'NONE',  ( 1.332020997375329197, -0.3162353388693405765, 0.4822834645669290543 ) ) ;
#82512=CARTESIAN_POINT ( 'NONE',  ( 0.06561679790026316017, -0.3690944881889763329, 0.3153832671262228327 ) ) ;
#82513=CARTESIAN_POINT ( 'NONE',  ( 0.8464566929133865436, 0.1660481256975883668, -0.3530559997133364547 ) ) ;
#82515=CARTESIAN_POINT ( 'NONE',  ( 0.9251968503937015864, 0.07958543189024071263, -0.2665933059059888421 ) ) ;
#82516=CARTESIAN_POINT ( 'NONE',  ( 0.5183727034120741983, 0.2952755905511810774, -0.1292274648535930714 ) ) ;
#82518=CARTESIAN_POINT ( 'NONE',  ( -0.6299212598425188991, -0.1870078740157479769, 0.4822834645669291653 ) ) ;
#82519=CARTESIAN_POINT ( 'NONE',  ( 0.4849061582275022153, 1.805669738366188382, 0.4921425059946344938 ) ) ;
#82520=CARTESIAN_POINT ( 'NONE',  ( 0.7874015748031503170, -0.1870078740157479769, 0.3641732283464567677 ) ) ;
#82521=CARTESIAN_POINT ( 'NONE',  ( 0.1674892343164159914, -2.191421614605370878E-15, 0.4445507791589071167 ) ) ;
#82522=CARTESIAN_POINT ( 'NONE',  ( -0.4002624671916004129, -0.05778040916215560624, -0.4822834645669293319 ) ) ;
#82523=CARTESIAN_POINT ( 'NONE',  ( 0.2690288713910767848, 0.1771653543307087630, 0.09757992244046791164 ) ) ;
#82525=CARTESIAN_POINT ( 'NONE',  ( -0.1115485564304456306, 0.2952755905511810774, -0.1292274648535930714 ) ) ;
#82526=CARTESIAN_POINT ( 'NONE',  ( 0.5052493438320215802, 0.1771653543307087630, 0.09757992244046791164 ) ) ;
#82527=EDGE_CURVE ( 'NONE', #55143, #33617, #47367, .T. ) ;
#82529=CARTESIAN_POINT ( 'NONE',  ( 0.5052493438320218022, -0.6692913385826773087, -0.1292274648535924053 ) ) ;
#82530=CARTESIAN_POINT ( 'NONE',  ( 1.023622047244095334, -0.1870078740157479769, 0.3641732283464567677 ) ) ;
#82531=CARTESIAN_POINT ( 'NONE',  ( 0.1706036745406830368, 0.05413385826771666132, 0.4176697321401328100 ) ) ;
#82532=CARTESIAN_POINT ( 'NONE',  ( -0.3543307086614165824, -0.5511811023622047445, 6.969142054262312111E-17 ) ) ;
#82533=CARTESIAN_POINT ( 'NONE',  ( -0.7349081364829390672, 0.1283753931104746893, -0.1820866141732285504 ) ) ;
#82534=CARTESIAN_POINT ( 'NONE',  ( -0.3608923884514428360, 0.2952755905511811885, 0.1292274648535926551 ) ) ;
#82535=CARTESIAN_POINT ( 'NONE',  ( 0.1181102362204730916, -0.6692913385826771977, 8.415575281601705876E-17 ) ) ;
#82536=CARTESIAN_POINT ( 'NONE',  ( 0.8005249343832028242, -0.3690944881889765550, -0.3153832671262227771 ) ) ;
#82538=CARTESIAN_POINT ( 'NONE',  ( 1.482939632545932307, -0.004921259842519870586, -0.3153832671262229437 ) ) ;
#82540=CARTESIAN_POINT ( 'NONE',  ( 0.8727034120734913358, -0.05778040916215522460, 0.4822834645669289988 ) ) ;
#82542=CARTESIAN_POINT ( 'NONE',  ( -0.2034120734908131112, -0.6692913385826773087, -0.1292274648535924053 ) ) ;
#82544=CARTESIAN_POINT ( 'NONE',  ( 0.7480314960629927956, 0.2952755905511811885, 0.000000000000000000 ) ) ;
#82545=CARTESIAN_POINT ( 'NONE',  ( 0.5708661417322842269, 0.1660481256975885056, 0.3530559997133364547 ) ) ;
#82547=CARTESIAN_POINT ( 'NONE',  ( 0.5774278215223104249, 0.1283753931104748280, 0.1820866141732283561 ) ) ;
#82548=CARTESIAN_POINT ( 'NONE',  ( 1.332020997375329197, -0.3162353388693405765, 0.4822834645669290543 ) ) ;
#82549=CARTESIAN_POINT ( 'NONE',  ( -0.4330708661417315697, 0.1771653543307087630, 0.000000000000000000 ) ) ;
#82551=CARTESIAN_POINT ( 'NONE',  ( -0.3149606299212590610, -0.1870078740157480879, -0.4822834645669291653 ) ) ;
#82553=CARTESIAN_POINT ( 'NONE',  ( 0.1115485564304467270, -0.6692913385826773087, -0.1292274648535924053 ) ) ;
#82554=CARTESIAN_POINT ( 'NONE',  ( -0.9383202099737524282, -0.3162353388693409650, -0.4822834645669289433 ) ) ;
#82555=CARTESIAN_POINT ( 'NONE',  ( -0.7742782152230965886, -0.004921259842519576551, 0.3153832671262227771 ) ) ;
#82556=CARTESIAN_POINT ( 'NONE',  ( 0.2493438320209980519, -0.4281496062992127816, -0.4176697321401328100 ) ) ;
#82557=CARTESIAN_POINT ( 'NONE',  ( -1.207349081364828880, 0.2306618581243847221, -0.2411417322834647770 ) ) ;
#82558=CARTESIAN_POINT ( 'NONE',  ( -0.3083989501312330295, -0.3162353388693409650, -0.4822834645669289433 ) ) ;
#82559=CARTESIAN_POINT ( 'NONE',  ( -0.9333857237505057691, -2.609244250047836720E-15, 0.3791475997938242304 ) ) ;
#82560=CARTESIAN_POINT ( 'NONE',  ( 1.430446194225722500, 0.05413385826771666132, 0.4176697321401328100 ) ) ;
#82561=CARTESIAN_POINT ( 'NONE',  ( 1.607611548556431069, -0.6692913385826773087, -0.1292274648535924053 ) ) ;
#82564=CARTESIAN_POINT ( 'NONE',  ( -0.7939632545931754048, -0.3162353388693405765, 0.4822834645669290543 ) ) ;
#82567=ORIENTED_EDGE ( 'NONE', *, *, #27771, .T. ) ;
#82568=CARTESIAN_POINT ( 'NONE',  ( 0.5380577427821529035, -0.3690944881889763329, 0.3153832671262228327 ) ) ;
#82570=CARTESIAN_POINT ( 'NONE',  ( 0.6167979002624678353, -0.4281496062992124485, 0.4176697321401328655 ) ) ;
#82571=PLANE ( 'NONE',  #74464 ) ;
#82572=CARTESIAN_POINT ( 'NONE',  ( -0.5636006452641416642, -2.613618158232546091E-15, -0.3464511005275220379 ) ) ;
#82573=CARTESIAN_POINT ( 'NONE',  ( -0.2887139107611542133, -0.5023911411419708095, -0.1820866141732282451 ) ) ;
#82574=CARTESIAN_POINT ( 'NONE',  ( -0.2478063387913458926, 0.02791078216816347476, -0.4328096321851898631 ) ) ;
#82575=CARTESIAN_POINT ( 'NONE',  ( 1.305774278215223960, -0.6692913385826771977, 0.1292274648535927661 ) ) ;
#82576=CARTESIAN_POINT ( 'NONE',  ( 0.7808398950131240079, -0.2845877964562159024, 0.3641732283464567677 ) ) ;
#82577=CARTESIAN_POINT ( 'NONE',  ( -0.1443569553805765515, -0.4281496062992127816, -0.4176697321401328100 ) ) ;
#82579=CARTESIAN_POINT ( 'NONE',  ( -0.3871391076115476282, -0.05778040916215522460, 0.4822834645669289988 ) ) ;
#82580=CARTESIAN_POINT ( 'NONE',  ( -1.377952755905511140, 0.1771653543307087630, 0.000000000000000000 ) ) ;
#82581=CARTESIAN_POINT ( 'NONE',  ( -0.3608923884514428360, -0.6692913385826773087, -0.1292274648535924053 ) ) ;
#82586=CARTESIAN_POINT ( 'NONE',  ( 0.5314960629921267055, -0.5400638737290844871, 0.3530559997133364547 ) ) ;
#82588=CARTESIAN_POINT ( 'NONE',  ( -0.4658792650918627265, -0.05778040916215522460, 0.4822834645669289988 ) ) ;
#82589=CARTESIAN_POINT ( 'NONE',  ( -1.653543307086613234, -0.1870078740157479769, 0.4822834645669291653 ) ) ;
#82591=CARTESIAN_POINT ( 'NONE',  ( 0.8070866141732288002, 0.1660481256975885056, 0.3530559997133364547 ) ) ;
#82592=CARTESIAN_POINT ( 'NONE',  ( -0.07874015748031421014, -0.1870078740157479769, 0.4822834645669291653 ) ) ;
#82594=CARTESIAN_POINT ( 'NONE',  ( -0.5774278215223089816, 0.2306618581243847221, -0.2411417322834647770 ) ) ;
#82595=CARTESIAN_POINT ( 'NONE',  ( -0.2624671916010490880, -0.6046776061558807314, 0.2411417322834647770 ) ) ;
#82596=CARTESIAN_POINT ( 'NONE',  ( -0.8661417322834640276, -0.1870078740157479769, 0.4822834645669291653 ) ) ;
#82598=EDGE_CURVE ( 'NONE', #40878, #71072, #78505, .T. ) ;
#82599=CARTESIAN_POINT ( 'NONE',  ( 0.4921259842519691285, -0.4536011799217368745, -0.2665933059059886201 ) ) ;
#82601=CARTESIAN_POINT ( 'NONE',  ( -0.2559055118110230564, 0.1660481256975883668, -0.3530559997133364547 ) ) ;
#82603=CARTESIAN_POINT ( 'NONE',  ( 1.128608923884514947, 0.2306618581243848609, 0.2411417322834645549 ) ) ;
#82607=CARTESIAN_POINT ( 'NONE',  ( 0.3083989501312343062, -0.05778040916215560624, -0.4822834645669293319 ) ) ;
#82608=CARTESIAN_POINT ( 'NONE',  ( 0.2887139107611556010, -0.5023911411419708095, 0.1820866141732285504 ) ) ;
#82609=CARTESIAN_POINT ( 'NONE',  ( 1.246719160104987623, -0.004921259842519870586, -0.3153832671262229437 ) ) ;
#82615=CARTESIAN_POINT ( 'NONE',  ( 0.5380577427821529035, 0.05413385826771626580, -0.4176697321401330321 ) ) ;
#82616=CARTESIAN_POINT ( 'NONE',  ( -1.272965879265091305, 0.05413385826771626580, -0.4176697321401330321 ) ) ;
#82617=CARTESIAN_POINT ( 'NONE',  ( -1.043307086614172707, 0.1660481256975883668, -0.3530559997133364547 ) ) ;
#82618=CARTESIAN_POINT ( 'NONE',  ( 0.07874015748031558404, -0.1870078740157480879, -0.4822834645669291653 ) ) ;
#82619=CARTESIAN_POINT ( 'NONE',  ( 1.089238845144357537, -0.4281496062992124485, 0.4176697321401328655 ) ) ;
#82620=CARTESIAN_POINT ( 'NONE',  ( 1.404199475065617708, -0.004921259842519870586, -0.3153832671262229437 ) ) ;
#82622=CARTESIAN_POINT ( 'NONE',  ( 0.8464566929133866546, -0.4536011799217367080, 0.2665933059059888421 ) ) ;
#82623=CARTESIAN_POINT ( 'NONE',  ( -0.7217847769028863381, -0.4281496062992124485, 0.4176697321401328655 ) ) ;
#82626=CARTESIAN_POINT ( 'NONE',  ( -1.548556430446193399, -0.5023911411419708095, -0.1820866141732282451 ) ) ;
#82628=CARTESIAN_POINT ( 'NONE',  ( 1.259842519685040019, -0.1870078740157480879, -0.4822834645669291653 ) ) ;
#82630=CARTESIAN_POINT ( 'NONE',  ( -1.712598425196849572, 0.07958543189024085140, 0.2665933059059887866 ) ) ;
#82631=CARTESIAN_POINT ( 'NONE',  ( 0.1312335958005257930, 0.2306618581243847221, -0.2411417322834647770 ) ) ;
#82632=CARTESIAN_POINT ( 'NONE',  ( 1.010498687664042716, -0.004921259842519870586, -0.3153832671262229437 ) ) ;
#82634=CARTESIAN_POINT ( 'NONE',  ( -1.502624671916009680, -0.08942795157528024563, -0.3641732283464568787 ) ) ;
#82635=CARTESIAN_POINT ( 'NONE',  ( 1.102362204724410155, -0.1870078740157480879, -0.4822834645669291653 ) ) ;
#82636=CARTESIAN_POINT ( 'NONE',  ( -0.4921259842519677963, 0.1660481256975883391, -0.3530559997133364547 ) ) ;
#82637=CARTESIAN_POINT ( 'NONE',  ( -0.5511811023622041894, -0.1870078740157480601, -0.3641732283464567677 ) ) ;
#82638=CARTESIAN_POINT ( 'NONE',  ( -0.7414698162729651543, 0.2952755905511810774, -0.1292274648535930714 ) ) ;
#82639=CARTESIAN_POINT ( 'NONE',  ( 1.404199475065617708, 0.05413385826771626580, -0.4176697321401330321 ) ) ;
#82640=CARTESIAN_POINT ( 'NONE',  ( -1.233595800524933894, 0.2306618581243848609, 0.2411417322834645549 ) ) ;
#82641=CARTESIAN_POINT ( 'NONE',  ( 1.548556430446194954, 0.2306618581243847221, -0.2411417322834647770 ) ) ;
#82643=CARTESIAN_POINT ( 'NONE',  ( -1.351706036745406347, -0.3690944881889763329, 0.3153832671262228327 ) ) ;
#82645=CARTESIAN_POINT ( 'NONE',  ( 1.102362204724410155, -0.1870078740157479769, 0.4822834645669291653 ) ) ;
#82647=CARTESIAN_POINT ( 'NONE',  ( -1.706036745406823485, 0.2306618581243848609, 0.2411417322834645549 ) ) ;
#82648=CARTESIAN_POINT ( 'NONE',  ( -1.397637795275589623, -0.4536011799217368745, -0.2665933059059886201 ) ) ;
#82649=CARTESIAN_POINT ( 'NONE',  ( -0.8923884514435688198, 0.1283753931104746893, -0.1820866141732285504 ) ) ;
#82650=CARTESIAN_POINT ( 'NONE',  ( 1.502624671916010790, -0.08942795157527998196, 0.3641732283464567121 ) ) ;
#82651=CARTESIAN_POINT ( 'NONE',  ( -0.5708661417322825615, -0.5400638737290844871, 0.3530559997133364547 ) ) ;
#82652=CARTESIAN_POINT ( 'NONE',  ( 0.1837270341207357105, -0.5023911411419708095, -0.1820866141732282451 ) ) ;
#82653=CARTESIAN_POINT ( 'NONE',  ( -1.417322834645668772, -0.1870078740157479769, 0.3641732283464567677 ) ) ;
#82654=CARTESIAN_POINT ( 'NONE',  ( 1.548556430446194954, -0.5023911411419708095, 0.1820866141732285504 ) ) ;
#82655=CARTESIAN_POINT ( 'NONE',  ( 0.7939632545931766261, -0.3162353388693409650, -0.4822834645669289433 ) ) ;
#82656=CARTESIAN_POINT ( 'NONE',  ( -0.6399301791983041943, -2.567464376874931580E-15, -0.4445507791589072832 ) ) ;
#82657=CARTESIAN_POINT ( 'NONE',  ( 0.09186351706036827158, -0.004921259842519576551, 0.3153832671262227771 ) ) ;
#82659=CARTESIAN_POINT ( 'NONE',  ( 0.5314960629921267055, -0.5400638737290844871, 0.3530559997133364547 ) ) ;
#82660=CARTESIAN_POINT ( 'NONE',  ( 0.9842519685039375910, 0.1771653543307087630, 0.000000000000000000 ) ) ;
#82662=CARTESIAN_POINT ( 'NONE',  ( -1.496062992125983815, -0.1870078740157479769, 0.4822834645669291653 ) ) ;
#82663=CARTESIAN_POINT ( 'NONE',  ( -1.299212598425196097, 0.2952755905511811885, 0.000000000000000000 ) ) ;
#82664=CARTESIAN_POINT ( 'NONE',  ( -0.1771653543307080136, -0.5400638737290844871, 0.3530559997133364547 ) ) ;
#82667=CARTESIAN_POINT ( 'NONE',  ( 0.5577427821522314977, -0.3162353388693409650, -0.4822834645669289433 ) ) ;
#82668=CARTESIAN_POINT ( 'NONE',  ( 1.003937007874016185, 0.07958543189024071263, -0.2665933059059888421 ) ) ;
#82669=CARTESIAN_POINT ( 'NONE',  ( -0.3083989501312330295, -0.3162353388693409650, -0.4822834645669289433 ) ) ;
#82670=CARTESIAN_POINT ( 'NONE',  ( 0.1574803149606306130, -0.1870078740157479769, 0.4822834645669291653 ) ) ;
#82676=CARTESIAN_POINT ( 'NONE',  ( -0.4790026246719154557, -0.2845877964562159024, 0.3641732283464567677 ) ) ;
#82677=CARTESIAN_POINT ( 'NONE',  ( -0.8005249343832013809, -0.4281496062992124485, 0.4176697321401328655 ) ) ;
#82679=CARTESIAN_POINT ( 'NONE',  ( 1.010498687664042716, -0.4281496062992124485, 0.4176697321401328655 ) ) ;
#82680=CARTESIAN_POINT ( 'NONE',  ( -1.581364829396324945, -0.05778040916215560624, -0.4822834645669293319 ) ) ;
#82681=CARTESIAN_POINT ( 'NONE',  ( 0.7808398950131240079, -0.3162353388693405765, 0.4822834645669290543 ) ) ;
#82684=CARTESIAN_POINT ( 'NONE',  ( 1.607611548556431069, -0.6692913385826773087, -0.1292274648535924053 ) ) ;
#82685=CARTESIAN_POINT ( 'NONE',  ( 0.7414698162729663755, -0.6692913385826773087, -0.1292274648535924053 ) ) ;
#82686=EDGE_CURVE ( 'NONE', #55143, #16761, #64606, .T. ) ;
#82687=CARTESIAN_POINT ( 'NONE',  ( 0.7611548556430451917, -0.6046776061558807314, 0.2411417322834647770 ) ) ;
#82688=CARTESIAN_POINT ( 'NONE',  ( 1.010498687664042716, -0.004921259842519870586, -0.3153832671262229437 ) ) ;
#82689=CARTESIAN_POINT ( 'NONE',  ( 1.246719160104987623, 0.05413385826771626580, -0.4176697321401330321 ) ) ;
#82692=CARTESIAN_POINT ( 'NONE',  ( 0.7611548556430454138, 0.2306618581243847221, -0.2411417322834647770 ) ) ;
#82693=CARTESIAN_POINT ( 'NONE',  ( 1.548556430446194954, 0.1283753931104746893, -0.1820866141732285504 ) ) ;
#82694=CARTESIAN_POINT ( 'NONE',  ( -0.8464566929133852113, -0.5400638737290845981, -0.3530559997133363437 ) ) ;
#82695=CARTESIAN_POINT ( 'NONE',  ( -0.8530183727034112984, -0.4281496062992127816, -0.4176697321401328100 ) ) ;
#82696=CARTESIAN_POINT ( 'NONE',  ( 0.9711286089238851948, 0.2306618581243848609, 0.2411417322834645549 ) ) ;
#82703=CARTESIAN_POINT ( 'NONE',  ( -1.595398199321657939, 0.4619154201552267414, 0.1559797534342468872 ) ) ;
#82704=CARTESIAN_POINT ( 'NONE',  ( 1.568241469816273437, -0.2845877964562159024, 0.3641732283464567677 ) ) ;
#82706=CARTESIAN_POINT ( 'NONE',  ( 1.325459317585302665, -0.3690944881889763329, 0.3153832671262228327 ) ) ;
#82708=DIRECTION ( 'NONE',  ( 0.000000000000000000, 1.000000000000000000, 0.000000000000000000 ) ) ;
#82711=( BOUNDED_CURVE ( )  B_SPLINE_CURVE ( 2, ( #54960, #53709, #60038, #22979, #15440, #67611, #16272, #47815, #28464, #28879, #61701, #48646, #23390 ),
 .UNSPECIFIED., .F., .F. ) 
 B_SPLINE_CURVE_WITH_KNOTS ( ( 3, 2, 2, 2, 2, 2, 3 ),
 ( 0.3551492764529827206, 0.3560606060606060774, 0.3598484848484848619, 0.3636363636363636465, 0.3674242424242424310, 0.3712121212121212155, 0.3721234508197446278 ),
 .UNSPECIFIED. ) 
 CURVE ( )  GEOMETRIC_REPRESENTATION_ITEM ( )  RATIONAL_B_SPLINE_CURVE ( ( 0.9875488213027530104, 0.9918020599134685922, 1.000000000000000000, 0.9659258262890683122, 1.000000000000000000, 0.9659258262890683122, 1.000000000000000000, 0.9659258262890683122, 1.000000000000000000, 0.9659258262890683122, 1.000000000000000000, 0.9918020599134680371, 0.9875488213027523443 ) ) 
 REPRESENTATION_ITEM ( '' )  );
#82712=CARTESIAN_POINT ( 'NONE',  ( -0.8464566929133852113, 0.07958543189024085140, 0.2665933059059887866 ) ) ;
#82713=CARTESIAN_POINT ( 'NONE',  ( -1.181102362204723644, -0.1870078740157479769, 0.4822834645669291653 ) ) ;
#82714=CARTESIAN_POINT ( 'NONE',  ( 0.2493438320209980519, -0.4281496062992127816, -0.4176697321401328100 ) ) ;
#82715=CARTESIAN_POINT ( 'NONE',  ( 1.404199475065617264, -0.4281496062992124485, 0.4176697321401328655 ) ) ;
#82721=CARTESIAN_POINT ( 'NONE',  ( -0.5314960629921250401, 0.07958543189024085140, 0.2665933059059887866 ) ) ;
#82722=CARTESIAN_POINT ( 'NONE',  ( -1.371391076115484609, -0.6692913385826771977, 0.1292274648535927661 ) ) ;
#82723=CARTESIAN_POINT ( 'NONE',  ( 0.8398950131233602345, -0.6046776061558807314, 0.2411417322834647770 ) ) ;
#82728=CARTESIAN_POINT ( 'NONE',  ( 1.338582677165355062, -0.1870078740157479769, 0.4822834645669291653 ) ) ;
#82729=CARTESIAN_POINT ( 'NONE',  ( -1.246719160104986512, 0.05413385826771666132, 0.4176697321401328100 ) ) ;
#82731=CARTESIAN_POINT ( 'NONE',  ( -0.3083989501312330295, -0.08942795157527998196, 0.3641732283464567121 ) ) ;
#82733=CARTESIAN_POINT ( 'NONE',  ( -0.3412073490813641308, 0.1283753931104746893, -0.1820866141732285504 ) ) ;
#82734=CARTESIAN_POINT ( 'NONE',  ( 0.3346456692913390985, 0.07958543189024085140, 0.2665933059059887866 ) ) ;
#82735=CARTESIAN_POINT ( 'NONE',  ( 0.2230971128608929543, 0.05413385826771626580, -0.4176697321401330321 ) ) ;
#82736=CARTESIAN_POINT ( 'NONE',  ( -0.5643044619422565855, -0.3690944881889763329, 0.3153832671262228327 ) ) ;
#82738=CARTESIAN_POINT ( 'NONE',  ( 1.299212598425197429, 0.2952755905511811885, 0.000000000000000000 ) ) ;
#82739=CARTESIAN_POINT ( 'NONE',  ( -0.9186351706036736120, -0.6046776061558809534, -0.2411417322834644161 ) ) ;
#82741=CARTESIAN_POINT ( 'NONE',  ( -0.2230971128608915943, -0.4281496062992127816, -0.4176697321401328100 ) ) ;
#82742=CARTESIAN_POINT ( 'NONE',  ( -0.9251968503937002541, -0.5400638737290845981, -0.3530559997133363437 ) ) ;
#82743=CARTESIAN_POINT ( 'NONE',  ( 1.089238845144357759, -0.004921259842519870586, -0.3153832671262229437 ) ) ;
#82744=CARTESIAN_POINT ( 'NONE',  ( -0.3608923884514428360, -0.5511811023622048555, -0.09757992244046775898 ) ) ;
#82745=CARTESIAN_POINT ( 'NONE',  ( -0.5708661417322828946, 0.1660481256975883668, -0.3530559997133364547 ) ) ;
#82746=CARTESIAN_POINT ( 'NONE',  ( -1.174540682414697335, -0.05778040916215522460, 0.4822834645669289988 ) ) ;
#82747=CARTESIAN_POINT ( 'NONE',  ( 1.410761154855643795, -0.08942795157528024563, -0.3641732283464568787 ) ) ;
#82748=CARTESIAN_POINT ( 'NONE',  ( -0.2887139107611542133, -0.6046776061558809534, -0.2411417322834644161 ) ) ;
#82749=CARTESIAN_POINT ( 'NONE',  ( -1.062992125984250968, 0.2952755905511811885, 0.000000000000000000 ) ) ;
#82752=CARTESIAN_POINT ( 'NONE',  ( -0.8464566929133852113, 0.07958543189024085140, 0.2665933059059887866 ) ) ;
#82753=CARTESIAN_POINT ( 'NONE',  ( 1.299212598425197429, 0.2952755905511811885, 0.000000000000000000 ) ) ;
#82754=CARTESIAN_POINT ( 'NONE',  ( -1.272965879265091305, -0.3690944881889763329, 0.3153832671262228327 ) ) ;
#82756=CARTESIAN_POINT ( 'NONE',  ( -1.023622047244094002, -0.1870078740157480879, -0.4822834645669291653 ) ) ;
#82758=CARTESIAN_POINT ( 'NONE',  ( 1.371391076115485941, 0.2952755905511811885, 0.1292274648535926551 ) ) ;
#82759=CARTESIAN_POINT ( 'NONE',  ( 0.9120734908136490793, 0.2952755905511810774, -0.1292274648535930714 ) ) ;
#82760=CARTESIAN_POINT ( 'NONE',  ( 1.555118110236221041, -0.5400638737290844871, 0.3530559997133364547 ) ) ;
#82761=CARTESIAN_POINT ( 'NONE',  ( -1.286089238845143479, -0.5023911411419708095, 0.1820866141732285504 ) ) ;
#82766=CARTESIAN_POINT ( 'NONE',  ( 1.207349081364829990, 0.1283753931104748280, 0.1820866141732283561 ) ) ;
#82767=CARTESIAN_POINT ( 'NONE',  ( 0.7217847769028878924, -0.3690944881889765550, -0.3153832671262227771 ) ) ;
#82768=CARTESIAN_POINT ( 'NONE',  ( 0.7086614173228352742, -0.1870078740157480879, -0.4822834645669291653 ) ) ;
#82771=CARTESIAN_POINT ( 'NONE',  ( 0.9186351706036752773, 0.1283753931104746893, -0.1820866141732285504 ) ) ;
#82773=CARTESIAN_POINT ( 'NONE',  ( -0.4527559055118102749, -0.5400638737290845981, -0.3530559997133363437 ) ) ;
#82774=CARTESIAN_POINT ( 'NONE',  ( -1.036745406824146176, -0.4281496062992124485, 0.4176697321401328655 ) ) ;
#82775=CARTESIAN_POINT ( 'NONE',  ( 0.8858267716535438430, 0.1660481256975885056, 0.3530559997133364547 ) ) ;
#82778=VECTOR ( 'NONE', #27019, 39.37007874015748143 ) ;
#82779=ORIENTED_EDGE ( 'NONE', *, *, #37456, .T. ) ;
#82780=EDGE_LOOP ( 'NONE', ( #58954, #64066, #20986, #34421 ) ) ;
#82781=CARTESIAN_POINT ( 'NONE',  ( -1.430446194225721390, -0.4281496062992124485, 0.4176697321401328655 ) ) ;
#82782=CARTESIAN_POINT ( 'NONE',  ( -0.6299212598425188991, -0.1870078740157480879, -0.4822834645669291653 ) ) ;
#82783=CARTESIAN_POINT ( 'NONE',  ( -0.9842519685039360366, 0.1771653543307087630, 0.000000000000000000 ) ) ;
#82784=CARTESIAN_POINT ( 'NONE',  ( -0.8661417322834640276, -0.1870078740157479769, 0.4822834645669291653 ) ) ;
#82785=CARTESIAN_POINT ( 'NONE',  ( 0.5446194225721792126, -0.3162353388693405765, 0.4822834645669290543 ) ) ;
#82786=CARTESIAN_POINT ( 'NONE',  ( -0.5774278215223089816, -0.6046776061558807314, 0.2411417322834647770 ) ) ;
#82787=CARTESIAN_POINT ( 'NONE',  ( -1.371391076115484609, -0.6692913385826771977, 0.1292274648535927661 ) ) ;
#82788=CARTESIAN_POINT ( 'NONE',  ( -0.8398950131233589023, -0.6046776061558809534, -0.2411417322834644161 ) ) ;
#82789=CARTESIAN_POINT ( 'NONE',  ( 0.7742782152230978099, -0.4281496062992124485, 0.4176697321401328655 ) ) ;
#82791=CARTESIAN_POINT ( 'NONE',  ( -0.9317585301837263412, -0.3690944881889765550, -0.3153832671262227771 ) ) ;
#82795=CARTESIAN_POINT ( 'NONE',  ( -1.213910761154854745, 0.1771653543307087075, -0.09757992244046823083 ) ) ;
#82796=CARTESIAN_POINT ( 'NONE',  ( -0.9448818897637790704, -0.1870078740157480879, -0.4822834645669291653 ) ) ;
#82797=CARTESIAN_POINT ( 'NONE',  ( -0.8530183727034112984, 0.05413385826771666132, 0.4176697321401328100 ) ) ;
#82799=CARTESIAN_POINT ( 'NONE',  ( -0.9186351706036736120, 0.2306618581243848609, 0.2411417322834645549 ) ) ;
#82800=CARTESIAN_POINT ( 'NONE',  ( -1.423884514435694859, -0.3162353388693405765, 0.4822834645669290543 ) ) ;
#82802=CARTESIAN_POINT ( 'NONE',  ( -1.614173228346457378, 0.4410134679336882302, 0.1372047244094476981 ) ) ;
#82803=CARTESIAN_POINT ( 'NONE',  ( 0.6692913385826778638, -0.5511811023622047445, 6.969142054262312111E-17 ) ) ;
#82804=CARTESIAN_POINT ( 'NONE',  ( -0.4839371108951621148, -3.153061149046662969E-15, -0.3791475997938244524 ) ) ;
#82806=CARTESIAN_POINT ( 'NONE',  ( 0.1377952755905518800, -0.4536011799217367080, 0.2665933059059888421 ) ) ;
#82807=CARTESIAN_POINT ( 'NONE',  ( -0.3412073490813641308, 0.2306618581243847221, -0.2411417322834647770 ) ) ;
#82808=CARTESIAN_POINT ( 'NONE',  ( 1.561679790026247350, -0.4281496062992124485, 0.4176697321401328655 ) ) ;
#82809=CARTESIAN_POINT ( 'NONE',  ( -0.3608923884514428360, 0.2952755905511811885, 0.1292274648535926551 ) ) ;
#82810=EDGE_LOOP ( 'NONE', ( #38602, #59210, #8482, #53623, #64765, #41110, #9542, #16053, #60529, #3718, #36112, #35889, #50186, #69542, #24163, #69148, #15950, #67973, #49985, #76818 ) ) ;
#82811=CARTESIAN_POINT ( 'NONE',  ( 0.2462293917967310342, -2.191421614605370878E-15, 0.4445507791589071167 ) ) ;
#82814=CARTESIAN_POINT ( 'NONE',  ( -0.6233595800524928121, -0.3162353388693409650, -0.4822834645669289433 ) ) ;
#82815=CARTESIAN_POINT ( 'NONE',  ( 1.469816272965879911, 0.2306618581243847221, -0.2411417322834647770 ) ) ;
#82816=CARTESIAN_POINT ( 'NONE',  ( -1.187664041994750175, -0.08942795157528024563, -0.3641732283464568787 ) ) ;
#82817=CARTESIAN_POINT ( 'NONE',  ( -1.456692913385826182, -0.6692913385826771977, 8.415575281601705876E-17 ) ) ;
#82819=CARTESIAN_POINT ( 'NONE',  ( 0.3249695492770460770, 1.223219560026271499E-15, 0.4445507791589056734 ) ) ;
#82821=CARTESIAN_POINT ( 'NONE',  ( 1.443569553805774897, -0.6046776061558809534, -0.2411417322834644161 ) ) ;
#82824=CARTESIAN_POINT ( 'NONE',  ( 0.1837270341207357105, -0.6046776061558809534, -0.2411417322834644161 ) ) ;
#82825=CARTESIAN_POINT ( 'NONE',  ( -0.8661417322834640276, -0.1870078740157479769, 0.3641732283464567677 ) ) ;
#82828=CARTESIAN_POINT ( 'NONE',  ( -0.4002624671916004129, -0.05778040916215560624, -0.4822834645669293319 ) ) ;
#82830=CARTESIAN_POINT ( 'NONE',  ( -0.7414698162729651543, 0.2952755905511810774, -0.1292274648535930714 ) ) ;
#82831=CARTESIAN_POINT ( 'NONE',  ( -1.161417322834644716, -0.5400638737290845981, -0.3530559997133363437 ) ) ;
#82833=CARTESIAN_POINT ( 'NONE',  ( 0.6692913385826777528, 0.1771653543307087630, 0.000000000000000000 ) ) ;
#82834=CARTESIAN_POINT ( 'NONE',  ( -0.3346456692913377662, -0.4536011799217367080, 0.2665933059059888421 ) ) ;
#82835=CARTESIAN_POINT ( 'NONE',  ( 0.9055118110236227702, 0.1771653543307087630, 0.000000000000000000 ) ) ;
#82836=CARTESIAN_POINT ( 'NONE',  ( -1.437007874015747477, -0.5400638737290844871, 0.3530559997133364547 ) ) ;
#82837=CARTESIAN_POINT ( 'NONE',  ( 1.358267716535433323, -0.5400638737290845981, -0.3530559997133363437 ) ) ;
#82838=CARTESIAN_POINT ( 'NONE',  ( 0.4527559055118117182, 0.07958543189024071263, -0.2665933059059888421 ) ) ;
#82839=CARTESIAN_POINT ( 'NONE',  ( -0.6496062992125976043, 0.1660481256975883668, -0.3530559997133364547 ) ) ;
#82840=CARTESIAN_POINT ( 'NONE',  ( 1.410761154855643795, -0.3162353388693405765, 0.4822834645669290543 ) ) ;
#82841=( BOUNDED_CURVE ( )  B_SPLINE_CURVE ( 2, ( #72675, #34374, #8703, #28051, #73518, #74341, #47401, #67200, #29707, #34795, #9531, #28465, #15867 ),
 .UNSPECIFIED., .F., .F. ) 
 B_SPLINE_CURVE_WITH_KNOTS ( ( 3, 2, 2, 2, 2, 2, 3 ),
 ( 0.5824220037257099580, 0.5833333333333333703, 0.5871212121212121549, 0.5909090909090909394, 0.5946969696969697239, 0.5984848484848485084, 0.5993961780924720317 ),
 .UNSPECIFIED. ) 
 CURVE ( )  GEOMETRIC_REPRESENTATION_ITEM ( )  RATIONAL_B_SPLINE_CURVE ( ( 0.9875488213027523443, 0.9918020599134680371, 1.000000000000000000, 0.9659258262890683122, 1.000000000000000000, 0.9659258262890683122, 1.000000000000000000, 0.9659258262890683122, 1.000000000000000000, 0.9659258262890683122, 1.000000000000000000, 0.9918020599134671489, 0.9875488213027514561 ) ) 
 REPRESENTATION_ITEM ( '' )  );
#82842=AXIS2_PLACEMENT_3D ( 'NONE', #28895, #66379, #47414 ) ;
#82844=CARTESIAN_POINT ( 'NONE',  ( -0.1574803149606292529, -0.1870078740157480601, -0.3641732283464567677 ) ) ;
#82845=CARTESIAN_POINT ( 'NONE',  ( 0.2462293917967310342, -2.191421614605370878E-15, 0.4445507791589071167 ) ) ;
#82846=CARTESIAN_POINT ( 'NONE',  ( 0.4855643044619430415, -0.4281496062992127816, -0.4176697321401328100 ) ) ;
#82848=CARTESIAN_POINT ( 'NONE',  ( 1.259842519685040019, -0.1870078740157479769, 0.3641732283464567677 ) ) ;
#82849=CARTESIAN_POINT ( 'NONE',  ( 0.1377952755905518800, -0.4536011799217367080, 0.2665933059059888421 ) ) ;
#82850=CARTESIAN_POINT ( 'NONE',  ( -1.502624671916009680, -0.05778040916215560624, -0.4822834645669293319 ) ) ;
#82851=CARTESIAN_POINT ( 'NONE',  ( -0.6364829396325453192, -0.08942795157528024563, -0.3641732283464568787 ) ) ;
#82853=CARTESIAN_POINT ( 'NONE',  ( -1.108923884514435132, -0.3162353388693405765, 0.4822834645669290543 ) ) ;
#82854=B_SPLINE_CURVE_WITH_KNOTS ( 'NONE', 3,
 ( #564, #51880, #26217, #43492, #69188, #11539, #62876 ),
 .UNSPECIFIED., .F., .F.,
 ( 4, 3, 4 ),
 ( 3.643951726750583631E-17, 0.001246232571205268744, 0.002492492258783277591 ),
 .UNSPECIFIED. ) ;
#82855=CARTESIAN_POINT ( 'NONE',  ( -0.6496062992125976043, 0.1660481256975883668, -0.3530559997133364547 ) ) ;
#82858=CARTESIAN_POINT ( 'NONE',  ( 0.5971128608923890191, -0.5511811023622046335, 0.09757992244046803654 ) ) ;
#82859=CARTESIAN_POINT ( 'NONE',  ( -0.1640419947506553400, -0.05778040916215560624, -0.4822834645669293319 ) ) ;
#82860=CARTESIAN_POINT ( 'NONE',  ( -0.6430446194225712953, 0.05413385826771626580, -0.4176697321401330321 ) ) ;
#82861=CARTESIAN_POINT ( 'NONE',  ( -0.7742782152230962556, -0.3690944881889765550, -0.3153832671262227771 ) ) ;
#82863=CARTESIAN_POINT ( 'NONE',  ( 0.1115485564304470323, 0.2952755905511811885, 0.1292274648535926551 ) ) ;
#82864=CARTESIAN_POINT ( 'NONE',  ( -1.607611548556429737, -0.5511811023622046335, 0.09757992244046803654 ) ) ;
#82865=CARTESIAN_POINT ( 'NONE',  ( 1.318897637795276356, 0.1660481256975883668, -0.3530559997133364547 ) ) ;
#82869=CARTESIAN_POINT ( 'NONE',  ( -1.187664041994750175, -0.05778040916215560624, -0.4822834645669293319 ) ) ;
#82870=CARTESIAN_POINT ( 'NONE',  ( -0.6824146981627291497, -0.6046776061558809534, -0.2411417322834644161 ) ) ;
#82871=CARTESIAN_POINT ( 'NONE',  ( 1.456692913385827515, 0.2952755905511811885, 0.000000000000000000 ) ) ;
#82875=CARTESIAN_POINT ( 'NONE',  ( 0.7808398950131241190, -0.05778040916215560624, -0.4822834645669293319 ) ) ;
#82876=CARTESIAN_POINT ( 'NONE',  ( 0.05905511811023709395, -0.5400638737290844871, 0.3530559997133364547 ) ) ;
#82880=VECTOR ( 'NONE', #13745, 39.37007874015748143 ) ;
#82882=CARTESIAN_POINT ( 'NONE',  ( 1.036745406824147508, -0.3690944881889765550, -0.3153832671262227771 ) ) ;
#82884=ORIENTED_EDGE ( 'NONE', *, *, #31934, .T. ) ;
#82887=CARTESIAN_POINT ( 'NONE',  ( 0.5446194225721792126, -0.05778040916215560624, -0.4822834645669293319 ) ) ;
#82888=CARTESIAN_POINT ( 'NONE',  ( -0.6102362204724400829, 0.1660481256975885056, 0.3530559997133364547 ) ) ;
#82889=CARTESIAN_POINT ( 'NONE',  ( -1.377952755905511140, -0.6692913385826771977, 8.415575281601705876E-17 ) ) ;
#82890=CARTESIAN_POINT ( 'NONE',  ( 0.6430446194225729606, -0.4281496062992127816, -0.4176697321401328100 ) ) ;
#82891=CARTESIAN_POINT ( 'NONE',  ( 1.653543307086614789, -0.1870078740157479769, 0.4822834645669291653 ) ) ;
#82892=CARTESIAN_POINT ( 'NONE',  ( 1.555118110236221041, -0.5400638737290844871, 0.3530559997133364547 ) ) ;
#82893=CARTESIAN_POINT ( 'NONE',  ( 0.09842519685039434474, 0.1660481256975885056, 0.3530559997133364547 ) ) ;
#82894=CARTESIAN_POINT ( 'NONE',  ( -1.174540682414697335, -0.05778040916215522460, 0.4822834645669289988 ) ) ;
#82895=CARTESIAN_POINT ( 'NONE',  ( 1.509186351706037543, -0.4281496062992127816, -0.4176697321401328100 ) ) ;
#82896=CARTESIAN_POINT ( 'NONE',  ( 1.548556430446194954, 0.2306618581243847221, -0.2411417322834647770 ) ) ;
#82898=CARTESIAN_POINT ( 'NONE',  ( 1.056430446194226658, 0.1771653543307087630, 0.09757992244046791164 ) ) ;
#82899=VERTEX_POINT ( 'NONE', #7792 ) ;
#82902=CARTESIAN_POINT ( 'NONE',  ( 0.1115485564304467270, -0.5511811023622048555, -0.09757992244046775898 ) ) ;
#82904=CARTESIAN_POINT ( 'NONE',  ( 0.1377952755905518800, -0.5400638737290844871, 0.3530559997133364547 ) ) ;
#82905=CARTESIAN_POINT ( 'NONE',  ( 0.5839895013123367340, -0.6692913385826773087, -0.1292274648535924053 ) ) ;
#82906=CARTESIAN_POINT ( 'NONE',  ( -0.6627296587926503335, -0.6692913385826771977, 0.1292274648535927661 ) ) ;
#82908=CARTESIAN_POINT ( 'NONE',  ( -1.174540682414697335, -0.05778040916215522460, 0.4822834645669289988 ) ) ;
#82910=CARTESIAN_POINT ( 'NONE',  ( 1.213910761154856299, -0.5511811023622048555, -0.09757992244046775898 ) ) ;
#82911=CARTESIAN_POINT ( 'NONE',  ( 0.7742782152230979209, 0.05413385826771626580, -0.4176697321401330321 ) ) ;
#82912=CARTESIAN_POINT ( 'NONE',  ( 0.5839895013123367340, 0.2952755905511811885, 0.1292274648535926551 ) ) ;
#82915=CARTESIAN_POINT ( 'NONE',  ( -1.443569553805773564, -0.6046776061558807314, 0.2411417322834647770 ) ) ;
#82918=CARTESIAN_POINT ( 'NONE',  ( -0.2493438320209966919, 0.05413385826771626580, -0.4176697321401330321 ) ) ;
#82921=CARTESIAN_POINT ( 'NONE',  ( 1.430446194225722500, 0.05413385826771666132, 0.4176697321401328100 ) ) ;
#82922=CARTESIAN_POINT ( 'NONE',  ( 1.561679790026247350, 0.05413385826771626580, -0.4176697321401330321 ) ) ;
#82923=CARTESIAN_POINT ( 'NONE',  ( 0.01968503937007957949, -0.4536011799217368745, -0.2665933059059886201 ) ) ;
#82924=CARTESIAN_POINT ( 'NONE',  ( 0.7086614173228352742, -0.1870078740157480879, -0.4822834645669291653 ) ) ;
#82926=CARTESIAN_POINT ( 'NONE',  ( 0.1902887139107617975, -0.5511811023622048555, -0.09757992244046775898 ) ) ;
#82927=CARTESIAN_POINT ( 'NONE',  ( 0.2099737532808405305, 0.2306618581243847221, -0.2411417322834647770 ) ) ;
#82929=CARTESIAN_POINT ( 'NONE',  ( -1.338582677165353729, -0.1870078740157480879, -0.4822834645669291653 ) ) ;
#82930=CARTESIAN_POINT ( 'NONE',  ( 0.9711286089238851948, 0.1283753931104748280, 0.1820866141732283561 ) ) ;
#82931=CARTESIAN_POINT ( 'NONE',  ( 0.3280839895013130669, 0.009842519685039463617, 0.3409548833797002576 ) ) ;
#82932=CARTESIAN_POINT ( 'NONE',  ( -0.2952755905511804668, 0.1660481256975885056, 0.3530559997133364547 ) ) ;
#82933=CARTESIAN_POINT ( 'NONE',  ( 0.02624671916010564918, -0.5023911411419708095, -0.1820866141732282451 ) ) ;
#82935=CARTESIAN_POINT ( 'NONE',  ( -0.3280839895013117347, -0.4281496062992124485, 0.4176697321401328655 ) ) ;
#82936=CARTESIAN_POINT ( 'NONE',  ( 0.2034120734908142214, 0.1771653543307087075, -0.09757992244046823083 ) ) ;
#82937=VECTOR ( 'NONE', #16550, 39.37007874015748143 ) ;
#82939=CARTESIAN_POINT ( 'NONE',  ( -0.2034120734908128059, 0.2952755905511811885, 0.1292274648535926551 ) ) ;
#82940=EDGE_CURVE ( 'NONE', #78564, #38952, #11223, .T. ) ;
#82943=CARTESIAN_POINT ( 'NONE',  ( 1.318897637795276356, -0.4536011799217367080, 0.2665933059059888421 ) ) ;
#82944=CARTESIAN_POINT ( 'NONE',  ( 0.4831401376419955929, 2.606013654608237919E-15, 0.4118477457932982477 ) ) ;
#82945=CARTESIAN_POINT ( 'NONE',  ( -0.3412073490813641308, -0.5023911411419708095, 0.1820866141732285504 ) ) ;
#82946=CARTESIAN_POINT ( 'NONE',  ( -0.8661417322834640276, -0.1870078740157480601, -0.3641732283464567677 ) ) ;
#82947=CARTESIAN_POINT ( 'NONE',  ( -0.3543307086614165824, 0.2952755905511811885, 0.000000000000000000 ) ) ;
#82948=CARTESIAN_POINT ( 'NONE',  ( -0.1574803149606292529, -0.1870078740157479769, 0.4822834645669291653 ) ) ;
#82949=CARTESIAN_POINT ( 'NONE',  ( 0.8923884514435703741, 0.1283753931104748280, 0.1820866141732283561 ) ) ;
#82950=CARTESIAN_POINT ( 'NONE',  ( -1.692913385826770645, 0.1771653543307087630, 0.000000000000000000 ) ) ;
#82951=CARTESIAN_POINT ( 'NONE',  ( 1.489501312335958172, -0.08942795157528024563, -0.3641732283464568787 ) ) ;
#82952=CARTESIAN_POINT ( 'NONE',  ( 0.6496062992125991586, -0.5400638737290845981, -0.3530559997133363437 ) ) ;
#82954=CARTESIAN_POINT ( 'NONE',  ( -0.2690288713910754526, 0.2952755905511810774, -0.1292274648535930714 ) ) ;
#82956=CARTESIAN_POINT ( 'NONE',  ( 0.9514435695538062676, -0.3162353388693409650, -0.4822834645669289433 ) ) ;
#82957=CARTESIAN_POINT ( 'NONE',  ( 0.4855643044619430415, -0.4281496062992127816, -0.4176697321401328100 ) ) ;
#82959=CARTESIAN_POINT ( 'NONE',  ( 0.3412073490813655186, -0.5023911411419708095, -0.1820866141732282451 ) ) ;
#82960=CARTESIAN_POINT ( 'NONE',  ( 1.266404199475066328, -0.3162353388693409650, -0.4822834645669289433 ) ) ;
#82961=CARTESIAN_POINT ( 'NONE',  ( -0.4133858267716528645, 0.07958543189024071263, -0.2665933059059888421 ) ) ;
#82962=CARTESIAN_POINT ( 'NONE',  ( -0.5708661417322825615, -0.5400638737290844871, 0.3530559997133364547 ) ) ;
#82964=CARTESIAN_POINT ( 'NONE',  ( 0.4002624671916016896, -0.3162353388693409650, -0.4822834645669289433 ) ) ;
#82965=CARTESIAN_POINT ( 'NONE',  ( -0.8267716535433065062, 0.2952755905511811885, 0.000000000000000000 ) ) ;
#82966=CARTESIAN_POINT ( 'NONE',  ( -0.5971128608923877978, 0.1771653543307087630, 0.09757992244046791164 ) ) ;
#82967=CARTESIAN_POINT ( 'NONE',  ( 0.4790026246719167324, -0.05778040916215522460, 0.4822834645669289988 ) ) ;
#82968=CARTESIAN_POINT ( 'NONE',  ( -1.423884514435694859, -0.3162353388693405765, 0.4822834645669290543 ) ) ;
#82969=CARTESIAN_POINT ( 'NONE',  ( -0.3740157480314953431, 0.1660481256975885056, 0.3530559997133364547 ) ) ;
#82972=CARTESIAN_POINT ( 'NONE',  ( 1.194225721784777594, -0.4281496062992127816, -0.4176697321401328100 ) ) ;
#82973=CARTESIAN_POINT ( 'NONE',  ( 1.266404199475066328, -0.3162353388693409650, -0.4822834645669289433 ) ) ;
#82975=DIRECTION ( 'NONE',  ( 0.000000000000000000, -1.000000000000000000, 0.000000000000000000 ) ) ;
#82976=CARTESIAN_POINT ( 'NONE',  ( -1.062992125984250968, 0.2952755905511811885, 0.000000000000000000 ) ) ;
#82979=VERTEX_POINT ( 'NONE', #25457 ) ;
#82980=CARTESIAN_POINT ( 'NONE',  ( 0.06561679790026316017, -0.3690944881889763329, 0.3153832671262228327 ) ) ;
#82982=CARTESIAN_POINT ( 'NONE',  ( 0.6758530183727039509, 0.2952755905511810774, -0.1292274648535930714 ) ) ;
#82985=CARTESIAN_POINT ( 'NONE',  ( -0.5905511811023613777, -0.5511811023622047445, 6.969142054262312111E-17 ) ) ;
#82987=CARTESIAN_POINT ( 'NONE',  ( 1.213910761154856299, 0.2952755905511811885, 0.1292274648535926551 ) ) ;
#82988=CARTESIAN_POINT ( 'NONE',  ( 1.036745406824147508, -0.3690944881889765550, -0.3153832671262227771 ) ) ;
#82989=CARTESIAN_POINT ( 'NONE',  ( -0.1115485564304453947, -0.6692913385826771977, 0.1292274648535927661 ) ) ;
#82991=CARTESIAN_POINT ( 'NONE',  ( -0.3674540682414689785, 0.2306618581243848609, 0.2411417322834645549 ) ) ;
#82992=CARTESIAN_POINT ( 'NONE',  ( -1.161417322834644716, -0.4536011799217368745, -0.2665933059059886201 ) ) ;
#82993=CARTESIAN_POINT ( 'NONE',  ( -0.3412073490813641308, -0.6046776061558807314, 0.2411417322834647770 ) ) ;
#82995=CARTESIAN_POINT ( 'NONE',  ( -8.318810292902005415E-17, 2.401574803149606474, -0.4915354330708645580 ) ) ;
#82998=CARTESIAN_POINT ( 'NONE',  ( 0.5774278215223104249, 0.2306618581243848609, 0.2411417322834645549 ) ) ;
#83000=CARTESIAN_POINT ( 'NONE',  ( -0.6824146981627291497, -0.6046776061558809534, -0.2411417322834644161 ) ) ;
#83001=CARTESIAN_POINT ( 'NONE',  ( 1.233595800524935227, -0.6046776061558807314, 0.2411417322834647770 ) ) ;
#83002=CARTESIAN_POINT ( 'NONE',  ( 0.4790026246719167324, -0.05778040916215522460, 0.4822834645669289988 ) ) ;
#83003=CARTESIAN_POINT ( 'NONE',  ( -0.1574803149606292529, -0.1870078740157480879, -0.4822834645669291653 ) ) ;
#83005=CARTESIAN_POINT ( 'NONE',  ( -0.8136482939632537770, -0.6046776061558807314, 0.2411417322834647770 ) ) ;
#83006=CARTESIAN_POINT ( 'NONE',  ( -0.006561679790025524116, -0.05778040916215560624, -0.4822834645669293319 ) ) ;
#83007=CARTESIAN_POINT ( 'NONE',  ( -0.9317585301837263412, -0.4281496062992127816, -0.4176697321401328100 ) ) ;
#83008=CARTESIAN_POINT ( 'NONE',  ( -0.04593175853018302557, 0.1771653543307087630, 0.09757992244046791164 ) ) ;
#83010=CARTESIAN_POINT ( 'NONE',  ( -0.1706036745406816491, -0.4281496062992124485, 0.4176697321401328655 ) ) ;
#83012=CARTESIAN_POINT ( 'NONE',  ( 1.049868766404200127, -0.6046776061558809534, -0.2411417322834644161 ) ) ;
#83014=VERTEX_POINT ( 'NONE', #20413 ) ;
#83015=ORIENTED_EDGE ( 'NONE', *, *, #47547, .T. ) ;
#83016=CARTESIAN_POINT ( 'NONE',  ( 0.1181102362204730916, 0.2952755905511811885, 0.000000000000000000 ) ) ;
#83017=CARTESIAN_POINT ( 'NONE',  ( 0.2821522309711292364, -0.5511811023622046335, 0.09757992244046803654 ) ) ;
#83018=CARTESIAN_POINT ( 'NONE',  ( 1.371391076115485941, 0.1771653543307087630, 0.09757992244046791164 ) ) ;
#83023=CARTESIAN_POINT ( 'NONE',  ( 1.594488188976378673, 0.1660481256975885056, 0.3530559997133364547 ) ) ;
#83025=CARTESIAN_POINT ( 'NONE',  ( 0.4461942257217855201, -0.6046776061558807314, 0.2411417322834647770 ) ) ;
#83026=CARTESIAN_POINT ( 'NONE',  ( -1.279527559055116948, 0.1660481256975883668, -0.3530559997133364547 ) ) ;
#83027=CARTESIAN_POINT ( 'NONE',  ( -1.292650918635170010, -0.6692913385826771977, 0.1292274648535927661 ) ) ;
#83028=CARTESIAN_POINT ( 'NONE',  ( 0.3083989501312343062, -0.3162353388693405765, 0.4822834645669290543 ) ) ;
#83030=CARTESIAN_POINT ( 'NONE',  ( 1.686351706036745890, 0.2952755905511811885, 0.1292274648535926551 ) ) ;
#83031=CARTESIAN_POINT ( 'NONE',  ( 0.9383202099737536495, -0.3162353388693405765, 0.4822834645669290543 ) ) ;
#83032=CARTESIAN_POINT ( 'NONE',  ( 1.574803149606299746, -0.1870078740157480601, -0.3641732283464567677 ) ) ;
#83033=CARTESIAN_POINT ( 'NONE',  ( 0.6758530183727039509, -0.5511811023622046335, 0.09757992244046803654 ) ) ;
#83034=CARTESIAN_POINT ( 'NONE',  ( -0.6496062992125976043, 0.1660481256975883668, -0.3530559997133364547 ) ) ;
#83036=CARTESIAN_POINT ( 'NONE',  ( 1.574803149606299746, -0.1870078740157480879, -0.4822834645669291653 ) ) ;
#83039=CARTESIAN_POINT ( 'NONE',  ( 0.7414698162729663755, 0.2952755905511811885, 0.1292274648535926551 ) ) ;
#83041=CARTESIAN_POINT ( 'NONE',  ( -1.476377952755905110, -0.4536011799217368745, -0.2665933059059886201 ) ) ;
#83042=CARTESIAN_POINT ( 'NONE',  ( -0.09186351706036663400, -0.4281496062992124485, 0.4176697321401328655 ) ) ;
#83043=CARTESIAN_POINT ( 'NONE',  ( 0.7020997375328090762, -0.08942795157528024563, -0.3641732283464568787 ) ) ;
#83044=CARTESIAN_POINT ( 'NONE',  ( 0.9120734908136490793, 0.2952755905511810774, -0.1292274648535930714 ) ) ;
#83046=CARTESIAN_POINT ( 'NONE',  ( -0.5380577427821514602, -0.3690944881889765550, -0.3153832671262227771 ) ) ;
#83047=CARTESIAN_POINT ( 'NONE',  ( -0.5118110236220466680, -0.6692913385826771977, 8.415575281601705876E-17 ) ) ;
#83048=CARTESIAN_POINT ( 'NONE',  ( 1.666666666666667185, 0.05413385826771666132, 0.4176697321401328100 ) ) ;
#83049=CARTESIAN_POINT ( 'NONE',  ( -0.9645669291338575535, -0.5400638737290844871, 0.3530559997133364547 ) ) ;
#83050=CARTESIAN_POINT ( 'NONE',  ( 1.069553805774278832, 0.2952755905511810774, -0.1292274648535930714 ) ) ;
#83052=CARTESIAN_POINT ( 'NONE',  ( -1.522309711286088607, -0.5023911411419708095, 0.1820866141732285504 ) ) ;
#83054=CARTESIAN_POINT ( 'NONE',  ( 1.181102362204724976, -0.1870078740157480879, -0.4822834645669291653 ) ) ;
#83057=CARTESIAN_POINT ( 'NONE',  ( -1.574803149606298636, -0.1870078740157479769, 0.4822834645669291653 ) ) ;
#83058=CARTESIAN_POINT ( 'NONE',  ( 1.620734908136483465, -0.6692913385826771977, 0.1292274648535927661 ) ) ;
#83059=CARTESIAN_POINT ( 'NONE',  ( -0.9251968503937002541, 0.07958543189024085140, 0.2665933059059887866 ) ) ;
#83061=CARTESIAN_POINT ( 'NONE',  ( 1.587926509186352586, -0.3690944881889765550, -0.3153832671262227771 ) ) ;
#83062=CARTESIAN_POINT ( 'NONE',  ( -0.4002624671916004129, -0.3162353388693405765, 0.4822834645669290543 ) ) ;
#83063=CARTESIAN_POINT ( 'NONE',  ( -0.3083989501312330295, -0.2845877964562161244, -0.3641732283464567121 ) ) ;
#83064=CARTESIAN_POINT ( 'NONE',  ( -1.640419947506561060, -0.3690944881889765550, -0.3153832671262227771 ) ) ;
#83065=CARTESIAN_POINT ( 'NONE',  ( 1.036745406824147508, -0.3690944881889765550, -0.3153832671262227771 ) ) ;
#83066=CARTESIAN_POINT ( 'NONE',  ( 0.9514435695538062676, -0.3162353388693409650, -0.4822834645669289433 ) ) ;
#83067=CARTESIAN_POINT ( 'NONE',  ( 1.450131233595801428, 0.2952755905511811885, 0.1292274648535926551 ) ) ;
#83068=CARTESIAN_POINT ( 'NONE',  ( 0.1902887139107617975, -0.5511811023622048555, -0.09757992244046775898 ) ) ;
#83069=CARTESIAN_POINT ( 'NONE',  ( 0.5971128608923891301, 0.2952755905511810774, -0.1292274648535930714 ) ) ;
#83071=CARTESIAN_POINT ( 'NONE',  ( 0.7677165354330716118, -0.4536011799217367080, 0.2665933059059888421 ) ) ;
#83072=CARTESIAN_POINT ( 'NONE',  ( 1.568241469816273437, -0.3162353388693405765, 0.4822834645669290543 ) ) ;
#83073=CARTESIAN_POINT ( 'NONE',  ( -1.200787401574802349, -0.5400638737290844871, 0.3530559997133364547 ) ) ;
#83074=CARTESIAN_POINT ( 'NONE',  ( -0.4396325459317579898, 0.2952755905511811885, 0.1292274648535926551 ) ) ;
#83077=CARTESIAN_POINT ( 'NONE',  ( 0.2821522309711292364, -0.6692913385826771977, 0.1292274648535927661 ) ) ;
#83078=CARTESIAN_POINT ( 'NONE',  ( 0.9645669291338588858, 0.07958543189024085140, 0.2665933059059887866 ) ) ;
#83079=CARTESIAN_POINT ( 'NONE',  ( -0.3412073490813641308, 0.2306618581243847221, -0.2411417322834647770 ) ) ;
#83080=CARTESIAN_POINT ( 'NONE',  ( 0.4396325459317590445, -0.6692913385826771977, 0.1292274648535927661 ) ) ;
#83086=CARTESIAN_POINT ( 'NONE',  ( -0.8005249343832013809, -0.3690944881889763329, 0.3153832671262228327 ) ) ;
#83087=CARTESIAN_POINT ( 'NONE',  ( -1.332020997375327642, -0.3162353388693409650, -0.4822834645669289433 ) ) ;
#83090=CARTESIAN_POINT ( 'NONE',  ( 0.8267716535433078384, -0.6692913385826771977, 8.415575281601705876E-17 ) ) ;
#83091=CARTESIAN_POINT ( 'NONE',  ( 1.371391076115485719, -0.6692913385826773087, -0.1292274648535924053 ) ) ;
#83092=CARTESIAN_POINT ( 'NONE',  ( 0.7611548556430451917, -0.6046776061558807314, 0.2411417322834647770 ) ) ;
#83095=CARTESIAN_POINT ( 'NONE',  ( 1.548556430446194954, 0.2306618581243847221, -0.2411417322834647770 ) ) ;
#83096=CARTESIAN_POINT ( 'NONE',  ( 0.5971128608923890191, -0.6692913385826771977, 0.1292274648535927661 ) ) ;
#83097=CARTESIAN_POINT ( 'NONE',  ( 0.6824146981627303710, 0.2306618581243847221, -0.2411417322834647770 ) ) ;
#83099=CARTESIAN_POINT ( 'NONE',  ( 0.8333333333333340365, 0.1771653543307087075, -0.09757992244046823083 ) ) ;
#83100=CARTESIAN_POINT ( 'NONE',  ( 1.240157480314961314, 0.1660481256975883668, -0.3530559997133364547 ) ) ;
#83103=CARTESIAN_POINT ( 'NONE',  ( 0.3215223097112867578, -0.05778040916215522460, 0.4822834645669289988 ) ) ;
#83104=CARTESIAN_POINT ( 'NONE',  ( 1.095800524934383846, -0.05778040916215560624, -0.4822834645669293319 ) ) ;
#83105=CARTESIAN_POINT ( 'NONE',  ( 0.2296587926509192634, -0.3162353388693405765, 0.4822834645669290543 ) ) ;
#83106=CARTESIAN_POINT ( 'NONE',  ( 1.102362204724410155, -0.1870078740157480601, -0.3641732283464567677 ) ) ;
#83107=CARTESIAN_POINT ( 'NONE',  ( -0.9580052493438311334, -0.4281496062992124485, 0.4176697321401328655 ) ) ;
#83108=CARTESIAN_POINT ( 'NONE',  ( -1.043307086614172707, 0.1660481256975883668, -0.3530559997133364547 ) ) ;
#83109=CARTESIAN_POINT ( 'NONE',  ( 1.200787401574803681, -0.5400638737290845981, -0.3530559997133363437 ) ) ;
#83113=EDGE_CURVE ( 'NONE', #41264, #78537, #22302, .T. ) ;
#83117=CARTESIAN_POINT ( 'NONE',  ( 1.502624671916010790, -0.05778040916215522460, 0.4822834645669289988 ) ) ;
#83118=CARTESIAN_POINT ( 'NONE',  ( 1.272965879265092637, -0.004921259842519576551, 0.3153832671262227771 ) ) ;
#83120=CARTESIAN_POINT ( 'NONE',  ( 1.443569553805774897, -0.5023911411419708095, -0.1820866141732282451 ) ) ;
#83124=CARTESIAN_POINT ( 'NONE',  ( -0.6824146981627288167, 0.1283753931104748280, 0.1820866141732283561 ) ) ;
#83125=CARTESIAN_POINT ( 'NONE',  ( -1.522309711286088607, 0.1283753931104746893, -0.1820866141732285504 ) ) ;
#83126=CARTESIAN_POINT ( 'NONE',  ( -1.443569553805773564, 0.2306618581243847221, -0.2411417322834647770 ) ) ;
#83127=CARTESIAN_POINT ( 'NONE',  ( 0.2034120734908142214, 0.2952755905511810774, -0.1292274648535930714 ) ) ;
#83128=CARTESIAN_POINT ( 'NONE',  ( 1.325459317585302665, 0.05413385826771626580, -0.4176697321401330321 ) ) ;
#83134=CARTESIAN_POINT ( 'NONE',  ( -0.6692913385826764205, 0.1771653543307087630, 0.000000000000000000 ) ) ;
#83135=CARTESIAN_POINT ( 'NONE',  ( -1.167979002624671470, 0.05413385826771666132, 0.4176697321401328100 ) ) ;
#83136=CARTESIAN_POINT ( 'NONE',  ( 0.9055118110236227702, 0.2952755905511811885, 0.000000000000000000 ) ) ;
#83140=CARTESIAN_POINT ( 'NONE',  ( 1.345144356955381593, -0.05778040916215522460, 0.4822834645669289988 ) ) ;
#83141=CARTESIAN_POINT ( 'NONE',  ( -1.437007874015747477, -0.5400638737290844871, 0.3530559997133364547 ) ) ;
#83144=CARTESIAN_POINT ( 'NONE',  ( -0.3477690288713905509, -0.5511811023622046335, 0.09757992244046803654 ) ) ;
#83146=CARTESIAN_POINT ( 'NONE',  ( -0.7086614173228339419, -0.1870078740157479769, 0.3641732283464567677 ) ) ;
#83147=CARTESIAN_POINT ( 'NONE',  ( 0.03280839895013198948, 0.1771653543307087630, 0.09757992244046791164 ) ) ;
#83148=CARTESIAN_POINT ( 'NONE',  ( -0.04593175853018302557, -0.6692913385826773087, -0.1292274648535924053 ) ) ;
#83149=CARTESIAN_POINT ( 'NONE',  ( -0.6955380577427815458, -0.004921259842519576551, 0.3153832671262227771 ) ) ;
#83151=CARTESIAN_POINT ( 'NONE',  ( 1.233595800524935227, -0.6046776061558807314, 0.2411417322834647770 ) ) ;
#83152=CARTESIAN_POINT ( 'NONE',  ( -1.266404199475064773, -0.05778040916215560624, -0.4822834645669293319 ) ) ;
#83154=CARTESIAN_POINT ( 'NONE',  ( -0.2821522309711278487, 0.2952755905511811885, 0.1292274648535926551 ) ) ;
#83155=ADVANCED_FACE ( 'NONE', ( #65868 ), #73443, .F. ) ;
#83156=CARTESIAN_POINT ( 'NONE',  ( -0.8989501312335946848, -0.6692913385826771977, 0.1292274648535927661 ) ) ;
#83157=CARTESIAN_POINT ( 'NONE',  ( 1.076115485564305141, 0.1283753931104746893, -0.1820866141732285504 ) ) ;
#83158=CARTESIAN_POINT ( 'NONE',  ( -0.2427821522309703550, -0.08942795157528024563, -0.3641732283464568787 ) ) ;
#83159=CARTESIAN_POINT ( 'NONE',  ( -0.5183727034120726440, -0.6692913385826773087, -0.1292274648535924053 ) ) ;
#83160=CARTESIAN_POINT ( 'NONE',  ( -0.9711286089238838626, 0.2306618581243847221, -0.2411417322834647770 ) ) ;
#83162=CARTESIAN_POINT ( 'NONE',  ( 1.227034120734908917, 0.1771653543307087075, -0.09757992244046823083 ) ) ;
#83163=CARTESIAN_POINT ( 'NONE',  ( -0.1377952755905504645, -0.5400638737290845981, -0.3530559997133363437 ) ) ;
#83164=CARTESIAN_POINT ( 'NONE',  ( -1.364829396325458521, 0.2306618581243847221, -0.2411417322834647770 ) ) ;
#83167=CARTESIAN_POINT ( 'NONE',  ( -0.9842519685039360366, 0.1771653543307087630, 0.000000000000000000 ) ) ;
#83168=CARTESIAN_POINT ( 'NONE',  ( 0.7414698162729663755, -0.6692913385826773087, -0.1292274648535924053 ) ) ;
#83169=CARTESIAN_POINT ( 'NONE',  ( -0.8727034120734901146, -0.08942795157528024563, -0.3641732283464568787 ) ) ;
#83171=CARTESIAN_POINT ( 'NONE',  ( -0.9186351706036736120, 0.2306618581243848609, 0.2411417322834645549 ) ) ;
#83172=CARTESIAN_POINT ( 'NONE',  ( 0.9186351706036752773, 0.2306618581243847221, -0.2411417322834647770 ) ) ;
#83173=CARTESIAN_POINT ( 'NONE',  ( 0.6102362204724416372, 0.1660481256975883668, -0.3530559997133364547 ) ) ;
#83174=CARTESIAN_POINT ( 'NONE',  ( 1.607611548556431069, 0.2952755905511811885, 0.1292274648535926551 ) ) ;
#83175=CARTESIAN_POINT ( 'NONE',  ( -1.476377952755905110, -0.4536011799217368745, -0.2665933059059886201 ) ) ;
#83180=CARTESIAN_POINT ( 'NONE',  ( 1.312335958005250269, -0.5023911411419708095, 0.1820866141732285504 ) ) ;
#83181=CARTESIAN_POINT ( 'NONE',  ( 0.7283464566929140904, -0.4536011799217368745, -0.2665933059059886201 ) ) ;
#83182=CARTESIAN_POINT ( 'NONE',  ( -0.06561679790026180015, -0.4281496062992127816, -0.4176697321401328100 ) ) ;
#83184=CARTESIAN_POINT ( 'NONE',  ( 0.4002624671916016896, -0.08942795157527998196, 0.3641732283464567121 ) ) ;
#83185=CARTESIAN_POINT ( 'NONE',  ( -0.8727034120734901146, -0.3162353388693405765, 0.4822834645669290543 ) ) ;
#83186=CARTESIAN_POINT ( 'NONE',  ( -1.089238845144356427, -0.4281496062992127816, -0.4176697321401328100 ) ) ;
#83187=CARTESIAN_POINT ( 'NONE',  ( 0.7283464566929143125, 0.1660481256975885056, 0.3530559997133364547 ) ) ;
#83190=( BOUNDED_CURVE ( )  B_SPLINE_CURVE ( 1, ( #35249, #60913 ),
 .UNSPECIFIED., .F., .F. ) 
 B_SPLINE_CURVE_WITH_KNOTS ( ( 2, 2 ),
 ( 8.673617379884035472E-19, 0.002000000000000002644 ),
 .UNSPECIFIED. ) 
 CURVE ( )  GEOMETRIC_REPRESENTATION_ITEM ( )  RATIONAL_B_SPLINE_CURVE ( ( 0.9875488213027530104, 0.9875488213027530104 ) ) 
 REPRESENTATION_ITEM ( '' )  );
#83192=ORIENTED_EDGE ( 'NONE', *, *, #64478, .F. ) ;
#83193=CARTESIAN_POINT ( 'NONE',  ( -1.364829396325458521, 0.2306618581243847221, -0.2411417322834647770 ) ) ;
#83194=CARTESIAN_POINT ( 'NONE',  ( -0.7152230971128602510, -0.3162353388693405765, 0.4822834645669290543 ) ) ;
#83195=CARTESIAN_POINT ( 'NONE',  ( -0.8661417322834640276, -0.1870078740157479769, 0.3641732283464567677 ) ) ;
#83196=CARTESIAN_POINT ( 'NONE',  ( -0.7283464566929126471, -0.5400638737290844871, 0.3530559997133364547 ) ) ;
#83198=DIRECTION ( 'NONE',  ( 0.000000000000000000, 1.000000000000000000, 0.000000000000000000 ) ) ;
#83199=CARTESIAN_POINT ( 'NONE',  ( 1.463254593175853824, -0.6692913385826771977, 0.1292274648535927661 ) ) ;
#83200=CARTESIAN_POINT ( 'NONE',  ( 1.377952755905512472, -0.6692913385826771977, 8.415575281601705876E-17 ) ) ;
#83201=CARTESIAN_POINT ( 'NONE',  ( -0.6889763779527552368, -0.5400638737290845981, -0.3530559997133363437 ) ) ;
#83202=CARTESIAN_POINT ( 'NONE',  ( 0.4461942257217855201, -0.6046776061558807314, 0.2411417322834647770 ) ) ;
#83203=CARTESIAN_POINT ( 'NONE',  ( -0.8005249343832011588, 0.05413385826771626580, -0.4176697321401330321 ) ) ;
#83205=CARTESIAN_POINT ( 'NONE',  ( -0.6167979002624665030, -0.3690944881889765550, -0.3153832671262227771 ) ) ;
#83206=ORIENTED_EDGE ( 'NONE', *, *, #68645, .F. ) ;
#83208=EDGE_LOOP ( 'NONE', ( #81243, #52242, #43726, #43550 ) ) ;
#83210=CARTESIAN_POINT ( 'NONE',  ( -1.128608923884513837, 0.2306618581243847221, -0.2411417322834647770 ) ) ;
#83211=CARTESIAN_POINT ( 'NONE',  ( -1.010498687664041384, 0.05413385826771666132, 0.4176697321401328100 ) ) ;
#83213=CARTESIAN_POINT ( 'NONE',  ( -1.102362204724408601, -0.1870078740157479769, 0.4822834645669291653 ) ) ;
#83214=CARTESIAN_POINT ( 'NONE',  ( -1.069553805774277722, 0.2952755905511811885, 0.1292274648535926551 ) ) ;
#83216=CARTESIAN_POINT ( 'NONE',  ( -1.646981627296586703, -0.05778040916215522460, 0.4822834645669289988 ) ) ;
#83218=CARTESIAN_POINT ( 'NONE',  ( 0.3608923884514443348, -0.5511811023622046335, 0.09757992244046803654 ) ) ;
#83219=CARTESIAN_POINT ( 'NONE',  ( -0.4848604877838266214, -2.609869883881465018E-15, -0.3464511005275220379 ) ) ;
#83221=CARTESIAN_POINT ( 'NONE',  ( -0.2887139107611542133, 0.1283753931104748280, 0.1820866141732283561 ) ) ;
#83222=CARTESIAN_POINT ( 'NONE',  ( -0.8595800524934373854, -0.05778040916215522460, 0.4822834645669289988 ) ) ;
#83223=CARTESIAN_POINT ( 'NONE',  ( 1.404199475065617264, -0.4281496062992124485, 0.4176697321401328655 ) ) ;
#83224=CARTESIAN_POINT ( 'NONE',  ( -0.4658792650918627265, -0.3162353388693409650, -0.4822834645669289433 ) ) ;
#83228=CARTESIAN_POINT ( 'NONE',  ( -0.7349081364829387342, -0.6046776061558807314, 0.2411417322834647770 ) ) ;
#83229=CARTESIAN_POINT ( 'NONE',  ( 1.450131233595801428, 0.2952755905511811885, 0.1292274648535926551 ) ) ;
#83230=CARTESIAN_POINT ( 'NONE',  ( -1.272965879265091305, -0.3690944881889763329, 0.3153832671262228327 ) ) ;
#83231=CARTESIAN_POINT ( 'NONE',  ( -1.528871391076114250, 0.2952755905511810774, -0.1292274648535930714 ) ) ;
#83236=CARTESIAN_POINT ( 'NONE',  ( 0.1115485564304470323, 0.2952755905511811885, 0.1292274648535926551 ) ) ;
#83237=CARTESIAN_POINT ( 'NONE',  ( -1.220472440944881054, -0.5511811023622047445, 6.969142054262312111E-17 ) ) ;
#83238=CARTESIAN_POINT ( 'NONE',  ( -0.9120734908136475250, 0.2952755905511811885, 0.1292274648535926551 ) ) ;
#83240=CARTESIAN_POINT ( 'NONE',  ( -0.9448818897637790704, -0.1870078740157479769, 0.4822834645669291653 ) ) ;
#83241=CARTESIAN_POINT ( 'NONE',  ( -0.8333333333333323711, -0.6692913385826773087, -0.1292274648535924053 ) ) ;
#83242=CARTESIAN_POINT ( 'NONE',  ( 0.1968503937007881344, 0.2952755905511811885, 0.000000000000000000 ) ) ;
#83244=CARTESIAN_POINT ( 'NONE',  ( 0.8005249343832027131, -0.004921259842519576551, 0.3153832671262227771 ) ) ;
#83245=CARTESIAN_POINT ( 'NONE',  ( -0.7939632545931754048, -0.2845877964562159024, 0.3641732283464567677 ) ) ;
#83246=CARTESIAN_POINT ( 'NONE',  ( 0.8136482939632553313, -0.5023911411419708095, -0.1820866141732282451 ) ) ;
#83247=CARTESIAN_POINT ( 'NONE',  ( -1.706036745406823485, 0.2306618581243848609, 0.2411417322834645549 ) ) ;
#83248=CARTESIAN_POINT ( 'NONE',  ( 1.509186351706037543, -0.4281496062992127816, -0.4176697321401328100 ) ) ;
#83249=CARTESIAN_POINT ( 'NONE',  ( 0.3805774278215230400, -0.3690944881889763329, 0.3153832671262228327 ) ) ;
#83251=CARTESIAN_POINT ( 'NONE',  ( -0.9251968503937002541, -0.5400638737290845981, -0.3530559997133363437 ) ) ;
#83252=CARTESIAN_POINT ( 'NONE',  ( 1.095800524934383846, -0.3162353388693405765, 0.4822834645669290543 ) ) ;
#83254=CARTESIAN_POINT ( 'NONE',  ( -0.1640419947506553400, -0.08942795157528024563, -0.3641732283464568787 ) ) ;
#83255=DIRECTION ( 'NONE',  ( -1.000000000000000000, -3.096699300667737957E-16, 1.692413147294446216E-16 ) ) ;
#83257=CARTESIAN_POINT ( 'NONE',  ( 0.3083989501312343062, -0.05778040916215560624, -0.4822834645669293319 ) ) ;
#83259=CARTESIAN_POINT ( 'NONE',  ( 1.128608923884514947, 0.1283753931104748280, 0.1820866141732283561 ) ) ;
#83260=CARTESIAN_POINT ( 'NONE',  ( 0.2099737532808405305, 0.1283753931104746893, -0.1820866141732285504 ) ) ;
#83261=CARTESIAN_POINT ( 'NONE',  ( -0.09186351706036663400, -0.4281496062992124485, 0.4176697321401328655 ) ) ;
#83262=CARTESIAN_POINT ( 'NONE',  ( -1.246719160104986512, 0.05413385826771666132, 0.4176697321401328100 ) ) ;
#83263=CARTESIAN_POINT ( 'NONE',  ( -0.8792650918635160906, -0.3690944881889763329, 0.3153832671262228327 ) ) ;
#83264=DIRECTION ( 'NONE',  ( 0.000000000000000000, 0.000000000000000000, -1.000000000000000000 ) ) ;
#83265=CARTESIAN_POINT ( 'NONE',  ( -0.4658792650918627265, -0.3162353388693409650, -0.4822834645669289433 ) ) ;
#83268=CARTESIAN_POINT ( 'NONE',  ( 0.3149606299212603933, -0.1870078740157479769, 0.3641732283464567677 ) ) ;
#83269=CARTESIAN_POINT ( 'NONE',  ( -0.2493438320209966919, -0.4281496062992124485, 0.4176697321401328655 ) ) ;
#83270=CARTESIAN_POINT ( 'NONE',  ( -1.076115485564303809, -0.6046776061558809534, -0.2411417322834644161 ) ) ;
#83271=CARTESIAN_POINT ( 'NONE',  ( -1.253280839895012377, -0.2845877964562161244, -0.3641732283464567121 ) ) ;
#83273=CARTESIAN_POINT ( 'NONE',  ( -0.4658792650918627265, -0.3162353388693409650, -0.4822834645669289433 ) ) ;
#83274=CARTESIAN_POINT ( 'NONE',  ( -0.7874015748031489847, -0.1870078740157480601, -0.3641732283464567677 ) ) ;
#83275=CARTESIAN_POINT ( 'NONE',  ( -1.397637795275589623, 0.07958543189024085140, 0.2665933059059887866 ) ) ;
#83276=CARTESIAN_POINT ( 'NONE',  ( 1.174540682414699111, -0.05778040916215560624, -0.4822834645669293319 ) ) ;
#83277=CARTESIAN_POINT ( 'NONE',  ( 0.01000891935578606708, -2.191421614605370878E-15, 0.4445507791589071167 ) ) ;
#83279=ORIENTED_EDGE ( 'NONE', *, *, #26454, .T. ) ;
#83280=CARTESIAN_POINT ( 'NONE',  ( -0.2247243262887786697, -4.992347309556208597E-15, 0.3791483426435189319 ) ) ;
#83281=CARTESIAN_POINT ( 'NONE',  ( -1.515748031496062076, 0.1660481256975883668, -0.3530559997133364547 ) ) ;
#83282=CARTESIAN_POINT ( 'NONE',  ( -0.8792650918635160906, 0.05413385826771626580, -0.4176697321401330321 ) ) ;
#83283=CARTESIAN_POINT ( 'NONE',  ( -1.640419947506561060, 0.05413385826771666132, 0.4176697321401328100 ) ) ;
#83286=CARTESIAN_POINT ( 'NONE',  ( 0.9908136482939640111, -0.6692913385826771977, 0.1292274648535927661 ) ) ;
#83287=CARTESIAN_POINT ( 'NONE',  ( 0.2099737532808405305, -0.6046776061558807314, 0.2411417322834647770 ) ) ;
#83290=CARTESIAN_POINT ( 'NONE',  ( 1.056430446194226436, -0.5511811023622048555, -0.09757992244046775898 ) ) ;
#83296=CARTESIAN_POINT ( 'NONE',  ( -0.1837270341207343505, -0.6046776061558807314, 0.2411417322834647770 ) ) ;
#83297=CARTESIAN_POINT ( 'NONE',  ( -0.9251968503937002541, 0.1660481256975885056, 0.3530559997133364547 ) ) ;
#83298=CARTESIAN_POINT ( 'NONE',  ( -1.351706036745406347, -0.4281496062992124485, 0.4176697321401328655 ) ) ;
#83299=CARTESIAN_POINT ( 'NONE',  ( 0.6364829396325465405, -0.3162353388693409650, -0.4822834645669289433 ) ) ;
#83300=CARTESIAN_POINT ( 'NONE',  ( 1.646981627296588035, -0.3162353388693405765, 0.4822834645669290543 ) ) ;
#83301=CARTESIAN_POINT ( 'NONE',  ( 1.325459317585302665, 0.05413385826771626580, -0.4176697321401330321 ) ) ;
#83302=CARTESIAN_POINT ( 'NONE',  ( -0.4330708661417315697, -0.6692913385826771977, 8.415575281601705876E-17 ) ) ;
#83303=CARTESIAN_POINT ( 'NONE',  ( 0.5774278215223103139, -0.6046776061558809534, -0.2411417322834644161 ) ) ;
#83304=CARTESIAN_POINT ( 'NONE',  ( -1.535433070866141225, -0.6692913385826771977, 8.415575281601705876E-17 ) ) ;
#83305=CARTESIAN_POINT ( 'NONE',  ( 1.332020997375328974, -0.05778040916215560624, -0.4822834645669293319 ) ) ;
#83306=CARTESIAN_POINT ( 'NONE',  ( 1.587926509186352586, -0.4281496062992127816, -0.4176697321401328100 ) ) ;
#83307=CARTESIAN_POINT ( 'NONE',  ( -0.1115485564304456306, 0.2952755905511810774, -0.1292274648535930714 ) ) ;
ENDSEC;
END-ISO-10303-21;
